#63272=CARTESIAN_POINT ( 'NONE',  ( 21.53943276465977519, 0.05219959533937863772, 71.25109039468568994 ) ) ;
#63273=CARTESIAN_POINT ( 'NONE',  ( -16.52544592524335698, -4.483927247898792601, 38.95942372801901854 ) ) ;
#63274=CARTESIAN_POINT ( 'NONE',  ( 16.53943276465976808, -0.05219959533910856209, 73.74890960531433848 ) ) ;
#63275=CARTESIAN_POINT ( 'NONE',  ( -15.80617190586768217, 15.72974639402176855, 88.12609039468570415 ) ) ;
#63276=CARTESIAN_POINT ( 'NONE',  ( 8.224510206698742110, 14.34966873604972548, 112.0844237280190185 ) ) ;
#63278=CARTESIAN_POINT ( 'NONE',  ( -4.379528057220086978, -16.55341960407618274, 39.79275706135235424 ) ) ;
#63279=CARTESIAN_POINT ( 'NONE',  ( 16.52544592524342804, -4.483927247898539470, 43.54057627198103830 ) ) ;
#63280=CARTESIAN_POINT ( 'NONE',  ( -4.379528057220086978, -16.55341960407618274, 89.79275706135236135 ) ) ;
#63281=CARTESIAN_POINT ( 'NONE',  ( -5.153800228976328057, -19.02544592524343514, 97.29057627198099567 ) ) ;
#63282=CARTESIAN_POINT ( 'NONE',  ( 19.03943276465977164, -0.05219959533909143690, 113.7489096053143669 ) ) ;
#63283=CARTESIAN_POINT ( 'NONE',  ( 21.55341960407619695, -5.719274019375665929, 101.0427570613523756 ) ) ;
#63284=CARTESIAN_POINT ( 'NONE',  ( 14.29746914071037800, 8.314922557961029526, 106.6677570613523756 ) ) ;
#63285=CARTESIAN_POINT ( 'NONE',  ( -12.06949235617756955, 12.14591786802309770, 75.62390960531439532 ) ) ;
#63286=CARTESIAN_POINT ( 'NONE',  ( -19.02544592524342804, 5.153800228976336051, 81.04057627198103830 ) ) ;
#63288=CARTESIAN_POINT ( 'NONE',  ( -14.34966873604972548, 8.224510206698743886, 23.33442372801901499 ) ) ;
#63289=CARTESIAN_POINT ( 'NONE',  ( 16.46253265017160672, -9.564922557960803928, 33.33224293864770260 ) ) ;
#63290=CARTESIAN_POINT ( 'NONE',  ( 9.474510206698971260, -16.51473224551069308, 87.91557627198102409 ) ) ;
#63291=CARTESIAN_POINT ( 'NONE',  ( 4.483927247898790824, -16.52544592524335698, 35.20942372801901854 ) ) ;
#63293=CARTESIAN_POINT ( 'NONE',  ( 5.049401038297881783, 19.05341960407617563, 37.29275706135232582 ) ) ;
#63294=CARTESIAN_POINT ( 'NONE',  ( -14.34966873604972548, 8.224510206698743886, 98.33442372801901854 ) ) ;
#63295=CARTESIAN_POINT ( 'NONE',  ( -19.02544592524334988, -5.153800228976617603, 108.9594237280189759 ) ) ;
#63296=CARTESIAN_POINT ( 'NONE',  ( -5.153800228976328057, -19.02544592524343514, 32.29057627198102409 ) ) ;
#63297=CARTESIAN_POINT ( 'NONE',  ( -8.224510206698735004, -14.34966873604973081, 79.58442372801903275 ) ) ;
#63298=CARTESIAN_POINT ( 'NONE',  ( 16.53943276465976808, 0.05219959533934440121, 66.25109039468567573 ) ) ;
#63299=CARTESIAN_POINT ( 'NONE',  ( -16.51473224551069308, -9.474510206698971260, 36.66557627198102409 ) ) ;
#63300=CARTESIAN_POINT ( 'NONE',  ( 5.049401038297881783, 19.05341960407617563, 72.29275706135234714 ) ) ;
#63301=CARTESIAN_POINT ( 'NONE',  ( -10.81492255796105439, 18.62759615963255655, 107.9177570613523471 ) ) ;
#63302=CARTESIAN_POINT ( 'NONE',  ( 16.46253265017160672, -9.564922557960803928, 53.33224293864768839 ) ) ;
#63304=CARTESIAN_POINT ( 'NONE',  ( -5.049401038298153566, 19.05341960407611168, 95.20724293864770971 ) ) ;
#63305=CARTESIAN_POINT ( 'NONE',  ( 4.379528057220339221, -16.55341960407611168, 87.70724293864769550 ) ) ;
#63307=CARTESIAN_POINT ( 'NONE',  ( -16.51473224551082808, 9.474510206698731452, 53.33442372801900433 ) ) ;
#63308=CARTESIAN_POINT ( 'NONE',  ( 21.55341960407610458, 5.719274019375980345, 53.95724293864770260 ) ) ;
#63309=CARTESIAN_POINT ( 'NONE',  ( -19.03943276465977164, -0.05219959533935918106, 28.75109039468566507 ) ) ;
#63310=CARTESIAN_POINT ( 'NONE',  ( -5.049401038298153566, 19.05341960407611168, 85.20724293864766707 ) ) ;
#63311=CARTESIAN_POINT ( 'NONE',  ( 5.153800228976615827, -19.02544592524334988, 20.20942372801899722 ) ) ;
#63312=CARTESIAN_POINT ( 'NONE',  ( 18.67979575497178502, 10.72451020669898547, 64.16557627198102409 ) ) ;
#63313=CARTESIAN_POINT ( 'NONE',  ( -5.153800228976328057, -19.02544592524343514, 107.2905762719810383 ) ) ;
#63314=CARTESIAN_POINT ( 'NONE',  ( -16.51473224551082808, 9.474510206698731452, 83.33442372801899012 ) ) ;
#63315=CARTESIAN_POINT ( 'NONE',  ( 0.05219959533909260263, 19.03943276465977164, 114.9989096053143669 ) ) ;
#63316=CARTESIAN_POINT ( 'NONE',  ( 9.474510206698729675, 16.51473224551082808, 112.0844237280190043 ) ) ;
#63317=CARTESIAN_POINT ( 'NONE',  ( 9.474510206698971260, -16.51473224551069308, 27.91557627198103120 ) ) ;
#63318=CARTESIAN_POINT ( 'NONE',  ( 16.51473224551069308, 9.474510206698969483, 99.16557627198102409 ) ) ;
#63319=CARTESIAN_POINT ( 'NONE',  ( 18.67979575497178502, 10.72451020669898547, 79.16557627198103830 ) ) ;
#63321=CARTESIAN_POINT ( 'NONE',  ( 16.53943276465976808, 0.05219959533934440121, 46.25109039468567573 ) ) ;
#63322=CARTESIAN_POINT ( 'NONE',  ( 18.67979575497194134, -10.72451020669871369, 40.83442372801901854 ) ) ;
#63323=CARTESIAN_POINT ( 'NONE',  ( 19.02544592524334988, 5.153800228976608722, 86.45942372801900433 ) ) ;
#63324=CARTESIAN_POINT ( 'NONE',  ( -0.05219959533937732626, 21.53943276465977519, 92.50109039468567573 ) ) ;
#63325=CARTESIAN_POINT ( 'NONE',  ( 16.52544592524335698, 4.483927247898782831, 91.45942372801901854 ) ) ;
#63326=CARTESIAN_POINT ( 'NONE',  ( 5.049401038298161559, -19.05341960407611168, 102.7072429386476955 ) ) ;
#63327=CARTESIAN_POINT ( 'NONE',  ( 8.314922557960818139, 14.29746914071049879, 84.58224293864769550 ) ) ;
#63328=CARTESIAN_POINT ( 'NONE',  ( -0.05219959533910754901, -16.53943276465976808, 37.49890960531436690 ) ) ;
#63329=CARTESIAN_POINT ( 'NONE',  ( 16.46253265017146816, 9.564922557961045513, 66.66775706135233293 ) ) ;
#63330=CARTESIAN_POINT ( 'NONE',  ( -21.52544592524334988, -5.823673210054445271, 53.95942372801900433 ) ) ;
#63331=CARTESIAN_POINT ( 'NONE',  ( 16.46253265017146816, 9.564922557961045513, 21.66775706135233648 ) ) ;
#63332=CARTESIAN_POINT ( 'NONE',  ( -12.14591786802309592, -12.06949235617757132, 91.87390960531436690 ) ) ;
#63333=CARTESIAN_POINT ( 'NONE',  ( 10.81492255796078972, 18.62759615963270932, 34.58224293864770260 ) ) ;
#63334=CARTESIAN_POINT ( 'NONE',  ( 16.52544592524335698, 4.483927247898782831, 111.4594237280190328 ) ) ;
#63336=CARTESIAN_POINT ( 'NONE',  ( -10.72451020669870658, -18.67979575497194134, 94.58442372801901854 ) ) ;
#63337=CARTESIAN_POINT ( 'NONE',  ( -8.314922557961024197, 14.29746914071037800, 62.91775706135236135 ) ) ;
#63338=CARTESIAN_POINT ( 'NONE',  ( 14.34966873604972726, -8.224510206698740333, 110.8344237280190043 ) ) ;
#63339=CARTESIAN_POINT ( 'NONE',  ( 5.719274019375673035, 21.55341960407619339, 52.29275706135236135 ) ) ;
#63340=CARTESIAN_POINT ( 'NONE',  ( -5.719274019375665041, -21.55341960407619695, 54.79275706135235424 ) ) ;
#63341=VERTEX_POINT ( 'NONE', #147524 ) ;
#63342=CARTESIAN_POINT ( 'NONE',  ( 15.80617190586769283, -15.72974639402175789, 30.62609039468567929 ) ) ;
#63343=CARTESIAN_POINT ( 'NONE',  ( 14.34966873604960469, 8.224510206698951720, 109.1655762719810383 ) ) ;
#63344=CARTESIAN_POINT ( 'NONE',  ( -16.46253265017160317, 9.564922557960807481, 30.83224293864769550 ) ) ;
#63345=CARTESIAN_POINT ( 'NONE',  ( 8.224510206698953496, -14.34966873604960469, 67.91557627198102409 ) ) ;
#63346=CARTESIAN_POINT ( 'NONE',  ( -16.46253265017160317, 9.564922557960807481, 65.83224293864769550 ) ) ;
#63347=CARTESIAN_POINT ( 'NONE',  ( 4.483927247898790824, -16.52544592524335698, 110.2094237280190185 ) ) ;
#63348=CARTESIAN_POINT ( 'NONE',  ( 21.53943276465977519, -0.05219959533907433946, 53.74890960531437401 ) ) ;
#63349=CARTESIAN_POINT ( 'NONE',  ( -4.379528057220328563, 16.55341960407611168, 95.20724293864769550 ) ) ;
#63350=CARTESIAN_POINT ( 'NONE',  ( 21.53943276465977519, -0.05219959533907433946, 98.74890960531438111 ) ) ;
#63351=CARTESIAN_POINT ( 'NONE',  ( -19.02544592524342804, 5.153800228976336051, 106.0405762719810241 ) ) ;
#63352=CARTESIAN_POINT ( 'NONE',  ( 5.049401038298161559, -19.05341960407611168, 47.70724293864770260 ) ) ;
#63353=CARTESIAN_POINT ( 'NONE',  ( -16.46253265017146816, -9.564922557961047289, 109.1677570613523471 ) ) ;
#63354=CARTESIAN_POINT ( 'NONE',  ( -15.72974639402197994, 15.80617190586746368, 50.62390960531435979 ) ) ;
#63355=CARTESIAN_POINT ( 'NONE',  ( -5.719274019375665041, -21.55341960407619695, 69.79275706135234714 ) ) ;
#63356=CARTESIAN_POINT ( 'NONE',  ( -5.049401038298153566, 19.05341960407611168, 70.20724293864769550 ) ) ;
#63357=CARTESIAN_POINT ( 'NONE',  ( 13.89961937509977652, -13.97604488694527269, 98.12390960531433848 ) ) ;
#63358=CARTESIAN_POINT ( 'NONE',  ( 14.34966873604972726, -8.224510206698740333, 65.83442372801900433 ) ) ;
#63359=CARTESIAN_POINT ( 'NONE',  ( 5.719274019375673035, 21.55341960407619339, 47.29275706135234003 ) ) ;
#63360=CARTESIAN_POINT ( 'NONE',  ( 21.53943276465977519, 0.05219959533937863772, 81.25109039468568994 ) ) ;
#63361=CARTESIAN_POINT ( 'NONE',  ( 10.72451020669898902, -18.67979575497178502, 92.91557627198103830 ) ) ;
#63362=CARTESIAN_POINT ( 'NONE',  ( -21.53943276465977519, -0.05219959533937600094, 38.75109039468567573 ) ) ;
#63363=CARTESIAN_POINT ( 'NONE',  ( -8.224510206698735004, -14.34966873604973081, 84.58442372801903275 ) ) ;
#63364=CARTESIAN_POINT ( 'NONE',  ( 0.05219959533907565091, 21.53943276465977519, 74.99890960531435269 ) ) ;
#63365=CARTESIAN_POINT ( 'NONE',  ( 19.02544592524334988, 5.153800228976608722, 31.45942372801900433 ) ) ;
#63366=CARTESIAN_POINT ( 'NONE',  ( -5.153800228976328057, -19.02544592524343514, 82.29057627198103830 ) ) ;
#63367=CARTESIAN_POINT ( 'NONE',  ( 16.55341960407611168, 4.379528057220329451, 23.95724293864769550 ) ) ;
#63368=CARTESIAN_POINT ( 'NONE',  ( -17.49999999999999645, -3.189878218039172264, 105.1294856257125758 ) ) ;
#63369=CARTESIAN_POINT ( 'NONE',  ( 9.474510206698971260, -16.51473224551069308, 97.91557627198102409 ) ) ;
#63371=CARTESIAN_POINT ( 'NONE',  ( 5.153800228976615827, -19.02544592524334988, 75.20942372801896170 ) ) ;
#63372=CARTESIAN_POINT ( 'NONE',  ( 15.72974639402199770, -15.80617190586745480, 58.12390960531435979 ) ) ;
#63373=CARTESIAN_POINT ( 'NONE',  ( -12.14591786802309592, -12.06949235617757132, 36.87390960531435979 ) ) ;
#63374=CARTESIAN_POINT ( 'NONE',  ( -9.474510206698720793, -16.51473224551083518, 109.5844237280190043 ) ) ;
#63375=CARTESIAN_POINT ( 'NONE',  ( 16.51473224551069308, 9.474510206698969483, 34.16557627198102409 ) ) ;
#63376=CARTESIAN_POINT ( 'NONE',  ( -16.53943276465976808, -0.05219959533934237506, 18.75109039468568639 ) ) ;
#63377=CARTESIAN_POINT ( 'NONE',  ( -18.67979575497178146, -10.72451020669898902, 96.66557627198102409 ) ) ;
#63378=CARTESIAN_POINT ( 'NONE',  ( -5.153800228976607833, 19.02544592524334988, 67.70942372801900433 ) ) ;
#63379=CARTESIAN_POINT ( 'NONE',  ( -8.314922557961024197, 14.29746914071037800, 82.91775706135234714 ) ) ;
#63380=CARTESIAN_POINT ( 'NONE',  ( 13.89961937509977652, -13.97604488694527269, 63.12390960531435979 ) ) ;
#63381=CARTESIAN_POINT ( 'NONE',  ( 0.05219959533910956823, 16.53943276465976808, 74.99890960531435269 ) ) ;
#63382=CARTESIAN_POINT ( 'NONE',  ( -9.564922557960796823, -16.46253265017161027, 62.08224293864769550 ) ) ;
#63383=CARTESIAN_POINT ( 'NONE',  ( 16.52544592524342804, -4.483927247898539470, 73.54057627198102409 ) ) ;
#63384=CARTESIAN_POINT ( 'NONE',  ( 9.564922557960805705, 16.46253265017160317, 24.58224293864769194 ) ) ;
#63386=CARTESIAN_POINT ( 'NONE',  ( -16.52544592524342804, 4.483927247898546575, 36.04057627198102409 ) ) ;
#63387=CARTESIAN_POINT ( 'NONE',  ( 19.05341960407611168, 5.049401038298154454, 78.95724293864769550 ) ) ;
#63388=DIRECTION ( 'NONE',  ( 0.000000000000000000, 0.000000000000000000, -1.000000000000000000 ) ) ;
#63389=CARTESIAN_POINT ( 'NONE',  ( 5.153800228976615827, -19.02544592524334988, 35.20942372801899722 ) ) ;
#63390=CARTESIAN_POINT ( 'NONE',  ( 12.14591786802327356, -12.06949235617739191, 55.62609039468568284 ) ) ;
#63391=CARTESIAN_POINT ( 'NONE',  ( -15.80617190586745835, -15.72974639402198527, 66.87390960531436690 ) ) ;
#63392=CARTESIAN_POINT ( 'NONE',  ( 10.72451020669871369, 18.67979575497193778, 112.0844237280190185 ) ) ;
#63393=CARTESIAN_POINT ( 'NONE',  ( -16.51473224551069308, -9.474510206698971260, 71.66557627198102409 ) ) ;
#63395=CARTESIAN_POINT ( 'NONE',  ( -21.55341960407610458, -5.719274019375992779, 21.45724293864769550 ) ) ;
#63396=CARTESIAN_POINT ( 'NONE',  ( 5.049401038298161559, -19.05341960407611168, 62.70724293864769550 ) ) ;
#63397=CARTESIAN_POINT ( 'NONE',  ( 18.67979575497194134, -10.72451020669871369, 35.83442372801901143 ) ) ;
#63398=CARTESIAN_POINT ( 'NONE',  ( 16.52544592524342804, -4.483927247898539470, 103.5405762719810383 ) ) ;
#63399=CARTESIAN_POINT ( 'NONE',  ( -21.52544592524343514, 5.823673210054127303, 106.0405762719810525 ) ) ;
#63400=CARTESIAN_POINT ( 'NONE',  ( -13.89961937509977652, 13.97604488694528158, 95.62390960531436690 ) ) ;
#63402=CARTESIAN_POINT ( 'NONE',  ( -18.67979575497193778, 10.72451020669871902, 28.33442372801902209 ) ) ;
#63404=CARTESIAN_POINT ( 'NONE',  ( 9.474510206698971260, -16.51473224551069308, 82.91557627198103830 ) ) ;
#63406=B_SPLINE_CURVE_WITH_KNOTS ( 'NONE', 3,
 ( #85740, #113077, #6891, #100897, #81725, #22079 ),
 .UNSPECIFIED., .F., .F.,
 ( 4, 2, 4 ),
 ( 3.469446951953613804E-18, 0.0003837532665554152424, 0.0007675065331108270154 ),
 .UNSPECIFIED. ) ;
#63408=CARTESIAN_POINT ( 'NONE',  ( -5.823673210054116645, -21.52544592524344225, 97.29057627198105251 ) ) ;
#63409=CARTESIAN_POINT ( 'NONE',  ( 5.153800228976335163, 19.02544592524342804, 44.79057627198103830 ) ) ;
#63410=CARTESIAN_POINT ( 'NONE',  ( 13.89961937509957401, 13.97604488694547697, 101.8760903946856331 ) ) ;
#63412=CARTESIAN_POINT ( 'NONE',  ( 16.46253265017160672, -9.564922557960803928, 23.33224293864769194 ) ) ;
#63413=CARTESIAN_POINT ( 'NONE',  ( -5.719274019375665041, -21.55341960407619695, 79.79275706135236135 ) ) ;
#63414=CARTESIAN_POINT ( 'NONE',  ( -19.02544592524342804, 5.153800228976336051, 81.04057627198103830 ) ) ;
#63415=CARTESIAN_POINT ( 'NONE',  ( 5.719274019375673035, 21.55341960407619339, 52.29275706135236135 ) ) ;
#63416=CARTESIAN_POINT ( 'NONE',  ( 21.55341960407619695, -5.719274019375665929, 31.04275706135234714 ) ) ;
#63418=CARTESIAN_POINT ( 'NONE',  ( 0.05219959533909260263, 19.03943276465977164, 89.99890960531436690 ) ) ;
#63419=CARTESIAN_POINT ( 'NONE',  ( 18.56399227203345248, 5.499999999999818812, 61.47830131249903474 ) ) ;
#63420=CARTESIAN_POINT ( 'NONE',  ( -12.14591786802326823, 12.06949235617739902, 38.12609039468567573 ) ) ;
#63421=CARTESIAN_POINT ( 'NONE',  ( 15.80617190586746368, 15.72974639402197994, 49.37390960531436690 ) ) ;
#63422=CARTESIAN_POINT ( 'NONE',  ( -15.72974639402176322, -15.80617190586768395, 39.37609039468567573 ) ) ;
#63423=CARTESIAN_POINT ( 'NONE',  ( -15.80617190586768217, 15.72974639402176855, 73.12609039468567573 ) ) ;
#63425=CARTESIAN_POINT ( 'NONE',  ( -19.05341960407617563, 5.049401038297882671, 108.5427570613523187 ) ) ;
#63426=CARTESIAN_POINT ( 'NONE',  ( -13.89961937509977652, 13.97604488694528158, 55.62390960531434558 ) ) ;
#63427=CARTESIAN_POINT ( 'NONE',  ( -16.46253265017160317, 9.564922557960807481, 80.83224293864769550 ) ) ;
#63428=CARTESIAN_POINT ( 'NONE',  ( 16.52544592524342804, -4.483927247898539470, 108.5405762719810241 ) ) ;
#63429=CARTESIAN_POINT ( 'NONE',  ( 4.379528057220339221, -16.55341960407611168, 107.7072429386476955 ) ) ;
#63430=CARTESIAN_POINT ( 'NONE',  ( -13.97604488694527625, -13.89961937509977652, 111.8739096053143243 ) ) ;
#63431=CARTESIAN_POINT ( 'NONE',  ( -12.06949235617739369, -12.14591786802326823, 84.37609039468570415 ) ) ;
#63432=CARTESIAN_POINT ( 'NONE',  ( -16.55341960407611168, -4.379528057220339221, 76.45724293864769550 ) ) ;
#63433=CARTESIAN_POINT ( 'NONE',  ( -5.049401038298153566, 19.05341960407611168, 60.20724293864768129 ) ) ;
#63434=CARTESIAN_POINT ( 'NONE',  ( -0.05219959533937732626, 21.53943276465977519, 82.50109039468568994 ) ) ;
#63435=CARTESIAN_POINT ( 'NONE',  ( 21.53943276465977519, 0.05219959533937863772, 66.25109039468567573 ) ) ;
#63436=CARTESIAN_POINT ( 'NONE',  ( 13.89961937509957401, 13.97604488694547697, 111.8760903946856757 ) ) ;
#63437=CARTESIAN_POINT ( 'NONE',  ( -14.34966873604960291, -8.224510206698953496, 61.66557627198103120 ) ) ;
#63438=CARTESIAN_POINT ( 'NONE',  ( 10.81492255796106328, -18.62759615963255655, 25.41775706135235779 ) ) ;
#63439=CARTESIAN_POINT ( 'NONE',  ( 0.05219959533907565091, 21.53943276465977519, 64.99890960531435269 ) ) ;
#63440=CARTESIAN_POINT ( 'NONE',  ( -17.49999999999999645, -5.500000000000000888, 104.2030961746582847 ) ) ;
#63442=CARTESIAN_POINT ( 'NONE',  ( 0.05219959533909260263, 19.03943276465977164, 69.99890960531435269 ) ) ;
#63443=CARTESIAN_POINT ( 'NONE',  ( 0.05219959533910956823, 16.53943276465976808, 39.99890960531436690 ) ) ;
#63445=CARTESIAN_POINT ( 'NONE',  ( -12.06949235617756955, 12.14591786802309770, 25.62390960531435624 ) ) ;
#63446=CARTESIAN_POINT ( 'NONE',  ( -8.314922557961024197, 14.29746914071037800, 92.91775706135236135 ) ) ;
#63447=CARTESIAN_POINT ( 'NONE',  ( 19.05341960407617918, -5.049401038297876454, 56.04275706135234714 ) ) ;
#63448=CARTESIAN_POINT ( 'NONE',  ( 17.12812012977023812, 6.668231424566063659, 48.85948759323144941 ) ) ;
#63449=CARTESIAN_POINT ( 'NONE',  ( -19.02544592524342804, 5.153800228976336051, 106.0405762719810241 ) ) ;
#63450=CARTESIAN_POINT ( 'NONE',  ( 0.05219959533910956823, 16.53943276465976808, 79.99890960531435269 ) ) ;
#63451=CARTESIAN_POINT ( 'NONE',  ( -16.46253265017146816, -9.564922557961047289, 44.16775706135232582 ) ) ;
#63452=CARTESIAN_POINT ( 'NONE',  ( 17.50000000000000000, -5.500000000000000888, 103.2969038253417153 ) ) ;
#63453=CARTESIAN_POINT ( 'NONE',  ( 19.05341960407611168, 5.049401038298154454, 113.9572429386477097 ) ) ;
#63454=CARTESIAN_POINT ( 'NONE',  ( 0.05219959533907565091, 21.53943276465977519, 59.99890960531436690 ) ) ;
#63455=VERTEX_POINT ( 'NONE', #133338 ) ;
#63456=CARTESIAN_POINT ( 'NONE',  ( -0.05219959533910754901, -16.53943276465976808, 102.4989096053143811 ) ) ;
#63457=CARTESIAN_POINT ( 'NONE',  ( 16.52544592524335698, 4.483927247898782831, 56.45942372801902565 ) ) ;
#63458=CARTESIAN_POINT ( 'NONE',  ( 14.29746914071049879, -8.314922557960816363, 93.33224293864769550 ) ) ;
#63460=CARTESIAN_POINT ( 'NONE',  ( -16.18388926212241685, 7.379444403734378710, 49.56046848633847191 ) ) ;
#63461=CARTESIAN_POINT ( 'NONE',  ( 19.03943276465977164, -0.05219959533909143690, 113.7489096053143669 ) ) ;
#63464=ORIENTED_EDGE ( 'NONE', *, *, #192158, .F. ) ;
#63465=CARTESIAN_POINT ( 'NONE',  ( 8.224510206698742110, 14.34966873604972548, 42.08442372801901854 ) ) ;
#63466=CARTESIAN_POINT ( 'NONE',  ( -12.06949235617756955, 12.14591786802309770, 35.62390960531437401 ) ) ;
#63467=CARTESIAN_POINT ( 'NONE',  ( -10.72451020669898014, 18.67979575497178502, 60.41557627198102409 ) ) ;
#63468=CARTESIAN_POINT ( 'NONE',  ( -9.474510206698720793, -16.51473224551083518, 89.58442372801900433 ) ) ;
#63469=CARTESIAN_POINT ( 'NONE',  ( 0.05219959533907565091, 21.53943276465977519, 49.99890960531437401 ) ) ;
#63470=CARTESIAN_POINT ( 'NONE',  ( -10.81492255796105439, 18.62759615963255655, 82.91775706135234714 ) ) ;
#63472=CARTESIAN_POINT ( 'NONE',  ( -0.05219959533934338120, 16.53943276465976808, 32.50109039468568284 ) ) ;
#63473=CARTESIAN_POINT ( 'NONE',  ( -0.05219959533909027116, -19.03943276465977164, 37.49890960531436690 ) ) ;
#63474=CARTESIAN_POINT ( 'NONE',  ( -13.89961937509977652, 13.97604488694528158, 105.6239096053143527 ) ) ;
#63475=CARTESIAN_POINT ( 'NONE',  ( 16.46253265017160672, -9.564922557960803928, 38.33224293864768839 ) ) ;
#63476=CARTESIAN_POINT ( 'NONE',  ( 12.14591786802309770, 12.06949235617756955, 104.3739096053143669 ) ) ;
#63477=CARTESIAN_POINT ( 'NONE',  ( -9.474510206698964154, 16.51473224551069663, 100.4155762719810241 ) ) ;
#63479=CARTESIAN_POINT ( 'NONE',  ( 16.55341960407618274, -4.379528057220086978, 51.04275706135234714 ) ) ;
#63480=CARTESIAN_POINT ( 'NONE',  ( 21.52544592524344225, -5.823673210054117533, 88.54057627198103830 ) ) ;
#63481=CARTESIAN_POINT ( 'NONE',  ( 0.05219959533909260263, 19.03943276465977164, 59.99890960531436690 ) ) ;
#63482=CARTESIAN_POINT ( 'NONE',  ( 18.62759615963255655, 10.81492255796105972, 21.66775706135235069 ) ) ;
#63483=CARTESIAN_POINT ( 'NONE',  ( -13.97604488694527625, -13.89961937509977652, 81.87390960531436690 ) ) ;
#63486=CARTESIAN_POINT ( 'NONE',  ( -12.06949235617739369, -12.14591786802326823, 44.37609039468567573 ) ) ;
#63487=CARTESIAN_POINT ( 'NONE',  ( -5.719274019375665041, -21.55341960407619695, 24.79275706135235779 ) ) ;
#63488=CARTESIAN_POINT ( 'NONE',  ( 9.474510206698971260, -16.51473224551069308, 22.91557627198102765 ) ) ;
#63489=CARTESIAN_POINT ( 'NONE',  ( -5.153800228976328057, -19.02544592524343514, 102.2905762719810383 ) ) ;
#63490=CARTESIAN_POINT ( 'NONE',  ( -9.564922557961040184, 16.46253265017147172, 77.91775706135234714 ) ) ;
#63492=CARTESIAN_POINT ( 'NONE',  ( -16.51473224551082808, 9.474510206698731452, 33.33442372801899722 ) ) ;
#63493=CARTESIAN_POINT ( 'NONE',  ( -15.72974639402197994, 15.80617190586746368, 85.62390960531436690 ) ) ;
#63494=CARTESIAN_POINT ( 'NONE',  ( 19.02544592524334988, 5.153800228976608722, 41.45942372801900433 ) ) ;
#63495=CARTESIAN_POINT ( 'NONE',  ( -4.483927247898782831, 16.52544592524335698, 72.70942372801901854 ) ) ;
#63496=CARTESIAN_POINT ( 'NONE',  ( -5.153800228976328057, -19.02544592524343514, 112.2905762719810099 ) ) ;
#63497=VERTEX_POINT ( 'NONE', #40334 ) ;
#63498=CARTESIAN_POINT ( 'NONE',  ( -13.89961937509977652, 13.97604488694528158, 60.62390960531436690 ) ) ;
#63500=CARTESIAN_POINT ( 'NONE',  ( -10.81492255796105439, 18.62759615963255655, 67.91775706135234714 ) ) ;
#63501=CARTESIAN_POINT ( 'NONE',  ( 15.80617190586769283, -15.72974639402175789, 85.62609039468568994 ) ) ;
#63502=CARTESIAN_POINT ( 'NONE',  ( -19.02544592524342804, 5.153800228976336051, 71.04057627198099567 ) ) ;
#63503=CARTESIAN_POINT ( 'NONE',  ( 18.62759615963255655, 10.81492255796105972, 46.66775706135234714 ) ) ;
#63504=CARTESIAN_POINT ( 'NONE',  ( 16.51473224551083163, -9.474510206698727899, 85.83442372801900433 ) ) ;
#63506=CARTESIAN_POINT ( 'NONE',  ( 5.153800228976335163, 19.02544592524342804, 54.79057627198103120 ) ) ;
#63507=CARTESIAN_POINT ( 'NONE',  ( 16.46253265017160672, -9.564922557960803928, 103.3322429386476955 ) ) ;
#63508=CARTESIAN_POINT ( 'NONE',  ( -19.03943276465977164, 0.05219959533909376836, 61.24890960531436690 ) ) ;
#63509=CARTESIAN_POINT ( 'NONE',  ( -5.153800228976328057, -19.02544592524343514, 112.2905762719810099 ) ) ;
#63510=CARTESIAN_POINT ( 'NONE',  ( -9.474510206698964154, 16.51473224551069663, 45.41557627198103120 ) ) ;
#63511=CARTESIAN_POINT ( 'NONE',  ( -15.80617190586745835, -15.72974639402198527, 101.8739096053143811 ) ) ;
#63512=CARTESIAN_POINT ( 'NONE',  ( -0.05219959533934338120, 16.53943276465976808, 77.50109039468567573 ) ) ;
#63514=CARTESIAN_POINT ( 'NONE',  ( 19.05341960407617918, -5.049401038297876454, 36.04275706135234003 ) ) ;
#63515=CARTESIAN_POINT ( 'NONE',  ( -9.474510206698964154, 16.51473224551069663, 70.41557627198102409 ) ) ;
#63516=CARTESIAN_POINT ( 'NONE',  ( -12.14591786802309592, -12.06949235617757132, 61.87390960531436690 ) ) ;
#63517=CARTESIAN_POINT ( 'NONE',  ( 14.34966873604960469, 8.224510206698951720, 99.16557627198100988 ) ) ;
#63518=CARTESIAN_POINT ( 'NONE',  ( 5.153800228976335163, 19.02544592524342804, 94.79057627198103830 ) ) ;
#63519=CARTESIAN_POINT ( 'NONE',  ( 16.46253265017160672, -9.564922557960803928, 88.33224293864769550 ) ) ;
#63520=CARTESIAN_POINT ( 'NONE',  ( -16.51473224551069308, -9.474510206698971260, 101.6655762719810241 ) ) ;
#63521=CARTESIAN_POINT ( 'NONE',  ( -5.049401038297874678, -19.05341960407617918, 19.79275706135233293 ) ) ;
#63522=CARTESIAN_POINT ( 'NONE',  ( 8.314922557961029526, -14.29746914071037800, 95.41775706135234714 ) ) ;
#63523=CARTESIAN_POINT ( 'NONE',  ( 5.719274019375673035, 21.55341960407619339, 37.29275706135235424 ) ) ;
#63524=CARTESIAN_POINT ( 'NONE',  ( -10.72451020669898014, 18.67979575497178502, 30.41557627198101699 ) ) ;
#63525=CARTESIAN_POINT ( 'NONE',  ( -18.67979575497178146, -10.72451020669898902, 106.6655762719810383 ) ) ;
#63526=CARTESIAN_POINT ( 'NONE',  ( -4.379528057220328563, 16.55341960407611168, 60.20724293864768839 ) ) ;
#63527=CARTESIAN_POINT ( 'NONE',  ( 5.153800228976335163, 19.02544592524342804, 49.79057627198100988 ) ) ;
#63528=CARTESIAN_POINT ( 'NONE',  ( 4.483927247898545687, 16.52544592524342804, 84.79057627198102409 ) ) ;
#63529=CARTESIAN_POINT ( 'NONE',  ( 15.80617190586746368, 15.72974639402197994, 39.37390960531436690 ) ) ;
#63530=CARTESIAN_POINT ( 'NONE',  ( -19.03943276465977164, -0.05219959533935918106, 38.75109039468566152 ) ) ;
#63531=CARTESIAN_POINT ( 'NONE',  ( -8.224510206698948167, 14.34966873604960824, 115.4155762719810241 ) ) ;
#63533=CARTESIAN_POINT ( 'NONE',  ( 4.483927247898790824, -16.52544592524335698, 65.20942372801901854 ) ) ;
#63534=CARTESIAN_POINT ( 'NONE',  ( 0.05219959533909260263, 19.03943276465977164, 64.99890960531436690 ) ) ;
#63536=CARTESIAN_POINT ( 'NONE',  ( -16.53943276465976808, 0.05219959533911058130, 86.24890960531436690 ) ) ;
#63537=CARTESIAN_POINT ( 'NONE',  ( -5.719274019375978568, 21.55341960407610458, 35.20724293864768839 ) ) ;
#63539=CARTESIAN_POINT ( 'NONE',  ( 8.314922557961029526, -14.29746914071037800, 105.4177570613523613 ) ) ;
#63540=CARTESIAN_POINT ( 'NONE',  ( -16.53943276465976808, -0.05219959533934237506, 23.75109039468567929 ) ) ;
#63541=CARTESIAN_POINT ( 'NONE',  ( -15.80617190586768217, 15.72974639402176855, 98.12609039468570415 ) ) ;
#63542=CARTESIAN_POINT ( 'NONE',  ( 19.05341960407611168, 5.049401038298154454, 83.95724293864766707 ) ) ;
#63543=CARTESIAN_POINT ( 'NONE',  ( 21.55341960407610458, 5.719274019375980345, 113.9572429386477239 ) ) ;
#63544=CARTESIAN_POINT ( 'NONE',  ( 5.153800228976335163, 19.02544592524342804, 29.79057627198102409 ) ) ;
#63545=CARTESIAN_POINT ( 'NONE',  ( 16.53943276465976808, 0.05219959533934440121, 36.25109039468567573 ) ) ;
#63546=CARTESIAN_POINT ( 'NONE',  ( -16.46253265017146816, -9.564922557961047289, 89.16775706135234714 ) ) ;
#63547=CARTESIAN_POINT ( 'NONE',  ( -15.80617190586745835, -15.72974639402198527, 91.87390960531436690 ) ) ;
#63548=CARTESIAN_POINT ( 'NONE',  ( 9.564922557961047289, -16.46253265017146816, 65.41775706135233293 ) ) ;
#63550=CARTESIAN_POINT ( 'NONE',  ( 18.67979575497178502, 10.72451020669898547, 114.1655762719810383 ) ) ;
#63551=CARTESIAN_POINT ( 'NONE',  ( 0.000000000000000000, 0.000000000000000000, 120.0000000000000142 ) ) ;
#63552=CARTESIAN_POINT ( 'NONE',  ( 5.049401038298161559, -19.05341960407611168, 77.70724293864765286 ) ) ;
#63553=CARTESIAN_POINT ( 'NONE',  ( 12.06949235617739724, 12.14591786802326823, 31.87609039468567929 ) ) ;
#63555=CARTESIAN_POINT ( 'NONE',  ( -9.564922557961040184, 16.46253265017147172, 57.91775706135233293 ) ) ;
#63556=CARTESIAN_POINT ( 'NONE',  ( -18.62759615963255300, -10.81492255796106328, 19.16775706135234714 ) ) ;
#63557=CARTESIAN_POINT ( 'NONE',  ( 16.55341960407611168, 4.379528057220329451, 78.95724293864769550 ) ) ;
#63558=CARTESIAN_POINT ( 'NONE',  ( 19.03943276465977164, -0.05219959533909143690, 78.74890960531436690 ) ) ;
#63559=CARTESIAN_POINT ( 'NONE',  ( 8.314922557961029526, -14.29746914071037800, 40.41775706135234714 ) ) ;
#63560=CARTESIAN_POINT ( 'NONE',  ( 0.05219959533936267826, -19.03943276465977164, 40.00109039468566152 ) ) ;
#63561=CARTESIAN_POINT ( 'NONE',  ( 15.72974639402176855, 15.80617190586768217, 66.87609039468568994 ) ) ;
#63562=CARTESIAN_POINT ( 'NONE',  ( -13.89961937509957401, -13.97604488694547875, 104.3760903946856757 ) ) ;
#63563=CARTESIAN_POINT ( 'NONE',  ( 0.05219959533909260263, 19.03943276465977164, 54.99890960531435979 ) ) ;
#63564=CARTESIAN_POINT ( 'NONE',  ( -16.51473224551082808, 9.474510206698731452, 83.33442372801899012 ) ) ;
#63565=CARTESIAN_POINT ( 'NONE',  ( 12.14591786802327356, -12.06949235617739191, 55.62609039468568284 ) ) ;
#63566=CARTESIAN_POINT ( 'NONE',  ( 5.823673210054444382, -21.52544592524334988, 100.2094237280190043 ) ) ;
#63567=CARTESIAN_POINT ( 'NONE',  ( -13.97604488694547697, 13.89961937509957934, 73.12609039468568994 ) ) ;
#63568=CARTESIAN_POINT ( 'NONE',  ( 19.05341960407611168, 5.049401038298154454, 53.95724293864770260 ) ) ;
#63569=CARTESIAN_POINT ( 'NONE',  ( -21.55341960407610458, -5.719274019375992779, 66.45724293864768129 ) ) ;
#63570=CARTESIAN_POINT ( 'NONE',  ( -4.379528057220328563, 16.55341960407611168, 60.20724293864768839 ) ) ;
#63571=CARTESIAN_POINT ( 'NONE',  ( -16.51473224551082808, 9.474510206698731452, 63.33442372801900433 ) ) ;
#63572=CARTESIAN_POINT ( 'NONE',  ( -17.26172910966780094, -6.454744622555795175, 24.19353091350776452 ) ) ;
#63573=CARTESIAN_POINT ( 'NONE',  ( -13.89961937509957401, -13.97604488694547875, 49.37609039468567573 ) ) ;
#63574=CARTESIAN_POINT ( 'NONE',  ( -14.34966873604972548, 8.224510206698743886, 98.33442372801901854 ) ) ;
#63575=CARTESIAN_POINT ( 'NONE',  ( 8.224510206698953496, -14.34966873604960469, 62.91557627198102409 ) ) ;
#63576=CARTESIAN_POINT ( 'NONE',  ( -5.719274019375665041, -21.55341960407619695, 94.79275706135234714 ) ) ;
#63578=CARTESIAN_POINT ( 'NONE',  ( 10.81492255796078972, 18.62759615963270932, 89.58224293864768129 ) ) ;
#63579=CARTESIAN_POINT ( 'NONE',  ( -19.05341960407611168, -5.049401038298163336, 56.45724293864768129 ) ) ;
#63580=CARTESIAN_POINT ( 'NONE',  ( -21.55341960407619339, 5.719274019375674811, 73.54275706135234714 ) ) ;
#63581=CARTESIAN_POINT ( 'NONE',  ( -9.564922557960796823, -16.46253265017161027, 52.08224293864768839 ) ) ;
#63583=CARTESIAN_POINT ( 'NONE',  ( 5.049401038298161559, -19.05341960407611168, 62.70724293864769550 ) ) ;
#63584=CARTESIAN_POINT ( 'NONE',  ( 19.03943276465977164, -0.05219959533909143690, 23.74890960531435269 ) ) ;
#63585=CARTESIAN_POINT ( 'NONE',  ( -19.03943276465977164, 0.05219959533909376836, 116.2489096053143669 ) ) ;
#63586=CARTESIAN_POINT ( 'NONE',  ( -4.483927247898539470, -16.52544592524342804, 57.29057627198103120 ) ) ;
#63587=CARTESIAN_POINT ( 'NONE',  ( -5.049401038298153566, 19.05341960407611168, 25.20724293864768484 ) ) ;
#63588=CARTESIAN_POINT ( 'NONE',  ( 4.483927247898545687, 16.52544592524342804, 89.79057627198103830 ) ) ;
#63589=CARTESIAN_POINT ( 'NONE',  ( -5.823673210054116645, -21.52544592524344225, 102.2905762719810383 ) ) ;
#63590=CARTESIAN_POINT ( 'NONE',  ( 21.55341960407619695, -5.719274019375665929, 31.04275706135234714 ) ) ;
#63592=CARTESIAN_POINT ( 'NONE',  ( -8.224510206698735004, -14.34966873604973081, 44.58442372801901854 ) ) ;
#63593=CARTESIAN_POINT ( 'NONE',  ( 21.52544592524344225, -5.823673210054117533, 78.54057627198103830 ) ) ;
#63594=CARTESIAN_POINT ( 'NONE',  ( -21.55341960407619339, 5.719274019375674811, 103.5427570613523613 ) ) ;
#63595=CARTESIAN_POINT ( 'NONE',  ( 9.564922557960805705, 16.46253265017160317, 109.5822429386476955 ) ) ;
#63596=CARTESIAN_POINT ( 'NONE',  ( -5.719274019375665041, -21.55341960407619695, 49.79275706135234714 ) ) ;
#63597=CARTESIAN_POINT ( 'NONE',  ( 10.81492255796078972, 18.62759615963270932, 39.58224293864769550 ) ) ;
#63598=CARTESIAN_POINT ( 'NONE',  ( -8.224510206698735004, -14.34966873604973081, 99.58442372801900433 ) ) ;
#63599=CARTESIAN_POINT ( 'NONE',  ( 21.52544592524334988, 5.823673210054432836, 61.45942372801901854 ) ) ;
#63600=CARTESIAN_POINT ( 'NONE',  ( -10.81492255796105439, 18.62759615963255655, 97.91775706135236135 ) ) ;
#63601=CARTESIAN_POINT ( 'NONE',  ( 9.474510206698729675, 16.51473224551082808, 37.08442372801899722 ) ) ;
#63602=CARTESIAN_POINT ( 'NONE',  ( -8.224510206698735004, -14.34966873604973081, 84.58442372801903275 ) ) ;
#63603=CARTESIAN_POINT ( 'NONE',  ( -0.05219959533937732626, 21.53943276465977519, 47.50109039468568994 ) ) ;
#63604=CARTESIAN_POINT ( 'NONE',  ( 19.05341960407611168, 5.049401038298154454, 48.95724293864768129 ) ) ;
#63605=CARTESIAN_POINT ( 'NONE',  ( -5.049401038297874678, -19.05341960407617918, 19.79275706135233293 ) ) ;
#63606=CARTESIAN_POINT ( 'NONE',  ( 18.62759615963271287, -10.81492255796078972, 23.33224293864769194 ) ) ;
#63607=CARTESIAN_POINT ( 'NONE',  ( -21.53943276465977519, 0.05219959533907696930, 111.2489096053143669 ) ) ;
#63608=CARTESIAN_POINT ( 'NONE',  ( 21.55341960407610458, 5.719274019375980345, 78.95724293864769550 ) ) ;
#63609=CARTESIAN_POINT ( 'NONE',  ( 14.34966873604972726, -8.224510206698740333, 35.83442372801901143 ) ) ;
#63610=CARTESIAN_POINT ( 'NONE',  ( -18.22780087662121673, -5.500000000000063061, 61.48459894673894155 ) ) ;
#63611=CARTESIAN_POINT ( 'NONE',  ( -5.823673210054116645, -21.52544592524344225, 82.29057627198103830 ) ) ;
#63612=CARTESIAN_POINT ( 'NONE',  ( 4.483927247898790824, -16.52544592524335698, 70.20942372801904696 ) ) ;
#63613=CARTESIAN_POINT ( 'NONE',  ( 4.379528057220339221, -16.55341960407611168, 62.70724293864769550 ) ) ;
#63615=CARTESIAN_POINT ( 'NONE',  ( 5.049401038297881783, 19.05341960407617563, 97.29275706135233293 ) ) ;
#63618=CARTESIAN_POINT ( 'NONE',  ( -12.06949235617739369, -12.14591786802326823, 39.37609039468567573 ) ) ;
#63619=CARTESIAN_POINT ( 'NONE',  ( 21.55341960407610458, 5.719274019375980345, 113.9572429386477239 ) ) ;
#63620=CARTESIAN_POINT ( 'NONE',  ( 10.81492255796078972, 18.62759615963270932, 74.58224293864768129 ) ) ;
#63621=CARTESIAN_POINT ( 'NONE',  ( 19.02544592524343514, -5.153800228976328945, 113.5405762719810241 ) ) ;
#63622=CARTESIAN_POINT ( 'NONE',  ( -0.05219959533934338120, 16.53943276465976808, 57.50109039468568994 ) ) ;
#63623=CARTESIAN_POINT ( 'NONE',  ( 13.89961937509977652, -13.97604488694527269, 68.12390960531436690 ) ) ;
#63624=CARTESIAN_POINT ( 'NONE',  ( 5.719274019375673035, 21.55341960407619339, 42.29275706135235424 ) ) ;
#63625=CARTESIAN_POINT ( 'NONE',  ( -13.97604488694547697, 13.89961937509957934, 108.1260903946856331 ) ) ;
#63626=CARTESIAN_POINT ( 'NONE',  ( 0.05219959533909260263, 19.03943276465977164, 114.9989096053143669 ) ) ;
#63627=CARTESIAN_POINT ( 'NONE',  ( 19.05341960407617918, -5.049401038297876454, 31.04275706135232227 ) ) ;
#63628=CARTESIAN_POINT ( 'NONE',  ( -14.29746914071037622, -8.314922557961029526, 44.16775706135234714 ) ) ;
#63629=CARTESIAN_POINT ( 'NONE',  ( 9.474510206698971260, -16.51473224551069308, 97.91557627198102409 ) ) ;
#63630=CARTESIAN_POINT ( 'NONE',  ( 5.823673210054125526, 21.52544592524343514, 109.7905762719810383 ) ) ;
#63631=CARTESIAN_POINT ( 'NONE',  ( -9.564922557960796823, -16.46253265017161027, 57.08224293864769550 ) ) ;
#63632=CARTESIAN_POINT ( 'NONE',  ( -16.62475595723696031, 7.163666690055234376, 25.52713351810466591 ) ) ;
#63633=CARTESIAN_POINT ( 'NONE',  ( 0.05219959533910956823, 16.53943276465976808, 84.99890960531436690 ) ) ;
#63634=CARTESIAN_POINT ( 'NONE',  ( -19.02544592524342804, 5.153800228976336051, 111.0405762719810099 ) ) ;
#63635=CARTESIAN_POINT ( 'NONE',  ( -17.44270441346513678, 5.991230190323086013, 33.63664920735774189 ) ) ;
#63636=CARTESIAN_POINT ( 'NONE',  ( 10.72451020669898902, -18.67979575497178502, 97.91557627198103830 ) ) ;
#63637=CARTESIAN_POINT ( 'NONE',  ( -0.05219959533936034679, 19.03943276465977164, 62.50109039468566863 ) ) ;
#63638=CARTESIAN_POINT ( 'NONE',  ( -5.719274019375978568, 21.55341960407610458, 30.20724293864769550 ) ) ;
#63639=CARTESIAN_POINT ( 'NONE',  ( -13.97604488694527625, -13.89961937509977652, 21.87390960531435979 ) ) ;
#63640=CARTESIAN_POINT ( 'NONE',  ( 21.53943276465977519, -0.05219959533907433946, 58.74890960531436690 ) ) ;
#63642=CARTESIAN_POINT ( 'NONE',  ( -16.46253265017160317, 9.564922557960807481, 100.8322429386477097 ) ) ;
#63643=CARTESIAN_POINT ( 'NONE',  ( -5.719274019375665041, -21.55341960407619695, 74.79275706135234714 ) ) ;
#63644=CARTESIAN_POINT ( 'NONE',  ( -9.474510206698964154, 16.51473224551069663, 50.41557627198102409 ) ) ;
#63645=CARTESIAN_POINT ( 'NONE',  ( 16.52544592524342804, -4.483927247898539470, 83.54057627198102409 ) ) ;
#63646=CARTESIAN_POINT ( 'NONE',  ( 0.05219959533934541429, -16.53943276465976808, 30.00109039468568284 ) ) ;
#63647=CARTESIAN_POINT ( 'NONE',  ( 19.03943276465977164, -0.05219959533909143690, 58.74890960531435979 ) ) ;
#63648=CARTESIAN_POINT ( 'NONE',  ( 5.823673210054444382, -21.52544592524334988, 65.20942372801901854 ) ) ;
#63649=EDGE_LOOP ( 'NONE', ( #119590, #37646, #82480, #150835 ) ) ;
#63650=CARTESIAN_POINT ( 'NONE',  ( -0.05219959533936034679, 19.03943276465977164, 22.50109039468566152 ) ) ;
#63652=CARTESIAN_POINT ( 'NONE',  ( 13.97604488694548053, -13.89961937509957401, 40.62609039468564731 ) ) ;
#63653=CARTESIAN_POINT ( 'NONE',  ( -17.50000000000002132, -5.499999999999948486, 91.28230962303565832 ) ) ;
#63654=CARTESIAN_POINT ( 'NONE',  ( 15.72974639402176855, 15.80617190586768217, 31.87609039468567929 ) ) ;
#63655=CARTESIAN_POINT ( 'NONE',  ( -18.22780087662121673, -5.500000000000063061, 46.48459894673893444 ) ) ;
#63656=CARTESIAN_POINT ( 'NONE',  ( -16.51473224551082808, 9.474510206698731452, 33.33442372801899722 ) ) ;
#63657=CARTESIAN_POINT ( 'NONE',  ( 19.02544592524343514, -5.153800228976328945, 83.54057627198100988 ) ) ;
#63658=CARTESIAN_POINT ( 'NONE',  ( 5.049401038298161559, -19.05341960407611168, 67.70724293864769550 ) ) ;
#63659=CARTESIAN_POINT ( 'NONE',  ( 16.52544592524342804, -4.483927247898539470, 23.54057627198102765 ) ) ;
#63660=CARTESIAN_POINT ( 'NONE',  ( -0.05219959533909027116, -19.03943276465977164, 112.4989096053143669 ) ) ;
#63661=CARTESIAN_POINT ( 'NONE',  ( -5.719274019375665041, -21.55341960407619695, 84.79275706135234714 ) ) ;
#63664=CARTESIAN_POINT ( 'NONE',  ( 5.823673210054444382, -21.52544592524334988, 90.20942372801903275 ) ) ;
#63666=CARTESIAN_POINT ( 'NONE',  ( 9.564922557960805705, 16.46253265017160317, 104.5822429386476955 ) ) ;
#63668=CARTESIAN_POINT ( 'NONE',  ( -5.823673210054116645, -21.52544592524344225, 67.29057627198103830 ) ) ;
#63669=CARTESIAN_POINT ( 'NONE',  ( -16.55341960407617563, 4.379528057220093196, 113.5427570613523756 ) ) ;
#63670=CARTESIAN_POINT ( 'NONE',  ( -8.224510206698948167, 14.34966873604960824, 110.4155762719810383 ) ) ;
#63671=CARTESIAN_POINT ( 'NONE',  ( 13.97604488694527802, 13.89961937509977652, 89.37390960531436690 ) ) ;
#63672=CARTESIAN_POINT ( 'NONE',  ( -19.02544592524334988, -5.153800228976617603, 18.95942372801899722 ) ) ;
#63673=CARTESIAN_POINT ( 'NONE',  ( -14.29746914071049879, 8.314922557960819915, 100.8322429386477097 ) ) ;
#63674=CARTESIAN_POINT ( 'NONE',  ( 5.719274019375673035, 21.55341960407619339, 62.29275706135236845 ) ) ;
#63676=CARTESIAN_POINT ( 'NONE',  ( -4.379528057220086978, -16.55341960407618274, 104.7927570613523898 ) ) ;
#63677=CARTESIAN_POINT ( 'NONE',  ( -9.564922557961040184, 16.46253265017147172, 62.91775706135233293 ) ) ;
#63679=CARTESIAN_POINT ( 'NONE',  ( 16.46253265017160672, -9.564922557960803928, 103.3322429386476955 ) ) ;
#63680=CARTESIAN_POINT ( 'NONE',  ( 8.314922557960818139, 14.29746914071049879, 79.58224293864769550 ) ) ;
#63681=CARTESIAN_POINT ( 'NONE',  ( -9.474510206698720793, -16.51473224551083518, 59.58442372801900433 ) ) ;
#63683=CARTESIAN_POINT ( 'NONE',  ( 19.03943276465977164, -0.05219959533909143690, 63.74890960531435979 ) ) ;
#63684=CARTESIAN_POINT ( 'NONE',  ( 16.55341960407611168, 4.379528057220329451, 63.95724293864770260 ) ) ;
#63685=CARTESIAN_POINT ( 'NONE',  ( 19.02544592524334988, 5.153800228976608722, 96.45942372801897591 ) ) ;
#63686=CARTESIAN_POINT ( 'NONE',  ( -10.81492255796078084, -18.62759615963271287, 47.08224293864770260 ) ) ;
#63688=CARTESIAN_POINT ( 'NONE',  ( 4.483927247898545687, 16.52544592524342804, 114.7905762719810383 ) ) ;
#63689=CARTESIAN_POINT ( 'NONE',  ( -17.31747979337949772, -6.344076630961024144, 31.37944868065185844 ) ) ;
#63690=CARTESIAN_POINT ( 'NONE',  ( 13.97604488694527802, 13.89961937509977652, 74.37390960531436690 ) ) ;
#63691=CARTESIAN_POINT ( 'NONE',  ( -5.719274019375978568, 21.55341960407610458, 65.20724293864768129 ) ) ;
#63692=CARTESIAN_POINT ( 'NONE',  ( 16.55341960407618274, -4.379528057220086978, 86.04275706135236135 ) ) ;
#63693=CARTESIAN_POINT ( 'NONE',  ( 5.153800228976335163, 19.02544592524342804, 74.79057627198103830 ) ) ;
#63694=CARTESIAN_POINT ( 'NONE',  ( 5.153800228976615827, -19.02544592524334988, 60.20942372801899012 ) ) ;
#63695=CARTESIAN_POINT ( 'NONE',  ( -10.72451020669870658, -18.67979575497194134, 79.58442372801903275 ) ) ;
#63696=CARTESIAN_POINT ( 'NONE',  ( 21.52544592524344225, -5.823673210054117533, 58.54057627198103120 ) ) ;
#63697=CARTESIAN_POINT ( 'NONE',  ( -5.153800228976328057, -19.02544592524343514, 107.2905762719810383 ) ) ;
#63698=CARTESIAN_POINT ( 'NONE',  ( 19.05341960407611168, 5.049401038298154454, 33.95724293864769550 ) ) ;
#63699=CARTESIAN_POINT ( 'NONE',  ( -14.29746914071037622, -8.314922557961029526, 104.1677570613523471 ) ) ;
#63700=CARTESIAN_POINT ( 'NONE',  ( 12.06949235617739724, 12.14591786802326823, 21.87609039468567573 ) ) ;
#63701=CARTESIAN_POINT ( 'NONE',  ( 17.50000000000000000, -5.500000000000000888, 43.29690382534172244 ) ) ;
#63702=CARTESIAN_POINT ( 'NONE',  ( -5.719274019375665041, -21.55341960407619695, 99.79275706135234714 ) ) ;
#63703=CARTESIAN_POINT ( 'NONE',  ( 14.29746914071049879, -8.314922557960816363, 63.33224293864770260 ) ) ;
#63704=CARTESIAN_POINT ( 'NONE',  ( 12.14591786802309770, 12.06949235617756955, 69.37390960531436690 ) ) ;
#63705=CARTESIAN_POINT ( 'NONE',  ( 18.67979575497178502, 10.72451020669898547, 94.16557627198103830 ) ) ;
#63706=CARTESIAN_POINT ( 'NONE',  ( -21.52544592524343514, 5.823673210054127303, 86.04057627198102409 ) ) ;
#63708=CARTESIAN_POINT ( 'NONE',  ( 18.62759615963271287, -10.81492255796078972, 48.33224293864770260 ) ) ;
#63709=CARTESIAN_POINT ( 'NONE',  ( 16.53943276465976808, 0.05219959533934440121, 61.25109039468567573 ) ) ;
#63710=CARTESIAN_POINT ( 'NONE',  ( -8.224510206698948167, 14.34966873604960824, 90.41557627198103830 ) ) ;
#63711=CARTESIAN_POINT ( 'NONE',  ( -19.02544592524342804, 5.153800228976336051, 51.04057627198103120 ) ) ;
#63713=CARTESIAN_POINT ( 'NONE',  ( -12.06949235617739369, -12.14591786802326823, 99.37609039468568994 ) ) ;
#63714=CARTESIAN_POINT ( 'NONE',  ( 21.52544592524334988, 5.823673210054432836, 31.45942372801901854 ) ) ;
#63715=CARTESIAN_POINT ( 'NONE',  ( -9.564922557960796823, -16.46253265017161027, 97.08224293864769550 ) ) ;
#63716=CARTESIAN_POINT ( 'NONE',  ( 10.72451020669871369, 18.67979575497193778, 67.08442372801901854 ) ) ;
#63717=CARTESIAN_POINT ( 'NONE',  ( -16.51473224551069308, -9.474510206698971260, 21.66557627198102765 ) ) ;
#63718=CARTESIAN_POINT ( 'NONE',  ( 19.05341960407611168, 5.049401038298154454, 23.95724293864769194 ) ) ;
#63720=CARTESIAN_POINT ( 'NONE',  ( -5.719274019375665041, -21.55341960407619695, 59.79275706135234714 ) ) ;
#63721=CARTESIAN_POINT ( 'NONE',  ( 9.564922557960805705, 16.46253265017160317, 49.58224293864770260 ) ) ;
#63722=CARTESIAN_POINT ( 'NONE',  ( 19.05341960407611168, 5.049401038298154454, 23.95724293864769194 ) ) ;
#63723=CARTESIAN_POINT ( 'NONE',  ( -16.51473224551069308, -9.474510206698971260, 96.66557627198102409 ) ) ;
#63724=CARTESIAN_POINT ( 'NONE',  ( 9.564922557961047289, -16.46253265017146816, 70.41775706135233293 ) ) ;
#63725=CARTESIAN_POINT ( 'NONE',  ( -21.53943276465977519, -0.05219959533937600094, 48.75109039468568284 ) ) ;
#63726=CARTESIAN_POINT ( 'NONE',  ( 16.51473224551083163, -9.474510206698727899, 60.83442372801900433 ) ) ;
#63727=CARTESIAN_POINT ( 'NONE',  ( -13.97604488694527625, -13.89961937509977652, 36.87390960531436690 ) ) ;
#63728=CARTESIAN_POINT ( 'NONE',  ( -16.55341960407617563, 4.379528057220093196, 108.5427570613523756 ) ) ;
#63729=CARTESIAN_POINT ( 'NONE',  ( -0.05219959533936034679, 19.03943276465977164, 77.50109039468566152 ) ) ;
#63730=CARTESIAN_POINT ( 'NONE',  ( -0.05219959533910754901, -16.53943276465976808, 32.49890960531435979 ) ) ;
#63731=CARTESIAN_POINT ( 'NONE',  ( -16.46253265017146816, -9.564922557961047289, 54.16775706135234003 ) ) ;
#63732=CARTESIAN_POINT ( 'NONE',  ( -13.97604488694527625, -13.89961937509977652, 96.87390960531433848 ) ) ;
#63733=CARTESIAN_POINT ( 'NONE',  ( 18.62759615963255655, 10.81492255796105972, 106.6677570613523756 ) ) ;
#63734=CARTESIAN_POINT ( 'NONE',  ( 19.05341960407617918, -5.049401038297876454, 26.04275706135233293 ) ) ;
#63735=CARTESIAN_POINT ( 'NONE',  ( 13.97604488694527802, 13.89961937509977652, 34.37390960531436690 ) ) ;
#63736=CARTESIAN_POINT ( 'NONE',  ( -0.05219959533937732626, 21.53943276465977519, 87.50109039468568994 ) ) ;
#63737=CARTESIAN_POINT ( 'NONE',  ( -4.483927247898782831, 16.52544592524335698, 37.70942372801900433 ) ) ;
#63739=CARTESIAN_POINT ( 'NONE',  ( -9.564922557960796823, -16.46253265017161027, 92.08224293864769550 ) ) ;
#63741=CARTESIAN_POINT ( 'NONE',  ( 16.46253265017160672, -9.564922557960803928, 73.33224293864769550 ) ) ;
#63743=CARTESIAN_POINT ( 'NONE',  ( 9.564922557961047289, -16.46253265017146816, 90.41775706135234714 ) ) ;
#63744=CARTESIAN_POINT ( 'NONE',  ( 9.474510206698971260, -16.51473224551069308, 102.9155762719810241 ) ) ;
#63745=CARTESIAN_POINT ( 'NONE',  ( 10.72451020669871369, 18.67979575497193778, 97.08442372801904696 ) ) ;
#63746=CARTESIAN_POINT ( 'NONE',  ( -0.05219959533910754901, -16.53943276465976808, 102.4989096053143811 ) ) ;
#63747=CARTESIAN_POINT ( 'NONE',  ( 16.51473224551069308, 9.474510206698969483, 24.16557627198102765 ) ) ;
#63748=CARTESIAN_POINT ( 'NONE',  ( -18.62759615963270932, 10.81492255796079327, 50.83224293864770971 ) ) ;
#63749=CARTESIAN_POINT ( 'NONE',  ( -15.72974639402197994, 15.80617190586746368, 30.62390960531436335 ) ) ;
#63750=CARTESIAN_POINT ( 'NONE',  ( 12.06949235617757843, -12.14591786802309237, 108.1239096053143811 ) ) ;
#63752=CARTESIAN_POINT ( 'NONE',  ( -16.51473224551082808, 9.474510206698731452, 58.33442372801900433 ) ) ;
#63753=CARTESIAN_POINT ( 'NONE',  ( -16.53943276465976808, 0.05219959533911058130, 41.24890960531435269 ) ) ;
#63754=CARTESIAN_POINT ( 'NONE',  ( -0.05219959533907301413, -21.53943276465977519, 22.49890960531436335 ) ) ;
#63755=CARTESIAN_POINT ( 'NONE',  ( 21.52544592524334988, 5.823673210054432836, 86.45942372801901854 ) ) ;
#63756=CARTESIAN_POINT ( 'NONE',  ( -0.05219959533907301413, -21.53943276465977519, 77.49890960531433848 ) ) ;
#63757=CARTESIAN_POINT ( 'NONE',  ( -10.72451020669870658, -18.67979575497194134, 44.58442372801901854 ) ) ;
#63758=CARTESIAN_POINT ( 'NONE',  ( 5.719274019375991003, -21.55341960407610458, 92.70724293864770971 ) ) ;
#63759=CARTESIAN_POINT ( 'NONE',  ( 18.67979575497194134, -10.72451020669871369, 55.83442372801901854 ) ) ;
#63760=CARTESIAN_POINT ( 'NONE',  ( 5.049401038298161559, -19.05341960407611168, 22.70724293864769194 ) ) ;
#63762=CARTESIAN_POINT ( 'NONE',  ( -19.02544592524342804, 5.153800228976336051, 86.04057627198103830 ) ) ;
#63763=CARTESIAN_POINT ( 'NONE',  ( 0.05219959533934541429, -16.53943276465976808, 80.00109039468568994 ) ) ;
#63764=CARTESIAN_POINT ( 'NONE',  ( 8.224510206698953496, -14.34966873604960469, 107.9155762719810241 ) ) ;
#63765=CARTESIAN_POINT ( 'NONE',  ( 13.89961937509977652, -13.97604488694527269, 108.1239096053143669 ) ) ;
#63766=CARTESIAN_POINT ( 'NONE',  ( -8.314922557960811034, -14.29746914071050412, 57.08224293864769550 ) ) ;
#63767=CARTESIAN_POINT ( 'NONE',  ( -8.224510206698948167, 14.34966873604960824, 25.41557627198103120 ) ) ;
#63768=CARTESIAN_POINT ( 'NONE',  ( 5.153800228976335163, 19.02544592524342804, 69.79057627198103830 ) ) ;
#63769=CARTESIAN_POINT ( 'NONE',  ( 16.51473224551069308, 9.474510206698969483, 29.16557627198103475 ) ) ;
#63770=CARTESIAN_POINT ( 'NONE',  ( -21.52544592524343514, 5.823673210054127303, 46.04057627198103830 ) ) ;
#63771=CARTESIAN_POINT ( 'NONE',  ( -13.89961937509957401, -13.97604488694547875, 34.37609039468566863 ) ) ;
#63773=CARTESIAN_POINT ( 'NONE',  ( -17.49999999999999645, -5.499999999999992895, 69.20309617465828467 ) ) ;
#63774=CARTESIAN_POINT ( 'NONE',  ( -12.14591786802309592, -12.06949235617757132, 31.87390960531435979 ) ) ;
#63775=CARTESIAN_POINT ( 'NONE',  ( 5.049401038298161559, -19.05341960407611168, 102.7072429386476955 ) ) ;
#63776=CARTESIAN_POINT ( 'NONE',  ( -5.719274019375665041, -21.55341960407619695, 64.79275706135234714 ) ) ;
#63778=CARTESIAN_POINT ( 'NONE',  ( -16.53943276465976808, -0.05219959533934237506, 58.75109039468568994 ) ) ;
#63779=CARTESIAN_POINT ( 'NONE',  ( -19.02544592524334988, -5.153800228976617603, 63.95942372801899012 ) ) ;
#63780=CARTESIAN_POINT ( 'NONE',  ( -16.53943276465976808, 0.05219959533911058130, 46.24890960531435979 ) ) ;
#63781=CARTESIAN_POINT ( 'NONE',  ( 17.50000000000000000, -5.499999999999992895, 51.21769037696435589 ) ) ;
#63782=CARTESIAN_POINT ( 'NONE',  ( -14.29746914071037622, -8.314922557961029526, 104.1677570613523471 ) ) ;
#63783=CARTESIAN_POINT ( 'NONE',  ( 5.049401038298161559, -19.05341960407611168, 37.70724293864768839 ) ) ;
#63784=CARTESIAN_POINT ( 'NONE',  ( -5.049401038298153566, 19.05341960407611168, 55.20724293864769550 ) ) ;
#63785=CARTESIAN_POINT ( 'NONE',  ( 16.51473224551069308, 9.474510206698969483, 29.16557627198103475 ) ) ;
#63786=CARTESIAN_POINT ( 'NONE',  ( -10.81492255796105439, 18.62759615963255655, 37.91775706135235424 ) ) ;
#63787=CARTESIAN_POINT ( 'NONE',  ( -0.05219959533909027116, -19.03943276465977164, 62.49890960531435979 ) ) ;
#63788=CARTESIAN_POINT ( 'NONE',  ( 5.049401038298161559, -19.05341960407611168, 112.7072429386476813 ) ) ;
#63789=CARTESIAN_POINT ( 'NONE',  ( -19.05341960407611168, -5.049401038298163336, 46.45724293864768129 ) ) ;
#63790=CARTESIAN_POINT ( 'NONE',  ( 18.62759615963271287, -10.81492255796078972, 23.33224293864769194 ) ) ;
#63791=CARTESIAN_POINT ( 'NONE',  ( 10.81492255796106328, -18.62759615963255655, 65.41775706135234714 ) ) ;
#63792=CARTESIAN_POINT ( 'NONE',  ( 19.02544592524343514, -5.153800228976328945, 23.54057627198102054 ) ) ;
#63793=CARTESIAN_POINT ( 'NONE',  ( 5.719274019375991003, -21.55341960407610458, 27.70724293864769905 ) ) ;
#63794=CARTESIAN_POINT ( 'NONE',  ( 12.14591786802327356, -12.06949235617739191, 75.62609039468567573 ) ) ;
#63795=CARTESIAN_POINT ( 'NONE',  ( -10.81492255796105439, 18.62759615963255655, 107.9177570613523471 ) ) ;
#63797=CARTESIAN_POINT ( 'NONE',  ( -4.483927247898782831, 16.52544592524335698, 72.70942372801901854 ) ) ;
#63798=CARTESIAN_POINT ( 'NONE',  ( 19.05341960407611168, 5.049401038298154454, 98.95724293864766707 ) ) ;
#63799=CARTESIAN_POINT ( 'NONE',  ( -12.14591786802326823, 12.06949235617739902, 48.12609039468568284 ) ) ;
#63800=CARTESIAN_POINT ( 'NONE',  ( 12.06949235617739724, 12.14591786802326823, 26.87609039468567218 ) ) ;
#63801=CARTESIAN_POINT ( 'NONE',  ( -4.483927247898782831, 16.52544592524335698, 97.70942372801904696 ) ) ;
#63802=CARTESIAN_POINT ( 'NONE',  ( 21.53943276465977519, 0.05219959533937863772, 56.25109039468568284 ) ) ;
#63803=CARTESIAN_POINT ( 'NONE',  ( -16.46253265017146816, -9.564922557961047289, 104.1677570613523329 ) ) ;
#63804=CARTESIAN_POINT ( 'NONE',  ( -0.05219959533907301413, -21.53943276465977519, 107.4989096053143669 ) ) ;
#63805=CARTESIAN_POINT ( 'NONE',  ( 4.483927247898545687, 16.52544592524342804, 99.79057627198103830 ) ) ;
#63806=CARTESIAN_POINT ( 'NONE',  ( -19.02544592524334988, -5.153800228976617603, 103.9594237280190043 ) ) ;
#63807=CARTESIAN_POINT ( 'NONE',  ( -14.29746914071037622, -8.314922557961029526, 89.16775706135236135 ) ) ;
#63809=CARTESIAN_POINT ( 'NONE',  ( 5.049401038297881783, 19.05341960407617563, 87.29275706135234714 ) ) ;
#63810=CARTESIAN_POINT ( 'NONE',  ( -14.29746914071049879, 8.314922557960819915, 40.83224293864769550 ) ) ;
#63811=CARTESIAN_POINT ( 'NONE',  ( -14.29746914071049879, 8.314922557960819915, 45.83224293864769550 ) ) ;
#63812=CARTESIAN_POINT ( 'NONE',  ( 14.34966873604960469, 8.224510206698951720, 109.1655762719810383 ) ) ;
#63813=CARTESIAN_POINT ( 'NONE',  ( 16.51473224551083163, -9.474510206698727899, 50.83442372801899722 ) ) ;
#63814=CARTESIAN_POINT ( 'NONE',  ( 5.719274019375673035, 21.55341960407619339, 32.29275706135235424 ) ) ;
#63815=CARTESIAN_POINT ( 'NONE',  ( -13.97604488694547697, 13.89961937509957934, 108.1260903946856331 ) ) ;
#63817=CARTESIAN_POINT ( 'NONE',  ( -16.46253265017160317, 9.564922557960807481, 110.8322429386476955 ) ) ;
#63818=CARTESIAN_POINT ( 'NONE',  ( 19.05341960407611168, 5.049401038298154454, 83.95724293864766707 ) ) ;
#63819=CARTESIAN_POINT ( 'NONE',  ( 18.62759615963271287, -10.81492255796078972, 58.33224293864768839 ) ) ;
#63820=CARTESIAN_POINT ( 'NONE',  ( -14.34966873604960291, -8.224510206698953496, 111.6655762719810525 ) ) ;
#63821=CARTESIAN_POINT ( 'NONE',  ( 19.05341960407611168, 5.049401038298154454, 68.95724293864769550 ) ) ;
#63822=CARTESIAN_POINT ( 'NONE',  ( -9.474510206698964154, 16.51473224551069663, 30.41557627198102054 ) ) ;
#63824=CARTESIAN_POINT ( 'NONE',  ( 10.72451020669871369, 18.67979575497193778, 32.08442372801901854 ) ) ;
#63825=CARTESIAN_POINT ( 'NONE',  ( 10.81492255796106328, -18.62759615963255655, 75.41775706135233293 ) ) ;
#63826=CARTESIAN_POINT ( 'NONE',  ( 14.29746914071037800, 8.314922557961029526, 96.66775706135234714 ) ) ;
#63827=CARTESIAN_POINT ( 'NONE',  ( 15.80617190586769283, -15.72974639402175789, 30.62609039468567929 ) ) ;
#63828=CARTESIAN_POINT ( 'NONE',  ( 15.80617190586769283, -15.72974639402175789, 30.62609039468567929 ) ) ;
#63829=CARTESIAN_POINT ( 'NONE',  ( -16.46253265017146816, -9.564922557961047289, 69.16775706135233293 ) ) ;
#63830=CARTESIAN_POINT ( 'NONE',  ( -5.153800228976328057, -19.02544592524343514, 77.29057627198099567 ) ) ;
#63831=CARTESIAN_POINT ( 'NONE',  ( 5.719274019375673035, 21.55341960407619339, 87.29275706135236135 ) ) ;
#63832=CARTESIAN_POINT ( 'NONE',  ( 15.80617190586746368, 15.72974639402197994, 84.37390960531438111 ) ) ;
#63833=CARTESIAN_POINT ( 'NONE',  ( -16.52544592524342804, 4.483927247898546575, 66.04057627198103830 ) ) ;
#63834=CARTESIAN_POINT ( 'NONE',  ( -21.55341960407619339, 5.719274019375674811, 98.54275706135234714 ) ) ;
#63835=CARTESIAN_POINT ( 'NONE',  ( 12.14591786802309770, 12.06949235617756955, 89.37390960531435269 ) ) ;
#63836=CARTESIAN_POINT ( 'NONE',  ( -9.474510206698964154, 16.51473224551069663, 25.41557627198103120 ) ) ;
#63837=CARTESIAN_POINT ( 'NONE',  ( 13.89961937509957401, 13.97604488694547697, 76.87609039468566152 ) ) ;
#63838=CARTESIAN_POINT ( 'NONE',  ( -16.52544592524342804, 4.483927247898546575, 31.04057627198102409 ) ) ;
#63839=CARTESIAN_POINT ( 'NONE',  ( 15.72974639402176855, 15.80617190586768217, 86.87609039468568994 ) ) ;
#63841=CARTESIAN_POINT ( 'NONE',  ( -5.153800228976328057, -19.02544592524343514, 87.29057627198103830 ) ) ;
#63842=CARTESIAN_POINT ( 'NONE',  ( -19.05341960407617563, 5.049401038297882671, 58.54275706135234003 ) ) ;
#63843=CARTESIAN_POINT ( 'NONE',  ( -5.719274019375978568, 21.55341960407610458, 70.20724293864769550 ) ) ;
#63844=CARTESIAN_POINT ( 'NONE',  ( -10.81492255796078084, -18.62759615963271287, 112.0822429386477097 ) ) ;
#63845=CARTESIAN_POINT ( 'NONE',  ( 8.224510206698742110, 14.34966873604972548, 22.08442372801901143 ) ) ;
#63846=CARTESIAN_POINT ( 'NONE',  ( -16.52544592524335698, -4.483927247898792601, 73.95942372801901854 ) ) ;
#63848=CARTESIAN_POINT ( 'NONE',  ( 15.72974639402176855, 15.80617190586768217, 21.87609039468567573 ) ) ;
#63849=( BOUNDED_CURVE ( )  B_SPLINE_CURVE ( 2, ( #144481, #5965, #114133, #175834, #37307, #98966, #160656, #22148, #191989, #53476, #115153, #176846, #38317 ),
 .UNSPECIFIED., .F., .T. ) 
 B_SPLINE_CURVE_WITH_KNOTS ( ( 3, 2, 2, 2, 2, 2, 3 ),
 ( 0.7129567522165188853, 0.7149122807017543879, 0.7192982456140351033, 0.7236842105263158187, 0.7280701754385965341, 0.7324561403508771384, 0.7343659890140226132 ),
 .UNSPECIFIED. ) 
 CURVE ( )  GEOMETRIC_REPRESENTATION_ITEM ( )  RATIONAL_B_SPLINE_CURVE ( ( 0.9831626618144007068, 0.9848076720550096308, 1.000000000000000000, 0.9659258262890683122, 1.000000000000000000, 0.9659258262890683122, 1.000000000000000000, 0.9659258262890683122, 1.000000000000000000, 0.9659258262890683122, 1.000000000000000000, 0.9851625545550091179, 0.9832469066685282089 ) ) 
 REPRESENTATION_ITEM ( '' )  );
#63850=CARTESIAN_POINT ( 'NONE',  ( 14.29746914071049879, -8.314922557960816363, 103.3322429386476955 ) ) ;
#63852=CARTESIAN_POINT ( 'NONE',  ( 4.379528057220092307, 16.55341960407617563, 32.29275706135235424 ) ) ;
#63853=CARTESIAN_POINT ( 'NONE',  ( 21.53943276465977519, -0.05219959533907433946, 63.74890960531435979 ) ) ;
#63854=CARTESIAN_POINT ( 'NONE',  ( -16.55341960407617563, 4.379528057220093196, 103.5427570613523613 ) ) ;
#63855=CARTESIAN_POINT ( 'NONE',  ( 4.379528057220092307, 16.55341960407617563, 42.29275706135235424 ) ) ;
#63856=CARTESIAN_POINT ( 'NONE',  ( 0.05219959533909260263, 19.03943276465977164, 34.99890960531435979 ) ) ;
#63857=CARTESIAN_POINT ( 'NONE',  ( -4.483927247898782831, 16.52544592524335698, 77.70942372801900433 ) ) ;
#63858=CARTESIAN_POINT ( 'NONE',  ( -19.02544592524334988, -5.153800228976617603, 68.95942372801896170 ) ) ;
#63859=CARTESIAN_POINT ( 'NONE',  ( -21.53943276465977519, 0.05219959533907696930, 76.24890960531435269 ) ) ;
#63860=CARTESIAN_POINT ( 'NONE',  ( -16.52544592524335698, -4.483927247898792601, 93.95942372801903275 ) ) ;
#63861=CARTESIAN_POINT ( 'NONE',  ( 15.80617190586769283, -15.72974639402175789, 80.62609039468567573 ) ) ;
#63862=CARTESIAN_POINT ( 'NONE',  ( 5.823673210054125526, 21.52544592524343514, 59.79057627198103120 ) ) ;
#63863=CARTESIAN_POINT ( 'NONE',  ( -15.80617190586745835, -15.72974639402198527, 46.87390960531435979 ) ) ;
#63864=ORIENTED_EDGE ( 'NONE', *, *, #14853, .T. ) ;
#63866=CARTESIAN_POINT ( 'NONE',  ( 14.34966873604972726, -8.224510206698740333, 75.83442372801900433 ) ) ;
#63867=CARTESIAN_POINT ( 'NONE',  ( -21.52544592524343514, 5.823673210054127303, 46.04057627198103830 ) ) ;
#63869=CARTESIAN_POINT ( 'NONE',  ( 19.05341960407611168, 5.049401038298154454, 108.9572429386477097 ) ) ;
#63871=CARTESIAN_POINT ( 'NONE',  ( -16.51473224551069308, -9.474510206698971260, 31.66557627198102054 ) ) ;
#63872=CARTESIAN_POINT ( 'NONE',  ( -5.719274019375978568, 21.55341960407610458, 65.20724293864768129 ) ) ;
#63873=CARTESIAN_POINT ( 'NONE',  ( -16.55341960407617563, 4.379528057220093196, 98.54275706135234714 ) ) ;
#63874=CARTESIAN_POINT ( 'NONE',  ( 15.72974639402176855, 15.80617190586768217, 46.87609039468568994 ) ) ;
#63875=CARTESIAN_POINT ( 'NONE',  ( -0.05219959533936034679, 19.03943276465977164, 97.50109039468567573 ) ) ;
#63876=CARTESIAN_POINT ( 'NONE',  ( 16.52544592524342804, -4.483927247898539470, 103.5405762719810383 ) ) ;
#63877=CARTESIAN_POINT ( 'NONE',  ( -5.049401038297874678, -19.05341960407617918, 104.7927570613523471 ) ) ;
#63878=CARTESIAN_POINT ( 'NONE',  ( -9.474510206698964154, 16.51473224551069663, 40.41557627198103120 ) ) ;
#63880=CARTESIAN_POINT ( 'NONE',  ( -5.153800228976328057, -19.02544592524343514, 97.29057627198099567 ) ) ;
#63881=CARTESIAN_POINT ( 'NONE',  ( 16.53943276465976808, 0.05219959533934440121, 71.25109039468568994 ) ) ;
#63882=CARTESIAN_POINT ( 'NONE',  ( 19.03943276465977164, 0.05219959533936151252, 76.25109039468566152 ) ) ;
#63883=CARTESIAN_POINT ( 'NONE',  ( 9.564922557961047289, -16.46253265017146816, 20.41775706135233293 ) ) ;
#63884=CARTESIAN_POINT ( 'NONE',  ( -21.52544592524343514, 5.823673210054127303, 56.04057627198102409 ) ) ;
#63885=CARTESIAN_POINT ( 'NONE',  ( -12.14591786802326823, 12.06949235617739902, 88.12609039468570415 ) ) ;
#63886=CARTESIAN_POINT ( 'NONE',  ( 5.049401038297881783, 19.05341960407617563, 77.29275706135231871 ) ) ;
#63887=CARTESIAN_POINT ( 'NONE',  ( -19.05341960407611168, -5.049401038298163336, 41.45724293864769550 ) ) ;
#63888=CARTESIAN_POINT ( 'NONE',  ( 13.89961937509977652, -13.97604488694527269, 73.12390960531436690 ) ) ;
#63889=CARTESIAN_POINT ( 'NONE',  ( -0.05219959533937732626, 21.53943276465977519, 52.50109039468567573 ) ) ;
#63890=CARTESIAN_POINT ( 'NONE',  ( -9.474510206698964154, 16.51473224551069663, 45.41557627198103120 ) ) ;
#63891=CARTESIAN_POINT ( 'NONE',  ( -16.46253265017146816, -9.564922557961047289, 79.16775706135234714 ) ) ;
#63892=LINE ( 'NONE', #191219, #173486 ) ;
#63893=CARTESIAN_POINT ( 'NONE',  ( 19.05341960407611168, 5.049401038298154454, 113.9572429386477097 ) ) ;
#63894=CARTESIAN_POINT ( 'NONE',  ( -4.379528057220328563, 16.55341960407611168, 60.20724293864768839 ) ) ;
#63895=CARTESIAN_POINT ( 'NONE',  ( 15.80617190586746368, 15.72974639402197994, 59.37390960531436690 ) ) ;
#63896=CARTESIAN_POINT ( 'NONE',  ( 20.28951144177217003, 1.856485852971841544, 102.5000000000000426 ) ) ;
#63897=CARTESIAN_POINT ( 'NONE',  ( 13.97604488694548053, -13.89961937509957401, 30.62609039468566863 ) ) ;
#63899=CARTESIAN_POINT ( 'NONE',  ( -0.05219959533909027116, -19.03943276465977164, 57.49890960531435979 ) ) ;
#63900=CARTESIAN_POINT ( 'NONE',  ( 16.51473224551069308, 9.474510206698969483, 79.16557627198103830 ) ) ;
#63901=CARTESIAN_POINT ( 'NONE',  ( 12.06949235617739724, 12.14591786802326823, 56.87609039468568994 ) ) ;
#63902=CARTESIAN_POINT ( 'NONE',  ( 16.51473224551083163, -9.474510206698727899, 80.83442372801899012 ) ) ;
#63903=CARTESIAN_POINT ( 'NONE',  ( -17.26172910966780805, 6.454744622555829814, 110.8064690864922568 ) ) ;
#63904=CARTESIAN_POINT ( 'NONE',  ( -4.483927247898782831, 16.52544592524335698, 87.70942372801901854 ) ) ;
#63906=CARTESIAN_POINT ( 'NONE',  ( -12.06949235617739369, -12.14591786802326823, 64.37609039468568994 ) ) ;
#63907=CARTESIAN_POINT ( 'NONE',  ( -8.314922557961024197, 14.29746914071037800, 37.91775706135235424 ) ) ;
#63908=CARTESIAN_POINT ( 'NONE',  ( 16.46253265017160672, -9.564922557960803928, 58.33224293864769550 ) ) ;
#63910=CARTESIAN_POINT ( 'NONE',  ( -0.05219959533937732626, 21.53943276465977519, 52.50109039468567573 ) ) ;
#63911=CARTESIAN_POINT ( 'NONE',  ( -16.51473224551082808, 9.474510206698731452, 68.33442372801900433 ) ) ;
#63912=CARTESIAN_POINT ( 'NONE',  ( -5.823673210054431948, 21.52544592524334988, 102.7094237280190185 ) ) ;
#63913=CARTESIAN_POINT ( 'NONE',  ( 5.153800228976335163, 19.02544592524342804, 24.79057627198102765 ) ) ;
#63915=CARTESIAN_POINT ( 'NONE',  ( -21.55341960407610458, -5.719274019375992779, 56.45724293864768839 ) ) ;
#63917=CARTESIAN_POINT ( 'NONE',  ( -19.02544592524342804, 5.153800228976336051, 111.0405762719810099 ) ) ;
#63918=CARTESIAN_POINT ( 'NONE',  ( 16.52544592524342804, -4.483927247898539470, 108.5405762719810241 ) ) ;
#63919=CARTESIAN_POINT ( 'NONE',  ( -16.53943276465976808, -0.05219959533934237506, 43.75109039468568284 ) ) ;
#63920=CARTESIAN_POINT ( 'NONE',  ( -12.14591786802309592, -12.06949235617757132, 26.87390960531435979 ) ) ;
#63922=CARTESIAN_POINT ( 'NONE',  ( -10.72451020669870658, -18.67979575497194134, 24.58442372801901499 ) ) ;
#63923=CARTESIAN_POINT ( 'NONE',  ( 14.34966873604960469, 8.224510206698951720, 39.16557627198102409 ) ) ;
#63924=CARTESIAN_POINT ( 'NONE',  ( -0.05219959533909027116, -19.03943276465977164, 107.4989096053143527 ) ) ;
#63925=CARTESIAN_POINT ( 'NONE',  ( 16.51473224551083163, -9.474510206698727899, 100.8344237280190043 ) ) ;
#63926=CARTESIAN_POINT ( 'NONE',  ( 13.89961937509957401, 13.97604488694547697, 26.87609039468566507 ) ) ;
#63927=CARTESIAN_POINT ( 'NONE',  ( -14.29746914071049879, 8.314922557960819915, 35.83224293864768839 ) ) ;
#63928=CARTESIAN_POINT ( 'NONE',  ( -0.05219959533907301413, -21.53943276465977519, 102.4989096053143811 ) ) ;
#63929=CARTESIAN_POINT ( 'NONE',  ( 0.05219959533907565091, 21.53943276465977519, 69.99890960531435269 ) ) ;
#63930=CARTESIAN_POINT ( 'NONE',  ( -5.049401038298153566, 19.05341960407611168, 80.20724293864769550 ) ) ;
#63931=CARTESIAN_POINT ( 'NONE',  ( 0.05219959533910956823, 16.53943276465976808, 44.99890960531435979 ) ) ;
#63932=CARTESIAN_POINT ( 'NONE',  ( 19.05341960407611168, 5.049401038298154454, 88.95724293864769550 ) ) ;
#63933=CARTESIAN_POINT ( 'NONE',  ( 13.97604488694527802, 13.89961937509977830, 79.37390960531436690 ) ) ;
#63934=CARTESIAN_POINT ( 'NONE',  ( 16.46253265017146816, 9.564922557961045513, 36.66775706135233293 ) ) ;
#63935=CARTESIAN_POINT ( 'NONE',  ( 15.80617190586746368, 15.72974639402197994, 89.37390960531435269 ) ) ;
#63936=CARTESIAN_POINT ( 'NONE',  ( 0.05219959533910956823, 16.53943276465976808, 99.99890960531436690 ) ) ;
#63937=CARTESIAN_POINT ( 'NONE',  ( 15.80617190586769283, -15.72974639402175789, 35.62609039468568994 ) ) ;
#63940=CARTESIAN_POINT ( 'NONE',  ( 16.53943276465976808, -0.05219959533910856209, 33.74890960531436690 ) ) ;
#63941=CARTESIAN_POINT ( 'NONE',  ( 5.153800228976335163, 19.02544592524342804, 29.79057627198102409 ) ) ;
#63942=CARTESIAN_POINT ( 'NONE',  ( 9.474510206698971260, -16.51473224551069308, 87.91557627198102409 ) ) ;
#63943=CARTESIAN_POINT ( 'NONE',  ( 18.62759615963271287, -10.81492255796078972, 58.33224293864768839 ) ) ;
#63945=CARTESIAN_POINT ( 'NONE',  ( -13.89961937509977652, 13.97604488694528158, 30.62390960531435269 ) ) ;
#63946=CARTESIAN_POINT ( 'NONE',  ( 4.483927247898545687, 16.52544592524342804, 44.79057627198103120 ) ) ;
#63947=CARTESIAN_POINT ( 'NONE',  ( -10.81492255796105439, 18.62759615963255655, 67.91775706135234714 ) ) ;
#63949=CARTESIAN_POINT ( 'NONE',  ( 16.55341960407618274, -4.379528057220086978, 66.04275706135236135 ) ) ;
#63950=CARTESIAN_POINT ( 'NONE',  ( 19.05341960407611168, 5.049401038298154454, 53.95724293864770260 ) ) ;
#63951=CARTESIAN_POINT ( 'NONE',  ( -16.46253265017160317, 9.564922557960807481, 70.83224293864770971 ) ) ;
#63953=CARTESIAN_POINT ( 'NONE',  ( -5.719274019375665041, -21.55341960407619695, 104.7927570613523898 ) ) ;
#63954=CARTESIAN_POINT ( 'NONE',  ( -16.52544592524335698, -4.483927247898792601, 78.95942372801901854 ) ) ;
#63955=CARTESIAN_POINT ( 'NONE',  ( 21.53943276465977519, 0.05219959533937863772, 101.2510903946856757 ) ) ;
#63956=CARTESIAN_POINT ( 'NONE',  ( 16.51473224551069308, 9.474510206698969483, 59.16557627198102409 ) ) ;
#63957=CARTESIAN_POINT ( 'NONE',  ( 21.55341960407610458, 5.719274019375980345, 28.95724293864769905 ) ) ;
#63958=CARTESIAN_POINT ( 'NONE',  ( -0.05219959533936034679, 19.03943276465977164, 102.5010903946856757 ) ) ;
#63959=CARTESIAN_POINT ( 'NONE',  ( 21.53943276465977519, 0.05219959533937863772, 86.25109039468568994 ) ) ;
#63960=CARTESIAN_POINT ( 'NONE',  ( -16.55341960407617563, 4.379528057220093196, 53.54275706135234714 ) ) ;
#63961=CARTESIAN_POINT ( 'NONE',  ( -10.72451020669898014, 18.67979575497178502, 100.4155762719810241 ) ) ;
#63962=CARTESIAN_POINT ( 'NONE',  ( -13.89961937509957401, -13.97604488694547875, 99.37609039468567573 ) ) ;
#63963=CARTESIAN_POINT ( 'NONE',  ( 5.153800228976335163, 19.02544592524342804, 84.79057627198099567 ) ) ;
#63964=CARTESIAN_POINT ( 'NONE',  ( -9.564922557961040184, 16.46253265017147172, 107.9177570613523471 ) ) ;
#63965=CARTESIAN_POINT ( 'NONE',  ( 0.05219959533909260263, 19.03943276465977164, 44.99890960531435979 ) ) ;
#63966=CARTESIAN_POINT ( 'NONE',  ( -4.379528057220086978, -16.55341960407618274, 24.79275706135235779 ) ) ;
#63967=CARTESIAN_POINT ( 'NONE',  ( 8.314922557960818139, 14.29746914071049879, 64.58224293864769550 ) ) ;
#63968=CARTESIAN_POINT ( 'NONE',  ( 16.52544592524335698, 4.483927247898782831, 71.45942372801901854 ) ) ;
#63969=CARTESIAN_POINT ( 'NONE',  ( -21.52544592524334988, -5.823673210054445271, 28.95942372801902209 ) ) ;
#63970=CARTESIAN_POINT ( 'NONE',  ( -16.51473224551069308, -9.474510206698971260, 56.66557627198103120 ) ) ;
#63971=CARTESIAN_POINT ( 'NONE',  ( -5.153800228976328057, -19.02544592524343514, 67.29057627198102409 ) ) ;
#63972=CARTESIAN_POINT ( 'NONE',  ( -12.14591786802326823, 12.06949235617739902, 73.12609039468567573 ) ) ;
#63975=CARTESIAN_POINT ( 'NONE',  ( -15.72974639402176322, -15.80617190586768395, 109.3760903946857042 ) ) ;
#63976=CARTESIAN_POINT ( 'NONE',  ( 5.049401038298161559, -19.05341960407611168, 37.70724293864768839 ) ) ;
#63979=CARTESIAN_POINT ( 'NONE',  ( -16.53943276465976808, -0.05219959533934237506, 28.75109039468567929 ) ) ;
#63980=CARTESIAN_POINT ( 'NONE',  ( -13.89961937509957401, -13.97604488694547875, 49.37609039468567573 ) ) ;
#63981=CARTESIAN_POINT ( 'NONE',  ( -4.379528057220086978, -16.55341960407618274, 44.79275706135234714 ) ) ;
#63982=CARTESIAN_POINT ( 'NONE',  ( 13.97604488694527802, 13.89961937509977652, 39.37390960531435269 ) ) ;
#63983=CARTESIAN_POINT ( 'NONE',  ( 5.153800228976335163, 19.02544592524342804, 69.79057627198103830 ) ) ;
#63984=CARTESIAN_POINT ( 'NONE',  ( -5.719274019375978568, 21.55341960407610458, 80.20724293864769550 ) ) ;
#63985=CARTESIAN_POINT ( 'NONE',  ( 16.46253265017160672, -9.564922557960803928, 83.33224293864768129 ) ) ;
#63986=CARTESIAN_POINT ( 'NONE',  ( 13.97604488694527802, 13.89961937509977652, 114.3739096053143669 ) ) ;
#63987=CARTESIAN_POINT ( 'NONE',  ( -19.05341960407611168, -5.049401038298163336, 61.45724293864769550 ) ) ;
#63988=DIRECTION ( 'NONE',  ( 0.000000000000000000, 0.000000000000000000, 1.000000000000000000 ) ) ;
#63989=CARTESIAN_POINT ( 'NONE',  ( 9.474510206698729675, 16.51473224551082808, 102.0844237280190043 ) ) ;
#63990=CARTESIAN_POINT ( 'NONE',  ( 13.89961937509957401, 13.97604488694547697, 26.87609039468566507 ) ) ;
#63991=CARTESIAN_POINT ( 'NONE',  ( -16.53943276465976808, 0.05219959533911058130, 56.24890960531436690 ) ) ;
#63992=CARTESIAN_POINT ( 'NONE',  ( 18.62759615963255655, 10.81492255796105972, 91.66775706135234714 ) ) ;
#63993=CARTESIAN_POINT ( 'NONE',  ( -16.52544592524342804, 4.483927247898546575, 116.0405762719810383 ) ) ;
#63994=EDGE_CURVE ( 'NONE', #197337, #169038, #135356, .T. ) ;
#63995=CARTESIAN_POINT ( 'NONE',  ( -12.14591786802309592, -12.06949235617757132, 31.87390960531435979 ) ) ;
#63996=CARTESIAN_POINT ( 'NONE',  ( -21.55341960407619339, 5.719274019375674811, 88.54275706135236135 ) ) ;
#63997=CARTESIAN_POINT ( 'NONE',  ( 16.51473224551069308, 9.474510206698969483, 74.16557627198103830 ) ) ;
#63998=CARTESIAN_POINT ( 'NONE',  ( -10.72451020669870658, -18.67979575497194134, 49.58442372801901143 ) ) ;
#63999=CARTESIAN_POINT ( 'NONE',  ( -0.05219959533909027116, -19.03943276465977164, 77.49890960531435269 ) ) ;
#64000=CARTESIAN_POINT ( 'NONE',  ( -14.29746914071049879, 8.314922557960819915, 100.8322429386477097 ) ) ;
#64001=CARTESIAN_POINT ( 'NONE',  ( 12.14591786802309770, 12.06949235617756955, 59.37390960531436690 ) ) ;
#64002=CARTESIAN_POINT ( 'NONE',  ( -0.05219959533907301413, -21.53943276465977519, 72.49890960531435269 ) ) ;
#64003=CARTESIAN_POINT ( 'NONE',  ( -0.05219959533909027116, -19.03943276465977164, 77.49890960531435269 ) ) ;
#64004=CARTESIAN_POINT ( 'NONE',  ( 5.823673210054125526, 21.52544592524343514, 89.79057627198103830 ) ) ;
#64005=CARTESIAN_POINT ( 'NONE',  ( -19.02544592524334988, -5.153800228976617603, 78.95942372801900433 ) ) ;
#64006=CARTESIAN_POINT ( 'NONE',  ( 16.46253265017146816, 9.564922557961045513, 36.66775706135233293 ) ) ;
#64007=CARTESIAN_POINT ( 'NONE',  ( -4.483927247898539470, -16.52544592524342804, 72.29057627198102409 ) ) ;
#64008=CARTESIAN_POINT ( 'NONE',  ( 9.564922557960805705, 16.46253265017160317, 64.58224293864769550 ) ) ;
#64009=CARTESIAN_POINT ( 'NONE',  ( 18.62759615963271287, -10.81492255796078972, 58.33224293864768839 ) ) ;
#64010=CARTESIAN_POINT ( 'NONE',  ( 16.38665767535054840, -7.295008042176022833, 27.76400864214547326 ) ) ;
#64011=CARTESIAN_POINT ( 'NONE',  ( 12.06949235617739724, 12.14591786802326823, 111.8760903946856615 ) ) ;
#64013=CARTESIAN_POINT ( 'NONE',  ( 16.46253265017146816, 9.564922557961045513, 101.6677570613523329 ) ) ;
#64014=CARTESIAN_POINT ( 'NONE',  ( -16.55341960407611168, -4.379528057220339221, 81.45724293864769550 ) ) ;
#64015=CARTESIAN_POINT ( 'NONE',  ( -17.49999999999998934, 4.013004640162638914, 35.44605720994410092 ) ) ;
#64016=CARTESIAN_POINT ( 'NONE',  ( 13.97604488694527802, 13.89961937509977652, 79.37390960531435269 ) ) ;
#64017=CARTESIAN_POINT ( 'NONE',  ( 5.153800228976335163, 19.02544592524342804, 29.79057627198102409 ) ) ;
#64018=CARTESIAN_POINT ( 'NONE',  ( -8.314922557960811034, -14.29746914071050412, 62.08224293864769550 ) ) ;
#64019=CARTESIAN_POINT ( 'NONE',  ( -19.02544592524342804, 5.153800228976336051, 96.04057627198103830 ) ) ;
#64020=CARTESIAN_POINT ( 'NONE',  ( -9.564922557961040184, 16.46253265017147172, 92.91775706135233293 ) ) ;
#64021=CARTESIAN_POINT ( 'NONE',  ( -19.02544592524342804, 5.153800228976336051, 61.04057627198103120 ) ) ;
#64022=CARTESIAN_POINT ( 'NONE',  ( 16.46253265017160672, -9.564922557960803928, 83.33224293864768129 ) ) ;
#64023=CARTESIAN_POINT ( 'NONE',  ( -18.67979575497178146, -10.72451020669898902, 81.66557627198103830 ) ) ;
#64024=CARTESIAN_POINT ( 'NONE',  ( -12.14591786802326823, 12.06949235617739902, 73.12609039468567573 ) ) ;
#64025=CARTESIAN_POINT ( 'NONE',  ( -19.03943276465977164, -0.05219959533935946555, 113.7510903946856757 ) ) ;
#64026=CARTESIAN_POINT ( 'NONE',  ( 19.03943276465977164, -0.05219959533909143690, 58.74890960531435979 ) ) ;
#64027=CARTESIAN_POINT ( 'NONE',  ( 15.72974639402199770, -15.80617190586745480, 68.12390960531436690 ) ) ;
#64028=CARTESIAN_POINT ( 'NONE',  ( -5.049401038297874678, -19.05341960407617918, 94.79275706135230450 ) ) ;
#64029=CARTESIAN_POINT ( 'NONE',  ( -16.53943276465976808, 0.05219959533911058130, 36.24890960531435979 ) ) ;
#64030=CARTESIAN_POINT ( 'NONE',  ( 10.81492255796106328, -18.62759615963255655, 45.41775706135234003 ) ) ;
#64032=CARTESIAN_POINT ( 'NONE',  ( -16.52544592524335698, -4.483927247898792601, 78.95942372801901854 ) ) ;
#64033=CARTESIAN_POINT ( 'NONE',  ( 5.049401038298161559, -19.05341960407611168, 107.7072429386476955 ) ) ;
#64034=CARTESIAN_POINT ( 'NONE',  ( 19.03943276465977164, -0.05219959533909143690, 108.7489096053143527 ) ) ;
#64035=CARTESIAN_POINT ( 'NONE',  ( -16.81555441253554051, -7.025013491695444756, 34.36314554665744225 ) ) ;
#64036=CARTESIAN_POINT ( 'NONE',  ( 12.14591786802327356, -12.06949235617739191, 95.62609039468568994 ) ) ;
#64037=CARTESIAN_POINT ( 'NONE',  ( 4.379528057220092307, 16.55341960407617563, 32.29275706135235424 ) ) ;
#64038=CARTESIAN_POINT ( 'NONE',  ( 13.89961937509977652, -13.97604488694527269, 48.12390960531435979 ) ) ;
#64039=CARTESIAN_POINT ( 'NONE',  ( -5.049401038298153566, 19.05341960407611168, 50.20724293864770260 ) ) ;
#64040=CARTESIAN_POINT ( 'NONE',  ( 0.05219959533909260263, 19.03943276465977164, 54.99890960531435979 ) ) ;
#64041=CARTESIAN_POINT ( 'NONE',  ( -21.53943276465977519, -0.05219959533937600094, 53.75109039468568994 ) ) ;
#64042=CARTESIAN_POINT ( 'NONE',  ( 16.52544592524335698, 4.483927247898782831, 66.45942372801903275 ) ) ;
#64043=CARTESIAN_POINT ( 'NONE',  ( 12.06949235617757843, -12.14591786802309237, 38.12390960531436690 ) ) ;
#64044=CARTESIAN_POINT ( 'NONE',  ( 16.51473224551069308, 9.474510206698969483, 39.16557627198103120 ) ) ;
#64045=CARTESIAN_POINT ( 'NONE',  ( -19.05341960407611168, -5.049401038298163336, 36.45724293864766707 ) ) ;
#64046=CARTESIAN_POINT ( 'NONE',  ( -4.379528057220086978, -16.55341960407618274, 34.79275706135235424 ) ) ;
#64047=CARTESIAN_POINT ( 'NONE',  ( -19.05341960407617563, 5.049401038297882671, 78.54275706135233293 ) ) ;
#64048=CARTESIAN_POINT ( 'NONE',  ( 16.52544592524342804, -4.483927247898539470, 83.54057627198102409 ) ) ;
#64049=CARTESIAN_POINT ( 'NONE',  ( 19.02544592524343514, -5.153800228976328945, 53.54057627198102409 ) ) ;
#64050=CARTESIAN_POINT ( 'NONE',  ( 13.89961937509957401, 13.97604488694547697, 81.87609039468564731 ) ) ;
#64052=CARTESIAN_POINT ( 'NONE',  ( 18.67979575497194134, -10.72451020669871369, 75.83442372801900433 ) ) ;
#64053=CARTESIAN_POINT ( 'NONE',  ( -8.314922557961024197, 14.29746914071037800, 52.91775706135235424 ) ) ;
#64054=CARTESIAN_POINT ( 'NONE',  ( -17.49999999999999645, 3.805241302050396346, 25.37352472782596280 ) ) ;
#64055=CARTESIAN_POINT ( 'NONE',  ( -18.67979575497178146, -10.72451020669898902, 51.66557627198102409 ) ) ;
#64056=CARTESIAN_POINT ( 'NONE',  ( -4.379528057220086978, -16.55341960407618274, 44.79275706135234714 ) ) ;
#64058=CARTESIAN_POINT ( 'NONE',  ( -5.153800228976607833, 19.02544592524334988, 22.70942372801899012 ) ) ;
#64060=CARTESIAN_POINT ( 'NONE',  ( -19.02544592524342804, 5.153800228976336051, 51.04057627198103120 ) ) ;
#64062=CARTESIAN_POINT ( 'NONE',  ( 9.564922557960805705, 16.46253265017160317, 69.58224293864770971 ) ) ;
#64063=CARTESIAN_POINT ( 'NONE',  ( 17.49999999999999645, -3.237210098469645470, 112.2123698737954243 ) ) ;
#64064=CARTESIAN_POINT ( 'NONE',  ( -13.97604488694547697, 13.89961937509957934, 23.12609039468565442 ) ) ;
#64065=CARTESIAN_POINT ( 'NONE',  ( 16.55341960407611168, 4.379528057220329451, 38.95724293864768839 ) ) ;
#64066=CARTESIAN_POINT ( 'NONE',  ( -13.89961937509977652, 13.97604488694528158, 45.62390960531433848 ) ) ;
#64067=CARTESIAN_POINT ( 'NONE',  ( -19.02544592524342804, 5.153800228976336051, 101.0405762719810241 ) ) ;
#64068=CARTESIAN_POINT ( 'NONE',  ( -15.72974639402176322, -15.80617190586768395, 74.37609039468568994 ) ) ;
#64069=CARTESIAN_POINT ( 'NONE',  ( -13.89961937509977652, 13.97604488694528158, 45.62390960531433848 ) ) ;
#64070=CARTESIAN_POINT ( 'NONE',  ( 15.72974639402176855, 15.80617190586768217, 66.87609039468568994 ) ) ;
#64071=CARTESIAN_POINT ( 'NONE',  ( 5.719274019375991003, -21.55341960407610458, 27.70724293864769905 ) ) ;
#64072=CARTESIAN_POINT ( 'NONE',  ( -5.153800228976328057, -19.02544592524343514, 32.29057627198102409 ) ) ;
#64073=CARTESIAN_POINT ( 'NONE',  ( -21.53943276465977519, -0.05219959533937600094, 28.75109039468567929 ) ) ;
#64074=CARTESIAN_POINT ( 'NONE',  ( 16.46253265017146816, 9.564922557961045513, 46.66775706135233293 ) ) ;
#64075=CARTESIAN_POINT ( 'NONE',  ( -16.51473224551069308, -9.474510206698971260, 26.66557627198103120 ) ) ;
#64076=CARTESIAN_POINT ( 'NONE',  ( -16.46253265017160317, 9.564922557960807481, 75.83224293864769550 ) ) ;
#64077=CARTESIAN_POINT ( 'NONE',  ( 5.153800228976615827, -19.02544592524334988, 105.2094237280190185 ) ) ;
#64078=CARTESIAN_POINT ( 'NONE',  ( -4.379528057220328563, 16.55341960407611168, 75.20724293864769550 ) ) ;
#64079=CARTESIAN_POINT ( 'NONE',  ( -0.05219959533907301413, -21.53943276465977519, 42.49890960531435979 ) ) ;
#64080=CARTESIAN_POINT ( 'NONE',  ( -5.049401038297874678, -19.05341960407617918, 99.79275706135234714 ) ) ;
#64081=CARTESIAN_POINT ( 'NONE',  ( 0.05219959533907565091, 21.53943276465977519, 109.9989096053143527 ) ) ;
#64082=CARTESIAN_POINT ( 'NONE',  ( 5.719274019375673035, 21.55341960407619339, 62.29275706135236845 ) ) ;
#64083=B_SPLINE_CURVE_WITH_KNOTS ( 'NONE', 3,
 ( #154783, #16280, #183149, #77932, #150831, #196355, #57823, #104316, #167971, #120464, #74967, #13302, #182156, #43640, #105303, #166991, #151811, #121457, #106286, #96089, #158750, #20239, #113243, #187141, #32441, #174934, #109270, #21246, #50598, #111260, #4071, #2092 ),
 .UNSPECIFIED., .F., .F.,
 ( 4, 2, 2, 2, 2, 2, 2, 2, 2, 2, 2, 2, 2, 2, 2, 4 ),
 ( 2.281672496420497865E-17, 0.0003712461730036943673, 0.0007424923460073658580, 0.001113738519011037457, 0.001484984692014708948, 0.002227477038022052363, 0.002598723211025727540, 0.002969969384029403584, 0.003341215557033078761, 0.003712461730036753938, 0.004083707903040429549, 0.004454954076044104726, 0.004826200249047780770, 0.005197446422051455947, 0.005568692595055131991, 0.005939938768058807168 ),
 .UNSPECIFIED. ) ;
#64084=CARTESIAN_POINT ( 'NONE',  ( -4.379528057220086978, -16.55341960407618274, 49.79275706135234714 ) ) ;
#64085=CARTESIAN_POINT ( 'NONE',  ( -12.06949235617739369, -12.14591786802326823, 49.37609039468569705 ) ) ;
#64086=CARTESIAN_POINT ( 'NONE',  ( 5.719274019375991003, -21.55341960407610458, 67.70724293864769550 ) ) ;
#64087=CARTESIAN_POINT ( 'NONE',  ( 5.049401038298161559, -19.05341960407611168, 42.70724293864767418 ) ) ;
#64088=CARTESIAN_POINT ( 'NONE',  ( -8.224510206698735004, -14.34966873604973081, 79.58442372801903275 ) ) ;
#64090=CARTESIAN_POINT ( 'NONE',  ( 10.72451020669898902, -18.67979575497178502, 102.9155762719810383 ) ) ;
#64091=CARTESIAN_POINT ( 'NONE',  ( -12.06949235617756955, 12.14591786802309770, 55.62390960531436690 ) ) ;
#64092=CARTESIAN_POINT ( 'NONE',  ( 16.46253265017160672, -9.564922557960803928, 68.33224293864770971 ) ) ;
#64093=CARTESIAN_POINT ( 'NONE',  ( 4.483927247898790824, -16.52544592524335698, 75.20942372801901854 ) ) ;
#64094=CARTESIAN_POINT ( 'NONE',  ( 14.34966873604972726, -8.224510206698740333, 20.83442372801901143 ) ) ;
#64095=CARTESIAN_POINT ( 'NONE',  ( -21.53943276465977519, 0.05219959533907696930, 116.2489096053143669 ) ) ;
#64096=CARTESIAN_POINT ( 'NONE',  ( 8.314922557960818139, 14.29746914071049879, 39.58224293864769550 ) ) ;
#64098=CARTESIAN_POINT ( 'NONE',  ( -17.40861289038999971, 6.110651285853370140, 73.62767529172565162 ) ) ;
#64099=( BOUNDED_CURVE ( )  B_SPLINE_CURVE ( 2, ( #1539, #139062, #185576, #199757, #197773, #170405, #91549, #30906, #60234, #137079, #119931, #123879, #181616 ),
 .UNSPECIFIED., .F., .T. ) 
 B_SPLINE_CURVE_WITH_KNOTS ( ( 3, 2, 2, 2, 2, 2, 3 ),
 ( 0.5551076951965037143, 0.5570175438596490780, 0.5614035087719297934, 0.5657894736842105088, 0.5701754385964912242, 0.5745614035087719396, 0.5765169319940076642 ),
 .UNSPECIFIED. ) 
 CURVE ( )  GEOMETRIC_REPRESENTATION_ITEM ( )  RATIONAL_B_SPLINE_CURVE ( ( 0.9832469066685283199, 0.9851625545550095620, 1.000000000000000000, 0.9659258262890683122, 1.000000000000000000, 0.9659258262890683122, 1.000000000000000000, 0.9659258262890683122, 1.000000000000000000, 0.9659258262890683122, 1.000000000000000000, 0.9848076720550078544, 0.9831626618144001517 ) ) 
 REPRESENTATION_ITEM ( '' )  );
#64100=CARTESIAN_POINT ( 'NONE',  ( -10.81492255796078084, -18.62759615963271287, 87.08224293864769550 ) ) ;
#64101=CARTESIAN_POINT ( 'NONE',  ( 14.34966873604960469, 8.224510206698951720, 24.16557627198103120 ) ) ;
#64102=ORIENTED_EDGE ( 'NONE', *, *, #166008, .T. ) ;
#64103=CARTESIAN_POINT ( 'NONE',  ( -17.44279575226823908, -5.990770900252486264, 54.16442432485681735 ) ) ;
#64104=CARTESIAN_POINT ( 'NONE',  ( 0.05219959533907565091, 21.53943276465977519, 99.99890960531436690 ) ) ;
#64105=CARTESIAN_POINT ( 'NONE',  ( 19.02544592524343514, -5.153800228976328945, 108.5405762719810383 ) ) ;
#64106=CARTESIAN_POINT ( 'NONE',  ( -15.72974639402197994, 15.80617190586746368, 115.6239096053143669 ) ) ;
#64107=CARTESIAN_POINT ( 'NONE',  ( 16.55341960407611168, 4.379528057220329451, 48.95724293864770971 ) ) ;
#64108=CARTESIAN_POINT ( 'NONE',  ( -16.53943276465976808, -0.05219959533934237506, 48.75109039468568284 ) ) ;
#64109=CARTESIAN_POINT ( 'NONE',  ( -5.049401038298153566, 19.05341960407611168, 55.20724293864769550 ) ) ;
#64111=CARTESIAN_POINT ( 'NONE',  ( -13.89961937509957401, -13.97604488694547875, 54.37609039468565442 ) ) ;
#64112=CARTESIAN_POINT ( 'NONE',  ( 16.46253265017160672, -9.564922557960803928, 83.33224293864768129 ) ) ;
#64114=CARTESIAN_POINT ( 'NONE',  ( -15.80617190586745835, -15.72974639402198527, 36.87390960531435979 ) ) ;
#64116=CARTESIAN_POINT ( 'NONE',  ( -19.03943276465977164, 0.05219959533909376836, 46.24890960531435979 ) ) ;
#64117=CARTESIAN_POINT ( 'NONE',  ( -19.05341960407617563, 5.049401038297882671, 113.5427570613523471 ) ) ;
#64118=CARTESIAN_POINT ( 'NONE',  ( 9.474510206698729675, 16.51473224551082808, 62.08442372801899722 ) ) ;
#64119=CARTESIAN_POINT ( 'NONE',  ( -15.80617190586745835, -15.72974639402198527, 101.8739096053143811 ) ) ;
#64120=CARTESIAN_POINT ( 'NONE',  ( -4.379528057220328563, 16.55341960407611168, 35.20724293864768839 ) ) ;
#64121=CARTESIAN_POINT ( 'NONE',  ( 0.05219959533909260263, 19.03943276465977164, 74.99890960531435269 ) ) ;
#64122=CARTESIAN_POINT ( 'NONE',  ( -0.05219959533907301413, -21.53943276465977519, 62.49890960531436690 ) ) ;
#64123=CARTESIAN_POINT ( 'NONE',  ( 0.05219959533907565091, 21.53943276465977519, 99.99890960531436690 ) ) ;
#64124=CARTESIAN_POINT ( 'NONE',  ( -16.52544592524335698, -4.483927247898792601, 23.95942372801901143 ) ) ;
#64125=CARTESIAN_POINT ( 'NONE',  ( -5.823673210054116645, -21.52544592524344225, 22.29057627198102765 ) ) ;
#64126=CARTESIAN_POINT ( 'NONE',  ( -10.72451020669870658, -18.67979575497194134, 94.58442372801901854 ) ) ;
#64127=CARTESIAN_POINT ( 'NONE',  ( -16.46253265017160317, 9.564922557960807481, 80.83224293864769550 ) ) ;
#64128=CARTESIAN_POINT ( 'NONE',  ( 19.02544592524343514, -5.153800228976328945, 23.54057627198102054 ) ) ;
#64129=CARTESIAN_POINT ( 'NONE',  ( -9.474510206698964154, 16.51473224551069663, 85.41557627198102409 ) ) ;
#64130=CARTESIAN_POINT ( 'NONE',  ( -16.53943276465976808, 0.05219959533911058130, 111.2489096053143669 ) ) ;
#64131=CARTESIAN_POINT ( 'NONE',  ( -0.05219959533909027116, -19.03943276465977164, 62.49890960531435979 ) ) ;
#64132=CARTESIAN_POINT ( 'NONE',  ( 16.53943276465976808, 0.05219959533934440121, 26.25109039468567573 ) ) ;
#64135=CARTESIAN_POINT ( 'NONE',  ( 0.05219959533937995610, -21.53943276465977519, 100.0010903946857042 ) ) ;
#64136=CARTESIAN_POINT ( 'NONE',  ( -13.97604488694527625, -13.89961937509977652, 111.8739096053143243 ) ) ;
#64137=CARTESIAN_POINT ( 'NONE',  ( 12.14591786802327356, -12.06949235617739191, 85.62609039468568994 ) ) ;
#64138=FACE_OUTER_BOUND ( 'NONE', #195502, .T. ) ;
#64139=CARTESIAN_POINT ( 'NONE',  ( 5.153800228976615827, -19.02544592524334988, 70.20942372801899012 ) ) ;
#64140=CARTESIAN_POINT ( 'NONE',  ( 5.049401038297881783, 19.05341960407617563, 37.29275706135232582 ) ) ;
#64142=CARTESIAN_POINT ( 'NONE',  ( 16.51473224551069308, 9.474510206698969483, 34.16557627198102409 ) ) ;
#64143=CARTESIAN_POINT ( 'NONE',  ( -12.14591786802309592, -12.06949235617757132, 36.87390960531435979 ) ) ;
#64145=CARTESIAN_POINT ( 'NONE',  ( 14.34966873604972726, -8.224510206698740333, 110.8344237280190043 ) ) ;
#64146=CARTESIAN_POINT ( 'NONE',  ( 16.38665767535055551, 7.295008042176072571, 67.23599135785453029 ) ) ;
#64147=CARTESIAN_POINT ( 'NONE',  ( -14.34966873604972548, 8.224510206698743886, 83.33442372801903275 ) ) ;
#64148=CARTESIAN_POINT ( 'NONE',  ( -16.51473224551069308, -9.474510206698971260, 36.66557627198102409 ) ) ;
#64149=CARTESIAN_POINT ( 'NONE',  ( 10.81492255796106328, -18.62759615963255655, 100.4177570613523471 ) ) ;
#64150=CARTESIAN_POINT ( 'NONE',  ( 9.474510206698729675, 16.51473224551082808, 97.08442372801900433 ) ) ;
#64151=CARTESIAN_POINT ( 'NONE',  ( -0.05219959533937732626, 21.53943276465977519, 77.50109039468567573 ) ) ;
#64152=CARTESIAN_POINT ( 'NONE',  ( -13.89961937509957401, -13.97604488694547875, 59.37609039468566863 ) ) ;
#64153=CARTESIAN_POINT ( 'NONE',  ( 19.05341960407611168, 5.049401038298154454, 98.95724293864766707 ) ) ;
#64154=CARTESIAN_POINT ( 'NONE',  ( -13.97604488694527625, -13.89961937509977652, 66.87390960531436690 ) ) ;
#64156=CARTESIAN_POINT ( 'NONE',  ( -12.06949235617756955, 12.14591786802309770, 65.62390960531436690 ) ) ;
#64157=CARTESIAN_POINT ( 'NONE',  ( 18.62759615963271287, -10.81492255796078972, 63.33224293864770260 ) ) ;
#64158=CARTESIAN_POINT ( 'NONE',  ( -9.474510206698964154, 16.51473224551069663, 50.41557627198102409 ) ) ;
#64159=CARTESIAN_POINT ( 'NONE',  ( 5.719274019375991003, -21.55341960407610458, 87.70724293864769550 ) ) ;
#64160=CARTESIAN_POINT ( 'NONE',  ( 16.53943276465976808, 0.05219959533934440121, 71.25109039468568994 ) ) ;
#64162=CARTESIAN_POINT ( 'NONE',  ( 19.02544592524343514, -5.153800228976328945, 43.54057627198103120 ) ) ;
#64163=CARTESIAN_POINT ( 'NONE',  ( 8.314922557960818139, 14.29746914071049879, 84.58224293864769550 ) ) ;
#64165=CARTESIAN_POINT ( 'NONE',  ( 16.51473224551069308, 9.474510206698969483, 54.16557627198103120 ) ) ;
#64166=CARTESIAN_POINT ( 'NONE',  ( -0.05219959533909027116, -19.03943276465977164, 22.49890960531436690 ) ) ;
#64167=CARTESIAN_POINT ( 'NONE',  ( -5.049401038297874678, -19.05341960407617918, 69.79275706135233293 ) ) ;
#64168=CARTESIAN_POINT ( 'NONE',  ( -14.29746914071049879, 8.314922557960819915, 70.83224293864770971 ) ) ;
#64169=CARTESIAN_POINT ( 'NONE',  ( -21.55341960407619339, 5.719274019375674811, 43.54275706135235424 ) ) ;
#64170=CARTESIAN_POINT ( 'NONE',  ( 16.51473224551069308, 9.474510206698969483, 39.16557627198103120 ) ) ;
#64171=CARTESIAN_POINT ( 'NONE',  ( -18.67979575497178146, -10.72451020669898902, 101.6655762719810383 ) ) ;
#64172=CARTESIAN_POINT ( 'NONE',  ( -17.50000000000000000, -5.499999999999992895, 37.50000000000000000 ) ) ;
#64173=CARTESIAN_POINT ( 'NONE',  ( 4.483927247898545687, 16.52544592524342804, 84.79057627198102409 ) ) ;
#64175=CARTESIAN_POINT ( 'NONE',  ( -16.46253265017160317, 9.564922557960807481, 40.83224293864769550 ) ) ;
#64176=CARTESIAN_POINT ( 'NONE',  ( 17.05116617787822975, 6.768360034955811955, 113.8432444674080557 ) ) ;
#64177=CARTESIAN_POINT ( 'NONE',  ( -19.03943276465977164, -0.05219959533935918106, 88.75109039468567573 ) ) ;
#64178=CARTESIAN_POINT ( 'NONE',  ( -5.823673210054431948, 21.52544592524334988, 42.70942372801901854 ) ) ;
#64179=CARTESIAN_POINT ( 'NONE',  ( -0.05219959533909027116, -19.03943276465977164, 77.49890960531435269 ) ) ;
#64180=CARTESIAN_POINT ( 'NONE',  ( 13.97604488694548053, -13.89961937509957401, 70.62609039468567573 ) ) ;
#64181=CARTESIAN_POINT ( 'NONE',  ( 5.153800228976335163, 19.02544592524342804, 39.79057627198100988 ) ) ;
#64182=CARTESIAN_POINT ( 'NONE',  ( -14.29746914071049879, 8.314922557960819915, 65.83224293864769550 ) ) ;
#64183=CARTESIAN_POINT ( 'NONE',  ( 0.05219959533910956823, 16.53943276465976808, 64.99890960531435269 ) ) ;
#64184=CARTESIAN_POINT ( 'NONE',  ( -13.89961937509977652, 13.97604488694528158, 70.62390960531432427 ) ) ;
#64185=CARTESIAN_POINT ( 'NONE',  ( -0.05219959533907301413, -21.53943276465977519, 97.49890960531436690 ) ) ;
#64186=CARTESIAN_POINT ( 'NONE',  ( 13.89961937509977652, -13.97604488694527269, 73.12390960531436690 ) ) ;
#64187=CARTESIAN_POINT ( 'NONE',  ( -15.80617190586768217, 15.72974639402176855, 108.1260903946856757 ) ) ;
#64188=CARTESIAN_POINT ( 'NONE',  ( 19.02544592524343514, -5.153800228976328945, 33.54057627198102409 ) ) ;
#64189=CARTESIAN_POINT ( 'NONE',  ( -12.14591786802309592, -12.06949235617757132, 21.87390960531436690 ) ) ;
#64190=CARTESIAN_POINT ( 'NONE',  ( 14.34966873604960469, 8.224510206698951720, 109.1655762719810383 ) ) ;
#64191=CARTESIAN_POINT ( 'NONE',  ( -13.89961937509957401, -13.97604488694547875, 99.37609039468567573 ) ) ;
#64193=CARTESIAN_POINT ( 'NONE',  ( 21.55341960407619695, -5.719274019375665929, 36.04275706135234714 ) ) ;
#64194=CARTESIAN_POINT ( 'NONE',  ( -19.02544592524334988, -5.153800228976617603, 53.95942372801898301 ) ) ;
#64195=CARTESIAN_POINT ( 'NONE',  ( -16.53943276465976808, -0.05219959533934237506, 113.7510903946856757 ) ) ;
#64196=CARTESIAN_POINT ( 'NONE',  ( 5.823673210054125526, 21.52544592524343514, 74.79057627198105251 ) ) ;
#64197=CARTESIAN_POINT ( 'NONE',  ( 10.72451020669898902, -18.67979575497178502, 22.91557627198102765 ) ) ;
#64198=CARTESIAN_POINT ( 'NONE',  ( 4.483927247898545687, 16.52544592524342804, 54.79057627198104541 ) ) ;
#64199=CARTESIAN_POINT ( 'NONE',  ( -19.02544592524342804, 5.153800228976336051, 36.04057627198100988 ) ) ;
#64200=CARTESIAN_POINT ( 'NONE',  ( -13.89961937509977652, 13.97604488694528158, 35.62390960531435269 ) ) ;
#64201=CARTESIAN_POINT ( 'NONE',  ( -19.03943276465977164, -0.05219959533935918106, 33.75109039468566863 ) ) ;
#64202=CARTESIAN_POINT ( 'NONE',  ( 4.483927247898790824, -16.52544592524335698, 90.20942372801903275 ) ) ;
#64203=CARTESIAN_POINT ( 'NONE',  ( -12.06949235617739369, -12.14591786802326823, 49.37609039468569705 ) ) ;
#64204=CARTESIAN_POINT ( 'NONE',  ( 21.55341960407610458, 5.719274019375980345, 23.95724293864769550 ) ) ;
#64205=CARTESIAN_POINT ( 'NONE',  ( 9.474510206698971260, -16.51473224551069308, 57.91557627198103120 ) ) ;
#64206=CARTESIAN_POINT ( 'NONE',  ( 21.53943276465977519, 0.05219959533937863772, 91.25109039468568994 ) ) ;
#64207=CARTESIAN_POINT ( 'NONE',  ( -5.049401038298153566, 19.05341960407611168, 85.20724293864766707 ) ) ;
#64208=CARTESIAN_POINT ( 'NONE',  ( -8.314922557961024197, 14.29746914071037800, 62.91775706135236135 ) ) ;
#64209=CARTESIAN_POINT ( 'NONE',  ( 16.55341960407611168, 4.379528057220329451, 108.9572429386476955 ) ) ;
#64211=CARTESIAN_POINT ( 'NONE',  ( -4.483927247898539470, -16.52544592524342804, 27.29057627198103120 ) ) ;
#64213=CARTESIAN_POINT ( 'NONE',  ( 15.80617190586769283, -15.72974639402175789, 70.62609039468567573 ) ) ;
#64214=CARTESIAN_POINT ( 'NONE',  ( 5.153800228976335163, 19.02544592524342804, 94.79057627198103830 ) ) ;
#64215=CARTESIAN_POINT ( 'NONE',  ( -19.03943276465977164, 0.05219959533909376836, 76.24890960531435269 ) ) ;
#64216=CARTESIAN_POINT ( 'NONE',  ( -13.97604488694527625, -13.89961937509977652, 111.8739096053143243 ) ) ;
#64217=CARTESIAN_POINT ( 'NONE',  ( -16.52544592524342804, 4.483927247898546575, 61.04057627198103120 ) ) ;
#64218=CARTESIAN_POINT ( 'NONE',  ( -14.29746914071037622, -8.314922557961029526, 109.1677570613523613 ) ) ;
#64220=CARTESIAN_POINT ( 'NONE',  ( -16.55341960407611168, -4.379528057220339221, 41.45724293864769550 ) ) ;
#64221=CARTESIAN_POINT ( 'NONE',  ( -8.224510206698735004, -14.34966873604973081, 39.58442372801901143 ) ) ;
#64223=CARTESIAN_POINT ( 'NONE',  ( -19.03943276465977164, -0.05219959533935918106, 33.75109039468566863 ) ) ;
#64224=CARTESIAN_POINT ( 'NONE',  ( 5.049401038298161559, -19.05341960407611168, 82.70724293864770971 ) ) ;
#64225=CARTESIAN_POINT ( 'NONE',  ( -19.02544592524334988, -5.153800228976617603, 53.95942372801898301 ) ) ;
#64228=CARTESIAN_POINT ( 'NONE',  ( 16.51473224551083163, -9.474510206698727899, 85.83442372801900433 ) ) ;
#64229=CARTESIAN_POINT ( 'NONE',  ( 8.224510206698742110, 14.34966873604972548, 82.08442372801901854 ) ) ;
#64230=CARTESIAN_POINT ( 'NONE',  ( -19.03943276465977164, 0.05219959533909376836, 26.24890960531435624 ) ) ;
#64231=CARTESIAN_POINT ( 'NONE',  ( 16.51473224551069308, 9.474510206698969483, 99.16557627198102409 ) ) ;
#64232=CARTESIAN_POINT ( 'NONE',  ( 10.81492255796106328, -18.62759615963255655, 45.41775706135234003 ) ) ;
#64233=CARTESIAN_POINT ( 'NONE',  ( 19.03943276465977164, 0.05219959533936151252, 96.25109039468567573 ) ) ;
#64235=CARTESIAN_POINT ( 'NONE',  ( 19.03943276465977164, -0.05219959533909143690, 53.74890960531436690 ) ) ;
#64236=CARTESIAN_POINT ( 'NONE',  ( -19.03943276465977164, 0.05219959533909376836, 106.2489096053143669 ) ) ;
#64237=CARTESIAN_POINT ( 'NONE',  ( 4.379528057220339221, -16.55341960407611168, 67.70724293864769550 ) ) ;
#64238=CARTESIAN_POINT ( 'NONE',  ( 9.474510206698971260, -16.51473224551069308, 52.91557627198102409 ) ) ;
#64239=CARTESIAN_POINT ( 'NONE',  ( -13.97604488694527625, -13.89961937509977652, 61.87390960531435979 ) ) ;
#64240=CARTESIAN_POINT ( 'NONE',  ( 0.05219959533936267826, -19.03943276465977164, 60.00109039468566863 ) ) ;
#64241=CARTESIAN_POINT ( 'NONE',  ( 19.03943276465977164, 0.05219959533936151252, 31.25109039468566863 ) ) ;
#64242=CARTESIAN_POINT ( 'NONE',  ( 9.474510206698971260, -16.51473224551069308, 62.91557627198102409 ) ) ;
#64243=CARTESIAN_POINT ( 'NONE',  ( 15.72974639402199770, -15.80617190586745480, 73.12390960531436690 ) ) ;
#64244=CARTESIAN_POINT ( 'NONE',  ( -4.483927247898539470, -16.52544592524342804, 62.29057627198102409 ) ) ;
#64245=CARTESIAN_POINT ( 'NONE',  ( 19.02544592524334988, 5.153800228976608722, 36.45942372801900433 ) ) ;
#64246=CARTESIAN_POINT ( 'NONE',  ( -18.67979575497178146, -10.72451020669898902, 51.66557627198102409 ) ) ;
#64247=CARTESIAN_POINT ( 'NONE',  ( -18.62759615963270932, 10.81492255796079327, 35.83224293864768839 ) ) ;
#64248=CARTESIAN_POINT ( 'NONE',  ( 5.153800228976335163, 19.02544592524342804, 59.79057627198100988 ) ) ;
#64249=CARTESIAN_POINT ( 'NONE',  ( 13.89961937509977652, -13.97604488694527269, 43.12390960531434558 ) ) ;
#64250=CARTESIAN_POINT ( 'NONE',  ( 0.05219959533910956823, 16.53943276465976808, 94.99890960531436690 ) ) ;
#64251=CARTESIAN_POINT ( 'NONE',  ( 0.05219959533907565091, 21.53943276465977519, 104.9989096053143669 ) ) ;
#64252=CARTESIAN_POINT ( 'NONE',  ( 9.564922557960805705, 16.46253265017160317, 109.5822429386476955 ) ) ;
#64253=CARTESIAN_POINT ( 'NONE',  ( 18.67979575497194134, -10.72451020669871369, 25.83442372801901499 ) ) ;
#64254=CARTESIAN_POINT ( 'NONE',  ( 9.564922557960805705, 16.46253265017160317, 39.58224293864768839 ) ) ;
#64255=CARTESIAN_POINT ( 'NONE',  ( 5.719274019375991003, -21.55341960407610458, 107.7072429386476955 ) ) ;
#64256=CARTESIAN_POINT ( 'NONE',  ( -16.46253265017146816, -9.564922557961047289, 49.16775706135233293 ) ) ;
#64257=CARTESIAN_POINT ( 'NONE',  ( -13.89961937509977652, 13.97604488694528158, 25.62390960531434558 ) ) ;
#64258=CARTESIAN_POINT ( 'NONE',  ( 18.87075004821566182, -5.500000000000074607, 76.17408112101045958 ) ) ;
#64260=CARTESIAN_POINT ( 'NONE',  ( -4.483927247898782831, 16.52544592524335698, 52.70942372801902565 ) ) ;
#64261=CARTESIAN_POINT ( 'NONE',  ( 19.05341960407611168, 5.049401038298154454, 23.95724293864769194 ) ) ;
#64263=CARTESIAN_POINT ( 'NONE',  ( 13.89961937509977652, -13.97604488694527269, 68.12390960531436690 ) ) ;
#64264=CARTESIAN_POINT ( 'NONE',  ( 4.379528057220339221, -16.55341960407611168, 107.7072429386476955 ) ) ;
#64265=CARTESIAN_POINT ( 'NONE',  ( -21.52544592524343514, 5.823673210054127303, 41.04057627198103120 ) ) ;
#64266=CARTESIAN_POINT ( 'NONE',  ( 8.314922557960818139, 14.29746914071049879, 79.58224293864769550 ) ) ;
#64267=CARTESIAN_POINT ( 'NONE',  ( -8.314922557961024197, 14.29746914071037800, 37.91775706135235424 ) ) ;
#64268=CARTESIAN_POINT ( 'NONE',  ( -5.823673210054431948, 21.52544592524334988, 87.70942372801901854 ) ) ;
#64269=CARTESIAN_POINT ( 'NONE',  ( -19.05341960407611168, -5.049401038298163336, 31.45724293864769550 ) ) ;
#64270=CARTESIAN_POINT ( 'NONE',  ( -14.34966873604972548, 8.224510206698743886, 113.3344237280190328 ) ) ;
#64271=CARTESIAN_POINT ( 'NONE',  ( -16.52544592524342804, 4.483927247898546575, 61.04057627198103120 ) ) ;
#64272=CARTESIAN_POINT ( 'NONE',  ( 9.564922557960805705, 16.46253265017160317, 54.58224293864769550 ) ) ;
#64273=CARTESIAN_POINT ( 'NONE',  ( -21.53943276465977519, -0.05219959533937600094, 93.75109039468567573 ) ) ;
#64274=CARTESIAN_POINT ( 'NONE',  ( 21.55341960407610458, 5.719274019375980345, 113.9572429386477239 ) ) ;
#64275=CARTESIAN_POINT ( 'NONE',  ( 18.67979575497194134, -10.72451020669871369, 70.83442372801901854 ) ) ;
#64276=CARTESIAN_POINT ( 'NONE',  ( -4.379528057220086978, -16.55341960407618274, 44.79275706135234714 ) ) ;
#64277=CARTESIAN_POINT ( 'NONE',  ( 0.05219959533910956823, 16.53943276465976808, 84.99890960531436690 ) ) ;
#64278=CARTESIAN_POINT ( 'NONE',  ( 18.62759615963255655, 10.81492255796105972, 86.66775706135234714 ) ) ;
#64279=CARTESIAN_POINT ( 'NONE',  ( -14.34966873604972548, 8.224510206698743886, 113.3344237280190328 ) ) ;
#64280=CARTESIAN_POINT ( 'NONE',  ( -17.50000000000000000, 5.624438216177581218, 115.8167034491465017 ) ) ;
#64281=CARTESIAN_POINT ( 'NONE',  ( 0.05219959533934541429, -16.53943276465976808, 40.00109039468567573 ) ) ;
#64282=CARTESIAN_POINT ( 'NONE',  ( -12.14591786802309592, -12.06949235617757132, 41.87390960531435979 ) ) ;
#64283=CARTESIAN_POINT ( 'NONE',  ( 12.14591786802327356, -12.06949235617739191, 85.62609039468568994 ) ) ;
#64284=CARTESIAN_POINT ( 'NONE',  ( 16.46253265017160672, -9.564922557960803928, 103.3322429386476955 ) ) ;
#64285=CARTESIAN_POINT ( 'NONE',  ( 16.51473224551069308, 9.474510206698969483, 94.16557627198103830 ) ) ;
#64286=CARTESIAN_POINT ( 'NONE',  ( -18.67979575497193778, 10.72451020669871902, 98.33442372801901854 ) ) ;
#64287=CARTESIAN_POINT ( 'NONE',  ( -0.05219959533934338120, 16.53943276465976808, 97.50109039468567573 ) ) ;
#64288=CARTESIAN_POINT ( 'NONE',  ( 8.314922557960818139, 14.29746914071049879, 69.58224293864769550 ) ) ;
#64289=CARTESIAN_POINT ( 'NONE',  ( 9.474510206698971260, -16.51473224551069308, 82.91557627198103830 ) ) ;
#64291=CARTESIAN_POINT ( 'NONE',  ( 8.224510206698742110, 14.34966873604972548, 27.08442372801901854 ) ) ;
#64292=CARTESIAN_POINT ( 'NONE',  ( 13.97604488694527802, 13.89961937509977652, 34.37390960531436690 ) ) ;
#64293=CARTESIAN_POINT ( 'NONE',  ( 13.97604488694527802, 13.89961937509977652, 89.37390960531436690 ) ) ;
#64294=CARTESIAN_POINT ( 'NONE',  ( -16.53943276465976808, -0.05219959533934237506, 28.75109039468567929 ) ) ;
#64295=CARTESIAN_POINT ( 'NONE',  ( 17.72662750342725602, 5.500000000000080824, 68.90179492283743912 ) ) ;
#64296=CARTESIAN_POINT ( 'NONE',  ( 13.89961937509957401, 13.97604488694547697, 41.87609039468566152 ) ) ;
#64297=CARTESIAN_POINT ( 'NONE',  ( 8.314922557961029526, -14.29746914071037800, 95.41775706135234714 ) ) ;
#64298=CARTESIAN_POINT ( 'NONE',  ( -5.153800228976607833, 19.02544592524334988, 107.7094237280189759 ) ) ;
#64299=CARTESIAN_POINT ( 'NONE',  ( 9.564922557960805705, 16.46253265017160317, 29.58224293864769550 ) ) ;
#64300=CARTESIAN_POINT ( 'NONE',  ( 16.55341960407618274, -4.379528057220086978, 86.04275706135236135 ) ) ;
#64301=CARTESIAN_POINT ( 'NONE',  ( 12.06949235617739724, 12.14591786802326823, 61.87609039468568284 ) ) ;
#64302=CARTESIAN_POINT ( 'NONE',  ( 0.05219959533909260263, 19.03943276465977164, 24.99890960531435269 ) ) ;
#64303=CARTESIAN_POINT ( 'NONE',  ( -19.03943276465977164, -0.05219959533935918106, 63.75109039468566863 ) ) ;
#64304=CARTESIAN_POINT ( 'NONE',  ( -10.72451020669870658, -18.67979575497194134, 109.5844237280190328 ) ) ;
#64305=CARTESIAN_POINT ( 'NONE',  ( 9.564922557960805705, 16.46253265017160317, 49.58224293864770260 ) ) ;
#64306=CARTESIAN_POINT ( 'NONE',  ( 19.05341960407611168, 5.049401038298154454, 88.95724293864769550 ) ) ;
#64307=CARTESIAN_POINT ( 'NONE',  ( 16.53943276465976808, -0.05219959533910856209, 83.74890960531435269 ) ) ;
#64308=CARTESIAN_POINT ( 'NONE',  ( 13.97604488694548053, -13.89961937509957401, 60.62609039468564731 ) ) ;
#64309=CARTESIAN_POINT ( 'NONE',  ( 5.823673210054125526, 21.52544592524343514, 49.79057627198102409 ) ) ;
#64310=CARTESIAN_POINT ( 'NONE',  ( -21.52544592524334988, -5.823673210054445271, 108.9594237280190185 ) ) ;
#64311=CARTESIAN_POINT ( 'NONE',  ( -13.89961937509977652, 13.97604488694528158, 90.62390960531432427 ) ) ;
#64312=CARTESIAN_POINT ( 'NONE',  ( 16.51473224551083163, -9.474510206698727899, 30.83442372801900433 ) ) ;
#64313=CARTESIAN_POINT ( 'NONE',  ( -15.72974639402197994, 15.80617190586746368, 60.62390960531437401 ) ) ;
#64314=CARTESIAN_POINT ( 'NONE',  ( -9.564922557960796823, -16.46253265017161027, 112.0822429386476955 ) ) ;
#64315=CARTESIAN_POINT ( 'NONE',  ( 5.153800228976615827, -19.02544592524334988, 85.20942372801900433 ) ) ;
#64317=CARTESIAN_POINT ( 'NONE',  ( 0.05219959533936267826, -19.03943276465977164, 110.0010903946856757 ) ) ;
#64318=CARTESIAN_POINT ( 'NONE',  ( 4.483927247898545687, 16.52544592524342804, 109.7905762719810383 ) ) ;
#64319=CARTESIAN_POINT ( 'NONE',  ( 5.153800228976335163, 19.02544592524342804, 99.79057627198102409 ) ) ;
#64320=CARTESIAN_POINT ( 'NONE',  ( -0.05219959533907301413, -21.53943276465977519, 72.49890960531435269 ) ) ;
#64321=AXIS2_PLACEMENT_3D ( 'NONE', #113127, #141492, #81773 ) ;
#64322=CARTESIAN_POINT ( 'NONE',  ( 14.29746914071037800, 8.314922557961029526, 41.66775706135235424 ) ) ;
#64323=CARTESIAN_POINT ( 'NONE',  ( 18.62759615963255655, 10.81492255796105972, 41.66775706135235424 ) ) ;
#64324=CARTESIAN_POINT ( 'NONE',  ( -5.823673210054431948, 21.52544592524334988, 97.70942372801904696 ) ) ;
#64325=CARTESIAN_POINT ( 'NONE',  ( 4.483927247898790824, -16.52544592524335698, 95.20942372801903275 ) ) ;
#64326=CARTESIAN_POINT ( 'NONE',  ( 0.05219959533909260263, 19.03943276465977164, 89.99890960531436690 ) ) ;
#64327=CARTESIAN_POINT ( 'NONE',  ( 16.53943276465976808, -0.05219959533910856209, 88.74890960531436690 ) ) ;
#64328=CARTESIAN_POINT ( 'NONE',  ( 0.05219959533910956823, 16.53943276465976808, 34.99890960531435979 ) ) ;
#64329=CARTESIAN_POINT ( 'NONE',  ( -5.049401038297874678, -19.05341960407617918, 69.79275706135233293 ) ) ;
#64330=CARTESIAN_POINT ( 'NONE',  ( 18.62759615963255655, 10.81492255796105972, 41.66775706135235424 ) ) ;
#64331=CARTESIAN_POINT ( 'NONE',  ( 13.97604488694548053, -13.89961937509957401, 25.62609039468566507 ) ) ;
#64332=CARTESIAN_POINT ( 'NONE',  ( -0.05219959533910754901, -16.53943276465976808, 92.49890960531436690 ) ) ;
#64333=CARTESIAN_POINT ( 'NONE',  ( 19.05341960407611168, 5.049401038298154454, 113.9572429386477097 ) ) ;
#64334=CARTESIAN_POINT ( 'NONE',  ( 8.224510206698742110, 14.34966873604972548, 112.0844237280190185 ) ) ;
#64335=CARTESIAN_POINT ( 'NONE',  ( 5.719274019375673035, 21.55341960407619339, 87.29275706135236135 ) ) ;
#64336=CARTESIAN_POINT ( 'NONE',  ( 16.53943276465976808, 0.05219959533934440121, 61.25109039468567573 ) ) ;
#64337=CARTESIAN_POINT ( 'NONE',  ( -4.483927247898782831, 16.52544592524335698, 102.7094237280190185 ) ) ;
#64338=CARTESIAN_POINT ( 'NONE',  ( -15.80617190586768217, 15.72974639402176855, 53.12609039468568284 ) ) ;
#64340=CARTESIAN_POINT ( 'NONE',  ( 18.62759615963255655, 10.81492255796105972, 31.66775706135234358 ) ) ;
#64341=CARTESIAN_POINT ( 'NONE',  ( -4.379528057220328563, 16.55341960407611168, 110.2072429386477239 ) ) ;
#64342=CARTESIAN_POINT ( 'NONE',  ( -9.564922557960796823, -16.46253265017161027, 22.08224293864768839 ) ) ;
#64343=CARTESIAN_POINT ( 'NONE',  ( 4.483927247898545687, 16.52544592524342804, 59.79057627198103120 ) ) ;
#64344=CARTESIAN_POINT ( 'NONE',  ( -9.474510206698964154, 16.51473224551069663, 75.41557627198103830 ) ) ;
#64345=CARTESIAN_POINT ( 'NONE',  ( -8.314922557961024197, 14.29746914071037800, 107.9177570613523471 ) ) ;
#64346=CARTESIAN_POINT ( 'NONE',  ( -0.05219959533909027116, -19.03943276465977164, 37.49890960531436690 ) ) ;
#64347=CARTESIAN_POINT ( 'NONE',  ( -21.53943276465977519, 0.05219959533907696930, 51.24890960531436690 ) ) ;
#64348=CARTESIAN_POINT ( 'NONE',  ( -8.314922557960811034, -14.29746914071050412, 97.08224293864770971 ) ) ;
#64349=CARTESIAN_POINT ( 'NONE',  ( -10.81492255796078084, -18.62759615963271287, 92.08224293864769550 ) ) ;
#64350=CARTESIAN_POINT ( 'NONE',  ( 5.153800228976335163, 19.02544592524342804, 94.79057627198103830 ) ) ;
#64351=CARTESIAN_POINT ( 'NONE',  ( -13.89961937509977652, 13.97604488694528158, 55.62390960531434558 ) ) ;
#64352=CARTESIAN_POINT ( 'NONE',  ( 16.51473224551083163, -9.474510206698727899, 95.83442372801900433 ) ) ;
#64353=CARTESIAN_POINT ( 'NONE',  ( 15.80617190586746368, 15.72974639402197994, 49.37390960531436690 ) ) ;
#64354=CARTESIAN_POINT ( 'NONE',  ( -21.52544592524334988, -5.823673210054445271, 68.95942372801901854 ) ) ;
#64355=CARTESIAN_POINT ( 'NONE',  ( -19.02544592524342804, 5.153800228976336051, 56.04057627198100988 ) ) ;
#64356=CARTESIAN_POINT ( 'NONE',  ( -0.05219959533909027116, -19.03943276465977164, 87.49890960531436690 ) ) ;
#64357=CARTESIAN_POINT ( 'NONE',  ( 0.05219959533934541429, -16.53943276465976808, 65.00109039468568994 ) ) ;
#64358=CARTESIAN_POINT ( 'NONE',  ( -15.72974639402176322, -15.80617190586768395, 49.37609039468569705 ) ) ;
#64359=CARTESIAN_POINT ( 'NONE',  ( -15.80617190586768217, 15.72974639402176855, 88.12609039468570415 ) ) ;
#64360=CARTESIAN_POINT ( 'NONE',  ( -21.55341960407610458, -5.719274019375992779, 101.4572429386476955 ) ) ;
#64361=CARTESIAN_POINT ( 'NONE',  ( 21.52544592524334988, 5.823673210054432836, 31.45942372801901854 ) ) ;
#64362=CARTESIAN_POINT ( 'NONE',  ( 12.14591786802327356, -12.06949235617739191, 65.62609039468568994 ) ) ;
#64363=CARTESIAN_POINT ( 'NONE',  ( 10.72451020669898902, -18.67979575497178502, 62.91557627198102409 ) ) ;
#64364=CARTESIAN_POINT ( 'NONE',  ( -16.51473224551082808, 9.474510206698731452, 33.33442372801899722 ) ) ;
#64365=CARTESIAN_POINT ( 'NONE',  ( -13.97604488694527625, -13.89961937509977652, 61.87390960531435979 ) ) ;
#64366=CARTESIAN_POINT ( 'NONE',  ( 14.34966873604960469, 8.224510206698951720, 29.16557627198103120 ) ) ;
#64368=CARTESIAN_POINT ( 'NONE',  ( -9.474510206698964154, 16.51473224551069663, 105.4155762719810383 ) ) ;
#64371=CARTESIAN_POINT ( 'NONE',  ( -19.02544592524334988, -5.153800228976617603, 83.95942372801901854 ) ) ;
#64372=CARTESIAN_POINT ( 'NONE',  ( 21.55341960407610458, 5.719274019375980345, 53.95724293864770260 ) ) ;
#64373=CARTESIAN_POINT ( 'NONE',  ( -14.34966873604960291, -8.224510206698953496, 36.66557627198103120 ) ) ;
#64374=CARTESIAN_POINT ( 'NONE',  ( 16.55341960407618274, -4.379528057220086978, 21.04275706135234714 ) ) ;
#64375=CARTESIAN_POINT ( 'NONE',  ( -16.51473224551069308, -9.474510206698971260, 31.66557627198102054 ) ) ;
#64376=CARTESIAN_POINT ( 'NONE',  ( 4.483927247898790824, -16.52544592524335698, 20.20942372801900788 ) ) ;
#64377=CARTESIAN_POINT ( 'NONE',  ( 5.823673210054125526, 21.52544592524343514, 94.79057627198105251 ) ) ;
#64378=CARTESIAN_POINT ( 'NONE',  ( 13.89961937509957401, 13.97604488694547697, 66.87609039468567573 ) ) ;
#64379=CARTESIAN_POINT ( 'NONE',  ( -4.483927247898782831, 16.52544592524335698, 82.70942372801900433 ) ) ;
#64380=CARTESIAN_POINT ( 'NONE',  ( 19.02544592524343514, -5.153800228976328945, 63.54057627198103830 ) ) ;
#64381=CARTESIAN_POINT ( 'NONE',  ( -4.379528057220328563, 16.55341960407611168, 70.20724293864769550 ) ) ;
#64382=CARTESIAN_POINT ( 'NONE',  ( -13.97604488694527625, -13.89961937509977652, 66.87390960531436690 ) ) ;
#64383=CARTESIAN_POINT ( 'NONE',  ( 4.483927247898545687, 16.52544592524342804, 59.79057627198103120 ) ) ;
#64384=CARTESIAN_POINT ( 'NONE',  ( -19.03943276465977164, 0.05219959533909376836, 21.24890960531436335 ) ) ;
#64386=CARTESIAN_POINT ( 'NONE',  ( 8.314922557960818139, 14.29746914071049879, 44.58224293864769550 ) ) ;
#64387=CARTESIAN_POINT ( 'NONE',  ( 16.51473224551069308, 9.474510206698969483, 74.16557627198103830 ) ) ;
#64389=CARTESIAN_POINT ( 'NONE',  ( 0.05219959533936267826, -19.03943276465977164, 40.00109039468566152 ) ) ;
#64390=CARTESIAN_POINT ( 'NONE',  ( 12.14591786802327356, -12.06949235617739191, 50.62609039468568994 ) ) ;
#64391=CARTESIAN_POINT ( 'NONE',  ( -18.67979575497178146, -10.72451020669898902, 66.66557627198102409 ) ) ;
#64392=CARTESIAN_POINT ( 'NONE',  ( 19.03943276465977164, 0.05219959533936151252, 21.25109039468565797 ) ) ;
#64393=CARTESIAN_POINT ( 'NONE',  ( 9.564922557960805705, 16.46253265017160317, 69.58224293864770971 ) ) ;
#64395=CARTESIAN_POINT ( 'NONE',  ( -13.97604488694527625, -13.89961937509977652, 111.8739096053143243 ) ) ;
#64396=CARTESIAN_POINT ( 'NONE',  ( -10.72451020669870658, -18.67979575497194134, 44.58442372801901854 ) ) ;
#64397=CARTESIAN_POINT ( 'NONE',  ( -16.53943276465976808, 0.05219959533911058130, 111.2489096053143669 ) ) ;
#64398=CARTESIAN_POINT ( 'NONE',  ( -15.72974639402197994, 15.80617190586746368, 95.62390960531436690 ) ) ;
#64399=CARTESIAN_POINT ( 'NONE',  ( 19.05341960407611168, 5.049401038298154454, 78.95724293864769550 ) ) ;
#64400=ORIENTED_EDGE ( 'NONE', *, *, #152637, .T. ) ;
#64401=CARTESIAN_POINT ( 'NONE',  ( 21.55341960407619695, -5.719274019375665929, 26.04275706135235779 ) ) ;
#64402=VERTEX_POINT ( 'NONE', #49046 ) ;
#64403=CARTESIAN_POINT ( 'NONE',  ( -5.049401038298153566, 19.05341960407611168, 90.20724293864766707 ) ) ;
#64405=CARTESIAN_POINT ( 'NONE',  ( 9.474510206698971260, -16.51473224551069308, 37.91557627198102409 ) ) ;
#64406=CARTESIAN_POINT ( 'NONE',  ( -9.564922557961040184, 16.46253265017147172, 102.9177570613523329 ) ) ;
#64408=CARTESIAN_POINT ( 'NONE',  ( -16.52544592524342804, 4.483927247898546575, 111.0405762719810525 ) ) ;
#64409=CARTESIAN_POINT ( 'NONE',  ( -15.72974639402176322, -15.80617190586768395, 84.37609039468570415 ) ) ;
#64410=CARTESIAN_POINT ( 'NONE',  ( 5.153800228976335163, 19.02544592524342804, 79.79057627198102409 ) ) ;
#64411=CARTESIAN_POINT ( 'NONE',  ( -18.62759615963255300, -10.81492255796106328, 44.16775706135234714 ) ) ;
#64412=CARTESIAN_POINT ( 'NONE',  ( -18.62759615963255300, -10.81492255796106328, 29.16775706135234003 ) ) ;
#64414=CARTESIAN_POINT ( 'NONE',  ( -13.97604488694527625, -13.89961937509977652, 86.87390960531436690 ) ) ;
#64416=CARTESIAN_POINT ( 'NONE',  ( -12.14591786802326823, 12.06949235617739902, 43.12609039468568284 ) ) ;
#64417=CARTESIAN_POINT ( 'NONE',  ( 15.72974639402199770, -15.80617190586745480, 38.12390960531436690 ) ) ;
#64418=CARTESIAN_POINT ( 'NONE',  ( 5.823673210054444382, -21.52544592524334988, 80.20942372801901854 ) ) ;
#64420=CARTESIAN_POINT ( 'NONE',  ( -14.29746914071037622, -8.314922557961029526, 19.16775706135234714 ) ) ;
#64421=CARTESIAN_POINT ( 'NONE',  ( -9.474510206698964154, 16.51473224551069663, 65.41557627198102409 ) ) ;
#64422=CARTESIAN_POINT ( 'NONE',  ( -19.02544592524342804, 5.153800228976336051, 91.04057627198100988 ) ) ;
#64423=CARTESIAN_POINT ( 'NONE',  ( -0.05219959533910754901, -16.53943276465976808, 107.4989096053143669 ) ) ;
#64424=CARTESIAN_POINT ( 'NONE',  ( 8.224510206698953496, -14.34966873604960469, 107.9155762719810241 ) ) ;
#64425=CARTESIAN_POINT ( 'NONE',  ( -5.049401038298153566, 19.05341960407611168, 105.2072429386476671 ) ) ;
#64426=CARTESIAN_POINT ( 'NONE',  ( 8.314922557961029526, -14.29746914071037800, 85.41775706135236135 ) ) ;
#64427=CARTESIAN_POINT ( 'NONE',  ( 16.52544592524342804, -4.483927247898539470, 53.54057627198103120 ) ) ;
#64428=CARTESIAN_POINT ( 'NONE',  ( 13.97604488694527802, 13.89961937509977652, 59.37390960531434558 ) ) ;
#64429=CARTESIAN_POINT ( 'NONE',  ( 15.72974639402176855, 15.80617190586768217, 76.87609039468567573 ) ) ;
#64430=CARTESIAN_POINT ( 'NONE',  ( 18.62759615963255655, 10.81492255796105972, 76.66775706135234714 ) ) ;
#64431=CARTESIAN_POINT ( 'NONE',  ( -0.05219959533936034679, 19.03943276465977164, 107.5010903946856615 ) ) ;
#64432=CARTESIAN_POINT ( 'NONE',  ( 16.53943276465976808, -0.05219959533910856209, 68.74890960531435269 ) ) ;
#64433=CARTESIAN_POINT ( 'NONE',  ( 15.80617190586769283, -15.72974639402175789, 20.62609039468568639 ) ) ;
#64434=CARTESIAN_POINT ( 'NONE',  ( 15.80617190586746368, 15.72974639402197994, 64.37390960531435269 ) ) ;
#64435=CARTESIAN_POINT ( 'NONE',  ( -16.88567814943161949, -6.947325034625708717, 106.2900112265259196 ) ) ;
#64437=CARTESIAN_POINT ( 'NONE',  ( 16.51473224551069308, 9.474510206698969483, 64.16557627198102409 ) ) ;
#64438=CARTESIAN_POINT ( 'NONE',  ( -4.483927247898539470, -16.52544592524342804, 37.29057627198102409 ) ) ;
#64439=CARTESIAN_POINT ( 'NONE',  ( -0.05219959533910754901, -16.53943276465976808, 22.49890960531436335 ) ) ;
#64440=CARTESIAN_POINT ( 'NONE',  ( -4.379528057220086978, -16.55341960407618274, 99.79275706135234714 ) ) ;
#64441=CARTESIAN_POINT ( 'NONE',  ( 5.049401038297881783, 19.05341960407617563, 57.29275706135231871 ) ) ;
#64443=CARTESIAN_POINT ( 'NONE',  ( -19.05341960407611168, -5.049401038298163336, 86.45724293864769550 ) ) ;
#64444=EDGE_CURVE ( 'NONE', #179366, #125647, #32586, .T. ) ;
#64445=CARTESIAN_POINT ( 'NONE',  ( -4.379528057220328563, 16.55341960407611168, 60.20724293864768839 ) ) ;
#64446=CARTESIAN_POINT ( 'NONE',  ( 16.62475595723698873, -7.163666690055304542, 103.0271335181047334 ) ) ;
#64447=CARTESIAN_POINT ( 'NONE',  ( -16.51473224551069308, -9.474510206698971260, 111.6655762719810383 ) ) ;
#64448=CARTESIAN_POINT ( 'NONE',  ( 21.53943276465977519, -0.05219959533907433946, 48.74890960531435979 ) ) ;
#64450=CARTESIAN_POINT ( 'NONE',  ( 16.55341960407611168, 4.379528057220329451, 103.9572429386476813 ) ) ;
#64451=CARTESIAN_POINT ( 'NONE',  ( 0.05219959533934541429, -16.53943276465976808, 55.00109039468568284 ) ) ;
#64452=CARTESIAN_POINT ( 'NONE',  ( 4.379528057220339221, -16.55341960407611168, 82.70724293864770971 ) ) ;
#64454=CARTESIAN_POINT ( 'NONE',  ( -16.51473224551082808, 9.474510206698731452, 78.33442372801900433 ) ) ;
#64455=CARTESIAN_POINT ( 'NONE',  ( 5.153800228976335163, 19.02544592524342804, 114.7905762719810241 ) ) ;
#64457=EDGE_CURVE ( 'NONE', #179909, #38745, #172381, .T. ) ;
#64460=CARTESIAN_POINT ( 'NONE',  ( -0.05219959533934338120, 16.53943276465976808, 42.50109039468567573 ) ) ;
#64461=CARTESIAN_POINT ( 'NONE',  ( -12.14591786802309592, -12.06949235617757132, 26.87390960531435979 ) ) ;
#64462=B_SPLINE_CURVE_WITH_KNOTS ( 'NONE', 3,
 ( #122734, #30742, #92390, #165295, #64054, #170241, #82170, #31735, #125724, #93383, #81185, #155069, #16564, #78211, #95374, #111544, #142867, #173229, #4346, #50875, #126697, #19540 ),
 .UNSPECIFIED., .F., .F.,
 ( 4, 2, 2, 2, 2, 2, 2, 2, 2, 2, 4 ),
 ( 1.179739509965479003E-17, 0.001309639967555226289, 0.001964459951332832386, 0.002291869943221635109, 0.002455574939166032568, 0.002619279935110430460, 0.002782984931054828352, 0.002946689926999226244, 0.003274099918888021595, 0.003928919902665609261, 0.005238559870220781123 ),
 .UNSPECIFIED. ) ;
#64463=CARTESIAN_POINT ( 'NONE',  ( 21.52544592524344225, -5.823673210054117533, 53.54057627198103120 ) ) ;
#64464=CARTESIAN_POINT ( 'NONE',  ( -13.89961937509957401, -13.97604488694547875, 79.37609039468567573 ) ) ;
#64465=CARTESIAN_POINT ( 'NONE',  ( 10.72451020669898902, -18.67979575497178502, 52.91557627198103830 ) ) ;
#64466=CARTESIAN_POINT ( 'NONE',  ( -18.67979575497193778, 10.72451020669871902, 78.33442372801901854 ) ) ;
#64468=CARTESIAN_POINT ( 'NONE',  ( -14.34966873604972548, 8.224510206698743886, 38.33442372801900433 ) ) ;
#64469=CARTESIAN_POINT ( 'NONE',  ( -16.46253265017160317, 9.564922557960807481, 35.83224293864768839 ) ) ;
#64470=CARTESIAN_POINT ( 'NONE',  ( 13.89961937509977652, -13.97604488694527269, 88.12390960531438111 ) ) ;
#64471=CARTESIAN_POINT ( 'NONE',  ( 9.474510206698971260, -16.51473224551069308, 37.91557627198102409 ) ) ;
#64472=CARTESIAN_POINT ( 'NONE',  ( -4.483927247898539470, -16.52544592524342804, 107.2905762719810525 ) ) ;
#64473=CARTESIAN_POINT ( 'NONE',  ( -5.153800228976328057, -19.02544592524343514, 107.2905762719810383 ) ) ;
#64475=CARTESIAN_POINT ( 'NONE',  ( 8.224510206698742110, 14.34966873604972548, 52.08442372801901854 ) ) ;
#64476=CARTESIAN_POINT ( 'NONE',  ( 0.05219959533907565091, 21.53943276465977519, 89.99890960531438111 ) ) ;
#64477=CARTESIAN_POINT ( 'NONE',  ( -13.89961937509977652, 13.97604488694528158, 40.62390960531435979 ) ) ;
#64478=CARTESIAN_POINT ( 'NONE',  ( -18.67979575497193778, 10.72451020669871902, 33.33442372801900433 ) ) ;
#64479=CARTESIAN_POINT ( 'NONE',  ( 5.049401038298161559, -19.05341960407611168, 77.70724293864765286 ) ) ;
#64482=CARTESIAN_POINT ( 'NONE',  ( -4.483927247898782831, 16.52544592524335698, 32.70942372801900433 ) ) ;
#64483=CARTESIAN_POINT ( 'NONE',  ( 21.52544592524344225, -5.823673210054117533, 113.5405762719810383 ) ) ;
#64484=CARTESIAN_POINT ( 'NONE',  ( 14.29746914071049879, -8.314922557960816363, 113.3322429386476955 ) ) ;
#64485=CARTESIAN_POINT ( 'NONE',  ( -19.03943276465977164, 0.05219959533909376836, 96.24890960531436690 ) ) ;
#64486=CARTESIAN_POINT ( 'NONE',  ( 19.03943276465977164, 0.05219959533936151252, 81.25109039468567573 ) ) ;
#64487=CARTESIAN_POINT ( 'NONE',  ( 16.46253265017146816, 9.564922557961045513, 31.66775706135232937 ) ) ;
#64488=CARTESIAN_POINT ( 'NONE',  ( -21.55341960407610458, -5.719274019375992779, 81.45724293864769550 ) ) ;
#64489=CARTESIAN_POINT ( 'NONE',  ( -19.02544592524334988, -5.153800228976617603, 28.95942372801900433 ) ) ;
#64490=CARTESIAN_POINT ( 'NONE',  ( 4.379528057220092307, 16.55341960407617563, 77.29275706135234714 ) ) ;
#64491=CARTESIAN_POINT ( 'NONE',  ( 0.05219959533909260263, 19.03943276465977164, 99.99890960531436690 ) ) ;
#64492=CARTESIAN_POINT ( 'NONE',  ( -5.153800228976328057, -19.02544592524343514, 57.29057627198103120 ) ) ;
#64494=CARTESIAN_POINT ( 'NONE',  ( 21.53943276465977519, 0.05219959533937863772, 46.25109039468567573 ) ) ;
#64495=CARTESIAN_POINT ( 'NONE',  ( 5.823673210054444382, -21.52544592524334988, 65.20942372801901854 ) ) ;
#64496=CARTESIAN_POINT ( 'NONE',  ( 5.153800228976335163, 19.02544592524342804, 79.79057627198102409 ) ) ;
#64497=CARTESIAN_POINT ( 'NONE',  ( -18.67979575497193778, 10.72451020669871902, 48.33442372801902565 ) ) ;
#64498=CARTESIAN_POINT ( 'NONE',  ( -19.03943276465977164, -0.05219959533935918106, 93.75109039468566152 ) ) ;
#64499=CARTESIAN_POINT ( 'NONE',  ( 19.03943276465977164, -0.05219959533909143690, 48.74890960531435979 ) ) ;
#64500=CARTESIAN_POINT ( 'NONE',  ( 16.46253265017160672, -9.564922557960803928, 98.33224293864769550 ) ) ;
#64501=CARTESIAN_POINT ( 'NONE',  ( -9.474510206698964154, 16.51473224551069663, 60.41557627198102409 ) ) ;
#64502=CARTESIAN_POINT ( 'NONE',  ( 13.97604488694527802, 13.89961937509977652, 114.3739096053143669 ) ) ;
#64503=CARTESIAN_POINT ( 'NONE',  ( -19.05341960407611168, -5.049401038298163336, 51.45724293864770260 ) ) ;
#64504=CARTESIAN_POINT ( 'NONE',  ( 21.52544592524344225, -5.823673210054117533, 83.54057627198102409 ) ) ;
#64505=CARTESIAN_POINT ( 'NONE',  ( -16.53943276465976808, -0.05219959533934237506, 73.75109039468567573 ) ) ;
#64507=CARTESIAN_POINT ( 'NONE',  ( 13.97604488694548053, -13.89961937509957401, 35.62609039468567573 ) ) ;
#64508=CARTESIAN_POINT ( 'NONE',  ( -5.153800228976328057, -19.02544592524343514, 62.29057627198100988 ) ) ;
#64509=CARTESIAN_POINT ( 'NONE',  ( -8.224510206698948167, 14.34966873604960824, 55.41557627198102409 ) ) ;
#64510=CARTESIAN_POINT ( 'NONE',  ( -14.29746914071049879, 8.314922557960819915, 95.83224293864770971 ) ) ;
#64511=CARTESIAN_POINT ( 'NONE',  ( 16.46253265017160672, -9.564922557960803928, 103.3322429386476955 ) ) ;
#64512=CARTESIAN_POINT ( 'NONE',  ( -9.474510206698964154, 16.51473224551069663, 90.41557627198103830 ) ) ;
#64513=CARTESIAN_POINT ( 'NONE',  ( -5.719274019375665041, -21.55341960407619695, 44.79275706135234714 ) ) ;
#64514=CARTESIAN_POINT ( 'NONE',  ( -13.97604488694527625, -13.89961937509977652, 101.8739096053143811 ) ) ;
#64515=CARTESIAN_POINT ( 'NONE',  ( 21.52544592524334988, 5.823673210054432836, 111.4594237280190328 ) ) ;
#64516=CARTESIAN_POINT ( 'NONE',  ( -12.06949235617739369, -12.14591786802326823, 74.37609039468568994 ) ) ;
#64517=CARTESIAN_POINT ( 'NONE',  ( 10.81492255796106328, -18.62759615963255655, 40.41775706135234714 ) ) ;
#64518=CARTESIAN_POINT ( 'NONE',  ( -21.53943276465977519, 0.05219959533907696930, 26.24890960531435624 ) ) ;
#64519=CARTESIAN_POINT ( 'NONE',  ( 5.719274019375991003, -21.55341960407610458, 102.7072429386476955 ) ) ;
#64520=CARTESIAN_POINT ( 'NONE',  ( 16.55341960407611168, 4.379528057220329451, 58.95724293864770971 ) ) ;
#64521=CARTESIAN_POINT ( 'NONE',  ( -5.049401038298153566, 19.05341960407611168, 55.20724293864769550 ) ) ;
#64522=CARTESIAN_POINT ( 'NONE',  ( -16.53943276465976808, 0.05219959533911058130, 76.24890960531435269 ) ) ;
#64523=CARTESIAN_POINT ( 'NONE',  ( 0.05219959533907565091, 21.53943276465977519, 44.99890960531435979 ) ) ;
#64524=CARTESIAN_POINT ( 'NONE',  ( -9.474510206698720793, -16.51473224551083518, 49.58442372801899722 ) ) ;
#64525=CARTESIAN_POINT ( 'NONE',  ( 12.14591786802309770, 12.06949235617756955, 114.3739096053143527 ) ) ;
#64527=CARTESIAN_POINT ( 'NONE',  ( -14.34966873604972548, 8.224510206698743886, 63.33442372801900433 ) ) ;
#64528=CARTESIAN_POINT ( 'NONE',  ( -0.05219959533909027116, -19.03943276465977164, 72.49890960531435269 ) ) ;
#64530=CARTESIAN_POINT ( 'NONE',  ( 16.55341960407611168, 4.379528057220329451, 88.95724293864769550 ) ) ;
#64531=CARTESIAN_POINT ( 'NONE',  ( -5.823673210054116645, -21.52544592524344225, 42.29057627198103120 ) ) ;
#64532=ORIENTED_EDGE ( 'NONE', *, *, #89272, .T. ) ;
#64533=CARTESIAN_POINT ( 'NONE',  ( 0.05219959533934541429, -16.53943276465976808, 110.0010903946856757 ) ) ;
#64534=CARTESIAN_POINT ( 'NONE',  ( -5.049401038297874678, -19.05341960407617918, 104.7927570613523471 ) ) ;
#64535=CARTESIAN_POINT ( 'NONE',  ( -21.52544592524334988, -5.823673210054445271, 83.95942372801900433 ) ) ;
#64536=CARTESIAN_POINT ( 'NONE',  ( 13.89961937509977652, -13.97604488694527269, 88.12390960531438111 ) ) ;
#64537=CARTESIAN_POINT ( 'NONE',  ( 0.05219959533907565091, 21.53943276465977519, 99.99890960531436690 ) ) ;
#64538=CARTESIAN_POINT ( 'NONE',  ( 4.483927247898790824, -16.52544592524335698, 60.20942372801902565 ) ) ;
#64539=CARTESIAN_POINT ( 'NONE',  ( 16.51473224551069308, 9.474510206698969483, 34.16557627198102409 ) ) ;
#64540=CARTESIAN_POINT ( 'NONE',  ( 16.52544592524335698, 4.483927247898782831, 26.45942372801901854 ) ) ;
#64541=CARTESIAN_POINT ( 'NONE',  ( 19.05341960407617918, -5.049401038297876454, 96.04275706135231871 ) ) ;
#64542=EDGE_CURVE ( 'NONE', #105512, #115616, #59090, .T. ) ;
#64543=CARTESIAN_POINT ( 'NONE',  ( 21.52544592524344225, -5.823673210054117533, 88.54057627198103830 ) ) ;
#64544=CARTESIAN_POINT ( 'NONE',  ( 19.05341960407617918, -5.049401038297876454, 61.04275706135232582 ) ) ;
#64546=CARTESIAN_POINT ( 'NONE',  ( -15.80617190586745835, -15.72974639402198527, 106.8739096053143811 ) ) ;
#64547=DIRECTION ( 'NONE',  ( -1.000000000000000000, 0.000000000000000000, -0.000000000000000000 ) ) ;
#64548=CARTESIAN_POINT ( 'NONE',  ( 16.46253265017160672, -9.564922557960803928, 78.33224293864769550 ) ) ;
#64549=CARTESIAN_POINT ( 'NONE',  ( -14.29746914071037622, -8.314922557961029526, 39.16775706135235424 ) ) ;
#64550=CARTESIAN_POINT ( 'NONE',  ( -17.97161686094259991, 5.499999999999981348, 100.9963720685924500 ) ) ;
#64551=B_SPLINE_CURVE_WITH_KNOTS ( 'NONE', 3,
 ( #89267, #104441, #195473, #197455, #180314, #118623, #149950, #55936, #117613, #102444, #150958, #25629, #151933, #13422, #24622, #56949, #164131, #41782, #12452, #103449 ),
 .UNSPECIFIED., .F., .F.,
 ( 4, 2, 2, 2, 2, 2, 2, 2, 2, 4 ),
 ( 3.469446951953614189E-18, 0.0004987090165372656553, 0.0009974180330745278412, 0.001246772541343162729, 0.001496127049611797400, 0.001994836066149071295, 0.002493545082686344973, 0.002742899590954982030, 0.002992254099223618218, 0.003989672132298151264 ),
 .UNSPECIFIED. ) ;
#64552=CARTESIAN_POINT ( 'NONE',  ( -19.03943276465977164, -0.05219959533935918106, 63.75109039468566863 ) ) ;
#64553=CARTESIAN_POINT ( 'NONE',  ( 18.67979575497178502, 10.72451020669898547, 114.1655762719810383 ) ) ;
#64554=CARTESIAN_POINT ( 'NONE',  ( -16.52544592524342804, 4.483927247898546575, 71.04057627198103830 ) ) ;
#64555=CARTESIAN_POINT ( 'NONE',  ( -13.89961937509977652, 13.97604488694528158, 70.62390960531432427 ) ) ;
#64556=CARTESIAN_POINT ( 'NONE',  ( -4.379528057220086978, -16.55341960407618274, 39.79275706135235424 ) ) ;
#64557=CARTESIAN_POINT ( 'NONE',  ( -19.03943276465977164, -0.05219959533935918106, 43.75109039468566863 ) ) ;
#64558=CARTESIAN_POINT ( 'NONE',  ( 15.80617190586769283, -15.72974639402175789, 55.62609039468568284 ) ) ;
#64559=CARTESIAN_POINT ( 'NONE',  ( -9.474510206698720793, -16.51473224551083518, 109.5844237280190043 ) ) ;
#64560=CARTESIAN_POINT ( 'NONE',  ( -16.46253265017160317, 9.564922557960807481, 50.83224293864770260 ) ) ;
#64561=CARTESIAN_POINT ( 'NONE',  ( 13.97604488694548053, -13.89961937509957401, 75.62609039468564731 ) ) ;
#64562=CARTESIAN_POINT ( 'NONE',  ( 10.72451020669871369, 18.67979575497193778, 97.08442372801904696 ) ) ;
#64563=CARTESIAN_POINT ( 'NONE',  ( -5.049401038297874678, -19.05341960407617918, 64.79275706135233293 ) ) ;
#64564=CARTESIAN_POINT ( 'NONE',  ( 5.153800228976335163, 19.02544592524342804, 34.79057627198102409 ) ) ;
#64565=CARTESIAN_POINT ( 'NONE',  ( -21.52544592524343514, 5.823673210054127303, 66.04057627198103830 ) ) ;
#64566=CARTESIAN_POINT ( 'NONE',  ( 0.05219959533910956823, 16.53943276465976808, 64.99890960531435269 ) ) ;
#64567=CARTESIAN_POINT ( 'NONE',  ( 16.46253265017146816, 9.564922557961045513, 66.66775706135233293 ) ) ;
#64569=CARTESIAN_POINT ( 'NONE',  ( -9.474510206698720793, -16.51473224551083518, 24.58442372801900078 ) ) ;
#64570=CARTESIAN_POINT ( 'NONE',  ( 8.314922557961029526, -14.29746914071037800, 95.41775706135234714 ) ) ;
#64571=CARTESIAN_POINT ( 'NONE',  ( -12.06949235617756955, 12.14591786802309770, 55.62390960531436690 ) ) ;
#64572=CARTESIAN_POINT ( 'NONE',  ( -21.55341960407619339, 5.719274019375674811, 83.54275706135234714 ) ) ;
#64574=CARTESIAN_POINT ( 'NONE',  ( -15.80617190586745835, -15.72974639402198527, 96.87390960531436690 ) ) ;
#64575=CARTESIAN_POINT ( 'NONE',  ( 16.46253265017160672, -9.564922557960803928, 53.33224293864768839 ) ) ;
#64576=CARTESIAN_POINT ( 'NONE',  ( -10.81492255796105439, 18.62759615963255655, 72.91775706135234714 ) ) ;
#64577=CARTESIAN_POINT ( 'NONE',  ( -19.05341960407611168, -5.049401038298163336, 51.45724293864770260 ) ) ;
#64578=CARTESIAN_POINT ( 'NONE',  ( -13.89961937509977652, 13.97604488694528158, 65.62390960531436690 ) ) ;
#64579=CARTESIAN_POINT ( 'NONE',  ( 4.379528057220339221, -16.55341960407611168, 112.7072429386476955 ) ) ;
#64580=CARTESIAN_POINT ( 'NONE',  ( -19.02544592524342804, 5.153800228976336051, 111.0405762719810099 ) ) ;
#64581=CARTESIAN_POINT ( 'NONE',  ( 16.53943276465976808, -0.05219959533910856209, 58.74890960531436690 ) ) ;
#64582=CARTESIAN_POINT ( 'NONE',  ( -0.05219959533909027116, -19.03943276465977164, 32.49890960531435979 ) ) ;
#64583=CARTESIAN_POINT ( 'NONE',  ( -16.52544592524342804, 4.483927247898546575, 86.04057627198102409 ) ) ;
#64584=CARTESIAN_POINT ( 'NONE',  ( -15.72974639402197994, 15.80617190586746368, 95.62390960531436690 ) ) ;
#64585=CARTESIAN_POINT ( 'NONE',  ( -15.80617190586768217, 15.72974639402176855, 38.12609039468567573 ) ) ;
#64587=CARTESIAN_POINT ( 'NONE',  ( -14.34966873604972548, 8.224510206698743886, 48.33442372801902565 ) ) ;
#64588=CARTESIAN_POINT ( 'NONE',  ( -15.80617190586745835, -15.72974639402198527, 86.87390960531438111 ) ) ;
#64590=CARTESIAN_POINT ( 'NONE',  ( -10.81492255796105439, 18.62759615963255655, 102.9177570613523756 ) ) ;
#64591=CARTESIAN_POINT ( 'NONE',  ( -13.89961937509977652, 13.97604488694528158, 95.62390960531436690 ) ) ;
#64592=CARTESIAN_POINT ( 'NONE',  ( -15.72974639402176322, -15.80617190586768395, 49.37609039468569705 ) ) ;
#64593=CARTESIAN_POINT ( 'NONE',  ( 0.05219959533907565091, 21.53943276465977519, 34.99890960531435979 ) ) ;
#64594=CARTESIAN_POINT ( 'NONE',  ( 12.06949235617739724, 12.14591786802326823, 101.8760903946857042 ) ) ;
#64595=CARTESIAN_POINT ( 'NONE',  ( 10.81492255796106328, -18.62759615963255655, 55.41775706135234714 ) ) ;
#64596=CARTESIAN_POINT ( 'NONE',  ( 18.67979575497194134, -10.72451020669871369, 80.83442372801901854 ) ) ;
#64597=CARTESIAN_POINT ( 'NONE',  ( -13.89961937509957401, -13.97604488694547875, 34.37609039468566863 ) ) ;
#64598=CARTESIAN_POINT ( 'NONE',  ( -16.55341960407617563, 4.379528057220093196, 93.54275706135234714 ) ) ;
#64599=CARTESIAN_POINT ( 'NONE',  ( 10.72451020669871369, 18.67979575497193778, 42.08442372801901854 ) ) ;
#64600=CARTESIAN_POINT ( 'NONE',  ( 9.474510206698971260, -16.51473224551069308, 42.91557627198103120 ) ) ;
#64601=CARTESIAN_POINT ( 'NONE',  ( 18.62759615963255655, 10.81492255796105972, 106.6677570613523756 ) ) ;
#64602=CARTESIAN_POINT ( 'NONE',  ( -5.823673210054116645, -21.52544592524344225, 27.29057627198103120 ) ) ;
#64603=CARTESIAN_POINT ( 'NONE',  ( -21.53943276465977519, -0.05219959533937600094, 18.75109039468568639 ) ) ;
#64605=CARTESIAN_POINT ( 'NONE',  ( -21.53943276465977519, 0.05219959533907696930, 76.24890960531435269 ) ) ;
#64606=CARTESIAN_POINT ( 'NONE',  ( -17.49999999999999645, -5.500000000000020428, 61.28230962303567964 ) ) ;
#64607=CARTESIAN_POINT ( 'NONE',  ( 10.81492255796078972, 18.62759615963270932, 69.58224293864769550 ) ) ;
#64608=CARTESIAN_POINT ( 'NONE',  ( 14.34966873604972726, -8.224510206698740333, 50.83442372801901143 ) ) ;
#64609=CARTESIAN_POINT ( 'NONE',  ( 8.224510206698953496, -14.34966873604960469, 57.91557627198103120 ) ) ;
#64611=CARTESIAN_POINT ( 'NONE',  ( 0.05219959533936267826, -19.03943276465977164, 85.00109039468567573 ) ) ;
#64614=CARTESIAN_POINT ( 'NONE',  ( -4.483927247898782831, 16.52544592524335698, 22.70942372801901499 ) ) ;
#64615=CARTESIAN_POINT ( 'NONE',  ( -10.72451020669898014, 18.67979575497178502, 95.41557627198102409 ) ) ;
#64616=CARTESIAN_POINT ( 'NONE',  ( -15.72974639402197994, 15.80617190586746368, 75.62390960531439532 ) ) ;
#64617=CARTESIAN_POINT ( 'NONE',  ( 16.51473224551069308, 9.474510206698969483, 109.1655762719810383 ) ) ;
#64618=CARTESIAN_POINT ( 'NONE',  ( -16.53943276465976808, -0.05219959533934237506, 63.75109039468568284 ) ) ;
#64619=CARTESIAN_POINT ( 'NONE',  ( -0.05219959533909027116, -19.03943276465977164, 77.49890960531435269 ) ) ;
#64620=CARTESIAN_POINT ( 'NONE',  ( -15.80617190586768217, 15.72974639402176855, 38.12609039468567573 ) ) ;
#64621=CARTESIAN_POINT ( 'NONE',  ( 16.51473224551083163, -9.474510206698727899, 110.8344237280190043 ) ) ;
#64622=CARTESIAN_POINT ( 'NONE',  ( 5.049401038298161559, -19.05341960407611168, 102.7072429386476955 ) ) ;
#64623=CARTESIAN_POINT ( 'NONE',  ( 9.564922557960805705, 16.46253265017160317, 104.5822429386476955 ) ) ;
#64624=CARTESIAN_POINT ( 'NONE',  ( -21.55341960407610458, -5.719274019375992779, 101.4572429386476955 ) ) ;
#64625=CARTESIAN_POINT ( 'NONE',  ( 13.89961937509977652, -13.97604488694527269, 63.12390960531435979 ) ) ;
#64626=CARTESIAN_POINT ( 'NONE',  ( -17.49999999999999645, 5.499999999999997335, 25.79690382534172244 ) ) ;
#64627=CARTESIAN_POINT ( 'NONE',  ( -4.483927247898539470, -16.52544592524342804, 87.29057627198103830 ) ) ;
#64628=CARTESIAN_POINT ( 'NONE',  ( 15.72974639402199770, -15.80617190586745480, 28.12390960531435979 ) ) ;
#64629=CARTESIAN_POINT ( 'NONE',  ( -5.153800228976328057, -19.02544592524343514, 22.29057627198102765 ) ) ;
#64630=CARTESIAN_POINT ( 'NONE',  ( 15.72974639402199770, -15.80617190586745480, 103.1239096053143811 ) ) ;
#64631=CARTESIAN_POINT ( 'NONE',  ( 0.05219959533936267826, -19.03943276465977164, 60.00109039468566863 ) ) ;
#64632=CARTESIAN_POINT ( 'NONE',  ( 19.03943276465977164, -0.05219959533909143690, 113.7489096053143669 ) ) ;
#64633=CARTESIAN_POINT ( 'NONE',  ( 5.153800228976335163, 19.02544592524342804, 24.79057627198102765 ) ) ;
#64634=CARTESIAN_POINT ( 'NONE',  ( -15.80617190586745835, -15.72974639402198527, 61.87390960531436690 ) ) ;
#64635=CARTESIAN_POINT ( 'NONE',  ( -19.02544592524342804, 5.153800228976336051, 96.04057627198103830 ) ) ;
#64636=CARTESIAN_POINT ( 'NONE',  ( -15.72974639402176322, -15.80617190586768395, 84.37609039468570415 ) ) ;
#64637=CARTESIAN_POINT ( 'NONE',  ( -19.05341960407611168, -5.049401038298163336, 46.45724293864768129 ) ) ;
#64639=CARTESIAN_POINT ( 'NONE',  ( 16.55341960407611168, 4.379528057220329451, 83.95724293864770971 ) ) ;
#64640=CARTESIAN_POINT ( 'NONE',  ( -14.29746914071037622, -8.314922557961029526, 39.16775706135235424 ) ) ;
#64641=CARTESIAN_POINT ( 'NONE',  ( 15.80617190586769283, -15.72974639402175789, 70.62609039468567573 ) ) ;
#64643=CARTESIAN_POINT ( 'NONE',  ( -13.97604488694547697, 13.89961937509957934, 23.12609039468565442 ) ) ;
#64644=CARTESIAN_POINT ( 'NONE',  ( 19.03943276465977164, 0.05219959533936151252, 86.25109039468567573 ) ) ;
#64645=CARTESIAN_POINT ( 'NONE',  ( 13.89961937509957401, 13.97604488694547697, 36.87609039468565442 ) ) ;
#64647=CARTESIAN_POINT ( 'NONE',  ( 5.719274019375673035, 21.55341960407619339, 42.29275706135235424 ) ) ;
#64648=CARTESIAN_POINT ( 'NONE',  ( -19.39720447994796970, -5.499999999999981348, 44.66317477297180005 ) ) ;
#64649=CARTESIAN_POINT ( 'NONE',  ( -16.46253265017146816, -9.564922557961047289, 34.16775706135233293 ) ) ;
#64650=CARTESIAN_POINT ( 'NONE',  ( 19.02544592524343514, -5.153800228976328945, 73.54057627198103830 ) ) ;
#64651=CARTESIAN_POINT ( 'NONE',  ( -0.05219959533910754901, -16.53943276465976808, 22.49890960531436335 ) ) ;
#64652=CARTESIAN_POINT ( 'NONE',  ( 13.89961937509977652, -13.97604488694527269, 113.1239096053143527 ) ) ;
#64653=CARTESIAN_POINT ( 'NONE',  ( -21.55341960407619339, 5.719274019375674811, 88.54275706135236135 ) ) ;
#64656=CARTESIAN_POINT ( 'NONE',  ( 21.55341960407619695, -5.719274019375665929, 91.04275706135236135 ) ) ;
#64657=CARTESIAN_POINT ( 'NONE',  ( 16.62475595723696742, -7.163666690055224606, 43.02713351810466946 ) ) ;
#64658=CARTESIAN_POINT ( 'NONE',  ( 0.05219959533909260263, 19.03943276465977164, 104.9989096053143669 ) ) ;
#64660=CARTESIAN_POINT ( 'NONE',  ( -19.05341960407611168, -5.049401038298163336, 56.45724293864768129 ) ) ;
#64661=CARTESIAN_POINT ( 'NONE',  ( -15.72974639402197994, 15.80617190586746368, 50.62390960531435979 ) ) ;
#64662=CARTESIAN_POINT ( 'NONE',  ( -16.53943276465976808, 0.05219959533911058130, 26.24890960531435624 ) ) ;
#64663=CARTESIAN_POINT ( 'NONE',  ( 14.34966873604960469, 8.224510206698951720, 109.1655762719810383 ) ) ;
#64664=CARTESIAN_POINT ( 'NONE',  ( 13.89961937509977652, -13.97604488694527269, 88.12390960531438111 ) ) ;
#64665=CARTESIAN_POINT ( 'NONE',  ( 5.153800228976615827, -19.02544592524334988, 25.20942372801900433 ) ) ;
#64666=CARTESIAN_POINT ( 'NONE',  ( -16.52544592524342804, 4.483927247898546575, 96.04057627198102409 ) ) ;
#64667=CARTESIAN_POINT ( 'NONE',  ( 15.72974639402176855, 15.80617190586768217, 56.87609039468568994 ) ) ;
#64668=CARTESIAN_POINT ( 'NONE',  ( 0.05219959533909260263, 19.03943276465977164, 114.9989096053143669 ) ) ;
#64669=CARTESIAN_POINT ( 'NONE',  ( 16.53943276465976808, 0.05219959533934440121, 101.2510903946856757 ) ) ;
#64670=CARTESIAN_POINT ( 'NONE',  ( -16.51473224551082808, 9.474510206698731452, 68.33442372801900433 ) ) ;
#64672=CARTESIAN_POINT ( 'NONE',  ( -19.03943276465977164, 0.05219959533909376836, 116.2489096053143669 ) ) ;
#64673=CARTESIAN_POINT ( 'NONE',  ( -12.06949235617756955, 12.14591786802309770, 75.62390960531439532 ) ) ;
#64674=CARTESIAN_POINT ( 'NONE',  ( 9.474510206698729675, 16.51473224551082808, 62.08442372801899722 ) ) ;
#64675=CARTESIAN_POINT ( 'NONE',  ( 5.049401038298161559, -19.05341960407611168, 57.70724293864769550 ) ) ;
#64676=CARTESIAN_POINT ( 'NONE',  ( -4.379528057220328563, 16.55341960407611168, 65.20724293864768129 ) ) ;
#64677=CARTESIAN_POINT ( 'NONE',  ( -5.153800228976607833, 19.02544592524334988, 92.70942372801901854 ) ) ;
#64678=CARTESIAN_POINT ( 'NONE',  ( 5.719274019375991003, -21.55341960407610458, 47.70724293864770260 ) ) ;
#64680=CARTESIAN_POINT ( 'NONE',  ( -14.29746914071049879, 8.314922557960819915, 100.8322429386477097 ) ) ;
#64681=CARTESIAN_POINT ( 'NONE',  ( -17.26058549869089376, -6.457015423128630971, 31.37745837476069255 ) ) ;
#64682=CARTESIAN_POINT ( 'NONE',  ( -9.474510206698964154, 16.51473224551069663, 55.41557627198103120 ) ) ;
#64683=CARTESIAN_POINT ( 'NONE',  ( -0.05219959533907301413, -21.53943276465977519, 57.49890960531435979 ) ) ;
#64684=CARTESIAN_POINT ( 'NONE',  ( 5.153800228976335163, 19.02544592524342804, 44.79057627198103830 ) ) ;
#64685=CARTESIAN_POINT ( 'NONE',  ( -16.55341960407617563, 4.379528057220093196, 93.54275706135234714 ) ) ;
#64686=CARTESIAN_POINT ( 'NONE',  ( 13.97604488694527802, 13.89961937509977652, 79.37390960531435269 ) ) ;
#64687=CARTESIAN_POINT ( 'NONE',  ( 19.02544592524334988, 5.153800228976608722, 56.45942372801898301 ) ) ;
#64688=CARTESIAN_POINT ( 'NONE',  ( 5.719274019375673035, 21.55341960407619339, 77.29275706135234714 ) ) ;
#64690=CARTESIAN_POINT ( 'NONE',  ( 10.72451020669898902, -18.67979575497178502, 57.91557627198103120 ) ) ;
#64691=CARTESIAN_POINT ( 'NONE',  ( 5.049401038298161559, -19.05341960407611168, 112.7072429386476813 ) ) ;
#64692=CARTESIAN_POINT ( 'NONE',  ( 9.474510206698971260, -16.51473224551069308, 37.91557627198102409 ) ) ;
#64693=CARTESIAN_POINT ( 'NONE',  ( 8.224510206698742110, 14.34966873604972548, 87.08442372801901854 ) ) ;
#64694=CARTESIAN_POINT ( 'NONE',  ( 16.46253265017146816, 9.564922557961045513, 106.6677570613523471 ) ) ;
#64695=CARTESIAN_POINT ( 'NONE',  ( -5.153800228976328057, -19.02544592524343514, 27.29057627198103120 ) ) ;
#64696=CARTESIAN_POINT ( 'NONE',  ( 17.26058549869089376, 6.457015423128627418, 53.87745837476069255 ) ) ;
#64697=CARTESIAN_POINT ( 'NONE',  ( -21.55341960407619339, 5.719274019375674811, 93.54275706135234714 ) ) ;
#64698=CARTESIAN_POINT ( 'NONE',  ( -14.29746914071049879, 8.314922557960819915, 60.83224293864769550 ) ) ;
#64699=CARTESIAN_POINT ( 'NONE',  ( -16.55341960407611168, -4.379528057220339221, 76.45724293864769550 ) ) ;
#64700=CARTESIAN_POINT ( 'NONE',  ( 15.72974639402199770, -15.80617190586745480, 93.12390960531436690 ) ) ;
#64701=CARTESIAN_POINT ( 'NONE',  ( 21.53943276465977519, -0.05219959533907433946, 88.74890960531436690 ) ) ;
#64703=CARTESIAN_POINT ( 'NONE',  ( -5.719274019375978568, 21.55341960407610458, 45.20724293864769550 ) ) ;
#64704=CARTESIAN_POINT ( 'NONE',  ( -0.05219959533934338120, 16.53943276465976808, 72.50109039468568994 ) ) ;
#64705=CARTESIAN_POINT ( 'NONE',  ( 14.34966873604960469, 8.224510206698951720, 89.16557627198102409 ) ) ;
#64706=CARTESIAN_POINT ( 'NONE',  ( -9.474510206698964154, 16.51473224551069663, 40.41557627198103120 ) ) ;
#64708=CARTESIAN_POINT ( 'NONE',  ( 16.53943276465976808, 0.05219959533934440121, 101.2510903946856757 ) ) ;
#64709=CARTESIAN_POINT ( 'NONE',  ( 0.05219959533937995610, -21.53943276465977519, 30.00109039468568284 ) ) ;
#64710=CARTESIAN_POINT ( 'NONE',  ( -19.02544592524342804, 5.153800228976336051, 86.04057627198103830 ) ) ;
#64711=CARTESIAN_POINT ( 'NONE',  ( 18.67979575497194134, -10.72451020669871369, 70.83442372801901854 ) ) ;
#64713=CARTESIAN_POINT ( 'NONE',  ( -0.05219959533909027116, -19.03943276465977164, 22.49890960531436690 ) ) ;
#64715=CARTESIAN_POINT ( 'NONE',  ( -5.719274019375665041, -21.55341960407619695, 54.79275706135235424 ) ) ;
#64716=CARTESIAN_POINT ( 'NONE',  ( -13.89961937509977652, 13.97604488694528158, 35.62390960531435269 ) ) ;
#64717=CARTESIAN_POINT ( 'NONE',  ( -0.05219959533909027116, -19.03943276465977164, 22.49890960531436690 ) ) ;
#64718=CARTESIAN_POINT ( 'NONE',  ( 0.05219959533909260263, 19.03943276465977164, 94.99890960531436690 ) ) ;
#64719=CARTESIAN_POINT ( 'NONE',  ( -16.51473224551082808, 9.474510206698731452, 73.33442372801900433 ) ) ;
#64720=CARTESIAN_POINT ( 'NONE',  ( -15.72974639402176322, -15.80617190586768395, 24.37609039468567573 ) ) ;
#64721=CARTESIAN_POINT ( 'NONE',  ( -19.02544592524334988, -5.153800228976617603, 53.95942372801898301 ) ) ;
#64722=CARTESIAN_POINT ( 'NONE',  ( 19.03943276465977164, -0.05219959533909143690, 33.74890960531435979 ) ) ;
#64723=CARTESIAN_POINT ( 'NONE',  ( -4.379528057220086978, -16.55341960407618274, 99.79275706135234714 ) ) ;
#64724=CARTESIAN_POINT ( 'NONE',  ( 9.474510206698729675, 16.51473224551082808, 82.08442372801899012 ) ) ;
#64725=CARTESIAN_POINT ( 'NONE',  ( -16.52544592524342804, 4.483927247898546575, 31.04057627198102409 ) ) ;
#64726=CARTESIAN_POINT ( 'NONE',  ( 19.05341960407617918, -5.049401038297876454, 56.04275706135234714 ) ) ;
#64727=CARTESIAN_POINT ( 'NONE',  ( 5.153800228976335163, 19.02544592524342804, 99.79057627198102409 ) ) ;
#64728=CARTESIAN_POINT ( 'NONE',  ( -5.719274019375665041, -21.55341960407619695, 104.7927570613523898 ) ) ;
#64730=CARTESIAN_POINT ( 'NONE',  ( -18.67979575497193778, 10.72451020669871902, 103.3344237280190043 ) ) ;
#64732=CARTESIAN_POINT ( 'NONE',  ( 18.67979575497194134, -10.72451020669871369, 85.83442372801901854 ) ) ;
#64733=CARTESIAN_POINT ( 'NONE',  ( -16.52544592524335698, -4.483927247898792601, 28.95942372801902209 ) ) ;
#64734=CARTESIAN_POINT ( 'NONE',  ( -0.05219959533909027116, -19.03943276465977164, 92.49890960531436690 ) ) ;
#64736=CARTESIAN_POINT ( 'NONE',  ( 5.049401038298161559, -19.05341960407611168, 72.70724293864768129 ) ) ;
#64737=CARTESIAN_POINT ( 'NONE',  ( 17.50000000000000000, 5.499999999999997335, 120.0000000000000142 ) ) ;
#64738=CARTESIAN_POINT ( 'NONE',  ( -5.049401038297874678, -19.05341960407617918, 64.79275706135233293 ) ) ;
#64739=CARTESIAN_POINT ( 'NONE',  ( -13.97604488694527625, -13.89961937509977652, 101.8739096053143811 ) ) ;
#64740=CARTESIAN_POINT ( 'NONE',  ( -18.62759615963255300, -10.81492255796106328, 99.16775706135234714 ) ) ;
#64741=CARTESIAN_POINT ( 'NONE',  ( -0.05219959533910754901, -16.53943276465976808, 97.49890960531436690 ) ) ;
#64742=CARTESIAN_POINT ( 'NONE',  ( 0.05219959533907565091, 21.53943276465977519, 44.99890960531435979 ) ) ;
#64743=CARTESIAN_POINT ( 'NONE',  ( -10.72451020669898014, 18.67979575497178502, 30.41557627198101699 ) ) ;
#64744=CARTESIAN_POINT ( 'NONE',  ( -16.53943276465976808, 0.05219959533911058130, 106.2489096053143811 ) ) ;
#64746=CARTESIAN_POINT ( 'NONE',  ( -19.03943276465977164, -0.05219959533935918106, 53.75109039468566863 ) ) ;
#64747=CARTESIAN_POINT ( 'NONE',  ( 8.224510206698953496, -14.34966873604960469, 32.91557627198102409 ) ) ;
#64748=CARTESIAN_POINT ( 'NONE',  ( -5.049401038298153566, 19.05341960407611168, 100.2072429386476955 ) ) ;
#64749=CARTESIAN_POINT ( 'NONE',  ( -10.72451020669870658, -18.67979575497194134, 79.58442372801903275 ) ) ;
#64750=CARTESIAN_POINT ( 'NONE',  ( 21.55341960407610458, 5.719274019375980345, 68.95724293864769550 ) ) ;
#64751=CARTESIAN_POINT ( 'NONE',  ( 0.05219959533937995610, -21.53943276465977519, 40.00109039468567573 ) ) ;
#64752=CARTESIAN_POINT ( 'NONE',  ( -21.55341960407610458, -5.719274019375992779, 101.4572429386476955 ) ) ;
#64753=CARTESIAN_POINT ( 'NONE',  ( -18.62759615963255300, -10.81492255796106328, 49.16775706135234003 ) ) ;
#64754=CARTESIAN_POINT ( 'NONE',  ( -13.97604488694527625, -13.89961937509977652, 31.87390960531435979 ) ) ;
#64755=CARTESIAN_POINT ( 'NONE',  ( -13.89961937509977652, 13.97604488694528158, 80.62390960531436690 ) ) ;
#64756=CARTESIAN_POINT ( 'NONE',  ( 16.53943276465976808, 0.05219959533934440121, 86.25109039468568994 ) ) ;
#64757=CARTESIAN_POINT ( 'NONE',  ( 12.14591786802309770, 12.06949235617756955, 104.3739096053143669 ) ) ;
#64758=CARTESIAN_POINT ( 'NONE',  ( 13.97604488694527802, 13.89961937509977652, 104.3739096053143385 ) ) ;
#64759=CARTESIAN_POINT ( 'NONE',  ( 14.29746914071049879, -8.314922557960816363, 58.33224293864768839 ) ) ;
#64760=CARTESIAN_POINT ( 'NONE',  ( -12.14591786802309592, -12.06949235617757132, 21.87390960531436690 ) ) ;
#64761=CARTESIAN_POINT ( 'NONE',  ( 19.03943276465977164, -0.05219959533909143690, 48.74890960531435979 ) ) ;
#64762=CARTESIAN_POINT ( 'NONE',  ( 16.46253265017160672, -9.564922557960803928, 28.33224293864769550 ) ) ;
#64763=CARTESIAN_POINT ( 'NONE',  ( -5.823673210054116645, -21.52544592524344225, 42.29057627198103120 ) ) ;
#64764=CARTESIAN_POINT ( 'NONE',  ( -19.03943276465977164, -0.05219959533935918106, 43.75109039468566863 ) ) ;
#64766=CARTESIAN_POINT ( 'NONE',  ( 8.314922557960818139, 14.29746914071049879, 39.58224293864769550 ) ) ;
#64767=VECTOR ( 'NONE', #16546, 1000.000000000000000 ) ;
#64768=CARTESIAN_POINT ( 'NONE',  ( 5.719274019375673035, 21.55341960407619339, 42.29275706135235424 ) ) ;
#64770=CARTESIAN_POINT ( 'NONE',  ( -14.34966873604972548, 8.224510206698743886, 53.33442372801901854 ) ) ;
#64771=CARTESIAN_POINT ( 'NONE',  ( 13.97604488694548053, -13.89961937509957401, 55.62609039468566863 ) ) ;
#64772=CARTESIAN_POINT ( 'NONE',  ( 0.05219959533910956823, 16.53943276465976808, 24.99890960531435624 ) ) ;
#64773=CARTESIAN_POINT ( 'NONE',  ( 16.20579543436676317, -7.371946100355162734, 51.93479165828130562 ) ) ;
#64774=CARTESIAN_POINT ( 'NONE',  ( 16.55341960407618274, -4.379528057220086978, 101.0427570613523756 ) ) ;
#64775=CARTESIAN_POINT ( 'NONE',  ( 19.02544592524343514, -5.153800228976328945, 33.54057627198102409 ) ) ;
#64777=CARTESIAN_POINT ( 'NONE',  ( -9.564922557960796823, -16.46253265017161027, 67.08224293864769550 ) ) ;
#64778=CARTESIAN_POINT ( 'NONE',  ( -9.564922557960796823, -16.46253265017161027, 27.08224293864769550 ) ) ;
#64779=CARTESIAN_POINT ( 'NONE',  ( -5.823673210054431948, 21.52544592524334988, 32.70942372801900433 ) ) ;
#64780=CARTESIAN_POINT ( 'NONE',  ( 9.564922557960805705, 16.46253265017160317, 49.58224293864770260 ) ) ;
#64781=CARTESIAN_POINT ( 'NONE',  ( -9.564922557960796823, -16.46253265017161027, 112.0822429386476955 ) ) ;
#64782=CARTESIAN_POINT ( 'NONE',  ( -9.564922557960796823, -16.46253265017161027, 52.08224293864768839 ) ) ;
#64783=CARTESIAN_POINT ( 'NONE',  ( 21.55341960407610458, 5.719274019375980345, 23.95724293864769550 ) ) ;
#64784=CARTESIAN_POINT ( 'NONE',  ( 10.72451020669871369, 18.67979575497193778, 57.08442372801901854 ) ) ;
#64785=CARTESIAN_POINT ( 'NONE',  ( 8.314922557960818139, 14.29746914071049879, 99.58224293864770971 ) ) ;
#64786=CARTESIAN_POINT ( 'NONE',  ( -21.52544592524343514, 5.823673210054127303, 26.04057627198103475 ) ) ;
#64787=CARTESIAN_POINT ( 'NONE',  ( -12.06949235617739369, -12.14591786802326823, 79.37609039468567573 ) ) ;
#64788=CARTESIAN_POINT ( 'NONE',  ( -18.62759615963255300, -10.81492255796106328, 94.16775706135237556 ) ) ;
#64789=CARTESIAN_POINT ( 'NONE',  ( 8.314922557961029526, -14.29746914071037800, 50.41775706135235424 ) ) ;
#64790=CARTESIAN_POINT ( 'NONE',  ( 0.05219959533909260263, 19.03943276465977164, 89.99890960531436690 ) ) ;
#64791=CARTESIAN_POINT ( 'NONE',  ( -16.55341960407617563, 4.379528057220093196, 43.54275706135235424 ) ) ;
#64792=CARTESIAN_POINT ( 'NONE',  ( -16.52544592524335698, -4.483927247898792601, 23.95942372801901143 ) ) ;
#64793=CARTESIAN_POINT ( 'NONE',  ( 14.34966873604972726, -8.224510206698740333, 100.8344237280190185 ) ) ;
#64794=CARTESIAN_POINT ( 'NONE',  ( 10.72451020669871369, 18.67979575497193778, 52.08442372801901854 ) ) ;
#64795=CARTESIAN_POINT ( 'NONE',  ( 19.05341960407617918, -5.049401038297876454, 101.0427570613523045 ) ) ;
#64796=CARTESIAN_POINT ( 'NONE',  ( -5.719274019375665041, -21.55341960407619695, 19.79275706135235069 ) ) ;
#64797=CARTESIAN_POINT ( 'NONE',  ( -16.52544592524342804, 4.483927247898546575, 101.0405762719810383 ) ) ;
#64798=CARTESIAN_POINT ( 'NONE',  ( -5.049401038297874678, -19.05341960407617918, 109.7927570613523187 ) ) ;
#64799=CARTESIAN_POINT ( 'NONE',  ( 14.29746914071037800, 8.314922557961029526, 71.66775706135234714 ) ) ;
#64801=CARTESIAN_POINT ( 'NONE',  ( 9.564922557961047289, -16.46253265017146816, 85.41775706135233293 ) ) ;
#64802=CARTESIAN_POINT ( 'NONE',  ( -16.55341960407611168, -4.379528057220339221, 46.45724293864769550 ) ) ;
#64803=CARTESIAN_POINT ( 'NONE',  ( 8.224510206698953496, -14.34966873604960469, 47.91557627198102409 ) ) ;
#64804=CARTESIAN_POINT ( 'NONE',  ( -16.53943276465976808, 0.05219959533911058130, 96.24890960531435269 ) ) ;
#64805=CARTESIAN_POINT ( 'NONE',  ( -9.474510206698720793, -16.51473224551083518, 29.58442372801900433 ) ) ;
#64806=CARTESIAN_POINT ( 'NONE',  ( -18.87075004821566537, 5.500000000000085265, 88.67408112101047379 ) ) ;
#64807=CARTESIAN_POINT ( 'NONE',  ( -21.55341960407619339, 5.719274019375674811, 38.54275706135234714 ) ) ;
#64808=CARTESIAN_POINT ( 'NONE',  ( 16.51473224551083163, -9.474510206698727899, 100.8344237280190043 ) ) ;
#64810=CARTESIAN_POINT ( 'NONE',  ( 19.03943276465977164, -0.05219959533909143690, 88.74890960531436690 ) ) ;
#64811=CARTESIAN_POINT ( 'NONE',  ( -5.153800228976328057, -19.02544592524343514, 87.29057627198103830 ) ) ;
#64812=CARTESIAN_POINT ( 'NONE',  ( -10.81492255796078084, -18.62759615963271287, 57.08224293864769550 ) ) ;
#64813=CARTESIAN_POINT ( 'NONE',  ( 14.29746914071049879, -8.314922557960816363, 98.33224293864769550 ) ) ;
#64814=CARTESIAN_POINT ( 'NONE',  ( 19.05341960407611168, 5.049401038298154454, 73.95724293864768129 ) ) ;
#64815=CARTESIAN_POINT ( 'NONE',  ( 16.46253265017160672, -9.564922557960803928, 23.33224293864769194 ) ) ;
#64816=CARTESIAN_POINT ( 'NONE',  ( -10.72451020669870658, -18.67979575497194134, 39.58442372801901143 ) ) ;
#64817=CARTESIAN_POINT ( 'NONE',  ( -15.72974639402176322, -15.80617190586768395, 69.37609039468567573 ) ) ;
#64818=CARTESIAN_POINT ( 'NONE',  ( 16.52544592524335698, 4.483927247898782831, 91.45942372801901854 ) ) ;
#64819=CARTESIAN_POINT ( 'NONE',  ( 0.05219959533937995610, -21.53943276465977519, 30.00109039468568284 ) ) ;
#64820=CARTESIAN_POINT ( 'NONE',  ( -21.55341960407619339, 5.719274019375674811, 23.54275706135235424 ) ) ;
#64821=CARTESIAN_POINT ( 'NONE',  ( 19.03943276465977164, 0.05219959533936151252, 51.25109039468567573 ) ) ;
#64822=CARTESIAN_POINT ( 'NONE',  ( 16.46253265017160672, -9.564922557960803928, 83.33224293864768129 ) ) ;
#64823=CARTESIAN_POINT ( 'NONE',  ( -15.80617190586768217, 15.72974639402176855, 83.12609039468568994 ) ) ;
#64824=CARTESIAN_POINT ( 'NONE',  ( 15.80617190586746368, 15.72974639402197994, 79.37390960531436690 ) ) ;
#64825=CARTESIAN_POINT ( 'NONE',  ( 16.55341960407611168, 4.379528057220329451, 53.95724293864770260 ) ) ;
#64826=CARTESIAN_POINT ( 'NONE',  ( 10.72451020669871369, 18.67979575497193778, 97.08442372801904696 ) ) ;
#64827=CARTESIAN_POINT ( 'NONE',  ( 13.89961937509957401, 13.97604488694547697, 31.87609039468566863 ) ) ;
#64828=CARTESIAN_POINT ( 'NONE',  ( 16.53943276465976808, -0.05219959533910856209, 73.74890960531433848 ) ) ;
#64829=CARTESIAN_POINT ( 'NONE',  ( 5.049401038298161559, -19.05341960407611168, 27.70724293864769550 ) ) ;
#64830=CARTESIAN_POINT ( 'NONE',  ( 5.049401038297881783, 19.05341960407617563, 77.29275706135231871 ) ) ;
#64831=CARTESIAN_POINT ( 'NONE',  ( -16.52544592524342804, 4.483927247898546575, 41.04057627198103120 ) ) ;
#64832=CARTESIAN_POINT ( 'NONE',  ( 21.53943276465977519, 0.05219959533937863772, 76.25109039468568994 ) ) ;
#64833=CARTESIAN_POINT ( 'NONE',  ( -5.049401038298153566, 19.05341960407611168, 80.20724293864769550 ) ) ;
#64834=CARTESIAN_POINT ( 'NONE',  ( -13.89961937509957401, -13.97604488694547875, 59.37609039468566863 ) ) ;
#64835=CARTESIAN_POINT ( 'NONE',  ( 5.823673210054125526, 21.52544592524343514, 69.79057627198102409 ) ) ;
#64836=CARTESIAN_POINT ( 'NONE',  ( -15.80617190586768217, 15.72974639402176855, 23.12609039468567573 ) ) ;
#64837=CARTESIAN_POINT ( 'NONE',  ( -19.05341960407617563, 5.049401038297882671, 108.5427570613523187 ) ) ;
#64838=CARTESIAN_POINT ( 'NONE',  ( 8.314922557961029526, -14.29746914071037800, 80.41775706135234714 ) ) ;
#64839=CARTESIAN_POINT ( 'NONE',  ( 17.48853670773241831, 5.747243402303172211, 63.83328700250011423 ) ) ;
#64840=CARTESIAN_POINT ( 'NONE',  ( -21.55341960407610458, -5.719274019375992779, 111.4572429386476813 ) ) ;
#64841=CARTESIAN_POINT ( 'NONE',  ( -16.52544592524342804, 4.483927247898546575, 101.0405762719810383 ) ) ;
#64842=CARTESIAN_POINT ( 'NONE',  ( -16.31925111598457434, -7.325300261831548809, 99.83575461032749843 ) ) ;
#64843=CARTESIAN_POINT ( 'NONE',  ( 14.29746914071037800, 8.314922557961029526, 31.66775706135234358 ) ) ;
#64844=CARTESIAN_POINT ( 'NONE',  ( -15.80617190586745835, -15.72974639402198527, 61.87390960531436690 ) ) ;
#64845=CARTESIAN_POINT ( 'NONE',  ( -14.29746914071037622, -8.314922557961029526, 99.16775706135234714 ) ) ;
#64846=CARTESIAN_POINT ( 'NONE',  ( -13.97604488694527625, -13.89961937509977652, 36.87390960531436690 ) ) ;
#64847=CARTESIAN_POINT ( 'NONE',  ( 16.55341960407618274, -4.379528057220086978, 61.04275706135234714 ) ) ;
#64848=CARTESIAN_POINT ( 'NONE',  ( 13.89961937509957401, 13.97604488694547697, 76.87609039468566152 ) ) ;
#64849=CARTESIAN_POINT ( 'NONE',  ( 15.72974639402176855, 15.80617190586768217, 46.87609039468568994 ) ) ;
#64850=CARTESIAN_POINT ( 'NONE',  ( 10.81492255796078972, 18.62759615963270932, 59.58224293864770260 ) ) ;
#64851=CARTESIAN_POINT ( 'NONE',  ( -16.55341960407617563, 4.379528057220093196, 98.54275706135234714 ) ) ;
#64852=CARTESIAN_POINT ( 'NONE',  ( -10.81492255796105439, 18.62759615963255655, 82.91775706135234714 ) ) ;
#64853=CARTESIAN_POINT ( 'NONE',  ( -18.67979575497178146, -10.72451020669898902, 51.66557627198102409 ) ) ;
#64854=CARTESIAN_POINT ( 'NONE',  ( -18.67979575497178146, -10.72451020669898902, 46.66557627198102409 ) ) ;
#64855=CARTESIAN_POINT ( 'NONE',  ( -12.14591786802326823, 12.06949235617739902, 78.12609039468570415 ) ) ;
#64856=CARTESIAN_POINT ( 'NONE',  ( -5.823673210054116645, -21.52544592524344225, 42.29057627198103120 ) ) ;
#64858=CARTESIAN_POINT ( 'NONE',  ( -5.153800228976328057, -19.02544592524343514, 102.2905762719810383 ) ) ;
#64860=CARTESIAN_POINT ( 'NONE',  ( 16.46253265017160672, -9.564922557960803928, 33.33224293864770260 ) ) ;
#64861=CARTESIAN_POINT ( 'NONE',  ( -21.53943276465977519, 0.05219959533907696930, 66.24890960531436690 ) ) ;
#64862=CARTESIAN_POINT ( 'NONE',  ( 0.05219959533934541429, -16.53943276465976808, 90.00109039468567573 ) ) ;
#64863=CARTESIAN_POINT ( 'NONE',  ( -5.719274019375665041, -21.55341960407619695, 44.79275706135234714 ) ) ;
#64864=CARTESIAN_POINT ( 'NONE',  ( 5.049401038297881783, 19.05341960407617563, 107.2927570613523187 ) ) ;
#64865=CARTESIAN_POINT ( 'NONE',  ( 0.05219959533910956823, 16.53943276465976808, 99.99890960531436690 ) ) ;
#64866=CARTESIAN_POINT ( 'NONE',  ( 19.02544592524334988, 5.153800228976608722, 111.4594237280190043 ) ) ;
#64867=CARTESIAN_POINT ( 'NONE',  ( 19.03943276465977164, -0.05219959533909143690, 38.74890960531436690 ) ) ;
#64869=CARTESIAN_POINT ( 'NONE',  ( 13.97604488694527802, 13.89961937509977652, 94.37390960531436690 ) ) ;
#64871=CARTESIAN_POINT ( 'NONE',  ( 16.55341960407618274, -4.379528057220086978, 76.04275706135237556 ) ) ;
#64872=CARTESIAN_POINT ( 'NONE',  ( -0.05219959533937732626, 21.53943276465977519, 112.5010903946857042 ) ) ;
#64873=CARTESIAN_POINT ( 'NONE',  ( 10.81492255796078972, 18.62759615963270932, 64.58224293864769550 ) ) ;
#64874=CARTESIAN_POINT ( 'NONE',  ( 16.53943276465976808, 0.05219959533934440121, 86.25109039468568994 ) ) ;
#64875=CARTESIAN_POINT ( 'NONE',  ( -9.564922557961040184, 16.46253265017147172, 82.91775706135233293 ) ) ;
#64876=CARTESIAN_POINT ( 'NONE',  ( 5.153800228976335163, 19.02544592524342804, 34.79057627198102409 ) ) ;
#64877=CARTESIAN_POINT ( 'NONE',  ( -19.03943276465977164, 0.05219959533909376836, 81.24890960531436690 ) ) ;
#64878=CARTESIAN_POINT ( 'NONE',  ( 13.97604488694527802, 13.89961937509977652, 29.37390960531435979 ) ) ;
#64879=CARTESIAN_POINT ( 'NONE',  ( -16.46253265017146816, -9.564922557961047289, 69.16775706135233293 ) ) ;
#64881=CARTESIAN_POINT ( 'NONE',  ( -19.05341960407611168, -5.049401038298163336, 111.4572429386476671 ) ) ;
#64882=CARTESIAN_POINT ( 'NONE',  ( -14.29746914071049879, 8.314922557960819915, 65.83224293864769550 ) ) ;
#64883=CARTESIAN_POINT ( 'NONE',  ( -18.62759615963270932, 10.81492255796079327, 60.83224293864769550 ) ) ;
#64885=CARTESIAN_POINT ( 'NONE',  ( 16.46253265017146816, 9.564922557961045513, 31.66775706135232937 ) ) ;
#64886=CARTESIAN_POINT ( 'NONE',  ( -18.22780087662122028, 5.500000000000031086, 88.51540105326107266 ) ) ;
#64887=CARTESIAN_POINT ( 'NONE',  ( -13.89961937509977652, 13.97604488694528158, 60.62390960531436690 ) ) ;
#64888=CARTESIAN_POINT ( 'NONE',  ( -19.03943276465977164, 0.05219959533909376836, 76.24890960531435269 ) ) ;
#64889=CARTESIAN_POINT ( 'NONE',  ( 16.53943276465976808, 0.05219959533934440121, 51.25109039468568994 ) ) ;
#64892=CARTESIAN_POINT ( 'NONE',  ( -14.34966873604972548, 8.224510206698743886, 73.33442372801901854 ) ) ;
#64893=CARTESIAN_POINT ( 'NONE',  ( -17.97182807773871005, 5.500000000000047073, 78.53038844047287625 ) ) ;
#64894=CARTESIAN_POINT ( 'NONE',  ( 16.55341960407618274, -4.379528057220086978, 61.04275706135234714 ) ) ;
#64895=CARTESIAN_POINT ( 'NONE',  ( 12.14591786802327356, -12.06949235617739191, 35.62609039468568994 ) ) ;
#64896=CARTESIAN_POINT ( 'NONE',  ( -9.564922557960796823, -16.46253265017161027, 52.08224293864768839 ) ) ;
#64898=CARTESIAN_POINT ( 'NONE',  ( 18.62759615963255655, 10.81492255796105972, 51.66775706135234714 ) ) ;
#64899=CARTESIAN_POINT ( 'NONE',  ( 9.474510206698729675, 16.51473224551082808, 62.08442372801899722 ) ) ;
#64900=CARTESIAN_POINT ( 'NONE',  ( -5.823673210054431948, 21.52544592524334988, 107.7094237280190328 ) ) ;
#64901=CARTESIAN_POINT ( 'NONE',  ( -9.564922557960796823, -16.46253265017161027, 27.08224293864769550 ) ) ;
#64903=CARTESIAN_POINT ( 'NONE',  ( 5.823673210054125526, 21.52544592524343514, 54.79057627198104541 ) ) ;
#64904=CARTESIAN_POINT ( 'NONE',  ( 5.049401038298161559, -19.05341960407611168, 107.7072429386476955 ) ) ;
#64905=CARTESIAN_POINT ( 'NONE',  ( 14.29746914071049879, -8.314922557960816363, 103.3322429386476955 ) ) ;
#64906=CARTESIAN_POINT ( 'NONE',  ( -16.53943276465976808, -0.05219959533934237506, 38.75109039468567573 ) ) ;
#64907=CARTESIAN_POINT ( 'NONE',  ( 4.483927247898545687, 16.52544592524342804, 34.79057627198103120 ) ) ;
#64909=CARTESIAN_POINT ( 'NONE',  ( -18.67979575497178146, -10.72451020669898902, 96.66557627198102409 ) ) ;
#64910=CARTESIAN_POINT ( 'NONE',  ( 4.379528057220339221, -16.55341960407611168, 42.70724293864770260 ) ) ;
#64911=CARTESIAN_POINT ( 'NONE',  ( -19.05341960407611168, -5.049401038298163336, 111.4572429386476671 ) ) ;
#64912=CARTESIAN_POINT ( 'NONE',  ( 0.05219959533936267826, -19.03943276465977164, 90.00109039468567573 ) ) ;
#64913=CARTESIAN_POINT ( 'NONE',  ( -19.05341960407617563, 5.049401038297882671, 28.54275706135232937 ) ) ;
#64914=CARTESIAN_POINT ( 'NONE',  ( 12.06949235617757843, -12.14591786802309237, 28.12390960531435979 ) ) ;
#64915=CARTESIAN_POINT ( 'NONE',  ( 5.823673210054125526, 21.52544592524343514, 109.7905762719810383 ) ) ;
#64916=CARTESIAN_POINT ( 'NONE',  ( -15.72974639402197994, 15.80617190586746368, 55.62390960531436690 ) ) ;
#64917=CARTESIAN_POINT ( 'NONE',  ( -9.564922557960796823, -16.46253265017161027, 82.08224293864768129 ) ) ;
#64918=CARTESIAN_POINT ( 'NONE',  ( 12.06949235617757843, -12.14591786802309237, 53.12390960531436690 ) ) ;
#64919=CARTESIAN_POINT ( 'NONE',  ( 19.02544592524343514, -5.153800228976328945, 88.54057627198102409 ) ) ;
#64922=CARTESIAN_POINT ( 'NONE',  ( -13.97604488694547697, 13.89961937509957934, 48.12609039468566863 ) ) ;
#64923=CARTESIAN_POINT ( 'NONE',  ( -5.719274019375978568, 21.55341960407610458, 85.20724293864770971 ) ) ;
#64924=CARTESIAN_POINT ( 'NONE',  ( 16.53943276465976808, -0.05219959533910856209, 103.7489096053143669 ) ) ;
#64925=CARTESIAN_POINT ( 'NONE',  ( 21.55341960407619695, -5.719274019375665929, 31.04275706135234714 ) ) ;
#64927=CARTESIAN_POINT ( 'NONE',  ( 14.29746914071037800, 8.314922557961029526, 106.6677570613523756 ) ) ;
#64928=CARTESIAN_POINT ( 'NONE',  ( 5.049401038298161559, -19.05341960407611168, 42.70724293864767418 ) ) ;
#64930=CARTESIAN_POINT ( 'NONE',  ( -19.02544592524342804, 5.153800228976336051, 81.04057627198103830 ) ) ;
#64932=CARTESIAN_POINT ( 'NONE',  ( 19.02544592524343514, -5.153800228976328945, 33.54057627198102409 ) ) ;
#64933=CARTESIAN_POINT ( 'NONE',  ( -12.14591786802309592, -12.06949235617757132, 36.87390960531435979 ) ) ;
#64934=CARTESIAN_POINT ( 'NONE',  ( 18.67979575497194134, -10.72451020669871369, 75.83442372801900433 ) ) ;
#64936=CARTESIAN_POINT ( 'NONE',  ( -16.55341960407617563, 4.379528057220093196, 68.54275706135234714 ) ) ;
#64937=CARTESIAN_POINT ( 'NONE',  ( -5.153800228976328057, -19.02544592524343514, 57.29057627198103120 ) ) ;
#64938=CARTESIAN_POINT ( 'NONE',  ( -9.474510206698964154, 16.51473224551069663, 65.41557627198102409 ) ) ;
#64939=ORIENTED_EDGE ( 'NONE', *, *, #19140, .T. ) ;
#64940=CARTESIAN_POINT ( 'NONE',  ( 0.05219959533937995610, -21.53943276465977519, 110.0010903946856757 ) ) ;
#64941=CARTESIAN_POINT ( 'NONE',  ( -14.29746914071037622, -8.314922557961029526, 69.16775706135234714 ) ) ;
#64942=CARTESIAN_POINT ( 'NONE',  ( 5.719274019375673035, 21.55341960407619339, 102.2927570613523613 ) ) ;
#64943=CARTESIAN_POINT ( 'NONE',  ( 19.02544592524343514, -5.153800228976328945, 68.54057627198103830 ) ) ;
#64944=CARTESIAN_POINT ( 'NONE',  ( -15.72974639402197994, 15.80617190586746368, 30.62390960531436335 ) ) ;
#64945=CARTESIAN_POINT ( 'NONE',  ( 19.05341960407617918, -5.049401038297876454, 111.0427570613523329 ) ) ;
#64946=CARTESIAN_POINT ( 'NONE',  ( -10.72451020669870658, -18.67979575497194134, 64.58442372801900433 ) ) ;
#64947=CARTESIAN_POINT ( 'NONE',  ( 4.379528057220092307, 16.55341960407617563, 52.29275706135236135 ) ) ;
#64948=CARTESIAN_POINT ( 'NONE',  ( -21.52544592524343514, 5.823673210054127303, 106.0405762719810525 ) ) ;
#64949=CARTESIAN_POINT ( 'NONE',  ( 16.51473224551083163, -9.474510206698727899, 100.8344237280190043 ) ) ;
#64950=CARTESIAN_POINT ( 'NONE',  ( -16.51473224551069308, -9.474510206698971260, 81.66557627198103830 ) ) ;
#64951=CARTESIAN_POINT ( 'NONE',  ( 5.049401038297881783, 19.05341960407617563, 112.2927570613523471 ) ) ;
#64952=CARTESIAN_POINT ( 'NONE',  ( -8.224510206698735004, -14.34966873604973081, 24.58442372801901499 ) ) ;
#64953=CARTESIAN_POINT ( 'NONE',  ( -14.29746914071049879, 8.314922557960819915, 60.83224293864769550 ) ) ;
#64954=CARTESIAN_POINT ( 'NONE',  ( 8.314922557961029526, -14.29746914071037800, 70.41775706135236135 ) ) ;
#64955=CARTESIAN_POINT ( 'NONE',  ( -15.72974639402197994, 15.80617190586746368, 115.6239096053143669 ) ) ;
#64956=CARTESIAN_POINT ( 'NONE',  ( -19.03943276465977164, 0.05219959533909376836, 56.24890960531435979 ) ) ;
#64957=CARTESIAN_POINT ( 'NONE',  ( -19.02544592524342804, 5.153800228976336051, 66.04057627198103830 ) ) ;
#64958=CARTESIAN_POINT ( 'NONE',  ( 8.224510206698742110, 14.34966873604972548, 67.08442372801901854 ) ) ;
#64961=CARTESIAN_POINT ( 'NONE',  ( 19.05341960407617918, -5.049401038297876454, 21.04275706135232582 ) ) ;
#64963=CARTESIAN_POINT ( 'NONE',  ( -16.46253265017160317, 9.564922557960807481, 35.83224293864768839 ) ) ;
#64965=CARTESIAN_POINT ( 'NONE',  ( -19.05341960407617563, 5.049401038297882671, 108.5427570613523187 ) ) ;
#64966=CARTESIAN_POINT ( 'NONE',  ( -9.564922557961040184, 16.46253265017147172, 42.91775706135234003 ) ) ;
#64967=CARTESIAN_POINT ( 'NONE',  ( -16.53943276465976808, -0.05219959533934237506, 23.75109039468567929 ) ) ;
#64968=CARTESIAN_POINT ( 'NONE',  ( 19.05341960407611168, 5.049401038298154454, 43.95724293864769550 ) ) ;
#64969=CARTESIAN_POINT ( 'NONE',  ( -5.153800228976328057, -19.02544592524343514, 62.29057627198100988 ) ) ;
#64970=CARTESIAN_POINT ( 'NONE',  ( 21.53943276465977519, -0.05219959533907433946, 88.74890960531436690 ) ) ;
#64971=CARTESIAN_POINT ( 'NONE',  ( 9.474510206698971260, -16.51473224551069308, 107.9155762719810383 ) ) ;
#64972=CARTESIAN_POINT ( 'NONE',  ( -13.97604488694527625, -13.89961937509977652, 56.87390960531434558 ) ) ;
#64974=CARTESIAN_POINT ( 'NONE',  ( -9.564922557961040184, 16.46253265017147172, 92.91775706135233293 ) ) ;
#64975=CARTESIAN_POINT ( 'NONE',  ( -15.72974639402197994, 15.80617190586746368, 75.62390960531439532 ) ) ;
#64976=CARTESIAN_POINT ( 'NONE',  ( 9.564922557961047289, -16.46253265017146816, 30.41775706135232937 ) ) ;
#64978=CARTESIAN_POINT ( 'NONE',  ( -4.379528057220328563, 16.55341960407611168, 65.20724293864768129 ) ) ;
#64979=CARTESIAN_POINT ( 'NONE',  ( 15.80617190586769283, -15.72974639402175789, 90.62609039468567573 ) ) ;
#64980=CARTESIAN_POINT ( 'NONE',  ( -13.89961937509977652, 13.97604488694528158, 25.62390960531434558 ) ) ;
#64981=CARTESIAN_POINT ( 'NONE',  ( -0.05219959533937732626, 21.53943276465977519, 87.50109039468568994 ) ) ;
#64982=CARTESIAN_POINT ( 'NONE',  ( 8.314922557960818139, 14.29746914071049879, 29.58224293864769905 ) ) ;
#64983=CARTESIAN_POINT ( 'NONE',  ( -5.823673210054431948, 21.52544592524334988, 87.70942372801901854 ) ) ;
#64984=CARTESIAN_POINT ( 'NONE',  ( 5.153800228976335163, 19.02544592524342804, 74.79057627198103830 ) ) ;
#64985=CARTESIAN_POINT ( 'NONE',  ( -21.55341960407619339, 5.719274019375674811, 38.54275706135234714 ) ) ;
#64986=CARTESIAN_POINT ( 'NONE',  ( -13.89961937509977652, 13.97604488694528158, 75.62390960531438111 ) ) ;
#64987=CARTESIAN_POINT ( 'NONE',  ( -16.53943276465976808, 0.05219959533911058130, 96.24890960531435269 ) ) ;
#64988=CARTESIAN_POINT ( 'NONE',  ( -8.314922557960811034, -14.29746914071050412, 67.08224293864770971 ) ) ;
#64989=CARTESIAN_POINT ( 'NONE',  ( -15.72974639402197994, 15.80617190586746368, 70.62390960531436690 ) ) ;
#64990=CARTESIAN_POINT ( 'NONE',  ( 16.46253265017160672, -9.564922557960803928, 73.33224293864769550 ) ) ;
#64991=CARTESIAN_POINT ( 'NONE',  ( -10.81492255796078084, -18.62759615963271287, 87.08224293864769550 ) ) ;
#64992=CARTESIAN_POINT ( 'NONE',  ( -9.564922557961040184, 16.46253265017147172, 77.91775706135234714 ) ) ;
#64993=CARTESIAN_POINT ( 'NONE',  ( -5.153800228976607833, 19.02544592524335343, 37.70942372801899722 ) ) ;
#64994=CARTESIAN_POINT ( 'NONE',  ( 4.483927247898545687, 16.52544592524342804, 79.79057627198102409 ) ) ;
#64995=CARTESIAN_POINT ( 'NONE',  ( -21.53943276465977519, 0.05219959533907696930, 51.24890960531436690 ) ) ;
#64997=CARTESIAN_POINT ( 'NONE',  ( -14.29746914071037622, -8.314922557961029526, 99.16775706135234714 ) ) ;
#64999=CARTESIAN_POINT ( 'NONE',  ( 16.51473224551083163, -9.474510206698727899, 105.8344237280190043 ) ) ;
#65000=CARTESIAN_POINT ( 'NONE',  ( 4.379528057220339221, -16.55341960407611168, 67.70724293864769550 ) ) ;
#65001=CARTESIAN_POINT ( 'NONE',  ( -17.50000000000001421, 3.209263204892553567, 34.76196825606270124 ) ) ;
#65002=CARTESIAN_POINT ( 'NONE',  ( 16.46253265017160672, -9.564922557960803928, 58.33224293864769550 ) ) ;
#65003=CARTESIAN_POINT ( 'NONE',  ( 8.314922557960818139, 14.29746914071049879, 54.58224293864769550 ) ) ;
#65005=CARTESIAN_POINT ( 'NONE',  ( -9.564922557960796823, -16.46253265017161027, 107.0822429386476955 ) ) ;
#65006=CARTESIAN_POINT ( 'NONE',  ( -5.049401038297874678, -19.05341960407617918, 89.79275706135230450 ) ) ;
#65007=CARTESIAN_POINT ( 'NONE',  ( 5.153800228976335163, 19.02544592524342804, 59.79057627198100988 ) ) ;
#65008=CARTESIAN_POINT ( 'NONE',  ( 0.05219959533909260263, 19.03943276465977164, 84.99890960531436690 ) ) ;
#65009=CARTESIAN_POINT ( 'NONE',  ( 5.049401038298161559, -19.05341960407611168, 92.70724293864769550 ) ) ;
#65010=CARTESIAN_POINT ( 'NONE',  ( 0.05219959533907565091, 21.53943276465977519, 64.99890960531435269 ) ) ;
#65011=CARTESIAN_POINT ( 'NONE',  ( -16.55341960407617563, 4.379528057220093196, 53.54275706135234714 ) ) ;
#65012=CARTESIAN_POINT ( 'NONE',  ( 9.474510206698729675, 16.51473224551082808, 102.0844237280190043 ) ) ;
#65013=CARTESIAN_POINT ( 'NONE',  ( 5.153800228976335163, 19.02544592524342804, 59.79057627198100988 ) ) ;
#65014=CARTESIAN_POINT ( 'NONE',  ( 18.62759615963271287, -10.81492255796078972, 63.33224293864770260 ) ) ;
#65015=SHAPE_REPRESENTATION ( 'Mica Insulated Heating Coil Unit', ( #82054 ), #78902 ) ;
#65016=CARTESIAN_POINT ( 'NONE',  ( 19.05341960407617918, -5.049401038297876454, 101.0427570613523045 ) ) ;
#65017=CARTESIAN_POINT ( 'NONE',  ( 16.53943276465976808, -0.05219959533910856209, 28.74890960531435624 ) ) ;
#65018=CARTESIAN_POINT ( 'NONE',  ( -10.72451020669870658, -18.67979575497194134, 44.58442372801901854 ) ) ;
#65020=CARTESIAN_POINT ( 'NONE',  ( -16.53943276465976808, -0.05219959533934237506, 78.75109039468568994 ) ) ;
#65021=CARTESIAN_POINT ( 'NONE',  ( 16.53943276465976808, 0.05219959533934440121, 96.25109039468568994 ) ) ;
#65023=CARTESIAN_POINT ( 'NONE',  ( -16.53943276465976808, -0.05219959533934237506, 78.75109039468568994 ) ) ;
#65024=CARTESIAN_POINT ( 'NONE',  ( -16.53943276465976808, -0.05219959533934237506, 33.75109039468568284 ) ) ;
#65025=CARTESIAN_POINT ( 'NONE',  ( -19.05341960407611168, -5.049401038298163336, 46.45724293864768129 ) ) ;
#65026=CARTESIAN_POINT ( 'NONE',  ( 9.564922557960805705, 16.46253265017160317, 54.58224293864769550 ) ) ;
#65027=CARTESIAN_POINT ( 'NONE',  ( -0.05219959533909027116, -19.03943276465977164, 62.49890960531435979 ) ) ;
#65028=CARTESIAN_POINT ( 'NONE',  ( -21.52544592524334988, -5.823673210054445271, 58.95942372801902565 ) ) ;
#65029=CARTESIAN_POINT ( 'NONE',  ( -12.06949235617739369, -12.14591786802326823, 49.37609039468569705 ) ) ;
#65030=CARTESIAN_POINT ( 'NONE',  ( -0.05219959533934338120, 16.53943276465976808, 112.5010903946857042 ) ) ;
#65031=CARTESIAN_POINT ( 'NONE',  ( 5.049401038298161559, -19.05341960407611168, 22.70724293864769194 ) ) ;
#65032=CARTESIAN_POINT ( 'NONE',  ( 19.05341960407611168, 5.049401038298154454, 38.95724293864767418 ) ) ;
#65033=CARTESIAN_POINT ( 'NONE',  ( -8.224510206698735004, -14.34966873604973081, 34.58442372801900433 ) ) ;
#65034=CARTESIAN_POINT ( 'NONE',  ( -13.97604488694547697, 13.89961937509957934, 88.12609039468563310 ) ) ;
#65035=CARTESIAN_POINT ( 'NONE',  ( 0.05219959533910956823, 16.53943276465976808, 84.99890960531436690 ) ) ;
#65036=CARTESIAN_POINT ( 'NONE',  ( 5.049401038298161559, -19.05341960407611168, 52.70724293864767418 ) ) ;
#65037=CARTESIAN_POINT ( 'NONE',  ( 13.89961937509957401, 13.97604488694547697, 71.87609039468567573 ) ) ;
#65038=CARTESIAN_POINT ( 'NONE',  ( 16.38665767535051998, -7.295008042176092999, 92.76400864214544129 ) ) ;
#65039=CARTESIAN_POINT ( 'NONE',  ( 5.719274019375673035, 21.55341960407619339, 77.29275706135234714 ) ) ;
#65040=CARTESIAN_POINT ( 'NONE',  ( -12.14591786802326823, 12.06949235617739902, 53.12609039468568284 ) ) ;
#65041=CARTESIAN_POINT ( 'NONE',  ( 17.50000000000000000, 5.499999999999997335, 36.70309617465829177 ) ) ;
#65042=CARTESIAN_POINT ( 'NONE',  ( -15.72974639402197994, 15.80617190586746368, 40.62390960531435269 ) ) ;
#65043=CARTESIAN_POINT ( 'NONE',  ( -14.29746914071037622, -8.314922557961029526, 29.16775706135234003 ) ) ;
#65044=CARTESIAN_POINT ( 'NONE',  ( -9.564922557960796823, -16.46253265017161027, 27.08224293864769550 ) ) ;
#65045=CARTESIAN_POINT ( 'NONE',  ( -9.474510206698720793, -16.51473224551083518, 29.58442372801900433 ) ) ;
#65047=CARTESIAN_POINT ( 'NONE',  ( 9.564922557960805705, 16.46253265017160317, 39.58224293864768839 ) ) ;
#65049=CARTESIAN_POINT ( 'NONE',  ( -9.474510206698964154, 16.51473224551069663, 75.41557627198103830 ) ) ;
#65050=CARTESIAN_POINT ( 'NONE',  ( -18.56101223717333326, -5.499999999999954703, 56.44978406935679516 ) ) ;
#65051=CARTESIAN_POINT ( 'NONE',  ( -5.049401038297874678, -19.05341960407617918, 19.79275706135233293 ) ) ;
#65052=CARTESIAN_POINT ( 'NONE',  ( -14.29746914071049879, 8.314922557960819915, 40.83224293864769550 ) ) ;
#65053=CARTESIAN_POINT ( 'NONE',  ( -13.89961937509977652, 13.97604488694528158, 40.62390960531435979 ) ) ;
#65054=CARTESIAN_POINT ( 'NONE',  ( -16.51473224551069308, -9.474510206698971260, 106.6655762719810383 ) ) ;
#65055=CARTESIAN_POINT ( 'NONE',  ( 21.55341960407619695, -5.719274019375665929, 66.04275706135236135 ) ) ;
#65056=CARTESIAN_POINT ( 'NONE',  ( -19.05341960407611168, -5.049401038298163336, 56.45724293864768129 ) ) ;
#65057=CARTESIAN_POINT ( 'NONE',  ( 15.80617190586769283, -15.72974639402175789, 70.62609039468567573 ) ) ;
#65058=CARTESIAN_POINT ( 'NONE',  ( 0.05219959533907565091, 21.53943276465977519, 24.99890960531435624 ) ) ;
#65059=CARTESIAN_POINT ( 'NONE',  ( 19.02544592524343514, -5.153800228976328945, 38.54057627198103120 ) ) ;
#65060=CARTESIAN_POINT ( 'NONE',  ( 0.05219959533937995610, -21.53943276465977519, 30.00109039468568284 ) ) ;
#65061=CARTESIAN_POINT ( 'NONE',  ( -19.02544592524334988, -5.153800228976617603, 53.95942372801898301 ) ) ;
#65062=CARTESIAN_POINT ( 'NONE',  ( -14.34966873604960291, -8.224510206698953496, 106.6655762719810383 ) ) ;
#65063=CARTESIAN_POINT ( 'NONE',  ( 13.89961937509977652, -13.97604488694527269, 58.12390960531436690 ) ) ;
#65064=CARTESIAN_POINT ( 'NONE',  ( -16.53943276465976808, -0.05219959533934237506, 18.75109039468568639 ) ) ;
#65065=CARTESIAN_POINT ( 'NONE',  ( -12.14591786802309592, -12.06949235617757132, 71.87390960531438111 ) ) ;
#65066=CARTESIAN_POINT ( 'NONE',  ( 16.51473224551069308, 9.474510206698969483, 114.1655762719810241 ) ) ;
#65067=CARTESIAN_POINT ( 'NONE',  ( -16.46253265017146816, -9.564922557961047289, 104.1677570613523329 ) ) ;
#65068=CARTESIAN_POINT ( 'NONE',  ( 5.823673210054125526, 21.52544592524343514, 109.7905762719810383 ) ) ;
#65069=CARTESIAN_POINT ( 'NONE',  ( -5.823673210054431948, 21.52544592524334988, 52.70942372801902565 ) ) ;
#65070=CARTESIAN_POINT ( 'NONE',  ( 12.14591786802327356, -12.06949235617739191, 60.62609039468567573 ) ) ;
#65071=CARTESIAN_POINT ( 'NONE',  ( 12.14591786802327356, -12.06949235617739191, 55.62609039468568284 ) ) ;
#65072=CARTESIAN_POINT ( 'NONE',  ( -21.52544592524343514, 5.823673210054127303, 51.04057627198103120 ) ) ;
#65073=CARTESIAN_POINT ( 'NONE',  ( 16.51473224551069308, 9.474510206698969483, 49.16557627198102409 ) ) ;
#65074=CARTESIAN_POINT ( 'NONE',  ( 12.06949235617739724, 12.14591786802326823, 76.87609039468567573 ) ) ;
#65075=CARTESIAN_POINT ( 'NONE',  ( -18.62759615963270932, 10.81492255796079327, 95.83224293864770971 ) ) ;
#65076=CARTESIAN_POINT ( 'NONE',  ( 8.314922557960818139, 14.29746914071049879, 54.58224293864769550 ) ) ;
#65077=CARTESIAN_POINT ( 'NONE',  ( -0.05219959533909027116, -19.03943276465977164, 67.49890960531436690 ) ) ;
#65078=CARTESIAN_POINT ( 'NONE',  ( -0.05219959533934338120, 16.53943276465976808, 72.50109039468568994 ) ) ;
#65079=CARTESIAN_POINT ( 'NONE',  ( -0.05219959533936034679, 19.03943276465977164, 107.5010903946856615 ) ) ;
#65080=CARTESIAN_POINT ( 'NONE',  ( 5.823673210054125526, 21.52544592524343514, 99.79057627198103830 ) ) ;
#65081=CARTESIAN_POINT ( 'NONE',  ( 14.34966873604960469, 8.224510206698951720, 44.16557627198103120 ) ) ;
#65083=CARTESIAN_POINT ( 'NONE',  ( -16.21995358207302473, 7.366697692864226710, 69.93551001512156517 ) ) ;
#65084=CARTESIAN_POINT ( 'NONE',  ( 18.67979575497178502, 10.72451020669898547, 84.16557627198103830 ) ) ;
#65085=CARTESIAN_POINT ( 'NONE',  ( 8.224510206698953496, -14.34966873604960469, 22.91557627198102765 ) ) ;
#65088=CARTESIAN_POINT ( 'NONE',  ( 18.67979575497178502, 10.72451020669898547, 99.16557627198100988 ) ) ;
#65089=CARTESIAN_POINT ( 'NONE',  ( 5.049401038298161559, -19.05341960407611168, 97.70724293864766707 ) ) ;
#65090=CARTESIAN_POINT ( 'NONE',  ( -5.719274019375665041, -21.55341960407619695, 19.79275706135235069 ) ) ;
#65091=CARTESIAN_POINT ( 'NONE',  ( 14.29746914071049879, -8.314922557960816363, 43.33224293864769550 ) ) ;
#65092=CARTESIAN_POINT ( 'NONE',  ( -16.52544592524335698, -4.483927247898792601, 53.95942372801900433 ) ) ;
#65093=CARTESIAN_POINT ( 'NONE',  ( 9.564922557960805705, 16.46253265017160317, 44.58224293864769550 ) ) ;
#65095=CARTESIAN_POINT ( 'NONE',  ( -19.03943276465977164, -0.05219959533935918106, 53.75109039468566863 ) ) ;
#65096=CARTESIAN_POINT ( 'NONE',  ( 16.46253265017160672, -9.564922557960803928, 78.33224293864769550 ) ) ;
#65097=CARTESIAN_POINT ( 'NONE',  ( -18.67979575497178146, -10.72451020669898902, 31.66557627198102054 ) ) ;
#65099=CARTESIAN_POINT ( 'NONE',  ( -0.05219959533936034679, 19.03943276465977164, 112.5010903946856757 ) ) ;
#65100=CARTESIAN_POINT ( 'NONE',  ( -5.153800228976607833, 19.02544592524334988, 47.70942372801900433 ) ) ;
#65101=CARTESIAN_POINT ( 'NONE',  ( 21.53943276465977519, -0.05219959533907433946, 98.74890960531438111 ) ) ;
#65102=CARTESIAN_POINT ( 'NONE',  ( 8.314922557960818139, 14.29746914071049879, 34.58224293864770260 ) ) ;
#65103=CARTESIAN_POINT ( 'NONE',  ( -0.05219959533909027116, -19.03943276465977164, 82.49890960531436690 ) ) ;
#65104=CARTESIAN_POINT ( 'NONE',  ( 5.719274019375991003, -21.55341960407610458, 62.70724293864769550 ) ) ;
#65105=CARTESIAN_POINT ( 'NONE',  ( -21.53943276465977519, 0.05219959533907696930, 101.2489096053143669 ) ) ;
#65106=CARTESIAN_POINT ( 'NONE',  ( 16.52544592524335698, 4.483927247898782831, 31.45942372801901854 ) ) ;
#65107=CARTESIAN_POINT ( 'NONE',  ( 18.67979575497178502, 10.72451020669898547, 24.16557627198103120 ) ) ;
#65108=CARTESIAN_POINT ( 'NONE',  ( 18.67979575497194134, -10.72451020669871369, 85.83442372801901854 ) ) ;
#65109=CARTESIAN_POINT ( 'NONE',  ( -19.02544592524342804, 5.153800228976336051, 86.04057627198103830 ) ) ;
#65110=CARTESIAN_POINT ( 'NONE',  ( -0.05219959533909027116, -19.03943276465977164, 22.49890960531436690 ) ) ;
#65111=CARTESIAN_POINT ( 'NONE',  ( 13.97604488694527802, 13.89961937509977652, 79.37390960531435269 ) ) ;
#65112=CARTESIAN_POINT ( 'NONE',  ( 12.06949235617757843, -12.14591786802309237, 108.1239096053143811 ) ) ;
#65113=CARTESIAN_POINT ( 'NONE',  ( -19.02544592524342804, 5.153800228976336051, 66.04057627198103830 ) ) ;
#65114=CARTESIAN_POINT ( 'NONE',  ( 9.474510206698729675, 16.51473224551082808, 112.0844237280190043 ) ) ;
#65115=CARTESIAN_POINT ( 'NONE',  ( 17.50000000000000355, 3.189878218039124302, 32.62948562571244793 ) ) ;
#65116=CARTESIAN_POINT ( 'NONE',  ( -5.153800228976328057, -19.02544592524343514, 72.29057627198102409 ) ) ;
#65117=CARTESIAN_POINT ( 'NONE',  ( -0.05219959533937732626, 21.53943276465977519, 102.5010903946856899 ) ) ;
#65118=CARTESIAN_POINT ( 'NONE',  ( 21.53943276465977519, -0.05219959533907433946, 23.74890960531435269 ) ) ;
#65119=CARTESIAN_POINT ( 'NONE',  ( 12.06949235617739724, 12.14591786802326823, 91.87609039468568994 ) ) ;
#65121=CARTESIAN_POINT ( 'NONE',  ( 19.02544592524334988, 5.153800228976608722, 76.45942372801897591 ) ) ;
#65122=CARTESIAN_POINT ( 'NONE',  ( -21.53943276465977519, -0.05219959533937600094, 113.7510903946856757 ) ) ;
#65123=CARTESIAN_POINT ( 'NONE',  ( -16.61371651742604172, -7.165104196376049117, 46.14584930007004715 ) ) ;
#65124=CARTESIAN_POINT ( 'NONE',  ( 13.97604488694527802, 13.89961937509977652, 34.37390960531436690 ) ) ;
#65125=CARTESIAN_POINT ( 'NONE',  ( 4.483927247898545687, 16.52544592524342804, 39.79057627198103830 ) ) ;
#65128=CARTESIAN_POINT ( 'NONE',  ( 16.55341960407618274, -4.379528057220086978, 101.0427570613523756 ) ) ;
#65129=CARTESIAN_POINT ( 'NONE',  ( -19.01529144963339846, -5.499999999999897859, 86.23431955728437970 ) ) ;
#65130=CARTESIAN_POINT ( 'NONE',  ( 16.55341960407618274, -4.379528057220086978, 76.04275706135237556 ) ) ;
#65131=CARTESIAN_POINT ( 'NONE',  ( 19.02544592524343514, -5.153800228976328945, 43.54057627198103120 ) ) ;
#65132=CARTESIAN_POINT ( 'NONE',  ( -10.81492255796105439, 18.62759615963255655, 92.91775706135236135 ) ) ;
#65133=CARTESIAN_POINT ( 'NONE',  ( -5.049401038297874678, -19.05341960407617918, 104.7927570613523471 ) ) ;
#65134=CARTESIAN_POINT ( 'NONE',  ( -18.62759615963255300, -10.81492255796106328, 79.16775706135234714 ) ) ;
#65135=CARTESIAN_POINT ( 'NONE',  ( -5.049401038297874678, -19.05341960407617918, 59.79275706135231871 ) ) ;
#65136=CARTESIAN_POINT ( 'NONE',  ( 9.474510206698971260, -16.51473224551069308, 82.91557627198103830 ) ) ;
#65137=CARTESIAN_POINT ( 'NONE',  ( 9.474510206698971260, -16.51473224551069308, 67.91557627198102409 ) ) ;
#65138=CARTESIAN_POINT ( 'NONE',  ( 16.31925111598459210, 7.325300261831483084, 72.33575461032744158 ) ) ;
#65139=CARTESIAN_POINT ( 'NONE',  ( -0.05219959533910754901, -16.53943276465976808, 72.49890960531435269 ) ) ;
#65140=CARTESIAN_POINT ( 'NONE',  ( 15.80617190586746368, 15.72974639402197994, 54.37390960531435979 ) ) ;
#65141=CARTESIAN_POINT ( 'NONE',  ( -9.564922557960796823, -16.46253265017161027, 47.08224293864769550 ) ) ;
#65142=CARTESIAN_POINT ( 'NONE',  ( -10.72451020669898014, 18.67979575497178502, 85.41557627198102409 ) ) ;
#65143=CARTESIAN_POINT ( 'NONE',  ( 16.53943276465976808, 0.05219959533934440121, 76.25109039468568994 ) ) ;
#65144=VERTEX_POINT ( 'NONE', #175368 ) ;
#65145=CARTESIAN_POINT ( 'NONE',  ( -8.314922557960811034, -14.29746914071050412, 77.08224293864769550 ) ) ;
#65147=CARTESIAN_POINT ( 'NONE',  ( -4.379528057220086978, -16.55341960407618274, 39.79275706135235424 ) ) ;
#65148=CARTESIAN_POINT ( 'NONE',  ( -12.06949235617756955, 12.14591786802309770, 110.6239096053143669 ) ) ;
#65149=CARTESIAN_POINT ( 'NONE',  ( -5.049401038297874678, -19.05341960407617918, 64.79275706135233293 ) ) ;
#65150=CARTESIAN_POINT ( 'NONE',  ( 16.53943276465976808, -0.05219959533910856209, 68.74890960531435269 ) ) ;
#65151=CARTESIAN_POINT ( 'NONE',  ( -10.72451020669870658, -18.67979575497194134, 44.58442372801901854 ) ) ;
#65152=DIRECTION ( 'NONE',  ( 0.000000000000000000, 0.000000000000000000, -1.000000000000000000 ) ) ;
#65153=CARTESIAN_POINT ( 'NONE',  ( 21.55341960407610458, 5.719274019375980345, 93.95724293864770971 ) ) ;
#65154=CARTESIAN_POINT ( 'NONE',  ( 16.46253265017160672, -9.564922557960803928, 113.3322429386476955 ) ) ;
#65155=CARTESIAN_POINT ( 'NONE',  ( -16.55341960407611168, -4.379528057220339221, 81.45724293864769550 ) ) ;
#65157=CARTESIAN_POINT ( 'NONE',  ( -16.46253265017160317, 9.564922557960807481, 45.83224293864769550 ) ) ;
#65159=CARTESIAN_POINT ( 'NONE',  ( 19.02544592524334988, 5.153800228976608722, 76.45942372801897591 ) ) ;
#65160=CARTESIAN_POINT ( 'NONE',  ( 15.72974639402176855, 15.80617190586768217, 36.87609039468568994 ) ) ;
#65161=CARTESIAN_POINT ( 'NONE',  ( 16.46253265017160672, -9.564922557960803928, 73.33224293864769550 ) ) ;
#65162=CARTESIAN_POINT ( 'NONE',  ( 9.564922557961047289, -16.46253265017146816, 60.41775706135233293 ) ) ;
#65163=CARTESIAN_POINT ( 'NONE',  ( -19.05341960407611168, -5.049401038298163336, 41.45724293864769550 ) ) ;
#65164=CARTESIAN_POINT ( 'NONE',  ( 4.379528057220339221, -16.55341960407611168, 57.70724293864770260 ) ) ;
#65165=CARTESIAN_POINT ( 'NONE',  ( -4.379528057220328563, 16.55341960407611168, 55.20724293864770260 ) ) ;
#65166=CARTESIAN_POINT ( 'NONE',  ( 13.89961937509977652, -13.97604488694527269, 78.12390960531433848 ) ) ;
#65167=CARTESIAN_POINT ( 'NONE',  ( -21.55341960407610458, -5.719274019375992779, 96.45724293864770971 ) ) ;
#65168=CARTESIAN_POINT ( 'NONE',  ( 13.97604488694527802, 13.89961937509977652, 74.37390960531436690 ) ) ;
#65169=CARTESIAN_POINT ( 'NONE',  ( 0.05219959533907565091, 21.53943276465977519, 79.99890960531435269 ) ) ;
#65170=CARTESIAN_POINT ( 'NONE',  ( -15.72974639402176322, -15.80617190586768395, 109.3760903946857042 ) ) ;
#65171=CARTESIAN_POINT ( 'NONE',  ( -16.51473224551069308, -9.474510206698971260, 31.66557627198102054 ) ) ;
#65172=CARTESIAN_POINT ( 'NONE',  ( -14.29746914071037622, -8.314922557961029526, 104.1677570613523471 ) ) ;
#65173=CARTESIAN_POINT ( 'NONE',  ( -8.314922557960811034, -14.29746914071050412, 97.08224293864770971 ) ) ;
#65174=CARTESIAN_POINT ( 'NONE',  ( -16.51473224551082808, 9.474510206698731452, 108.3344237280190043 ) ) ;
#65176=CARTESIAN_POINT ( 'NONE',  ( -15.80617190586768217, 15.72974639402176855, 33.12609039468569705 ) ) ;
#65177=CARTESIAN_POINT ( 'NONE',  ( -5.049401038297874678, -19.05341960407617918, 54.79275706135234003 ) ) ;
#65178=CARTESIAN_POINT ( 'NONE',  ( 16.52544592524342804, -4.483927247898539470, 23.54057627198102765 ) ) ;
#65179=CARTESIAN_POINT ( 'NONE',  ( -10.72451020669898014, 18.67979575497178502, 70.41557627198102409 ) ) ;
#65180=CARTESIAN_POINT ( 'NONE',  ( -19.03943276465977164, 0.05219959533909376836, 101.2489096053143669 ) ) ;
#65181=CARTESIAN_POINT ( 'NONE',  ( -14.34966873604960291, -8.224510206698953496, 61.66557627198103120 ) ) ;
#65182=CARTESIAN_POINT ( 'NONE',  ( -9.564922557960796823, -16.46253265017161027, 27.08224293864769550 ) ) ;
#65183=CARTESIAN_POINT ( 'NONE',  ( 19.03943276465977164, -0.05219959533909143690, 33.74890960531435979 ) ) ;
#65184=CARTESIAN_POINT ( 'NONE',  ( 13.97604488694548053, -13.89961937509957401, 25.62609039468566507 ) ) ;
#65185=CARTESIAN_POINT ( 'NONE',  ( -16.52544592524335698, -4.483927247898792601, 88.95942372801901854 ) ) ;
#65186=CARTESIAN_POINT ( 'NONE',  ( -5.823673210054431948, 21.52544592524334988, 37.70942372801900433 ) ) ;
#65187=CARTESIAN_POINT ( 'NONE',  ( -12.14591786802326823, 12.06949235617739902, 43.12609039468568284 ) ) ;
#65188=CARTESIAN_POINT ( 'NONE',  ( 0.05219959533909260263, 19.03943276465977164, 114.9989096053143669 ) ) ;
#65189=CARTESIAN_POINT ( 'NONE',  ( 5.049401038298161559, -19.05341960407611168, 57.70724293864769550 ) ) ;
#65190=CARTESIAN_POINT ( 'NONE',  ( 21.52544592524334988, 5.823673210054432836, 91.45942372801901854 ) ) ;
#65191=CARTESIAN_POINT ( 'NONE',  ( -9.474510206698964154, 16.51473224551069663, 75.41557627198103830 ) ) ;
#65192=CARTESIAN_POINT ( 'NONE',  ( 0.05219959533934541429, -16.53943276465976808, 65.00109039468568994 ) ) ;
#65193=CARTESIAN_POINT ( 'NONE',  ( 12.14591786802309770, 12.06949235617756955, 109.3739096053143811 ) ) ;
#65194=CARTESIAN_POINT ( 'NONE',  ( -12.06949235617739369, -12.14591786802326823, 109.3760903946857042 ) ) ;
#65196=CARTESIAN_POINT ( 'NONE',  ( 21.53943276465977519, 0.05219959533937863772, 56.25109039468568284 ) ) ;
#65197=CARTESIAN_POINT ( 'NONE',  ( -19.05341960407611168, -5.049401038298163336, 96.45724293864769550 ) ) ;
#65198=CARTESIAN_POINT ( 'NONE',  ( 9.474510206698971260, -16.51473224551069308, 82.91557627198103830 ) ) ;
#65199=CARTESIAN_POINT ( 'NONE',  ( 19.03943276465977164, -0.05219959533909143690, 103.7489096053143669 ) ) ;
#65200=CARTESIAN_POINT ( 'NONE',  ( -16.53943276465976808, 0.05219959533911058130, 46.24890960531435979 ) ) ;
#65201=CARTESIAN_POINT ( 'NONE',  ( 12.14591786802327356, -12.06949235617739191, 110.6260903946857042 ) ) ;
#65202=CARTESIAN_POINT ( 'NONE',  ( 12.06949235617757843, -12.14591786802309237, 43.12390960531435269 ) ) ;
#65204=CARTESIAN_POINT ( 'NONE',  ( 19.02544592524334988, 5.153800228976608722, 36.45942372801900433 ) ) ;
#65205=CARTESIAN_POINT ( 'NONE',  ( -19.02544592524342804, 5.153800228976336051, 81.04057627198103830 ) ) ;
#65206=CARTESIAN_POINT ( 'NONE',  ( 9.474510206698729675, 16.51473224551082808, 57.08442372801900433 ) ) ;
#65208=CARTESIAN_POINT ( 'NONE',  ( 18.22780087662119897, -5.500000000000096811, 68.51763182126893525 ) ) ;
#65209=CARTESIAN_POINT ( 'NONE',  ( 13.89961937509957401, 13.97604488694547697, 81.87609039468564731 ) ) ;
#65210=CARTESIAN_POINT ( 'NONE',  ( -8.224510206698735004, -14.34966873604973081, 74.58442372801901854 ) ) ;
#65211=DIRECTION ( 'NONE',  ( 6.718897857320949450E-15, -0.9991276842514722478, 0.04175967627138119087 ) ) ;
#65212=CARTESIAN_POINT ( 'NONE',  ( -0.05219959533909027116, -19.03943276465977164, 102.4989096053143669 ) ) ;
#65213=CARTESIAN_POINT ( 'NONE',  ( -18.67979575497193778, 10.72451020669871902, 23.33442372801901499 ) ) ;
#65214=CARTESIAN_POINT ( 'NONE',  ( -13.89961937509957401, -13.97604488694547875, 94.37609039468566152 ) ) ;
#65215=CARTESIAN_POINT ( 'NONE',  ( -13.89961937509977652, 13.97604488694528158, 115.6239096053143669 ) ) ;
#65216=CARTESIAN_POINT ( 'NONE',  ( -0.05219959533909027116, -19.03943276465977164, 47.49890960531435979 ) ) ;
#65217=CARTESIAN_POINT ( 'NONE',  ( 5.153800228976335163, 19.02544592524342804, 94.79057627198103830 ) ) ;
#65218=CARTESIAN_POINT ( 'NONE',  ( -16.53943276465976808, 0.05219959533911058130, 56.24890960531436690 ) ) ;
#65219=CARTESIAN_POINT ( 'NONE',  ( 13.97604488694527802, 13.89961937509977652, 54.37390960531435979 ) ) ;
#65220=CARTESIAN_POINT ( 'NONE',  ( 13.97604488694527802, 13.89961937509977652, 59.37390960531434558 ) ) ;
#65221=CARTESIAN_POINT ( 'NONE',  ( 19.02544592524334988, 5.153800228976608722, 61.45942372801900433 ) ) ;
#65222=CARTESIAN_POINT ( 'NONE',  ( 9.564922557961047289, -16.46253265017146816, 25.41775706135234003 ) ) ;
#65223=CARTESIAN_POINT ( 'NONE',  ( -5.049401038298153566, 19.05341960407611168, 60.20724293864768129 ) ) ;
#65224=CARTESIAN_POINT ( 'NONE',  ( 0.05219959533907565091, 21.53943276465977519, 69.99890960531435269 ) ) ;
#65225=CARTESIAN_POINT ( 'NONE',  ( 12.06949235617757843, -12.14591786802309237, 73.12390960531436690 ) ) ;
#65226=CARTESIAN_POINT ( 'NONE',  ( -5.049401038297874678, -19.05341960407617918, 29.79275706135232227 ) ) ;
#65228=CARTESIAN_POINT ( 'NONE',  ( -0.05219959533907301413, -21.53943276465977519, 52.49890960531435979 ) ) ;
#65229=CARTESIAN_POINT ( 'NONE',  ( -18.67979575497178146, -10.72451020669898902, 26.66557627198103475 ) ) ;
#65230=CARTESIAN_POINT ( 'NONE',  ( -13.97604488694527625, -13.89961937509977652, 46.87390960531435979 ) ) ;
#65231=CARTESIAN_POINT ( 'NONE',  ( 13.97604488694527802, 13.89961937509977652, 34.37390960531436690 ) ) ;
#65232=CARTESIAN_POINT ( 'NONE',  ( 12.14591786802309770, 12.06949235617756955, 104.3739096053143669 ) ) ;
#65233=CARTESIAN_POINT ( 'NONE',  ( 10.72451020669898902, -18.67979575497178502, 107.9155762719810241 ) ) ;
#65235=CARTESIAN_POINT ( 'NONE',  ( 18.62759615963255655, 10.81492255796105972, 31.66775706135234358 ) ) ;
#65236=CARTESIAN_POINT ( 'NONE',  ( -16.55341960407611168, -4.379528057220339221, 111.4572429386476813 ) ) ;
#65237=CARTESIAN_POINT ( 'NONE',  ( -18.67979575497193778, 10.72451020669871902, 83.33442372801903275 ) ) ;
#65238=CARTESIAN_POINT ( 'NONE',  ( 5.719274019375991003, -21.55341960407610458, 87.70724293864769550 ) ) ;
#65239=CARTESIAN_POINT ( 'NONE',  ( 9.564922557961047289, -16.46253265017146816, 40.41775706135234003 ) ) ;
#65240=CARTESIAN_POINT ( 'NONE',  ( 5.049401038298161559, -19.05341960407611168, 22.70724293864769194 ) ) ;
#65241=CARTESIAN_POINT ( 'NONE',  ( 18.22780087662123805, -5.499999999999976019, 78.51763182126894947 ) ) ;
#65243=CARTESIAN_POINT ( 'NONE',  ( -4.379528057220086978, -16.55341960407618274, 49.79275706135234714 ) ) ;
#65244=CARTESIAN_POINT ( 'NONE',  ( 5.153800228976335163, 19.02544592524342804, 29.79057627198102409 ) ) ;
#65246=CARTESIAN_POINT ( 'NONE',  ( -19.05341960407611168, -5.049401038298163336, 76.45724293864769550 ) ) ;
#65247=CARTESIAN_POINT ( 'NONE',  ( -8.314922557960811034, -14.29746914071050412, 97.08224293864770971 ) ) ;
#65248=CARTESIAN_POINT ( 'NONE',  ( -18.67979575497178146, -10.72451020669898902, 51.66557627198102409 ) ) ;
#65249=CARTESIAN_POINT ( 'NONE',  ( 12.14591786802309770, 12.06949235617756955, 79.37390960531436690 ) ) ;
#65250=CARTESIAN_POINT ( 'NONE',  ( -16.52544592524335698, -4.483927247898792601, 38.95942372801901854 ) ) ;
#65251=CARTESIAN_POINT ( 'NONE',  ( -15.72974639402176322, -15.80617190586768395, 89.37609039468568994 ) ) ;
#65252=CARTESIAN_POINT ( 'NONE',  ( -0.05219959533909027116, -19.03943276465977164, 27.49890960531435624 ) ) ;
#65253=CARTESIAN_POINT ( 'NONE',  ( 8.224510206698742110, 14.34966873604972548, 97.08442372801904696 ) ) ;
#65254=CARTESIAN_POINT ( 'NONE',  ( 16.53943276465976808, -0.05219959533910856209, 43.74890960531435979 ) ) ;
#65255=CARTESIAN_POINT ( 'NONE',  ( 13.97604488694527802, 13.89961937509977652, 49.37390960531434558 ) ) ;
#65256=CARTESIAN_POINT ( 'NONE',  ( 21.53943276465977519, 0.05219959533937863772, 91.25109039468568994 ) ) ;
#65257=CARTESIAN_POINT ( 'NONE',  ( -21.55341960407610458, -5.719274019375992779, 101.4572429386476955 ) ) ;
#65258=CARTESIAN_POINT ( 'NONE',  ( 5.823673210054444382, -21.52544592524334988, 65.20942372801901854 ) ) ;
#65259=CARTESIAN_POINT ( 'NONE',  ( 4.483927247898790824, -16.52544592524335698, 45.20942372801901854 ) ) ;
#65260=CARTESIAN_POINT ( 'NONE',  ( -14.29746914071049879, 8.314922557960819915, 70.83224293864770971 ) ) ;
#65261=CARTESIAN_POINT ( 'NONE',  ( 21.55341960407619695, -5.719274019375665929, 86.04275706135236135 ) ) ;
#65262=CARTESIAN_POINT ( 'NONE',  ( 8.224510206698953496, -14.34966873604960469, 22.91557627198102765 ) ) ;
#65263=CARTESIAN_POINT ( 'NONE',  ( 16.52216118717246118, -7.221426719304361974, 46.42400978952972679 ) ) ;
#65265=CARTESIAN_POINT ( 'NONE',  ( 4.379528057220339221, -16.55341960407611168, 47.70724293864770260 ) ) ;
#65266=CARTESIAN_POINT ( 'NONE',  ( -16.55341960407617563, 4.379528057220093196, 78.54275706135236135 ) ) ;
#65267=CARTESIAN_POINT ( 'NONE',  ( -13.89961937509977652, 13.97604488694528158, 90.62390960531432427 ) ) ;
#65268=CARTESIAN_POINT ( 'NONE',  ( -19.03943276465977164, 0.05219959533909376836, 101.2489096053143669 ) ) ;
#65269=CARTESIAN_POINT ( 'NONE',  ( -21.55341960407619339, 5.719274019375674811, 83.54275706135234714 ) ) ;
#65270=CARTESIAN_POINT ( 'NONE',  ( -16.53943276465976808, -0.05219959533934237506, 88.75109039468567573 ) ) ;
#65271=CARTESIAN_POINT ( 'NONE',  ( -8.314922557960811034, -14.29746914071050412, 67.08224293864770971 ) ) ;
#65272=CARTESIAN_POINT ( 'NONE',  ( 19.05341960407611168, 5.049401038298154454, 83.95724293864766707 ) ) ;
#65275=CARTESIAN_POINT ( 'NONE',  ( -14.34966873604972548, 8.224510206698743886, 28.33442372801902209 ) ) ;
#65276=CARTESIAN_POINT ( 'NONE',  ( 16.46253265017160672, -9.564922557960803928, 23.33224293864769194 ) ) ;
#65277=CARTESIAN_POINT ( 'NONE',  ( -5.049401038298153566, 19.05341960407611168, 95.20724293864770971 ) ) ;
#65278=CARTESIAN_POINT ( 'NONE',  ( 16.53943276465976808, 0.05219959533934440121, 26.25109039468567573 ) ) ;
#65280=CARTESIAN_POINT ( 'NONE',  ( 18.67979575497194134, -10.72451020669871369, 110.8344237280190043 ) ) ;
#65281=CARTESIAN_POINT ( 'NONE',  ( -14.29746914071037622, -8.314922557961029526, 89.16775706135236135 ) ) ;
#65282=CARTESIAN_POINT ( 'NONE',  ( 16.46253265017146816, 9.564922557961045513, 111.6677570613523329 ) ) ;
#65283=CARTESIAN_POINT ( 'NONE',  ( 19.05341960407611168, 5.049401038298154454, 38.95724293864767418 ) ) ;
#65284=CARTESIAN_POINT ( 'NONE',  ( 14.29746914071037800, 8.314922557961029526, 76.66775706135234714 ) ) ;
#65285=CARTESIAN_POINT ( 'NONE',  ( 8.224510206698742110, 14.34966873604972548, 67.08442372801901854 ) ) ;
#65287=CARTESIAN_POINT ( 'NONE',  ( 16.51473224551083163, -9.474510206698727899, 75.83442372801900433 ) ) ;
#65288=CARTESIAN_POINT ( 'NONE',  ( -10.72451020669870658, -18.67979575497194134, 104.5844237280190185 ) ) ;
#65289=CARTESIAN_POINT ( 'NONE',  ( -19.02544592524342804, 5.153800228976336051, 51.04057627198103120 ) ) ;
#65290=CARTESIAN_POINT ( 'NONE',  ( -0.05219959533909027116, -19.03943276465977164, 92.49890960531436690 ) ) ;
#65291=CARTESIAN_POINT ( 'NONE',  ( -8.314922557960811034, -14.29746914071050412, 82.08224293864768129 ) ) ;
#65292=CARTESIAN_POINT ( 'NONE',  ( 19.03943276465977164, 0.05219959533936151252, 51.25109039468567573 ) ) ;
#65293=CARTESIAN_POINT ( 'NONE',  ( -21.55341960407610458, -5.719274019375992779, 46.45724293864769550 ) ) ;
#65294=CARTESIAN_POINT ( 'NONE',  ( -21.53943276465977519, -0.05219959533937600094, 103.7510903946857042 ) ) ;
#65295=CARTESIAN_POINT ( 'NONE',  ( 19.05341960407611168, 5.049401038298154454, 93.95724293864769550 ) ) ;
#65296=CARTESIAN_POINT ( 'NONE',  ( 18.62759615963255655, 10.81492255796105972, 111.6677570613523613 ) ) ;
#65297=CARTESIAN_POINT ( 'NONE',  ( 21.55341960407610458, 5.719274019375980345, 58.95724293864770971 ) ) ;
#65298=CARTESIAN_POINT ( 'NONE',  ( -5.153800228976328057, -19.02544592524343514, 92.29057627198099567 ) ) ;
#65299=CARTESIAN_POINT ( 'NONE',  ( -13.89961937509957401, -13.97604488694547875, 84.37609039468567573 ) ) ;
#65300=CARTESIAN_POINT ( 'NONE',  ( 13.97604488694527802, 13.89961937509977652, 104.3739096053143385 ) ) ;
#65301=CARTESIAN_POINT ( 'NONE',  ( -4.379528057220086978, -16.55341960407618274, 19.79275706135235069 ) ) ;
#65302=CARTESIAN_POINT ( 'NONE',  ( 0.05219959533910956823, 16.53943276465976808, 109.9989096053143527 ) ) ;
#65303=CARTESIAN_POINT ( 'NONE',  ( 13.89961937509977652, -13.97604488694527269, 83.12390960531436690 ) ) ;
#65304=CARTESIAN_POINT ( 'NONE',  ( 10.72451020669898902, -18.67979575497178502, 77.91557627198102409 ) ) ;
#65305=CARTESIAN_POINT ( 'NONE',  ( 16.53943276465976808, 0.05219959533934440121, 41.25109039468568284 ) ) ;
#65306=CARTESIAN_POINT ( 'NONE',  ( -15.72974639402176322, -15.80617190586768395, 44.37609039468567573 ) ) ;
#65307=CARTESIAN_POINT ( 'NONE',  ( -15.80617190586768217, 15.72974639402176855, 98.12609039468570415 ) ) ;
#65308=CARTESIAN_POINT ( 'NONE',  ( 14.34966873604972726, -8.224510206698740333, 90.83442372801901854 ) ) ;
#65309=CARTESIAN_POINT ( 'NONE',  ( 13.97604488694527802, 13.89961937509977652, 94.37390960531436690 ) ) ;
#65310=CARTESIAN_POINT ( 'NONE',  ( -12.14591786802309592, -12.06949235617757132, 86.87390960531438111 ) ) ;
#65311=CARTESIAN_POINT ( 'NONE',  ( 14.34966873604960469, 8.224510206698951720, 29.16557627198103120 ) ) ;
#65312=CARTESIAN_POINT ( 'NONE',  ( -19.05341960407617563, 5.049401038297882671, 63.54275706135234003 ) ) ;
#65313=CARTESIAN_POINT ( 'NONE',  ( 18.67979575497194134, -10.72451020669871369, 45.83442372801901854 ) ) ;
#65314=CARTESIAN_POINT ( 'NONE',  ( -16.51473224551082808, 9.474510206698731452, 28.33442372801900433 ) ) ;
#65315=CARTESIAN_POINT ( 'NONE',  ( -4.483927247898539470, -16.52544592524342804, 97.29057627198105251 ) ) ;
#65316=CARTESIAN_POINT ( 'NONE',  ( 16.46253265017160672, -9.564922557960803928, 108.3322429386476955 ) ) ;
#65317=CARTESIAN_POINT ( 'NONE',  ( 4.379528057220092307, 16.55341960407617563, 112.2927570613523471 ) ) ;
#65318=CARTESIAN_POINT ( 'NONE',  ( -15.72974639402176322, -15.80617190586768395, 84.37609039468570415 ) ) ;
#65319=CARTESIAN_POINT ( 'NONE',  ( -0.05219959533934338120, 16.53943276465976808, 52.50109039468567573 ) ) ;
#65320=CARTESIAN_POINT ( 'NONE',  ( 8.314922557961029526, -14.29746914071037800, 100.4177570613523471 ) ) ;
#65321=CARTESIAN_POINT ( 'NONE',  ( -10.81492255796105439, 18.62759615963255655, 52.91775706135235424 ) ) ;
#65322=VERTEX_POINT ( 'NONE', #129829 ) ;
#65323=CARTESIAN_POINT ( 'NONE',  ( 0.05219959533937995610, -21.53943276465977519, 25.00109039468567218 ) ) ;
#65324=CARTESIAN_POINT ( 'NONE',  ( -12.14591786802309592, -12.06949235617757132, 106.8739096053143811 ) ) ;
#65325=CARTESIAN_POINT ( 'NONE',  ( 9.474510206698971260, -16.51473224551069308, 27.91557627198103120 ) ) ;
#65326=CARTESIAN_POINT ( 'NONE',  ( -16.53943276465976808, 0.05219959533911058130, 66.24890960531436690 ) ) ;
#65327=CARTESIAN_POINT ( 'NONE',  ( 9.474510206698971260, -16.51473224551069308, 77.91557627198103830 ) ) ;
#65328=CARTESIAN_POINT ( 'NONE',  ( 12.06949235617739724, 12.14591786802326823, 101.8760903946857042 ) ) ;
#65329=CARTESIAN_POINT ( 'NONE',  ( 5.153800228976335163, 19.02544592524342804, 39.79057627198100988 ) ) ;
#65330=CARTESIAN_POINT ( 'NONE',  ( -15.80617190586745835, -15.72974639402198527, 56.87390960531436690 ) ) ;
#65331=CARTESIAN_POINT ( 'NONE',  ( -0.05219959533910754901, -16.53943276465976808, 87.49890960531436690 ) ) ;
#65332=CARTESIAN_POINT ( 'NONE',  ( 21.52544592524344225, -5.823673210054117533, 88.54057627198103830 ) ) ;
#65333=CARTESIAN_POINT ( 'NONE',  ( 9.564922557960805705, 16.46253265017160317, 89.58224293864769550 ) ) ;
#65334=CARTESIAN_POINT ( 'NONE',  ( -0.05219959533909027116, -19.03943276465977164, 57.49890960531435979 ) ) ;
#65335=CARTESIAN_POINT ( 'NONE',  ( 19.03943276465977164, 0.05219959533936151252, 86.25109039468567573 ) ) ;
#65336=CARTESIAN_POINT ( 'NONE',  ( 10.81492255796078972, 18.62759615963270932, 44.58224293864769550 ) ) ;
#65337=CARTESIAN_POINT ( 'NONE',  ( -21.53943276465977519, -0.05219959533937600094, 73.75109039468567573 ) ) ;
#65338=CARTESIAN_POINT ( 'NONE',  ( 16.51473224551069308, 9.474510206698969483, 54.16557627198103120 ) ) ;
#65339=CARTESIAN_POINT ( 'NONE',  ( -16.46253265017160317, 9.564922557960807481, 80.83224293864769550 ) ) ;
#65340=CARTESIAN_POINT ( 'NONE',  ( 16.55341960407618274, -4.379528057220086978, 61.04275706135234714 ) ) ;
#65341=CARTESIAN_POINT ( 'NONE',  ( -18.62759615963255300, -10.81492255796106328, 44.16775706135234714 ) ) ;
#65342=CARTESIAN_POINT ( 'NONE',  ( 0.05219959533937995610, -21.53943276465977519, 70.00109039468568994 ) ) ;
#65343=CARTESIAN_POINT ( 'NONE',  ( 0.05219959533907565091, 21.53943276465977519, 24.99890960531435624 ) ) ;
#65344=CARTESIAN_POINT ( 'NONE',  ( 15.72974639402199770, -15.80617190586745480, 98.12390960531436690 ) ) ;
#65345=CARTESIAN_POINT ( 'NONE',  ( -15.80617190586768217, 15.72974639402176855, 33.12609039468569705 ) ) ;
#65346=CARTESIAN_POINT ( 'NONE',  ( -8.314922557961024197, 14.29746914071037800, 67.91775706135234714 ) ) ;
#65347=CARTESIAN_POINT ( 'NONE',  ( 5.823673210054125526, 21.52544592524343514, 59.79057627198103120 ) ) ;
#65348=CARTESIAN_POINT ( 'NONE',  ( -13.97604488694547697, 13.89961937509957934, 38.12609039468566152 ) ) ;
#65349=CARTESIAN_POINT ( 'NONE',  ( -16.46253265017160317, 9.564922557960807481, 70.83224293864770971 ) ) ;
#65350=CARTESIAN_POINT ( 'NONE',  ( 14.29746914071049879, -8.314922557960816363, 23.33224293864769194 ) ) ;
#65352=CARTESIAN_POINT ( 'NONE',  ( 19.05341960407611168, 5.049401038298154454, 103.9572429386476671 ) ) ;
#65354=CARTESIAN_POINT ( 'NONE',  ( -9.564922557961040184, 16.46253265017147172, 87.91775706135233293 ) ) ;
#65355=CARTESIAN_POINT ( 'NONE',  ( 15.80617190586746368, 15.72974639402197994, 54.37390960531435979 ) ) ;
#65356=CARTESIAN_POINT ( 'NONE',  ( -8.314922557960811034, -14.29746914071050412, 42.08224293864769550 ) ) ;
#65357=CARTESIAN_POINT ( 'NONE',  ( 19.02544592524334988, 5.153800228976608722, 96.45942372801897591 ) ) ;
#65358=CARTESIAN_POINT ( 'NONE',  ( -19.02544592524342804, 5.153800228976336051, 36.04057627198100988 ) ) ;
#65359=CARTESIAN_POINT ( 'NONE',  ( -19.05341960407617563, 5.049401038297882671, 108.5427570613523187 ) ) ;
#65360=CARTESIAN_POINT ( 'NONE',  ( 15.72974639402199770, -15.80617190586745480, 93.12390960531436690 ) ) ;
#65361=CARTESIAN_POINT ( 'NONE',  ( 9.564922557961047289, -16.46253265017146816, 60.41775706135233293 ) ) ;
#65362=CARTESIAN_POINT ( 'NONE',  ( -16.52544592524335698, -4.483927247898792601, 78.95942372801901854 ) ) ;
#65363=CARTESIAN_POINT ( 'NONE',  ( 0.05219959533909260263, 19.03943276465977164, 64.99890960531436690 ) ) ;
#65364=CARTESIAN_POINT ( 'NONE',  ( -8.314922557960811034, -14.29746914071050412, 77.08224293864769550 ) ) ;
#65366=CARTESIAN_POINT ( 'NONE',  ( 16.51473224551069308, 9.474510206698969483, 54.16557627198103120 ) ) ;
#65367=CARTESIAN_POINT ( 'NONE',  ( 0.05219959533910956823, 16.53943276465976808, 59.99890960531436690 ) ) ;
#65368=CARTESIAN_POINT ( 'NONE',  ( 16.51473224551069308, 9.474510206698969483, 24.16557627198102765 ) ) ;
#65370=CARTESIAN_POINT ( 'NONE',  ( 8.224510206698953496, -14.34966873604960469, 22.91557627198102765 ) ) ;
#65371=CARTESIAN_POINT ( 'NONE',  ( -0.05219959533909027116, -19.03943276465977164, 72.49890960531435269 ) ) ;
#65372=CARTESIAN_POINT ( 'NONE',  ( -18.09805431107246676, 5.500000000000103029, 51.01606229291886763 ) ) ;
#65373=CARTESIAN_POINT ( 'NONE',  ( -13.97604488694547697, 13.89961937509957934, 33.12609039468566863 ) ) ;
#65374=CARTESIAN_POINT ( 'NONE',  ( -8.314922557961024197, 14.29746914071037800, 47.91775706135234714 ) ) ;
#65375=CARTESIAN_POINT ( 'NONE',  ( 15.72974639402199770, -15.80617190586745480, 63.12390960531435979 ) ) ;
#65376=CARTESIAN_POINT ( 'NONE',  ( -16.46253265017146816, -9.564922557961047289, 19.16775706135233293 ) ) ;
#65377=CARTESIAN_POINT ( 'NONE',  ( -5.049401038298153566, 19.05341960407611168, 80.20724293864769550 ) ) ;
#65379=CARTESIAN_POINT ( 'NONE',  ( -16.46253265017160317, 9.564922557960807481, 115.8322429386477097 ) ) ;
#65380=CARTESIAN_POINT ( 'NONE',  ( 10.72451020669871369, 18.67979575497193778, 37.08442372801901143 ) ) ;
#65381=CARTESIAN_POINT ( 'NONE',  ( -16.55341960407611168, -4.379528057220339221, 101.4572429386476955 ) ) ;
#65382=CARTESIAN_POINT ( 'NONE',  ( -10.81492255796078084, -18.62759615963271287, 107.0822429386476955 ) ) ;
#65383=CARTESIAN_POINT ( 'NONE',  ( 19.02544592524343514, -5.153800228976328945, 78.54057627198099567 ) ) ;
#65385=CARTESIAN_POINT ( 'NONE',  ( -5.823673210054431948, 21.52544592524334988, 32.70942372801900433 ) ) ;
#65387=CARTESIAN_POINT ( 'NONE',  ( 19.05341960407611168, 5.049401038298154454, 88.95724293864769550 ) ) ;
#65388=CARTESIAN_POINT ( 'NONE',  ( -17.50000000000002842, -5.499999999999952927, 76.28230962303568674 ) ) ;
#65389=CARTESIAN_POINT ( 'NONE',  ( -9.474510206698964154, 16.51473224551069663, 25.41557627198103120 ) ) ;
#65390=CARTESIAN_POINT ( 'NONE',  ( 19.03943276465977164, -0.05219959533909143690, 38.74890960531436690 ) ) ;
#65391=CARTESIAN_POINT ( 'NONE',  ( 9.564922557961047289, -16.46253265017146816, 105.4177570613523471 ) ) ;
#65393=CARTESIAN_POINT ( 'NONE',  ( -16.53943276465976808, 0.05219959533911058130, 116.2489096053143669 ) ) ;
#65394=CARTESIAN_POINT ( 'NONE',  ( 21.55341960407619695, -5.719274019375665929, 86.04275706135236135 ) ) ;
#65395=CARTESIAN_POINT ( 'NONE',  ( -0.05219959533909027116, -19.03943276465977164, 57.49890960531435979 ) ) ;
#65396=CARTESIAN_POINT ( 'NONE',  ( 10.81492255796106328, -18.62759615963255655, 40.41775706135234714 ) ) ;
#65397=CARTESIAN_POINT ( 'NONE',  ( -18.67979575497193778, 10.72451020669871902, 28.33442372801902209 ) ) ;
#65399=CARTESIAN_POINT ( 'NONE',  ( 13.89961937509977652, -13.97604488694527269, 83.12390960531436690 ) ) ;
#65401=CARTESIAN_POINT ( 'NONE',  ( 0.05219959533934541429, -16.53943276465976808, 30.00109039468568284 ) ) ;
#65402=CARTESIAN_POINT ( 'NONE',  ( 5.823673210054125526, 21.52544592524343514, 44.79057627198103120 ) ) ;
#65403=CARTESIAN_POINT ( 'NONE',  ( 21.53943276465977519, 0.05219959533937863772, 76.25109039468568994 ) ) ;
#65404=CARTESIAN_POINT ( 'NONE',  ( 5.153800228976335163, 19.02544592524342804, 109.7905762719810099 ) ) ;
#65405=CARTESIAN_POINT ( 'NONE',  ( 9.564922557961047289, -16.46253265017146816, 100.4177570613523329 ) ) ;
#65406=CARTESIAN_POINT ( 'NONE',  ( 16.46253265017160672, -9.564922557960803928, 63.33224293864769550 ) ) ;
#65407=CARTESIAN_POINT ( 'NONE',  ( 5.153800228976335163, 19.02544592524342804, 89.79057627198102409 ) ) ;
#65408=CARTESIAN_POINT ( 'NONE',  ( -16.52544592524342804, 4.483927247898546575, 101.0405762719810383 ) ) ;
#65409=CARTESIAN_POINT ( 'NONE',  ( 8.314922557960818139, 14.29746914071049879, 104.5822429386477097 ) ) ;
#65410=CARTESIAN_POINT ( 'NONE',  ( 5.049401038298161559, -19.05341960407611168, 112.7072429386476813 ) ) ;
#65411=CARTESIAN_POINT ( 'NONE',  ( 16.53943276465976808, 0.05219959533934440121, 81.25109039468568994 ) ) ;
#65412=CARTESIAN_POINT ( 'NONE',  ( -0.05219959533910754901, -16.53943276465976808, 62.49890960531436690 ) ) ;
#65413=CARTESIAN_POINT ( 'NONE',  ( 13.97604488694527802, 13.89961937509977652, 44.37390960531435269 ) ) ;
#65414=CARTESIAN_POINT ( 'NONE',  ( -15.80617190586768217, 15.72974639402176855, 68.12609039468567573 ) ) ;
#65415=CARTESIAN_POINT ( 'NONE',  ( -9.564922557961040184, 16.46253265017147172, 92.91775706135233293 ) ) ;
#65416=CARTESIAN_POINT ( 'NONE',  ( -4.379528057220328563, 16.55341960407611168, 60.20724293864768839 ) ) ;
#65417=CARTESIAN_POINT ( 'NONE',  ( 21.53943276465977519, 0.05219959533937863772, 21.25109039468567218 ) ) ;
#65418=CARTESIAN_POINT ( 'NONE',  ( 10.81492255796078972, 18.62759615963270932, 49.58224293864769550 ) ) ;
#65419=CARTESIAN_POINT ( 'NONE',  ( -17.31747979337945509, -6.344076630961063223, 106.3794486806518194 ) ) ;
#65421=CARTESIAN_POINT ( 'NONE',  ( -19.03943276465977164, 0.05219959533909376836, 71.24890960531435269 ) ) ;
#65422=CARTESIAN_POINT ( 'NONE',  ( -16.52544592524342804, 4.483927247898546575, 41.04057627198103120 ) ) ;
#65423=CARTESIAN_POINT ( 'NONE',  ( -16.55341960407611168, -4.379528057220339221, 21.45724293864769550 ) ) ;
#65424=CARTESIAN_POINT ( 'NONE',  ( -12.14591786802326823, 12.06949235617739902, 83.12609039468568994 ) ) ;
#65425=CARTESIAN_POINT ( 'NONE',  ( 19.03943276465977164, 0.05219959533936151252, 36.25109039468567573 ) ) ;
#65427=CARTESIAN_POINT ( 'NONE',  ( -5.049401038298153566, 19.05341960407611168, 85.20724293864766707 ) ) ;
#65428=CARTESIAN_POINT ( 'NONE',  ( -12.14591786802309592, -12.06949235617757132, 66.87390960531436690 ) ) ;
#65429=CARTESIAN_POINT ( 'NONE',  ( 17.31728774477273802, -6.344390552232379576, 103.3190665168931730 ) ) ;
#65430=CARTESIAN_POINT ( 'NONE',  ( 13.97604488694527802, 13.89961937509977652, 114.3739096053143669 ) ) ;
#65431=CARTESIAN_POINT ( 'NONE',  ( 0.05219959533907565091, 21.53943276465977519, 49.99890960531437401 ) ) ;
#65433=CARTESIAN_POINT ( 'NONE',  ( 14.34966873604960469, 8.224510206698951720, 104.1655762719810241 ) ) ;
#65434=CARTESIAN_POINT ( 'NONE',  ( 12.06949235617739724, 12.14591786802326823, 41.87609039468568284 ) ) ;
#65435=CARTESIAN_POINT ( 'NONE',  ( 0.05219959533910956823, 16.53943276465976808, 84.99890960531436690 ) ) ;
#65437=CARTESIAN_POINT ( 'NONE',  ( 5.049401038297881783, 19.05341960407617563, 77.29275706135231871 ) ) ;
#65438=CARTESIAN_POINT ( 'NONE',  ( -15.80617190586745835, -15.72974639402198527, 26.87390960531435979 ) ) ;
#65440=CARTESIAN_POINT ( 'NONE',  ( -30.00000000000000000, -5.510910596163089556E-15, 47.50000000000000000 ) ) ;
#65441=CARTESIAN_POINT ( 'NONE',  ( 12.06949235617739724, 12.14591786802326823, 31.87609039468567929 ) ) ;
#65442=CARTESIAN_POINT ( 'NONE',  ( 4.379528057220339221, -16.55341960407611168, 32.70724293864770260 ) ) ;
#65443=CARTESIAN_POINT ( 'NONE',  ( 15.72974639402199770, -15.80617190586745480, 53.12390960531436690 ) ) ;
#65444=CARTESIAN_POINT ( 'NONE',  ( 5.049401038297881783, 19.05341960407617563, 67.29275706135234714 ) ) ;
#65445=CARTESIAN_POINT ( 'NONE',  ( -5.823673210054116645, -21.52544592524344225, 52.29057627198102409 ) ) ;
#65446=CARTESIAN_POINT ( 'NONE',  ( -18.62759615963255300, -10.81492255796106328, 69.16775706135234714 ) ) ;
#65448=CARTESIAN_POINT ( 'NONE',  ( -4.379528057220086978, -16.55341960407618274, 39.79275706135235424 ) ) ;
#65449=CARTESIAN_POINT ( 'NONE',  ( 13.97604488694527802, 13.89961937509977652, 29.37390960531435979 ) ) ;
#65450=CARTESIAN_POINT ( 'NONE',  ( -16.51473224551069308, -9.474510206698971260, 86.66557627198102409 ) ) ;
#65451=CARTESIAN_POINT ( 'NONE',  ( -19.05341960407611168, -5.049401038298163336, 31.45724293864769550 ) ) ;
#65452=CARTESIAN_POINT ( 'NONE',  ( -8.314922557960811034, -14.29746914071050412, 107.0822429386476955 ) ) ;
#65454=CARTESIAN_POINT ( 'NONE',  ( 9.474510206698971260, -16.51473224551069308, 97.91557627198102409 ) ) ;
#65456=CARTESIAN_POINT ( 'NONE',  ( -12.14591786802326823, 12.06949235617739902, 58.12609039468568994 ) ) ;
#65457=CARTESIAN_POINT ( 'NONE',  ( 10.72451020669898902, -18.67979575497178502, 92.91557627198103830 ) ) ;
#65458=CARTESIAN_POINT ( 'NONE',  ( 13.89961937509977652, -13.97604488694527269, 48.12390960531435979 ) ) ;
#65459=CARTESIAN_POINT ( 'NONE',  ( -19.03943276465977164, -0.05219959533935918106, 73.75109039468566152 ) ) ;
#65460=CARTESIAN_POINT ( 'NONE',  ( 18.62759615963271287, -10.81492255796078972, 108.3322429386477097 ) ) ;
#65461=CARTESIAN_POINT ( 'NONE',  ( -13.97604488694527625, -13.89961937509977652, 71.87390960531433848 ) ) ;
#65462=CARTESIAN_POINT ( 'NONE',  ( -5.049401038298153566, 19.05341960407611168, 110.2072429386476671 ) ) ;
#65463=VERTEX_POINT ( 'NONE', #189555 ) ;
#65464=CARTESIAN_POINT ( 'NONE',  ( 0.05219959533934541429, -16.53943276465976808, 40.00109039468567573 ) ) ;
#65465=CARTESIAN_POINT ( 'NONE',  ( 21.55341960407619695, -5.719274019375665929, 21.04275706135234714 ) ) ;
#65466=CARTESIAN_POINT ( 'NONE',  ( 0.05219959533910956823, 16.53943276465976808, 109.9989096053143527 ) ) ;
#65467=CARTESIAN_POINT ( 'NONE',  ( 16.51473224551069308, 9.474510206698969483, 94.16557627198103830 ) ) ;
#65468=CARTESIAN_POINT ( 'NONE',  ( 19.05341960407617918, -5.049401038297876454, 81.04275706135231871 ) ) ;
#65469=CARTESIAN_POINT ( 'NONE',  ( 10.72451020669898902, -18.67979575497178502, 87.91557627198103830 ) ) ;
#65470=CARTESIAN_POINT ( 'NONE',  ( 8.314922557960818139, 14.29746914071049879, 49.58224293864769550 ) ) ;
#65471=CARTESIAN_POINT ( 'NONE',  ( -19.03943276465977164, -0.05219959533935918106, 18.75109039468567218 ) ) ;
#65472=CARTESIAN_POINT ( 'NONE',  ( -16.52544592524335698, -4.483927247898792601, 73.95942372801901854 ) ) ;
#65473=CARTESIAN_POINT ( 'NONE',  ( 19.05341960407611168, 5.049401038298154454, 93.95724293864769550 ) ) ;
#65475=CARTESIAN_POINT ( 'NONE',  ( 9.564922557960805705, 16.46253265017160317, 44.58224293864769550 ) ) ;
#65476=CARTESIAN_POINT ( 'NONE',  ( -18.62759615963255300, -10.81492255796106328, 54.16775706135235424 ) ) ;
#65477=CARTESIAN_POINT ( 'NONE',  ( 21.53943276465977519, 0.05219959533937863772, 61.25109039468567573 ) ) ;
#65478=CARTESIAN_POINT ( 'NONE',  ( -5.049401038298153566, 19.05341960407611168, 55.20724293864769550 ) ) ;
#65479=CARTESIAN_POINT ( 'NONE',  ( -18.62759615963255300, -10.81492255796106328, 39.16775706135235424 ) ) ;
#65480=CARTESIAN_POINT ( 'NONE',  ( -16.51473224551082808, 9.474510206698731452, 83.33442372801899012 ) ) ;
#65481=CARTESIAN_POINT ( 'NONE',  ( -13.97604488694527625, -13.89961937509977652, 36.87390960531436690 ) ) ;
#65482=CARTESIAN_POINT ( 'NONE',  ( 16.55341960407618274, -4.379528057220086978, 86.04275706135236135 ) ) ;
#65483=CARTESIAN_POINT ( 'NONE',  ( -13.97604488694527625, -13.89961937509977652, 61.87390960531435979 ) ) ;
#65484=CARTESIAN_POINT ( 'NONE',  ( 16.46253265017160672, -9.564922557960803928, 108.3322429386476955 ) ) ;
#65485=CARTESIAN_POINT ( 'NONE',  ( 5.049401038298161559, -19.05341960407611168, 52.70724293864767418 ) ) ;
#65486=CARTESIAN_POINT ( 'NONE',  ( -21.55341960407610458, -5.719274019375992779, 91.45724293864769550 ) ) ;
#65487=CARTESIAN_POINT ( 'NONE',  ( -12.06949235617739369, -12.14591786802326823, 74.37609039468568994 ) ) ;
#65489=CARTESIAN_POINT ( 'NONE',  ( 19.03943276465977164, 0.05219959533936151252, 36.25109039468567573 ) ) ;
#65490=CARTESIAN_POINT ( 'NONE',  ( -19.03943276465977164, 0.05219959533909376836, 61.24890960531436690 ) ) ;
#65491=CARTESIAN_POINT ( 'NONE',  ( 12.14591786802309770, 12.06949235617756955, 54.37390960531435979 ) ) ;
#65492=CARTESIAN_POINT ( 'NONE',  ( -8.224510206698948167, 14.34966873604960824, 85.41557627198102409 ) ) ;
#65493=CARTESIAN_POINT ( 'NONE',  ( -5.049401038298153566, 19.05341960407611168, 100.2072429386476955 ) ) ;
#65494=CARTESIAN_POINT ( 'NONE',  ( 5.049401038298161559, -19.05341960407611168, 92.70724293864769550 ) ) ;
#65495=CARTESIAN_POINT ( 'NONE',  ( 15.80617190586769283, -15.72974639402175789, 50.62609039468568994 ) ) ;
#65496=CARTESIAN_POINT ( 'NONE',  ( -13.89961937509977652, 13.97604488694528158, 105.6239096053143527 ) ) ;
#65497=CARTESIAN_POINT ( 'NONE',  ( -5.719274019375665041, -21.55341960407619695, 109.7927570613523613 ) ) ;
#65498=CARTESIAN_POINT ( 'NONE',  ( -4.483927247898782831, 16.52544592524335698, 77.70942372801900433 ) ) ;
#65499=EDGE_CURVE ( 'NONE', #93191, #158898, #97714, .T. ) ;
#65500=CARTESIAN_POINT ( 'NONE',  ( 0.05219959533937995610, -21.53943276465977519, 35.00109039468568284 ) ) ;
#65501=CARTESIAN_POINT ( 'NONE',  ( 16.51473224551069308, 9.474510206698969483, 114.1655762719810241 ) ) ;
#65502=CARTESIAN_POINT ( 'NONE',  ( 5.823673210054125526, 21.52544592524343514, 104.7905762719810241 ) ) ;
#65503=CARTESIAN_POINT ( 'NONE',  ( 16.53943276465976808, -0.05219959533910856209, 58.74890960531436690 ) ) ;
#65504=CARTESIAN_POINT ( 'NONE',  ( -5.153800228976328057, -19.02544592524343514, 52.29057627198100988 ) ) ;
#65505=CARTESIAN_POINT ( 'NONE',  ( -0.05219959533910754901, -16.53943276465976808, 77.49890960531433848 ) ) ;
#65506=CARTESIAN_POINT ( 'NONE',  ( 18.67979575497178502, 10.72451020669898547, 34.16557627198102409 ) ) ;
#65507=CARTESIAN_POINT ( 'NONE',  ( -19.05341960407617563, 5.049401038297882671, 43.54275706135232582 ) ) ;
#65508=CARTESIAN_POINT ( 'NONE',  ( -9.564922557960796823, -16.46253265017161027, 22.08224293864768839 ) ) ;
#65510=CARTESIAN_POINT ( 'NONE',  ( 16.53943276465976808, 0.05219959533934440121, 61.25109039468567573 ) ) ;
#65511=CARTESIAN_POINT ( 'NONE',  ( 13.97604488694527802, 13.89961937509977652, 74.37390960531436690 ) ) ;
#65513=CARTESIAN_POINT ( 'NONE',  ( -14.29746914071049879, 8.314922557960819915, 90.83224293864769550 ) ) ;
#65514=CARTESIAN_POINT ( 'NONE',  ( -15.80617190586745835, -15.72974639402198527, 41.87390960531435979 ) ) ;
#65516=CARTESIAN_POINT ( 'NONE',  ( 14.29746914071037800, 8.314922557961029526, 106.6677570613523756 ) ) ;
#65517=CARTESIAN_POINT ( 'NONE',  ( 19.03943276465977164, 0.05219959533936151252, 111.2510903946856757 ) ) ;
#65518=CARTESIAN_POINT ( 'NONE',  ( 0.05219959533937995610, -21.53943276465977519, 75.00109039468568994 ) ) ;
#65519=CARTESIAN_POINT ( 'NONE',  ( -0.05219959533909027116, -19.03943276465977164, 87.49890960531436690 ) ) ;
#65520=CARTESIAN_POINT ( 'NONE',  ( -21.55341960407610458, -5.719274019375992779, 101.4572429386476955 ) ) ;
#65521=CARTESIAN_POINT ( 'NONE',  ( -16.52544592524335698, -4.483927247898792601, 48.95942372801902565 ) ) ;
#65522=CARTESIAN_POINT ( 'NONE',  ( -0.05219959533909027116, -19.03943276465977164, 32.49890960531435979 ) ) ;
#65523=CARTESIAN_POINT ( 'NONE',  ( -4.379528057220086978, -16.55341960407618274, 34.79275706135235424 ) ) ;
#65524=CARTESIAN_POINT ( 'NONE',  ( -5.049401038297874678, -19.05341960407617918, 94.79275706135230450 ) ) ;
#65525=CARTESIAN_POINT ( 'NONE',  ( 18.62759615963271287, -10.81492255796078972, 93.33224293864769550 ) ) ;
#65526=CARTESIAN_POINT ( 'NONE',  ( -9.564922557961040184, 16.46253265017147172, 52.91775706135233293 ) ) ;
#65528=CARTESIAN_POINT ( 'NONE',  ( -21.55341960407610458, -5.719274019375992779, 106.4572429386477097 ) ) ;
#65529=CARTESIAN_POINT ( 'NONE',  ( -17.50000000000000000, -5.499999999999992895, 102.5000000000000142 ) ) ;
#65530=CARTESIAN_POINT ( 'NONE',  ( -0.05219959533909027116, -19.03943276465977164, 72.49890960531435269 ) ) ;
#65532=CARTESIAN_POINT ( 'NONE',  ( -16.52544592524335698, -4.483927247898792601, 33.95942372801901143 ) ) ;
#65534=CARTESIAN_POINT ( 'NONE',  ( 10.72451020669871369, 18.67979575497193778, 22.08442372801901143 ) ) ;
#65535=CARTESIAN_POINT ( 'NONE',  ( 4.379528057220339221, -16.55341960407611168, 67.70724293864769550 ) ) ;
#65536=CARTESIAN_POINT ( 'NONE',  ( 13.89961937509977652, -13.97604488694527269, 73.12390960531436690 ) ) ;
#65537=CARTESIAN_POINT ( 'NONE',  ( -16.53943276465976808, -0.05219959533934237506, 43.75109039468568284 ) ) ;
#65538=CARTESIAN_POINT ( 'NONE',  ( 13.97604488694548053, -13.89961937509957401, 45.62609039468566863 ) ) ;
#65540=CARTESIAN_POINT ( 'NONE',  ( -21.52544592524334988, -5.823673210054445271, 53.95942372801900433 ) ) ;
#65541=CARTESIAN_POINT ( 'NONE',  ( -0.05219959533936034679, 19.03943276465977164, 102.5010903946856757 ) ) ;
#65542=CARTESIAN_POINT ( 'NONE',  ( 19.03943276465977164, -0.05219959533909143690, 58.74890960531435979 ) ) ;
#65543=CARTESIAN_POINT ( 'NONE',  ( -9.474510206698720793, -16.51473224551083518, 79.58442372801899012 ) ) ;
#65544=CARTESIAN_POINT ( 'NONE',  ( 0.05219959533937995610, -21.53943276465977519, 85.00109039468568994 ) ) ;
#65545=CARTESIAN_POINT ( 'NONE',  ( 9.564922557961047289, -16.46253265017146816, 65.41775706135233293 ) ) ;
#65546=CARTESIAN_POINT ( 'NONE',  ( -5.153800228976328057, -19.02544592524343514, 42.29057627198101699 ) ) ;
#65547=CARTESIAN_POINT ( 'NONE',  ( 21.52544592524344225, -5.823673210054117533, 53.54057627198103120 ) ) ;
#65548=CARTESIAN_POINT ( 'NONE',  ( 14.34966873604960469, 8.224510206698951720, 69.16557627198102409 ) ) ;
#65549=CARTESIAN_POINT ( 'NONE',  ( 19.05341960407617918, -5.049401038297876454, 66.04275706135233293 ) ) ;
#65550=CARTESIAN_POINT ( 'NONE',  ( -16.20579543436676673, -7.371946100355209808, 25.56520834171879386 ) ) ;
#65551=CARTESIAN_POINT ( 'NONE',  ( -16.46253265017146816, -9.564922557961047289, 24.16775706135233648 ) ) ;
#65552=CARTESIAN_POINT ( 'NONE',  ( 4.379528057220092307, 16.55341960407617563, 102.2927570613523613 ) ) ;
#65553=CARTESIAN_POINT ( 'NONE',  ( -0.05219959533910754901, -16.53943276465976808, 47.49890960531435979 ) ) ;
#65554=CARTESIAN_POINT ( 'NONE',  ( 18.67979575497194134, -10.72451020669871369, 85.83442372801901854 ) ) ;
#65556=CARTESIAN_POINT ( 'NONE',  ( -21.55341960407619339, 5.719274019375674811, 88.54275706135236135 ) ) ;
#65557=CARTESIAN_POINT ( 'NONE',  ( 15.80617190586746368, 15.72974639402197994, 94.37390960531436690 ) ) ;
#65558=CARTESIAN_POINT ( 'NONE',  ( 0.05219959533909260263, 19.03943276465977164, 49.99890960531435979 ) ) ;
#65559=CARTESIAN_POINT ( 'NONE',  ( -18.62759615963255300, -10.81492255796106328, 64.16775706135234714 ) ) ;
#65560=CARTESIAN_POINT ( 'NONE',  ( 16.51473224551069308, 9.474510206698969483, 49.16557627198102409 ) ) ;
#65561=CARTESIAN_POINT ( 'NONE',  ( 13.89961937509977652, -13.97604488694527269, 68.12390960531436690 ) ) ;
#65562=CARTESIAN_POINT ( 'NONE',  ( -8.224510206698948167, 14.34966873604960824, 105.4155762719810383 ) ) ;
#65563=CARTESIAN_POINT ( 'NONE',  ( -9.564922557960796823, -16.46253265017161027, 112.0822429386476955 ) ) ;
#65564=CARTESIAN_POINT ( 'NONE',  ( 4.483927247898545687, 16.52544592524342804, 49.79057627198102409 ) ) ;
#65565=CARTESIAN_POINT ( 'NONE',  ( 16.46253265017160672, -9.564922557960803928, 33.33224293864770260 ) ) ;
#65566=CARTESIAN_POINT ( 'NONE',  ( -0.05219959533910754901, -16.53943276465976808, 72.49890960531435269 ) ) ;
#65567=CARTESIAN_POINT ( 'NONE',  ( -21.53943276465977519, 0.05219959533907696930, 96.24890960531435269 ) ) ;
#65568=CARTESIAN_POINT ( 'NONE',  ( 10.72451020669871369, 18.67979575497193778, 37.08442372801901143 ) ) ;
#65571=CARTESIAN_POINT ( 'NONE',  ( -0.05219959533934338120, 16.53943276465976808, 42.50109039468567573 ) ) ;
#65572=CARTESIAN_POINT ( 'NONE',  ( -15.72974639402197994, 15.80617190586746368, 80.62390960531438111 ) ) ;
#65573=CARTESIAN_POINT ( 'NONE',  ( -9.474510206698720793, -16.51473224551083518, 19.58442372801899722 ) ) ;
#65574=CARTESIAN_POINT ( 'NONE',  ( 13.89961937509977652, -13.97604488694527269, 98.12390960531433848 ) ) ;
#65575=CARTESIAN_POINT ( 'NONE',  ( -15.80617190586768217, 15.72974639402176855, 38.12609039468567573 ) ) ;
#65577=CARTESIAN_POINT ( 'NONE',  ( -5.719274019375978568, 21.55341960407610458, 25.20724293864769550 ) ) ;
#65578=CARTESIAN_POINT ( 'NONE',  ( -8.314922557961024197, 14.29746914071037800, 97.91775706135236135 ) ) ;
#65579=CARTESIAN_POINT ( 'NONE',  ( -5.719274019375665041, -21.55341960407619695, 54.79275706135235424 ) ) ;
#65580=CARTESIAN_POINT ( 'NONE',  ( -15.72974639402176322, -15.80617190586768395, 89.37609039468568994 ) ) ;
#65581=CARTESIAN_POINT ( 'NONE',  ( 9.474510206698729675, 16.51473224551082808, 32.08442372801900433 ) ) ;
#65582=CARTESIAN_POINT ( 'NONE',  ( 14.29746914071037800, 8.314922557961029526, 86.66775706135234714 ) ) ;
#65583=CARTESIAN_POINT ( 'NONE',  ( -5.823673210054431948, 21.52544592524334988, 42.70942372801901854 ) ) ;
#65584=CARTESIAN_POINT ( 'NONE',  ( -0.05219959533909027116, -19.03943276465977164, 27.49890960531435624 ) ) ;
#65585=CARTESIAN_POINT ( 'NONE',  ( -18.67979575497193778, 10.72451020669871902, 98.33442372801901854 ) ) ;
#65586=CARTESIAN_POINT ( 'NONE',  ( 19.05341960407611168, 5.049401038298154454, 108.9572429386477097 ) ) ;
#65587=CARTESIAN_POINT ( 'NONE',  ( -18.67979575497178146, -10.72451020669898902, 106.6655762719810383 ) ) ;
#65588=CARTESIAN_POINT ( 'NONE',  ( 0.05219959533907565091, 21.53943276465977519, 59.99890960531436690 ) ) ;
#65589=DIRECTION ( 'NONE',  ( -0.000000000000000000, -0.000000000000000000, 1.000000000000000000 ) ) ;
#65590=CARTESIAN_POINT ( 'NONE',  ( -10.81492255796078084, -18.62759615963271287, 72.08224293864769550 ) ) ;
#65591=CARTESIAN_POINT ( 'NONE',  ( 14.29746914071037800, 8.314922557961029526, 46.66775706135234714 ) ) ;
#65592=CARTESIAN_POINT ( 'NONE',  ( 4.379528057220339221, -16.55341960407611168, 67.70724293864769550 ) ) ;
#65593=CARTESIAN_POINT ( 'NONE',  ( 18.22780087662122384, -5.500000000000022204, 101.0154010532610869 ) ) ;
#65594=CARTESIAN_POINT ( 'NONE',  ( -5.153800228976607833, 19.02544592524334988, 92.70942372801901854 ) ) ;
#65596=CARTESIAN_POINT ( 'NONE',  ( 0.05219959533934541429, -16.53943276465976808, 20.00109039468568639 ) ) ;
#65597=CARTESIAN_POINT ( 'NONE',  ( -5.823673210054116645, -21.52544592524344225, 92.29057627198103830 ) ) ;
#65598=CARTESIAN_POINT ( 'NONE',  ( 0.05219959533907565091, 21.53943276465977519, 79.99890960531435269 ) ) ;
#65599=CARTESIAN_POINT ( 'NONE',  ( 5.823673210054125526, 21.52544592524343514, 24.79057627198103120 ) ) ;
#65600=CARTESIAN_POINT ( 'NONE',  ( -4.483927247898782831, 16.52544592524335698, 52.70942372801902565 ) ) ;
#65601=CARTESIAN_POINT ( 'NONE',  ( 13.89961937509977652, -13.97604488694527269, 78.12390960531433848 ) ) ;
#65602=CARTESIAN_POINT ( 'NONE',  ( -21.53943276465977519, -0.05219959533937600094, 28.75109039468567929 ) ) ;
#65603=CARTESIAN_POINT ( 'NONE',  ( -12.06949235617739369, -12.14591786802326823, 19.37609039468568639 ) ) ;
#65604=CARTESIAN_POINT ( 'NONE',  ( -9.474510206698964154, 16.51473224551069663, 105.4155762719810383 ) ) ;
#65605=CARTESIAN_POINT ( 'NONE',  ( -5.153800228976328057, -19.02544592524343514, 82.29057627198103830 ) ) ;
#65606=CARTESIAN_POINT ( 'NONE',  ( 0.05219959533907565091, 21.53943276465977519, 84.99890960531436690 ) ) ;
#65607=CARTESIAN_POINT ( 'NONE',  ( -13.89961937509977652, 13.97604488694528158, 55.62390960531434558 ) ) ;
#65609=CARTESIAN_POINT ( 'NONE',  ( 16.55341960407611168, 4.379528057220329451, 63.95724293864770260 ) ) ;
#65610=CARTESIAN_POINT ( 'NONE',  ( -21.53943276465977519, 0.05219959533907696930, 26.24890960531435624 ) ) ;
#65611=CARTESIAN_POINT ( 'NONE',  ( -18.22780087662119541, 5.500000000000102141, 61.01763182126894947 ) ) ;
#65612=CARTESIAN_POINT ( 'NONE',  ( -21.53943276465977519, 0.05219959533907696930, 106.2489096053143811 ) ) ;
#65613=CARTESIAN_POINT ( 'NONE',  ( -19.03943276465977164, -0.05219959533935918106, 58.75109039468566863 ) ) ;
#65614=CARTESIAN_POINT ( 'NONE',  ( 5.049401038298161559, -19.05341960407611168, 112.7072429386476813 ) ) ;
#65615=CARTESIAN_POINT ( 'NONE',  ( 18.22780087662122739, 5.500000000000000888, 66.48236817873106475 ) ) ;
#65616=CARTESIAN_POINT ( 'NONE',  ( 15.72974639402199770, -15.80617190586745480, 58.12390960531435979 ) ) ;
#65617=CARTESIAN_POINT ( 'NONE',  ( -19.02544592524342804, 5.153800228976336051, 86.04057627198103830 ) ) ;
#65618=CARTESIAN_POINT ( 'NONE',  ( -15.80617190586768217, 15.72974639402176855, 83.12609039468568994 ) ) ;
#65619=CARTESIAN_POINT ( 'NONE',  ( 16.51473224551069308, 9.474510206698969483, 49.16557627198102409 ) ) ;
#65620=CARTESIAN_POINT ( 'NONE',  ( -16.53943276465976808, 0.05219959533911058130, 81.24890960531436690 ) ) ;
#65621=CARTESIAN_POINT ( 'NONE',  ( 16.53943276465976808, 0.05219959533934440121, 41.25109039468568284 ) ) ;
#65622=CARTESIAN_POINT ( 'NONE',  ( 21.52544592524334988, 5.823673210054432836, 66.45942372801903275 ) ) ;
#65623=ORIENTED_EDGE ( 'NONE', *, *, #118181, .T. ) ;
#65624=CARTESIAN_POINT ( 'NONE',  ( -19.05341960407617563, 5.049401038297882671, 23.54275706135233648 ) ) ;
#65625=CARTESIAN_POINT ( 'NONE',  ( 13.97604488694548053, -13.89961937509957401, 85.62609039468568994 ) ) ;
#65626=CARTESIAN_POINT ( 'NONE',  ( -5.153800228976607833, 19.02544592524334988, 37.70942372801899722 ) ) ;
#65628=CARTESIAN_POINT ( 'NONE',  ( -0.05219959533937732626, 21.53943276465977519, 37.50109039468568284 ) ) ;
#65629=CARTESIAN_POINT ( 'NONE',  ( -19.49190055781009079, -5.500000000000054179, 45.56116087098781264 ) ) ;
#65630=CARTESIAN_POINT ( 'NONE',  ( 5.153800228976615827, -19.02544592524334988, 30.20942372801900433 ) ) ;
#65631=CARTESIAN_POINT ( 'NONE',  ( -19.03943276465977164, 0.05219959533909376836, 61.24890960531436690 ) ) ;
#65632=CARTESIAN_POINT ( 'NONE',  ( 19.05341960407617918, -5.049401038297876454, 36.04275706135234003 ) ) ;
#65633=CARTESIAN_POINT ( 'NONE',  ( 12.14591786802327356, -12.06949235617739191, 100.6260903946857184 ) ) ;
#65634=CARTESIAN_POINT ( 'NONE',  ( -10.72451020669898014, 18.67979575497178502, 25.41557627198103120 ) ) ;
#65635=CARTESIAN_POINT ( 'NONE',  ( 10.72451020669871369, 18.67979575497193778, 87.08442372801901854 ) ) ;
#65637=CARTESIAN_POINT ( 'NONE',  ( -17.49999999999998934, -4.640572885337524767, 34.36211835451161534 ) ) ;
#65638=CARTESIAN_POINT ( 'NONE',  ( 21.53943276465977519, 0.05219959533937863772, 91.25109039468568994 ) ) ;
#65639=VECTOR ( 'NONE', #43937, 1000.000000000000000 ) ;
#65641=CARTESIAN_POINT ( 'NONE',  ( -9.564922557960796823, -16.46253265017161027, 97.08224293864769550 ) ) ;
#65643=CARTESIAN_POINT ( 'NONE',  ( 19.03943276465977164, -0.05219959533909143690, 53.74890960531436690 ) ) ;
#65644=CARTESIAN_POINT ( 'NONE',  ( -10.81492255796078084, -18.62759615963271287, 52.08224293864768839 ) ) ;
#65645=CARTESIAN_POINT ( 'NONE',  ( 4.379528057220339221, -16.55341960407611168, 22.70724293864769194 ) ) ;
#65646=CARTESIAN_POINT ( 'NONE',  ( -8.224510206698948167, 14.34966873604960824, 95.41557627198102409 ) ) ;
#65647=CARTESIAN_POINT ( 'NONE',  ( 19.02544592524343514, -5.153800228976328945, 98.54057627198100988 ) ) ;
#65648=CARTESIAN_POINT ( 'NONE',  ( 16.51473224551083163, -9.474510206698727899, 20.83442372801899722 ) ) ;
#65649=CARTESIAN_POINT ( 'NONE',  ( -5.153800228976328057, -19.02544592524343514, 42.29057627198101699 ) ) ;
#65650=CARTESIAN_POINT ( 'NONE',  ( 8.314922557960818139, 14.29746914071049879, 99.58224293864770971 ) ) ;
#65651=CARTESIAN_POINT ( 'NONE',  ( 15.72974639402176855, 15.80617190586768217, 51.87609039468568284 ) ) ;
#65652=CARTESIAN_POINT ( 'NONE',  ( 8.224510206698742110, 14.34966873604972548, 107.0844237280190043 ) ) ;
#65653=CARTESIAN_POINT ( 'NONE',  ( 0.05219959533936267826, -19.03943276465977164, 65.00109039468567573 ) ) ;
#65655=CARTESIAN_POINT ( 'NONE',  ( 9.474510206698971260, -16.51473224551069308, 107.9155762719810383 ) ) ;
#65656=CARTESIAN_POINT ( 'NONE',  ( 16.53943276465976808, -0.05219959533910856209, 78.74890960531436690 ) ) ;
#65657=CARTESIAN_POINT ( 'NONE',  ( 9.564922557961047289, -16.46253265017146816, 40.41775706135234003 ) ) ;
#65658=CARTESIAN_POINT ( 'NONE',  ( -19.03943276465977164, 0.05219959533909376836, 66.24890960531436690 ) ) ;
#65659=CARTESIAN_POINT ( 'NONE',  ( 14.34966873604960469, 8.224510206698951720, 64.16557627198102409 ) ) ;
#65660=CARTESIAN_POINT ( 'NONE',  ( -16.51473224551082808, 9.474510206698731452, 83.33442372801899012 ) ) ;
#65661=CARTESIAN_POINT ( 'NONE',  ( 10.72451020669898902, -18.67979575497178502, 42.91557627198103120 ) ) ;
#65663=CARTESIAN_POINT ( 'NONE',  ( -12.06949235617756955, 12.14591786802309770, 105.6239096053143669 ) ) ;
#65664=CARTESIAN_POINT ( 'NONE',  ( -17.50000000000003908, -4.658240926743031807, 26.05529582183195103 ) ) ;
#65665=CARTESIAN_POINT ( 'NONE',  ( -5.049401038298153566, 19.05341960407611168, 55.20724293864769550 ) ) ;
#65666=CARTESIAN_POINT ( 'NONE',  ( -15.80617190586745835, -15.72974639402198527, 56.87390960531436690 ) ) ;
#65667=CARTESIAN_POINT ( 'NONE',  ( 16.51473224551069308, 9.474510206698969483, 49.16557627198102409 ) ) ;
#65668=CARTESIAN_POINT ( 'NONE',  ( 16.53943276465976808, 0.05219959533934440121, 96.25109039468568994 ) ) ;
#65669=CARTESIAN_POINT ( 'NONE',  ( -19.03943276465977164, 0.05219959533909376836, 76.24890960531435269 ) ) ;
#65670=CARTESIAN_POINT ( 'NONE',  ( -16.46253265017146816, -9.564922557961047289, 59.16775706135233293 ) ) ;
#65671=CARTESIAN_POINT ( 'NONE',  ( 15.72974639402176855, 15.80617190586768217, 71.87609039468568994 ) ) ;
#65672=CARTESIAN_POINT ( 'NONE',  ( 0.05219959533907565091, 21.53943276465977519, 44.99890960531435979 ) ) ;
#65673=CARTESIAN_POINT ( 'NONE',  ( -5.049401038298153566, 19.05341960407611168, 100.2072429386476955 ) ) ;
#65674=CARTESIAN_POINT ( 'NONE',  ( 9.564922557960805705, 16.46253265017160317, 24.58224293864769194 ) ) ;
#65675=CARTESIAN_POINT ( 'NONE',  ( -14.34966873604972548, 8.224510206698743886, 93.33442372801901854 ) ) ;
#65676=CARTESIAN_POINT ( 'NONE',  ( 16.46253265017146816, 9.564922557961045513, 101.6677570613523329 ) ) ;
#65679=CARTESIAN_POINT ( 'NONE',  ( -18.67979575497193778, 10.72451020669871902, 93.33442372801901854 ) ) ;
#65680=CARTESIAN_POINT ( 'NONE',  ( 12.06949235617757843, -12.14591786802309237, 63.12390960531435979 ) ) ;
#65681=CARTESIAN_POINT ( 'NONE',  ( 16.55341960407611168, 4.379528057220329451, 68.95724293864769550 ) ) ;
#65682=CARTESIAN_POINT ( 'NONE',  ( 21.53943276465977519, -0.05219959533907433946, 98.74890960531438111 ) ) ;
#65683=CARTESIAN_POINT ( 'NONE',  ( 5.719274019375991003, -21.55341960407610458, 82.70724293864770971 ) ) ;
#65684=CARTESIAN_POINT ( 'NONE',  ( 17.50000000000001066, -5.622605283950869115, 96.18792689403893803 ) ) ;
#65685=CARTESIAN_POINT ( 'NONE',  ( 15.80617190586746368, 15.72974639402197994, 39.37390960531436690 ) ) ;
#65686=CARTESIAN_POINT ( 'NONE',  ( 16.55341960407618274, -4.379528057220086978, 61.04275706135234714 ) ) ;
#65687=CARTESIAN_POINT ( 'NONE',  ( 16.52544592524342804, -4.483927247898539470, 88.54057627198103830 ) ) ;
#65688=CARTESIAN_POINT ( 'NONE',  ( 0.05219959533909260263, 19.03943276465977164, 49.99890960531435979 ) ) ;
#65690=CARTESIAN_POINT ( 'NONE',  ( 4.379528057220092307, 16.55341960407617563, 102.2927570613523613 ) ) ;
#65691=CARTESIAN_POINT ( 'NONE',  ( 21.53943276465977519, 0.05219959533937863772, 31.25109039468568639 ) ) ;
#65692=CARTESIAN_POINT ( 'NONE',  ( -19.03943276465977164, 0.05219959533909376836, 86.24890960531436690 ) ) ;
#65693=CARTESIAN_POINT ( 'NONE',  ( 5.823673210054444382, -21.52544592524334988, 65.20942372801901854 ) ) ;
#65694=CARTESIAN_POINT ( 'NONE',  ( 16.51473224551069308, 9.474510206698969483, 109.1655762719810383 ) ) ;
#65697=CARTESIAN_POINT ( 'NONE',  ( 21.53943276465977519, 0.05219959533937863772, 61.25109039468567573 ) ) ;
#65698=CARTESIAN_POINT ( 'NONE',  ( -13.97604488694527625, -13.89961937509977652, 36.87390960531436690 ) ) ;
#65699=CARTESIAN_POINT ( 'NONE',  ( 16.51473224551069308, 9.474510206698969483, 114.1655762719810241 ) ) ;
#65700=CARTESIAN_POINT ( 'NONE',  ( -16.46253265017146816, -9.564922557961047289, 64.16775706135233293 ) ) ;
#65701=CARTESIAN_POINT ( 'NONE',  ( -18.67979575497193778, 10.72451020669871902, 28.33442372801902209 ) ) ;
#65702=CARTESIAN_POINT ( 'NONE',  ( -13.97604488694547697, 13.89961937509957934, 53.12609039468565442 ) ) ;
#65703=CARTESIAN_POINT ( 'NONE',  ( 19.02544592524343514, -5.153800228976328945, 28.54057627198102409 ) ) ;
#65704=CARTESIAN_POINT ( 'NONE',  ( -0.05219959533934338120, 16.53943276465976808, 97.50109039468567573 ) ) ;
#65705=CARTESIAN_POINT ( 'NONE',  ( 19.03943276465977164, 0.05219959533936151252, 61.25109039468566863 ) ) ;
#65706=CARTESIAN_POINT ( 'NONE',  ( -14.34966873604972548, 8.224510206698743886, 113.3344237280190328 ) ) ;
#65707=CARTESIAN_POINT ( 'NONE',  ( 13.97604488694548053, -13.89961937509957401, 50.62609039468566152 ) ) ;
#65709=CARTESIAN_POINT ( 'NONE',  ( -9.564922557960796823, -16.46253265017161027, 92.08224293864769550 ) ) ;
#65710=CARTESIAN_POINT ( 'NONE',  ( -18.62759615963255300, -10.81492255796106328, 99.16775706135234714 ) ) ;
#65711=CARTESIAN_POINT ( 'NONE',  ( 15.80617190586769283, -15.72974639402175789, 110.6260903946857042 ) ) ;
#65713=CARTESIAN_POINT ( 'NONE',  ( -21.53943276465977519, -0.05219959533937600094, 88.75109039468567573 ) ) ;
#65714=CARTESIAN_POINT ( 'NONE',  ( -14.29746914071037622, -8.314922557961029526, 34.16775706135234714 ) ) ;
#65715=CARTESIAN_POINT ( 'NONE',  ( 5.049401038298161559, -19.05341960407611168, 87.70724293864769550 ) ) ;
#65716=CARTESIAN_POINT ( 'NONE',  ( -5.719274019375978568, 21.55341960407610458, 30.20724293864769550 ) ) ;
#65718=CARTESIAN_POINT ( 'NONE',  ( 16.46253265017160672, -9.564922557960803928, 83.33224293864768129 ) ) ;
#65719=CARTESIAN_POINT ( 'NONE',  ( -19.34837522270367671, -5.499999999999745981, 40.86337684832578532 ) ) ;
#65720=CARTESIAN_POINT ( 'NONE',  ( 5.153800228976615827, -19.02544592524334988, 75.20942372801896170 ) ) ;
#65721=CARTESIAN_POINT ( 'NONE',  ( -9.474510206698964154, 16.51473224551069663, 100.4155762719810241 ) ) ;
#65722=CARTESIAN_POINT ( 'NONE',  ( -5.823673210054431948, 21.52544592524334988, 102.7094237280190185 ) ) ;
#65723=CARTESIAN_POINT ( 'NONE',  ( 16.52544592524342804, -4.483927247898539470, 103.5405762719810383 ) ) ;
#65724=CARTESIAN_POINT ( 'NONE',  ( 10.81492255796078972, 18.62759615963270932, 44.58224293864769550 ) ) ;
#65725=CARTESIAN_POINT ( 'NONE',  ( -10.81492255796078084, -18.62759615963271287, 42.08224293864769550 ) ) ;
#65726=CARTESIAN_POINT ( 'NONE',  ( -12.06949235617756955, 12.14591786802309770, 100.6239096053143811 ) ) ;
#65728=CARTESIAN_POINT ( 'NONE',  ( 9.474510206698729675, 16.51473224551082808, 57.08442372801900433 ) ) ;
#65729=CARTESIAN_POINT ( 'NONE',  ( -8.314922557961024197, 14.29746914071037800, 112.9177570613523329 ) ) ;
#65730=CARTESIAN_POINT ( 'NONE',  ( -19.02544592524342804, 5.153800228976336051, 96.04057627198103830 ) ) ;
#65732=CARTESIAN_POINT ( 'NONE',  ( 5.823673210054444382, -21.52544592524334988, 85.20942372801901854 ) ) ;
#65733=CARTESIAN_POINT ( 'NONE',  ( 15.80617190586746368, 15.72974639402197994, 59.37390960531436690 ) ) ;
#65734=CARTESIAN_POINT ( 'NONE',  ( 10.81492255796106328, -18.62759615963255655, 50.41775706135235424 ) ) ;
#65735=CARTESIAN_POINT ( 'NONE',  ( 21.55341960407610458, 5.719274019375980345, 93.95724293864770971 ) ) ;
#65736=CARTESIAN_POINT ( 'NONE',  ( 21.55341960407619695, -5.719274019375665929, 41.04275706135236135 ) ) ;
#65737=CARTESIAN_POINT ( 'NONE',  ( -19.05341960407611168, -5.049401038298163336, 21.45724293864768839 ) ) ;
#65738=CARTESIAN_POINT ( 'NONE',  ( -5.153800228976328057, -19.02544592524343514, 87.29057627198103830 ) ) ;
#65739=CARTESIAN_POINT ( 'NONE',  ( -8.224510206698735004, -14.34966873604973081, 84.58442372801903275 ) ) ;
#65740=CARTESIAN_POINT ( 'NONE',  ( -0.05219959533910754901, -16.53943276465976808, 107.4989096053143669 ) ) ;
#65741=CARTESIAN_POINT ( 'NONE',  ( 9.474510206698971260, -16.51473224551069308, 112.9155762719810383 ) ) ;
#65742=CARTESIAN_POINT ( 'NONE',  ( -4.379528057220328563, 16.55341960407611168, 55.20724293864770260 ) ) ;
#65743=CARTESIAN_POINT ( 'NONE',  ( 12.06949235617739724, 12.14591786802326823, 111.8760903946856615 ) ) ;
#65744=CARTESIAN_POINT ( 'NONE',  ( 0.05219959533909260263, 19.03943276465977164, 54.99890960531435979 ) ) ;
#65745=CARTESIAN_POINT ( 'NONE',  ( 9.474510206698971260, -16.51473224551069308, 32.91557627198102409 ) ) ;
#65746=CARTESIAN_POINT ( 'NONE',  ( 21.55341960407610458, 5.719274019375980345, 48.95724293864770971 ) ) ;
#65747=CARTESIAN_POINT ( 'NONE',  ( 19.03943276465977164, 0.05219959533936151252, 21.25109039468565797 ) ) ;
#65749=CARTESIAN_POINT ( 'NONE',  ( -16.53943276465976808, 0.05219959533911058130, 36.24890960531435979 ) ) ;
#65750=CARTESIAN_POINT ( 'NONE',  ( 0.05219959533937995610, -21.53943276465977519, 50.00109039468568994 ) ) ;
#65751=CARTESIAN_POINT ( 'NONE',  ( -19.03943276465977164, 0.05219959533909376836, 116.2489096053143669 ) ) ;
#65752=CARTESIAN_POINT ( 'NONE',  ( 4.379528057220092307, 16.55341960407617563, 57.29275706135234714 ) ) ;
#65753=CARTESIAN_POINT ( 'NONE',  ( 9.564922557961047289, -16.46253265017146816, 65.41775706135233293 ) ) ;
#65755=CARTESIAN_POINT ( 'NONE',  ( -12.14591786802309592, -12.06949235617757132, 31.87390960531435979 ) ) ;
#65756=CARTESIAN_POINT ( 'NONE',  ( 14.34966873604972726, -8.224510206698740333, 110.8344237280190043 ) ) ;
#65757=CARTESIAN_POINT ( 'NONE',  ( -5.153800228976328057, -19.02544592524343514, 42.29057627198101699 ) ) ;
#65758=CARTESIAN_POINT ( 'NONE',  ( 0.05219959533909260263, 19.03943276465977164, 59.99890960531436690 ) ) ;
#65759=CARTESIAN_POINT ( 'NONE',  ( 16.51473224551069308, 9.474510206698969483, 24.16557627198102765 ) ) ;
#65760=CARTESIAN_POINT ( 'NONE',  ( 21.53943276465977519, 0.05219959533937863772, 36.25109039468567573 ) ) ;
#65761=CARTESIAN_POINT ( 'NONE',  ( -5.153800228976328057, -19.02544592524343514, 47.29057627198102409 ) ) ;
#65763=CARTESIAN_POINT ( 'NONE',  ( -5.049401038298153566, 19.05341960407611168, 40.20724293864768839 ) ) ;
#65764=CARTESIAN_POINT ( 'NONE',  ( 10.81492255796078972, 18.62759615963270932, 29.58224293864769905 ) ) ;
#65765=CARTESIAN_POINT ( 'NONE',  ( 18.67979575497194134, -10.72451020669871369, 55.83442372801901854 ) ) ;
#65766=CARTESIAN_POINT ( 'NONE',  ( 16.55341960407611168, 4.379528057220329451, 103.9572429386476813 ) ) ;
#65767=CARTESIAN_POINT ( 'NONE',  ( 5.049401038298161559, -19.05341960407611168, 107.7072429386476955 ) ) ;
#65768=VECTOR ( 'NONE', #136928, 1000.000000000000000 ) ;
#65769=CARTESIAN_POINT ( 'NONE',  ( -8.314922557961024197, 14.29746914071037800, 82.91775706135234714 ) ) ;
#65770=CARTESIAN_POINT ( 'NONE',  ( 18.62759615963255655, 10.81492255796105972, 86.66775706135234714 ) ) ;
#65771=CARTESIAN_POINT ( 'NONE',  ( -8.314922557961024197, 14.29746914071037800, 57.91775706135234714 ) ) ;
#65772=CARTESIAN_POINT ( 'NONE',  ( 13.89961937509977652, -13.97604488694527269, 98.12390960531433848 ) ) ;
#65773=CARTESIAN_POINT ( 'NONE',  ( 12.06949235617739724, 12.14591786802326823, 46.87609039468568994 ) ) ;
#65774=CARTESIAN_POINT ( 'NONE',  ( -4.379528057220086978, -16.55341960407618274, 24.79275706135235779 ) ) ;
#65775=CARTESIAN_POINT ( 'NONE',  ( 4.379528057220092307, 16.55341960407617563, 87.29275706135236135 ) ) ;
#65776=CARTESIAN_POINT ( 'NONE',  ( -0.05219959533936034679, 19.03943276465977164, 112.5010903946856757 ) ) ;
#65777=CARTESIAN_POINT ( 'NONE',  ( 21.52544592524344225, -5.823673210054117533, 98.54057627198105251 ) ) ;
#65778=CARTESIAN_POINT ( 'NONE',  ( 14.29746914071049879, -8.314922557960816363, 103.3322429386476955 ) ) ;
#65779=CARTESIAN_POINT ( 'NONE',  ( -19.02544592524334988, -5.153800228976617603, 98.95942372801900433 ) ) ;
#65780=CARTESIAN_POINT ( 'NONE',  ( 8.314922557961029526, -14.29746914071037800, 75.41775706135233293 ) ) ;
#65781=CARTESIAN_POINT ( 'NONE',  ( -16.29526858892908336, 7.335722546920052878, 44.20329402199734403 ) ) ;
#65782=CARTESIAN_POINT ( 'NONE',  ( -13.89961937509957401, -13.97604488694547875, 74.37609039468566152 ) ) ;
#65783=CARTESIAN_POINT ( 'NONE',  ( 16.52544592524342804, -4.483927247898539470, 48.54057627198103120 ) ) ;
#65784=CARTESIAN_POINT ( 'NONE',  ( 16.55341960407611168, 4.379528057220329451, 28.95724293864769905 ) ) ;
#65785=CARTESIAN_POINT ( 'NONE',  ( -4.379528057220328563, 16.55341960407611168, 90.20724293864770971 ) ) ;
#65786=CARTESIAN_POINT ( 'NONE',  ( -9.474510206698720793, -16.51473224551083518, 39.58442372801899722 ) ) ;
#65787=CARTESIAN_POINT ( 'NONE',  ( -17.26058549869092218, 6.457015423128481757, 88.62254162523936429 ) ) ;
#65788=CARTESIAN_POINT ( 'NONE',  ( -10.72451020669870658, -18.67979575497194134, 39.58442372801901143 ) ) ;
#65789=CARTESIAN_POINT ( 'NONE',  ( -5.153800228976607833, 19.02544592524334988, 92.70942372801901854 ) ) ;
#65791=CARTESIAN_POINT ( 'NONE',  ( -16.46253265017160317, 9.564922557960807481, 85.83224293864769550 ) ) ;
#65792=CARTESIAN_POINT ( 'NONE',  ( -19.03943276465977164, 0.05219959533909376836, 96.24890960531436690 ) ) ;
#65793=CARTESIAN_POINT ( 'NONE',  ( -15.72974639402197994, 15.80617190586746368, 50.62390960531435979 ) ) ;
#65794=CARTESIAN_POINT ( 'NONE',  ( 12.06949235617757843, -12.14591786802309237, 88.12390960531436690 ) ) ;
#65795=CARTESIAN_POINT ( 'NONE',  ( -13.97604488694527625, -13.89961937509977652, 76.87390960531433848 ) ) ;
#65796=CARTESIAN_POINT ( 'NONE',  ( -16.51473224551069308, -9.474510206698971260, 26.66557627198103120 ) ) ;
#65797=CARTESIAN_POINT ( 'NONE',  ( 5.719274019375673035, 21.55341960407619339, 37.29275706135235424 ) ) ;
#65798=CARTESIAN_POINT ( 'NONE',  ( 5.823673210054444382, -21.52544592524334988, 80.20942372801901854 ) ) ;
#65799=CARTESIAN_POINT ( 'NONE',  ( 19.05341960407611168, 5.049401038298154454, 58.95724293864768129 ) ) ;
#65801=CARTESIAN_POINT ( 'NONE',  ( -0.05219959533934338120, 16.53943276465976808, 82.50109039468568994 ) ) ;
#65802=CARTESIAN_POINT ( 'NONE',  ( 10.81492255796106328, -18.62759615963255655, 30.41775706135234358 ) ) ;
#65803=CARTESIAN_POINT ( 'NONE',  ( 18.67979575497194134, -10.72451020669871369, 30.83442372801902209 ) ) ;
#65804=CARTESIAN_POINT ( 'NONE',  ( -5.153800228976607833, 19.02544592524334988, 47.70942372801900433 ) ) ;
#65805=CARTESIAN_POINT ( 'NONE',  ( 0.05219959533909260263, 19.03943276465977164, 84.99890960531436690 ) ) ;
#65806=CARTESIAN_POINT ( 'NONE',  ( -9.474510206698720793, -16.51473224551083518, 34.58442372801899722 ) ) ;
#65807=CARTESIAN_POINT ( 'NONE',  ( -5.823673210054431948, 21.52544592524334988, 82.70942372801900433 ) ) ;
#65808=CARTESIAN_POINT ( 'NONE',  ( -10.81492255796078084, -18.62759615963271287, 67.08224293864770971 ) ) ;
#65809=CARTESIAN_POINT ( 'NONE',  ( -0.05219959533910754901, -16.53943276465976808, 57.49890960531435979 ) ) ;
#65810=CARTESIAN_POINT ( 'NONE',  ( -10.72451020669870658, -18.67979575497194134, 84.58442372801903275 ) ) ;
#65811=CARTESIAN_POINT ( 'NONE',  ( 5.153800228976615827, -19.02544592524334988, 25.20942372801900433 ) ) ;
#65812=CARTESIAN_POINT ( 'NONE',  ( -14.34966873604960291, -8.224510206698953496, 76.66557627198103830 ) ) ;
#65813=CARTESIAN_POINT ( 'NONE',  ( -14.34966873604960291, -8.224510206698953496, 111.6655762719810525 ) ) ;
#65814=CARTESIAN_POINT ( 'NONE',  ( -16.46253265017146816, -9.564922557961047289, 74.16775706135234714 ) ) ;
#65815=CARTESIAN_POINT ( 'NONE',  ( 14.34966873604960469, 8.224510206698951720, 34.16557627198102409 ) ) ;
#65816=CARTESIAN_POINT ( 'NONE',  ( -21.55341960407619339, 5.719274019375674811, 78.54275706135236135 ) ) ;
#65817=CARTESIAN_POINT ( 'NONE',  ( 19.02544592524343514, -5.153800228976328945, 73.54057627198103830 ) ) ;
#65818=CARTESIAN_POINT ( 'NONE',  ( -19.03943276465977164, -0.05219959533935918106, 53.75109039468566863 ) ) ;
#65819=CARTESIAN_POINT ( 'NONE',  ( 5.719274019375991003, -21.55341960407610458, 47.70724293864770260 ) ) ;
#65820=CARTESIAN_POINT ( 'NONE',  ( -0.05219959533907301413, -21.53943276465977519, 97.49890960531436690 ) ) ;
#65821=CARTESIAN_POINT ( 'NONE',  ( 14.34966873604972726, -8.224510206698740333, 20.83442372801901143 ) ) ;
#65822=CARTESIAN_POINT ( 'NONE',  ( -8.314922557961024197, 14.29746914071037800, 67.91775706135234714 ) ) ;
#65823=CARTESIAN_POINT ( 'NONE',  ( 16.20579543436681647, 7.371946100354970000, 63.06520834171877254 ) ) ;
#65824=CARTESIAN_POINT ( 'NONE',  ( -5.823673210054116645, -21.52544592524344225, 102.2905762719810383 ) ) ;
#65825=CARTESIAN_POINT ( 'NONE',  ( -8.224510206698948167, 14.34966873604960824, 105.4155762719810383 ) ) ;
#65826=CARTESIAN_POINT ( 'NONE',  ( -17.49999999999998934, -3.305555262949607886, 30.37482847843398659 ) ) ;
#65827=CARTESIAN_POINT ( 'NONE',  ( -14.29746914071037622, -8.314922557961029526, 39.16775706135235424 ) ) ;
#65828=CARTESIAN_POINT ( 'NONE',  ( 10.72451020669898902, -18.67979575497178502, 57.91557627198103120 ) ) ;
#65829=CARTESIAN_POINT ( 'NONE',  ( 4.483927247898790824, -16.52544592524335698, 110.2094237280190185 ) ) ;
#65830=CARTESIAN_POINT ( 'NONE',  ( -19.03943276465977164, 0.05219959533909376836, 31.24890960531435979 ) ) ;
#65831=CARTESIAN_POINT ( 'NONE',  ( 16.55341960407618274, -4.379528057220086978, 71.04275706135234714 ) ) ;
#65832=CARTESIAN_POINT ( 'NONE',  ( -0.05219959533936034679, 19.03943276465977164, 57.50109039468566863 ) ) ;
#65833=CARTESIAN_POINT ( 'NONE',  ( -15.72974639402176322, -15.80617190586768395, 39.37609039468567573 ) ) ;
#65834=CARTESIAN_POINT ( 'NONE',  ( 5.823673210054125526, 21.52544592524343514, 59.79057627198103120 ) ) ;
#65835=CARTESIAN_POINT ( 'NONE',  ( -14.34966873604972548, 8.224510206698743886, 98.33442372801901854 ) ) ;
#65836=CARTESIAN_POINT ( 'NONE',  ( 10.81492255796106328, -18.62759615963255655, 80.41775706135234714 ) ) ;
#65837=CARTESIAN_POINT ( 'NONE',  ( -18.67979575497178146, -10.72451020669898902, 46.66557627198102409 ) ) ;
#65838=CARTESIAN_POINT ( 'NONE',  ( -10.81492255796078084, -18.62759615963271287, 32.08224293864769550 ) ) ;
#65839=CARTESIAN_POINT ( 'NONE',  ( -16.53943276465976808, -0.05219959533934237506, 78.75109039468568994 ) ) ;
#65840=CARTESIAN_POINT ( 'NONE',  ( 21.52544592524344225, -5.823673210054117533, 38.54057627198103120 ) ) ;
#65841=ORIENTED_EDGE ( 'NONE', *, *, #9309, .T. ) ;
#65842=CARTESIAN_POINT ( 'NONE',  ( 9.474510206698971260, -16.51473224551069308, 97.91557627198102409 ) ) ;
#65843=CARTESIAN_POINT ( 'NONE',  ( -4.483927247898539470, -16.52544592524342804, 27.29057627198103120 ) ) ;
#65845=CARTESIAN_POINT ( 'NONE',  ( 12.06949235617757843, -12.14591786802309237, 108.1239096053143811 ) ) ;
#65846=CARTESIAN_POINT ( 'NONE',  ( 10.81492255796078972, 18.62759615963270932, 64.58224293864769550 ) ) ;
#65847=CARTESIAN_POINT ( 'NONE',  ( 12.14591786802327356, -12.06949235617739191, 85.62609039468568994 ) ) ;
#65848=CARTESIAN_POINT ( 'NONE',  ( 15.80617190586769283, -15.72974639402175789, 45.62609039468567573 ) ) ;
#65849=CARTESIAN_POINT ( 'NONE',  ( -16.51473224551082808, 9.474510206698731452, 103.3344237280190043 ) ) ;
#65850=CARTESIAN_POINT ( 'NONE',  ( -14.34966873604960291, -8.224510206698953496, 106.6655762719810383 ) ) ;
#65851=CARTESIAN_POINT ( 'NONE',  ( -13.97604488694547697, 13.89961937509957934, 108.1260903946856331 ) ) ;
#65852=CARTESIAN_POINT ( 'NONE',  ( -13.97604488694527625, -13.89961937509977652, 36.87390960531436690 ) ) ;
#65854=CARTESIAN_POINT ( 'NONE',  ( -5.049401038298153566, 19.05341960407611168, 90.20724293864766707 ) ) ;
#65855=CARTESIAN_POINT ( 'NONE',  ( -16.55341960407617563, 4.379528057220093196, 78.54275706135236135 ) ) ;
#65856=CARTESIAN_POINT ( 'NONE',  ( 21.52544592524334988, 5.823673210054432836, 101.4594237280190185 ) ) ;
#65857=CARTESIAN_POINT ( 'NONE',  ( 18.67979575497178502, 10.72451020669898547, 64.16557627198102409 ) ) ;
#65858=CARTESIAN_POINT ( 'NONE',  ( 4.483927247898790824, -16.52544592524335698, 85.20942372801901854 ) ) ;
#65859=VECTOR ( 'NONE', #26409, 1000.000000000000000 ) ;
#65860=CARTESIAN_POINT ( 'NONE',  ( -5.153800228976607833, 19.02544592524334988, 82.70942372801897591 ) ) ;
#65861=CARTESIAN_POINT ( 'NONE',  ( 19.03943276465977164, -0.05219959533909143690, 38.74890960531436690 ) ) ;
#65862=CARTESIAN_POINT ( 'NONE',  ( 9.564922557960805705, 16.46253265017160317, 79.58224293864769550 ) ) ;
#65863=CARTESIAN_POINT ( 'NONE',  ( 9.474510206698971260, -16.51473224551069308, 27.91557627198103120 ) ) ;
#65864=CARTESIAN_POINT ( 'NONE',  ( 9.474510206698729675, 16.51473224551082808, 67.08442372801900433 ) ) ;
#65866=CARTESIAN_POINT ( 'NONE',  ( -9.474510206698964154, 16.51473224551069663, 100.4155762719810241 ) ) ;
#65867=CARTESIAN_POINT ( 'NONE',  ( -0.05219959533910754901, -16.53943276465976808, 57.49890960531435979 ) ) ;
#65868=CARTESIAN_POINT ( 'NONE',  ( -0.05219959533907301413, -21.53943276465977519, 62.49890960531436690 ) ) ;
#65869=CARTESIAN_POINT ( 'NONE',  ( 17.97182807773874202, -5.499999999999957367, 91.03038844047289047 ) ) ;
#65870=CARTESIAN_POINT ( 'NONE',  ( -16.46253265017146816, -9.564922557961047289, 34.16775706135233293 ) ) ;
#65872=CARTESIAN_POINT ( 'NONE',  ( -13.97604488694527625, -13.89961937509977652, 56.87390960531434558 ) ) ;
#65873=CARTESIAN_POINT ( 'NONE',  ( 13.89961937509977652, -13.97604488694527269, 68.12390960531436690 ) ) ;
#65874=CARTESIAN_POINT ( 'NONE',  ( -16.52544592524335698, -4.483927247898792601, 38.95942372801901854 ) ) ;
#65877=CARTESIAN_POINT ( 'NONE',  ( 16.55341960407618274, -4.379528057220086978, 71.04275706135234714 ) ) ;
#65878=CARTESIAN_POINT ( 'NONE',  ( -14.34966873604972548, 8.224510206698743886, 68.33442372801900433 ) ) ;
#65879=CARTESIAN_POINT ( 'NONE',  ( -0.05219959533907301413, -21.53943276465977519, 97.49890960531436690 ) ) ;
#65880=CARTESIAN_POINT ( 'NONE',  ( 12.06949235617739724, 12.14591786802326823, 46.87609039468568994 ) ) ;
#65881=CARTESIAN_POINT ( 'NONE',  ( -9.564922557960796823, -16.46253265017161027, 42.08224293864769550 ) ) ;
#65883=CARTESIAN_POINT ( 'NONE',  ( 10.81492255796106328, -18.62759615963255655, 60.41775706135235424 ) ) ;
#65884=CARTESIAN_POINT ( 'NONE',  ( -9.564922557961040184, 16.46253265017147172, 62.91775706135233293 ) ) ;
#65885=CARTESIAN_POINT ( 'NONE',  ( 15.80617190586769283, -15.72974639402175789, 95.62609039468568994 ) ) ;
#65886=CARTESIAN_POINT ( 'NONE',  ( 19.03943276465977164, -0.05219959533909143690, 33.74890960531435979 ) ) ;
#65888=CARTESIAN_POINT ( 'NONE',  ( -18.67979575497178146, -10.72451020669898902, 56.66557627198103830 ) ) ;
#65889=CARTESIAN_POINT ( 'NONE',  ( 13.97604488694527802, 13.89961937509977652, 99.37390960531436690 ) ) ;
#65890=CARTESIAN_POINT ( 'NONE',  ( -16.52544592524342804, 4.483927247898546575, 101.0405762719810383 ) ) ;
#65891=CARTESIAN_POINT ( 'NONE',  ( 0.05219959533934541429, -16.53943276465976808, 40.00109039468567573 ) ) ;
#65892=CARTESIAN_POINT ( 'NONE',  ( -12.06949235617739369, -12.14591786802326823, 109.3760903946857042 ) ) ;
#65895=CARTESIAN_POINT ( 'NONE',  ( 21.55341960407610458, 5.719274019375980345, 98.95724293864770971 ) ) ;
#65896=CARTESIAN_POINT ( 'NONE',  ( -12.14591786802309592, -12.06949235617757132, 41.87390960531435979 ) ) ;
#65897=CARTESIAN_POINT ( 'NONE',  ( -9.474510206698964154, 16.51473224551069663, 110.4155762719810383 ) ) ;
#65898=CARTESIAN_POINT ( 'NONE',  ( -19.05341960407617563, 5.049401038297882671, 88.54275706135230450 ) ) ;
#65899=CARTESIAN_POINT ( 'NONE',  ( 19.05341960407617918, -5.049401038297876454, 31.04275706135232227 ) ) ;
#65900=CARTESIAN_POINT ( 'NONE',  ( -0.05219959533910754901, -16.53943276465976808, 32.49890960531435979 ) ) ;
#65901=CARTESIAN_POINT ( 'NONE',  ( -21.53943276465977519, 0.05219959533907696930, 96.24890960531435269 ) ) ;
#65902=CARTESIAN_POINT ( 'NONE',  ( -15.80617190586745835, -15.72974639402198527, 56.87390960531436690 ) ) ;
#65904=CARTESIAN_POINT ( 'NONE',  ( 9.564922557960805705, 16.46253265017160317, 69.58224293864770971 ) ) ;
#65905=CARTESIAN_POINT ( 'NONE',  ( 8.314922557960818139, 14.29746914071049879, 34.58224293864770260 ) ) ;
#65906=CARTESIAN_POINT ( 'NONE',  ( 5.049401038298161559, -19.05341960407611168, 92.70724293864769550 ) ) ;
#65908=CARTESIAN_POINT ( 'NONE',  ( 18.39443945427642291, -5.499999999999864997, 61.01745347608654413 ) ) ;
#65909=CARTESIAN_POINT ( 'NONE',  ( -5.153800228976607833, 19.02544592524334988, 42.70942372801901143 ) ) ;
#65910=CARTESIAN_POINT ( 'NONE',  ( -5.719274019375978568, 21.55341960407610458, 75.20724293864769550 ) ) ;
#65911=CARTESIAN_POINT ( 'NONE',  ( -4.483927247898539470, -16.52544592524342804, 102.2905762719810383 ) ) ;
#65913=CARTESIAN_POINT ( 'NONE',  ( 15.72974639402176855, 15.80617190586768217, 36.87609039468568994 ) ) ;
#65915=CARTESIAN_POINT ( 'NONE',  ( -16.52544592524335698, -4.483927247898792601, 108.9594237280190185 ) ) ;
#65916=CARTESIAN_POINT ( 'NONE',  ( -9.474510206698964154, 16.51473224551069663, 40.41557627198103120 ) ) ;
#65917=CARTESIAN_POINT ( 'NONE',  ( 5.153800228976335163, 19.02544592524342804, 84.79057627198099567 ) ) ;
#65919=CARTESIAN_POINT ( 'NONE',  ( -5.153800228976328057, -19.02544592524343514, 27.29057627198103120 ) ) ;
#65920=CARTESIAN_POINT ( 'NONE',  ( -4.379528057220328563, 16.55341960407611168, 40.20724293864769550 ) ) ;
#65921=CARTESIAN_POINT ( 'NONE',  ( 10.81492255796106328, -18.62759615963255655, 75.41775706135233293 ) ) ;
#65923=CARTESIAN_POINT ( 'NONE',  ( -4.483927247898782831, 16.52544592524335698, 72.70942372801901854 ) ) ;
#65924=CARTESIAN_POINT ( 'NONE',  ( -13.89961937509977652, 13.97604488694528158, 55.62390960531434558 ) ) ;
#65925=CARTESIAN_POINT ( 'NONE',  ( 0.05219959533909260263, 19.03943276465977164, 64.99890960531436690 ) ) ;
#65927=CARTESIAN_POINT ( 'NONE',  ( 21.52544592524334988, 5.823673210054432836, 111.4594237280190328 ) ) ;
#65928=CARTESIAN_POINT ( 'NONE',  ( -16.55341960407617563, 4.379528057220093196, 68.54275706135234714 ) ) ;
#65929=CARTESIAN_POINT ( 'NONE',  ( -5.823673210054431948, 21.52544592524334988, 97.70942372801904696 ) ) ;
#65930=CARTESIAN_POINT ( 'NONE',  ( -19.05341960407611168, -5.049401038298163336, 56.45724293864768129 ) ) ;
#65931=CARTESIAN_POINT ( 'NONE',  ( 10.81492255796078972, 18.62759615963270932, 34.58224293864770260 ) ) ;
#65932=CARTESIAN_POINT ( 'NONE',  ( 9.564922557961047289, -16.46253265017146816, 105.4177570613523471 ) ) ;
#65933=CARTESIAN_POINT ( 'NONE',  ( -5.823673210054431948, 21.52544592524334988, 62.70942372801902565 ) ) ;
#65934=CARTESIAN_POINT ( 'NONE',  ( -8.224510206698735004, -14.34966873604973081, 54.58442372801901143 ) ) ;
#65935=CARTESIAN_POINT ( 'NONE',  ( -21.55341960407610458, -5.719274019375992779, 96.45724293864770971 ) ) ;
#65936=CARTESIAN_POINT ( 'NONE',  ( -13.89961937509957401, -13.97604488694547875, 104.3760903946856757 ) ) ;
#65937=CARTESIAN_POINT ( 'NONE',  ( 0.05219959533909260263, 19.03943276465977164, 74.99890960531435269 ) ) ;
#65938=CARTESIAN_POINT ( 'NONE',  ( -14.29746914071037622, -8.314922557961029526, 19.16775706135234714 ) ) ;
#65940=CARTESIAN_POINT ( 'NONE',  ( 19.05341960407617918, -5.049401038297876454, 106.0427570613523471 ) ) ;
#65941=CARTESIAN_POINT ( 'NONE',  ( -8.314922557960811034, -14.29746914071050412, 62.08224293864769550 ) ) ;
#65942=CARTESIAN_POINT ( 'NONE',  ( 8.224510206698742110, 14.34966873604972548, 77.08442372801901854 ) ) ;
#65943=CARTESIAN_POINT ( 'NONE',  ( 15.72974639402176855, 15.80617190586768217, 21.87609039468567573 ) ) ;
#65944=CARTESIAN_POINT ( 'NONE',  ( -5.049401038298153566, 19.05341960407611168, 55.20724293864769550 ) ) ;
#65945=CARTESIAN_POINT ( 'NONE',  ( -19.03943276465977164, 0.05219959533909376836, 61.24890960531436690 ) ) ;
#65946=CARTESIAN_POINT ( 'NONE',  ( 12.14591786802327356, -12.06949235617739191, 75.62609039468567573 ) ) ;
#65949=CARTESIAN_POINT ( 'NONE',  ( 0.05219959533937995610, -21.53943276465977519, 110.0010903946856757 ) ) ;
#65952=CARTESIAN_POINT ( 'NONE',  ( 0.05219959533936267826, -19.03943276465977164, 105.0010903946856615 ) ) ;
#65953=CARTESIAN_POINT ( 'NONE',  ( 18.62759615963271287, -10.81492255796078972, 48.33224293864770260 ) ) ;
#65954=CARTESIAN_POINT ( 'NONE',  ( -19.05341960407617563, 5.049401038297882671, 38.54275706135233293 ) ) ;
#65955=CARTESIAN_POINT ( 'NONE',  ( -4.483927247898782831, 16.52544592524335698, 22.70942372801901499 ) ) ;
#65956=CARTESIAN_POINT ( 'NONE',  ( 13.89961937509977652, -13.97604488694527269, 43.12390960531434558 ) ) ;
#65957=CARTESIAN_POINT ( 'NONE',  ( -19.03943276465977164, 0.05219959533909376836, 66.24890960531436690 ) ) ;
#65958=CARTESIAN_POINT ( 'NONE',  ( 15.80617190586746368, 15.72974639402197994, 84.37390960531438111 ) ) ;
#65959=CARTESIAN_POINT ( 'NONE',  ( -9.564922557960796823, -16.46253265017161027, 112.0822429386476955 ) ) ;
#65960=CARTESIAN_POINT ( 'NONE',  ( 5.153800228976335163, 19.02544592524342804, 49.79057627198100988 ) ) ;
#65962=CARTESIAN_POINT ( 'NONE',  ( 16.46253265017146816, 9.564922557961045513, 96.66775706135233293 ) ) ;
#65963=CARTESIAN_POINT ( 'NONE',  ( -16.52544592524342804, 4.483927247898546575, 66.04057627198103830 ) ) ;
#65964=CARTESIAN_POINT ( 'NONE',  ( 9.564922557961047289, -16.46253265017146816, 25.41775706135234003 ) ) ;
#65966=CARTESIAN_POINT ( 'NONE',  ( -0.05219959533910754901, -16.53943276465976808, 57.49890960531435979 ) ) ;
#65967=CARTESIAN_POINT ( 'NONE',  ( -18.67979575497193778, 10.72451020669871902, 83.33442372801903275 ) ) ;
#65968=CARTESIAN_POINT ( 'NONE',  ( 5.049401038298161559, -19.05341960407611168, 32.70724293864768129 ) ) ;
#65969=CARTESIAN_POINT ( 'NONE',  ( -10.81492255796105439, 18.62759615963255655, 92.91775706135236135 ) ) ;
#65970=CARTESIAN_POINT ( 'NONE',  ( -14.34966873604960291, -8.224510206698953496, 26.66557627198103475 ) ) ;
#65971=CARTESIAN_POINT ( 'NONE',  ( -10.81492255796105439, 18.62759615963255655, 77.91775706135231871 ) ) ;
#65972=CARTESIAN_POINT ( 'NONE',  ( -13.89961937509977652, 13.97604488694528158, 65.62390960531436690 ) ) ;
#65974=CARTESIAN_POINT ( 'NONE',  ( -5.719274019375665041, -21.55341960407619695, 44.79275706135234714 ) ) ;
#65975=CARTESIAN_POINT ( 'NONE',  ( -13.89961937509977652, 13.97604488694528158, 85.62390960531433848 ) ) ;
#65976=CARTESIAN_POINT ( 'NONE',  ( 4.379528057220339221, -16.55341960407611168, 97.70724293864772392 ) ) ;
#65977=CARTESIAN_POINT ( 'NONE',  ( -16.55341960407611168, -4.379528057220339221, 66.45724293864768129 ) ) ;
#65978=CARTESIAN_POINT ( 'NONE',  ( -21.52544592524343514, 5.823673210054127303, 66.04057627198103830 ) ) ;
#65979=CARTESIAN_POINT ( 'NONE',  ( 9.474510206698971260, -16.51473224551069308, 72.91557627198102409 ) ) ;
#65980=CARTESIAN_POINT ( 'NONE',  ( 21.53943276465977519, -0.05219959533907433946, 83.74890960531435269 ) ) ;
#65981=CARTESIAN_POINT ( 'NONE',  ( 5.049401038297881783, 19.05341960407617563, 67.29275706135234714 ) ) ;
#65982=CARTESIAN_POINT ( 'NONE',  ( -16.51473224551082808, 9.474510206698731452, 38.33442372801899722 ) ) ;
#65983=CARTESIAN_POINT ( 'NONE',  ( -4.379528057220328563, 16.55341960407611168, 80.20724293864769550 ) ) ;
#65984=CARTESIAN_POINT ( 'NONE',  ( 10.72451020669898902, -18.67979575497178502, 47.91557627198102409 ) ) ;
#65986=CARTESIAN_POINT ( 'NONE',  ( -4.483927247898782831, 16.52544592524335698, 92.70942372801901854 ) ) ;
#65988=CARTESIAN_POINT ( 'NONE',  ( 9.474510206698729675, 16.51473224551082808, 107.0844237280190043 ) ) ;
#65989=EDGE_CURVE ( 'NONE', #134824, #103535, #22203, .T. ) ;
#65990=CARTESIAN_POINT ( 'NONE',  ( -12.14591786802309592, -12.06949235617757132, 61.87390960531436690 ) ) ;
#65992=CARTESIAN_POINT ( 'NONE',  ( 5.153800228976335163, 19.02544592524342804, 54.79057627198103120 ) ) ;
#65993=CARTESIAN_POINT ( 'NONE',  ( -8.224510206698948167, 14.34966873604960824, 55.41557627198102409 ) ) ;
#65994=CARTESIAN_POINT ( 'NONE',  ( 13.97604488694527802, 13.89961937509977652, 99.37390960531436690 ) ) ;
#65995=CARTESIAN_POINT ( 'NONE',  ( -19.05341960407617563, 5.049401038297882671, 78.54275706135233293 ) ) ;
#65996=CARTESIAN_POINT ( 'NONE',  ( 0.05219959533909260263, 19.03943276465977164, 64.99890960531436690 ) ) ;
#65997=CARTESIAN_POINT ( 'NONE',  ( 13.89961937509977652, -13.97604488694527269, 83.12390960531436690 ) ) ;
#65998=CARTESIAN_POINT ( 'NONE',  ( -5.049401038298153566, 19.05341960407611168, 90.20724293864766707 ) ) ;
#65999=CARTESIAN_POINT ( 'NONE',  ( -10.81492255796078084, -18.62759615963271287, 62.08224293864769550 ) ) ;
#66000=CARTESIAN_POINT ( 'NONE',  ( 14.34966873604972726, -8.224510206698740333, 60.83442372801901854 ) ) ;
#66001=CARTESIAN_POINT ( 'NONE',  ( 5.049401038297881783, 19.05341960407617918, 102.2927570613523187 ) ) ;
#66002=CARTESIAN_POINT ( 'NONE',  ( -16.51473224551069308, -9.474510206698971260, 46.66557627198102409 ) ) ;
#66003=CARTESIAN_POINT ( 'NONE',  ( -10.81492255796078084, -18.62759615963271287, 52.08224293864768839 ) ) ;
#66004=CARTESIAN_POINT ( 'NONE',  ( -16.46253265017146816, -9.564922557961047289, 99.16775706135233293 ) ) ;
#66006=CARTESIAN_POINT ( 'NONE',  ( 4.379528057220339221, -16.55341960407611168, 27.70724293864769905 ) ) ;
#66007=CARTESIAN_POINT ( 'NONE',  ( 10.72451020669871369, 18.67979575497193778, 47.08442372801901854 ) ) ;
#66008=CARTESIAN_POINT ( 'NONE',  ( 19.02544592524334988, 5.153800228976608722, 36.45942372801900433 ) ) ;
#66009=CARTESIAN_POINT ( 'NONE',  ( 8.314922557961029526, -14.29746914071037800, 55.41775706135234714 ) ) ;
#66010=CARTESIAN_POINT ( 'NONE',  ( 16.55341960407618274, -4.379528057220086978, 91.04275706135236135 ) ) ;
#66011=CARTESIAN_POINT ( 'NONE',  ( -17.49999999999999645, 5.499999999999992895, 53.71769037696436300 ) ) ;
#66012=CARTESIAN_POINT ( 'NONE',  ( 4.379528057220092307, 16.55341960407617563, 87.29275706135236135 ) ) ;
#66013=CARTESIAN_POINT ( 'NONE',  ( 4.483927247898790824, -16.52544592524335698, 30.20942372801902565 ) ) ;
#66014=CARTESIAN_POINT ( 'NONE',  ( 9.474510206698971260, -16.51473224551069308, 42.91557627198103120 ) ) ;
#66015=CARTESIAN_POINT ( 'NONE',  ( 13.89961937509977652, -13.97604488694527269, 48.12390960531435979 ) ) ;
#66016=CARTESIAN_POINT ( 'NONE',  ( -19.02544592524342804, 5.153800228976336051, 61.04057627198103120 ) ) ;
#66017=CARTESIAN_POINT ( 'NONE',  ( -21.55341960407619339, 5.719274019375674811, 53.54275706135234714 ) ) ;
#66018=CARTESIAN_POINT ( 'NONE',  ( -16.55341960407617563, 4.379528057220093196, 43.54275706135235424 ) ) ;
#66019=CARTESIAN_POINT ( 'NONE',  ( 0.05219959533934541429, -16.53943276465976808, 110.0010903946856757 ) ) ;
#66020=CARTESIAN_POINT ( 'NONE',  ( 16.46253265017160672, -9.564922557960803928, 28.33224293864769550 ) ) ;
#66021=CARTESIAN_POINT ( 'NONE',  ( -5.153800228976607833, 19.02544592524334988, 22.70942372801899012 ) ) ;
#66022=CARTESIAN_POINT ( 'NONE',  ( 16.53943276465976808, 0.05219959533934440121, 21.25109039468567218 ) ) ;
#66024=CARTESIAN_POINT ( 'NONE',  ( 5.153800228976615827, -19.02544592524334988, 75.20942372801896170 ) ) ;
#66025=CARTESIAN_POINT ( 'NONE',  ( -4.379528057220328563, 16.55341960407611168, 85.20724293864770971 ) ) ;
#66026=CARTESIAN_POINT ( 'NONE',  ( 19.05341960407611168, 5.049401038298154454, 38.95724293864767418 ) ) ;
#66027=CARTESIAN_POINT ( 'NONE',  ( -16.46253265017146816, -9.564922557961047289, 79.16775706135234714 ) ) ;
#66028=CARTESIAN_POINT ( 'NONE',  ( 16.61371651742601685, -7.165104196376144152, 91.35415069992995996 ) ) ;
#66029=CARTESIAN_POINT ( 'NONE',  ( -5.823673210054431948, 21.52544592524334988, 82.70942372801900433 ) ) ;
#66030=CARTESIAN_POINT ( 'NONE',  ( -12.14591786802326823, 12.06949235617739902, 43.12609039468568284 ) ) ;
#66032=CARTESIAN_POINT ( 'NONE',  ( 21.53943276465977519, -0.05219959533907433946, 38.74890960531435979 ) ) ;
#66033=CARTESIAN_POINT ( 'NONE',  ( -12.14591786802326823, 12.06949235617739902, 28.12609039468568284 ) ) ;
#66034=CARTESIAN_POINT ( 'NONE',  ( 13.89961937509978007, -13.97604488694527269, 23.12390960531435979 ) ) ;
#66035=CARTESIAN_POINT ( 'NONE',  ( -9.564922557961040184, 16.46253265017147172, 32.91775706135233293 ) ) ;
#66037=CARTESIAN_POINT ( 'NONE',  ( 16.46253265017160672, -9.564922557960803928, 43.33224293864769550 ) ) ;
#66039=CARTESIAN_POINT ( 'NONE',  ( -9.564922557960796823, -16.46253265017161027, 72.08224293864770971 ) ) ;
#66040=CARTESIAN_POINT ( 'NONE',  ( -19.01533133064923575, 5.499999999999444000, 98.76586590595738357 ) ) ;
#66041=CARTESIAN_POINT ( 'NONE',  ( -16.51473224551082808, 9.474510206698731452, 23.33442372801900078 ) ) ;
#66042=CARTESIAN_POINT ( 'NONE',  ( 0.05219959533910956823, 16.53943276465976808, 34.99890960531435979 ) ) ;
#66043=CARTESIAN_POINT ( 'NONE',  ( -19.02544592524342804, 5.153800228976336051, 46.04057627198101699 ) ) ;
#66044=CARTESIAN_POINT ( 'NONE',  ( 5.049401038298161559, -19.05341960407611168, 97.70724293864766707 ) ) ;
#66045=CARTESIAN_POINT ( 'NONE',  ( -0.05219959533937732626, 21.53943276465977519, 72.50109039468568994 ) ) ;
#66046=CARTESIAN_POINT ( 'NONE',  ( 19.02544592524343514, -5.153800228976328945, 48.54057627198103120 ) ) ;
#66047=CARTESIAN_POINT ( 'NONE',  ( -10.72451020669870658, -18.67979575497194134, 64.58442372801900433 ) ) ;
#66048=CARTESIAN_POINT ( 'NONE',  ( 19.05341960407611168, 5.049401038298154454, 113.9572429386477097 ) ) ;
#66049=CARTESIAN_POINT ( 'NONE',  ( 13.97604488694527802, 13.89961937509977652, 29.37390960531435979 ) ) ;
#66050=CARTESIAN_POINT ( 'NONE',  ( 5.719274019375991003, -21.55341960407610458, 112.7072429386476955 ) ) ;
#66051=CARTESIAN_POINT ( 'NONE',  ( -16.46253265017146816, -9.564922557961047289, 29.16775706135232937 ) ) ;
#66052=CARTESIAN_POINT ( 'NONE',  ( -16.53943276465976808, 0.05219959533911058130, 106.2489096053143811 ) ) ;
#66053=CARTESIAN_POINT ( 'NONE',  ( -0.05219959533909027116, -19.03943276465977164, 67.49890960531436690 ) ) ;
#66054=CARTESIAN_POINT ( 'NONE',  ( -19.05341960407617563, 5.049401038297882671, 113.5427570613523471 ) ) ;
#66055=AXIS2_PLACEMENT_3D ( 'NONE', #196597, #27747, #103577 ) ;
#66056=CARTESIAN_POINT ( 'NONE',  ( 14.34966873604960469, 8.224510206698951720, 74.16557627198102409 ) ) ;
#66057=CARTESIAN_POINT ( 'NONE',  ( -16.46253265017160317, 9.564922557960807481, 115.8322429386477097 ) ) ;
#66058=CARTESIAN_POINT ( 'NONE',  ( 19.02544592524334988, 5.153800228976608722, 86.45942372801900433 ) ) ;
#66059=CARTESIAN_POINT ( 'NONE',  ( 15.72974639402199770, -15.80617190586745480, 88.12390960531436690 ) ) ;
#66060=CARTESIAN_POINT ( 'NONE',  ( 21.53943276465977519, 0.05219959533937863772, 61.25109039468567573 ) ) ;
#66061=CARTESIAN_POINT ( 'NONE',  ( -0.05219959533934338120, 16.53943276465976808, 62.50109039468568284 ) ) ;
#66062=CARTESIAN_POINT ( 'NONE',  ( 14.34966873604972726, -8.224510206698740333, 55.83442372801901854 ) ) ;
#66063=CARTESIAN_POINT ( 'NONE',  ( 0.05219959533907565091, 21.53943276465977519, 59.99890960531436690 ) ) ;
#66065=CARTESIAN_POINT ( 'NONE',  ( -19.02544592524342804, 5.153800228976336051, 46.04057627198101699 ) ) ;
#66067=CARTESIAN_POINT ( 'NONE',  ( 14.29746914071037800, 8.314922557961029526, 81.66775706135236135 ) ) ;
#66068=CARTESIAN_POINT ( 'NONE',  ( -21.53943276465977519, 0.05219959533907696930, 101.2489096053143669 ) ) ;
#66069=CARTESIAN_POINT ( 'NONE',  ( 0.05219959533910956823, 16.53943276465976808, 49.99890960531437401 ) ) ;
#66070=CARTESIAN_POINT ( 'NONE',  ( -16.53943276465976808, -0.05219959533934237506, 58.75109039468568994 ) ) ;
#66071=CARTESIAN_POINT ( 'NONE',  ( 16.46253265017146816, 9.564922557961045513, 106.6677570613523471 ) ) ;
#66072=CARTESIAN_POINT ( 'NONE',  ( 21.52544592524344225, -5.823673210054117533, 93.54057627198103830 ) ) ;
#66073=CARTESIAN_POINT ( 'NONE',  ( -12.06949235617756955, 12.14591786802309770, 50.62390960531435979 ) ) ;
#66075=CARTESIAN_POINT ( 'NONE',  ( -17.44270441346519362, 5.991230190322972327, 68.63664920735773478 ) ) ;
#66076=CARTESIAN_POINT ( 'NONE',  ( 21.55341960407610458, 5.719274019375980345, 78.95724293864769550 ) ) ;
#66077=CARTESIAN_POINT ( 'NONE',  ( 8.224510206698953496, -14.34966873604960469, 27.91557627198103830 ) ) ;
#66080=CARTESIAN_POINT ( 'NONE',  ( -0.05219959533907301413, -21.53943276465977519, 102.4989096053143811 ) ) ;
#66081=CARTESIAN_POINT ( 'NONE',  ( -18.67979575497193778, 10.72451020669871902, 23.33442372801901499 ) ) ;
#66082=CARTESIAN_POINT ( 'NONE',  ( 14.29746914071049879, -8.314922557960816363, 33.33224293864769550 ) ) ;
#66084=CARTESIAN_POINT ( 'NONE',  ( -14.34966873604972548, 8.224510206698743886, 48.33442372801902565 ) ) ;
#66085=CARTESIAN_POINT ( 'NONE',  ( 13.97604488694527802, 13.89961937509977652, 49.37390960531434558 ) ) ;
#66086=CARTESIAN_POINT ( 'NONE',  ( -19.05341960407611168, -5.049401038298163336, 81.45724293864769550 ) ) ;
#66088=CARTESIAN_POINT ( 'NONE',  ( -18.62759615963270932, 10.81492255796079327, 30.83224293864770260 ) ) ;
#66089=CARTESIAN_POINT ( 'NONE',  ( -13.89961937509977830, 13.97604488694528158, 65.62390960531436690 ) ) ;
#66090=CARTESIAN_POINT ( 'NONE',  ( 4.379528057220092307, 16.55341960407617563, 22.29275706135235069 ) ) ;
#66091=CARTESIAN_POINT ( 'NONE',  ( -13.89961937509957401, -13.97604488694547875, 49.37609039468567573 ) ) ;
#66092=CARTESIAN_POINT ( 'NONE',  ( -10.81492255796078084, -18.62759615963271287, 97.08224293864770971 ) ) ;
#66093=CARTESIAN_POINT ( 'NONE',  ( 14.34966873604960469, 8.224510206698951720, 39.16557627198102409 ) ) ;
#66094=CARTESIAN_POINT ( 'NONE',  ( 16.46253265017160672, -9.564922557960803928, 78.33224293864769550 ) ) ;
#66095=CARTESIAN_POINT ( 'NONE',  ( -5.823673210054116645, -21.52544592524344225, 57.29057627198103120 ) ) ;
#66096=CARTESIAN_POINT ( 'NONE',  ( -10.81492255796078084, -18.62759615963271287, 97.08224293864770971 ) ) ;
#66097=CARTESIAN_POINT ( 'NONE',  ( -19.05341960407617563, 5.049401038297882671, 113.5427570613523471 ) ) ;
#66099=CARTESIAN_POINT ( 'NONE',  ( 5.719274019375991003, -21.55341960407610458, 27.70724293864769905 ) ) ;
#66100=CARTESIAN_POINT ( 'NONE',  ( -18.67979575497193778, 10.72451020669871902, 83.33442372801903275 ) ) ;
#66101=CARTESIAN_POINT ( 'NONE',  ( -5.153800228976328057, -19.02544592524343514, 72.29057627198102409 ) ) ;
#66102=CARTESIAN_POINT ( 'NONE',  ( -13.89961937509977652, 13.97604488694528158, 30.62390960531435269 ) ) ;
#66103=CARTESIAN_POINT ( 'NONE',  ( -13.97604488694527625, -13.89961937509977652, 81.87390960531436690 ) ) ;
#66104=CARTESIAN_POINT ( 'NONE',  ( -8.224510206698948167, 14.34966873604960824, 100.4155762719810241 ) ) ;
#66105=ORIENTED_EDGE ( 'NONE', *, *, #89035, .T. ) ;
#66106=CARTESIAN_POINT ( 'NONE',  ( 5.153800228976615827, -19.02544592524334988, 105.2094237280190185 ) ) ;
#66108=CARTESIAN_POINT ( 'NONE',  ( -0.05219959533909027116, -19.03943276465977164, 72.49890960531435269 ) ) ;
#66109=CARTESIAN_POINT ( 'NONE',  ( -18.62759615963255300, -10.81492255796106328, 99.16775706135234714 ) ) ;
#66110=CARTESIAN_POINT ( 'NONE',  ( -19.05341960407611168, -5.049401038298163336, 111.4572429386476671 ) ) ;
#66111=CARTESIAN_POINT ( 'NONE',  ( 14.34966873604972726, -8.224510206698740333, 90.83442372801901854 ) ) ;
#66113=CARTESIAN_POINT ( 'NONE',  ( -16.31925111598454947, -7.325300261831594106, 74.83575461032751264 ) ) ;
#66114=CARTESIAN_POINT ( 'NONE',  ( -19.05341960407617563, 5.049401038297882671, 63.54275706135234003 ) ) ;
#66115=CARTESIAN_POINT ( 'NONE',  ( 5.823673210054444382, -21.52544592524334988, 110.2094237280190185 ) ) ;
#66117=CARTESIAN_POINT ( 'NONE',  ( -9.564922557960796823, -16.46253265017161027, 22.08224293864768839 ) ) ;
#66118=CARTESIAN_POINT ( 'NONE',  ( 12.14591786802309770, 12.06949235617756955, 29.37390960531435269 ) ) ;
#66120=CARTESIAN_POINT ( 'NONE',  ( 14.29746914071037800, 8.314922557961029526, 106.6677570613523756 ) ) ;
#66121=CARTESIAN_POINT ( 'NONE',  ( -18.22780087662123094, -5.499999999999984901, 86.48459894673892734 ) ) ;
#66122=CARTESIAN_POINT ( 'NONE',  ( -4.483927247898782831, 16.52544592524335698, 87.70942372801901854 ) ) ;
#66123=CARTESIAN_POINT ( 'NONE',  ( 19.05341960407611168, 5.049401038298154454, 28.95724293864769550 ) ) ;
#66124=CARTESIAN_POINT ( 'NONE',  ( 21.53943276465977519, 0.05219959533937863772, 91.25109039468568994 ) ) ;
#66125=CARTESIAN_POINT ( 'NONE',  ( -19.03943276465977164, -0.05219959533935918106, 103.7510903946856757 ) ) ;
#66126=CARTESIAN_POINT ( 'NONE',  ( -18.67979575497193778, 10.72451020669871902, 63.33442372801900433 ) ) ;
#66127=CARTESIAN_POINT ( 'NONE',  ( 5.049401038297881783, 19.05341960407617563, 37.29275706135232582 ) ) ;
#66128=CARTESIAN_POINT ( 'NONE',  ( 19.05341960407611168, 5.049401038298154454, 83.95724293864766707 ) ) ;
#66129=CARTESIAN_POINT ( 'NONE',  ( -19.03943276465977164, 0.05219959533909376836, 76.24890960531435269 ) ) ;
#66131=CARTESIAN_POINT ( 'NONE',  ( -15.80617190586745835, -15.72974639402198527, 41.87390960531435979 ) ) ;
#66132=CARTESIAN_POINT ( 'NONE',  ( -13.97604488694527625, -13.89961937509977652, 51.87390960531436690 ) ) ;
#66133=CARTESIAN_POINT ( 'NONE',  ( -14.34966873604972548, 8.224510206698743886, 78.33442372801901854 ) ) ;
#66134=ORIENTED_EDGE ( 'NONE', *, *, #135901, .F. ) ;
#66137=CARTESIAN_POINT ( 'NONE',  ( 8.224510206698953496, -14.34966873604960469, 72.91557627198103830 ) ) ;
#66139=CARTESIAN_POINT ( 'NONE',  ( 4.483927247898790824, -16.52544592524335698, 40.20942372801901854 ) ) ;
#66140=CARTESIAN_POINT ( 'NONE',  ( -5.153800228976328057, -19.02544592524343514, 22.29057627198102765 ) ) ;
#66141=CARTESIAN_POINT ( 'NONE',  ( 5.049401038297881783, 19.05341960407617563, 62.29275706135234003 ) ) ;
#66142=CARTESIAN_POINT ( 'NONE',  ( -8.314922557960811034, -14.29746914071050412, 67.08224293864770971 ) ) ;
#66143=CARTESIAN_POINT ( 'NONE',  ( -21.55341960407619339, 5.719274019375674811, 28.54275706135234358 ) ) ;
#66144=CARTESIAN_POINT ( 'NONE',  ( -16.46253265017160317, 9.564922557960807481, 25.83224293864769194 ) ) ;
#66145=CARTESIAN_POINT ( 'NONE',  ( -18.67979575497178146, -10.72451020669898902, 86.66557627198102409 ) ) ;
#66146=CARTESIAN_POINT ( 'NONE',  ( -13.89961937509977652, 13.97604488694528158, 115.6239096053143669 ) ) ;
#66147=CARTESIAN_POINT ( 'NONE',  ( -8.224510206698948167, 14.34966873604960824, 70.41557627198102409 ) ) ;
#66149=CARTESIAN_POINT ( 'NONE',  ( -13.89961937509977652, 13.97604488694528158, 50.62390960531435979 ) ) ;
#66151=CARTESIAN_POINT ( 'NONE',  ( 5.049401038297881783, 19.05341960407617563, 87.29275706135234714 ) ) ;
#66152=CARTESIAN_POINT ( 'NONE',  ( 21.53943276465977519, 0.05219959533937863772, 21.25109039468567218 ) ) ;
#66153=CARTESIAN_POINT ( 'NONE',  ( -9.564922557960796823, -16.46253265017161027, 67.08224293864769550 ) ) ;
#66154=CARTESIAN_POINT ( 'NONE',  ( -19.02544592524334988, -5.153800228976617603, 58.95942372801900433 ) ) ;
#66155=CARTESIAN_POINT ( 'NONE',  ( -5.049401038298153566, 19.05341960407611168, 40.20724293864768839 ) ) ;
#66156=CARTESIAN_POINT ( 'NONE',  ( -12.06949235617756955, 12.14591786802309770, 65.62390960531436690 ) ) ;
#66157=CARTESIAN_POINT ( 'NONE',  ( 16.52544592524342804, -4.483927247898539470, 48.54057627198103120 ) ) ;
#66158=CARTESIAN_POINT ( 'NONE',  ( -9.474510206698964154, 16.51473224551069663, 80.41557627198103830 ) ) ;
#66160=CARTESIAN_POINT ( 'NONE',  ( 21.53943276465977519, -0.05219959533907433946, 83.74890960531435269 ) ) ;
#66161=CARTESIAN_POINT ( 'NONE',  ( -5.153800228976328057, -19.02544592524343514, 77.29057627198099567 ) ) ;
#66162=CARTESIAN_POINT ( 'NONE',  ( 21.53943276465977519, -0.05219959533907433946, 73.74890960531433848 ) ) ;
#66163=CARTESIAN_POINT ( 'NONE',  ( 10.72451020669871369, 18.67979575497193778, 112.0844237280190185 ) ) ;
#66164=CARTESIAN_POINT ( 'NONE',  ( -5.153800228976328057, -19.02544592524343514, 22.29057627198102765 ) ) ;
#66165=CARTESIAN_POINT ( 'NONE',  ( -4.379528057220086978, -16.55341960407618274, 109.7927570613523613 ) ) ;
#66166=CARTESIAN_POINT ( 'NONE',  ( 16.55341960407611168, 4.379528057220329451, 93.95724293864770971 ) ) ;
#66167=CARTESIAN_POINT ( 'NONE',  ( -13.97604488694547697, 13.89961937509957934, 103.1260903946856473 ) ) ;
#66169=CARTESIAN_POINT ( 'NONE',  ( -18.62759615963270932, 10.81492255796079327, 115.8322429386477097 ) ) ;
#66170=CARTESIAN_POINT ( 'NONE',  ( 0.05219959533936267826, -19.03943276465977164, 55.00109039468566863 ) ) ;
#66171=CARTESIAN_POINT ( 'NONE',  ( -16.53943276465976808, 0.05219959533911058130, 21.24890960531436690 ) ) ;
#66172=CARTESIAN_POINT ( 'NONE',  ( -5.719274019375978568, 21.55341960407610458, 70.20724293864769550 ) ) ;
#66173=CARTESIAN_POINT ( 'NONE',  ( -5.153800228976328057, -19.02544592524343514, 102.2905762719810383 ) ) ;
#66174=CARTESIAN_POINT ( 'NONE',  ( 16.52544592524342804, -4.483927247898539470, 58.54057627198103120 ) ) ;
#66176=CARTESIAN_POINT ( 'NONE',  ( 5.153800228976335163, 19.02544592524342804, 39.79057627198100988 ) ) ;
#66177=CARTESIAN_POINT ( 'NONE',  ( 15.80617190586769283, -15.72974639402175789, 110.6260903946857042 ) ) ;
#66178=CARTESIAN_POINT ( 'NONE',  ( 12.14591786802327356, -12.06949235617739191, 85.62609039468568994 ) ) ;
#66179=CARTESIAN_POINT ( 'NONE',  ( -21.52544592524334988, -5.823673210054445271, 43.95942372801902565 ) ) ;
#66180=CARTESIAN_POINT ( 'NONE',  ( -16.55341960407617563, 4.379528057220093196, 38.54275706135234714 ) ) ;
#66181=CARTESIAN_POINT ( 'NONE',  ( 21.53943276465977519, -0.05219959533907433946, 28.74890960531435624 ) ) ;
#66182=CARTESIAN_POINT ( 'NONE',  ( 19.03943276465977164, -0.05219959533909143690, 53.74890960531436690 ) ) ;
#66183=CARTESIAN_POINT ( 'NONE',  ( 16.51473224551069308, 9.474510206698969483, 64.16557627198102409 ) ) ;
#66185=CARTESIAN_POINT ( 'NONE',  ( 16.53943276465976808, 0.05219959533934440121, 56.25109039468568284 ) ) ;
#66186=CARTESIAN_POINT ( 'NONE',  ( 8.224510206698953496, -14.34966873604960469, 102.9155762719810383 ) ) ;
#66187=CARTESIAN_POINT ( 'NONE',  ( -0.05219959533910754901, -16.53943276465976808, 27.49890960531435269 ) ) ;
#66189=CARTESIAN_POINT ( 'NONE',  ( 15.72974639402176855, 15.80617190586768217, 51.87609039468568284 ) ) ;
#66190=CARTESIAN_POINT ( 'NONE',  ( -19.02544592524342804, 5.153800228976336051, 91.04057627198100988 ) ) ;
#66191=CARTESIAN_POINT ( 'NONE',  ( 19.05341960407611168, 5.049401038298154454, 83.95724293864766707 ) ) ;
#66192=CARTESIAN_POINT ( 'NONE',  ( 9.564922557960805705, 16.46253265017160317, 99.58224293864770971 ) ) ;
#66193=CARTESIAN_POINT ( 'NONE',  ( -12.14591786802309592, -12.06949235617757132, 41.87390960531435979 ) ) ;
#66194=CARTESIAN_POINT ( 'NONE',  ( 4.483927247898790824, -16.52544592524335698, 110.2094237280190185 ) ) ;
#66195=CARTESIAN_POINT ( 'NONE',  ( 14.29746914071049879, -8.314922557960816363, 43.33224293864769550 ) ) ;
#66197=CARTESIAN_POINT ( 'NONE',  ( 19.03943276465977164, 0.05219959533936151252, 41.25109039468566152 ) ) ;
#66198=CARTESIAN_POINT ( 'NONE',  ( -16.46253265017160317, 9.564922557960807481, 80.83224293864769550 ) ) ;
#66199=CARTESIAN_POINT ( 'NONE',  ( 16.46253265017146816, 9.564922557961045513, 56.66775706135233293 ) ) ;
#66203=CARTESIAN_POINT ( 'NONE',  ( -9.474510206698720793, -16.51473224551083518, 89.58442372801900433 ) ) ;
#66204=CARTESIAN_POINT ( 'NONE',  ( 4.483927247898790824, -16.52544592524335698, 75.20942372801901854 ) ) ;
#66205=CARTESIAN_POINT ( 'NONE',  ( 0.05219959533936267826, -19.03943276465977164, 20.00109039468567218 ) ) ;
#66206=CARTESIAN_POINT ( 'NONE',  ( -17.50000000000000355, -5.500000000000022204, 66.28230962303567253 ) ) ;
#66208=CARTESIAN_POINT ( 'NONE',  ( -16.51473224551069308, -9.474510206698971260, 101.6655762719810241 ) ) ;
#66209=CARTESIAN_POINT ( 'NONE',  ( -15.80617190586768217, 15.72974639402176855, 28.12609039468568284 ) ) ;
#66210=CARTESIAN_POINT ( 'NONE',  ( -19.05341960407617563, 5.049401038297882671, 88.54275706135230450 ) ) ;
#66211=CARTESIAN_POINT ( 'NONE',  ( 16.62475595723699939, 7.163666690055252140, 86.97286648189536606 ) ) ;
#66212=CARTESIAN_POINT ( 'NONE',  ( -5.049401038298153566, 19.05341960407611168, 45.20724293864769550 ) ) ;
#66213=CARTESIAN_POINT ( 'NONE',  ( -19.05341960407611168, -5.049401038298163336, 86.45724293864769550 ) ) ;
#66214=CARTESIAN_POINT ( 'NONE',  ( 16.53943276465976808, -0.05219959533910856209, 43.74890960531435979 ) ) ;
#66215=CARTESIAN_POINT ( 'NONE',  ( 19.03943276465977164, -0.05219959533909143690, 53.74890960531436690 ) ) ;
#66216=CARTESIAN_POINT ( 'NONE',  ( 5.049401038297881783, 19.05341960407617563, 62.29275706135234003 ) ) ;
#66217=CARTESIAN_POINT ( 'NONE',  ( -16.46253265017146816, -9.564922557961047289, 24.16775706135233648 ) ) ;
#66218=CARTESIAN_POINT ( 'NONE',  ( -9.474510206698964154, 16.51473224551069663, 60.41557627198102409 ) ) ;
#66219=CARTESIAN_POINT ( 'NONE',  ( -10.81492255796078084, -18.62759615963271287, 67.08224293864770971 ) ) ;
#66220=CARTESIAN_POINT ( 'NONE',  ( -16.55341960407611168, -4.379528057220339221, 66.45724293864768129 ) ) ;
#66221=CARTESIAN_POINT ( 'NONE',  ( -16.51473224551082808, 9.474510206698731452, 23.33442372801900078 ) ) ;
#66222=CARTESIAN_POINT ( 'NONE',  ( -17.60691670004650788, -5.500000000000066613, 54.13333313366441502 ) ) ;
#66223=CARTESIAN_POINT ( 'NONE',  ( -13.89961937509977652, 13.97604488694528158, 115.6239096053143669 ) ) ;
#66224=CARTESIAN_POINT ( 'NONE',  ( -19.05341960407611168, -5.049401038298163336, 51.45724293864770260 ) ) ;
#66225=CARTESIAN_POINT ( 'NONE',  ( -13.97604488694527625, -13.89961937509977652, 36.87390960531436690 ) ) ;
#66226=CARTESIAN_POINT ( 'NONE',  ( -12.06949235617756955, 12.14591786802309770, 100.6239096053143811 ) ) ;
#66227=AXIS2_PLACEMENT_3D ( 'NONE', #105942, #43287, #89784 ) ;
#66228=CARTESIAN_POINT ( 'NONE',  ( -5.719274019375978568, 21.55341960407610458, 110.2072429386477239 ) ) ;
#66230=CARTESIAN_POINT ( 'NONE',  ( -18.67979575497193778, 10.72451020669871902, 28.33442372801902209 ) ) ;
#66231=CARTESIAN_POINT ( 'NONE',  ( -5.049401038298153566, 19.05341960407611168, 100.2072429386476955 ) ) ;
#66232=CARTESIAN_POINT ( 'NONE',  ( 16.46253265017160672, -9.564922557960803928, 23.33224293864769194 ) ) ;
#66233=CARTESIAN_POINT ( 'NONE',  ( -21.55341960407619339, 5.719274019375674811, 73.54275706135234714 ) ) ;
#66234=CARTESIAN_POINT ( 'NONE',  ( 15.72974639402199770, -15.80617190586745480, 88.12390960531436690 ) ) ;
#66235=CARTESIAN_POINT ( 'NONE',  ( 5.153800228976615827, -19.02544592524334988, 40.20942372801898301 ) ) ;
#66236=CARTESIAN_POINT ( 'NONE',  ( -16.46253265017160317, 9.564922557960807481, 25.83224293864769194 ) ) ;
#66239=CARTESIAN_POINT ( 'NONE',  ( -8.314922557961024197, 14.29746914071037800, 47.91775706135234714 ) ) ;
#66240=CARTESIAN_POINT ( 'NONE',  ( -0.05219959533910754901, -16.53943276465976808, 102.4989096053143811 ) ) ;
#66242=CARTESIAN_POINT ( 'NONE',  ( -13.89961937509977652, 13.97604488694528158, 70.62390960531432427 ) ) ;
#66243=CARTESIAN_POINT ( 'NONE',  ( 4.379528057220339221, -16.55341960407611168, 97.70724293864772392 ) ) ;
#66244=CARTESIAN_POINT ( 'NONE',  ( -21.53943276465977519, 0.05219959533907696930, 51.24890960531436690 ) ) ;
#66245=CARTESIAN_POINT ( 'NONE',  ( 0.05219959533910956823, 16.53943276465976808, 64.99890960531435269 ) ) ;
#66246=CARTESIAN_POINT ( 'NONE',  ( -16.53943276465976808, -0.05219959533934237506, 28.75109039468567929 ) ) ;
#66247=CARTESIAN_POINT ( 'NONE',  ( -10.81492255796105439, 18.62759615963255655, 82.91775706135234714 ) ) ;
#66249=CARTESIAN_POINT ( 'NONE',  ( 8.224510206698742110, 14.34966873604972548, 102.0844237280190185 ) ) ;
#66250=CARTESIAN_POINT ( 'NONE',  ( -4.379528057220328563, 16.55341960407611168, 40.20724293864769550 ) ) ;
#66251=CARTESIAN_POINT ( 'NONE',  ( 13.89961937509977652, -13.97604488694527269, 38.12390960531436690 ) ) ;
#66252=CARTESIAN_POINT ( 'NONE',  ( 5.049401038298161559, -19.05341960407611168, 82.70724293864770971 ) ) ;
#66253=CARTESIAN_POINT ( 'NONE',  ( 15.72974639402199770, -15.80617190586745480, 113.1239096053143953 ) ) ;
#66254=CARTESIAN_POINT ( 'NONE',  ( 18.67979575497194134, -10.72451020669871369, 55.83442372801901854 ) ) ;
#66255=CARTESIAN_POINT ( 'NONE',  ( 16.52544592524335698, 4.483927247898782831, 36.45942372801901143 ) ) ;
#66256=CARTESIAN_POINT ( 'NONE',  ( 16.53943276465976808, -0.05219959533910856209, 58.74890960531436690 ) ) ;
#66257=CARTESIAN_POINT ( 'NONE',  ( 21.55341960407619695, -5.719274019375665929, 91.04275706135236135 ) ) ;
#66258=CARTESIAN_POINT ( 'NONE',  ( 16.53943276465976808, 0.05219959533934440121, 96.25109039468568994 ) ) ;
#66259=CARTESIAN_POINT ( 'NONE',  ( 17.48847506799968698, 5.747544572773807481, 26.67302562156720924 ) ) ;
#66260=CARTESIAN_POINT ( 'NONE',  ( -19.49190055781010145, -5.500000000000057732, 65.56116087098779133 ) ) ;
#66261=CARTESIAN_POINT ( 'NONE',  ( 12.06949235617757843, -12.14591786802309237, 33.12390960531435979 ) ) ;
#66262=CARTESIAN_POINT ( 'NONE',  ( 8.314922557961029526, -14.29746914071037800, 70.41775706135236135 ) ) ;
#66263=CARTESIAN_POINT ( 'NONE',  ( 19.02544592524343514, -5.153800228976328945, 83.54057627198100988 ) ) ;
#66264=CARTESIAN_POINT ( 'NONE',  ( 0.05219959533909260263, 19.03943276465977164, 94.99890960531436690 ) ) ;
#66265=CARTESIAN_POINT ( 'NONE',  ( -10.72451020669870658, -18.67979575497194134, 79.58442372801903275 ) ) ;
#66266=EDGE_CURVE ( 'NONE', #81647, #194062, #8617, .T. ) ;
#66267=CARTESIAN_POINT ( 'NONE',  ( -12.06949235617739369, -12.14591786802326823, 89.37609039468568994 ) ) ;
#66268=CARTESIAN_POINT ( 'NONE',  ( -16.55341960407611168, -4.379528057220339221, 66.45724293864768129 ) ) ;
#66269=CARTESIAN_POINT ( 'NONE',  ( 5.049401038298161559, -19.05341960407611168, 67.70724293864769550 ) ) ;
#66270=ORIENTED_EDGE ( 'NONE', *, *, #90349, .T. ) ;
#66271=CARTESIAN_POINT ( 'NONE',  ( -0.05219959533934338120, 16.53943276465976808, 22.50109039468567573 ) ) ;
#66272=CARTESIAN_POINT ( 'NONE',  ( -19.02544592524342804, 5.153800228976336051, 31.04057627198102409 ) ) ;
#66273=CARTESIAN_POINT ( 'NONE',  ( -5.049401038298153566, 19.05341960407611168, 75.20724293864769550 ) ) ;
#66274=CARTESIAN_POINT ( 'NONE',  ( 12.14591786802327356, -12.06949235617739191, 20.62609039468568639 ) ) ;
#66276=CARTESIAN_POINT ( 'NONE',  ( -5.153800228976607833, 19.02544592524334988, 27.70942372801899722 ) ) ;
#66277=CARTESIAN_POINT ( 'NONE',  ( -14.29746914071037622, -8.314922557961029526, 79.16775706135234714 ) ) ;
#66278=CARTESIAN_POINT ( 'NONE',  ( 13.89961937509957401, 13.97604488694547697, 101.8760903946856331 ) ) ;
#66279=CARTESIAN_POINT ( 'NONE',  ( 0.05219959533909260263, 19.03943276465977164, 24.99890960531435269 ) ) ;
#66280=CARTESIAN_POINT ( 'NONE',  ( 8.314922557961029526, -14.29746914071037800, 70.41775706135236135 ) ) ;
#66281=CARTESIAN_POINT ( 'NONE',  ( 16.53943276465976808, 0.05219959533934440121, 56.25109039468568284 ) ) ;
#66282=CARTESIAN_POINT ( 'NONE',  ( 19.02544592524343514, -5.153800228976328945, 23.54057627198102054 ) ) ;
#66283=CARTESIAN_POINT ( 'NONE',  ( -5.049401038297874678, -19.05341960407617918, 74.79275706135231871 ) ) ;
#66284=CARTESIAN_POINT ( 'NONE',  ( 0.05219959533936267826, -19.03943276465977164, 20.00109039468567218 ) ) ;
#66285=CARTESIAN_POINT ( 'NONE',  ( -9.474510206698964154, 16.51473224551069663, 30.41557627198102054 ) ) ;
#66286=CARTESIAN_POINT ( 'NONE',  ( 9.474510206698971260, -16.51473224551069308, 82.91557627198103830 ) ) ;
#66287=CARTESIAN_POINT ( 'NONE',  ( -12.06949235617756955, 12.14591786802309770, 75.62390960531439532 ) ) ;
#66288=CARTESIAN_POINT ( 'NONE',  ( 9.564922557961047289, -16.46253265017146816, 45.41775706135232582 ) ) ;
#66289=CARTESIAN_POINT ( 'NONE',  ( -0.05219959533907301413, -21.53943276465977519, 42.49890960531435979 ) ) ;
#66290=CARTESIAN_POINT ( 'NONE',  ( -18.67979575497193778, 10.72451020669871902, 113.3344237280190328 ) ) ;
#66291=CARTESIAN_POINT ( 'NONE',  ( -19.05341960407611168, -5.049401038298163336, 96.45724293864769550 ) ) ;
#66292=CARTESIAN_POINT ( 'NONE',  ( -15.80617190586768217, 15.72974639402176855, 103.1260903946856757 ) ) ;
#66293=CARTESIAN_POINT ( 'NONE',  ( 10.72451020669898902, -18.67979575497178502, 57.91557627198103120 ) ) ;
#66294=CARTESIAN_POINT ( 'NONE',  ( 16.46253265017160672, -9.564922557960803928, 98.33224293864769550 ) ) ;
#66295=CARTESIAN_POINT ( 'NONE',  ( 5.049401038297881783, 19.05341960407617563, 92.29275706135234714 ) ) ;
#66296=CARTESIAN_POINT ( 'NONE',  ( 9.474510206698971260, -16.51473224551069308, 107.9155762719810383 ) ) ;
#66297=CARTESIAN_POINT ( 'NONE',  ( 9.474510206698729675, 16.51473224551082808, 97.08442372801900433 ) ) ;
#66298=CARTESIAN_POINT ( 'NONE',  ( 0.05219959533910956823, 16.53943276465976808, 114.9989096053143669 ) ) ;
#66299=CARTESIAN_POINT ( 'NONE',  ( 0.05219959533909260263, 19.03943276465977164, 84.99890960531436690 ) ) ;
#66300=CARTESIAN_POINT ( 'NONE',  ( 5.823673210054125526, 21.52544592524343514, 64.79057627198103830 ) ) ;
#66301=CARTESIAN_POINT ( 'NONE',  ( -8.224510206698735004, -14.34966873604973081, 39.58442372801901143 ) ) ;
#66302=CARTESIAN_POINT ( 'NONE',  ( 0.05219959533937995610, -21.53943276465977519, 45.00109039468568284 ) ) ;
#66303=CARTESIAN_POINT ( 'NONE',  ( -18.62759615963255300, -10.81492255796106328, 99.16775706135234714 ) ) ;
#66304=CARTESIAN_POINT ( 'NONE',  ( -8.314922557961024197, 14.29746914071037800, 97.91775706135236135 ) ) ;
#66305=CARTESIAN_POINT ( 'NONE',  ( 19.05341960407611168, 5.049401038298154454, 88.95724293864769550 ) ) ;
#66306=CARTESIAN_POINT ( 'NONE',  ( -12.06949235617756955, 12.14591786802309770, 95.62390960531436690 ) ) ;
#66307=CARTESIAN_POINT ( 'NONE',  ( 12.14591786802309770, 12.06949235617756955, 24.37390960531435979 ) ) ;
#66308=CARTESIAN_POINT ( 'NONE',  ( 5.153800228976615827, -19.02544592524334988, 75.20942372801896170 ) ) ;
#66309=CARTESIAN_POINT ( 'NONE',  ( -15.80617190586768217, 15.72974639402176855, 48.12609039468568284 ) ) ;
#66310=CARTESIAN_POINT ( 'NONE',  ( 4.379528057220339221, -16.55341960407611168, 92.70724293864770971 ) ) ;
#66311=CARTESIAN_POINT ( 'NONE',  ( 16.46253265017160672, -9.564922557960803928, 113.3322429386476955 ) ) ;
#66312=CARTESIAN_POINT ( 'NONE',  ( -4.379528057220328563, 16.55341960407611168, 25.20724293864769550 ) ) ;
#66313=CARTESIAN_POINT ( 'NONE',  ( -21.52544592524334988, -5.823673210054445271, 83.95942372801900433 ) ) ;
#66314=CARTESIAN_POINT ( 'NONE',  ( 16.52544592524335698, 4.483927247898782831, 46.45942372801901854 ) ) ;
#66315=CARTESIAN_POINT ( 'NONE',  ( 21.53943276465977519, 0.05219959533937863772, 41.25109039468568284 ) ) ;
#66316=ORIENTED_EDGE ( 'NONE', *, *, #195850, .T. ) ;
#66317=CARTESIAN_POINT ( 'NONE',  ( -15.80617190586768217, 15.72974639402176855, 28.12609039468568284 ) ) ;
#66318=CARTESIAN_POINT ( 'NONE',  ( -16.55341960407611168, -4.379528057220339221, 96.45724293864770971 ) ) ;
#66319=CARTESIAN_POINT ( 'NONE',  ( 20.22402473803820300, 1.857821124618833641, 37.49999999999998579 ) ) ;
#66320=CARTESIAN_POINT ( 'NONE',  ( -12.14591786802309592, -12.06949235617757132, 66.87390960531436690 ) ) ;
#66321=CARTESIAN_POINT ( 'NONE',  ( 9.474510206698971260, -16.51473224551069308, 52.91557627198102409 ) ) ;
#66322=CARTESIAN_POINT ( 'NONE',  ( 4.483927247898790824, -16.52544592524335698, 105.2094237280190328 ) ) ;
#66323=CARTESIAN_POINT ( 'NONE',  ( -19.03943276465977164, 0.05219959533909376836, 41.24890960531435269 ) ) ;
#66324=CARTESIAN_POINT ( 'NONE',  ( 21.55341960407610458, 5.719274019375980345, 48.95724293864770971 ) ) ;
#66325=CARTESIAN_POINT ( 'NONE',  ( -8.224510206698948167, 14.34966873604960824, 75.41557627198102409 ) ) ;
#66326=VECTOR ( 'NONE', #181084, 1000.000000000000000 ) ;
#66327=CARTESIAN_POINT ( 'NONE',  ( 21.55341960407610458, 5.719274019375980345, 98.95724293864770971 ) ) ;
#66328=CARTESIAN_POINT ( 'NONE',  ( 13.97604488694527802, 13.89961937509977652, 94.37390960531436690 ) ) ;
#66329=CARTESIAN_POINT ( 'NONE',  ( 19.03943276465977164, -0.05219959533909143690, 43.74890960531435979 ) ) ;
#66330=CARTESIAN_POINT ( 'NONE',  ( -9.564922557961040184, 16.46253265017147172, 87.91775706135233293 ) ) ;
#66331=CARTESIAN_POINT ( 'NONE',  ( 18.67979575497178502, 10.72451020669898547, 49.16557627198102409 ) ) ;
#66332=CARTESIAN_POINT ( 'NONE',  ( -18.67979575497193778, 10.72451020669871902, 68.33442372801900433 ) ) ;
#66333=CARTESIAN_POINT ( 'NONE',  ( 13.97604488694527802, 13.89961937509977652, 54.37390960531435979 ) ) ;
#66334=CARTESIAN_POINT ( 'NONE',  ( -16.51473224551069308, -9.474510206698971260, 86.66557627198102409 ) ) ;
#66336=CARTESIAN_POINT ( 'NONE',  ( -4.379528057220086978, -16.55341960407618274, 59.79275706135234714 ) ) ;
#66337=CARTESIAN_POINT ( 'NONE',  ( 15.80617190586769283, -15.72974639402175789, 50.62609039468568994 ) ) ;
#66338=CARTESIAN_POINT ( 'NONE',  ( 10.72451020669871369, 18.67979575497193778, 72.08442372801899012 ) ) ;
#66339=CARTESIAN_POINT ( 'NONE',  ( -10.81492255796078084, -18.62759615963271287, 22.08224293864769194 ) ) ;
#66340=CARTESIAN_POINT ( 'NONE',  ( -18.62759615963270932, 10.81492255796079327, 105.8322429386476955 ) ) ;
#66341=CARTESIAN_POINT ( 'NONE',  ( -5.823673210054431948, 21.52544592524334988, 32.70942372801900433 ) ) ;
#66342=CARTESIAN_POINT ( 'NONE',  ( 12.06949235617739724, 12.14591786802326823, 66.87609039468568994 ) ) ;
#66343=CARTESIAN_POINT ( 'NONE',  ( 21.53943276465977519, -0.05219959533907433946, 63.74890960531435979 ) ) ;
#66344=CARTESIAN_POINT ( 'NONE',  ( -9.564922557961040184, 16.46253265017147172, 37.91775706135233293 ) ) ;
#66345=CARTESIAN_POINT ( 'NONE',  ( -19.05341960407611168, -5.049401038298163336, 66.45724293864769550 ) ) ;
#66346=CARTESIAN_POINT ( 'NONE',  ( 14.29746914071037800, 8.314922557961029526, 101.6677570613523613 ) ) ;
#66347=CARTESIAN_POINT ( 'NONE',  ( -22.00000000000000000, -1.163414459189985801E-14, 97.50000000000000000 ) ) ;
#66348=CARTESIAN_POINT ( 'NONE',  ( -5.049401038298153566, 19.05341960407611168, 100.2072429386476955 ) ) ;
#66350=CARTESIAN_POINT ( 'NONE',  ( 9.474510206698729675, 16.51473224551082808, 87.08442372801900433 ) ) ;
#66352=CARTESIAN_POINT ( 'NONE',  ( 0.05219959533907565091, 21.53943276465977519, 64.99890960531435269 ) ) ;
#66353=CARTESIAN_POINT ( 'NONE',  ( -0.05219959533910754901, -16.53943276465976808, 32.49890960531435979 ) ) ;
#66354=CARTESIAN_POINT ( 'NONE',  ( 13.97604488694548053, -13.89961937509957401, 95.62609039468563310 ) ) ;
#66356=CARTESIAN_POINT ( 'NONE',  ( -13.97604488694547697, 13.89961937509957934, 93.12609039468566152 ) ) ;
#66357=CARTESIAN_POINT ( 'NONE',  ( -15.80617190586745835, -15.72974639402198527, 81.87390960531435269 ) ) ;
#66358=CARTESIAN_POINT ( 'NONE',  ( -19.03943276465977164, -0.05219959533935918106, 63.75109039468566863 ) ) ;
#66360=CARTESIAN_POINT ( 'NONE',  ( -9.474510206698964154, 16.51473224551069663, 70.41557627198102409 ) ) ;
#66361=CARTESIAN_POINT ( 'NONE',  ( -16.55341960407611168, -4.379528057220339221, 61.45724293864770260 ) ) ;
#66363=CARTESIAN_POINT ( 'NONE',  ( -13.89961937509977652, 13.97604488694528158, 50.62390960531435979 ) ) ;
#66364=CARTESIAN_POINT ( 'NONE',  ( 12.06949235617757843, -12.14591786802309237, 48.12390960531436690 ) ) ;
#66365=CARTESIAN_POINT ( 'NONE',  ( 19.05341960407611168, 5.049401038298154454, 23.95724293864769194 ) ) ;
#66367=CARTESIAN_POINT ( 'NONE',  ( 12.14591786802309770, 12.06949235617756955, 34.37390960531435979 ) ) ;
#66368=CARTESIAN_POINT ( 'NONE',  ( -19.05341960407611168, -5.049401038298163336, 76.45724293864769550 ) ) ;
#66370=CARTESIAN_POINT ( 'NONE',  ( 0.05219959533936267826, -19.03943276465977164, 35.00109039468566863 ) ) ;
#66371=CARTESIAN_POINT ( 'NONE',  ( -0.05219959533934338120, 16.53943276465976808, 47.50109039468568994 ) ) ;
#66372=CARTESIAN_POINT ( 'NONE',  ( 0.05219959533907565091, 21.53943276465977519, 49.99890960531437401 ) ) ;
#66373=CARTESIAN_POINT ( 'NONE',  ( 0.05219959533937995610, -21.53943276465977519, 110.0010903946856757 ) ) ;
#66374=CARTESIAN_POINT ( 'NONE',  ( -13.97604488694527625, -13.89961937509977652, 76.87390960531433848 ) ) ;
#66375=CARTESIAN_POINT ( 'NONE',  ( 16.46253265017160672, -9.564922557960803928, 113.3322429386476955 ) ) ;
#66376=CARTESIAN_POINT ( 'NONE',  ( -16.51473224551069308, -9.474510206698971260, 106.6655762719810383 ) ) ;
#66377=CARTESIAN_POINT ( 'NONE',  ( -10.72451020669870658, -18.67979575497194134, 39.58442372801901143 ) ) ;
#66378=CARTESIAN_POINT ( 'NONE',  ( -4.483927247898539470, -16.52544592524342804, 92.29057627198103830 ) ) ;
#66379=CARTESIAN_POINT ( 'NONE',  ( -5.823673210054116645, -21.52544592524344225, 92.29057627198103830 ) ) ;
#66380=CARTESIAN_POINT ( 'NONE',  ( 13.89961937509977652, -13.97604488694527269, 88.12390960531438111 ) ) ;
#66382=CARTESIAN_POINT ( 'NONE',  ( 21.55341960407619695, -5.719274019375665929, 21.04275706135234714 ) ) ;
#66384=CARTESIAN_POINT ( 'NONE',  ( -16.46253265017160317, 9.564922557960807481, 80.83224293864769550 ) ) ;
#66385=CARTESIAN_POINT ( 'NONE',  ( 17.50000000001358558, -5.500000000000039968, 48.29690382535059001 ) ) ;
#66386=CARTESIAN_POINT ( 'NONE',  ( -12.06949235617756955, 12.14591786802309770, 115.6239096053143669 ) ) ;
#66387=CARTESIAN_POINT ( 'NONE',  ( 19.05341960407611168, 5.049401038298154454, 38.95724293864767418 ) ) ;
#66388=CARTESIAN_POINT ( 'NONE',  ( 19.02544592524334988, 5.153800228976608722, 106.4594237280190185 ) ) ;
#66390=CARTESIAN_POINT ( 'NONE',  ( 12.06949235617757843, -12.14591786802309237, 113.1239096053143953 ) ) ;
#66391=CARTESIAN_POINT ( 'NONE',  ( 21.52544592524334988, 5.823673210054432836, 81.45942372801900433 ) ) ;
#66392=CARTESIAN_POINT ( 'NONE',  ( -13.97604488694527625, -13.89961937509977652, 61.87390960531435979 ) ) ;
#66393=CARTESIAN_POINT ( 'NONE',  ( -10.81492255796105439, 18.62759615963255655, 32.91775706135234714 ) ) ;
#66394=CARTESIAN_POINT ( 'NONE',  ( -15.80617190586745835, -15.72974639402198527, 111.8739096053143669 ) ) ;
#66396=CARTESIAN_POINT ( 'NONE',  ( -13.89961937509977652, 13.97604488694528158, 90.62390960531432427 ) ) ;
#66398=CARTESIAN_POINT ( 'NONE',  ( -16.53943276465976808, -0.05219959533934237506, 28.75109039468567929 ) ) ;
#66399=CARTESIAN_POINT ( 'NONE',  ( 18.62759615963271287, -10.81492255796078972, 43.33224293864769550 ) ) ;
#66400=CARTESIAN_POINT ( 'NONE',  ( -10.72451020669870658, -18.67979575497194134, 59.58442372801901854 ) ) ;
#66401=CARTESIAN_POINT ( 'NONE',  ( 19.03943276465977164, -0.05219959533909143690, 108.7489096053143527 ) ) ;
#66402=CARTESIAN_POINT ( 'NONE',  ( -16.51473224551082808, 9.474510206698731452, 98.33442372801900433 ) ) ;
#66403=CARTESIAN_POINT ( 'NONE',  ( -0.05219959533909027116, -19.03943276465977164, 62.49890960531435979 ) ) ;
#66404=CARTESIAN_POINT ( 'NONE',  ( 5.049401038298161559, -19.05341960407611168, 82.70724293864770971 ) ) ;
#66405=CARTESIAN_POINT ( 'NONE',  ( 16.52544592524342804, -4.483927247898539470, 93.54057627198103830 ) ) ;
#66406=CARTESIAN_POINT ( 'NONE',  ( 12.06949235617757843, -12.14591786802309237, 103.1239096053143811 ) ) ;
#66407=CARTESIAN_POINT ( 'NONE',  ( -21.55341960407610458, -5.719274019375992779, 21.45724293864769550 ) ) ;
#66408=CARTESIAN_POINT ( 'NONE',  ( 4.483927247898545687, 16.52544592524342804, 59.79057627198103120 ) ) ;
#66409=CARTESIAN_POINT ( 'NONE',  ( -5.049401038298153566, 19.05341960407611168, 35.20724293864768839 ) ) ;
#66410=CARTESIAN_POINT ( 'NONE',  ( -10.81492255796105439, 18.62759615963255655, 67.91775706135234714 ) ) ;
#66411=CARTESIAN_POINT ( 'NONE',  ( -5.049401038297874678, -19.05341960407617918, 89.79275706135230450 ) ) ;
#66412=CARTESIAN_POINT ( 'NONE',  ( -0.05219959533910754901, -16.53943276465976808, 67.49890960531436690 ) ) ;
#66413=CARTESIAN_POINT ( 'NONE',  ( -21.55341960407610458, -5.719274019375992779, 106.4572429386477097 ) ) ;
#66414=CARTESIAN_POINT ( 'NONE',  ( -21.53943276465977519, 0.05219959533907696930, 46.24890960531435979 ) ) ;
#66416=CARTESIAN_POINT ( 'NONE',  ( -19.05341960407611168, -5.049401038298163336, 111.4572429386476671 ) ) ;
#66418=CARTESIAN_POINT ( 'NONE',  ( -0.05219959533909027116, -19.03943276465977164, 72.49890960531435269 ) ) ;
#66419=CARTESIAN_POINT ( 'NONE',  ( 16.55341960407611168, 4.379528057220329451, 33.95724293864769550 ) ) ;
#66420=CARTESIAN_POINT ( 'NONE',  ( -4.483927247898782831, 16.52544592524335698, 107.7094237280190328 ) ) ;
#66421=CARTESIAN_POINT ( 'NONE',  ( -16.55341960407617563, 4.379528057220093196, 88.54275706135236135 ) ) ;
#66422=CARTESIAN_POINT ( 'NONE',  ( -0.05219959533936034679, 19.03943276465977164, 42.50109039468566152 ) ) ;
#66423=CARTESIAN_POINT ( 'NONE',  ( -18.22780087662122028, -5.500000000000014211, 101.4845989467389273 ) ) ;
#66424=CARTESIAN_POINT ( 'NONE',  ( -5.049401038298153566, 19.05341960407611168, 95.20724293864770971 ) ) ;
#66425=CARTESIAN_POINT ( 'NONE',  ( 16.51473224551069308, 9.474510206698969483, 44.16557627198103120 ) ) ;
#66426=CARTESIAN_POINT ( 'NONE',  ( 4.483927247898545687, 16.52544592524342804, 54.79057627198104541 ) ) ;
#66427=CARTESIAN_POINT ( 'NONE',  ( -13.89961937509977652, 13.97604488694528158, 25.62390960531434558 ) ) ;
#66428=CARTESIAN_POINT ( 'NONE',  ( -16.46253265017160317, 9.564922557960807481, 115.8322429386477097 ) ) ;
#66429=CARTESIAN_POINT ( 'NONE',  ( -15.72974639402197994, 15.80617190586746368, 55.62390960531436690 ) ) ;
#66430=CARTESIAN_POINT ( 'NONE',  ( -4.379528057220328563, 16.55341960407611168, 90.20724293864770971 ) ) ;
#66431=CARTESIAN_POINT ( 'NONE',  ( -12.14591786802326823, 12.06949235617739902, 33.12609039468569705 ) ) ;
#66432=CARTESIAN_POINT ( 'NONE',  ( 4.483927247898545687, 16.52544592524342804, 79.79057627198102409 ) ) ;
#66433=CARTESIAN_POINT ( 'NONE',  ( -19.48894818550241581, 5.500000000000113687, 65.10307310435243267 ) ) ;
#66434=CARTESIAN_POINT ( 'NONE',  ( -19.02544592524334988, -5.153800228976617603, 73.95942372801900433 ) ) ;
#66435=CARTESIAN_POINT ( 'NONE',  ( -19.05341960407611168, -5.049401038298163336, 111.4572429386476671 ) ) ;
#66438=CARTESIAN_POINT ( 'NONE',  ( -4.379528057220086978, -16.55341960407618274, 24.79275706135235779 ) ) ;
#66439=CARTESIAN_POINT ( 'NONE',  ( -16.53943276465976808, -0.05219959533934237506, 113.7510903946856757 ) ) ;
#66440=CARTESIAN_POINT ( 'NONE',  ( 19.02544592524334988, 5.153800228976608722, 71.45942372801900433 ) ) ;
#66441=CARTESIAN_POINT ( 'NONE',  ( 15.80617190586746368, 15.72974639402197994, 49.37390960531436690 ) ) ;
#66442=CARTESIAN_POINT ( 'NONE',  ( 18.67979575497194134, -10.72451020669871369, 70.83442372801901854 ) ) ;
#66444=CARTESIAN_POINT ( 'NONE',  ( 16.52544592524335698, 4.483927247898782831, 36.45942372801901143 ) ) ;
#66445=CARTESIAN_POINT ( 'NONE',  ( -9.474510206698964154, 16.51473224551069663, 30.41557627198102054 ) ) ;
#66446=CARTESIAN_POINT ( 'NONE',  ( 5.153800228976335163, 19.02544592524342804, 84.79057627198099567 ) ) ;
#66447=CARTESIAN_POINT ( 'NONE',  ( -13.97604488694527625, -13.89961937509977652, 21.87390960531435979 ) ) ;
#66448=CARTESIAN_POINT ( 'NONE',  ( -14.34966873604960291, -8.224510206698953496, 96.66557627198102409 ) ) ;
#66450=CARTESIAN_POINT ( 'NONE',  ( 5.049401038298161559, -19.05341960407611168, 97.70724293864766707 ) ) ;
#66451=ORIENTED_EDGE ( 'NONE', *, *, #11076, .F. ) ;
#66452=CARTESIAN_POINT ( 'NONE',  ( 9.564922557961047289, -16.46253265017146816, 110.4177570613523471 ) ) ;
#66453=CARTESIAN_POINT ( 'NONE',  ( 0.05219959533907565091, 21.53943276465977519, 74.99890960531435269 ) ) ;
#66454=CARTESIAN_POINT ( 'NONE',  ( 16.46253265017160672, -9.564922557960803928, 48.33224293864769550 ) ) ;
#66455=CARTESIAN_POINT ( 'NONE',  ( 19.05341960407617918, -5.049401038297876454, 71.04275706135234714 ) ) ;
#66456=CARTESIAN_POINT ( 'NONE',  ( -10.81492255796078084, -18.62759615963271287, 112.0822429386477097 ) ) ;
#66457=CARTESIAN_POINT ( 'NONE',  ( 13.89961937509977652, -13.97604488694527269, 73.12390960531436690 ) ) ;
#66458=CARTESIAN_POINT ( 'NONE',  ( -19.05341960407611168, -5.049401038298163336, 106.4572429386476955 ) ) ;
#66460=CARTESIAN_POINT ( 'NONE',  ( 16.53943276465976808, 0.05219959533934440121, 36.25109039468567573 ) ) ;
#66461=( BOUNDED_CURVE ( )  B_SPLINE_CURVE ( 2, ( #11561, #61000, #122672, #134898, #28712, #73227, #184361, #169171, #44856, #61984, #185348, #30675, #90348 ),
 .UNSPECIFIED., .F., .F. ) 
 B_SPLINE_CURVE_WITH_KNOTS ( ( 3, 2, 2, 2, 2, 2, 3 ),
 ( 0.4761146469533609205, 0.4780701754385964786, 0.4824561403508771940, 0.4868421052631579093, 0.4912280701754385692, 0.4956140350877192846, 0.4975238837508647594 ),
 .UNSPECIFIED. ) 
 CURVE ( )  GEOMETRIC_REPRESENTATION_ITEM ( )  RATIONAL_B_SPLINE_CURVE ( ( 0.9831626618144004848, 0.9848076720550091867, 1.000000000000000000, 0.9659258262890683122, 1.000000000000000000, 0.9659258262890683122, 1.000000000000000000, 0.9659258262890683122, 1.000000000000000000, 0.9659258262890683122, 1.000000000000000000, 0.9851625545550091179, 0.9832469066685282089 ) ) 
 REPRESENTATION_ITEM ( '' )  );
#66462=CARTESIAN_POINT ( 'NONE',  ( 21.55341960407610458, 5.719274019375980345, 98.95724293864770971 ) ) ;
#66463=CARTESIAN_POINT ( 'NONE',  ( 8.224510206698953496, -14.34966873604960469, 102.9155762719810383 ) ) ;
#66464=CARTESIAN_POINT ( 'NONE',  ( -5.153800228976328057, -19.02544592524343514, 92.29057627198099567 ) ) ;
#66465=CARTESIAN_POINT ( 'NONE',  ( 5.049401038297881783, 19.05341960407617563, 62.29275706135234003 ) ) ;
#66466=CARTESIAN_POINT ( 'NONE',  ( -10.81492255796078084, -18.62759615963271287, 92.08224293864769550 ) ) ;
#66467=CARTESIAN_POINT ( 'NONE',  ( -16.55341960407611168, -4.379528057220339221, 51.45724293864770260 ) ) ;
#66468=CARTESIAN_POINT ( 'NONE',  ( 13.89961937509957401, 13.97604488694547697, 26.87609039468566507 ) ) ;
#66469=CARTESIAN_POINT ( 'NONE',  ( 8.314922557961029526, -14.29746914071037800, 65.41775706135234714 ) ) ;
#66470=CARTESIAN_POINT ( 'NONE',  ( 5.049401038298161559, -19.05341960407611168, 87.70724293864769550 ) ) ;
#66472=CARTESIAN_POINT ( 'NONE',  ( 19.02544592524343514, -5.153800228976328945, 43.54057627198103120 ) ) ;
#66473=CARTESIAN_POINT ( 'NONE',  ( -5.719274019375665041, -21.55341960407619695, 54.79275706135235424 ) ) ;
#66475=CARTESIAN_POINT ( 'NONE',  ( 18.67979575497194134, -10.72451020669871369, 65.83442372801900433 ) ) ;
#66476=CARTESIAN_POINT ( 'NONE',  ( 5.049401038298161559, -19.05341960407611168, 67.70724293864769550 ) ) ;
#66477=CARTESIAN_POINT ( 'NONE',  ( 0.05219959533937995610, -21.53943276465977519, 30.00109039468568284 ) ) ;
#66478=CARTESIAN_POINT ( 'NONE',  ( -9.564922557961040184, 16.46253265017147172, 72.91775706135233293 ) ) ;
#66479=CARTESIAN_POINT ( 'NONE',  ( 13.97604488694527802, 13.89961937509977652, 39.37390960531435269 ) ) ;
#66480=CARTESIAN_POINT ( 'NONE',  ( 12.06949235617739724, 12.14591786802326823, 86.87609039468568994 ) ) ;
#66481=CARTESIAN_POINT ( 'NONE',  ( 5.049401038298161559, -19.05341960407611168, 52.70724293864767418 ) ) ;
#66482=CARTESIAN_POINT ( 'NONE',  ( -19.03943276465977164, 0.05219959533909376836, 106.2489096053143669 ) ) ;
#66483=CARTESIAN_POINT ( 'NONE',  ( 16.51473224551069308, 9.474510206698969483, 34.16557627198102409 ) ) ;
#66484=CARTESIAN_POINT ( 'NONE',  ( -10.81492255796078084, -18.62759615963271287, 87.08224293864769550 ) ) ;
#66485=CARTESIAN_POINT ( 'NONE',  ( -16.53943276465976808, -0.05219959533934237506, 68.75109039468568994 ) ) ;
#66487=CARTESIAN_POINT ( 'NONE',  ( 9.564922557961047289, -16.46253265017146816, 30.41775706135232937 ) ) ;
#66488=CARTESIAN_POINT ( 'NONE',  ( 19.03943276465977164, -0.05219959533909143690, 53.74890960531436690 ) ) ;
#66489=CARTESIAN_POINT ( 'NONE',  ( -12.14591786802309592, -12.06949235617757132, 46.87390960531435979 ) ) ;
#66490=CARTESIAN_POINT ( 'NONE',  ( -4.483927247898539470, -16.52544592524342804, 77.29057627198102409 ) ) ;
#66491=CARTESIAN_POINT ( 'NONE',  ( 13.97604488694527802, 13.89961937509977652, 104.3739096053143385 ) ) ;
#66492=CARTESIAN_POINT ( 'NONE',  ( 19.03943276465977164, -0.05219959533909143690, 78.74890960531436690 ) ) ;
#66493=CARTESIAN_POINT ( 'NONE',  ( -21.52544592524334988, -5.823673210054445271, 53.95942372801900433 ) ) ;
#66494=CARTESIAN_POINT ( 'NONE',  ( 9.564922557960805705, 16.46253265017160317, 94.58224293864769550 ) ) ;
#66495=CARTESIAN_POINT ( 'NONE',  ( 5.823673210054444382, -21.52544592524334988, 95.20942372801903275 ) ) ;
#66496=CARTESIAN_POINT ( 'NONE',  ( 4.483927247898790824, -16.52544592524335698, 80.20942372801901854 ) ) ;
#66497=CARTESIAN_POINT ( 'NONE',  ( -10.72451020669870658, -18.67979575497194134, 24.58442372801901499 ) ) ;
#66498=CARTESIAN_POINT ( 'NONE',  ( -15.72974639402197994, 15.80617190586746368, 105.6239096053143669 ) ) ;
#66499=CARTESIAN_POINT ( 'NONE',  ( 0.05219959533910956823, 16.53943276465976808, 64.99890960531435269 ) ) ;
#66500=CARTESIAN_POINT ( 'NONE',  ( 19.03943276465977164, -0.05219959533909143690, 38.74890960531436690 ) ) ;
#66501=CARTESIAN_POINT ( 'NONE',  ( -12.14591786802309592, -12.06949235617757132, 66.87390960531436690 ) ) ;
#66502=CARTESIAN_POINT ( 'NONE',  ( 21.55341960407610458, 5.719274019375980345, 23.95724293864769550 ) ) ;
#66503=CARTESIAN_POINT ( 'NONE',  ( -19.02544592524334988, -5.153800228976617603, 28.95942372801900433 ) ) ;
#66505=CARTESIAN_POINT ( 'NONE',  ( 4.379528057220339221, -16.55341960407611168, 102.7072429386476955 ) ) ;
#66506=ORIENTED_EDGE ( 'NONE', *, *, #92660, .T. ) ;
#66507=CARTESIAN_POINT ( 'NONE',  ( -16.55341960407617563, 4.379528057220093196, 63.54275706135234003 ) ) ;
#66508=CARTESIAN_POINT ( 'NONE',  ( -19.03943276465977164, 0.05219959533909376836, 66.24890960531436690 ) ) ;
#66509=CARTESIAN_POINT ( 'NONE',  ( -16.61815367056139436, -6.523988306745442500, 20.69395534479570387 ) ) ;
#66510=CARTESIAN_POINT ( 'NONE',  ( 14.34966873604960469, 8.224510206698951720, 84.16557627198103830 ) ) ;
#66511=CARTESIAN_POINT ( 'NONE',  ( -21.53943276465977519, 0.05219959533907696930, 31.24890960531435979 ) ) ;
#66512=CARTESIAN_POINT ( 'NONE',  ( 4.379528057220092307, 16.55341960407617563, 97.29275706135234714 ) ) ;
#66513=CARTESIAN_POINT ( 'NONE',  ( -19.03943276465977164, -0.05219959533935918106, 113.7510903946856757 ) ) ;
#66514=CARTESIAN_POINT ( 'NONE',  ( 10.72451020669871369, 18.67979575497193778, 82.08442372801901854 ) ) ;
#66515=CARTESIAN_POINT ( 'NONE',  ( 9.564922557960805705, 16.46253265017160317, 89.58224293864769550 ) ) ;
#66516=CARTESIAN_POINT ( 'NONE',  ( 15.72974639402199770, -15.80617190586745480, 108.1239096053143811 ) ) ;
#66517=CARTESIAN_POINT ( 'NONE',  ( 12.14591786802327356, -12.06949235617739191, 60.62609039468567573 ) ) ;
#66518=CARTESIAN_POINT ( 'NONE',  ( 4.483927247898545687, 16.52544592524342804, 114.7905762719810383 ) ) ;
#66519=CARTESIAN_POINT ( 'NONE',  ( 4.379528057220092307, 16.55341960407617563, 22.29275706135235069 ) ) ;
#66520=CARTESIAN_POINT ( 'NONE',  ( -16.46253265017146816, -9.564922557961047289, 84.16775706135233293 ) ) ;
#66521=CARTESIAN_POINT ( 'NONE',  ( -10.81492255796078084, -18.62759615963271287, 72.08224293864769550 ) ) ;
#66522=CARTESIAN_POINT ( 'NONE',  ( -13.97604488694547697, 13.89961937509957934, 53.12609039468565442 ) ) ;
#66524=CARTESIAN_POINT ( 'NONE',  ( 21.53943276465977519, -0.05219959533907433946, 108.7489096053143669 ) ) ;
#66526=CARTESIAN_POINT ( 'NONE',  ( 0.05219959533909260263, 19.03943276465977164, 74.99890960531435269 ) ) ;
#66528=CARTESIAN_POINT ( 'NONE',  ( -14.29746914071037622, -8.314922557961029526, 29.16775706135234003 ) ) ;
#66530=CARTESIAN_POINT ( 'NONE',  ( 15.80617190586746368, 15.72974639402197994, 99.37390960531436690 ) ) ;
#66531=CARTESIAN_POINT ( 'NONE',  ( -12.06949235617756955, 12.14591786802309770, 60.62390960531437401 ) ) ;
#66532=CARTESIAN_POINT ( 'NONE',  ( 13.97604488694527802, 13.89961937509977652, 64.37390960531436690 ) ) ;
#66533=CARTESIAN_POINT ( 'NONE',  ( 15.80617190586769283, -15.72974639402175789, 90.62609039468567573 ) ) ;
#66534=CARTESIAN_POINT ( 'NONE',  ( -4.483927247898782831, 16.52544592524335698, 37.70942372801900433 ) ) ;
#66535=CARTESIAN_POINT ( 'NONE',  ( -13.97604488694547697, 13.89961937509957934, 48.12609039468566863 ) ) ;
#66536=CARTESIAN_POINT ( 'NONE',  ( -18.67979575497193778, 10.72451020669871902, 53.33442372801901854 ) ) ;
#66537=CARTESIAN_POINT ( 'NONE',  ( 21.53943276465977519, -0.05219959533907433946, 58.74890960531436690 ) ) ;
#66538=CARTESIAN_POINT ( 'NONE',  ( -13.89961937509957401, -13.97604488694547875, 109.3760903946856331 ) ) ;
#66539=CARTESIAN_POINT ( 'NONE',  ( 5.153800228976335163, 19.02544592524342804, 59.79057627198100988 ) ) ;
#66540=CARTESIAN_POINT ( 'NONE',  ( 19.05341960407617918, -5.049401038297876454, 86.04275706135233293 ) ) ;
#66541=CARTESIAN_POINT ( 'NONE',  ( -5.719274019375665041, -21.55341960407619695, 79.79275706135236135 ) ) ;
#66542=CARTESIAN_POINT ( 'NONE',  ( 13.89961937509957401, 13.97604488694547697, 71.87609039468567573 ) ) ;
#66543=CARTESIAN_POINT ( 'NONE',  ( -19.02544592524342804, 5.153800228976336051, 41.04057627198103120 ) ) ;
#66544=CARTESIAN_POINT ( 'NONE',  ( -10.72451020669898014, 18.67979575497178502, 55.41557627198102409 ) ) ;
#66545=CARTESIAN_POINT ( 'NONE',  ( -8.224510206698948167, 14.34966873604960824, 65.41557627198102409 ) ) ;
#66546=CARTESIAN_POINT ( 'NONE',  ( 15.50000000000000178, -5.500000000000000888, 20.00000000000000000 ) ) ;
#66547=CARTESIAN_POINT ( 'NONE',  ( -5.153800228976607833, 19.02544592524334988, 27.70942372801899722 ) ) ;
#66548=CARTESIAN_POINT ( 'NONE',  ( 16.52544592524335698, 4.483927247898782831, 96.45942372801901854 ) ) ;
#66549=CARTESIAN_POINT ( 'NONE',  ( -8.314922557960811034, -14.29746914071050412, 52.08224293864768839 ) ) ;
#66550=CARTESIAN_POINT ( 'NONE',  ( 15.72974639402176855, 15.80617190586768217, 91.87609039468568994 ) ) ;
#66551=CARTESIAN_POINT ( 'NONE',  ( 10.81492255796106328, -18.62759615963255655, 85.41775706135236135 ) ) ;
#66552=CARTESIAN_POINT ( 'NONE',  ( 0.05219959533907565091, 21.53943276465977519, 89.99890960531438111 ) ) ;
#66553=CARTESIAN_POINT ( 'NONE',  ( 5.049401038298161559, -19.05341960407611168, 52.70724293864767418 ) ) ;
#66554=CARTESIAN_POINT ( 'NONE',  ( -15.72974639402176322, -15.80617190586768395, 64.37609039468568994 ) ) ;
#66555=CARTESIAN_POINT ( 'NONE',  ( -9.474510206698964154, 16.51473224551069663, 45.41557627198103120 ) ) ;
#66556=CARTESIAN_POINT ( 'NONE',  ( -19.03943276465977164, 0.05219959533909376836, 61.24890960531436690 ) ) ;
#66557=CARTESIAN_POINT ( 'NONE',  ( -4.483927247898539470, -16.52544592524342804, 102.2905762719810383 ) ) ;
#66558=CARTESIAN_POINT ( 'NONE',  ( -19.05341960407611168, -5.049401038298163336, 96.45724293864769550 ) ) ;
#66559=CARTESIAN_POINT ( 'NONE',  ( 12.14591786802309770, 12.06949235617756955, 54.37390960531435979 ) ) ;
#66560=CARTESIAN_POINT ( 'NONE',  ( -8.224510206698948167, 14.34966873604960824, 110.4155762719810383 ) ) ;
#66561=CARTESIAN_POINT ( 'NONE',  ( -21.55341960407610458, -5.719274019375992779, 81.45724293864769550 ) ) ;
#66562=CARTESIAN_POINT ( 'NONE',  ( -15.80617190586768217, 15.72974639402176855, 33.12609039468569705 ) ) ;
#66564=CARTESIAN_POINT ( 'NONE',  ( 4.379528057220092307, 16.55341960407617563, 42.29275706135235424 ) ) ;
#66565=CARTESIAN_POINT ( 'NONE',  ( -5.823673210054116645, -21.52544592524344225, 87.29057627198103830 ) ) ;
#66566=CARTESIAN_POINT ( 'NONE',  ( 15.80617190586769283, -15.72974639402175789, 105.6260903946856899 ) ) ;
#66567=CARTESIAN_POINT ( 'NONE',  ( 19.03943276465977164, -0.05219959533909143690, 93.74890960531435269 ) ) ;
#66568=CARTESIAN_POINT ( 'NONE',  ( 5.719274019375673035, 21.55341960407619339, 37.29275706135235424 ) ) ;
#66569=CARTESIAN_POINT ( 'NONE',  ( -21.55341960407610458, -5.719274019375992779, 31.45724293864769550 ) ) ;
#66570=CARTESIAN_POINT ( 'NONE',  ( -14.29746914071037622, -8.314922557961029526, 99.16775706135234714 ) ) ;
#66571=CARTESIAN_POINT ( 'NONE',  ( -21.53943276465977519, -0.05219959533937600094, 48.75109039468568284 ) ) ;
#66572=CARTESIAN_POINT ( 'NONE',  ( 15.80617190586769283, -15.72974639402175789, 80.62609039468567573 ) ) ;
#66573=CARTESIAN_POINT ( 'NONE',  ( -18.67979575497193778, 10.72451020669871902, 108.3344237280190185 ) ) ;
#66574=CARTESIAN_POINT ( 'NONE',  ( -4.483927247898782831, 16.52544592524335698, 77.70942372801900433 ) ) ;
#66575=CARTESIAN_POINT ( 'NONE',  ( 18.67979575497194134, -10.72451020669871369, 40.83442372801901854 ) ) ;
#66576=CARTESIAN_POINT ( 'NONE',  ( -16.46253265017160317, 9.564922557960807481, 35.83224293864768839 ) ) ;
#66577=CARTESIAN_POINT ( 'NONE',  ( -10.81492255796105439, 18.62759615963255655, 107.9177570613523471 ) ) ;
#66578=CARTESIAN_POINT ( 'NONE',  ( 9.564922557960805705, 16.46253265017160317, 109.5822429386476955 ) ) ;
#66579=CARTESIAN_POINT ( 'NONE',  ( -21.53943276465977519, 0.05219959533907696930, 101.2489096053143669 ) ) ;
#66580=CARTESIAN_POINT ( 'NONE',  ( 18.87255363501903815, 5.499999999999947597, 83.82513748171827217 ) ) ;
#66581=CARTESIAN_POINT ( 'NONE',  ( -0.05219959533907301413, -21.53943276465977519, 72.49890960531435269 ) ) ;
#66582=CARTESIAN_POINT ( 'NONE',  ( 16.55341960407618274, -4.379528057220086978, 46.04275706135234714 ) ) ;
#66584=CARTESIAN_POINT ( 'NONE',  ( 14.34966873604960469, 8.224510206698951720, 54.16557627198103120 ) ) ;
#66585=DIRECTION ( 'NONE',  ( -0.000000000000000000, -0.000000000000000000, 1.000000000000000000 ) ) ;
#66586=CARTESIAN_POINT ( 'NONE',  ( -13.89961937509957401, -13.97604488694547875, 89.37609039468563310 ) ) ;
#66588=CARTESIAN_POINT ( 'NONE',  ( 14.34966873604972726, -8.224510206698740333, 30.83442372801902209 ) ) ;
#66589=CARTESIAN_POINT ( 'NONE',  ( 10.72451020669898902, -18.67979575497178502, 102.9155762719810383 ) ) ;
#66590=CARTESIAN_POINT ( 'NONE',  ( -21.52544592524343514, 5.823673210054127303, 71.04057627198103830 ) ) ;
#66591=CARTESIAN_POINT ( 'NONE',  ( 0.05219959533909260263, 19.03943276465977164, 109.9989096053143669 ) ) ;
#66592=CARTESIAN_POINT ( 'NONE',  ( -14.29746914071037622, -8.314922557961029526, 44.16775706135234714 ) ) ;
#66593=CARTESIAN_POINT ( 'NONE',  ( -9.564922557960796823, -16.46253265017161027, 72.08224293864770971 ) ) ;
#66594=CARTESIAN_POINT ( 'NONE',  ( 18.62759615963255655, 10.81492255796105972, 26.66775706135235424 ) ) ;
#66595=CARTESIAN_POINT ( 'NONE',  ( -9.474510206698720793, -16.51473224551083518, 94.58442372801900433 ) ) ;
#66596=CARTESIAN_POINT ( 'NONE',  ( -5.153800228976328057, -19.02544592524343514, 107.2905762719810383 ) ) ;
#66597=CARTESIAN_POINT ( 'NONE',  ( 19.05341960407611168, 5.049401038298154454, 93.95724293864769550 ) ) ;
#66598=CARTESIAN_POINT ( 'NONE',  ( -0.05219959533907301413, -21.53943276465977519, 87.49890960531436690 ) ) ;
#66599=CARTESIAN_POINT ( 'NONE',  ( 13.97604488694527802, 13.89961937509977652, 54.37390960531435979 ) ) ;
#66600=CARTESIAN_POINT ( 'NONE',  ( -17.26172910966778318, -6.454744622555873335, 59.19353091350777873 ) ) ;
#66601=CARTESIAN_POINT ( 'NONE',  ( 12.14591786802309770, 12.06949235617756955, 69.37390960531436690 ) ) ;
#66602=CARTESIAN_POINT ( 'NONE',  ( -5.823673210054116645, -21.52544592524344225, 27.29057627198103120 ) ) ;
#66604=CARTESIAN_POINT ( 'NONE',  ( 15.80617190586746368, 15.72974639402197994, 89.37390960531435269 ) ) ;
#66605=CARTESIAN_POINT ( 'NONE',  ( 19.05341960407617918, -5.049401038297876454, 66.04275706135233293 ) ) ;
#66606=CARTESIAN_POINT ( 'NONE',  ( -18.67979575497178146, -10.72451020669898902, 21.66557627198102409 ) ) ;
#66607=CARTESIAN_POINT ( 'NONE',  ( 19.39720447994795549, 5.499999999999969802, 67.16317477297174321 ) ) ;
#66608=CARTESIAN_POINT ( 'NONE',  ( -21.53943276465977519, 0.05219959533907696930, 61.24890960531435979 ) ) ;
#66609=CARTESIAN_POINT ( 'NONE',  ( -19.03943276465977164, 0.05219959533909376836, 81.24890960531436690 ) ) ;
#66610=B_SPLINE_CURVE_WITH_KNOTS ( 'NONE', 3,
 ( #55223, #43056, #57238, #116892, #178584, #42070, #163413, #10734, #179595, #24909, #151237, #101724, #9734, #71398, #180596, #166414, #133062, #27908, #12726, #194752, #164419, #141007, #1493, #64176, #90533, #15690, #154200, #137036, #171360, #46022, #31853, #109679 ),
 .UNSPECIFIED., .F., .F.,
 ( 4, 2, 2, 2, 2, 2, 2, 2, 2, 2, 2, 2, 2, 2, 2, 4 ),
 ( 8.673617379884035472E-19, 0.0003712461730036666118, 0.0007424923460073323562, 0.001113738519010998209, 0.001484984692014663845, 0.002227477038021997285, 0.002598723211025675064, 0.002969969384029352410, 0.003341215557033029755, 0.003712461730036707968, 0.004083707903040385313, 0.004454954076044063092, 0.004826200249047740004, 0.005197446422051418650, 0.005568692595055095562, 0.005939938768058774209 ),
 .UNSPECIFIED. ) ;
#66611=CARTESIAN_POINT ( 'NONE',  ( 21.55341960407619695, -5.719274019375665929, 76.04275706135237556 ) ) ;
#66612=CARTESIAN_POINT ( 'NONE',  ( 9.474510206698971260, -16.51473224551069308, 57.91557627198103120 ) ) ;
#66613=CARTESIAN_POINT ( 'NONE',  ( -12.06949235617756955, 12.14591786802309770, 75.62390960531439532 ) ) ;
#66614=CARTESIAN_POINT ( 'NONE',  ( 4.483927247898790824, -16.52544592524335698, 40.20942372801901854 ) ) ;
#66615=CARTESIAN_POINT ( 'NONE',  ( 21.52544592524334988, 5.823673210054432836, 71.45942372801901854 ) ) ;
#66617=CARTESIAN_POINT ( 'NONE',  ( -16.46253265017146816, -9.564922557961047289, 19.16775706135233293 ) ) ;
#66618=CARTESIAN_POINT ( 'NONE',  ( 19.03943276465977164, 0.05219959533936151252, 76.25109039468566152 ) ) ;
#66620=CARTESIAN_POINT ( 'NONE',  ( -21.55341960407619339, 5.719274019375674811, 38.54275706135234714 ) ) ;
#66622=CARTESIAN_POINT ( 'NONE',  ( -9.564922557961040184, 16.46253265017147172, 32.91775706135233293 ) ) ;
#66623=CARTESIAN_POINT ( 'NONE',  ( -13.97604488694527625, -13.89961937509977652, 56.87390960531434558 ) ) ;
#66624=CARTESIAN_POINT ( 'NONE',  ( 5.049401038297881783, 19.05341960407617563, 32.29275706135233293 ) ) ;
#66625=CARTESIAN_POINT ( 'NONE',  ( 0.05219959533934541429, -16.53943276465976808, 105.0010903946856757 ) ) ;
#66626=CARTESIAN_POINT ( 'NONE',  ( -5.153800228976328057, -19.02544592524343514, 107.2905762719810383 ) ) ;
#66627=CARTESIAN_POINT ( 'NONE',  ( -15.72974639402176322, -15.80617190586768395, 69.37609039468567573 ) ) ;
#66630=CARTESIAN_POINT ( 'NONE',  ( -21.52544592524334988, -5.823673210054445271, 88.95942372801901854 ) ) ;
#66631=CARTESIAN_POINT ( 'NONE',  ( 17.48853670773242897, -5.747243402303147342, 41.16671299749989998 ) ) ;
#66632=CARTESIAN_POINT ( 'NONE',  ( 19.05341960407611168, 5.049401038298154454, 98.95724293864766707 ) ) ;
#66633=ADVANCED_FACE ( 'NONE', ( #75672 ), #165717, .F. ) ;
#66634=CARTESIAN_POINT ( 'NONE',  ( 5.049401038297881783, 19.05341960407617563, 27.29275706135232937 ) ) ;
#66636=CARTESIAN_POINT ( 'NONE',  ( 0.05219959533909260263, 19.03943276465977164, 44.99890960531435979 ) ) ;
#66637=CARTESIAN_POINT ( 'NONE',  ( 18.62759615963271287, -10.81492255796078972, 53.33224293864769550 ) ) ;
#66638=CARTESIAN_POINT ( 'NONE',  ( -12.06949235617756955, 12.14591786802309770, 25.62390960531435624 ) ) ;
#66639=CARTESIAN_POINT ( 'NONE',  ( -8.314922557960811034, -14.29746914071050412, 92.08224293864769550 ) ) ;
#66640=CARTESIAN_POINT ( 'NONE',  ( 0.05219959533909260263, 19.03943276465977164, 74.99890960531435269 ) ) ;
#66641=CARTESIAN_POINT ( 'NONE',  ( 0.05219959533937995610, -21.53943276465977519, 100.0010903946857042 ) ) ;
#66642=CARTESIAN_POINT ( 'NONE',  ( -19.05341960407611168, -5.049401038298163336, 31.45724293864769550 ) ) ;
#66643=CARTESIAN_POINT ( 'NONE',  ( -4.379528057220328563, 16.55341960407611168, 105.2072429386477097 ) ) ;
#66644=CARTESIAN_POINT ( 'NONE',  ( 21.53943276465977519, 0.05219959533937863772, 56.25109039468568284 ) ) ;
#66646=CARTESIAN_POINT ( 'NONE',  ( -10.81492255796078084, -18.62759615963271287, 82.08224293864768129 ) ) ;
#66647=CARTESIAN_POINT ( 'NONE',  ( -19.02544592524334988, -5.153800228976617603, 48.95942372801900433 ) ) ;
#66649=CARTESIAN_POINT ( 'NONE',  ( 5.153800228976335163, 19.02544592524342804, 104.7905762719809957 ) ) ;
#66650=CARTESIAN_POINT ( 'NONE',  ( -16.55341960407611168, -4.379528057220339221, 76.45724293864769550 ) ) ;
#66652=CARTESIAN_POINT ( 'NONE',  ( -19.02544592524334988, -5.153800228976617603, 38.95942372801900433 ) ) ;
#66653=CARTESIAN_POINT ( 'NONE',  ( -16.46253265017160317, 9.564922557960807481, 60.83224293864769550 ) ) ;
#66654=CARTESIAN_POINT ( 'NONE',  ( -16.53943276465976808, 0.05219959533911058130, 61.24890960531435979 ) ) ;
#66655=CARTESIAN_POINT ( 'NONE',  ( -16.51473224551082808, 9.474510206698731452, 73.33442372801900433 ) ) ;
#66656=CARTESIAN_POINT ( 'NONE',  ( -5.049401038297874678, -19.05341960407618274, 89.79275706135233293 ) ) ;
#66657=CARTESIAN_POINT ( 'NONE',  ( -0.05219959533907301413, -21.53943276465977519, 32.49890960531435979 ) ) ;
#66658=VERTEX_POINT ( 'NONE', #166716 ) ;
#66659=CARTESIAN_POINT ( 'NONE',  ( -4.379528057220328563, 16.55341960407611168, 95.20724293864769550 ) ) ;
#66661=CARTESIAN_POINT ( 'NONE',  ( 19.02544592524343514, -5.153800228976328945, 58.54057627198102409 ) ) ;
#66662=CARTESIAN_POINT ( 'NONE',  ( -15.80617190586745835, -15.72974639402198527, 66.87390960531436690 ) ) ;
#66663=CARTESIAN_POINT ( 'NONE',  ( 9.474510206698971260, -16.51473224551069308, 32.91557627198102409 ) ) ;
#66664=CARTESIAN_POINT ( 'NONE',  ( 12.06949235617739724, 12.14591786802326823, 76.87609039468567573 ) ) ;
#66665=CARTESIAN_POINT ( 'NONE',  ( -9.564922557960796823, -16.46253265017161027, 57.08224293864769550 ) ) ;
#66666=CARTESIAN_POINT ( 'NONE',  ( 19.05341960407617918, -5.049401038297876454, 51.04275706135231871 ) ) ;
#66667=CARTESIAN_POINT ( 'NONE',  ( -5.823673210054431948, 21.52544592524334988, 62.70942372801902565 ) ) ;
#66668=CARTESIAN_POINT ( 'NONE',  ( -18.62759615963270932, 10.81492255796079327, 50.83224293864770971 ) ) ;
#66669=CARTESIAN_POINT ( 'NONE',  ( 14.29746914071049879, -8.314922557960816363, 113.3322429386476955 ) ) ;
#66670=CARTESIAN_POINT ( 'NONE',  ( -14.34966873604972548, 8.224510206698743886, 83.33442372801903275 ) ) ;
#66671=CARTESIAN_POINT ( 'NONE',  ( -9.564922557961040184, 16.46253265017147172, 102.9177570613523329 ) ) ;
#66673=CARTESIAN_POINT ( 'NONE',  ( 17.50000000000001421, 5.622605283950889543, 53.81207310596115434 ) ) ;
#66674=CARTESIAN_POINT ( 'NONE',  ( 15.80617190586769283, -15.72974639402175789, 100.6260903946857184 ) ) ;
#66676=CARTESIAN_POINT ( 'NONE',  ( -12.14591786802309592, -12.06949235617757132, 51.87390960531437401 ) ) ;
#66677=CARTESIAN_POINT ( 'NONE',  ( -14.29746914071049879, 8.314922557960819915, 55.83224293864770260 ) ) ;
#66678=CARTESIAN_POINT ( 'NONE',  ( 5.719274019375991003, -21.55341960407610458, 92.70724293864770971 ) ) ;
#66679=CARTESIAN_POINT ( 'NONE',  ( -10.81492255796078084, -18.62759615963271287, 92.08224293864769550 ) ) ;
#66681=CARTESIAN_POINT ( 'NONE',  ( -0.05219959533907301413, -21.53943276465977519, 32.49890960531435979 ) ) ;
#66682=CARTESIAN_POINT ( 'NONE',  ( 12.06949235617739724, 12.14591786802326823, 71.87609039468568994 ) ) ;
#66683=CARTESIAN_POINT ( 'NONE',  ( -12.14591786802309592, -12.06949235617757132, 76.87390960531439532 ) ) ;
#66684=CARTESIAN_POINT ( 'NONE',  ( -13.89961937509977652, 13.97604488694528158, 50.62390960531435979 ) ) ;
#66687=CARTESIAN_POINT ( 'NONE',  ( 14.34966873604972726, -8.224510206698740333, 95.83442372801903275 ) ) ;
#66688=CARTESIAN_POINT ( 'NONE',  ( -15.72974639402197994, 15.80617190586746368, 115.6239096053143669 ) ) ;
#66689=CARTESIAN_POINT ( 'NONE',  ( 19.05341960407611168, 5.049401038298154454, 88.95724293864769550 ) ) ;
#66690=CARTESIAN_POINT ( 'NONE',  ( 18.67979575497194134, -10.72451020669871369, 50.83442372801901143 ) ) ;
#66693=CARTESIAN_POINT ( 'NONE',  ( 5.719274019375673035, 21.55341960407619339, 52.29275706135236135 ) ) ;
#66694=CARTESIAN_POINT ( 'NONE',  ( 13.97604488694527802, 13.89961937509977652, 39.37390960531435269 ) ) ;
#66695=CARTESIAN_POINT ( 'NONE',  ( 0.05219959533909260263, 19.03943276465977164, 114.9989096053143669 ) ) ;
#66696=CARTESIAN_POINT ( 'NONE',  ( 9.564922557961047289, -16.46253265017146816, 50.41775706135233293 ) ) ;
#66697=CARTESIAN_POINT ( 'NONE',  ( 21.53943276465977519, 0.05219959533937863772, 26.25109039468567573 ) ) ;
#66698=CARTESIAN_POINT ( 'NONE',  ( 5.153800228976615827, -19.02544592524334988, 65.20942372801900433 ) ) ;
#66699=CARTESIAN_POINT ( 'NONE',  ( -9.474510206698964154, 16.51473224551069663, 25.41557627198103120 ) ) ;
#66700=CARTESIAN_POINT ( 'NONE',  ( 4.379528057220092307, 16.55341960407617563, 87.29275706135236135 ) ) ;
#66701=CARTESIAN_POINT ( 'NONE',  ( 5.153800228976615827, -19.02544592524334988, 65.20942372801900433 ) ) ;
#66702=CARTESIAN_POINT ( 'NONE',  ( 4.379528057220092307, 16.55341960407617563, 107.2927570613523471 ) ) ;
#66705=CARTESIAN_POINT ( 'NONE',  ( -13.97604488694527625, -13.89961937509977652, 91.87390960531432427 ) ) ;
#66707=CARTESIAN_POINT ( 'NONE',  ( -15.72974639402176322, -15.80617190586768395, 99.37609039468568994 ) ) ;
#66708=CARTESIAN_POINT ( 'NONE',  ( -21.52544592524334988, -5.823673210054445271, 108.9594237280190185 ) ) ;
#66711=CARTESIAN_POINT ( 'NONE',  ( 13.89961937509977652, -13.97604488694527269, 98.12390960531433848 ) ) ;
#66712=CARTESIAN_POINT ( 'NONE',  ( -10.72451020669870658, -18.67979575497194134, 74.58442372801901854 ) ) ;
#66713=CARTESIAN_POINT ( 'NONE',  ( -12.06949235617739369, -12.14591786802326823, 19.37609039468568639 ) ) ;
#66714=CARTESIAN_POINT ( 'NONE',  ( 13.89961937509977652, -13.97604488694527269, 78.12390960531433848 ) ) ;
#66715=CARTESIAN_POINT ( 'NONE',  ( 15.72974639402199770, -15.80617190586745480, 33.12390960531435979 ) ) ;
#66716=CARTESIAN_POINT ( 'NONE',  ( 0.05219959533909260263, 19.03943276465977164, 94.99890960531436690 ) ) ;
#66718=CARTESIAN_POINT ( 'NONE',  ( 16.51473224551069308, 9.474510206698969483, 59.16557627198102409 ) ) ;
#66719=CARTESIAN_POINT ( 'NONE',  ( -16.52544592524342804, 4.483927247898546575, 26.04057627198103475 ) ) ;
#66721=CARTESIAN_POINT ( 'NONE',  ( -9.474510206698720793, -16.51473224551083518, 69.58442372801901854 ) ) ;
#66722=CARTESIAN_POINT ( 'NONE',  ( -16.46253265017160317, 9.564922557960807481, 100.8322429386477097 ) ) ;
#66723=CARTESIAN_POINT ( 'NONE',  ( -21.55341960407619339, 5.719274019375674811, 98.54275706135234714 ) ) ;
#66724=CARTESIAN_POINT ( 'NONE',  ( 8.314922557960818139, 14.29746914071049879, 79.58224293864769550 ) ) ;
#66725=CARTESIAN_POINT ( 'NONE',  ( 0.05219959533907565091, 21.53943276465977519, 49.99890960531437401 ) ) ;
#66726=CARTESIAN_POINT ( 'NONE',  ( -18.67979575497178146, -10.72451020669898902, 41.66557627198103120 ) ) ;
#66727=CARTESIAN_POINT ( 'NONE',  ( 14.29746914071049879, -8.314922557960816363, 108.3322429386477097 ) ) ;
#66729=CARTESIAN_POINT ( 'NONE',  ( 13.97604488694548053, -13.89961937509957401, 45.62609039468566863 ) ) ;
#66730=CARTESIAN_POINT ( 'NONE',  ( -14.29746914071049879, 8.314922557960819915, 25.83224293864769194 ) ) ;
#66731=CARTESIAN_POINT ( 'NONE',  ( -5.153800228976328057, -19.02544592524343514, 97.29057627198099567 ) ) ;
#66732=CARTESIAN_POINT ( 'NONE',  ( 21.52544592524334988, 5.823673210054432836, 71.45942372801901854 ) ) ;
#66733=CARTESIAN_POINT ( 'NONE',  ( 21.52544592524344225, -5.823673210054117533, 53.54057627198103120 ) ) ;
#66734=CARTESIAN_POINT ( 'NONE',  ( -21.53943276465977519, -0.05219959533937600094, 48.75109039468568284 ) ) ;
#66735=CARTESIAN_POINT ( 'NONE',  ( -18.62759615963270932, 10.81492255796079327, 95.83224293864770971 ) ) ;
#66736=CARTESIAN_POINT ( 'NONE',  ( 18.67979575497194134, -10.72451020669871369, 35.83442372801901143 ) ) ;
#66737=CARTESIAN_POINT ( 'NONE',  ( -14.34966873604960291, -8.224510206698953496, 101.6655762719810383 ) ) ;
#66738=CARTESIAN_POINT ( 'NONE',  ( -5.049401038297874678, -19.05341960407617918, 69.79275706135233293 ) ) ;
#66739=CARTESIAN_POINT ( 'NONE',  ( 4.483927247898545687, 16.52544592524342804, 109.7905762719810383 ) ) ;
#66740=CARTESIAN_POINT ( 'NONE',  ( -9.564922557960796823, -16.46253265017161027, 107.0822429386476955 ) ) ;
#66741=CARTESIAN_POINT ( 'NONE',  ( 16.55341960407611168, 4.379528057220329451, 48.95724293864770971 ) ) ;
#66742=CARTESIAN_POINT ( 'NONE',  ( 0.05219959533910956823, 16.53943276465976808, 24.99890960531435624 ) ) ;
#66743=CARTESIAN_POINT ( 'NONE',  ( 16.51473224551069308, 9.474510206698969483, 49.16557627198102409 ) ) ;
#66744=CARTESIAN_POINT ( 'NONE',  ( -13.97604488694527625, -13.89961937509977652, 26.87390960531434558 ) ) ;
#66745=CARTESIAN_POINT ( 'NONE',  ( 21.52544592524344225, -5.823673210054117533, 28.54057627198103120 ) ) ;
#66746=CARTESIAN_POINT ( 'NONE',  ( -19.02544592524334988, -5.153800228976617603, 18.95942372801899722 ) ) ;
#66748=CARTESIAN_POINT ( 'NONE',  ( 16.52544592524342804, -4.483927247898539470, 33.54057627198102409 ) ) ;
#66749=CARTESIAN_POINT ( 'NONE',  ( 21.55341960407619695, -5.719274019375665929, 51.04275706135234714 ) ) ;
#66751=CARTESIAN_POINT ( 'NONE',  ( 4.483927247898790824, -16.52544592524335698, 55.20942372801902565 ) ) ;
#66752=CARTESIAN_POINT ( 'NONE',  ( 14.34966873604960469, 8.224510206698951720, 29.16557627198103120 ) ) ;
#66753=CARTESIAN_POINT ( 'NONE',  ( -16.53943276465976808, -0.05219959533934237506, 108.7510903946857042 ) ) ;
#66754=CARTESIAN_POINT ( 'NONE',  ( 5.049401038298161559, -19.05341960407611168, 32.70724293864768129 ) ) ;
#66755=CARTESIAN_POINT ( 'NONE',  ( 9.564922557960805705, 16.46253265017160317, 59.58224293864769550 ) ) ;
#66756=CARTESIAN_POINT ( 'NONE',  ( 16.46253265017160672, -9.564922557960803928, 23.33224293864769194 ) ) ;
#66757=CARTESIAN_POINT ( 'NONE',  ( 10.81492255796106328, -18.62759615963255655, 30.41775706135234358 ) ) ;
#66758=CARTESIAN_POINT ( 'NONE',  ( -13.97604488694527625, -13.89961937509977652, 46.87390960531435979 ) ) ;
#66760=CARTESIAN_POINT ( 'NONE',  ( 16.46253265017160672, -9.564922557960803928, 33.33224293864770260 ) ) ;
#66761=CARTESIAN_POINT ( 'NONE',  ( -16.51473224551069308, -9.474510206698971260, 111.6655762719810383 ) ) ;
#66762=CARTESIAN_POINT ( 'NONE',  ( -10.81492255796105439, 18.62759615963255655, 62.91775706135236135 ) ) ;
#66763=CARTESIAN_POINT ( 'NONE',  ( -4.379528057220328563, 16.55341960407611168, 110.2072429386477239 ) ) ;
#66764=CARTESIAN_POINT ( 'NONE',  ( -9.564922557960796823, -16.46253265017161027, 112.0822429386476955 ) ) ;
#66765=CARTESIAN_POINT ( 'NONE',  ( -14.34966873604972548, 8.224510206698743886, 78.33442372801901854 ) ) ;
#66766=CARTESIAN_POINT ( 'NONE',  ( -18.62759615963255300, -10.81492255796106328, 89.16775706135236135 ) ) ;
#66767=CARTESIAN_POINT ( 'NONE',  ( -4.483927247898782831, 16.52544592524335698, 47.70942372801902565 ) ) ;
#66768=CARTESIAN_POINT ( 'NONE',  ( -0.05219959533909027116, -19.03943276465977164, 97.49890960531436690 ) ) ;
#66769=CARTESIAN_POINT ( 'NONE',  ( 14.34966873604972726, -8.224510206698740333, 45.83442372801901854 ) ) ;
#66770=CARTESIAN_POINT ( 'NONE',  ( 8.314922557961029526, -14.29746914071037800, 25.41775706135235779 ) ) ;
#66771=CARTESIAN_POINT ( 'NONE',  ( 14.34966873604972726, -8.224510206698740333, 80.83442372801901854 ) ) ;
#66772=CARTESIAN_POINT ( 'NONE',  ( 5.153800228976615827, -19.02544592524334988, 110.2094237280189901 ) ) ;
#66773=CARTESIAN_POINT ( 'NONE',  ( 5.153800228976335163, 19.02544592524342804, 79.79057627198102409 ) ) ;
#66774=CARTESIAN_POINT ( 'NONE',  ( -0.05219959533907301413, -21.53943276465977519, 102.4989096053143811 ) ) ;
#66775=CARTESIAN_POINT ( 'NONE',  ( 4.379528057220339221, -16.55341960407611168, 107.7072429386476955 ) ) ;
#66776=CARTESIAN_POINT ( 'NONE',  ( -19.05341960407617563, 5.049401038297882671, 108.5427570613523187 ) ) ;
#66777=CARTESIAN_POINT ( 'NONE',  ( -4.483927247898782831, 16.52544592524335698, 72.70942372801901854 ) ) ;
#66779=CARTESIAN_POINT ( 'NONE',  ( 19.05341960407617918, -5.049401038297876454, 76.04275706135230450 ) ) ;
#66780=CARTESIAN_POINT ( 'NONE',  ( -16.52544592524342804, 4.483927247898546575, 46.04057627198103830 ) ) ;
#66781=CARTESIAN_POINT ( 'NONE',  ( -14.34966873604960291, -8.224510206698953496, 96.66557627198102409 ) ) ;
#66782=CARTESIAN_POINT ( 'NONE',  ( 19.03943276465977164, 0.05219959533936151252, 31.25109039468566863 ) ) ;
#66783=CARTESIAN_POINT ( 'NONE',  ( -5.719274019375665041, -21.55341960407619695, 39.79275706135235424 ) ) ;
#66784=CARTESIAN_POINT ( 'NONE',  ( -19.02544592524334988, -5.153800228976617603, 93.95942372801900433 ) ) ;
#66785=CARTESIAN_POINT ( 'NONE',  ( -16.46253265017160317, 9.564922557960807481, 90.83224293864769550 ) ) ;
#66786=CARTESIAN_POINT ( 'NONE',  ( 5.719274019375673035, 21.55341960407619339, 112.2927570613523471 ) ) ;
#66787=CARTESIAN_POINT ( 'NONE',  ( 16.51473224551069308, 9.474510206698969483, 94.16557627198103830 ) ) ;
#66788=CARTESIAN_POINT ( 'NONE',  ( 18.62759615963271287, -10.81492255796078972, 53.33224293864769550 ) ) ;
#66789=CARTESIAN_POINT ( 'NONE',  ( -0.05219959533910754901, -16.53943276465976808, 87.49890960531436690 ) ) ;
#66790=CARTESIAN_POINT ( 'NONE',  ( -9.474510206698964154, 16.51473224551069663, 75.41557627198103830 ) ) ;
#66791=CARTESIAN_POINT ( 'NONE',  ( -4.379528057220328563, 16.55341960407611168, 115.2072429386476955 ) ) ;
#66793=CARTESIAN_POINT ( 'NONE',  ( 21.53943276465977519, 0.05219959533937863772, 31.25109039468568639 ) ) ;
#66794=CARTESIAN_POINT ( 'NONE',  ( 15.80617190586769283, -15.72974639402175789, 75.62609039468567573 ) ) ;
#66795=CARTESIAN_POINT ( 'NONE',  ( -13.89961937509977652, 13.97604488694528158, 45.62390960531433848 ) ) ;
#66796=CARTESIAN_POINT ( 'NONE',  ( 8.224510206698742110, 14.34966873604972548, 72.08442372801899012 ) ) ;
#66797=CARTESIAN_POINT ( 'NONE',  ( 15.72974639402176855, 15.80617190586768217, 26.87609039468567218 ) ) ;
#66798=CARTESIAN_POINT ( 'NONE',  ( 15.80617190586769283, -15.72974639402175789, 25.62609039468567929 ) ) ;
#66799=CARTESIAN_POINT ( 'NONE',  ( -19.03943276465977164, -0.05219959533935918106, 58.75109039468566863 ) ) ;
#66800=CARTESIAN_POINT ( 'NONE',  ( -19.02544592524342804, 5.153800228976336051, 66.04057627198103830 ) ) ;
#66801=CARTESIAN_POINT ( 'NONE',  ( 19.02544592524334988, 5.153800228976608722, 26.45942372801899722 ) ) ;
#66802=CARTESIAN_POINT ( 'NONE',  ( 10.72451020669871369, 18.67979575497193778, 87.08442372801901854 ) ) ;
#66803=CARTESIAN_POINT ( 'NONE',  ( 5.823673210054125526, 21.52544592524343514, 64.79057627198103830 ) ) ;
#66804=CARTESIAN_POINT ( 'NONE',  ( 0.05219959533910956823, 16.53943276465976808, 54.99890960531435269 ) ) ;
#66805=CARTESIAN_POINT ( 'NONE',  ( -5.719274019375665041, -21.55341960407619695, 84.79275706135234714 ) ) ;
#66806=CARTESIAN_POINT ( 'NONE',  ( -19.03943276465977164, -0.05219959533935918106, 23.75109039468566152 ) ) ;
#66807=CARTESIAN_POINT ( 'NONE',  ( 14.34966873604960469, 8.224510206698951720, 74.16557627198102409 ) ) ;
#66808=CARTESIAN_POINT ( 'NONE',  ( 9.564922557960805705, 16.46253265017160317, 29.58224293864769550 ) ) ;
#66809=CARTESIAN_POINT ( 'NONE',  ( -19.02544592524334988, -5.153800228976617603, 53.95942372801898301 ) ) ;
#66810=CARTESIAN_POINT ( 'NONE',  ( -16.55341960407611168, -4.379528057220339221, 31.45724293864769550 ) ) ;
#66812=CARTESIAN_POINT ( 'NONE',  ( 15.80617190586769283, -15.72974639402175789, 80.62609039468567573 ) ) ;
#66813=CARTESIAN_POINT ( 'NONE',  ( -9.474510206698964154, 16.51473224551069663, 75.41557627198103830 ) ) ;
#66814=CARTESIAN_POINT ( 'NONE',  ( 16.51473224551083163, -9.474510206698727899, 50.83442372801899722 ) ) ;
#66815=CARTESIAN_POINT ( 'NONE',  ( -21.55341960407610458, -5.719274019375992779, 46.45724293864769550 ) ) ;
#66816=CARTESIAN_POINT ( 'NONE',  ( -21.52544592524334988, -5.823673210054445271, 38.95942372801901854 ) ) ;
#66817=CARTESIAN_POINT ( 'NONE',  ( -21.53943276465977519, 0.05219959533907696930, 96.24890960531435269 ) ) ;
#66818=CARTESIAN_POINT ( 'NONE',  ( 16.46253265017146816, 9.564922557961045513, 96.66775706135233293 ) ) ;
#66819=CARTESIAN_POINT ( 'NONE',  ( 12.06949235617739724, 12.14591786802326823, 61.87609039468568284 ) ) ;
#66821=CARTESIAN_POINT ( 'NONE',  ( -18.62759615963270932, 10.81492255796079327, 100.8322429386477097 ) ) ;
#66822=CARTESIAN_POINT ( 'NONE',  ( 4.483927247898545687, 16.52544592524342804, 109.7905762719810383 ) ) ;
#66823=CARTESIAN_POINT ( 'NONE',  ( -17.49999999999999645, -5.499999999999992895, 99.20309617465831309 ) ) ;
#66824=CARTESIAN_POINT ( 'NONE',  ( 14.34966873604972726, -8.224510206698740333, 30.83442372801902209 ) ) ;
#66825=CARTESIAN_POINT ( 'NONE',  ( -21.55341960407610458, -5.719274019375992779, 66.45724293864768129 ) ) ;
#66826=CARTESIAN_POINT ( 'NONE',  ( -4.483927247898782831, 16.52544592524335698, 97.70942372801904696 ) ) ;
#66827=CARTESIAN_POINT ( 'NONE',  ( 5.049401038298161559, -19.05341960407611168, 32.70724293864768129 ) ) ;
#66828=CARTESIAN_POINT ( 'NONE',  ( -14.34966873604972548, 8.224510206698743886, 63.33442372801900433 ) ) ;
#66829=CARTESIAN_POINT ( 'NONE',  ( -5.049401038297874678, -19.05341960407617918, 54.79275706135234003 ) ) ;
#66830=CARTESIAN_POINT ( 'NONE',  ( 21.52544592524334988, 5.823673210054432836, 41.45942372801901143 ) ) ;
#66831=CARTESIAN_POINT ( 'NONE',  ( -5.823673210054116645, -21.52544592524344225, 62.29057627198102409 ) ) ;
#66832=CARTESIAN_POINT ( 'NONE',  ( -12.06949235617739369, -12.14591786802326823, 89.37609039468568994 ) ) ;
#66833=CARTESIAN_POINT ( 'NONE',  ( -21.55341960407619339, 5.719274019375674811, 73.54275706135234714 ) ) ;
#66834=CARTESIAN_POINT ( 'NONE',  ( -10.81492255796078084, -18.62759615963271287, 57.08224293864769550 ) ) ;
#66835=CARTESIAN_POINT ( 'NONE',  ( -5.719274019375978568, 21.55341960407610458, 40.20724293864769550 ) ) ;
#66837=CARTESIAN_POINT ( 'NONE',  ( 16.55341960407618274, -4.379528057220086978, 71.04275706135234714 ) ) ;
#66838=CARTESIAN_POINT ( 'NONE',  ( 18.67979575497178502, 10.72451020669898547, 34.16557627198102409 ) ) ;
#66839=VERTEX_POINT ( 'NONE', #26217 ) ;
#66840=CARTESIAN_POINT ( 'NONE',  ( -13.89961937509977652, 13.97604488694528158, 100.6239096053143669 ) ) ;
#66841=CARTESIAN_POINT ( 'NONE',  ( -0.05219959533934338120, 16.53943276465976808, 112.5010903946857042 ) ) ;
#66843=CARTESIAN_POINT ( 'NONE',  ( 4.379528057220339221, -16.55341960407611168, 102.7072429386476955 ) ) ;
#66844=CARTESIAN_POINT ( 'NONE',  ( -0.05219959533907301413, -21.53943276465977519, 67.49890960531436690 ) ) ;
#66845=CARTESIAN_POINT ( 'NONE',  ( -4.379528057220086978, -16.55341960407618274, 84.79275706135234714 ) ) ;
#66846=CARTESIAN_POINT ( 'NONE',  ( -21.53943276465977519, -0.05219959533937600094, 48.75109039468568284 ) ) ;
#66847=CARTESIAN_POINT ( 'NONE',  ( 9.564922557961047289, -16.46253265017146816, 105.4177570613523471 ) ) ;
#66848=CARTESIAN_POINT ( 'NONE',  ( -12.06949235617756955, 12.14591786802309770, 105.6239096053143669 ) ) ;
#66849=CARTESIAN_POINT ( 'NONE',  ( -16.51473224551069308, -9.474510206698971260, 51.66557627198102409 ) ) ;
#66851=CARTESIAN_POINT ( 'NONE',  ( -19.03943276465977164, 0.05219959533909376836, 26.24890960531435624 ) ) ;
#66853=CARTESIAN_POINT ( 'NONE',  ( -19.03943276465977164, 0.05219959533909376836, 96.24890960531436690 ) ) ;
#66854=CARTESIAN_POINT ( 'NONE',  ( -16.53943276465976808, -0.05219959533934237506, 73.75109039468567573 ) ) ;
#66855=CARTESIAN_POINT ( 'NONE',  ( 21.53943276465977519, 0.05219959533937863772, 111.2510903946856899 ) ) ;
#66856=CARTESIAN_POINT ( 'NONE',  ( -5.823673210054116645, -21.52544592524344225, 47.29057627198103120 ) ) ;
#66857=CARTESIAN_POINT ( 'NONE',  ( 4.483927247898790824, -16.52544592524335698, 75.20942372801901854 ) ) ;
#66858=CARTESIAN_POINT ( 'NONE',  ( -13.97604488694547697, 13.89961937509957934, 78.12609039468567573 ) ) ;
#66859=CARTESIAN_POINT ( 'NONE',  ( 5.153800228976335163, 19.02544592524342804, 39.79057627198100988 ) ) ;
#66860=CARTESIAN_POINT ( 'NONE',  ( -9.474510206698964154, 16.51473224551069663, 80.41557627198103830 ) ) ;
#66861=CARTESIAN_POINT ( 'NONE',  ( 5.049401038298161559, -19.05341960407611168, 37.70724293864768839 ) ) ;
#66862=CARTESIAN_POINT ( 'NONE',  ( -16.46253265017146816, -9.564922557961047289, 74.16775706135234714 ) ) ;
#66864=CARTESIAN_POINT ( 'NONE',  ( -5.049401038298153566, 19.05341960407611168, 100.2072429386476955 ) ) ;
#66865=CARTESIAN_POINT ( 'NONE',  ( 0.05219959533910956823, 16.53943276465976808, 54.99890960531435269 ) ) ;
#66866=CARTESIAN_POINT ( 'NONE',  ( 5.719274019375991003, -21.55341960407610458, 47.70724293864770260 ) ) ;
#66867=CARTESIAN_POINT ( 'NONE',  ( -17.50000000000000000, 3.471454075611697832, 104.4833258114436347 ) ) ;
#66868=CARTESIAN_POINT ( 'NONE',  ( 5.153800228976615827, -19.02544592524334988, 35.20942372801899722 ) ) ;
#66870=CARTESIAN_POINT ( 'NONE',  ( -19.02544592524342804, 5.153800228976336051, 56.04057627198100988 ) ) ;
#66872=CARTESIAN_POINT ( 'NONE',  ( -14.29746914071037622, -8.314922557961029526, 34.16775706135234714 ) ) ;
#66875=CARTESIAN_POINT ( 'NONE',  ( 8.224510206698742110, 14.34966873604972548, 82.08442372801901854 ) ) ;
#66876=CARTESIAN_POINT ( 'NONE',  ( -15.72974639402197994, 15.80617190586746368, 100.6239096053143811 ) ) ;
#66877=CARTESIAN_POINT ( 'NONE',  ( 4.483927247898790824, -16.52544592524335698, 40.20942372801901854 ) ) ;
#66878=CARTESIAN_POINT ( 'NONE',  ( 16.46253265017160672, -9.564922557960803928, 48.33224293864769550 ) ) ;
#66879=CARTESIAN_POINT ( 'NONE',  ( 5.153800228976335163, 19.02544592524342804, 114.7905762719810241 ) ) ;
#66880=CARTESIAN_POINT ( 'NONE',  ( -21.52544592524334988, -5.823673210054445271, 43.95942372801902565 ) ) ;
#66881=CARTESIAN_POINT ( 'NONE',  ( 16.51473224551083163, -9.474510206698727899, 55.83442372801899722 ) ) ;
#66882=CARTESIAN_POINT ( 'NONE',  ( 0.05219959533937995610, -21.53943276465977519, 100.0010903946857042 ) ) ;
#66883=CARTESIAN_POINT ( 'NONE',  ( 9.474510206698971260, -16.51473224551069308, 22.91557627198102765 ) ) ;
#66884=CARTESIAN_POINT ( 'NONE',  ( 16.53943276465976808, -0.05219959533910856209, 43.74890960531435979 ) ) ;
#66885=CARTESIAN_POINT ( 'NONE',  ( 19.01529144963332030, 5.500000000000156319, 43.73431955728440101 ) ) ;
#66886=CARTESIAN_POINT ( 'NONE',  ( -5.823673210054116645, -21.52544592524344225, 57.29057627198103120 ) ) ;
#66888=CARTESIAN_POINT ( 'NONE',  ( 9.474510206698971260, -16.51473224551069308, 102.9155762719810241 ) ) ;
#66889=CARTESIAN_POINT ( 'NONE',  ( 4.379528057220339221, -16.55341960407611168, 97.70724293864772392 ) ) ;
#66890=CARTESIAN_POINT ( 'NONE',  ( -14.29746914071037622, -8.314922557961029526, 19.16775706135234714 ) ) ;
#66891=CARTESIAN_POINT ( 'NONE',  ( 0.05219959533934541429, -16.53943276465976808, 105.0010903946856757 ) ) ;
#66893=CARTESIAN_POINT ( 'NONE',  ( -13.97604488694527625, -13.89961937509977652, 101.8739096053143811 ) ) ;
#66894=CARTESIAN_POINT ( 'NONE',  ( 18.67979575497178502, 10.72451020669898547, 104.1655762719810241 ) ) ;
#66895=CARTESIAN_POINT ( 'NONE',  ( -4.379528057220328563, 16.55341960407611168, 30.20724293864769550 ) ) ;
#66897=CARTESIAN_POINT ( 'NONE',  ( 5.153800228976615827, -19.02544592524334988, 95.20942372801897591 ) ) ;
#66898=CARTESIAN_POINT ( 'NONE',  ( -10.81492255796105439, 18.62759615963255655, 107.9177570613523471 ) ) ;
#66899=CARTESIAN_POINT ( 'NONE',  ( 16.55341960407611168, 4.379528057220329451, 33.95724293864769550 ) ) ;
#66900=CARTESIAN_POINT ( 'NONE',  ( 18.67979575497178502, 10.72451020669898547, 94.16557627198103830 ) ) ;
#66901=CARTESIAN_POINT ( 'NONE',  ( 18.62759615963271287, -10.81492255796078972, 53.33224293864769550 ) ) ;
#66902=CARTESIAN_POINT ( 'NONE',  ( 5.049401038298161559, -19.05341960407611168, 62.70724293864769550 ) ) ;
#66903=CARTESIAN_POINT ( 'NONE',  ( 16.52544592524342804, -4.483927247898539470, 28.54057627198103120 ) ) ;
#66904=CARTESIAN_POINT ( 'NONE',  ( -0.05219959533909027116, -19.03943276465977164, 82.49890960531436690 ) ) ;
#66905=ORIENTED_EDGE ( 'NONE', *, *, #74286, .T. ) ;
#66906=CARTESIAN_POINT ( 'NONE',  ( -9.474510206698964154, 16.51473224551069663, 80.41557627198103830 ) ) ;
#66907=CARTESIAN_POINT ( 'NONE',  ( -19.05341960407617563, 5.049401038297882671, 38.54275706135233293 ) ) ;
#66908=CARTESIAN_POINT ( 'NONE',  ( -10.72451020669898014, 18.67979575497178502, 80.41557627198103830 ) ) ;
#66909=CARTESIAN_POINT ( 'NONE',  ( 12.14591786802309770, 12.06949235617756955, 84.37390960531438111 ) ) ;
#66910=CARTESIAN_POINT ( 'NONE',  ( -21.55341960407619339, 5.719274019375674811, 38.54275706135234714 ) ) ;
#66912=CARTESIAN_POINT ( 'NONE',  ( -8.224510206698735004, -14.34966873604973081, 109.5844237280190328 ) ) ;
#66913=CARTESIAN_POINT ( 'NONE',  ( 12.14591786802309770, 12.06949235617756955, 114.3739096053143527 ) ) ;
#66914=CARTESIAN_POINT ( 'NONE',  ( -9.564922557960796823, -16.46253265017161027, 82.08224293864768129 ) ) ;
#66916=CARTESIAN_POINT ( 'NONE',  ( -9.564922557960796823, -16.46253265017161027, 22.08224293864768839 ) ) ;
#66917=CARTESIAN_POINT ( 'NONE',  ( 14.29746914071049879, -8.314922557960816363, 48.33224293864770260 ) ) ;
#66918=CARTESIAN_POINT ( 'NONE',  ( 15.72974639402176855, 15.80617190586768217, 56.87609039468568994 ) ) ;
#66920=CARTESIAN_POINT ( 'NONE',  ( -5.049401038298153566, 19.05341960407611168, 40.20724293864768839 ) ) ;
#66921=CARTESIAN_POINT ( 'NONE',  ( 19.03943276465977164, -0.05219959533909143690, 53.74890960531436690 ) ) ;
#66923=CARTESIAN_POINT ( 'NONE',  ( 10.72451020669871369, 18.67979575497193778, 107.0844237280190043 ) ) ;
#66924=CARTESIAN_POINT ( 'NONE',  ( -4.379528057220086978, -16.55341960407618274, 64.79275706135234714 ) ) ;
#66925=B_SPLINE_CURVE_WITH_KNOTS ( 'NONE', 3,
 ( #20345, #81994, #113350, #175042, #77630, #167668, #59475, #124122, #154477, #32132, #14974, #76634, #125135, #31141, #151509, #15970, #186833, #13001, #121149, #60465, #153478, #109958, #185821, #74664, #182842, #48301, #183828, #138312, #46302, #107958, #92789, #89828 ),
 .UNSPECIFIED., .F., .F.,
 ( 4, 2, 2, 2, 2, 2, 2, 2, 2, 2, 2, 2, 2, 2, 2, 4 ),
 ( 1.599336020787782259E-17, 0.0003712461730036926326, 0.0007424923460073693275, 0.001113738519011045914, 0.001484984692014722609, 0.002227477038022073613, 0.002598723211025752260, 0.002969969384029431340, 0.003341215557033109986, 0.003712461730036789500, 0.004083707903040468580, 0.004454954076044147226, 0.004826200249047826740, 0.005197446422051505387, 0.005568692595055184900, 0.005939938768058864414 ),
 .UNSPECIFIED. ) ;
#66926=CARTESIAN_POINT ( 'NONE',  ( 21.53943276465977519, 0.05219959533937863772, 96.25109039468568994 ) ) ;
#66927=CARTESIAN_POINT ( 'NONE',  ( 19.03943276465977164, -0.05219959533909143690, 113.7489096053143669 ) ) ;
#66928=CARTESIAN_POINT ( 'NONE',  ( -0.05219959533936034679, 19.03943276465977164, 107.5010903946856615 ) ) ;
#66929=CARTESIAN_POINT ( 'NONE',  ( -15.80617190586768217, 15.72974639402176855, 68.12609039468567573 ) ) ;
#66930=CARTESIAN_POINT ( 'NONE',  ( -16.52544592524335698, -4.483927247898792601, 33.95942372801901143 ) ) ;
#66931=CARTESIAN_POINT ( 'NONE',  ( -10.72451020669898014, 18.67979575497178502, 90.41557627198103830 ) ) ;
#66932=CARTESIAN_POINT ( 'NONE',  ( -19.05341960407617563, 5.049401038297882671, 98.54275706135233293 ) ) ;
#66933=CARTESIAN_POINT ( 'NONE',  ( -13.89961937509977652, 13.97604488694528158, 65.62390960531436690 ) ) ;
#66934=CARTESIAN_POINT ( 'NONE',  ( -19.05341960407617563, 5.049401038297882671, 108.5427570613523187 ) ) ;
#66936=CARTESIAN_POINT ( 'NONE',  ( 5.153800228976615827, -19.02544592524334988, 100.2094237280190043 ) ) ;
#66937=CARTESIAN_POINT ( 'NONE',  ( 4.483927247898545687, 16.52544592524342804, 59.79057627198103120 ) ) ;
#66938=CARTESIAN_POINT ( 'NONE',  ( 0.05219959533936267826, -19.03943276465977164, 75.00109039468566152 ) ) ;
#66939=CARTESIAN_POINT ( 'NONE',  ( -4.379528057220086978, -16.55341960407618274, 79.79275706135236135 ) ) ;
#66940=ADVANCED_FACE ( 'NONE', ( #136363 ), #7389, .T. ) ;
#66941=CARTESIAN_POINT ( 'NONE',  ( 21.53943276465977519, -0.05219959533907433946, 113.7489096053143527 ) ) ;
#66942=CARTESIAN_POINT ( 'NONE',  ( 0.05219959533909260263, 19.03943276465977164, 44.99890960531435979 ) ) ;
#66943=CARTESIAN_POINT ( 'NONE',  ( -0.05219959533909027116, -19.03943276465977164, 62.49890960531435979 ) ) ;
#66944=CARTESIAN_POINT ( 'NONE',  ( -8.314922557961024197, 14.29746914071037800, 77.91775706135231871 ) ) ;
#66947=ORIENTED_EDGE ( 'NONE', *, *, #8998, .T. ) ;
#66948=CARTESIAN_POINT ( 'NONE',  ( 15.80617190586769283, -15.72974639402175789, 110.6260903946857042 ) ) ;
#66949=CARTESIAN_POINT ( 'NONE',  ( -16.51473224551069308, -9.474510206698971260, 26.66557627198103120 ) ) ;
#66951=CARTESIAN_POINT ( 'NONE',  ( 16.55341960407618274, -4.379528057220086978, 21.04275706135234714 ) ) ;
#66952=CARTESIAN_POINT ( 'NONE',  ( 15.72974639402199770, -15.80617190586745480, 48.12390960531436690 ) ) ;
#66953=CARTESIAN_POINT ( 'NONE',  ( 9.474510206698729675, 16.51473224551082808, 47.08442372801900433 ) ) ;
#66954=CARTESIAN_POINT ( 'NONE',  ( -8.314922557961024197, 14.29746914071037800, 32.91775706135234714 ) ) ;
#66955=CARTESIAN_POINT ( 'NONE',  ( -9.564922557960796823, -16.46253265017161027, 27.08224293864769550 ) ) ;
#66956=B_SPLINE_CURVE_WITH_KNOTS ( 'NONE', 3,
 ( #53867, #191372, #161037, #69025, #177229, #178223 ),
 .UNSPECIFIED., .F., .F.,
 ( 4, 2, 4 ),
 ( 0.000000000000000000, 0.0003837532665554159472, 0.0007675065331108318943 ),
 .UNSPECIFIED. ) ;
#66957=CARTESIAN_POINT ( 'NONE',  ( 19.05341960407611168, 5.049401038298154454, 53.95724293864770260 ) ) ;
#66958=CARTESIAN_POINT ( 'NONE',  ( 21.52544592524344225, -5.823673210054117533, 88.54057627198103830 ) ) ;
#66960=CARTESIAN_POINT ( 'NONE',  ( 19.03943276465977164, -0.05219959533909143690, 48.74890960531435979 ) ) ;
#66962=CARTESIAN_POINT ( 'NONE',  ( 19.03943276465977164, 0.05219959533936151252, 91.25109039468566152 ) ) ;
#66963=CARTESIAN_POINT ( 'NONE',  ( -12.06949235617756955, 12.14591786802309770, 60.62390960531437401 ) ) ;
#66965=CARTESIAN_POINT ( 'NONE',  ( 5.719274019375673035, 21.55341960407619339, 102.2927570613523613 ) ) ;
#66966=CARTESIAN_POINT ( 'NONE',  ( -18.67979575497178146, -10.72451020669898902, 101.6655762719810383 ) ) ;
#66967=CARTESIAN_POINT ( 'NONE',  ( 21.53943276465977519, 0.05219959533937863772, 86.25109039468568994 ) ) ;
#66968=CARTESIAN_POINT ( 'NONE',  ( 9.474510206698971260, -16.51473224551069308, 27.91557627198103120 ) ) ;
#66969=CARTESIAN_POINT ( 'NONE',  ( 5.823673210054444382, -21.52544592524334988, 80.20942372801901854 ) ) ;
#66970=CARTESIAN_POINT ( 'NONE',  ( -12.14591786802326823, 12.06949235617739902, 113.1260903946856899 ) ) ;
#66971=CARTESIAN_POINT ( 'NONE',  ( -21.52544592524334988, -5.823673210054445271, 73.95942372801901854 ) ) ;
#66972=CARTESIAN_POINT ( 'NONE',  ( -5.049401038298153566, 19.05341960407611168, 70.20724293864769550 ) ) ;
#66973=CARTESIAN_POINT ( 'NONE',  ( 5.719274019375673035, 21.55341960407619339, 37.29275706135235424 ) ) ;
#66974=CARTESIAN_POINT ( 'NONE',  ( -19.03943276465977164, 0.05219959533909376836, 86.24890960531436690 ) ) ;
#66975=CARTESIAN_POINT ( 'NONE',  ( 14.29746914071049879, -8.314922557960816363, 98.33224293864769550 ) ) ;
#66976=CARTESIAN_POINT ( 'NONE',  ( -4.483927247898539470, -16.52544592524342804, 67.29057627198103830 ) ) ;
#66977=CARTESIAN_POINT ( 'NONE',  ( -10.81492255796078084, -18.62759615963271287, 67.08224293864770971 ) ) ;
#66978=CARTESIAN_POINT ( 'NONE',  ( -0.05219959533909027116, -19.03943276465977164, 67.49890960531436690 ) ) ;
#66979=CARTESIAN_POINT ( 'NONE',  ( 21.55341960407610458, 5.719274019375980345, 88.95724293864769550 ) ) ;
#66980=CARTESIAN_POINT ( 'NONE',  ( 13.97604488694548053, -13.89961937509957401, 60.62609039468564731 ) ) ;
#66981=CARTESIAN_POINT ( 'NONE',  ( -9.564922557961040184, 16.46253265017147172, 37.91775706135233293 ) ) ;
#66982=CARTESIAN_POINT ( 'NONE',  ( -16.55341960407611168, -4.379528057220339221, 76.45724293864769550 ) ) ;
#66984=CARTESIAN_POINT ( 'NONE',  ( 10.81492255796078972, 18.62759615963270932, 59.58224293864770260 ) ) ;
#66986=CARTESIAN_POINT ( 'NONE',  ( -12.06949235617739369, -12.14591786802326823, 94.37609039468568994 ) ) ;
#66988=CARTESIAN_POINT ( 'NONE',  ( 16.51473224551083163, -9.474510206698727899, 95.83442372801900433 ) ) ;
#66989=CARTESIAN_POINT ( 'NONE',  ( 16.52544592524342804, -4.483927247898539470, 63.54057627198103830 ) ) ;
#66991=CARTESIAN_POINT ( 'NONE',  ( 19.05341960407611168, 5.049401038298154454, 58.95724293864768129 ) ) ;
#66992=CARTESIAN_POINT ( 'NONE',  ( 4.379528057220339221, -16.55341960407611168, 57.70724293864770260 ) ) ;
#66993=CARTESIAN_POINT ( 'NONE',  ( -5.049401038298153566, 19.05341960407611168, 105.2072429386476671 ) ) ;
#66994=CARTESIAN_POINT ( 'NONE',  ( -5.153800228976607833, 19.02544592524334988, 72.70942372801900433 ) ) ;
#66995=CARTESIAN_POINT ( 'NONE',  ( -5.049401038298153566, 19.05341960407611168, 70.20724293864769550 ) ) ;
#66996=CARTESIAN_POINT ( 'NONE',  ( -0.05219959533909027116, -19.03943276465977164, 82.49890960531436690 ) ) ;
#66997=CARTESIAN_POINT ( 'NONE',  ( 5.153800228976335163, 19.02544592524342804, 69.79057627198103830 ) ) ;
#66998=CARTESIAN_POINT ( 'NONE',  ( -15.72974639402197994, 15.80617190586746368, 65.62390960531436690 ) ) ;
#66999=CARTESIAN_POINT ( 'NONE',  ( 8.314922557961029526, -14.29746914071037800, 60.41775706135235424 ) ) ;
#67000=CARTESIAN_POINT ( 'NONE',  ( -16.46253265017146816, -9.564922557961047289, 104.1677570613523329 ) ) ;
#67001=CARTESIAN_POINT ( 'NONE',  ( 19.02544592524343514, -5.153800228976328945, 43.54057627198103120 ) ) ;
#67002=CARTESIAN_POINT ( 'NONE',  ( 15.80617190586746368, 15.72974639402197994, 49.37390960531436690 ) ) ;
#67003=CARTESIAN_POINT ( 'NONE',  ( 16.46253265017146816, 9.564922557961045513, 91.66775706135234714 ) ) ;
#67004=CARTESIAN_POINT ( 'NONE',  ( -16.55341960407611168, -4.379528057220339221, 26.45724293864768839 ) ) ;
#67005=CARTESIAN_POINT ( 'NONE',  ( 10.72451020669871369, 18.67979575497193778, 32.08442372801901854 ) ) ;
#67006=CARTESIAN_POINT ( 'NONE',  ( 19.03943276465977164, 0.05219959533936151252, 31.25109039468566863 ) ) ;
#67007=CARTESIAN_POINT ( 'NONE',  ( 16.52544592524335698, 4.483927247898782831, 66.45942372801903275 ) ) ;
#67008=CARTESIAN_POINT ( 'NONE',  ( -8.224510206698735004, -14.34966873604973081, 99.58442372801900433 ) ) ;
#67010=CARTESIAN_POINT ( 'NONE',  ( -8.224510206698735004, -14.34966873604973081, 84.58442372801903275 ) ) ;
#67011=CARTESIAN_POINT ( 'NONE',  ( -15.80617190586745835, -15.72974639402198527, 31.87390960531435979 ) ) ;
#67012=CARTESIAN_POINT ( 'NONE',  ( -14.34966873604972548, 8.224510206698743886, 33.33442372801900433 ) ) ;
#67013=CARTESIAN_POINT ( 'NONE',  ( -13.89961937509977652, 13.97604488694528158, 40.62390960531435979 ) ) ;
#67014=CARTESIAN_POINT ( 'NONE',  ( 19.03943276465977164, -0.05219959533909143690, 43.74890960531435979 ) ) ;
#67015=CARTESIAN_POINT ( 'NONE',  ( -9.564922557960796823, -16.46253265017161027, 67.08224293864769550 ) ) ;
#67016=CARTESIAN_POINT ( 'NONE',  ( -10.72451020669870658, -18.67979575497194134, 44.58442372801901854 ) ) ;
#67017=CARTESIAN_POINT ( 'NONE',  ( 16.53943276465976808, 0.05219959533934440121, 46.25109039468567573 ) ) ;
#67018=CARTESIAN_POINT ( 'NONE',  ( -12.14591786802309592, -12.06949235617757132, 21.87390960531436690 ) ) ;
#67019=CARTESIAN_POINT ( 'NONE',  ( 19.05341960407611168, 5.049401038298154454, 33.95724293864769550 ) ) ;
#67020=CARTESIAN_POINT ( 'NONE',  ( -18.67979575497193778, 10.72451020669871902, 113.3344237280190328 ) ) ;
#67021=CARTESIAN_POINT ( 'NONE',  ( -13.89961937509957401, -13.97604488694547875, 104.3760903946856757 ) ) ;
#67022=CARTESIAN_POINT ( 'NONE',  ( 9.564922557961047289, -16.46253265017146816, 75.41775706135234714 ) ) ;
#67023=CARTESIAN_POINT ( 'NONE',  ( -8.314922557960811034, -14.29746914071050412, 67.08224293864770971 ) ) ;
#67024=CARTESIAN_POINT ( 'NONE',  ( 5.049401038298161559, -19.05341960407611168, 32.70724293864768129 ) ) ;
#67025=CARTESIAN_POINT ( 'NONE',  ( 5.049401038297881783, 19.05341960407617563, 77.29275706135231871 ) ) ;
#67027=CARTESIAN_POINT ( 'NONE',  ( -18.67979575497193778, 10.72451020669871902, 78.33442372801901854 ) ) ;
#67028=CARTESIAN_POINT ( 'NONE',  ( -12.06949235617739369, -12.14591786802326823, 34.37609039468568284 ) ) ;
#67030=CARTESIAN_POINT ( 'NONE',  ( -5.719274019375978568, 21.55341960407610458, 30.20724293864769550 ) ) ;
#67031=CARTESIAN_POINT ( 'NONE',  ( -16.55341960407617563, 4.379528057220093196, 28.54275706135234358 ) ) ;
#67032=CARTESIAN_POINT ( 'NONE',  ( 13.97604488694527802, 13.89961937509977830, 29.37390960531435624 ) ) ;
#67033=CARTESIAN_POINT ( 'NONE',  ( 19.05341960407617918, -5.049401038297876454, 31.04275706135232227 ) ) ;
#67035=CARTESIAN_POINT ( 'NONE',  ( 5.153800228976335163, 19.02544592524342804, 39.79057627198100988 ) ) ;
#67036=CARTESIAN_POINT ( 'NONE',  ( 18.22780087662126647, 5.499999999999818812, 56.48236817873107185 ) ) ;
#67037=CARTESIAN_POINT ( 'NONE',  ( -5.049401038298153566, 19.05341960407611168, 55.20724293864769550 ) ) ;
#67038=CARTESIAN_POINT ( 'NONE',  ( 17.50000000000001776, -4.049696124445898882, 111.6803967066594794 ) ) ;
#67039=CARTESIAN_POINT ( 'NONE',  ( 19.05341960407617918, -5.049401038297876454, 26.04275706135233293 ) ) ;
#67040=CARTESIAN_POINT ( 'NONE',  ( -14.29746914071049879, 8.314922557960819915, 30.83224293864770260 ) ) ;
#67041=CARTESIAN_POINT ( 'NONE',  ( 16.51473224551069308, 9.474510206698969483, 34.16557627198102409 ) ) ;
#67042=CARTESIAN_POINT ( 'NONE',  ( 9.474510206698971260, -16.51473224551069308, 92.91557627198103830 ) ) ;
#67043=CARTESIAN_POINT ( 'NONE',  ( -15.80617190586768217, 15.72974639402176855, 68.12609039468567573 ) ) ;
#67044=CARTESIAN_POINT ( 'NONE',  ( 16.46253265017160672, -9.564922557960803928, 33.33224293864770260 ) ) ;
#67046=CARTESIAN_POINT ( 'NONE',  ( 18.62759615963255655, 10.81492255796105972, 71.66775706135234714 ) ) ;
#67047=CARTESIAN_POINT ( 'NONE',  ( -16.51473224551082808, 9.474510206698731452, 93.33442372801900433 ) ) ;
#67048=CARTESIAN_POINT ( 'NONE',  ( -5.719274019375978568, 21.55341960407610458, 30.20724293864769550 ) ) ;
#67049=CARTESIAN_POINT ( 'NONE',  ( 9.564922557960805705, 16.46253265017160317, 39.58224293864768839 ) ) ;
#67050=CARTESIAN_POINT ( 'NONE',  ( 10.81492255796078972, 18.62759615963270932, 114.5822429386477097 ) ) ;
#67051=CARTESIAN_POINT ( 'NONE',  ( -9.474510206698720793, -16.51473224551083518, 29.58442372801900433 ) ) ;
#67052=CARTESIAN_POINT ( 'NONE',  ( 14.34966873604960469, 8.224510206698951720, 114.1655762719810383 ) ) ;
#67053=CARTESIAN_POINT ( 'NONE',  ( -19.05341960407611168, -5.049401038298163336, 66.45724293864769550 ) ) ;
#67054=CARTESIAN_POINT ( 'NONE',  ( 19.05341960407617918, -5.049401038297876454, 101.0427570613523045 ) ) ;
#67055=CARTESIAN_POINT ( 'NONE',  ( -14.29746914071049879, 8.314922557960819915, 75.83224293864769550 ) ) ;
#67056=CARTESIAN_POINT ( 'NONE',  ( 21.55341960407610458, 5.719274019375980345, 23.95724293864769550 ) ) ;
#67057=CARTESIAN_POINT ( 'NONE',  ( -9.564922557961040184, 16.46253265017147172, 82.91775706135233293 ) ) ;
#67058=CARTESIAN_POINT ( 'NONE',  ( -10.81492255796078084, -18.62759615963271287, 87.08224293864769550 ) ) ;
#67059=CARTESIAN_POINT ( 'NONE',  ( 0.05219959533937995610, -21.53943276465977519, 45.00109039468568284 ) ) ;
#67060=CARTESIAN_POINT ( 'NONE',  ( -12.06949235617739369, -12.14591786802326823, 49.37609039468569705 ) ) ;
#67061=CARTESIAN_POINT ( 'NONE',  ( -8.224510206698735004, -14.34966873604973081, 49.58442372801901143 ) ) ;
#67062=CARTESIAN_POINT ( 'NONE',  ( 0.05219959533937995610, -21.53943276465977519, 55.00109039468568284 ) ) ;
#67063=CARTESIAN_POINT ( 'NONE',  ( 15.80617190586746368, 15.72974639402197994, 59.37390960531436690 ) ) ;
#67064=CARTESIAN_POINT ( 'NONE',  ( -5.153800228976328057, -19.02544592524343514, 47.29057627198102409 ) ) ;
#67066=CARTESIAN_POINT ( 'NONE',  ( 14.34966873604972726, -8.224510206698740333, 80.83442372801901854 ) ) ;
#67067=CARTESIAN_POINT ( 'NONE',  ( -21.52544592524343514, 5.823673210054127303, 101.0405762719810383 ) ) ;
#67068=CARTESIAN_POINT ( 'NONE',  ( 0.05219959533910956823, 16.53943276465976808, 54.99890960531435269 ) ) ;
#67069=CARTESIAN_POINT ( 'NONE',  ( 4.379528057220092307, 16.55341960407617563, 62.29275706135236845 ) ) ;
#67070=CARTESIAN_POINT ( 'NONE',  ( -19.02544592524334988, -5.153800228976617603, 103.9594237280190043 ) ) ;
#67071=CARTESIAN_POINT ( 'NONE',  ( 15.80617190586746368, 15.72974639402197994, 99.37390960531436690 ) ) ;
#67072=CARTESIAN_POINT ( 'NONE',  ( 8.224510206698953496, -14.34966873604960469, 42.91557627198103120 ) ) ;
#67073=ORIENTED_EDGE ( 'NONE', *, *, #19257, .F. ) ;
#67075=CARTESIAN_POINT ( 'NONE',  ( -5.719274019375978568, 21.55341960407610458, 75.20724293864769550 ) ) ;
#67076=CARTESIAN_POINT ( 'NONE',  ( -8.314922557960811034, -14.29746914071050412, 22.08224293864769194 ) ) ;
#67077=ORIENTED_EDGE ( 'NONE', *, *, #69228, .T. ) ;
#67079=CARTESIAN_POINT ( 'NONE',  ( 21.52544592524344225, -5.823673210054117533, 103.5405762719810383 ) ) ;
#67080=CARTESIAN_POINT ( 'NONE',  ( -5.719274019375978568, 21.55341960407610458, 110.2072429386477239 ) ) ;
#67081=CARTESIAN_POINT ( 'NONE',  ( -12.14591786802309592, -12.06949235617757132, 36.87390960531435979 ) ) ;
#67082=CARTESIAN_POINT ( 'NONE',  ( 16.53943276465976808, 0.05219959533934440121, 46.25109039468567573 ) ) ;
#67084=CARTESIAN_POINT ( 'NONE',  ( -13.97604488694527625, -13.89961937509977652, 51.87390960531436690 ) ) ;
#67085=CARTESIAN_POINT ( 'NONE',  ( -16.46253265017160317, 9.564922557960807481, 70.83224293864770971 ) ) ;
#67087=CARTESIAN_POINT ( 'NONE',  ( -18.67979575497178146, -10.72451020669898902, 36.66557627198103120 ) ) ;
#67089=CARTESIAN_POINT ( 'NONE',  ( 9.474510206698729675, 16.51473224551082808, 102.0844237280190043 ) ) ;
#67090=CARTESIAN_POINT ( 'NONE',  ( -9.564922557961040184, 16.46253265017147172, 52.91775706135233293 ) ) ;
#67091=CARTESIAN_POINT ( 'NONE',  ( 18.62759615963271287, -10.81492255796078972, 108.3322429386477097 ) ) ;
#67092=CARTESIAN_POINT ( 'NONE',  ( 12.14591786802309770, 12.06949235617756955, 29.37390960531435269 ) ) ;
#67093=CARTESIAN_POINT ( 'NONE',  ( 13.89961937509977652, -13.97604488694527269, 78.12390960531433848 ) ) ;
#67094=CARTESIAN_POINT ( 'NONE',  ( 5.719274019375991003, -21.55341960407610458, 42.70724293864770260 ) ) ;
#67095=CARTESIAN_POINT ( 'NONE',  ( 21.53943276465977519, -0.05219959533907433946, 83.74890960531435269 ) ) ;
#67096=CARTESIAN_POINT ( 'NONE',  ( -8.314922557961024197, 14.29746914071037800, 27.91775706135234358 ) ) ;
#67097=CARTESIAN_POINT ( 'NONE',  ( 15.80617190586746368, 15.72974639402197994, 29.37390960531435269 ) ) ;
#67098=CARTESIAN_POINT ( 'NONE',  ( -5.823673210054431948, 21.52544592524334988, 77.70942372801900433 ) ) ;
#67099=CARTESIAN_POINT ( 'NONE',  ( 13.89961937509977652, -13.97604488694527269, 73.12390960531436690 ) ) ;
#67100=CARTESIAN_POINT ( 'NONE',  ( 13.97604488694527802, 13.89961937509977652, 34.37390960531436690 ) ) ;
#67101=CARTESIAN_POINT ( 'NONE',  ( 19.05341960407611168, 5.049401038298154454, 83.95724293864766707 ) ) ;
#67102=CARTESIAN_POINT ( 'NONE',  ( -14.34966873604960291, -8.224510206698953496, 91.66557627198103830 ) ) ;
#67103=ORIENTED_EDGE ( 'NONE', *, *, #92660, .F. ) ;
#67104=CARTESIAN_POINT ( 'NONE',  ( -13.97604488694547697, 13.89961937509957934, 108.1260903946856331 ) ) ;
#67106=CARTESIAN_POINT ( 'NONE',  ( 5.049401038298161559, -19.05341960407611168, 67.70724293864769550 ) ) ;
#67108=CARTESIAN_POINT ( 'NONE',  ( 18.67979575497194134, -10.72451020669871369, 90.83442372801901854 ) ) ;
#67109=CARTESIAN_POINT ( 'NONE',  ( 16.51473224551069308, 9.474510206698969483, 114.1655762719810241 ) ) ;
#67110=CARTESIAN_POINT ( 'NONE',  ( -4.483927247898782831, 16.52544592524335698, 82.70942372801900433 ) ) ;
#67112=CARTESIAN_POINT ( 'NONE',  ( -0.05219959533936034679, 19.03943276465977164, 52.50109039468566863 ) ) ;
#67113=CARTESIAN_POINT ( 'NONE',  ( 0.05219959533936267826, -19.03943276465977164, 20.00109039468567218 ) ) ;
#67117=CARTESIAN_POINT ( 'NONE',  ( -12.14591786802309592, -12.06949235617757132, 26.87390960531435979 ) ) ;
#67119=CARTESIAN_POINT ( 'NONE',  ( -16.52544592524335698, -4.483927247898792601, 103.9594237280190185 ) ) ;
#67121=CARTESIAN_POINT ( 'NONE',  ( 16.53943276465976808, 0.05219959533934440121, 86.25109039468568994 ) ) ;
#67122=CARTESIAN_POINT ( 'NONE',  ( 5.823673210054444382, -21.52544592524334988, 100.2094237280190043 ) ) ;
#67123=CARTESIAN_POINT ( 'NONE',  ( -13.97604488694547697, 13.89961937509957934, 108.1260903946856331 ) ) ;
#67124=CARTESIAN_POINT ( 'NONE',  ( 18.67979575497194134, -10.72451020669871369, 60.83442372801901854 ) ) ;
#67125=CARTESIAN_POINT ( 'NONE',  ( -19.02544592524334988, -5.153800228976617603, 38.95942372801900433 ) ) ;
#67126=CARTESIAN_POINT ( 'NONE',  ( -16.51473224551069308, -9.474510206698971260, 81.66557627198103830 ) ) ;
#67127=CARTESIAN_POINT ( 'NONE',  ( -19.03943276465977164, 0.05219959533909376836, 56.24890960531435979 ) ) ;
#67129=CARTESIAN_POINT ( 'NONE',  ( -18.67979575497178146, -10.72451020669898902, 96.66557627198102409 ) ) ;
#67130=CARTESIAN_POINT ( 'NONE',  ( 21.55341960407610458, 5.719274019375980345, 48.95724293864770971 ) ) ;
#67131=CARTESIAN_POINT ( 'NONE',  ( -0.05219959533909027116, -19.03943276465977164, 42.49890960531435269 ) ) ;
#67132=CARTESIAN_POINT ( 'NONE',  ( -12.14591786802326823, 12.06949235617739902, 63.12609039468568994 ) ) ;
#67133=EDGE_CURVE ( 'NONE', #174275, #44164, #61583, .T. ) ;
#67134=ORIENTED_EDGE ( 'NONE', *, *, #34865, .T. ) ;
#67135=CARTESIAN_POINT ( 'NONE',  ( -15.72974639402176322, -15.80617190586768395, 49.37609039468569705 ) ) ;
#67136=CARTESIAN_POINT ( 'NONE',  ( -16.52544592524342804, 4.483927247898546575, 66.04057627198103830 ) ) ;
#67138=CARTESIAN_POINT ( 'NONE',  ( 4.483927247898790824, -16.52544592524335698, 45.20942372801901854 ) ) ;
#67139=CARTESIAN_POINT ( 'NONE',  ( -8.314922557960811034, -14.29746914071050412, 107.0822429386476955 ) ) ;
#67140=CARTESIAN_POINT ( 'NONE',  ( -16.51473224551082808, 9.474510206698731452, 58.33442372801900433 ) ) ;
#67141=CARTESIAN_POINT ( 'NONE',  ( 0.05219959533910956823, 16.53943276465976808, 74.99890960531435269 ) ) ;
#67142=CARTESIAN_POINT ( 'NONE',  ( 18.62759615963255655, 10.81492255796105972, 26.66775706135235424 ) ) ;
#67144=CARTESIAN_POINT ( 'NONE',  ( -15.72974639402197994, 15.80617190586746368, 90.62390960531436690 ) ) ;
#67145=CARTESIAN_POINT ( 'NONE',  ( -0.05219959533909027116, -19.03943276465977164, 97.49890960531436690 ) ) ;
#67146=CARTESIAN_POINT ( 'NONE',  ( 14.29746914071049879, -8.314922557960816363, 78.33224293864770971 ) ) ;
#67149=CARTESIAN_POINT ( 'NONE',  ( 19.02544592524334988, 5.153800228976608722, 86.45942372801900433 ) ) ;
#67150=CARTESIAN_POINT ( 'NONE',  ( 15.72974639402176855, 15.80617190586768217, 26.87609039468567218 ) ) ;
#67151=CARTESIAN_POINT ( 'NONE',  ( -19.05341960407611168, -5.049401038298163336, 76.45724293864769550 ) ) ;
#67152=CARTESIAN_POINT ( 'NONE',  ( -9.474510206698720793, -16.51473224551083518, 59.58442372801900433 ) ) ;
#67153=CARTESIAN_POINT ( 'NONE',  ( 19.02544592524343514, -5.153800228976328945, 43.54057627198103120 ) ) ;
#67155=CARTESIAN_POINT ( 'NONE',  ( -12.06949235617756955, 12.14591786802309770, 60.62390960531437401 ) ) ;
#67156=CARTESIAN_POINT ( 'NONE',  ( 4.379528057220339221, -16.55341960407611168, 57.70724293864770260 ) ) ;
#67157=CARTESIAN_POINT ( 'NONE',  ( -9.564922557960796823, -16.46253265017161027, 77.08224293864769550 ) ) ;
#67158=CARTESIAN_POINT ( 'NONE',  ( -21.53943276465977519, 0.05219959533907696930, 81.24890960531436690 ) ) ;
#67159=CARTESIAN_POINT ( 'NONE',  ( -9.564922557960796823, -16.46253265017161027, 67.08224293864769550 ) ) ;
#67160=CARTESIAN_POINT ( 'NONE',  ( -5.719274019375978568, 21.55341960407610458, 85.20724293864770971 ) ) ;
#67161=CARTESIAN_POINT ( 'NONE',  ( 0.05219959533936267826, -19.03943276465977164, 20.00109039468567218 ) ) ;
#67162=DIRECTION ( 'NONE',  ( 1.000000000000000000, 0.000000000000000000, 0.000000000000000000 ) ) ;
#67163=CARTESIAN_POINT ( 'NONE',  ( 8.314922557961029526, -14.29746914071037800, 110.4177570613523756 ) ) ;
#67164=CARTESIAN_POINT ( 'NONE',  ( -14.29746914071049879, 8.314922557960819915, 90.83224293864769550 ) ) ;
#67165=CARTESIAN_POINT ( 'NONE',  ( -19.05341960407617563, 5.049401038297882671, 88.54275706135230450 ) ) ;
#67167=CARTESIAN_POINT ( 'NONE',  ( -18.62759615963255300, -10.81492255796106328, 24.16775706135235424 ) ) ;
#67168=CARTESIAN_POINT ( 'NONE',  ( -16.46253265017146816, -9.564922557961047289, 59.16775706135233293 ) ) ;
#67169=CARTESIAN_POINT ( 'NONE',  ( -8.224510206698735004, -14.34966873604973081, 99.58442372801900433 ) ) ;
#67170=CARTESIAN_POINT ( 'NONE',  ( 9.564922557961047289, -16.46253265017146816, 45.41775706135232582 ) ) ;
#67171=CARTESIAN_POINT ( 'NONE',  ( -19.02544592524342804, 5.153800228976336051, 101.0405762719810241 ) ) ;
#67172=CARTESIAN_POINT ( 'NONE',  ( 4.483927247898545687, 16.52544592524342804, 59.79057627198103120 ) ) ;
#67173=DIRECTION ( 'NONE',  ( 0.000000000000000000, 0.000000000000000000, -1.000000000000000000 ) ) ;
#67174=CARTESIAN_POINT ( 'NONE',  ( 13.89961937509977652, -13.97604488694527269, 38.12390960531436690 ) ) ;
#67175=CARTESIAN_POINT ( 'NONE',  ( -5.823673210054431948, 21.52544592524334988, 102.7094237280190185 ) ) ;
#67176=CARTESIAN_POINT ( 'NONE',  ( -16.52544592524335698, -4.483927247898792601, 78.95942372801901854 ) ) ;
#67177=CARTESIAN_POINT ( 'NONE',  ( -21.55341960407619339, 5.719274019375674811, 38.54275706135234714 ) ) ;
#67178=CARTESIAN_POINT ( 'NONE',  ( 16.55341960407618274, -4.379528057220086978, 41.04275706135236135 ) ) ;
#67179=CARTESIAN_POINT ( 'NONE',  ( -19.02544592524342804, 5.153800228976336051, 101.0405762719810241 ) ) ;
#67180=CARTESIAN_POINT ( 'NONE',  ( 19.05341960407611168, 5.049401038298154454, 53.95724293864770260 ) ) ;
#67181=CARTESIAN_POINT ( 'NONE',  ( 16.46253265017160672, -9.564922557960803928, 68.33224293864770971 ) ) ;
#67182=CARTESIAN_POINT ( 'NONE',  ( 16.53943276465976808, 0.05219959533934440121, 51.25109039468568994 ) ) ;
#67183=CARTESIAN_POINT ( 'NONE',  ( -8.314922557960811034, -14.29746914071050412, 112.0822429386477097 ) ) ;
#67184=CARTESIAN_POINT ( 'NONE',  ( -0.05219959533910754901, -16.53943276465976808, 22.49890960531436335 ) ) ;
#67186=CARTESIAN_POINT ( 'NONE',  ( -18.62759615963255300, -10.81492255796106328, 54.16775706135235424 ) ) ;
#67187=CARTESIAN_POINT ( 'NONE',  ( 16.46253265017160672, -9.564922557960803928, 93.33224293864769550 ) ) ;
#67188=CARTESIAN_POINT ( 'NONE',  ( 16.46253265017160672, -9.564922557960803928, 58.33224293864769550 ) ) ;
#67189=CARTESIAN_POINT ( 'NONE',  ( 16.51473224551069308, 9.474510206698969483, 94.16557627198103830 ) ) ;
#67190=CARTESIAN_POINT ( 'NONE',  ( 16.53943276465976808, -0.05219959533910856209, 38.74890960531435979 ) ) ;
#67191=CARTESIAN_POINT ( 'NONE',  ( 16.53943276465976808, 0.05219959533934440121, 111.2510903946856899 ) ) ;
#67192=CARTESIAN_POINT ( 'NONE',  ( -12.06949235617756955, 12.14591786802309770, 35.62390960531437401 ) ) ;
#67193=CARTESIAN_POINT ( 'NONE',  ( 18.09867054820433907, 5.499999999999817923, 56.48393025253586330 ) ) ;
#67194=CARTESIAN_POINT ( 'NONE',  ( -9.564922557960796823, -16.46253265017161027, 67.08224293864769550 ) ) ;
#67195=CARTESIAN_POINT ( 'NONE',  ( -0.05219959533936034679, 19.03943276465977164, 42.50109039468566152 ) ) ;
#67197=CARTESIAN_POINT ( 'NONE',  ( 9.474510206698971260, -16.51473224551069308, 67.91557627198102409 ) ) ;
#67198=CARTESIAN_POINT ( 'NONE',  ( -9.564922557961040184, 16.46253265017147172, 82.91775706135233293 ) ) ;
#67199=CARTESIAN_POINT ( 'NONE',  ( -4.483927247898782831, 16.52544592524335698, 62.70942372801902565 ) ) ;
#67201=CARTESIAN_POINT ( 'NONE',  ( 16.51473224551069308, 9.474510206698969483, 94.16557627198103830 ) ) ;
#67202=CARTESIAN_POINT ( 'NONE',  ( -5.719274019375665041, -21.55341960407619695, 24.79275706135235779 ) ) ;
#67203=CARTESIAN_POINT ( 'NONE',  ( 16.51473224551083163, -9.474510206698727899, 85.83442372801900433 ) ) ;
#67204=CARTESIAN_POINT ( 'NONE',  ( 17.26172910966779028, 6.454744622555872446, 86.69353091350778584 ) ) ;
#67205=CARTESIAN_POINT ( 'NONE',  ( 16.46253265017160672, -9.564922557960803928, 53.33224293864768839 ) ) ;
#67206=CARTESIAN_POINT ( 'NONE',  ( -13.89961937509977652, 13.97604488694528158, 85.62390960531433848 ) ) ;
#67207=CARTESIAN_POINT ( 'NONE',  ( -16.55341960407611168, -4.379528057220339221, 51.45724293864770260 ) ) ;
#67208=CARTESIAN_POINT ( 'NONE',  ( -16.46253265017160317, 9.564922557960807481, 45.83224293864769550 ) ) ;
#67209=CARTESIAN_POINT ( 'NONE',  ( -5.049401038297874678, -19.05341960407617918, 64.79275706135233293 ) ) ;
#67210=CARTESIAN_POINT ( 'NONE',  ( -14.29746914071049879, 8.314922557960819915, 90.83224293864769550 ) ) ;
#67211=CARTESIAN_POINT ( 'NONE',  ( 19.05341960407617918, -5.049401038297876454, 31.04275706135232227 ) ) ;
#67212=CARTESIAN_POINT ( 'NONE',  ( 13.89961937509977652, -13.97604488694527269, 68.12390960531436690 ) ) ;
#67213=CARTESIAN_POINT ( 'NONE',  ( 5.823673210054125526, 21.52544592524343514, 64.79057627198103830 ) ) ;
#67214=CARTESIAN_POINT ( 'NONE',  ( -16.53943276465976808, 0.05219959533911058130, 66.24890960531436690 ) ) ;
#67215=CARTESIAN_POINT ( 'NONE',  ( 21.53943276465977519, 0.05219959533937863772, 111.2510903946856899 ) ) ;
#67216=CARTESIAN_POINT ( 'NONE',  ( 9.564922557960805705, 16.46253265017160317, 109.5822429386476955 ) ) ;
#67217=CARTESIAN_POINT ( 'NONE',  ( -21.52544592524343514, 5.823673210054127303, 31.04057627198102409 ) ) ;
#67218=CARTESIAN_POINT ( 'NONE',  ( 9.474510206698971260, -16.51473224551069308, 47.91557627198102409 ) ) ;
#67219=CARTESIAN_POINT ( 'NONE',  ( 13.97604488694527802, 13.89961937509977652, 44.37390960531435269 ) ) ;
#67220=CARTESIAN_POINT ( 'NONE',  ( -8.224510206698948167, 14.34966873604960824, 95.41557627198102409 ) ) ;
#67221=CARTESIAN_POINT ( 'NONE',  ( 0.05219959533907565091, 21.53943276465977519, 114.9989096053143669 ) ) ;
#67222=CARTESIAN_POINT ( 'NONE',  ( 9.474510206698971260, -16.51473224551069308, 97.91557627198102409 ) ) ;
#67223=CARTESIAN_POINT ( 'NONE',  ( -18.62759615963255300, -10.81492255796106328, 34.16775706135234714 ) ) ;
#67224=CARTESIAN_POINT ( 'NONE',  ( -19.02544592524342804, 5.153800228976336051, 101.0405762719810241 ) ) ;
#67225=CARTESIAN_POINT ( 'NONE',  ( 5.049401038298161559, -19.05341960407611168, 22.70724293864769194 ) ) ;
#67226=CARTESIAN_POINT ( 'NONE',  ( -21.52544592524334988, -5.823673210054445271, 83.95942372801900433 ) ) ;
#67227=CARTESIAN_POINT ( 'NONE',  ( -5.823673210054116645, -21.52544592524344225, 97.29057627198105251 ) ) ;
#67229=CARTESIAN_POINT ( 'NONE',  ( -18.22780087662121673, -5.500000000000062172, 51.48459894673893444 ) ) ;
#67231=CARTESIAN_POINT ( 'NONE',  ( -16.52544592524335698, -4.483927247898792601, 48.95942372801902565 ) ) ;
#67232=CARTESIAN_POINT ( 'NONE',  ( -14.34966873604960291, -8.224510206698953496, 101.6655762719810383 ) ) ;
#67234=CARTESIAN_POINT ( 'NONE',  ( 9.564922557960805705, 16.46253265017160317, 54.58224293864769550 ) ) ;
#67235=CARTESIAN_POINT ( 'NONE',  ( -16.52544592524342804, 4.483927247898546575, 91.04057627198103830 ) ) ;
#67236=CARTESIAN_POINT ( 'NONE',  ( 10.72451020669898902, -18.67979575497178502, 42.91557627198103120 ) ) ;
#67237=CARTESIAN_POINT ( 'NONE',  ( -4.483927247898539470, -16.52544592524342804, 62.29057627198102409 ) ) ;
#67238=CARTESIAN_POINT ( 'NONE',  ( 8.224510206698742110, 14.34966873604972548, 27.08442372801901854 ) ) ;
#67239=CARTESIAN_POINT ( 'NONE',  ( 21.55341960407619695, -5.719274019375665929, 86.04275706135236135 ) ) ;
#67240=CARTESIAN_POINT ( 'NONE',  ( 17.44270441346514389, -5.991230190323080684, 76.13664920735770636 ) ) ;
#67241=CARTESIAN_POINT ( 'NONE',  ( -16.55341960407617563, 4.379528057220093196, 93.54275706135234714 ) ) ;
#67242=CARTESIAN_POINT ( 'NONE',  ( 16.55341960407611168, 4.379528057220329451, 38.95724293864768839 ) ) ;
#67243=CARTESIAN_POINT ( 'NONE',  ( 19.02544592524343514, -5.153800228976328945, 38.54057627198103120 ) ) ;
#67244=CARTESIAN_POINT ( 'NONE',  ( -16.46253265017160317, 9.564922557960807481, 85.83224293864769550 ) ) ;
#67245=CARTESIAN_POINT ( 'NONE',  ( 5.823673210054125526, 21.52544592524343514, 99.79057627198103830 ) ) ;
#67246=CARTESIAN_POINT ( 'NONE',  ( -12.06949235617739369, -12.14591786802326823, 44.37609039468567573 ) ) ;
#67247=CARTESIAN_POINT ( 'NONE',  ( -4.483927247898539470, -16.52544592524342804, 62.29057627198102409 ) ) ;
#67248=CARTESIAN_POINT ( 'NONE',  ( 15.72974639402176855, 15.80617190586768217, 86.87609039468568994 ) ) ;
#67250=CARTESIAN_POINT ( 'NONE',  ( 8.314922557961029526, -14.29746914071037800, 100.4177570613523471 ) ) ;
#67251=CARTESIAN_POINT ( 'NONE',  ( 16.21995358207305671, 7.366697692864113911, 27.56448998487843127 ) ) ;
#67253=CARTESIAN_POINT ( 'NONE',  ( 16.55341960407611168, 4.379528057220329451, 23.95724293864769550 ) ) ;
#67254=CARTESIAN_POINT ( 'NONE',  ( 14.34966873604972726, -8.224510206698740333, 75.83442372801900433 ) ) ;
#67255=CARTESIAN_POINT ( 'NONE',  ( -16.46253265017160317, 9.564922557960807481, 80.83224293864769550 ) ) ;
#67256=CARTESIAN_POINT ( 'NONE',  ( 5.153800228976335163, 19.02544592524342804, 94.79057627198103830 ) ) ;
#67257=CARTESIAN_POINT ( 'NONE',  ( -5.719274019375665041, -21.55341960407619695, 89.79275706135236135 ) ) ;
#67258=CARTESIAN_POINT ( 'NONE',  ( 16.52544592524335698, 4.483927247898782831, 86.45942372801901854 ) ) ;
#67259=CARTESIAN_POINT ( 'NONE',  ( -14.34966873604960291, -8.224510206698953496, 66.66557627198102409 ) ) ;
#67260=CARTESIAN_POINT ( 'NONE',  ( 5.049401038298161559, -19.05341960407611168, 72.70724293864768129 ) ) ;
#67262=CARTESIAN_POINT ( 'NONE',  ( -19.03943276465977164, -0.05219959533935918106, 103.7510903946856757 ) ) ;
#67263=CARTESIAN_POINT ( 'NONE',  ( 16.52544592524342804, -4.483927247898539470, 108.5405762719810241 ) ) ;
#67264=CARTESIAN_POINT ( 'NONE',  ( -9.564922557960796823, -16.46253265017161027, 72.08224293864770971 ) ) ;
#67265=CARTESIAN_POINT ( 'NONE',  ( -0.05219959533936034679, 19.03943276465977164, 112.5010903946856757 ) ) ;
#67267=CARTESIAN_POINT ( 'NONE',  ( -19.03943276465977164, -0.05219959533935918106, 18.75109039468567218 ) ) ;
#67268=CARTESIAN_POINT ( 'NONE',  ( 4.379528057220092307, 16.55341960407617563, 87.29275706135236135 ) ) ;
#67269=CARTESIAN_POINT ( 'NONE',  ( 13.89961937509957401, 13.97604488694547697, 106.8760903946856757 ) ) ;
#67270=CARTESIAN_POINT ( 'NONE',  ( -16.52544592524342804, 4.483927247898546575, 116.0405762719810383 ) ) ;
#67271=CARTESIAN_POINT ( 'NONE',  ( 4.379528057220092307, 16.55341960407617563, 72.29275706135236135 ) ) ;
#67272=CARTESIAN_POINT ( 'NONE',  ( -8.314922557961024197, 14.29746914071037800, 47.91775706135234714 ) ) ;
#67274=CARTESIAN_POINT ( 'NONE',  ( -19.02544592524334988, -5.153800228976617603, 73.95942372801900433 ) ) ;
#67275=CARTESIAN_POINT ( 'NONE',  ( 5.719274019375673035, 21.55341960407619339, 112.2927570613523471 ) ) ;
#67276=CARTESIAN_POINT ( 'NONE',  ( -9.564922557960796823, -16.46253265017161027, 32.08224293864769550 ) ) ;
#67277=CARTESIAN_POINT ( 'NONE',  ( 13.89961937509977652, -13.97604488694527269, 73.12390960531436690 ) ) ;
#67278=CARTESIAN_POINT ( 'NONE',  ( 12.06949235617757843, -12.14591786802309237, 68.12390960531436690 ) ) ;
#67279=CARTESIAN_POINT ( 'NONE',  ( 9.474510206698729675, 16.51473224551082808, 47.08442372801900433 ) ) ;
#67280=CARTESIAN_POINT ( 'NONE',  ( 21.53943276465977519, -0.05219959533907433946, 43.74890960531435979 ) ) ;
#67281=CARTESIAN_POINT ( 'NONE',  ( -0.05219959533937732626, 21.53943276465977519, 112.5010903946857042 ) ) ;
#67282=CARTESIAN_POINT ( 'NONE',  ( -19.02544592524342804, 5.153800228976336051, 86.04057627198103830 ) ) ;
#67284=CARTESIAN_POINT ( 'NONE',  ( -21.53943276465977519, -0.05219959533937600094, 103.7510903946857042 ) ) ;
#67285=CARTESIAN_POINT ( 'NONE',  ( -21.52544592524343514, 5.823673210054127303, 61.04057627198103120 ) ) ;
#67286=CARTESIAN_POINT ( 'NONE',  ( -13.89961937509977652, 13.97604488694528158, 90.62390960531432427 ) ) ;
#67287=CARTESIAN_POINT ( 'NONE',  ( -9.564922557961040184, 16.46253265017147172, 72.91775706135233293 ) ) ;
#67288=CARTESIAN_POINT ( 'NONE',  ( -5.153800228976328057, -19.02544592524343514, 97.29057627198099567 ) ) ;
#67289=CARTESIAN_POINT ( 'NONE',  ( -0.05219959533936034679, 19.03943276465977164, 102.5010903946856757 ) ) ;
#67290=CARTESIAN_POINT ( 'NONE',  ( 8.314922557961029526, -14.29746914071037800, 60.41775706135235424 ) ) ;
#67291=CARTESIAN_POINT ( 'NONE',  ( -16.51473224551069308, -9.474510206698971260, 21.66557627198102765 ) ) ;
#67292=CARTESIAN_POINT ( 'NONE',  ( 16.51473224551069308, 9.474510206698969483, 79.16557627198103830 ) ) ;
#67293=CARTESIAN_POINT ( 'NONE',  ( -10.81492255796078084, -18.62759615963271287, 62.08224293864769550 ) ) ;
#67294=CARTESIAN_POINT ( 'NONE',  ( -16.52544592524335698, -4.483927247898792601, 38.95942372801901854 ) ) ;
#67295=CARTESIAN_POINT ( 'NONE',  ( -21.53943276465977519, -0.05219959533937600094, 28.75109039468567929 ) ) ;
#67296=CARTESIAN_POINT ( 'NONE',  ( -21.52544592524334988, -5.823673210054445271, 83.95942372801900433 ) ) ;
#67297=CARTESIAN_POINT ( 'NONE',  ( 14.34966873604972726, -8.224510206698740333, 100.8344237280190185 ) ) ;
#67298=CARTESIAN_POINT ( 'NONE',  ( 16.46253265017160672, -9.564922557960803928, 83.33224293864768129 ) ) ;
#67299=CARTESIAN_POINT ( 'NONE',  ( -14.29746914071049879, 8.314922557960819915, 75.83224293864769550 ) ) ;
#67300=CARTESIAN_POINT ( 'NONE',  ( 8.314922557960818139, 14.29746914071049879, 24.58224293864768839 ) ) ;
#67301=CARTESIAN_POINT ( 'NONE',  ( -13.89961937509957401, -13.97604488694547875, 74.37609039468566152 ) ) ;
#67302=CARTESIAN_POINT ( 'NONE',  ( 5.823673210054444382, -21.52544592524334988, 50.20942372801901854 ) ) ;
#67303=CARTESIAN_POINT ( 'NONE',  ( -0.05219959533910754901, -16.53943276465976808, 97.49890960531436690 ) ) ;
#67304=CARTESIAN_POINT ( 'NONE',  ( -19.03943276465977164, 0.05219959533909376836, 116.2489096053143669 ) ) ;
#67305=CARTESIAN_POINT ( 'NONE',  ( -8.224510206698735004, -14.34966873604973081, 99.58442372801900433 ) ) ;
#67306=CARTESIAN_POINT ( 'NONE',  ( 10.72451020669871369, 18.67979575497193778, 92.08442372801901854 ) ) ;
#67307=CARTESIAN_POINT ( 'NONE',  ( 0.05219959533934541429, -16.53943276465976808, 40.00109039468567573 ) ) ;
#67308=CARTESIAN_POINT ( 'NONE',  ( 21.52544592524334988, 5.823673210054432836, 36.45942372801901143 ) ) ;
#67310=CARTESIAN_POINT ( 'NONE',  ( -21.52544592524343514, 5.823673210054127303, 116.0405762719810383 ) ) ;
#67311=CARTESIAN_POINT ( 'NONE',  ( 4.379528057220339221, -16.55341960407611168, 87.70724293864769550 ) ) ;
#67313=CARTESIAN_POINT ( 'NONE',  ( -4.483927247898539470, -16.52544592524342804, 62.29057627198102409 ) ) ;
#67314=CARTESIAN_POINT ( 'NONE',  ( -12.06949235617739369, -12.14591786802326823, 104.3760903946856899 ) ) ;
#67315=CARTESIAN_POINT ( 'NONE',  ( -16.51473224551069308, -9.474510206698971260, 36.66557627198102409 ) ) ;
#67316=CARTESIAN_POINT ( 'NONE',  ( 5.823673210054125526, 21.52544592524343514, 39.79057627198103830 ) ) ;
#67317=CARTESIAN_POINT ( 'NONE',  ( -4.483927247898539470, -16.52544592524342804, 72.29057627198102409 ) ) ;
#67318=CARTESIAN_POINT ( 'NONE',  ( -21.52544592524343514, 5.823673210054127303, 81.04057627198102409 ) ) ;
#67319=CARTESIAN_POINT ( 'NONE',  ( 13.89961937509977652, -13.97604488694527269, 83.12390960531436690 ) ) ;
#67320=CARTESIAN_POINT ( 'NONE',  ( -16.46253265017160317, 9.564922557960807481, 35.83224293864768839 ) ) ;
#67321=CARTESIAN_POINT ( 'NONE',  ( 5.153800228976615827, -19.02544592524334988, 95.20942372801897591 ) ) ;
#67322=CARTESIAN_POINT ( 'NONE',  ( -21.53943276465977519, 0.05219959533907696930, 36.24890960531435979 ) ) ;
#67323=CARTESIAN_POINT ( 'NONE',  ( 0.05219959533937995610, -21.53943276465977519, 70.00109039468568994 ) ) ;
#67324=CARTESIAN_POINT ( 'NONE',  ( 5.049401038298161559, -19.05341960407611168, 47.70724293864770260 ) ) ;
#67325=CARTESIAN_POINT ( 'NONE',  ( 5.153800228976335163, 19.02544592524342804, 89.79057627198102409 ) ) ;
#67326=VERTEX_POINT ( 'NONE', #124300 ) ;
#67327=CARTESIAN_POINT ( 'NONE',  ( 4.483927247898790824, -16.52544592524335698, 65.20942372801901854 ) ) ;
#67328=CARTESIAN_POINT ( 'NONE',  ( -5.823673210054431948, 21.52544592524334988, 42.70942372801901854 ) ) ;
#67329=CARTESIAN_POINT ( 'NONE',  ( -21.53943276465977519, -0.05219959533937600094, 78.75109039468568994 ) ) ;
#67330=CARTESIAN_POINT ( 'NONE',  ( -15.72974639402197994, 15.80617190586746368, 25.62390960531435624 ) ) ;
#67331=CARTESIAN_POINT ( 'NONE',  ( -18.67979575497178146, -10.72451020669898902, 91.66557627198103830 ) ) ;
#67332=CARTESIAN_POINT ( 'NONE',  ( -15.72974639402176322, -15.80617190586768395, 19.37609039468568639 ) ) ;
#67333=CARTESIAN_POINT ( 'NONE',  ( 16.52544592524335698, 4.483927247898782831, 66.45942372801903275 ) ) ;
#67334=CARTESIAN_POINT ( 'NONE',  ( 5.719274019375991003, -21.55341960407610458, 57.70724293864770260 ) ) ;
#67335=CARTESIAN_POINT ( 'NONE',  ( -19.05341960407617563, 5.049401038297882671, 23.54275706135233648 ) ) ;
#67336=CARTESIAN_POINT ( 'NONE',  ( 19.03943276465977164, -0.05219959533909143690, 63.74890960531435979 ) ) ;
#67337=CARTESIAN_POINT ( 'NONE',  ( 8.224510206698742110, 14.34966873604972548, 107.0844237280190043 ) ) ;
#67340=CARTESIAN_POINT ( 'NONE',  ( 5.049401038298161559, -19.05341960407611168, 92.70724293864769550 ) ) ;
#67342=CARTESIAN_POINT ( 'NONE',  ( 19.02544592524334988, 5.153800228976608722, 76.45942372801897591 ) ) ;
#67343=CARTESIAN_POINT ( 'NONE',  ( 21.53943276465977519, -0.05219959533907433946, 58.74890960531436690 ) ) ;
#67344=CARTESIAN_POINT ( 'NONE',  ( 0.05219959533910956823, 16.53943276465976808, 24.99890960531435624 ) ) ;
#67345=CARTESIAN_POINT ( 'NONE',  ( -13.97604488694547697, 13.89961937509957934, 93.12609039468566152 ) ) ;
#67346=CARTESIAN_POINT ( 'NONE',  ( -16.46253265017160317, 9.564922557960807481, 40.83224293864769550 ) ) ;
#67347=CARTESIAN_POINT ( 'NONE',  ( 19.03943276465977164, 0.05219959533936151252, 91.25109039468566152 ) ) ;
#67348=CARTESIAN_POINT ( 'NONE',  ( 21.52544592524344225, -5.823673210054117533, 93.54057627198103830 ) ) ;
#67349=CARTESIAN_POINT ( 'NONE',  ( -16.46253265017146816, -9.564922557961047289, 64.16775706135233293 ) ) ;
#67350=CARTESIAN_POINT ( 'NONE',  ( 17.31728774477274513, 6.344390552232368918, 106.6809334831068128 ) ) ;
#67351=CARTESIAN_POINT ( 'NONE',  ( -19.03943276465977164, 0.05219959533909376836, 51.24890960531436690 ) ) ;
#67352=CARTESIAN_POINT ( 'NONE',  ( -0.05219959533910754901, -16.53943276465976808, 62.49890960531436690 ) ) ;
#67353=CARTESIAN_POINT ( 'NONE',  ( 19.05341960407611168, 5.049401038298154454, 48.95724293864768129 ) ) ;
#67354=CARTESIAN_POINT ( 'NONE',  ( 14.34966873604960469, 8.224510206698951720, 49.16557627198102409 ) ) ;
#67357=CARTESIAN_POINT ( 'NONE',  ( 12.06949235617757843, -12.14591786802309237, 33.12390960531435979 ) ) ;
#67358=CARTESIAN_POINT ( 'NONE',  ( 19.02544592524343514, -5.153800228976328945, 58.54057627198102409 ) ) ;
#67359=CARTESIAN_POINT ( 'NONE',  ( -9.564922557961040184, 16.46253265017147172, 72.91775706135233293 ) ) ;
#67360=CARTESIAN_POINT ( 'NONE',  ( -19.05341960407617563, 5.049401038297882671, 43.54275706135232582 ) ) ;
#67361=CARTESIAN_POINT ( 'NONE',  ( 8.224510206698742110, 14.34966873604972548, 47.08442372801901854 ) ) ;
#67362=CARTESIAN_POINT ( 'NONE',  ( -5.823673210054116645, -21.52544592524344225, 47.29057627198103120 ) ) ;
#67363=CARTESIAN_POINT ( 'NONE',  ( -10.72451020669870658, -18.67979575497194134, 109.5844237280190328 ) ) ;
#67364=CARTESIAN_POINT ( 'NONE',  ( -5.049401038298153566, 19.05341960407611168, 70.20724293864769550 ) ) ;
#67366=CARTESIAN_POINT ( 'NONE',  ( 19.03943276465977164, -0.05219959533909143690, 113.7489096053143669 ) ) ;
#67368=CARTESIAN_POINT ( 'NONE',  ( 0.05219959533937995610, -21.53943276465977519, 45.00109039468568284 ) ) ;
#67369=CARTESIAN_POINT ( 'NONE',  ( -4.483927247898539470, -16.52544592524342804, 87.29057627198103830 ) ) ;
#67370=CARTESIAN_POINT ( 'NONE',  ( -15.72974639402197994, 15.80617190586746368, 90.62390960531436690 ) ) ;
#67371=CARTESIAN_POINT ( 'NONE',  ( -0.05219959533909027116, -19.03943276465977164, 87.49890960531436690 ) ) ;
#67372=CARTESIAN_POINT ( 'NONE',  ( 13.89961937509977652, -13.97604488694527269, 83.12390960531436690 ) ) ;
#67373=CARTESIAN_POINT ( 'NONE',  ( -21.55341960407619339, 5.719274019375674811, 23.54275706135235424 ) ) ;
#67376=CARTESIAN_POINT ( 'NONE',  ( -5.153800228976328057, -19.02544592524343514, 77.29057627198099567 ) ) ;
#67378=CARTESIAN_POINT ( 'NONE',  ( -9.564922557960796823, -16.46253265017161027, 22.08224293864768839 ) ) ;
#67379=CARTESIAN_POINT ( 'NONE',  ( -16.51473224551069308, -9.474510206698971260, 36.66557627198102409 ) ) ;
#67380=CARTESIAN_POINT ( 'NONE',  ( 19.03943276465977164, 0.05219959533936151252, 106.2510903946856615 ) ) ;
#67382=CARTESIAN_POINT ( 'NONE',  ( -14.34966873604960291, -8.224510206698953496, 111.6655762719810525 ) ) ;
#67383=CARTESIAN_POINT ( 'NONE',  ( 21.52544592524334988, 5.823673210054432836, 76.45942372801901854 ) ) ;
#67384=CARTESIAN_POINT ( 'NONE',  ( 16.46253265017160672, -9.564922557960803928, 68.33224293864770971 ) ) ;
#67385=CARTESIAN_POINT ( 'NONE',  ( -5.719274019375665041, -21.55341960407619695, 29.79275706135234358 ) ) ;
#67386=CARTESIAN_POINT ( 'NONE',  ( 18.67979575497178502, 10.72451020669898547, 114.1655762719810383 ) ) ;
#67388=CARTESIAN_POINT ( 'NONE',  ( 0.05219959533909260263, 19.03943276465977164, 79.99890960531436690 ) ) ;
#67390=CARTESIAN_POINT ( 'NONE',  ( -14.34966873604972548, 8.224510206698743886, 28.33442372801902209 ) ) ;
#67391=CARTESIAN_POINT ( 'NONE',  ( 10.81492255796078972, 18.62759615963270932, 39.58224293864769550 ) ) ;
#67392=CARTESIAN_POINT ( 'NONE',  ( -0.05219959533937732626, 21.53943276465977519, 62.50109039468568284 ) ) ;
#67393=CARTESIAN_POINT ( 'NONE',  ( 19.02544592524343514, -5.153800228976328945, 108.5405762719810383 ) ) ;
#67394=( BOUNDED_CURVE ( )  B_SPLINE_CURVE ( 2, ( #132814, #194500, #27662, #197489, #135819, #102480, #40810, #116646, #58956, #117650, #178336, #100471, #179347 ),
 .UNSPECIFIED., .F., .T. ) 
 B_SPLINE_CURVE_WITH_KNOTS ( ( 3, 2, 2, 2, 2, 2, 3 ),
 ( 0.1603251732691504117, 0.1622807017543859698, 0.1666666666666666574, 0.1710526315789473728, 0.1754385964912280604, 0.1798245614035087758, 0.1817344100666542506 ),
 .UNSPECIFIED. ) 
 CURVE ( )  GEOMETRIC_REPRESENTATION_ITEM ( )  RATIONAL_B_SPLINE_CURVE ( ( 0.9831626618144004848, 0.9848076720550091867, 1.000000000000000000, 0.9659258262890683122, 1.000000000000000000, 0.9659258262890683122, 1.000000000000000000, 0.9659258262890683122, 1.000000000000000000, 0.9659258262890683122, 1.000000000000000000, 0.9851625545550090068, 0.9832469066685280978 ) ) 
 REPRESENTATION_ITEM ( '' )  );
#67395=CARTESIAN_POINT ( 'NONE',  ( -9.564922557961040184, 16.46253265017147172, 97.91775706135233293 ) ) ;
#67396=CARTESIAN_POINT ( 'NONE',  ( 19.05341960407611168, 5.049401038298154454, 43.95724293864769550 ) ) ;
#67397=CARTESIAN_POINT ( 'NONE',  ( 5.049401038298161559, -19.05341960407611168, 87.70724293864769550 ) ) ;
#67398=CARTESIAN_POINT ( 'NONE',  ( -12.14591786802309592, -12.06949235617757132, 91.87390960531436690 ) ) ;
#67399=CARTESIAN_POINT ( 'NONE',  ( 0.05219959533910956823, 16.53943276465976808, 94.99890960531436690 ) ) ;
#67400=CARTESIAN_POINT ( 'NONE',  ( 13.89961937509977652, -13.97604488694527269, 108.1239096053143669 ) ) ;
#67402=CARTESIAN_POINT ( 'NONE',  ( -16.52544592524342804, 4.483927247898546575, 51.04057627198103120 ) ) ;
#67403=CARTESIAN_POINT ( 'NONE',  ( 19.02544592524343514, -5.153800228976328945, 38.54057627198103120 ) ) ;
#67404=CARTESIAN_POINT ( 'NONE',  ( 0.05219959533937995610, -21.53943276465977519, 60.00109039468568284 ) ) ;
#67405=CARTESIAN_POINT ( 'NONE',  ( 19.05341960407617918, -5.049401038297876454, 96.04275706135231871 ) ) ;
#67406=CARTESIAN_POINT ( 'NONE',  ( -4.483927247898539470, -16.52544592524342804, 57.29057627198103120 ) ) ;
#67407=CARTESIAN_POINT ( 'NONE',  ( -10.72451020669898014, 18.67979575497178502, 115.4155762719810241 ) ) ;
#67408=CARTESIAN_POINT ( 'NONE',  ( 21.55341960407610458, 5.719274019375980345, 48.95724293864770971 ) ) ;
#67409=CARTESIAN_POINT ( 'NONE',  ( -19.05341960407611168, -5.049401038298163336, 106.4572429386476955 ) ) ;
#67411=CARTESIAN_POINT ( 'NONE',  ( -13.97604488694527625, -13.89961937509977652, 61.87390960531435979 ) ) ;
#67412=CARTESIAN_POINT ( 'NONE',  ( 16.53943276465976808, -0.05219959533910856209, 38.74890960531435979 ) ) ;
#67413=CARTESIAN_POINT ( 'NONE',  ( 4.379528057220092307, 16.55341960407617563, 97.29275706135234714 ) ) ;
#67414=CARTESIAN_POINT ( 'NONE',  ( -12.06949235617739369, -12.14591786802326823, 79.37609039468567573 ) ) ;
#67415=CARTESIAN_POINT ( 'NONE',  ( -16.51473224551082808, 9.474510206698731452, 33.33442372801899722 ) ) ;
#67417=CARTESIAN_POINT ( 'NONE',  ( -13.89961937509977652, 13.97604488694528158, 95.62390960531436690 ) ) ;
#67418=CARTESIAN_POINT ( 'NONE',  ( 16.46253265017160672, -9.564922557960803928, 48.33224293864769550 ) ) ;
#67419=CARTESIAN_POINT ( 'NONE',  ( -16.53943276465976808, 0.05219959533911058130, 56.24890960531436690 ) ) ;
#67420=CARTESIAN_POINT ( 'NONE',  ( -13.97604488694527625, -13.89961937509977652, 21.87390960531435979 ) ) ;
#67421=CARTESIAN_POINT ( 'NONE',  ( 21.55341960407610458, 5.719274019375980345, 23.95724293864769550 ) ) ;
#67422=CARTESIAN_POINT ( 'NONE',  ( -18.62759615963270932, 10.81492255796079327, 40.83224293864769550 ) ) ;
#67423=CARTESIAN_POINT ( 'NONE',  ( 16.55341960407611168, 4.379528057220329451, 83.95724293864770971 ) ) ;
#67424=CARTESIAN_POINT ( 'NONE',  ( 4.379528057220092307, 16.55341960407617563, 32.29275706135235424 ) ) ;
#67425=CARTESIAN_POINT ( 'NONE',  ( 8.224510206698953496, -14.34966873604960469, 72.91557627198103830 ) ) ;
#67427=CARTESIAN_POINT ( 'NONE',  ( -16.51473224551082808, 9.474510206698731452, 73.33442372801900433 ) ) ;
#67428=CARTESIAN_POINT ( 'NONE',  ( 13.97604488694527802, 13.89961937509977652, 104.3739096053143385 ) ) ;
#67430=CARTESIAN_POINT ( 'NONE',  ( 18.82182630884605601, 5.499999999999964473, 101.5751632728302383 ) ) ;
#67431=CARTESIAN_POINT ( 'NONE',  ( -14.34966873604972548, 8.224510206698743886, 33.33442372801900433 ) ) ;
#67432=CARTESIAN_POINT ( 'NONE',  ( -16.53943276465976808, 0.05219959533911058130, 21.24890960531436690 ) ) ;
#67433=CARTESIAN_POINT ( 'NONE',  ( 9.474510206698729675, 16.51473224551082808, 77.08442372801900433 ) ) ;
#67434=CARTESIAN_POINT ( 'NONE',  ( -10.72451020669898014, 18.67979575497178502, 55.41557627198102409 ) ) ;
#67435=CARTESIAN_POINT ( 'NONE',  ( -21.55341960407619339, 5.719274019375674811, 68.54275706135234714 ) ) ;
#67437=CARTESIAN_POINT ( 'NONE',  ( 12.14591786802327356, -12.06949235617739191, 40.62609039468567573 ) ) ;
#67438=CARTESIAN_POINT ( 'NONE',  ( 19.03943276465977164, -0.05219959533909143690, 28.74890960531435624 ) ) ;
#67439=CARTESIAN_POINT ( 'NONE',  ( -19.05341960407611168, -5.049401038298163336, 81.45724293864769550 ) ) ;
#67440=CARTESIAN_POINT ( 'NONE',  ( 19.03943276465977164, -0.05219959533909143690, 23.74890960531435269 ) ) ;
#67441=CARTESIAN_POINT ( 'NONE',  ( 8.314922557960818139, 14.29746914071049879, 84.58224293864769550 ) ) ;
#67443=CARTESIAN_POINT ( 'NONE',  ( 16.51473224551069308, 9.474510206698969483, 89.16557627198103830 ) ) ;
#67445=CARTESIAN_POINT ( 'NONE',  ( 5.153800228976615827, -19.02544592524334988, 100.2094237280190043 ) ) ;
#67446=CARTESIAN_POINT ( 'NONE',  ( -21.55341960407610458, -5.719274019375992779, 76.45724293864769550 ) ) ;
#67447=CARTESIAN_POINT ( 'NONE',  ( -5.153800228976328057, -19.02544592524343514, 47.29057627198102409 ) ) ;
#67448=CARTESIAN_POINT ( 'NONE',  ( -13.97604488694547697, 13.89961937509957934, 68.12609039468563310 ) ) ;
#67449=CARTESIAN_POINT ( 'NONE',  ( 10.81492255796106328, -18.62759615963255655, 20.41775706135234714 ) ) ;
#67450=CARTESIAN_POINT ( 'NONE',  ( 19.03943276465977164, -0.05219959533909143690, 63.74890960531435979 ) ) ;
#67451=CARTESIAN_POINT ( 'NONE',  ( 13.97604488694527802, 13.89961937509977652, 109.3739096053143669 ) ) ;
#67452=ORIENTED_EDGE ( 'NONE', *, *, #128971, .T. ) ;
#67453=CARTESIAN_POINT ( 'NONE',  ( 16.52544592524335698, 4.483927247898782831, 31.45942372801901854 ) ) ;
#67454=CARTESIAN_POINT ( 'NONE',  ( 15.72974639402199770, -15.80617190586745480, 103.1239096053143811 ) ) ;
#67455=CARTESIAN_POINT ( 'NONE',  ( 16.52544592524342804, -4.483927247898539470, 103.5405762719810383 ) ) ;
#67456=CARTESIAN_POINT ( 'NONE',  ( -16.51473224551069308, -9.474510206698971260, 91.66557627198103830 ) ) ;
#67457=CARTESIAN_POINT ( 'NONE',  ( 19.03943276465977164, 0.05219959533936151252, 66.25109039468567573 ) ) ;
#67458=CARTESIAN_POINT ( 'NONE',  ( -21.55341960407610458, -5.719274019375992779, 86.45724293864770971 ) ) ;
#67459=CARTESIAN_POINT ( 'NONE',  ( -0.05219959533910754901, -16.53943276465976808, 52.49890960531435979 ) ) ;
#67460=CARTESIAN_POINT ( 'NONE',  ( 9.474510206698729675, 16.51473224551082808, 22.08442372801899722 ) ) ;
#67461=CARTESIAN_POINT ( 'NONE',  ( -16.53943276465976808, -0.05219959533934237506, 58.75109039468568994 ) ) ;
#67462=CARTESIAN_POINT ( 'NONE',  ( 9.564922557960805705, 16.46253265017160317, 94.58224293864769550 ) ) ;
#67463=CARTESIAN_POINT ( 'NONE',  ( -19.03943276465977164, 0.05219959533909376836, 41.24890960531435269 ) ) ;
#67464=CARTESIAN_POINT ( 'NONE',  ( -0.05219959533937732626, 21.53943276465977519, 52.50109039468567573 ) ) ;
#67465=CARTESIAN_POINT ( 'NONE',  ( 5.719274019375673035, 21.55341960407619339, 67.29275706135234714 ) ) ;
#67466=CARTESIAN_POINT ( 'NONE',  ( 5.153800228976335163, 19.02544592524342804, 54.79057627198103120 ) ) ;
#67467=CARTESIAN_POINT ( 'NONE',  ( -15.80617190586768217, 15.72974639402176855, 33.12609039468569705 ) ) ;
#67468=CARTESIAN_POINT ( 'NONE',  ( -13.89961937509957401, -13.97604488694547875, 69.37609039468564731 ) ) ;
#67469=CARTESIAN_POINT ( 'NONE',  ( -5.153800228976607833, 19.02544592524334988, 72.70942372801900433 ) ) ;
#67470=CARTESIAN_POINT ( 'NONE',  ( 19.03943276465977164, -0.05219959533909143690, 33.74890960531435979 ) ) ;
#67471=CARTESIAN_POINT ( 'NONE',  ( 12.14591786802327356, -12.06949235617739191, 85.62609039468568994 ) ) ;
#67472=CARTESIAN_POINT ( 'NONE',  ( -5.049401038298153566, 19.05341960407611168, 50.20724293864770260 ) ) ;
#67473=CARTESIAN_POINT ( 'NONE',  ( 19.05341960407611168, 5.049401038298154454, 23.95724293864769194 ) ) ;
#67474=CARTESIAN_POINT ( 'NONE',  ( 19.02544592524343514, -5.153800228976328945, 98.54057627198100988 ) ) ;
#67475=CARTESIAN_POINT ( 'NONE',  ( 19.03943276465977164, -0.05219959533909143690, 38.74890960531436690 ) ) ;
#67476=CARTESIAN_POINT ( 'NONE',  ( -0.05219959533907301413, -21.53943276465977519, 87.49890960531436690 ) ) ;
#67477=CARTESIAN_POINT ( 'NONE',  ( -0.05219959533934338120, 16.53943276465976808, 57.50109039468568994 ) ) ;
#67478=CARTESIAN_POINT ( 'NONE',  ( -0.05219959533936034679, 19.03943276465977164, 32.50109039468566863 ) ) ;
#67480=CARTESIAN_POINT ( 'NONE',  ( 19.05341960407611168, 5.049401038298154454, 53.95724293864770260 ) ) ;
#67481=CARTESIAN_POINT ( 'NONE',  ( -8.224510206698948167, 14.34966873604960824, 50.41557627198103120 ) ) ;
#67482=CARTESIAN_POINT ( 'NONE',  ( -0.05219959533910754901, -16.53943276465976808, 82.49890960531436690 ) ) ;
#67484=CARTESIAN_POINT ( 'NONE',  ( -19.02544592524342804, 5.153800228976336051, 91.04057627198100988 ) ) ;
#67485=CARTESIAN_POINT ( 'NONE',  ( -19.02544592524342804, 5.153800228976336051, 76.04057627198102409 ) ) ;
#67486=CARTESIAN_POINT ( 'NONE',  ( 18.62759615963255655, 10.81492255796105972, 31.66775706135234358 ) ) ;
#67487=CARTESIAN_POINT ( 'NONE',  ( -13.97604488694527625, -13.89961937509977652, 96.87390960531433848 ) ) ;
#67488=CARTESIAN_POINT ( 'NONE',  ( -15.72974639402176322, -15.80617190586768395, 94.37609039468568994 ) ) ;
#67489=CARTESIAN_POINT ( 'NONE',  ( -16.53943276465976808, -0.05219959533934237506, 73.75109039468567573 ) ) ;
#67490=CARTESIAN_POINT ( 'NONE',  ( -15.72974639402176322, -15.80617190586768395, 29.37609039468568284 ) ) ;
#67492=CARTESIAN_POINT ( 'NONE',  ( -21.53943276465977519, 0.05219959533907696930, 96.24890960531435269 ) ) ;
#67493=CARTESIAN_POINT ( 'NONE',  ( -4.379528057220328563, 16.55341960407611168, 45.20724293864769550 ) ) ;
#67494=CARTESIAN_POINT ( 'NONE',  ( -19.05341960407611168, -5.049401038298163336, 36.45724293864766707 ) ) ;
#67495=CARTESIAN_POINT ( 'NONE',  ( -4.483927247898539470, -16.52544592524342804, 72.29057627198102409 ) ) ;
#67496=CARTESIAN_POINT ( 'NONE',  ( -0.05219959533907301413, -21.53943276465977519, 32.49890960531435979 ) ) ;
#67497=CARTESIAN_POINT ( 'NONE',  ( -19.05341960407617563, 5.049401038297882671, 28.54275706135232937 ) ) ;
#67498=CARTESIAN_POINT ( 'NONE',  ( -14.34966873604960291, -8.224510206698953496, 101.6655762719810383 ) ) ;
#67499=CARTESIAN_POINT ( 'NONE',  ( 0.05219959533909260263, 19.03943276465977164, 104.9989096053143669 ) ) ;
#67500=ORIENTED_EDGE ( 'NONE', *, *, #198323, .F. ) ;
#67501=CARTESIAN_POINT ( 'NONE',  ( 12.14591786802327356, -12.06949235617739191, 55.62609039468568284 ) ) ;
#67502=CARTESIAN_POINT ( 'NONE',  ( 13.97604488694527802, 13.89961937509977652, 69.37390960531436690 ) ) ;
#67504=CARTESIAN_POINT ( 'NONE',  ( 5.823673210054125526, 21.52544592524343514, 29.79057627198102409 ) ) ;
#67505=CARTESIAN_POINT ( 'NONE',  ( 14.29746914071037800, 8.314922557961029526, 91.66775706135234714 ) ) ;
#67506=CARTESIAN_POINT ( 'NONE',  ( -0.05219959533936034679, 19.03943276465977164, 112.5010903946856757 ) ) ;
#67507=CARTESIAN_POINT ( 'NONE',  ( -10.72451020669870658, -18.67979575497194134, 79.58442372801903275 ) ) ;
#67508=CARTESIAN_POINT ( 'NONE',  ( 0.05219959533909260263, 19.03943276465977164, 69.99890960531435269 ) ) ;
#67509=CARTESIAN_POINT ( 'NONE',  ( -5.719274019375978568, 21.55341960407610458, 110.2072429386477239 ) ) ;
#67510=CARTESIAN_POINT ( 'NONE',  ( 14.29746914071037800, 8.314922557961029526, 56.66775706135235424 ) ) ;
#67511=CARTESIAN_POINT ( 'NONE',  ( 16.55341960407611168, 4.379528057220329451, 113.9572429386477239 ) ) ;
#67512=CARTESIAN_POINT ( 'NONE',  ( -12.06949235617739369, -12.14591786802326823, 24.37609039468567573 ) ) ;
#67513=CARTESIAN_POINT ( 'NONE',  ( -13.97604488694547697, 13.89961937509957934, 88.12609039468563310 ) ) ;
#67514=CARTESIAN_POINT ( 'NONE',  ( 18.67979575497178502, 10.72451020669898547, 74.16557627198102409 ) ) ;
#67515=CARTESIAN_POINT ( 'NONE',  ( 5.049401038297881783, 19.05341960407617563, 57.29275706135231871 ) ) ;
#67517=CARTESIAN_POINT ( 'NONE',  ( -5.823673210054116645, -21.52544592524344225, 97.29057627198105251 ) ) ;
#67519=CARTESIAN_POINT ( 'NONE',  ( -9.564922557960796823, -16.46253265017161027, 72.08224293864770971 ) ) ;
#67521=CARTESIAN_POINT ( 'NONE',  ( 16.53943276465976808, 0.05219959533934440121, 26.25109039468567573 ) ) ;
#67523=CARTESIAN_POINT ( 'NONE',  ( -15.80617190586745835, -15.72974639402198527, 96.87390960531436690 ) ) ;
#67524=CARTESIAN_POINT ( 'NONE',  ( -8.314922557960811034, -14.29746914071050412, 62.08224293864769550 ) ) ;
#67525=CARTESIAN_POINT ( 'NONE',  ( 19.03943276465977164, -0.05219959533909143690, 73.74890960531435269 ) ) ;
#67526=CARTESIAN_POINT ( 'NONE',  ( -15.72974639402176322, -15.80617190586768395, 74.37609039468568994 ) ) ;
#67527=CARTESIAN_POINT ( 'NONE',  ( 12.14591786802327356, -12.06949235617739191, 35.62609039468568994 ) ) ;
#67528=CARTESIAN_POINT ( 'NONE',  ( -13.89961937509957401, -13.97604488694547875, 44.37609039468566863 ) ) ;
#67529=CARTESIAN_POINT ( 'NONE',  ( 21.55341960407619695, -5.719274019375665929, 46.04275706135234714 ) ) ;
#67530=CARTESIAN_POINT ( 'NONE',  ( 0.05219959533907565091, 21.53943276465977519, 64.99890960531435269 ) ) ;
#67531=CARTESIAN_POINT ( 'NONE',  ( -16.53943276465976808, -0.05219959533934237506, 18.75109039468568639 ) ) ;
#67532=CARTESIAN_POINT ( 'NONE',  ( 16.51473224551069308, 9.474510206698969483, 54.16557627198103120 ) ) ;
#67533=CARTESIAN_POINT ( 'NONE',  ( -9.564922557961040184, 16.46253265017147172, 72.91775706135233293 ) ) ;
#67534=CARTESIAN_POINT ( 'NONE',  ( 18.62759615963255655, 10.81492255796105972, 86.66775706135234714 ) ) ;
#67535=CARTESIAN_POINT ( 'NONE',  ( -9.474510206698720793, -16.51473224551083518, 54.58442372801899722 ) ) ;
#67536=CARTESIAN_POINT ( 'NONE',  ( -13.89961937509977652, 13.97604488694528158, 35.62390960531435269 ) ) ;
#67537=CARTESIAN_POINT ( 'NONE',  ( -5.823673210054116645, -21.52544592524344225, 62.29057627198102409 ) ) ;
#67538=CARTESIAN_POINT ( 'NONE',  ( -8.314922557960811034, -14.29746914071050412, 47.08224293864770260 ) ) ;
#67540=CARTESIAN_POINT ( 'NONE',  ( -19.02544592524334988, -5.153800228976617603, 33.95942372801897591 ) ) ;
#67541=CARTESIAN_POINT ( 'NONE',  ( -14.34966873604972548, 8.224510206698743886, 83.33442372801903275 ) ) ;
#67542=CARTESIAN_POINT ( 'NONE',  ( 16.52544592524342804, -4.483927247898539470, 58.54057627198103120 ) ) ;
#67543=CARTESIAN_POINT ( 'NONE',  ( -21.53943276465977519, -0.05219959533937600094, 93.75109039468567573 ) ) ;
#67544=CARTESIAN_POINT ( 'NONE',  ( 15.80617190586769283, -15.72974639402175789, 85.62609039468568994 ) ) ;
#67545=CARTESIAN_POINT ( 'NONE',  ( -0.05219959533907301413, -21.53943276465977519, 87.49890960531436690 ) ) ;
#67546=CARTESIAN_POINT ( 'NONE',  ( -19.02544592524342804, 5.153800228976336051, 51.04057627198103120 ) ) ;
#67547=CARTESIAN_POINT ( 'NONE',  ( 0.05219959533937995610, -21.53943276465977519, 60.00109039468568284 ) ) ;
#67548=CARTESIAN_POINT ( 'NONE',  ( -19.03943276465977164, 0.05219959533909376836, 36.24890960531436690 ) ) ;
#67550=CARTESIAN_POINT ( 'NONE',  ( -19.03943276465977164, 0.05219959533909376836, 56.24890960531435979 ) ) ;
#67551=CARTESIAN_POINT ( 'NONE',  ( 12.14591786802309770, 12.06949235617756955, 109.3739096053143811 ) ) ;
#67552=CARTESIAN_POINT ( 'NONE',  ( -13.89961937509977652, 13.97604488694528158, 95.62390960531436690 ) ) ;
#67553=CARTESIAN_POINT ( 'NONE',  ( -0.05219959533910754901, -16.53943276465976808, 57.49890960531435979 ) ) ;
#67554=CARTESIAN_POINT ( 'NONE',  ( -14.34966873604960291, -8.224510206698953496, 106.6655762719810383 ) ) ;
#67555=CARTESIAN_POINT ( 'NONE',  ( 15.80617190586746368, 15.72974639402197994, 79.37390960531436690 ) ) ;
#67556=CARTESIAN_POINT ( 'NONE',  ( -21.52544592524334988, -5.823673210054445271, 23.95942372801901143 ) ) ;
#67558=CARTESIAN_POINT ( 'NONE',  ( -8.314922557961024197, 14.29746914071037800, 42.91775706135235424 ) ) ;
#67559=ORIENTED_EDGE ( 'NONE', *, *, #193913, .F. ) ;
#67560=CARTESIAN_POINT ( 'NONE',  ( -5.823673210054116645, -21.52544592524344225, 67.29057627198103830 ) ) ;
#67561=CARTESIAN_POINT ( 'NONE',  ( 10.72451020669871369, 18.67979575497193778, 112.0844237280190185 ) ) ;
#67562=CARTESIAN_POINT ( 'NONE',  ( -0.05219959533909027116, -19.03943276465977164, 92.49890960531436690 ) ) ;
#67563=CARTESIAN_POINT ( 'NONE',  ( 10.72451020669871369, 18.67979575497193778, 27.08442372801901854 ) ) ;
#67564=CARTESIAN_POINT ( 'NONE',  ( -10.72451020669898014, 18.67979575497178502, 30.41557627198101699 ) ) ;
#67565=CARTESIAN_POINT ( 'NONE',  ( 14.34966873604972726, -8.224510206698740333, 105.8344237280190328 ) ) ;
#67566=CARTESIAN_POINT ( 'NONE',  ( 18.62759615963255655, 10.81492255796105972, 46.66775706135234714 ) ) ;
#67567=CARTESIAN_POINT ( 'NONE',  ( 18.67979575497194134, -10.72451020669871369, 85.83442372801901854 ) ) ;
#67568=CARTESIAN_POINT ( 'NONE',  ( -16.46253265017146816, -9.564922557961047289, 19.16775706135233293 ) ) ;
#67569=CARTESIAN_POINT ( 'NONE',  ( 8.314922557961029526, -14.29746914071037800, 70.41775706135236135 ) ) ;
#67570=CARTESIAN_POINT ( 'NONE',  ( -15.72974639402176322, -15.80617190586768395, 44.37609039468567573 ) ) ;
#67571=CARTESIAN_POINT ( 'NONE',  ( -19.05341960407611168, -5.049401038298163336, 36.45724293864766707 ) ) ;
#67572=CARTESIAN_POINT ( 'NONE',  ( -21.53943276465977519, -0.05219959533937600094, 103.7510903946857042 ) ) ;
#67573=CARTESIAN_POINT ( 'NONE',  ( 13.89961937509977652, -13.97604488694527269, 113.1239096053143527 ) ) ;
#67574=B_SPLINE_CURVE_WITH_KNOTS ( 'NONE', 3,
 ( #115457, #116454, #98253, #190300, #117451, #144780 ),
 .UNSPECIFIED., .F., .F.,
 ( 4, 2, 4 ),
 ( 0.000000000000000000, 0.0003837532665554014731, 0.0007675065331108029461 ),
 .UNSPECIFIED. ) ;
#67575=CARTESIAN_POINT ( 'NONE',  ( -0.05219959533907301413, -21.53943276465977519, 107.4989096053143669 ) ) ;
#67576=CARTESIAN_POINT ( 'NONE',  ( 19.01529144963338069, 5.499999999999978684, 83.73431955728436549 ) ) ;
#67577=CARTESIAN_POINT ( 'NONE',  ( 5.823673210054125526, 21.52544592524343514, 64.79057627198103830 ) ) ;
#67578=CARTESIAN_POINT ( 'NONE',  ( -14.34966873604972548, 8.224510206698743886, 48.33442372801902565 ) ) ;
#67579=CARTESIAN_POINT ( 'NONE',  ( 14.29746914071049879, -8.314922557960816363, 43.33224293864769550 ) ) ;
#67581=CARTESIAN_POINT ( 'NONE',  ( -16.46253265017146816, -9.564922557961047289, 79.16775706135234714 ) ) ;
#67582=CARTESIAN_POINT ( 'NONE',  ( -16.88567814943161949, 6.947325034625681184, 103.7099887734741372 ) ) ;
#67583=CARTESIAN_POINT ( 'NONE',  ( 8.314922557961029526, -14.29746914071037800, 30.41775706135234358 ) ) ;
#67584=CARTESIAN_POINT ( 'NONE',  ( 21.55341960407610458, 5.719274019375980345, 98.95724293864770971 ) ) ;
#67585=CARTESIAN_POINT ( 'NONE',  ( 0.05219959533910956823, 16.53943276465976808, 64.99890960531435269 ) ) ;
#67586=CARTESIAN_POINT ( 'NONE',  ( 16.46253265017160672, -9.564922557960803928, 108.3322429386476955 ) ) ;
#67587=CARTESIAN_POINT ( 'NONE',  ( -0.05219959533934338120, 16.53943276465976808, 42.50109039468567573 ) ) ;
#67588=CARTESIAN_POINT ( 'NONE',  ( 5.049401038298161559, -19.05341960407611168, 62.70724293864769550 ) ) ;
#67589=CARTESIAN_POINT ( 'NONE',  ( -15.72974639402176322, -15.80617190586768395, 34.37609039468568284 ) ) ;
#67590=CARTESIAN_POINT ( 'NONE',  ( 5.049401038297881783, 19.05341960407617563, 92.29275706135234714 ) ) ;
#67591=CARTESIAN_POINT ( 'NONE',  ( -0.05219959533909027116, -19.03943276465977164, 112.4989096053143669 ) ) ;
#67592=CARTESIAN_POINT ( 'NONE',  ( -16.46253265017160317, 9.564922557960807481, 90.83224293864769550 ) ) ;
#67593=CARTESIAN_POINT ( 'NONE',  ( -18.62759615963270932, 10.81492255796079327, 95.83224293864770971 ) ) ;
#67594=CARTESIAN_POINT ( 'NONE',  ( 16.51473224551069308, 9.474510206698969483, 59.16557627198102409 ) ) ;
#67596=CARTESIAN_POINT ( 'NONE',  ( 16.55341960407611168, 4.379528057220329451, 68.95724293864769550 ) ) ;
#67597=CARTESIAN_POINT ( 'NONE',  ( -13.89961937509977652, 13.97604488694528158, 105.6239096053143527 ) ) ;
#67599=CARTESIAN_POINT ( 'NONE',  ( -13.89961937509957401, -13.97604488694547875, 84.37609039468567573 ) ) ;
#67600=CARTESIAN_POINT ( 'NONE',  ( -21.53943276465977519, 0.05219959533907696930, 86.24890960531436690 ) ) ;
#67601=CARTESIAN_POINT ( 'NONE',  ( 19.05341960407617918, -5.049401038297876454, 46.04275706135233293 ) ) ;
#67602=CARTESIAN_POINT ( 'NONE',  ( -19.02544592524342804, 5.153800228976336051, 111.0405762719810099 ) ) ;
#67603=CARTESIAN_POINT ( 'NONE',  ( 10.81492255796078972, 18.62759615963270932, 59.58224293864770260 ) ) ;
#67604=CARTESIAN_POINT ( 'NONE',  ( 13.89961937509977652, -13.97604488694527269, 83.12390960531436690 ) ) ;
#67605=CARTESIAN_POINT ( 'NONE',  ( 21.55341960407619695, -5.719274019375665929, 81.04275706135236135 ) ) ;
#67606=CARTESIAN_POINT ( 'NONE',  ( 19.02544592524343514, -5.153800228976328945, 43.54057627198103120 ) ) ;
#67607=CARTESIAN_POINT ( 'NONE',  ( 0.05219959533910956823, 16.53943276465976808, 69.99890960531435269 ) ) ;
#67608=CARTESIAN_POINT ( 'NONE',  ( 14.34966873604972726, -8.224510206698740333, 25.83442372801901499 ) ) ;
#67609=CARTESIAN_POINT ( 'NONE',  ( 10.72451020669871369, 18.67979575497193778, 72.08442372801899012 ) ) ;
#67611=CARTESIAN_POINT ( 'NONE',  ( 5.049401038297881783, 19.05341960407617563, 32.29275706135233293 ) ) ;
#67612=CARTESIAN_POINT ( 'NONE',  ( 19.03943276465977164, 0.05219959533936151252, 81.25109039468567573 ) ) ;
#67614=CARTESIAN_POINT ( 'NONE',  ( -21.52544592524343514, 5.823673210054127303, 116.0405762719810383 ) ) ;
#67616=CARTESIAN_POINT ( 'NONE',  ( -9.474510206698720793, -16.51473224551083518, 24.58442372801900078 ) ) ;
#67617=CARTESIAN_POINT ( 'NONE',  ( -0.05219959533909027116, -19.03943276465977164, 57.49890960531435979 ) ) ;
#67618=CARTESIAN_POINT ( 'NONE',  ( -0.05219959533936034679, 19.03943276465977164, 22.50109039468566152 ) ) ;
#67619=CARTESIAN_POINT ( 'NONE',  ( -12.06949235617739369, -12.14591786802326823, 104.3760903946856899 ) ) ;
#67620=CARTESIAN_POINT ( 'NONE',  ( 19.02544592524343514, -5.153800228976328945, 98.54057627198100988 ) ) ;
#67621=CARTESIAN_POINT ( 'NONE',  ( 18.62759615963255655, 10.81492255796105972, 66.66775706135234714 ) ) ;
#67625=CARTESIAN_POINT ( 'NONE',  ( -0.05219959533937732626, 21.53943276465977519, 87.50109039468568994 ) ) ;
#67626=CARTESIAN_POINT ( 'NONE',  ( 18.67979575497194134, -10.72451020669871369, 100.8344237280190185 ) ) ;
#67628=CARTESIAN_POINT ( 'NONE',  ( 13.97604488694527802, 13.89961937509977652, 104.3739096053143385 ) ) ;
#67629=CARTESIAN_POINT ( 'NONE',  ( 13.97604488694548053, -13.89961937509957401, 25.62609039468566507 ) ) ;
#67631=CARTESIAN_POINT ( 'NONE',  ( -5.049401038298153566, 19.05341960407611168, 35.20724293864768839 ) ) ;
#67632=CARTESIAN_POINT ( 'NONE',  ( -21.55341960407610458, -5.719274019375992779, 61.45724293864770260 ) ) ;
#67634=CARTESIAN_POINT ( 'NONE',  ( -4.483927247898782831, 16.52544592524335698, 102.7094237280190185 ) ) ;
#67635=CARTESIAN_POINT ( 'NONE',  ( -4.483927247898539470, -16.52544592524342804, 102.2905762719810383 ) ) ;
#67636=CARTESIAN_POINT ( 'NONE',  ( -19.05341960407611168, -5.049401038298163336, 81.45724293864769550 ) ) ;
#67637=CARTESIAN_POINT ( 'NONE',  ( 18.67979575497194134, -10.72451020669871369, 100.8344237280190185 ) ) ;
#67638=CARTESIAN_POINT ( 'NONE',  ( 9.564922557960805705, 16.46253265017160317, 34.58224293864770260 ) ) ;
#67639=CARTESIAN_POINT ( 'NONE',  ( -0.05219959533910754901, -16.53943276465976808, 97.49890960531436690 ) ) ;
#67640=CARTESIAN_POINT ( 'NONE',  ( -5.823673210054431948, 21.52544592524334988, 52.70942372801902565 ) ) ;
#67641=CARTESIAN_POINT ( 'NONE',  ( -10.81492255796078084, -18.62759615963271287, 92.08224293864769550 ) ) ;
#67642=CARTESIAN_POINT ( 'NONE',  ( -16.46253265017146816, -9.564922557961047289, 49.16775706135233293 ) ) ;
#67644=CARTESIAN_POINT ( 'NONE',  ( 16.46253265017160672, -9.564922557960803928, 93.33224293864769550 ) ) ;
#67645=CARTESIAN_POINT ( 'NONE',  ( -8.224510206698948167, 14.34966873604960824, 75.41557627198102409 ) ) ;
#67647=CARTESIAN_POINT ( 'NONE',  ( 5.153800228976615827, -19.02544592524334988, 50.20942372801897591 ) ) ;
#67648=CARTESIAN_POINT ( 'NONE',  ( 16.51473224551069308, 9.474510206698969483, 69.16557627198102409 ) ) ;
#67649=VECTOR ( 'NONE', #170791, 1000.000000000000000 ) ;
#67650=CARTESIAN_POINT ( 'NONE',  ( -4.379528057220328563, 16.55341960407611168, 50.20724293864769550 ) ) ;
#67651=CARTESIAN_POINT ( 'NONE',  ( -13.89961937509957401, -13.97604488694547875, 84.37609039468567573 ) ) ;
#67653=CARTESIAN_POINT ( 'NONE',  ( 5.823673210054125526, 21.52544592524343514, 34.79057627198103120 ) ) ;
#67654=CARTESIAN_POINT ( 'NONE',  ( 16.52544592524342804, -4.483927247898539470, 103.5405762719810383 ) ) ;
#67655=CARTESIAN_POINT ( 'NONE',  ( -17.50000000000001776, -3.850315288878612741, 25.73370869396545046 ) ) ;
#67656=CARTESIAN_POINT ( 'NONE',  ( -19.05341960407611168, -5.049401038298163336, 61.45724293864769550 ) ) ;
#67657=CARTESIAN_POINT ( 'NONE',  ( 18.62759615963271287, -10.81492255796078972, 58.33224293864768839 ) ) ;
#67658=CARTESIAN_POINT ( 'NONE',  ( 9.474510206698971260, -16.51473224551069308, 27.91557627198103120 ) ) ;
#67659=CARTESIAN_POINT ( 'NONE',  ( -14.34966873604972548, 8.224510206698743886, 83.33442372801903275 ) ) ;
#67660=CARTESIAN_POINT ( 'NONE',  ( 5.153800228976335163, 19.02544592524342804, 59.79057627198100988 ) ) ;
#67661=CARTESIAN_POINT ( 'NONE',  ( -16.46253265017146816, -9.564922557961047289, 54.16775706135234003 ) ) ;
#67662=CARTESIAN_POINT ( 'NONE',  ( -21.53943276465977519, -0.05219959533937600094, 68.75109039468568994 ) ) ;
#67664=CARTESIAN_POINT ( 'NONE',  ( -15.80617190586745835, -15.72974639402198527, 46.87390960531435979 ) ) ;
#67665=CARTESIAN_POINT ( 'NONE',  ( -16.51473224551069308, -9.474510206698971260, 26.66557627198103120 ) ) ;
#67666=CARTESIAN_POINT ( 'NONE',  ( 0.05219959533934541429, -16.53943276465976808, 90.00109039468567573 ) ) ;
#67667=CARTESIAN_POINT ( 'NONE',  ( -5.153800228976607833, 19.02544592524334988, 107.7094237280189759 ) ) ;
#67668=CARTESIAN_POINT ( 'NONE',  ( -9.474510206698964154, 16.51473224551069663, 25.41557627198103120 ) ) ;
#67669=CARTESIAN_POINT ( 'NONE',  ( 17.48853670773243962, 5.747243402303178428, 53.83328700250012133 ) ) ;
#67670=CARTESIAN_POINT ( 'NONE',  ( -21.53943276465977519, 0.05219959533907696930, 56.24890960531436690 ) ) ;
#67671=CARTESIAN_POINT ( 'NONE',  ( -21.52544592524334988, -5.823673210054445271, 93.95942372801903275 ) ) ;
#67672=CARTESIAN_POINT ( 'NONE',  ( -14.29746914071049879, 8.314922557960819915, 50.83224293864770971 ) ) ;
#67673=CARTESIAN_POINT ( 'NONE',  ( -16.53943276465976808, 0.05219959533911058130, 51.24890960531436690 ) ) ;
#67674=CARTESIAN_POINT ( 'NONE',  ( -0.05219959533907301413, -21.53943276465977519, 82.49890960531436690 ) ) ;
#67675=CARTESIAN_POINT ( 'NONE',  ( -18.67979575497178146, -10.72451020669898902, 91.66557627198103830 ) ) ;
#67677=CARTESIAN_POINT ( 'NONE',  ( 21.53943276465977519, -0.05219959533907433946, 38.74890960531435979 ) ) ;
#67678=CARTESIAN_POINT ( 'NONE',  ( 4.483927247898790824, -16.52544592524335698, 70.20942372801904696 ) ) ;
#67679=CARTESIAN_POINT ( 'NONE',  ( -14.29746914071049879, 8.314922557960819915, 75.83224293864769550 ) ) ;
#67680=CARTESIAN_POINT ( 'NONE',  ( 19.03943276465977164, -0.05219959533909143690, 38.74890960531436690 ) ) ;
#67684=CARTESIAN_POINT ( 'NONE',  ( 4.483927247898790824, -16.52544592524335698, 90.20942372801903275 ) ) ;
#67685=CARTESIAN_POINT ( 'NONE',  ( 15.72974639402199770, -15.80617190586745480, 113.1239096053143953 ) ) ;
#67686=CARTESIAN_POINT ( 'NONE',  ( -5.049401038298153566, 19.05341960407611168, 80.20724293864769550 ) ) ;
#67687=CARTESIAN_POINT ( 'NONE',  ( -0.05219959533937732626, 21.53943276465977519, 52.50109039468567573 ) ) ;
#67688=CARTESIAN_POINT ( 'NONE',  ( -19.03943276465977164, 0.05219959533909376836, 106.2489096053143669 ) ) ;
#67691=CARTESIAN_POINT ( 'NONE',  ( -15.80617190586768217, 15.72974639402176855, 43.12609039468568284 ) ) ;
#67692=CARTESIAN_POINT ( 'NONE',  ( 5.049401038298161559, -19.05341960407611168, 37.70724293864768839 ) ) ;
#67693=CARTESIAN_POINT ( 'NONE',  ( 5.049401038298161559, -19.05341960407611168, 97.70724293864766707 ) ) ;
#67694=CARTESIAN_POINT ( 'NONE',  ( -9.474510206698720793, -16.51473224551083518, 54.58442372801899722 ) ) ;
#67695=CARTESIAN_POINT ( 'NONE',  ( -5.823673210054431948, 21.52544592524334988, 32.70942372801900433 ) ) ;
#67696=CARTESIAN_POINT ( 'NONE',  ( 19.03943276465977164, 0.05219959533936151252, 51.25109039468567573 ) ) ;
#67697=CARTESIAN_POINT ( 'NONE',  ( -16.46253265017160317, 9.564922557960807481, 25.83224293864769194 ) ) ;
#67698=CARTESIAN_POINT ( 'NONE',  ( -12.14591786802326823, 12.06949235617739902, 93.12609039468568994 ) ) ;
#67699=CARTESIAN_POINT ( 'NONE',  ( 16.46253265017146816, 9.564922557961045513, 61.66775706135234003 ) ) ;
#67700=CARTESIAN_POINT ( 'NONE',  ( -12.14591786802326823, 12.06949235617739902, 108.1260903946856757 ) ) ;
#67702=CARTESIAN_POINT ( 'NONE',  ( -5.049401038298153566, 19.05341960407611168, 80.20724293864769550 ) ) ;
#67703=CARTESIAN_POINT ( 'NONE',  ( -10.81492255796105439, 18.62759615963255655, 97.91775706135236135 ) ) ;
#67704=CARTESIAN_POINT ( 'NONE',  ( 10.81492255796106328, -18.62759615963255655, 105.4177570613523613 ) ) ;
#67706=CARTESIAN_POINT ( 'NONE',  ( -13.89961937509977652, 13.97604488694528158, 100.6239096053143669 ) ) ;
#67707=CARTESIAN_POINT ( 'NONE',  ( -15.72974639402176322, -15.80617190586768395, 69.37609039468567573 ) ) ;
#67708=CARTESIAN_POINT ( 'NONE',  ( 4.483927247898790824, -16.52544592524335698, 20.20942372801900788 ) ) ;
#67709=CARTESIAN_POINT ( 'NONE',  ( 0.05219959533909260263, 19.03943276465977164, 79.99890960531436690 ) ) ;
#67710=CARTESIAN_POINT ( 'NONE',  ( 18.62759615963271287, -10.81492255796078972, 28.33224293864769550 ) ) ;
#67711=CARTESIAN_POINT ( 'NONE',  ( -19.03943276465977164, 0.05219959533909376836, 91.24890960531436690 ) ) ;
#67713=CARTESIAN_POINT ( 'NONE',  ( 13.97604488694527802, 13.89961937509977652, 74.37390960531436690 ) ) ;
#67714=CARTESIAN_POINT ( 'NONE',  ( -9.564922557960796823, -16.46253265017161027, 67.08224293864769550 ) ) ;
#67715=CARTESIAN_POINT ( 'NONE',  ( -14.29746914071037622, -8.314922557961029526, 109.1677570613523613 ) ) ;
#67716=CARTESIAN_POINT ( 'NONE',  ( -19.01529144963332030, -5.500000000000166978, 41.23431955728439391 ) ) ;
#67717=CARTESIAN_POINT ( 'NONE',  ( 9.564922557961047289, -16.46253265017146816, 70.41775706135233293 ) ) ;
#67718=CARTESIAN_POINT ( 'NONE',  ( 16.46253265017160672, -9.564922557960803928, 88.33224293864769550 ) ) ;
#67719=CARTESIAN_POINT ( 'NONE',  ( -12.14591786802309592, -12.06949235617757132, 86.87390960531438111 ) ) ;
#67720=CARTESIAN_POINT ( 'NONE',  ( -18.62759615963270932, 10.81492255796079327, 40.83224293864769550 ) ) ;
#67721=CARTESIAN_POINT ( 'NONE',  ( 21.53943276465977519, -0.05219959533907433946, 23.74890960531435269 ) ) ;
#67722=CARTESIAN_POINT ( 'NONE',  ( -14.34966873604960291, -8.224510206698953496, 106.6655762719810383 ) ) ;
#67723=CARTESIAN_POINT ( 'NONE',  ( -17.48853670773242541, 5.747243402303156223, 53.66671299749993551 ) ) ;
#67724=CARTESIAN_POINT ( 'NONE',  ( -16.46253265017146816, -9.564922557961047289, 39.16775706135234003 ) ) ;
#67725=CARTESIAN_POINT ( 'NONE',  ( 12.06949235617757843, -12.14591786802309237, 28.12390960531435979 ) ) ;
#67726=CARTESIAN_POINT ( 'NONE',  ( -5.049401038298153566, 19.05341960407611168, 105.2072429386476671 ) ) ;
#67727=CARTESIAN_POINT ( 'NONE',  ( -10.72451020669870658, -18.67979575497194134, 64.58442372801900433 ) ) ;
#67728=CARTESIAN_POINT ( 'NONE',  ( 0.05219959533907565091, 21.53943276465977519, 59.99890960531436690 ) ) ;
#67729=CARTESIAN_POINT ( 'NONE',  ( 10.81492255796106328, -18.62759615963255655, 25.41775706135235779 ) ) ;
#67730=CARTESIAN_POINT ( 'NONE',  ( -15.72974639402197994, 15.80617190586746368, 80.62390960531438111 ) ) ;
#67731=CARTESIAN_POINT ( 'NONE',  ( -21.53943276465977519, -0.05219959533937600094, 43.75109039468568284 ) ) ;
#67732=CARTESIAN_POINT ( 'NONE',  ( 14.29746914071049879, -8.314922557960816363, 108.3322429386477097 ) ) ;
#67733=CARTESIAN_POINT ( 'NONE',  ( -16.46253265017146816, -9.564922557961047289, 64.16775706135233293 ) ) ;
#67734=CARTESIAN_POINT ( 'NONE',  ( 13.97604488694527802, 13.89961937509977652, 49.37390960531434558 ) ) ;
#67735=CARTESIAN_POINT ( 'NONE',  ( -16.52544592524342804, 4.483927247898546575, 86.04057627198102409 ) ) ;
#67736=CARTESIAN_POINT ( 'NONE',  ( 19.05341960407611168, 5.049401038298154454, 103.9572429386476671 ) ) ;
#67737=CARTESIAN_POINT ( 'NONE',  ( -19.03943276465977164, 0.05219959533909376836, 26.24890960531435624 ) ) ;
#67738=CARTESIAN_POINT ( 'NONE',  ( -8.314922557960811034, -14.29746914071050412, 42.08224293864769550 ) ) ;
#67739=CARTESIAN_POINT ( 'NONE',  ( -8.224510206698735004, -14.34966873604973081, 94.58442372801901854 ) ) ;
#67740=CARTESIAN_POINT ( 'NONE',  ( -19.03943276465977164, 0.05219959533909376836, 56.24890960531435979 ) ) ;
#67741=CARTESIAN_POINT ( 'NONE',  ( 19.02544592524343514, -5.153800228976328945, 23.54057627198102054 ) ) ;
#67742=CARTESIAN_POINT ( 'NONE',  ( 16.46253265017146816, 9.564922557961045513, 26.66775706135234003 ) ) ;
#67743=CARTESIAN_POINT ( 'NONE',  ( 5.153800228976335163, 19.02544592524342804, 109.7905762719810099 ) ) ;
#67744=CARTESIAN_POINT ( 'NONE',  ( -8.224510206698948167, 14.34966873604960824, 35.41557627198102409 ) ) ;
#67745=CARTESIAN_POINT ( 'NONE',  ( 18.67979575497194134, -10.72451020669871369, 45.83442372801901854 ) ) ;
#67746=CARTESIAN_POINT ( 'NONE',  ( 19.05341960407611168, 5.049401038298154454, 113.9572429386477097 ) ) ;
#67747=CARTESIAN_POINT ( 'NONE',  ( 4.379528057220092307, 16.55341960407617563, 62.29275706135236845 ) ) ;
#67748=CARTESIAN_POINT ( 'NONE',  ( 16.53943276465976808, -0.05219959533910856209, 23.74890960531435269 ) ) ;
#67749=CARTESIAN_POINT ( 'NONE',  ( 16.55341960407618274, -4.379528057220086978, 106.0427570613523471 ) ) ;
#67750=CARTESIAN_POINT ( 'NONE',  ( -8.314922557961024197, 14.29746914071037800, 22.91775706135235069 ) ) ;
#67751=CARTESIAN_POINT ( 'NONE',  ( 9.474510206698971260, -16.51473224551069308, 47.91557627198102409 ) ) ;
#67752=CARTESIAN_POINT ( 'NONE',  ( 12.06949235617757843, -12.14591786802309237, 108.1239096053143811 ) ) ;
#67753=CARTESIAN_POINT ( 'NONE',  ( -18.62759615963255300, -10.81492255796106328, 24.16775706135235424 ) ) ;
#67754=CARTESIAN_POINT ( 'NONE',  ( 13.89961937509977652, -13.97604488694527269, 43.12390960531434558 ) ) ;
#67756=CARTESIAN_POINT ( 'NONE',  ( -16.46253265017160317, 9.564922557960807481, 35.83224293864768839 ) ) ;
#67757=CARTESIAN_POINT ( 'NONE',  ( 10.72451020669898902, -18.67979575497178502, 22.91557627198102765 ) ) ;
#67758=CARTESIAN_POINT ( 'NONE',  ( -17.26172910966780805, -6.454744622555800504, 34.19353091350776452 ) ) ;
#67760=CARTESIAN_POINT ( 'NONE',  ( -19.05341960407611168, -5.049401038298163336, 96.45724293864769550 ) ) ;
#67761=CARTESIAN_POINT ( 'NONE',  ( 15.72974639402176855, 15.80617190586768217, 46.87609039468568994 ) ) ;
#67762=CARTESIAN_POINT ( 'NONE',  ( -12.06949235617756955, 12.14591786802309770, 100.6239096053143811 ) ) ;
#67763=CARTESIAN_POINT ( 'NONE',  ( 19.02544592524343514, -5.153800228976328945, 108.5405762719810383 ) ) ;
#67765=CARTESIAN_POINT ( 'NONE',  ( -14.29746914071037622, -8.314922557961029526, 74.16775706135231871 ) ) ;
#67766=CARTESIAN_POINT ( 'NONE',  ( -5.823673210054431948, 21.52544592524334988, 97.70942372801904696 ) ) ;
#67767=CARTESIAN_POINT ( 'NONE',  ( -4.483927247898782831, 16.52544592524335698, 52.70942372801902565 ) ) ;
#67768=CARTESIAN_POINT ( 'NONE',  ( 9.474510206698971260, -16.51473224551069308, 97.91557627198102409 ) ) ;
#67769=CARTESIAN_POINT ( 'NONE',  ( -4.379528057220086978, -16.55341960407618274, 44.79275706135234714 ) ) ;
#67770=CARTESIAN_POINT ( 'NONE',  ( 13.89961937509957401, 13.97604488694547697, 111.8760903946856757 ) ) ;
#67771=CARTESIAN_POINT ( 'NONE',  ( -16.55341960407617563, 4.379528057220093196, 88.54275706135236135 ) ) ;
#67772=CARTESIAN_POINT ( 'NONE',  ( 5.049401038297881783, 19.05341960407617563, 112.2927570613523471 ) ) ;
#67773=CARTESIAN_POINT ( 'NONE',  ( -19.05341960407611168, -5.049401038298163336, 76.45724293864769550 ) ) ;
#67774=CARTESIAN_POINT ( 'NONE',  ( -21.55341960407610458, -5.719274019375992779, 91.45724293864769550 ) ) ;
#67775=CARTESIAN_POINT ( 'NONE',  ( 4.483927247898545687, 16.52544592524342804, 104.7905762719810241 ) ) ;
#67776=CARTESIAN_POINT ( 'NONE',  ( 9.564922557961047289, -16.46253265017146816, 105.4177570613523471 ) ) ;
#67777=CARTESIAN_POINT ( 'NONE',  ( 16.55341960407618274, -4.379528057220086978, 71.04275706135234714 ) ) ;
#67779=CARTESIAN_POINT ( 'NONE',  ( 19.05341960407617918, -5.049401038297876454, 71.04275706135234714 ) ) ;
#67780=CARTESIAN_POINT ( 'NONE',  ( -16.53943276465976808, 0.05219959533911058130, 26.24890960531435624 ) ) ;
#67781=CARTESIAN_POINT ( 'NONE',  ( 16.53943276465976808, -0.05219959533910856209, 93.74890960531436690 ) ) ;
#67782=CARTESIAN_POINT ( 'NONE',  ( 9.474510206698729675, 16.51473224551082808, 37.08442372801899722 ) ) ;
#67783=CARTESIAN_POINT ( 'NONE',  ( -17.12812012977028431, 6.668231424565927767, 88.64051240676862164 ) ) ;
#67784=CARTESIAN_POINT ( 'NONE',  ( -15.80617190586768217, 15.72974639402176855, 33.12609039468569705 ) ) ;
#67785=CARTESIAN_POINT ( 'NONE',  ( 5.049401038297881783, 19.05341960407617563, 92.29275706135234714 ) ) ;
#67786=CARTESIAN_POINT ( 'NONE',  ( -16.46253265017160317, 9.564922557960807481, 115.8322429386477097 ) ) ;
#67787=CARTESIAN_POINT ( 'NONE',  ( 0.05219959533909260263, 19.03943276465977164, 94.99890960531436690 ) ) ;
#67788=CARTESIAN_POINT ( 'NONE',  ( 5.823673210054444382, -21.52544592524334988, 90.20942372801903275 ) ) ;
#67789=CARTESIAN_POINT ( 'NONE',  ( 19.02544592524343514, -5.153800228976328945, 73.54057627198103830 ) ) ;
#67791=CARTESIAN_POINT ( 'NONE',  ( -21.53943276465977519, 0.05219959533907696930, 41.24890960531435269 ) ) ;
#67792=CARTESIAN_POINT ( 'NONE',  ( 12.14591786802309770, 12.06949235617756955, 99.37390960531436690 ) ) ;
#67793=CARTESIAN_POINT ( 'NONE',  ( 13.89961937509977652, -13.97604488694527269, 53.12390960531434558 ) ) ;
#67794=CARTESIAN_POINT ( 'NONE',  ( 14.29746914071049879, -8.314922557960816363, 108.3322429386477097 ) ) ;
#67795=CARTESIAN_POINT ( 'NONE',  ( 15.72974639402176855, 15.80617190586768217, 26.87609039468567218 ) ) ;
#67797=CARTESIAN_POINT ( 'NONE',  ( 10.72451020669871369, 18.67979575497193778, 77.08442372801901854 ) ) ;
#67798=CARTESIAN_POINT ( 'NONE',  ( 0.05219959533909260263, 19.03943276465977164, 44.99890960531435979 ) ) ;
#67799=CARTESIAN_POINT ( 'NONE',  ( -16.53943276465976808, -0.05219959533934237506, 78.75109039468568994 ) ) ;
#67800=CARTESIAN_POINT ( 'NONE',  ( 21.53943276465977519, 0.05219959533937863772, 21.25109039468567218 ) ) ;
#67802=CARTESIAN_POINT ( 'NONE',  ( 15.72974639402176855, 15.80617190586768217, 31.87609039468567929 ) ) ;
#67803=CARTESIAN_POINT ( 'NONE',  ( 0.05219959533936267826, -19.03943276465977164, 55.00109039468566863 ) ) ;
#67804=CARTESIAN_POINT ( 'NONE',  ( -16.51473224551069308, -9.474510206698971260, 61.66557627198103120 ) ) ;
#67805=CARTESIAN_POINT ( 'NONE',  ( -19.05341960407617563, 5.049401038297882671, 38.54275706135233293 ) ) ;
#67806=CARTESIAN_POINT ( 'NONE',  ( 5.719274019375673035, 21.55341960407619339, 72.29275706135236135 ) ) ;
#67807=CARTESIAN_POINT ( 'NONE',  ( 18.67979575497178502, 10.72451020669898547, 74.16557627198102409 ) ) ;
#67808=CARTESIAN_POINT ( 'NONE',  ( -14.29746914071049879, 8.314922557960819915, 45.83224293864769550 ) ) ;
#67809=CARTESIAN_POINT ( 'NONE',  ( -18.67979575497193778, 10.72451020669871902, 93.33442372801901854 ) ) ;
#67810=CARTESIAN_POINT ( 'NONE',  ( -9.474510206698720793, -16.51473224551083518, 34.58442372801899722 ) ) ;
#67811=CARTESIAN_POINT ( 'NONE',  ( 4.379528057220339221, -16.55341960407611168, 67.70724293864769550 ) ) ;
#67812=CARTESIAN_POINT ( 'NONE',  ( -4.379528057220328563, 16.55341960407611168, 115.2072429386476955 ) ) ;
#67813=CARTESIAN_POINT ( 'NONE',  ( -0.05219959533936034679, 19.03943276465977164, 52.50109039468566863 ) ) ;
#67814=CARTESIAN_POINT ( 'NONE',  ( -12.14591786802326823, 12.06949235617739902, 113.1260903946856899 ) ) ;
#67815=CARTESIAN_POINT ( 'NONE',  ( 15.80617190586769283, -15.72974639402175789, 85.62609039468568994 ) ) ;
#67816=CARTESIAN_POINT ( 'NONE',  ( -16.46253265017146816, -9.564922557961047289, 44.16775706135232582 ) ) ;
#67817=CARTESIAN_POINT ( 'NONE',  ( -21.55341960407610458, -5.719274019375992779, 56.45724293864768839 ) ) ;
#67818=CARTESIAN_POINT ( 'NONE',  ( -18.62759615963255300, -10.81492255796106328, 49.16775706135234003 ) ) ;
#67819=CARTESIAN_POINT ( 'NONE',  ( 15.72974639402199770, -15.80617190586745480, 98.12390960531436690 ) ) ;
#67820=CARTESIAN_POINT ( 'NONE',  ( -16.46253265017146816, -9.564922557961047289, 99.16775706135233293 ) ) ;
#67821=CARTESIAN_POINT ( 'NONE',  ( 14.34966873604972726, -8.224510206698740333, 70.83442372801901854 ) ) ;
#67823=CARTESIAN_POINT ( 'NONE',  ( 21.55341960407610458, 5.719274019375980345, 103.9572429386476813 ) ) ;
#67824=CARTESIAN_POINT ( 'NONE',  ( -14.34966873604960291, -8.224510206698953496, 91.66557627198103830 ) ) ;
#67825=CARTESIAN_POINT ( 'NONE',  ( -17.50000000000011369, -3.417042746627175109, 29.82619603767520644 ) ) ;
#67826=CARTESIAN_POINT ( 'NONE',  ( 14.34966873604972726, -8.224510206698740333, 35.83442372801901143 ) ) ;
#67827=CARTESIAN_POINT ( 'NONE',  ( 15.80617190586746368, 15.72974639402197994, 54.37390960531435979 ) ) ;
#67828=CARTESIAN_POINT ( 'NONE',  ( 14.34966873604972726, -8.224510206698740333, 95.83442372801903275 ) ) ;
#67829=DIRECTION ( 'NONE',  ( 0.000000000000000000, 0.000000000000000000, -1.000000000000000000 ) ) ;
#67830=CARTESIAN_POINT ( 'NONE',  ( -8.314922557961024197, 14.29746914071037800, 72.91775706135234714 ) ) ;
#67831=CARTESIAN_POINT ( 'NONE',  ( 0.05219959533937995610, -21.53943276465977519, 45.00109039468568284 ) ) ;
#67832=CARTESIAN_POINT ( 'NONE',  ( 21.52544592524344225, -5.823673210054117533, 63.54057627198103830 ) ) ;
#67833=CARTESIAN_POINT ( 'NONE',  ( -16.53943276465976808, -0.05219959533934237506, 83.75109039468568994 ) ) ;
#67834=CARTESIAN_POINT ( 'NONE',  ( 21.53943276465977519, 0.05219959533937863772, 76.25109039468568994 ) ) ;
#67835=CARTESIAN_POINT ( 'NONE',  ( 21.55341960407610458, 5.719274019375980345, 58.95724293864770971 ) ) ;
#67836=CARTESIAN_POINT ( 'NONE',  ( -18.67979575497178146, -10.72451020669898902, 36.66557627198103120 ) ) ;
#67837=CARTESIAN_POINT ( 'NONE',  ( -12.06949235617739369, -12.14591786802326823, 59.37609039468568284 ) ) ;
#67838=CARTESIAN_POINT ( 'NONE',  ( -10.81492255796078084, -18.62759615963271287, 32.08224293864769550 ) ) ;
#67840=CARTESIAN_POINT ( 'NONE',  ( 9.474510206698971260, -16.51473224551069308, 92.91557627198103830 ) ) ;
#67841=CARTESIAN_POINT ( 'NONE',  ( 12.06949235617739724, 12.14591786802326823, 106.8760903946856899 ) ) ;
#67843=CARTESIAN_POINT ( 'NONE',  ( 16.55341960407611168, 4.379528057220329451, 113.9572429386477239 ) ) ;
#67844=CARTESIAN_POINT ( 'NONE',  ( -0.05219959533907301413, -21.53943276465977519, 52.49890960531435979 ) ) ;
#67845=CARTESIAN_POINT ( 'NONE',  ( 16.51473224551069308, 9.474510206698969483, 49.16557627198102409 ) ) ;
#67846=CARTESIAN_POINT ( 'NONE',  ( 4.483927247898790824, -16.52544592524335698, 95.20942372801903275 ) ) ;
#67847=CARTESIAN_POINT ( 'NONE',  ( -5.719274019375665041, -21.55341960407619695, 39.79275706135235424 ) ) ;
#67848=CARTESIAN_POINT ( 'NONE',  ( 5.153800228976615827, -19.02544592524334988, 85.20942372801900433 ) ) ;
#67849=CARTESIAN_POINT ( 'NONE',  ( -16.52544592524342804, 4.483927247898546575, 106.0405762719810525 ) ) ;
#67850=CARTESIAN_POINT ( 'NONE',  ( 9.564922557960805705, 16.46253265017160317, 54.58224293864769550 ) ) ;
#67852=CARTESIAN_POINT ( 'NONE',  ( 17.97161686093727795, -5.499999999999996447, 63.49637206859166838 ) ) ;
#67853=CARTESIAN_POINT ( 'NONE',  ( 13.97604488694527802, 13.89961937509977652, 79.37390960531435269 ) ) ;
#67854=CARTESIAN_POINT ( 'NONE',  ( -16.52544592524335698, -4.483927247898792601, 68.95942372801901854 ) ) ;
#67855=CARTESIAN_POINT ( 'NONE',  ( 21.53943276465977519, 0.05219959533937863772, 106.2510903946856757 ) ) ;
#67856=CARTESIAN_POINT ( 'NONE',  ( -10.81492255796078084, -18.62759615963271287, 47.08224293864770260 ) ) ;
#67857=CARTESIAN_POINT ( 'NONE',  ( 4.483927247898790824, -16.52544592524335698, 70.20942372801904696 ) ) ;
#67858=CARTESIAN_POINT ( 'NONE',  ( -9.564922557961040184, 16.46253265017147172, 67.91775706135233293 ) ) ;
#67860=CARTESIAN_POINT ( 'NONE',  ( -21.55341960407619339, 5.719274019375674811, 68.54275706135234714 ) ) ;
#67861=CARTESIAN_POINT ( 'NONE',  ( 0.05219959533909260263, 19.03943276465977164, 64.99890960531436690 ) ) ;
#67862=CARTESIAN_POINT ( 'NONE',  ( 13.97604488694527802, 13.89961937509977652, 34.37390960531436690 ) ) ;
#67863=CARTESIAN_POINT ( 'NONE',  ( -13.97604488694547697, 13.89961937509957934, 53.12609039468565442 ) ) ;
#67864=CARTESIAN_POINT ( 'NONE',  ( -16.46253265017160317, 9.564922557960807481, 115.8322429386477097 ) ) ;
#67865=CARTESIAN_POINT ( 'NONE',  ( -16.51473224551069308, -9.474510206698971260, 91.66557627198103830 ) ) ;
#67866=CARTESIAN_POINT ( 'NONE',  ( 4.379528057220339221, -16.55341960407611168, 57.70724293864770260 ) ) ;
#67867=CARTESIAN_POINT ( 'NONE',  ( 10.81492255796078972, 18.62759615963270932, 44.58224293864769550 ) ) ;
#67869=CARTESIAN_POINT ( 'NONE',  ( 13.89961937509957401, 13.97604488694547697, 26.87609039468566507 ) ) ;
#67871=CARTESIAN_POINT ( 'NONE',  ( 19.02544592524343514, -5.153800228976328945, 48.54057627198103120 ) ) ;
#67872=CARTESIAN_POINT ( 'NONE',  ( 16.52544592524335698, 4.483927247898782831, 31.45942372801901854 ) ) ;
#67873=CARTESIAN_POINT ( 'NONE',  ( -18.39639308325437739, -5.500000000000015099, 101.4825224618219863 ) ) ;
#67875=CARTESIAN_POINT ( 'NONE',  ( -16.53943276465976808, -0.05219959533934237506, 78.75109039468568994 ) ) ;
#67876=CARTESIAN_POINT ( 'NONE',  ( -0.05219959533907301413, -21.53943276465977519, 102.4989096053143811 ) ) ;
#67877=EDGE_CURVE ( 'NONE', #48812, #96464, #102423, .T. ) ;
#67878=CARTESIAN_POINT ( 'NONE',  ( 13.97604488694527802, 13.89961937509977652, 39.37390960531435269 ) ) ;
#67880=CARTESIAN_POINT ( 'NONE',  ( 10.72451020669871369, 18.67979575497193778, 37.08442372801901143 ) ) ;
#67881=CARTESIAN_POINT ( 'NONE',  ( 9.564922557961047289, -16.46253265017146816, 50.41775706135233293 ) ) ;
#67882=CARTESIAN_POINT ( 'NONE',  ( 5.153800228976335163, 19.02544592524342804, 44.79057627198103830 ) ) ;
#67883=CARTESIAN_POINT ( 'NONE',  ( 21.55341960407619695, -5.719274019375665929, 101.0427570613523756 ) ) ;
#67884=CARTESIAN_POINT ( 'NONE',  ( -13.97604488694527625, -13.89961937509977652, 21.87390960531435979 ) ) ;
#67885=CARTESIAN_POINT ( 'NONE',  ( -4.483927247898539470, -16.52544592524342804, 42.29057627198103120 ) ) ;
#67886=CARTESIAN_POINT ( 'NONE',  ( 19.35543954521082100, 5.499999999999578115, 42.08901960356453031 ) ) ;
#67887=CARTESIAN_POINT ( 'NONE',  ( -10.72451020669898014, 18.67979575497178502, 60.41557627198102409 ) ) ;
#67889=CARTESIAN_POINT ( 'NONE',  ( 13.97604488694527802, 13.89961937509977652, 109.3739096053143669 ) ) ;
#67890=CARTESIAN_POINT ( 'NONE',  ( 16.55341960407611168, 4.379528057220329451, 88.95724293864769550 ) ) ;
#67891=CARTESIAN_POINT ( 'NONE',  ( -14.34966873604972548, 8.224510206698743886, 28.33442372801902209 ) ) ;
#67892=CARTESIAN_POINT ( 'NONE',  ( -16.55341960407617563, 4.379528057220093196, 103.5427570613523613 ) ) ;
#67894=CARTESIAN_POINT ( 'NONE',  ( -5.049401038298153566, 19.05341960407611168, 100.2072429386476955 ) ) ;
#67895=CARTESIAN_POINT ( 'NONE',  ( 18.67979575497178502, 10.72451020669898547, 99.16557627198100988 ) ) ;
#67896=CARTESIAN_POINT ( 'NONE',  ( 12.06949235617757843, -12.14591786802309237, 28.12390960531435979 ) ) ;
#67897=CARTESIAN_POINT ( 'NONE',  ( -5.153800228976328057, -19.02544592524343514, 97.29057627198099567 ) ) ;
#67898=CARTESIAN_POINT ( 'NONE',  ( -16.51473224551082808, 9.474510206698731452, 93.33442372801900433 ) ) ;
#67899=CARTESIAN_POINT ( 'NONE',  ( 21.52544592524334988, 5.823673210054432836, 106.4594237280190328 ) ) ;
#67900=CARTESIAN_POINT ( 'NONE',  ( -10.72451020669898014, 18.67979575497178502, 85.41557627198102409 ) ) ;
#67901=CARTESIAN_POINT ( 'NONE',  ( 15.80617190586746368, 15.72974639402197994, 54.37390960531435979 ) ) ;
#67902=CARTESIAN_POINT ( 'NONE',  ( 5.049401038298161559, -19.05341960407611168, 57.70724293864769550 ) ) ;
#67903=CARTESIAN_POINT ( 'NONE',  ( -16.55341960407611168, -4.379528057220339221, 36.45724293864768839 ) ) ;
#67904=CARTESIAN_POINT ( 'NONE',  ( 0.05219959533909260263, 19.03943276465977164, 79.99890960531436690 ) ) ;
#67907=CARTESIAN_POINT ( 'NONE',  ( -16.51473224551082808, 9.474510206698731452, 43.33442372801900433 ) ) ;
#67908=CARTESIAN_POINT ( 'NONE',  ( -0.05219959533907301413, -21.53943276465977519, 77.49890960531433848 ) ) ;
#67909=CARTESIAN_POINT ( 'NONE',  ( 14.29746914071049879, -8.314922557960816363, 83.33224293864769550 ) ) ;
#67910=CARTESIAN_POINT ( 'NONE',  ( -18.67979575497193778, 10.72451020669871902, 23.33442372801901499 ) ) ;
#67912=CARTESIAN_POINT ( 'NONE',  ( 4.483927247898790824, -16.52544592524335698, 110.2094237280190185 ) ) ;
#67913=CARTESIAN_POINT ( 'NONE',  ( -5.049401038298153566, 19.05341960407611168, 25.20724293864768484 ) ) ;
#67914=CARTESIAN_POINT ( 'NONE',  ( -19.03943276465977164, 0.05219959533909376836, 71.24890960531435269 ) ) ;
#67917=CARTESIAN_POINT ( 'NONE',  ( 16.53943276465976808, -0.05219959533910856209, 48.74890960531435979 ) ) ;
#67918=CARTESIAN_POINT ( 'NONE',  ( 10.81492255796106328, -18.62759615963255655, 55.41775706135234714 ) ) ;
#67920=CARTESIAN_POINT ( 'NONE',  ( -5.153800228976328057, -19.02544592524343514, 37.29057627198102409 ) ) ;
#67921=CARTESIAN_POINT ( 'NONE',  ( 0.05219959533909260263, 19.03943276465977164, 54.99890960531435979 ) ) ;
#67923=CARTESIAN_POINT ( 'NONE',  ( -15.72974639402176322, -15.80617190586768395, 109.3760903946857042 ) ) ;
#67924=CARTESIAN_POINT ( 'NONE',  ( -16.53943276465976808, -0.05219959533934237506, 63.75109039468568284 ) ) ;
#67925=CARTESIAN_POINT ( 'NONE',  ( 21.52544592524334988, 5.823673210054432836, 86.45942372801901854 ) ) ;
#67926=CARTESIAN_POINT ( 'NONE',  ( -19.02544592524342804, 5.153800228976336051, 116.0405762719810383 ) ) ;
#67927=CARTESIAN_POINT ( 'NONE',  ( 0.05219959533936267826, -19.03943276465977164, 95.00109039468567573 ) ) ;
#67928=CARTESIAN_POINT ( 'NONE',  ( -21.53943276465977519, -0.05219959533937600094, 68.75109039468568994 ) ) ;
#67929=CARTESIAN_POINT ( 'NONE',  ( 16.52544592524335698, 4.483927247898782831, 41.45942372801901143 ) ) ;
#67930=CARTESIAN_POINT ( 'NONE',  ( 21.53943276465977519, -0.05219959533907433946, 88.74890960531436690 ) ) ;
#67931=CARTESIAN_POINT ( 'NONE',  ( 9.564922557961047289, -16.46253265017146816, 105.4177570613523471 ) ) ;
#67932=CARTESIAN_POINT ( 'NONE',  ( 16.51473224551069308, 9.474510206698969483, 59.16557627198102409 ) ) ;
#67933=CARTESIAN_POINT ( 'NONE',  ( 13.97604488694548053, -13.89961937509957401, 95.62609039468563310 ) ) ;
#67935=CARTESIAN_POINT ( 'NONE',  ( -9.564922557961040184, 16.46253265017147172, 97.91775706135233293 ) ) ;
#67936=CARTESIAN_POINT ( 'NONE',  ( -0.05219959533910754901, -16.53943276465976808, 52.49890960531435979 ) ) ;
#67937=CARTESIAN_POINT ( 'NONE',  ( -5.153800228976607833, 19.02544592524334988, 82.70942372801897591 ) ) ;
#67938=CARTESIAN_POINT ( 'NONE',  ( 16.53943276465976808, 0.05219959533934440121, 61.25109039468567573 ) ) ;
#67939=CARTESIAN_POINT ( 'NONE',  ( -21.52544592524334988, -5.823673210054445271, 18.95942372801901143 ) ) ;
#67940=CARTESIAN_POINT ( 'NONE',  ( 13.89961937509977652, -13.97604488694527269, 38.12390960531436690 ) ) ;
#67941=CARTESIAN_POINT ( 'NONE',  ( 9.564922557960805705, 16.46253265017160317, 49.58224293864770260 ) ) ;
#67942=CARTESIAN_POINT ( 'NONE',  ( -14.29746914071037622, -8.314922557961029526, 54.16775706135235424 ) ) ;
#67945=CARTESIAN_POINT ( 'NONE',  ( -5.049401038298153566, 19.05341960407611168, 100.2072429386476955 ) ) ;
#67947=CARTESIAN_POINT ( 'NONE',  ( -5.153800228976607833, 19.02544592524334988, 112.7094237280190043 ) ) ;
#67948=CARTESIAN_POINT ( 'NONE',  ( 5.823673210054125526, 21.52544592524343514, 34.79057627198103120 ) ) ;
#67949=CARTESIAN_POINT ( 'NONE',  ( 9.474510206698729675, 16.51473224551082808, 42.08442372801900433 ) ) ;
#67950=CARTESIAN_POINT ( 'NONE',  ( -8.224510206698735004, -14.34966873604973081, 34.58442372801900433 ) ) ;
#67951=CARTESIAN_POINT ( 'NONE',  ( 19.05341960407611168, 5.049401038298154454, 33.95724293864769550 ) ) ;
#67952=CARTESIAN_POINT ( 'NONE',  ( -13.97604488694527625, -13.89961937509977652, 51.87390960531436690 ) ) ;
#67953=CARTESIAN_POINT ( 'NONE',  ( 15.72974639402199770, -15.80617190586745480, 88.12390960531436690 ) ) ;
#67954=CARTESIAN_POINT ( 'NONE',  ( -5.153800228976328057, -19.02544592524343514, 97.29057627198099567 ) ) ;
#67955=CARTESIAN_POINT ( 'NONE',  ( -5.153800228976328057, -19.02544592524343514, 47.29057627198102409 ) ) ;
#67957=CARTESIAN_POINT ( 'NONE',  ( -16.46253265017146816, -9.564922557961047289, 84.16775706135233293 ) ) ;
#67958=CARTESIAN_POINT ( 'NONE',  ( -4.483927247898539470, -16.52544592524342804, 72.29057627198102409 ) ) ;
#67959=CARTESIAN_POINT ( 'NONE',  ( 18.67979575497194134, -10.72451020669871369, 100.8344237280190185 ) ) ;
#67960=CARTESIAN_POINT ( 'NONE',  ( 21.55341960407610458, 5.719274019375980345, 93.95724293864770971 ) ) ;
#67961=CARTESIAN_POINT ( 'NONE',  ( -5.823673210054431948, 21.52544592524334988, 82.70942372801900433 ) ) ;
#67963=CARTESIAN_POINT ( 'NONE',  ( 15.80617190586769283, -15.72974639402175789, 80.62609039468567573 ) ) ;
#67964=CARTESIAN_POINT ( 'NONE',  ( 13.89961937509977652, -13.97604488694527269, 103.1239096053143527 ) ) ;
#67965=CARTESIAN_POINT ( 'NONE',  ( 0.05219959533934541429, -16.53943276465976808, 110.0010903946856757 ) ) ;
#67966=CARTESIAN_POINT ( 'NONE',  ( 18.67979575497194134, -10.72451020669871369, 80.83442372801901854 ) ) ;
#67967=CARTESIAN_POINT ( 'NONE',  ( -19.03943276465977164, 0.05219959533909376836, 61.24890960531436690 ) ) ;
#67968=CARTESIAN_POINT ( 'NONE',  ( -21.55341960407619339, 5.719274019375674811, 43.54275706135235424 ) ) ;
#67969=CARTESIAN_POINT ( 'NONE',  ( -13.97604488694527625, -13.89961937509977652, 81.87390960531436690 ) ) ;
#67970=CARTESIAN_POINT ( 'NONE',  ( 4.379528057220339221, -16.55341960407611168, 82.70724293864770971 ) ) ;
#67971=CARTESIAN_POINT ( 'NONE',  ( 8.314922557960818139, 14.29746914071049879, 54.58224293864769550 ) ) ;
#67972=CARTESIAN_POINT ( 'NONE',  ( 10.81492255796078972, 18.62759615963270932, 54.58224293864769550 ) ) ;
#67973=CARTESIAN_POINT ( 'NONE',  ( 5.049401038298161559, -19.05341960407611168, 62.70724293864769550 ) ) ;
#67974=CARTESIAN_POINT ( 'NONE',  ( -0.05219959533907301413, -21.53943276465977519, 77.49890960531433848 ) ) ;
#67975=CARTESIAN_POINT ( 'NONE',  ( 19.05341960407617918, -5.049401038297876454, 71.04275706135234714 ) ) ;
#67976=CARTESIAN_POINT ( 'NONE',  ( 13.97604488694548053, -13.89961937509957401, 35.62609039468567573 ) ) ;
#67977=CARTESIAN_POINT ( 'NONE',  ( -0.05219959533910754901, -16.53943276465976808, 72.49890960531435269 ) ) ;
#67978=CARTESIAN_POINT ( 'NONE',  ( 21.53943276465977519, -0.05219959533907433946, 58.74890960531436690 ) ) ;
#67979=CARTESIAN_POINT ( 'NONE',  ( -17.49999999999999289, 5.500000000000032863, 70.79690382534172954 ) ) ;
#67980=CARTESIAN_POINT ( 'NONE',  ( 14.34966873604972726, -8.224510206698740333, 95.83442372801903275 ) ) ;
#67982=CARTESIAN_POINT ( 'NONE',  ( 0.05219959533936267826, -19.03943276465977164, 105.0010903946856615 ) ) ;
#67983=CARTESIAN_POINT ( 'NONE',  ( -16.55341960407611168, -4.379528057220339221, 71.45724293864769550 ) ) ;
#67984=CARTESIAN_POINT ( 'NONE',  ( -17.50000000000002132, 3.850315288878720654, 34.26629130603451046 ) ) ;
#67985=CARTESIAN_POINT ( 'NONE',  ( -0.05219959533909027116, -19.03943276465977164, 62.49890960531435979 ) ) ;
#67986=CARTESIAN_POINT ( 'NONE',  ( 8.224510206698953496, -14.34966873604960469, 47.91557627198102409 ) ) ;
#67987=CARTESIAN_POINT ( 'NONE',  ( -13.97604488694527625, -13.89961937509977652, 91.87390960531432427 ) ) ;
#67988=CARTESIAN_POINT ( 'NONE',  ( 13.89961937509957401, 13.97604488694547697, 76.87609039468566152 ) ) ;
#67989=CARTESIAN_POINT ( 'NONE',  ( -19.03943276465977164, 0.05219959533909376836, 61.24890960531436690 ) ) ;
#67990=CARTESIAN_POINT ( 'NONE',  ( 19.02544592524343514, -5.153800228976328945, 83.54057627198100988 ) ) ;
#67992=CARTESIAN_POINT ( 'NONE',  ( -0.05219959533909027116, -19.03943276465977164, 67.49890960531436690 ) ) ;
#67993=CARTESIAN_POINT ( 'NONE',  ( -21.53943276465977519, 0.05219959533907696930, 66.24890960531436690 ) ) ;
#67994=CARTESIAN_POINT ( 'NONE',  ( -14.29746914071037622, -8.314922557961029526, 54.16775706135235424 ) ) ;
#67995=CARTESIAN_POINT ( 'NONE',  ( -16.51473224551082808, 9.474510206698731452, 103.3344237280190043 ) ) ;
#67996=CARTESIAN_POINT ( 'NONE',  ( 5.153800228976335163, 19.02544592524342804, 44.79057627198103830 ) ) ;
#67997=CARTESIAN_POINT ( 'NONE',  ( -18.67979575497178146, -10.72451020669898902, 56.66557627198103830 ) ) ;
#67998=CARTESIAN_POINT ( 'NONE',  ( 19.03943276465977164, 0.05219959533936151252, 81.25109039468567573 ) ) ;
#67999=CARTESIAN_POINT ( 'NONE',  ( 8.224510206698953496, -14.34966873604960469, 22.91557627198102765 ) ) ;
#68001=CARTESIAN_POINT ( 'NONE',  ( 19.03943276465977164, 0.05219959533936151252, 41.25109039468566152 ) ) ;
#68002=CARTESIAN_POINT ( 'NONE',  ( 14.34966873604972726, -8.224510206698740333, 60.83442372801901854 ) ) ;
#68003=CARTESIAN_POINT ( 'NONE',  ( -12.06949235617739369, -12.14591786802326823, 99.37609039468568994 ) ) ;
#68004=CARTESIAN_POINT ( 'NONE',  ( -17.97182807773874558, 5.499999999999870326, 53.53038844047288336 ) ) ;
#68005=CARTESIAN_POINT ( 'NONE',  ( -12.06949235617739369, -12.14591786802326823, 79.37609039468567573 ) ) ;
#68006=CARTESIAN_POINT ( 'NONE',  ( 21.53943276465977519, -0.05219959533907433946, 23.74890960531435269 ) ) ;
#68007=CARTESIAN_POINT ( 'NONE',  ( -19.02544592524342804, 5.153800228976336051, 46.04057627198101699 ) ) ;
#68008=CARTESIAN_POINT ( 'NONE',  ( -16.51473224551069308, -9.474510206698971260, 46.66557627198102409 ) ) ;
#68009=CARTESIAN_POINT ( 'NONE',  ( -16.51473224551069308, -9.474510206698971260, 46.66557627198102409 ) ) ;
#68010=CARTESIAN_POINT ( 'NONE',  ( 10.81492255796106328, -18.62759615963255655, 40.41775706135234714 ) ) ;
#68011=CARTESIAN_POINT ( 'NONE',  ( -8.314922557961024197, 14.29746914071037800, 47.91775706135234714 ) ) ;
#68012=CARTESIAN_POINT ( 'NONE',  ( 14.29746914071037800, 8.314922557961029526, 111.6677570613523613 ) ) ;
#68013=CARTESIAN_POINT ( 'NONE',  ( -19.02544592524342804, 5.153800228976336051, 26.04057627198103120 ) ) ;
#68014=CARTESIAN_POINT ( 'NONE',  ( -13.89961937509957401, -13.97604488694547875, 19.37609039468566507 ) ) ;
#68015=CARTESIAN_POINT ( 'NONE',  ( 0.05219959533936267826, -19.03943276465977164, 110.0010903946856757 ) ) ;
#68016=CARTESIAN_POINT ( 'NONE',  ( 5.049401038297881783, 19.05341960407617563, 62.29275706135234003 ) ) ;
#68017=CARTESIAN_POINT ( 'NONE',  ( 16.53943276465976808, -0.05219959533910856209, 63.74890960531435979 ) ) ;
#68018=CARTESIAN_POINT ( 'NONE',  ( 16.46253265017160672, -9.564922557960803928, 38.33224293864768839 ) ) ;
#68019=CARTESIAN_POINT ( 'NONE',  ( -19.02544592524334988, -5.153800228976617603, 73.95942372801900433 ) ) ;
#68020=CARTESIAN_POINT ( 'NONE',  ( 17.31728774477273092, -6.344390552232384017, 93.31906651689317300 ) ) ;
#68021=CARTESIAN_POINT ( 'NONE',  ( -15.72974639402176322, -15.80617190586768395, 74.37609039468568994 ) ) ;
#68022=CARTESIAN_POINT ( 'NONE',  ( 8.224510206698742110, 14.34966873604972548, 37.08442372801901143 ) ) ;
#68024=CARTESIAN_POINT ( 'NONE',  ( 15.72974639402199770, -15.80617190586745480, 33.12390960531435979 ) ) ;
#68025=CARTESIAN_POINT ( 'NONE',  ( 14.34966873604972726, -8.224510206698740333, 25.83442372801901499 ) ) ;
#68026=CARTESIAN_POINT ( 'NONE',  ( -16.46253265017160317, 9.564922557960807481, 30.83224293864769550 ) ) ;
#68027=CARTESIAN_POINT ( 'NONE',  ( -19.02544592524334988, -5.153800228976617603, 18.95942372801899722 ) ) ;
#68028=DIRECTION ( 'NONE',  ( 1.000000000000000000, 0.000000000000000000, 0.000000000000000000 ) ) ;
#68029=CARTESIAN_POINT ( 'NONE',  ( 9.474510206698971260, -16.51473224551069308, 37.91557627198102409 ) ) ;
#68030=CARTESIAN_POINT ( 'NONE',  ( -13.97604488694547520, 13.89961937509957934, 58.12609039468566863 ) ) ;
#68031=CARTESIAN_POINT ( 'NONE',  ( -9.564922557960796823, -16.46253265017161027, 62.08224293864769550 ) ) ;
#68032=CARTESIAN_POINT ( 'NONE',  ( -15.72974639402176322, -15.80617190586768395, 64.37609039468568994 ) ) ;
#68033=CARTESIAN_POINT ( 'NONE',  ( 21.55341960407619695, -5.719274019375665929, 111.0427570613523613 ) ) ;
#68034=CARTESIAN_POINT ( 'NONE',  ( 8.224510206698953496, -14.34966873604960469, 27.91557627198103830 ) ) ;
#68035=CARTESIAN_POINT ( 'NONE',  ( 19.05341960407611168, 5.049401038298154454, 28.95724293864769550 ) ) ;
#68036=CARTESIAN_POINT ( 'NONE',  ( -16.51473224551069308, -9.474510206698971260, 96.66557627198102409 ) ) ;
#68037=CARTESIAN_POINT ( 'NONE',  ( -5.719274019375665041, -21.55341960407619695, 59.79275706135234714 ) ) ;
#68038=CARTESIAN_POINT ( 'NONE',  ( -19.02544592524342804, 5.153800228976336051, 36.04057627198100988 ) ) ;
#68039=CARTESIAN_POINT ( 'NONE',  ( 5.719274019375673035, 21.55341960407619339, 62.29275706135236845 ) ) ;
#68040=CARTESIAN_POINT ( 'NONE',  ( 0.05219959533936267826, -19.03943276465977164, 90.00109039468567573 ) ) ;
#68041=CARTESIAN_POINT ( 'NONE',  ( -9.564922557960796823, -16.46253265017161027, 107.0822429386476955 ) ) ;
#68042=CARTESIAN_POINT ( 'NONE',  ( -16.51473224551069308, -9.474510206698971260, 26.66557627198103120 ) ) ;
#68043=CARTESIAN_POINT ( 'NONE',  ( 10.72451020669898902, -18.67979575497178502, 112.9155762719810383 ) ) ;
#68044=CARTESIAN_POINT ( 'NONE',  ( 13.97604488694548053, -13.89961937509957401, 30.62609039468566863 ) ) ;
#68045=CARTESIAN_POINT ( 'NONE',  ( 14.29746914071049879, -8.314922557960816363, 113.3322429386476955 ) ) ;
#68046=CARTESIAN_POINT ( 'NONE',  ( 9.564922557960805705, 16.46253265017160317, 59.58224293864769550 ) ) ;
#68047=CARTESIAN_POINT ( 'NONE',  ( -19.05341960407617563, 5.049401038297882671, 98.54275706135233293 ) ) ;
#68048=CARTESIAN_POINT ( 'NONE',  ( 8.224510206698953496, -14.34966873604960469, 62.91557627198102409 ) ) ;
#68049=CARTESIAN_POINT ( 'NONE',  ( 5.823673210054125526, 21.52544592524343514, 24.79057627198103120 ) ) ;
#68050=CARTESIAN_POINT ( 'NONE',  ( -19.05341960407617563, 5.049401038297882671, 88.54275706135230450 ) ) ;
#68051=CARTESIAN_POINT ( 'NONE',  ( -15.72974639402197994, 15.80617190586746368, 85.62390960531436690 ) ) ;
#68052=CARTESIAN_POINT ( 'NONE',  ( -0.05219959533937732626, 21.53943276465977519, 47.50109039468568994 ) ) ;
#68053=CARTESIAN_POINT ( 'NONE',  ( -14.34966873604972548, 8.224510206698743886, 38.33442372801900433 ) ) ;
#68054=CARTESIAN_POINT ( 'NONE',  ( -16.55341960407617563, 4.379528057220093196, 38.54275706135234714 ) ) ;
#68055=CARTESIAN_POINT ( 'NONE',  ( -21.52544592524334988, -5.823673210054445271, 53.95942372801900433 ) ) ;
#68056=CARTESIAN_POINT ( 'NONE',  ( -21.52544592524343514, 5.823673210054127303, 61.04057627198103120 ) ) ;
#68057=CARTESIAN_POINT ( 'NONE',  ( 19.05341960407611168, 5.049401038298154454, 33.95724293864769550 ) ) ;
#68059=CARTESIAN_POINT ( 'NONE',  ( -4.379528057220086978, -16.55341960407618274, 69.79275706135234714 ) ) ;
#68060=CARTESIAN_POINT ( 'NONE',  ( 21.53943276465977519, -0.05219959533907433946, 103.7489096053143669 ) ) ;
#68061=CARTESIAN_POINT ( 'NONE',  ( -12.14591786802309592, -12.06949235617757132, 41.87390960531435979 ) ) ;
#68062=CARTESIAN_POINT ( 'NONE',  ( -4.483927247898782831, 16.52544592524335698, 62.70942372801902565 ) ) ;
#68063=CARTESIAN_POINT ( 'NONE',  ( 9.564922557961047289, -16.46253265017146816, 100.4177570613523329 ) ) ;
#68064=CARTESIAN_POINT ( 'NONE',  ( 15.72974639402199770, -15.80617190586745480, 98.12390960531436690 ) ) ;
#68065=CARTESIAN_POINT ( 'NONE',  ( -8.314922557960811034, -14.29746914071050412, 27.08224293864769550 ) ) ;
#68067=CARTESIAN_POINT ( 'NONE',  ( -16.52544592524335698, -4.483927247898792601, 78.95942372801901854 ) ) ;
#68069=CARTESIAN_POINT ( 'NONE',  ( 10.81492255796078972, 18.62759615963270932, 74.58224293864768129 ) ) ;
#68070=CARTESIAN_POINT ( 'NONE',  ( 4.483927247898790824, -16.52544592524335698, 110.2094237280190185 ) ) ;
#68073=CARTESIAN_POINT ( 'NONE',  ( -5.823673210054116645, -21.52544592524344225, 102.2905762719810383 ) ) ;
#68074=CARTESIAN_POINT ( 'NONE',  ( -21.53943276465977519, 0.05219959533907696930, 106.2489096053143811 ) ) ;
#68075=CARTESIAN_POINT ( 'NONE',  ( -16.55341960407611168, -4.379528057220339221, 36.45724293864768839 ) ) ;
#68076=CARTESIAN_POINT ( 'NONE',  ( 12.06949235617739724, 12.14591786802326823, 41.87609039468568284 ) ) ;
#68077=CARTESIAN_POINT ( 'NONE',  ( 19.02544592524343514, -5.153800228976328945, 43.54057627198103120 ) ) ;
#68078=CARTESIAN_POINT ( 'NONE',  ( -9.564922557960796823, -16.46253265017161027, 62.08224293864769550 ) ) ;
#68081=CARTESIAN_POINT ( 'NONE',  ( -13.89961937509977652, 13.97604488694528158, 110.6239096053143243 ) ) ;
#68083=CARTESIAN_POINT ( 'NONE',  ( 0.05219959533936267826, -19.03943276465977164, 105.0010903946856615 ) ) ;
#68084=CARTESIAN_POINT ( 'NONE',  ( 13.89961937509957401, 13.97604488694547697, 46.87609039468565442 ) ) ;
#68085=CARTESIAN_POINT ( 'NONE',  ( 15.72974639402199770, -15.80617190586745480, 83.12390960531436690 ) ) ;
#68086=CARTESIAN_POINT ( 'NONE',  ( -0.05219959533934338120, 16.53943276465976808, 112.5010903946857042 ) ) ;
#68087=CARTESIAN_POINT ( 'NONE',  ( -10.81492255796078084, -18.62759615963271287, 47.08224293864770260 ) ) ;
#68088=CARTESIAN_POINT ( 'NONE',  ( 5.719274019375991003, -21.55341960407610458, 82.70724293864770971 ) ) ;
#68089=CARTESIAN_POINT ( 'NONE',  ( 9.564922557961047289, -16.46253265017146816, 110.4177570613523471 ) ) ;
#68090=CARTESIAN_POINT ( 'NONE',  ( 15.80617190586746368, 15.72974639402197994, 24.37390960531435979 ) ) ;
#68091=CARTESIAN_POINT ( 'NONE',  ( 18.62759615963255655, 10.81492255796105972, 76.66775706135234714 ) ) ;
#68092=CARTESIAN_POINT ( 'NONE',  ( 19.03943276465977164, -0.05219959533909143690, 73.74890960531435269 ) ) ;
#68095=CARTESIAN_POINT ( 'NONE',  ( -13.97604488694527625, -13.89961937509977652, 76.87390960531433848 ) ) ;
#68096=CARTESIAN_POINT ( 'NONE',  ( -8.314922557960811034, -14.29746914071050412, 87.08224293864769550 ) ) ;
#68098=CARTESIAN_POINT ( 'NONE',  ( 19.05341960407617918, -5.049401038297876454, 111.0427570613523329 ) ) ;
#68099=CARTESIAN_POINT ( 'NONE',  ( 17.50000000000000355, -5.624438216177593652, 83.31670344914645909 ) ) ;
#68100=CARTESIAN_POINT ( 'NONE',  ( -13.97604488694527625, -13.89961937509977652, 76.87390960531433848 ) ) ;
#68101=CARTESIAN_POINT ( 'NONE',  ( -15.72974639402176322, -15.80617190586768395, 79.37609039468567573 ) ) ;
#68102=CARTESIAN_POINT ( 'NONE',  ( -19.02544592524342804, 5.153800228976336051, 96.04057627198103830 ) ) ;
#68103=CARTESIAN_POINT ( 'NONE',  ( -8.224510206698735004, -14.34966873604973081, 74.58442372801901854 ) ) ;
#68104=CARTESIAN_POINT ( 'NONE',  ( -17.26058549869093284, -6.457015423128470211, 76.37745837476069255 ) ) ;
#68105=CARTESIAN_POINT ( 'NONE',  ( 19.02544592524334988, 5.153800228976608722, 61.45942372801900433 ) ) ;
#68106=CARTESIAN_POINT ( 'NONE',  ( 13.89961937509957401, 13.97604488694547697, 21.87609039468566152 ) ) ;
#68110=CARTESIAN_POINT ( 'NONE',  ( -14.34966873604960291, -8.224510206698953496, 26.66557627198103475 ) ) ;
#68112=CARTESIAN_POINT ( 'NONE',  ( 14.29746914071037800, 8.314922557961029526, 101.6677570613523613 ) ) ;
#68113=CARTESIAN_POINT ( 'NONE',  ( 16.19135201231365784, 7.376712067591955524, 67.68680854052030327 ) ) ;
#68114=CARTESIAN_POINT ( 'NONE',  ( 4.483927247898790824, -16.52544592524335698, 80.20942372801901854 ) ) ;
#68115=CARTESIAN_POINT ( 'NONE',  ( 10.81492255796106328, -18.62759615963255655, 85.41775706135236135 ) ) ;
#68116=CARTESIAN_POINT ( 'NONE',  ( -5.049401038297874678, -19.05341960407617918, 94.79275706135230450 ) ) ;
#68117=CARTESIAN_POINT ( 'NONE',  ( -5.153800228976607833, 19.02544592524334988, 42.70942372801901143 ) ) ;
#68118=CARTESIAN_POINT ( 'NONE',  ( 16.51473224551069308, 9.474510206698969483, 74.16557627198103830 ) ) ;
#68119=CARTESIAN_POINT ( 'NONE',  ( -19.05341960407611168, -5.049401038298163336, 51.45724293864770260 ) ) ;
#68120=CARTESIAN_POINT ( 'NONE',  ( 18.22780087662123805, -5.499999999999976019, 88.51763182126893525 ) ) ;
#68121=CARTESIAN_POINT ( 'NONE',  ( -15.72974639402197994, 15.80617190586746368, 95.62390960531436690 ) ) ;
#68122=CARTESIAN_POINT ( 'NONE',  ( 10.81492255796078972, 18.62759615963270932, 44.58224293864769550 ) ) ;
#68123=CARTESIAN_POINT ( 'NONE',  ( 5.049401038298161559, -19.05341960407611168, 42.70724293864767418 ) ) ;
#68124=CARTESIAN_POINT ( 'NONE',  ( -8.314922557961024197, 14.29746914071037800, 57.91775706135234714 ) ) ;
#68126=VERTEX_POINT ( 'NONE', #8937 ) ;
#68127=CARTESIAN_POINT ( 'NONE',  ( -21.53943276465977519, -0.05219959533937600094, 48.75109039468568284 ) ) ;
#68128=CARTESIAN_POINT ( 'NONE',  ( 0.05219959533910956823, 16.53943276465976808, 64.99890960531435269 ) ) ;
#68130=CARTESIAN_POINT ( 'NONE',  ( -14.34966873604972548, 8.224510206698743886, 43.33442372801901143 ) ) ;
#68131=CARTESIAN_POINT ( 'NONE',  ( -12.06949235617756955, 12.14591786802309770, 105.6239096053143669 ) ) ;
#68132=CARTESIAN_POINT ( 'NONE',  ( -9.564922557961040184, 16.46253265017147172, 57.91775706135233293 ) ) ;
#68133=CARTESIAN_POINT ( 'NONE',  ( 14.34966873604960469, 8.224510206698951720, 69.16557627198102409 ) ) ;
#68134=CARTESIAN_POINT ( 'NONE',  ( -0.05219959533937732626, 21.53943276465977519, 32.50109039468568284 ) ) ;
#68136=CARTESIAN_POINT ( 'NONE',  ( 15.80617190586746368, 15.72974639402197994, 94.37390960531436690 ) ) ;
#68137=CARTESIAN_POINT ( 'NONE',  ( -5.153800228976328057, -19.02544592524343514, 107.2905762719810383 ) ) ;
#68138=CARTESIAN_POINT ( 'NONE',  ( 12.06949235617757843, -12.14591786802309237, 68.12390960531436690 ) ) ;
#68139=CARTESIAN_POINT ( 'NONE',  ( 13.97604488694527802, 13.89961937509977652, 114.3739096053143669 ) ) ;
#68141=CARTESIAN_POINT ( 'NONE',  ( 9.474510206698729675, 16.51473224551082808, 77.08442372801900433 ) ) ;
#68142=CARTESIAN_POINT ( 'NONE',  ( -15.72974639402176322, -15.80617190586768395, 29.37609039468568284 ) ) ;
#68143=CARTESIAN_POINT ( 'NONE',  ( 9.474510206698971260, -16.51473224551069308, 72.91557627198102409 ) ) ;
#68144=CARTESIAN_POINT ( 'NONE',  ( -5.153800228976607833, 19.02544592524334988, 57.70942372801899012 ) ) ;
#68145=CARTESIAN_POINT ( 'NONE',  ( 16.51473224551069308, 9.474510206698969483, 29.16557627198103475 ) ) ;
#68146=CARTESIAN_POINT ( 'NONE',  ( 21.55341960407619695, -5.719274019375665929, 76.04275706135237556 ) ) ;
#68147=CARTESIAN_POINT ( 'NONE',  ( 16.53943276465976808, -0.05219959533910856209, 63.74890960531435979 ) ) ;
#68148=CARTESIAN_POINT ( 'NONE',  ( -4.379528057220328563, 16.55341960407611168, 60.20724293864768839 ) ) ;
#68149=CARTESIAN_POINT ( 'NONE',  ( -16.46253265017160317, 9.564922557960807481, 65.83224293864769550 ) ) ;
#68150=CARTESIAN_POINT ( 'NONE',  ( -21.55341960407610458, -5.719274019375992779, 91.45724293864769550 ) ) ;
#68151=CARTESIAN_POINT ( 'NONE',  ( 9.474510206698971260, -16.51473224551069308, 62.91557627198102409 ) ) ;
#68152=CARTESIAN_POINT ( 'NONE',  ( -18.67979575497178146, -10.72451020669898902, 76.66557627198103830 ) ) ;
#68153=CARTESIAN_POINT ( 'NONE',  ( 0.05219959533937995610, -21.53943276465977519, 100.0010903946857042 ) ) ;
#68154=DIRECTION ( 'NONE',  ( 0.000000000000000000, 0.000000000000000000, -1.000000000000000000 ) ) ;
#68155=CARTESIAN_POINT ( 'NONE',  ( -16.52544592524335698, -4.483927247898792601, 108.9594237280190185 ) ) ;
#68156=CARTESIAN_POINT ( 'NONE',  ( -16.53943276465976808, 0.05219959533911058130, 101.2489096053143669 ) ) ;
#68157=CARTESIAN_POINT ( 'NONE',  ( -19.05341960407617563, 5.049401038297882671, 98.54275706135233293 ) ) ;
#68158=VERTEX_POINT ( 'NONE', #163617 ) ;
#68159=CARTESIAN_POINT ( 'NONE',  ( 0.05219959533907565091, 21.53943276465977519, 114.9989096053143669 ) ) ;
#68160=CARTESIAN_POINT ( 'NONE',  ( -9.564922557961040184, 16.46253265017147172, 57.91775706135233293 ) ) ;
#68161=CARTESIAN_POINT ( 'NONE',  ( -8.314922557961024197, 14.29746914071037800, 97.91775706135236135 ) ) ;
#68162=CARTESIAN_POINT ( 'NONE',  ( 19.03943276465977164, 0.05219959533936151252, 36.25109039468567573 ) ) ;
#68163=CARTESIAN_POINT ( 'NONE',  ( -5.049401038298153566, 19.05341960407611168, 105.2072429386476671 ) ) ;
#68164=CARTESIAN_POINT ( 'NONE',  ( -18.62759615963270932, 10.81492255796079327, 65.83224293864769550 ) ) ;
#68166=CARTESIAN_POINT ( 'NONE',  ( -5.049401038298153566, 19.05341960407611168, 30.20724293864768839 ) ) ;
#68167=CARTESIAN_POINT ( 'NONE',  ( -19.03943276465977164, -0.05219959533935918106, 18.75109039468567218 ) ) ;
#68168=CARTESIAN_POINT ( 'NONE',  ( 8.314922557961029526, -14.29746914071037800, 70.41775706135236135 ) ) ;
#68169=CARTESIAN_POINT ( 'NONE',  ( 0.05219959533937995610, -21.53943276465977519, 25.00109039468567218 ) ) ;
#68170=CARTESIAN_POINT ( 'NONE',  ( -0.05219959533934338120, 16.53943276465976808, 42.50109039468567573 ) ) ;
#68171=CARTESIAN_POINT ( 'NONE',  ( -19.05341960407611168, -5.049401038298163336, 106.4572429386476955 ) ) ;
#68172=CARTESIAN_POINT ( 'NONE',  ( -19.02544592524342804, 5.153800228976336051, 51.04057627198103120 ) ) ;
#68173=CARTESIAN_POINT ( 'NONE',  ( 9.474510206698971260, -16.51473224551069308, 62.91557627198102409 ) ) ;
#68174=CARTESIAN_POINT ( 'NONE',  ( 4.379528057220092307, 16.55341960407617563, 52.29275706135236135 ) ) ;
#68175=CARTESIAN_POINT ( 'NONE',  ( 16.52544592524342804, -4.483927247898539470, 93.54057627198103830 ) ) ;
#68176=CARTESIAN_POINT ( 'NONE',  ( 16.55341960407618274, -4.379528057220086978, 106.0427570613523471 ) ) ;
#68178=CARTESIAN_POINT ( 'NONE',  ( -21.53943276465977519, -0.05219959533937600094, 53.75109039468568994 ) ) ;
#68179=CARTESIAN_POINT ( 'NONE',  ( -9.564922557960796823, -16.46253265017161027, 77.08224293864769550 ) ) ;
#68180=CARTESIAN_POINT ( 'NONE',  ( -0.05219959533909027116, -19.03943276465977164, 62.49890960531435979 ) ) ;
#68181=CARTESIAN_POINT ( 'NONE',  ( -16.46253265017160317, 9.564922557960807481, 90.83224293864769550 ) ) ;
#68182=CARTESIAN_POINT ( 'NONE',  ( 12.06949235617757843, -12.14591786802309237, 48.12390960531436690 ) ) ;
#68183=CARTESIAN_POINT ( 'NONE',  ( 16.52544592524335698, 4.483927247898782831, 96.45942372801901854 ) ) ;
#68184=CARTESIAN_POINT ( 'NONE',  ( 8.314922557960818139, 14.29746914071049879, 39.58224293864769550 ) ) ;
#68185=ORIENTED_EDGE ( 'NONE', *, *, #141668, .F. ) ;
#68186=CARTESIAN_POINT ( 'NONE',  ( -5.153800228976607833, 19.02544592524334988, 37.70942372801899722 ) ) ;
#68187=CARTESIAN_POINT ( 'NONE',  ( 16.51473224551069308, 9.474510206698969483, 114.1655762719810241 ) ) ;
#68188=CARTESIAN_POINT ( 'NONE',  ( -0.05219959533909027116, -19.03943276465977164, 62.49890960531435979 ) ) ;
#68189=CARTESIAN_POINT ( 'NONE',  ( -9.564922557961040184, 16.46253265017147172, 37.91775706135233293 ) ) ;
#68191=CARTESIAN_POINT ( 'NONE',  ( 17.97214573761830536, 5.500000000000079048, 58.96970049038655759 ) ) ;
#68192=CARTESIAN_POINT ( 'NONE',  ( 19.05341960407617918, -5.049401038297876454, 81.04275706135231871 ) ) ;
#68193=CARTESIAN_POINT ( 'NONE',  ( -8.314922557961024197, 14.29746914071037800, 67.91775706135234714 ) ) ;
#68194=DIRECTION ( 'NONE',  ( 0.000000000000000000, -0.04175967627138118393, -0.9991276842514721368 ) ) ;
#68195=CARTESIAN_POINT ( 'NONE',  ( -19.03943276465977164, 0.05219959533909376836, 86.24890960531436690 ) ) ;
#68196=CARTESIAN_POINT ( 'NONE',  ( 5.719274019375673035, 21.55341960407619339, 32.29275706135235424 ) ) ;
#68197=CARTESIAN_POINT ( 'NONE',  ( -19.02544592524334988, -5.153800228976617603, 73.95942372801900433 ) ) ;
#68199=CARTESIAN_POINT ( 'NONE',  ( -19.03943276465977164, 0.05219959533909376836, 46.24890960531435979 ) ) ;
#68200=CARTESIAN_POINT ( 'NONE',  ( -5.153800228976328057, -19.02544592524343514, 92.29057627198099567 ) ) ;
#68201=CARTESIAN_POINT ( 'NONE',  ( 16.53943276465976808, -0.05219959533910856209, 48.74890960531435979 ) ) ;
#68202=CARTESIAN_POINT ( 'NONE',  ( 19.05341960407611168, 5.049401038298154454, 33.95724293864769550 ) ) ;
#68203=CARTESIAN_POINT ( 'NONE',  ( 16.46253265017146816, 9.564922557961045513, 46.66775706135233293 ) ) ;
#68204=CARTESIAN_POINT ( 'NONE',  ( 14.34966873604960469, 8.224510206698951720, 89.16557627198102409 ) ) ;
#68205=CARTESIAN_POINT ( 'NONE',  ( -16.46253265017146816, -9.564922557961047289, 29.16775706135232937 ) ) ;
#68206=CARTESIAN_POINT ( 'NONE',  ( -19.03943276465977164, 0.05219959533909376836, 71.24890960531435269 ) ) ;
#68208=CARTESIAN_POINT ( 'NONE',  ( 21.55341960407610458, 5.719274019375980345, 63.95724293864770260 ) ) ;
#68209=CARTESIAN_POINT ( 'NONE',  ( -0.05219959533910754901, -16.53943276465976808, 57.49890960531435979 ) ) ;
#68210=CARTESIAN_POINT ( 'NONE',  ( -5.153800228976607833, 19.02544592524334988, 27.70942372801899722 ) ) ;
#68211=CARTESIAN_POINT ( 'NONE',  ( 9.474510206698971260, -16.51473224551069308, 112.9155762719810383 ) ) ;
#68212=CARTESIAN_POINT ( 'NONE',  ( 5.823673210054125526, 21.52544592524343514, 24.79057627198103120 ) ) ;
#68213=CARTESIAN_POINT ( 'NONE',  ( -16.51473224551069308, -9.474510206698971260, 46.66557627198102409 ) ) ;
#68214=CARTESIAN_POINT ( 'NONE',  ( 19.03943276465977164, -0.05219959533909143690, 43.74890960531435979 ) ) ;
#68215=CARTESIAN_POINT ( 'NONE',  ( 16.55341960407611168, 4.379528057220329451, 103.9572429386476813 ) ) ;
#68216=CARTESIAN_POINT ( 'NONE',  ( 18.67979575497178502, 10.72451020669898547, 109.1655762719810383 ) ) ;
#68217=CARTESIAN_POINT ( 'NONE',  ( 0.05219959533909260263, 19.03943276465977164, 94.99890960531436690 ) ) ;
#68218=CARTESIAN_POINT ( 'NONE',  ( 5.823673210054444382, -21.52544592524334988, 20.20942372801900788 ) ) ;
#68219=CARTESIAN_POINT ( 'NONE',  ( -13.97604488694527625, -13.89961937509977652, 101.8739096053143811 ) ) ;
#68220=CARTESIAN_POINT ( 'NONE',  ( 8.224510206698953496, -14.34966873604960469, 112.9155762719810383 ) ) ;
#68221=CARTESIAN_POINT ( 'NONE',  ( -5.823673210054431948, 21.52544592524334988, 82.70942372801900433 ) ) ;
#68222=CARTESIAN_POINT ( 'NONE',  ( 21.53943276465977519, -0.05219959533907433946, 93.74890960531436690 ) ) ;
#68223=CARTESIAN_POINT ( 'NONE',  ( 16.52216118717207749, -7.221426719304518294, 106.4240097895300892 ) ) ;
#68224=CARTESIAN_POINT ( 'NONE',  ( 9.564922557960805705, 16.46253265017160317, 59.58224293864769550 ) ) ;
#68225=CARTESIAN_POINT ( 'NONE',  ( -12.06949235617739369, -12.14591786802326823, 44.37609039468567573 ) ) ;
#68226=CARTESIAN_POINT ( 'NONE',  ( 8.224510206698953496, -14.34966873604960469, 107.9155762719810241 ) ) ;
#68227=CARTESIAN_POINT ( 'NONE',  ( -17.50000000000001066, -3.237210098469584185, 110.2876301262045615 ) ) ;
#68228=CARTESIAN_POINT ( 'NONE',  ( 9.474510206698971260, -16.51473224551069308, 52.91557627198102409 ) ) ;
#68229=CARTESIAN_POINT ( 'NONE',  ( 4.483927247898545687, 16.52544592524342804, 99.79057627198103830 ) ) ;
#68230=CARTESIAN_POINT ( 'NONE',  ( -0.05219959533907301413, -21.53943276465977519, 47.49890960531435979 ) ) ;
#68231=CARTESIAN_POINT ( 'NONE',  ( 12.14591786802309770, 12.06949235617756955, 64.37390960531435269 ) ) ;
#68232=CARTESIAN_POINT ( 'NONE',  ( -12.06949235617739369, -12.14591786802326823, 24.37609039468567573 ) ) ;
#68233=CARTESIAN_POINT ( 'NONE',  ( -15.80617190586768217, 15.72974639402176855, 68.12609039468567573 ) ) ;
#68234=CARTESIAN_POINT ( 'NONE',  ( 16.46253265017146816, 9.564922557961045513, 61.66775706135234003 ) ) ;
#68235=CARTESIAN_POINT ( 'NONE',  ( 16.55341960407618274, -4.379528057220086978, 101.0427570613523756 ) ) ;
#68236=CARTESIAN_POINT ( 'NONE',  ( 0.05219959533910956823, 16.53943276465976808, 44.99890960531435979 ) ) ;
#68237=CARTESIAN_POINT ( 'NONE',  ( 5.049401038298161559, -19.05341960407611168, 37.70724293864768839 ) ) ;
#68238=CARTESIAN_POINT ( 'NONE',  ( -19.05341960407611168, -5.049401038298163336, 91.45724293864766707 ) ) ;
#68239=CARTESIAN_POINT ( 'NONE',  ( 21.52544592524344225, -5.823673210054117533, 98.54057627198105251 ) ) ;
#68240=CARTESIAN_POINT ( 'NONE',  ( 4.483927247898790824, -16.52544592524335698, 30.20942372801902565 ) ) ;
#68241=CARTESIAN_POINT ( 'NONE',  ( -12.14591786802309592, -12.06949235617757132, 61.87390960531436690 ) ) ;
#68242=CARTESIAN_POINT ( 'NONE',  ( 18.67979575497194134, -10.72451020669871369, 75.83442372801900433 ) ) ;
#68245=CARTESIAN_POINT ( 'NONE',  ( -16.55341960407617563, 4.379528057220093196, 93.54275706135234714 ) ) ;
#68248=CARTESIAN_POINT ( 'NONE',  ( -4.483927247898539470, -16.52544592524342804, 22.29057627198102765 ) ) ;
#68249=CARTESIAN_POINT ( 'NONE',  ( 14.29746914071037800, 8.314922557961029526, 71.66775706135234714 ) ) ;
#68250=CARTESIAN_POINT ( 'NONE',  ( -16.46253265017160317, 9.564922557960807481, 85.83224293864769550 ) ) ;
#68251=CARTESIAN_POINT ( 'NONE',  ( -5.049401038298153566, 19.05341960407611168, 105.2072429386476671 ) ) ;
#68252=CARTESIAN_POINT ( 'NONE',  ( -18.67979575497193778, 10.72451020669871902, 83.33442372801903275 ) ) ;
#68253=CARTESIAN_POINT ( 'NONE',  ( -16.55341960407617563, 4.379528057220093196, 93.54275706135234714 ) ) ;
#68254=CARTESIAN_POINT ( 'NONE',  ( -14.34966873604960291, -8.224510206698953496, 56.66557627198103830 ) ) ;
#68255=CARTESIAN_POINT ( 'NONE',  ( -13.97604488694527625, -13.89961937509977652, 71.87390960531433848 ) ) ;
#68256=ORIENTED_EDGE ( 'NONE', *, *, #42127, .F. ) ;
#68257=CARTESIAN_POINT ( 'NONE',  ( -16.51473224551082808, 9.474510206698731452, 113.3344237280190043 ) ) ;
#68258=CARTESIAN_POINT ( 'NONE',  ( -12.14591786802309592, -12.06949235617757132, 106.8739096053143811 ) ) ;
#68259=CARTESIAN_POINT ( 'NONE',  ( 13.89961937509977652, -13.97604488694527269, 73.12390960531436690 ) ) ;
#68260=CARTESIAN_POINT ( 'NONE',  ( 8.314922557961029526, -14.29746914071037800, 25.41775706135235779 ) ) ;
#68262=CARTESIAN_POINT ( 'NONE',  ( -13.89961937509957401, -13.97604488694547875, 19.37609039468566507 ) ) ;
#68263=CARTESIAN_POINT ( 'NONE',  ( 12.06949235617739724, 12.14591786802326823, 76.87609039468567573 ) ) ;
#68264=CARTESIAN_POINT ( 'NONE',  ( 0.05219959533936267826, -19.03943276465977164, 95.00109039468567573 ) ) ;
#68265=CARTESIAN_POINT ( 'NONE',  ( 9.564922557960805705, 16.46253265017160317, 24.58224293864769194 ) ) ;
#68266=CARTESIAN_POINT ( 'NONE',  ( 8.224510206698742110, 14.34966873604972548, 67.08442372801901854 ) ) ;
#68267=CARTESIAN_POINT ( 'NONE',  ( -16.55341960407617563, 4.379528057220093196, 58.54275706135235424 ) ) ;
#68268=CARTESIAN_POINT ( 'NONE',  ( -13.97604488694527625, -13.89961937509977652, 26.87390960531434558 ) ) ;
#68269=CARTESIAN_POINT ( 'NONE',  ( 19.03943276465977164, 0.05219959533936151252, 51.25109039468567573 ) ) ;
#68270=CARTESIAN_POINT ( 'NONE',  ( 5.719274019375673035, 21.55341960407619339, 92.29275706135236135 ) ) ;
#68271=CARTESIAN_POINT ( 'NONE',  ( 9.564922557960805705, 16.46253265017160317, 29.58224293864769550 ) ) ;
#68272=CARTESIAN_POINT ( 'NONE',  ( 19.02544592524343514, -5.153800228976328945, 73.54057627198103830 ) ) ;
#68273=CARTESIAN_POINT ( 'NONE',  ( 12.06949235617757843, -12.14591786802309237, 73.12390960531436690 ) ) ;
#68274=CARTESIAN_POINT ( 'NONE',  ( -18.62759615963255300, -10.81492255796106328, 89.16775706135236135 ) ) ;
#68276=CARTESIAN_POINT ( 'NONE',  ( -13.89961937509957401, -13.97604488694547875, 64.37609039468567573 ) ) ;
#68277=CARTESIAN_POINT ( 'NONE',  ( -5.153800228976607833, 19.02544592524334988, 42.70942372801901143 ) ) ;
#68278=CARTESIAN_POINT ( 'NONE',  ( 21.52544592524344225, -5.823673210054117533, 38.54057627198103120 ) ) ;
#68279=CARTESIAN_POINT ( 'NONE',  ( 18.67979575497194134, -10.72451020669871369, 105.8344237280190328 ) ) ;
#68280=CARTESIAN_POINT ( 'NONE',  ( -0.05219959533909027116, -19.03943276465977164, 77.49890960531435269 ) ) ;
#68281=CARTESIAN_POINT ( 'NONE',  ( -18.67979575497193778, 10.72451020669871902, 103.3344237280190043 ) ) ;
#68282=CARTESIAN_POINT ( 'NONE',  ( 0.05219959533907565091, 21.53943276465977519, 44.99890960531435979 ) ) ;
#68283=CARTESIAN_POINT ( 'NONE',  ( 5.153800228976335163, 19.02544592524342804, 99.79057627198102409 ) ) ;
#68284=CARTESIAN_POINT ( 'NONE',  ( 5.049401038297881783, 19.05341960407617563, 77.29275706135231871 ) ) ;
#68285=CARTESIAN_POINT ( 'NONE',  ( -9.564922557960796823, -16.46253265017161027, 107.0822429386476955 ) ) ;
#68286=CARTESIAN_POINT ( 'NONE',  ( -5.153800228976607833, 19.02544592524334988, 92.70942372801901854 ) ) ;
#68287=CARTESIAN_POINT ( 'NONE',  ( 16.52544592524335698, 4.483927247898782831, 41.45942372801901143 ) ) ;
#68288=CARTESIAN_POINT ( 'NONE',  ( -12.14591786802309592, -12.06949235617757132, 96.87390960531436690 ) ) ;
#68289=CARTESIAN_POINT ( 'NONE',  ( 16.51473224551069308, 9.474510206698969483, 89.16557627198103830 ) ) ;
#68290=CARTESIAN_POINT ( 'NONE',  ( -21.53943276465977519, 0.05219959533907696930, 66.24890960531436690 ) ) ;
#68291=CARTESIAN_POINT ( 'NONE',  ( -0.05219959533934338120, 16.53943276465976808, 32.50109039468568284 ) ) ;
#68292=CARTESIAN_POINT ( 'NONE',  ( -5.823673210054431948, 21.52544592524334988, 27.70942372801901854 ) ) ;
#68293=CARTESIAN_POINT ( 'NONE',  ( -15.80617190586768217, 15.72974639402176855, 83.12609039468568994 ) ) ;
#68294=CARTESIAN_POINT ( 'NONE',  ( -4.483927247898782831, 16.52544592524335698, 87.70942372801901854 ) ) ;
#68295=CARTESIAN_POINT ( 'NONE',  ( 19.03943276465977164, -0.05219959533909143690, 78.74890960531436690 ) ) ;
#68296=CARTESIAN_POINT ( 'NONE',  ( -14.29746914071049879, 8.314922557960819915, 80.83224293864769550 ) ) ;
#68297=CARTESIAN_POINT ( 'NONE',  ( -16.53943276465976808, -0.05219959533934237506, 113.7510903946856757 ) ) ;
#68298=CARTESIAN_POINT ( 'NONE',  ( -19.05341960407617563, 5.049401038297882671, 58.54275706135234003 ) ) ;
#68299=CARTESIAN_POINT ( 'NONE',  ( -18.62759615963255300, -10.81492255796106328, 39.16775706135235424 ) ) ;
#68300=CARTESIAN_POINT ( 'NONE',  ( 12.06949235617757843, -12.14591786802309237, 78.12390960531436690 ) ) ;
#68301=CARTESIAN_POINT ( 'NONE',  ( 19.05341960407611168, 5.049401038298154454, 108.9572429386477097 ) ) ;
#68302=CARTESIAN_POINT ( 'NONE',  ( 16.53943276465976808, 0.05219959533934440121, 96.25109039468568994 ) ) ;
#68303=CARTESIAN_POINT ( 'NONE',  ( 15.80617190586769283, -15.72974639402175789, 80.62609039468567573 ) ) ;
#68304=CARTESIAN_POINT ( 'NONE',  ( 16.53943276465976808, 0.05219959533934440121, 41.25109039468568284 ) ) ;
#68305=CARTESIAN_POINT ( 'NONE',  ( -15.80617190586768217, 15.72974639402176855, 43.12609039468568284 ) ) ;
#68307=CARTESIAN_POINT ( 'NONE',  ( -10.72451020669870658, -18.67979575497194134, 19.58442372801901143 ) ) ;
#68308=CARTESIAN_POINT ( 'NONE',  ( -8.224510206698948167, 14.34966873604960824, 95.41557627198102409 ) ) ;
#68309=CARTESIAN_POINT ( 'NONE',  ( -18.22780087662121673, -5.500000000000063061, 51.48459894673893444 ) ) ;
#68310=CARTESIAN_POINT ( 'NONE',  ( 14.29746914071049879, -8.314922557960816363, 53.33224293864769550 ) ) ;
#68311=CARTESIAN_POINT ( 'NONE',  ( -8.314922557961024197, 14.29746914071037800, 97.91775706135236135 ) ) ;
#68312=CARTESIAN_POINT ( 'NONE',  ( -13.89961937509977652, 13.97604488694528158, 35.62390960531435269 ) ) ;
#68313=CARTESIAN_POINT ( 'NONE',  ( -15.72974639402197994, 15.80617190586746368, 40.62390960531435269 ) ) ;
#68314=CARTESIAN_POINT ( 'NONE',  ( 4.379528057220339221, -16.55341960407611168, 82.70724293864770971 ) ) ;
#68315=CARTESIAN_POINT ( 'NONE',  ( -10.81492255796078084, -18.62759615963271287, 77.08224293864769550 ) ) ;
#68316=CARTESIAN_POINT ( 'NONE',  ( -16.51473224551069308, -9.474510206698971260, 91.66557627198103830 ) ) ;
#68317=CARTESIAN_POINT ( 'NONE',  ( 16.51473224551069308, 9.474510206698969483, 44.16557627198103120 ) ) ;
#68318=CARTESIAN_POINT ( 'NONE',  ( 9.474510206698729675, 16.51473224551082808, 92.08442372801900433 ) ) ;
#68320=CARTESIAN_POINT ( 'NONE',  ( -18.67979575497178146, -10.72451020669898902, 26.66557627198103475 ) ) ;
#68321=CARTESIAN_POINT ( 'NONE',  ( -0.05219959533937732626, 21.53943276465977519, 52.50109039468567573 ) ) ;
#68322=CARTESIAN_POINT ( 'NONE',  ( 16.51473224551069308, 9.474510206698969483, 49.16557627198102409 ) ) ;
#68323=CARTESIAN_POINT ( 'NONE',  ( -19.03943276465977164, 0.05219959533909376836, 86.24890960531436690 ) ) ;
#68325=CARTESIAN_POINT ( 'NONE',  ( -12.06949235617739369, -12.14591786802326823, 54.37609039468568994 ) ) ;
#68326=CARTESIAN_POINT ( 'NONE',  ( 15.80617190586769283, -15.72974639402175789, 25.62609039468567929 ) ) ;
#68327=CARTESIAN_POINT ( 'NONE',  ( -18.62759615963255300, -10.81492255796106328, 79.16775706135234714 ) ) ;
#68328=CARTESIAN_POINT ( 'NONE',  ( 18.62759615963271287, -10.81492255796078972, 23.33224293864769194 ) ) ;
#68329=CARTESIAN_POINT ( 'NONE',  ( -0.05219959533907301413, -21.53943276465977519, 87.49890960531436690 ) ) ;
#68330=CARTESIAN_POINT ( 'NONE',  ( -21.53943276465977519, 0.05219959533907696930, 116.2489096053143669 ) ) ;
#68331=CARTESIAN_POINT ( 'NONE',  ( 4.483927247898790824, -16.52544592524335698, 60.20942372801902565 ) ) ;
#68332=CARTESIAN_POINT ( 'NONE',  ( -18.62759615963270932, 10.81492255796079327, 60.83224293864769550 ) ) ;
#68333=CARTESIAN_POINT ( 'NONE',  ( 16.46253265017146816, 9.564922557961045513, 21.66775706135233648 ) ) ;
#68334=CARTESIAN_POINT ( 'NONE',  ( 0.05219959533909260263, 19.03943276465977164, 64.99890960531436690 ) ) ;
#68335=CARTESIAN_POINT ( 'NONE',  ( -19.05341960407611168, -5.049401038298163336, 106.4572429386476955 ) ) ;
#68336=CARTESIAN_POINT ( 'NONE',  ( -19.03943276465977164, 0.05219959533909376836, 86.24890960531436690 ) ) ;
#68338=CARTESIAN_POINT ( 'NONE',  ( -16.51473224551082808, 9.474510206698731452, 63.33442372801900433 ) ) ;
#68339=CARTESIAN_POINT ( 'NONE',  ( -18.67979575497178146, -10.72451020669898902, 51.66557627198102409 ) ) ;
#68340=CARTESIAN_POINT ( 'NONE',  ( -14.34966873604960291, -8.224510206698953496, 26.66557627198103475 ) ) ;
#68341=CARTESIAN_POINT ( 'NONE',  ( -16.51473224551082808, 9.474510206698731452, 103.3344237280190043 ) ) ;
#68343=CARTESIAN_POINT ( 'NONE',  ( 5.049401038297881783, 19.05341960407617563, 97.29275706135233293 ) ) ;
#68344=CARTESIAN_POINT ( 'NONE',  ( -18.62759615963270932, 10.81492255796079327, 90.83224293864769550 ) ) ;
#68345=CARTESIAN_POINT ( 'NONE',  ( 9.474510206698729675, 16.51473224551082808, 52.08442372801900433 ) ) ;
#68346=CARTESIAN_POINT ( 'NONE',  ( 17.05587630539787369, 6.762274262135677283, 106.7581969096268750 ) ) ;
#68347=CARTESIAN_POINT ( 'NONE',  ( -19.02544592524342804, 5.153800228976336051, 61.04057627198103120 ) ) ;
#68348=CARTESIAN_POINT ( 'NONE',  ( -12.14591786802309592, -12.06949235617757132, 61.87390960531436690 ) ) ;
#68349=CARTESIAN_POINT ( 'NONE',  ( 5.049401038298161559, -19.05341960407611168, 42.70724293864767418 ) ) ;
#68350=CARTESIAN_POINT ( 'NONE',  ( 14.34966873604960469, 8.224510206698951720, 59.16557627198103120 ) ) ;
#68352=CARTESIAN_POINT ( 'NONE',  ( -16.52544592524342804, 4.483927247898546575, 26.04057627198103475 ) ) ;
#68353=CARTESIAN_POINT ( 'NONE',  ( -19.03943276465977164, 0.05219959533909376836, 61.24890960531436690 ) ) ;
#68354=CARTESIAN_POINT ( 'NONE',  ( -17.60728821186567217, 5.500000000000037303, 50.86690927743004664 ) ) ;
#68355=CARTESIAN_POINT ( 'NONE',  ( -16.51473224551082808, 9.474510206698731452, 23.33442372801900078 ) ) ;
#68356=CARTESIAN_POINT ( 'NONE',  ( -14.29746914071037622, -8.314922557961029526, 44.16775706135234714 ) ) ;
#68357=CARTESIAN_POINT ( 'NONE',  ( -21.55341960407610458, -5.719274019375992779, 51.45724293864770260 ) ) ;
#68358=CARTESIAN_POINT ( 'NONE',  ( -15.80617190586768217, 15.72974639402176855, 103.1260903946856757 ) ) ;
#68359=ORIENTED_EDGE ( 'NONE', *, *, #190638, .F. ) ;
#68360=CARTESIAN_POINT ( 'NONE',  ( -5.153800228976328057, -19.02544592524343514, 57.29057627198103120 ) ) ;
#68362=CARTESIAN_POINT ( 'NONE',  ( -16.46253265017160317, 9.564922557960807481, 95.83224293864769550 ) ) ;
#68364=CARTESIAN_POINT ( 'NONE',  ( -18.62759615963255300, -10.81492255796106328, 24.16775706135235424 ) ) ;
#68365=CARTESIAN_POINT ( 'NONE',  ( 8.314922557960818139, 14.29746914071049879, 99.58224293864770971 ) ) ;
#68366=CARTESIAN_POINT ( 'NONE',  ( -21.55341960407610458, -5.719274019375992779, 86.45724293864770971 ) ) ;
#68367=CARTESIAN_POINT ( 'NONE',  ( 9.474510206698971260, -16.51473224551069308, 67.91557627198102409 ) ) ;
#68368=CARTESIAN_POINT ( 'NONE',  ( 9.474510206698971260, -16.51473224551069308, 82.91557627198103830 ) ) ;
#68369=CARTESIAN_POINT ( 'NONE',  ( -18.62759615963270932, 10.81492255796079327, 110.8322429386476955 ) ) ;
#68370=ORIENTED_EDGE ( 'NONE', *, *, #142150, .F. ) ;
#68371=CARTESIAN_POINT ( 'NONE',  ( 19.05341960407611168, 5.049401038298154454, 68.95724293864769550 ) ) ;
#68372=CARTESIAN_POINT ( 'NONE',  ( 19.46398650005388120, -5.500000000000036415, 97.68269651486373562 ) ) ;
#68373=CARTESIAN_POINT ( 'NONE',  ( 0.05219959533910956823, 16.53943276465976808, 109.9989096053143527 ) ) ;
#68374=CARTESIAN_POINT ( 'NONE',  ( -13.89961937509977652, 13.97604488694528158, 35.62390960531435269 ) ) ;
#68375=CARTESIAN_POINT ( 'NONE',  ( 5.049401038297881783, 19.05341960407617563, 97.29275706135233293 ) ) ;
#68376=CARTESIAN_POINT ( 'NONE',  ( 4.483927247898545687, 16.52544592524342804, 104.7905762719810241 ) ) ;
#68377=CARTESIAN_POINT ( 'NONE',  ( 5.719274019375673035, 21.55341960407619339, 72.29275706135236135 ) ) ;
#68378=CARTESIAN_POINT ( 'NONE',  ( -5.153800228976328057, -19.02544592524343514, 57.29057627198103120 ) ) ;
#68379=CARTESIAN_POINT ( 'NONE',  ( 15.72974639402176855, 15.80617190586768217, 36.87609039468568994 ) ) ;
#68380=CARTESIAN_POINT ( 'NONE',  ( -10.72451020669870658, -18.67979575497194134, 19.58442372801901143 ) ) ;
#68382=CARTESIAN_POINT ( 'NONE',  ( 9.564922557960805705, 16.46253265017160317, 69.58224293864770971 ) ) ;
#68384=CARTESIAN_POINT ( 'NONE',  ( -16.55341960407617563, 4.379528057220093196, 23.54275706135235424 ) ) ;
#68385=CARTESIAN_POINT ( 'NONE',  ( -15.80617190586745835, -15.72974639402198527, 26.87390960531435979 ) ) ;
#68386=CARTESIAN_POINT ( 'NONE',  ( -21.52544592524334988, -5.823673210054445271, 63.95942372801901854 ) ) ;
#68387=CARTESIAN_POINT ( 'NONE',  ( -19.05341960407611168, -5.049401038298163336, 106.4572429386476955 ) ) ;
#68388=CARTESIAN_POINT ( 'NONE',  ( 19.02544592524334988, 5.153800228976608722, 101.4594237280189759 ) ) ;
#68389=CARTESIAN_POINT ( 'NONE',  ( 0.05219959533909260263, 19.03943276465977164, 49.99890960531435979 ) ) ;
#68390=CARTESIAN_POINT ( 'NONE',  ( 9.564922557960805705, 16.46253265017160317, 74.58224293864769550 ) ) ;
#68391=CARTESIAN_POINT ( 'NONE',  ( 4.379528057220339221, -16.55341960407611168, 92.70724293864770971 ) ) ;
#68392=CARTESIAN_POINT ( 'NONE',  ( 19.02544592524343514, -5.153800228976328945, 108.5405762719810383 ) ) ;
#68393=CARTESIAN_POINT ( 'NONE',  ( -16.53943276465976808, 0.05219959533911058130, 86.24890960531436690 ) ) ;
#68394=CARTESIAN_POINT ( 'NONE',  ( -19.05341960407611168, -5.049401038298163336, 101.4572429386476955 ) ) ;
#68395=CARTESIAN_POINT ( 'NONE',  ( 12.06949235617757843, -12.14591786802309237, 63.12390960531435979 ) ) ;
#68396=CARTESIAN_POINT ( 'NONE',  ( -13.89961937509977652, 13.97604488694528158, 35.62390960531435269 ) ) ;
#68397=CARTESIAN_POINT ( 'NONE',  ( 5.823673210054444382, -21.52544592524334988, 55.20942372801902565 ) ) ;
#68398=CARTESIAN_POINT ( 'NONE',  ( 5.153800228976615827, -19.02544592524334988, 95.20942372801897591 ) ) ;
#68399=CARTESIAN_POINT ( 'NONE',  ( 8.314922557960818139, 14.29746914071049879, 49.58224293864769550 ) ) ;
#68400=CARTESIAN_POINT ( 'NONE',  ( 18.67979575497194134, -10.72451020669871369, 20.83442372801901143 ) ) ;
#68401=CARTESIAN_POINT ( 'NONE',  ( -5.823673210054116645, -21.52544592524344225, 42.29057627198103120 ) ) ;
#68402=CARTESIAN_POINT ( 'NONE',  ( 0.05219959533909260263, 19.03943276465977164, 114.9989096053143669 ) ) ;
#68403=CARTESIAN_POINT ( 'NONE',  ( 4.483927247898545687, 16.52544592524342804, 89.79057627198103830 ) ) ;
#68405=CARTESIAN_POINT ( 'NONE',  ( 9.474510206698971260, -16.51473224551069308, 62.91557627198102409 ) ) ;
#68406=CARTESIAN_POINT ( 'NONE',  ( -8.314922557961024197, 14.29746914071037800, 112.9177570613523329 ) ) ;
#68407=CARTESIAN_POINT ( 'NONE',  ( 14.29746914071037800, 8.314922557961029526, 101.6677570613523613 ) ) ;
#68408=CARTESIAN_POINT ( 'NONE',  ( 0.05219959533934541429, -16.53943276465976808, 80.00109039468568994 ) ) ;
#68409=CARTESIAN_POINT ( 'NONE',  ( -19.02544592524334988, -5.153800228976617603, 38.95942372801900433 ) ) ;
#68411=CARTESIAN_POINT ( 'NONE',  ( 9.474510206698971260, -16.51473224551069308, 97.91557627198102409 ) ) ;
#68412=CARTESIAN_POINT ( 'NONE',  ( 5.049401038298161559, -19.05341960407611168, 47.70724293864770260 ) ) ;
#68413=CARTESIAN_POINT ( 'NONE',  ( 14.29746914071049879, -8.314922557960816363, 58.33224293864768839 ) ) ;
#68414=CARTESIAN_POINT ( 'NONE',  ( 9.474510206698971260, -16.51473224551069308, 112.9155762719810383 ) ) ;
#68415=CARTESIAN_POINT ( 'NONE',  ( -13.97604488694527625, -13.89961937509977652, 106.8739096053143669 ) ) ;
#68416=CARTESIAN_POINT ( 'NONE',  ( -10.72451020669898014, 18.67979575497178502, 45.41557627198103830 ) ) ;
#68417=CARTESIAN_POINT ( 'NONE',  ( 0.05219959533910956823, 16.53943276465976808, 84.99890960531436690 ) ) ;
#68418=CARTESIAN_POINT ( 'NONE',  ( -14.29746914071037622, -8.314922557961029526, 39.16775706135235424 ) ) ;
#68421=CARTESIAN_POINT ( 'NONE',  ( 14.29746914071049879, -8.314922557960816363, 78.33224293864770971 ) ) ;
#68423=CARTESIAN_POINT ( 'NONE',  ( 16.46253265017146816, 9.564922557961045513, 71.66775706135233293 ) ) ;
#68424=CARTESIAN_POINT ( 'NONE',  ( 19.05341960407611168, 5.049401038298154454, 108.9572429386477097 ) ) ;
#68425=CARTESIAN_POINT ( 'NONE',  ( -19.03943276465977164, -0.05219959533935918106, 73.75109039468566152 ) ) ;
#68426=DIRECTION ( 'NONE',  ( -0.000000000000000000, -0.000000000000000000, 1.000000000000000000 ) ) ;
#68427=CARTESIAN_POINT ( 'NONE',  ( -14.29746914071037622, -8.314922557961029526, 24.16775706135235424 ) ) ;
#68428=CARTESIAN_POINT ( 'NONE',  ( -4.379528057220086978, -16.55341960407618274, 109.7927570613523613 ) ) ;
#68429=CARTESIAN_POINT ( 'NONE',  ( 19.03943276465977164, 0.05219959533936151252, 71.25109039468566152 ) ) ;
#68430=CARTESIAN_POINT ( 'NONE',  ( 15.72974639402199770, -15.80617190586745480, 33.12390960531435979 ) ) ;
#68431=CARTESIAN_POINT ( 'NONE',  ( 21.53943276465977519, 0.05219959533937863772, 71.25109039468568994 ) ) ;
#68433=CARTESIAN_POINT ( 'NONE',  ( -4.379528057220086978, -16.55341960407618274, 24.79275706135235779 ) ) ;
#68435=CARTESIAN_POINT ( 'NONE',  ( 13.89961937509977652, -13.97604488694527269, 93.12390960531436690 ) ) ;
#68436=CARTESIAN_POINT ( 'NONE',  ( 5.049401038298161559, -19.05341960407611168, 27.70724293864769550 ) ) ;
#68437=CARTESIAN_POINT ( 'NONE',  ( 14.34966873604960469, 8.224510206698951720, 94.16557627198103830 ) ) ;
#68438=CARTESIAN_POINT ( 'NONE',  ( -19.02544592524342804, 5.153800228976336051, 86.04057627198103830 ) ) ;
#68440=CARTESIAN_POINT ( 'NONE',  ( -16.51473224551069308, -9.474510206698971260, 81.66557627198103830 ) ) ;
#68442=CARTESIAN_POINT ( 'NONE',  ( 5.153800228976615827, -19.02544592524334988, 85.20942372801900433 ) ) ;
#68443=CARTESIAN_POINT ( 'NONE',  ( -0.05219959533907301413, -21.53943276465977519, 77.49890960531433848 ) ) ;
#68444=CARTESIAN_POINT ( 'NONE',  ( -9.564922557960796823, -16.46253265017161027, 42.08224293864769550 ) ) ;
#68445=CARTESIAN_POINT ( 'NONE',  ( -5.049401038297874678, -19.05341960407617918, 74.79275706135231871 ) ) ;
#68446=CARTESIAN_POINT ( 'NONE',  ( -0.05219959533907301413, -21.53943276465977519, 112.4989096053143669 ) ) ;
#68447=CARTESIAN_POINT ( 'NONE',  ( -19.02544592524342804, 5.153800228976336051, 71.04057627198099567 ) ) ;
#68448=CARTESIAN_POINT ( 'NONE',  ( 0.05219959533909260263, 19.03943276465977164, 104.9989096053143669 ) ) ;
#68450=CARTESIAN_POINT ( 'NONE',  ( -8.314922557961024197, 14.29746914071037800, 32.91775706135234714 ) ) ;
#68451=CARTESIAN_POINT ( 'NONE',  ( 18.67979575497178502, 10.72451020669898547, 104.1655762719810241 ) ) ;
#68452=CARTESIAN_POINT ( 'NONE',  ( -14.34966873604960291, -8.224510206698953496, 101.6655762719810383 ) ) ;
#68453=CARTESIAN_POINT ( 'NONE',  ( 9.474510206698971260, -16.51473224551069308, 82.91557627198103830 ) ) ;
#68454=CARTESIAN_POINT ( 'NONE',  ( -13.89961937509957401, -13.97604488694547875, 59.37609039468566863 ) ) ;
#68455=CARTESIAN_POINT ( 'NONE',  ( 10.72451020669898902, -18.67979575497178502, 92.91557627198103830 ) ) ;
#68456=CARTESIAN_POINT ( 'NONE',  ( 10.81492255796078972, 18.62759615963270932, 69.58224293864769550 ) ) ;
#68457=CARTESIAN_POINT ( 'NONE',  ( 4.379528057220339221, -16.55341960407611168, 42.70724293864770260 ) ) ;
#68458=CARTESIAN_POINT ( 'NONE',  ( 13.89961937509957401, 13.97604488694547697, 21.87609039468566152 ) ) ;
#68459=CARTESIAN_POINT ( 'NONE',  ( -4.483927247898782831, 16.52544592524335698, 67.70942372801901854 ) ) ;
#68460=CARTESIAN_POINT ( 'NONE',  ( -19.05341960407611168, -5.049401038298163336, 96.45724293864769550 ) ) ;
#68461=CARTESIAN_POINT ( 'NONE',  ( 16.51473224551069308, 9.474510206698969483, 49.16557627198102409 ) ) ;
#68462=CARTESIAN_POINT ( 'NONE',  ( 10.72451020669871369, 18.67979575497193778, 47.08442372801901854 ) ) ;
#68463=CARTESIAN_POINT ( 'NONE',  ( -21.53943276465977519, -0.05219959533937600094, 48.75109039468568284 ) ) ;
#68464=CARTESIAN_POINT ( 'NONE',  ( 19.05341960407611168, 5.049401038298154454, 63.95724293864769550 ) ) ;
#68465=CARTESIAN_POINT ( 'NONE',  ( 21.52544592524334988, 5.823673210054432836, 36.45942372801901143 ) ) ;
#68466=CARTESIAN_POINT ( 'NONE',  ( -5.153800228976607833, 19.02544592524334988, 72.70942372801900433 ) ) ;
#68467=CARTESIAN_POINT ( 'NONE',  ( 5.153800228976615827, -19.02544592524334988, 75.20942372801896170 ) ) ;
#68468=CARTESIAN_POINT ( 'NONE',  ( 0.05219959533909260263, 19.03943276465977164, 39.99890960531436690 ) ) ;
#68469=CARTESIAN_POINT ( 'NONE',  ( 16.55341960407618274, -4.379528057220086978, 91.04275706135236135 ) ) ;
#68470=CARTESIAN_POINT ( 'NONE',  ( 16.51473224551069308, 9.474510206698969483, 59.16557627198102409 ) ) ;
#68472=CARTESIAN_POINT ( 'NONE',  ( 13.89961937509977652, -13.97604488694527269, 98.12390960531433848 ) ) ;
#68473=CARTESIAN_POINT ( 'NONE',  ( -13.89961937509977652, 13.97604488694528158, 35.62390960531435269 ) ) ;
#68474=CARTESIAN_POINT ( 'NONE',  ( 5.823673210054125526, 21.52544592524343514, 89.79057627198103830 ) ) ;
#68475=CARTESIAN_POINT ( 'NONE',  ( 0.05219959533934541429, -16.53943276465976808, 65.00109039468568994 ) ) ;
#68476=CARTESIAN_POINT ( 'NONE',  ( -15.80617190586768217, 15.72974639402176855, 108.1260903946856757 ) ) ;
#68477=CARTESIAN_POINT ( 'NONE',  ( -16.51473224551069308, -9.474510206698971260, 46.66557627198102409 ) ) ;
#68478=CARTESIAN_POINT ( 'NONE',  ( 12.06949235617757843, -12.14591786802309237, 48.12390960531436690 ) ) ;
#68479=CARTESIAN_POINT ( 'NONE',  ( -8.314922557960811034, -14.29746914071050412, 82.08224293864768129 ) ) ;
#68480=CARTESIAN_POINT ( 'NONE',  ( -0.05219959533909027116, -19.03943276465977164, 72.49890960531435269 ) ) ;
#68481=CARTESIAN_POINT ( 'NONE',  ( 10.72451020669871369, 18.67979575497193778, 37.08442372801901143 ) ) ;
#68482=CARTESIAN_POINT ( 'NONE',  ( 13.89961937509977652, -13.97604488694527269, 98.12390960531433848 ) ) ;
#68483=CARTESIAN_POINT ( 'NONE',  ( 15.80617190586769283, -15.72974639402175789, 95.62609039468568994 ) ) ;
#68484=CARTESIAN_POINT ( 'NONE',  ( 8.224510206698742110, 14.34966873604972548, 82.08442372801901854 ) ) ;
#68485=CARTESIAN_POINT ( 'NONE',  ( -15.72974639402176322, -15.80617190586768395, 24.37609039468567573 ) ) ;
#68486=CARTESIAN_POINT ( 'NONE',  ( 16.51473224551069308, 9.474510206698969483, 114.1655762719810241 ) ) ;
#68487=CARTESIAN_POINT ( 'NONE',  ( 5.823673210054125526, 21.52544592524343514, 84.79057627198102409 ) ) ;
#68488=CARTESIAN_POINT ( 'NONE',  ( 14.29746914071049879, -8.314922557960816363, 53.33224293864769550 ) ) ;
#68489=CARTESIAN_POINT ( 'NONE',  ( 9.474510206698971260, -16.51473224551069308, 42.91557627198103120 ) ) ;
#68490=CARTESIAN_POINT ( 'NONE',  ( 16.52544592524342804, -4.483927247898539470, 63.54057627198103830 ) ) ;
#68491=CARTESIAN_POINT ( 'NONE',  ( 10.81492255796078972, 18.62759615963270932, 34.58224293864770260 ) ) ;
#68492=CARTESIAN_POINT ( 'NONE',  ( -16.51473224551082808, 9.474510206698731452, 28.33442372801900433 ) ) ;
#68493=CARTESIAN_POINT ( 'NONE',  ( 16.53943276465976808, -0.05219959533910856209, 93.74890960531436690 ) ) ;
#68494=CARTESIAN_POINT ( 'NONE',  ( -5.049401038298153566, 19.05341960407611168, 105.2072429386476671 ) ) ;
#68496=CARTESIAN_POINT ( 'NONE',  ( 8.224510206698742110, 14.34966873604972548, 47.08442372801901854 ) ) ;
#68497=CARTESIAN_POINT ( 'NONE',  ( -5.153800228976328057, -19.02544592524343514, 52.29057627198100988 ) ) ;
#68499=CARTESIAN_POINT ( 'NONE',  ( 8.314922557961029526, -14.29746914071037800, 95.41775706135234714 ) ) ;
#68500=CARTESIAN_POINT ( 'NONE',  ( -16.51473224551082808, 9.474510206698731452, 103.3344237280190043 ) ) ;
#68501=CARTESIAN_POINT ( 'NONE',  ( 21.53943276465977519, 0.05219959533937863772, 76.25109039468568994 ) ) ;
#68502=CARTESIAN_POINT ( 'NONE',  ( 9.564922557960805705, 16.46253265017160317, 69.58224293864770971 ) ) ;
#68503=CARTESIAN_POINT ( 'NONE',  ( -15.72974639402197994, 15.80617190586746368, 110.6239096053143669 ) ) ;
#68504=CARTESIAN_POINT ( 'NONE',  ( 16.52544592524335698, 4.483927247898782831, 51.45942372801901854 ) ) ;
#68505=CARTESIAN_POINT ( 'NONE',  ( -8.224510206698948167, 14.34966873604960824, 115.4155762719810241 ) ) ;
#68506=CARTESIAN_POINT ( 'NONE',  ( -14.34966873604972548, 8.224510206698743886, 23.33442372801901499 ) ) ;
#68508=CARTESIAN_POINT ( 'NONE',  ( 9.564922557961047289, -16.46253265017146816, 80.41775706135234714 ) ) ;
#68509=CARTESIAN_POINT ( 'NONE',  ( -5.823673210054116645, -21.52544592524344225, 82.29057627198103830 ) ) ;
#68510=CARTESIAN_POINT ( 'NONE',  ( 0.05219959533936267826, -19.03943276465977164, 60.00109039468566863 ) ) ;
#68511=CARTESIAN_POINT ( 'NONE',  ( 5.153800228976335163, 19.02544592524342804, 114.7905762719810241 ) ) ;
#68512=CARTESIAN_POINT ( 'NONE',  ( -5.823673210054116645, -21.52544592524344225, 102.2905762719810383 ) ) ;
#68514=CARTESIAN_POINT ( 'NONE',  ( -16.46253265017160317, 9.564922557960807481, 65.83224293864769550 ) ) ;
#68515=CARTESIAN_POINT ( 'NONE',  ( -17.49999999999999645, 7.499999999999998224, 22.00000000000000711 ) ) ;
#68516=CARTESIAN_POINT ( 'NONE',  ( 19.02544592524334988, 5.153800228976608722, 111.4594237280190043 ) ) ;
#68518=CARTESIAN_POINT ( 'NONE',  ( -21.52544592524334988, -5.823673210054445271, 53.95942372801900433 ) ) ;
#68519=CARTESIAN_POINT ( 'NONE',  ( -15.80617190586745835, -15.72974639402198527, 106.8739096053143811 ) ) ;
#68520=CARTESIAN_POINT ( 'NONE',  ( -12.14591786802309592, -12.06949235617757132, 66.87390960531436690 ) ) ;
#68521=CARTESIAN_POINT ( 'NONE',  ( -13.97604488694527625, -13.89961937509977652, 71.87390960531433848 ) ) ;
#68522=CARTESIAN_POINT ( 'NONE',  ( 15.72974639402176855, 15.80617190586768217, 76.87609039468567573 ) ) ;
#68523=CARTESIAN_POINT ( 'NONE',  ( 4.379528057220092307, 16.55341960407617563, 27.29275706135234358 ) ) ;
#68524=CARTESIAN_POINT ( 'NONE',  ( 19.05341960407617918, -5.049401038297876454, 31.04275706135232227 ) ) ;
#68525=CARTESIAN_POINT ( 'NONE',  ( 18.67979575497194134, -10.72451020669871369, 45.83442372801901854 ) ) ;
#68526=CARTESIAN_POINT ( 'NONE',  ( 0.05219959533907565091, 21.53943276465977519, 109.9989096053143527 ) ) ;
#68527=CARTESIAN_POINT ( 'NONE',  ( -10.81492255796078084, -18.62759615963271287, 62.08224293864769550 ) ) ;
#68528=CARTESIAN_POINT ( 'NONE',  ( -19.05341960407617563, 5.049401038297882671, 93.54275706135234714 ) ) ;
#68529=CARTESIAN_POINT ( 'NONE',  ( 19.02544592524334988, 5.153800228976608722, 66.45942372801899012 ) ) ;
#68530=CARTESIAN_POINT ( 'NONE',  ( 18.67979575497194134, -10.72451020669871369, 85.83442372801901854 ) ) ;
#68531=CARTESIAN_POINT ( 'NONE',  ( 13.89961937509957401, 13.97604488694547697, 51.87609039468566863 ) ) ;
#68532=CARTESIAN_POINT ( 'NONE',  ( -16.46253265017160317, 9.564922557960807481, 35.83224293864768839 ) ) ;
#68533=CARTESIAN_POINT ( 'NONE',  ( 21.52544592524344225, -5.823673210054117533, 58.54057627198103120 ) ) ;
#68534=CARTESIAN_POINT ( 'NONE',  ( -12.06949235617756955, 12.14591786802309770, 55.62390960531436690 ) ) ;
#68535=CARTESIAN_POINT ( 'NONE',  ( -18.56453257813365809, 5.499999999999960920, 95.99000423690688422 ) ) ;
#68536=CARTESIAN_POINT ( 'NONE',  ( -16.46253265017146816, -9.564922557961047289, 29.16775706135232937 ) ) ;
#68537=CARTESIAN_POINT ( 'NONE',  ( 14.29746914071037800, 8.314922557961029526, 86.66775706135234714 ) ) ;
#68538=CARTESIAN_POINT ( 'NONE',  ( 4.483927247898545687, 16.52544592524342804, 54.79057627198104541 ) ) ;
#68539=CARTESIAN_POINT ( 'NONE',  ( 10.81492255796106328, -18.62759615963255655, 80.41775706135234714 ) ) ;
#68540=CARTESIAN_POINT ( 'NONE',  ( 10.72451020669871369, 18.67979575497193778, 77.08442372801901854 ) ) ;
#68541=CARTESIAN_POINT ( 'NONE',  ( -10.72451020669898014, 18.67979575497178502, 75.41557627198102409 ) ) ;
#68542=CARTESIAN_POINT ( 'NONE',  ( 13.97604488694527802, 13.89961937509977652, 39.37390960531435269 ) ) ;
#68543=CARTESIAN_POINT ( 'NONE',  ( -10.72451020669870658, -18.67979575497194134, 54.58442372801901143 ) ) ;
#68544=CARTESIAN_POINT ( 'NONE',  ( 19.05341960407611168, 5.049401038298154454, 33.95724293864769550 ) ) ;
#68545=CARTESIAN_POINT ( 'NONE',  ( -19.05341960407611168, -5.049401038298163336, 46.45724293864768129 ) ) ;
#68546=CARTESIAN_POINT ( 'NONE',  ( -16.53943276465976808, 0.05219959533911058130, 106.2489096053143811 ) ) ;
#68547=CARTESIAN_POINT ( 'NONE',  ( 16.51473224551069308, 9.474510206698969483, 104.1655762719810241 ) ) ;
#68548=CARTESIAN_POINT ( 'NONE',  ( 16.52544592524342804, -4.483927247898539470, 38.54057627198103120 ) ) ;
#68549=CARTESIAN_POINT ( 'NONE',  ( 16.55341960407611168, 4.379528057220329451, 113.9572429386477239 ) ) ;
#68550=CARTESIAN_POINT ( 'NONE',  ( 15.72974639402199770, -15.80617190586745480, 88.12390960531436690 ) ) ;
#68551=CARTESIAN_POINT ( 'NONE',  ( 0.05219959533937995610, -21.53943276465977519, 20.00109039468568639 ) ) ;
#68553=CARTESIAN_POINT ( 'NONE',  ( -0.05219959533934338120, 16.53943276465976808, 32.50109039468568284 ) ) ;
#68555=CARTESIAN_POINT ( 'NONE',  ( -15.80617190586745835, -15.72974639402198527, 66.87390960531436690 ) ) ;
#68556=CARTESIAN_POINT ( 'NONE',  ( -18.67979575497193778, 10.72451020669871902, 88.33442372801901854 ) ) ;
#68557=CARTESIAN_POINT ( 'NONE',  ( 13.97604488694527802, 13.89961937509977652, 89.37390960531436690 ) ) ;
#68558=CARTESIAN_POINT ( 'NONE',  ( 21.53943276465977519, 0.05219959533937863772, 36.25109039468567573 ) ) ;
#68559=CARTESIAN_POINT ( 'NONE',  ( -18.67979575497178146, -10.72451020669898902, 26.66557627198103475 ) ) ;
#68560=CARTESIAN_POINT ( 'NONE',  ( 16.55341960407618274, -4.379528057220086978, 86.04275706135236135 ) ) ;
#68561=CARTESIAN_POINT ( 'NONE',  ( -21.52544592524334988, -5.823673210054445271, 88.95942372801901854 ) ) ;
#68562=CARTESIAN_POINT ( 'NONE',  ( -5.153800228976607833, 19.02544592524334988, 22.70942372801899012 ) ) ;
#68563=CARTESIAN_POINT ( 'NONE',  ( 16.52544592524335698, 4.483927247898782831, 71.45942372801901854 ) ) ;
#68564=CARTESIAN_POINT ( 'NONE',  ( -18.67979575497193778, 10.72451020669871902, 23.33442372801901499 ) ) ;
#68565=CARTESIAN_POINT ( 'NONE',  ( 9.564922557960805705, 16.46253265017160317, 34.58224293864770260 ) ) ;
#68566=CARTESIAN_POINT ( 'NONE',  ( -18.62759615963255300, -10.81492255796106328, 109.1677570613523613 ) ) ;
#68567=CARTESIAN_POINT ( 'NONE',  ( 13.89961937509977652, -13.97604488694527269, 108.1239096053143669 ) ) ;
#68568=CARTESIAN_POINT ( 'NONE',  ( 10.72451020669898902, -18.67979575497178502, 107.9155762719810241 ) ) ;
#68570=CARTESIAN_POINT ( 'NONE',  ( -18.62759615963270932, 10.81492255796079327, 60.83224293864769550 ) ) ;
#68571=CARTESIAN_POINT ( 'NONE',  ( 14.29746914071037800, 8.314922557961029526, 51.66775706135234714 ) ) ;
#68572=CARTESIAN_POINT ( 'NONE',  ( 4.483927247898545687, 16.52544592524342804, 54.79057627198104541 ) ) ;
#68573=CARTESIAN_POINT ( 'NONE',  ( 19.33860699428957020, -5.500000000000004441, 101.6010922787093733 ) ) ;
#68574=CARTESIAN_POINT ( 'NONE',  ( 5.049401038297881783, 19.05341960407617563, 72.29275706135234714 ) ) ;
#68576=CARTESIAN_POINT ( 'NONE',  ( -17.49999999999999645, 5.624438216177585659, 105.8167034491464449 ) ) ;
#68577=CARTESIAN_POINT ( 'NONE',  ( 4.379528057220092307, 16.55341960407617563, 22.29275706135235069 ) ) ;
#68578=CARTESIAN_POINT ( 'NONE',  ( -5.719274019375978568, 21.55341960407610458, 100.2072429386476955 ) ) ;
#68579=CARTESIAN_POINT ( 'NONE',  ( 16.53943276465976808, -0.05219959533910856209, 58.74890960531436690 ) ) ;
#68580=CARTESIAN_POINT ( 'NONE',  ( -9.564922557960796823, -16.46253265017161027, 107.0822429386476955 ) ) ;
#68581=CARTESIAN_POINT ( 'NONE',  ( 16.53943276465976808, 0.05219959533934440121, 46.25109039468567573 ) ) ;
#68582=CARTESIAN_POINT ( 'NONE',  ( -0.05219959533909027116, -19.03943276465977164, 52.49890960531436690 ) ) ;
#68583=CARTESIAN_POINT ( 'NONE',  ( -21.55341960407619339, 5.719274019375674811, 28.54275706135234358 ) ) ;
#68584=CARTESIAN_POINT ( 'NONE',  ( -13.97604488694547697, 13.89961937509957934, 103.1260903946856473 ) ) ;
#68585=CARTESIAN_POINT ( 'NONE',  ( -16.51473224551069308, -9.474510206698971260, 101.6655762719810241 ) ) ;
#68586=CARTESIAN_POINT ( 'NONE',  ( -16.46253265017160317, 9.564922557960807481, 85.83224293864769550 ) ) ;
#68587=CARTESIAN_POINT ( 'NONE',  ( -5.823673210054116645, -21.52544592524344225, 92.29057627198103830 ) ) ;
#68588=CARTESIAN_POINT ( 'NONE',  ( -9.564922557960796823, -16.46253265017161027, 52.08224293864768839 ) ) ;
#68590=CARTESIAN_POINT ( 'NONE',  ( -16.53943276465976808, 0.05219959533911058130, 66.24890960531436690 ) ) ;
#68591=CARTESIAN_POINT ( 'NONE',  ( 5.153800228976335163, 19.02544592524342804, 109.7905762719810099 ) ) ;
#68593=CARTESIAN_POINT ( 'NONE',  ( 16.51473224551083163, -9.474510206698727899, 80.83442372801899012 ) ) ;
#68594=CARTESIAN_POINT ( 'NONE',  ( -10.72451020669898014, 18.67979575497178502, 85.41557627198102409 ) ) ;
#68595=CARTESIAN_POINT ( 'NONE',  ( 5.153800228976615827, -19.02544592524334988, 45.20942372801901143 ) ) ;
#68596=CARTESIAN_POINT ( 'NONE',  ( 16.51473224551069308, 9.474510206698969483, 104.1655762719810241 ) ) ;
#68597=CARTESIAN_POINT ( 'NONE',  ( 17.72560187377284890, 5.500000000000043521, 76.57814504131320632 ) ) ;
#68598=CARTESIAN_POINT ( 'NONE',  ( 15.80617190586746368, 15.72974639402197994, 39.37390960531436690 ) ) ;
#68599=CARTESIAN_POINT ( 'NONE',  ( -9.564922557960796823, -16.46253265017161027, 82.08224293864768129 ) ) ;
#68600=CARTESIAN_POINT ( 'NONE',  ( -10.81492255796105439, 18.62759615963255655, 67.91775706135234714 ) ) ;
#68601=CARTESIAN_POINT ( 'NONE',  ( 19.05341960407611168, 5.049401038298154454, 33.95724293864769550 ) ) ;
#68602=CARTESIAN_POINT ( 'NONE',  ( -16.53943276465976808, 0.05219959533911058130, 71.24890960531435269 ) ) ;
#68603=CARTESIAN_POINT ( 'NONE',  ( 16.55341960407618274, -4.379528057220086978, 21.04275706135234714 ) ) ;
#68604=CARTESIAN_POINT ( 'NONE',  ( 5.719274019375673035, 21.55341960407619339, 52.29275706135236135 ) ) ;
#68605=ORIENTED_EDGE ( 'NONE', *, *, #42638, .T. ) ;
#68607=CARTESIAN_POINT ( 'NONE',  ( 5.153800228976615827, -19.02544592524334988, 75.20942372801896170 ) ) ;
#68609=CARTESIAN_POINT ( 'NONE',  ( 15.72974639402176855, 15.80617190586768217, 26.87609039468567218 ) ) ;
#68611=CARTESIAN_POINT ( 'NONE',  ( -19.25176906914649422, -5.499999999999741540, 45.99927264242278113 ) ) ;
#68612=CARTESIAN_POINT ( 'NONE',  ( -21.53943276465977519, -0.05219959533937600094, 108.7510903946857042 ) ) ;
#68613=CARTESIAN_POINT ( 'NONE',  ( 9.564922557960805705, 16.46253265017160317, 49.58224293864770260 ) ) ;
#68614=CARTESIAN_POINT ( 'NONE',  ( 18.67979575497194134, -10.72451020669871369, 110.8344237280190043 ) ) ;
#68615=CARTESIAN_POINT ( 'NONE',  ( 16.55341960407618274, -4.379528057220086978, 101.0427570613523756 ) ) ;
#68616=CARTESIAN_POINT ( 'NONE',  ( -13.97604488694527625, -13.89961937509977652, 96.87390960531433848 ) ) ;
#68617=CARTESIAN_POINT ( 'NONE',  ( -10.72451020669870658, -18.67979575497194134, 79.58442372801903275 ) ) ;
#68619=CARTESIAN_POINT ( 'NONE',  ( -18.10062525802553424, 5.500000000000031974, 98.51383468041922242 ) ) ;
#68621=CARTESIAN_POINT ( 'NONE',  ( 18.62759615963255655, 10.81492255796105972, 71.66775706135234714 ) ) ;
#68622=CARTESIAN_POINT ( 'NONE',  ( 5.719274019375673035, 21.55341960407619339, 107.2927570613523471 ) ) ;
#68624=CARTESIAN_POINT ( 'NONE',  ( -9.564922557960796823, -16.46253265017161027, 87.08224293864769550 ) ) ;
#68625=CARTESIAN_POINT ( 'NONE',  ( -0.05219959533936034679, 19.03943276465977164, 27.50109039468566507 ) ) ;
#68626=EDGE_CURVE ( 'NONE', #91848, #141307, #100919, .T. ) ;
#68628=CARTESIAN_POINT ( 'NONE',  ( 13.97604488694527802, 13.89961937509977652, 34.37390960531436690 ) ) ;
#68629=CARTESIAN_POINT ( 'NONE',  ( -18.62759615963270932, 10.81492255796079327, 55.83224293864770260 ) ) ;
#68630=CARTESIAN_POINT ( 'NONE',  ( -14.34966873604972548, 8.224510206698743886, 103.3344237280190043 ) ) ;
#68631=CARTESIAN_POINT ( 'NONE',  ( 14.29746914071049879, -8.314922557960816363, 98.33224293864769550 ) ) ;
#68632=CARTESIAN_POINT ( 'NONE',  ( -5.153800228976328057, -19.02544592524343514, 87.29057627198103830 ) ) ;
#68633=CARTESIAN_POINT ( 'NONE',  ( -10.72451020669870658, -18.67979575497194134, 104.5844237280190185 ) ) ;
#68634=CARTESIAN_POINT ( 'NONE',  ( -13.97604488694527625, -13.89961937509977652, 41.87390960531435979 ) ) ;
#68635=CARTESIAN_POINT ( 'NONE',  ( 14.34966873604960469, 8.224510206698951720, 89.16557627198102409 ) ) ;
#68636=CARTESIAN_POINT ( 'NONE',  ( -18.62759615963255300, -10.81492255796106328, 49.16775706135234003 ) ) ;
#68637=CARTESIAN_POINT ( 'NONE',  ( -0.05219959533907301413, -21.53943276465977519, 87.49890960531436690 ) ) ;
#68638=CARTESIAN_POINT ( 'NONE',  ( 5.049401038297881783, 19.05341960407617563, 52.29275706135234003 ) ) ;
#68640=CARTESIAN_POINT ( 'NONE',  ( -13.97604488694527625, -13.89961937509977652, 91.87390960531432427 ) ) ;
#68641=CARTESIAN_POINT ( 'NONE',  ( 8.224510206698953496, -14.34966873604960469, 57.91557627198103120 ) ) ;
#68642=CARTESIAN_POINT ( 'NONE',  ( 19.02544592524334988, 5.153800228976608722, 46.45942372801899012 ) ) ;
#68643=CARTESIAN_POINT ( 'NONE',  ( 0.05219959533909260263, 19.03943276465977164, 49.99890960531435979 ) ) ;
#68644=CARTESIAN_POINT ( 'NONE',  ( -8.224510206698948167, 14.34966873604960824, 45.41557627198103830 ) ) ;
#68645=CARTESIAN_POINT ( 'NONE',  ( 9.564922557961047289, -16.46253265017146816, 80.41775706135234714 ) ) ;
#68646=CARTESIAN_POINT ( 'NONE',  ( -19.01533133064924996, 5.499999999999451106, 83.76586590595742621 ) ) ;
#68647=CARTESIAN_POINT ( 'NONE',  ( -10.81492255796078084, -18.62759615963271287, 42.08224293864769550 ) ) ;
#68648=CARTESIAN_POINT ( 'NONE',  ( 0.05219959533910956823, 16.53943276465976808, 104.9989096053143669 ) ) ;
#68650=CARTESIAN_POINT ( 'NONE',  ( 13.97604488694527802, 13.89961937509977652, 54.37390960531435979 ) ) ;
#68651=CARTESIAN_POINT ( 'NONE',  ( -21.52544592524343514, 5.823673210054127303, 51.04057627198103120 ) ) ;
#68652=CARTESIAN_POINT ( 'NONE',  ( -9.474510206698964154, 16.51473224551069663, 30.41557627198102054 ) ) ;
#68653=CARTESIAN_POINT ( 'NONE',  ( -8.314922557961024197, 14.29746914071037800, 77.91775706135231871 ) ) ;
#68654=CARTESIAN_POINT ( 'NONE',  ( -13.97604488694527625, -13.89961937509977652, 61.87390960531435979 ) ) ;
#68655=CARTESIAN_POINT ( 'NONE',  ( 13.89961937509957401, 13.97604488694547697, 46.87609039468565442 ) ) ;
#68657=CARTESIAN_POINT ( 'NONE',  ( -10.81492255796105439, 18.62759615963255655, 67.91775706135234714 ) ) ;
#68658=CARTESIAN_POINT ( 'NONE',  ( 15.72974639402199770, -15.80617190586745480, 48.12390960531436690 ) ) ;
#68659=CARTESIAN_POINT ( 'NONE',  ( 19.03943276465977164, -0.05219959533909143690, 28.74890960531435624 ) ) ;
#68660=CARTESIAN_POINT ( 'NONE',  ( 19.03943276465977164, 0.05219959533936151252, 106.2510903946856615 ) ) ;
#68661=CARTESIAN_POINT ( 'NONE',  ( -0.05219959533909027116, -19.03943276465977164, 22.49890960531436690 ) ) ;
#68663=CARTESIAN_POINT ( 'NONE',  ( 21.53943276465977519, -0.05219959533907433946, 53.74890960531437401 ) ) ;
#68664=CARTESIAN_POINT ( 'NONE',  ( 5.049401038298161559, -19.05341960407611168, 22.70724293864769194 ) ) ;
#68665=CARTESIAN_POINT ( 'NONE',  ( -21.55341960407619339, 5.719274019375674811, 78.54275706135236135 ) ) ;
#68666=CARTESIAN_POINT ( 'NONE',  ( 16.55341960407611168, 4.379528057220329451, 48.95724293864770971 ) ) ;
#68667=CARTESIAN_POINT ( 'NONE',  ( 12.06949235617757843, -12.14591786802309237, 58.12390960531435979 ) ) ;
#68668=CARTESIAN_POINT ( 'NONE',  ( -5.823673210054116645, -21.52544592524344225, 77.29057627198102409 ) ) ;
#68670=CARTESIAN_POINT ( 'NONE',  ( 5.719274019375991003, -21.55341960407610458, 72.70724293864769550 ) ) ;
#68672=CARTESIAN_POINT ( 'NONE',  ( 18.67979575497178502, 10.72451020669898547, 29.16557627198103120 ) ) ;
#68673=CARTESIAN_POINT ( 'NONE',  ( -12.14591786802326823, 12.06949235617739902, 48.12609039468568284 ) ) ;
#68674=CARTESIAN_POINT ( 'NONE',  ( 16.55341960407611168, 4.379528057220329451, 83.95724293864770971 ) ) ;
#68675=CARTESIAN_POINT ( 'NONE',  ( -13.97604488694527625, -13.89961937509977652, 26.87390960531434558 ) ) ;
#68676=CARTESIAN_POINT ( 'NONE',  ( 18.09918380851992481, 5.500000000000035527, 48.98618307335610922 ) ) ;
#68678=CARTESIAN_POINT ( 'NONE',  ( -8.224510206698735004, -14.34966873604973081, 84.58442372801903275 ) ) ;
#68679=CARTESIAN_POINT ( 'NONE',  ( 5.823673210054444382, -21.52544592524334988, 25.20942372801901854 ) ) ;
#68680=CARTESIAN_POINT ( 'NONE',  ( -5.049401038298153566, 19.05341960407611168, 85.20724293864766707 ) ) ;
#68681=CARTESIAN_POINT ( 'NONE',  ( 18.62759615963255655, 10.81492255796105972, 51.66775706135234714 ) ) ;
#68682=CARTESIAN_POINT ( 'NONE',  ( -16.51473224551069308, -9.474510206698971260, 111.6655762719810383 ) ) ;
#68685=CARTESIAN_POINT ( 'NONE',  ( -5.719274019375665041, -21.55341960407619695, 39.79275706135235424 ) ) ;
#68686=CARTESIAN_POINT ( 'NONE',  ( 13.97604488694527802, 13.89961937509977652, 34.37390960531436690 ) ) ;
#68687=CARTESIAN_POINT ( 'NONE',  ( 0.05219959533909260263, 19.03943276465977164, 104.9989096053143669 ) ) ;
#68688=CARTESIAN_POINT ( 'NONE',  ( -0.05219959533936034679, 19.03943276465977164, 52.50109039468566863 ) ) ;
#68689=CARTESIAN_POINT ( 'NONE',  ( -10.72451020669870658, -18.67979575497194134, 29.58442372801901854 ) ) ;
#68690=CARTESIAN_POINT ( 'NONE',  ( -16.46253265017146816, -9.564922557961047289, 44.16775706135232582 ) ) ;
#68691=CARTESIAN_POINT ( 'NONE',  ( -5.049401038298153566, 19.05341960407611168, 25.20724293864768484 ) ) ;
#68692=CARTESIAN_POINT ( 'NONE',  ( -8.224510206698735004, -14.34966873604973081, 89.58442372801901854 ) ) ;
#68693=CARTESIAN_POINT ( 'NONE',  ( -0.05219959533936034679, 19.03943276465977164, 67.50109039468566152 ) ) ;
#68694=CARTESIAN_POINT ( 'NONE',  ( -16.55341960407617563, 4.379528057220093196, 108.5427570613523756 ) ) ;
#68696=CARTESIAN_POINT ( 'NONE',  ( -0.05219959533909027116, -19.03943276465977164, 87.49890960531436690 ) ) ;
#68697=CARTESIAN_POINT ( 'NONE',  ( -0.05219959533937732626, 21.53943276465977519, 97.50109039468567573 ) ) ;
#68698=CARTESIAN_POINT ( 'NONE',  ( -10.81492255796105439, 18.62759615963255655, 107.9177570613523471 ) ) ;
#68700=CARTESIAN_POINT ( 'NONE',  ( -19.05341960407611168, -5.049401038298163336, 106.4572429386476955 ) ) ;
#68701=CARTESIAN_POINT ( 'NONE',  ( -21.52544592524334988, -5.823673210054445271, 68.95942372801901854 ) ) ;
#68702=CARTESIAN_POINT ( 'NONE',  ( 16.53943276465976808, 0.05219959533934440121, 21.25109039468567218 ) ) ;
#68703=CARTESIAN_POINT ( 'NONE',  ( 19.05341960407611168, 5.049401038298154454, 83.95724293864766707 ) ) ;
#68704=CARTESIAN_POINT ( 'NONE',  ( 10.81492255796078972, 18.62759615963270932, 29.58224293864769905 ) ) ;
#68705=CARTESIAN_POINT ( 'NONE',  ( 13.97604488694527802, 13.89961937509977652, 94.37390960531436690 ) ) ;
#68706=CARTESIAN_POINT ( 'NONE',  ( -16.52216118717209170, -7.221426719304498754, 91.07599021046998189 ) ) ;
#68707=CARTESIAN_POINT ( 'NONE',  ( -9.564922557960796823, -16.46253265017161027, 72.08224293864770971 ) ) ;
#68708=CARTESIAN_POINT ( 'NONE',  ( -13.89961937509977652, 13.97604488694528158, 70.62390960531432427 ) ) ;
#68709=CARTESIAN_POINT ( 'NONE',  ( 16.55341960407618274, -4.379528057220086978, 106.0427570613523471 ) ) ;
#68711=CARTESIAN_POINT ( 'NONE',  ( -5.049401038297874678, -19.05341960407617918, 69.79275706135233293 ) ) ;
#68712=CARTESIAN_POINT ( 'NONE',  ( 19.05341960407611168, 5.049401038298154454, 98.95724293864766707 ) ) ;
#68713=CARTESIAN_POINT ( 'NONE',  ( -4.379528057220328563, 16.55341960407611168, 85.20724293864770971 ) ) ;
#68714=CARTESIAN_POINT ( 'NONE',  ( -10.72451020669898014, 18.67979575497178502, 30.41557627198101699 ) ) ;
#68715=CARTESIAN_POINT ( 'NONE',  ( 9.564922557960805705, 16.46253265017160317, 114.5822429386476955 ) ) ;
#68716=CARTESIAN_POINT ( 'NONE',  ( -4.379528057220328563, 16.55341960407611168, 90.20724293864770971 ) ) ;
#68718=CARTESIAN_POINT ( 'NONE',  ( 16.46253265017146816, 9.564922557961045513, 41.66775706135234003 ) ) ;
#68719=CARTESIAN_POINT ( 'NONE',  ( -4.483927247898539470, -16.52544592524342804, 27.29057627198103120 ) ) ;
#68720=CARTESIAN_POINT ( 'NONE',  ( -0.05219959533909027116, -19.03943276465977164, 102.4989096053143669 ) ) ;
#68721=CARTESIAN_POINT ( 'NONE',  ( 0.05219959533937995610, -21.53943276465977519, 60.00109039468568284 ) ) ;
#68722=CARTESIAN_POINT ( 'NONE',  ( 21.53943276465977519, -0.05219959533907433946, 53.74890960531437401 ) ) ;
#68723=CARTESIAN_POINT ( 'NONE',  ( 5.719274019375673035, 21.55341960407619339, 32.29275706135235424 ) ) ;
#68724=CARTESIAN_POINT ( 'NONE',  ( -15.80617190586745835, -15.72974639402198527, 76.87390960531439532 ) ) ;
#68725=CARTESIAN_POINT ( 'NONE',  ( 10.81492255796106328, -18.62759615963255655, 35.41775706135234003 ) ) ;
#68726=CARTESIAN_POINT ( 'NONE',  ( 12.14591786802309770, 12.06949235617756955, 104.3739096053143669 ) ) ;
#68727=CARTESIAN_POINT ( 'NONE',  ( -16.46253265017146816, -9.564922557961047289, 69.16775706135233293 ) ) ;
#68728=CARTESIAN_POINT ( 'NONE',  ( 9.474510206698971260, -16.51473224551069308, 47.91557627198102409 ) ) ;
#68729=CARTESIAN_POINT ( 'NONE',  ( 16.52544592524342804, -4.483927247898539470, 93.54057627198103830 ) ) ;
#68730=CARTESIAN_POINT ( 'NONE',  ( -9.564922557960796823, -16.46253265017161027, 92.08224293864769550 ) ) ;
#68731=CARTESIAN_POINT ( 'NONE',  ( -13.89961937509977652, 13.97604488694528158, 95.62390960531436690 ) ) ;
#68732=CARTESIAN_POINT ( 'NONE',  ( 12.06949235617757843, -12.14591786802309237, 113.1239096053143953 ) ) ;
#68733=CARTESIAN_POINT ( 'NONE',  ( 16.55341960407611168, 4.379528057220329451, 43.95724293864769550 ) ) ;
#68734=CARTESIAN_POINT ( 'NONE',  ( -0.05219959533934338120, 16.53943276465976808, 97.50109039468567573 ) ) ;
#68735=CARTESIAN_POINT ( 'NONE',  ( 16.51473224551069308, 9.474510206698969483, 54.16557627198103120 ) ) ;
#68736=CARTESIAN_POINT ( 'NONE',  ( -16.51473224551069308, -9.474510206698971260, 21.66557627198102765 ) ) ;
#68737=CARTESIAN_POINT ( 'NONE',  ( 16.46253265017146816, 9.564922557961045513, 21.66775706135233648 ) ) ;
#68739=CARTESIAN_POINT ( 'NONE',  ( 14.34966873604960469, 8.224510206698951720, 24.16557627198103120 ) ) ;
#68740=CARTESIAN_POINT ( 'NONE',  ( -5.823673210054431948, 21.52544592524334988, 47.70942372801902565 ) ) ;
#68741=CARTESIAN_POINT ( 'NONE',  ( 19.02544592524343514, -5.153800228976328945, 108.5405762719810383 ) ) ;
#68742=CARTESIAN_POINT ( 'NONE',  ( 8.314922557961029526, -14.29746914071037800, 45.41775706135234003 ) ) ;
#68743=CARTESIAN_POINT ( 'NONE',  ( -0.05219959533910754901, -16.53943276465976808, 32.49890960531435979 ) ) ;
#68744=CARTESIAN_POINT ( 'NONE',  ( 0.05219959533909260263, 19.03943276465977164, 49.99890960531435979 ) ) ;
#68745=CARTESIAN_POINT ( 'NONE',  ( 8.314922557961029526, -14.29746914071037800, 90.41775706135236135 ) ) ;
#68746=CARTESIAN_POINT ( 'NONE',  ( 16.52544592524335698, 4.483927247898782831, 26.45942372801901854 ) ) ;
#68747=CARTESIAN_POINT ( 'NONE',  ( -16.51473224551069308, -9.474510206698971260, 41.66557627198103120 ) ) ;
#68749=CARTESIAN_POINT ( 'NONE',  ( -4.483927247898539470, -16.52544592524342804, 102.2905762719810383 ) ) ;
#68750=CARTESIAN_POINT ( 'NONE',  ( -18.62759615963255300, -10.81492255796106328, 19.16775706135234714 ) ) ;
#68751=CARTESIAN_POINT ( 'NONE',  ( 5.153800228976335163, 19.02544592524342804, 44.79057627198103830 ) ) ;
#68752=CARTESIAN_POINT ( 'NONE',  ( 13.89961937509977652, -13.97604488694527269, 103.1239096053143527 ) ) ;
#68753=CARTESIAN_POINT ( 'NONE',  ( 5.153800228976335163, 19.02544592524342804, 29.79057627198102409 ) ) ;
#68754=CARTESIAN_POINT ( 'NONE',  ( -9.564922557960796823, -16.46253265017161027, 107.0822429386476955 ) ) ;
#68755=CARTESIAN_POINT ( 'NONE',  ( -17.49999999999999645, -5.500000000000000888, 104.2030961746582847 ) ) ;
#68756=CARTESIAN_POINT ( 'NONE',  ( -13.97604488694527625, -13.89961937509977652, 101.8739096053143811 ) ) ;
#68757=CARTESIAN_POINT ( 'NONE',  ( -15.72974639402176322, -15.80617190586768395, 39.37609039468567573 ) ) ;
#68758=CARTESIAN_POINT ( 'NONE',  ( 12.06949235617757843, -12.14591786802309237, 103.1239096053143811 ) ) ;
#68759=CARTESIAN_POINT ( 'NONE',  ( 5.153800228976335163, 19.02544592524342804, 104.7905762719809957 ) ) ;
#68761=CARTESIAN_POINT ( 'NONE',  ( 8.224510206698742110, 14.34966873604972548, 67.08442372801901854 ) ) ;
#68762=CARTESIAN_POINT ( 'NONE',  ( -10.81492255796105439, 18.62759615963255655, 87.91775706135234714 ) ) ;
#68763=CARTESIAN_POINT ( 'NONE',  ( -12.14591786802326823, 12.06949235617739902, 38.12609039468567573 ) ) ;
#68764=CARTESIAN_POINT ( 'NONE',  ( -19.05341960407611168, -5.049401038298163336, 76.45724293864769550 ) ) ;
#68765=CARTESIAN_POINT ( 'NONE',  ( -0.05219959533934338120, 16.53943276465976808, 37.50109039468568284 ) ) ;
#68766=CARTESIAN_POINT ( 'NONE',  ( 5.049401038297881783, 19.05341960407617563, 102.2927570613523045 ) ) ;
#68767=CARTESIAN_POINT ( 'NONE',  ( -0.05219959533934338120, 16.53943276465976808, 82.50109039468568994 ) ) ;
#68768=CARTESIAN_POINT ( 'NONE',  ( -19.02544592524334988, -5.153800228976617603, 93.95942372801900433 ) ) ;
#68769=CARTESIAN_POINT ( 'NONE',  ( -13.89961937509977652, 13.97604488694528158, 75.62390960531438111 ) ) ;
#68770=CARTESIAN_POINT ( 'NONE',  ( -10.72451020669898014, 18.67979575497178502, 100.4155762719810241 ) ) ;
#68771=CARTESIAN_POINT ( 'NONE',  ( -4.379528057220328563, 16.55341960407611168, 95.20724293864769550 ) ) ;
#68772=CARTESIAN_POINT ( 'NONE',  ( 19.03943276465977164, 0.05219959533936151252, 91.25109039468566152 ) ) ;
#68773=CARTESIAN_POINT ( 'NONE',  ( -14.29746914071037622, -8.314922557961029526, 74.16775706135231871 ) ) ;
#68774=CARTESIAN_POINT ( 'NONE',  ( -16.20579543436696568, 7.371946100355094345, 44.43479165828048849 ) ) ;
#68775=CARTESIAN_POINT ( 'NONE',  ( -16.46253265017146816, -9.564922557961047289, 74.16775706135234714 ) ) ;
#68777=CARTESIAN_POINT ( 'NONE',  ( 14.29746914071049879, -8.314922557960816363, 33.33224293864769550 ) ) ;
#68778=CARTESIAN_POINT ( 'NONE',  ( 4.483927247898545687, 16.52544592524342804, 99.79057627198103830 ) ) ;
#68779=CARTESIAN_POINT ( 'NONE',  ( -16.51473224551082808, 9.474510206698731452, 33.33442372801899722 ) ) ;
#68780=CARTESIAN_POINT ( 'NONE',  ( 5.153800228976617603, -19.02544592524335343, 45.20942372801900433 ) ) ;
#68781=CARTESIAN_POINT ( 'NONE',  ( -15.72974639402197994, 15.80617190586746368, 115.6239096053143669 ) ) ;
#68782=CARTESIAN_POINT ( 'NONE',  ( 15.50000000000000178, -5.500000000000000888, 22.00000000000000000 ) ) ;
#68783=CARTESIAN_POINT ( 'NONE',  ( 13.89961937509977652, -13.97604488694527269, 93.12390960531436690 ) ) ;
#68784=CARTESIAN_POINT ( 'NONE',  ( -10.81492255796105439, 18.62759615963255655, 102.9177570613523756 ) ) ;
#68785=CARTESIAN_POINT ( 'NONE',  ( -19.03943276465977164, 0.05219959533909376836, 71.24890960531435269 ) ) ;
#68786=CARTESIAN_POINT ( 'NONE',  ( -5.823673210054116645, -21.52544592524344225, 47.29057627198103120 ) ) ;
#68787=CARTESIAN_POINT ( 'NONE',  ( 4.483927247898545687, 16.52544592524342804, 94.79057627198105251 ) ) ;
#68788=CARTESIAN_POINT ( 'NONE',  ( -9.474510206698964154, 16.51473224551069663, 60.41557627198102409 ) ) ;
#68790=CARTESIAN_POINT ( 'NONE',  ( 16.55341960407611168, 4.379528057220329451, 108.9572429386476955 ) ) ;
#68791=CARTESIAN_POINT ( 'NONE',  ( -18.62759615963255300, -10.81492255796106328, 29.16775706135234003 ) ) ;
#68792=CARTESIAN_POINT ( 'NONE',  ( -15.80617190586768217, 15.72974639402176855, 68.12609039468567573 ) ) ;
#68793=CARTESIAN_POINT ( 'NONE',  ( 19.03943276465977164, -0.05219959533909143690, 48.74890960531435979 ) ) ;
#68794=CARTESIAN_POINT ( 'NONE',  ( -14.34966873604972548, 8.224510206698743886, 83.33442372801903275 ) ) ;
#68795=CARTESIAN_POINT ( 'NONE',  ( 21.55341960407610458, 5.719274019375980345, 113.9572429386477239 ) ) ;
#68796=VERTEX_POINT ( 'NONE', #149440 ) ;
#68797=CARTESIAN_POINT ( 'NONE',  ( -5.823673210054116645, -21.52544592524344225, 107.2905762719810525 ) ) ;
#68798=CARTESIAN_POINT ( 'NONE',  ( -19.05341960407617563, 5.049401038297882671, 53.54275706135231871 ) ) ;
#68799=CARTESIAN_POINT ( 'NONE',  ( -9.474510206698964154, 16.51473224551069663, 60.41557627198102409 ) ) ;
#68800=CARTESIAN_POINT ( 'NONE',  ( 5.153800228976615827, -19.02544592524334988, 35.20942372801899722 ) ) ;
#68801=CARTESIAN_POINT ( 'NONE',  ( 10.81492255796106328, -18.62759615963255655, 70.41775706135236135 ) ) ;
#68802=CARTESIAN_POINT ( 'NONE',  ( 21.52544592524344225, -5.823673210054117533, 68.54057627198103830 ) ) ;
#68803=CARTESIAN_POINT ( 'NONE',  ( 14.34966873604960469, 8.224510206698951720, 54.16557627198103120 ) ) ;
#68804=CARTESIAN_POINT ( 'NONE',  ( -5.719274019375665041, -21.55341960407619695, 89.79275706135236135 ) ) ;
#68805=CARTESIAN_POINT ( 'NONE',  ( 13.97604488694548053, -13.89961937509957401, 30.62609039468566863 ) ) ;
#68806=CARTESIAN_POINT ( 'NONE',  ( -4.379528057220328563, 16.55341960407611168, 65.20724293864768129 ) ) ;
#68807=CARTESIAN_POINT ( 'NONE',  ( 12.06949235617757843, -12.14591786802309237, 108.1239096053143811 ) ) ;
#68808=CARTESIAN_POINT ( 'NONE',  ( 19.02544592524334988, 5.153800228976608722, 51.45942372801900433 ) ) ;
#68809=CARTESIAN_POINT ( 'NONE',  ( 8.314922557960818139, 14.29746914071049879, 24.58224293864768839 ) ) ;
#68810=CARTESIAN_POINT ( 'NONE',  ( -21.53943276465977519, -0.05219959533937600094, 73.75109039468567573 ) ) ;
#68811=B_SPLINE_CURVE_WITH_KNOTS ( 'NONE', 3,
 ( #125612, #139770, #17443, #170126, #109442, #184314, #93271, #92279, #107447, #49769, #3257, #157941, #95266, #153963, #4238, #45795, #62935, #124615, #173121, #77117 ),
 .UNSPECIFIED., .F., .F.,
 ( 4, 2, 2, 2, 2, 2, 2, 2, 2, 4 ),
 ( 0.004000878361811927020, 0.004499404418915936912, 0.004997930476019946805, 0.005496456533123957565, 0.005994982590227967457, 0.006244245618779961995, 0.006493508647331957401, 0.006992034704435969895, 0.007490560761539982390, 0.007989086818643994017 ),
 .UNSPECIFIED. ) ;
#68812=CARTESIAN_POINT ( 'NONE',  ( -16.51473224551069308, -9.474510206698971260, 71.66557627198102409 ) ) ;
#68813=CARTESIAN_POINT ( 'NONE',  ( 13.97604488694548053, -13.89961937509957401, 45.62609039468566863 ) ) ;
#68814=CARTESIAN_POINT ( 'NONE',  ( -0.05219959533907301413, -21.53943276465977519, 52.49890960531435979 ) ) ;
#68815=CARTESIAN_POINT ( 'NONE',  ( -15.72974639402176322, -15.80617190586768395, 44.37609039468567573 ) ) ;
#68816=CARTESIAN_POINT ( 'NONE',  ( -0.05219959533907301413, -21.53943276465977519, 107.4989096053143669 ) ) ;
#68817=CARTESIAN_POINT ( 'NONE',  ( -9.474510206698720793, -16.51473224551083518, 104.5844237280190043 ) ) ;
#68818=CARTESIAN_POINT ( 'NONE',  ( 12.06949235617739724, 12.14591786802326823, 71.87609039468568994 ) ) ;
#68820=CARTESIAN_POINT ( 'NONE',  ( -5.719274019375978568, 21.55341960407610458, 105.2072429386477097 ) ) ;
#68821=CARTESIAN_POINT ( 'NONE',  ( -16.52544592524342804, 4.483927247898546575, 96.04057627198102409 ) ) ;
#68822=CARTESIAN_POINT ( 'NONE',  ( -17.49999999999998579, -3.805241302050414998, 29.62647527217406562 ) ) ;
#68823=CARTESIAN_POINT ( 'NONE',  ( 16.53943276465976808, 0.05219959533934440121, 26.25109039468567573 ) ) ;
#68824=CARTESIAN_POINT ( 'NONE',  ( -21.53943276465977519, 0.05219959533907696930, 46.24890960531435979 ) ) ;
#68825=CARTESIAN_POINT ( 'NONE',  ( 0.05219959533934541429, -16.53943276465976808, 85.00109039468568994 ) ) ;
#68828=CARTESIAN_POINT ( 'NONE',  ( 4.379528057220092307, 16.55341960407617563, 62.29275706135236845 ) ) ;
#68829=CARTESIAN_POINT ( 'NONE',  ( 0.05219959533937995610, -21.53943276465977519, 35.00109039468568284 ) ) ;
#68830=CARTESIAN_POINT ( 'NONE',  ( -21.52544592524343514, 5.823673210054127303, 61.04057627198103120 ) ) ;
#68831=CARTESIAN_POINT ( 'NONE',  ( -14.29746914071037622, -8.314922557961029526, 84.16775706135234714 ) ) ;
#68832=CARTESIAN_POINT ( 'NONE',  ( -0.05219959533909027116, -19.03943276465977164, 102.4989096053143669 ) ) ;
#68833=CARTESIAN_POINT ( 'NONE',  ( 10.81492255796106328, -18.62759615963255655, 70.41775706135236135 ) ) ;
#68834=CARTESIAN_POINT ( 'NONE',  ( -15.72974639402197994, 15.80617190586746368, 45.62390960531436690 ) ) ;
#68835=CARTESIAN_POINT ( 'NONE',  ( -21.52544592524343514, 5.823673210054127303, 31.04057627198102409 ) ) ;
#68837=CARTESIAN_POINT ( 'NONE',  ( -16.51473224551082808, 9.474510206698731452, 58.33442372801900433 ) ) ;
#68838=CARTESIAN_POINT ( 'NONE',  ( -14.34966873604972548, 8.224510206698743886, 68.33442372801900433 ) ) ;
#68839=CARTESIAN_POINT ( 'NONE',  ( -0.05219959533907301413, -21.53943276465977519, 37.49890960531436690 ) ) ;
#68841=CARTESIAN_POINT ( 'NONE',  ( -16.46253265017160317, 9.564922557960807481, 85.83224293864769550 ) ) ;
#68842=CARTESIAN_POINT ( 'NONE',  ( -16.52544592524342804, 4.483927247898546575, 26.04057627198103475 ) ) ;
#68844=CARTESIAN_POINT ( 'NONE',  ( -12.06949235617756955, 12.14591786802309770, 110.6239096053143669 ) ) ;
#68845=CARTESIAN_POINT ( 'NONE',  ( -5.719274019375978568, 21.55341960407610458, 50.20724293864769550 ) ) ;
#68846=CARTESIAN_POINT ( 'NONE',  ( -9.474510206698964154, 16.51473224551069663, 50.41557627198102409 ) ) ;
#68847=CARTESIAN_POINT ( 'NONE',  ( -14.29746914071037622, -8.314922557961029526, 89.16775706135236135 ) ) ;
#68848=CARTESIAN_POINT ( 'NONE',  ( 21.52544592524334988, 5.823673210054432836, 36.45942372801901143 ) ) ;
#68849=CARTESIAN_POINT ( 'NONE',  ( 16.51473224551083163, -9.474510206698727899, 85.83442372801900433 ) ) ;
#68850=CARTESIAN_POINT ( 'NONE',  ( 4.379528057220339221, -16.55341960407611168, 92.70724293864770971 ) ) ;
#68851=CARTESIAN_POINT ( 'NONE',  ( 13.89961937509977652, -13.97604488694527269, 58.12390960531436690 ) ) ;
#68852=CARTESIAN_POINT ( 'NONE',  ( -19.05341960407611168, -5.049401038298163336, 31.45724293864769550 ) ) ;
#68853=DIRECTION ( 'NONE',  ( 0.000000000000000000, 0.000000000000000000, -1.000000000000000000 ) ) ;
#68854=CARTESIAN_POINT ( 'NONE',  ( -0.05219959533909027116, -19.03943276465977164, 72.49890960531435269 ) ) ;
#68855=CARTESIAN_POINT ( 'NONE',  ( -8.314922557961024197, 14.29746914071037800, 57.91775706135234714 ) ) ;
#68856=CARTESIAN_POINT ( 'NONE',  ( -18.67979575497193778, 10.72451020669871902, 108.3344237280190185 ) ) ;
#68857=CARTESIAN_POINT ( 'NONE',  ( -5.719274019375978568, 21.55341960407610458, 55.20724293864770260 ) ) ;
#68858=CARTESIAN_POINT ( 'NONE',  ( -8.224510206698735004, -14.34966873604973081, 69.58442372801900433 ) ) ;
#68859=CARTESIAN_POINT ( 'NONE',  ( -5.049401038297874678, -19.05341960407617918, 54.79275706135234003 ) ) ;
#68860=CARTESIAN_POINT ( 'NONE',  ( 16.46253265017146816, 9.564922557961045513, 61.66775706135234003 ) ) ;
#68861=ORIENTED_EDGE ( 'NONE', *, *, #163318, .F. ) ;
#68862=CARTESIAN_POINT ( 'NONE',  ( 5.719274019375673035, 21.55341960407619339, 62.29275706135236845 ) ) ;
#68863=CARTESIAN_POINT ( 'NONE',  ( 9.564922557960805705, 16.46253265017160317, 64.58224293864769550 ) ) ;
#68864=CARTESIAN_POINT ( 'NONE',  ( -19.02544592524342804, 5.153800228976336051, 31.04057627198102409 ) ) ;
#68865=CARTESIAN_POINT ( 'NONE',  ( -19.02544592524334988, -5.153800228976617603, 58.95942372801900433 ) ) ;
#68866=CARTESIAN_POINT ( 'NONE',  ( 19.05341960407611168, 5.049401038298154454, 113.9572429386477097 ) ) ;
#68867=CARTESIAN_POINT ( 'NONE',  ( 16.46253265017160672, -9.564922557960803928, 93.33224293864769550 ) ) ;
#68868=CARTESIAN_POINT ( 'NONE',  ( -16.53943276465976808, 0.05219959533911058130, 56.24890960531436690 ) ) ;
#68869=CARTESIAN_POINT ( 'NONE',  ( 5.719274019375991003, -21.55341960407610458, 52.70724293864769550 ) ) ;
#68870=CARTESIAN_POINT ( 'NONE',  ( -17.50000000000000355, 5.076555817581253294, 103.8204850795022907 ) ) ;
#68871=CARTESIAN_POINT ( 'NONE',  ( 15.72974639402176855, 15.80617190586768217, 111.8760903946856615 ) ) ;
#68872=CARTESIAN_POINT ( 'NONE',  ( -17.05587630539788435, -6.762274262135696823, 79.25819690962690345 ) ) ;
#68873=CARTESIAN_POINT ( 'NONE',  ( 0.05219959533909260263, 19.03943276465977164, 49.99890960531435979 ) ) ;
#68876=CARTESIAN_POINT ( 'NONE',  ( 4.483927247898790824, -16.52544592524335698, 70.20942372801904696 ) ) ;
#68877=CARTESIAN_POINT ( 'NONE',  ( 18.67979575497178502, 10.72451020669898547, 94.16557627198103830 ) ) ;
#68878=CARTESIAN_POINT ( 'NONE',  ( 4.379528057220339221, -16.55341960407611168, 47.70724293864770260 ) ) ;
#68879=CARTESIAN_POINT ( 'NONE',  ( 13.89961937509977652, -13.97604488694527269, 48.12390960531435979 ) ) ;
#68881=CARTESIAN_POINT ( 'NONE',  ( 0.05219959533937995610, -21.53943276465977519, 35.00109039468568284 ) ) ;
#68882=CARTESIAN_POINT ( 'NONE',  ( 5.153800228976615827, -19.02544592524334988, 45.20942372801901143 ) ) ;
#68883=CARTESIAN_POINT ( 'NONE',  ( -16.46253265017160317, 9.564922557960807481, 45.83224293864769550 ) ) ;
#68884=CARTESIAN_POINT ( 'NONE',  ( -15.80617190586768217, 15.72974639402176855, 98.12609039468570415 ) ) ;
#68885=CARTESIAN_POINT ( 'NONE',  ( 17.44270441346517941, 5.991230190323027394, 98.86335079264229364 ) ) ;
#68887=CARTESIAN_POINT ( 'NONE',  ( 4.483927247898545687, 16.52544592524342804, 44.79057627198103120 ) ) ;
#68888=CARTESIAN_POINT ( 'NONE',  ( 19.49190055781009079, 5.500000000000045297, 43.06116087098784817 ) ) ;
#68889=CARTESIAN_POINT ( 'NONE',  ( -5.823673210054116645, -21.52544592524344225, 47.29057627198103120 ) ) ;
#68891=CARTESIAN_POINT ( 'NONE',  ( -16.51473224551069308, -9.474510206698971260, 101.6655762719810241 ) ) ;
#68892=CARTESIAN_POINT ( 'NONE',  ( 0.05219959533910956823, 16.53943276465976808, 84.99890960531436690 ) ) ;
#68893=CARTESIAN_POINT ( 'NONE',  ( 0.05219959533934541429, -16.53943276465976808, 20.00109039468568639 ) ) ;
#68894=CARTESIAN_POINT ( 'NONE',  ( 0.05219959533934541429, -16.53943276465976808, 110.0010903946856757 ) ) ;
#68896=CARTESIAN_POINT ( 'NONE',  ( 19.03943276465977164, -0.05219959533909143690, 93.74890960531435269 ) ) ;
#68897=CARTESIAN_POINT ( 'NONE',  ( -15.72974639402197994, 15.80617190586746368, 105.6239096053143669 ) ) ;
#68899=CARTESIAN_POINT ( 'NONE',  ( -12.06949235617756955, 12.14591786802309770, 30.62390960531436335 ) ) ;
#68900=CARTESIAN_POINT ( 'NONE',  ( 0.05219959533909260263, 19.03943276465977164, 104.9989096053143669 ) ) ;
#68901=CARTESIAN_POINT ( 'NONE',  ( -5.153800228976607833, 19.02544592524334988, 77.70942372801900433 ) ) ;
#68902=CARTESIAN_POINT ( 'NONE',  ( -19.03943276465977164, -0.05219959533935918106, 18.75109039468567218 ) ) ;
#68903=CARTESIAN_POINT ( 'NONE',  ( 21.55341960407610458, 5.719274019375980345, 88.95724293864769550 ) ) ;
#68904=CARTESIAN_POINT ( 'NONE',  ( -18.67979575497178146, -10.72451020669898902, 56.66557627198103830 ) ) ;
#68905=CARTESIAN_POINT ( 'NONE',  ( -13.97604488694527625, -13.89961937509977652, 66.87390960531436690 ) ) ;
#68906=CARTESIAN_POINT ( 'NONE',  ( -12.14591786802309592, -12.06949235617757132, 31.87390960531435979 ) ) ;
#68907=CARTESIAN_POINT ( 'NONE',  ( 5.049401038298161559, -19.05341960407611168, 72.70724293864768129 ) ) ;
#68910=CARTESIAN_POINT ( 'NONE',  ( -13.89961937509957401, -13.97604488694547875, 29.37609039468565797 ) ) ;
#68911=CARTESIAN_POINT ( 'NONE',  ( 8.314922557960818139, 14.29746914071049879, 84.58224293864769550 ) ) ;
#68912=CARTESIAN_POINT ( 'NONE',  ( 5.719274019375673035, 21.55341960407619339, 27.29275706135234358 ) ) ;
#68914=CARTESIAN_POINT ( 'NONE',  ( 8.314922557961029526, -14.29746914071037800, 100.4177570613523471 ) ) ;
#68915=CARTESIAN_POINT ( 'NONE',  ( -19.05341960407611168, -5.049401038298163336, 21.45724293864768839 ) ) ;
#68916=CARTESIAN_POINT ( 'NONE',  ( -5.153800228976328057, -19.02544592524343514, 72.29057627198102409 ) ) ;
#68919=CARTESIAN_POINT ( 'NONE',  ( 12.14591786802309770, 12.06949235617756955, 29.37390960531435269 ) ) ;
#68920=CARTESIAN_POINT ( 'NONE',  ( -18.62759615963255300, -10.81492255796106328, 59.16775706135234714 ) ) ;
#68922=CARTESIAN_POINT ( 'NONE',  ( -15.80617190586768217, 15.72974639402176855, 88.12609039468570415 ) ) ;
#68923=CARTESIAN_POINT ( 'NONE',  ( 16.46253265017160672, -9.564922557960803928, 43.33224293864769550 ) ) ;
#68924=CARTESIAN_POINT ( 'NONE',  ( 9.564922557960805705, 16.46253265017160317, 54.58224293864769550 ) ) ;
#68926=CARTESIAN_POINT ( 'NONE',  ( 18.67979575497194134, -10.72451020669871369, 100.8344237280190185 ) ) ;
#68927=CARTESIAN_POINT ( 'NONE',  ( -4.483927247898782831, 16.52544592524335698, 62.70942372801902565 ) ) ;
#68928=CARTESIAN_POINT ( 'NONE',  ( -5.823673210054431948, 21.52544592524334988, 82.70942372801900433 ) ) ;
#68929=CARTESIAN_POINT ( 'NONE',  ( 15.72974639402199770, -15.80617190586745480, 28.12390960531435979 ) ) ;
#68930=CARTESIAN_POINT ( 'NONE',  ( 16.51473224551083163, -9.474510206698727899, 90.83442372801900433 ) ) ;
#68931=CARTESIAN_POINT ( 'NONE',  ( -15.72974639402176322, -15.80617190586768395, 64.37609039468568994 ) ) ;
#68932=CARTESIAN_POINT ( 'NONE',  ( 4.483927247898790824, -16.52544592524335698, 40.20942372801901854 ) ) ;
#68933=CARTESIAN_POINT ( 'NONE',  ( 15.72974639402199770, -15.80617190586745480, 83.12390960531436690 ) ) ;
#68934=CARTESIAN_POINT ( 'NONE',  ( 9.474510206698729675, 16.51473224551082808, 82.08442372801899012 ) ) ;
#68935=CARTESIAN_POINT ( 'NONE',  ( -16.46253265017160317, 9.564922557960807481, 65.83224293864769550 ) ) ;
#68936=CARTESIAN_POINT ( 'NONE',  ( -9.474510206698720793, -16.51473224551083518, 94.58442372801900433 ) ) ;
#68937=CARTESIAN_POINT ( 'NONE',  ( 16.51473224551083163, -9.474510206698727899, 105.8344237280190043 ) ) ;
#68938=CARTESIAN_POINT ( 'NONE',  ( -16.52544592524342804, 4.483927247898546575, 51.04057627198103120 ) ) ;
#68939=CARTESIAN_POINT ( 'NONE',  ( 13.97604488694548053, -13.89961937509957401, 80.62609039468567573 ) ) ;
#68940=CARTESIAN_POINT ( 'NONE',  ( 0.05219959533934541429, -16.53943276465976808, 65.00109039468568994 ) ) ;
#68941=CARTESIAN_POINT ( 'NONE',  ( 19.03943276465977164, -0.05219959533909143690, 38.74890960531436690 ) ) ;
#68942=CARTESIAN_POINT ( 'NONE',  ( -19.05341960407611168, -5.049401038298163336, 56.45724293864768129 ) ) ;
#68943=CARTESIAN_POINT ( 'NONE',  ( 16.53943276465976808, 0.05219959533934440121, 56.25109039468568284 ) ) ;
#68946=CARTESIAN_POINT ( 'NONE',  ( -9.564922557960796823, -16.46253265017161027, 112.0822429386476955 ) ) ;
#68947=CARTESIAN_POINT ( 'NONE',  ( -9.564922557960796823, -16.46253265017161027, 27.08224293864769550 ) ) ;
#68949=CARTESIAN_POINT ( 'NONE',  ( -16.51473224551082808, 9.474510206698731452, 108.3344237280190043 ) ) ;
#68950=CARTESIAN_POINT ( 'NONE',  ( -0.05219959533907301413, -21.53943276465977519, 42.49890960531435979 ) ) ;
#68951=CARTESIAN_POINT ( 'NONE',  ( -9.564922557961040184, 16.46253265017147172, 32.91775706135233293 ) ) ;
#68952=CARTESIAN_POINT ( 'NONE',  ( 4.483927247898790824, -16.52544592524335698, 30.20942372801902565 ) ) ;
#68953=CARTESIAN_POINT ( 'NONE',  ( -5.049401038298153566, 19.05341960407611168, 25.20724293864768484 ) ) ;
#68954=CARTESIAN_POINT ( 'NONE',  ( 19.03943276465977164, -0.05219959533909143690, 48.74890960531435979 ) ) ;
#68955=CARTESIAN_POINT ( 'NONE',  ( -0.05219959533907301413, -21.53943276465977519, 77.49890960531433848 ) ) ;
#68956=CARTESIAN_POINT ( 'NONE',  ( -16.51473224551069308, -9.474510206698971260, 96.66557627198102409 ) ) ;
#68957=VECTOR ( 'NONE', #99707, 1000.000000000000000 ) ;
#68958=CARTESIAN_POINT ( 'NONE',  ( 13.97604488694527802, 13.89961937509977652, 44.37390960531435269 ) ) ;
#68960=CARTESIAN_POINT ( 'NONE',  ( -9.474510206698720793, -16.51473224551083518, 79.58442372801899012 ) ) ;
#68961=CARTESIAN_POINT ( 'NONE',  ( 14.29746914071049879, -8.314922557960816363, 68.33224293864769550 ) ) ;
#68962=CARTESIAN_POINT ( 'NONE',  ( 10.72451020669898902, -18.67979575497178502, 52.91557627198103830 ) ) ;
#68963=CARTESIAN_POINT ( 'NONE',  ( 21.52544592524334988, 5.823673210054432836, 111.4594237280190328 ) ) ;
#68964=CARTESIAN_POINT ( 'NONE',  ( 21.55341960407610458, 5.719274019375980345, 98.95724293864770971 ) ) ;
#68965=CARTESIAN_POINT ( 'NONE',  ( 10.81492255796106328, -18.62759615963255655, 70.41775706135236135 ) ) ;
#68966=CARTESIAN_POINT ( 'NONE',  ( 0.05219959533937995610, -21.53943276465977519, 80.00109039468568994 ) ) ;
#68967=CARTESIAN_POINT ( 'NONE',  ( 19.05341960407611168, 5.049401038298154454, 113.9572429386477097 ) ) ;
#68968=CARTESIAN_POINT ( 'NONE',  ( 16.53943276465976808, 0.05219959533934440121, 106.2510903946856757 ) ) ;
#68969=CARTESIAN_POINT ( 'NONE',  ( 10.72451020669871369, 18.67979575497193778, 72.08442372801899012 ) ) ;
#68970=CARTESIAN_POINT ( 'NONE',  ( -13.97604488694527625, -13.89961937509977652, 66.87390960531436690 ) ) ;
#68971=CARTESIAN_POINT ( 'NONE',  ( 0.05219959533937995610, -21.53943276465977519, 30.00109039468568284 ) ) ;
#68972=CARTESIAN_POINT ( 'NONE',  ( -16.46253265017160317, 9.564922557960807481, 65.83224293864769550 ) ) ;
#68973=CARTESIAN_POINT ( 'NONE',  ( 8.314922557960818139, 14.29746914071049879, 74.58224293864768129 ) ) ;
#68974=CARTESIAN_POINT ( 'NONE',  ( 14.34966873604960469, 8.224510206698951720, 54.16557627198103120 ) ) ;
#68975=CARTESIAN_POINT ( 'NONE',  ( 21.53943276465977519, -0.05219959533907433946, 53.74890960531437401 ) ) ;
#68976=CARTESIAN_POINT ( 'NONE',  ( 5.049401038298161559, -19.05341960407611168, 67.70724293864769550 ) ) ;
#68977=CARTESIAN_POINT ( 'NONE',  ( -10.72451020669898014, 18.67979575497178502, 75.41557627198102409 ) ) ;
#68978=CARTESIAN_POINT ( 'NONE',  ( 19.03943276465977164, 0.05219959533936151252, 61.25109039468566863 ) ) ;
#68979=CARTESIAN_POINT ( 'NONE',  ( -5.153800228976607833, 19.02544592524335343, 22.70942372801899367 ) ) ;
#68980=CARTESIAN_POINT ( 'NONE',  ( -12.14591786802309592, -12.06949235617757132, 66.87390960531436690 ) ) ;
#68981=CARTESIAN_POINT ( 'NONE',  ( -0.05219959533907301413, -21.53943276465977519, 37.49890960531436690 ) ) ;
#68982=ORIENTED_EDGE ( 'NONE', *, *, #9460, .F. ) ;
#68984=CARTESIAN_POINT ( 'NONE',  ( -17.72662750342724891, -5.500000000000089706, 41.40179492283743912 ) ) ;
#68985=CARTESIAN_POINT ( 'NONE',  ( 8.224510206698742110, 14.34966873604972548, 97.08442372801904696 ) ) ;
#68987=CARTESIAN_POINT ( 'NONE',  ( -16.46253265017146816, -9.564922557961047289, 94.16775706135233293 ) ) ;
#68988=CARTESIAN_POINT ( 'NONE',  ( 4.379528057220339221, -16.55341960407611168, 72.70724293864769550 ) ) ;
#68990=CARTESIAN_POINT ( 'NONE',  ( -9.564922557960796823, -16.46253265017161027, 57.08224293864769550 ) ) ;
#68991=CARTESIAN_POINT ( 'NONE',  ( 12.06949235617757843, -12.14591786802309237, 58.12390960531435979 ) ) ;
#68992=CARTESIAN_POINT ( 'NONE',  ( 19.02544592524343514, -5.153800228976328945, 83.54057627198100988 ) ) ;
#68993=CARTESIAN_POINT ( 'NONE',  ( -19.03943276465977164, -0.05219959533935918106, 78.75109039468567573 ) ) ;
#68994=CARTESIAN_POINT ( 'NONE',  ( -19.02544592524342804, 5.153800228976336051, 51.04057627198103120 ) ) ;
#68995=CARTESIAN_POINT ( 'NONE',  ( -13.89961937509977652, 13.97604488694528158, 80.62390960531436690 ) ) ;
#68996=CARTESIAN_POINT ( 'NONE',  ( 9.564922557960805705, 16.46253265017160317, 69.58224293864770971 ) ) ;
#68997=CARTESIAN_POINT ( 'NONE',  ( -21.55341960407610458, -5.719274019375992779, 61.45724293864770260 ) ) ;
#68998=CARTESIAN_POINT ( 'NONE',  ( 13.97604488694527802, 13.89961937509977652, 49.37390960531434558 ) ) ;
#68999=CARTESIAN_POINT ( 'NONE',  ( -18.67979575497178146, -10.72451020669898902, 51.66557627198102409 ) ) ;
#69000=CARTESIAN_POINT ( 'NONE',  ( 5.049401038297881783, 19.05341960407617563, 77.29275706135231871 ) ) ;
#69001=CARTESIAN_POINT ( 'NONE',  ( -8.314922557961024197, 14.29746914071037800, 97.91775706135236135 ) ) ;
#69002=CARTESIAN_POINT ( 'NONE',  ( 5.049401038297881783, 19.05341960407617563, 32.29275706135233293 ) ) ;
#69003=CARTESIAN_POINT ( 'NONE',  ( 14.34966873604972726, -8.224510206698740333, 65.83442372801900433 ) ) ;
#69004=CARTESIAN_POINT ( 'NONE',  ( -14.29746914071037622, -8.314922557961029526, 94.16775706135237556 ) ) ;
#69006=CARTESIAN_POINT ( 'NONE',  ( 4.379528057220092307, 16.55341960407617563, 77.29275706135234714 ) ) ;
#69007=CARTESIAN_POINT ( 'NONE',  ( 15.80617190586746368, 15.72974639402197994, 29.37390960531435269 ) ) ;
#69008=CARTESIAN_POINT ( 'NONE',  ( -19.03943276465977164, 0.05219959533909376836, 36.24890960531436690 ) ) ;
#69009=CARTESIAN_POINT ( 'NONE',  ( 14.34966873604972726, -8.224510206698740333, 35.83442372801901143 ) ) ;
#69010=CARTESIAN_POINT ( 'NONE',  ( 5.153800228976335163, 19.02544592524342804, 44.79057627198103830 ) ) ;
#69011=CARTESIAN_POINT ( 'NONE',  ( 21.55341960407619695, -5.719274019375665929, 46.04275706135234714 ) ) ;
#69012=CARTESIAN_POINT ( 'NONE',  ( -4.379528057220086978, -16.55341960407618274, 44.79275706135234714 ) ) ;
#69013=CARTESIAN_POINT ( 'NONE',  ( -16.53943276465976808, 0.05219959533911058130, 21.24890960531436690 ) ) ;
#69014=CARTESIAN_POINT ( 'NONE',  ( -13.89961937509977652, 13.97604488694528158, 30.62390960531435269 ) ) ;
#69015=CARTESIAN_POINT ( 'NONE',  ( 0.05219959533936267826, -19.03943276465977164, 25.00109039468566152 ) ) ;
#69016=CARTESIAN_POINT ( 'NONE',  ( -5.153800228976607833, 19.02544592524334988, 107.7094237280189759 ) ) ;
#69018=CARTESIAN_POINT ( 'NONE',  ( -13.97604488694547697, 13.89961937509957934, 68.12609039468563310 ) ) ;
#69019=CARTESIAN_POINT ( 'NONE',  ( 8.224510206698953496, -14.34966873604960469, 72.91557627198103830 ) ) ;
#69020=CARTESIAN_POINT ( 'NONE',  ( 9.564922557960805705, 16.46253265017160317, 34.58224293864770260 ) ) ;
#69021=CARTESIAN_POINT ( 'NONE',  ( -13.97604488694547697, 13.89961937509957934, 68.12609039468563310 ) ) ;
#69023=CARTESIAN_POINT ( 'NONE',  ( -21.55341960407619339, 5.719274019375674811, 68.54275706135234714 ) ) ;
#69024=CARTESIAN_POINT ( 'NONE',  ( 8.314922557961029526, -14.29746914071037800, 45.41775706135234003 ) ) ;
#69025=CARTESIAN_POINT ( 'NONE',  ( 17.72517630441461023, -5.499999999999981348, 73.42175719257603816 ) ) ;
#69026=CARTESIAN_POINT ( 'NONE',  ( 5.719274019375991003, -21.55341960407610458, 32.70724293864770260 ) ) ;
#69027=CARTESIAN_POINT ( 'NONE',  ( -4.483927247898782831, 16.52544592524335698, 22.70942372801901499 ) ) ;
#69028=CARTESIAN_POINT ( 'NONE',  ( 17.97161686093727795, -5.499999999999970690, 98.49637206859168259 ) ) ;
#69030=CARTESIAN_POINT ( 'NONE',  ( -9.564922557960796823, -16.46253265017161027, 42.08224293864769550 ) ) ;
#69031=CARTESIAN_POINT ( 'NONE',  ( -15.72974639402176322, -15.80617190586768395, 109.3760903946857042 ) ) ;
#69032=CARTESIAN_POINT ( 'NONE',  ( -16.51473224551069308, -9.474510206698971260, 51.66557627198102409 ) ) ;
#69033=CARTESIAN_POINT ( 'NONE',  ( 18.62759615963255655, 10.81492255796105972, 66.66775706135234714 ) ) ;
#69034=CARTESIAN_POINT ( 'NONE',  ( -10.81492255796105439, 18.62759615963255655, 107.9177570613523471 ) ) ;
#69035=CARTESIAN_POINT ( 'NONE',  ( -16.53943276465976808, -0.05219959533934237506, 113.7510903946856757 ) ) ;
#69036=CARTESIAN_POINT ( 'NONE',  ( -16.46253265017160317, 9.564922557960807481, 35.83224293864768839 ) ) ;
#69037=CARTESIAN_POINT ( 'NONE',  ( -13.89961937509977652, 13.97604488694528158, 90.62390960531432427 ) ) ;
#69038=CARTESIAN_POINT ( 'NONE',  ( -10.81492255796105439, 18.62759615963255655, 52.91775706135235424 ) ) ;
#69039=CARTESIAN_POINT ( 'NONE',  ( -19.05341960407611168, -5.049401038298163336, 36.45724293864766707 ) ) ;
#69041=CARTESIAN_POINT ( 'NONE',  ( -21.53943276465977519, -0.05219959533937600094, 48.75109039468568284 ) ) ;
#69042=CARTESIAN_POINT ( 'NONE',  ( 13.89961937509957401, 13.97604488694547697, 96.87609039468566152 ) ) ;
#69043=CARTESIAN_POINT ( 'NONE',  ( 19.02544592524343514, -5.153800228976328945, 103.5405762719809957 ) ) ;
#69044=CARTESIAN_POINT ( 'NONE',  ( -8.314922557960811034, -14.29746914071050412, 112.0822429386477097 ) ) ;
#69045=CARTESIAN_POINT ( 'NONE',  ( -18.62759615963270932, 10.81492255796079327, 110.8322429386476955 ) ) ;
#69046=CARTESIAN_POINT ( 'NONE',  ( -9.474510206698720793, -16.51473224551083518, 34.58442372801899722 ) ) ;
#69047=CARTESIAN_POINT ( 'NONE',  ( 16.55341960407611168, 4.379528057220329451, 113.9572429386477239 ) ) ;
#69048=CARTESIAN_POINT ( 'NONE',  ( 13.89961937509977652, -13.97604488694527269, 63.12390960531435979 ) ) ;
#69049=CARTESIAN_POINT ( 'NONE',  ( 16.46253265017146816, 9.564922557961045513, 96.66775706135233293 ) ) ;
#69050=CARTESIAN_POINT ( 'NONE',  ( 14.29746914071049879, -8.314922557960816363, 68.33224293864769550 ) ) ;
#69051=CARTESIAN_POINT ( 'NONE',  ( -16.46253265017146816, -9.564922557961047289, 24.16775706135233648 ) ) ;
#69052=CARTESIAN_POINT ( 'NONE',  ( 19.02544592524343514, -5.153800228976328945, 113.5405762719810241 ) ) ;
#69053=CARTESIAN_POINT ( 'NONE',  ( -5.153800228976607833, 19.02544592524334988, 92.70942372801901854 ) ) ;
#69054=CARTESIAN_POINT ( 'NONE',  ( 0.05219959533907565091, 21.53943276465977519, 89.99890960531438111 ) ) ;
#69055=CARTESIAN_POINT ( 'NONE',  ( -21.52544592524334988, -5.823673210054445271, 38.95942372801901854 ) ) ;
#69056=CARTESIAN_POINT ( 'NONE',  ( 12.06949235617739724, 12.14591786802326823, 46.87609039468568994 ) ) ;
#69057=CARTESIAN_POINT ( 'NONE',  ( -14.34966873604972548, 8.224510206698743886, 103.3344237280190043 ) ) ;
#69058=CARTESIAN_POINT ( 'NONE',  ( -16.53943276465976808, -0.05219959533934237506, 43.75109039468568284 ) ) ;
#69059=CARTESIAN_POINT ( 'NONE',  ( -15.72974639402176322, -15.80617190586768395, 44.37609039468567573 ) ) ;
#69060=CARTESIAN_POINT ( 'NONE',  ( 0.05219959533907565091, 21.53943276465977519, 49.99890960531437401 ) ) ;
#69061=CARTESIAN_POINT ( 'NONE',  ( 13.97604488694527802, 13.89961937509977652, 29.37390960531435979 ) ) ;
#69063=CARTESIAN_POINT ( 'NONE',  ( 16.55341960407618274, -4.379528057220086978, 61.04275706135234714 ) ) ;
#69064=CARTESIAN_POINT ( 'NONE',  ( 18.67979575497178502, 10.72451020669898547, 89.16557627198102409 ) ) ;
#69065=CARTESIAN_POINT ( 'NONE',  ( 4.483927247898545687, 16.52544592524342804, 44.79057627198103120 ) ) ;
#69066=CARTESIAN_POINT ( 'NONE',  ( 12.06949235617739724, 12.14591786802326823, 66.87609039468568994 ) ) ;
#69067=CARTESIAN_POINT ( 'NONE',  ( 9.564922557961047289, -16.46253265017146816, 105.4177570613523471 ) ) ;
#69068=CARTESIAN_POINT ( 'NONE',  ( 10.72451020669898902, -18.67979575497178502, 97.91557627198103830 ) ) ;
#69069=CARTESIAN_POINT ( 'NONE',  ( -12.14591786802309592, -12.06949235617757132, 36.87390960531435979 ) ) ;
#69070=ORIENTED_EDGE ( 'NONE', *, *, #120968, .T. ) ;
#69071=CARTESIAN_POINT ( 'NONE',  ( -8.224510206698735004, -14.34966873604973081, 79.58442372801903275 ) ) ;
#69073=CARTESIAN_POINT ( 'NONE',  ( -18.62759615963270932, 10.81492255796079327, 80.83224293864769550 ) ) ;
#69074=ORIENTED_EDGE ( 'NONE', *, *, #53677, .T. ) ;
#69075=CARTESIAN_POINT ( 'NONE',  ( -16.55341960407617563, 4.379528057220093196, 103.5427570613523613 ) ) ;
#69076=ORIENTED_EDGE ( 'NONE', *, *, #107363, .F. ) ;
#69077=CARTESIAN_POINT ( 'NONE',  ( 19.52851543214743657, 5.500000000000030198, 87.89357721762581832 ) ) ;
#69078=CARTESIAN_POINT ( 'NONE',  ( -5.719274019375978568, 21.55341960407610458, 90.20724293864770971 ) ) ;
#69079=CARTESIAN_POINT ( 'NONE',  ( 0.05219959533907565091, 21.53943276465977519, 104.9989096053143669 ) ) ;
#69080=CARTESIAN_POINT ( 'NONE',  ( 12.06949235617757843, -12.14591786802309237, 38.12390960531436690 ) ) ;
#69081=CARTESIAN_POINT ( 'NONE',  ( -12.06949235617739369, -12.14591786802326823, 29.37609039468568284 ) ) ;
#69082=CARTESIAN_POINT ( 'NONE',  ( -19.05341960407611168, -5.049401038298163336, 41.45724293864769550 ) ) ;
#69083=CARTESIAN_POINT ( 'NONE',  ( -13.89961937509977652, 13.97604488694528158, 65.62390960531436690 ) ) ;
#69084=CARTESIAN_POINT ( 'NONE',  ( 5.719274019375991003, -21.55341960407610458, 27.70724293864769905 ) ) ;
#69085=CARTESIAN_POINT ( 'NONE',  ( -13.89961937509977652, 13.97604488694528158, 115.6239096053143669 ) ) ;
#69086=CARTESIAN_POINT ( 'NONE',  ( 9.474510206698729675, 16.51473224551082808, 107.0844237280190043 ) ) ;
#69087=CARTESIAN_POINT ( 'NONE',  ( 13.97604488694548053, -13.89961937509957401, 50.62609039468566152 ) ) ;
#69088=CARTESIAN_POINT ( 'NONE',  ( -10.72451020669898014, 18.67979575497178502, 90.41557627198103830 ) ) ;
#69089=CARTESIAN_POINT ( 'NONE',  ( 8.224510206698742110, 14.34966873604972548, 107.0844237280190043 ) ) ;
#69090=CARTESIAN_POINT ( 'NONE',  ( -15.80617190586745835, -15.72974639402198527, 46.87390960531435979 ) ) ;
#69091=CARTESIAN_POINT ( 'NONE',  ( -21.55341960407610458, -5.719274019375992779, 86.45724293864770971 ) ) ;
#69092=CARTESIAN_POINT ( 'NONE',  ( 19.05341960407617918, -5.049401038297876454, 111.0427570613523329 ) ) ;
#69093=CARTESIAN_POINT ( 'NONE',  ( -13.89961937509977652, 13.97604488694528158, 100.6239096053143669 ) ) ;
#69094=CARTESIAN_POINT ( 'NONE',  ( -15.80617190586768217, 15.72974639402176855, 78.12609039468570415 ) ) ;
#69095=CARTESIAN_POINT ( 'NONE',  ( -16.51473224551069308, -9.474510206698971260, 71.66557627198102409 ) ) ;
#69097=CARTESIAN_POINT ( 'NONE',  ( -13.89961937509977652, 13.97604488694528158, 70.62390960531432427 ) ) ;
#69098=CARTESIAN_POINT ( 'NONE',  ( 16.55341960407611168, 4.379528057220329451, 88.95724293864769550 ) ) ;
#69100=CARTESIAN_POINT ( 'NONE',  ( 16.51473224551083163, -9.474510206698727899, 110.8344237280190043 ) ) ;
#69102=CARTESIAN_POINT ( 'NONE',  ( 16.19135201231366494, -7.376712067591922661, 82.31319145947968252 ) ) ;
#69103=CARTESIAN_POINT ( 'NONE',  ( 16.51473224551069308, 9.474510206698969483, 69.16557627198102409 ) ) ;
#69104=CARTESIAN_POINT ( 'NONE',  ( -18.67979575497193778, 10.72451020669871902, 88.33442372801901854 ) ) ;
#69105=CARTESIAN_POINT ( 'NONE',  ( -16.51473224551069308, -9.474510206698971260, 106.6655762719810383 ) ) ;
#69106=CARTESIAN_POINT ( 'NONE',  ( 16.55341960407618274, -4.379528057220086978, 76.04275706135237556 ) ) ;
#69108=CARTESIAN_POINT ( 'NONE',  ( 9.564922557961047289, -16.46253265017146816, 50.41775706135233293 ) ) ;
#69109=CARTESIAN_POINT ( 'NONE',  ( -10.81492255796105439, 18.62759615963255655, 107.9177570613523471 ) ) ;
#69113=CARTESIAN_POINT ( 'NONE',  ( 0.05219959533934541429, -16.53943276465976808, 110.0010903946856757 ) ) ;
#69115=CARTESIAN_POINT ( 'NONE',  ( 14.29746914071037800, 8.314922557961029526, 91.66775706135234714 ) ) ;
#69117=CARTESIAN_POINT ( 'NONE',  ( 14.29746914071037800, 8.314922557961029526, 66.66775706135234714 ) ) ;
#69118=CARTESIAN_POINT ( 'NONE',  ( -5.823673210054431948, 21.52544592524334988, 77.70942372801900433 ) ) ;
#69119=CARTESIAN_POINT ( 'NONE',  ( 19.02544592524334988, 5.153800228976608722, 86.45942372801900433 ) ) ;
#69120=CARTESIAN_POINT ( 'NONE',  ( 16.51473224551083163, -9.474510206698727899, 35.83442372801899722 ) ) ;
#69121=CARTESIAN_POINT ( 'NONE',  ( -5.049401038298153566, 19.05341960407611168, 65.20724293864765286 ) ) ;
#69122=CARTESIAN_POINT ( 'NONE',  ( -19.02544592524342804, 5.153800228976336051, 56.04057627198100988 ) ) ;
#69123=CARTESIAN_POINT ( 'NONE',  ( -9.564922557960796823, -16.46253265017161027, 87.08224293864769550 ) ) ;
#69124=CARTESIAN_POINT ( 'NONE',  ( -10.72451020669898014, 18.67979575497178502, 85.41557627198102409 ) ) ;
#69126=CARTESIAN_POINT ( 'NONE',  ( -10.81492255796078084, -18.62759615963271287, 52.08224293864768839 ) ) ;
#69127=CARTESIAN_POINT ( 'NONE',  ( -19.05341960407611168, -5.049401038298163336, 31.45724293864769550 ) ) ;
#69128=CARTESIAN_POINT ( 'NONE',  ( 16.53943276465976808, 0.05219959533934440121, 66.25109039468567573 ) ) ;
#69130=CARTESIAN_POINT ( 'NONE',  ( -10.81492255796105439, 18.62759615963255655, 47.91775706135234714 ) ) ;
#69131=CARTESIAN_POINT ( 'NONE',  ( -4.483927247898539470, -16.52544592524342804, 62.29057627198102409 ) ) ;
#69133=CARTESIAN_POINT ( 'NONE',  ( -0.05219959533934338120, 16.53943276465976808, 37.50109039468568284 ) ) ;
#69134=CARTESIAN_POINT ( 'NONE',  ( 0.05219959533910956823, 16.53943276465976808, 104.9989096053143669 ) ) ;
#69135=CARTESIAN_POINT ( 'NONE',  ( -19.05341960407617563, 5.049401038297882671, 58.54275706135234003 ) ) ;
#69136=CARTESIAN_POINT ( 'NONE',  ( 12.14591786802309770, 12.06949235617756955, 54.37390960531435979 ) ) ;
#69137=CARTESIAN_POINT ( 'NONE',  ( -15.80617190586768217, 15.72974639402176855, 38.12609039468567573 ) ) ;
#69138=CARTESIAN_POINT ( 'NONE',  ( 13.97604488694527802, 13.89961937509977652, 24.37390960531435624 ) ) ;
#69139=CARTESIAN_POINT ( 'NONE',  ( 10.72451020669898902, -18.67979575497178502, 92.91557627198103830 ) ) ;
#69140=CARTESIAN_POINT ( 'NONE',  ( 9.474510206698971260, -16.51473224551069308, 97.91557627198102409 ) ) ;
#69141=CARTESIAN_POINT ( 'NONE',  ( 4.483927247898545687, 16.52544592524342804, 79.79057627198102409 ) ) ;
#69142=CARTESIAN_POINT ( 'NONE',  ( -5.153800228976328057, -19.02544592524343514, 112.2905762719810099 ) ) ;
#69144=CARTESIAN_POINT ( 'NONE',  ( -13.89961937509957401, -13.97604488694547875, 79.37609039468567573 ) ) ;
#69145=CARTESIAN_POINT ( 'NONE',  ( -15.72974639402176322, -15.80617190586768395, 24.37609039468567573 ) ) ;
#69146=CARTESIAN_POINT ( 'NONE',  ( 5.153800228976335163, 19.02544592524342804, 64.79057627198100988 ) ) ;
#69147=CARTESIAN_POINT ( 'NONE',  ( -13.97604488694547697, 13.89961937509957934, 63.12609039468566152 ) ) ;
#69148=CARTESIAN_POINT ( 'NONE',  ( 19.05341960407611168, 5.049401038298154454, 28.95724293864769550 ) ) ;
#69150=CARTESIAN_POINT ( 'NONE',  ( 21.55341960407619695, -5.719274019375665929, 66.04275706135236135 ) ) ;
#69151=CARTESIAN_POINT ( 'NONE',  ( -16.31925111598454947, -7.325300261831595883, 69.83575461032751264 ) ) ;
#69152=CARTESIAN_POINT ( 'NONE',  ( -4.483927247898539470, -16.52544592524342804, 52.29057627198102409 ) ) ;
#69153=CARTESIAN_POINT ( 'NONE',  ( 0.05219959533909260263, 19.03943276465977164, 59.99890960531436690 ) ) ;
#69154=CARTESIAN_POINT ( 'NONE',  ( -21.55341960407610458, -5.719274019375992779, 86.45724293864770971 ) ) ;
#69155=CARTESIAN_POINT ( 'NONE',  ( 16.46253265017160672, -9.564922557960803928, 63.33224293864769550 ) ) ;
#69156=ORIENTED_EDGE ( 'NONE', *, *, #22880, .F. ) ;
#69157=CARTESIAN_POINT ( 'NONE',  ( 21.53943276465977519, -0.05219959533907433946, 78.74890960531436690 ) ) ;
#69158=CARTESIAN_POINT ( 'NONE',  ( 18.67979575497194134, -10.72451020669871369, 95.83442372801903275 ) ) ;
#69159=CARTESIAN_POINT ( 'NONE',  ( -16.51473224551069308, -9.474510206698971260, 21.66557627198102765 ) ) ;
#69160=CARTESIAN_POINT ( 'NONE',  ( 4.379528057220092307, 16.55341960407617563, 97.29275706135234714 ) ) ;
#69161=CARTESIAN_POINT ( 'NONE',  ( 4.379528057220339221, -16.55341960407611168, 97.70724293864772392 ) ) ;
#69162=CARTESIAN_POINT ( 'NONE',  ( 9.474510206698729675, 16.51473224551082808, 87.08442372801900433 ) ) ;
#69164=CARTESIAN_POINT ( 'NONE',  ( -15.72974639402176322, -15.80617190586768395, 24.37609039468567573 ) ) ;
#69165=CARTESIAN_POINT ( 'NONE',  ( 19.03943276465977164, 0.05219959533936151252, 46.25109039468566863 ) ) ;
#69166=CARTESIAN_POINT ( 'NONE',  ( -12.14591786802326823, 12.06949235617739902, 103.1260903946856757 ) ) ;
#69167=CARTESIAN_POINT ( 'NONE',  ( 16.51473224551083163, -9.474510206698727899, 35.83442372801899722 ) ) ;
#69168=CARTESIAN_POINT ( 'NONE',  ( 19.03943276465977164, -0.05219959533909143690, 98.74890960531436690 ) ) ;
#69169=CARTESIAN_POINT ( 'NONE',  ( 10.72451020669898902, -18.67979575497178502, 62.91557627198102409 ) ) ;
#69171=CARTESIAN_POINT ( 'NONE',  ( 13.97604488694527802, 13.89961937509977652, 24.37390960531435624 ) ) ;
#69172=EDGE_CURVE ( 'NONE', #63497, #71844, #108895, .T. ) ;
#69173=CARTESIAN_POINT ( 'NONE',  ( -19.02544592524334988, -5.153800228976617603, 18.95942372801899722 ) ) ;
#69174=CARTESIAN_POINT ( 'NONE',  ( 16.55341960407618274, -4.379528057220086978, 71.04275706135234714 ) ) ;
#69175=CARTESIAN_POINT ( 'NONE',  ( 15.72974639402176855, 15.80617190586768217, 31.87609039468567929 ) ) ;
#69176=CARTESIAN_POINT ( 'NONE',  ( 4.483927247898790824, -16.52544592524335698, 35.20942372801901854 ) ) ;
#69177=CARTESIAN_POINT ( 'NONE',  ( 19.03943276465977164, -0.05219959533909143690, 103.7489096053143669 ) ) ;
#69178=CARTESIAN_POINT ( 'NONE',  ( -5.153800228976328057, -19.02544592524343514, 42.29057627198101699 ) ) ;
#69179=CARTESIAN_POINT ( 'NONE',  ( -5.153800228976328057, -19.02544592524343514, 72.29057627198102409 ) ) ;
#69180=CARTESIAN_POINT ( 'NONE',  ( -12.14591786802326823, 12.06949235617739902, 48.12609039468568284 ) ) ;
#69181=CARTESIAN_POINT ( 'NONE',  ( -4.483927247898539470, -16.52544592524342804, 87.29057627198103830 ) ) ;
#69182=CARTESIAN_POINT ( 'NONE',  ( 16.53943276465976808, 0.05219959533934440121, 96.25109039468568994 ) ) ;
#69183=CARTESIAN_POINT ( 'NONE',  ( 21.55341960407619695, -5.719274019375665929, 56.04275706135235424 ) ) ;
#69184=CARTESIAN_POINT ( 'NONE',  ( -19.02544592524342804, 5.153800228976336051, 76.04057627198102409 ) ) ;
#69185=CARTESIAN_POINT ( 'NONE',  ( 19.03943276465977164, -0.05219959533909143690, 58.74890960531435979 ) ) ;
#69186=CARTESIAN_POINT ( 'NONE',  ( -19.02544592524342804, 5.153800228976336051, 91.04057627198100988 ) ) ;
#69187=CARTESIAN_POINT ( 'NONE',  ( 16.52544592524342804, -4.483927247898539470, 43.54057627198103830 ) ) ;
#69188=CARTESIAN_POINT ( 'NONE',  ( -16.55341960407617563, 4.379528057220093196, 93.54275706135234714 ) ) ;
#69190=CARTESIAN_POINT ( 'NONE',  ( 13.97604488694548053, -13.89961937509957401, 50.62609039468566152 ) ) ;
#69191=CARTESIAN_POINT ( 'NONE',  ( 5.153800228976335163, 19.02544592524342804, 114.7905762719810241 ) ) ;
#69192=CARTESIAN_POINT ( 'NONE',  ( 13.89961937509977652, -13.97604488694527269, 63.12390960531435979 ) ) ;
#69193=CARTESIAN_POINT ( 'NONE',  ( -19.05341960407617563, 5.049401038297882671, 33.54275706135231871 ) ) ;
#69195=CARTESIAN_POINT ( 'NONE',  ( 19.25663599770061651, -5.499999999999440448, 71.49419308057203182 ) ) ;
#69196=CARTESIAN_POINT ( 'NONE',  ( 14.29746914071037800, 8.314922557961029526, 51.66775706135234714 ) ) ;
#69197=CARTESIAN_POINT ( 'NONE',  ( -0.05219959533936034679, 19.03943276465977164, 77.50109039468566152 ) ) ;
#69198=CARTESIAN_POINT ( 'NONE',  ( -16.52544592524335698, -4.483927247898792601, 73.95942372801901854 ) ) ;
#69199=CARTESIAN_POINT ( 'NONE',  ( 17.44270441346517231, 5.991230190323027394, 93.86335079264232206 ) ) ;
#69200=CARTESIAN_POINT ( 'NONE',  ( 13.97604488694527802, 13.89961937509977652, 84.37390960531433848 ) ) ;
#69201=CARTESIAN_POINT ( 'NONE',  ( 21.55341960407619695, -5.719274019375665929, 31.04275706135234714 ) ) ;
#69202=CARTESIAN_POINT ( 'NONE',  ( 9.474510206698729675, 16.51473224551082808, 82.08442372801899012 ) ) ;
#69203=CARTESIAN_POINT ( 'NONE',  ( 16.31925111598457434, 7.325300261831476867, 87.33575461032751264 ) ) ;
#69204=CARTESIAN_POINT ( 'NONE',  ( 9.564922557960805705, 16.46253265017160317, 39.58224293864768839 ) ) ;
#69205=CARTESIAN_POINT ( 'NONE',  ( -19.05341960407611168, -5.049401038298163336, 96.45724293864769550 ) ) ;
#69206=CARTESIAN_POINT ( 'NONE',  ( 8.224510206698953496, -14.34966873604960469, 42.91557627198103120 ) ) ;
#69207=CARTESIAN_POINT ( 'NONE',  ( -9.564922557960796823, -16.46253265017161027, 42.08224293864769550 ) ) ;
#69208=CARTESIAN_POINT ( 'NONE',  ( -16.46253265017146816, -9.564922557961047289, 49.16775706135233293 ) ) ;
#69209=CARTESIAN_POINT ( 'NONE',  ( 8.224510206698953496, -14.34966873604960469, 82.91557627198103830 ) ) ;
#69210=CARTESIAN_POINT ( 'NONE',  ( 16.51473224551083163, -9.474510206698727899, 20.83442372801899722 ) ) ;
#69211=CARTESIAN_POINT ( 'NONE',  ( 5.049401038298161559, -19.05341960407611168, 52.70724293864767418 ) ) ;
#69213=CARTESIAN_POINT ( 'NONE',  ( 18.67979575497178502, 10.72451020669898547, 59.16557627198103120 ) ) ;
#69214=CARTESIAN_POINT ( 'NONE',  ( 0.05219959533910956823, 16.53943276465976808, 54.99890960531435269 ) ) ;
#69215=CARTESIAN_POINT ( 'NONE',  ( 19.05341960407617918, -5.049401038297876454, 21.04275706135232582 ) ) ;
#69216=CARTESIAN_POINT ( 'NONE',  ( 16.51473224551069308, 9.474510206698969483, 104.1655762719810241 ) ) ;
#69217=CARTESIAN_POINT ( 'NONE',  ( 13.89961937509977652, -13.97604488694527269, 113.1239096053143527 ) ) ;
#69218=CARTESIAN_POINT ( 'NONE',  ( 13.97604488694527802, 13.89961937509977652, 49.37390960531434558 ) ) ;
#69219=CARTESIAN_POINT ( 'NONE',  ( 19.05341960407611168, 5.049401038298154454, 23.95724293864769194 ) ) ;
#69220=CARTESIAN_POINT ( 'NONE',  ( 14.34966873604960469, 8.224510206698951720, 94.16557627198103830 ) ) ;
#69221=CARTESIAN_POINT ( 'NONE',  ( -0.05219959533907301413, -21.53943276465977519, 102.4989096053143811 ) ) ;
#69222=CARTESIAN_POINT ( 'NONE',  ( -19.05341960407611168, -5.049401038298163336, 106.4572429386476955 ) ) ;
#69223=CARTESIAN_POINT ( 'NONE',  ( 10.81492255796078972, 18.62759615963270932, 114.5822429386477097 ) ) ;
#69224=CARTESIAN_POINT ( 'NONE',  ( -0.05219959533909027116, -19.03943276465977164, 102.4989096053143669 ) ) ;
#69225=CARTESIAN_POINT ( 'NONE',  ( -5.153800228976328057, -19.02544592524343514, 22.29057627198102765 ) ) ;
#69226=CARTESIAN_POINT ( 'NONE',  ( -18.62759615963255300, -10.81492255796106328, 79.16775706135234714 ) ) ;
#69227=CARTESIAN_POINT ( 'NONE',  ( -18.67979575497178146, -10.72451020669898902, 91.66557627198103830 ) ) ;
#69228=EDGE_CURVE ( 'NONE', #33312, #61533, #2711, .T. ) ;
#69230=CARTESIAN_POINT ( 'NONE',  ( -16.51473224551069308, -9.474510206698971260, 51.66557627198102409 ) ) ;
#69232=CARTESIAN_POINT ( 'NONE',  ( 8.314922557961029526, -14.29746914071037800, 35.41775706135234003 ) ) ;
#69233=CARTESIAN_POINT ( 'NONE',  ( 8.314922557960818139, 14.29746914071049879, 104.5822429386477097 ) ) ;
#69234=VECTOR ( 'NONE', #90097, 1000.000000000000000 ) ;
#69235=CARTESIAN_POINT ( 'NONE',  ( -17.50000000000013500, -3.292511757969763586, 109.9347972978946331 ) ) ;
#69236=CARTESIAN_POINT ( 'NONE',  ( 13.97604488694527802, 13.89961937509977652, 59.37390960531434558 ) ) ;
#69237=CARTESIAN_POINT ( 'NONE',  ( 12.06949235617757843, -12.14591786802309237, 93.12390960531436690 ) ) ;
#69238=CARTESIAN_POINT ( 'NONE',  ( 18.67979575497178502, 10.72451020669898547, 39.16557627198102409 ) ) ;
#69239=CARTESIAN_POINT ( 'NONE',  ( -14.29746914071049879, 8.314922557960819915, 65.83224293864769550 ) ) ;
#69240=CARTESIAN_POINT ( 'NONE',  ( 0.05219959533934541429, -16.53943276465976808, 20.00109039468568639 ) ) ;
#69241=CARTESIAN_POINT ( 'NONE',  ( 10.72451020669871369, 18.67979575497193778, 67.08442372801901854 ) ) ;
#69243=CARTESIAN_POINT ( 'NONE',  ( 9.474510206698971260, -16.51473224551069308, 107.9155762719810383 ) ) ;
#69244=CARTESIAN_POINT ( 'NONE',  ( 4.483927247898790824, -16.52544592524335698, 100.2094237280190043 ) ) ;
#69245=CARTESIAN_POINT ( 'NONE',  ( -0.05219959533909027116, -19.03943276465977164, 42.49890960531435269 ) ) ;
#69246=CARTESIAN_POINT ( 'NONE',  ( -13.89961937509977652, 13.97604488694528158, 85.62390960531433848 ) ) ;
#69247=CARTESIAN_POINT ( 'NONE',  ( -5.823673210054116645, -21.52544592524344225, 92.29057627198103830 ) ) ;
#69248=CARTESIAN_POINT ( 'NONE',  ( -4.379528057220086978, -16.55341960407618274, 19.79275706135235069 ) ) ;
#69249=CARTESIAN_POINT ( 'NONE',  ( -8.224510206698948167, 14.34966873604960824, 60.41557627198102409 ) ) ;
#69250=CARTESIAN_POINT ( 'NONE',  ( -5.823673210054431948, 21.52544592524334988, 67.70942372801901854 ) ) ;
#69251=CARTESIAN_POINT ( 'NONE',  ( 12.06949235617739724, 12.14591786802326823, 101.8760903946857042 ) ) ;
#69252=CARTESIAN_POINT ( 'NONE',  ( 16.38665767535053774, 7.295008042176051255, 27.23599135785455871 ) ) ;
#69254=CARTESIAN_POINT ( 'NONE',  ( -4.379528057220328563, 16.55341960407611168, 25.20724293864769550 ) ) ;
#69255=CARTESIAN_POINT ( 'NONE',  ( -16.53943276465976808, -0.05219959533934237506, 68.75109039468568994 ) ) ;
#69256=CARTESIAN_POINT ( 'NONE',  ( -9.564922557960796823, -16.46253265017161027, 92.08224293864769550 ) ) ;
#69257=CARTESIAN_POINT ( 'NONE',  ( -19.02544592524342804, 5.153800228976336051, 81.04057627198103830 ) ) ;
#69258=CARTESIAN_POINT ( 'NONE',  ( -15.72974639402176322, -15.80617190586768395, 84.37609039468570415 ) ) ;
#69259=CARTESIAN_POINT ( 'NONE',  ( -4.483927247898782831, 16.52544592524335698, 87.70942372801901854 ) ) ;
#69260=CARTESIAN_POINT ( 'NONE',  ( -8.314922557960811034, -14.29746914071050412, 57.08224293864769550 ) ) ;
#69261=CARTESIAN_POINT ( 'NONE',  ( -0.05219959533909027116, -19.03943276465977164, 67.49890960531436690 ) ) ;
#69263=CARTESIAN_POINT ( 'NONE',  ( -9.564922557961040184, 16.46253265017147172, 112.9177570613523329 ) ) ;
#69264=CARTESIAN_POINT ( 'NONE',  ( 0.05219959533910956823, 16.53943276465976808, 114.9989096053143669 ) ) ;
#69265=CARTESIAN_POINT ( 'NONE',  ( 13.89961937509977652, -13.97604488694527269, 78.12390960531433848 ) ) ;
#69266=CARTESIAN_POINT ( 'NONE',  ( -13.97604488694547697, 13.89961937509957934, 108.1260903946856331 ) ) ;
#69268=CARTESIAN_POINT ( 'NONE',  ( -19.05341960407617563, 5.049401038297882671, 28.54275706135232937 ) ) ;
#69269=CARTESIAN_POINT ( 'NONE',  ( 8.314922557961029526, -14.29746914071037800, 80.41775706135234714 ) ) ;
#69270=CARTESIAN_POINT ( 'NONE',  ( -19.03943276465977164, -0.05219959533935918106, 88.75109039468567573 ) ) ;
#69271=CARTESIAN_POINT ( 'NONE',  ( 0.05219959533910956823, 16.53943276465976808, 109.9989096053143527 ) ) ;
#69272=CARTESIAN_POINT ( 'NONE',  ( 16.52544592524335698, 4.483927247898782831, 71.45942372801901854 ) ) ;
#69273=CARTESIAN_POINT ( 'NONE',  ( -17.49999999999999645, -5.500000000000000888, 34.20309617465829177 ) ) ;
#69274=CARTESIAN_POINT ( 'NONE',  ( -9.474510206698720793, -16.51473224551083518, 54.58442372801899722 ) ) ;
#69275=CARTESIAN_POINT ( 'NONE',  ( 21.55341960407619695, -5.719274019375665929, 96.04275706135236135 ) ) ;
#69276=CARTESIAN_POINT ( 'NONE',  ( -5.049401038298153566, 19.05341960407611168, 40.20724293864768839 ) ) ;
#69277=CARTESIAN_POINT ( 'NONE',  ( -5.153800228976328057, -19.02544592524343514, 77.29057627198099567 ) ) ;
#69278=CARTESIAN_POINT ( 'NONE',  ( -0.05219959533910754901, -16.53943276465976808, 72.49890960531435269 ) ) ;
#69280=CARTESIAN_POINT ( 'NONE',  ( 5.823673210054444382, -21.52544592524334988, 85.20942372801901854 ) ) ;
#69281=CARTESIAN_POINT ( 'NONE',  ( 5.049401038297881783, 19.05341960407617563, 57.29275706135231871 ) ) ;
#69282=CARTESIAN_POINT ( 'NONE',  ( 13.89961937509957401, 13.97604488694547697, 46.87609039468565442 ) ) ;
#69283=CARTESIAN_POINT ( 'NONE',  ( -10.81492255796078084, -18.62759615963271287, 42.08224293864769550 ) ) ;
#69284=CARTESIAN_POINT ( 'NONE',  ( 21.55341960407619695, -5.719274019375665929, 96.04275706135236135 ) ) ;
#69285=CARTESIAN_POINT ( 'NONE',  ( 9.474510206698971260, -16.51473224551069308, 72.91557627198102409 ) ) ;
#69286=CARTESIAN_POINT ( 'NONE',  ( 10.72451020669871369, 18.67979575497193778, 107.0844237280190043 ) ) ;
#69287=CARTESIAN_POINT ( 'NONE',  ( -21.53943276465977519, 0.05219959533907696930, 56.24890960531436690 ) ) ;
#69288=CARTESIAN_POINT ( 'NONE',  ( 16.46253265017160672, -9.564922557960803928, 103.3322429386476955 ) ) ;
#69289=CARTESIAN_POINT ( 'NONE',  ( -13.89961937509957401, -13.97604488694547875, 69.37609039468564731 ) ) ;
#69290=CARTESIAN_POINT ( 'NONE',  ( 16.46253265017160672, -9.564922557960803928, 103.3322429386476955 ) ) ;
#69291=CARTESIAN_POINT ( 'NONE',  ( 19.03943276465977164, 0.05219959533936151252, 101.2510903946856757 ) ) ;
#69292=CARTESIAN_POINT ( 'NONE',  ( 8.224510206698742110, 14.34966873604972548, 42.08442372801901854 ) ) ;
#69293=CARTESIAN_POINT ( 'NONE',  ( 12.14591786802309770, 12.06949235617756955, 99.37390960531436690 ) ) ;
#69294=CARTESIAN_POINT ( 'NONE',  ( 13.97604488694527802, 13.89961937509977652, 89.37390960531436690 ) ) ;
#69295=CARTESIAN_POINT ( 'NONE',  ( 21.55341960407610458, 5.719274019375980345, 58.95724293864770971 ) ) ;
#69296=CARTESIAN_POINT ( 'NONE',  ( -12.14591786802326823, 12.06949235617739902, 33.12609039468569705 ) ) ;
#69297=CARTESIAN_POINT ( 'NONE',  ( -18.62759615963255300, -10.81492255796106328, 34.16775706135234714 ) ) ;
#69298=CARTESIAN_POINT ( 'NONE',  ( -10.81492255796105439, 18.62759615963255655, 77.91775706135231871 ) ) ;
#69299=CARTESIAN_POINT ( 'NONE',  ( 14.29746914071037800, 8.314922557961029526, 81.66775706135236135 ) ) ;
#69300=CARTESIAN_POINT ( 'NONE',  ( -19.03943276465977164, 0.05219959533909376836, 76.24890960531435269 ) ) ;
#69301=CARTESIAN_POINT ( 'NONE',  ( 12.06949235617757843, -12.14591786802309237, 73.12390960531436690 ) ) ;
#69302=CARTESIAN_POINT ( 'NONE',  ( -8.224510206698735004, -14.34966873604973081, 109.5844237280190328 ) ) ;
#69303=CARTESIAN_POINT ( 'NONE',  ( 16.46253265017146816, 9.564922557961045513, 56.66775706135233293 ) ) ;
#69304=CARTESIAN_POINT ( 'NONE',  ( 0.05219959533937995610, -21.53943276465977519, 30.00109039468568284 ) ) ;
#69305=CARTESIAN_POINT ( 'NONE',  ( -16.52544592524342804, 4.483927247898546575, 81.04057627198102409 ) ) ;
#69306=CARTESIAN_POINT ( 'NONE',  ( -19.02544592524342804, 5.153800228976336051, 106.0405762719810241 ) ) ;
#69307=CARTESIAN_POINT ( 'NONE',  ( 16.55341960407618274, -4.379528057220086978, 106.0427570613523471 ) ) ;
#69308=CARTESIAN_POINT ( 'NONE',  ( -10.72451020669870658, -18.67979575497194134, 69.58442372801900433 ) ) ;
#69309=CARTESIAN_POINT ( 'NONE',  ( -8.224510206698735004, -14.34966873604973081, 49.58442372801901143 ) ) ;
#69310=CARTESIAN_POINT ( 'NONE',  ( -18.62759615963255300, -10.81492255796106328, 44.16775706135234714 ) ) ;
#69311=CARTESIAN_POINT ( 'NONE',  ( -12.14591786802309592, -12.06949235617757132, 66.87390960531436690 ) ) ;
#69313=CARTESIAN_POINT ( 'NONE',  ( -15.72974639402176322, -15.80617190586768395, 19.37609039468568639 ) ) ;
#69314=CARTESIAN_POINT ( 'NONE',  ( -16.55341960407611168, -4.379528057220339221, 91.45724293864769550 ) ) ;
#69315=CARTESIAN_POINT ( 'NONE',  ( -19.49671883438229258, -5.499999999999982236, 49.89279849105685116 ) ) ;
#69316=CARTESIAN_POINT ( 'NONE',  ( -16.55341960407611168, -4.379528057220339221, 46.45724293864769550 ) ) ;
#69317=CARTESIAN_POINT ( 'NONE',  ( -19.05341960407611168, -5.049401038298163336, 26.45724293864769550 ) ) ;
#69318=CARTESIAN_POINT ( 'NONE',  ( -21.55341960407610458, -5.719274019375992779, 41.45724293864769550 ) ) ;
#69319=CARTESIAN_POINT ( 'NONE',  ( 8.224510206698953496, -14.34966873604960469, 82.91557627198103830 ) ) ;
#69320=CARTESIAN_POINT ( 'NONE',  ( 15.72974639402199770, -15.80617190586745480, 83.12390960531436690 ) ) ;
#69321=CARTESIAN_POINT ( 'NONE',  ( 9.564922557960805705, 16.46253265017160317, 84.58224293864769550 ) ) ;
#69322=CARTESIAN_POINT ( 'NONE',  ( 16.46253265017160672, -9.564922557960803928, 43.33224293864769550 ) ) ;
#69323=CARTESIAN_POINT ( 'NONE',  ( -9.474510206698720793, -16.51473224551083518, 74.58442372801900433 ) ) ;
#69324=CARTESIAN_POINT ( 'NONE',  ( -18.67979575497193778, 10.72451020669871902, 58.33442372801901143 ) ) ;
#69325=CARTESIAN_POINT ( 'NONE',  ( -5.823673210054116645, -21.52544592524344225, 62.29057627198102409 ) ) ;
#69326=CARTESIAN_POINT ( 'NONE',  ( -16.46253265017160317, 9.564922557960807481, 40.83224293864769550 ) ) ;
#69327=CARTESIAN_POINT ( 'NONE',  ( -5.049401038298153566, 19.05341960407611168, 70.20724293864769550 ) ) ;
#69329=CARTESIAN_POINT ( 'NONE',  ( 14.29746914071037800, 8.314922557961029526, 51.66775706135234714 ) ) ;
#69330=CARTESIAN_POINT ( 'NONE',  ( -0.05219959533937732626, 21.53943276465977519, 32.50109039468568284 ) ) ;
#69331=CARTESIAN_POINT ( 'NONE',  ( -15.72974639402176322, -15.80617190586768395, 74.37609039468568994 ) ) ;
#69332=CARTESIAN_POINT ( 'NONE',  ( 21.52544592524344225, -5.823673210054117533, 28.54057627198103120 ) ) ;
#69333=CARTESIAN_POINT ( 'NONE',  ( -10.72451020669898014, 18.67979575497178502, 80.41557627198103830 ) ) ;
#69334=CARTESIAN_POINT ( 'NONE',  ( -10.72451020669870658, -18.67979575497194134, 19.58442372801901143 ) ) ;
#69335=CARTESIAN_POINT ( 'NONE',  ( 12.14591786802327356, -12.06949235617739191, 50.62609039468568994 ) ) ;
#69336=CARTESIAN_POINT ( 'NONE',  ( -18.62759615963270932, 10.81492255796079327, 45.83224293864769550 ) ) ;
#69337=CARTESIAN_POINT ( 'NONE',  ( 0.05219959533937995610, -21.53943276465977519, 110.0010903946856757 ) ) ;
#69338=CARTESIAN_POINT ( 'NONE',  ( -5.153800228976328057, -19.02544592524343514, 52.29057627198100988 ) ) ;
#69339=CARTESIAN_POINT ( 'NONE',  ( -13.89961937509977652, 13.97604488694528158, 115.6239096053143669 ) ) ;
#69340=CARTESIAN_POINT ( 'NONE',  ( 9.564922557960805705, 16.46253265017160317, 94.58224293864769550 ) ) ;
#69342=CARTESIAN_POINT ( 'NONE',  ( -13.89961937509957401, -13.97604488694547875, 74.37609039468566152 ) ) ;
#69343=CARTESIAN_POINT ( 'NONE',  ( -18.67979575497178146, -10.72451020669898902, 46.66557627198102409 ) ) ;
#69344=CARTESIAN_POINT ( 'NONE',  ( -4.483927247898539470, -16.52544592524342804, 27.29057627198103120 ) ) ;
#69345=CARTESIAN_POINT ( 'NONE',  ( -9.564922557961040184, 16.46253265017147172, 102.9177570613523329 ) ) ;
#69346=CARTESIAN_POINT ( 'NONE',  ( 17.60769864724392875, -5.499999999999830358, 51.15024842019163742 ) ) ;
#69347=CARTESIAN_POINT ( 'NONE',  ( -19.03943276465977164, -0.05219959533935918106, 18.75109039468567218 ) ) ;
#69348=CARTESIAN_POINT ( 'NONE',  ( -9.564922557961040184, 16.46253265017147172, 92.91775706135233293 ) ) ;
#69349=CARTESIAN_POINT ( 'NONE',  ( -21.55341960407610458, -5.719274019375992779, 81.45724293864769550 ) ) ;
#69350=CARTESIAN_POINT ( 'NONE',  ( 13.89961937509957401, 13.97604488694547697, 56.87609039468564731 ) ) ;
#69351=CARTESIAN_POINT ( 'NONE',  ( 18.22780087662126647, 5.499999999999818812, 51.48236817873107896 ) ) ;
#69352=CARTESIAN_POINT ( 'NONE',  ( -13.97604488694527625, -13.89961937509977652, 56.87390960531434558 ) ) ;
#69353=CARTESIAN_POINT ( 'NONE',  ( 16.55341960407611168, 4.379528057220329451, 68.95724293864769550 ) ) ;
#69354=CARTESIAN_POINT ( 'NONE',  ( -0.05219959533909027116, -19.03943276465977164, 37.49890960531436690 ) ) ;
#69355=CARTESIAN_POINT ( 'NONE',  ( -8.314922557960811034, -14.29746914071050412, 37.08224293864768129 ) ) ;
#69357=CARTESIAN_POINT ( 'NONE',  ( -16.52544592524335698, -4.483927247898792601, 108.9594237280190185 ) ) ;
#69358=CARTESIAN_POINT ( 'NONE',  ( 13.89961937509977652, -13.97604488694527269, 58.12390960531436690 ) ) ;
#69359=CARTESIAN_POINT ( 'NONE',  ( -5.049401038297874678, -19.05341960407617918, 24.79275706135233648 ) ) ;
#69360=CARTESIAN_POINT ( 'NONE',  ( -12.14591786802326823, 12.06949235617739902, 38.12609039468567573 ) ) ;
#69361=CARTESIAN_POINT ( 'NONE',  ( -10.72451020669898014, 18.67979575497178502, 55.41557627198102409 ) ) ;
#69362=CARTESIAN_POINT ( 'NONE',  ( -5.823673210054431948, 21.52544592524334988, 102.7094237280190185 ) ) ;
#69363=ORIENTED_EDGE ( 'NONE', *, *, #25526, .T. ) ;
#69364=CARTESIAN_POINT ( 'NONE',  ( -13.97604488694527625, -13.89961937509977652, 56.87390960531434558 ) ) ;
#69365=CARTESIAN_POINT ( 'NONE',  ( 13.97604488694527802, 13.89961937509977652, 114.3739096053143669 ) ) ;
#69366=CARTESIAN_POINT ( 'NONE',  ( -19.03943276465977164, 0.05219959533909376836, 96.24890960531436690 ) ) ;
#69368=CARTESIAN_POINT ( 'NONE',  ( 21.53943276465977519, 0.05219959533937863772, 21.25109039468567218 ) ) ;
#69369=CARTESIAN_POINT ( 'NONE',  ( -4.379528057220328563, 16.55341960407611168, 95.20724293864769550 ) ) ;
#69370=CARTESIAN_POINT ( 'NONE',  ( -10.81492255796078084, -18.62759615963271287, 87.08224293864769550 ) ) ;
#69371=CARTESIAN_POINT ( 'NONE',  ( 5.153800228976335163, 19.02544592524342804, 64.79057627198100988 ) ) ;
#69372=CARTESIAN_POINT ( 'NONE',  ( 19.02544592524343514, -5.153800228976328945, 68.54057627198103830 ) ) ;
#69373=CARTESIAN_POINT ( 'NONE',  ( 18.67979575497178502, 10.72451020669898547, 114.1655762719810383 ) ) ;
#69374=ORIENTED_EDGE ( 'NONE', *, *, #148621, .T. ) ;
#69375=CARTESIAN_POINT ( 'NONE',  ( 13.89961937509977652, -13.97604488694527269, 73.12390960531436690 ) ) ;
#69377=CARTESIAN_POINT ( 'NONE',  ( 0.05219959533910956823, 16.53943276465976808, 104.9989096053143669 ) ) ;
#69378=CARTESIAN_POINT ( 'NONE',  ( 9.474510206698971260, -16.51473224551069308, 22.91557627198102765 ) ) ;
#69379=CARTESIAN_POINT ( 'NONE',  ( -13.89961937509957401, -13.97604488694547875, 99.37609039468567573 ) ) ;
#69381=CARTESIAN_POINT ( 'NONE',  ( 12.14591786802309770, 12.06949235617756955, 94.37390960531436690 ) ) ;
#69382=CARTESIAN_POINT ( 'NONE',  ( 21.55341960407619695, -5.719274019375665929, 76.04275706135237556 ) ) ;
#69383=CARTESIAN_POINT ( 'NONE',  ( 16.51473224551069308, 9.474510206698969483, 59.16557627198102409 ) ) ;
#69384=CARTESIAN_POINT ( 'NONE',  ( 5.719274019375673035, 21.55341960407619339, 32.29275706135235424 ) ) ;
#69385=CARTESIAN_POINT ( 'NONE',  ( -10.81492255796078084, -18.62759615963271287, 112.0822429386477097 ) ) ;
#69387=CARTESIAN_POINT ( 'NONE',  ( 13.97604488694527802, 13.89961937509977652, 74.37390960531436690 ) ) ;
#69389=CARTESIAN_POINT ( 'NONE',  ( -14.29746914071037622, -8.314922557961029526, 24.16775706135235424 ) ) ;
#69390=CARTESIAN_POINT ( 'NONE',  ( 18.67979575497178502, 10.72451020669898547, 24.16557627198103120 ) ) ;
#69391=CARTESIAN_POINT ( 'NONE',  ( 15.72974639402176855, 15.80617190586768217, 66.87609039468568994 ) ) ;
#69393=CARTESIAN_POINT ( 'NONE',  ( -5.049401038298153566, 19.05341960407611168, 105.2072429386476671 ) ) ;
#69394=CARTESIAN_POINT ( 'NONE',  ( -19.02544592524334988, -5.153800228976617603, 98.95942372801900433 ) ) ;
#69395=CARTESIAN_POINT ( 'NONE',  ( -9.474510206698964154, 16.51473224551069663, 45.41557627198103120 ) ) ;
#69396=CARTESIAN_POINT ( 'NONE',  ( 5.049401038298161559, -19.05341960407611168, 72.70724293864768129 ) ) ;
#69398=CARTESIAN_POINT ( 'NONE',  ( -14.29746914071049879, 8.314922557960819915, 95.83224293864770971 ) ) ;
#69399=CARTESIAN_POINT ( 'NONE',  ( 16.51473224551069308, 9.474510206698969483, 99.16557627198102409 ) ) ;
#69400=CARTESIAN_POINT ( 'NONE',  ( -14.29746914071049879, 8.314922557960819915, 90.83224293864769550 ) ) ;
#69401=CARTESIAN_POINT ( 'NONE',  ( 13.89961937509977652, -13.97604488694527269, 103.1239096053143527 ) ) ;
#69402=CARTESIAN_POINT ( 'NONE',  ( 14.29746914071049879, -8.314922557960816363, 48.33224293864770260 ) ) ;
#69404=CARTESIAN_POINT ( 'NONE',  ( -13.89961937509977652, 13.97604488694528158, 45.62390960531433848 ) ) ;
#69405=CARTESIAN_POINT ( 'NONE',  ( -5.823673210054431948, 21.52544592524334988, 62.70942372801902565 ) ) ;
#69406=CARTESIAN_POINT ( 'NONE',  ( 19.02544592524334988, 5.153800228976608722, 96.45942372801897591 ) ) ;
#69407=CARTESIAN_POINT ( 'NONE',  ( 0.05219959533910956823, 16.53943276465976808, 44.99890960531435979 ) ) ;
#69408=CARTESIAN_POINT ( 'NONE',  ( -5.823673210054116645, -21.52544592524344225, 102.2905762719810383 ) ) ;
#69409=CARTESIAN_POINT ( 'NONE',  ( 15.72974639402199770, -15.80617190586745480, 48.12390960531436690 ) ) ;
#69410=CARTESIAN_POINT ( 'NONE',  ( -13.89961937509977652, 13.97604488694528158, 110.6239096053143243 ) ) ;
#69411=CARTESIAN_POINT ( 'NONE',  ( 16.52544592524342804, -4.483927247898539470, 83.54057627198102409 ) ) ;
#69412=CARTESIAN_POINT ( 'NONE',  ( -16.51473224551069308, -9.474510206698971260, 56.66557627198103120 ) ) ;
#69413=CARTESIAN_POINT ( 'NONE',  ( 4.379528057220339221, -16.55341960407611168, 27.70724293864769905 ) ) ;
#69414=CARTESIAN_POINT ( 'NONE',  ( 0.05219959533934541429, -16.53943276465976808, 105.0010903946856757 ) ) ;
#69415=CARTESIAN_POINT ( 'NONE',  ( -14.29746914071037622, -8.314922557961029526, 84.16775706135234714 ) ) ;
#69416=CARTESIAN_POINT ( 'NONE',  ( -13.97604488694547697, 13.89961937509957934, 38.12609039468566152 ) ) ;
#69418=CARTESIAN_POINT ( 'NONE',  ( 9.564922557960805705, 16.46253265017160317, 104.5822429386476955 ) ) ;
#69419=CARTESIAN_POINT ( 'NONE',  ( 19.02544592524343514, -5.153800228976328945, 73.54057627198103830 ) ) ;
#69420=CARTESIAN_POINT ( 'NONE',  ( 13.97604488694527802, 13.89961937509977652, 34.37390960531436690 ) ) ;
#69421=CARTESIAN_POINT ( 'NONE',  ( -8.314922557960811034, -14.29746914071050412, 42.08224293864769550 ) ) ;
#69422=CARTESIAN_POINT ( 'NONE',  ( 19.05341960407611168, 5.049401038298154454, 113.9572429386477097 ) ) ;
#69423=CARTESIAN_POINT ( 'NONE',  ( -9.564922557960796823, -16.46253265017161027, 102.0822429386477097 ) ) ;
#69424=CARTESIAN_POINT ( 'NONE',  ( -21.52544592524343514, 5.823673210054127303, 46.04057627198103830 ) ) ;
#69425=CARTESIAN_POINT ( 'NONE',  ( -12.14591786802309592, -12.06949235617757132, 86.87390960531438111 ) ) ;
#69426=CARTESIAN_POINT ( 'NONE',  ( -12.14591786802326823, 12.06949235617739902, 38.12609039468567573 ) ) ;
#69427=CARTESIAN_POINT ( 'NONE',  ( 4.483927247898545687, 16.52544592524342804, 59.79057627198103120 ) ) ;
#69429=CARTESIAN_POINT ( 'NONE',  ( 13.97604488694548053, -13.89961937509957401, 60.62609039468564731 ) ) ;
#69430=CARTESIAN_POINT ( 'NONE',  ( 19.02544592524343514, -5.153800228976328945, 98.54057627198100988 ) ) ;
#69431=CARTESIAN_POINT ( 'NONE',  ( -0.05219959533936034679, 19.03943276465977164, 72.50109039468566152 ) ) ;
#69432=CARTESIAN_POINT ( 'NONE',  ( 16.51473224551083163, -9.474510206698727899, 95.83442372801900433 ) ) ;
#69433=CARTESIAN_POINT ( 'NONE',  ( 16.55341960407618274, -4.379528057220086978, 31.04275706135234714 ) ) ;
#69434=CARTESIAN_POINT ( 'NONE',  ( -8.314922557961024197, 14.29746914071037800, 102.9177570613523756 ) ) ;
#69435=CARTESIAN_POINT ( 'NONE',  ( 16.51473224551083163, -9.474510206698727899, 70.83442372801900433 ) ) ;
#69436=CARTESIAN_POINT ( 'NONE',  ( 18.67979575497178502, 10.72451020669898547, 39.16557627198102409 ) ) ;
#69437=CARTESIAN_POINT ( 'NONE',  ( -5.719274019375665041, -21.55341960407619695, 69.79275706135234714 ) ) ;
#69439=CARTESIAN_POINT ( 'NONE',  ( 19.05341960407617918, -5.049401038297876454, 111.0427570613523329 ) ) ;
#69441=CARTESIAN_POINT ( 'NONE',  ( -13.89961937509977652, 13.97604488694528158, 75.62390960531438111 ) ) ;
#69443=CARTESIAN_POINT ( 'NONE',  ( 16.53943276465976808, -0.05219959533910856209, 83.74890960531435269 ) ) ;
#69444=CARTESIAN_POINT ( 'NONE',  ( -0.05219959533909027116, -19.03943276465977164, 72.49890960531435269 ) ) ;
#69446=CARTESIAN_POINT ( 'NONE',  ( 19.03943276465977164, -0.05219959533909143690, 93.74890960531435269 ) ) ;
#69448=CARTESIAN_POINT ( 'NONE',  ( 9.474510206698729675, 16.51473224551082808, 87.08442372801900433 ) ) ;
#69449=CARTESIAN_POINT ( 'NONE',  ( -21.52544592524343514, 5.823673210054127303, 76.04057627198102409 ) ) ;
#69450=CARTESIAN_POINT ( 'NONE',  ( -13.97604488694527625, -13.89961937509977652, 26.87390960531434558 ) ) ;
#69451=CARTESIAN_POINT ( 'NONE',  ( -9.564922557961040184, 16.46253265017147172, 72.91775706135233293 ) ) ;
#69452=CARTESIAN_POINT ( 'NONE',  ( -21.53943276465977519, 0.05219959533907696930, 111.2489096053143669 ) ) ;
#69453=CARTESIAN_POINT ( 'NONE',  ( -5.153800228976328057, -19.02544592524343514, 72.29057627198102409 ) ) ;
#69454=CARTESIAN_POINT ( 'NONE',  ( -9.564922557960796823, -16.46253265017161027, 102.0822429386477097 ) ) ;
#69456=CARTESIAN_POINT ( 'NONE',  ( 15.80617190586746368, 15.72974639402197994, 99.37390960531436690 ) ) ;
#69457=CARTESIAN_POINT ( 'NONE',  ( -4.483927247898539470, -16.52544592524342804, 97.29057627198105251 ) ) ;
#69458=CARTESIAN_POINT ( 'NONE',  ( 0.05219959533909260263, 19.03943276465977164, 84.99890960531436690 ) ) ;
#69459=CARTESIAN_POINT ( 'NONE',  ( -0.05219959533936034679, 19.03943276465977164, 57.50109039468566863 ) ) ;
#69460=CARTESIAN_POINT ( 'NONE',  ( 21.52544592524344225, -5.823673210054117533, 83.54057627198102409 ) ) ;
#69461=CARTESIAN_POINT ( 'NONE',  ( -5.823673210054116645, -21.52544592524344225, 67.29057627198103830 ) ) ;
#69463=CARTESIAN_POINT ( 'NONE',  ( -4.379528057220328563, 16.55341960407611168, 40.20724293864769550 ) ) ;
#69464=CARTESIAN_POINT ( 'NONE',  ( 15.80617190586769283, -15.72974639402175789, 110.6260903946857042 ) ) ;
#69465=CARTESIAN_POINT ( 'NONE',  ( 8.224510206698742110, 14.34966873604972548, 62.08442372801901143 ) ) ;
#69466=CARTESIAN_POINT ( 'NONE',  ( -16.46253265017160317, 9.564922557960807481, 90.83224293864769550 ) ) ;
#69467=CARTESIAN_POINT ( 'NONE',  ( -19.05341960407611168, -5.049401038298163336, 31.45724293864769550 ) ) ;
#69468=CARTESIAN_POINT ( 'NONE',  ( 18.67979575497194134, -10.72451020669871369, 40.83442372801901854 ) ) ;
#69469=CARTESIAN_POINT ( 'NONE',  ( 5.719274019375673035, 21.55341960407619339, 57.29275706135234714 ) ) ;
#69470=CARTESIAN_POINT ( 'NONE',  ( 13.97604488694527802, 13.89961937509977652, 64.37390960531436690 ) ) ;
#69471=CARTESIAN_POINT ( 'NONE',  ( -21.53943276465977519, -0.05219959533937600094, 33.75109039468568284 ) ) ;
#69473=CARTESIAN_POINT ( 'NONE',  ( 19.05341960407617918, -5.049401038297876454, 76.04275706135230450 ) ) ;
#69474=CARTESIAN_POINT ( 'NONE',  ( 13.97604488694548053, -13.89961937509957401, 75.62609039468564731 ) ) ;
#69475=CARTESIAN_POINT ( 'NONE',  ( 19.05341960407611168, 5.049401038298154454, 43.95724293864769550 ) ) ;
#69476=CARTESIAN_POINT ( 'NONE',  ( -16.53943276465976808, -0.05219959533934237506, 83.75109039468568994 ) ) ;
#69477=CARTESIAN_POINT ( 'NONE',  ( 9.474510206698971260, -16.51473224551069308, 57.91557627198103120 ) ) ;
#69479=CARTESIAN_POINT ( 'NONE',  ( 13.97604488694527802, 13.89961937509977652, 99.37390960531436690 ) ) ;
#69480=CARTESIAN_POINT ( 'NONE',  ( 13.89961937509977652, -13.97604488694527269, 43.12390960531434558 ) ) ;
#69482=CARTESIAN_POINT ( 'NONE',  ( 0.05219959533907565091, 21.53943276465977519, 74.99890960531435269 ) ) ;
#69483=CARTESIAN_POINT ( 'NONE',  ( -8.314922557961024197, 14.29746914071037800, 62.91775706135236135 ) ) ;
#69484=CARTESIAN_POINT ( 'NONE',  ( -19.02544592524334988, -5.153800228976617603, 18.95942372801899722 ) ) ;
#69485=CARTESIAN_POINT ( 'NONE',  ( 16.46253265017160672, -9.564922557960803928, 48.33224293864769550 ) ) ;
#69486=CARTESIAN_POINT ( 'NONE',  ( 8.224510206698953496, -14.34966873604960469, 47.91557627198102409 ) ) ;
#69487=CARTESIAN_POINT ( 'NONE',  ( -12.14591786802309592, -12.06949235617757132, 76.87390960531439532 ) ) ;
#69488=CARTESIAN_POINT ( 'NONE',  ( -5.153800228976328057, -19.02544592524343514, 82.29057627198103830 ) ) ;
#69489=CARTESIAN_POINT ( 'NONE',  ( 21.55341960407619695, -5.719274019375665929, 41.04275706135236135 ) ) ;
#69490=CARTESIAN_POINT ( 'NONE',  ( 19.05341960407611168, 5.049401038298154454, 93.95724293864769550 ) ) ;
#69491=CARTESIAN_POINT ( 'NONE',  ( 18.67979575497194134, -10.72451020669871369, 105.8344237280190328 ) ) ;
#69492=CARTESIAN_POINT ( 'NONE',  ( -12.14591786802326823, 12.06949235617739902, 63.12609039468568994 ) ) ;
#69493=CARTESIAN_POINT ( 'NONE',  ( -15.80617190586768217, 15.72974639402176855, 28.12609039468568284 ) ) ;
#69494=CARTESIAN_POINT ( 'NONE',  ( -16.46253265017160317, 9.564922557960807481, 105.8322429386476955 ) ) ;
#69495=CARTESIAN_POINT ( 'NONE',  ( 21.55341960407610458, 5.719274019375980345, 88.95724293864769550 ) ) ;
#69496=CARTESIAN_POINT ( 'NONE',  ( 16.53943276465976808, -0.05219959533910856209, 48.74890960531435979 ) ) ;
#69497=CARTESIAN_POINT ( 'NONE',  ( -9.474510206698964154, 16.51473224551069663, 35.41557627198102409 ) ) ;
#69498=CARTESIAN_POINT ( 'NONE',  ( -12.06949235617756955, 12.14591786802309770, 65.62390960531436690 ) ) ;
#69499=CARTESIAN_POINT ( 'NONE',  ( -5.823673210054116645, -21.52544592524344225, 32.29057627198102409 ) ) ;
#69500=CARTESIAN_POINT ( 'NONE',  ( 16.46253265017146816, 9.564922557961045513, 26.66775706135234003 ) ) ;
#69501=CARTESIAN_POINT ( 'NONE',  ( -14.29746914071049879, 8.314922557960819915, 95.83224293864770971 ) ) ;
#69502=CARTESIAN_POINT ( 'NONE',  ( -16.46253265017160317, 9.564922557960807481, 105.8322429386476955 ) ) ;
#69504=CARTESIAN_POINT ( 'NONE',  ( -16.52544592524335698, -4.483927247898792601, 53.95942372801900433 ) ) ;
#69505=CARTESIAN_POINT ( 'NONE',  ( 13.89961937509977652, -13.97604488694527269, 53.12390960531434558 ) ) ;
#69506=CARTESIAN_POINT ( 'NONE',  ( -16.60608727067442558, -6.680868421854470718, 20.82238414752631073 ) ) ;
#69507=CARTESIAN_POINT ( 'NONE',  ( 13.97604488694548053, -13.89961937509957401, 65.62609039468567573 ) ) ;
#69508=CARTESIAN_POINT ( 'NONE',  ( -8.314922557961024197, 14.29746914071037800, 92.91775706135236135 ) ) ;
#69509=CARTESIAN_POINT ( 'NONE',  ( 9.564922557961047289, -16.46253265017146816, 100.4177570613523329 ) ) ;
#69510=CARTESIAN_POINT ( 'NONE',  ( 21.53943276465977519, 0.05219959533937863772, 71.25109039468568994 ) ) ;
#69511=CARTESIAN_POINT ( 'NONE',  ( -9.564922557960796823, -16.46253265017161027, 72.08224293864770971 ) ) ;
#69512=CARTESIAN_POINT ( 'NONE',  ( -21.55341960407610458, -5.719274019375992779, 86.45724293864770971 ) ) ;
#69513=CARTESIAN_POINT ( 'NONE',  ( -4.379528057220086978, -16.55341960407618274, 44.79275706135234714 ) ) ;
#69514=VECTOR ( 'NONE', #113856, 1000.000000000000000 ) ;
#69515=CARTESIAN_POINT ( 'NONE',  ( 16.55341960407611168, 4.379528057220329451, 108.9572429386476955 ) ) ;
#69516=CARTESIAN_POINT ( 'NONE',  ( -5.153800228976607833, 19.02544592524334988, 82.70942372801897591 ) ) ;
#69517=CARTESIAN_POINT ( 'NONE',  ( -15.80617190586745835, -15.72974639402198527, 71.87390960531438111 ) ) ;
#69518=CARTESIAN_POINT ( 'NONE',  ( -5.049401038297874678, -19.05341960407617918, 44.79275706135232582 ) ) ;
#69520=CARTESIAN_POINT ( 'NONE',  ( 0.05219959533907565091, 21.53943276465977519, 89.99890960531438111 ) ) ;
#69521=CARTESIAN_POINT ( 'NONE',  ( 17.50000000000147082, 3.202012800152233662, 27.57177583972747215 ) ) ;
#69522=CARTESIAN_POINT ( 'NONE',  ( -5.049401038298153566, 19.05341960407611168, 65.20724293864765286 ) ) ;
#69524=CARTESIAN_POINT ( 'NONE',  ( -14.29746914071037622, -8.314922557961029526, 24.16775706135235424 ) ) ;
#69526=CARTESIAN_POINT ( 'NONE',  ( -9.564922557960796823, -16.46253265017161027, 52.08224293864768839 ) ) ;
#69527=CARTESIAN_POINT ( 'NONE',  ( 5.719274019375991003, -21.55341960407610458, 107.7072429386476955 ) ) ;
#69528=CARTESIAN_POINT ( 'NONE',  ( -0.05219959533910754901, -16.53943276465976808, 57.49890960531435979 ) ) ;
#69529=CARTESIAN_POINT ( 'NONE',  ( 19.02544592524343514, -5.153800228976328945, 53.54057627198102409 ) ) ;
#69531=CARTESIAN_POINT ( 'NONE',  ( -21.52544592524334988, -5.823673210054445271, 73.95942372801901854 ) ) ;
#69532=CARTESIAN_POINT ( 'NONE',  ( 4.483927247898790824, -16.52544592524335698, 20.20942372801900788 ) ) ;
#69533=CARTESIAN_POINT ( 'NONE',  ( 19.05341960407617918, -5.049401038297876454, 26.04275706135233293 ) ) ;
#69534=CARTESIAN_POINT ( 'NONE',  ( 16.52544592524342804, -4.483927247898539470, 33.54057627198102409 ) ) ;
#69535=CARTESIAN_POINT ( 'NONE',  ( -5.719274019375665041, -21.55341960407619695, 44.79275706135234714 ) ) ;
#69536=CARTESIAN_POINT ( 'NONE',  ( 10.81492255796106328, -18.62759615963255655, 20.41775706135234714 ) ) ;
#69537=CARTESIAN_POINT ( 'NONE',  ( -15.72974639402197994, 15.80617190586746368, 65.62390960531436690 ) ) ;
#69538=CARTESIAN_POINT ( 'NONE',  ( 5.153800228976615827, -19.02544592524334988, 95.20942372801897591 ) ) ;
#69539=CARTESIAN_POINT ( 'NONE',  ( -0.05219959533936034679, 19.03943276465977164, 62.50109039468566863 ) ) ;
#69540=CARTESIAN_POINT ( 'NONE',  ( 18.67979575497194134, -10.72451020669871369, 65.83442372801900433 ) ) ;
#69541=CARTESIAN_POINT ( 'NONE',  ( -13.89961937509957401, -13.97604488694547875, 54.37609039468565442 ) ) ;
#69542=CARTESIAN_POINT ( 'NONE',  ( -19.03943276465977164, 0.05219959533909376836, 21.24890960531436335 ) ) ;
#69543=CARTESIAN_POINT ( 'NONE',  ( 15.80617190586746368, 15.72974639402197994, 59.37390960531436690 ) ) ;
#69544=CARTESIAN_POINT ( 'NONE',  ( -0.05219959533910754901, -16.53943276465976808, 47.49890960531435979 ) ) ;
#69545=CARTESIAN_POINT ( 'NONE',  ( -19.35633801406907750, 5.499999999999677591, 94.13373818172762242 ) ) ;
#69546=CARTESIAN_POINT ( 'NONE',  ( 21.52544592524334988, 5.823673210054432836, 111.4594237280190328 ) ) ;
#69547=CARTESIAN_POINT ( 'NONE',  ( 8.224510206698742110, 14.34966873604972548, 87.08442372801901854 ) ) ;
#69548=CARTESIAN_POINT ( 'NONE',  ( 16.55341960407611168, 4.379528057220329451, 38.95724293864768839 ) ) ;
#69549=CARTESIAN_POINT ( 'NONE',  ( -5.719274019375665041, -21.55341960407619695, 79.79275706135236135 ) ) ;
#69550=CARTESIAN_POINT ( 'NONE',  ( 10.81492255796106328, -18.62759615963255655, 75.41775706135233293 ) ) ;
#69551=CARTESIAN_POINT ( 'NONE',  ( -21.55341960407610458, -5.719274019375992779, 81.45724293864769550 ) ) ;
#69552=CARTESIAN_POINT ( 'NONE',  ( 19.02544592524343514, -5.153800228976328945, 43.54057627198103120 ) ) ;
#69553=CARTESIAN_POINT ( 'NONE',  ( 21.55341960407619695, -5.719274019375665929, 61.04275706135234714 ) ) ;
#69554=CARTESIAN_POINT ( 'NONE',  ( -9.474510206698964154, 16.51473224551069663, 35.41557627198102409 ) ) ;
#69555=CARTESIAN_POINT ( 'NONE',  ( 19.02544592524343514, -5.153800228976328945, 53.54057627198102409 ) ) ;
#69556=CARTESIAN_POINT ( 'NONE',  ( 12.06949235617757843, -12.14591786802309237, 88.12390960531436690 ) ) ;
#69557=CARTESIAN_POINT ( 'NONE',  ( -16.46253265017160317, 9.564922557960807481, 100.8322429386477097 ) ) ;
#69558=CARTESIAN_POINT ( 'NONE',  ( -14.29746914071049879, 8.314922557960819915, 40.83224293864769550 ) ) ;
#69559=CARTESIAN_POINT ( 'NONE',  ( -4.379528057220328563, 16.55341960407611168, 110.2072429386477239 ) ) ;
#69560=CARTESIAN_POINT ( 'NONE',  ( -15.72974639402197994, 15.80617190586746368, 80.62390960531438111 ) ) ;
#69561=CARTESIAN_POINT ( 'NONE',  ( -0.05219959533937732626, 21.53943276465977519, 22.50109039468567573 ) ) ;
#69563=CARTESIAN_POINT ( 'NONE',  ( -16.52544592524335698, -4.483927247898792601, 38.95942372801901854 ) ) ;
#69564=CARTESIAN_POINT ( 'NONE',  ( 0.05219959533907565091, 21.53943276465977519, 74.99890960531435269 ) ) ;
#69565=CARTESIAN_POINT ( 'NONE',  ( -5.719274019375665041, -21.55341960407619695, 94.79275706135234714 ) ) ;
#69566=CARTESIAN_POINT ( 'NONE',  ( -19.02544592524342804, 5.153800228976336051, 76.04057627198102409 ) ) ;
#69567=CARTESIAN_POINT ( 'NONE',  ( -15.72974639402176322, -15.80617190586768395, 24.37609039468567573 ) ) ;
#69569=CARTESIAN_POINT ( 'NONE',  ( 0.05219959533909260263, 19.03943276465977164, 114.9989096053143669 ) ) ;
#69570=CARTESIAN_POINT ( 'NONE',  ( 14.34966873604972726, -8.224510206698740333, 95.83442372801903275 ) ) ;
#69571=CARTESIAN_POINT ( 'NONE',  ( -15.80617190586768217, 15.72974639402176855, 73.12609039468567573 ) ) ;
#69572=CARTESIAN_POINT ( 'NONE',  ( 13.97604488694548053, -13.89961937509957401, 20.62609039468567573 ) ) ;
#69573=CARTESIAN_POINT ( 'NONE',  ( 16.53943276465976808, 0.05219959533934440121, 71.25109039468568994 ) ) ;
#69574=CARTESIAN_POINT ( 'NONE',  ( 0.05219959533937995610, -21.53943276465977519, 30.00109039468568284 ) ) ;
#69575=CARTESIAN_POINT ( 'NONE',  ( -16.46253265017160317, 9.564922557960807481, 30.83224293864769550 ) ) ;
#69576=CARTESIAN_POINT ( 'NONE',  ( -15.72974639402176322, -15.80617190586768395, 89.37609039468568994 ) ) ;
#69577=CARTESIAN_POINT ( 'NONE',  ( 5.153800228976335163, 19.02544592524342804, 94.79057627198103830 ) ) ;
#69578=CARTESIAN_POINT ( 'NONE',  ( -18.67979575497178146, -10.72451020669898902, 96.66557627198102409 ) ) ;
#69580=CARTESIAN_POINT ( 'NONE',  ( 5.823673210054125526, 21.52544592524343514, 54.79057627198104541 ) ) ;
#69581=CARTESIAN_POINT ( 'NONE',  ( -16.51473224551069308, -9.474510206698971260, 96.66557627198102409 ) ) ;
#69582=CARTESIAN_POINT ( 'NONE',  ( 12.06949235617757843, -12.14591786802309237, 48.12390960531436690 ) ) ;
#69584=CARTESIAN_POINT ( 'NONE',  ( 16.51473224551083163, -9.474510206698727899, 75.83442372801900433 ) ) ;
#69586=CARTESIAN_POINT ( 'NONE',  ( 5.049401038297881783, 19.05341960407617563, 107.2927570613523187 ) ) ;
#69587=CARTESIAN_POINT ( 'NONE',  ( 15.80617190586746368, 15.72974639402197994, 89.37390960531435269 ) ) ;
#69588=CARTESIAN_POINT ( 'NONE',  ( -16.55341960407611168, -4.379528057220339221, 66.45724293864768129 ) ) ;
#69589=CARTESIAN_POINT ( 'NONE',  ( -16.51473224551069308, -9.474510206698971260, 96.66557627198102409 ) ) ;
#69590=CARTESIAN_POINT ( 'NONE',  ( -16.52544592524335698, -4.483927247898792601, 38.95942372801901854 ) ) ;
#69591=CARTESIAN_POINT ( 'NONE',  ( -13.89961937509977652, 13.97604488694528158, 55.62390960531434558 ) ) ;
#69592=CARTESIAN_POINT ( 'NONE',  ( 15.72974639402176855, 15.80617190586768217, 26.87609039468567218 ) ) ;
#69593=CARTESIAN_POINT ( 'NONE',  ( -16.51473224551082808, 9.474510206698731452, 98.33442372801900433 ) ) ;
#69594=CARTESIAN_POINT ( 'NONE',  ( -5.049401038298153566, 19.05341960407611168, 100.2072429386476955 ) ) ;
#69595=CARTESIAN_POINT ( 'NONE',  ( 5.049401038298161559, -19.05341960407611168, 87.70724293864769550 ) ) ;
#69596=CARTESIAN_POINT ( 'NONE',  ( -10.72451020669898014, 18.67979575497178502, 90.41557627198103830 ) ) ;
#69597=CARTESIAN_POINT ( 'NONE',  ( 16.46253265017160672, -9.564922557960803928, 48.33224293864769550 ) ) ;
#69598=CARTESIAN_POINT ( 'NONE',  ( -17.05116617787826883, -6.768360034955705373, 61.34324446740804859 ) ) ;
#69599=CARTESIAN_POINT ( 'NONE',  ( 14.34966873604960469, 8.224510206698951720, 74.16557627198102409 ) ) ;
#69600=CARTESIAN_POINT ( 'NONE',  ( -16.51473224551069308, -9.474510206698971260, 106.6655762719810383 ) ) ;
#69602=CARTESIAN_POINT ( 'NONE',  ( -5.049401038297874678, -19.05341960407617918, 59.79275706135231871 ) ) ;
#69604=CARTESIAN_POINT ( 'NONE',  ( -21.55341960407610458, -5.719274019375992779, 86.45724293864770971 ) ) ;
#69605=CARTESIAN_POINT ( 'NONE',  ( 13.97604488694548053, -13.89961937509957401, 55.62609039468566863 ) ) ;
#69606=CARTESIAN_POINT ( 'NONE',  ( -19.03943276465977164, 0.05219959533909376836, 106.2489096053143669 ) ) ;
#69608=CARTESIAN_POINT ( 'NONE',  ( -18.62759615963270932, 10.81492255796079327, 40.83224293864769550 ) ) ;
#69609=CARTESIAN_POINT ( 'NONE',  ( 16.46253265017160672, -9.564922557960803928, 88.33224293864769550 ) ) ;
#69610=CARTESIAN_POINT ( 'NONE',  ( 21.55341960407619695, -5.719274019375665929, 66.04275706135236135 ) ) ;
#69611=CARTESIAN_POINT ( 'NONE',  ( -9.564922557960796823, -16.46253265017161027, 32.08224293864769550 ) ) ;
#69612=CARTESIAN_POINT ( 'NONE',  ( -16.52544592524342804, 4.483927247898546575, 76.04057627198102409 ) ) ;
#69613=CARTESIAN_POINT ( 'NONE',  ( -8.314922557961024197, 14.29746914071037800, 22.91775706135235069 ) ) ;
#69614=CARTESIAN_POINT ( 'NONE',  ( 18.62759615963255655, 10.81492255796105972, 56.66775706135235424 ) ) ;
#69615=ORIENTED_EDGE ( 'NONE', *, *, #157116, .T. ) ;
#69616=CARTESIAN_POINT ( 'NONE',  ( -9.474510206698964154, 16.51473224551069663, 115.4155762719810241 ) ) ;
#69617=CARTESIAN_POINT ( 'NONE',  ( 5.049401038297881783, 19.05341960407617563, 62.29275706135234003 ) ) ;
#69619=CARTESIAN_POINT ( 'NONE',  ( 15.80617190586769283, -15.72974639402175789, 20.62609039468568639 ) ) ;
#69620=CARTESIAN_POINT ( 'NONE',  ( 19.03943276465977164, -0.05219959533909143690, 63.74890960531435979 ) ) ;
#69622=CARTESIAN_POINT ( 'NONE',  ( -16.46253265017146816, -9.564922557961047289, 24.16775706135233648 ) ) ;
#69623=CARTESIAN_POINT ( 'NONE',  ( -19.05341960407611168, -5.049401038298163336, 56.45724293864768129 ) ) ;
#69624=CARTESIAN_POINT ( 'NONE',  ( -21.55341960407619339, 5.719274019375674811, 108.5427570613523756 ) ) ;
#69625=CARTESIAN_POINT ( 'NONE',  ( 14.34966873604972726, -8.224510206698740333, 105.8344237280190328 ) ) ;
#69626=CARTESIAN_POINT ( 'NONE',  ( 9.474510206698971260, -16.51473224551069308, 107.9155762719810383 ) ) ;
#69627=CARTESIAN_POINT ( 'NONE',  ( -15.80617190586768217, 15.72974639402176855, 73.12609039468567573 ) ) ;
#69629=CARTESIAN_POINT ( 'NONE',  ( 5.153800228976335163, 19.02544592524342804, 109.7905762719810099 ) ) ;
#69630=CARTESIAN_POINT ( 'NONE',  ( 17.50000000000000000, 5.499999999999992895, 96.70309617465829888 ) ) ;
#69631=CARTESIAN_POINT ( 'NONE',  ( 8.314922557961029526, -14.29746914071037800, 60.41775706135235424 ) ) ;
#69632=CARTESIAN_POINT ( 'NONE',  ( -21.52544592524334988, -5.823673210054445271, 73.95942372801901854 ) ) ;
#69633=CARTESIAN_POINT ( 'NONE',  ( -21.53943276465977519, -0.05219959533937600094, 108.7510903946857042 ) ) ;
#69635=CARTESIAN_POINT ( 'NONE',  ( 16.46253265017160672, -9.564922557960803928, 88.33224293864769550 ) ) ;
#69636=CARTESIAN_POINT ( 'NONE',  ( -19.03943276465977164, 0.05219959533909376836, 106.2489096053143669 ) ) ;
#69638=CARTESIAN_POINT ( 'NONE',  ( 17.48847506799967277, 5.747544572773803928, 41.67302562156719858 ) ) ;
#69639=CARTESIAN_POINT ( 'NONE',  ( 9.564922557960805705, 16.46253265017160317, 39.58224293864768839 ) ) ;
#69640=CARTESIAN_POINT ( 'NONE',  ( 10.81492255796078972, 18.62759615963270932, 39.58224293864769550 ) ) ;
#69641=CARTESIAN_POINT ( 'NONE',  ( 8.314922557961029526, -14.29746914071037800, 110.4177570613523756 ) ) ;
#69642=CARTESIAN_POINT ( 'NONE',  ( 16.55341960407611168, 4.379528057220329451, 98.95724293864770971 ) ) ;
#69643=CARTESIAN_POINT ( 'NONE',  ( 9.474510206698971260, -16.51473224551069308, 82.91557627198103830 ) ) ;
#69644=CARTESIAN_POINT ( 'NONE',  ( -21.55341960407619339, 5.719274019375674811, 103.5427570613523613 ) ) ;
#69645=CARTESIAN_POINT ( 'NONE',  ( 16.51473224551069308, 9.474510206698969483, 34.16557627198102409 ) ) ;
#69646=CARTESIAN_POINT ( 'NONE',  ( 16.52544592524342804, -4.483927247898539470, 93.54057627198103830 ) ) ;
#69647=CARTESIAN_POINT ( 'NONE',  ( 10.81492255796106328, -18.62759615963255655, 40.41775706135234714 ) ) ;
#69648=CARTESIAN_POINT ( 'NONE',  ( 15.80617190586746368, 15.72974639402197994, 84.37390960531438111 ) ) ;
#69649=CARTESIAN_POINT ( 'NONE',  ( -9.474510206698720793, -16.51473224551083518, 49.58442372801899722 ) ) ;
#69650=CARTESIAN_POINT ( 'NONE',  ( 18.22780087662121673, 5.500000000000056843, 63.98459894673894155 ) ) ;
#69651=CARTESIAN_POINT ( 'NONE',  ( 9.564922557960805705, 16.46253265017160317, 99.58224293864770971 ) ) ;
#69652=CARTESIAN_POINT ( 'NONE',  ( 12.14591786802309770, 12.06949235617756955, 69.37390960531436690 ) ) ;
#69653=CARTESIAN_POINT ( 'NONE',  ( 16.53943276465976808, -0.05219959533910856209, 53.74890960531437401 ) ) ;
#69654=CARTESIAN_POINT ( 'NONE',  ( -9.474510206698720793, -16.51473224551083518, 84.58442372801900433 ) ) ;
#69656=CARTESIAN_POINT ( 'NONE',  ( 21.53943276465977519, -0.05219959533907433946, 23.74890960531435269 ) ) ;
#69658=CARTESIAN_POINT ( 'NONE',  ( -14.29746914071049879, 8.314922557960819915, 90.83224293864769550 ) ) ;
#69660=CARTESIAN_POINT ( 'NONE',  ( -19.02544592524342804, 5.153800228976336051, 51.04057627198103120 ) ) ;
#69661=CARTESIAN_POINT ( 'NONE',  ( 21.53943276465977519, -0.05219959533907433946, 53.74890960531437401 ) ) ;
#69662=CARTESIAN_POINT ( 'NONE',  ( -19.05341960407611168, -5.049401038298163336, 31.45724293864769550 ) ) ;
#69663=CARTESIAN_POINT ( 'NONE',  ( -16.55341960407617563, 4.379528057220093196, 73.54275706135234714 ) ) ;
#69664=CARTESIAN_POINT ( 'NONE',  ( 19.05341960407611168, 5.049401038298154454, 63.95724293864769550 ) ) ;
#69665=CARTESIAN_POINT ( 'NONE',  ( -5.049401038297874678, -19.05341960407617918, 34.79275706135233293 ) ) ;
#69666=CARTESIAN_POINT ( 'NONE',  ( -21.52544592524334988, -5.823673210054445271, 73.95942372801901854 ) ) ;
#69667=CARTESIAN_POINT ( 'NONE',  ( -21.53943276465977519, 0.05219959533907696930, 31.24890960531435979 ) ) ;
#69668=CARTESIAN_POINT ( 'NONE',  ( -0.05219959533910754901, -16.53943276465976808, 112.4989096053143669 ) ) ;
#69669=CARTESIAN_POINT ( 'NONE',  ( -19.02544592524334988, -5.153800228976617603, 88.95942372801897591 ) ) ;
#69671=CARTESIAN_POINT ( 'NONE',  ( 17.50000000000000711, 3.556738311678228737, 37.24728836128200982 ) ) ;
#69672=CARTESIAN_POINT ( 'NONE',  ( 5.719274019375991003, -21.55341960407610458, 42.70724293864770260 ) ) ;
#69673=CARTESIAN_POINT ( 'NONE',  ( 16.52216118717209525, -7.221426719304495201, 66.42400978953006074 ) ) ;
#69674=CARTESIAN_POINT ( 'NONE',  ( 10.72451020669871369, 18.67979575497193778, 77.08442372801901854 ) ) ;
#69675=CARTESIAN_POINT ( 'NONE',  ( -12.14591786802309592, -12.06949235617757132, 46.87390960531435979 ) ) ;
#69676=CARTESIAN_POINT ( 'NONE',  ( 0.05219959533934541429, -16.53943276465976808, 75.00109039468568994 ) ) ;
#69677=CARTESIAN_POINT ( 'NONE',  ( 4.483927247898545687, 16.52544592524342804, 54.79057627198104541 ) ) ;
#69678=CARTESIAN_POINT ( 'NONE',  ( -15.72974639402197994, 15.80617190586746368, 80.62390960531438111 ) ) ;
#69679=CARTESIAN_POINT ( 'NONE',  ( -21.53943276465977519, 0.05219959533907696930, 81.24890960531436690 ) ) ;
#69681=CARTESIAN_POINT ( 'NONE',  ( -15.80617190586745835, -15.72974639402198527, 26.87390960531435979 ) ) ;
#69682=CARTESIAN_POINT ( 'NONE',  ( -4.483927247898782831, 16.52544592524335698, 47.70942372801902565 ) ) ;
#69683=CARTESIAN_POINT ( 'NONE',  ( -16.55341960407611168, -4.379528057220339221, 76.45724293864769550 ) ) ;
#69684=CARTESIAN_POINT ( 'NONE',  ( 5.153800228976335163, 19.02544592524342804, 64.79057627198100988 ) ) ;
#69685=CARTESIAN_POINT ( 'NONE',  ( 9.474510206698971260, -16.51473224551069308, 37.91557627198102409 ) ) ;
#69687=CARTESIAN_POINT ( 'NONE',  ( -16.53943276465976808, -0.05219959533934237506, 83.75109039468568994 ) ) ;
#69688=CARTESIAN_POINT ( 'NONE',  ( 10.81492255796106328, -18.62759615963255655, 20.41775706135234714 ) ) ;
#69689=CARTESIAN_POINT ( 'NONE',  ( -19.05341960407611168, -5.049401038298163336, 66.45724293864769550 ) ) ;
#69690=CARTESIAN_POINT ( 'NONE',  ( -10.72451020669870658, -18.67979575497194134, 54.58442372801901143 ) ) ;
#69691=CARTESIAN_POINT ( 'NONE',  ( -16.46253265017160317, 9.564922557960807481, 115.8322429386477097 ) ) ;
#69693=ORIENTED_EDGE ( 'NONE', *, *, #12667, .T. ) ;
#69694=CARTESIAN_POINT ( 'NONE',  ( 18.67979575497194134, -10.72451020669871369, 45.83442372801901854 ) ) ;
#69695=CARTESIAN_POINT ( 'NONE',  ( -16.46253265017160317, 9.564922557960807481, 115.8322429386477097 ) ) ;
#69696=CARTESIAN_POINT ( 'NONE',  ( 19.05341960407611168, 5.049401038298154454, 103.9572429386476671 ) ) ;
#69697=CARTESIAN_POINT ( 'NONE',  ( -16.51473224551082808, 9.474510206698731452, 58.33442372801900433 ) ) ;
#69698=CARTESIAN_POINT ( 'NONE',  ( 21.53943276465977519, 0.05219959533937863772, 21.25109039468567218 ) ) ;
#69699=CARTESIAN_POINT ( 'NONE',  ( 5.153800228976615827, -19.02544592524334988, 45.20942372801901143 ) ) ;
#69700=CARTESIAN_POINT ( 'NONE',  ( -19.05341960407617563, 5.049401038297882671, 63.54275706135234003 ) ) ;
#69701=CARTESIAN_POINT ( 'NONE',  ( -14.34966873604972548, 8.224510206698743886, 103.3344237280190043 ) ) ;
#69704=CARTESIAN_POINT ( 'NONE',  ( -9.474510206698964154, 16.51473224551069663, 80.41557627198103830 ) ) ;
#69706=CARTESIAN_POINT ( 'NONE',  ( -0.05219959533937732626, 21.53943276465977519, 87.50109039468568994 ) ) ;
#69707=CARTESIAN_POINT ( 'NONE',  ( 18.62759615963255655, 10.81492255796105972, 91.66775706135234714 ) ) ;
#69709=CARTESIAN_POINT ( 'NONE',  ( -9.564922557960796823, -16.46253265017161027, 102.0822429386477097 ) ) ;
#69710=CARTESIAN_POINT ( 'NONE',  ( -18.62759615963255300, -10.81492255796106328, 79.16775706135234714 ) ) ;
#69711=CARTESIAN_POINT ( 'NONE',  ( -16.52544592524335698, -4.483927247898792601, 18.95942372801901143 ) ) ;
#69712=CARTESIAN_POINT ( 'NONE',  ( -13.89961937509977652, 13.97604488694528158, 75.62390960531438111 ) ) ;
#69713=CARTESIAN_POINT ( 'NONE',  ( 5.719274019375991003, -21.55341960407610458, 27.70724293864769905 ) ) ;
#69714=CARTESIAN_POINT ( 'NONE',  ( -16.46253265017160317, 9.564922557960807481, 90.83224293864769550 ) ) ;
#69715=CARTESIAN_POINT ( 'NONE',  ( -16.88567814943164436, -6.947325034625694506, 91.29001122652587696 ) ) ;
#69716=CARTESIAN_POINT ( 'NONE',  ( 9.564922557960805705, 16.46253265017160317, 79.58224293864769550 ) ) ;
#69717=CARTESIAN_POINT ( 'NONE',  ( 19.05341960407611168, 5.049401038298154454, 63.95724293864769550 ) ) ;
#69718=CARTESIAN_POINT ( 'NONE',  ( -15.72974639402197994, 15.80617190586746368, 110.6239096053143669 ) ) ;
#69719=CARTESIAN_POINT ( 'NONE',  ( -4.483927247898782831, 16.52544592524335698, 102.7094237280190185 ) ) ;
#69721=CARTESIAN_POINT ( 'NONE',  ( 0.05219959533936267826, -19.03943276465977164, 60.00109039468566863 ) ) ;
#69722=CARTESIAN_POINT ( 'NONE',  ( 9.474510206698971260, -16.51473224551069308, 97.91557627198102409 ) ) ;
#69723=CARTESIAN_POINT ( 'NONE',  ( -0.05219959533910754901, -16.53943276465976808, 87.49890960531436690 ) ) ;
#69724=CARTESIAN_POINT ( 'NONE',  ( 21.55341960407610458, 5.719274019375980345, 33.95724293864769550 ) ) ;
#69725=CARTESIAN_POINT ( 'NONE',  ( -5.153800228976328057, -19.02544592524343514, 112.2905762719810099 ) ) ;
#69726=CARTESIAN_POINT ( 'NONE',  ( 12.06949235617757843, -12.14591786802309237, 93.12390960531436690 ) ) ;
#69727=CARTESIAN_POINT ( 'NONE',  ( -17.31728774477274158, 6.344390552232391123, 55.81906651689321563 ) ) ;
#69728=CARTESIAN_POINT ( 'NONE',  ( 19.02544592524334988, 5.153800228976608722, 41.45942372801900433 ) ) ;
#69729=CARTESIAN_POINT ( 'NONE',  ( -14.29746914071037622, -8.314922557961029526, 104.1677570613523471 ) ) ;
#69730=CARTESIAN_POINT ( 'NONE',  ( 5.049401038298161559, -19.05341960407611168, 87.70724293864769550 ) ) ;
#69731=CARTESIAN_POINT ( 'NONE',  ( 15.72974639402176855, 15.80617190586768217, 66.87609039468568994 ) ) ;
#69732=CARTESIAN_POINT ( 'NONE',  ( -21.55341960407610458, -5.719274019375992779, 51.45724293864770260 ) ) ;
#69733=CARTESIAN_POINT ( 'NONE',  ( 15.80617190586769283, -15.72974639402175789, 35.62609039468568994 ) ) ;
#69734=CARTESIAN_POINT ( 'NONE',  ( 18.62759615963271287, -10.81492255796078972, 88.33224293864769550 ) ) ;
#69735=CARTESIAN_POINT ( 'NONE',  ( 16.52544592524342804, -4.483927247898539470, 103.5405762719810383 ) ) ;
#69736=CARTESIAN_POINT ( 'NONE',  ( -13.89961937509957401, -13.97604488694547875, 74.37609039468566152 ) ) ;
#69737=CARTESIAN_POINT ( 'NONE',  ( 9.564922557960805705, 16.46253265017160317, 44.58224293864769550 ) ) ;
#69738=CARTESIAN_POINT ( 'NONE',  ( 16.51473224551069308, 9.474510206698969483, 99.16557627198102409 ) ) ;
#69739=CARTESIAN_POINT ( 'NONE',  ( 19.05341960407611168, 5.049401038298154454, 88.95724293864769550 ) ) ;
#69740=CARTESIAN_POINT ( 'NONE',  ( 12.14591786802309770, 12.06949235617756955, 114.3739096053143527 ) ) ;
#69741=CARTESIAN_POINT ( 'NONE',  ( -4.379528057220328563, 16.55341960407611168, 45.20724293864769550 ) ) ;
#69742=CARTESIAN_POINT ( 'NONE',  ( -16.55341960407617563, 4.379528057220093196, 38.54275706135234714 ) ) ;
#69743=CARTESIAN_POINT ( 'NONE',  ( 5.153800228976335163, 19.02544592524342804, 24.79057627198102765 ) ) ;
#69744=CARTESIAN_POINT ( 'NONE',  ( 10.81492255796106328, -18.62759615963255655, 100.4177570613523471 ) ) ;
#69745=CARTESIAN_POINT ( 'NONE',  ( 19.03943276465977164, -0.05219959533909143690, 108.7489096053143527 ) ) ;
#69746=CARTESIAN_POINT ( 'NONE',  ( 4.379528057220339221, -16.55341960407611168, 22.70724293864769194 ) ) ;
#69747=CARTESIAN_POINT ( 'NONE',  ( -10.72451020669870658, -18.67979575497194134, 29.58442372801901854 ) ) ;
#69748=CARTESIAN_POINT ( 'NONE',  ( 0.05219959533909260263, 19.03943276465977164, 104.9989096053143669 ) ) ;
#69749=CARTESIAN_POINT ( 'NONE',  ( 12.06949235617739724, 12.14591786802326823, 51.87609039468568284 ) ) ;
#69750=CARTESIAN_POINT ( 'NONE',  ( 12.14591786802327356, -12.06949235617739191, 110.6260903946857042 ) ) ;
#69751=CARTESIAN_POINT ( 'NONE',  ( 8.224510206698742110, 14.34966873604972548, 87.08442372801901854 ) ) ;
#69752=CARTESIAN_POINT ( 'NONE',  ( 14.29746914071037800, 8.314922557961029526, 31.66775706135234358 ) ) ;
#69753=CARTESIAN_POINT ( 'NONE',  ( -13.97604488694527625, -13.89961937509977652, 51.87390960531436690 ) ) ;
#69754=CARTESIAN_POINT ( 'NONE',  ( 14.29746914071049879, -8.314922557960816363, 103.3322429386476955 ) ) ;
#69755=CARTESIAN_POINT ( 'NONE',  ( 18.67979575497194134, -10.72451020669871369, 20.83442372801901143 ) ) ;
#69756=CARTESIAN_POINT ( 'NONE',  ( -5.049401038298153566, 19.05341960407611168, 30.20724293864768839 ) ) ;
#69757=CARTESIAN_POINT ( 'NONE',  ( 16.51473224551069308, 9.474510206698969483, 99.16557627198102409 ) ) ;
#69758=CARTESIAN_POINT ( 'NONE',  ( -9.564922557960796823, -16.46253265017161027, 32.08224293864769550 ) ) ;
#69760=CARTESIAN_POINT ( 'NONE',  ( 16.46253265017160672, -9.564922557960803928, 98.33224293864769550 ) ) ;
#69762=CARTESIAN_POINT ( 'NONE',  ( -5.153800228976328057, -19.02544592524343514, 102.2905762719810383 ) ) ;
#69763=CARTESIAN_POINT ( 'NONE',  ( -21.52544592524334988, -5.823673210054445271, 43.95942372801902565 ) ) ;
#69764=CARTESIAN_POINT ( 'NONE',  ( 0.05219959533910956823, 16.53943276465976808, 94.99890960531436690 ) ) ;
#69765=CARTESIAN_POINT ( 'NONE',  ( 5.153800228976335163, 19.02544592524342804, 114.7905762719810241 ) ) ;
#69767=CARTESIAN_POINT ( 'NONE',  ( -8.314922557961024197, 14.29746914071037800, 62.91775706135236135 ) ) ;
#69768=( BOUNDED_SURFACE ( )  B_SPLINE_SURFACE ( 3, 2, ( 
 ( #65751, #82903, #110269, #34432, #7060, #112260, #96092, #125449, #173952, #187145, #4074, #67746, #35419, #158753, #127420, #171950, #156787, #114235, #48618, #20242, #79935, #141605, #152330, #86914, #45159, #121984, #84898, #162755, #29987, #195107, #198844, #29009, #102087, #163771, #105826, #147601, #24264, #68741, #161760, #71747, #115256, #85913, #120984, #59315, #131417, #133418, #9088, #137155, #25272, #146577, #106815, #101070, #13816, #8072, #69748, #75482, #148597, #182682, #70756, #193105, #44167, #10089, #168489, #167513, #60308, #132424, #194115, #192097, #90648, #53579, #55579, #176949, #183674, #54579, #117253, #91626, #153314, #178945, #130399, #38418, #40416, #100075, #23255, #116251, #177943, #39410, #199834, #50123, #109794, #3598, #138153, #110787, #107794, #48137, #80440, #96596, #142113, #169478, #184658, #32966, #126936, #65277, #188644, #171477, #111783, #78449, #49129, #94620, #33955, #172468, #170479, #61301, #46140, #95613, #156299, #173471, #140123, #34944, #122971, #2616, #14815, #17800, #30979, #79457, #125960, #76476, #92626, #141126, #155310, #64293, #154317, #15806, #77467, #1614, #139137, #614, #63290, #62284, #47142, #187658, #124970, #186667, #16799, #123952, #185650, #157298, #108800, #31969, #18795, #93625, #38936, #176461, #131944, #8603, #174461, #52098, #116770, #84418, #85425, #115778, #191610, #53089, #192622, #36922, #51109, #161275, #4580, #113755, #7579, #146095, #20760, #22770, #175451, #23775, #114767, #35930, #193628, #190623, #100593, #97576, #159264, #162275, #37934, #69265, #98584, #82415, #130931, #99595, #55100, #54104, #147116, #160278, #21769, #81415, #177467, #143101, #83420, #66273, #70276, #144104, #145097, #178461, #39928, #6580, #158285, #19774, #129910, #68259, #127932, #189634, #5584, #112768, #67264, #128922, #196636, #90408, #24786, #197612, #194629, #134958, #167271, #183430, #28770, #56099, #71276, #119775, #13577, #152093, #75244, #58105, #198602, #165290, #135942, #181459, #120744, #59077, #57114, #148120, #132941, #182443, #42937, #136915, #26783, #60070, #9611, #89427, #121738, #104601, #117780, #166289, #12608, #101597, #163285, #27785, #41948, #151116, #86434, #102611, #179474, #88425, #164297, #40939, #150119, #25790, #133950, #74272, #11620, #73288, #103614, #87436, #149121, #43923, #10612, #72273, #105585, #195641, #118788, #180477, #18551, #95369, #61057, #138893, #3361, #171232, #172222, #2369, #78206, #139876, #79210, #123710, #373, #44915, #33707, #157054, #124723, #80199, #32721, #137908, #108558, #186421, #106571, #64049, #168248, #29744, #141870, #65036, #1365, #63044, #170236, #47897, #93378, #91379, #153068, #45900, #126692, #187418, #14570, #125719, #48886, #76228, #199590, #122729, #184420, #109551, #94373, #107553, #156053, #169231, #31730, #30738, #92385, #17550, #154072, #15566, #140879, #110541, #77224, #155064, #62045, #185407, #46898, #16559, #35691, #85174, #100353, #162032, #70030, #99349, #160033, #52844, #50870, #161032, #173224, #130685, #144855, #112528, #81180, #98334, #159024, #21520, #19535, #114514, #142862, #83181, #192379, #6338, #4341, #49874, #97338, #190380, #20517, #66026, #145853, #188396, #68018, #22526, #115536, #174222, #129670, #177224, #176215, #38697, #84173, #191367, #158045, #37684, #23528, #146863, #8355, #7335, #82165, #127693, #69020, #189393, #143861, #53862, #111539, #34700, #5340, #96357, #175209, #67024, #128683, #36674, #51855, #113515, #167028, #10366, #25550, #101344, #135700, #89180, #133696, #103365, #147880, #118541, #116530, #72023, #41700, #104355, #180231, #194387, #90166, #195388, #151849, #164051, #88180, #56866, #165043, #26536, #178218, #39682, #42694, #120503, #9366, #166039, #11369, #12366, #149864, #105341, #182194, #71031, #87194, #13340, #57863, #58836, #150872, #73039, #134711, #27539, #196394, #148875, #131699, #24540, #119535, #163033, #181218 ),
 ( #197371, #74029, #43679, #28530, #132698, #193380, #54856, #86190, #55854, #117528, #179226, #40692, #102362, #139636, #59825, #138651, #183189, #47658, #14323, #15321, #140641, #1124, #123471, #93136, #78966, #46654, #107311, #77969, #121495, #91140, #44671, #106324, #110304, #169993, #63812, #198351, #170988, #168010, #108313, #2131, #156822, #125485, #29506, #152829, #154821, #187181, #48652, #171986, #31484, #33474, #132, #109309, #16319, #94134, #32481, #30488, #75988, #137661, #155813, #62798, #95132, #61801, #75004, #199348, #124480, #136669, #186176, #60813, #17311, #122487, #184178, #45660, #168984, #76980, #92139, #153826, #185163, #53615, #98089, #68778, #6101, #111299, #81922, #159787, #79971, #175976, #141639, #18314, #130435, #7096, #174970, #113279, #143614, #36434, #66781, #3129, #64804, #19304, #38454, #160797, #188163, #37445, #99105, #126465, #172988, #34466, #115291, #21282, #67781, #49636, #82939, #96125, #5098, #100109, #145617, #191137, #176984, #157814, #144617, #80952, #142627, #4106, #22285, #114272, #173984, #65785, #127454, #83936, #129438, #189160, #128442, #192134, #50633, #52610, #112294, #35453, #97104, #158788, #20276, #190139, #51614, #195144, #102122, #26299, #146613, #162789, #197136, #148634, #24298, #120269, #25308, #181961, #194149, #118299, #86950, #10124, #163806, #8105, #69783, #72800, #150635, #39443, #134470, #41458, #42454, #179991, #135468, #12131, #177975, #55613, #43443, #87940, #88944, #119295, #56625, #103123, #196155, #40448, #117287, #161793, #54611, #164804, #131451, #178981, #11125, #149627, #85946, #57628, #71784, #27297, #180978, #101103, #58603, #133454, #104118, #147635, #9124, #165800, #73795, #23288, #84932, #70790, #193138, #116285, #132458, #92901, #105112, #198120, #108072, #151620, #199107, #154587, #16083, #167778, #169756, #122250, #170756, #61569, #182955, #140406, #137427, #185936, #44438, #106092, #109077, #123238, #31251, #60574, #29276, #77741, #46414, #1895, #139407, #32245, #107078, #168750, #28299, #889, #89939, #30253, #13113, #62564, #90908, #45425, #93903, #124241, #153587, #184929, #155581, #76746, #183940, #47421, #74777, #121261, #136439, #59587, #63575, #200101, #17076, #152593, #78730, #14084, #138421, #125249, #186947, #166798, #75750, #91896, #15085, #160558, #175728, #114031, #4864, #82695, #49400, #83699, #156585, #67542, #144379, #3874, #94901, #18080, #5866, #143372, #145377, #112064, #98863, #79735, #36201, #6859, #189910, #64571, #51385, #159544, #22048, #68538, #81690, #188926, #113046, #33243, #111063, #130193, #35220, #172751, #48418, #173752, #110074, #80717, #66549, #96873, #158557, #50404, #141404, #2892, #21042, #37207, #126236, #129200, #128213, #190898, #174738, #171754, #187931, #34232, #142395, #95894, #97855, #157577, #52374, #19070, #65553, #127212, #20047, #85708, #99872, #56376, #161556, #117043, #11898, #119064, #164565, #150402, #23049, #133211, #53373, #192903, #57391, #7861, #177741, #10883, #165563, #39210, #88706, #103883, #27060, #73561, #102880, #163563, #118059, #54380, #26059, #176743, #134231, #148391, #116052, #84694, #101881, #162548, #25063, #146374, #179749, #69548, #86706, #195916, #9885, #131212, #115051, #100866, #193909, #24052, #147394, #149387, #191889, #71545, #87702, #180746, #8882, #194902, #42222, #41219, #38216, #72553, #70550, #132217, #55373, #178738, #40201, #32012, #92668, #105864, #151390, #138193, #74545, #182720, #14856, #106853, #108842, #197885, #58373, #122022, #59354, #44205, #183713, #123995, #120040, #170523, #13853, #29046, #104875, #139179, #154356, #137195, #168528, #12880, #45199, #181727, #75520, #30026, #107834, #62325, #185693, #76517, #47183, #123011, #28063, #198881, #199876, #196906, #15849, #43208, #135234, #93669, #155354, #91664, #153354, #60348, #61340, #184697, #166564, #89704, #136210, #16844, #77508, #121023, #655, #167551, #90686 ),
 ( #152368, #46181, #169518, #31018, #17844, #18839, #146902, #145889, #126979, #99385, #85212, #50168, #110831, #84209, #63338, #94665, #48182, #125015, #116566, #176252, #70067, #1660, #177260, #171521, #114554, #8392, #163070, #131735, #33010, #109838, #161068, #193417, #54892, #178255, #37723, #115573, #79502, #39716, #186711, #100390, #38732, #34000, #156344, #141171, #162068, #22563, #101379, #142158, #78494, #2660, #69057, #140167, #7372, #64337, #130724, #192416, #126006, #187702, #53898, #80484, #23564, #49172, #172515, #95656, #65320, #157344, #3642, #188688, #44707, #56901, #181253, #149898, #88214, #26571, #9400, #71066, #135736, #13376, #102398, #197407, #104392, #105378, #42730, #198387, #75040, #40728, #118575, #183226, #150909, #151886, #182232, #57898, #119570, #58873, #103399, #180265, #24575, #117563, #27578, #132732, #41735, #74065, #12403, #87228, #89216, #165077, #90203, #166075, #164085, #59864, #11405, #167065, #25584, #148910, #28566, #120539, #43717, #73074, #10400, #136706, #196428, #121531, #72057, #106361, #194420, #86224, #147914, #133731, #179263, #134746, #195424, #55890, #199384, #32517, #60848, #1159, #172019, #62834, #184213, #29542, #77015, #170030, #138687, #45695, #125518, #168045, #124518, #79001, #95167, #92176, #186213, #156855, #155848, #18350, #2167, #109344, #137699, #171026, #80005, #141674, #64838, #187215, #168, #107346, #94169, #169019, #15359, #47694, #139671, #3165, #30524, #91175, #154858, #153861, #61836, #16356, #126500, #152864, #188198, #46690, #123506, #122523, #33508, #48686, #31520, #17345, #185199, #78004, #14359, #108351, #140675, #63846, #49670, #76024, #110338, #93173, #99146, #4143, #175009, #52649, #173024, #68818, #34503, #111334, #161830, #100149, #67821, #6139, #36473, #129476, #159827, #96161, #157850, #112331, #131489, #53655, #80989, #130477, #192174, #19342, #65822, #127491, #146651, #191175, #160835, #142664, #176015, #189196, #98130, #193176, #38493, #83974, #69822, #50671, #114313, #174021, #35492, #177023, #97142, #158825, #115332, #84969, #20313, #8145, #23325, #81961, #143653, #22324, #5137, #66819, #128482, #37484, #190178, #51653, #113317, #145654, #7135, #21322, #82980, #144656, #73834, #150671, #10162, #101140, #24335, #12169, #149666, #89975, #118336, #105149, #162826, #42493, #151656, #196194, #70829, #57666, #165838, #28336, #13150, #87978, #195182, #119333, #39479, #55651, #74813, #41498, #117323, #136475, #180029, #54649, #86987, #11164, #103162, #164842, #56663, #85985, #147674, #27335, #43482, #132497, #88981, #134508, #135505, #72838, #116323, #166835, #194186, #148674, #178012, #181019, #181999, #197175, #104157, #58640, #120306, #133490, #71822, #9162, #179019, #40487, #102159, #26338, #163845, #25346, #137464, #31284, #168785, #170790, #184963, #152629, #78763, #45460, #185971, #14119, #75786, #109111, #46447, #92935, #107114, #199144, #169791, #154623, #140440, #16117, #32282, #153624, #15120, #121299, #77774, #182991, #76782, #44474, #139441, #60610, #91932, #93937, #923, #138453, #108107, #155616, #61603, #183974, #62597, #106129, #122285, #167813, #29312, #17112, #123272, #1930, #59625, #124275, #90942, #47455, #63609, #198155, #30287, #200134, #163494, #57316, #88632, #151317, #105791, #28972, #58302, #90614, #166492, #71475, #42151, #119969, #40128, #136138, #101806, #178665, #152296, #167477, #135161, #73488, #103811, #196834, #26987, #24992, #86636, #179676, #198808, #120949, #148319, #197814, #59279, #9814, #133140, #194831, #13780, #181655, #27990, #56304, #43134, #117986, #165491, #60273, #75447, #12806, #137122, #41148, #104803, #102811, #164496, #44132, #25989, #87632, #182648, #149318, #10812, #72482, #134155, #195843, #118992, #89629, #150328, #74473, #180675, #11823, #170562, #18878, #110869, #173556, #35025, #33048, #140206, #64376, #184736, #695, #96680, #186750, #62367, #158368, #63376 ),
 ( #80524, #17885, #19857, #50212, #15890, #93709, #81497, #126044, #127020, #157385, #94703, #156380, #34040, #78532, #155391, #199915, #92707, #2699, #46221, #16881, #49211, #187740, #124036, #172554, #1700, #65359, #79539, #77548, #61379, #32052, #142198, #139220, #185735, #3681, #95697, #154395, #141209, #188727, #123050, #111866, #47224, #169562, #107874, #31059, #108883, #125053, #48220, #109874, #171558, #178544, #51192, #162358, #39021, #98669, #189719, #112853, #100676, #38023, #40010, #6665, #193715, #174544, #131016, #176547, #36011, #113838, #23859, #54189, #116853, #101683, #99679, #83504, #7664, #128017, #144185, #163372, #129994, #5671, #24869, #68343, #143184, #175534, #161363, #191694, #53177, #145181, #97660, #159349, #115862, #132026, #20845, #177552, #22854, #85510, #84501, #4664, #55184, #82503, #37008, #66356, #69348, #70359, #147198, #146179, #192706, #8689, #21853, #160363, #67347, #129007, #190707, #52180, #114853, #136022, #74356, #149206, #151202, #103697, #152179, #43020, #164381, #121825, #118875, #167359, #25874, #87518, #90497, #104687, #12690, #180559, #10697, #89512, #27871, #183519, #197696, #13663, #88513, #150209, #9695, #59162, #71360, #11706, #194714, #120830, #72360, #26870, #75330, #182530, #135045, #166375, #137001, #58189, #42033, #44012, #133024, #102693, #56183, #117867, #45002, #181541, #198689, #179557, #106662, #73373, #60156, #41027, #105673, #119857, #134034, #57200, #28857, #168335, #86518, #148202, #195727, #196721, #165376, #14657, #30825, #65121, #16645, #92473, #188485, #93466, #49964, #62133, #186512, #155153, #78292, #31815, #76317, #137995, #140969, #18638, #107641, #2457, #109639, #110627, #47986, #3445, #80284, #45986, #123797, #111628, #156142, #157142, #187505, #63133, #124812, #64139, #108645, #185495, #29831, #122816, #32810, #199679, #46986, #79300, #17640, #154161, #94461, #170323, #141956, #139966, #1455, #61144, #33797, #48972, #171322, #125803, #169318, #172308, #184506, #95457, #126779, #91468, #153156, #15653, #77312, #138980, #458, #66114, #36762, #114606, #34788, #130774, #96443, #173313, #23619, #162122, #129757, #68105, #98425, #191454, #21610, #158130, #19622, #174308, #193469, #115625, #142945, #192466, #53949, #81264, #127779, #189479, #8445, #52931, #22616, #4427, #37775, #50957, #160122, #54946, #100442, #145943, #131789, #112616, #176303, #35777, #97424, #38785, #159110, #20604, #177314, #146957, #82256, #70118, #85266, #83268, #99439, #144942, #143948, #5428, #67112, #128770, #190469, #51942, #113602, #175296, #6424, #161119, #84262, #7424, #69108, #166132, #24628, #181308, #86276, #41789, #136760, #43771, #89275, #75093, #147967, #57954, #178307, #117620, #182291, #132785, #102451, #135791, #90257, #164139, #13429, #28620, #151940, #198445, #27634, #88269, #42786, #179318, #133788, #103456, #9455, #197462, #40782, #71119, #26626, #87280, #149957, #194472, #104449, #55944, #11463, #120596, #73134, #25636, #39770, #148965, #118630, #10454, #72115, #74120, #116618, #134804, #150965, #105435, #195480, #196484, #167120, #12460, #101434, #58928, #119625, #56956, #163125, #180321, #165134, #159625, #20124, #30582, #76077, #65632, #199437, #107403, #142475, #34311, #36277, #122581, #183280, #49479, #184269, #169076, #21120, #111142, #81768, #113122, #138742, #153919, #29595, #66624, #143455, #61892, #95974, #137753, #172832, #44762, #224, #157658, #35297, #189986, #174812, #3953, #97932, #50480, #152917, #123562, #127292, #121585, #4940, #106416, #59917, #82776, #51460, #19147, #80797, #144457, #173832, #189005, #112140, #45751, #77072, #188009, #91226, #128288, #92234, #14413, #96953, #15414, #158633, #60905, #168097, #37284, #39286, #9963, #100943, #22123, #67618, #115126, #7941, #176819, #83773, #163641, #5942, #162627, #117122, #133289, #130270, #24134, #194979, #193989, #56458, #40286, #147472, #175811, #8962 ),
 ( #52451, #99945, #55451, #178816, #25143, #38291, #161631, #118137, #85786, #145453, #41296, #23125, #86785, #6935, #68614, #71623, #70630, #132297, #84770, #191965, #101960, #148470, #102957, #179826, #164641, #69624, #131290, #129279, #26136, #190974, #192978, #114108, #87779, #53451, #146448, #98941, #160632, #54457, #116127, #177816, #121102, #181803, #152440, #134308, #165637, #119139, #195994, #184771, #44279, #138267, #72633, #45271, #42298, #182796, #14931, #31095, #76591, #103958, #180819, #167622, #61414, #199950, #123085, #105937, #183785, #150475, #46257, #57467, #168598, #106925, #104951, #27135, #88782, #30098, #29118, #107912, #11970, #73635, #60421, #169597, #135306, #122094, #90757, #91738, #13926, #149464, #10959, #196978, #43282, #58445, #75593, #120113, #153433, #137272, #198954, #166637, #28139, #89779, #151464, #12952, #74617, #136283, #197959, #59428, #80557, #111902, #125088, #1735, #4701, #49244, #170598, #128053, #186786, #173590, #32088, #93745, #96714, #110902, #18912, #48256, #155426, #95732, #34074, #189755, #142232, #158402, #94738, #156418, #15925, #157418, #77583, #17919, #731, #65394, #16916, #33082, #19891, #3717, #141243, #172588, #81532, #64409, #109910, #127055, #139255, #108918, #62403, #124073, #51227, #187774, #143219, #185774, #188762, #47261, #126078, #66391, #174582, #112888, #78569, #140243, #50246, #92743, #154431, #63413, #35059, #171594, #79574, #2732, #144222, #55217, #132060, #191728, #82540, #5706, #193749, #131051, #71392, #99712, #86550, #67383, #23892, #69382, #129040, #6699, #116886, #147231, #9728, #133056, #192741, #176582, #100709, #20882, #37046, #194746, #22888, #98705, #56218, #161396, #117900, #68377, #54223, #84534, #146211, #38056, #115894, #36047, #7699, #148234, #190741, #85545, #177584, #52215, #130029, #178578, #8723, #97696, #159387, #39051, #162389, #70392, #113872, #160399, #175569, #40043, #21888, #83538, #101717, #145217, #53210, #163407, #24903, #114888, #181572, #164413, #25905, #90527, #168366, #57232, #152209, #59192, #60187, #197726, #153186, #29862, #195758, #73404, #138028, #105704, #106693, #137030, #12720, #74386, #13693, #58218, #135075, #179589, #72392, #182561, #87550, #196751, #28887, #167391, #198720, #11737, #88544, #91499, #136051, #118906, #14689, #119887, #121857, #180590, #42064, #183549, #120861, #75360, #43050, #103728, #44044, #45035, #76351, #199711, #61176, #104716, #166407, #102724, #41061, #149237, #27902, #10728, #134068, #165408, #89545, #26901, #150242, #151231, #141000, #126808, #94491, #155185, #125834, #107672, #139011, #92505, #169349, #158159, #17672, #111658, #46016, #18667, #15684, #156173, #188516, #4453, #49993, #77345, #154194, #2488, #34816, #173345, #96471, #79330, #157173, #123828, #19651, #30858, #141986, #80313, #78324, #491, #62164, #3474, #65151, #47018, #185526, #32841, #93498, #64169, #108677, #187537, #170355, #49002, #81292, #110658, #31847, #184536, #16675, #124843, #139997, #1486, #142976, #122848, #172338, #33827, #63164, #186543, #95487, #48016, #109672, #171352, #100470, #7453, #35806, #69137, #54975, #193496, #163153, #23645, #36792, #82287, #130804, #5460, #113631, #145971, #37806, #39798, #128800, #189510, #52960, #190499, #175326, #24656, #114636, #85293, #116645, #144972, #160151, #97452, #70147, #146985, #68134, #99468, #143979, #176335, #50984, #6453, #161148, #38812, #178335, #101462, #192495, #86305, #53979, #159138, #129785, #115651, #127806, #8472, #112644, #66143, #147994, #174336, #22645, #84292, #191482, #177341, #162149, #20635, #67142, #51972, #98458, #131817, #21643, #83296, #167148, #194499, #164166, #102479, #44789, #27661, #58955, #117649, #74146, #179346, #134831, #29619, #136787, #182319, #168123, #40809, #150993, #71147, #10482, #75119, #25664, #195509, #28647, #183307, #56982, #106442, #121612, #91251, #9483, #120623, #181334, #135818, #72142 ),
 ( #55972, #43799, #198473, #87309, #105462, #89301, #90283, #12485, #132813, #59944, #148992, #103483, #133818, #197488, #118656, #151967, #42813, #104475, #13455, #88296, #165161, #180347, #41815, #26653, #149984, #11490, #73161, #196510, #57980, #119652, #166160, #64915, #109427, #30609, #188277, #185283, #33587, #92262, #153946, #156935, #171106, #79084, #46775, #15441, #155932, #94252, #49750, #140757, #18432, #154939, #16436, #76104, #17427, #137779, #78085, #60932, #125597, #77100, #93253, #80082, #2245, #1240, #32599, #141751, #124599, #108434, #63928, #199465, #169102, #122606, #184296, #111419, #47774, #3241, #45778, #48765, #107430, #186294, #126576, #34582, #173105, #138769, #250, #187294, #152942, #14441, #61919, #110420, #172101, #123589, #170110, #31604, #95250, #139753, #62919, #142743, #65901, #53742, #191253, #131577, #159913, #146737, #4223, #84059, #129553, #127575, #66900, #115416, #7218, #69911, #193261, #52728, #36555, #160915, #81065, #97219, #54735, #83060, #177105, #189276, #50752, #112410, #116407, #114393, #145737, #174102, #22408, #35571, #21402, #178096, #23408, #68903, #96239, #158905, #37565, #157927, #20396, #161914, #82043, #143740, #38576, #19417, #5219, #128563, #8233, #190258, #51735, #130562, #67900, #192260, #113397, #175087, #144734, #98209, #100232, #6221, #176095, #99228, #85056, #72925, #70913, #104240, #132581, #134594, #43566, #196280, #55736, #101224, #148757, #41583, #10246, #117410, #197258, #39566, #57749, #150756, #166919, #163934, #119419, #28420, #27419, #90057, #73916, #181103, #9246, #42577, #151739, #13232, #136558, #58720, #71905, #179107, #165923, #40576, #87072, #89065, #11251, #74895, #102246, #162913, #26422, #25431, #133577, #198239, #88062, #120389, #59710, #118422, #195267, #194269, #105231, #182083, #103247, #12254, #56751, #149749, #24421, #180115, #135586, #121383, #86070, #147760, #164929, #33358, #170875, #75872, #46538, #124363, #44558, #140527, #106213, #183075, #95017, #171869, #139525, #77858, #108197, #1008, #31372, #167897, #29397, #184061, #3013, #125371, #152713, #2017, #186059, #47542, #79857, #32366, #187067, #185050, #169879, #91027, #109196, #14204, #93022, #137548, #155700, #122372, #123357, #48537, #94019, #154710, #62682, #110191, #16203, #15207, #17195, #199231, #60696, #45544, #107199, #18199, #78849, #156705, #168869, #63696, #30374, #141525, #64690, #92018, #153711, #76866, #138536, #14, #61688, #53494, #192009, #82819, #160674, #127334, #161674, #34352, #145497, #22166, #81810, #172871, #96013, #83817, #21163, #23170, #190030, #176864, #157698, #114152, #159667, #19188, #96993, #6977, #37326, #99989, #84813, #144500, #66668, #191017, #111181, #189046, #146493, #113165, #50521, #7984, #51504, #126351, #158676, #112184, #142514, #68658, #188048, #5984, #98985, #115171, #173872, #67664, #38333, #175854, #49518, #130313, #129320, #80837, #52492, #3992, #65672, #35342, #20165, #143498, #4982, #128331, #174854, #36320, #97974, #44078, #46050, #132342, #193022, #59225, #194034, #178863, #30892, #120894, #91533, #122881, #151263, #166439, #39330, #76385, #29895, #74418, #105737, #85830, #182594, #54499, #12753, #13727, #131334, #70676, #138062, #147519, #55498, #153220, #107705, #117167, #169384, #184569, #92539, #154228, #183583, #167424, #137065, #43081, #89577, #197758, #100989, #14725, #104748, #162673, #28920, #27934, #90560, #24180, #198755, #9008, #152242, #199743, #75393, #136084, #60220, #121890, #69667, #45068, #106726, #61209, #116171, #168400, #177861, #143013, #140033, #33864, #4491, #3512, #66181, #50031, #157210, #185560, #18704, #127843, #189549, #112682, #173383, #186579, #31881, #80351, #155220, #63200, #95524, #187571, #51021, #78359, #139046, #2524, #1522, #124880, #174374, #64204, #34853, #35844, #94527, #109708, #47054, #19688, #96508, #17709, #49039, #93535, #125871, #526, #156209 ),
 ( #188553, #16709, #79366, #81330, #142023, #110694, #65188, #97490, #172374, #48052, #126847, #62198, #171390, #108711, #123862, #15718, #111696, #77378, #170390, #158198, #32877, #141037, #24695, #40846, #86344, #113668, #128836, #177379, #71186, #148031, #9520, #115691, #132850, #56009, #116682, #129823, #175362, #162187, #98496, #6491, #38851, #130843, #194538, #21679, #82325, #146009, #83333, #68171, #117687, #7492, #178372, #179384, #37846, #52999, #190535, #163191, #39836, #161187, #192534, #36830, #69177, #144015, #99506, #54017, #131855, #159176, #20671, #100508, #5496, #147025, #52009, #22683, #23685, #67179, #101502, #160189, #145010, #191522, #114677, #85333, #8509, #84330, #70187, #193538, #176373, #55012, #103522, #122643, #44826, #72183, #121649, #59982, #87346, #57021, #195547, #137819, #120659, #152005, #10520, #167185, #133857, #27696, #184333, #29657, #75156, #60969, #118694, #43835, #164203, #165198, #168160, #180386, #88333, #183344, #76141, #150024, #199503, #14479, #102520, #25701, #13491, #74184, #28684, #26693, #119687, #89337, #41856, #106481, #11529, #73199, #12520, #134869, #135854, #196547, #90319, #58017, #197524, #91289, #58992, #181370, #104514, #42849, #149032, #166195, #151029, #152980, #182357, #105499, #136827, #198511, #170146, #63963, #173140, #33622, #96274, #80116, #187330, #15481, #48801, #34615, #138807, #110455, #92300, #139789, #95285, #156969, #64950, #78120, #154975, #157960, #2280, #123624, #81099, #1277, #126609, #185319, #46810, #49788, #125632, #172136, #62954, #108469, #18465, #141784, #142777, #3278, #111454, #47811, #109461, #169142, #188311, #30647, #171144, #153984, #19451, #31641, #186329, #4258, #65937, #94287, #127609, #45815, #17462, #124635, #107466, #77138, #61957, #288, #93290, #16471, #140792, #32633, #155965, #79119, #82078, #22440, #54768, #70944, #116442, #143771, #158939, #7250, #101257, #178131, #39598, #145768, #23441, #190290, #24453, #97251, #8266, #85088, #144768, #35605, #20428, #146772, #84089, #86102, #52757, #162946, #5252, #177138, #68935, #66933, #159945, #69945, #100265, #147793, #9279, #130597, #129586, #53773, #174134, #51766, #189308, #176128, #113427, #50785, #112445, #6253, #128596, #175119, #114426, #37598, #191282, #36587, #98242, #161946, #21432, #83092, #131609, #192294, #193294, #115447, #67932, #99260, #160947, #38609, #91057, #58750, #59743, #90086, #165954, #27454, #166947, #11282, #26452, #132612, #104272, #106244, #195300, #55767, #119449, #56782, #41614, #152744, #181134, #151768, #183106, #72956, #88094, #102278, #136587, #13261, #134625, #89096, #148789, #42608, #117441, #196309, #150787, #105261, #121413, #44587, #12282, #167926, #120419, #25464, #57779, #73947, #194301, #74924, #179139, #40608, #29426, #14234, #135616, #197287, #182110, #43595, #28450, #163966, #87104, #133607, #10278, #198267, #71937, #118454, #180145, #103279, #164959, #149780, #111215, #94052, #125402, #184094, #140559, #45577, #1042, #96045, #3046, #48569, #34385, #107230, #17228, #137580, #76897, #141557, #92053, #61721, #95050, #49552, #123389, #172907, #188081, #157732, #75905, #187099, #47574, #2048, #138568, #93055, #62715, #168901, #156739, #46, #30407, #186092, #46570, #109226, #153743, #63727, #15238, #170905, #79887, #32397, #185081, #77890, #108231, #199263, #169912, #31404, #33391, #60730, #155730, #110222, #64722, #154742, #78880, #126384, #171903, #122404, #18233, #16238, #139558, #124397, #53526, #192045, #161709, #83848, #5017, #112214, #191050, #35373, #81841, #129355, #130346, #6018, #160708, #97025, #100022, #65703, #145530, #22199, #190059, #4025, #127369, #7009, #144532, #23205, #174887, #115204, #189081, #175888, #67697, #50554, #66699, #68691, #99017, #38367, #84848, #52523, #113198, #114184, #173904, #158706, #19221, #21197, #20195, #80871, #142547, #37359, #143529, #128363, #176896, #51535, #36353 ) ),
 .UNSPECIFIED., .T., .F., .F. ) 
 B_SPLINE_SURFACE_WITH_KNOTS ( ( 4, 3, 4 ),
 ( 3, 2, 2, 2, 2, 2, 2, 2, 2, 2, 2, 2, 2, 2, 2, 2, 2, 2, 2, 2, 2, 2, 2, 2, 2, 2, 2, 2, 2, 2, 2, 2, 2, 2, 2, 2, 2, 2, 2, 2, 2, 2, 2, 2, 2, 2, 2, 2, 2, 2, 2, 2, 2, 2, 2, 2, 2, 2, 2, 2, 2, 2, 2, 2, 2, 2, 2, 2, 2, 2, 2, 2, 2, 2, 2, 2, 2, 2, 2, 2, 2, 2, 2, 2, 2, 2, 2, 2, 2, 2, 2, 2, 2, 2, 2, 2, 2, 2, 2, 2, 2, 2, 2, 2, 2, 2, 2, 2, 2, 2, 2, 2, 2, 2, 2, 2, 2, 2, 2, 2, 2, 2, 2, 2, 2, 2, 2, 2, 2, 2, 2, 2, 2, 2, 2, 2, 2, 2, 2, 2, 2, 2, 2, 2, 2, 2, 2, 2, 2, 2, 2, 2, 2, 2, 2, 2, 2, 2, 2, 2, 2, 2, 2, 2, 2, 2, 2, 2, 2, 2, 2, 2, 2, 2, 2, 2, 2, 2, 2, 2, 2, 2, 2, 2, 2, 2, 2, 2, 2, 2, 2, 2, 2, 2, 2, 2, 2, 2, 2, 2, 2, 2, 2, 2, 2, 2, 2, 2, 2, 2, 2, 2, 2, 2, 2, 2, 2, 2, 2, 2, 2, 2, 2, 2, 2, 2, 2, 2, 3 ),
 ( 0.000000000000000000, 0.5000000000000000000, 1.000000000000000000 ),
 ( 0.000000000000000000, 0.004385964912280701511, 0.008771929824561403022, 0.01315789473684210453, 0.01754385964912280604, 0.02192982456140350755, 0.02631578947368420907, 0.03070175438596491058, 0.03508771929824561209, 0.03947368421052631360, 0.04385964912280701511, 0.04824561403508771662, 0.05263157894736841813, 0.05701754385964911964, 0.06140350877192982115, 0.06578947368421052266, 0.07017543859649122417, 0.07456140350877192569, 0.07894736842105262720, 0.08333333333333332871, 0.08771929824561403022, 0.09210526315789473173, 0.09649122807017543324, 0.1008771929824561348, 0.1052631578947368363, 0.1096491228070175378, 0.1140350877192982393, 0.1184210526315789408, 0.1228070175438596423, 0.1271929824561403577, 0.1315789473684210453, 0.1359649122807017607, 0.1403508771929824483, 0.1447368421052631637, 0.1491228070175438514, 0.1535087719298245668, 0.1578947368421052544, 0.1622807017543859698, 0.1666666666666666574, 0.1710526315789473728, 0.1754385964912280604, 0.1798245614035087758, 0.1842105263157894635, 0.1885964912280701788, 0.1929824561403508665, 0.1973684210526315819, 0.2017543859649122695, 0.2061403508771929849, 0.2105263157894736725, 0.2149122807017543879, 0.2192982456140350755, 0.2236842105263157909, 0.2280701754385964786, 0.2324561403508771940, 0.2368421052631578816, 0.2412280701754385970, 0.2456140350877192846, 0.2500000000000000000, 0.2543859649122807154, 0.2587719298245614308, 0.2631578947368420907, 0.2675438596491228060, 0.2719298245614035214, 0.2763157894736842368, 0.2807017543859648967, 0.2850877192982456121, 0.2894736842105263275, 0.2938596491228070429, 0.2982456140350877027, 0.3026315789473684181, 0.3070175438596491335, 0.3114035087719298489, 0.3157894736842105088, 0.3201754385964912242, 0.3245614035087719396, 0.3289473684210526550, 0.3333333333333333148, 0.3377192982456140302, 0.3421052631578947456, 0.3464912280701754610, 0.3508771929824561209, 0.3552631578947368363, 0.3596491228070175517, 0.3640350877192982670, 0.3684210526315789269, 0.3728070175438596423, 0.3771929824561403577, 0.3815789473684210731, 0.3859649122807017330, 0.3903508771929824483, 0.3947368421052631637, 0.3991228070175438791, 0.4035087719298245390, 0.4078947368421052544, 0.4122807017543859698, 0.4166666666666666852, 0.4210526315789473450, 0.4254385964912280604, 0.4298245614035087758, 0.4342105263157894912, 0.4385964912280701511, 0.4429824561403508665, 0.4473684210526315819, 0.4517543859649122973, 0.4561403508771929571, 0.4605263157894736725, 0.4649122807017543879, 0.4692982456140351033, 0.4736842105263157632, 0.4780701754385964786, 0.4824561403508771940, 0.4868421052631579093, 0.4912280701754385692, 0.4956140350877192846, 0.5000000000000000000, 0.5043859649122807154, 0.5087719298245614308, 0.5131578947368421462, 0.5175438596491228616, 0.5219298245614034659, 0.5263157894736841813, 0.5307017543859648967, 0.5350877192982456121, 0.5394736842105263275, 0.5438596491228070429, 0.5482456140350877583, 0.5526315789473684736, 0.5570175438596490780, 0.5614035087719297934, 0.5657894736842105088, 0.5701754385964912242, 0.5745614035087719396, 0.5789473684210526550, 0.5833333333333333703, 0.5877192982456140857, 0.5921052631578946901, 0.5964912280701754055, 0.6008771929824561209, 0.6052631578947368363, 0.6096491228070175517, 0.6140350877192982670, 0.6184210526315789824, 0.6228070175438596978, 0.6271929824561403022, 0.6315789473684210176, 0.6359649122807017330, 0.6403508771929824483, 0.6447368421052631637, 0.6491228070175438791, 0.6535087719298245945, 0.6578947368421053099, 0.6622807017543859143, 0.6666666666666666297, 0.6710526315789473450, 0.6754385964912280604, 0.6798245614035087758, 0.6842105263157894912, 0.6885964912280702066, 0.6929824561403509220, 0.6973684210526315264, 0.7017543859649122417, 0.7061403508771929571, 0.7105263157894736725, 0.7149122807017543879, 0.7192982456140351033, 0.7236842105263158187, 0.7280701754385965341, 0.7324561403508771384, 0.7368421052631578538, 0.7412280701754385692, 0.7456140350877192846, 0.7500000000000000000, 0.7543859649122807154, 0.7587719298245614308, 0.7631578947368421462, 0.7675438596491228616, 0.7719298245614034659, 0.7763157894736841813, 0.7807017543859648967, 0.7850877192982456121, 0.7894736842105263275, 0.7938596491228070429, 0.7982456140350877583, 0.8026315789473684736, 0.8070175438596490780, 0.8114035087719297934, 0.8157894736842105088, 0.8201754385964912242, 0.8245614035087719396, 0.8289473684210526550, 0.8333333333333333703, 0.8377192982456140857, 0.8421052631578946901, 0.8464912280701754055, 0.8508771929824561209, 0.8552631578947368363, 0.8596491228070175517, 0.8640350877192982670, 0.8684210526315789824, 0.8728070175438596978, 0.8771929824561403022, 0.8815789473684210176, 0.8859649122807017330, 0.8903508771929824483, 0.8947368421052631637, 0.8991228070175438791, 0.9035087719298245945, 0.9078947368421053099, 0.9122807017543859143, 0.9166666666666666297, 0.9210526315789473450, 0.9254385964912280604, 0.9298245614035087758, 0.9342105263157894912, 0.9385964912280702066, 0.9429824561403509220, 0.9473684210526315264, 0.9517543859649122417, 0.9561403508771929571, 0.9605263157894736725, 0.9649122807017543879, 0.9692982456140351033, 0.9736842105263158187, 0.9780701754385965341, 0.9824561403508771384, 0.9868421052631578538, 0.9912280701754385692, 0.9956140350877192846, 1.000000000000000000 ),
 .UNSPECIFIED. ) 
 GEOMETRIC_REPRESENTATION_ITEM ( )  RATIONAL_B_SPLINE_SURFACE ( (
 ( 1.000000000000000000, 0.9659258262890683122, 1.000000000000000000, 0.9659258262890683122, 1.000000000000000000, 0.9659258262890683122, 1.000000000000000000, 0.9659258262890683122, 1.000000000000000000, 0.9659258262890683122, 1.000000000000000000, 0.9659258262890683122, 1.000000000000000000, 0.9659258262890683122, 1.000000000000000000, 0.9659258262890683122, 1.000000000000000000, 0.9659258262890683122, 1.000000000000000000, 0.9659258262890683122, 1.000000000000000000, 0.9659258262890683122, 1.000000000000000000, 0.9659258262890683122, 1.000000000000000000, 0.9659258262890683122, 1.000000000000000000, 0.9659258262890683122, 1.000000000000000000, 0.9659258262890683122, 1.000000000000000000, 0.9659258262890683122, 1.000000000000000000, 0.9659258262890683122, 1.000000000000000000, 0.9659258262890683122, 1.000000000000000000, 0.9659258262890683122, 1.000000000000000000, 0.9659258262890683122, 1.000000000000000000, 0.9659258262890683122, 1.000000000000000000, 0.9659258262890683122, 1.000000000000000000, 0.9659258262890683122, 1.000000000000000000, 0.9659258262890683122, 1.000000000000000000, 0.9659258262890683122, 1.000000000000000000, 0.9659258262890683122, 1.000000000000000000, 0.9659258262890683122, 1.000000000000000000, 0.9659258262890683122, 1.000000000000000000, 0.9659258262890683122, 1.000000000000000000, 0.9659258262890683122, 1.000000000000000000, 0.9659258262890683122, 1.000000000000000000, 0.9659258262890683122, 1.000000000000000000, 0.9659258262890683122, 1.000000000000000000, 0.9659258262890683122, 1.000000000000000000, 0.9659258262890683122, 1.000000000000000000, 0.9659258262890683122, 1.000000000000000000, 0.9659258262890683122, 1.000000000000000000, 0.9659258262890683122, 1.000000000000000000, 0.9659258262890683122, 1.000000000000000000, 0.9659258262890683122, 1.000000000000000000, 0.9659258262890683122, 1.000000000000000000, 0.9659258262890683122, 1.000000000000000000, 0.9659258262890683122, 1.000000000000000000, 0.9659258262890683122, 1.000000000000000000, 0.9659258262890683122, 1.000000000000000000, 0.9659258262890683122, 1.000000000000000000, 0.9659258262890683122, 1.000000000000000000, 0.9659258262890683122, 1.000000000000000000, 0.9659258262890683122, 1.000000000000000000, 0.9659258262890683122, 1.000000000000000000, 0.9659258262890683122, 1.000000000000000000, 0.9659258262890683122, 1.000000000000000000, 0.9659258262890683122, 1.000000000000000000, 0.9659258262890683122, 1.000000000000000000, 0.9659258262890683122, 1.000000000000000000, 0.9659258262890683122, 1.000000000000000000, 0.9659258262890683122, 1.000000000000000000, 0.9659258262890683122, 1.000000000000000000, 0.9659258262890683122, 1.000000000000000000, 0.9659258262890683122, 1.000000000000000000, 0.9659258262890683122, 1.000000000000000000, 0.9659258262890683122, 1.000000000000000000, 0.9659258262890683122, 1.000000000000000000, 0.9659258262890683122, 1.000000000000000000, 0.9659258262890683122, 1.000000000000000000, 0.9659258262890683122, 1.000000000000000000, 0.9659258262890683122, 1.000000000000000000, 0.9659258262890683122, 1.000000000000000000, 0.9659258262890683122, 1.000000000000000000, 0.9659258262890683122, 1.000000000000000000, 0.9659258262890683122, 1.000000000000000000, 0.9659258262890683122, 1.000000000000000000, 0.9659258262890683122, 1.000000000000000000, 0.9659258262890683122, 1.000000000000000000, 0.9659258262890683122, 1.000000000000000000, 0.9659258262890683122, 1.000000000000000000, 0.9659258262890683122, 1.000000000000000000, 0.9659258262890683122, 1.000000000000000000, 0.9659258262890683122, 1.000000000000000000, 0.9659258262890683122, 1.000000000000000000, 0.9659258262890683122, 1.000000000000000000, 0.9659258262890683122, 1.000000000000000000, 0.9659258262890683122, 1.000000000000000000, 0.9659258262890683122, 1.000000000000000000, 0.9659258262890683122, 1.000000000000000000, 0.9659258262890683122, 1.000000000000000000, 0.9659258262890683122, 1.000000000000000000, 0.9659258262890683122, 1.000000000000000000, 0.9659258262890683122, 1.000000000000000000, 0.9659258262890683122, 1.000000000000000000, 0.9659258262890683122, 1.000000000000000000, 0.9659258262890683122, 1.000000000000000000, 0.9659258262890683122, 1.000000000000000000, 0.9659258262890683122, 1.000000000000000000, 0.9659258262890683122, 1.000000000000000000, 0.9659258262890683122, 1.000000000000000000, 0.9659258262890683122, 1.000000000000000000, 0.9659258262890683122, 1.000000000000000000, 0.9659258262890683122, 1.000000000000000000, 0.9659258262890683122, 1.000000000000000000, 0.9659258262890683122, 1.000000000000000000, 0.9659258262890683122, 1.000000000000000000, 0.9659258262890683122, 1.000000000000000000, 0.9659258262890683122, 1.000000000000000000, 0.9659258262890683122, 1.000000000000000000, 0.9659258262890683122, 1.000000000000000000, 0.9659258262890683122, 1.000000000000000000, 0.9659258262890683122, 1.000000000000000000, 0.9659258262890683122, 1.000000000000000000, 0.9659258262890683122, 1.000000000000000000, 0.9659258262890683122, 1.000000000000000000, 0.9659258262890683122, 1.000000000000000000, 0.9659258262890683122, 1.000000000000000000, 0.9659258262890683122, 1.000000000000000000, 0.9659258262890683122, 1.000000000000000000, 0.9659258262890683122, 1.000000000000000000, 0.9659258262890683122, 1.000000000000000000, 0.9659258262890683122, 1.000000000000000000, 0.9659258262890683122, 1.000000000000000000, 0.9659258262890683122, 1.000000000000000000, 0.9659258262890683122, 1.000000000000000000, 0.9659258262890683122, 1.000000000000000000, 0.9659258262890683122, 1.000000000000000000, 0.9659258262890683122, 1.000000000000000000, 0.9659258262890683122, 1.000000000000000000, 0.9659258262890683122, 1.000000000000000000, 0.9659258262890683122, 1.000000000000000000, 0.9659258262890683122, 1.000000000000000000, 0.9659258262890683122, 1.000000000000000000, 0.9659258262890683122, 1.000000000000000000, 0.9659258262890683122, 1.000000000000000000, 0.9659258262890683122, 1.000000000000000000, 0.9659258262890683122, 1.000000000000000000, 0.9659258262890683122, 1.000000000000000000, 0.9659258262890683122, 1.000000000000000000, 0.9659258262890683122, 1.000000000000000000, 0.9659258262890683122, 1.000000000000000000, 0.9659258262890683122, 1.000000000000000000, 0.9659258262890683122, 1.000000000000000000, 0.9659258262890683122, 1.000000000000000000, 0.9659258262890683122, 1.000000000000000000, 0.9659258262890683122, 1.000000000000000000, 0.9659258262890683122, 1.000000000000000000, 0.9659258262890683122, 1.000000000000000000, 0.9659258262890683122, 1.000000000000000000, 0.9659258262890683122, 1.000000000000000000, 0.9659258262890683122, 1.000000000000000000, 0.9659258262890683122, 1.000000000000000000, 0.9659258262890683122, 1.000000000000000000, 0.9659258262890683122, 1.000000000000000000, 0.9659258262890683122, 1.000000000000000000, 0.9659258262890683122, 1.000000000000000000, 0.9659258262890683122, 1.000000000000000000, 0.9659258262890683122, 1.000000000000000000, 0.9659258262890683122, 1.000000000000000000, 0.9659258262890683122, 1.000000000000000000, 0.9659258262890683122, 1.000000000000000000, 0.9659258262890683122, 1.000000000000000000, 0.9659258262890683122, 1.000000000000000000, 0.9659258262890683122, 1.000000000000000000, 0.9659258262890683122, 1.000000000000000000, 0.9659258262890683122, 1.000000000000000000, 0.9659258262890683122, 1.000000000000000000, 0.9659258262890683122, 1.000000000000000000, 0.9659258262890683122, 1.000000000000000000, 0.9659258262890683122, 1.000000000000000000, 0.9659258262890683122, 1.000000000000000000, 0.9659258262890683122, 1.000000000000000000, 0.9659258262890683122, 1.000000000000000000, 0.9659258262890683122, 1.000000000000000000, 0.9659258262890683122, 1.000000000000000000, 0.9659258262890683122, 1.000000000000000000, 0.9659258262890683122, 1.000000000000000000, 0.9659258262890683122, 1.000000000000000000, 0.9659258262890683122, 1.000000000000000000, 0.9659258262890683122, 1.000000000000000000, 0.9659258262890683122, 1.000000000000000000, 0.9659258262890683122, 1.000000000000000000, 0.9659258262890683122, 1.000000000000000000, 0.9659258262890683122, 1.000000000000000000, 0.9659258262890683122, 1.000000000000000000, 0.9659258262890683122, 1.000000000000000000, 0.9659258262890683122, 1.000000000000000000, 0.9659258262890683122, 1.000000000000000000, 0.9659258262890683122, 1.000000000000000000, 0.9659258262890683122, 1.000000000000000000, 0.9659258262890683122, 1.000000000000000000, 0.9659258262890683122, 1.000000000000000000, 0.9659258262890683122, 1.000000000000000000, 0.9659258262890683122, 1.000000000000000000, 0.9659258262890683122, 1.000000000000000000, 0.9659258262890683122, 1.000000000000000000, 0.9659258262890683122, 1.000000000000000000, 0.9659258262890683122, 1.000000000000000000, 0.9659258262890683122, 1.000000000000000000, 0.9659258262890683122, 1.000000000000000000, 0.9659258262890683122, 1.000000000000000000, 0.9659258262890683122, 1.000000000000000000, 0.9659258262890683122, 1.000000000000000000, 0.9659258262890683122, 1.000000000000000000, 0.9659258262890683122, 1.000000000000000000, 0.9659258262890683122, 1.000000000000000000, 0.9659258262890683122, 1.000000000000000000, 0.9659258262890683122, 1.000000000000000000, 0.9659258262890683122, 1.000000000000000000, 0.9659258262890683122, 1.000000000000000000, 0.9659258262890683122, 1.000000000000000000, 0.9659258262890683122, 1.000000000000000000, 0.9659258262890683122, 1.000000000000000000, 0.9659258262890683122, 1.000000000000000000, 0.9659258262890683122, 1.000000000000000000, 0.9659258262890683122, 1.000000000000000000, 0.9659258262890683122, 1.000000000000000000, 0.9659258262890683122, 1.000000000000000000, 0.9659258262890683122, 1.000000000000000000, 0.9659258262890683122, 1.000000000000000000, 0.9659258262890683122, 1.000000000000000000, 0.9659258262890683122, 1.000000000000000000, 0.9659258262890683122, 1.000000000000000000, 0.9659258262890683122, 1.000000000000000000, 0.9659258262890683122, 1.000000000000000000, 0.9659258262890683122, 1.000000000000000000, 0.9659258262890683122, 1.000000000000000000, 0.9659258262890683122, 1.000000000000000000, 0.9659258262890683122, 1.000000000000000000, 0.9659258262890683122, 1.000000000000000000, 0.9659258262890683122, 1.000000000000000000, 0.9659258262890683122, 1.000000000000000000),
 ( 0.3333333333333333703, 0.3219752754296894559, 0.3333333333333333703, 0.3219752754296894559, 0.3333333333333333703, 0.3219752754296894559, 0.3333333333333333703, 0.3219752754296894559, 0.3333333333333333703, 0.3219752754296894559, 0.3333333333333333703, 0.3219752754296894559, 0.3333333333333333703, 0.3219752754296894559, 0.3333333333333333703, 0.3219752754296894559, 0.3333333333333333703, 0.3219752754296894559, 0.3333333333333333703, 0.3219752754296894559, 0.3333333333333333703, 0.3219752754296894559, 0.3333333333333333703, 0.3219752754296894559, 0.3333333333333333703, 0.3219752754296894559, 0.3333333333333333703, 0.3219752754296894559, 0.3333333333333333703, 0.3219752754296894559, 0.3333333333333333703, 0.3219752754296894559, 0.3333333333333333703, 0.3219752754296894559, 0.3333333333333333703, 0.3219752754296894559, 0.3333333333333333703, 0.3219752754296894559, 0.3333333333333333703, 0.3219752754296894559, 0.3333333333333333703, 0.3219752754296894559, 0.3333333333333333703, 0.3219752754296894559, 0.3333333333333333703, 0.3219752754296894559, 0.3333333333333333703, 0.3219752754296894559, 0.3333333333333333703, 0.3219752754296894559, 0.3333333333333333703, 0.3219752754296894559, 0.3333333333333333703, 0.3219752754296894559, 0.3333333333333333703, 0.3219752754296894559, 0.3333333333333333703, 0.3219752754296894559, 0.3333333333333333703, 0.3219752754296894559, 0.3333333333333333703, 0.3219752754296894559, 0.3333333333333333703, 0.3219752754296894559, 0.3333333333333333703, 0.3219752754296894559, 0.3333333333333333703, 0.3219752754296894559, 0.3333333333333333703, 0.3219752754296894559, 0.3333333333333333703, 0.3219752754296894559, 0.3333333333333333703, 0.3219752754296894559, 0.3333333333333333703, 0.3219752754296894559, 0.3333333333333333703, 0.3219752754296894559, 0.3333333333333333703, 0.3219752754296894559, 0.3333333333333333703, 0.3219752754296894559, 0.3333333333333333703, 0.3219752754296894559, 0.3333333333333333703, 0.3219752754296894559, 0.3333333333333333703, 0.3219752754296894559, 0.3333333333333333703, 0.3219752754296894559, 0.3333333333333333703, 0.3219752754296894559, 0.3333333333333333703, 0.3219752754296894559, 0.3333333333333333703, 0.3219752754296894559, 0.3333333333333333703, 0.3219752754296894559, 0.3333333333333333703, 0.3219752754296894559, 0.3333333333333333703, 0.3219752754296894559, 0.3333333333333333703, 0.3219752754296894559, 0.3333333333333333703, 0.3219752754296894559, 0.3333333333333333703, 0.3219752754296894559, 0.3333333333333333703, 0.3219752754296894559, 0.3333333333333333703, 0.3219752754296894559, 0.3333333333333333703, 0.3219752754296894559, 0.3333333333333333703, 0.3219752754296894559, 0.3333333333333333703, 0.3219752754296894559, 0.3333333333333333703, 0.3219752754296894559, 0.3333333333333333703, 0.3219752754296894559, 0.3333333333333333703, 0.3219752754296894559, 0.3333333333333333703, 0.3219752754296894559, 0.3333333333333333703, 0.3219752754296894559, 0.3333333333333333703, 0.3219752754296894559, 0.3333333333333333703, 0.3219752754296894559, 0.3333333333333333703, 0.3219752754296894559, 0.3333333333333333703, 0.3219752754296894559, 0.3333333333333333703, 0.3219752754296894559, 0.3333333333333333703, 0.3219752754296894559, 0.3333333333333333703, 0.3219752754296894559, 0.3333333333333333703, 0.3219752754296894559, 0.3333333333333333703, 0.3219752754296894559, 0.3333333333333333703, 0.3219752754296894559, 0.3333333333333333703, 0.3219752754296894559, 0.3333333333333333703, 0.3219752754296894559, 0.3333333333333333703, 0.3219752754296894559, 0.3333333333333333703, 0.3219752754296894559, 0.3333333333333333703, 0.3219752754296894559, 0.3333333333333333703, 0.3219752754296894559, 0.3333333333333333703, 0.3219752754296894559, 0.3333333333333333703, 0.3219752754296894559, 0.3333333333333333703, 0.3219752754296894559, 0.3333333333333333703, 0.3219752754296894559, 0.3333333333333333703, 0.3219752754296894559, 0.3333333333333333703, 0.3219752754296894559, 0.3333333333333333703, 0.3219752754296894559, 0.3333333333333333703, 0.3219752754296894559, 0.3333333333333333703, 0.3219752754296894559, 0.3333333333333333703, 0.3219752754296894559, 0.3333333333333333703, 0.3219752754296894559, 0.3333333333333333703, 0.3219752754296894559, 0.3333333333333333703, 0.3219752754296894559, 0.3333333333333333703, 0.3219752754296894559, 0.3333333333333333703, 0.3219752754296894559, 0.3333333333333333703, 0.3219752754296894559, 0.3333333333333333703, 0.3219752754296894559, 0.3333333333333333703, 0.3219752754296894559, 0.3333333333333333703, 0.3219752754296894559, 0.3333333333333333703, 0.3219752754296894559, 0.3333333333333333703, 0.3219752754296894559, 0.3333333333333333703, 0.3219752754296894559, 0.3333333333333333703, 0.3219752754296894559, 0.3333333333333333703, 0.3219752754296894559, 0.3333333333333333703, 0.3219752754296894559, 0.3333333333333333703, 0.3219752754296894559, 0.3333333333333333703, 0.3219752754296894559, 0.3333333333333333703, 0.3219752754296894559, 0.3333333333333333703, 0.3219752754296894559, 0.3333333333333333703, 0.3219752754296894559, 0.3333333333333333703, 0.3219752754296894559, 0.3333333333333333703, 0.3219752754296894559, 0.3333333333333333703, 0.3219752754296894559, 0.3333333333333333703, 0.3219752754296894559, 0.3333333333333333703, 0.3219752754296894559, 0.3333333333333333703, 0.3219752754296894559, 0.3333333333333333703, 0.3219752754296894559, 0.3333333333333333703, 0.3219752754296894559, 0.3333333333333333703, 0.3219752754296894559, 0.3333333333333333703, 0.3219752754296894559, 0.3333333333333333703, 0.3219752754296894559, 0.3333333333333333703, 0.3219752754296894559, 0.3333333333333333703, 0.3219752754296894559, 0.3333333333333333703, 0.3219752754296894559, 0.3333333333333333703, 0.3219752754296894559, 0.3333333333333333703, 0.3219752754296894559, 0.3333333333333333703, 0.3219752754296894559, 0.3333333333333333703, 0.3219752754296894559, 0.3333333333333333703, 0.3219752754296894559, 0.3333333333333333703, 0.3219752754296894559, 0.3333333333333333703, 0.3219752754296894559, 0.3333333333333333703, 0.3219752754296894559, 0.3333333333333333703, 0.3219752754296894559, 0.3333333333333333703, 0.3219752754296894559, 0.3333333333333333703, 0.3219752754296894559, 0.3333333333333333703, 0.3219752754296894559, 0.3333333333333333703, 0.3219752754296894559, 0.3333333333333333703, 0.3219752754296894559, 0.3333333333333333703, 0.3219752754296894559, 0.3333333333333333703, 0.3219752754296894559, 0.3333333333333333703, 0.3219752754296894559, 0.3333333333333333703, 0.3219752754296894559, 0.3333333333333333703, 0.3219752754296894559, 0.3333333333333333703, 0.3219752754296894559, 0.3333333333333333703, 0.3219752754296894559, 0.3333333333333333703, 0.3219752754296894559, 0.3333333333333333703, 0.3219752754296894559, 0.3333333333333333703, 0.3219752754296894559, 0.3333333333333333703, 0.3219752754296894559, 0.3333333333333333703, 0.3219752754296894559, 0.3333333333333333703, 0.3219752754296894559, 0.3333333333333333703, 0.3219752754296894559, 0.3333333333333333703, 0.3219752754296894559, 0.3333333333333333703, 0.3219752754296894559, 0.3333333333333333703, 0.3219752754296894559, 0.3333333333333333703, 0.3219752754296894559, 0.3333333333333333703, 0.3219752754296894559, 0.3333333333333333703, 0.3219752754296894559, 0.3333333333333333703, 0.3219752754296894559, 0.3333333333333333703, 0.3219752754296894559, 0.3333333333333333703, 0.3219752754296894559, 0.3333333333333333703, 0.3219752754296894559, 0.3333333333333333703, 0.3219752754296894559, 0.3333333333333333703, 0.3219752754296894559, 0.3333333333333333703, 0.3219752754296894559, 0.3333333333333333703, 0.3219752754296894559, 0.3333333333333333703, 0.3219752754296894559, 0.3333333333333333703, 0.3219752754296894559, 0.3333333333333333703, 0.3219752754296894559, 0.3333333333333333703, 0.3219752754296894559, 0.3333333333333333703, 0.3219752754296894559, 0.3333333333333333703, 0.3219752754296894559, 0.3333333333333333703, 0.3219752754296894559, 0.3333333333333333703, 0.3219752754296894559, 0.3333333333333333703, 0.3219752754296894559, 0.3333333333333333703, 0.3219752754296894559, 0.3333333333333333703, 0.3219752754296894559, 0.3333333333333333703, 0.3219752754296894559, 0.3333333333333333703, 0.3219752754296894559, 0.3333333333333333703, 0.3219752754296894559, 0.3333333333333333703, 0.3219752754296894559, 0.3333333333333333703, 0.3219752754296894559, 0.3333333333333333703, 0.3219752754296894559, 0.3333333333333333703, 0.3219752754296894559, 0.3333333333333333703, 0.3219752754296894559, 0.3333333333333333703, 0.3219752754296894559, 0.3333333333333333703, 0.3219752754296894559, 0.3333333333333333703, 0.3219752754296894559, 0.3333333333333333703, 0.3219752754296894559, 0.3333333333333333703, 0.3219752754296894559, 0.3333333333333333703, 0.3219752754296894559, 0.3333333333333333703, 0.3219752754296894559, 0.3333333333333333703, 0.3219752754296894559, 0.3333333333333333703, 0.3219752754296894559, 0.3333333333333333703, 0.3219752754296894559, 0.3333333333333333703, 0.3219752754296894559, 0.3333333333333333703, 0.3219752754296894559, 0.3333333333333333703, 0.3219752754296894559, 0.3333333333333333703, 0.3219752754296894559, 0.3333333333333333703, 0.3219752754296894559, 0.3333333333333333703, 0.3219752754296894559, 0.3333333333333333703, 0.3219752754296894559, 0.3333333333333333703, 0.3219752754296894559, 0.3333333333333333703, 0.3219752754296894559, 0.3333333333333333703, 0.3219752754296894559, 0.3333333333333333703, 0.3219752754296894559, 0.3333333333333333703, 0.3219752754296894559, 0.3333333333333333703, 0.3219752754296894559, 0.3333333333333333703, 0.3219752754296894559, 0.3333333333333333703, 0.3219752754296894559, 0.3333333333333333703, 0.3219752754296894559, 0.3333333333333333703, 0.3219752754296894559, 0.3333333333333333703, 0.3219752754296894559, 0.3333333333333333703, 0.3219752754296894559, 0.3333333333333333703, 0.3219752754296894559, 0.3333333333333333703, 0.3219752754296894559, 0.3333333333333333703, 0.3219752754296894559, 0.3333333333333333703, 0.3219752754296894559, 0.3333333333333333703, 0.3219752754296894559, 0.3333333333333333703, 0.3219752754296894559, 0.3333333333333333703, 0.3219752754296894559, 0.3333333333333333703, 0.3219752754296894559, 0.3333333333333333703, 0.3219752754296894559, 0.3333333333333333703, 0.3219752754296894559, 0.3333333333333333703, 0.3219752754296894559, 0.3333333333333333703, 0.3219752754296894559, 0.3333333333333333703, 0.3219752754296894559, 0.3333333333333333703, 0.3219752754296894559, 0.3333333333333333703),
 ( 0.3333333333333333703, 0.3219752754296894559, 0.3333333333333333703, 0.3219752754296894559, 0.3333333333333333703, 0.3219752754296894559, 0.3333333333333333703, 0.3219752754296894559, 0.3333333333333333703, 0.3219752754296894559, 0.3333333333333333703, 0.3219752754296894559, 0.3333333333333333703, 0.3219752754296894559, 0.3333333333333333703, 0.3219752754296894559, 0.3333333333333333703, 0.3219752754296894559, 0.3333333333333333703, 0.3219752754296894559, 0.3333333333333333703, 0.3219752754296894559, 0.3333333333333333703, 0.3219752754296894559, 0.3333333333333333703, 0.3219752754296894559, 0.3333333333333333703, 0.3219752754296894559, 0.3333333333333333703, 0.3219752754296894559, 0.3333333333333333703, 0.3219752754296894559, 0.3333333333333333703, 0.3219752754296894559, 0.3333333333333333703, 0.3219752754296894559, 0.3333333333333333703, 0.3219752754296894559, 0.3333333333333333703, 0.3219752754296894559, 0.3333333333333333703, 0.3219752754296894559, 0.3333333333333333703, 0.3219752754296894559, 0.3333333333333333703, 0.3219752754296894559, 0.3333333333333333703, 0.3219752754296894559, 0.3333333333333333703, 0.3219752754296894559, 0.3333333333333333703, 0.3219752754296894559, 0.3333333333333333703, 0.3219752754296894559, 0.3333333333333333703, 0.3219752754296894559, 0.3333333333333333703, 0.3219752754296894559, 0.3333333333333333703, 0.3219752754296894559, 0.3333333333333333703, 0.3219752754296894559, 0.3333333333333333703, 0.3219752754296894559, 0.3333333333333333703, 0.3219752754296894559, 0.3333333333333333703, 0.3219752754296894559, 0.3333333333333333703, 0.3219752754296894559, 0.3333333333333333703, 0.3219752754296894559, 0.3333333333333333703, 0.3219752754296894559, 0.3333333333333333703, 0.3219752754296894559, 0.3333333333333333703, 0.3219752754296894559, 0.3333333333333333703, 0.3219752754296894559, 0.3333333333333333703, 0.3219752754296894559, 0.3333333333333333703, 0.3219752754296894559, 0.3333333333333333703, 0.3219752754296894559, 0.3333333333333333703, 0.3219752754296894559, 0.3333333333333333703, 0.3219752754296894559, 0.3333333333333333703, 0.3219752754296894559, 0.3333333333333333703, 0.3219752754296894559, 0.3333333333333333703, 0.3219752754296894559, 0.3333333333333333703, 0.3219752754296894559, 0.3333333333333333703, 0.3219752754296894559, 0.3333333333333333703, 0.3219752754296894559, 0.3333333333333333703, 0.3219752754296894559, 0.3333333333333333703, 0.3219752754296894559, 0.3333333333333333703, 0.3219752754296894559, 0.3333333333333333703, 0.3219752754296894559, 0.3333333333333333703, 0.3219752754296894559, 0.3333333333333333703, 0.3219752754296894559, 0.3333333333333333703, 0.3219752754296894559, 0.3333333333333333703, 0.3219752754296894559, 0.3333333333333333703, 0.3219752754296894559, 0.3333333333333333703, 0.3219752754296894559, 0.3333333333333333703, 0.3219752754296894559, 0.3333333333333333703, 0.3219752754296894559, 0.3333333333333333703, 0.3219752754296894559, 0.3333333333333333703, 0.3219752754296894559, 0.3333333333333333703, 0.3219752754296894559, 0.3333333333333333703, 0.3219752754296894559, 0.3333333333333333703, 0.3219752754296894559, 0.3333333333333333703, 0.3219752754296894559, 0.3333333333333333703, 0.3219752754296894559, 0.3333333333333333703, 0.3219752754296894559, 0.3333333333333333703, 0.3219752754296894559, 0.3333333333333333703, 0.3219752754296894559, 0.3333333333333333703, 0.3219752754296894559, 0.3333333333333333703, 0.3219752754296894559, 0.3333333333333333703, 0.3219752754296894559, 0.3333333333333333703, 0.3219752754296894559, 0.3333333333333333703, 0.3219752754296894559, 0.3333333333333333703, 0.3219752754296894559, 0.3333333333333333703, 0.3219752754296894559, 0.3333333333333333703, 0.3219752754296894559, 0.3333333333333333703, 0.3219752754296894559, 0.3333333333333333703, 0.3219752754296894559, 0.3333333333333333703, 0.3219752754296894559, 0.3333333333333333703, 0.3219752754296894559, 0.3333333333333333703, 0.3219752754296894559, 0.3333333333333333703, 0.3219752754296894559, 0.3333333333333333703, 0.3219752754296894559, 0.3333333333333333703, 0.3219752754296894559, 0.3333333333333333703, 0.3219752754296894559, 0.3333333333333333703, 0.3219752754296894559, 0.3333333333333333703, 0.3219752754296894559, 0.3333333333333333703, 0.3219752754296894559, 0.3333333333333333703, 0.3219752754296894559, 0.3333333333333333703, 0.3219752754296894559, 0.3333333333333333703, 0.3219752754296894559, 0.3333333333333333703, 0.3219752754296894559, 0.3333333333333333703, 0.3219752754296894559, 0.3333333333333333703, 0.3219752754296894559, 0.3333333333333333703, 0.3219752754296894559, 0.3333333333333333703, 0.3219752754296894559, 0.3333333333333333703, 0.3219752754296894559, 0.3333333333333333703, 0.3219752754296894559, 0.3333333333333333703, 0.3219752754296894559, 0.3333333333333333703, 0.3219752754296894559, 0.3333333333333333703, 0.3219752754296894559, 0.3333333333333333703, 0.3219752754296894559, 0.3333333333333333703, 0.3219752754296894559, 0.3333333333333333703, 0.3219752754296894559, 0.3333333333333333703, 0.3219752754296894559, 0.3333333333333333703, 0.3219752754296894559, 0.3333333333333333703, 0.3219752754296894559, 0.3333333333333333703, 0.3219752754296894559, 0.3333333333333333703, 0.3219752754296894559, 0.3333333333333333703, 0.3219752754296894559, 0.3333333333333333703, 0.3219752754296894559, 0.3333333333333333703, 0.3219752754296894559, 0.3333333333333333703, 0.3219752754296894559, 0.3333333333333333703, 0.3219752754296894559, 0.3333333333333333703, 0.3219752754296894559, 0.3333333333333333703, 0.3219752754296894559, 0.3333333333333333703, 0.3219752754296894559, 0.3333333333333333703, 0.3219752754296894559, 0.3333333333333333703, 0.3219752754296894559, 0.3333333333333333703, 0.3219752754296894559, 0.3333333333333333703, 0.3219752754296894559, 0.3333333333333333703, 0.3219752754296894559, 0.3333333333333333703, 0.3219752754296894559, 0.3333333333333333703, 0.3219752754296894559, 0.3333333333333333703, 0.3219752754296894559, 0.3333333333333333703, 0.3219752754296894559, 0.3333333333333333703, 0.3219752754296894559, 0.3333333333333333703, 0.3219752754296894559, 0.3333333333333333703, 0.3219752754296894559, 0.3333333333333333703, 0.3219752754296894559, 0.3333333333333333703, 0.3219752754296894559, 0.3333333333333333703, 0.3219752754296894559, 0.3333333333333333703, 0.3219752754296894559, 0.3333333333333333703, 0.3219752754296894559, 0.3333333333333333703, 0.3219752754296894559, 0.3333333333333333703, 0.3219752754296894559, 0.3333333333333333703, 0.3219752754296894559, 0.3333333333333333703, 0.3219752754296894559, 0.3333333333333333703, 0.3219752754296894559, 0.3333333333333333703, 0.3219752754296894559, 0.3333333333333333703, 0.3219752754296894559, 0.3333333333333333703, 0.3219752754296894559, 0.3333333333333333703, 0.3219752754296894559, 0.3333333333333333703, 0.3219752754296894559, 0.3333333333333333703, 0.3219752754296894559, 0.3333333333333333703, 0.3219752754296894559, 0.3333333333333333703, 0.3219752754296894559, 0.3333333333333333703, 0.3219752754296894559, 0.3333333333333333703, 0.3219752754296894559, 0.3333333333333333703, 0.3219752754296894559, 0.3333333333333333703, 0.3219752754296894559, 0.3333333333333333703, 0.3219752754296894559, 0.3333333333333333703, 0.3219752754296894559, 0.3333333333333333703, 0.3219752754296894559, 0.3333333333333333703, 0.3219752754296894559, 0.3333333333333333703, 0.3219752754296894559, 0.3333333333333333703, 0.3219752754296894559, 0.3333333333333333703, 0.3219752754296894559, 0.3333333333333333703, 0.3219752754296894559, 0.3333333333333333703, 0.3219752754296894559, 0.3333333333333333703, 0.3219752754296894559, 0.3333333333333333703, 0.3219752754296894559, 0.3333333333333333703, 0.3219752754296894559, 0.3333333333333333703, 0.3219752754296894559, 0.3333333333333333703, 0.3219752754296894559, 0.3333333333333333703, 0.3219752754296894559, 0.3333333333333333703, 0.3219752754296894559, 0.3333333333333333703, 0.3219752754296894559, 0.3333333333333333703, 0.3219752754296894559, 0.3333333333333333703, 0.3219752754296894559, 0.3333333333333333703, 0.3219752754296894559, 0.3333333333333333703, 0.3219752754296894559, 0.3333333333333333703, 0.3219752754296894559, 0.3333333333333333703, 0.3219752754296894559, 0.3333333333333333703, 0.3219752754296894559, 0.3333333333333333703, 0.3219752754296894559, 0.3333333333333333703, 0.3219752754296894559, 0.3333333333333333703, 0.3219752754296894559, 0.3333333333333333703, 0.3219752754296894559, 0.3333333333333333703, 0.3219752754296894559, 0.3333333333333333703, 0.3219752754296894559, 0.3333333333333333703, 0.3219752754296894559, 0.3333333333333333703, 0.3219752754296894559, 0.3333333333333333703, 0.3219752754296894559, 0.3333333333333333703, 0.3219752754296894559, 0.3333333333333333703, 0.3219752754296894559, 0.3333333333333333703, 0.3219752754296894559, 0.3333333333333333703, 0.3219752754296894559, 0.3333333333333333703, 0.3219752754296894559, 0.3333333333333333703, 0.3219752754296894559, 0.3333333333333333703, 0.3219752754296894559, 0.3333333333333333703, 0.3219752754296894559, 0.3333333333333333703, 0.3219752754296894559, 0.3333333333333333703, 0.3219752754296894559, 0.3333333333333333703, 0.3219752754296894559, 0.3333333333333333703, 0.3219752754296894559, 0.3333333333333333703, 0.3219752754296894559, 0.3333333333333333703, 0.3219752754296894559, 0.3333333333333333703, 0.3219752754296894559, 0.3333333333333333703, 0.3219752754296894559, 0.3333333333333333703, 0.3219752754296894559, 0.3333333333333333703, 0.3219752754296894559, 0.3333333333333333703, 0.3219752754296894559, 0.3333333333333333703, 0.3219752754296894559, 0.3333333333333333703, 0.3219752754296894559, 0.3333333333333333703, 0.3219752754296894559, 0.3333333333333333703, 0.3219752754296894559, 0.3333333333333333703, 0.3219752754296894559, 0.3333333333333333703, 0.3219752754296894559, 0.3333333333333333703, 0.3219752754296894559, 0.3333333333333333703, 0.3219752754296894559, 0.3333333333333333703, 0.3219752754296894559, 0.3333333333333333703, 0.3219752754296894559, 0.3333333333333333703, 0.3219752754296894559, 0.3333333333333333703, 0.3219752754296894559, 0.3333333333333333703, 0.3219752754296894559, 0.3333333333333333703, 0.3219752754296894559, 0.3333333333333333703, 0.3219752754296894559, 0.3333333333333333703, 0.3219752754296894559, 0.3333333333333333703, 0.3219752754296894559, 0.3333333333333333703, 0.3219752754296894559, 0.3333333333333333703, 0.3219752754296894559, 0.3333333333333333703, 0.3219752754296894559, 0.3333333333333333703),
 ( 1.000000000000000000, 0.9659258262890683122, 1.000000000000000000, 0.9659258262890683122, 1.000000000000000000, 0.9659258262890683122, 1.000000000000000000, 0.9659258262890683122, 1.000000000000000000, 0.9659258262890683122, 1.000000000000000000, 0.9659258262890683122, 1.000000000000000000, 0.9659258262890683122, 1.000000000000000000, 0.9659258262890683122, 1.000000000000000000, 0.9659258262890683122, 1.000000000000000000, 0.9659258262890683122, 1.000000000000000000, 0.9659258262890683122, 1.000000000000000000, 0.9659258262890683122, 1.000000000000000000, 0.9659258262890683122, 1.000000000000000000, 0.9659258262890683122, 1.000000000000000000, 0.9659258262890683122, 1.000000000000000000, 0.9659258262890683122, 1.000000000000000000, 0.9659258262890683122, 1.000000000000000000, 0.9659258262890683122, 1.000000000000000000, 0.9659258262890683122, 1.000000000000000000, 0.9659258262890683122, 1.000000000000000000, 0.9659258262890683122, 1.000000000000000000, 0.9659258262890683122, 1.000000000000000000, 0.9659258262890683122, 1.000000000000000000, 0.9659258262890683122, 1.000000000000000000, 0.9659258262890683122, 1.000000000000000000, 0.9659258262890683122, 1.000000000000000000, 0.9659258262890683122, 1.000000000000000000, 0.9659258262890683122, 1.000000000000000000, 0.9659258262890683122, 1.000000000000000000, 0.9659258262890683122, 1.000000000000000000, 0.9659258262890683122, 1.000000000000000000, 0.9659258262890683122, 1.000000000000000000, 0.9659258262890683122, 1.000000000000000000, 0.9659258262890683122, 1.000000000000000000, 0.9659258262890683122, 1.000000000000000000, 0.9659258262890683122, 1.000000000000000000, 0.9659258262890683122, 1.000000000000000000, 0.9659258262890683122, 1.000000000000000000, 0.9659258262890683122, 1.000000000000000000, 0.9659258262890683122, 1.000000000000000000, 0.9659258262890683122, 1.000000000000000000, 0.9659258262890683122, 1.000000000000000000, 0.9659258262890683122, 1.000000000000000000, 0.9659258262890683122, 1.000000000000000000, 0.9659258262890683122, 1.000000000000000000, 0.9659258262890683122, 1.000000000000000000, 0.9659258262890683122, 1.000000000000000000, 0.9659258262890683122, 1.000000000000000000, 0.9659258262890683122, 1.000000000000000000, 0.9659258262890683122, 1.000000000000000000, 0.9659258262890683122, 1.000000000000000000, 0.9659258262890683122, 1.000000000000000000, 0.9659258262890683122, 1.000000000000000000, 0.9659258262890683122, 1.000000000000000000, 0.9659258262890683122, 1.000000000000000000, 0.9659258262890683122, 1.000000000000000000, 0.9659258262890683122, 1.000000000000000000, 0.9659258262890683122, 1.000000000000000000, 0.9659258262890683122, 1.000000000000000000, 0.9659258262890683122, 1.000000000000000000, 0.9659258262890683122, 1.000000000000000000, 0.9659258262890683122, 1.000000000000000000, 0.9659258262890683122, 1.000000000000000000, 0.9659258262890683122, 1.000000000000000000, 0.9659258262890683122, 1.000000000000000000, 0.9659258262890683122, 1.000000000000000000, 0.9659258262890683122, 1.000000000000000000, 0.9659258262890683122, 1.000000000000000000, 0.9659258262890683122, 1.000000000000000000, 0.9659258262890683122, 1.000000000000000000, 0.9659258262890683122, 1.000000000000000000, 0.9659258262890683122, 1.000000000000000000, 0.9659258262890683122, 1.000000000000000000, 0.9659258262890683122, 1.000000000000000000, 0.9659258262890683122, 1.000000000000000000, 0.9659258262890683122, 1.000000000000000000, 0.9659258262890683122, 1.000000000000000000, 0.9659258262890683122, 1.000000000000000000, 0.9659258262890683122, 1.000000000000000000, 0.9659258262890683122, 1.000000000000000000, 0.9659258262890683122, 1.000000000000000000, 0.9659258262890683122, 1.000000000000000000, 0.9659258262890683122, 1.000000000000000000, 0.9659258262890683122, 1.000000000000000000, 0.9659258262890683122, 1.000000000000000000, 0.9659258262890683122, 1.000000000000000000, 0.9659258262890683122, 1.000000000000000000, 0.9659258262890683122, 1.000000000000000000, 0.9659258262890683122, 1.000000000000000000, 0.9659258262890683122, 1.000000000000000000, 0.9659258262890683122, 1.000000000000000000, 0.9659258262890683122, 1.000000000000000000, 0.9659258262890683122, 1.000000000000000000, 0.9659258262890683122, 1.000000000000000000, 0.9659258262890683122, 1.000000000000000000, 0.9659258262890683122, 1.000000000000000000, 0.9659258262890683122, 1.000000000000000000, 0.9659258262890683122, 1.000000000000000000, 0.9659258262890683122, 1.000000000000000000, 0.9659258262890683122, 1.000000000000000000, 0.9659258262890683122, 1.000000000000000000, 0.9659258262890683122, 1.000000000000000000, 0.9659258262890683122, 1.000000000000000000, 0.9659258262890683122, 1.000000000000000000, 0.9659258262890683122, 1.000000000000000000, 0.9659258262890683122, 1.000000000000000000, 0.9659258262890683122, 1.000000000000000000, 0.9659258262890683122, 1.000000000000000000, 0.9659258262890683122, 1.000000000000000000, 0.9659258262890683122, 1.000000000000000000, 0.9659258262890683122, 1.000000000000000000, 0.9659258262890683122, 1.000000000000000000, 0.9659258262890683122, 1.000000000000000000, 0.9659258262890683122, 1.000000000000000000, 0.9659258262890683122, 1.000000000000000000, 0.9659258262890683122, 1.000000000000000000, 0.9659258262890683122, 1.000000000000000000, 0.9659258262890683122, 1.000000000000000000, 0.9659258262890683122, 1.000000000000000000, 0.9659258262890683122, 1.000000000000000000, 0.9659258262890683122, 1.000000000000000000, 0.9659258262890683122, 1.000000000000000000, 0.9659258262890683122, 1.000000000000000000, 0.9659258262890683122, 1.000000000000000000, 0.9659258262890683122, 1.000000000000000000, 0.9659258262890683122, 1.000000000000000000, 0.9659258262890683122, 1.000000000000000000, 0.9659258262890683122, 1.000000000000000000, 0.9659258262890683122, 1.000000000000000000, 0.9659258262890683122, 1.000000000000000000, 0.9659258262890683122, 1.000000000000000000, 0.9659258262890683122, 1.000000000000000000, 0.9659258262890683122, 1.000000000000000000, 0.9659258262890683122, 1.000000000000000000, 0.9659258262890683122, 1.000000000000000000, 0.9659258262890683122, 1.000000000000000000, 0.9659258262890683122, 1.000000000000000000, 0.9659258262890683122, 1.000000000000000000, 0.9659258262890683122, 1.000000000000000000, 0.9659258262890683122, 1.000000000000000000, 0.9659258262890683122, 1.000000000000000000, 0.9659258262890683122, 1.000000000000000000, 0.9659258262890683122, 1.000000000000000000, 0.9659258262890683122, 1.000000000000000000, 0.9659258262890683122, 1.000000000000000000, 0.9659258262890683122, 1.000000000000000000, 0.9659258262890683122, 1.000000000000000000, 0.9659258262890683122, 1.000000000000000000, 0.9659258262890683122, 1.000000000000000000, 0.9659258262890683122, 1.000000000000000000, 0.9659258262890683122, 1.000000000000000000, 0.9659258262890683122, 1.000000000000000000, 0.9659258262890683122, 1.000000000000000000, 0.9659258262890683122, 1.000000000000000000, 0.9659258262890683122, 1.000000000000000000, 0.9659258262890683122, 1.000000000000000000, 0.9659258262890683122, 1.000000000000000000, 0.9659258262890683122, 1.000000000000000000, 0.9659258262890683122, 1.000000000000000000, 0.9659258262890683122, 1.000000000000000000, 0.9659258262890683122, 1.000000000000000000, 0.9659258262890683122, 1.000000000000000000, 0.9659258262890683122, 1.000000000000000000, 0.9659258262890683122, 1.000000000000000000, 0.9659258262890683122, 1.000000000000000000, 0.9659258262890683122, 1.000000000000000000, 0.9659258262890683122, 1.000000000000000000, 0.9659258262890683122, 1.000000000000000000, 0.9659258262890683122, 1.000000000000000000, 0.9659258262890683122, 1.000000000000000000, 0.9659258262890683122, 1.000000000000000000, 0.9659258262890683122, 1.000000000000000000, 0.9659258262890683122, 1.000000000000000000, 0.9659258262890683122, 1.000000000000000000, 0.9659258262890683122, 1.000000000000000000, 0.9659258262890683122, 1.000000000000000000, 0.9659258262890683122, 1.000000000000000000, 0.9659258262890683122, 1.000000000000000000, 0.9659258262890683122, 1.000000000000000000, 0.9659258262890683122, 1.000000000000000000, 0.9659258262890683122, 1.000000000000000000, 0.9659258262890683122, 1.000000000000000000, 0.9659258262890683122, 1.000000000000000000, 0.9659258262890683122, 1.000000000000000000, 0.9659258262890683122, 1.000000000000000000, 0.9659258262890683122, 1.000000000000000000, 0.9659258262890683122, 1.000000000000000000, 0.9659258262890683122, 1.000000000000000000, 0.9659258262890683122, 1.000000000000000000, 0.9659258262890683122, 1.000000000000000000, 0.9659258262890683122, 1.000000000000000000, 0.9659258262890683122, 1.000000000000000000, 0.9659258262890683122, 1.000000000000000000, 0.9659258262890683122, 1.000000000000000000, 0.9659258262890683122, 1.000000000000000000, 0.9659258262890683122, 1.000000000000000000, 0.9659258262890683122, 1.000000000000000000, 0.9659258262890683122, 1.000000000000000000, 0.9659258262890683122, 1.000000000000000000, 0.9659258262890683122, 1.000000000000000000, 0.9659258262890683122, 1.000000000000000000, 0.9659258262890683122, 1.000000000000000000, 0.9659258262890683122, 1.000000000000000000, 0.9659258262890683122, 1.000000000000000000, 0.9659258262890683122, 1.000000000000000000, 0.9659258262890683122, 1.000000000000000000, 0.9659258262890683122, 1.000000000000000000, 0.9659258262890683122, 1.000000000000000000, 0.9659258262890683122, 1.000000000000000000, 0.9659258262890683122, 1.000000000000000000, 0.9659258262890683122, 1.000000000000000000, 0.9659258262890683122, 1.000000000000000000, 0.9659258262890683122, 1.000000000000000000, 0.9659258262890683122, 1.000000000000000000, 0.9659258262890683122, 1.000000000000000000, 0.9659258262890683122, 1.000000000000000000, 0.9659258262890683122, 1.000000000000000000, 0.9659258262890683122, 1.000000000000000000, 0.9659258262890683122, 1.000000000000000000, 0.9659258262890683122, 1.000000000000000000, 0.9659258262890683122, 1.000000000000000000, 0.9659258262890683122, 1.000000000000000000, 0.9659258262890683122, 1.000000000000000000, 0.9659258262890683122, 1.000000000000000000, 0.9659258262890683122, 1.000000000000000000, 0.9659258262890683122, 1.000000000000000000, 0.9659258262890683122, 1.000000000000000000, 0.9659258262890683122, 1.000000000000000000),
 ( 0.3333333333333333703, 0.3219752754296894559, 0.3333333333333333703, 0.3219752754296894559, 0.3333333333333333703, 0.3219752754296894559, 0.3333333333333333703, 0.3219752754296894559, 0.3333333333333333703, 0.3219752754296894559, 0.3333333333333333703, 0.3219752754296894559, 0.3333333333333333703, 0.3219752754296894559, 0.3333333333333333703, 0.3219752754296894559, 0.3333333333333333703, 0.3219752754296894559, 0.3333333333333333703, 0.3219752754296894559, 0.3333333333333333703, 0.3219752754296894559, 0.3333333333333333703, 0.3219752754296894559, 0.3333333333333333703, 0.3219752754296894559, 0.3333333333333333703, 0.3219752754296894559, 0.3333333333333333703, 0.3219752754296894559, 0.3333333333333333703, 0.3219752754296894559, 0.3333333333333333703, 0.3219752754296894559, 0.3333333333333333703, 0.3219752754296894559, 0.3333333333333333703, 0.3219752754296894559, 0.3333333333333333703, 0.3219752754296894559, 0.3333333333333333703, 0.3219752754296894559, 0.3333333333333333703, 0.3219752754296894559, 0.3333333333333333703, 0.3219752754296894559, 0.3333333333333333703, 0.3219752754296894559, 0.3333333333333333703, 0.3219752754296894559, 0.3333333333333333703, 0.3219752754296894559, 0.3333333333333333703, 0.3219752754296894559, 0.3333333333333333703, 0.3219752754296894559, 0.3333333333333333703, 0.3219752754296894559, 0.3333333333333333703, 0.3219752754296894559, 0.3333333333333333703, 0.3219752754296894559, 0.3333333333333333703, 0.3219752754296894559, 0.3333333333333333703, 0.3219752754296894559, 0.3333333333333333703, 0.3219752754296894559, 0.3333333333333333703, 0.3219752754296894559, 0.3333333333333333703, 0.3219752754296894559, 0.3333333333333333703, 0.3219752754296894559, 0.3333333333333333703, 0.3219752754296894559, 0.3333333333333333703, 0.3219752754296894559, 0.3333333333333333703, 0.3219752754296894559, 0.3333333333333333703, 0.3219752754296894559, 0.3333333333333333703, 0.3219752754296894559, 0.3333333333333333703, 0.3219752754296894559, 0.3333333333333333703, 0.3219752754296894559, 0.3333333333333333703, 0.3219752754296894559, 0.3333333333333333703, 0.3219752754296894559, 0.3333333333333333703, 0.3219752754296894559, 0.3333333333333333703, 0.3219752754296894559, 0.3333333333333333703, 0.3219752754296894559, 0.3333333333333333703, 0.3219752754296894559, 0.3333333333333333703, 0.3219752754296894559, 0.3333333333333333703, 0.3219752754296894559, 0.3333333333333333703, 0.3219752754296894559, 0.3333333333333333703, 0.3219752754296894559, 0.3333333333333333703, 0.3219752754296894559, 0.3333333333333333703, 0.3219752754296894559, 0.3333333333333333703, 0.3219752754296894559, 0.3333333333333333703, 0.3219752754296894559, 0.3333333333333333703, 0.3219752754296894559, 0.3333333333333333703, 0.3219752754296894559, 0.3333333333333333703, 0.3219752754296894559, 0.3333333333333333703, 0.3219752754296894559, 0.3333333333333333703, 0.3219752754296894559, 0.3333333333333333703, 0.3219752754296894559, 0.3333333333333333703, 0.3219752754296894559, 0.3333333333333333703, 0.3219752754296894559, 0.3333333333333333703, 0.3219752754296894559, 0.3333333333333333703, 0.3219752754296894559, 0.3333333333333333703, 0.3219752754296894559, 0.3333333333333333703, 0.3219752754296894559, 0.3333333333333333703, 0.3219752754296894559, 0.3333333333333333703, 0.3219752754296894559, 0.3333333333333333703, 0.3219752754296894559, 0.3333333333333333703, 0.3219752754296894559, 0.3333333333333333703, 0.3219752754296894559, 0.3333333333333333703, 0.3219752754296894559, 0.3333333333333333703, 0.3219752754296894559, 0.3333333333333333703, 0.3219752754296894559, 0.3333333333333333703, 0.3219752754296894559, 0.3333333333333333703, 0.3219752754296894559, 0.3333333333333333703, 0.3219752754296894559, 0.3333333333333333703, 0.3219752754296894559, 0.3333333333333333703, 0.3219752754296894559, 0.3333333333333333703, 0.3219752754296894559, 0.3333333333333333703, 0.3219752754296894559, 0.3333333333333333703, 0.3219752754296894559, 0.3333333333333333703, 0.3219752754296894559, 0.3333333333333333703, 0.3219752754296894559, 0.3333333333333333703, 0.3219752754296894559, 0.3333333333333333703, 0.3219752754296894559, 0.3333333333333333703, 0.3219752754296894559, 0.3333333333333333703, 0.3219752754296894559, 0.3333333333333333703, 0.3219752754296894559, 0.3333333333333333703, 0.3219752754296894559, 0.3333333333333333703, 0.3219752754296894559, 0.3333333333333333703, 0.3219752754296894559, 0.3333333333333333703, 0.3219752754296894559, 0.3333333333333333703, 0.3219752754296894559, 0.3333333333333333703, 0.3219752754296894559, 0.3333333333333333703, 0.3219752754296894559, 0.3333333333333333703, 0.3219752754296894559, 0.3333333333333333703, 0.3219752754296894559, 0.3333333333333333703, 0.3219752754296894559, 0.3333333333333333703, 0.3219752754296894559, 0.3333333333333333703, 0.3219752754296894559, 0.3333333333333333703, 0.3219752754296894559, 0.3333333333333333703, 0.3219752754296894559, 0.3333333333333333703, 0.3219752754296894559, 0.3333333333333333703, 0.3219752754296894559, 0.3333333333333333703, 0.3219752754296894559, 0.3333333333333333703, 0.3219752754296894559, 0.3333333333333333703, 0.3219752754296894559, 0.3333333333333333703, 0.3219752754296894559, 0.3333333333333333703, 0.3219752754296894559, 0.3333333333333333703, 0.3219752754296894559, 0.3333333333333333703, 0.3219752754296894559, 0.3333333333333333703, 0.3219752754296894559, 0.3333333333333333703, 0.3219752754296894559, 0.3333333333333333703, 0.3219752754296894559, 0.3333333333333333703, 0.3219752754296894559, 0.3333333333333333703, 0.3219752754296894559, 0.3333333333333333703, 0.3219752754296894559, 0.3333333333333333703, 0.3219752754296894559, 0.3333333333333333703, 0.3219752754296894559, 0.3333333333333333703, 0.3219752754296894559, 0.3333333333333333703, 0.3219752754296894559, 0.3333333333333333703, 0.3219752754296894559, 0.3333333333333333703, 0.3219752754296894559, 0.3333333333333333703, 0.3219752754296894559, 0.3333333333333333703, 0.3219752754296894559, 0.3333333333333333703, 0.3219752754296894559, 0.3333333333333333703, 0.3219752754296894559, 0.3333333333333333703, 0.3219752754296894559, 0.3333333333333333703, 0.3219752754296894559, 0.3333333333333333703, 0.3219752754296894559, 0.3333333333333333703, 0.3219752754296894559, 0.3333333333333333703, 0.3219752754296894559, 0.3333333333333333703, 0.3219752754296894559, 0.3333333333333333703, 0.3219752754296894559, 0.3333333333333333703, 0.3219752754296894559, 0.3333333333333333703, 0.3219752754296894559, 0.3333333333333333703, 0.3219752754296894559, 0.3333333333333333703, 0.3219752754296894559, 0.3333333333333333703, 0.3219752754296894559, 0.3333333333333333703, 0.3219752754296894559, 0.3333333333333333703, 0.3219752754296894559, 0.3333333333333333703, 0.3219752754296894559, 0.3333333333333333703, 0.3219752754296894559, 0.3333333333333333703, 0.3219752754296894559, 0.3333333333333333703, 0.3219752754296894559, 0.3333333333333333703, 0.3219752754296894559, 0.3333333333333333703, 0.3219752754296894559, 0.3333333333333333703, 0.3219752754296894559, 0.3333333333333333703, 0.3219752754296894559, 0.3333333333333333703, 0.3219752754296894559, 0.3333333333333333703, 0.3219752754296894559, 0.3333333333333333703, 0.3219752754296894559, 0.3333333333333333703, 0.3219752754296894559, 0.3333333333333333703, 0.3219752754296894559, 0.3333333333333333703, 0.3219752754296894559, 0.3333333333333333703, 0.3219752754296894559, 0.3333333333333333703, 0.3219752754296894559, 0.3333333333333333703, 0.3219752754296894559, 0.3333333333333333703, 0.3219752754296894559, 0.3333333333333333703, 0.3219752754296894559, 0.3333333333333333703, 0.3219752754296894559, 0.3333333333333333703, 0.3219752754296894559, 0.3333333333333333703, 0.3219752754296894559, 0.3333333333333333703, 0.3219752754296894559, 0.3333333333333333703, 0.3219752754296894559, 0.3333333333333333703, 0.3219752754296894559, 0.3333333333333333703, 0.3219752754296894559, 0.3333333333333333703, 0.3219752754296894559, 0.3333333333333333703, 0.3219752754296894559, 0.3333333333333333703, 0.3219752754296894559, 0.3333333333333333703, 0.3219752754296894559, 0.3333333333333333703, 0.3219752754296894559, 0.3333333333333333703, 0.3219752754296894559, 0.3333333333333333703, 0.3219752754296894559, 0.3333333333333333703, 0.3219752754296894559, 0.3333333333333333703, 0.3219752754296894559, 0.3333333333333333703, 0.3219752754296894559, 0.3333333333333333703, 0.3219752754296894559, 0.3333333333333333703, 0.3219752754296894559, 0.3333333333333333703, 0.3219752754296894559, 0.3333333333333333703, 0.3219752754296894559, 0.3333333333333333703, 0.3219752754296894559, 0.3333333333333333703, 0.3219752754296894559, 0.3333333333333333703, 0.3219752754296894559, 0.3333333333333333703, 0.3219752754296894559, 0.3333333333333333703, 0.3219752754296894559, 0.3333333333333333703, 0.3219752754296894559, 0.3333333333333333703, 0.3219752754296894559, 0.3333333333333333703, 0.3219752754296894559, 0.3333333333333333703, 0.3219752754296894559, 0.3333333333333333703, 0.3219752754296894559, 0.3333333333333333703, 0.3219752754296894559, 0.3333333333333333703, 0.3219752754296894559, 0.3333333333333333703, 0.3219752754296894559, 0.3333333333333333703, 0.3219752754296894559, 0.3333333333333333703, 0.3219752754296894559, 0.3333333333333333703, 0.3219752754296894559, 0.3333333333333333703, 0.3219752754296894559, 0.3333333333333333703, 0.3219752754296894559, 0.3333333333333333703, 0.3219752754296894559, 0.3333333333333333703, 0.3219752754296894559, 0.3333333333333333703, 0.3219752754296894559, 0.3333333333333333703, 0.3219752754296894559, 0.3333333333333333703, 0.3219752754296894559, 0.3333333333333333703, 0.3219752754296894559, 0.3333333333333333703, 0.3219752754296894559, 0.3333333333333333703, 0.3219752754296894559, 0.3333333333333333703, 0.3219752754296894559, 0.3333333333333333703, 0.3219752754296894559, 0.3333333333333333703, 0.3219752754296894559, 0.3333333333333333703, 0.3219752754296894559, 0.3333333333333333703, 0.3219752754296894559, 0.3333333333333333703, 0.3219752754296894559, 0.3333333333333333703, 0.3219752754296894559, 0.3333333333333333703, 0.3219752754296894559, 0.3333333333333333703, 0.3219752754296894559, 0.3333333333333333703, 0.3219752754296894559, 0.3333333333333333703, 0.3219752754296894559, 0.3333333333333333703, 0.3219752754296894559, 0.3333333333333333703, 0.3219752754296894559, 0.3333333333333333703, 0.3219752754296894559, 0.3333333333333333703, 0.3219752754296894559, 0.3333333333333333703, 0.3219752754296894559, 0.3333333333333333703),
 ( 0.3333333333333333703, 0.3219752754296894559, 0.3333333333333333703, 0.3219752754296894559, 0.3333333333333333703, 0.3219752754296894559, 0.3333333333333333703, 0.3219752754296894559, 0.3333333333333333703, 0.3219752754296894559, 0.3333333333333333703, 0.3219752754296894559, 0.3333333333333333703, 0.3219752754296894559, 0.3333333333333333703, 0.3219752754296894559, 0.3333333333333333703, 0.3219752754296894559, 0.3333333333333333703, 0.3219752754296894559, 0.3333333333333333703, 0.3219752754296894559, 0.3333333333333333703, 0.3219752754296894559, 0.3333333333333333703, 0.3219752754296894559, 0.3333333333333333703, 0.3219752754296894559, 0.3333333333333333703, 0.3219752754296894559, 0.3333333333333333703, 0.3219752754296894559, 0.3333333333333333703, 0.3219752754296894559, 0.3333333333333333703, 0.3219752754296894559, 0.3333333333333333703, 0.3219752754296894559, 0.3333333333333333703, 0.3219752754296894559, 0.3333333333333333703, 0.3219752754296894559, 0.3333333333333333703, 0.3219752754296894559, 0.3333333333333333703, 0.3219752754296894559, 0.3333333333333333703, 0.3219752754296894559, 0.3333333333333333703, 0.3219752754296894559, 0.3333333333333333703, 0.3219752754296894559, 0.3333333333333333703, 0.3219752754296894559, 0.3333333333333333703, 0.3219752754296894559, 0.3333333333333333703, 0.3219752754296894559, 0.3333333333333333703, 0.3219752754296894559, 0.3333333333333333703, 0.3219752754296894559, 0.3333333333333333703, 0.3219752754296894559, 0.3333333333333333703, 0.3219752754296894559, 0.3333333333333333703, 0.3219752754296894559, 0.3333333333333333703, 0.3219752754296894559, 0.3333333333333333703, 0.3219752754296894559, 0.3333333333333333703, 0.3219752754296894559, 0.3333333333333333703, 0.3219752754296894559, 0.3333333333333333703, 0.3219752754296894559, 0.3333333333333333703, 0.3219752754296894559, 0.3333333333333333703, 0.3219752754296894559, 0.3333333333333333703, 0.3219752754296894559, 0.3333333333333333703, 0.3219752754296894559, 0.3333333333333333703, 0.3219752754296894559, 0.3333333333333333703, 0.3219752754296894559, 0.3333333333333333703, 0.3219752754296894559, 0.3333333333333333703, 0.3219752754296894559, 0.3333333333333333703, 0.3219752754296894559, 0.3333333333333333703, 0.3219752754296894559, 0.3333333333333333703, 0.3219752754296894559, 0.3333333333333333703, 0.3219752754296894559, 0.3333333333333333703, 0.3219752754296894559, 0.3333333333333333703, 0.3219752754296894559, 0.3333333333333333703, 0.3219752754296894559, 0.3333333333333333703, 0.3219752754296894559, 0.3333333333333333703, 0.3219752754296894559, 0.3333333333333333703, 0.3219752754296894559, 0.3333333333333333703, 0.3219752754296894559, 0.3333333333333333703, 0.3219752754296894559, 0.3333333333333333703, 0.3219752754296894559, 0.3333333333333333703, 0.3219752754296894559, 0.3333333333333333703, 0.3219752754296894559, 0.3333333333333333703, 0.3219752754296894559, 0.3333333333333333703, 0.3219752754296894559, 0.3333333333333333703, 0.3219752754296894559, 0.3333333333333333703, 0.3219752754296894559, 0.3333333333333333703, 0.3219752754296894559, 0.3333333333333333703, 0.3219752754296894559, 0.3333333333333333703, 0.3219752754296894559, 0.3333333333333333703, 0.3219752754296894559, 0.3333333333333333703, 0.3219752754296894559, 0.3333333333333333703, 0.3219752754296894559, 0.3333333333333333703, 0.3219752754296894559, 0.3333333333333333703, 0.3219752754296894559, 0.3333333333333333703, 0.3219752754296894559, 0.3333333333333333703, 0.3219752754296894559, 0.3333333333333333703, 0.3219752754296894559, 0.3333333333333333703, 0.3219752754296894559, 0.3333333333333333703, 0.3219752754296894559, 0.3333333333333333703, 0.3219752754296894559, 0.3333333333333333703, 0.3219752754296894559, 0.3333333333333333703, 0.3219752754296894559, 0.3333333333333333703, 0.3219752754296894559, 0.3333333333333333703, 0.3219752754296894559, 0.3333333333333333703, 0.3219752754296894559, 0.3333333333333333703, 0.3219752754296894559, 0.3333333333333333703, 0.3219752754296894559, 0.3333333333333333703, 0.3219752754296894559, 0.3333333333333333703, 0.3219752754296894559, 0.3333333333333333703, 0.3219752754296894559, 0.3333333333333333703, 0.3219752754296894559, 0.3333333333333333703, 0.3219752754296894559, 0.3333333333333333703, 0.3219752754296894559, 0.3333333333333333703, 0.3219752754296894559, 0.3333333333333333703, 0.3219752754296894559, 0.3333333333333333703, 0.3219752754296894559, 0.3333333333333333703, 0.3219752754296894559, 0.3333333333333333703, 0.3219752754296894559, 0.3333333333333333703, 0.3219752754296894559, 0.3333333333333333703, 0.3219752754296894559, 0.3333333333333333703, 0.3219752754296894559, 0.3333333333333333703, 0.3219752754296894559, 0.3333333333333333703, 0.3219752754296894559, 0.3333333333333333703, 0.3219752754296894559, 0.3333333333333333703, 0.3219752754296894559, 0.3333333333333333703, 0.3219752754296894559, 0.3333333333333333703, 0.3219752754296894559, 0.3333333333333333703, 0.3219752754296894559, 0.3333333333333333703, 0.3219752754296894559, 0.3333333333333333703, 0.3219752754296894559, 0.3333333333333333703, 0.3219752754296894559, 0.3333333333333333703, 0.3219752754296894559, 0.3333333333333333703, 0.3219752754296894559, 0.3333333333333333703, 0.3219752754296894559, 0.3333333333333333703, 0.3219752754296894559, 0.3333333333333333703, 0.3219752754296894559, 0.3333333333333333703, 0.3219752754296894559, 0.3333333333333333703, 0.3219752754296894559, 0.3333333333333333703, 0.3219752754296894559, 0.3333333333333333703, 0.3219752754296894559, 0.3333333333333333703, 0.3219752754296894559, 0.3333333333333333703, 0.3219752754296894559, 0.3333333333333333703, 0.3219752754296894559, 0.3333333333333333703, 0.3219752754296894559, 0.3333333333333333703, 0.3219752754296894559, 0.3333333333333333703, 0.3219752754296894559, 0.3333333333333333703, 0.3219752754296894559, 0.3333333333333333703, 0.3219752754296894559, 0.3333333333333333703, 0.3219752754296894559, 0.3333333333333333703, 0.3219752754296894559, 0.3333333333333333703, 0.3219752754296894559, 0.3333333333333333703, 0.3219752754296894559, 0.3333333333333333703, 0.3219752754296894559, 0.3333333333333333703, 0.3219752754296894559, 0.3333333333333333703, 0.3219752754296894559, 0.3333333333333333703, 0.3219752754296894559, 0.3333333333333333703, 0.3219752754296894559, 0.3333333333333333703, 0.3219752754296894559, 0.3333333333333333703, 0.3219752754296894559, 0.3333333333333333703, 0.3219752754296894559, 0.3333333333333333703, 0.3219752754296894559, 0.3333333333333333703, 0.3219752754296894559, 0.3333333333333333703, 0.3219752754296894559, 0.3333333333333333703, 0.3219752754296894559, 0.3333333333333333703, 0.3219752754296894559, 0.3333333333333333703, 0.3219752754296894559, 0.3333333333333333703, 0.3219752754296894559, 0.3333333333333333703, 0.3219752754296894559, 0.3333333333333333703, 0.3219752754296894559, 0.3333333333333333703, 0.3219752754296894559, 0.3333333333333333703, 0.3219752754296894559, 0.3333333333333333703, 0.3219752754296894559, 0.3333333333333333703, 0.3219752754296894559, 0.3333333333333333703, 0.3219752754296894559, 0.3333333333333333703, 0.3219752754296894559, 0.3333333333333333703, 0.3219752754296894559, 0.3333333333333333703, 0.3219752754296894559, 0.3333333333333333703, 0.3219752754296894559, 0.3333333333333333703, 0.3219752754296894559, 0.3333333333333333703, 0.3219752754296894559, 0.3333333333333333703, 0.3219752754296894559, 0.3333333333333333703, 0.3219752754296894559, 0.3333333333333333703, 0.3219752754296894559, 0.3333333333333333703, 0.3219752754296894559, 0.3333333333333333703, 0.3219752754296894559, 0.3333333333333333703, 0.3219752754296894559, 0.3333333333333333703, 0.3219752754296894559, 0.3333333333333333703, 0.3219752754296894559, 0.3333333333333333703, 0.3219752754296894559, 0.3333333333333333703, 0.3219752754296894559, 0.3333333333333333703, 0.3219752754296894559, 0.3333333333333333703, 0.3219752754296894559, 0.3333333333333333703, 0.3219752754296894559, 0.3333333333333333703, 0.3219752754296894559, 0.3333333333333333703, 0.3219752754296894559, 0.3333333333333333703, 0.3219752754296894559, 0.3333333333333333703, 0.3219752754296894559, 0.3333333333333333703, 0.3219752754296894559, 0.3333333333333333703, 0.3219752754296894559, 0.3333333333333333703, 0.3219752754296894559, 0.3333333333333333703, 0.3219752754296894559, 0.3333333333333333703, 0.3219752754296894559, 0.3333333333333333703, 0.3219752754296894559, 0.3333333333333333703, 0.3219752754296894559, 0.3333333333333333703, 0.3219752754296894559, 0.3333333333333333703, 0.3219752754296894559, 0.3333333333333333703, 0.3219752754296894559, 0.3333333333333333703, 0.3219752754296894559, 0.3333333333333333703, 0.3219752754296894559, 0.3333333333333333703, 0.3219752754296894559, 0.3333333333333333703, 0.3219752754296894559, 0.3333333333333333703, 0.3219752754296894559, 0.3333333333333333703, 0.3219752754296894559, 0.3333333333333333703, 0.3219752754296894559, 0.3333333333333333703, 0.3219752754296894559, 0.3333333333333333703, 0.3219752754296894559, 0.3333333333333333703, 0.3219752754296894559, 0.3333333333333333703, 0.3219752754296894559, 0.3333333333333333703, 0.3219752754296894559, 0.3333333333333333703, 0.3219752754296894559, 0.3333333333333333703, 0.3219752754296894559, 0.3333333333333333703, 0.3219752754296894559, 0.3333333333333333703, 0.3219752754296894559, 0.3333333333333333703, 0.3219752754296894559, 0.3333333333333333703, 0.3219752754296894559, 0.3333333333333333703, 0.3219752754296894559, 0.3333333333333333703, 0.3219752754296894559, 0.3333333333333333703, 0.3219752754296894559, 0.3333333333333333703, 0.3219752754296894559, 0.3333333333333333703, 0.3219752754296894559, 0.3333333333333333703, 0.3219752754296894559, 0.3333333333333333703, 0.3219752754296894559, 0.3333333333333333703, 0.3219752754296894559, 0.3333333333333333703, 0.3219752754296894559, 0.3333333333333333703, 0.3219752754296894559, 0.3333333333333333703, 0.3219752754296894559, 0.3333333333333333703, 0.3219752754296894559, 0.3333333333333333703, 0.3219752754296894559, 0.3333333333333333703, 0.3219752754296894559, 0.3333333333333333703, 0.3219752754296894559, 0.3333333333333333703, 0.3219752754296894559, 0.3333333333333333703, 0.3219752754296894559, 0.3333333333333333703, 0.3219752754296894559, 0.3333333333333333703, 0.3219752754296894559, 0.3333333333333333703, 0.3219752754296894559, 0.3333333333333333703, 0.3219752754296894559, 0.3333333333333333703, 0.3219752754296894559, 0.3333333333333333703, 0.3219752754296894559, 0.3333333333333333703),
 ( 1.000000000000000000, 0.9659258262890683122, 1.000000000000000000, 0.9659258262890683122, 1.000000000000000000, 0.9659258262890683122, 1.000000000000000000, 0.9659258262890683122, 1.000000000000000000, 0.9659258262890683122, 1.000000000000000000, 0.9659258262890683122, 1.000000000000000000, 0.9659258262890683122, 1.000000000000000000, 0.9659258262890683122, 1.000000000000000000, 0.9659258262890683122, 1.000000000000000000, 0.9659258262890683122, 1.000000000000000000, 0.9659258262890683122, 1.000000000000000000, 0.9659258262890683122, 1.000000000000000000, 0.9659258262890683122, 1.000000000000000000, 0.9659258262890683122, 1.000000000000000000, 0.9659258262890683122, 1.000000000000000000, 0.9659258262890683122, 1.000000000000000000, 0.9659258262890683122, 1.000000000000000000, 0.9659258262890683122, 1.000000000000000000, 0.9659258262890683122, 1.000000000000000000, 0.9659258262890683122, 1.000000000000000000, 0.9659258262890683122, 1.000000000000000000, 0.9659258262890683122, 1.000000000000000000, 0.9659258262890683122, 1.000000000000000000, 0.9659258262890683122, 1.000000000000000000, 0.9659258262890683122, 1.000000000000000000, 0.9659258262890683122, 1.000000000000000000, 0.9659258262890683122, 1.000000000000000000, 0.9659258262890683122, 1.000000000000000000, 0.9659258262890683122, 1.000000000000000000, 0.9659258262890683122, 1.000000000000000000, 0.9659258262890683122, 1.000000000000000000, 0.9659258262890683122, 1.000000000000000000, 0.9659258262890683122, 1.000000000000000000, 0.9659258262890683122, 1.000000000000000000, 0.9659258262890683122, 1.000000000000000000, 0.9659258262890683122, 1.000000000000000000, 0.9659258262890683122, 1.000000000000000000, 0.9659258262890683122, 1.000000000000000000, 0.9659258262890683122, 1.000000000000000000, 0.9659258262890683122, 1.000000000000000000, 0.9659258262890683122, 1.000000000000000000, 0.9659258262890683122, 1.000000000000000000, 0.9659258262890683122, 1.000000000000000000, 0.9659258262890683122, 1.000000000000000000, 0.9659258262890683122, 1.000000000000000000, 0.9659258262890683122, 1.000000000000000000, 0.9659258262890683122, 1.000000000000000000, 0.9659258262890683122, 1.000000000000000000, 0.9659258262890683122, 1.000000000000000000, 0.9659258262890683122, 1.000000000000000000, 0.9659258262890683122, 1.000000000000000000, 0.9659258262890683122, 1.000000000000000000, 0.9659258262890683122, 1.000000000000000000, 0.9659258262890683122, 1.000000000000000000, 0.9659258262890683122, 1.000000000000000000, 0.9659258262890683122, 1.000000000000000000, 0.9659258262890683122, 1.000000000000000000, 0.9659258262890683122, 1.000000000000000000, 0.9659258262890683122, 1.000000000000000000, 0.9659258262890683122, 1.000000000000000000, 0.9659258262890683122, 1.000000000000000000, 0.9659258262890683122, 1.000000000000000000, 0.9659258262890683122, 1.000000000000000000, 0.9659258262890683122, 1.000000000000000000, 0.9659258262890683122, 1.000000000000000000, 0.9659258262890683122, 1.000000000000000000, 0.9659258262890683122, 1.000000000000000000, 0.9659258262890683122, 1.000000000000000000, 0.9659258262890683122, 1.000000000000000000, 0.9659258262890683122, 1.000000000000000000, 0.9659258262890683122, 1.000000000000000000, 0.9659258262890683122, 1.000000000000000000, 0.9659258262890683122, 1.000000000000000000, 0.9659258262890683122, 1.000000000000000000, 0.9659258262890683122, 1.000000000000000000, 0.9659258262890683122, 1.000000000000000000, 0.9659258262890683122, 1.000000000000000000, 0.9659258262890683122, 1.000000000000000000, 0.9659258262890683122, 1.000000000000000000, 0.9659258262890683122, 1.000000000000000000, 0.9659258262890683122, 1.000000000000000000, 0.9659258262890683122, 1.000000000000000000, 0.9659258262890683122, 1.000000000000000000, 0.9659258262890683122, 1.000000000000000000, 0.9659258262890683122, 1.000000000000000000, 0.9659258262890683122, 1.000000000000000000, 0.9659258262890683122, 1.000000000000000000, 0.9659258262890683122, 1.000000000000000000, 0.9659258262890683122, 1.000000000000000000, 0.9659258262890683122, 1.000000000000000000, 0.9659258262890683122, 1.000000000000000000, 0.9659258262890683122, 1.000000000000000000, 0.9659258262890683122, 1.000000000000000000, 0.9659258262890683122, 1.000000000000000000, 0.9659258262890683122, 1.000000000000000000, 0.9659258262890683122, 1.000000000000000000, 0.9659258262890683122, 1.000000000000000000, 0.9659258262890683122, 1.000000000000000000, 0.9659258262890683122, 1.000000000000000000, 0.9659258262890683122, 1.000000000000000000, 0.9659258262890683122, 1.000000000000000000, 0.9659258262890683122, 1.000000000000000000, 0.9659258262890683122, 1.000000000000000000, 0.9659258262890683122, 1.000000000000000000, 0.9659258262890683122, 1.000000000000000000, 0.9659258262890683122, 1.000000000000000000, 0.9659258262890683122, 1.000000000000000000, 0.9659258262890683122, 1.000000000000000000, 0.9659258262890683122, 1.000000000000000000, 0.9659258262890683122, 1.000000000000000000, 0.9659258262890683122, 1.000000000000000000, 0.9659258262890683122, 1.000000000000000000, 0.9659258262890683122, 1.000000000000000000, 0.9659258262890683122, 1.000000000000000000, 0.9659258262890683122, 1.000000000000000000, 0.9659258262890683122, 1.000000000000000000, 0.9659258262890683122, 1.000000000000000000, 0.9659258262890683122, 1.000000000000000000, 0.9659258262890683122, 1.000000000000000000, 0.9659258262890683122, 1.000000000000000000, 0.9659258262890683122, 1.000000000000000000, 0.9659258262890683122, 1.000000000000000000, 0.9659258262890683122, 1.000000000000000000, 0.9659258262890683122, 1.000000000000000000, 0.9659258262890683122, 1.000000000000000000, 0.9659258262890683122, 1.000000000000000000, 0.9659258262890683122, 1.000000000000000000, 0.9659258262890683122, 1.000000000000000000, 0.9659258262890683122, 1.000000000000000000, 0.9659258262890683122, 1.000000000000000000, 0.9659258262890683122, 1.000000000000000000, 0.9659258262890683122, 1.000000000000000000, 0.9659258262890683122, 1.000000000000000000, 0.9659258262890683122, 1.000000000000000000, 0.9659258262890683122, 1.000000000000000000, 0.9659258262890683122, 1.000000000000000000, 0.9659258262890683122, 1.000000000000000000, 0.9659258262890683122, 1.000000000000000000, 0.9659258262890683122, 1.000000000000000000, 0.9659258262890683122, 1.000000000000000000, 0.9659258262890683122, 1.000000000000000000, 0.9659258262890683122, 1.000000000000000000, 0.9659258262890683122, 1.000000000000000000, 0.9659258262890683122, 1.000000000000000000, 0.9659258262890683122, 1.000000000000000000, 0.9659258262890683122, 1.000000000000000000, 0.9659258262890683122, 1.000000000000000000, 0.9659258262890683122, 1.000000000000000000, 0.9659258262890683122, 1.000000000000000000, 0.9659258262890683122, 1.000000000000000000, 0.9659258262890683122, 1.000000000000000000, 0.9659258262890683122, 1.000000000000000000, 0.9659258262890683122, 1.000000000000000000, 0.9659258262890683122, 1.000000000000000000, 0.9659258262890683122, 1.000000000000000000, 0.9659258262890683122, 1.000000000000000000, 0.9659258262890683122, 1.000000000000000000, 0.9659258262890683122, 1.000000000000000000, 0.9659258262890683122, 1.000000000000000000, 0.9659258262890683122, 1.000000000000000000, 0.9659258262890683122, 1.000000000000000000, 0.9659258262890683122, 1.000000000000000000, 0.9659258262890683122, 1.000000000000000000, 0.9659258262890683122, 1.000000000000000000, 0.9659258262890683122, 1.000000000000000000, 0.9659258262890683122, 1.000000000000000000, 0.9659258262890683122, 1.000000000000000000, 0.9659258262890683122, 1.000000000000000000, 0.9659258262890683122, 1.000000000000000000, 0.9659258262890683122, 1.000000000000000000, 0.9659258262890683122, 1.000000000000000000, 0.9659258262890683122, 1.000000000000000000, 0.9659258262890683122, 1.000000000000000000, 0.9659258262890683122, 1.000000000000000000, 0.9659258262890683122, 1.000000000000000000, 0.9659258262890683122, 1.000000000000000000, 0.9659258262890683122, 1.000000000000000000, 0.9659258262890683122, 1.000000000000000000, 0.9659258262890683122, 1.000000000000000000, 0.9659258262890683122, 1.000000000000000000, 0.9659258262890683122, 1.000000000000000000, 0.9659258262890683122, 1.000000000000000000, 0.9659258262890683122, 1.000000000000000000, 0.9659258262890683122, 1.000000000000000000, 0.9659258262890683122, 1.000000000000000000, 0.9659258262890683122, 1.000000000000000000, 0.9659258262890683122, 1.000000000000000000, 0.9659258262890683122, 1.000000000000000000, 0.9659258262890683122, 1.000000000000000000, 0.9659258262890683122, 1.000000000000000000, 0.9659258262890683122, 1.000000000000000000, 0.9659258262890683122, 1.000000000000000000, 0.9659258262890683122, 1.000000000000000000, 0.9659258262890683122, 1.000000000000000000, 0.9659258262890683122, 1.000000000000000000, 0.9659258262890683122, 1.000000000000000000, 0.9659258262890683122, 1.000000000000000000, 0.9659258262890683122, 1.000000000000000000, 0.9659258262890683122, 1.000000000000000000, 0.9659258262890683122, 1.000000000000000000, 0.9659258262890683122, 1.000000000000000000, 0.9659258262890683122, 1.000000000000000000, 0.9659258262890683122, 1.000000000000000000, 0.9659258262890683122, 1.000000000000000000, 0.9659258262890683122, 1.000000000000000000, 0.9659258262890683122, 1.000000000000000000, 0.9659258262890683122, 1.000000000000000000, 0.9659258262890683122, 1.000000000000000000, 0.9659258262890683122, 1.000000000000000000, 0.9659258262890683122, 1.000000000000000000, 0.9659258262890683122, 1.000000000000000000, 0.9659258262890683122, 1.000000000000000000, 0.9659258262890683122, 1.000000000000000000, 0.9659258262890683122, 1.000000000000000000, 0.9659258262890683122, 1.000000000000000000, 0.9659258262890683122, 1.000000000000000000, 0.9659258262890683122, 1.000000000000000000, 0.9659258262890683122, 1.000000000000000000, 0.9659258262890683122, 1.000000000000000000, 0.9659258262890683122, 1.000000000000000000, 0.9659258262890683122, 1.000000000000000000, 0.9659258262890683122, 1.000000000000000000, 0.9659258262890683122, 1.000000000000000000, 0.9659258262890683122, 1.000000000000000000, 0.9659258262890683122, 1.000000000000000000, 0.9659258262890683122, 1.000000000000000000, 0.9659258262890683122, 1.000000000000000000, 0.9659258262890683122, 1.000000000000000000) ) ) 
 REPRESENTATION_ITEM ( '' )  SURFACE ( )  );
#69769=CARTESIAN_POINT ( 'NONE',  ( -5.823673210054431948, 21.52544592524334988, 72.70942372801901854 ) ) ;
#69770=CARTESIAN_POINT ( 'NONE',  ( 16.53943276465976808, 0.05219959533934440121, 46.25109039468567573 ) ) ;
#69771=CARTESIAN_POINT ( 'NONE',  ( -5.153800228976328057, -19.02544592524343514, 77.29057627198099567 ) ) ;
#69772=CARTESIAN_POINT ( 'NONE',  ( 19.05341960407617918, -5.049401038297876454, 106.0427570613523471 ) ) ;
#69773=CARTESIAN_POINT ( 'NONE',  ( 16.53943276465976808, 0.05219959533934440121, 86.25109039468568994 ) ) ;
#69774=CARTESIAN_POINT ( 'NONE',  ( -9.474510206698720793, -16.51473224551083518, 89.58442372801900433 ) ) ;
#69775=CARTESIAN_POINT ( 'NONE',  ( 19.02544592524343514, -5.153800228976328945, 58.54057627198102409 ) ) ;
#69776=CARTESIAN_POINT ( 'NONE',  ( 5.719274019375991003, -21.55341960407610458, 92.70724293864770971 ) ) ;
#69777=CARTESIAN_POINT ( 'NONE',  ( -12.06949235617756955, 12.14591786802309770, 95.62390960531436690 ) ) ;
#69778=CARTESIAN_POINT ( 'NONE',  ( 13.89961937509957401, 13.97604488694547697, 91.87609039468567573 ) ) ;
#69779=CARTESIAN_POINT ( 'NONE',  ( -4.483927247898782831, 16.52544592524335698, 62.70942372801902565 ) ) ;
#69780=CARTESIAN_POINT ( 'NONE',  ( 17.48847506799971185, -5.747544572773693794, 63.32697437843280852 ) ) ;
#69781=CARTESIAN_POINT ( 'NONE',  ( -13.97604488694547697, 13.89961937509957934, 68.12609039468563310 ) ) ;
#69782=CARTESIAN_POINT ( 'NONE',  ( -16.52544592524342804, 4.483927247898546575, 26.04057627198103475 ) ) ;
#69783=CARTESIAN_POINT ( 'NONE',  ( 14.29746914071049879, -8.314922557960816363, 83.33224293864769550 ) ) ;
#69784=CARTESIAN_POINT ( 'NONE',  ( 13.97604488694548053, -13.89961937509957401, 25.62609039468566507 ) ) ;
#69785=CARTESIAN_POINT ( 'NONE',  ( -17.26058549869106429, 6.457015423128171783, 38.62254162523935008 ) ) ;
#69786=CARTESIAN_POINT ( 'NONE',  ( 10.81492255796106328, -18.62759615963255655, 20.41775706135234714 ) ) ;
#69787=CARTESIAN_POINT ( 'NONE',  ( -19.02544592524342804, 5.153800228976336051, 116.0405762719810383 ) ) ;
#69788=CARTESIAN_POINT ( 'NONE',  ( 19.03943276465977164, -0.05219959533909143690, 83.74890960531436690 ) ) ;
#69789=CARTESIAN_POINT ( 'NONE',  ( -18.62759615963255300, -10.81492255796106328, 99.16775706135234714 ) ) ;
#69790=CARTESIAN_POINT ( 'NONE',  ( -13.89961937509977652, 13.97604488694528158, 75.62390960531438111 ) ) ;
#69791=CARTESIAN_POINT ( 'NONE',  ( 10.81492255796078972, 18.62759615963270932, 49.58224293864769550 ) ) ;
#69792=CARTESIAN_POINT ( 'NONE',  ( 4.483927247898545687, 16.52544592524342804, 79.79057627198102409 ) ) ;
#69793=CARTESIAN_POINT ( 'NONE',  ( -19.05341960407611168, -5.049401038298163336, 56.45724293864768129 ) ) ;
#69795=CARTESIAN_POINT ( 'NONE',  ( -12.14591786802309592, -12.06949235617757132, 106.8739096053143811 ) ) ;
#69796=CARTESIAN_POINT ( 'NONE',  ( 15.80617190586769283, -15.72974639402175789, 25.62609039468567929 ) ) ;
#69797=CARTESIAN_POINT ( 'NONE',  ( 21.55341960407619695, -5.719274019375665929, 56.04275706135235424 ) ) ;
#69798=CARTESIAN_POINT ( 'NONE',  ( 9.474510206698971260, -16.51473224551069308, 42.91557627198103120 ) ) ;
#69799=CARTESIAN_POINT ( 'NONE',  ( -12.14591786802326823, 12.06949235617739902, 83.12609039468568994 ) ) ;
#69800=CARTESIAN_POINT ( 'NONE',  ( -10.81492255796078084, -18.62759615963271287, 112.0822429386477097 ) ) ;
#69801=CARTESIAN_POINT ( 'NONE',  ( -0.05219959533907301413, -21.53943276465977519, 112.4989096053143669 ) ) ;
#69802=CARTESIAN_POINT ( 'NONE',  ( 19.03943276465977164, 0.05219959533936151252, 46.25109039468566863 ) ) ;
#69803=CARTESIAN_POINT ( 'NONE',  ( -13.89961937509977652, 13.97604488694528158, 60.62390960531436690 ) ) ;
#69804=CARTESIAN_POINT ( 'NONE',  ( -13.97604488694547697, 13.89961937509957934, 38.12609039468566152 ) ) ;
#69805=CARTESIAN_POINT ( 'NONE',  ( 21.53943276465977519, 0.05219959533937863772, 71.25109039468568994 ) ) ;
#69807=CARTESIAN_POINT ( 'NONE',  ( 18.62759615963271287, -10.81492255796078972, 68.33224293864769550 ) ) ;
#69808=CARTESIAN_POINT ( 'NONE',  ( 14.29746914071049879, -8.314922557960816363, 33.33224293864769550 ) ) ;
#69809=CARTESIAN_POINT ( 'NONE',  ( 15.80617190586769283, -15.72974639402175789, 95.62609039468568994 ) ) ;
#69810=CARTESIAN_POINT ( 'NONE',  ( -15.80617190586768217, 15.72974639402176855, 108.1260903946856757 ) ) ;
#69811=CARTESIAN_POINT ( 'NONE',  ( -14.29746914071049879, 8.314922557960819915, 55.83224293864770260 ) ) ;
#69812=CARTESIAN_POINT ( 'NONE',  ( -12.06949235617756955, 12.14591786802309770, 105.6239096053143669 ) ) ;
#69813=CARTESIAN_POINT ( 'NONE',  ( 19.03943276465977164, 0.05219959533936151252, 61.25109039468566863 ) ) ;
#69814=CARTESIAN_POINT ( 'NONE',  ( 4.379528057220339221, -16.55341960407611168, 22.70724293864769194 ) ) ;
#69815=CARTESIAN_POINT ( 'NONE',  ( -15.80617190586768217, 15.72974639402176855, 63.12609039468568994 ) ) ;
#69816=CARTESIAN_POINT ( 'NONE',  ( 16.51473224551069308, 9.474510206698969483, 74.16557627198103830 ) ) ;
#69817=CARTESIAN_POINT ( 'NONE',  ( -0.05219959533936034679, 19.03943276465977164, 42.50109039468566152 ) ) ;
#69818=CARTESIAN_POINT ( 'NONE',  ( 21.55341960407610458, 5.719274019375980345, 48.95724293864770971 ) ) ;
#69819=CARTESIAN_POINT ( 'NONE',  ( 21.55341960407619695, -5.719274019375665929, 41.04275706135236135 ) ) ;
#69820=CARTESIAN_POINT ( 'NONE',  ( 0.05219959533907565091, 21.53943276465977519, 104.9989096053143669 ) ) ;
#69821=CARTESIAN_POINT ( 'NONE',  ( -9.564922557961040184, 16.46253265017147172, 97.91775706135233293 ) ) ;
#69822=CARTESIAN_POINT ( 'NONE',  ( 8.314922557961029526, -14.29746914071037800, 65.41775706135234714 ) ) ;
#69824=CARTESIAN_POINT ( 'NONE',  ( 15.72974639402199770, -15.80617190586745480, 98.12390960531436690 ) ) ;
#69825=CARTESIAN_POINT ( 'NONE',  ( -12.06949235617756955, 12.14591786802309770, 90.62390960531436690 ) ) ;
#69827=CARTESIAN_POINT ( 'NONE',  ( 8.314922557961029526, -14.29746914071037800, 20.41775706135234714 ) ) ;
#69828=CARTESIAN_POINT ( 'NONE',  ( 21.52544592524344225, -5.823673210054117533, 43.54057627198103830 ) ) ;
#69829=CARTESIAN_POINT ( 'NONE',  ( 16.55341960407618274, -4.379528057220086978, 91.04275706135236135 ) ) ;
#69830=CARTESIAN_POINT ( 'NONE',  ( -5.153800228976328057, -19.02544592524343514, 22.29057627198102765 ) ) ;
#69831=CARTESIAN_POINT ( 'NONE',  ( -12.06949235617739369, -12.14591786802326823, 59.37609039468568284 ) ) ;
#69832=CARTESIAN_POINT ( 'NONE',  ( 21.53943276465977519, 0.05219959533937863772, 26.25109039468567573 ) ) ;
#69833=CARTESIAN_POINT ( 'NONE',  ( 5.823673210054125526, 21.52544592524343514, 49.79057627198102409 ) ) ;
#69834=CARTESIAN_POINT ( 'NONE',  ( 14.34966873604972726, -8.224510206698740333, 90.83442372801901854 ) ) ;
#69835=CARTESIAN_POINT ( 'NONE',  ( 9.474510206698971260, -16.51473224551069308, 102.9155762719810241 ) ) ;
#69836=CARTESIAN_POINT ( 'NONE',  ( -18.62759615963255300, -10.81492255796106328, 74.16775706135231871 ) ) ;
#69837=CARTESIAN_POINT ( 'NONE',  ( 0.05219959533907565091, 21.53943276465977519, 44.99890960531435979 ) ) ;
#69838=CARTESIAN_POINT ( 'NONE',  ( 10.81492255796078972, 18.62759615963270932, 34.58224293864770260 ) ) ;
#69839=VERTEX_POINT ( 'NONE', #157397 ) ;
#69840=CARTESIAN_POINT ( 'NONE',  ( -13.89961937509957401, -13.97604488694547875, 49.37609039468567573 ) ) ;
#69841=CARTESIAN_POINT ( 'NONE',  ( 8.314922557961029526, -14.29746914071037800, 65.41775706135234714 ) ) ;
#69842=CARTESIAN_POINT ( 'NONE',  ( 21.53943276465977519, -0.05219959533907433946, 33.74890960531436690 ) ) ;
#69844=CARTESIAN_POINT ( 'NONE',  ( -19.05341960407611168, -5.049401038298163336, 91.45724293864766707 ) ) ;
#69845=CARTESIAN_POINT ( 'NONE',  ( -4.379528057220086978, -16.55341960407618274, 109.7927570613523613 ) ) ;
#69847=CARTESIAN_POINT ( 'NONE',  ( -4.379528057220328563, 16.55341960407611168, 105.2072429386477097 ) ) ;
#69848=CARTESIAN_POINT ( 'NONE',  ( -5.823673210054116645, -21.52544592524344225, 42.29057627198103120 ) ) ;
#69849=CARTESIAN_POINT ( 'NONE',  ( 9.564922557960805705, 16.46253265017160317, 44.58224293864769550 ) ) ;
#69850=CARTESIAN_POINT ( 'NONE',  ( 14.29746914071037800, 8.314922557961029526, 81.66775706135236135 ) ) ;
#69851=CARTESIAN_POINT ( 'NONE',  ( 15.72974639402176855, 15.80617190586768217, 31.87609039468567929 ) ) ;
#69852=CARTESIAN_POINT ( 'NONE',  ( -13.97604488694547697, 13.89961937509957934, 88.12609039468563310 ) ) ;
#69853=CARTESIAN_POINT ( 'NONE',  ( -8.224510206698948167, 14.34966873604960824, 85.41557627198102409 ) ) ;
#69854=CARTESIAN_POINT ( 'NONE',  ( 5.153800228976335163, 19.02544592524342804, 59.79057627198100988 ) ) ;
#69855=CIRCLE ( 'NONE', #102193, 2.000000000000001776 ) ;
#69856=CARTESIAN_POINT ( 'NONE',  ( -5.049401038298153566, 19.05341960407611168, 25.20724293864768484 ) ) ;
#69857=CARTESIAN_POINT ( 'NONE',  ( -5.719274019375665041, -21.55341960407619695, 104.7927570613523898 ) ) ;
#69858=CARTESIAN_POINT ( 'NONE',  ( 0.05219959533909260263, 19.03943276465977164, 79.99890960531436690 ) ) ;
#69859=CARTESIAN_POINT ( 'NONE',  ( -8.224510206698735004, -14.34966873604973081, 59.58442372801901854 ) ) ;
#69860=CARTESIAN_POINT ( 'NONE',  ( -15.80617190586768217, 15.72974639402176855, 98.12609039468570415 ) ) ;
#69861=CARTESIAN_POINT ( 'NONE',  ( -0.05219959533907301413, -21.53943276465977519, 47.49890960531435979 ) ) ;
#69862=CARTESIAN_POINT ( 'NONE',  ( -12.14591786802326823, 12.06949235617739902, 78.12609039468570415 ) ) ;
#69863=CARTESIAN_POINT ( 'NONE',  ( 16.51473224551083163, -9.474510206698727899, 45.83442372801900433 ) ) ;
#69864=CARTESIAN_POINT ( 'NONE',  ( -19.02544592524334988, -5.153800228976617603, 63.95942372801899012 ) ) ;
#69866=CARTESIAN_POINT ( 'NONE',  ( -18.67979575497193778, 10.72451020669871902, 68.33442372801900433 ) ) ;
#69867=CARTESIAN_POINT ( 'NONE',  ( -16.51473224551069308, -9.474510206698971260, 66.66557627198102409 ) ) ;
#69868=CARTESIAN_POINT ( 'NONE',  ( 13.89961937509978007, -13.97604488694527269, 58.12390960531435979 ) ) ;
#69869=CARTESIAN_POINT ( 'NONE',  ( -16.51473224551082808, 9.474510206698731452, 58.33442372801900433 ) ) ;
#69871=CARTESIAN_POINT ( 'NONE',  ( -13.97604488694527625, -13.89961937509977652, 91.87390960531432427 ) ) ;
#69872=CARTESIAN_POINT ( 'NONE',  ( -8.224510206698948167, 14.34966873604960824, 50.41557627198103120 ) ) ;
#69873=CARTESIAN_POINT ( 'NONE',  ( 21.53943276465977519, -0.05219959533907433946, 48.74890960531435979 ) ) ;
#69874=DIRECTION ( 'NONE',  ( -0.000000000000000000, 1.000000000000000000, 0.000000000000000000 ) ) ;
#69875=CARTESIAN_POINT ( 'NONE',  ( 19.05341960407617918, -5.049401038297876454, 21.04275706135232582 ) ) ;
#69877=CARTESIAN_POINT ( 'NONE',  ( 0.05219959533909260263, 19.03943276465977164, 44.99890960531435979 ) ) ;
#69878=CARTESIAN_POINT ( 'NONE',  ( 18.22780087662121673, 5.500000000000056843, 83.98459894673892734 ) ) ;
#69881=CARTESIAN_POINT ( 'NONE',  ( 14.34966873604972726, -8.224510206698740333, 60.83442372801901854 ) ) ;
#69882=CARTESIAN_POINT ( 'NONE',  ( -21.55341960407610458, -5.719274019375992779, 86.45724293864770971 ) ) ;
#69883=CARTESIAN_POINT ( 'NONE',  ( 8.314922557960818139, 14.29746914071049879, 59.58224293864770260 ) ) ;
#69884=CARTESIAN_POINT ( 'NONE',  ( -13.97604488694527625, -13.89961937509977652, 46.87390960531435979 ) ) ;
#69886=CARTESIAN_POINT ( 'NONE',  ( 15.72974639402176855, 15.80617190586768217, 36.87609039468568994 ) ) ;
#69887=CARTESIAN_POINT ( 'NONE',  ( -5.153800228976607833, 19.02544592524334988, 47.70942372801900433 ) ) ;
#69888=CARTESIAN_POINT ( 'NONE',  ( 19.05341960407611168, 5.049401038298154454, 38.95724293864767418 ) ) ;
#69889=CARTESIAN_POINT ( 'NONE',  ( -10.72451020669870658, -18.67979575497194134, 89.58442372801901854 ) ) ;
#69891=CARTESIAN_POINT ( 'NONE',  ( -17.72696623605160582, 5.499999999999857003, 48.59811031808417425 ) ) ;
#69892=ORIENTED_EDGE ( 'NONE', *, *, #138165, .F. ) ;
#69893=CARTESIAN_POINT ( 'NONE',  ( -16.53943276465976808, 0.05219959533911058130, 36.24890960531435979 ) ) ;
#69895=CARTESIAN_POINT ( 'NONE',  ( 10.81492255796078972, 18.62759615963270932, 34.58224293864770260 ) ) ;
#69898=CARTESIAN_POINT ( 'NONE',  ( -19.03943276465977164, 0.05219959533909376836, 91.24890960531436690 ) ) ;
#69899=CARTESIAN_POINT ( 'NONE',  ( 8.224510206698953496, -14.34966873604960469, 82.91557627198103830 ) ) ;
#69900=CARTESIAN_POINT ( 'NONE',  ( 8.314922557961029526, -14.29746914071037800, 30.41775706135234358 ) ) ;
#69901=CARTESIAN_POINT ( 'NONE',  ( -4.483927247898782831, 16.52544592524335698, 112.7094237280190328 ) ) ;
#69904=CARTESIAN_POINT ( 'NONE',  ( -5.153800228976328057, -19.02544592524343514, 52.29057627198100988 ) ) ;
#69905=CARTESIAN_POINT ( 'NONE',  ( -9.474510206698964154, 16.51473224551069663, 80.41557627198103830 ) ) ;
#69906=CARTESIAN_POINT ( 'NONE',  ( 21.55341960407610458, 5.719274019375980345, 93.95724293864770971 ) ) ;
#69907=CARTESIAN_POINT ( 'NONE',  ( 14.29746914071049879, -8.314922557960816363, 23.33224293864769194 ) ) ;
#69908=CARTESIAN_POINT ( 'NONE',  ( -5.153800228976328057, -19.02544592524343514, 107.2905762719810383 ) ) ;
#69909=CARTESIAN_POINT ( 'NONE',  ( 19.03943276465977164, 0.05219959533936151252, 76.25109039468566152 ) ) ;
#69910=CARTESIAN_POINT ( 'NONE',  ( -21.52544592524334988, -5.823673210054445271, 103.9594237280190185 ) ) ;
#69911=CARTESIAN_POINT ( 'NONE',  ( 21.52544592524344225, -5.823673210054117533, 93.54057627198103830 ) ) ;
#69912=CARTESIAN_POINT ( 'NONE',  ( 15.80617190586746368, 15.72974639402197994, 34.37390960531435979 ) ) ;
#69913=CARTESIAN_POINT ( 'NONE',  ( 9.474510206698971260, -16.51473224551069308, 67.91557627198102409 ) ) ;
#69914=CARTESIAN_POINT ( 'NONE',  ( 0.05219959533934541429, -16.53943276465976808, 110.0010903946856757 ) ) ;
#69915=CARTESIAN_POINT ( 'NONE',  ( -5.153800228976328057, -19.02544592524343514, 72.29057627198102409 ) ) ;
#69916=VERTEX_POINT ( 'NONE', #111878 ) ;
#69918=CARTESIAN_POINT ( 'NONE',  ( 5.153800228976615827, -19.02544592524334988, 30.20942372801900433 ) ) ;
#69919=CARTESIAN_POINT ( 'NONE',  ( -14.34966873604960291, -8.224510206698953496, 91.66557627198103830 ) ) ;
#69920=CARTESIAN_POINT ( 'NONE',  ( -18.67979575497193778, 10.72451020669871902, 28.33442372801902209 ) ) ;
#69922=CARTESIAN_POINT ( 'NONE',  ( 10.81492255796078972, 18.62759615963270932, 69.58224293864769550 ) ) ;
#69923=CARTESIAN_POINT ( 'NONE',  ( 4.483927247898790824, -16.52544592524335698, 95.20942372801903275 ) ) ;
#69924=CARTESIAN_POINT ( 'NONE',  ( -16.51473224551069308, -9.474510206698971260, 26.66557627198103120 ) ) ;
#69925=CARTESIAN_POINT ( 'NONE',  ( 19.03943276465977164, -0.05219959533909143690, 78.74890960531436690 ) ) ;
#69928=CARTESIAN_POINT ( 'NONE',  ( -14.34966873604960291, -8.224510206698953496, 36.66557627198103120 ) ) ;
#69930=CARTESIAN_POINT ( 'NONE',  ( -5.719274019375665041, -21.55341960407619695, 64.79275706135234714 ) ) ;
#69931=CARTESIAN_POINT ( 'NONE',  ( -0.05219959533909027116, -19.03943276465977164, 107.4989096053143527 ) ) ;
#69932=CARTESIAN_POINT ( 'NONE',  ( 21.55341960407619695, -5.719274019375665929, 91.04275706135236135 ) ) ;
#69933=CARTESIAN_POINT ( 'NONE',  ( -5.049401038298153566, 19.05341960407611168, 45.20724293864769550 ) ) ;
#69934=CARTESIAN_POINT ( 'NONE',  ( -5.153800228976328057, -19.02544592524343514, 57.29057627198103120 ) ) ;
#69936=CARTESIAN_POINT ( 'NONE',  ( -5.823673210054431948, 21.52544592524334988, 97.70942372801904696 ) ) ;
#69937=CARTESIAN_POINT ( 'NONE',  ( -0.05219959533934338120, 16.53943276465976808, 67.50109039468568994 ) ) ;
#69938=CARTESIAN_POINT ( 'NONE',  ( -21.55341960407619339, 5.719274019375674811, 88.54275706135236135 ) ) ;
#69939=CARTESIAN_POINT ( 'NONE',  ( 18.67979575497178502, 10.72451020669898547, 24.16557627198103120 ) ) ;
#69940=CARTESIAN_POINT ( 'NONE',  ( -19.03943276465977164, -0.05219959533935918106, 93.75109039468566152 ) ) ;
#69941=CARTESIAN_POINT ( 'NONE',  ( 10.81492255796106328, -18.62759615963255655, 60.41775706135235424 ) ) ;
#69942=CARTESIAN_POINT ( 'NONE',  ( -8.224510206698735004, -14.34966873604973081, 34.58442372801900433 ) ) ;
#69943=CARTESIAN_POINT ( 'NONE',  ( 5.719274019375991003, -21.55341960407610458, 87.70724293864769550 ) ) ;
#69944=CARTESIAN_POINT ( 'NONE',  ( -19.05341960407617563, 5.049401038297882671, 83.54275706135233293 ) ) ;
#69945=CARTESIAN_POINT ( 'NONE',  ( -5.049401038298153566, 19.05341960407611168, 65.20724293864765286 ) ) ;
#69946=CARTESIAN_POINT ( 'NONE',  ( 13.89961937509957401, 13.97604488694547697, 96.87609039468566152 ) ) ;
#69947=CARTESIAN_POINT ( 'NONE',  ( -5.049401038297874678, -19.05341960407617918, 104.7927570613523471 ) ) ;
#69948=CARTESIAN_POINT ( 'NONE',  ( 16.55341960407611168, 4.379528057220329451, 48.95724293864770971 ) ) ;
#69949=CARTESIAN_POINT ( 'NONE',  ( -19.05341960407617563, 5.049401038297882671, 83.54275706135233293 ) ) ;
#69950=CARTESIAN_POINT ( 'NONE',  ( -16.53943276465976808, -0.05219959533934237506, 58.75109039468568994 ) ) ;
#69951=CARTESIAN_POINT ( 'NONE',  ( -5.153800228976607833, 19.02544592524334988, 42.70942372801901143 ) ) ;
#69952=CARTESIAN_POINT ( 'NONE',  ( 19.05341960407611168, 5.049401038298154454, 38.95724293864767418 ) ) ;
#69953=CARTESIAN_POINT ( 'NONE',  ( 5.049401038298161559, -19.05341960407611168, 52.70724293864767418 ) ) ;
#69954=CARTESIAN_POINT ( 'NONE',  ( -16.52544592524335698, -4.483927247898792601, 53.95942372801900433 ) ) ;
#69957=CARTESIAN_POINT ( 'NONE',  ( 5.153800228976335163, 19.02544592524342804, 109.7905762719810099 ) ) ;
#69958=CARTESIAN_POINT ( 'NONE',  ( -19.02544592524342804, 5.153800228976336051, 26.04057627198103120 ) ) ;
#69960=CARTESIAN_POINT ( 'NONE',  ( -19.03943276465977164, -0.05219959533935918106, 98.75109039468567573 ) ) ;
#69961=CARTESIAN_POINT ( 'NONE',  ( -15.72974639402197994, 15.80617190586746368, 40.62390960531435269 ) ) ;
#69962=CARTESIAN_POINT ( 'NONE',  ( -19.05341960407617563, 5.049401038297882671, 33.54275706135231871 ) ) ;
#69963=CARTESIAN_POINT ( 'NONE',  ( -16.51473224551082808, 9.474510206698731452, 113.3344237280190043 ) ) ;
#69964=CARTESIAN_POINT ( 'NONE',  ( -13.89961937509977652, 13.97604488694528158, 35.62390960531435269 ) ) ;
#69965=CARTESIAN_POINT ( 'NONE',  ( 0.05219959533909260263, 19.03943276465977164, 44.99890960531435979 ) ) ;
#69966=CARTESIAN_POINT ( 'NONE',  ( -0.05219959533907301413, -21.53943276465977519, 67.49890960531436690 ) ) ;
#69967=CARTESIAN_POINT ( 'NONE',  ( 9.474510206698971260, -16.51473224551069308, 102.9155762719810241 ) ) ;
#69968=CARTESIAN_POINT ( 'NONE',  ( 19.03943276465977164, -0.05219959533909143690, 38.74890960531436690 ) ) ;
#69970=CARTESIAN_POINT ( 'NONE',  ( -16.46253265017146816, -9.564922557961047289, 89.16775706135234714 ) ) ;
#69971=CARTESIAN_POINT ( 'NONE',  ( -16.53943276465976808, 0.05219959533911058130, 51.24890960531436690 ) ) ;
#69972=CARTESIAN_POINT ( 'NONE',  ( 10.72451020669898902, -18.67979575497178502, 47.91557627198102409 ) ) ;
#69973=CARTESIAN_POINT ( 'NONE',  ( -21.52544592524334988, -5.823673210054445271, 108.9594237280190185 ) ) ;
#69974=CARTESIAN_POINT ( 'NONE',  ( -18.67979575497178146, -10.72451020669898902, 96.66557627198102409 ) ) ;
#69975=CARTESIAN_POINT ( 'NONE',  ( 21.52544592524334988, 5.823673210054432836, 66.45942372801903275 ) ) ;
#69976=CARTESIAN_POINT ( 'NONE',  ( -15.72974639402176322, -15.80617190586768395, 79.37609039468567573 ) ) ;
#69977=CARTESIAN_POINT ( 'NONE',  ( -16.46253265017160317, 9.564922557960807481, 110.8322429386476955 ) ) ;
#69978=CARTESIAN_POINT ( 'NONE',  ( -4.483927247898782831, 16.52544592524335698, 102.7094237280190185 ) ) ;
#69979=CARTESIAN_POINT ( 'NONE',  ( -5.719274019375665041, -21.55341960407619695, 59.79275706135234714 ) ) ;
#69980=CARTESIAN_POINT ( 'NONE',  ( -13.89961937509977652, 13.97604488694528158, 70.62390960531432427 ) ) ;
#69981=CARTESIAN_POINT ( 'NONE',  ( 9.474510206698729675, 16.51473224551082808, 32.08442372801900433 ) ) ;
#69982=CARTESIAN_POINT ( 'NONE',  ( -15.72974639402176322, -15.80617190586768395, 34.37609039468568284 ) ) ;
#69983=CARTESIAN_POINT ( 'NONE',  ( 16.46253265017160672, -9.564922557960803928, 73.33224293864769550 ) ) ;
#69984=CARTESIAN_POINT ( 'NONE',  ( 14.34966873604960469, 8.224510206698951720, 79.16557627198103830 ) ) ;
#69985=CARTESIAN_POINT ( 'NONE',  ( 16.55341960407611168, 4.379528057220329451, 43.95724293864769550 ) ) ;
#69986=CARTESIAN_POINT ( 'NONE',  ( -10.81492255796078084, -18.62759615963271287, 52.08224293864768839 ) ) ;
#69987=CARTESIAN_POINT ( 'NONE',  ( 9.474510206698971260, -16.51473224551069308, 67.91557627198102409 ) ) ;
#69988=CARTESIAN_POINT ( 'NONE',  ( 18.62759615963271287, -10.81492255796078972, 68.33224293864769550 ) ) ;
#69989=CARTESIAN_POINT ( 'NONE',  ( 9.564922557961047289, -16.46253265017146816, 60.41775706135233293 ) ) ;
#69990=CARTESIAN_POINT ( 'NONE',  ( 5.153800228976617603, -19.02544592524335343, 20.20942372801899722 ) ) ;
#69991=CARTESIAN_POINT ( 'NONE',  ( 4.379528057220339221, -16.55341960407611168, 57.70724293864770260 ) ) ;
#69992=CARTESIAN_POINT ( 'NONE',  ( 0.05219959533907565091, 21.53943276465977519, 39.99890960531436690 ) ) ;
#69995=CARTESIAN_POINT ( 'NONE',  ( -16.52544592524335698, -4.483927247898792601, 83.95942372801900433 ) ) ;
#69997=CARTESIAN_POINT ( 'NONE',  ( 5.049401038297881783, 19.05341960407617563, 82.29275706135229029 ) ) ;
#69998=CARTESIAN_POINT ( 'NONE',  ( 12.14591786802309770, 12.06949235617756955, 54.37390960531435979 ) ) ;
#69999=CARTESIAN_POINT ( 'NONE',  ( -9.564922557960796823, -16.46253265017161027, 47.08224293864769550 ) ) ;
#70000=CARTESIAN_POINT ( 'NONE',  ( -12.06949235617756955, 12.14591786802309770, 45.62390960531436690 ) ) ;
#70001=CARTESIAN_POINT ( 'NONE',  ( 16.51473224551069308, 9.474510206698969483, 89.16557627198103830 ) ) ;
#70002=CARTESIAN_POINT ( 'NONE',  ( -9.564922557960796823, -16.46253265017161027, 47.08224293864769550 ) ) ;
#70003=CARTESIAN_POINT ( 'NONE',  ( 21.52544592524334988, 5.823673210054432836, 61.45942372801901854 ) ) ;
#70004=CARTESIAN_POINT ( 'NONE',  ( 16.46253265017160672, -9.564922557960803928, 68.33224293864770971 ) ) ;
#70005=CARTESIAN_POINT ( 'NONE',  ( 19.02544592524343514, -5.153800228976328945, 23.54057627198102054 ) ) ;
#70006=CARTESIAN_POINT ( 'NONE',  ( 5.049401038298161559, -19.05341960407611168, 77.70724293864765286 ) ) ;
#70008=CARTESIAN_POINT ( 'NONE',  ( -21.52544592524343514, 5.823673210054127303, 46.04057627198103830 ) ) ;
#70009=CARTESIAN_POINT ( 'NONE',  ( -9.474510206698964154, 16.51473224551069663, 55.41557627198103120 ) ) ;
#70010=CARTESIAN_POINT ( 'NONE',  ( -18.62759615963270932, 10.81492255796079327, 50.83224293864770971 ) ) ;
#70011=CARTESIAN_POINT ( 'NONE',  ( -5.049401038297874678, -19.05341960407617918, 79.79275706135233293 ) ) ;
#70012=CARTESIAN_POINT ( 'NONE',  ( 0.05219959533934541429, -16.53943276465976808, 100.0010903946857042 ) ) ;
#70013=CARTESIAN_POINT ( 'NONE',  ( -13.97604488694547697, 13.89961937509957934, 38.12609039468566152 ) ) ;
#70014=CARTESIAN_POINT ( 'NONE',  ( 16.53943276465976808, 0.05219959533934440121, 66.25109039468567573 ) ) ;
#70015=CARTESIAN_POINT ( 'NONE',  ( 8.224510206698742110, 14.34966873604972548, 82.08442372801901854 ) ) ;
#70016=FACE_OUTER_BOUND ( 'NONE', #16194, .T. ) ;
#70017=CARTESIAN_POINT ( 'NONE',  ( 4.483927247898790824, -16.52544592524335698, 65.20942372801901854 ) ) ;
#70018=CARTESIAN_POINT ( 'NONE',  ( 0.05219959533909260263, 19.03943276465977164, 114.9989096053143669 ) ) ;
#70019=CARTESIAN_POINT ( 'NONE',  ( 19.02544592524343514, -5.153800228976328945, 28.54057627198102409 ) ) ;
#70020=CARTESIAN_POINT ( 'NONE',  ( -8.224510206698735004, -14.34966873604973081, 44.58442372801901854 ) ) ;
#70021=CARTESIAN_POINT ( 'NONE',  ( 19.03943276465977164, -0.05219959533909143690, 43.74890960531435979 ) ) ;
#70022=CARTESIAN_POINT ( 'NONE',  ( -15.80617190586768217, 15.72974639402176855, 43.12609039468568284 ) ) ;
#70023=CARTESIAN_POINT ( 'NONE',  ( 4.483927247898790824, -16.52544592524335698, 40.20942372801901854 ) ) ;
#70024=CARTESIAN_POINT ( 'NONE',  ( -0.05219959533934338120, 16.53943276465976808, 102.5010903946856899 ) ) ;
#70026=CARTESIAN_POINT ( 'NONE',  ( 15.80617190586769283, -15.72974639402175789, 110.6260903946857042 ) ) ;
#70027=CARTESIAN_POINT ( 'NONE',  ( 0.05219959533936267826, -19.03943276465977164, 105.0010903946856615 ) ) ;
#70028=CARTESIAN_POINT ( 'NONE',  ( -5.049401038297874678, -19.05341960407617918, 64.79275706135233293 ) ) ;
#70029=CARTESIAN_POINT ( 'NONE',  ( 4.379528057220339221, -16.55341960407611168, 67.70724293864769550 ) ) ;
#70030=CARTESIAN_POINT ( 'NONE',  ( 16.51473224551069308, 9.474510206698969483, 44.16557627198103120 ) ) ;
#70031=CARTESIAN_POINT ( 'NONE',  ( -9.564922557961040184, 16.46253265017147172, 62.91775706135233293 ) ) ;
#70032=CARTESIAN_POINT ( 'NONE',  ( 17.31728774477212696, -6.344390552233678982, 58.31906651689306642 ) ) ;
#70033=CARTESIAN_POINT ( 'NONE',  ( 18.62759615963255655, 10.81492255796105972, 66.66775706135234714 ) ) ;
#70034=CARTESIAN_POINT ( 'NONE',  ( 14.34966873604972726, -8.224510206698740333, 40.83442372801901854 ) ) ;
#70035=CARTESIAN_POINT ( 'NONE',  ( 17.49999999999999289, 5.622605283950886879, 38.81207310596112592 ) ) ;
#70036=CARTESIAN_POINT ( 'NONE',  ( -15.80617190586745835, -15.72974639402198527, 21.87390960531436690 ) ) ;
#70037=CARTESIAN_POINT ( 'NONE',  ( -13.97604488694547697, 13.89961937509957934, 103.1260903946856473 ) ) ;
#70038=CARTESIAN_POINT ( 'NONE',  ( -13.97604488694527625, -13.89961937509977652, 111.8739096053143243 ) ) ;
#70039=FACE_OUTER_BOUND ( 'NONE', #140806, .T. ) ;
#70040=CARTESIAN_POINT ( 'NONE',  ( -0.05219959533909027116, -19.03943276465977164, 27.49890960531435624 ) ) ;
#70041=CARTESIAN_POINT ( 'NONE',  ( 21.55341960407619695, -5.719274019375665929, 111.0427570613523613 ) ) ;
#70042=CARTESIAN_POINT ( 'NONE',  ( 9.474510206698971260, -16.51473224551069308, 52.91557627198102409 ) ) ;
#70044=CARTESIAN_POINT ( 'NONE',  ( -10.72451020669870658, -18.67979575497194134, 59.58442372801901854 ) ) ;
#70045=CARTESIAN_POINT ( 'NONE',  ( 21.52544592524334988, 5.823673210054432836, 96.45942372801901854 ) ) ;
#70046=CARTESIAN_POINT ( 'NONE',  ( 16.52544592524342804, -4.483927247898539470, 23.54057627198102765 ) ) ;
#70047=CARTESIAN_POINT ( 'NONE',  ( -16.51473224551069308, -9.474510206698971260, 31.66557627198102054 ) ) ;
#70048=CARTESIAN_POINT ( 'NONE',  ( -5.049401038298153566, 19.05341960407611168, 75.20724293864769550 ) ) ;
#70049=CARTESIAN_POINT ( 'NONE',  ( 10.72451020669871369, 18.67979575497193778, 57.08442372801901854 ) ) ;
#70050=CARTESIAN_POINT ( 'NONE',  ( -5.049401038298153566, 19.05341960407611168, 40.20724293864768839 ) ) ;
#70051=CARTESIAN_POINT ( 'NONE',  ( -5.823673210054431948, 21.52544592524334988, 52.70942372801902565 ) ) ;
#70052=CARTESIAN_POINT ( 'NONE',  ( 9.564922557961047289, -16.46253265017146816, 80.41775706135234714 ) ) ;
#70053=CARTESIAN_POINT ( 'NONE',  ( 16.51473224551069308, 9.474510206698969483, 99.16557627198102409 ) ) ;
#70054=CARTESIAN_POINT ( 'NONE',  ( -16.55341960407611168, -4.379528057220339221, 111.4572429386476813 ) ) ;
#70055=CARTESIAN_POINT ( 'NONE',  ( -21.52544592524343514, 5.823673210054127303, 106.0405762719810525 ) ) ;
#70056=CARTESIAN_POINT ( 'NONE',  ( 19.02544592524334988, 5.153800228976608722, 31.45942372801900433 ) ) ;
#70057=CARTESIAN_POINT ( 'NONE',  ( 4.379528057220339221, -16.55341960407611168, 92.70724293864770971 ) ) ;
#70058=CARTESIAN_POINT ( 'NONE',  ( 19.02544592524343514, -5.153800228976328945, 48.54057627198103120 ) ) ;
#70059=CARTESIAN_POINT ( 'NONE',  ( -5.049401038297874678, -19.05341960407617918, 94.79275706135230450 ) ) ;
#70060=CARTESIAN_POINT ( 'NONE',  ( 16.55341960407611168, 4.379528057220329451, 58.95724293864770971 ) ) ;
#70061=CARTESIAN_POINT ( 'NONE',  ( 5.719274019375673035, 21.55341960407619339, 107.2927570613523471 ) ) ;
#70062=CARTESIAN_POINT ( 'NONE',  ( -13.89961937509977652, 13.97604488694528158, 100.6239096053143669 ) ) ;
#70063=CARTESIAN_POINT ( 'NONE',  ( -19.03943276465977164, -0.05219959533935918106, 93.75109039468566152 ) ) ;
#70064=CARTESIAN_POINT ( 'NONE',  ( 18.67979575497178502, 10.72451020669898547, 94.16557627198103830 ) ) ;
#70065=CARTESIAN_POINT ( 'NONE',  ( 15.80617190586769283, -15.72974639402175789, 50.62609039468568994 ) ) ;
#70066=CARTESIAN_POINT ( 'NONE',  ( 12.14591786802327356, -12.06949235617739191, 45.62609039468567573 ) ) ;
#70067=CARTESIAN_POINT ( 'NONE',  ( -8.224510206698735004, -14.34966873604973081, 109.5844237280190328 ) ) ;
#70068=CARTESIAN_POINT ( 'NONE',  ( 12.14591786802327356, -12.06949235617739191, 45.62609039468567573 ) ) ;
#70069=CARTESIAN_POINT ( 'NONE',  ( -5.719274019375665041, -21.55341960407619695, 49.79275706135234714 ) ) ;
#70070=CARTESIAN_POINT ( 'NONE',  ( 21.55341960407610458, 5.719274019375980345, 38.95724293864768839 ) ) ;
#70071=CARTESIAN_POINT ( 'NONE',  ( 19.03943276465977164, -0.05219959533909143690, 33.74890960531435979 ) ) ;
#70073=CARTESIAN_POINT ( 'NONE',  ( 14.29746914071037800, 8.314922557961029526, 66.66775706135234714 ) ) ;
#70074=CARTESIAN_POINT ( 'NONE',  ( 15.72974639402199770, -15.80617190586745480, 83.12390960531436690 ) ) ;
#70075=CARTESIAN_POINT ( 'NONE',  ( 14.34966873604960469, 8.224510206698951720, 34.16557627198102409 ) ) ;
#70076=CARTESIAN_POINT ( 'NONE',  ( -12.14591786802326823, 12.06949235617739902, 63.12609039468568994 ) ) ;
#70077=CARTESIAN_POINT ( 'NONE',  ( 13.89961937509977652, -13.97604488694527269, 63.12390960531435979 ) ) ;
#70078=CARTESIAN_POINT ( 'NONE',  ( 13.97604488694548053, -13.89961937509957401, 95.62609039468563310 ) ) ;
#70079=CARTESIAN_POINT ( 'NONE',  ( 5.823673210054125526, 21.52544592524343514, 79.79057627198102409 ) ) ;
#70080=CARTESIAN_POINT ( 'NONE',  ( -16.55341960407611168, -4.379528057220339221, 31.45724293864769550 ) ) ;
#70081=VERTEX_POINT ( 'NONE', #95709 ) ;
#70083=CARTESIAN_POINT ( 'NONE',  ( -15.72974639402197994, 15.80617190586746368, 70.62390960531436690 ) ) ;
#70084=CARTESIAN_POINT ( 'NONE',  ( -16.52544592524335698, -4.483927247898792601, 108.9594237280190185 ) ) ;
#70085=ORIENTED_EDGE ( 'NONE', *, *, #122826, .F. ) ;
#70086=CARTESIAN_POINT ( 'NONE',  ( 17.49999999999999645, -5.099703775203614065, 103.2332118591204448 ) ) ;
#70087=CARTESIAN_POINT ( 'NONE',  ( -0.05219959533907301413, -21.53943276465977519, 92.49890960531436690 ) ) ;
#70088=CARTESIAN_POINT ( 'NONE',  ( 18.62759615963271287, -10.81492255796078972, 108.3322429386477097 ) ) ;
#70089=CARTESIAN_POINT ( 'NONE',  ( -16.52544592524342804, 4.483927247898546575, 31.04057627198102409 ) ) ;
#70090=CARTESIAN_POINT ( 'NONE',  ( -16.55341960407617563, 4.379528057220093196, 28.54275706135234358 ) ) ;
#70091=CARTESIAN_POINT ( 'NONE',  ( 16.51473224551069308, 9.474510206698969483, 39.16557627198103120 ) ) ;
#70092=CARTESIAN_POINT ( 'NONE',  ( -9.474510206698964154, 16.51473224551069663, 65.41557627198102409 ) ) ;
#70094=CARTESIAN_POINT ( 'NONE',  ( -5.823673210054116645, -21.52544592524344225, 27.29057627198103120 ) ) ;
#70096=CARTESIAN_POINT ( 'NONE',  ( 9.564922557961047289, -16.46253265017146816, 110.4177570613523471 ) ) ;
#70097=CARTESIAN_POINT ( 'NONE',  ( 16.46253265017146816, 9.564922557961045513, 41.66775706135234003 ) ) ;
#70098=CARTESIAN_POINT ( 'NONE',  ( -15.72974639402197994, 15.80617190586746368, 85.62390960531436690 ) ) ;
#70099=CARTESIAN_POINT ( 'NONE',  ( -4.379528057220086978, -16.55341960407618274, 109.7927570613523613 ) ) ;
#70100=CARTESIAN_POINT ( 'NONE',  ( 10.81492255796078972, 18.62759615963270932, 39.58224293864769550 ) ) ;
#70101=CARTESIAN_POINT ( 'NONE',  ( 5.823673210054125526, 21.52544592524343514, 84.79057627198102409 ) ) ;
#70102=CARTESIAN_POINT ( 'NONE',  ( 16.46253265017146816, 9.564922557961045513, 101.6677570613523329 ) ) ;
#70103=CARTESIAN_POINT ( 'NONE',  ( 13.89961937509977652, -13.97604488694527269, 103.1239096053143527 ) ) ;
#70104=CARTESIAN_POINT ( 'NONE',  ( -21.53943276465977519, -0.05219959533937600094, 78.75109039468568994 ) ) ;
#70105=CARTESIAN_POINT ( 'NONE',  ( 9.474510206698971260, -16.51473224551069308, 77.91557627198103830 ) ) ;
#70106=CARTESIAN_POINT ( 'NONE',  ( 16.53943276465976808, -0.05219959533910856209, 98.74890960531438111 ) ) ;
#70108=CARTESIAN_POINT ( 'NONE',  ( 9.564922557960805705, 16.46253265017160317, 69.58224293864770971 ) ) ;
#70109=CARTESIAN_POINT ( 'NONE',  ( 4.483927247898545687, 16.52544592524342804, 84.79057627198102409 ) ) ;
#70111=CARTESIAN_POINT ( 'NONE',  ( 5.049401038297881783, 19.05341960407617563, 107.2927570613523187 ) ) ;
#70113=CARTESIAN_POINT ( 'NONE',  ( 19.03943276465977164, -0.05219959533909143690, 53.74890960531436690 ) ) ;
#70114=CARTESIAN_POINT ( 'NONE',  ( -5.823673210054431948, 21.52544592524334988, 87.70942372801901854 ) ) ;
#70115=CARTESIAN_POINT ( 'NONE',  ( -19.05341960407611168, -5.049401038298163336, 96.45724293864769550 ) ) ;
#70116=CARTESIAN_POINT ( 'NONE',  ( -14.34966873604972548, 8.224510206698743886, 83.33442372801903275 ) ) ;
#70118=CARTESIAN_POINT ( 'NONE',  ( -19.02544592524334988, -5.153800228976617603, 53.95942372801898301 ) ) ;
#70119=CARTESIAN_POINT ( 'NONE',  ( 10.81492255796106328, -18.62759615963255655, 100.4177570613523471 ) ) ;
#70122=CARTESIAN_POINT ( 'NONE',  ( -16.55341960407617563, 4.379528057220093196, 108.5427570613523756 ) ) ;
#70124=CARTESIAN_POINT ( 'NONE',  ( 8.314922557961029526, -14.29746914071037800, 90.41775706135236135 ) ) ;
#70126=CARTESIAN_POINT ( 'NONE',  ( 4.483927247898790824, -16.52544592524335698, 65.20942372801901854 ) ) ;
#70128=CARTESIAN_POINT ( 'NONE',  ( -10.81492255796105439, 18.62759615963255655, 77.91775706135231871 ) ) ;
#70129=CARTESIAN_POINT ( 'NONE',  ( -9.474510206698720793, -16.51473224551083518, 89.58442372801900433 ) ) ;
#70130=CARTESIAN_POINT ( 'NONE',  ( -13.89961937509957401, -13.97604488694547875, 44.37609039468566863 ) ) ;
#70131=CARTESIAN_POINT ( 'NONE',  ( -16.51473224551069308, -9.474510206698971260, 61.66557627198103120 ) ) ;
#70132=CARTESIAN_POINT ( 'NONE',  ( -16.51473224551069308, -9.474510206698971260, 61.66557627198103120 ) ) ;
#70134=CARTESIAN_POINT ( 'NONE',  ( -21.53943276465977519, 0.05219959533907696930, 76.24890960531435269 ) ) ;
#70136=CARTESIAN_POINT ( 'NONE',  ( -18.62759615963270932, 10.81492255796079327, 40.83224293864769550 ) ) ;
#70137=CARTESIAN_POINT ( 'NONE',  ( -13.89961937509977652, 13.97604488694528158, 35.62390960531435269 ) ) ;
#70138=CARTESIAN_POINT ( 'NONE',  ( -4.483927247898782831, 16.52544592524335698, 67.70942372801901854 ) ) ;
#70140=CARTESIAN_POINT ( 'NONE',  ( -21.53943276465977519, -0.05219959533937600094, 33.75109039468568284 ) ) ;
#70141=CARTESIAN_POINT ( 'NONE',  ( 14.34966873604960469, 8.224510206698951720, 64.16557627198102409 ) ) ;
#70143=CARTESIAN_POINT ( 'NONE',  ( -8.314922557961024197, 14.29746914071037800, 27.91775706135234358 ) ) ;
#70144=CARTESIAN_POINT ( 'NONE',  ( 13.97604488694548053, -13.89961937509957401, 55.62609039468566863 ) ) ;
#70146=CARTESIAN_POINT ( 'NONE',  ( 12.06949235617757843, -12.14591786802309237, 58.12390960531435979 ) ) ;
#70147=CARTESIAN_POINT ( 'NONE',  ( -10.81492255796105439, 18.62759615963255655, 32.91775706135234714 ) ) ;
#70149=CARTESIAN_POINT ( 'NONE',  ( -21.55341960407610458, -5.719274019375992779, 71.45724293864769550 ) ) ;
#70150=CARTESIAN_POINT ( 'NONE',  ( 19.03943276465977164, -0.05219959533909143690, 98.74890960531436690 ) ) ;
#70151=CARTESIAN_POINT ( 'NONE',  ( -8.314922557960811034, -14.29746914071050412, 72.08224293864769550 ) ) ;
#70153=LINE ( 'NONE', #10488, #76388 ) ;
#70154=CARTESIAN_POINT ( 'NONE',  ( -5.049401038297874678, -19.05341960407617918, 74.79275706135231871 ) ) ;
#70155=CARTESIAN_POINT ( 'NONE',  ( -21.52544592524334988, -5.823673210054445271, 23.95942372801901143 ) ) ;
#70156=CARTESIAN_POINT ( 'NONE',  ( -19.02544592524342804, 5.153800228976336051, 56.04057627198100988 ) ) ;
#70157=CARTESIAN_POINT ( 'NONE',  ( 13.89961937509957401, 13.97604488694547697, 41.87609039468566152 ) ) ;
#70158=CARTESIAN_POINT ( 'NONE',  ( 13.89961937509977652, -13.97604488694527269, 33.12390960531434558 ) ) ;
#70159=CARTESIAN_POINT ( 'NONE',  ( 5.823673210054444382, -21.52544592524334988, 60.20942372801902565 ) ) ;
#70162=CARTESIAN_POINT ( 'NONE',  ( -4.483927247898539470, -16.52544592524342804, 47.29057627198103120 ) ) ;
#70163=CARTESIAN_POINT ( 'NONE',  ( 16.46253265017160672, -9.564922557960803928, 68.33224293864770971 ) ) ;
#70164=CARTESIAN_POINT ( 'NONE',  ( -5.719274019375978568, 21.55341960407610458, 85.20724293864770971 ) ) ;
#70165=CARTESIAN_POINT ( 'NONE',  ( -5.153800228976328057, -19.02544592524343514, 62.29057627198100988 ) ) ;
#70167=CARTESIAN_POINT ( 'NONE',  ( -10.81492255796078084, -18.62759615963271287, 72.08224293864769550 ) ) ;
#70169=CARTESIAN_POINT ( 'NONE',  ( 5.823673210054444382, -21.52544592524334988, 105.2094237280190328 ) ) ;
#70170=FACE_OUTER_BOUND ( 'NONE', #191446, .T. ) ;
#70171=CARTESIAN_POINT ( 'NONE',  ( 16.53943276465976808, 0.05219959533934440121, 91.25109039468568994 ) ) ;
#70172=CARTESIAN_POINT ( 'NONE',  ( -12.14591786802309592, -12.06949235617757132, 76.87390960531439532 ) ) ;
#70173=CARTESIAN_POINT ( 'NONE',  ( -13.97604488694547697, 13.89961937509957934, 98.12609039468566152 ) ) ;
#70175=CARTESIAN_POINT ( 'NONE',  ( -21.55341960407619339, 5.719274019375674811, 23.54275706135235424 ) ) ;
#70176=CARTESIAN_POINT ( 'NONE',  ( 19.02544592524334988, 5.153800228976608722, 46.45942372801899012 ) ) ;
#70177=CARTESIAN_POINT ( 'NONE',  ( 4.379528057220092307, 16.55341960407617563, 97.29275706135234714 ) ) ;
#70178=CARTESIAN_POINT ( 'NONE',  ( 13.89961937509957401, 13.97604488694547697, 36.87609039468565442 ) ) ;
#70179=CARTESIAN_POINT ( 'NONE',  ( 9.564922557960805705, 16.46253265017160317, 89.58224293864769550 ) ) ;
#70180=CARTESIAN_POINT ( 'NONE',  ( 15.72974639402199770, -15.80617190586745480, 58.12390960531435979 ) ) ;
#70182=CARTESIAN_POINT ( 'NONE',  ( -0.05219959533909027116, -19.03943276465977164, 22.49890960531436690 ) ) ;
#70183=CARTESIAN_POINT ( 'NONE',  ( 21.55341960407619695, -5.719274019375665929, 111.0427570613523613 ) ) ;
#70184=CARTESIAN_POINT ( 'NONE',  ( 16.53943276465976808, 0.05219959533934440121, 76.25109039468568994 ) ) ;
#70185=CARTESIAN_POINT ( 'NONE',  ( 10.72451020669871369, 18.67979575497193778, 32.08442372801901854 ) ) ;
#70186=CARTESIAN_POINT ( 'NONE',  ( -16.52544592524335698, -4.483927247898792601, 33.95942372801901143 ) ) ;
#70187=CARTESIAN_POINT ( 'NONE',  ( 16.51473224551069308, 9.474510206698969483, 99.16557627198102409 ) ) ;
#70188=CARTESIAN_POINT ( 'NONE',  ( -16.46253265017160317, 9.564922557960807481, 35.83224293864768839 ) ) ;
#70189=CARTESIAN_POINT ( 'NONE',  ( -19.03943276465977164, 0.05219959533909376836, 61.24890960531436690 ) ) ;
#70191=CARTESIAN_POINT ( 'NONE',  ( 16.55341960407618274, -4.379528057220086978, 51.04275706135234714 ) ) ;
#70192=CARTESIAN_POINT ( 'NONE',  ( 14.34966873604960469, 8.224510206698951720, 99.16557627198100988 ) ) ;
#70193=CARTESIAN_POINT ( 'NONE',  ( 0.05219959533934541429, -16.53943276465976808, 95.00109039468568994 ) ) ;
#70194=CARTESIAN_POINT ( 'NONE',  ( -10.72451020669870658, -18.67979575497194134, 49.58442372801901143 ) ) ;
#70195=CARTESIAN_POINT ( 'NONE',  ( 5.049401038298161559, -19.05341960407611168, 72.70724293864768129 ) ) ;
#70196=CARTESIAN_POINT ( 'NONE',  ( -0.05219959533909027116, -19.03943276465977164, 67.49890960531436690 ) ) ;
#70197=CARTESIAN_POINT ( 'NONE',  ( -16.51473224551069308, -9.474510206698971260, 101.6655762719810241 ) ) ;
#70198=CARTESIAN_POINT ( 'NONE',  ( -0.05219959533910754901, -16.53943276465976808, 32.49890960531435979 ) ) ;
#70199=CARTESIAN_POINT ( 'NONE',  ( 4.483927247898790824, -16.52544592524335698, 105.2094237280190328 ) ) ;
#70201=CARTESIAN_POINT ( 'NONE',  ( 19.02544592524334988, 5.153800228976608722, 41.45942372801900433 ) ) ;
#70202=CARTESIAN_POINT ( 'NONE',  ( -9.474510206698964154, 16.51473224551069663, 110.4155762719810383 ) ) ;
#70203=CARTESIAN_POINT ( 'NONE',  ( 13.97604488694527802, 13.89961937509977652, 69.37390960531436690 ) ) ;
#70204=CARTESIAN_POINT ( 'NONE',  ( -19.05341960407617563, 5.049401038297882671, 38.54275706135233293 ) ) ;
#70206=CARTESIAN_POINT ( 'NONE',  ( -16.18388926212241330, -7.379444403734410685, 65.43953151366150678 ) ) ;
#70207=CARTESIAN_POINT ( 'NONE',  ( 16.52544592524335698, 4.483927247898782831, 36.45942372801901143 ) ) ;
#70208=CARTESIAN_POINT ( 'NONE',  ( 13.97604488694548053, -13.89961937509957401, 75.62609039468564731 ) ) ;
#70209=CARTESIAN_POINT ( 'NONE',  ( -12.14591786802326823, 12.06949235617739902, 53.12609039468568284 ) ) ;
#70211=CARTESIAN_POINT ( 'NONE',  ( -16.51473224551069308, -9.474510206698971260, 96.66557627198102409 ) ) ;
#70212=CARTESIAN_POINT ( 'NONE',  ( -5.719274019375978568, 21.55341960407610458, 110.2072429386477239 ) ) ;
#70213=CARTESIAN_POINT ( 'NONE',  ( -16.51473224551082808, 9.474510206698731452, 83.33442372801899012 ) ) ;
#70214=CARTESIAN_POINT ( 'NONE',  ( -0.05219959533909027116, -19.03943276465977164, 102.4989096053143669 ) ) ;
#70215=CARTESIAN_POINT ( 'NONE',  ( -9.474510206698964154, 16.51473224551069663, 35.41557627198102409 ) ) ;
#70216=CARTESIAN_POINT ( 'NONE',  ( 16.51473224551069308, 9.474510206698969483, 74.16557627198103830 ) ) ;
#70217=CARTESIAN_POINT ( 'NONE',  ( -0.05219959533910754901, -16.53943276465976808, 47.49890960531435979 ) ) ;
#70218=CARTESIAN_POINT ( 'NONE',  ( -0.05219959533909027116, -19.03943276465977164, 32.49890960531435979 ) ) ;
#70219=CARTESIAN_POINT ( 'NONE',  ( -19.02544592524334988, -5.153800228976617603, 53.95942372801898301 ) ) ;
#70220=CARTESIAN_POINT ( 'NONE',  ( -8.314922557960811034, -14.29746914071050412, 87.08224293864769550 ) ) ;
#70221=CARTESIAN_POINT ( 'NONE',  ( 5.049401038297881783, 19.05341960407617563, 22.29275706135233648 ) ) ;
#70222=CARTESIAN_POINT ( 'NONE',  ( 19.05341960407611168, 5.049401038298154454, 48.95724293864768129 ) ) ;
#70223=CARTESIAN_POINT ( 'NONE',  ( -0.05219959533907301413, -21.53943276465977519, 52.49890960531435979 ) ) ;
#70224=CARTESIAN_POINT ( 'NONE',  ( -12.14591786802309592, -12.06949235617757132, 56.87390960531436690 ) ) ;
#70225=CARTESIAN_POINT ( 'NONE',  ( -16.51473224551082808, 9.474510206698731452, 28.33442372801900433 ) ) ;
#70226=CARTESIAN_POINT ( 'NONE',  ( -19.03943276465977164, 0.05219959533909376836, 101.2489096053143669 ) ) ;
#70227=CARTESIAN_POINT ( 'NONE',  ( 19.03943276465977164, -0.05219959533909143690, 108.7489096053143527 ) ) ;
#70228=CARTESIAN_POINT ( 'NONE',  ( -5.153800228976328057, -19.02544592524343514, 42.29057627198101699 ) ) ;
#70229=CARTESIAN_POINT ( 'NONE',  ( -16.46253265017160317, 9.564922557960807481, 30.83224293864769550 ) ) ;
#70230=CARTESIAN_POINT ( 'NONE',  ( -16.55341960407611168, -4.379528057220339221, 91.45724293864769550 ) ) ;
#70231=CARTESIAN_POINT ( 'NONE',  ( 21.53943276465977519, -0.05219959533907433946, 98.74890960531438111 ) ) ;
#70232=CARTESIAN_POINT ( 'NONE',  ( 19.02544592524343514, -5.153800228976328945, 98.54057627198100988 ) ) ;
#70233=CARTESIAN_POINT ( 'NONE',  ( -10.81492255796078084, -18.62759615963271287, 107.0822429386476955 ) ) ;
#70234=CARTESIAN_POINT ( 'NONE',  ( -16.51473224551069308, -9.474510206698971260, 106.6655762719810383 ) ) ;
#70236=CARTESIAN_POINT ( 'NONE',  ( -0.05219959533910754901, -16.53943276465976808, 107.4989096053143669 ) ) ;
#70237=CARTESIAN_POINT ( 'NONE',  ( 16.51473224551069308, 9.474510206698969483, 74.16557627198103830 ) ) ;
#70238=CARTESIAN_POINT ( 'NONE',  ( -21.52544592524343514, 5.823673210054127303, 86.04057627198102409 ) ) ;
#70239=CARTESIAN_POINT ( 'NONE',  ( 17.12812012977027365, -6.668231424565973064, 106.1405124067685506 ) ) ;
#70241=CARTESIAN_POINT ( 'NONE',  ( 18.67979575497178502, 10.72451020669898547, 34.16557627198102409 ) ) ;
#70242=CARTESIAN_POINT ( 'NONE',  ( 18.22780087662122384, -5.500000000000022204, 66.01540105326107266 ) ) ;
#70243=CARTESIAN_POINT ( 'NONE',  ( 14.29746914071037800, 8.314922557961029526, 36.66775706135234714 ) ) ;
#70244=CARTESIAN_POINT ( 'NONE',  ( 8.314922557960818139, 14.29746914071049879, 89.58224293864768129 ) ) ;
#70246=CARTESIAN_POINT ( 'NONE',  ( -19.02544592524342804, 5.153800228976336051, 56.04057627198100988 ) ) ;
#70247=CARTESIAN_POINT ( 'NONE',  ( -8.224510206698948167, 14.34966873604960824, 75.41557627198102409 ) ) ;
#70248=CARTESIAN_POINT ( 'NONE',  ( -15.80617190586745835, -15.72974639402198527, 26.87390960531435979 ) ) ;
#70249=CARTESIAN_POINT ( 'NONE',  ( -16.53943276465976808, 0.05219959533911058130, 61.24890960531435979 ) ) ;
#70250=CARTESIAN_POINT ( 'NONE',  ( 14.29746914071037800, 8.314922557961029526, 26.66775706135235424 ) ) ;
#70251=CARTESIAN_POINT ( 'NONE',  ( -15.72974639402176322, -15.80617190586768395, 74.37609039468568994 ) ) ;
#70252=CARTESIAN_POINT ( 'NONE',  ( 16.20579543436678449, -7.371946100355083686, 76.93479165828125588 ) ) ;
#70253=CARTESIAN_POINT ( 'NONE',  ( 0.05219959533909260263, 19.03943276465977164, 114.9989096053143669 ) ) ;
#70254=CARTESIAN_POINT ( 'NONE',  ( 16.53943276465976808, 0.05219959533934440121, 86.25109039468568994 ) ) ;
#70255=CARTESIAN_POINT ( 'NONE',  ( 16.46253265017160672, -9.564922557960803928, 33.33224293864770260 ) ) ;
#70256=CARTESIAN_POINT ( 'NONE',  ( 13.97604488694527802, 13.89961937509977652, 84.37390960531433848 ) ) ;
#70257=CARTESIAN_POINT ( 'NONE',  ( 21.55341960407610458, 5.719274019375980345, 88.95724293864769550 ) ) ;
#70258=CARTESIAN_POINT ( 'NONE',  ( -12.14591786802326823, 12.06949235617739902, 23.12609039468567573 ) ) ;
#70259=CARTESIAN_POINT ( 'NONE',  ( -4.379528057220328563, 16.55341960407611168, 45.20724293864769550 ) ) ;
#70260=CARTESIAN_POINT ( 'NONE',  ( 5.719274019375673035, 21.55341960407619339, 72.29275706135236135 ) ) ;
#70261=CARTESIAN_POINT ( 'NONE',  ( 16.55341960407618274, -4.379528057220086978, 106.0427570613523471 ) ) ;
#70262=CARTESIAN_POINT ( 'NONE',  ( 19.02544592524343514, -5.153800228976328945, 113.5405762719810241 ) ) ;
#70264=CARTESIAN_POINT ( 'NONE',  ( -12.14591786802326823, 12.06949235617739902, 108.1260903946856757 ) ) ;
#70265=CARTESIAN_POINT ( 'NONE',  ( 14.34966873604972726, -8.224510206698740333, 65.83442372801900433 ) ) ;
#70266=CARTESIAN_POINT ( 'NONE',  ( -5.153800228976328057, -19.02544592524343514, 77.29057627198099567 ) ) ;
#70268=CARTESIAN_POINT ( 'NONE',  ( -0.05219959533909027116, -19.03943276465977164, 82.49890960531436690 ) ) ;
#70269=CARTESIAN_POINT ( 'NONE',  ( -21.52544592524334988, -5.823673210054445271, 73.95942372801901854 ) ) ;
#70270=CARTESIAN_POINT ( 'NONE',  ( -12.06949235617739369, -12.14591786802326823, 69.37609039468567573 ) ) ;
#70271=CARTESIAN_POINT ( 'NONE',  ( 16.55341960407611168, 4.379528057220329451, 63.95724293864770260 ) ) ;
#70272=CARTESIAN_POINT ( 'NONE',  ( -5.049401038298153566, 19.05341960407611168, 50.20724293864770260 ) ) ;
#70274=CARTESIAN_POINT ( 'NONE',  ( 0.05219959533936267826, -19.03943276465977164, 105.0010903946856615 ) ) ;
#70275=CARTESIAN_POINT ( 'NONE',  ( 14.34966873604960469, 8.224510206698951720, 109.1655762719810383 ) ) ;
#70276=CARTESIAN_POINT ( 'NONE',  ( 0.05219959533909260263, 19.03943276465977164, 74.99890960531435269 ) ) ;
#70277=CARTESIAN_POINT ( 'NONE',  ( 16.55341960407618274, -4.379528057220086978, 21.04275706135234714 ) ) ;
#70279=CARTESIAN_POINT ( 'NONE',  ( -15.72974639402176322, -15.80617190586768395, 99.37609039468568994 ) ) ;
#70280=CARTESIAN_POINT ( 'NONE',  ( 16.52544592524335698, 4.483927247898782831, 76.45942372801901854 ) ) ;
#70281=CARTESIAN_POINT ( 'NONE',  ( 9.474510206698729675, 16.51473224551082808, 87.08442372801900433 ) ) ;
#70282=CARTESIAN_POINT ( 'NONE',  ( 19.02544592524343514, -5.153800228976328945, 23.54057627198102054 ) ) ;
#70283=CARTESIAN_POINT ( 'NONE',  ( 4.483927247898790824, -16.52544592524335698, 70.20942372801904696 ) ) ;
#70285=CARTESIAN_POINT ( 'NONE',  ( 5.153800228976615827, -19.02544592524334988, 60.20942372801899012 ) ) ;
#70286=CARTESIAN_POINT ( 'NONE',  ( -21.52544592524334988, -5.823673210054445271, 93.95942372801903275 ) ) ;
#70287=CARTESIAN_POINT ( 'NONE',  ( -5.153800228976328057, -19.02544592524343514, 32.29057627198102409 ) ) ;
#70288=CARTESIAN_POINT ( 'NONE',  ( 19.02544592524343514, -5.153800228976328945, 78.54057627198099567 ) ) ;
#70289=CARTESIAN_POINT ( 'NONE',  ( 16.52544592524342804, -4.483927247898539470, 78.54057627198103830 ) ) ;
#70290=CARTESIAN_POINT ( 'NONE',  ( -21.52544592524334988, -5.823673210054445271, 83.95942372801900433 ) ) ;
#70291=CARTESIAN_POINT ( 'NONE',  ( -0.05219959533936034679, 19.03943276465977164, 52.50109039468566863 ) ) ;
#70292=CARTESIAN_POINT ( 'NONE',  ( 19.03943276465977164, 0.05219959533936151252, 36.25109039468567573 ) ) ;
#70293=CARTESIAN_POINT ( 'NONE',  ( -0.05219959533907301413, -21.53943276465977519, 32.49890960531435979 ) ) ;
#70294=CARTESIAN_POINT ( 'NONE',  ( -0.05219959533937732626, 21.53943276465977519, 102.5010903946856899 ) ) ;
#70295=CARTESIAN_POINT ( 'NONE',  ( -19.05341960407611168, -5.049401038298163336, 81.45724293864769550 ) ) ;
#70296=CARTESIAN_POINT ( 'NONE',  ( 18.62759615963255655, 10.81492255796105972, 86.66775706135234714 ) ) ;
#70297=CARTESIAN_POINT ( 'NONE',  ( -10.81492255796078084, -18.62759615963271287, 57.08224293864769550 ) ) ;
#70298=CARTESIAN_POINT ( 'NONE',  ( 0.05219959533909260263, 19.03943276465977164, 89.99890960531436690 ) ) ;
#70299=CARTESIAN_POINT ( 'NONE',  ( -9.474510206698720793, -16.51473224551083518, 69.58442372801901854 ) ) ;
#70300=CARTESIAN_POINT ( 'NONE',  ( 16.51473224551069308, 9.474510206698969483, 89.16557627198103830 ) ) ;
#70301=CARTESIAN_POINT ( 'NONE',  ( 19.03943276465977164, 0.05219959533936151252, 91.25109039468566152 ) ) ;
#70302=CARTESIAN_POINT ( 'NONE',  ( 16.52544592524335698, 4.483927247898782831, 36.45942372801901143 ) ) ;
#70303=CARTESIAN_POINT ( 'NONE',  ( 4.379528057220339221, -16.55341960407611168, 97.70724293864772392 ) ) ;
#70304=CARTESIAN_POINT ( 'NONE',  ( 5.153800228976335163, 19.02544592524342804, 74.79057627198103830 ) ) ;
#70305=CARTESIAN_POINT ( 'NONE',  ( -0.05219959533907301413, -21.53943276465977519, 62.49890960531436690 ) ) ;
#70306=CARTESIAN_POINT ( 'NONE',  ( 4.483927247898790824, -16.52544592524335698, 30.20942372801902565 ) ) ;
#70307=CARTESIAN_POINT ( 'NONE',  ( -5.823673210054431948, 21.52544592524334988, 32.70942372801900433 ) ) ;
#70308=CARTESIAN_POINT ( 'NONE',  ( 15.80617190586769283, -15.72974639402175789, 85.62609039468568994 ) ) ;
#70309=CARTESIAN_POINT ( 'NONE',  ( 4.483927247898790824, -16.52544592524335698, 80.20942372801901854 ) ) ;
#70310=CARTESIAN_POINT ( 'NONE',  ( 13.89961937509977652, -13.97604488694527269, 78.12390960531433848 ) ) ;
#70311=CARTESIAN_POINT ( 'NONE',  ( 8.314922557960818139, 14.29746914071049879, 79.58224293864769550 ) ) ;
#70312=CARTESIAN_POINT ( 'NONE',  ( 8.314922557961029526, -14.29746914071037800, 100.4177570613523471 ) ) ;
#70313=CARTESIAN_POINT ( 'NONE',  ( -16.46253265017146816, -9.564922557961047289, 49.16775706135233293 ) ) ;
#70314=EDGE_CURVE ( 'NONE', #93191, #45948, #167116, .T. ) ;
#70316=CARTESIAN_POINT ( 'NONE',  ( -0.05219959533937732626, 21.53943276465977519, 27.50109039468567929 ) ) ;
#70317=CARTESIAN_POINT ( 'NONE',  ( 12.06949235617757843, -12.14591786802309237, 83.12390960531436690 ) ) ;
#70318=CARTESIAN_POINT ( 'NONE',  ( -19.03943276465977164, 0.05219959533909376836, 96.24890960531436690 ) ) ;
#70319=CARTESIAN_POINT ( 'NONE',  ( 16.53943276465976808, 0.05219959533934440121, 101.2510903946856757 ) ) ;
#70320=CARTESIAN_POINT ( 'NONE',  ( 21.53943276465977519, 0.05219959533937863772, 71.25109039468568994 ) ) ;
#70321=CARTESIAN_POINT ( 'NONE',  ( 14.34966873604972726, -8.224510206698740333, 45.83442372801901854 ) ) ;
#70322=CARTESIAN_POINT ( 'NONE',  ( 10.81492255796106328, -18.62759615963255655, 40.41775706135234714 ) ) ;
#70323=CARTESIAN_POINT ( 'NONE',  ( 4.483927247898545687, 16.52544592524342804, 69.79057627198102409 ) ) ;
#70324=ORIENTED_EDGE ( 'NONE', *, *, #150999, .T. ) ;
#70325=CARTESIAN_POINT ( 'NONE',  ( 10.72451020669898902, -18.67979575497178502, 112.9155762719810383 ) ) ;
#70326=CARTESIAN_POINT ( 'NONE',  ( 17.50000000000000355, -5.499999999999992006, 26.21769037696436300 ) ) ;
#70327=CARTESIAN_POINT ( 'NONE',  ( -16.53943276465976808, 0.05219959533911058130, 46.24890960531435979 ) ) ;
#70328=CARTESIAN_POINT ( 'NONE',  ( 9.564922557960805705, 16.46253265017160317, 24.58224293864769194 ) ) ;
#70329=CARTESIAN_POINT ( 'NONE',  ( -18.67979575497178146, -10.72451020669898902, 31.66557627198102054 ) ) ;
#70330=CARTESIAN_POINT ( 'NONE',  ( 8.314922557960818139, 14.29746914071049879, 74.58224293864768129 ) ) ;
#70331=CARTESIAN_POINT ( 'NONE',  ( -0.05219959533907301413, -21.53943276465977519, 82.49890960531436690 ) ) ;
#70332=CARTESIAN_POINT ( 'NONE',  ( 16.51473224551069308, 9.474510206698969483, 79.16557627198103830 ) ) ;
#70333=CARTESIAN_POINT ( 'NONE',  ( 9.564922557960805705, 16.46253265017160317, 39.58224293864768839 ) ) ;
#70334=CARTESIAN_POINT ( 'NONE',  ( 9.474510206698729675, 16.51473224551082808, 77.08442372801900433 ) ) ;
#70335=CARTESIAN_POINT ( 'NONE',  ( 18.67979575497194134, -10.72451020669871369, 50.83442372801901143 ) ) ;
#70336=CARTESIAN_POINT ( 'NONE',  ( -15.72974639402197994, 15.80617190586746368, 60.62390960531437401 ) ) ;
#70337=CARTESIAN_POINT ( 'NONE',  ( 19.02544592524343514, -5.153800228976328945, 33.54057627198102409 ) ) ;
#70338=CARTESIAN_POINT ( 'NONE',  ( 0.05219959533909260263, 19.03943276465977164, 74.99890960531435269 ) ) ;
#70339=ORIENTED_EDGE ( 'NONE', *, *, #46382, .T. ) ;
#70340=CARTESIAN_POINT ( 'NONE',  ( 8.314922557961029526, -14.29746914071037800, 55.41775706135234714 ) ) ;
#70341=CARTESIAN_POINT ( 'NONE',  ( 21.52544592524334988, 5.823673210054432836, 36.45942372801901143 ) ) ;
#70342=CARTESIAN_POINT ( 'NONE',  ( -21.55341960407619339, 5.719274019375674811, 58.54275706135235424 ) ) ;
#70343=CARTESIAN_POINT ( 'NONE',  ( 19.03943276465977164, -0.05219959533909143690, 108.7489096053143527 ) ) ;
#70344=CARTESIAN_POINT ( 'NONE',  ( -21.53943276465977519, 0.05219959533907696930, 91.24890960531436690 ) ) ;
#70345=CARTESIAN_POINT ( 'NONE',  ( 5.823673210054444382, -21.52544592524334988, 25.20942372801901854 ) ) ;
#70346=CARTESIAN_POINT ( 'NONE',  ( 4.483927247898790824, -16.52544592524335698, 45.20942372801901854 ) ) ;
#70347=CARTESIAN_POINT ( 'NONE',  ( -5.719274019375978568, 21.55341960407610458, 45.20724293864769550 ) ) ;
#70348=CARTESIAN_POINT ( 'NONE',  ( -9.474510206698720793, -16.51473224551083518, 19.58442372801899722 ) ) ;
#70349=CARTESIAN_POINT ( 'NONE',  ( 19.02544592524343514, -5.153800228976328945, 53.54057627198102409 ) ) ;
#70350=CARTESIAN_POINT ( 'NONE',  ( -19.03943276465977164, 0.05219959533909376836, 116.2489096053143669 ) ) ;
#70351=CARTESIAN_POINT ( 'NONE',  ( -19.05341960407611168, -5.049401038298163336, 91.45724293864766707 ) ) ;
#70352=CARTESIAN_POINT ( 'NONE',  ( -13.97604488694547520, 13.89961937509957934, 53.12609039468566152 ) ) ;
#70353=CARTESIAN_POINT ( 'NONE',  ( 0.05219959533936267826, -19.03943276465977164, 70.00109039468566152 ) ) ;
#70354=CARTESIAN_POINT ( 'NONE',  ( -21.52544592524343514, 5.823673210054127303, 46.04057627198103830 ) ) ;
#70355=CARTESIAN_POINT ( 'NONE',  ( 4.379528057220339221, -16.55341960407611168, 22.70724293864769194 ) ) ;
#70356=CARTESIAN_POINT ( 'NONE',  ( 5.049401038297881783, 19.05341960407617563, 87.29275706135234714 ) ) ;
#70357=CARTESIAN_POINT ( 'NONE',  ( 16.46253265017160672, -9.564922557960803928, 23.33224293864769194 ) ) ;
#70358=CARTESIAN_POINT ( 'NONE',  ( 18.62759615963255655, 10.81492255796105972, 111.6677570613523613 ) ) ;
#70359=CARTESIAN_POINT ( 'NONE',  ( -5.153800228976607833, 19.02544592524334988, 92.70942372801901854 ) ) ;
#70360=CARTESIAN_POINT ( 'NONE',  ( -19.03943276465977164, -0.05219959533935918106, 38.75109039468566152 ) ) ;
#70362=CARTESIAN_POINT ( 'NONE',  ( -5.153800228976328057, -19.02544592524343514, 52.29057627198100988 ) ) ;
#70363=CARTESIAN_POINT ( 'NONE',  ( 4.483927247898545687, 16.52544592524342804, 64.79057627198103830 ) ) ;
#70364=CARTESIAN_POINT ( 'NONE',  ( 19.03943276465977164, -0.05219959533909143690, 33.74890960531435979 ) ) ;
#70365=CARTESIAN_POINT ( 'NONE',  ( 8.314922557960818139, 14.29746914071049879, 34.58224293864770260 ) ) ;
#70366=CARTESIAN_POINT ( 'NONE',  ( 18.22780087662122384, -5.500000000000022204, 56.01540105326107977 ) ) ;
#70367=CARTESIAN_POINT ( 'NONE',  ( -4.483927247898782831, 16.52544592524335698, 102.7094237280190185 ) ) ;
#70368=CARTESIAN_POINT ( 'NONE',  ( 16.46253265017160672, -9.564922557960803928, 63.33224293864769550 ) ) ;
#70369=CARTESIAN_POINT ( 'NONE',  ( 9.564922557961047289, -16.46253265017146816, 20.41775706135233293 ) ) ;
#70370=CARTESIAN_POINT ( 'NONE',  ( -4.483927247898782831, 16.52544592524335698, 27.70942372801901854 ) ) ;
#70371=CARTESIAN_POINT ( 'NONE',  ( 21.55341960407610458, 5.719274019375980345, 48.95724293864770971 ) ) ;
#70372=CARTESIAN_POINT ( 'NONE',  ( 21.55341960407619695, -5.719274019375665929, 106.0427570613523471 ) ) ;
#70373=ORIENTED_EDGE ( 'NONE', *, *, #11302, .F. ) ;
#70374=CARTESIAN_POINT ( 'NONE',  ( -19.05341960407611168, -5.049401038298163336, 61.45724293864769550 ) ) ;
#70375=CARTESIAN_POINT ( 'NONE',  ( -19.02544592524342804, 5.153800228976336051, 111.0405762719810099 ) ) ;
#70376=CARTESIAN_POINT ( 'NONE',  ( -9.564922557960796823, -16.46253265017161027, 102.0822429386477097 ) ) ;
#70378=CARTESIAN_POINT ( 'NONE',  ( -15.80617190586768217, 15.72974639402176855, 28.12609039468568284 ) ) ;
#70379=CARTESIAN_POINT ( 'NONE',  ( -16.52544592524342804, 4.483927247898546575, 91.04057627198103830 ) ) ;
#70380=CARTESIAN_POINT ( 'NONE',  ( 15.72974639402199770, -15.80617190586745480, 83.12390960531436690 ) ) ;
#70381=CARTESIAN_POINT ( 'NONE',  ( -5.153800228976328057, -19.02544592524343514, 62.29057627198100988 ) ) ;
#70382=CARTESIAN_POINT ( 'NONE',  ( 9.564922557960805705, 16.46253265017160317, 69.58224293864770971 ) ) ;
#70383=CARTESIAN_POINT ( 'NONE',  ( 15.72974639402199770, -15.80617190586745480, 113.1239096053143953 ) ) ;
#70385=CARTESIAN_POINT ( 'NONE',  ( 19.02544592524343514, -5.153800228976328945, 68.54057627198103830 ) ) ;
#70387=CARTESIAN_POINT ( 'NONE',  ( 8.224510206698953496, -14.34966873604960469, 107.9155762719810241 ) ) ;
#70389=CARTESIAN_POINT ( 'NONE',  ( 9.474510206698971260, -16.51473224551069308, 67.91557627198102409 ) ) ;
#70390=CARTESIAN_POINT ( 'NONE',  ( 19.05341960407617918, -5.049401038297876454, 91.04275706135234714 ) ) ;
#70391=CARTESIAN_POINT ( 'NONE',  ( 14.34966873604960469, 8.224510206698951720, 99.16557627198100988 ) ) ;
#70392=CARTESIAN_POINT ( 'NONE',  ( -15.80617190586768217, 15.72974639402176855, 68.12609039468567573 ) ) ;
#70393=CARTESIAN_POINT ( 'NONE',  ( 13.89961937509977652, -13.97604488694527269, 43.12390960531434558 ) ) ;
#70394=CARTESIAN_POINT ( 'NONE',  ( -21.55341960407619339, 5.719274019375674811, 33.54275706135234714 ) ) ;
#70395=CARTESIAN_POINT ( 'NONE',  ( -0.05219959533907301413, -21.53943276465977519, 107.4989096053143669 ) ) ;
#70397=CARTESIAN_POINT ( 'NONE',  ( -5.153800228976328057, -19.02544592524343514, 72.29057627198102409 ) ) ;
#70399=CARTESIAN_POINT ( 'NONE',  ( -16.46253265017146816, -9.564922557961047289, 104.1677570613523329 ) ) ;
#70400=CARTESIAN_POINT ( 'NONE',  ( 0.05219959533907565091, 21.53943276465977519, 34.99890960531435979 ) ) ;
#70401=CARTESIAN_POINT ( 'NONE',  ( 18.62759615963255655, 10.81492255796105972, 66.66775706135234714 ) ) ;
#70402=CARTESIAN_POINT ( 'NONE',  ( -16.46253265017160317, 9.564922557960807481, 90.83224293864769550 ) ) ;
#70403=CARTESIAN_POINT ( 'NONE',  ( -13.97604488694547697, 13.89961937509957934, 78.12609039468567573 ) ) ;
#70404=CARTESIAN_POINT ( 'NONE',  ( -9.474510206698964154, 16.51473224551069663, 50.41557627198102409 ) ) ;
#70405=CARTESIAN_POINT ( 'NONE',  ( 13.89961937509977652, -13.97604488694527269, 68.12390960531436690 ) ) ;
#70406=CARTESIAN_POINT ( 'NONE',  ( -4.379528057220328563, 16.55341960407611168, 90.20724293864770971 ) ) ;
#70407=CARTESIAN_POINT ( 'NONE',  ( 9.474510206698971260, -16.51473224551069308, 97.91557627198102409 ) ) ;
#70408=CARTESIAN_POINT ( 'NONE',  ( -14.34966873604960291, -8.224510206698953496, 86.66557627198102409 ) ) ;
#70409=CARTESIAN_POINT ( 'NONE',  ( 19.05341960407611168, 5.049401038298154454, 93.95724293864769550 ) ) ;
#70410=EDGE_CURVE ( 'NONE', #183245, #67326, #56426, .T. ) ;
#70411=CARTESIAN_POINT ( 'NONE',  ( 0.05219959533910956823, 16.53943276465976808, 39.99890960531436690 ) ) ;
#70412=CARTESIAN_POINT ( 'NONE',  ( -9.564922557960796823, -16.46253265017161027, 32.08224293864769550 ) ) ;
#70414=CARTESIAN_POINT ( 'NONE',  ( -0.05219959533937732626, 21.53943276465977519, 57.50109039468568994 ) ) ;
#70415=CARTESIAN_POINT ( 'NONE',  ( 19.05341960407617918, -5.049401038297876454, 86.04275706135233293 ) ) ;
#70416=CARTESIAN_POINT ( 'NONE',  ( 12.14591786802309770, 12.06949235617756955, 44.37390960531435979 ) ) ;
#70417=CARTESIAN_POINT ( 'NONE',  ( -10.72451020669898014, 18.67979575497178502, 95.41557627198102409 ) ) ;
#70418=CARTESIAN_POINT ( 'NONE',  ( 10.72451020669898902, -18.67979575497178502, 27.91557627198103830 ) ) ;
#70419=CARTESIAN_POINT ( 'NONE',  ( 14.29746914071049879, -8.314922557960816363, 88.33224293864769550 ) ) ;
#70420=CARTESIAN_POINT ( 'NONE',  ( 9.474510206698971260, -16.51473224551069308, 57.91557627198103120 ) ) ;
#70421=CARTESIAN_POINT ( 'NONE',  ( 14.29746914071049879, -8.314922557960816363, 23.33224293864769194 ) ) ;
#70423=CARTESIAN_POINT ( 'NONE',  ( -12.06949235617739369, -12.14591786802326823, 99.37609039468568994 ) ) ;
#70424=CARTESIAN_POINT ( 'NONE',  ( 12.06949235617739724, 12.14591786802326823, 76.87609039468567573 ) ) ;
#70425=CARTESIAN_POINT ( 'NONE',  ( 9.564922557961047289, -16.46253265017146816, 25.41775706135234003 ) ) ;
#70426=CARTESIAN_POINT ( 'NONE',  ( -19.03943276465977164, 0.05219959533909376836, 101.2489096053143669 ) ) ;
#70427=CARTESIAN_POINT ( 'NONE',  ( 0.05219959533909260263, 19.03943276465977164, 74.99890960531435269 ) ) ;
#70428=CARTESIAN_POINT ( 'NONE',  ( -19.03943276465977164, 0.05219959533909376836, 31.24890960531435979 ) ) ;
#70429=CARTESIAN_POINT ( 'NONE',  ( 16.52544592524342804, -4.483927247898539470, 48.54057627198103120 ) ) ;
#70430=CARTESIAN_POINT ( 'NONE',  ( -13.97604488694527625, -13.89961937509977652, 101.8739096053143811 ) ) ;
#70431=CARTESIAN_POINT ( 'NONE',  ( 10.72451020669898902, -18.67979575497178502, 42.91557627198103120 ) ) ;
#70432=CARTESIAN_POINT ( 'NONE',  ( 16.55341960407611168, 4.379528057220329451, 78.95724293864769550 ) ) ;
#70433=CARTESIAN_POINT ( 'NONE',  ( -0.05219959533934338120, 16.53943276465976808, 27.50109039468567929 ) ) ;
#70434=CARTESIAN_POINT ( 'NONE',  ( -0.05219959533910754901, -16.53943276465976808, 67.49890960531436690 ) ) ;
#70436=CARTESIAN_POINT ( 'NONE',  ( 19.03943276465977164, 0.05219959533936151252, 66.25109039468567573 ) ) ;
#70437=CARTESIAN_POINT ( 'NONE',  ( 19.05341960407611168, 5.049401038298154454, 103.9572429386476671 ) ) ;
#70438=CARTESIAN_POINT ( 'NONE',  ( -5.153800228976607833, 19.02544592524334988, 77.70942372801900433 ) ) ;
#70439=CARTESIAN_POINT ( 'NONE',  ( -17.58332526062528345, -7.635886036038592728, 39.07665040441535353 ) ) ;
#70440=CARTESIAN_POINT ( 'NONE',  ( -16.51473224551082808, 9.474510206698731452, 113.3344237280190043 ) ) ;
#70441=CARTESIAN_POINT ( 'NONE',  ( 14.34966873604972726, -8.224510206698740333, 105.8344237280190328 ) ) ;
#70442=CARTESIAN_POINT ( 'NONE',  ( -5.153800228976328057, -19.02544592524343514, 37.29057627198102409 ) ) ;
#70443=CARTESIAN_POINT ( 'NONE',  ( -5.719274019375978568, 21.55341960407610458, 35.20724293864768839 ) ) ;
#70444=CARTESIAN_POINT ( 'NONE',  ( 10.81492255796106328, -18.62759615963255655, 60.41775706135235424 ) ) ;
#70446=CARTESIAN_POINT ( 'NONE',  ( -8.224510206698735004, -14.34966873604973081, 24.58442372801901499 ) ) ;
#70447=CARTESIAN_POINT ( 'NONE',  ( 17.49999999999985079, 3.193340300986046820, 22.66536441064387475 ) ) ;
#70448=CARTESIAN_POINT ( 'NONE',  ( -5.049401038298153566, 19.05341960407611168, 70.20724293864769550 ) ) ;
#70450=CARTESIAN_POINT ( 'NONE',  ( -16.51473224551069308, -9.474510206698971260, 21.66557627198102765 ) ) ;
#70451=CARTESIAN_POINT ( 'NONE',  ( 12.14591786802309770, 12.06949235617756955, 84.37390960531438111 ) ) ;
#70452=CARTESIAN_POINT ( 'NONE',  ( -9.474510206698964154, 16.51473224551069663, 70.41557627198102409 ) ) ;
#70453=CARTESIAN_POINT ( 'NONE',  ( -16.46253265017160317, 9.564922557960807481, 90.83224293864769550 ) ) ;
#70455=CARTESIAN_POINT ( 'NONE',  ( -9.564922557961040184, 16.46253265017147172, 87.91775706135233293 ) ) ;
#70456=CARTESIAN_POINT ( 'NONE',  ( 5.719274019375991003, -21.55341960407610458, 62.70724293864769550 ) ) ;
#70457=CARTESIAN_POINT ( 'NONE',  ( 16.51473224551069308, 9.474510206698969483, 24.16557627198102765 ) ) ;
#70458=CARTESIAN_POINT ( 'NONE',  ( -16.51473224551082808, 9.474510206698731452, 53.33442372801900433 ) ) ;
#70459=CARTESIAN_POINT ( 'NONE',  ( -19.03943276465977164, 0.05219959533909376836, 61.24890960531436690 ) ) ;
#70460=CARTESIAN_POINT ( 'NONE',  ( 16.46253265017160672, -9.564922557960803928, 88.33224293864769550 ) ) ;
#70462=CARTESIAN_POINT ( 'NONE',  ( -15.72974639402197994, 15.80617190586746368, 100.6239096053143811 ) ) ;
#70463=CARTESIAN_POINT ( 'NONE',  ( -12.14591786802309592, -12.06949235617757132, 91.87390960531436690 ) ) ;
#70464=CARTESIAN_POINT ( 'NONE',  ( -16.46253265017160317, 9.564922557960807481, 85.83224293864769550 ) ) ;
#70465=CARTESIAN_POINT ( 'NONE',  ( -19.05341960407617563, 5.049401038297882671, 58.54275706135234003 ) ) ;
#70466=CARTESIAN_POINT ( 'NONE',  ( 5.823673210054125526, 21.52544592524343514, 94.79057627198105251 ) ) ;
#70467=CARTESIAN_POINT ( 'NONE',  ( 21.55341960407610458, 5.719274019375980345, 68.95724293864769550 ) ) ;
#70468=CARTESIAN_POINT ( 'NONE',  ( 4.483927247898545687, 16.52544592524342804, 34.79057627198103120 ) ) ;
#70469=CARTESIAN_POINT ( 'NONE',  ( -15.80617190586768217, 15.72974639402176855, 98.12609039468570415 ) ) ;
#70470=CARTESIAN_POINT ( 'NONE',  ( 12.14591786802327356, -12.06949235617739191, 60.62609039468567573 ) ) ;
#70471=CARTESIAN_POINT ( 'NONE',  ( -19.05341960407611168, -5.049401038298163336, 81.45724293864769550 ) ) ;
#70472=CARTESIAN_POINT ( 'NONE',  ( 13.89961937509977652, -13.97604488694527269, 28.12390960531435624 ) ) ;
#70473=CARTESIAN_POINT ( 'NONE',  ( -21.53943276465977519, -0.05219959533937600094, 33.75109039468568284 ) ) ;
#70474=CARTESIAN_POINT ( 'NONE',  ( -21.52544592524334988, -5.823673210054445271, 48.95942372801902565 ) ) ;
#70475=CARTESIAN_POINT ( 'NONE',  ( -9.564922557960796823, -16.46253265017161027, 47.08224293864769550 ) ) ;
#70476=CARTESIAN_POINT ( 'NONE',  ( -5.719274019375978568, 21.55341960407610458, 115.2072429386476955 ) ) ;
#70477=CARTESIAN_POINT ( 'NONE',  ( 13.97604488694548053, -13.89961937509957401, 70.62609039468567573 ) ) ;
#70478=CARTESIAN_POINT ( 'NONE',  ( -16.46253265017146816, -9.564922557961047289, 74.16775706135234714 ) ) ;
#70479=CARTESIAN_POINT ( 'NONE',  ( 9.564922557960805705, 16.46253265017160317, 29.58224293864769550 ) ) ;
#70480=CARTESIAN_POINT ( 'NONE',  ( -16.53943276465976808, -0.05219959533934237506, 78.75109039468568994 ) ) ;
#70481=CARTESIAN_POINT ( 'NONE',  ( 9.474510206698971260, -16.51473224551069308, 47.91557627198102409 ) ) ;
#70483=CARTESIAN_POINT ( 'NONE',  ( -13.97604488694527625, -13.89961937509977652, 96.87390960531433848 ) ) ;
#70484=CARTESIAN_POINT ( 'NONE',  ( 19.05341960407611168, 5.049401038298154454, 38.95724293864767418 ) ) ;
#70485=CARTESIAN_POINT ( 'NONE',  ( 21.53943276465977519, -0.05219959533907433946, 68.74890960531435269 ) ) ;
#70486=CARTESIAN_POINT ( 'NONE',  ( 14.34966873604972726, -8.224510206698740333, 55.83442372801901854 ) ) ;
#70487=CARTESIAN_POINT ( 'NONE',  ( -18.62759615963255300, -10.81492255796106328, 109.1677570613523613 ) ) ;
#70488=CARTESIAN_POINT ( 'NONE',  ( 0.05219959533909260263, 19.03943276465977164, 54.99890960531435979 ) ) ;
#70489=CARTESIAN_POINT ( 'NONE',  ( 12.06949235617757843, -12.14591786802309237, 33.12390960531435979 ) ) ;
#70490=CARTESIAN_POINT ( 'NONE',  ( 14.29746914071049879, -8.314922557960816363, 68.33224293864769550 ) ) ;
#70491=CARTESIAN_POINT ( 'NONE',  ( -19.03943276465977164, 0.05219959533909376836, 76.24890960531435269 ) ) ;
#70492=CARTESIAN_POINT ( 'NONE',  ( -0.05219959533937732626, 21.53943276465977519, 42.50109039468567573 ) ) ;
#70493=CARTESIAN_POINT ( 'NONE',  ( 5.049401038298161559, -19.05341960407611168, 87.70724293864769550 ) ) ;
#70494=CARTESIAN_POINT ( 'NONE',  ( 0.05219959533937995610, -21.53943276465977519, 100.0010903946857042 ) ) ;
#70495=CARTESIAN_POINT ( 'NONE',  ( 4.379528057220092307, 16.55341960407617563, 67.29275706135234714 ) ) ;
#70496=CARTESIAN_POINT ( 'NONE',  ( -19.05341960407611168, -5.049401038298163336, 111.4572429386476671 ) ) ;
#70497=CARTESIAN_POINT ( 'NONE',  ( 5.823673210054125526, 21.52544592524343514, 94.79057627198105251 ) ) ;
#70498=CARTESIAN_POINT ( 'NONE',  ( 0.05219959533910956823, 16.53943276465976808, 49.99890960531437401 ) ) ;
#70499=CARTESIAN_POINT ( 'NONE',  ( 19.03943276465977164, -0.05219959533909143690, 43.74890960531435979 ) ) ;
#70500=CARTESIAN_POINT ( 'NONE',  ( -8.224510206698735004, -14.34966873604973081, 54.58442372801901143 ) ) ;
#70501=CARTESIAN_POINT ( 'NONE',  ( 12.06949235617757843, -12.14591786802309237, 63.12390960531435979 ) ) ;
#70502=CARTESIAN_POINT ( 'NONE',  ( 19.05341960407611168, 5.049401038298154454, 113.9572429386477097 ) ) ;
#70503=CARTESIAN_POINT ( 'NONE',  ( 18.62759615963271287, -10.81492255796078972, 38.33224293864768839 ) ) ;
#70504=CARTESIAN_POINT ( 'NONE',  ( 13.89961937509957401, 13.97604488694547697, 26.87609039468566507 ) ) ;
#70505=CARTESIAN_POINT ( 'NONE',  ( -4.379528057220328563, 16.55341960407611168, 95.20724293864769550 ) ) ;
#70506=CARTESIAN_POINT ( 'NONE',  ( 0.05219959533909260263, 19.03943276465977164, 109.9989096053143669 ) ) ;
#70508=CARTESIAN_POINT ( 'NONE',  ( 4.379528057220092307, 16.55341960407617563, 52.29275706135236135 ) ) ;
#70509=CARTESIAN_POINT ( 'NONE',  ( 16.51473224551069308, 9.474510206698969483, 59.16557627198102409 ) ) ;
#70511=CARTESIAN_POINT ( 'NONE',  ( 9.474510206698729675, 16.51473224551082808, 52.08442372801900433 ) ) ;
#70512=CARTESIAN_POINT ( 'NONE',  ( -14.29746914071037622, -8.314922557961029526, 99.16775706135234714 ) ) ;
#70513=CARTESIAN_POINT ( 'NONE',  ( -16.51473224551082808, 9.474510206698731452, 98.33442372801900433 ) ) ;
#70514=CARTESIAN_POINT ( 'NONE',  ( 5.823673210054444382, -21.52544592524334988, 65.20942372801901854 ) ) ;
#70515=CARTESIAN_POINT ( 'NONE',  ( 0.05219959533909260263, 19.03943276465977164, 74.99890960531435269 ) ) ;
#70516=CARTESIAN_POINT ( 'NONE',  ( -5.719274019375978568, 21.55341960407610458, 95.20724293864769550 ) ) ;
#70517=CARTESIAN_POINT ( 'NONE',  ( -8.224510206698948167, 14.34966873604960824, 110.4155762719810383 ) ) ;
#70518=CARTESIAN_POINT ( 'NONE',  ( -13.89961937509957401, -13.97604488694547875, 79.37609039468567573 ) ) ;
#70519=CARTESIAN_POINT ( 'NONE',  ( 15.72974639402199770, -15.80617190586745480, 73.12390960531436690 ) ) ;
#70520=CARTESIAN_POINT ( 'NONE',  ( -13.97604488694547697, 13.89961937509957934, 38.12609039468566152 ) ) ;
#70521=CARTESIAN_POINT ( 'NONE',  ( 19.01529144963337004, 5.500000000000029310, 98.73431955728440812 ) ) ;
#70522=CARTESIAN_POINT ( 'NONE',  ( -15.72974639402197994, 15.80617190586746368, 90.62390960531436690 ) ) ;
#70523=CARTESIAN_POINT ( 'NONE',  ( -19.25663599770061651, 5.499999999999450218, 53.99419308057203182 ) ) ;
#70524=CARTESIAN_POINT ( 'NONE',  ( -19.05341960407611168, -5.049401038298163336, 66.45724293864769550 ) ) ;
#70526=CARTESIAN_POINT ( 'NONE',  ( 12.14591786802327356, -12.06949235617739191, 25.62609039468567929 ) ) ;
#70528=CARTESIAN_POINT ( 'NONE',  ( 16.46253265017160672, -9.564922557960803928, 48.33224293864769550 ) ) ;
#70529=CARTESIAN_POINT ( 'NONE',  ( -19.05341960407611168, -5.049401038298163336, 111.4572429386476671 ) ) ;
#70530=CARTESIAN_POINT ( 'NONE',  ( -10.81492255796078084, -18.62759615963271287, 102.0822429386476955 ) ) ;
#70531=CARTESIAN_POINT ( 'NONE',  ( -0.05219959533910754901, -16.53943276465976808, 52.49890960531435979 ) ) ;
#70532=CARTESIAN_POINT ( 'NONE',  ( -5.719274019375665041, -21.55341960407619695, 74.79275706135234714 ) ) ;
#70533=CARTESIAN_POINT ( 'NONE',  ( 14.34966873604972726, -8.224510206698740333, 30.83442372801902209 ) ) ;
#70534=CARTESIAN_POINT ( 'NONE',  ( -16.46253265017146816, -9.564922557961047289, 34.16775706135233293 ) ) ;
#70535=CARTESIAN_POINT ( 'NONE',  ( 12.06949235617757843, -12.14591786802309237, 33.12390960531435979 ) ) ;
#70536=CARTESIAN_POINT ( 'NONE',  ( 21.55341960407619695, -5.719274019375665929, 41.04275706135236135 ) ) ;
#70537=CARTESIAN_POINT ( 'NONE',  ( -0.05219959533907301413, -21.53943276465977519, 112.4989096053143669 ) ) ;
#70538=CARTESIAN_POINT ( 'NONE',  ( 12.06949235617757843, -12.14591786802309237, 43.12390960531435269 ) ) ;
#70539=CARTESIAN_POINT ( 'NONE',  ( 16.51473224551083163, -9.474510206698727899, 100.8344237280190043 ) ) ;
#70541=CARTESIAN_POINT ( 'NONE',  ( 0.05219959533936267826, -19.03943276465977164, 70.00109039468566152 ) ) ;
#70542=CARTESIAN_POINT ( 'NONE',  ( 5.719274019375673035, 21.55341960407619339, 67.29275706135234714 ) ) ;
#70543=CARTESIAN_POINT ( 'NONE',  ( -5.049401038297874678, -19.05341960407617918, 49.79275706135231871 ) ) ;
#70544=CARTESIAN_POINT ( 'NONE',  ( 0.05219959533909260263, 19.03943276465977164, 24.99890960531435269 ) ) ;
#70545=CARTESIAN_POINT ( 'NONE',  ( 21.53943276465977519, -0.05219959533907433946, 43.74890960531435979 ) ) ;
#70546=CARTESIAN_POINT ( 'NONE',  ( 8.314922557960818139, 14.29746914071049879, 54.58224293864769550 ) ) ;
#70548=CARTESIAN_POINT ( 'NONE',  ( 5.823673210054444382, -21.52544592524334988, 110.2094237280190185 ) ) ;
#70549=CARTESIAN_POINT ( 'NONE',  ( 4.379528057220092307, 16.55341960407617563, 87.29275706135236135 ) ) ;
#70550=CARTESIAN_POINT ( 'NONE',  ( 8.314922557960818139, 14.29746914071049879, 34.58224293864770260 ) ) ;
#70551=CARTESIAN_POINT ( 'NONE',  ( -15.72974639402176322, -15.80617190586768395, 69.37609039468567573 ) ) ;
#70552=CARTESIAN_POINT ( 'NONE',  ( -10.72451020669870658, -18.67979575497194134, 84.58442372801903275 ) ) ;
#70553=CARTESIAN_POINT ( 'NONE',  ( -10.81492255796078084, -18.62759615963271287, 82.08224293864768129 ) ) ;
#70554=CARTESIAN_POINT ( 'NONE',  ( 16.46253265017160672, -9.564922557960803928, 38.33224293864768839 ) ) ;
#70555=CARTESIAN_POINT ( 'NONE',  ( 21.53943276465977519, 0.05219959533937863772, 61.25109039468567573 ) ) ;
#70556=CARTESIAN_POINT ( 'NONE',  ( 13.89961937509977652, -13.97604488694527269, 38.12390960531436690 ) ) ;
#70557=CARTESIAN_POINT ( 'NONE',  ( 13.97604488694527802, 13.89961937509977652, 49.37390960531434558 ) ) ;
#70558=CARTESIAN_POINT ( 'NONE',  ( -16.55341960407611168, -4.379528057220339221, 86.45724293864770971 ) ) ;
#70559=CARTESIAN_POINT ( 'NONE',  ( 9.564922557960805705, 16.46253265017160317, 94.58224293864769550 ) ) ;
#70560=CARTESIAN_POINT ( 'NONE',  ( -16.52544592524342804, 4.483927247898546575, 41.04057627198103120 ) ) ;
#70561=CARTESIAN_POINT ( 'NONE',  ( 12.14591786802309770, 12.06949235617756955, 114.3739096053143527 ) ) ;
#70562=CARTESIAN_POINT ( 'NONE',  ( -18.67979575497178146, -10.72451020669898902, 76.66557627198103830 ) ) ;
#70563=CARTESIAN_POINT ( 'NONE',  ( 5.823673210054125526, 21.52544592524343514, 114.7905762719810383 ) ) ;
#70565=CARTESIAN_POINT ( 'NONE',  ( -13.97604488694527625, -13.89961937509977652, 81.87390960531436690 ) ) ;
#70566=CARTESIAN_POINT ( 'NONE',  ( 14.34966873604972726, -8.224510206698740333, 20.83442372801901143 ) ) ;
#70567=CARTESIAN_POINT ( 'NONE',  ( 10.81492255796078972, 18.62759615963270932, 74.58224293864768129 ) ) ;
#70568=CARTESIAN_POINT ( 'NONE',  ( 21.55341960407619695, -5.719274019375665929, 96.04275706135236135 ) ) ;
#70569=CARTESIAN_POINT ( 'NONE',  ( -16.46253265017160317, 9.564922557960807481, 75.83224293864769550 ) ) ;
#70570=CARTESIAN_POINT ( 'NONE',  ( 10.81492255796106328, -18.62759615963255655, 35.41775706135234003 ) ) ;
#70571=CARTESIAN_POINT ( 'NONE',  ( -15.80617190586745835, -15.72974639402198527, 21.87390960531436690 ) ) ;
#70572=CARTESIAN_POINT ( 'NONE',  ( -8.224510206698735004, -14.34966873604973081, 84.58442372801903275 ) ) ;
#70573=CARTESIAN_POINT ( 'NONE',  ( 15.72974639402176855, 15.80617190586768217, 66.87609039468568994 ) ) ;
#70574=CARTESIAN_POINT ( 'NONE',  ( -21.55341960407619339, 5.719274019375674811, 103.5427570613523613 ) ) ;
#70575=CARTESIAN_POINT ( 'NONE',  ( 14.34966873604972726, -8.224510206698740333, 80.83442372801901854 ) ) ;
#70576=CARTESIAN_POINT ( 'NONE',  ( -21.53943276465977519, -0.05219959533937600094, 23.75109039468567929 ) ) ;
#70577=CARTESIAN_POINT ( 'NONE',  ( 9.474510206698971260, -16.51473224551069308, 22.91557627198102765 ) ) ;
#70578=CARTESIAN_POINT ( 'NONE',  ( 0.05219959533937995610, -21.53943276465977519, 95.00109039468568994 ) ) ;
#70579=CARTESIAN_POINT ( 'NONE',  ( 5.049401038298161559, -19.05341960407611168, 87.70724293864769550 ) ) ;
#70580=CARTESIAN_POINT ( 'NONE',  ( -15.72974639402197994, 15.80617190586746368, 85.62390960531436690 ) ) ;
#70581=CARTESIAN_POINT ( 'NONE',  ( 19.05341960407617918, -5.049401038297876454, 56.04275706135234714 ) ) ;
#70583=CARTESIAN_POINT ( 'NONE',  ( 21.53943276465977519, -0.05219959533907433946, 53.74890960531437401 ) ) ;
#70584=CARTESIAN_POINT ( 'NONE',  ( 9.564922557960805705, 16.46253265017160317, 89.58224293864769550 ) ) ;
#70585=CARTESIAN_POINT ( 'NONE',  ( -0.05219959533910754901, -16.53943276465976808, 52.49890960531435979 ) ) ;
#70587=CARTESIAN_POINT ( 'NONE',  ( -19.02544592524334988, -5.153800228976617603, 83.95942372801901854 ) ) ;
#70588=AXIS2_PLACEMENT_3D ( 'NONE', #93550, #13740, #183598 ) ;
#70590=CARTESIAN_POINT ( 'NONE',  ( -19.05341960407617563, 5.049401038297882671, 113.5427570613523471 ) ) ;
#70591=CARTESIAN_POINT ( 'NONE',  ( 21.55341960407610458, 5.719274019375980345, 78.95724293864769550 ) ) ;
#70592=CARTESIAN_POINT ( 'NONE',  ( -12.14591786802309592, -12.06949235617757132, 66.87390960531436690 ) ) ;
#70593=CARTESIAN_POINT ( 'NONE',  ( -19.03943276465977164, 0.05219959533909376836, 96.24890960531436690 ) ) ;
#70594=CARTESIAN_POINT ( 'NONE',  ( 12.06949235617739724, 12.14591786802326823, 41.87609039468568284 ) ) ;
#70595=CARTESIAN_POINT ( 'NONE',  ( 16.46253265017160672, -9.564922557960803928, 58.33224293864769550 ) ) ;
#70596=CARTESIAN_POINT ( 'NONE',  ( -18.67979575497178146, -10.72451020669898902, 111.6655762719810525 ) ) ;
#70597=CARTESIAN_POINT ( 'NONE',  ( 13.89961937509957401, 13.97604488694547697, 86.87609039468567573 ) ) ;
#70598=CARTESIAN_POINT ( 'NONE',  ( -13.97604488694527625, -13.89961937509977652, 96.87390960531433848 ) ) ;
#70599=( BOUNDED_CURVE ( )  B_SPLINE_CURVE ( 2, ( #162723, #24228, #85879, #39378, #146541, #102053, #118229, #54546, #177910, #103052, #9052, #52539, #194083 ),
 .UNSPECIFIED., .F., .F. ) 
 B_SPLINE_CURVE_WITH_KNOTS ( ( 3, 2, 2, 2, 2, 2, 3 ),
 ( 0.2656340109859774423, 0.2675438596491228060, 0.2719298245614035214, 0.2763157894736842368, 0.2807017543859648967, 0.2850877192982456121, 0.2870432477834812812 ),
 .UNSPECIFIED. ) 
 CURVE ( )  GEOMETRIC_REPRESENTATION_ITEM ( )  RATIONAL_B_SPLINE_CURVE ( ( 0.9832469066685285419, 0.9851625545550100060, 1.000000000000000000, 0.9659258262890683122, 1.000000000000000000, 0.9659258262890683122, 1.000000000000000000, 0.9659258262890683122, 1.000000000000000000, 0.9659258262890683122, 1.000000000000000000, 0.9848076720550082985, 0.9831626618144002627 ) ) 
 REPRESENTATION_ITEM ( '' )  );
#70600=CARTESIAN_POINT ( 'NONE',  ( 13.89961937509977652, -13.97604488694527269, 78.12390960531433848 ) ) ;
#70601=CARTESIAN_POINT ( 'NONE',  ( -10.72451020669898014, 18.67979575497178502, 80.41557627198103830 ) ) ;
#70602=CARTESIAN_POINT ( 'NONE',  ( -9.564922557960796823, -16.46253265017161027, 47.08224293864769550 ) ) ;
#70604=CARTESIAN_POINT ( 'NONE',  ( 4.379528057220339221, -16.55341960407611168, 52.70724293864769550 ) ) ;
#70605=CARTESIAN_POINT ( 'NONE',  ( -9.564922557960796823, -16.46253265017161027, 97.08224293864769550 ) ) ;
#70607=CARTESIAN_POINT ( 'NONE',  ( 9.474510206698729675, 16.51473224551082808, 67.08442372801900433 ) ) ;
#70608=CARTESIAN_POINT ( 'NONE',  ( 10.72451020669898902, -18.67979575497178502, 92.91557627198103830 ) ) ;
#70609=CARTESIAN_POINT ( 'NONE',  ( -5.049401038297874678, -19.05341960407617918, 44.79275706135232582 ) ) ;
#70610=CARTESIAN_POINT ( 'NONE',  ( -9.564922557960796823, -16.46253265017161027, 97.08224293864769550 ) ) ;
#70612=CARTESIAN_POINT ( 'NONE',  ( 5.719274019375991003, -21.55341960407610458, 42.70724293864770260 ) ) ;
#70613=CARTESIAN_POINT ( 'NONE',  ( 13.97604488694527802, 13.89961937509977652, 69.37390960531436690 ) ) ;
#70614=CARTESIAN_POINT ( 'NONE',  ( 18.67979575497194134, -10.72451020669871369, 65.83442372801900433 ) ) ;
#70615=CARTESIAN_POINT ( 'NONE',  ( -16.46253265017160317, 9.564922557960807481, 35.83224293864768839 ) ) ;
#70617=CARTESIAN_POINT ( 'NONE',  ( 4.483927247898545687, 16.52544592524342804, 74.79057627198105251 ) ) ;
#70619=CARTESIAN_POINT ( 'NONE',  ( 16.52544592524335698, 4.483927247898782831, 26.45942372801901854 ) ) ;
#70620=CARTESIAN_POINT ( 'NONE',  ( 15.72974639402176855, 15.80617190586768217, 56.87609039468568994 ) ) ;
#70621=ORIENTED_EDGE ( 'NONE', *, *, #59834, .F. ) ;
#70623=CARTESIAN_POINT ( 'NONE',  ( -0.05219959533936034679, 19.03943276465977164, 67.50109039468566152 ) ) ;
#70625=CARTESIAN_POINT ( 'NONE',  ( -21.53943276465977519, 0.05219959533907696930, 116.2489096053143669 ) ) ;
#70626=CARTESIAN_POINT ( 'NONE',  ( 13.97604488694527802, 13.89961937509977652, 54.37390960531435979 ) ) ;
#70628=CARTESIAN_POINT ( 'NONE',  ( 19.05341960407617918, -5.049401038297876454, 26.04275706135233293 ) ) ;
#70629=CARTESIAN_POINT ( 'NONE',  ( 19.05341960407611168, 5.049401038298154454, 43.95724293864769550 ) ) ;
#70630=CARTESIAN_POINT ( 'NONE',  ( 10.81492255796106328, -18.62759615963255655, 110.4177570613523756 ) ) ;
#70631=CARTESIAN_POINT ( 'NONE',  ( 12.06949235617739724, 12.14591786802326823, 86.87609039468568994 ) ) ;
#70633=CARTESIAN_POINT ( 'NONE',  ( 16.51473224551069308, 9.474510206698969483, 99.16557627198102409 ) ) ;
#70634=CARTESIAN_POINT ( 'NONE',  ( -21.53943276465977519, -0.05219959533937600094, 68.75109039468568994 ) ) ;
#70636=CARTESIAN_POINT ( 'NONE',  ( -19.03943276465977164, 0.05219959533909376836, 116.2489096053143669 ) ) ;
#70638=CARTESIAN_POINT ( 'NONE',  ( -12.14591786802326823, 12.06949235617739902, 53.12609039468568284 ) ) ;
#70639=CARTESIAN_POINT ( 'NONE',  ( -18.62759615963255300, -10.81492255796106328, 69.16775706135234714 ) ) ;
#70640=CARTESIAN_POINT ( 'NONE',  ( 5.823673210054444382, -21.52544592524334988, 100.2094237280190043 ) ) ;
#70642=CARTESIAN_POINT ( 'NONE',  ( -16.53943276465976808, -0.05219959533934237506, 38.75109039468567573 ) ) ;
#70643=CARTESIAN_POINT ( 'NONE',  ( 13.89961937509977652, -13.97604488694527269, 83.12390960531436690 ) ) ;
#70644=CARTESIAN_POINT ( 'NONE',  ( -19.02544592524342804, 5.153800228976336051, 111.0405762719810099 ) ) ;
#70646=CARTESIAN_POINT ( 'NONE',  ( 16.88567814943166212, 6.947325034625596807, 43.79001122652586986 ) ) ;
#70647=CARTESIAN_POINT ( 'NONE',  ( 13.97604488694527802, 13.89961937509977652, 39.37390960531435269 ) ) ;
#70648=CARTESIAN_POINT ( 'NONE',  ( 10.81492255796078972, 18.62759615963270932, 49.58224293864769550 ) ) ;
#70649=CARTESIAN_POINT ( 'NONE',  ( -16.52544592524335698, -4.483927247898792601, 108.9594237280190185 ) ) ;
#70650=CARTESIAN_POINT ( 'NONE',  ( -4.379528057220328563, 16.55341960407611168, 85.20724293864770971 ) ) ;
#70651=CARTESIAN_POINT ( 'NONE',  ( -16.51473224551069308, -9.474510206698971260, 76.66557627198103830 ) ) ;
#70652=CARTESIAN_POINT ( 'NONE',  ( -10.81492255796105439, 18.62759615963255655, 107.9177570613523471 ) ) ;
#70653=CARTESIAN_POINT ( 'NONE',  ( 8.314922557961029526, -14.29746914071037800, 20.41775706135234714 ) ) ;
#70654=CARTESIAN_POINT ( 'NONE',  ( -14.29746914071049879, 8.314922557960819915, 85.83224293864768129 ) ) ;
#70655=CARTESIAN_POINT ( 'NONE',  ( 10.81492255796106328, -18.62759615963255655, 35.41775706135234003 ) ) ;
#70656=CARTESIAN_POINT ( 'NONE',  ( 5.823673210054125526, 21.52544592524343514, 69.79057627198102409 ) ) ;
#70657=CARTESIAN_POINT ( 'NONE',  ( 13.89961937509957401, 13.97604488694547697, 56.87609039468564731 ) ) ;
#70659=CARTESIAN_POINT ( 'NONE',  ( -0.05219959533909027116, -19.03943276465977164, 92.49890960531436690 ) ) ;
#70660=CARTESIAN_POINT ( 'NONE',  ( -0.05219959533910754901, -16.53943276465976808, 62.49890960531436690 ) ) ;
#70661=CARTESIAN_POINT ( 'NONE',  ( -12.06949235617756955, 12.14591786802309770, 50.62390960531435979 ) ) ;
#70662=CARTESIAN_POINT ( 'NONE',  ( 14.29746914071037800, 8.314922557961029526, 111.6677570613523613 ) ) ;
#70663=CARTESIAN_POINT ( 'NONE',  ( 5.153800228976615827, -19.02544592524334988, 70.20942372801899012 ) ) ;
#70665=CARTESIAN_POINT ( 'NONE',  ( -5.823673210054116645, -21.52544592524344225, 27.29057627198103120 ) ) ;
#70666=CARTESIAN_POINT ( 'NONE',  ( 4.379528057220339221, -16.55341960407611168, 87.70724293864769550 ) ) ;
#70668=CARTESIAN_POINT ( 'NONE',  ( -9.564922557960796823, -16.46253265017161027, 42.08224293864769550 ) ) ;
#70669=CARTESIAN_POINT ( 'NONE',  ( 5.719274019375991003, -21.55341960407610458, 42.70724293864770260 ) ) ;
#70670=CARTESIAN_POINT ( 'NONE',  ( -9.474510206698964154, 16.51473224551069663, 25.41557627198103120 ) ) ;
#70671=CARTESIAN_POINT ( 'NONE',  ( -12.06949235617739369, -12.14591786802326823, 64.37609039468568994 ) ) ;
#70672=CARTESIAN_POINT ( 'NONE',  ( 9.564922557960805705, 16.46253265017160317, 64.58224293864769550 ) ) ;
#70673=CARTESIAN_POINT ( 'NONE',  ( 5.153800228976615827, -19.02544592524334988, 40.20942372801898301 ) ) ;
#70674=CARTESIAN_POINT ( 'NONE',  ( -18.67979575497193778, 10.72451020669871902, 53.33442372801901854 ) ) ;
#70676=CARTESIAN_POINT ( 'NONE',  ( 15.72974639402199770, -15.80617190586745480, 38.12390960531436690 ) ) ;
#70677=CARTESIAN_POINT ( 'NONE',  ( 8.314922557960818139, 14.29746914071049879, 99.58224293864770971 ) ) ;
#70678=CARTESIAN_POINT ( 'NONE',  ( -9.564922557961040184, 16.46253265017147172, 92.91775706135233293 ) ) ;
#70681=CARTESIAN_POINT ( 'NONE',  ( 21.53943276465977519, -0.05219959533907433946, 48.74890960531435979 ) ) ;
#70682=CARTESIAN_POINT ( 'NONE',  ( -5.153800228976328057, -19.02544592524343514, 27.29057627198103120 ) ) ;
#70683=CARTESIAN_POINT ( 'NONE',  ( -15.72974639402176322, -15.80617190586768395, 89.37609039468568994 ) ) ;
#70684=CARTESIAN_POINT ( 'NONE',  ( -14.29746914071049879, 8.314922557960819915, 45.83224293864769550 ) ) ;
#70685=CARTESIAN_POINT ( 'NONE',  ( -14.34966873604972548, 8.224510206698743886, 58.33442372801901143 ) ) ;
#70686=CARTESIAN_POINT ( 'NONE',  ( -16.55341960407611168, -4.379528057220339221, 56.45724293864768839 ) ) ;
#70687=CARTESIAN_POINT ( 'NONE',  ( 15.72974639402199770, -15.80617190586745480, 88.12390960531436690 ) ) ;
#70688=CARTESIAN_POINT ( 'NONE',  ( -18.62759615963270932, 10.81492255796079327, 70.83224293864770971 ) ) ;
#70690=CARTESIAN_POINT ( 'NONE',  ( -0.05219959533936034679, 19.03943276465977164, 87.50109039468567573 ) ) ;
#70691=CARTESIAN_POINT ( 'NONE',  ( 15.80617190586746368, 15.72974639402197994, 24.37390960531435979 ) ) ;
#70692=CARTESIAN_POINT ( 'NONE',  ( -5.049401038298153566, 19.05341960407611168, 65.20724293864765286 ) ) ;
#70693=CARTESIAN_POINT ( 'NONE',  ( -16.51473224551069308, -9.474510206698971260, 36.66557627198102409 ) ) ;
#70695=CARTESIAN_POINT ( 'NONE',  ( -8.314922557961024197, 14.29746914071037800, 87.91775706135234714 ) ) ;
#70696=CARTESIAN_POINT ( 'NONE',  ( 0.05219959533937995610, -21.53943276465977519, 25.00109039468567218 ) ) ;
#70697=CARTESIAN_POINT ( 'NONE',  ( -9.564922557960796823, -16.46253265017161027, 67.08224293864769550 ) ) ;
#70698=CARTESIAN_POINT ( 'NONE',  ( -18.67979575497193778, 10.72451020669871902, 53.33442372801901854 ) ) ;
#70699=CARTESIAN_POINT ( 'NONE',  ( -5.049401038298153566, 19.05341960407611168, 90.20724293864766707 ) ) ;
#70702=CARTESIAN_POINT ( 'NONE',  ( -21.52544592524334988, -5.823673210054445271, 43.95942372801902565 ) ) ;
#70703=CARTESIAN_POINT ( 'NONE',  ( -19.05341960407611168, -5.049401038298163336, 26.45724293864769550 ) ) ;
#70704=CARTESIAN_POINT ( 'NONE',  ( -9.564922557960796823, -16.46253265017161027, 107.0822429386476955 ) ) ;
#70705=CARTESIAN_POINT ( 'NONE',  ( -0.05219959533936034679, 19.03943276465977164, 47.50109039468566863 ) ) ;
#70706=CARTESIAN_POINT ( 'NONE',  ( -15.80617190586745835, -15.72974639402198527, 106.8739096053143811 ) ) ;
#70707=CARTESIAN_POINT ( 'NONE',  ( -19.05341960407617563, 5.049401038297882671, 48.54275706135233293 ) ) ;
#70708=CARTESIAN_POINT ( 'NONE',  ( 16.51473224551083163, -9.474510206698727899, 45.83442372801900433 ) ) ;
#70709=CARTESIAN_POINT ( 'NONE',  ( 16.53943276465976808, 0.05219959533934440121, 111.2510903946856899 ) ) ;
#70711=ORIENTED_EDGE ( 'NONE', *, *, #44529, .T. ) ;
#70712=CARTESIAN_POINT ( 'NONE',  ( -19.02544592524342804, 5.153800228976336051, 76.04057627198102409 ) ) ;
#70713=CARTESIAN_POINT ( 'NONE',  ( 5.719274019375673035, 21.55341960407619339, 82.29275706135234714 ) ) ;
#70714=CARTESIAN_POINT ( 'NONE',  ( -5.719274019375665041, -21.55341960407619695, 94.79275706135234714 ) ) ;
#70716=CARTESIAN_POINT ( 'NONE',  ( -16.51473224551069308, -9.474510206698971260, 96.66557627198102409 ) ) ;
#70717=CARTESIAN_POINT ( 'NONE',  ( -21.53943276465977519, -0.05219959533937600094, 73.75109039468567573 ) ) ;
#70718=CARTESIAN_POINT ( 'NONE',  ( -8.224510206698735004, -14.34966873604973081, 19.58442372801901143 ) ) ;
#70719=CARTESIAN_POINT ( 'NONE',  ( 9.474510206698971260, -16.51473224551069308, 77.91557627198103830 ) ) ;
#70720=CARTESIAN_POINT ( 'NONE',  ( 0.05219959533909260263, 19.03943276465977164, 114.9989096053143669 ) ) ;
#70722=CARTESIAN_POINT ( 'NONE',  ( 19.03943276465977164, -0.05219959533909143690, 88.74890960531436690 ) ) ;
#70724=CARTESIAN_POINT ( 'NONE',  ( 9.564922557960805705, 16.46253265017160317, 84.58224293864769550 ) ) ;
#70725=CARTESIAN_POINT ( 'NONE',  ( 16.46253265017160672, -9.564922557960803928, 63.33224293864769550 ) ) ;
#70726=CARTESIAN_POINT ( 'NONE',  ( -10.81492255796078084, -18.62759615963271287, 107.0822429386476955 ) ) ;
#70727=CARTESIAN_POINT ( 'NONE',  ( 12.14591786802327356, -12.06949235617739191, 105.6260903946856899 ) ) ;
#70729=CARTESIAN_POINT ( 'NONE',  ( 19.03943276465977164, 0.05219959533936151252, 56.25109039468566863 ) ) ;
#70730=CARTESIAN_POINT ( 'NONE',  ( 16.51473224551069308, 9.474510206698969483, 94.16557627198103830 ) ) ;
#70731=CARTESIAN_POINT ( 'NONE',  ( 4.379528057220339221, -16.55341960407611168, 87.70724293864769550 ) ) ;
#70732=CARTESIAN_POINT ( 'NONE',  ( 9.564922557960805705, 16.46253265017160317, 24.58224293864769194 ) ) ;
#70733=CARTESIAN_POINT ( 'NONE',  ( -15.80617190586745835, -15.72974639402198527, 31.87390960531435979 ) ) ;
#70734=CARTESIAN_POINT ( 'NONE',  ( 21.52544592524344225, -5.823673210054117533, 23.54057627198102765 ) ) ;
#70735=CARTESIAN_POINT ( 'NONE',  ( 16.53943276465976808, -0.05219959533910856209, 98.74890960531438111 ) ) ;
#70737=CARTESIAN_POINT ( 'NONE',  ( -19.02544592524334988, -5.153800228976617603, 38.95942372801900433 ) ) ;
#70738=CARTESIAN_POINT ( 'NONE',  ( -4.483927247898782831, 16.52544592524335698, 107.7094237280190328 ) ) ;
#70739=CARTESIAN_POINT ( 'NONE',  ( 5.049401038298161559, -19.05341960407611168, 82.70724293864770971 ) ) ;
#70740=CARTESIAN_POINT ( 'NONE',  ( -18.62759615963255300, -10.81492255796106328, 69.16775706135234714 ) ) ;
#70741=CARTESIAN_POINT ( 'NONE',  ( 21.52544592524344225, -5.823673210054117533, 43.54057627198103830 ) ) ;
#70742=CARTESIAN_POINT ( 'NONE',  ( -5.719274019375665041, -21.55341960407619695, 34.79275706135235424 ) ) ;
#70743=CARTESIAN_POINT ( 'NONE',  ( -18.67979575497178146, -10.72451020669898902, 86.66557627198102409 ) ) ;
#70744=CARTESIAN_POINT ( 'NONE',  ( -4.379528057220328563, 16.55341960407611168, 105.2072429386477097 ) ) ;
#70745=CARTESIAN_POINT ( 'NONE',  ( -0.05219959533936034679, 19.03943276465977164, 67.50109039468566152 ) ) ;
#70746=CARTESIAN_POINT ( 'NONE',  ( -16.46253265017160317, 9.564922557960807481, 50.83224293864770260 ) ) ;
#70747=CARTESIAN_POINT ( 'NONE',  ( 19.02544592524343514, -5.153800228976328945, 98.54057627198100988 ) ) ;
#70748=CARTESIAN_POINT ( 'NONE',  ( -5.153800228976328057, -19.02544592524343514, 97.29057627198099567 ) ) ;
#70749=CARTESIAN_POINT ( 'NONE',  ( 16.52544592524342804, -4.483927247898539470, 113.5405762719810383 ) ) ;
#70750=CARTESIAN_POINT ( 'NONE',  ( -14.29746914071049879, 8.314922557960819915, 45.83224293864769550 ) ) ;
#70751=CARTESIAN_POINT ( 'NONE',  ( -0.05219959533934338120, 16.53943276465976808, 37.50109039468568284 ) ) ;
#70752=CARTESIAN_POINT ( 'NONE',  ( 10.81492255796106328, -18.62759615963255655, 105.4177570613523613 ) ) ;
#70753=SPHERICAL_SURFACE ( 'NONE', #175277, 2.000000000000000000 ) ;
#70754=CARTESIAN_POINT ( 'NONE',  ( 14.29746914071049879, -8.314922557960816363, 23.33224293864769194 ) ) ;
#70755=CARTESIAN_POINT ( 'NONE',  ( 18.62759615963255655, 10.81492255796105972, 26.66775706135235424 ) ) ;
#70756=CARTESIAN_POINT ( 'NONE',  ( 16.51473224551069308, 9.474510206698969483, 104.1655762719810241 ) ) ;
#70757=CARTESIAN_POINT ( 'NONE',  ( 16.55341960407618274, -4.379528057220086978, 111.0427570613523613 ) ) ;
#70758=CARTESIAN_POINT ( 'NONE',  ( -16.55341960407617563, 4.379528057220093196, 93.54275706135234714 ) ) ;
#70759=CARTESIAN_POINT ( 'NONE',  ( 12.14591786802327356, -12.06949235617739191, 30.62609039468567929 ) ) ;
#70760=CARTESIAN_POINT ( 'NONE',  ( -13.89961937509977652, 13.97604488694528158, 45.62390960531433848 ) ) ;
#70761=CARTESIAN_POINT ( 'NONE',  ( -12.06949235617756955, 12.14591786802309770, 105.6239096053143669 ) ) ;
#70762=CARTESIAN_POINT ( 'NONE',  ( -18.62759615963270932, 10.81492255796079327, 115.8322429386477097 ) ) ;
#70763=CARTESIAN_POINT ( 'NONE',  ( -5.049401038298153566, 19.05341960407611168, 35.20724293864768839 ) ) ;
#70764=CARTESIAN_POINT ( 'NONE',  ( -19.05341960407611168, -5.049401038298163336, 111.4572429386476671 ) ) ;
#70765=CARTESIAN_POINT ( 'NONE',  ( 21.53943276465977519, 0.05219959533937863772, 26.25109039468567573 ) ) ;
#70766=CARTESIAN_POINT ( 'NONE',  ( 13.97604488694527802, 13.89961937509977652, 34.37390960531436690 ) ) ;
#70767=CARTESIAN_POINT ( 'NONE',  ( -19.02544592524342804, 5.153800228976336051, 106.0405762719810241 ) ) ;
#70769=CARTESIAN_POINT ( 'NONE',  ( -5.049401038298153566, 19.05341960407611168, 100.2072429386476955 ) ) ;
#70770=CARTESIAN_POINT ( 'NONE',  ( 10.81492255796106328, -18.62759615963255655, 45.41775706135234003 ) ) ;
#70771=CARTESIAN_POINT ( 'NONE',  ( 12.14591786802309770, 12.06949235617756955, 89.37390960531435269 ) ) ;
#70772=CARTESIAN_POINT ( 'NONE',  ( 16.51473224551069308, 9.474510206698969483, 94.16557627198103830 ) ) ;
#70774=CARTESIAN_POINT ( 'NONE',  ( -14.34966873604972548, 8.224510206698743886, 68.33442372801900433 ) ) ;
#70775=CARTESIAN_POINT ( 'NONE',  ( -21.55341960407619339, 5.719274019375674811, 83.54275706135234714 ) ) ;
#70776=CARTESIAN_POINT ( 'NONE',  ( 16.53943276465976808, 0.05219959533934440121, 36.25109039468567573 ) ) ;
#70777=CARTESIAN_POINT ( 'NONE',  ( 5.049401038298161559, -19.05341960407611168, 77.70724293864765286 ) ) ;
#70779=CARTESIAN_POINT ( 'NONE',  ( 19.02544592524334988, 5.153800228976608722, 106.4594237280190185 ) ) ;
#70780=CARTESIAN_POINT ( 'NONE',  ( 14.34966873604972726, -8.224510206698740333, 75.83442372801900433 ) ) ;
#70781=CARTESIAN_POINT ( 'NONE',  ( 19.03943276465977164, 0.05219959533936151252, 91.25109039468566152 ) ) ;
#70782=CARTESIAN_POINT ( 'NONE',  ( -9.474510206698964154, 16.51473224551069663, 65.41557627198102409 ) ) ;
#70783=CARTESIAN_POINT ( 'NONE',  ( 10.81492255796078972, 18.62759615963270932, 89.58224293864768129 ) ) ;
#70784=CARTESIAN_POINT ( 'NONE',  ( -16.53943276465976808, 0.05219959533911058130, 96.24890960531435269 ) ) ;
#70785=CARTESIAN_POINT ( 'NONE',  ( -16.51473224551082808, 9.474510206698731452, 88.33442372801900433 ) ) ;
#70786=CARTESIAN_POINT ( 'NONE',  ( -16.53943276465976808, -0.05219959533934237506, 53.75109039468568994 ) ) ;
#70788=CARTESIAN_POINT ( 'NONE',  ( -13.97604488694547697, 13.89961937509957934, 63.12609039468566152 ) ) ;
#70789=CARTESIAN_POINT ( 'NONE',  ( -12.14591786802309592, -12.06949235617757132, 36.87390960531435979 ) ) ;
#70790=CARTESIAN_POINT ( 'NONE',  ( 12.14591786802309770, 12.06949235617756955, 74.37390960531436690 ) ) ;
#70791=CARTESIAN_POINT ( 'NONE',  ( 19.03943276465977164, 0.05219959533936151252, 26.25109039468566507 ) ) ;
#70792=CARTESIAN_POINT ( 'NONE',  ( -16.61371651742640410, 7.165104196375922108, 38.85415069992971127 ) ) ;
#70793=CARTESIAN_POINT ( 'NONE',  ( 21.52544592524334988, 5.823673210054432836, 21.45942372801901499 ) ) ;
#70795=CARTESIAN_POINT ( 'NONE',  ( -9.564922557960796823, -16.46253265017161027, 77.08224293864769550 ) ) ;
#70796=CARTESIAN_POINT ( 'NONE',  ( 21.52544592524334988, 5.823673210054432836, 96.45942372801901854 ) ) ;
#70797=CARTESIAN_POINT ( 'NONE',  ( -9.564922557960796823, -16.46253265017161027, 77.08224293864769550 ) ) ;
#70798=CARTESIAN_POINT ( 'NONE',  ( 10.81492255796078972, 18.62759615963270932, 44.58224293864769550 ) ) ;
#70799=CARTESIAN_POINT ( 'NONE',  ( -14.34966873604960291, -8.224510206698953496, 81.66557627198103830 ) ) ;
#70800=CARTESIAN_POINT ( 'NONE',  ( -19.02544592524342804, 5.153800228976336051, 61.04057627198103120 ) ) ;
#70801=CARTESIAN_POINT ( 'NONE',  ( -8.314922557960811034, -14.29746914071050412, 112.0822429386477097 ) ) ;
#70802=CARTESIAN_POINT ( 'NONE',  ( 5.823673210054444382, -21.52544592524334988, 20.20942372801900788 ) ) ;
#70803=CARTESIAN_POINT ( 'NONE',  ( -5.719274019375665041, -21.55341960407619695, 64.79275706135234714 ) ) ;
#70804=CARTESIAN_POINT ( 'NONE',  ( -13.97604488694527625, -13.89961937509977652, 46.87390960531435979 ) ) ;
#70805=CARTESIAN_POINT ( 'NONE',  ( -8.224510206698735004, -14.34966873604973081, 69.58442372801900433 ) ) ;
#70807=CARTESIAN_POINT ( 'NONE',  ( -18.62759615963270932, 10.81492255796079327, 115.8322429386477097 ) ) ;
#70808=CARTESIAN_POINT ( 'NONE',  ( 21.52544592524344225, -5.823673210054117533, 108.5405762719810241 ) ) ;
#70809=CARTESIAN_POINT ( 'NONE',  ( -13.97604488694547697, 13.89961937509957934, 33.12609039468566863 ) ) ;
#70810=CARTESIAN_POINT ( 'NONE',  ( 16.51473224551069308, 9.474510206698969483, 59.16557627198102409 ) ) ;
#70812=CARTESIAN_POINT ( 'NONE',  ( 15.80617190586769283, -15.72974639402175789, 65.62609039468568994 ) ) ;
#70813=CARTESIAN_POINT ( 'NONE',  ( 18.62759615963271287, -10.81492255796078972, 53.33224293864769550 ) ) ;
#70814=CARTESIAN_POINT ( 'NONE',  ( 8.314922557960818139, 14.29746914071049879, 39.58224293864769550 ) ) ;
#70815=CARTESIAN_POINT ( 'NONE',  ( -5.719274019375665041, -21.55341960407619695, 74.79275706135234714 ) ) ;
#70816=CARTESIAN_POINT ( 'NONE',  ( 10.81492255796106328, -18.62759615963255655, 110.4177570613523756 ) ) ;
#70817=CARTESIAN_POINT ( 'NONE',  ( 16.55341960407611168, 4.379528057220329451, 58.95724293864770971 ) ) ;
#70818=CARTESIAN_POINT ( 'NONE',  ( 12.14591786802309770, 12.06949235617756955, 99.37390960531436690 ) ) ;
#70819=CARTESIAN_POINT ( 'NONE',  ( -16.51473224551082808, 9.474510206698731452, 58.33442372801900433 ) ) ;
#70820=CARTESIAN_POINT ( 'NONE',  ( 12.06949235617757843, -12.14591786802309237, 28.12390960531435979 ) ) ;
#70821=CARTESIAN_POINT ( 'NONE',  ( -18.62759615963255300, -10.81492255796106328, 69.16775706135234714 ) ) ;
#70822=CARTESIAN_POINT ( 'NONE',  ( 13.89961937509977652, -13.97604488694527269, 78.12390960531433848 ) ) ;
#70823=CARTESIAN_POINT ( 'NONE',  ( 5.153800228976615827, -19.02544592524334988, 35.20942372801899722 ) ) ;
#70824=CARTESIAN_POINT ( 'NONE',  ( -18.62759615963270932, 10.81492255796079327, 40.83224293864769550 ) ) ;
#70825=CARTESIAN_POINT ( 'NONE',  ( 21.52544592524334988, 5.823673210054432836, 36.45942372801901143 ) ) ;
#70827=CARTESIAN_POINT ( 'NONE',  ( -5.823673210054116645, -21.52544592524344225, 87.29057627198103830 ) ) ;
#70828=CARTESIAN_POINT ( 'NONE',  ( -13.89961937509957401, -13.97604488694547875, 104.3760903946856757 ) ) ;
#70829=CARTESIAN_POINT ( 'NONE',  ( 14.29746914071037800, 8.314922557961029526, 56.66775706135235424 ) ) ;
#70831=CARTESIAN_POINT ( 'NONE',  ( -15.72974639402197994, 15.80617190586746368, 90.62390960531436690 ) ) ;
#70832=CARTESIAN_POINT ( 'NONE',  ( 8.314922557960818139, 14.29746914071049879, 84.58224293864769550 ) ) ;
#70833=CARTESIAN_POINT ( 'NONE',  ( -17.26058549869091507, -6.457015423128549259, 101.3774583747607210 ) ) ;
#70834=CARTESIAN_POINT ( 'NONE',  ( 9.474510206698729675, 16.51473224551082808, 112.0844237280190043 ) ) ;
#70835=CARTESIAN_POINT ( 'NONE',  ( -18.67979575497178146, -10.72451020669898902, 51.66557627198102409 ) ) ;
#70836=CARTESIAN_POINT ( 'NONE',  ( 12.14591786802327356, -12.06949235617739191, 90.62609039468567573 ) ) ;
#70837=DIRECTION ( 'NONE',  ( -1.000000000000000000, 0.000000000000000000, 0.000000000000000000 ) ) ;
#70838=CARTESIAN_POINT ( 'NONE',  ( -0.05219959533934338120, 16.53943276465976808, 47.50109039468568994 ) ) ;
#70839=CARTESIAN_POINT ( 'NONE',  ( -18.62759615963255300, -10.81492255796106328, 29.16775706135234003 ) ) ;
#70840=CARTESIAN_POINT ( 'NONE',  ( -15.80617190586745835, -15.72974639402198527, 41.87390960531435979 ) ) ;
#70841=CARTESIAN_POINT ( 'NONE',  ( 8.224510206698742110, 14.34966873604972548, 87.08442372801901854 ) ) ;
#70842=CARTESIAN_POINT ( 'NONE',  ( -9.474510206698964154, 16.51473224551069663, 95.41557627198102409 ) ) ;
#70843=CARTESIAN_POINT ( 'NONE',  ( 0.05219959533937995610, -21.53943276465977519, 75.00109039468568994 ) ) ;
#70844=CARTESIAN_POINT ( 'NONE',  ( -21.55341960407610458, -5.719274019375992779, 36.45724293864768839 ) ) ;
#70845=CARTESIAN_POINT ( 'NONE',  ( 16.46253265017160672, -9.564922557960803928, 113.3322429386476955 ) ) ;
#70846=CARTESIAN_POINT ( 'NONE',  ( -19.02544592524334988, -5.153800228976617603, 53.95942372801898301 ) ) ;
#70847=CARTESIAN_POINT ( 'NONE',  ( 14.34966873604972726, -8.224510206698740333, 70.83442372801901854 ) ) ;
#70848=CARTESIAN_POINT ( 'NONE',  ( 15.72974639402199770, -15.80617190586745480, 23.12390960531436335 ) ) ;
#70850=CARTESIAN_POINT ( 'NONE',  ( -16.51473224551069308, -9.474510206698971260, 86.66557627198102409 ) ) ;
#70851=CARTESIAN_POINT ( 'NONE',  ( -12.14591786802326823, 12.06949235617739902, 103.1260903946856757 ) ) ;
#70852=CARTESIAN_POINT ( 'NONE',  ( -17.97058386085788229, -5.499999999999976019, 79.00390968646219392 ) ) ;
#70853=CARTESIAN_POINT ( 'NONE',  ( -16.53943276465976808, 0.05219959533911058130, 91.24890960531436690 ) ) ;
#70854=CARTESIAN_POINT ( 'NONE',  ( 21.53943276465977519, -0.05219959533907433946, 43.74890960531435979 ) ) ;
#70855=CARTESIAN_POINT ( 'NONE',  ( -19.05341960407611168, -5.049401038298163336, 36.45724293864766707 ) ) ;
#70856=CARTESIAN_POINT ( 'NONE',  ( -14.34966873604972548, 8.224510206698743886, 83.33442372801903275 ) ) ;
#70857=CARTESIAN_POINT ( 'NONE',  ( 15.80617190586769283, -15.72974639402175789, 35.62609039468568994 ) ) ;
#70858=CARTESIAN_POINT ( 'NONE',  ( 9.564922557961047289, -16.46253265017146816, 95.41775706135233293 ) ) ;
#70859=CARTESIAN_POINT ( 'NONE',  ( 4.379528057220339221, -16.55341960407611168, 87.70724293864769550 ) ) ;
#70860=CARTESIAN_POINT ( 'NONE',  ( 5.153800228976335163, 19.02544592524342804, 54.79057627198103120 ) ) ;
#70862=CARTESIAN_POINT ( 'NONE',  ( 19.02544592524343514, -5.153800228976328945, 23.54057627198102054 ) ) ;
#70863=CARTESIAN_POINT ( 'NONE',  ( 10.81492255796106328, -18.62759615963255655, 105.4177570613523613 ) ) ;
#70864=CARTESIAN_POINT ( 'NONE',  ( 13.89961937509977652, -13.97604488694527269, 83.12390960531436690 ) ) ;
#70865=CARTESIAN_POINT ( 'NONE',  ( -14.29746914071037622, -8.314922557961029526, 59.16775706135234714 ) ) ;
#70866=CARTESIAN_POINT ( 'NONE',  ( -10.72451020669870658, -18.67979575497194134, 94.58442372801901854 ) ) ;
#70867=CARTESIAN_POINT ( 'NONE',  ( 8.224510206698742110, 14.34966873604972548, 77.08442372801901854 ) ) ;
#70868=CARTESIAN_POINT ( 'NONE',  ( 5.153800228976615827, -19.02544592524334988, 55.20942372801899722 ) ) ;
#70869=CARTESIAN_POINT ( 'NONE',  ( 0.05219959533936267826, -19.03943276465977164, 65.00109039468567573 ) ) ;
#70871=CARTESIAN_POINT ( 'NONE',  ( 0.05219959533937995610, -21.53943276465977519, 65.00109039468568994 ) ) ;
#70872=CARTESIAN_POINT ( 'NONE',  ( 19.02544592524343514, -5.153800228976328945, 63.54057627198103830 ) ) ;
#70873=CARTESIAN_POINT ( 'NONE',  ( -13.97604488694527625, -13.89961937509977652, 26.87390960531434558 ) ) ;
#70874=CARTESIAN_POINT ( 'NONE',  ( -16.46253265017146816, -9.564922557961047289, 59.16775706135233293 ) ) ;
#70876=CARTESIAN_POINT ( 'NONE',  ( -9.564922557960796823, -16.46253265017161027, 87.08224293864769550 ) ) ;
#70877=CARTESIAN_POINT ( 'NONE',  ( -16.53943276465976808, 0.05219959533911058130, 36.24890960531435979 ) ) ;
#70878=CARTESIAN_POINT ( 'NONE',  ( -0.05219959533907301413, -21.53943276465977519, 47.49890960531435979 ) ) ;
#70880=CARTESIAN_POINT ( 'NONE',  ( -15.80617190586768217, 15.72974639402176855, 108.1260903946856757 ) ) ;
#70881=CARTESIAN_POINT ( 'NONE',  ( -16.29526858892875296, -7.335722546920122156, 80.79670597800208043 ) ) ;
#70882=CARTESIAN_POINT ( 'NONE',  ( -16.51473224551069308, -9.474510206698971260, 31.66557627198102054 ) ) ;
#70883=CARTESIAN_POINT ( 'NONE',  ( 16.51473224551069308, 9.474510206698969483, 24.16557627198102765 ) ) ;
#70885=CARTESIAN_POINT ( 'NONE',  ( -5.719274019375665041, -21.55341960407619695, 69.79275706135234714 ) ) ;
#70887=CARTESIAN_POINT ( 'NONE',  ( -8.314922557961024197, 14.29746914071037800, 62.91775706135236135 ) ) ;
#70888=CARTESIAN_POINT ( 'NONE',  ( -15.72974639402197994, 15.80617190586746368, 85.62390960531436690 ) ) ;
#70889=CARTESIAN_POINT ( 'NONE',  ( 4.379528057220339221, -16.55341960407611168, 57.70724293864770260 ) ) ;
#70890=CARTESIAN_POINT ( 'NONE',  ( 16.51473224551069308, 9.474510206698969483, 34.16557627198102409 ) ) ;
#70891=CARTESIAN_POINT ( 'NONE',  ( 0.05219959533909260263, 19.03943276465977164, 114.9989096053143669 ) ) ;
#70892=CARTESIAN_POINT ( 'NONE',  ( -15.72974639402176322, -15.80617190586768395, 39.37609039468567573 ) ) ;
#70893=CARTESIAN_POINT ( 'NONE',  ( -13.89961937509957401, -13.97604488694547875, 44.37609039468566863 ) ) ;
#70894=CARTESIAN_POINT ( 'NONE',  ( 13.89961937509977652, -13.97604488694527269, 28.12390960531435624 ) ) ;
#70895=CARTESIAN_POINT ( 'NONE',  ( 18.67979575497194134, -10.72451020669871369, 85.83442372801901854 ) ) ;
#70896=CARTESIAN_POINT ( 'NONE',  ( -5.153800228976328057, -19.02544592524343514, 22.29057627198102765 ) ) ;
#70897=CARTESIAN_POINT ( 'NONE',  ( 12.06949235617757843, -12.14591786802309237, 38.12390960531436690 ) ) ;
#70899=CARTESIAN_POINT ( 'NONE',  ( -10.72451020669898014, 18.67979575497178502, 45.41557627198103830 ) ) ;
#70901=CARTESIAN_POINT ( 'NONE',  ( 0.05219959533909260263, 19.03943276465977164, 94.99890960531436690 ) ) ;
#70902=CARTESIAN_POINT ( 'NONE',  ( 4.483927247898545687, 16.52544592524342804, 89.79057627198103830 ) ) ;
#70903=CARTESIAN_POINT ( 'NONE',  ( 12.14591786802327356, -12.06949235617739191, 30.62609039468567929 ) ) ;
#70904=CARTESIAN_POINT ( 'NONE',  ( -10.81492255796078084, -18.62759615963271287, 62.08224293864769550 ) ) ;
#70906=CARTESIAN_POINT ( 'NONE',  ( -13.97604488694527625, -13.89961937509977652, 36.87390960531436690 ) ) ;
#70907=CARTESIAN_POINT ( 'NONE',  ( 9.564922557960805705, 16.46253265017160317, 79.58224293864769550 ) ) ;
#70908=CARTESIAN_POINT ( 'NONE',  ( 18.67979575497178502, 10.72451020669898547, 94.16557627198103830 ) ) ;
#70909=CARTESIAN_POINT ( 'NONE',  ( -0.05219959533910754901, -16.53943276465976808, 27.49890960531435269 ) ) ;
#70910=CARTESIAN_POINT ( 'NONE',  ( 16.46253265017160672, -9.564922557960803928, 98.33224293864769550 ) ) ;
#70911=CARTESIAN_POINT ( 'NONE',  ( -13.89961937509957401, -13.97604488694547875, 84.37609039468567573 ) ) ;
#70912=CARTESIAN_POINT ( 'NONE',  ( -21.53943276465977519, -0.05219959533937600094, 108.7510903946857042 ) ) ;
#70913=CARTESIAN_POINT ( 'NONE',  ( 10.72451020669898902, -18.67979575497178502, 82.91557627198103830 ) ) ;
#70914=CARTESIAN_POINT ( 'NONE',  ( 21.52544592524344225, -5.823673210054117533, 33.54057627198102409 ) ) ;
#70915=CARTESIAN_POINT ( 'NONE',  ( -5.049401038298153566, 19.05341960407611168, 55.20724293864769550 ) ) ;
#70916=CARTESIAN_POINT ( 'NONE',  ( -8.314922557960811034, -14.29746914071050412, 27.08224293864769550 ) ) ;
#70917=CARTESIAN_POINT ( 'NONE',  ( 13.89961937509977652, -13.97604488694527269, 73.12390960531436690 ) ) ;
#70920=CARTESIAN_POINT ( 'NONE',  ( -9.474510206698720793, -16.51473224551083518, 29.58442372801900433 ) ) ;
#70921=CARTESIAN_POINT ( 'NONE',  ( 16.55341960407611168, 4.379528057220329451, 83.95724293864770971 ) ) ;
#70922=CARTESIAN_POINT ( 'NONE',  ( -10.72451020669870658, -18.67979575497194134, 19.58442372801901143 ) ) ;
#70924=CARTESIAN_POINT ( 'NONE',  ( 21.53943276465977519, -0.05219959533907433946, 53.74890960531437401 ) ) ;
#70925=CARTESIAN_POINT ( 'NONE',  ( -0.05219959533934338120, 16.53943276465976808, 87.50109039468568994 ) ) ;
#70926=CARTESIAN_POINT ( 'NONE',  ( -8.224510206698948167, 14.34966873604960824, 115.4155762719810241 ) ) ;
#70927=CARTESIAN_POINT ( 'NONE',  ( -5.049401038298153566, 19.05341960407611168, 70.20724293864769550 ) ) ;
#70929=CARTESIAN_POINT ( 'NONE',  ( 16.52544592524342804, -4.483927247898539470, 23.54057627198102765 ) ) ;
#70930=CARTESIAN_POINT ( 'NONE',  ( -21.52544592524334988, -5.823673210054445271, 63.95942372801901854 ) ) ;
#70931=CARTESIAN_POINT ( 'NONE',  ( 19.02544592524343514, -5.153800228976328945, 113.5405762719810241 ) ) ;
#70932=CARTESIAN_POINT ( 'NONE',  ( 10.81492255796106328, -18.62759615963255655, 95.41775706135234714 ) ) ;
#70933=CARTESIAN_POINT ( 'NONE',  ( -16.51473224551069308, -9.474510206698971260, 41.66557627198103120 ) ) ;
#70934=CARTESIAN_POINT ( 'NONE',  ( 13.89961937509977652, -13.97604488694527269, 48.12390960531435979 ) ) ;
#70936=CARTESIAN_POINT ( 'NONE',  ( 21.52544592524334988, 5.823673210054432836, 101.4594237280190185 ) ) ;
#70937=CARTESIAN_POINT ( 'NONE',  ( 12.14591786802327356, -12.06949235617739191, 65.62609039468568994 ) ) ;
#70938=CARTESIAN_POINT ( 'NONE',  ( -0.05219959533937732626, 21.53943276465977519, 82.50109039468568994 ) ) ;
#70939=CARTESIAN_POINT ( 'NONE',  ( -0.05219959533907301413, -21.53943276465977519, 27.49890960531435269 ) ) ;
#70940=CARTESIAN_POINT ( 'NONE',  ( -16.46253265017146816, -9.564922557961047289, 99.16775706135233293 ) ) ;
#70941=CARTESIAN_POINT ( 'NONE',  ( -18.62759615963255300, -10.81492255796106328, 49.16775706135234003 ) ) ;
#70942=CARTESIAN_POINT ( 'NONE',  ( 16.52544592524335698, 4.483927247898782831, 36.45942372801901143 ) ) ;
#70943=CARTESIAN_POINT ( 'NONE',  ( 19.02544592524334988, 5.153800228976608722, 81.45942372801897591 ) ) ;
#70944=CARTESIAN_POINT ( 'NONE',  ( -19.02544592524342804, 5.153800228976336051, 71.04057627198099567 ) ) ;
#70945=CARTESIAN_POINT ( 'NONE',  ( -16.46253265017146816, -9.564922557961047289, 99.16775706135233293 ) ) ;
#70946=CARTESIAN_POINT ( 'NONE',  ( 9.564922557961047289, -16.46253265017146816, 95.41775706135233293 ) ) ;
#70947=CARTESIAN_POINT ( 'NONE',  ( 8.314922557960818139, 14.29746914071049879, 54.58224293864769550 ) ) ;
#70948=CARTESIAN_POINT ( 'NONE',  ( -19.03943276465977164, -0.05219959533935918106, 73.75109039468566152 ) ) ;
#70949=CARTESIAN_POINT ( 'NONE',  ( -12.14591786802326823, 12.06949235617739902, 58.12609039468568994 ) ) ;
#70950=CARTESIAN_POINT ( 'NONE',  ( -19.03943276465977164, -0.05219959533935918106, 23.75109039468566152 ) ) ;
#70951=CARTESIAN_POINT ( 'NONE',  ( 5.153800228976335163, 19.02544592524342804, 34.79057627198102409 ) ) ;
#70952=CARTESIAN_POINT ( 'NONE',  ( -16.51473224551069308, -9.474510206698971260, 36.66557627198102409 ) ) ;
#70953=CARTESIAN_POINT ( 'NONE',  ( 14.34966873604972726, -8.224510206698740333, 60.83442372801901854 ) ) ;
#70955=EDGE_CURVE ( 'NONE', #40791, #53699, #125901, .T. ) ;
#70957=CARTESIAN_POINT ( 'NONE',  ( 5.049401038298161559, -19.05341960407611168, 102.7072429386476955 ) ) ;
#70958=CARTESIAN_POINT ( 'NONE',  ( -17.49999999999999645, 5.499999999999997335, 120.0000000000000142 ) ) ;
#70960=CARTESIAN_POINT ( 'NONE',  ( -16.46253265017146816, -9.564922557961047289, 104.1677570613523329 ) ) ;
#70962=CARTESIAN_POINT ( 'NONE',  ( 15.80617190586746368, 15.72974639402197994, 34.37390960531435979 ) ) ;
#70963=CARTESIAN_POINT ( 'NONE',  ( -9.474510206698720793, -16.51473224551083518, 29.58442372801900433 ) ) ;
#70964=CARTESIAN_POINT ( 'NONE',  ( -12.06949235617739369, -12.14591786802326823, 19.37609039468568639 ) ) ;
#70965=CARTESIAN_POINT ( 'NONE',  ( 13.97604488694527802, 13.89961937509977652, 29.37390960531435979 ) ) ;
#70966=CARTESIAN_POINT ( 'NONE',  ( -13.97604488694527625, -13.89961937509977652, 56.87390960531434558 ) ) ;
#70967=CARTESIAN_POINT ( 'NONE',  ( -21.53943276465977519, 0.05219959533907696930, 76.24890960531435269 ) ) ;
#70968=CARTESIAN_POINT ( 'NONE',  ( 5.049401038298161559, -19.05341960407611168, 102.7072429386476955 ) ) ;
#70969=CARTESIAN_POINT ( 'NONE',  ( -9.474510206698964154, 16.51473224551069663, 35.41557627198102409 ) ) ;
#70971=CARTESIAN_POINT ( 'NONE',  ( 16.51473224551083163, -9.474510206698727899, 85.83442372801900433 ) ) ;
#70972=CARTESIAN_POINT ( 'NONE',  ( 16.52544592524342804, -4.483927247898539470, 48.54057627198103120 ) ) ;
#70973=CARTESIAN_POINT ( 'NONE',  ( 5.719274019375991003, -21.55341960407610458, 27.70724293864769905 ) ) ;
#70974=CARTESIAN_POINT ( 'NONE',  ( -15.72974639402176322, -15.80617190586768395, 104.3760903946856899 ) ) ;
#70975=CARTESIAN_POINT ( 'NONE',  ( -18.62759615963270932, 10.81492255796079327, 100.8322429386477097 ) ) ;
#70976=CARTESIAN_POINT ( 'NONE',  ( -21.55341960407619339, 5.719274019375674811, 68.54275706135234714 ) ) ;
#70977=CARTESIAN_POINT ( 'NONE',  ( -0.05219959533937732626, 21.53943276465977519, 77.50109039468567573 ) ) ;
#70978=CARTESIAN_POINT ( 'NONE',  ( -19.05341960407611168, -5.049401038298163336, 106.4572429386476955 ) ) ;
#70979=CARTESIAN_POINT ( 'NONE',  ( 16.52544592524335698, 4.483927247898782831, 111.4594237280190328 ) ) ;
#70980=CARTESIAN_POINT ( 'NONE',  ( -0.05219959533937732626, 21.53943276465977519, 62.50109039468568284 ) ) ;
#70981=CARTESIAN_POINT ( 'NONE',  ( -13.97604488694527625, -13.89961937509977652, 56.87390960531434558 ) ) ;
#70982=CARTESIAN_POINT ( 'NONE',  ( 0.05219959533936267826, -19.03943276465977164, 40.00109039468566152 ) ) ;
#70983=CARTESIAN_POINT ( 'NONE',  ( 5.823673210054444382, -21.52544592524334988, 30.20942372801902565 ) ) ;
#70984=CARTESIAN_POINT ( 'NONE',  ( -0.05219959533909027116, -19.03943276465977164, 72.49890960531435269 ) ) ;
#70985=CARTESIAN_POINT ( 'NONE',  ( 4.379528057220339221, -16.55341960407611168, 77.70724293864770971 ) ) ;
#70986=CARTESIAN_POINT ( 'NONE',  ( 0.05219959533910956823, 16.53943276465976808, 49.99890960531437401 ) ) ;
#70987=CARTESIAN_POINT ( 'NONE',  ( -5.719274019375978568, 21.55341960407610458, 60.20724293864768839 ) ) ;
#70988=CARTESIAN_POINT ( 'NONE',  ( 9.474510206698971260, -16.51473224551069308, 57.91557627198103120 ) ) ;
#70989=CARTESIAN_POINT ( 'NONE',  ( 15.72974639402199770, -15.80617190586745480, 78.12390960531436690 ) ) ;
#70990=CARTESIAN_POINT ( 'NONE',  ( 9.474510206698729675, 16.51473224551082808, 57.08442372801900433 ) ) ;
#70991=CARTESIAN_POINT ( 'NONE',  ( -19.02544592524335343, -5.153800228976618492, 18.95942372801899367 ) ) ;
#70992=CARTESIAN_POINT ( 'NONE',  ( 0.05219959533910956823, 16.53943276465976808, 59.99890960531436690 ) ) ;
#70993=CARTESIAN_POINT ( 'NONE',  ( -10.81492255796078084, -18.62759615963271287, 37.08224293864768129 ) ) ;
#70997=CARTESIAN_POINT ( 'NONE',  ( 16.55341960407618274, -4.379528057220086978, 81.04275706135236135 ) ) ;
#70999=CARTESIAN_POINT ( 'NONE',  ( -19.03943276465977164, -0.05219959533935918106, 88.75109039468567573 ) ) ;
#71000=CARTESIAN_POINT ( 'NONE',  ( 14.29746914071049879, -8.314922557960816363, 48.33224293864770260 ) ) ;
#71002=CARTESIAN_POINT ( 'NONE',  ( -16.51473224551069308, -9.474510206698971260, 46.66557627198102409 ) ) ;
#71003=CARTESIAN_POINT ( 'NONE',  ( -4.379528057220328563, 16.55341960407611168, 40.20724293864769550 ) ) ;
#71004=CARTESIAN_POINT ( 'NONE',  ( 16.51473224551069308, 9.474510206698969483, 94.16557627198103830 ) ) ;
#71005=CARTESIAN_POINT ( 'NONE',  ( 13.97604488694527802, 13.89961937509977652, 54.37390960531435979 ) ) ;
#71006=CARTESIAN_POINT ( 'NONE',  ( -15.80617190586768217, 15.72974639402176855, 58.12609039468568994 ) ) ;
#71007=CARTESIAN_POINT ( 'NONE',  ( -9.564922557960796823, -16.46253265017161027, 77.08224293864769550 ) ) ;
#71008=CARTESIAN_POINT ( 'NONE',  ( -19.02544592524342804, 5.153800228976336051, 31.04057627198102409 ) ) ;
#71009=CARTESIAN_POINT ( 'NONE',  ( 9.474510206698971260, -16.51473224551069308, 77.91557627198103830 ) ) ;
#71010=CARTESIAN_POINT ( 'NONE',  ( 5.823673210054125526, 21.52544592524343514, 49.79057627198102409 ) ) ;
#71011=CARTESIAN_POINT ( 'NONE',  ( -9.474510206698964154, 16.51473224551069663, 40.41557627198103120 ) ) ;
#71012=CARTESIAN_POINT ( 'NONE',  ( -18.67979575497178146, -10.72451020669898902, 36.66557627198103120 ) ) ;
#71013=CARTESIAN_POINT ( 'NONE',  ( 14.34966873604972726, -8.224510206698740333, 110.8344237280190043 ) ) ;
#71014=CARTESIAN_POINT ( 'NONE',  ( -0.05219959533936034679, 19.03943276465977164, 22.50109039468566152 ) ) ;
#71015=CARTESIAN_POINT ( 'NONE',  ( -4.379528057220086978, -16.55341960407618274, 44.79275706135234714 ) ) ;
#71016=CARTESIAN_POINT ( 'NONE',  ( 16.53943276465976808, 0.05219959533934440121, 81.25109039468568994 ) ) ;
#71018=CARTESIAN_POINT ( 'NONE',  ( 14.34966873604972726, -8.224510206698740333, 70.83442372801901854 ) ) ;
#71019=CARTESIAN_POINT ( 'NONE',  ( -18.67979575497178146, -10.72451020669898902, 31.66557627198102054 ) ) ;
#71020=CARTESIAN_POINT ( 'NONE',  ( -19.02544592524342804, 5.153800228976336051, 31.04057627198102409 ) ) ;
#71021=CARTESIAN_POINT ( 'NONE',  ( -14.29746914071037622, -8.314922557961029526, 44.16775706135234714 ) ) ;
#71022=CARTESIAN_POINT ( 'NONE',  ( -19.05341960407611168, -5.049401038298163336, 46.45724293864768129 ) ) ;
#71023=CARTESIAN_POINT ( 'NONE',  ( 15.80617190586769283, -15.72974639402175789, 45.62609039468567573 ) ) ;
#71024=CARTESIAN_POINT ( 'NONE',  ( 16.55341960407618274, -4.379528057220086978, 41.04275706135236135 ) ) ;
#71025=CARTESIAN_POINT ( 'NONE',  ( -0.05219959533934338120, 16.53943276465976808, 97.50109039468567573 ) ) ;
#71027=CARTESIAN_POINT ( 'NONE',  ( 21.55341960407619695, -5.719274019375665929, 96.04275706135236135 ) ) ;
#71028=CARTESIAN_POINT ( 'NONE',  ( -19.05341960407617563, 5.049401038297882671, 93.54275706135234714 ) ) ;
#71029=CARTESIAN_POINT ( 'NONE',  ( -13.89961937509957401, -13.97604488694547875, 49.37609039468567573 ) ) ;
#71030=CARTESIAN_POINT ( 'NONE',  ( -14.29746914071049879, 8.314922557960819915, 75.83224293864769550 ) ) ;
#71031=CARTESIAN_POINT ( 'NONE',  ( 13.97604488694527802, 13.89961937509977652, 24.37390960531435624 ) ) ;
#71032=CARTESIAN_POINT ( 'NONE',  ( -0.05219959533936034679, 19.03943276465977164, 62.50109039468566863 ) ) ;
#71033=CARTESIAN_POINT ( 'NONE',  ( 16.18388926212238133, 7.379444403734545688, 77.93953151366154941 ) ) ;
#71034=CARTESIAN_POINT ( 'NONE',  ( -0.05219959533937732626, 21.53943276465977519, 57.50109039468568994 ) ) ;
#71035=CARTESIAN_POINT ( 'NONE',  ( -8.224510206698735004, -14.34966873604973081, 29.58442372801901854 ) ) ;
#71037=CARTESIAN_POINT ( 'NONE',  ( 5.823673210054125526, 21.52544592524343514, 24.79057627198103120 ) ) ;
#71038=CARTESIAN_POINT ( 'NONE',  ( 5.049401038297881783, 19.05341960407617563, 102.2927570613523045 ) ) ;
#71039=CARTESIAN_POINT ( 'NONE',  ( -13.89961937509977652, 13.97604488694528158, 110.6239096053143243 ) ) ;
#71041=CARTESIAN_POINT ( 'NONE',  ( -4.379528057220328563, 16.55341960407611168, 115.2072429386476955 ) ) ;
#71042=CARTESIAN_POINT ( 'NONE',  ( 10.81492255796106328, -18.62759615963255655, 110.4177570613523756 ) ) ;
#71043=CARTESIAN_POINT ( 'NONE',  ( 19.05341960407611168, 5.049401038298154454, 58.95724293864768129 ) ) ;
#71044=CARTESIAN_POINT ( 'NONE',  ( -5.719274019375665041, -21.55341960407619695, 59.79275706135234714 ) ) ;
#71045=CARTESIAN_POINT ( 'NONE',  ( 5.719274019375673035, 21.55341960407619339, 107.2927570613523471 ) ) ;
#71046=CARTESIAN_POINT ( 'NONE',  ( -16.53943276465976808, -0.05219959533934237506, 98.75109039468568994 ) ) ;
#71048=CARTESIAN_POINT ( 'NONE',  ( -16.46253265017160317, 9.564922557960807481, 80.83224293864769550 ) ) ;
#71049=CARTESIAN_POINT ( 'NONE',  ( -21.52544592524334988, -5.823673210054445271, 53.95942372801900433 ) ) ;
#71050=CARTESIAN_POINT ( 'NONE',  ( -18.67979575497193778, 10.72451020669871902, 58.33442372801901143 ) ) ;
#71051=CARTESIAN_POINT ( 'NONE',  ( 0.05219959533936267826, -19.03943276465977164, 75.00109039468566152 ) ) ;
#71052=CARTESIAN_POINT ( 'NONE',  ( 19.03943276465977164, -0.05219959533909143690, 108.7489096053143527 ) ) ;
#71053=CARTESIAN_POINT ( 'NONE',  ( 16.51473224551069308, 9.474510206698969483, 24.16557627198102765 ) ) ;
#71054=CARTESIAN_POINT ( 'NONE',  ( 21.55341960407610458, 5.719274019375980345, 93.95724293864770971 ) ) ;
#71055=CARTESIAN_POINT ( 'NONE',  ( 5.049401038297881783, 19.05341960407617563, 27.29275706135232937 ) ) ;
#71056=CARTESIAN_POINT ( 'NONE',  ( 8.314922557960818139, 14.29746914071049879, 99.58224293864770971 ) ) ;
#71057=CARTESIAN_POINT ( 'NONE',  ( 0.05219959533909260263, 19.03943276465977164, 49.99890960531435979 ) ) ;
#71058=CARTESIAN_POINT ( 'NONE',  ( -13.97604488694547697, 13.89961937509957934, 103.1260903946856473 ) ) ;
#71059=CARTESIAN_POINT ( 'NONE',  ( -14.29746914071049879, 8.314922557960819915, 65.83224293864769550 ) ) ;
#71060=CARTESIAN_POINT ( 'NONE',  ( -18.62759615963255300, -10.81492255796106328, 109.1677570613523613 ) ) ;
#71061=CARTESIAN_POINT ( 'NONE',  ( 19.03943276465977164, -0.05219959533909143690, 98.74890960531436690 ) ) ;
#71062=CARTESIAN_POINT ( 'NONE',  ( -13.89961937509957401, -13.97604488694547875, 74.37609039468566152 ) ) ;
#71063=CARTESIAN_POINT ( 'NONE',  ( -0.05219959533907301413, -21.53943276465977519, 82.49890960531436690 ) ) ;
#71064=CARTESIAN_POINT ( 'NONE',  ( 15.80617190586769283, -15.72974639402175789, 40.62609039468567573 ) ) ;
#71065=CARTESIAN_POINT ( 'NONE',  ( -0.05219959533934338120, 16.53943276465976808, 42.50109039468567573 ) ) ;
#71066=CARTESIAN_POINT ( 'NONE',  ( -12.14591786802326823, 12.06949235617739902, 98.12609039468570415 ) ) ;
#71067=CARTESIAN_POINT ( 'NONE',  ( -4.483927247898782831, 16.52544592524335698, 37.70942372801900433 ) ) ;
#71068=CARTESIAN_POINT ( 'NONE',  ( 15.72974639402176855, 15.80617190586768217, 31.87609039468567929 ) ) ;
#71069=CARTESIAN_POINT ( 'NONE',  ( 21.55341960407610458, 5.719274019375980345, 43.95724293864769550 ) ) ;
#71070=CARTESIAN_POINT ( 'NONE',  ( -13.97604488694527625, -13.89961937509977652, 31.87390960531435979 ) ) ;
#71072=CARTESIAN_POINT ( 'NONE',  ( 16.55341960407618274, -4.379528057220086978, 56.04275706135235424 ) ) ;
#71073=CARTESIAN_POINT ( 'NONE',  ( 15.80617190586746368, 15.72974639402197994, 89.37390960531435269 ) ) ;
#71074=CARTESIAN_POINT ( 'NONE',  ( -16.55341960407611168, -4.379528057220339221, 36.45724293864768839 ) ) ;
#71075=CARTESIAN_POINT ( 'NONE',  ( -8.224510206698735004, -14.34966873604973081, 44.58442372801901854 ) ) ;
#71076=CARTESIAN_POINT ( 'NONE',  ( -19.05341960407611168, -5.049401038298163336, 56.45724293864768129 ) ) ;
#71077=CARTESIAN_POINT ( 'NONE',  ( -9.474510206698720793, -16.51473224551083518, 89.58442372801900433 ) ) ;
#71078=CARTESIAN_POINT ( 'NONE',  ( -5.719274019375978568, 21.55341960407610458, 85.20724293864770971 ) ) ;
#71079=CARTESIAN_POINT ( 'NONE',  ( -16.52544592524342804, 4.483927247898546575, 36.04057627198102409 ) ) ;
#71080=ORIENTED_EDGE ( 'NONE', *, *, #122412, .F. ) ;
#71082=CARTESIAN_POINT ( 'NONE',  ( 21.55341960407610458, 5.719274019375980345, 58.95724293864770971 ) ) ;
#71083=CARTESIAN_POINT ( 'NONE',  ( -16.55341960407617563, 4.379528057220093196, 108.5427570613523756 ) ) ;
#71085=CARTESIAN_POINT ( 'NONE',  ( 19.39056639909673763, 5.500000000000049738, 88.28948781074345220 ) ) ;
#71086=CARTESIAN_POINT ( 'NONE',  ( -0.05219959533907301413, -21.53943276465977519, 87.49890960531436690 ) ) ;
#71087=CARTESIAN_POINT ( 'NONE',  ( -12.06949235617756955, 12.14591786802309770, 25.62390960531435624 ) ) ;
#71088=CARTESIAN_POINT ( 'NONE',  ( -16.53943276465976808, -0.05219959533934237506, 38.75109039468567573 ) ) ;
#71089=CARTESIAN_POINT ( 'NONE',  ( -19.03943276465977164, 0.05219959533909376836, 41.24890960531435269 ) ) ;
#71090=CARTESIAN_POINT ( 'NONE',  ( 5.049401038298161559, -19.05341960407611168, 67.70724293864769550 ) ) ;
#71092=CARTESIAN_POINT ( 'NONE',  ( 18.62759615963271287, -10.81492255796078972, 28.33224293864769550 ) ) ;
#71094=CARTESIAN_POINT ( 'NONE',  ( 14.34966873604972726, -8.224510206698740333, 105.8344237280190328 ) ) ;
#71095=CARTESIAN_POINT ( 'NONE',  ( -16.46253265017146816, -9.564922557961047289, 109.1677570613523471 ) ) ;
#71096=CARTESIAN_POINT ( 'NONE',  ( 0.05219959533936267826, -19.03943276465977164, 40.00109039468566152 ) ) ;
#71097=CARTESIAN_POINT ( 'NONE',  ( -15.80617190586745835, -15.72974639402198527, 86.87390960531438111 ) ) ;
#71098=CARTESIAN_POINT ( 'NONE',  ( -0.05219959533910754901, -16.53943276465976808, 27.49890960531435269 ) ) ;
#71099=CARTESIAN_POINT ( 'NONE',  ( -15.80617190586745835, -15.72974639402198527, 51.87390960531437401 ) ) ;
#71100=CARTESIAN_POINT ( 'NONE',  ( -21.55341960407610458, -5.719274019375992779, 76.45724293864769550 ) ) ;
#71101=CARTESIAN_POINT ( 'NONE',  ( -19.02544592524334988, -5.153800228976617603, 103.9594237280190043 ) ) ;
#71102=CARTESIAN_POINT ( 'NONE',  ( 9.474510206698971260, -16.51473224551069308, 107.9155762719810383 ) ) ;
#71103=CARTESIAN_POINT ( 'NONE',  ( -18.62759615963255300, -10.81492255796106328, 69.16775706135234714 ) ) ;
#71104=CARTESIAN_POINT ( 'NONE',  ( 16.51473224551069308, 9.474510206698969483, 59.16557627198102409 ) ) ;
#71106=CARTESIAN_POINT ( 'NONE',  ( -16.55341960407611168, -4.379528057220339221, 96.45724293864770971 ) ) ;
#71108=CARTESIAN_POINT ( 'NONE',  ( -5.049401038298153566, 19.05341960407611168, 75.20724293864769550 ) ) ;
#71109=CARTESIAN_POINT ( 'NONE',  ( -16.52544592524342804, 4.483927247898546575, 96.04057627198102409 ) ) ;
#71110=ORIENTED_EDGE ( 'NONE', *, *, #80930, .T. ) ;
#71111=CARTESIAN_POINT ( 'NONE',  ( -19.02544592524334988, -5.153800228976617603, 88.95942372801897591 ) ) ;
#71112=CARTESIAN_POINT ( 'NONE',  ( 17.12812012977029852, -6.668231424565925991, 81.14051240676860743 ) ) ;
#71113=CARTESIAN_POINT ( 'NONE',  ( 13.97604488694527802, 13.89961937509977652, 54.37390960531435979 ) ) ;
#71115=CARTESIAN_POINT ( 'NONE',  ( 5.823673210054444382, -21.52544592524334988, 85.20942372801901854 ) ) ;
#71116=CARTESIAN_POINT ( 'NONE',  ( 5.153800228976335163, 19.02544592524342804, 94.79057627198103830 ) ) ;
#71117=CARTESIAN_POINT ( 'NONE',  ( -16.55341960407617563, 4.379528057220093196, 63.54275706135234003 ) ) ;
#71119=CARTESIAN_POINT ( 'NONE',  ( -19.05341960407617563, 5.049401038297882671, 43.54275706135232582 ) ) ;
#71120=CARTESIAN_POINT ( 'NONE',  ( 21.55341960407619695, -5.719274019375665929, 101.0427570613523756 ) ) ;
#71123=CARTESIAN_POINT ( 'NONE',  ( -8.314922557961024197, 14.29746914071037800, 97.91775706135236135 ) ) ;
#71125=CARTESIAN_POINT ( 'NONE',  ( -16.52544592524335698, -4.483927247898792601, 98.95942372801903275 ) ) ;
#71127=CARTESIAN_POINT ( 'NONE',  ( 8.224510206698742110, 14.34966873604972548, 62.08442372801901143 ) ) ;
#71129=CARTESIAN_POINT ( 'NONE',  ( -5.719274019375665041, -21.55341960407619695, 79.79275706135236135 ) ) ;
#71130=CARTESIAN_POINT ( 'NONE',  ( -19.03943276465977164, -0.05219959533935918106, 93.75109039468566152 ) ) ;
#71131=CARTESIAN_POINT ( 'NONE',  ( -5.153800228976607833, 19.02544592524334988, 32.70942372801899722 ) ) ;
#71132=CARTESIAN_POINT ( 'NONE',  ( -5.153800228976328057, -19.02544592524343514, 72.29057627198102409 ) ) ;
#71133=CARTESIAN_POINT ( 'NONE',  ( 0.05219959533909260263, 19.03943276465977164, 54.99890960531435979 ) ) ;
#71134=CARTESIAN_POINT ( 'NONE',  ( 16.30887417027163622, -7.330987202194335417, 22.64566514850552181 ) ) ;
#71135=CARTESIAN_POINT ( 'NONE',  ( 10.81492255796078972, 18.62759615963270932, 74.58224293864768129 ) ) ;
#71137=CARTESIAN_POINT ( 'NONE',  ( 0.05219959533907565091, 21.53943276465977519, 39.99890960531436690 ) ) ;
#71138=CARTESIAN_POINT ( 'NONE',  ( 9.564922557960805705, 16.46253265017160317, 29.58224293864769550 ) ) ;
#71139=CARTESIAN_POINT ( 'NONE',  ( 16.52544592524335698, 4.483927247898782831, 66.45942372801903275 ) ) ;
#71141=CARTESIAN_POINT ( 'NONE',  ( 18.67979575497194134, -10.72451020669871369, 25.83442372801901499 ) ) ;
#71142=CARTESIAN_POINT ( 'NONE',  ( -4.379528057220328563, 16.55341960407611168, 65.20724293864768129 ) ) ;
#71144=CARTESIAN_POINT ( 'NONE',  ( 12.06949235617739724, 12.14591786802326823, 26.87609039468567218 ) ) ;
#71145=CARTESIAN_POINT ( 'NONE',  ( -19.02544592524334988, -5.153800228976617603, 53.95942372801898301 ) ) ;
#71146=CARTESIAN_POINT ( 'NONE',  ( -12.14591786802309592, -12.06949235617757132, 51.87390960531437401 ) ) ;
#71147=CARTESIAN_POINT ( 'NONE',  ( 15.72974639402176855, 15.80617190586768217, 21.87609039468567573 ) ) ;
#71149=CARTESIAN_POINT ( 'NONE',  ( 10.72451020669898902, -18.67979575497178502, 72.91557627198103830 ) ) ;
#71150=CARTESIAN_POINT ( 'NONE',  ( -13.97604488694527625, -13.89961937509977652, 101.8739096053143811 ) ) ;
#71151=CARTESIAN_POINT ( 'NONE',  ( -14.29746914071049879, 8.314922557960819915, 65.83224293864769550 ) ) ;
#71152=CARTESIAN_POINT ( 'NONE',  ( -16.46253265017160317, 9.564922557960807481, 115.8322429386477097 ) ) ;
#71154=CARTESIAN_POINT ( 'NONE',  ( 19.02544592524334988, 5.153800228976608722, 66.45942372801899012 ) ) ;
#71155=CARTESIAN_POINT ( 'NONE',  ( 21.55341960407610458, 5.719274019375980345, 113.9572429386477239 ) ) ;
#71156=CARTESIAN_POINT ( 'NONE',  ( 19.03943276465977164, -0.05219959533909143690, 53.74890960531436690 ) ) ;
#71157=CARTESIAN_POINT ( 'NONE',  ( -16.51473224551082808, 9.474510206698731452, 48.33442372801900433 ) ) ;
#71158=CARTESIAN_POINT ( 'NONE',  ( 0.05219959533909260263, 19.03943276465977164, 34.99890960531435979 ) ) ;
#71159=CARTESIAN_POINT ( 'NONE',  ( 18.67979575497194134, -10.72451020669871369, 65.83442372801900433 ) ) ;
#71162=CARTESIAN_POINT ( 'NONE',  ( -12.14591786802309592, -12.06949235617757132, 36.87390960531435979 ) ) ;
#71163=CARTESIAN_POINT ( 'NONE',  ( 5.153800228976335163, 19.02544592524342804, 59.79057627198100988 ) ) ;
#71164=CARTESIAN_POINT ( 'NONE',  ( -10.81492255796078084, -18.62759615963271287, 72.08224293864769550 ) ) ;
#71165=CARTESIAN_POINT ( 'NONE',  ( -19.03943276465977164, 0.05219959533909376836, 61.24890960531436690 ) ) ;
#71167=CARTESIAN_POINT ( 'NONE',  ( -21.52544592524343514, 5.823673210054127303, 66.04057627198103830 ) ) ;
#71169=CARTESIAN_POINT ( 'NONE',  ( -0.05219959533937732626, 21.53943276465977519, 102.5010903946856899 ) ) ;
#71171=CARTESIAN_POINT ( 'NONE',  ( 14.29746914071037800, 8.314922557961029526, 101.6677570613523613 ) ) ;
#71172=CARTESIAN_POINT ( 'NONE',  ( 4.483927247898545687, 16.52544592524342804, 79.79057627198102409 ) ) ;
#71173=CARTESIAN_POINT ( 'NONE',  ( -5.049401038297874678, -19.05341960407617918, 89.79275706135230450 ) ) ;
#71175=CARTESIAN_POINT ( 'NONE',  ( 0.05219959533936267826, -19.03943276465977164, 45.00109039468566863 ) ) ;
#71176=CARTESIAN_POINT ( 'NONE',  ( 16.53943276465976808, 0.05219959533934440121, 106.2510903946856757 ) ) ;
#71177=CARTESIAN_POINT ( 'NONE',  ( 16.46253265017146816, 9.564922557961045513, 31.66775706135232937 ) ) ;
#71178=CARTESIAN_POINT ( 'NONE',  ( 5.153800228976335163, 19.02544592524342804, 94.79057627198103830 ) ) ;
#71179=CARTESIAN_POINT ( 'NONE',  ( 21.52544592524344225, -5.823673210054117533, 63.54057627198103830 ) ) ;
#71181=CARTESIAN_POINT ( 'NONE',  ( -13.97604488694527625, -13.89961937509977652, 21.87390960531435979 ) ) ;
#71182=CARTESIAN_POINT ( 'NONE',  ( 18.62759615963255655, 10.81492255796105972, 91.66775706135234714 ) ) ;
#71183=CARTESIAN_POINT ( 'NONE',  ( 14.34966873604972726, -8.224510206698740333, 70.83442372801901854 ) ) ;
#71184=CARTESIAN_POINT ( 'NONE',  ( -5.719274019375665041, -21.55341960407619695, 29.79275706135234358 ) ) ;
#71185=CARTESIAN_POINT ( 'NONE',  ( 14.29746914071037800, 8.314922557961029526, 36.66775706135234714 ) ) ;
#71186=CARTESIAN_POINT ( 'NONE',  ( -9.474510206698964154, 16.51473224551069663, 110.4155762719810383 ) ) ;
#71187=CARTESIAN_POINT ( 'NONE',  ( 13.97604488694527802, 13.89961937509977652, 34.37390960531436690 ) ) ;
#71188=CARTESIAN_POINT ( 'NONE',  ( 9.474510206698971260, -16.51473224551069308, 47.91557627198102409 ) ) ;
#71189=CARTESIAN_POINT ( 'NONE',  ( 12.06949235617739724, 12.14591786802326823, 51.87609039468568284 ) ) ;
#71190=CARTESIAN_POINT ( 'NONE',  ( -12.14591786802309592, -12.06949235617757132, 91.87390960531436690 ) ) ;
#71191=CARTESIAN_POINT ( 'NONE',  ( 4.379528057220092307, 16.55341960407617563, 97.29275706135234714 ) ) ;
#71192=CARTESIAN_POINT ( 'NONE',  ( 21.53943276465977519, 0.05219959533937863772, 41.25109039468568284 ) ) ;
#71193=CARTESIAN_POINT ( 'NONE',  ( 9.564922557960805705, 16.46253265017160317, 84.58224293864769550 ) ) ;
#71194=CARTESIAN_POINT ( 'NONE',  ( -5.153800228976328057, -19.02544592524343514, 62.29057627198100988 ) ) ;
#71195=CARTESIAN_POINT ( 'NONE',  ( -16.51473224551069308, -9.474510206698971260, 81.66557627198103830 ) ) ;
#71196=CARTESIAN_POINT ( 'NONE',  ( 8.314922557960818139, 14.29746914071049879, 34.58224293864770260 ) ) ;
#71197=CARTESIAN_POINT ( 'NONE',  ( -16.55341960407617563, 4.379528057220093196, 103.5427570613523613 ) ) ;
#71200=CARTESIAN_POINT ( 'NONE',  ( -13.89961937509957401, -13.97604488694547875, 39.37609039468566152 ) ) ;
#71201=CARTESIAN_POINT ( 'NONE',  ( 5.049401038298161559, -19.05341960407611168, 112.7072429386476813 ) ) ;
#71202=CARTESIAN_POINT ( 'NONE',  ( -9.564922557960796823, -16.46253265017161027, 57.08224293864769550 ) ) ;
#71203=CARTESIAN_POINT ( 'NONE',  ( 5.049401038297881783, 19.05341960407617563, 37.29275706135232582 ) ) ;
#71205=CARTESIAN_POINT ( 'NONE',  ( 8.314922557961029526, -14.29746914071037800, 40.41775706135234714 ) ) ;
#71206=CARTESIAN_POINT ( 'NONE',  ( -5.153800228976607833, 19.02544592524334988, 77.70942372801900433 ) ) ;
#71207=CARTESIAN_POINT ( 'NONE',  ( 8.314922557961029526, -14.29746914071037800, 55.41775706135234714 ) ) ;
#71208=CARTESIAN_POINT ( 'NONE',  ( -16.46253265017160317, 9.564922557960807481, 115.8322429386477097 ) ) ;
#71209=CARTESIAN_POINT ( 'NONE',  ( -9.474510206698964154, 16.51473224551069663, 90.41557627198103830 ) ) ;
#71210=CARTESIAN_POINT ( 'NONE',  ( -15.80617190586745835, -15.72974639402198527, 106.8739096053143811 ) ) ;
#71211=CARTESIAN_POINT ( 'NONE',  ( -19.05341960407617563, 5.049401038297882671, 83.54275706135233293 ) ) ;
#71212=CARTESIAN_POINT ( 'NONE',  ( 19.05341960407611168, 5.049401038298154454, 103.9572429386476671 ) ) ;
#71213=CARTESIAN_POINT ( 'NONE',  ( 19.02544592524343514, -5.153800228976328945, 38.54057627198103120 ) ) ;
#71214=CARTESIAN_POINT ( 'NONE',  ( -9.474510206698964154, 16.51473224551069663, 70.41557627198102409 ) ) ;
#71215=CARTESIAN_POINT ( 'NONE',  ( 14.29746914071049879, -8.314922557960816363, 38.33224293864768839 ) ) ;
#71216=CARTESIAN_POINT ( 'NONE',  ( -0.05219959533909027116, -19.03943276465977164, 42.49890960531435269 ) ) ;
#71217=CARTESIAN_POINT ( 'NONE',  ( 5.153800228976615827, -19.02544592524334988, 50.20942372801897591 ) ) ;
#71218=CARTESIAN_POINT ( 'NONE',  ( 4.483927247898545687, 16.52544592524342804, 89.79057627198103830 ) ) ;
#71219=CARTESIAN_POINT ( 'NONE',  ( -18.67979575497193778, 10.72451020669871902, 108.3344237280190185 ) ) ;
#71220=CARTESIAN_POINT ( 'NONE',  ( -5.153800228976328057, -19.02544592524343514, 47.29057627198102409 ) ) ;
#71221=CARTESIAN_POINT ( 'NONE',  ( 21.52544592524344225, -5.823673210054117533, 53.54057627198103120 ) ) ;
#71222=CARTESIAN_POINT ( 'NONE',  ( -8.314922557960811034, -14.29746914071050412, 52.08224293864768839 ) ) ;
#71223=CARTESIAN_POINT ( 'NONE',  ( -5.719274019375665041, -21.55341960407619695, 99.79275706135234714 ) ) ;
#71224=CARTESIAN_POINT ( 'NONE',  ( 13.89961937509977652, -13.97604488694527269, 113.1239096053143527 ) ) ;
#71225=CARTESIAN_POINT ( 'NONE',  ( -16.51473224551069308, -9.474510206698971260, 101.6655762719810241 ) ) ;
#71226=CARTESIAN_POINT ( 'NONE',  ( 13.97604488694527802, 13.89961937509977652, 34.37390960531436690 ) ) ;
#71227=CARTESIAN_POINT ( 'NONE',  ( -19.03943276465977164, 0.05219959533909376836, 26.24890960531435624 ) ) ;
#71228=CARTESIAN_POINT ( 'NONE',  ( 16.55341960407611168, 4.379528057220329451, 88.95724293864769550 ) ) ;
#71229=CARTESIAN_POINT ( 'NONE',  ( 15.72974639402199770, -15.80617190586745480, 98.12390960531436690 ) ) ;
#71230=CARTESIAN_POINT ( 'NONE',  ( 5.153800228976335163, 19.02544592524342804, 104.7905762719809957 ) ) ;
#71231=CARTESIAN_POINT ( 'NONE',  ( -18.67979575497178146, -10.72451020669898902, 111.6655762719810525 ) ) ;
#71232=CARTESIAN_POINT ( 'NONE',  ( -13.89961937509977652, 13.97604488694528158, 85.62390960531433848 ) ) ;
#71234=CARTESIAN_POINT ( 'NONE',  ( 14.29746914071049879, -8.314922557960816363, 98.33224293864769550 ) ) ;
#71235=CARTESIAN_POINT ( 'NONE',  ( -19.05341960407611168, -5.049401038298163336, 71.45724293864766707 ) ) ;
#71236=CARTESIAN_POINT ( 'NONE',  ( -15.72974639402197994, 15.80617190586746368, 75.62390960531439532 ) ) ;
#71239=CARTESIAN_POINT ( 'NONE',  ( 10.72451020669898902, -18.67979575497178502, 27.91557627198103830 ) ) ;
#71240=CARTESIAN_POINT ( 'NONE',  ( 18.56453257813360835, -5.500000000000033751, 68.49000423690685579 ) ) ;
#71241=CARTESIAN_POINT ( 'NONE',  ( -8.314922557961024197, 14.29746914071037800, 37.91775706135235424 ) ) ;
#71242=CARTESIAN_POINT ( 'NONE',  ( 12.14591786802309770, 12.06949235617756955, 89.37390960531435269 ) ) ;
#71244=CARTESIAN_POINT ( 'NONE',  ( 9.564922557960805705, 16.46253265017160317, 94.58224293864769550 ) ) ;
#71245=CARTESIAN_POINT ( 'NONE',  ( -5.049401038298153566, 19.05341960407611168, 45.20724293864769550 ) ) ;
#71246=CARTESIAN_POINT ( 'NONE',  ( -8.314922557960811034, -14.29746914071050412, 82.08224293864768129 ) ) ;
#71247=CARTESIAN_POINT ( 'NONE',  ( 21.53943276465977519, -0.05219959533907433946, 38.74890960531435979 ) ) ;
#71248=CARTESIAN_POINT ( 'NONE',  ( 12.14591786802309770, 12.06949235617756955, 54.37390960531435979 ) ) ;
#71249=CARTESIAN_POINT ( 'NONE',  ( 19.05341960407617918, -5.049401038297876454, 111.0427570613523329 ) ) ;
#71250=CARTESIAN_POINT ( 'NONE',  ( -10.72451020669870658, -18.67979575497194134, 79.58442372801903275 ) ) ;
#71252=CARTESIAN_POINT ( 'NONE',  ( -15.80617190586745835, -15.72974639402198527, 21.87390960531436690 ) ) ;
#71253=CARTESIAN_POINT ( 'NONE',  ( -14.29746914071037622, -8.314922557961029526, 89.16775706135236135 ) ) ;
#71254=CARTESIAN_POINT ( 'NONE',  ( -19.05341960407611168, -5.049401038298163336, 26.45724293864769550 ) ) ;
#71255=CARTESIAN_POINT ( 'NONE',  ( -5.049401038298153566, 19.05341960407611168, 80.20724293864769550 ) ) ;
#71256=CARTESIAN_POINT ( 'NONE',  ( -21.55341960407610458, -5.719274019375992779, 96.45724293864770971 ) ) ;
#71257=CARTESIAN_POINT ( 'NONE',  ( 8.314922557961029526, -14.29746914071037800, 25.41775706135235779 ) ) ;
#71258=CARTESIAN_POINT ( 'NONE',  ( -16.55341960407611168, -4.379528057220339221, 46.45724293864769550 ) ) ;
#71259=CARTESIAN_POINT ( 'NONE',  ( -18.62759615963255300, -10.81492255796106328, 74.16775706135231871 ) ) ;
#71260=CARTESIAN_POINT ( 'NONE',  ( 8.224510206698742110, 14.34966873604972548, 92.08442372801901854 ) ) ;
#71261=CARTESIAN_POINT ( 'NONE',  ( 10.72451020669898902, -18.67979575497178502, 22.91557627198102765 ) ) ;
#71264=CARTESIAN_POINT ( 'NONE',  ( -4.379528057220086978, -16.55341960407618274, 109.7927570613523613 ) ) ;
#71265=CARTESIAN_POINT ( 'NONE',  ( -16.52544592524335698, -4.483927247898792601, 63.95942372801901854 ) ) ;
#71266=CARTESIAN_POINT ( 'NONE',  ( -5.049401038298153566, 19.05341960407611168, 70.20724293864769550 ) ) ;
#71267=CARTESIAN_POINT ( 'NONE',  ( -19.03943276465977164, 0.05219959533909376836, 91.24890960531436690 ) ) ;
#71268=CARTESIAN_POINT ( 'NONE',  ( 18.67979575497194134, -10.72451020669871369, 65.83442372801900433 ) ) ;
#71269=CARTESIAN_POINT ( 'NONE',  ( -16.55341960407617563, 4.379528057220093196, 78.54275706135236135 ) ) ;
#71270=CARTESIAN_POINT ( 'NONE',  ( -8.314922557960811034, -14.29746914071050412, 42.08224293864769550 ) ) ;
#71271=CARTESIAN_POINT ( 'NONE',  ( 19.03943276465977164, -0.05219959533909143690, 58.74890960531435979 ) ) ;
#71272=CARTESIAN_POINT ( 'NONE',  ( 16.51473224551069308, 9.474510206698969483, 44.16557627198103120 ) ) ;
#71274=CARTESIAN_POINT ( 'NONE',  ( -16.51473224551082808, 9.474510206698731452, 108.3344237280190043 ) ) ;
#71275=CARTESIAN_POINT ( 'NONE',  ( -16.52544592524342804, 4.483927247898546575, 116.0405762719810383 ) ) ;
#71276=CARTESIAN_POINT ( 'NONE',  ( 9.564922557960805705, 16.46253265017160317, 69.58224293864770971 ) ) ;
#71277=CARTESIAN_POINT ( 'NONE',  ( 16.46253265017146816, 9.564922557961045513, 101.6677570613523329 ) ) ;
#71279=CARTESIAN_POINT ( 'NONE',  ( -0.05219959533937732626, 21.53943276465977519, 97.50109039468567573 ) ) ;
#71280=CARTESIAN_POINT ( 'NONE',  ( 8.314922557961029526, -14.29746914071037800, 70.41775706135236135 ) ) ;
#71281=CARTESIAN_POINT ( 'NONE',  ( 13.97604488694548053, -13.89961937509957401, 95.62609039468563310 ) ) ;
#71282=CARTESIAN_POINT ( 'NONE',  ( 21.52544592524344225, -5.823673210054117533, 63.54057627198103830 ) ) ;
#71283=CARTESIAN_POINT ( 'NONE',  ( 12.06949235617739724, 12.14591786802326823, 51.87609039468568284 ) ) ;
#71285=CARTESIAN_POINT ( 'NONE',  ( 19.05341960407617918, -5.049401038297876454, 56.04275706135234714 ) ) ;
#71286=CARTESIAN_POINT ( 'NONE',  ( 18.67979575497194134, -10.72451020669871369, 90.83442372801901854 ) ) ;
#71287=CARTESIAN_POINT ( 'NONE',  ( -5.049401038298153566, 19.05341960407611168, 25.20724293864768484 ) ) ;
#71288=CARTESIAN_POINT ( 'NONE',  ( 9.564922557960805705, 16.46253265017160317, 64.58224293864769550 ) ) ;
#71289=CARTESIAN_POINT ( 'NONE',  ( 12.14591786802309770, 12.06949235617756955, 64.37390960531435269 ) ) ;
#71292=CARTESIAN_POINT ( 'NONE',  ( -15.80617190586768217, 15.72974639402176855, 93.12609039468568994 ) ) ;
#71293=CARTESIAN_POINT ( 'NONE',  ( -16.51473224551082808, 9.474510206698731452, 43.33442372801900433 ) ) ;
#71294=CARTESIAN_POINT ( 'NONE',  ( -9.474510206698720793, -16.51473224551083518, 24.58442372801900078 ) ) ;
#71295=CARTESIAN_POINT ( 'NONE',  ( 5.823673210054125526, 21.52544592524343514, 24.79057627198103120 ) ) ;
#71296=CARTESIAN_POINT ( 'NONE',  ( -15.80617190586768217, 15.72974639402176855, 103.1260903946856757 ) ) ;
#71297=CARTESIAN_POINT ( 'NONE',  ( -19.03943276465977164, 0.05219959533909376836, 76.24890960531435269 ) ) ;
#71298=CARTESIAN_POINT ( 'NONE',  ( 21.55341960407619695, -5.719274019375665929, 91.04275706135236135 ) ) ;
#71299=CARTESIAN_POINT ( 'NONE',  ( 15.72974639402199770, -15.80617190586745480, 53.12390960531436690 ) ) ;
#71300=CARTESIAN_POINT ( 'NONE',  ( 5.049401038298161559, -19.05341960407611168, 77.70724293864765286 ) ) ;
#71301=CARTESIAN_POINT ( 'NONE',  ( 16.46253265017146816, 9.564922557961045513, 81.66775706135233293 ) ) ;
#71302=CARTESIAN_POINT ( 'NONE',  ( -19.05341960407611168, -5.049401038298163336, 41.45724293864769550 ) ) ;
#71303=CARTESIAN_POINT ( 'NONE',  ( 19.03943276465977164, -0.05219959533909143690, 83.74890960531436690 ) ) ;
#71304=CARTESIAN_POINT ( 'NONE',  ( -5.153800228976607833, 19.02544592524334988, 87.70942372801897591 ) ) ;
#71305=CARTESIAN_POINT ( 'NONE',  ( -16.55341960407617563, 4.379528057220093196, 48.54275706135234714 ) ) ;
#71306=CARTESIAN_POINT ( 'NONE',  ( 16.53943276465976808, -0.05219959533910856209, 103.7489096053143669 ) ) ;
#71307=CARTESIAN_POINT ( 'NONE',  ( 19.03943276465977164, -0.05219959533909143690, 68.74890960531436690 ) ) ;
#71308=CARTESIAN_POINT ( 'NONE',  ( 5.823673210054125526, 21.52544592524343514, 44.79057627198103120 ) ) ;
#71309=CARTESIAN_POINT ( 'NONE',  ( -5.153800228976607833, 19.02544592524334988, 112.7094237280190043 ) ) ;
#71310=CARTESIAN_POINT ( 'NONE',  ( -21.53943276465977519, -0.05219959533937600094, 33.75109039468568284 ) ) ;
#71311=CARTESIAN_POINT ( 'NONE',  ( 15.80617190586769283, -15.72974639402175789, 90.62609039468567573 ) ) ;
#71312=CARTESIAN_POINT ( 'NONE',  ( -14.29746914071037622, -8.314922557961029526, 89.16775706135236135 ) ) ;
#71313=CARTESIAN_POINT ( 'NONE',  ( 16.46253265017160672, -9.564922557960803928, 73.33224293864769550 ) ) ;
#71314=CARTESIAN_POINT ( 'NONE',  ( 12.06949235617739724, 12.14591786802326823, 101.8760903946857042 ) ) ;
#71315=CARTESIAN_POINT ( 'NONE',  ( 5.049401038297881783, 19.05341960407617563, 52.29275706135234003 ) ) ;
#71316=CARTESIAN_POINT ( 'NONE',  ( -5.823673210054431948, 21.52544592524334988, 32.70942372801900433 ) ) ;
#71317=CARTESIAN_POINT ( 'NONE',  ( 14.29746914071049879, -8.314922557960816363, 78.33224293864770971 ) ) ;
#71318=CARTESIAN_POINT ( 'NONE',  ( -16.51473224551069308, -9.474510206698971260, 96.66557627198102409 ) ) ;
#71319=CARTESIAN_POINT ( 'NONE',  ( 4.483927247898790824, -16.52544592524335698, 105.2094237280190328 ) ) ;
#71320=CARTESIAN_POINT ( 'NONE',  ( -21.55341960407619339, 5.719274019375674811, 78.54275706135236135 ) ) ;
#71321=CARTESIAN_POINT ( 'NONE',  ( 16.52544592524335698, 4.483927247898782831, 36.45942372801901143 ) ) ;
#71322=CARTESIAN_POINT ( 'NONE',  ( 21.53943276465977519, 0.05219959533937863772, 31.25109039468568639 ) ) ;
#71323=CARTESIAN_POINT ( 'NONE',  ( 8.224510206698953496, -14.34966873604960469, 72.91557627198103830 ) ) ;
#71324=EDGE_CURVE ( 'NONE', #88586, #4577, #27098, .T. ) ;
#71326=CARTESIAN_POINT ( 'NONE',  ( 18.62759615963271287, -10.81492255796078972, 103.3322429386476955 ) ) ;
#71327=CARTESIAN_POINT ( 'NONE',  ( -12.14591786802309592, -12.06949235617757132, 56.87390960531436690 ) ) ;
#71328=CARTESIAN_POINT ( 'NONE',  ( 13.97604488694527802, 13.89961937509977652, 24.37390960531435624 ) ) ;
#71329=CARTESIAN_POINT ( 'NONE',  ( 0.05219959533907565091, 21.53943276465977519, 24.99890960531435624 ) ) ;
#71330=CARTESIAN_POINT ( 'NONE',  ( 5.719274019375673035, 21.55341960407619339, 52.29275706135236135 ) ) ;
#71331=CARTESIAN_POINT ( 'NONE',  ( 8.314922557960818139, 14.29746914071049879, 59.58224293864770260 ) ) ;
#71332=CARTESIAN_POINT ( 'NONE',  ( 21.55341960407610458, 5.719274019375980345, 83.95724293864770971 ) ) ;
#71333=CARTESIAN_POINT ( 'NONE',  ( -13.89961937509977652, 13.97604488694528158, 70.62390960531432427 ) ) ;
#71334=CARTESIAN_POINT ( 'NONE',  ( -19.05341960407611168, -5.049401038298163336, 31.45724293864769550 ) ) ;
#71335=CARTESIAN_POINT ( 'NONE',  ( -13.89961937509957401, -13.97604488694547875, 79.37609039468567573 ) ) ;
#71336=CARTESIAN_POINT ( 'NONE',  ( -21.53943276465977519, -0.05219959533937600094, 53.75109039468568994 ) ) ;
#71337=CARTESIAN_POINT ( 'NONE',  ( 10.72451020669898902, -18.67979575497178502, 62.91557627198102409 ) ) ;
#71338=CARTESIAN_POINT ( 'NONE',  ( 19.03943276465977164, -0.05219959533909143690, 38.74890960531436690 ) ) ;
#71339=CARTESIAN_POINT ( 'NONE',  ( -0.05219959533909027116, -19.03943276465977164, 72.49890960531435269 ) ) ;
#71341=CARTESIAN_POINT ( 'NONE',  ( 8.314922557961029526, -14.29746914071037800, 45.41775706135234003 ) ) ;
#71342=CARTESIAN_POINT ( 'NONE',  ( 0.05219959533937995610, -21.53943276465977519, 35.00109039468568284 ) ) ;
#71343=CARTESIAN_POINT ( 'NONE',  ( 15.80617190586769283, -15.72974639402175789, 65.62609039468568994 ) ) ;
#71344=CARTESIAN_POINT ( 'NONE',  ( 9.564922557960805705, 16.46253265017160317, 99.58224293864770971 ) ) ;
#71345=CARTESIAN_POINT ( 'NONE',  ( 21.55341960407610458, 5.719274019375980345, 83.95724293864770971 ) ) ;
#71346=CARTESIAN_POINT ( 'NONE',  ( 21.53943276465977519, 0.05219959533937863772, 26.25109039468567573 ) ) ;
#71347=CARTESIAN_POINT ( 'NONE',  ( 8.224510206698742110, 14.34966873604972548, 47.08442372801901854 ) ) ;
#71348=CARTESIAN_POINT ( 'NONE',  ( -5.719274019375978568, 21.55341960407610458, 50.20724293864769550 ) ) ;
#71349=CARTESIAN_POINT ( 'NONE',  ( -9.474510206698720793, -16.51473224551083518, 24.58442372801900078 ) ) ;
#71350=CARTESIAN_POINT ( 'NONE',  ( 16.46253265017160672, -9.564922557960803928, 53.33224293864768839 ) ) ;
#71351=CARTESIAN_POINT ( 'NONE',  ( -5.153800228976328057, -19.02544592524343514, 112.2905762719810099 ) ) ;
#71352=CARTESIAN_POINT ( 'NONE',  ( -5.153800228976328057, -19.02544592524343514, 92.29057627198099567 ) ) ;
#71354=CARTESIAN_POINT ( 'NONE',  ( -16.46253265017146816, -9.564922557961047289, 74.16775706135234714 ) ) ;
#71355=CARTESIAN_POINT ( 'NONE',  ( 18.67979575497178502, 10.72451020669898547, 49.16557627198102409 ) ) ;
#71356=CARTESIAN_POINT ( 'NONE',  ( 16.52544592524342804, -4.483927247898539470, 28.54057627198103120 ) ) ;
#71357=CARTESIAN_POINT ( 'NONE',  ( -9.474510206698720793, -16.51473224551083518, 79.58442372801899012 ) ) ;
#71359=CARTESIAN_POINT ( 'NONE',  ( -9.564922557961040184, 16.46253265017147172, 22.91775706135233648 ) ) ;
#71360=CARTESIAN_POINT ( 'NONE',  ( -9.474510206698720793, -16.51473224551083518, 84.58442372801900433 ) ) ;
#71361=CARTESIAN_POINT ( 'NONE',  ( 16.51473224551083163, -9.474510206698727899, 45.83442372801900433 ) ) ;
#71362=CARTESIAN_POINT ( 'NONE',  ( 16.88567814943159817, 6.947325034625697171, 108.7900112265258912 ) ) ;
#71363=CARTESIAN_POINT ( 'NONE',  ( 16.46253265017160672, -9.564922557960803928, 58.33224293864769550 ) ) ;
#71364=CARTESIAN_POINT ( 'NONE',  ( -4.379528057220328563, 16.55341960407611168, 50.20724293864769550 ) ) ;
#71365=CARTESIAN_POINT ( 'NONE',  ( 19.03943276465977164, -0.05219959533909143690, 28.74890960531435624 ) ) ;
#71366=CARTESIAN_POINT ( 'NONE',  ( -4.483927247898539470, -16.52544592524342804, 42.29057627198103120 ) ) ;
#71368=CARTESIAN_POINT ( 'NONE',  ( 14.29746914071037800, 8.314922557961029526, 111.6677570613523613 ) ) ;
#71369=CARTESIAN_POINT ( 'NONE',  ( -5.049401038298153566, 19.05341960407611168, 45.20724293864769550 ) ) ;
#71370=CARTESIAN_POINT ( 'NONE',  ( -16.46253265017146816, -9.564922557961047289, 19.16775706135233293 ) ) ;
#71371=CARTESIAN_POINT ( 'NONE',  ( -16.55341960407617563, 4.379528057220093196, 38.54275706135234714 ) ) ;
#71372=CARTESIAN_POINT ( 'NONE',  ( 18.62759615963271287, -10.81492255796078972, 33.33224293864769550 ) ) ;
#71373=CARTESIAN_POINT ( 'NONE',  ( 5.823673210054444382, -21.52544592524334988, 90.20942372801903275 ) ) ;
#71375=CARTESIAN_POINT ( 'NONE',  ( 16.46253265017160672, -9.564922557960803928, 63.33224293864769550 ) ) ;
#71376=CARTESIAN_POINT ( 'NONE',  ( -5.049401038298153566, 19.05341960407611168, 105.2072429386476671 ) ) ;
#71377=CARTESIAN_POINT ( 'NONE',  ( 16.46253265017160672, -9.564922557960803928, 93.33224293864769550 ) ) ;
#71379=CARTESIAN_POINT ( 'NONE',  ( 0.05219959533937995610, -21.53943276465977519, 30.00109039468568284 ) ) ;
#71380=CARTESIAN_POINT ( 'NONE',  ( 16.52544592524342804, -4.483927247898539470, 83.54057627198102409 ) ) ;
#71381=CARTESIAN_POINT ( 'NONE',  ( -0.05219959533907301413, -21.53943276465977519, 77.49890960531433848 ) ) ;
#71382=CARTESIAN_POINT ( 'NONE',  ( -19.05341960407611168, -5.049401038298163336, 71.45724293864766707 ) ) ;
#71383=CARTESIAN_POINT ( 'NONE',  ( -16.46253265017160317, 9.564922557960807481, 70.83224293864770971 ) ) ;
#71384=CARTESIAN_POINT ( 'NONE',  ( -18.62759615963270932, 10.81492255796079327, 115.8322429386477097 ) ) ;
#71386=CARTESIAN_POINT ( 'NONE',  ( -19.03943276465977164, 0.05219959533909376836, 71.24890960531435269 ) ) ;
#71387=CARTESIAN_POINT ( 'NONE',  ( 16.55341960407611168, 4.379528057220329451, 103.9572429386476813 ) ) ;
#71389=CARTESIAN_POINT ( 'NONE',  ( 0.05219959533909260263, 19.03943276465977164, 59.99890960531436690 ) ) ;
#71390=CARTESIAN_POINT ( 'NONE',  ( -5.049401038297874678, -19.05341960407617918, 89.79275706135230450 ) ) ;
#71391=CARTESIAN_POINT ( 'NONE',  ( -8.224510206698948167, 14.34966873604960824, 95.41557627198102409 ) ) ;
#71392=CARTESIAN_POINT ( 'NONE',  ( 10.72451020669871369, 18.67979575497193778, 77.08442372801901854 ) ) ;
#71393=CARTESIAN_POINT ( 'NONE',  ( -16.46253265017160317, 9.564922557960807481, 55.83224293864769550 ) ) ;
#71394=CARTESIAN_POINT ( 'NONE',  ( -10.72451020669870658, -18.67979575497194134, 24.58442372801901499 ) ) ;
#71395=CARTESIAN_POINT ( 'NONE',  ( -16.53943276465976808, 0.05219959533911058130, 96.24890960531435269 ) ) ;
#71397=CARTESIAN_POINT ( 'NONE',  ( 19.02544592524343514, -5.153800228976328945, 68.54057627198103830 ) ) ;
#71398=CARTESIAN_POINT ( 'NONE',  ( 16.21995358207305316, 7.366697692864170754, 112.5644899848783496 ) ) ;
#71399=CARTESIAN_POINT ( 'NONE',  ( -9.564922557961040184, 16.46253265017147172, 107.9177570613523471 ) ) ;
#71400=CARTESIAN_POINT ( 'NONE',  ( -5.823673210054116645, -21.52544592524344225, 32.29057627198102409 ) ) ;
#71401=CARTESIAN_POINT ( 'NONE',  ( 18.62759615963255655, 10.81492255796105972, 51.66775706135234714 ) ) ;
#71402=CARTESIAN_POINT ( 'NONE',  ( -9.474510206698964154, 16.51473224551069663, 90.41557627198103830 ) ) ;
#71403=CARTESIAN_POINT ( 'NONE',  ( 16.51473224551083163, -9.474510206698727899, 85.83442372801900433 ) ) ;
#71404=CARTESIAN_POINT ( 'NONE',  ( 19.03943276465977164, -0.05219959533909143690, 68.74890960531436690 ) ) ;
#71405=CARTESIAN_POINT ( 'NONE',  ( 4.379528057220339221, -16.55341960407611168, 82.70724293864770971 ) ) ;
#71406=CARTESIAN_POINT ( 'NONE',  ( -5.153800228976328057, -19.02544592524343514, 102.2905762719810383 ) ) ;
#71407=CARTESIAN_POINT ( 'NONE',  ( 12.14591786802309770, 12.06949235617756955, 94.37390960531436690 ) ) ;
#71408=CARTESIAN_POINT ( 'NONE',  ( 19.02544592524343514, -5.153800228976328945, 93.54057627198102409 ) ) ;
#71409=CARTESIAN_POINT ( 'NONE',  ( -12.06949235617756955, 12.14591786802309770, 45.62390960531436690 ) ) ;
#71410=CARTESIAN_POINT ( 'NONE',  ( -19.05341960407611168, -5.049401038298163336, 21.45724293864768839 ) ) ;
#71412=CARTESIAN_POINT ( 'NONE',  ( 18.62759615963255655, 10.81492255796105972, 61.66775706135235424 ) ) ;
#71413=CARTESIAN_POINT ( 'NONE',  ( -9.564922557961040184, 16.46253265017147172, 77.91775706135234714 ) ) ;
#71414=CARTESIAN_POINT ( 'NONE',  ( 4.379528057220339221, -16.55341960407611168, 52.70724293864769550 ) ) ;
#71415=CARTESIAN_POINT ( 'NONE',  ( -15.80617190586745835, -15.72974639402198527, 96.87390960531436690 ) ) ;
#71416=CARTESIAN_POINT ( 'NONE',  ( 15.80617190586746368, 15.72974639402197994, 34.37390960531435979 ) ) ;
#71417=CARTESIAN_POINT ( 'NONE',  ( 4.379528057220339221, -16.55341960407611168, 82.70724293864770971 ) ) ;
#71418=CARTESIAN_POINT ( 'NONE',  ( 5.049401038298161559, -19.05341960407611168, 52.70724293864767418 ) ) ;
#71419=CARTESIAN_POINT ( 'NONE',  ( 0.05219959533910956823, 16.53943276465976808, 29.99890960531435979 ) ) ;
#71420=CARTESIAN_POINT ( 'NONE',  ( -14.29746914071037622, -8.314922557961029526, 89.16775706135236135 ) ) ;
#71421=CARTESIAN_POINT ( 'NONE',  ( 14.34966873604972726, -8.224510206698740333, 75.83442372801900433 ) ) ;
#71422=CARTESIAN_POINT ( 'NONE',  ( 19.03943276465977164, 0.05219959533936151252, 26.25109039468566507 ) ) ;
#71423=CARTESIAN_POINT ( 'NONE',  ( 0.05219959533909260263, 19.03943276465977164, 89.99890960531436690 ) ) ;
#71424=CARTESIAN_POINT ( 'NONE',  ( -9.474510206698964154, 16.51473224551069663, 75.41557627198103830 ) ) ;
#71425=CARTESIAN_POINT ( 'NONE',  ( 14.29746914071037800, 8.314922557961029526, 81.66775706135236135 ) ) ;
#71426=CARTESIAN_POINT ( 'NONE',  ( 0.05219959533909260263, 19.03943276465977164, 34.99890960531435979 ) ) ;
#71427=CARTESIAN_POINT ( 'NONE',  ( -16.53943276465976808, 0.05219959533911058130, 51.24890960531436690 ) ) ;
#71428=CARTESIAN_POINT ( 'NONE',  ( 19.03943276465977164, -0.05219959533909143690, 113.7489096053143669 ) ) ;
#71429=CARTESIAN_POINT ( 'NONE',  ( 5.049401038298161559, -19.05341960407611168, 102.7072429386476955 ) ) ;
#71430=CARTESIAN_POINT ( 'NONE',  ( 0.05219959533907565091, 21.53943276465977519, 39.99890960531436690 ) ) ;
#71431=CARTESIAN_POINT ( 'NONE',  ( -16.55341960407611168, -4.379528057220339221, 76.45724293864769550 ) ) ;
#71432=CARTESIAN_POINT ( 'NONE',  ( 16.53943276465976808, 0.05219959533934440121, 21.25109039468567218 ) ) ;
#71434=CARTESIAN_POINT ( 'NONE',  ( -8.314922557960811034, -14.29746914071050412, 72.08224293864769550 ) ) ;
#71436=CARTESIAN_POINT ( 'NONE',  ( -13.97604488694547697, 13.89961937509957934, 58.12609039468566863 ) ) ;
#71437=CARTESIAN_POINT ( 'NONE',  ( 16.51473224551069308, 9.474510206698969483, 109.1655762719810383 ) ) ;
#71438=CARTESIAN_POINT ( 'NONE',  ( -9.474510206698720793, -16.51473224551083518, 79.58442372801899012 ) ) ;
#71439=CARTESIAN_POINT ( 'NONE',  ( 16.46253265017146816, 9.564922557961045513, 106.6677570613523471 ) ) ;
#71440=CARTESIAN_POINT ( 'NONE',  ( -8.314922557961024197, 14.29746914071037800, 92.91775706135236135 ) ) ;
#71441=CARTESIAN_POINT ( 'NONE',  ( 0.05219959533909260263, 19.03943276465977164, 34.99890960531435979 ) ) ;
#71442=CARTESIAN_POINT ( 'NONE',  ( 15.80617190586746368, 15.72974639402197994, 29.37390960531435269 ) ) ;
#71443=CARTESIAN_POINT ( 'NONE',  ( -10.72451020669870658, -18.67979575497194134, 54.58442372801901143 ) ) ;
#71444=CARTESIAN_POINT ( 'NONE',  ( -19.03943276465977164, -0.05219959533935918106, 113.7510903946856757 ) ) ;
#71445=CARTESIAN_POINT ( 'NONE',  ( 9.564922557961047289, -16.46253265017146816, 55.41775706135234003 ) ) ;
#71446=CARTESIAN_POINT ( 'NONE',  ( 13.89961937509977652, -13.97604488694527269, 68.12390960531436690 ) ) ;
#71447=CARTESIAN_POINT ( 'NONE',  ( -5.049401038298153566, 19.05341960407611168, 115.2072429386477097 ) ) ;
#71448=CARTESIAN_POINT ( 'NONE',  ( -14.29746914071049879, 8.314922557960819915, 80.83224293864769550 ) ) ;
#71449=CARTESIAN_POINT ( 'NONE',  ( 13.89961937509977652, -13.97604488694527269, 73.12390960531436690 ) ) ;
#71450=CARTESIAN_POINT ( 'NONE',  ( -5.049401038298153566, 19.05341960407611168, 85.20724293864766707 ) ) ;
#71452=CARTESIAN_POINT ( 'NONE',  ( 16.51473224551083163, -9.474510206698727899, 90.83442372801900433 ) ) ;
#71453=CARTESIAN_POINT ( 'NONE',  ( 15.80617190586746368, 15.72974639402197994, 59.37390960531436690 ) ) ;
#71454=CARTESIAN_POINT ( 'NONE',  ( 0.05219959533909260263, 19.03943276465977164, 34.99890960531435979 ) ) ;
#71455=CARTESIAN_POINT ( 'NONE',  ( -16.51473224551082808, 9.474510206698731452, 63.33442372801900433 ) ) ;
#71456=CARTESIAN_POINT ( 'NONE',  ( -16.51473224551069308, -9.474510206698971260, 51.66557627198102409 ) ) ;
#71457=CARTESIAN_POINT ( 'NONE',  ( -19.05341960407611168, -5.049401038298163336, 86.45724293864769550 ) ) ;
#71459=CARTESIAN_POINT ( 'NONE',  ( -15.80617190586745835, -15.72974639402198527, 91.87390960531436690 ) ) ;
#71460=CARTESIAN_POINT ( 'NONE',  ( 8.314922557960818139, 14.29746914071049879, 99.58224293864770971 ) ) ;
#71461=CARTESIAN_POINT ( 'NONE',  ( -19.02544592524334988, -5.153800228976617603, 53.95942372801898301 ) ) ;
#71462=CARTESIAN_POINT ( 'NONE',  ( -5.823673210054116645, -21.52544592524344225, 87.29057627198103830 ) ) ;
#71463=CARTESIAN_POINT ( 'NONE',  ( 18.67979575497178502, 10.72451020669898547, 74.16557627198102409 ) ) ;
#71464=CARTESIAN_POINT ( 'NONE',  ( 16.53943276465976808, -0.05219959533910856209, 33.74890960531436690 ) ) ;
#71465=CARTESIAN_POINT ( 'NONE',  ( -10.81492255796105439, 18.62759615963255655, 102.9177570613523756 ) ) ;
#71466=CARTESIAN_POINT ( 'NONE',  ( 0.05219959533934541429, -16.53943276465976808, 50.00109039468568994 ) ) ;
#71467=CARTESIAN_POINT ( 'NONE',  ( 13.89961937509977652, -13.97604488694527269, 83.12390960531436690 ) ) ;
#71468=CARTESIAN_POINT ( 'NONE',  ( -19.03943276465977164, 0.05219959533909376836, 26.24890960531435624 ) ) ;
#71469=CARTESIAN_POINT ( 'NONE',  ( -15.80617190586768217, 15.72974639402176855, 38.12609039468567573 ) ) ;
#71470=CARTESIAN_POINT ( 'NONE',  ( 15.80617190586769283, -15.72974639402175789, 60.62609039468567573 ) ) ;
#71471=CARTESIAN_POINT ( 'NONE',  ( 16.51473224551069308, 9.474510206698969483, 54.16557627198103120 ) ) ;
#71472=CARTESIAN_POINT ( 'NONE',  ( 0.05219959533907565091, 21.53943276465977519, 114.9989096053143669 ) ) ;
#71473=CARTESIAN_POINT ( 'NONE',  ( -5.153800228976607833, 19.02544592524334988, 57.70942372801899012 ) ) ;
#71474=CARTESIAN_POINT ( 'NONE',  ( -16.51473224551082808, 9.474510206698731452, 68.33442372801900433 ) ) ;
#71475=CARTESIAN_POINT ( 'NONE',  ( -12.14591786802326823, 12.06949235617739902, 33.12609039468569705 ) ) ;
#71477=CARTESIAN_POINT ( 'NONE',  ( -14.29746914071037622, -8.314922557961029526, 74.16775706135231871 ) ) ;
#71478=CARTESIAN_POINT ( 'NONE',  ( 19.02544592524343514, -5.153800228976328945, 43.54057627198103120 ) ) ;
#71480=CARTESIAN_POINT ( 'NONE',  ( 9.474510206698971260, -16.51473224551069308, 92.91557627198103830 ) ) ;
#71481=CARTESIAN_POINT ( 'NONE',  ( 16.55341960407611168, 4.379528057220329451, 113.9572429386477239 ) ) ;
#71482=CARTESIAN_POINT ( 'NONE',  ( -21.53943276465977519, 0.05219959533907696930, 76.24890960531435269 ) ) ;
#71483=CARTESIAN_POINT ( 'NONE',  ( -0.05219959533934338120, 16.53943276465976808, 62.50109039468568284 ) ) ;
#71484=CARTESIAN_POINT ( 'NONE',  ( -21.52544592524334988, -5.823673210054445271, 108.9594237280190185 ) ) ;
#71485=CARTESIAN_POINT ( 'NONE',  ( -9.474510206698964154, 16.51473224551069663, 45.41557627198103120 ) ) ;
#71486=CARTESIAN_POINT ( 'NONE',  ( -16.53943276465976808, 0.05219959533911058130, 26.24890960531435624 ) ) ;
#71487=CARTESIAN_POINT ( 'NONE',  ( -0.05219959533910754901, -16.53943276465976808, 62.49890960531436690 ) ) ;
#71488=CARTESIAN_POINT ( 'NONE',  ( -16.46253265017160317, 9.564922557960807481, 70.83224293864770971 ) ) ;
#71489=CARTESIAN_POINT ( 'NONE',  ( -0.05219959533937732626, 21.53943276465977519, 32.50109039468568284 ) ) ;
#71490=CARTESIAN_POINT ( 'NONE',  ( 5.049401038298161559, -19.05341960407611168, 77.70724293864765286 ) ) ;
#71491=CARTESIAN_POINT ( 'NONE',  ( 5.719274019375673035, 21.55341960407619339, 82.29275706135234714 ) ) ;
#71492=CARTESIAN_POINT ( 'NONE',  ( -16.55341960407617563, 4.379528057220093196, 63.54275706135234003 ) ) ;
#71493=CARTESIAN_POINT ( 'NONE',  ( 9.564922557960805705, 16.46253265017160317, 104.5822429386476955 ) ) ;
#71494=CARTESIAN_POINT ( 'NONE',  ( 4.483927247898545687, 16.52544592524342804, 44.79057627198103120 ) ) ;
#71495=CARTESIAN_POINT ( 'NONE',  ( -13.97604488694527625, -13.89961937509977652, 21.87390960531435979 ) ) ;
#71496=CARTESIAN_POINT ( 'NONE',  ( 16.55341960407618274, -4.379528057220086978, 51.04275706135234714 ) ) ;
#71497=CARTESIAN_POINT ( 'NONE',  ( 8.314922557960818139, 14.29746914071049879, 54.58224293864769550 ) ) ;
#71498=CARTESIAN_POINT ( 'NONE',  ( 16.46253265017160672, -9.564922557960803928, 113.3322429386476955 ) ) ;
#71499=CARTESIAN_POINT ( 'NONE',  ( -10.72451020669898014, 18.67979575497178502, 30.41557627198101699 ) ) ;
#71500=CARTESIAN_POINT ( 'NONE',  ( 0.05219959533936267826, -19.03943276465977164, 20.00109039468567218 ) ) ;
#71501=CARTESIAN_POINT ( 'NONE',  ( -14.34966873604960291, -8.224510206698953496, 91.66557627198103830 ) ) ;
#71502=CARTESIAN_POINT ( 'NONE',  ( -13.89961937509977652, 13.97604488694528158, 90.62390960531432427 ) ) ;
#71504=CARTESIAN_POINT ( 'NONE',  ( -4.483927247898782831, 16.52544592524335698, 57.70942372801901143 ) ) ;
#71505=CARTESIAN_POINT ( 'NONE',  ( 19.03943276465977164, -0.05219959533909143690, 58.74890960531435979 ) ) ;
#71507=CARTESIAN_POINT ( 'NONE',  ( -0.05219959533936034679, 19.03943276465977164, 42.50109039468566152 ) ) ;
#71508=CARTESIAN_POINT ( 'NONE',  ( 0.05219959533934541429, -16.53943276465976808, 80.00109039468568994 ) ) ;
#71509=CARTESIAN_POINT ( 'NONE',  ( -19.03943276465977164, -0.05219959533935918106, 98.75109039468567573 ) ) ;
#71510=CARTESIAN_POINT ( 'NONE',  ( 10.81492255796106328, -18.62759615963255655, 70.41775706135236135 ) ) ;
#71511=CARTESIAN_POINT ( 'NONE',  ( 9.474510206698971260, -16.51473224551069308, 72.91557627198102409 ) ) ;
#71512=CARTESIAN_POINT ( 'NONE',  ( 5.823673210054125526, 21.52544592524343514, 89.79057627198103830 ) ) ;
#71513=CARTESIAN_POINT ( 'NONE',  ( 16.52544592524342804, -4.483927247898539470, 98.54057627198105251 ) ) ;
#71514=CARTESIAN_POINT ( 'NONE',  ( 5.049401038297881783, 19.05341960407617563, 67.29275706135234714 ) ) ;
#71515=CARTESIAN_POINT ( 'NONE',  ( -18.67979575497178146, -10.72451020669898902, 61.66557627198103120 ) ) ;
#71516=CARTESIAN_POINT ( 'NONE',  ( 19.05341960407617918, -5.049401038297876454, 36.04275706135234003 ) ) ;
#71517=FACE_BOUND ( 'NONE', #186012, .T. ) ;
#71518=CARTESIAN_POINT ( 'NONE',  ( -18.67979575497178146, -10.72451020669898902, 96.66557627198102409 ) ) ;
#71519=CARTESIAN_POINT ( 'NONE',  ( -19.46398650005389541, 5.499999999999947597, 55.18269651486371430 ) ) ;
#71520=CARTESIAN_POINT ( 'NONE',  ( 0.05219959533909260263, 19.03943276465977164, 69.99890960531435269 ) ) ;
#71521=CARTESIAN_POINT ( 'NONE',  ( -5.153800228976328057, -19.02544592524343514, 92.29057627198102409 ) ) ;
#71522=CARTESIAN_POINT ( 'NONE',  ( 9.564922557961047289, -16.46253265017146816, 110.4177570613523471 ) ) ;
#71524=CARTESIAN_POINT ( 'NONE',  ( -9.564922557960796823, -16.46253265017161027, 42.08224293864769550 ) ) ;
#71525=CARTESIAN_POINT ( 'NONE',  ( -19.02544592524342804, 5.153800228976336051, 116.0405762719810383 ) ) ;
#71526=CARTESIAN_POINT ( 'NONE',  ( -15.80617190586745835, -15.72974639402198527, 86.87390960531438111 ) ) ;
#71527=CARTESIAN_POINT ( 'NONE',  ( -16.52544592524342804, 4.483927247898546575, 46.04057627198103830 ) ) ;
#71528=CARTESIAN_POINT ( 'NONE',  ( 5.823673210054444382, -21.52544592524334988, 70.20942372801904696 ) ) ;
#71530=CARTESIAN_POINT ( 'NONE',  ( -14.29746914071037622, -8.314922557961029526, 29.16775706135234003 ) ) ;
#71531=CARTESIAN_POINT ( 'NONE',  ( -5.049401038297874678, -19.05341960407617918, 29.79275706135232227 ) ) ;
#71532=CARTESIAN_POINT ( 'NONE',  ( 16.53943276465976808, -0.05219959533910856209, 28.74890960531435624 ) ) ;
#71533=CARTESIAN_POINT ( 'NONE',  ( -15.72974639402197994, 15.80617190586746368, 115.6239096053143669 ) ) ;
#71534=CARTESIAN_POINT ( 'NONE',  ( -4.483927247898539470, -16.52544592524342804, 52.29057627198102409 ) ) ;
#71535=CARTESIAN_POINT ( 'NONE',  ( 13.97604488694548053, -13.89961937509957401, 100.6260903946856615 ) ) ;
#71536=CARTESIAN_POINT ( 'NONE',  ( 9.564922557961047289, -16.46253265017146816, 65.41775706135233293 ) ) ;
#71537=CARTESIAN_POINT ( 'NONE',  ( -21.55341960407619339, 5.719274019375674811, 73.54275706135234714 ) ) ;
#71538=CARTESIAN_POINT ( 'NONE',  ( -9.564922557961040184, 16.46253265017147172, 52.91775706135233293 ) ) ;
#71539=CARTESIAN_POINT ( 'NONE',  ( -0.05219959533910754901, -16.53943276465976808, 112.4989096053143669 ) ) ;
#71540=CARTESIAN_POINT ( 'NONE',  ( -5.719274019375978568, 21.55341960407610458, 50.20724293864769550 ) ) ;
#71541=CARTESIAN_POINT ( 'NONE',  ( 16.52544592524342804, -4.483927247898539470, 43.54057627198103830 ) ) ;
#71542=CARTESIAN_POINT ( 'NONE',  ( -18.09918380851992481, -5.500000000000039968, 51.48618307335613054 ) ) ;
#71543=CARTESIAN_POINT ( 'NONE',  ( 10.72451020669871369, 18.67979575497193778, 112.0844237280190185 ) ) ;
#71544=CARTESIAN_POINT ( 'NONE',  ( 12.14591786802327356, -12.06949235617739191, 90.62609039468567573 ) ) ;
#71545=CARTESIAN_POINT ( 'NONE',  ( -16.55341960407611168, -4.379528057220339221, 36.45724293864768839 ) ) ;
#71546=CARTESIAN_POINT ( 'NONE',  ( 0.05219959533937995610, -21.53943276465977519, 75.00109039468568994 ) ) ;
#71547=CARTESIAN_POINT ( 'NONE',  ( 18.62759615963255655, 10.81492255796105972, 71.66775706135234714 ) ) ;
#71548=CARTESIAN_POINT ( 'NONE',  ( 10.72451020669898902, -18.67979575497178502, 77.91557627198102409 ) ) ;
#71550=CARTESIAN_POINT ( 'NONE',  ( -13.97604488694527625, -13.89961937509977652, 36.87390960531436690 ) ) ;
#71551=CARTESIAN_POINT ( 'NONE',  ( -15.80617190586768217, 15.72974639402176855, 53.12609039468568284 ) ) ;
#71552=CARTESIAN_POINT ( 'NONE',  ( 13.97604488694527802, 13.89961937509977652, 39.37390960531435269 ) ) ;
#71553=CARTESIAN_POINT ( 'NONE',  ( -0.05219959533909027116, -19.03943276465977164, 47.49890960531435979 ) ) ;
#71554=CARTESIAN_POINT ( 'NONE',  ( 16.52544592524342804, -4.483927247898539470, 93.54057627198103830 ) ) ;
#71555=CARTESIAN_POINT ( 'NONE',  ( -16.51473224551069308, -9.474510206698971260, 81.66557627198103830 ) ) ;
#71556=CARTESIAN_POINT ( 'NONE',  ( -16.55341960407611168, -4.379528057220339221, 46.45724293864769550 ) ) ;
#71557=CARTESIAN_POINT ( 'NONE',  ( -0.05219959533910754901, -16.53943276465976808, 102.4989096053143811 ) ) ;
#71558=CARTESIAN_POINT ( 'NONE',  ( -18.67979575497178146, -10.72451020669898902, 66.66557627198102409 ) ) ;
#71559=CARTESIAN_POINT ( 'NONE',  ( -0.05219959533937732626, 21.53943276465977519, 27.50109039468567929 ) ) ;
#71561=CARTESIAN_POINT ( 'NONE',  ( 13.97604488694527802, 13.89961937509977652, 84.37390960531433848 ) ) ;
#71562=CARTESIAN_POINT ( 'NONE',  ( 16.52544592524335698, 4.483927247898782831, 21.45942372801901499 ) ) ;
#71563=CARTESIAN_POINT ( 'NONE',  ( -10.81492255796078084, -18.62759615963271287, 77.08224293864769550 ) ) ;
#71564=CARTESIAN_POINT ( 'NONE',  ( 10.81492255796106328, -18.62759615963255655, 100.4177570613523471 ) ) ;
#71565=CARTESIAN_POINT ( 'NONE',  ( 19.03943276465977164, -0.05219959533909143690, 83.74890960531436690 ) ) ;
#71566=CARTESIAN_POINT ( 'NONE',  ( -21.53943276465977519, -0.05219959533937600094, 18.75109039468568639 ) ) ;
#71567=CARTESIAN_POINT ( 'NONE',  ( -16.46253265017160317, 9.564922557960807481, 110.8322429386476955 ) ) ;
#71568=CARTESIAN_POINT ( 'NONE',  ( 14.34966873604972726, -8.224510206698740333, 90.83442372801901854 ) ) ;
#71569=CARTESIAN_POINT ( 'NONE',  ( -18.62759615963255300, -10.81492255796106328, 69.16775706135234714 ) ) ;
#71570=CARTESIAN_POINT ( 'NONE',  ( -10.72451020669870658, -18.67979575497194134, 99.58442372801900433 ) ) ;
#71571=CARTESIAN_POINT ( 'NONE',  ( 12.06949235617739724, 12.14591786802326823, 66.87609039468568994 ) ) ;
#71572=CARTESIAN_POINT ( 'NONE',  ( -10.72451020669870658, -18.67979575497194134, 29.58442372801901854 ) ) ;
#71573=CARTESIAN_POINT ( 'NONE',  ( -18.67979575497193778, 10.72451020669871902, 93.33442372801901854 ) ) ;
#71574=CARTESIAN_POINT ( 'NONE',  ( 16.46253265017160672, -9.564922557960803928, 98.33224293864769550 ) ) ;
#71575=CARTESIAN_POINT ( 'NONE',  ( -21.52544592524343514, 5.823673210054127303, 91.04057627198103830 ) ) ;
#71576=CARTESIAN_POINT ( 'NONE',  ( 9.564922557961047289, -16.46253265017146816, 65.41775706135233293 ) ) ;
#71578=CARTESIAN_POINT ( 'NONE',  ( 15.72974639402199770, -15.80617190586745480, 58.12390960531435979 ) ) ;
#71579=CARTESIAN_POINT ( 'NONE',  ( 19.02544592524343514, -5.153800228976328945, 88.54057627198102409 ) ) ;
#71580=CARTESIAN_POINT ( 'NONE',  ( -16.53943276465976808, 0.05219959533911058130, 36.24890960531435979 ) ) ;
#71582=CARTESIAN_POINT ( 'NONE',  ( 16.46253265017146816, 9.564922557961045513, 71.66775706135233293 ) ) ;
#71584=CARTESIAN_POINT ( 'NONE',  ( -0.05219959533936034679, 19.03943276465977164, 107.5010903946856615 ) ) ;
#71585=CARTESIAN_POINT ( 'NONE',  ( -21.53943276465977519, 0.05219959533907696930, 81.24890960531436690 ) ) ;
#71586=CARTESIAN_POINT ( 'NONE',  ( 8.224510206698953496, -14.34966873604960469, 67.91557627198102409 ) ) ;
#71587=CARTESIAN_POINT ( 'NONE',  ( -9.474510206698964154, 16.51473224551069663, 95.41557627198102409 ) ) ;
#71588=CARTESIAN_POINT ( 'NONE',  ( -4.379528057220086978, -16.55341960407618274, 24.79275706135235779 ) ) ;
#71589=CARTESIAN_POINT ( 'NONE',  ( 16.51473224551069308, 9.474510206698969483, 64.16557627198102409 ) ) ;
#71590=CARTESIAN_POINT ( 'NONE',  ( -15.80617190586745835, -15.72974639402198527, 111.8739096053143669 ) ) ;
#71591=CARTESIAN_POINT ( 'NONE',  ( -19.03943276465977164, -0.05219959533935918106, 78.75109039468567573 ) ) ;
#71592=CARTESIAN_POINT ( 'NONE',  ( -9.474510206698964154, 16.51473224551069663, 95.41557627198102409 ) ) ;
#71593=CARTESIAN_POINT ( 'NONE',  ( 5.153800228976335163, 19.02544592524342804, 69.79057627198103830 ) ) ;
#71594=CARTESIAN_POINT ( 'NONE',  ( -5.823673210054116645, -21.52544592524344225, 72.29057627198102409 ) ) ;
#71595=CARTESIAN_POINT ( 'NONE',  ( -5.153800228976328057, -19.02544592524343514, 42.29057627198101699 ) ) ;
#71597=CARTESIAN_POINT ( 'NONE',  ( 0.05219959533910956823, 16.53943276465976808, 49.99890960531437401 ) ) ;
#71598=CARTESIAN_POINT ( 'NONE',  ( -13.89961937509977652, 13.97604488694528158, 100.6239096053143669 ) ) ;
#71600=CARTESIAN_POINT ( 'NONE',  ( 9.474510206698729675, 16.51473224551082808, 62.08442372801899722 ) ) ;
#71601=CARTESIAN_POINT ( 'NONE',  ( 18.67979575497178502, 10.72451020669898547, 84.16557627198103830 ) ) ;
#71602=CARTESIAN_POINT ( 'NONE',  ( -16.46253265017146816, -9.564922557961047289, 49.16775706135233293 ) ) ;
#71603=CARTESIAN_POINT ( 'NONE',  ( 5.049401038298161559, -19.05341960407611168, 102.7072429386476955 ) ) ;
#71605=CARTESIAN_POINT ( 'NONE',  ( 15.80617190586746368, 15.72974639402197994, 44.37390960531435979 ) ) ;
#71606=CARTESIAN_POINT ( 'NONE',  ( 19.05341960407611168, 5.049401038298154454, 78.95724293864769550 ) ) ;
#71607=CARTESIAN_POINT ( 'NONE',  ( 0.05219959533937995610, -21.53943276465977519, 65.00109039468568994 ) ) ;
#71608=CARTESIAN_POINT ( 'NONE',  ( -16.51473224551069308, -9.474510206698971260, 41.66557627198103120 ) ) ;
#71609=CARTESIAN_POINT ( 'NONE',  ( -10.72451020669898014, 18.67979575497178502, 115.4155762719810241 ) ) ;
#71611=CARTESIAN_POINT ( 'NONE',  ( -15.80617190586768217, 15.72974639402176855, 58.12609039468568994 ) ) ;
#71613=CARTESIAN_POINT ( 'NONE',  ( 19.05341960407611168, 5.049401038298154454, 113.9572429386477097 ) ) ;
#71614=CARTESIAN_POINT ( 'NONE',  ( -13.97604488694547697, 13.89961937509957934, 68.12609039468563310 ) ) ;
#71615=CIRCLE ( 'NONE', #103950, 1.250000000000006439 ) ;
#71617=CARTESIAN_POINT ( 'NONE',  ( -18.67979575497178146, -10.72451020669898902, 111.6655762719810525 ) ) ;
#71618=CARTESIAN_POINT ( 'NONE',  ( 19.05341960407611168, 5.049401038298154454, 63.95724293864769550 ) ) ;
#71619=CARTESIAN_POINT ( 'NONE',  ( -4.483927247898782831, 16.52544592524335698, 37.70942372801900433 ) ) ;
#71621=CARTESIAN_POINT ( 'NONE',  ( -18.67979575497193778, 10.72451020669871902, 98.33442372801901854 ) ) ;
#71622=CARTESIAN_POINT ( 'NONE',  ( -5.153800228976328057, -19.02544592524343514, 37.29057627198102409 ) ) ;
#71623=CARTESIAN_POINT ( 'NONE',  ( 15.80617190586769283, -15.72974639402175789, 110.6260903946857042 ) ) ;
#71624=CARTESIAN_POINT ( 'NONE',  ( -8.314922557961024197, 14.29746914071037800, 87.91775706135234714 ) ) ;
#71625=CARTESIAN_POINT ( 'NONE',  ( -0.05219959533909027116, -19.03943276465977164, 92.49890960531436690 ) ) ;
#71626=CARTESIAN_POINT ( 'NONE',  ( 10.81492255796106328, -18.62759615963255655, 55.41775706135234714 ) ) ;
#71628=CARTESIAN_POINT ( 'NONE',  ( -19.02544592524342804, 5.153800228976336051, 116.0405762719810383 ) ) ;
#71630=CARTESIAN_POINT ( 'NONE',  ( -14.34966873604972548, 8.224510206698743886, 53.33442372801901854 ) ) ;
#71631=CARTESIAN_POINT ( 'NONE',  ( 15.80617190586769283, -15.72974639402175789, 70.62609039468567573 ) ) ;
#71632=CARTESIAN_POINT ( 'NONE',  ( 15.72974639402176855, 15.80617190586768217, 106.8760903946856899 ) ) ;
#71634=CARTESIAN_POINT ( 'NONE',  ( 16.55341960407618274, -4.379528057220086978, 26.04275706135235779 ) ) ;
#71635=CARTESIAN_POINT ( 'NONE',  ( 13.97604488694527802, 13.89961937509977652, 89.37390960531436690 ) ) ;
#71636=CARTESIAN_POINT ( 'NONE',  ( 13.97604488694527802, 13.89961937509977652, 109.3739096053143669 ) ) ;
#71637=ORIENTED_EDGE ( 'NONE', *, *, #85633, .T. ) ;
#71638=CARTESIAN_POINT ( 'NONE',  ( 16.18388926212241685, 7.379444403734403579, 42.93953151366154231 ) ) ;
#71639=CARTESIAN_POINT ( 'NONE',  ( -12.06949235617756955, 12.14591786802309770, 115.6239096053143669 ) ) ;
#71640=CARTESIAN_POINT ( 'NONE',  ( -18.62759615963270932, 10.81492255796079327, 40.83224293864769550 ) ) ;
#71641=CARTESIAN_POINT ( 'NONE',  ( -16.53943276465976808, -0.05219959533934237506, 108.7510903946857042 ) ) ;
#71642=CARTESIAN_POINT ( 'NONE',  ( 4.379528057220339221, -16.55341960407611168, 87.70724293864769550 ) ) ;
#71643=CARTESIAN_POINT ( 'NONE',  ( 5.153800228976335163, 19.02544592524342804, 64.79057627198100988 ) ) ;
#71644=CARTESIAN_POINT ( 'NONE',  ( -5.823673210054431948, 21.52544592524334988, 87.70942372801901854 ) ) ;
#71645=CARTESIAN_POINT ( 'NONE',  ( 4.483927247898790824, -16.52544592524335698, 30.20942372801902565 ) ) ;
#71646=CARTESIAN_POINT ( 'NONE',  ( 16.52544592524342804, -4.483927247898539470, 88.54057627198103830 ) ) ;
#71647=CARTESIAN_POINT ( 'NONE',  ( -21.53943276465977519, -0.05219959533937600094, 38.75109039468567573 ) ) ;
#71648=CARTESIAN_POINT ( 'NONE',  ( -18.67979575497178146, -10.72451020669898902, 76.66557627198103830 ) ) ;
#71649=CARTESIAN_POINT ( 'NONE',  ( -9.474510206698720793, -16.51473224551083518, 34.58442372801899722 ) ) ;
#71651=CARTESIAN_POINT ( 'NONE',  ( -0.05219959533909027116, -19.03943276465977164, 97.49890960531436690 ) ) ;
#71652=CARTESIAN_POINT ( 'NONE',  ( 16.53943276465976808, -0.05219959533910856209, 68.74890960531435269 ) ) ;
#71653=CARTESIAN_POINT ( 'NONE',  ( 14.34966873604960469, 8.224510206698951720, 54.16557627198103120 ) ) ;
#71654=CARTESIAN_POINT ( 'NONE',  ( -14.34966873604960291, -8.224510206698953496, 21.66557627198102409 ) ) ;
#71655=CARTESIAN_POINT ( 'NONE',  ( 9.564922557961047289, -16.46253265017146816, 70.41775706135233293 ) ) ;
#71656=CARTESIAN_POINT ( 'NONE',  ( 19.39056639909672342, 5.500000000000042633, 53.28948781074348773 ) ) ;
#71657=CARTESIAN_POINT ( 'NONE',  ( -16.46253265017160317, 9.564922557960807481, 115.8322429386477097 ) ) ;
#71658=CARTESIAN_POINT ( 'NONE',  ( 16.52544592524342804, -4.483927247898539470, 83.54057627198102409 ) ) ;
#71660=CARTESIAN_POINT ( 'NONE',  ( 13.97604488694527802, 13.89961937509977652, 44.37390960531435269 ) ) ;
#71661=CARTESIAN_POINT ( 'NONE',  ( 21.53943276465977519, -0.05219959533907433946, 48.74890960531435979 ) ) ;
#71662=CARTESIAN_POINT ( 'NONE',  ( -15.80617190586745835, -15.72974639402198527, 86.87390960531438111 ) ) ;
#71663=CARTESIAN_POINT ( 'NONE',  ( 12.14591786802309770, 12.06949235617756955, 114.3739096053143527 ) ) ;
#71664=CARTESIAN_POINT ( 'NONE',  ( -14.34966873604972548, 8.224510206698743886, 63.33442372801900433 ) ) ;
#71665=CARTESIAN_POINT ( 'NONE',  ( -19.02544592524342804, 5.153800228976336051, 51.04057627198103120 ) ) ;
#71666=CARTESIAN_POINT ( 'NONE',  ( 0.05219959533936267826, -19.03943276465977164, 40.00109039468566152 ) ) ;
#71667=CARTESIAN_POINT ( 'NONE',  ( 21.55341960407619695, -5.719274019375665929, 56.04275706135235424 ) ) ;
#71668=CARTESIAN_POINT ( 'NONE',  ( 12.14591786802309770, 12.06949235617756955, 109.3739096053143811 ) ) ;
#71669=CARTESIAN_POINT ( 'NONE',  ( 9.564922557961047289, -16.46253265017146816, 85.41775706135233293 ) ) ;
#71671=CARTESIAN_POINT ( 'NONE',  ( 17.50000000000000000, 5.499999999999997335, 36.70309617465829177 ) ) ;
#71672=CARTESIAN_POINT ( 'NONE',  ( -0.05219959533907301413, -21.53943276465977519, 52.49890960531435979 ) ) ;
#71673=CARTESIAN_POINT ( 'NONE',  ( 16.51473224551069308, 9.474510206698969483, 29.16557627198103475 ) ) ;
#71674=CARTESIAN_POINT ( 'NONE',  ( -10.72451020669870658, -18.67979575497194134, 79.58442372801903275 ) ) ;
#71675=CARTESIAN_POINT ( 'NONE',  ( 16.55341960407611168, 4.379528057220329451, 28.95724293864769905 ) ) ;
#71676=CARTESIAN_POINT ( 'NONE',  ( 16.53943276465976808, 0.05219959533934440121, 56.25109039468568284 ) ) ;
#71677=CARTESIAN_POINT ( 'NONE',  ( 8.314922557960818139, 14.29746914071049879, 44.58224293864769550 ) ) ;
#71678=CARTESIAN_POINT ( 'NONE',  ( -10.72451020669898014, 18.67979575497178502, 75.41557627198102409 ) ) ;
#71679=CARTESIAN_POINT ( 'NONE',  ( -21.55341960407610458, -5.719274019375992779, 81.45724293864769550 ) ) ;
#71680=CARTESIAN_POINT ( 'NONE',  ( -18.22780087662122028, 5.500000000000031086, 68.51540105326107266 ) ) ;
#71681=CARTESIAN_POINT ( 'NONE',  ( 0.05219959533936267826, -19.03943276465977164, 85.00109039468567573 ) ) ;
#71682=CARTESIAN_POINT ( 'NONE',  ( -0.05219959533909027116, -19.03943276465977164, 112.4989096053143669 ) ) ;
#71684=CARTESIAN_POINT ( 'NONE',  ( 16.46253265017160672, -9.564922557960803928, 43.33224293864769550 ) ) ;
#71685=CARTESIAN_POINT ( 'NONE',  ( -16.46253265017160317, 9.564922557960807481, 35.83224293864768839 ) ) ;
#71686=CARTESIAN_POINT ( 'NONE',  ( -17.97161686093728150, 5.499999999999980460, 75.99637206859166838 ) ) ;
#71688=CARTESIAN_POINT ( 'NONE',  ( -14.29746914071037622, -8.314922557961029526, 89.16775706135236135 ) ) ;
#71689=CARTESIAN_POINT ( 'NONE',  ( -21.55341960407610458, -5.719274019375992779, 106.4572429386477097 ) ) ;
#71690=CARTESIAN_POINT ( 'NONE',  ( 16.46253265017160672, -9.564922557960803928, 68.33224293864770971 ) ) ;
#71691=CARTESIAN_POINT ( 'NONE',  ( 10.72451020669871369, 18.67979575497193778, 47.08442372801901854 ) ) ;
#71692=CARTESIAN_POINT ( 'NONE',  ( -5.049401038298153566, 19.05341960407611168, 100.2072429386476955 ) ) ;
#71695=CARTESIAN_POINT ( 'NONE',  ( 21.52544592524334988, 5.823673210054432836, 36.45942372801901143 ) ) ;
#71696=CARTESIAN_POINT ( 'NONE',  ( 16.51473224551069308, 9.474510206698969483, 114.1655762719810241 ) ) ;
#71697=CARTESIAN_POINT ( 'NONE',  ( 9.564922557960805705, 16.46253265017160317, 104.5822429386476955 ) ) ;
#71698=CARTESIAN_POINT ( 'NONE',  ( 16.51473224551083163, -9.474510206698727899, 35.83442372801899722 ) ) ;
#71699=CARTESIAN_POINT ( 'NONE',  ( 15.72974639402176855, 15.80617190586768217, 21.87609039468567573 ) ) ;
#71700=CARTESIAN_POINT ( 'NONE',  ( -13.89961937509957401, -13.97604488694547875, 44.37609039468566863 ) ) ;
#71701=CARTESIAN_POINT ( 'NONE',  ( 19.03943276465977164, 0.05219959533936151252, 51.25109039468567573 ) ) ;
#71702=CARTESIAN_POINT ( 'NONE',  ( -12.06949235617739369, -12.14591786802326823, 89.37609039468568994 ) ) ;
#71703=CARTESIAN_POINT ( 'NONE',  ( 13.97604488694527802, 13.89961937509977652, 114.3739096053143669 ) ) ;
#71704=CARTESIAN_POINT ( 'NONE',  ( 13.89961937509977652, -13.97604488694527269, 73.12390960531436690 ) ) ;
#71705=CARTESIAN_POINT ( 'NONE',  ( 21.52544592524334988, 5.823673210054432836, 76.45942372801901854 ) ) ;
#71706=CARTESIAN_POINT ( 'NONE',  ( -15.72974639402176322, -15.80617190586768395, 89.37609039468568994 ) ) ;
#71708=CARTESIAN_POINT ( 'NONE',  ( -9.564922557960796823, -16.46253265017161027, 87.08224293864769550 ) ) ;
#71709=CARTESIAN_POINT ( 'NONE',  ( -15.80617190586768217, 15.72974639402176855, 68.12609039468567573 ) ) ;
#71710=CARTESIAN_POINT ( 'NONE',  ( 19.05341960407617918, -5.049401038297876454, 106.0427570613523471 ) ) ;
#71711=CARTESIAN_POINT ( 'NONE',  ( 13.89961937509977652, -13.97604488694527269, 63.12390960531435979 ) ) ;
#71712=CARTESIAN_POINT ( 'NONE',  ( -16.46253265017160317, 9.564922557960807481, 115.8322429386477097 ) ) ;
#71713=CARTESIAN_POINT ( 'NONE',  ( -19.02544592524342804, 5.153800228976336051, 76.04057627198102409 ) ) ;
#71715=CARTESIAN_POINT ( 'NONE',  ( 19.05341960407611168, 5.049401038298154454, 68.95724293864769550 ) ) ;
#71716=CARTESIAN_POINT ( 'NONE',  ( -13.89961937509977652, 13.97604488694528158, 55.62390960531434558 ) ) ;
#71717=CARTESIAN_POINT ( 'NONE',  ( 15.72974639402199770, -15.80617190586745480, 108.1239096053143811 ) ) ;
#71718=CARTESIAN_POINT ( 'NONE',  ( 8.314922557961029526, -14.29746914071037800, 105.4177570613523613 ) ) ;
#71720=CARTESIAN_POINT ( 'NONE',  ( -16.51473224551082808, 9.474510206698731452, 63.33442372801900433 ) ) ;
#71721=CARTESIAN_POINT ( 'NONE',  ( -5.049401038298153566, 19.05341960407611168, 90.20724293864766707 ) ) ;
#71722=CARTESIAN_POINT ( 'NONE',  ( 8.224510206698953496, -14.34966873604960469, 67.91557627198102409 ) ) ;
#71723=CARTESIAN_POINT ( 'NONE',  ( 16.55341960407611168, 4.379528057220329451, 103.9572429386476813 ) ) ;
#71724=CARTESIAN_POINT ( 'NONE',  ( -5.823673210054116645, -21.52544592524344225, 27.29057627198103120 ) ) ;
#71725=CARTESIAN_POINT ( 'NONE',  ( 10.81492255796078972, 18.62759615963270932, 29.58224293864769905 ) ) ;
#71726=CARTESIAN_POINT ( 'NONE',  ( -8.224510206698948167, 14.34966873604960824, 90.41557627198103830 ) ) ;
#71727=CARTESIAN_POINT ( 'NONE',  ( -16.51473224551069308, -9.474510206698971260, 81.66557627198103830 ) ) ;
#71728=CARTESIAN_POINT ( 'NONE',  ( 5.049401038297881783, 19.05341960407617563, 27.29275706135232937 ) ) ;
#71729=CARTESIAN_POINT ( 'NONE',  ( 8.224510206698742110, 14.34966873604972548, 102.0844237280190185 ) ) ;
#71730=CARTESIAN_POINT ( 'NONE',  ( 19.05341960407611168, 5.049401038298154454, 93.95724293864769550 ) ) ;
#71731=CARTESIAN_POINT ( 'NONE',  ( -18.67979575497193778, 10.72451020669871902, 48.33442372801902565 ) ) ;
#71732=CARTESIAN_POINT ( 'NONE',  ( 0.05219959533907565091, 21.53943276465977519, 49.99890960531437401 ) ) ;
#71733=CARTESIAN_POINT ( 'NONE',  ( 18.62759615963255655, 10.81492255796105972, 26.66775706135235424 ) ) ;
#71734=CARTESIAN_POINT ( 'NONE',  ( 21.55341960407610458, 5.719274019375980345, 78.95724293864769550 ) ) ;
#71735=CARTESIAN_POINT ( 'NONE',  ( 16.55341960407611168, 4.379528057220329451, 98.95724293864770971 ) ) ;
#71736=CARTESIAN_POINT ( 'NONE',  ( -13.97604488694547697, 13.89961937509957934, 53.12609039468565442 ) ) ;
#71737=CARTESIAN_POINT ( 'NONE',  ( -19.03943276465977164, 0.05219959533909376836, 41.24890960531435269 ) ) ;
#71738=CARTESIAN_POINT ( 'NONE',  ( 19.02544592524343514, -5.153800228976328945, 93.54057627198102409 ) ) ;
#71739=CARTESIAN_POINT ( 'NONE',  ( 9.474510206698971260, -16.51473224551069308, 92.91557627198103830 ) ) ;
#71740=CARTESIAN_POINT ( 'NONE',  ( -8.224510206698948167, 14.34966873604960824, 110.4155762719810383 ) ) ;
#71741=CARTESIAN_POINT ( 'NONE',  ( 12.14591786802309770, 12.06949235617756955, 44.37390960531435979 ) ) ;
#71742=CARTESIAN_POINT ( 'NONE',  ( 16.52544592524335698, 4.483927247898782831, 36.45942372801901143 ) ) ;
#71743=CARTESIAN_POINT ( 'NONE',  ( -10.72451020669870658, -18.67979575497194134, 104.5844237280190185 ) ) ;
#71745=CARTESIAN_POINT ( 'NONE',  ( 14.34966873604972726, -8.224510206698740333, 110.8344237280190043 ) ) ;
#71746=CARTESIAN_POINT ( 'NONE',  ( 15.80617190586769283, -15.72974639402175789, 30.62609039468567929 ) ) ;
#71747=CARTESIAN_POINT ( 'NONE',  ( 13.89961937509977652, -13.97604488694527269, 108.1239096053143669 ) ) ;
#71749=CARTESIAN_POINT ( 'NONE',  ( 8.224510206698742110, 14.34966873604972548, 57.08442372801901854 ) ) ;
#71750=CARTESIAN_POINT ( 'NONE',  ( -16.53943276465976808, 0.05219959533911058130, 21.24890960531436690 ) ) ;
#71751=B_SPLINE_CURVE_WITH_KNOTS ( 'NONE', 3,
 ( #154478, #136332, #47309, #170645, #198006, #93791, #199994, #92790, #139300, #155471, #122141, #106969, #16963, #1782, #61461, #63460, #90803, #91785, #125136, #153479, #107959, #14975, #186834, #76635, #48302, #109959, #28187, #138313, #152486, #184818, #169646, #4568 ),
 .UNSPECIFIED., .F., .F.,
 ( 4, 2, 2, 2, 2, 2, 2, 2, 2, 2, 2, 2, 2, 2, 2, 4 ),
 ( 2.711112516444420852E-17, 0.0003712461730036998968, 0.0007424923460073726885, 0.001113738519011045480, 0.001484984692014718272, 0.002227477038022064072, 0.002598723211025740984, 0.002969969384029417896, 0.003341215557033094374, 0.003712461730036770852, 0.004083707903040447763, 0.004454954076044124675, 0.004826200249047800719, 0.005197446422051477631, 0.005568692595055154543, 0.005939938768058831454 ),
 .UNSPECIFIED. ) ;
#71752=CARTESIAN_POINT ( 'NONE',  ( 0.05219959533934541429, -16.53943276465976808, 90.00109039468567573 ) ) ;
#71753=CARTESIAN_POINT ( 'NONE',  ( 12.14591786802327356, -12.06949235617739191, 25.62609039468567929 ) ) ;
#71754=CARTESIAN_POINT ( 'NONE',  ( 5.049401038298161559, -19.05341960407611168, 42.70724293864767418 ) ) ;
#71755=CARTESIAN_POINT ( 'NONE',  ( -0.05219959533910754901, -16.53943276465976808, 112.4989096053143669 ) ) ;
#71756=CARTESIAN_POINT ( 'NONE',  ( -21.53943276465977519, 0.05219959533907696930, 116.2489096053143669 ) ) ;
#71757=CARTESIAN_POINT ( 'NONE',  ( -19.05341960407611168, -5.049401038298163336, 36.45724293864766707 ) ) ;
#71758=CARTESIAN_POINT ( 'NONE',  ( 0.05219959533909260263, 19.03943276465977164, 104.9989096053143669 ) ) ;
#71759=CARTESIAN_POINT ( 'NONE',  ( -10.81492255796105439, 18.62759615963255655, 27.91775706135234358 ) ) ;
#71760=CARTESIAN_POINT ( 'NONE',  ( 9.474510206698971260, -16.51473224551069308, 22.91557627198102765 ) ) ;
#71761=CARTESIAN_POINT ( 'NONE',  ( -5.049401038298153566, 19.05341960407611168, 105.2072429386476671 ) ) ;
#71762=CARTESIAN_POINT ( 'NONE',  ( 16.18388926212238843, -7.379444403734509272, 112.0604684863385074 ) ) ;
#71763=CARTESIAN_POINT ( 'NONE',  ( -16.46253265017160317, 9.564922557960807481, 100.8322429386477097 ) ) ;
#71764=CARTESIAN_POINT ( 'NONE',  ( 5.719274019375673035, 21.55341960407619339, 52.29275706135236135 ) ) ;
#71765=CARTESIAN_POINT ( 'NONE',  ( 16.53943276465976808, -0.05219959533910856209, 93.74890960531436690 ) ) ;
#71766=CARTESIAN_POINT ( 'NONE',  ( -9.564922557960796823, -16.46253265017161027, 97.08224293864769550 ) ) ;
#71767=CARTESIAN_POINT ( 'NONE',  ( 18.10062525802553424, -5.500000000000022204, 96.01383468041922242 ) ) ;
#71768=CARTESIAN_POINT ( 'NONE',  ( 14.29746914071037800, 8.314922557961029526, 66.66775706135234714 ) ) ;
#71769=CARTESIAN_POINT ( 'NONE',  ( 5.823673210054444382, -21.52544592524334988, 85.20942372801901854 ) ) ;
#71770=CARTESIAN_POINT ( 'NONE',  ( -16.52544592524335698, -4.483927247898792601, 38.95942372801901854 ) ) ;
#71771=CARTESIAN_POINT ( 'NONE',  ( 16.51473224551069308, 9.474510206698969483, 84.16557627198102409 ) ) ;
#71772=CARTESIAN_POINT ( 'NONE',  ( -4.379528057220086978, -16.55341960407618274, 19.79275706135235069 ) ) ;
#71773=CARTESIAN_POINT ( 'NONE',  ( 12.14591786802327356, -12.06949235617739191, 65.62609039468568994 ) ) ;
#71774=CARTESIAN_POINT ( 'NONE',  ( 16.51473224551083163, -9.474510206698727899, 20.83442372801899722 ) ) ;
#71775=CARTESIAN_POINT ( 'NONE',  ( -19.03943276465977164, -0.05219959533935918106, 88.75109039468567573 ) ) ;
#71776=CARTESIAN_POINT ( 'NONE',  ( 13.97604488694527802, 13.89961937509977652, 69.37390960531436690 ) ) ;
#71777=CARTESIAN_POINT ( 'NONE',  ( -21.52544592524343514, 5.823673210054127303, 81.04057627198102409 ) ) ;
#71778=CARTESIAN_POINT ( 'NONE',  ( -8.314922557960811034, -14.29746914071050412, 87.08224293864769550 ) ) ;
#71779=CARTESIAN_POINT ( 'NONE',  ( 19.05341960407617918, -5.049401038297876454, 96.04275706135231871 ) ) ;
#71780=CARTESIAN_POINT ( 'NONE',  ( -8.314922557961024197, 14.29746914071037800, 57.91775706135234714 ) ) ;
#71782=CARTESIAN_POINT ( 'NONE',  ( 19.05341960407617918, -5.049401038297876454, 61.04275706135232582 ) ) ;
#71783=CARTESIAN_POINT ( 'NONE',  ( -4.483927247898539470, -16.52544592524342804, 32.29057627198102409 ) ) ;
#71784=CARTESIAN_POINT ( 'NONE',  ( -8.314922557960811034, -14.29746914071050412, 77.08224293864769550 ) ) ;
#71785=CARTESIAN_POINT ( 'NONE',  ( -5.719274019375665041, -21.55341960407619695, 109.7927570613523613 ) ) ;
#71786=CARTESIAN_POINT ( 'NONE',  ( -16.20579543436696568, 7.371946100355090792, 39.43479165828050270 ) ) ;
#71787=CARTESIAN_POINT ( 'NONE',  ( 21.55341960407619695, -5.719274019375665929, 21.04275706135234714 ) ) ;
#71789=CARTESIAN_POINT ( 'NONE',  ( 5.153800228976335163, 19.02544592524342804, 104.7905762719809957 ) ) ;
#71790=CARTESIAN_POINT ( 'NONE',  ( 16.51473224551069308, 9.474510206698969483, 84.16557627198102409 ) ) ;
#71791=CARTESIAN_POINT ( 'NONE',  ( -18.67979575497193778, 10.72451020669871902, 93.33442372801901854 ) ) ;
#71792=CARTESIAN_POINT ( 'NONE',  ( 9.564922557960805705, 16.46253265017160317, 74.58224293864769550 ) ) ;
#71793=CARTESIAN_POINT ( 'NONE',  ( 18.62759615963271287, -10.81492255796078972, 43.33224293864769550 ) ) ;
#71794=CARTESIAN_POINT ( 'NONE',  ( 4.483927247898545687, 16.52544592524342804, 74.79057627198105251 ) ) ;
#71795=CARTESIAN_POINT ( 'NONE',  ( 16.51473224551069308, 9.474510206698969483, 39.16557627198103120 ) ) ;
#71796=CARTESIAN_POINT ( 'NONE',  ( -12.14591786802309592, -12.06949235617757132, 91.87390960531436690 ) ) ;
#71797=CARTESIAN_POINT ( 'NONE',  ( 21.52544592524344225, -5.823673210054117533, 113.5405762719810383 ) ) ;
#71798=CARTESIAN_POINT ( 'NONE',  ( -10.72451020669870658, -18.67979575497194134, 59.58442372801901854 ) ) ;
#71799=CARTESIAN_POINT ( 'NONE',  ( 9.474510206698971260, -16.51473224551069308, 27.91557627198103120 ) ) ;
#71800=CARTESIAN_POINT ( 'NONE',  ( -16.52544592524335698, -4.483927247898792601, 58.95942372801902565 ) ) ;
#71801=CARTESIAN_POINT ( 'NONE',  ( 18.67979575497194134, -10.72451020669871369, 20.83442372801901143 ) ) ;
#71802=CARTESIAN_POINT ( 'NONE',  ( -0.05219959533907301413, -21.53943276465977519, 107.4989096053143669 ) ) ;
#71803=CARTESIAN_POINT ( 'NONE',  ( 13.97604488694548053, -13.89961937509957401, 40.62609039468564731 ) ) ;
#71804=CARTESIAN_POINT ( 'NONE',  ( 19.05341960407611168, 5.049401038298154454, 48.95724293864768129 ) ) ;
#71805=FACE_OUTER_BOUND ( 'NONE', #197279, .T. ) ;
#71806=CARTESIAN_POINT ( 'NONE',  ( -21.55341960407619339, 5.719274019375674811, 68.54275706135234714 ) ) ;
#71807=CARTESIAN_POINT ( 'NONE',  ( 18.62759615963271287, -10.81492255796078972, 58.33224293864768839 ) ) ;
#71808=CARTESIAN_POINT ( 'NONE',  ( 16.53943276465976808, -0.05219959533910856209, 33.74890960531436690 ) ) ;
#71809=CARTESIAN_POINT ( 'NONE',  ( -15.80617190586768217, 15.72974639402176855, 78.12609039468570415 ) ) ;
#71810=CARTESIAN_POINT ( 'NONE',  ( 15.80617190586769283, -15.72974639402175789, 110.6260903946857042 ) ) ;
#71811=CARTESIAN_POINT ( 'NONE',  ( 16.52544592524342804, -4.483927247898539470, 53.54057627198103120 ) ) ;
#71812=CARTESIAN_POINT ( 'NONE',  ( 4.379528057220339221, -16.55341960407611168, 107.7072429386476955 ) ) ;
#71813=CARTESIAN_POINT ( 'NONE',  ( 13.89961937509957401, 13.97604488694547697, 46.87609039468565442 ) ) ;
#71814=CARTESIAN_POINT ( 'NONE',  ( -8.314922557961024197, 14.29746914071037800, 102.9177570613523756 ) ) ;
#71815=CARTESIAN_POINT ( 'NONE',  ( -5.823673210054431948, 21.52544592524334988, 67.70942372801901854 ) ) ;
#71816=CARTESIAN_POINT ( 'NONE',  ( -13.89961937509977652, 13.97604488694528158, 55.62390960531434558 ) ) ;
#71817=CARTESIAN_POINT ( 'NONE',  ( -5.153800228976607833, 19.02544592524334988, 32.70942372801899722 ) ) ;
#71818=CARTESIAN_POINT ( 'NONE',  ( 21.55341960407610458, 5.719274019375980345, 38.95724293864768839 ) ) ;
#71819=CARTESIAN_POINT ( 'NONE',  ( 15.80617190586769283, -15.72974639402175789, 30.62609039468567929 ) ) ;
#71820=CARTESIAN_POINT ( 'NONE',  ( 5.719274019375991003, -21.55341960407610458, 82.70724293864770971 ) ) ;
#71821=CARTESIAN_POINT ( 'NONE',  ( 9.564922557961047289, -16.46253265017146816, 80.41775706135234714 ) ) ;
#71822=CARTESIAN_POINT ( 'NONE',  ( -8.314922557961024197, 14.29746914071037800, 47.91775706135234714 ) ) ;
#71823=CARTESIAN_POINT ( 'NONE',  ( 17.50000000000050449, -4.380085919831727459, 36.54968126928942240 ) ) ;
#71824=CARTESIAN_POINT ( 'NONE',  ( -5.823673210054116645, -21.52544592524344225, 87.29057627198103830 ) ) ;
#71825=CARTESIAN_POINT ( 'NONE',  ( 16.53943276465976808, -0.05219959533910856209, 73.74890960531433848 ) ) ;
#71827=CARTESIAN_POINT ( 'NONE',  ( -16.52544592524335698, -4.483927247898792601, 18.95942372801901143 ) ) ;
#71828=CARTESIAN_POINT ( 'NONE',  ( -5.719274019375978568, 21.55341960407610458, 45.20724293864769550 ) ) ;
#71829=CARTESIAN_POINT ( 'NONE',  ( -16.53943276465976808, -0.05219959533934237506, 78.75109039468568994 ) ) ;
#71830=CARTESIAN_POINT ( 'NONE',  ( 22.00000000000000000, -5.510910596163089556E-15, 42.49999999999999289 ) ) ;
#71831=CARTESIAN_POINT ( 'NONE',  ( 12.06949235617739724, 12.14591786802326823, 51.87609039468568284 ) ) ;
#71832=CARTESIAN_POINT ( 'NONE',  ( -10.81492255796105439, 18.62759615963255655, 27.91775706135234358 ) ) ;
#71833=CARTESIAN_POINT ( 'NONE',  ( -21.52544592524343514, 5.823673210054127303, 46.04057627198103830 ) ) ;
#71834=CARTESIAN_POINT ( 'NONE',  ( -14.34966873604972548, 8.224510206698743886, 68.33442372801900433 ) ) ;
#71835=CARTESIAN_POINT ( 'NONE',  ( -19.05341960407611168, -5.049401038298163336, 101.4572429386476955 ) ) ;
#71836=CARTESIAN_POINT ( 'NONE',  ( -5.823673210054431948, 21.52544592524334988, 62.70942372801902565 ) ) ;
#71837=CARTESIAN_POINT ( 'NONE',  ( -16.46253265017160317, 9.564922557960807481, 30.83224293864769550 ) ) ;
#71838=CARTESIAN_POINT ( 'NONE',  ( -5.823673210054116645, -21.52544592524344225, 37.29057627198102409 ) ) ;
#71839=CARTESIAN_POINT ( 'NONE',  ( -21.52544592524343514, 5.823673210054127303, 26.04057627198103475 ) ) ;
#71840=ORIENTED_EDGE ( 'NONE', *, *, #100439, .F. ) ;
#71841=CARTESIAN_POINT ( 'NONE',  ( 9.474510206698729675, 16.51473224551082808, 37.08442372801899722 ) ) ;
#71842=CARTESIAN_POINT ( 'NONE',  ( 16.55341960407618274, -4.379528057220086978, 56.04275706135235424 ) ) ;
#71843=CARTESIAN_POINT ( 'NONE',  ( 5.049401038298161559, -19.05341960407611168, 112.7072429386476813 ) ) ;
#71844=VERTEX_POINT ( 'NONE', #92959 ) ;
#71845=CARTESIAN_POINT ( 'NONE',  ( -5.153800228976328057, -19.02544592524343514, 82.29057627198103830 ) ) ;
#71846=CARTESIAN_POINT ( 'NONE',  ( 4.483927247898790824, -16.52544592524335698, 95.20942372801903275 ) ) ;
#71848=CARTESIAN_POINT ( 'NONE',  ( -8.224510206698948167, 14.34966873604960824, 90.41557627198103830 ) ) ;
#71849=CARTESIAN_POINT ( 'NONE',  ( 5.823673210054125526, 21.52544592524343514, 54.79057627198104541 ) ) ;
#71850=CARTESIAN_POINT ( 'NONE',  ( -5.153800228976328057, -19.02544592524343514, 32.29057627198102409 ) ) ;
#71851=CARTESIAN_POINT ( 'NONE',  ( -12.06949235617739369, -12.14591786802326823, 79.37609039468567573 ) ) ;
#71852=CARTESIAN_POINT ( 'NONE',  ( 10.81492255796106328, -18.62759615963255655, 35.41775706135234003 ) ) ;
#71853=CARTESIAN_POINT ( 'NONE',  ( 19.05341960407617918, -5.049401038297876454, 91.04275706135234714 ) ) ;
#71854=CARTESIAN_POINT ( 'NONE',  ( -13.89961937509977652, 13.97604488694528158, 45.62390960531433848 ) ) ;
#71855=CARTESIAN_POINT ( 'NONE',  ( -5.153800228976328057, -19.02544592524343514, 107.2905762719810383 ) ) ;
#71856=CARTESIAN_POINT ( 'NONE',  ( 18.62759615963255655, 10.81492255796105972, 101.6677570613523613 ) ) ;
#71857=CARTESIAN_POINT ( 'NONE',  ( 19.05341960407611168, 5.049401038298154454, 78.95724293864769550 ) ) ;
#71858=CARTESIAN_POINT ( 'NONE',  ( 12.06949235617739724, 12.14591786802326823, 66.87609039468568994 ) ) ;
#71859=CARTESIAN_POINT ( 'NONE',  ( -10.81492255796105439, 18.62759615963255655, 92.91775706135236135 ) ) ;
#71860=CARTESIAN_POINT ( 'NONE',  ( -5.049401038297874678, -19.05341960407617918, 49.79275706135231871 ) ) ;
#71861=CARTESIAN_POINT ( 'NONE',  ( -19.03943276465977164, -0.05219959533935918106, 63.75109039468566863 ) ) ;
#71863=CARTESIAN_POINT ( 'NONE',  ( -18.67979575497193778, 10.72451020669871902, 63.33442372801900433 ) ) ;
#71864=CARTESIAN_POINT ( 'NONE',  ( -19.05341960407611168, -5.049401038298163336, 66.45724293864769550 ) ) ;
#71865=CARTESIAN_POINT ( 'NONE',  ( 15.50000000000000178, -5.500000000000000888, 22.00000000000000711 ) ) ;
#71866=CARTESIAN_POINT ( 'NONE',  ( -5.049401038297874678, -19.05341960407617918, 54.79275706135234003 ) ) ;
#71867=FACE_OUTER_BOUND ( 'NONE', #5882, .T. ) ;
#71868=CARTESIAN_POINT ( 'NONE',  ( -0.05219959533909027116, -19.03943276465977164, 82.49890960531436690 ) ) ;
#71869=CARTESIAN_POINT ( 'NONE',  ( -14.29746914071049879, 8.314922557960819915, 40.83224293864769550 ) ) ;
#71870=CARTESIAN_POINT ( 'NONE',  ( 10.72451020669898902, -18.67979575497178502, 37.91557627198102409 ) ) ;
#71871=CARTESIAN_POINT ( 'NONE',  ( -18.09918380851993192, -5.500000000000014211, 96.48618307335613054 ) ) ;
#71872=CARTESIAN_POINT ( 'NONE',  ( 5.049401038297881783, 19.05341960407617563, 22.29275706135233648 ) ) ;
#71874=CARTESIAN_POINT ( 'NONE',  ( 5.049401038298161559, -19.05341960407611168, 42.70724293864767418 ) ) ;
#71875=CARTESIAN_POINT ( 'NONE',  ( 9.564922557960805705, 16.46253265017160317, 29.58224293864769550 ) ) ;
#71877=CARTESIAN_POINT ( 'NONE',  ( 15.80617190586769283, -15.72974639402175789, 70.62609039468567573 ) ) ;
#71879=CARTESIAN_POINT ( 'NONE',  ( 16.55341960407618274, -4.379528057220086978, 66.04275706135236135 ) ) ;
#71880=CARTESIAN_POINT ( 'NONE',  ( 10.81492255796078972, 18.62759615963270932, 79.58224293864769550 ) ) ;
#71881=CARTESIAN_POINT ( 'NONE',  ( 16.55341960407611168, 4.379528057220329451, 48.95724293864770971 ) ) ;
#71882=CARTESIAN_POINT ( 'NONE',  ( -5.153800228976328057, -19.02544592524343514, 27.29057627198103120 ) ) ;
#71883=CARTESIAN_POINT ( 'NONE',  ( -9.564922557960796823, -16.46253265017161027, 107.0822429386476955 ) ) ;
#71884=CARTESIAN_POINT ( 'NONE',  ( 21.52544592524334988, 5.823673210054432836, 31.45942372801901854 ) ) ;
#71885=CARTESIAN_POINT ( 'NONE',  ( -9.474510206698720793, -16.51473224551083518, 49.58442372801899722 ) ) ;
#71886=CARTESIAN_POINT ( 'NONE',  ( 0.05219959533909260263, 19.03943276465977164, 29.99890960531435979 ) ) ;
#71887=CARTESIAN_POINT ( 'NONE',  ( 15.72974639402176855, 15.80617190586768217, 86.87609039468568994 ) ) ;
#71888=CARTESIAN_POINT ( 'NONE',  ( 17.26058549869090086, -6.457015423128600773, 31.12254162523932166 ) ) ;
#71889=CARTESIAN_POINT ( 'NONE',  ( 12.06949235617757843, -12.14591786802309237, 33.12390960531435979 ) ) ;
#71890=CARTESIAN_POINT ( 'NONE',  ( 17.50000000000000000, 3.345213924137398820, 112.9123137690565528 ) ) ;
#71891=CARTESIAN_POINT ( 'NONE',  ( -15.72974639402197994, 15.80617190586746368, 45.62390960531436690 ) ) ;
#71893=CARTESIAN_POINT ( 'NONE',  ( 19.03943276465977164, -0.05219959533909143690, 93.74890960531435269 ) ) ;
#71894=CARTESIAN_POINT ( 'NONE',  ( 4.379528057220339221, -16.55341960407611168, 87.70724293864769550 ) ) ;
#71895=CARTESIAN_POINT ( 'NONE',  ( -19.03943276465977164, -0.05219959533935918106, 108.7510903946856615 ) ) ;
#71896=CARTESIAN_POINT ( 'NONE',  ( 5.719274019375991003, -21.55341960407610458, 57.70724293864770260 ) ) ;
#71898=CARTESIAN_POINT ( 'NONE',  ( 16.51473224551069308, 9.474510206698969483, 34.16557627198102409 ) ) ;
#71899=CARTESIAN_POINT ( 'NONE',  ( -16.51473224551069308, -9.474510206698971260, 81.66557627198103830 ) ) ;
#71900=CARTESIAN_POINT ( 'NONE',  ( 10.81492255796078972, 18.62759615963270932, 94.58224293864769550 ) ) ;
#71901=CARTESIAN_POINT ( 'NONE',  ( 4.483927247898790824, -16.52544592524335698, 105.2094237280190328 ) ) ;
#71902=CARTESIAN_POINT ( 'NONE',  ( -13.97604488694527625, -13.89961937509977652, 106.8739096053143669 ) ) ;
#71903=CARTESIAN_POINT ( 'NONE',  ( -19.02544592524334988, -5.153800228976617603, 73.95942372801900433 ) ) ;
#71904=CARTESIAN_POINT ( 'NONE',  ( -10.72451020669870658, -18.67979575497194134, 94.58442372801901854 ) ) ;
#71905=CARTESIAN_POINT ( 'NONE',  ( -18.67979575497178146, -10.72451020669898902, 76.66557627198103830 ) ) ;
#71906=CARTESIAN_POINT ( 'NONE',  ( 15.72974639402199770, -15.80617190586745480, 38.12390960531436690 ) ) ;
#71907=CARTESIAN_POINT ( 'NONE',  ( 13.89961937509977652, -13.97604488694527269, 48.12390960531435979 ) ) ;
#71908=CARTESIAN_POINT ( 'NONE',  ( -16.55341960407617563, 4.379528057220093196, 108.5427570613523756 ) ) ;
#71909=CARTESIAN_POINT ( 'NONE',  ( -0.05219959533909027116, -19.03943276465977164, 67.49890960531436690 ) ) ;
#71910=ORIENTED_EDGE ( 'NONE', *, *, #194452, .F. ) ;
#71912=CARTESIAN_POINT ( 'NONE',  ( -13.97604488694547697, 13.89961937509957934, 33.12609039468566863 ) ) ;
#71913=CARTESIAN_POINT ( 'NONE',  ( -12.06949235617756955, 12.14591786802309770, 75.62390960531439532 ) ) ;
#71914=CARTESIAN_POINT ( 'NONE',  ( 10.81492255796106328, -18.62759615963255655, 25.41775706135235779 ) ) ;
#71916=CARTESIAN_POINT ( 'NONE',  ( -15.80617190586745835, -15.72974639402198527, 56.87390960531436690 ) ) ;
#71917=ADVANCED_FACE ( 'NONE', ( #49455 ), #111117, .T. ) ;
#71918=CARTESIAN_POINT ( 'NONE',  ( 16.55341960407618274, -4.379528057220086978, 96.04275706135236135 ) ) ;
#71919=CARTESIAN_POINT ( 'NONE',  ( -12.06949235617756955, 12.14591786802309770, 105.6239096053143669 ) ) ;
#71920=CARTESIAN_POINT ( 'NONE',  ( 16.51473224551069308, 9.474510206698969483, 79.16557627198103830 ) ) ;
#71921=CARTESIAN_POINT ( 'NONE',  ( 8.224510206698953496, -14.34966873604960469, 32.91557627198102409 ) ) ;
#71922=ORIENTED_EDGE ( 'NONE', *, *, #62447, .F. ) ;
#71923=CARTESIAN_POINT ( 'NONE',  ( -18.62759615963255300, -10.81492255796106328, 44.16775706135234714 ) ) ;
#71924=CARTESIAN_POINT ( 'NONE',  ( -5.153800228976328057, -19.02544592524343514, 107.2905762719810383 ) ) ;
#71925=CARTESIAN_POINT ( 'NONE',  ( -15.72974639402176322, -15.80617190586768395, 79.37609039468567573 ) ) ;
#71926=CARTESIAN_POINT ( 'NONE',  ( -9.474510206698964154, 16.51473224551069663, 30.41557627198102054 ) ) ;
#71927=CARTESIAN_POINT ( 'NONE',  ( 5.049401038298161559, -19.05341960407611168, 32.70724293864768129 ) ) ;
#71929=CARTESIAN_POINT ( 'NONE',  ( 10.72451020669871369, 18.67979575497193778, 92.08442372801901854 ) ) ;
#71930=CARTESIAN_POINT ( 'NONE',  ( 16.55341960407618274, -4.379528057220086978, 46.04275706135234714 ) ) ;
#71931=CARTESIAN_POINT ( 'NONE',  ( -10.81492255796105439, 18.62759615963255655, 72.91775706135234714 ) ) ;
#71932=CARTESIAN_POINT ( 'NONE',  ( 9.474510206698971260, -16.51473224551069308, 107.9155762719810383 ) ) ;
#71933=CARTESIAN_POINT ( 'NONE',  ( -13.97604488694547697, 13.89961937509957934, 98.12609039468566152 ) ) ;
#71934=CARTESIAN_POINT ( 'NONE',  ( 0.05219959533937995610, -21.53943276465977519, 60.00109039468568284 ) ) ;
#71935=CARTESIAN_POINT ( 'NONE',  ( -12.14591786802326823, 12.06949235617739902, 23.12609039468567573 ) ) ;
#71936=CARTESIAN_POINT ( 'NONE',  ( 9.564922557961047289, -16.46253265017146816, 80.41775706135234714 ) ) ;
#71937=CARTESIAN_POINT ( 'NONE',  ( -19.03943276465977164, 0.05219959533909376836, 46.24890960531435979 ) ) ;
#71938=CARTESIAN_POINT ( 'NONE',  ( 16.46253265017146816, 9.564922557961045513, 101.6677570613523329 ) ) ;
#71939=CARTESIAN_POINT ( 'NONE',  ( 16.53943276465976808, -0.05219959533910856209, 23.74890960531435269 ) ) ;
#71940=CARTESIAN_POINT ( 'NONE',  ( -19.03943276465977164, -0.05219959533935918106, 83.75109039468567573 ) ) ;
#71941=CARTESIAN_POINT ( 'NONE',  ( 4.379528057220339221, -16.55341960407611168, 47.70724293864770260 ) ) ;
#71942=CARTESIAN_POINT ( 'NONE',  ( 16.46253265017146816, 9.564922557961045513, 61.66775706135234003 ) ) ;
#71943=CARTESIAN_POINT ( 'NONE',  ( -4.379528057220086978, -16.55341960407618274, 64.79275706135234714 ) ) ;
#71944=CARTESIAN_POINT ( 'NONE',  ( 16.46253265017146816, 9.564922557961045513, 21.66775706135233648 ) ) ;
#71945=CARTESIAN_POINT ( 'NONE',  ( 5.049401038298161559, -19.05341960407611168, 22.70724293864769194 ) ) ;
#71946=CARTESIAN_POINT ( 'NONE',  ( 16.46253265017160672, -9.564922557960803928, 38.33224293864768839 ) ) ;
#71947=CARTESIAN_POINT ( 'NONE',  ( 4.483927247898790824, -16.52544592524335698, 55.20942372801902565 ) ) ;
#71948=LINE ( 'NONE', #137591, #69234 ) ;
#71950=CARTESIAN_POINT ( 'NONE',  ( 19.05341960407611168, 5.049401038298154454, 88.95724293864769550 ) ) ;
#71951=CARTESIAN_POINT ( 'NONE',  ( -13.89961937509957401, -13.97604488694547697, 84.37609039468567573 ) ) ;
#71953=CARTESIAN_POINT ( 'NONE',  ( -19.03943276465977164, -0.05219959533935918106, 103.7510903946856757 ) ) ;
#71954=CARTESIAN_POINT ( 'NONE',  ( -18.62759615963270932, 10.81492255796079327, 35.83224293864768839 ) ) ;
#71955=CARTESIAN_POINT ( 'NONE',  ( 0.05219959533936267826, -19.03943276465977164, 25.00109039468566152 ) ) ;
#71956=CARTESIAN_POINT ( 'NONE',  ( 19.02544592524334988, 5.153800228976608722, 111.4594237280190043 ) ) ;
#71957=CARTESIAN_POINT ( 'NONE',  ( 16.55341960407611168, 4.379528057220329451, 108.9572429386476955 ) ) ;
#71958=CARTESIAN_POINT ( 'NONE',  ( 9.564922557960805705, 16.46253265017160317, 34.58224293864770260 ) ) ;
#71959=CARTESIAN_POINT ( 'NONE',  ( -18.62759615963270932, 10.81492255796079327, 70.83224293864770971 ) ) ;
#71960=CARTESIAN_POINT ( 'NONE',  ( -13.89961937509977652, 13.97604488694528158, 30.62390960531435269 ) ) ;
#71962=CARTESIAN_POINT ( 'NONE',  ( 19.03943276465977164, 0.05219959533936151252, 81.25109039468567573 ) ) ;
#71963=CARTESIAN_POINT ( 'NONE',  ( 16.52544592524342804, -4.483927247898539470, 53.54057627198103120 ) ) ;
#71964=CARTESIAN_POINT ( 'NONE',  ( -5.823673210054116645, -21.52544592524344225, 27.29057627198103120 ) ) ;
#71965=CARTESIAN_POINT ( 'NONE',  ( 18.67979575497194134, -10.72451020669871369, 90.83442372801901854 ) ) ;
#71966=CARTESIAN_POINT ( 'NONE',  ( 21.55341960407610458, 5.719274019375980345, 83.95724293864770971 ) ) ;
#71967=CARTESIAN_POINT ( 'NONE',  ( -15.80617190586768217, 15.72974639402176855, 78.12609039468570415 ) ) ;
#71968=CARTESIAN_POINT ( 'NONE',  ( 21.52544592524334988, 5.823673210054432836, 66.45942372801903275 ) ) ;
#71969=CARTESIAN_POINT ( 'NONE',  ( -19.03943276465977164, 0.05219959533909376836, 116.2489096053143669 ) ) ;
#71970=CARTESIAN_POINT ( 'NONE',  ( 16.53943276465976808, 0.05219959533934440121, 111.2510903946856899 ) ) ;
#71971=CARTESIAN_POINT ( 'NONE',  ( 21.55341960407619695, -5.719274019375665929, 61.04275706135234714 ) ) ;
#71972=CARTESIAN_POINT ( 'NONE',  ( -9.564922557960796823, -16.46253265017161027, 57.08224293864769550 ) ) ;
#71973=CARTESIAN_POINT ( 'NONE',  ( 18.62759615963255655, 10.81492255796105972, 36.66775706135234714 ) ) ;
#71974=CARTESIAN_POINT ( 'NONE',  ( 5.049401038298161559, -19.05341960407611168, 72.70724293864768129 ) ) ;
#71975=CARTESIAN_POINT ( 'NONE',  ( 4.483927247898545687, 16.52544592524342804, 79.79057627198102409 ) ) ;
#71976=CARTESIAN_POINT ( 'NONE',  ( -14.29746914071049879, 8.314922557960819915, 50.83224293864770971 ) ) ;
#71977=CARTESIAN_POINT ( 'NONE',  ( 15.72974639402199770, -15.80617190586745480, 58.12390960531435979 ) ) ;
#71978=CARTESIAN_POINT ( 'NONE',  ( 13.89961937509977652, -13.97604488694527269, 48.12390960531435979 ) ) ;
#71979=CARTESIAN_POINT ( 'NONE',  ( -10.81492255796078084, -18.62759615963271287, 62.08224293864769550 ) ) ;
#71980=CARTESIAN_POINT ( 'NONE',  ( 9.474510206698729675, 16.51473224551082808, 52.08442372801900433 ) ) ;
#71981=CARTESIAN_POINT ( 'NONE',  ( 13.97604488694548053, -13.89961937509957401, 20.62609039468567218 ) ) ;
#71982=CARTESIAN_POINT ( 'NONE',  ( -4.483927247898539470, -16.52544592524342804, 67.29057627198103830 ) ) ;
#71983=CARTESIAN_POINT ( 'NONE',  ( -18.62759615963270932, 10.81492255796079327, 45.83224293864769550 ) ) ;
#71986=CARTESIAN_POINT ( 'NONE',  ( 4.379528057220092307, 16.55341960407617563, 87.29275706135236135 ) ) ;
#71989=CARTESIAN_POINT ( 'NONE',  ( 9.474510206698729675, 16.51473224551082808, 87.08442372801900433 ) ) ;
#71990=CARTESIAN_POINT ( 'NONE',  ( 14.34966873604960469, 8.224510206698951720, 59.16557627198103120 ) ) ;
#71992=CARTESIAN_POINT ( 'NONE',  ( 0.05219959533909260263, 19.03943276465977164, 49.99890960531435979 ) ) ;
#71993=CARTESIAN_POINT ( 'NONE',  ( 4.483927247898545687, 16.52544592524342804, 44.79057627198103120 ) ) ;
#71994=CARTESIAN_POINT ( 'NONE',  ( -16.46253265017160317, 9.564922557960807481, 90.83224293864769550 ) ) ;
#71995=CARTESIAN_POINT ( 'NONE',  ( 19.03943276465977164, -0.05219959533909143690, 48.74890960531435979 ) ) ;
#71996=CARTESIAN_POINT ( 'NONE',  ( -15.72974639402176322, -15.80617190586768395, 54.37609039468568994 ) ) ;
#71997=CARTESIAN_POINT ( 'NONE',  ( 19.03943276465977164, -0.05219959533909143690, 78.74890960531436690 ) ) ;
#71998=CARTESIAN_POINT ( 'NONE',  ( -13.89961937509977652, 13.97604488694528158, 25.62390960531434558 ) ) ;
#71999=CARTESIAN_POINT ( 'NONE',  ( 16.51473224551069308, 9.474510206698969483, 64.16557627198102409 ) ) ;
#72000=CARTESIAN_POINT ( 'NONE',  ( 18.62759615963271287, -10.81492255796078972, 43.33224293864769550 ) ) ;
#72001=CARTESIAN_POINT ( 'NONE',  ( 0.05219959533909260263, 19.03943276465977164, 34.99890960531435979 ) ) ;
#72002=CARTESIAN_POINT ( 'NONE',  ( 5.719274019375991003, -21.55341960407610458, 47.70724293864770260 ) ) ;
#72003=B_SPLINE_CURVE_WITH_KNOTS ( 'NONE', 3,
 ( #151446, #105918, #163622, #150458, #165619, #148450, #44261, #41276, #196960, #102938, #27118, #136265, #26117, #195976, #180802, #182778, #10941, #117103, #29099, #178798, #72614, #197940 ),
 .UNSPECIFIED., .F., .F.,
 ( 4, 2, 2, 2, 2, 2, 2, 2, 2, 2, 4 ),
 ( 0.000000000000000000, 0.001309639967555287438, 0.001964459951332926061, 0.002291869943221736157, 0.002455574939166141855, 0.002619279935110547120, 0.002782984931054952819, 0.002946689926999358517, 0.003274099918888195501, 0.003928919902665849520, 0.005238559870221154088 ),
 .UNSPECIFIED. ) ;
#72004=CARTESIAN_POINT ( 'NONE',  ( -16.55341960407617563, 4.379528057220093196, 103.5427570613523613 ) ) ;
#72005=CARTESIAN_POINT ( 'NONE',  ( 5.153800228976615827, -19.02544592524334988, 20.20942372801899722 ) ) ;
#72006=CARTESIAN_POINT ( 'NONE',  ( 12.06949235617739724, 12.14591786802326823, 41.87609039468568284 ) ) ;
#72007=CARTESIAN_POINT ( 'NONE',  ( -12.06949235617739369, -12.14591786802326823, 79.37609039468567573 ) ) ;
#72009=CARTESIAN_POINT ( 'NONE',  ( -14.29746914071037622, -8.314922557961029526, 64.16775706135234714 ) ) ;
#72010=CARTESIAN_POINT ( 'NONE',  ( -8.224510206698735004, -14.34966873604973081, 59.58442372801901854 ) ) ;
#72011=CARTESIAN_POINT ( 'NONE',  ( -0.05219959533909027116, -19.03943276465977164, 112.4989096053143669 ) ) ;
#72012=CARTESIAN_POINT ( 'NONE',  ( 5.049401038298161559, -19.05341960407611168, 32.70724293864768129 ) ) ;
#72013=CARTESIAN_POINT ( 'NONE',  ( -8.314922557961024197, 14.29746914071037800, 32.91775706135234714 ) ) ;
#72014=CARTESIAN_POINT ( 'NONE',  ( 13.89961937509977652, -13.97604488694527269, 53.12390960531434558 ) ) ;
#72015=CARTESIAN_POINT ( 'NONE',  ( -0.05219959533937732626, 21.53943276465977519, 32.50109039468568284 ) ) ;
#72016=CARTESIAN_POINT ( 'NONE',  ( 16.53943276465976808, 0.05219959533934440121, 41.25109039468568284 ) ) ;
#72017=CARTESIAN_POINT ( 'NONE',  ( -8.314922557961024197, 14.29746914071037800, 92.91775706135236135 ) ) ;
#72018=CARTESIAN_POINT ( 'NONE',  ( 18.22780087662121673, 5.500000000000056843, 58.98459894673892023 ) ) ;
#72019=CARTESIAN_POINT ( 'NONE',  ( -5.719274019375665041, -21.55341960407619695, 99.79275706135234714 ) ) ;
#72020=CARTESIAN_POINT ( 'NONE',  ( 5.049401038297881783, 19.05341960407617563, 92.29275706135234714 ) ) ;
#72021=CARTESIAN_POINT ( 'NONE',  ( -13.89961937509957401, -13.97604488694547875, 59.37609039468566863 ) ) ;
#72022=CARTESIAN_POINT ( 'NONE',  ( -0.05219959533910754901, -16.53943276465976808, 62.49890960531436690 ) ) ;
#72023=CARTESIAN_POINT ( 'NONE',  ( 13.97604488694527802, 13.89961937509977652, 29.37390960531435979 ) ) ;
#72024=CARTESIAN_POINT ( 'NONE',  ( -9.474510206698720793, -16.51473224551083518, 64.58442372801900433 ) ) ;
#72026=CARTESIAN_POINT ( 'NONE',  ( -0.05219959533937732626, 21.53943276465977519, 67.50109039468568994 ) ) ;
#72027=CARTESIAN_POINT ( 'NONE',  ( 12.14591786802327356, -12.06949235617739191, 25.62609039468567929 ) ) ;
#72028=CARTESIAN_POINT ( 'NONE',  ( 16.20579543436677383, 7.371946100355107667, 83.06520834171875833 ) ) ;
#72029=CARTESIAN_POINT ( 'NONE',  ( -0.05219959533907301413, -21.53943276465977519, 27.49890960531435269 ) ) ;
#72030=CARTESIAN_POINT ( 'NONE',  ( 16.46253265017146816, 9.564922557961045513, 111.6677570613523329 ) ) ;
#72033=CARTESIAN_POINT ( 'NONE',  ( -19.02544592524342804, 5.153800228976336051, 26.04057627198103120 ) ) ;
#72034=CARTESIAN_POINT ( 'NONE',  ( -10.81492255796105439, 18.62759615963255655, 107.9177570613523471 ) ) ;
#72035=CARTESIAN_POINT ( 'NONE',  ( 16.46253265017160672, -9.564922557960803928, 43.33224293864769550 ) ) ;
#72036=CARTESIAN_POINT ( 'NONE',  ( -18.62759615963255300, -10.81492255796106328, 64.16775706135234714 ) ) ;
#72037=CARTESIAN_POINT ( 'NONE',  ( 5.823673210054444382, -21.52544592524334988, 105.2094237280190328 ) ) ;
#72038=CARTESIAN_POINT ( 'NONE',  ( -12.06949235617739369, -12.14591786802326823, 104.3760903946856899 ) ) ;
#72039=CARTESIAN_POINT ( 'NONE',  ( -19.05341960407611168, -5.049401038298163336, 81.45724293864769550 ) ) ;
#72040=CARTESIAN_POINT ( 'NONE',  ( -15.80617190586768217, 15.72974639402176855, 58.12609039468568994 ) ) ;
#72041=CARTESIAN_POINT ( 'NONE',  ( -0.05219959533937732626, 21.53943276465977519, 57.50109039468568994 ) ) ;
#72042=CARTESIAN_POINT ( 'NONE',  ( -13.97604488694547697, 13.89961937509957934, 73.12609039468568994 ) ) ;
#72043=CARTESIAN_POINT ( 'NONE',  ( 9.564922557960805705, 16.46253265017160317, 109.5822429386476955 ) ) ;
#72044=CARTESIAN_POINT ( 'NONE',  ( -16.46253265017160317, 9.564922557960807481, 25.83224293864769194 ) ) ;
#72045=CARTESIAN_POINT ( 'NONE',  ( -15.80617190586745835, -15.72974639402198527, 96.87390960531436690 ) ) ;
#72046=CARTESIAN_POINT ( 'NONE',  ( 19.02544592524334988, 5.153800228976608722, 26.45942372801899722 ) ) ;
#72047=CARTESIAN_POINT ( 'NONE',  ( -12.06949235617756955, 12.14591786802309770, 100.6239096053143811 ) ) ;
#72048=CARTESIAN_POINT ( 'NONE',  ( 13.89961937509977652, -13.97604488694527269, 48.12390960531435979 ) ) ;
#72049=CARTESIAN_POINT ( 'NONE',  ( 13.97604488694548053, -13.89961937509957401, 80.62609039468567573 ) ) ;
#72050=CARTESIAN_POINT ( 'NONE',  ( 4.483927247898545687, 16.52544592524342804, 59.79057627198103120 ) ) ;
#72051=CARTESIAN_POINT ( 'NONE',  ( -10.81492255796105439, 18.62759615963255655, 102.9177570613523756 ) ) ;
#72052=CARTESIAN_POINT ( 'NONE',  ( -5.049401038298153566, 19.05341960407611168, 110.2072429386476671 ) ) ;
#72053=CARTESIAN_POINT ( 'NONE',  ( 13.89961937509957401, 13.97604488694547697, 76.87609039468566152 ) ) ;
#72054=CARTESIAN_POINT ( 'NONE',  ( 0.05219959533907565091, 21.53943276465977519, 74.99890960531435269 ) ) ;
#72055=CARTESIAN_POINT ( 'NONE',  ( 15.72974639402176855, 15.80617190586768217, 36.87609039468568994 ) ) ;
#72056=CARTESIAN_POINT ( 'NONE',  ( 14.34966873604972726, -8.224510206698740333, 30.83442372801902209 ) ) ;
#72057=CARTESIAN_POINT ( 'NONE',  ( -14.34966873604972548, 8.224510206698743886, 88.33442372801901854 ) ) ;
#72058=CARTESIAN_POINT ( 'NONE',  ( -8.314922557961024197, 14.29746914071037800, 42.91775706135235424 ) ) ;
#72059=CARTESIAN_POINT ( 'NONE',  ( 5.719274019375673035, 21.55341960407619339, 42.29275706135235424 ) ) ;
#72060=CARTESIAN_POINT ( 'NONE',  ( 18.62759615963271287, -10.81492255796078972, 43.33224293864769550 ) ) ;
#72061=CARTESIAN_POINT ( 'NONE',  ( 5.153800228976335163, 19.02544592524342804, 34.79057627198102409 ) ) ;
#72063=CARTESIAN_POINT ( 'NONE',  ( 16.53943276465976808, 0.05219959533934440121, 66.25109039468567573 ) ) ;
#72065=CARTESIAN_POINT ( 'NONE',  ( 21.52544592524344225, -5.823673210054117533, 88.54057627198103830 ) ) ;
#72066=CARTESIAN_POINT ( 'NONE',  ( 16.55341960407611168, 4.379528057220329451, 43.95724293864769550 ) ) ;
#72067=CARTESIAN_POINT ( 'NONE',  ( -8.224510206698735004, -14.34966873604973081, 49.58442372801901143 ) ) ;
#72068=CARTESIAN_POINT ( 'NONE',  ( 13.97604488694527802, 13.89961937509977652, 54.37390960531435979 ) ) ;
#72069=CARTESIAN_POINT ( 'NONE',  ( -16.53943276465976808, -0.05219959533934237506, 88.75109039468567573 ) ) ;
#72070=CARTESIAN_POINT ( 'NONE',  ( -19.03943276465977164, -0.05219959533935918106, 83.75109039468567573 ) ) ;
#72071=CARTESIAN_POINT ( 'NONE',  ( 21.53943276465977519, -0.05219959533907433946, 88.74890960531436690 ) ) ;
#72072=CARTESIAN_POINT ( 'NONE',  ( 8.314922557960818139, 14.29746914071049879, 29.58224293864769905 ) ) ;
#72075=CARTESIAN_POINT ( 'NONE',  ( 5.823673210054125526, 21.52544592524343514, 54.79057627198104541 ) ) ;
#72076=VERTEX_POINT ( 'NONE', #173808 ) ;
#72077=CARTESIAN_POINT ( 'NONE',  ( -4.483927247898782831, 16.52544592524335698, 102.7094237280190185 ) ) ;
#72078=ORIENTED_EDGE ( 'NONE', *, *, #81519, .F. ) ;
#72079=CARTESIAN_POINT ( 'NONE',  ( 21.55341960407610458, 5.719274019375980345, 28.95724293864769905 ) ) ;
#72081=CARTESIAN_POINT ( 'NONE',  ( -21.52544592524343514, 5.823673210054127303, 91.04057627198103830 ) ) ;
#72082=CARTESIAN_POINT ( 'NONE',  ( -14.34966873604960291, -8.224510206698953496, 26.66557627198103475 ) ) ;
#72083=CARTESIAN_POINT ( 'NONE',  ( 4.379528057220092307, 16.55341960407617563, 37.29275706135235424 ) ) ;
#72084=CARTESIAN_POINT ( 'NONE',  ( 9.564922557960805705, 16.46253265017160317, 29.58224293864769550 ) ) ;
#72085=CARTESIAN_POINT ( 'NONE',  ( 8.314922557961029526, -14.29746914071037800, 30.41775706135234358 ) ) ;
#72086=CARTESIAN_POINT ( 'NONE',  ( -9.564922557960796823, -16.46253265017161027, 57.08224293864769550 ) ) ;
#72088=CARTESIAN_POINT ( 'NONE',  ( 5.153800228976335163, 19.02544592524342804, 109.7905762719810099 ) ) ;
#72089=CARTESIAN_POINT ( 'NONE',  ( 19.05341960407611168, 5.049401038298154454, 113.9572429386477097 ) ) ;
#72090=CARTESIAN_POINT ( 'NONE',  ( 12.06949235617739724, 12.14591786802326823, 101.8760903946857042 ) ) ;
#72091=CARTESIAN_POINT ( 'NONE',  ( -0.05219959533936034679, 19.03943276465977164, 87.50109039468567573 ) ) ;
#72092=CARTESIAN_POINT ( 'NONE',  ( 5.153800228976615827, -19.02544592524334988, 40.20942372801898301 ) ) ;
#72093=CARTESIAN_POINT ( 'NONE',  ( 0.05219959533907565091, 21.53943276465977519, 89.99890960531438111 ) ) ;
#72095=CARTESIAN_POINT ( 'NONE',  ( -14.34966873604960291, -8.224510206698953496, 21.66557627198102409 ) ) ;
#72096=AXIS2_PLACEMENT_3D ( 'NONE', #6544, #115744, #177431 ) ;
#72097=CARTESIAN_POINT ( 'NONE',  ( -15.72974639402197994, 15.80617190586746368, 35.62390960531437401 ) ) ;
#72098=CARTESIAN_POINT ( 'NONE',  ( 5.153800228976615827, -19.02544592524334988, 105.2094237280190185 ) ) ;
#72099=CARTESIAN_POINT ( 'NONE',  ( 13.97604488694527802, 13.89961937509977652, 109.3739096053143669 ) ) ;
#72100=CARTESIAN_POINT ( 'NONE',  ( 18.67979575497194134, -10.72451020669871369, 65.83442372801900433 ) ) ;
#72101=CARTESIAN_POINT ( 'NONE',  ( 0.05219959533909260263, 19.03943276465977164, 59.99890960531436690 ) ) ;
#72102=CARTESIAN_POINT ( 'NONE',  ( -8.224510206698948167, 14.34966873604960824, 95.41557627198102409 ) ) ;
#72104=CARTESIAN_POINT ( 'NONE',  ( 14.34966873604960469, 8.224510206698951720, 84.16557627198103830 ) ) ;
#72106=CARTESIAN_POINT ( 'NONE',  ( -13.89961937509957401, -13.97604488694547875, 94.37609039468566152 ) ) ;
#72108=CARTESIAN_POINT ( 'NONE',  ( -13.89961937509977652, 13.97604488694528158, 65.62390960531436690 ) ) ;
#72109=CARTESIAN_POINT ( 'NONE',  ( 16.36317988757097552, -7.306389748694710917, 71.59789608363172420 ) ) ;
#72110=CARTESIAN_POINT ( 'NONE',  ( 9.564922557960805705, 16.46253265017160317, 79.58224293864769550 ) ) ;
#72111=CARTESIAN_POINT ( 'NONE',  ( -16.46253265017160317, 9.564922557960807481, 100.8322429386477097 ) ) ;
#72112=CARTESIAN_POINT ( 'NONE',  ( 12.06949235617739724, 12.14591786802326823, 66.87609039468568994 ) ) ;
#72113=CARTESIAN_POINT ( 'NONE',  ( -17.13100169013299734, -6.664070546373170423, 49.23210164300151348 ) ) ;
#72115=CARTESIAN_POINT ( 'NONE',  ( 9.564922557961047289, -16.46253265017146816, 40.41775706135234003 ) ) ;
#72116=CARTESIAN_POINT ( 'NONE',  ( 15.80617190586769283, -15.72974639402175789, 95.62609039468568994 ) ) ;
#72118=CARTESIAN_POINT ( 'NONE',  ( -5.153800228976328057, -19.02544592524343514, 107.2905762719810383 ) ) ;
#72119=CARTESIAN_POINT ( 'NONE',  ( 16.53943276465976808, 0.05219959533934440121, 96.25109039468568994 ) ) ;
#72121=CARTESIAN_POINT ( 'NONE',  ( 12.06949235617739724, 12.14591786802326823, 96.87609039468568994 ) ) ;
#72123=CARTESIAN_POINT ( 'NONE',  ( -16.52544592524335698, -4.483927247898792601, 68.95942372801901854 ) ) ;
#72125=CARTESIAN_POINT ( 'NONE',  ( -18.62759615963255300, -10.81492255796106328, 84.16775706135234714 ) ) ;
#72126=CARTESIAN_POINT ( 'NONE',  ( -16.51473224551082808, 9.474510206698731452, 83.33442372801899012 ) ) ;
#72127=CARTESIAN_POINT ( 'NONE',  ( 16.46253265017146816, 9.564922557961045513, 21.66775706135233648 ) ) ;
#72128=CARTESIAN_POINT ( 'NONE',  ( -19.05341960407611168, -5.049401038298163336, 61.45724293864769550 ) ) ;
#72129=CARTESIAN_POINT ( 'NONE',  ( 19.05341960407611168, 5.049401038298154454, 43.95724293864769550 ) ) ;
#72131=CARTESIAN_POINT ( 'NONE',  ( 10.81492255796078972, 18.62759615963270932, 84.58224293864769550 ) ) ;
#72132=CARTESIAN_POINT ( 'NONE',  ( 18.62759615963271287, -10.81492255796078972, 38.33224293864768839 ) ) ;
#72133=CARTESIAN_POINT ( 'NONE',  ( 0.05219959533909260263, 19.03943276465977164, 29.99890960531435979 ) ) ;
#72134=CARTESIAN_POINT ( 'NONE',  ( 16.53943276465976808, 0.05219959533934440121, 56.25109039468568284 ) ) ;
#72136=CARTESIAN_POINT ( 'NONE',  ( -15.80617190586768217, 15.72974639402176855, 38.12609039468567573 ) ) ;
#72137=CARTESIAN_POINT ( 'NONE',  ( -16.53943276465976808, 0.05219959533911058130, 56.24890960531436690 ) ) ;
#72139=CARTESIAN_POINT ( 'NONE',  ( -12.14591786802326823, 12.06949235617739902, 23.12609039468567573 ) ) ;
#72140=CARTESIAN_POINT ( 'NONE',  ( -19.02544592524334988, -5.153800228976617603, 43.95942372801899012 ) ) ;
#72141=CARTESIAN_POINT ( 'NONE',  ( 12.14591786802309770, 12.06949235617756955, 64.37390960531435269 ) ) ;
#72142=CARTESIAN_POINT ( 'NONE',  ( -21.53943276465977519, -0.05219959533937600094, 18.75109039468568639 ) ) ;
#72144=CARTESIAN_POINT ( 'NONE',  ( 15.72974639402199770, -15.80617190586745480, 73.12390960531436690 ) ) ;
#72145=CARTESIAN_POINT ( 'NONE',  ( -19.05341960407611168, -5.049401038298163336, 86.45724293864769550 ) ) ;
#72146=CARTESIAN_POINT ( 'NONE',  ( -0.05219959533910754901, -16.53943276465976808, 67.49890960531436690 ) ) ;
#72147=CARTESIAN_POINT ( 'NONE',  ( 16.46253265017160672, -9.564922557960803928, 98.33224293864769550 ) ) ;
#72148=CARTESIAN_POINT ( 'NONE',  ( -18.22780087662119541, 5.500000000000102141, 46.01763182126894947 ) ) ;
#72149=CARTESIAN_POINT ( 'NONE',  ( -13.89961937509957401, -13.97604488694547875, 74.37609039468566152 ) ) ;
#72150=CARTESIAN_POINT ( 'NONE',  ( -0.05219959533907301413, -21.53943276465977519, 112.4989096053143669 ) ) ;
#72151=CARTESIAN_POINT ( 'NONE',  ( 9.474510206698971260, -16.51473224551069308, 62.91557627198102409 ) ) ;
#72152=CARTESIAN_POINT ( 'NONE',  ( -9.474510206698720793, -16.51473224551083518, 44.58442372801900433 ) ) ;
#72153=CARTESIAN_POINT ( 'NONE',  ( 0.05219959533909260263, 19.03943276465977164, 24.99890960531435269 ) ) ;
#72155=CARTESIAN_POINT ( 'NONE',  ( 18.62759615963255655, 10.81492255796105972, 66.66775706135234714 ) ) ;
#72156=CARTESIAN_POINT ( 'NONE',  ( -16.61371651742604172, -7.165104196376156587, 71.14584930007008268 ) ) ;
#72157=CARTESIAN_POINT ( 'NONE',  ( 8.314922557960818139, 14.29746914071049879, 39.58224293864769550 ) ) ;
#72158=CARTESIAN_POINT ( 'NONE',  ( -13.97604488694527625, -13.89961937509977652, 56.87390960531434558 ) ) ;
#72159=CARTESIAN_POINT ( 'NONE',  ( 21.55341960407610458, 5.719274019375980345, 68.95724293864769550 ) ) ;
#72161=CARTESIAN_POINT ( 'NONE',  ( -16.46253265017160317, 9.564922557960807481, 60.83224293864769550 ) ) ;
#72163=CARTESIAN_POINT ( 'NONE',  ( -0.05219959533907301413, -21.53943276465977519, 72.49890960531435269 ) ) ;
#72165=CARTESIAN_POINT ( 'NONE',  ( 21.52544592524334988, 5.823673210054432836, 106.4594237280190328 ) ) ;
#72167=CARTESIAN_POINT ( 'NONE',  ( -16.52544592524335698, -4.483927247898792601, 98.95942372801903275 ) ) ;
#72168=CARTESIAN_POINT ( 'NONE',  ( 16.52544592524342804, -4.483927247898539470, 78.54057627198103830 ) ) ;
#72169=CARTESIAN_POINT ( 'NONE',  ( -5.049401038298153566, 19.05341960407611168, 65.20724293864765286 ) ) ;
#72171=CARTESIAN_POINT ( 'NONE',  ( -19.02544592524334988, -5.153800228976617603, 33.95942372801897591 ) ) ;
#72172=CARTESIAN_POINT ( 'NONE',  ( 14.29746914071037800, 8.314922557961029526, 86.66775706135234714 ) ) ;
#72174=CARTESIAN_POINT ( 'NONE',  ( 13.97604488694548053, -13.89961937509957401, 35.62609039468567573 ) ) ;
#72175=CARTESIAN_POINT ( 'NONE',  ( 16.46253265017160672, -9.564922557960803928, 93.33224293864769550 ) ) ;
#72176=CARTESIAN_POINT ( 'NONE',  ( -5.719274019375978568, 21.55341960407610458, 55.20724293864770260 ) ) ;
#72178=CARTESIAN_POINT ( 'NONE',  ( -5.153800228976328057, -19.02544592524343514, 27.29057627198103120 ) ) ;
#72179=CARTESIAN_POINT ( 'NONE',  ( -15.80617190586768217, 15.72974639402176855, 98.12609039468570415 ) ) ;
#72180=CARTESIAN_POINT ( 'NONE',  ( 14.29746914071037800, 8.314922557961029526, 61.66775706135235424 ) ) ;
#72181=CARTESIAN_POINT ( 'NONE',  ( -21.53943276465977519, -0.05219959533937600094, 28.75109039468567929 ) ) ;
#72182=CARTESIAN_POINT ( 'NONE',  ( -16.52544592524335698, -4.483927247898792601, 23.95942372801901143 ) ) ;
#72183=CARTESIAN_POINT ( 'NONE',  ( 5.049401038298161559, -19.05341960407611168, 97.70724293864766707 ) ) ;
#72184=CARTESIAN_POINT ( 'NONE',  ( -19.05341960407611168, -5.049401038298163336, 41.45724293864769550 ) ) ;
#72185=CARTESIAN_POINT ( 'NONE',  ( -19.05341960407611168, -5.049401038298163336, 51.45724293864770260 ) ) ;
#72186=CARTESIAN_POINT ( 'NONE',  ( 4.379528057220092307, 16.55341960407617563, 37.29275706135235424 ) ) ;
#72187=CARTESIAN_POINT ( 'NONE',  ( -8.224510206698948167, 14.34966873604960824, 95.41557627198102409 ) ) ;
#72188=CARTESIAN_POINT ( 'NONE',  ( 16.55341960407618274, -4.379528057220086978, 101.0427570613523756 ) ) ;
#72189=CARTESIAN_POINT ( 'NONE',  ( -10.72451020669870658, -18.67979575497194134, 44.58442372801901854 ) ) ;
#72190=CARTESIAN_POINT ( 'NONE',  ( 0.05219959533909260263, 19.03943276465977164, 74.99890960531435269 ) ) ;
#72191=CARTESIAN_POINT ( 'NONE',  ( -19.02544592524342804, 5.153800228976336051, 46.04057627198101699 ) ) ;
#72192=CARTESIAN_POINT ( 'NONE',  ( -19.05341960407611168, -5.049401038298163336, 86.45724293864769550 ) ) ;
#72194=CARTESIAN_POINT ( 'NONE',  ( 14.29746914071049879, -8.314922557960816363, 33.33224293864769550 ) ) ;
#72195=CARTESIAN_POINT ( 'NONE',  ( 8.224510206698742110, 14.34966873604972548, 97.08442372801904696 ) ) ;
#72197=CARTESIAN_POINT ( 'NONE',  ( -19.05341960407617563, 5.049401038297882671, 43.54275706135232582 ) ) ;
#72198=CARTESIAN_POINT ( 'NONE',  ( 13.97604488694527802, 13.89961937509977652, 114.3739096053143669 ) ) ;
#72199=CARTESIAN_POINT ( 'NONE',  ( 19.02544592524343514, -5.153800228976328945, 53.54057627198102409 ) ) ;
#72200=CARTESIAN_POINT ( 'NONE',  ( 16.46253265017146816, 9.564922557961045513, 21.66775706135233648 ) ) ;
#72202=CARTESIAN_POINT ( 'NONE',  ( 4.379528057220092307, 16.55341960407617563, 37.29275706135235424 ) ) ;
#72203=CARTESIAN_POINT ( 'NONE',  ( 0.05219959533936267826, -19.03943276465977164, 75.00109039468566152 ) ) ;
#72204=CARTESIAN_POINT ( 'NONE',  ( 8.314922557961029526, -14.29746914071037800, 50.41775706135235424 ) ) ;
#72205=CARTESIAN_POINT ( 'NONE',  ( -9.474510206698964154, 16.51473224551069663, 115.4155762719810241 ) ) ;
#72206=CARTESIAN_POINT ( 'NONE',  ( 5.153800228976335163, 19.02544592524342804, 79.79057627198102409 ) ) ;
#72207=CARTESIAN_POINT ( 'NONE',  ( 21.52544592524334988, 5.823673210054432836, 21.45942372801901499 ) ) ;
#72208=CARTESIAN_POINT ( 'NONE',  ( -13.97604488694547697, 13.89961937509957934, 83.12609039468564731 ) ) ;
#72209=CARTESIAN_POINT ( 'NONE',  ( -5.049401038298153566, 19.05341960407611168, 105.2072429386476671 ) ) ;
#72210=CARTESIAN_POINT ( 'NONE',  ( -9.474510206698964154, 16.51473224551069663, 30.41557627198102054 ) ) ;
#72211=CARTESIAN_POINT ( 'NONE',  ( 0.05219959533909260263, 19.03943276465977164, 74.99890960531435269 ) ) ;
#72212=CARTESIAN_POINT ( 'NONE',  ( 16.53943276465976808, -0.05219959533910856209, 28.74890960531435624 ) ) ;
#72213=CARTESIAN_POINT ( 'NONE',  ( 5.153800228976335163, 19.02544592524342804, 34.79057627198102409 ) ) ;
#72214=CARTESIAN_POINT ( 'NONE',  ( -19.05341960407617563, 5.049401038297882671, 53.54275706135231871 ) ) ;
#72215=CARTESIAN_POINT ( 'NONE',  ( -12.14591786802309592, -12.06949235617757132, 76.87390960531439532 ) ) ;
#72216=CARTESIAN_POINT ( 'NONE',  ( 9.474510206698729675, 16.51473224551082808, 22.08442372801899722 ) ) ;
#72217=CARTESIAN_POINT ( 'NONE',  ( -5.049401038298153566, 19.05341960407611168, 50.20724293864770260 ) ) ;
#72218=CARTESIAN_POINT ( 'NONE',  ( 10.72451020669898902, -18.67979575497178502, 52.91557627198103830 ) ) ;
#72219=CARTESIAN_POINT ( 'NONE',  ( -16.53943276465976808, 0.05219959533911058130, 51.24890960531436690 ) ) ;
#72220=CARTESIAN_POINT ( 'NONE',  ( 15.80617190586769283, -15.72974639402175789, 100.6260903946857184 ) ) ;
#72221=CARTESIAN_POINT ( 'NONE',  ( 9.564922557960805705, 16.46253265017160317, 94.58224293864769550 ) ) ;
#72222=CARTESIAN_POINT ( 'NONE',  ( 13.97604488694527802, 13.89961937509977652, 114.3739096053143669 ) ) ;
#72223=CARTESIAN_POINT ( 'NONE',  ( -19.05341960407611168, -5.049401038298163336, 41.45724293864769550 ) ) ;
#72224=CARTESIAN_POINT ( 'NONE',  ( -8.224510206698948167, 14.34966873604960824, 115.4155762719810241 ) ) ;
#72225=CARTESIAN_POINT ( 'NONE',  ( 8.314922557960818139, 14.29746914071049879, 89.58224293864768129 ) ) ;
#72226=CARTESIAN_POINT ( 'NONE',  ( -21.53943276465977519, 0.05219959533907696930, 101.2489096053143669 ) ) ;
#72227=CARTESIAN_POINT ( 'NONE',  ( -13.89961937509977652, 13.97604488694528158, 85.62390960531433848 ) ) ;
#72228=CARTESIAN_POINT ( 'NONE',  ( 0.05219959533907565091, 21.53943276465977519, 114.9989096053143669 ) ) ;
#72229=CARTESIAN_POINT ( 'NONE',  ( -5.049401038298153566, 19.05341960407611168, 95.20724293864770971 ) ) ;
#72231=CARTESIAN_POINT ( 'NONE',  ( 12.14591786802309770, 12.06949235617756955, 104.3739096053143669 ) ) ;
#72232=CARTESIAN_POINT ( 'NONE',  ( 5.049401038298161559, -19.05341960407611168, 72.70724293864768129 ) ) ;
#72233=CARTESIAN_POINT ( 'NONE',  ( 0.05219959533907565091, 21.53943276465977519, 79.99890960531435269 ) ) ;
#72235=CARTESIAN_POINT ( 'NONE',  ( -18.62759615963270932, 10.81492255796079327, 25.83224293864769194 ) ) ;
#72237=CARTESIAN_POINT ( 'NONE',  ( -16.53943276465976808, -0.05219959533934237506, 33.75109039468568284 ) ) ;
#72238=CARTESIAN_POINT ( 'NONE',  ( -14.29746914071049879, 8.314922557960819915, 100.8322429386477097 ) ) ;
#72239=CARTESIAN_POINT ( 'NONE',  ( -17.49999999999999645, -5.500000000000000000, 111.2823096230356725 ) ) ;
#72240=CARTESIAN_POINT ( 'NONE',  ( 5.049401038298161559, -19.05341960407611168, 82.70724293864770971 ) ) ;
#72241=CARTESIAN_POINT ( 'NONE',  ( 19.03943276465977164, -0.05219959533909143690, 43.74890960531435979 ) ) ;
#72242=CARTESIAN_POINT ( 'NONE',  ( 16.55341960407611168, 4.379528057220329451, 73.95724293864769550 ) ) ;
#72243=CARTESIAN_POINT ( 'NONE',  ( -21.52544592524343514, 5.823673210054127303, 36.04057627198102409 ) ) ;
#72244=CARTESIAN_POINT ( 'NONE',  ( 16.52544592524342804, -4.483927247898539470, 53.54057627198103120 ) ) ;
#72245=CARTESIAN_POINT ( 'NONE',  ( -19.05341960407617563, 5.049401038297882671, 108.5427570613523187 ) ) ;
#72246=CARTESIAN_POINT ( 'NONE',  ( 15.72974639402176855, 15.80617190586768217, 71.87609039468568994 ) ) ;
#72248=CARTESIAN_POINT ( 'NONE',  ( 5.153800228976335163, 19.02544592524342804, 109.7905762719810099 ) ) ;
#72249=CARTESIAN_POINT ( 'NONE',  ( -4.483927247898782831, 16.52544592524335698, 87.70942372801901854 ) ) ;
#72250=CARTESIAN_POINT ( 'NONE',  ( -17.40805194821983548, 6.112264579160783917, 95.83371272510609629 ) ) ;
#72251=CARTESIAN_POINT ( 'NONE',  ( 5.049401038298161559, -19.05341960407611168, 72.70724293864768129 ) ) ;
#72252=CARTESIAN_POINT ( 'NONE',  ( 15.80617190586746368, 15.72974639402197994, 79.37390960531436690 ) ) ;
#72253=CARTESIAN_POINT ( 'NONE',  ( -8.224510206698735004, -14.34966873604973081, 24.58442372801901499 ) ) ;
#72254=CARTESIAN_POINT ( 'NONE',  ( -8.314922557960811034, -14.29746914071050412, 52.08224293864768839 ) ) ;
#72255=CARTESIAN_POINT ( 'NONE',  ( -5.719274019375665041, -21.55341960407619695, 74.79275706135234714 ) ) ;
#72256=CARTESIAN_POINT ( 'NONE',  ( -12.06949235617739369, -12.14591786802326823, 84.37609039468570415 ) ) ;
#72257=CARTESIAN_POINT ( 'NONE',  ( -21.52544592524343514, 5.823673210054127303, 26.04057627198103475 ) ) ;
#72258=CARTESIAN_POINT ( 'NONE',  ( -19.03943276465977164, 0.05219959533909376836, 116.2489096053143669 ) ) ;
#72260=CARTESIAN_POINT ( 'NONE',  ( 0.05219959533934541429, -16.53943276465976808, 110.0010903946856757 ) ) ;
#72261=CARTESIAN_POINT ( 'NONE',  ( -4.379528057220086978, -16.55341960407618274, 54.79275706135235424 ) ) ;
#72262=CARTESIAN_POINT ( 'NONE',  ( 13.89961937509977652, -13.97604488694527269, 78.12390960531433848 ) ) ;
#72264=CARTESIAN_POINT ( 'NONE',  ( 13.97604488694527802, 13.89961937509977652, 84.37390960531433848 ) ) ;
#72265=CARTESIAN_POINT ( 'NONE',  ( -18.67979575497193778, 10.72451020669871902, 73.33442372801901854 ) ) ;
#72266=CARTESIAN_POINT ( 'NONE',  ( -14.34966873604972548, 8.224510206698743886, 73.33442372801901854 ) ) ;
#72267=CARTESIAN_POINT ( 'NONE',  ( -0.05219959533910754901, -16.53943276465976808, 52.49890960531435979 ) ) ;
#72268=CARTESIAN_POINT ( 'NONE',  ( 19.03943276465977164, -0.05219959533909143690, 48.74890960531435979 ) ) ;
#72269=CARTESIAN_POINT ( 'NONE',  ( 13.97604488694527802, 13.89961937509977652, 49.37390960531434558 ) ) ;
#72270=ORIENTED_EDGE ( 'NONE', *, *, #115041, .F. ) ;
#72271=CARTESIAN_POINT ( 'NONE',  ( 13.97604488694548053, -13.89961937509957401, 90.62609039468567573 ) ) ;
#72272=CARTESIAN_POINT ( 'NONE',  ( 16.52544592524342804, -4.483927247898539470, 93.54057627198103830 ) ) ;
#72273=CARTESIAN_POINT ( 'NONE',  ( 13.97604488694527802, 13.89961937509977652, 59.37390960531434558 ) ) ;
#72274=CARTESIAN_POINT ( 'NONE',  ( -16.46253265017146816, -9.564922557961047289, 94.16775706135233293 ) ) ;
#72276=CARTESIAN_POINT ( 'NONE',  ( -18.62759615963255300, -10.81492255796106328, 109.1677570613523613 ) ) ;
#72277=CARTESIAN_POINT ( 'NONE',  ( 12.06949235617739724, 12.14591786802326823, 66.87609039468568994 ) ) ;
#72278=CARTESIAN_POINT ( 'NONE',  ( -5.153800228976607833, 19.02544592524334988, 87.70942372801897591 ) ) ;
#72279=CARTESIAN_POINT ( 'NONE',  ( 21.52544592524344225, -5.823673210054117533, 68.54057627198103830 ) ) ;
#72280=CARTESIAN_POINT ( 'NONE',  ( -0.05219959533934338120, 16.53943276465976808, 52.50109039468567573 ) ) ;
#72282=CARTESIAN_POINT ( 'NONE',  ( -19.02544592524334988, -5.153800228976617603, 53.95942372801898301 ) ) ;
#72283=CARTESIAN_POINT ( 'NONE',  ( -21.55341960407619339, 5.719274019375674811, 98.54275706135234714 ) ) ;
#72284=CARTESIAN_POINT ( 'NONE',  ( -16.53943276465976808, 0.05219959533911058130, 111.2489096053143669 ) ) ;
#72285=CARTESIAN_POINT ( 'NONE',  ( -19.02544592524342804, 5.153800228976336051, 66.04057627198103830 ) ) ;
#72286=CARTESIAN_POINT ( 'NONE',  ( -16.52544592524342804, 4.483927247898546575, 61.04057627198103120 ) ) ;
#72287=CARTESIAN_POINT ( 'NONE',  ( -5.823673210054431948, 21.52544592524334988, 87.70942372801901854 ) ) ;
#72288=CARTESIAN_POINT ( 'NONE',  ( 5.049401038297881783, 19.05341960407617563, 52.29275706135234003 ) ) ;
#72289=CARTESIAN_POINT ( 'NONE',  ( -13.97604488694547697, 13.89961937509957934, 28.12609039468565797 ) ) ;
#72290=CARTESIAN_POINT ( 'NONE',  ( -10.81492255796078084, -18.62759615963271287, 27.08224293864769550 ) ) ;
#72291=CARTESIAN_POINT ( 'NONE',  ( 10.81492255796106328, -18.62759615963255655, 100.4177570613523471 ) ) ;
#72292=CARTESIAN_POINT ( 'NONE',  ( 16.51473224551069308, 9.474510206698969483, 79.16557627198103830 ) ) ;
#72293=CARTESIAN_POINT ( 'NONE',  ( -18.67979575497193778, 10.72451020669871902, 98.33442372801901854 ) ) ;
#72294=CARTESIAN_POINT ( 'NONE',  ( 21.53943276465977519, -0.05219959533907433946, 53.74890960531437401 ) ) ;
#72295=CARTESIAN_POINT ( 'NONE',  ( 13.97604488694527802, 13.89961937509977652, 89.37390960531436690 ) ) ;
#72296=CARTESIAN_POINT ( 'NONE',  ( 9.564922557961047289, -16.46253265017146816, 60.41775706135233293 ) ) ;
#72297=CARTESIAN_POINT ( 'NONE',  ( -9.564922557960796823, -16.46253265017161027, 42.08224293864769550 ) ) ;
#72298=CARTESIAN_POINT ( 'NONE',  ( 19.03943276465977164, -0.05219959533909143690, 88.74890960531436690 ) ) ;
#72299=EDGE_CURVE ( 'NONE', #29646, #44580, #3071, .T. ) ;
#72300=CARTESIAN_POINT ( 'NONE',  ( 19.05341960407617918, -5.049401038297876454, 86.04275706135233293 ) ) ;
#72301=CARTESIAN_POINT ( 'NONE',  ( 12.14591786802327356, -12.06949235617739191, 45.62609039468567573 ) ) ;
#72302=CARTESIAN_POINT ( 'NONE',  ( -8.224510206698948167, 14.34966873604960824, 100.4155762719810241 ) ) ;
#72303=CARTESIAN_POINT ( 'NONE',  ( -19.03943276465977164, 0.05219959533909376836, 71.24890960531435269 ) ) ;
#72304=CARTESIAN_POINT ( 'NONE',  ( -18.62759615963270932, 10.81492255796079327, 50.83224293864770971 ) ) ;
#72305=CARTESIAN_POINT ( 'NONE',  ( -19.02544592524334988, -5.153800228976617603, 108.9594237280189759 ) ) ;
#72306=CARTESIAN_POINT ( 'NONE',  ( -18.67979575497193778, 10.72451020669871902, 23.33442372801901499 ) ) ;
#72307=CARTESIAN_POINT ( 'NONE',  ( 21.52544592524334988, 5.823673210054432836, 76.45942372801901854 ) ) ;
#72308=CARTESIAN_POINT ( 'NONE',  ( -4.483927247898782831, 16.52544592524335698, 77.70942372801900433 ) ) ;
#72310=CARTESIAN_POINT ( 'NONE',  ( -5.153800228976328057, -19.02544592524343514, 72.29057627198102409 ) ) ;
#72311=CARTESIAN_POINT ( 'NONE',  ( 4.483927247898790824, -16.52544592524335698, 100.2094237280190043 ) ) ;
#72312=CARTESIAN_POINT ( 'NONE',  ( -13.89961937509957401, -13.97604488694547875, 44.37609039468566863 ) ) ;
#72313=CARTESIAN_POINT ( 'NONE',  ( 5.823673210054444382, -21.52544592524334988, 35.20942372801901854 ) ) ;
#72315=CARTESIAN_POINT ( 'NONE',  ( -4.379528057220328563, 16.55341960407611168, 85.20724293864770971 ) ) ;
#72316=CARTESIAN_POINT ( 'NONE',  ( -13.89961937509977652, 13.97604488694528158, 105.6239096053143527 ) ) ;
#72317=CARTESIAN_POINT ( 'NONE',  ( -16.53943276465976808, -0.05219959533934237506, 88.75109039468567573 ) ) ;
#72318=CARTESIAN_POINT ( 'NONE',  ( -15.72974639402176322, -15.80617190586768395, 69.37609039468567573 ) ) ;
#72319=CARTESIAN_POINT ( 'NONE',  ( -16.53943276465976808, -0.05219959533934237506, 33.75109039468568284 ) ) ;
#72320=CARTESIAN_POINT ( 'NONE',  ( 15.72974639402176855, 15.80617190586768217, 31.87609039468567929 ) ) ;
#72321=CARTESIAN_POINT ( 'NONE',  ( 14.34966873604960469, 8.224510206698951720, 74.16557627198102409 ) ) ;
#72323=CARTESIAN_POINT ( 'NONE',  ( -18.67979575497178146, -10.72451020669898902, 96.66557627198102409 ) ) ;
#72324=CARTESIAN_POINT ( 'NONE',  ( 8.314922557960818139, 14.29746914071049879, 54.58224293864769550 ) ) ;
#72325=ORIENTED_EDGE ( 'NONE', *, *, #172057, .T. ) ;
#72326=CARTESIAN_POINT ( 'NONE',  ( 0.05219959533909260263, 19.03943276465977164, 29.99890960531435979 ) ) ;
#72327=CARTESIAN_POINT ( 'NONE',  ( 5.823673210054125526, 21.52544592524343514, 34.79057627198103120 ) ) ;
#72328=CARTESIAN_POINT ( 'NONE',  ( -0.05219959533937732626, 21.53943276465977519, 32.50109039468568284 ) ) ;
#72329=CARTESIAN_POINT ( 'NONE',  ( -16.53943276465976808, 0.05219959533911058130, 66.24890960531436690 ) ) ;
#72331=CARTESIAN_POINT ( 'NONE',  ( 21.55341960407610458, 5.719274019375980345, 68.95724293864769550 ) ) ;
#72332=CARTESIAN_POINT ( 'NONE',  ( 9.564922557960805705, 16.46253265017160317, 74.58224293864769550 ) ) ;
#72333=CARTESIAN_POINT ( 'NONE',  ( -19.02544592524342804, 5.153800228976336051, 26.04057627198103120 ) ) ;
#72334=CARTESIAN_POINT ( 'NONE',  ( -13.89961937509957401, -13.97604488694547875, 84.37609039468567573 ) ) ;
#72335=CARTESIAN_POINT ( 'NONE',  ( 10.81492255796078972, 18.62759615963270932, 59.58224293864770260 ) ) ;
#72336=CARTESIAN_POINT ( 'NONE',  ( -19.05341960407611168, -5.049401038298163336, 41.45724293864769550 ) ) ;
#72337=CARTESIAN_POINT ( 'NONE',  ( 19.05341960407611168, 5.049401038298154454, 73.95724293864768129 ) ) ;
#72339=CARTESIAN_POINT ( 'NONE',  ( -8.224510206698735004, -14.34966873604973081, 54.58442372801901143 ) ) ;
#72340=CARTESIAN_POINT ( 'NONE',  ( 5.719274019375673035, 21.55341960407619339, 27.29275706135234358 ) ) ;
#72342=CARTESIAN_POINT ( 'NONE',  ( -21.55341960407619339, 5.719274019375674811, 53.54275706135234714 ) ) ;
#72343=CARTESIAN_POINT ( 'NONE',  ( 13.89961937509977652, -13.97604488694527269, 98.12390960531433848 ) ) ;
#72344=CARTESIAN_POINT ( 'NONE',  ( 10.81492255796078972, 18.62759615963270932, 69.58224293864769550 ) ) ;
#72345=CARTESIAN_POINT ( 'NONE',  ( 15.80617190586746368, 15.72974639402197994, 114.3739096053143527 ) ) ;
#72346=CARTESIAN_POINT ( 'NONE',  ( 0.05219959533934541429, -16.53943276465976808, 50.00109039468568994 ) ) ;
#72347=CARTESIAN_POINT ( 'NONE',  ( 18.67979575497178502, 10.72451020669898547, 49.16557627198102409 ) ) ;
#72348=CARTESIAN_POINT ( 'NONE',  ( -21.55341960407619339, 5.719274019375674811, 108.5427570613523756 ) ) ;
#72349=CARTESIAN_POINT ( 'NONE',  ( -16.46253265017160317, 9.564922557960807481, 55.83224293864769550 ) ) ;
#72350=CARTESIAN_POINT ( 'NONE',  ( -13.89961937509977652, 13.97604488694528158, 110.6239096053143243 ) ) ;
#72351=CARTESIAN_POINT ( 'NONE',  ( -16.46253265017160317, 9.564922557960807481, 75.83224293864769550 ) ) ;
#72353=CARTESIAN_POINT ( 'NONE',  ( -19.03943276465977164, -0.05219959533935918106, 73.75109039468566152 ) ) ;
#72354=CARTESIAN_POINT ( 'NONE',  ( -13.89961937509957401, -13.97604488694547875, 19.37609039468566507 ) ) ;
#72355=CARTESIAN_POINT ( 'NONE',  ( -15.72974639402197994, 15.80617190586746368, 40.62390960531435269 ) ) ;
#72356=CARTESIAN_POINT ( 'NONE',  ( -0.05219959533934338120, 16.53943276465976808, 102.5010903946856899 ) ) ;
#72357=CARTESIAN_POINT ( 'NONE',  ( -9.564922557961040184, 16.46253265017147172, 82.91775706135233293 ) ) ;
#72358=CARTESIAN_POINT ( 'NONE',  ( -17.49999999999999645, 5.624438216177593652, 60.81670344914646620 ) ) ;
#72359=CARTESIAN_POINT ( 'NONE',  ( 16.51473224551083163, -9.474510206698727899, 25.83442372801900078 ) ) ;
#72360=CARTESIAN_POINT ( 'NONE',  ( -19.03943276465977164, -0.05219959533935918106, 83.75109039468567573 ) ) ;
#72361=CARTESIAN_POINT ( 'NONE',  ( 5.153800228976615827, -19.02544592524334988, 45.20942372801901143 ) ) ;
#72362=CARTESIAN_POINT ( 'NONE',  ( -17.48847506799968698, -5.747544572773811034, 44.17302562156721280 ) ) ;
#72363=CARTESIAN_POINT ( 'NONE',  ( -19.02544592524342804, 5.153800228976336051, 41.04057627198103120 ) ) ;
#72364=CARTESIAN_POINT ( 'NONE',  ( -0.05219959533910754901, -16.53943276465976808, 52.49890960531435979 ) ) ;
#72365=CARTESIAN_POINT ( 'NONE',  ( -19.03943276465977164, 0.05219959533909376836, 36.24890960531436690 ) ) ;
#72366=CARTESIAN_POINT ( 'NONE',  ( 0.05219959533910956823, 16.53943276465976808, 44.99890960531435979 ) ) ;
#72367=CARTESIAN_POINT ( 'NONE',  ( 17.97182807773875979, -5.499999999999868550, 46.03038844047287625 ) ) ;
#72368=CARTESIAN_POINT ( 'NONE',  ( -12.14591786802309592, -12.06949235617757132, 21.87390960531436690 ) ) ;
#72369=CARTESIAN_POINT ( 'NONE',  ( -9.474510206698964154, 16.51473224551069663, 55.41557627198103120 ) ) ;
#72370=CARTESIAN_POINT ( 'NONE',  ( 5.049401038297881783, 19.05341960407617563, 27.29275706135232937 ) ) ;
#72371=CARTESIAN_POINT ( 'NONE',  ( -0.05219959533934338120, 16.53943276465976808, 37.50109039468568284 ) ) ;
#72372=CARTESIAN_POINT ( 'NONE',  ( 18.67979575497178502, 10.72451020669898547, 39.16557627198102409 ) ) ;
#72373=CARTESIAN_POINT ( 'NONE',  ( 5.719274019375673035, 21.55341960407619339, 97.29275706135234714 ) ) ;
#72374=ORIENTED_EDGE ( 'NONE', *, *, #155151, .F. ) ;
#72375=CARTESIAN_POINT ( 'NONE',  ( -16.51473224551069308, -9.474510206698971260, 111.6655762719810383 ) ) ;
#72376=CARTESIAN_POINT ( 'NONE',  ( -16.46253265017160317, 9.564922557960807481, 100.8322429386477097 ) ) ;
#72378=CARTESIAN_POINT ( 'NONE',  ( -21.52544592524334988, -5.823673210054445271, 18.95942372801901143 ) ) ;
#72379=CARTESIAN_POINT ( 'NONE',  ( -14.34966873604960291, -8.224510206698953496, 76.66557627198103830 ) ) ;
#72380=CARTESIAN_POINT ( 'NONE',  ( -10.81492255796078084, -18.62759615963271287, 77.08224293864769550 ) ) ;
#72381=CARTESIAN_POINT ( 'NONE',  ( -19.03943276465977164, 0.05219959533909376836, 66.24890960531436690 ) ) ;
#72382=CARTESIAN_POINT ( 'NONE',  ( 16.51473224551069308, 9.474510206698969483, 79.16557627198103830 ) ) ;
#72383=CARTESIAN_POINT ( 'NONE',  ( -18.67979575497178146, -10.72451020669898902, 106.6655762719810383 ) ) ;
#72385=CARTESIAN_POINT ( 'NONE',  ( -16.46253265017160317, 9.564922557960807481, 55.83224293864769550 ) ) ;
#72387=CARTESIAN_POINT ( 'NONE',  ( 4.379528057220339221, -16.55341960407611168, 102.7072429386476955 ) ) ;
#72389=CARTESIAN_POINT ( 'NONE',  ( 13.89961937509977652, -13.97604488694527269, 58.12390960531436690 ) ) ;
#72390=CARTESIAN_POINT ( 'NONE',  ( 16.46253265017146816, 9.564922557961045513, 86.66775706135233293 ) ) ;
#72391=CARTESIAN_POINT ( 'NONE',  ( 14.29746914071049879, -8.314922557960816363, 98.33224293864769550 ) ) ;
#72392=CARTESIAN_POINT ( 'NONE',  ( 10.81492255796106328, -18.62759615963255655, 60.41775706135235424 ) ) ;
#72393=CARTESIAN_POINT ( 'NONE',  ( 9.564922557960805705, 16.46253265017160317, 54.58224293864769550 ) ) ;
#72394=CARTESIAN_POINT ( 'NONE',  ( 18.67979575497194134, -10.72451020669871369, 20.83442372801901143 ) ) ;
#72395=CARTESIAN_POINT ( 'NONE',  ( -14.34966873604960291, -8.224510206698953496, 101.6655762719810383 ) ) ;
#72397=CARTESIAN_POINT ( 'NONE',  ( -0.05219959533909027116, -19.03943276465977164, 77.49890960531435269 ) ) ;
#72399=CARTESIAN_POINT ( 'NONE',  ( -5.153800228976607833, 19.02544592524334988, 107.7094237280189759 ) ) ;
#72400=CARTESIAN_POINT ( 'NONE',  ( -21.55341960407610458, -5.719274019375992779, 31.45724293864769550 ) ) ;
#72401=CARTESIAN_POINT ( 'NONE',  ( -15.80617190586768217, 15.72974639402176855, 48.12609039468568284 ) ) ;
#72402=CARTESIAN_POINT ( 'NONE',  ( -19.03943276465977164, 0.05219959533909376836, 91.24890960531436690 ) ) ;
#72403=CARTESIAN_POINT ( 'NONE',  ( -13.89961937509957401, -13.97604488694547875, 89.37609039468563310 ) ) ;
#72404=CARTESIAN_POINT ( 'NONE',  ( -19.03943276465977164, 0.05219959533909376836, 66.24890960531436690 ) ) ;
#72405=CARTESIAN_POINT ( 'NONE',  ( -12.06949235617756955, 12.14591786802309770, 85.62390960531436690 ) ) ;
#72406=CARTESIAN_POINT ( 'NONE',  ( -5.153800228976328057, -19.02544592524343514, 107.2905762719810383 ) ) ;
#72407=CARTESIAN_POINT ( 'NONE',  ( -12.06949235617756955, 12.14591786802309770, 75.62390960531439532 ) ) ;
#72408=CARTESIAN_POINT ( 'NONE',  ( 13.89961937509977652, -13.97604488694527269, 98.12390960531433848 ) ) ;
#72409=CARTESIAN_POINT ( 'NONE',  ( 13.97604488694548053, -13.89961937509957401, 50.62609039468566152 ) ) ;
#72410=CARTESIAN_POINT ( 'NONE',  ( -19.05341960407611168, -5.049401038298163336, 46.45724293864768129 ) ) ;
#72411=CARTESIAN_POINT ( 'NONE',  ( 8.314922557960818139, 14.29746914071049879, 39.58224293864769550 ) ) ;
#72412=CARTESIAN_POINT ( 'NONE',  ( -5.153800228976328057, -19.02544592524343514, 27.29057627198103120 ) ) ;
#72413=ORIENTED_EDGE ( 'NONE', *, *, #173531, .F. ) ;
#72414=CARTESIAN_POINT ( 'NONE',  ( 18.67979575497194134, -10.72451020669871369, 50.83442372801901143 ) ) ;
#72415=CARTESIAN_POINT ( 'NONE',  ( 19.02544592524334988, 5.153800228976608722, 76.45942372801897591 ) ) ;
#72416=CARTESIAN_POINT ( 'NONE',  ( 16.55341960407611168, 4.379528057220329451, 48.95724293864770971 ) ) ;
#72417=CARTESIAN_POINT ( 'NONE',  ( -5.719274019375978568, 21.55341960407610458, 100.2072429386476955 ) ) ;
#72418=CARTESIAN_POINT ( 'NONE',  ( 18.67979575497178502, 10.72451020669898547, 39.16557627198102409 ) ) ;
#72419=CARTESIAN_POINT ( 'NONE',  ( -4.379528057220328563, 16.55341960407611168, 80.20724293864769550 ) ) ;
#72420=CARTESIAN_POINT ( 'NONE',  ( 19.03943276465977164, -0.05219959533909143690, 48.74890960531435979 ) ) ;
#72421=CARTESIAN_POINT ( 'NONE',  ( -14.34966873604972548, 8.224510206698743886, 113.3344237280190328 ) ) ;
#72422=CARTESIAN_POINT ( 'NONE',  ( 8.224510206698742110, 14.34966873604972548, 87.08442372801901854 ) ) ;
#72423=CARTESIAN_POINT ( 'NONE',  ( 4.483927247898790824, -16.52544592524335698, 65.20942372801901854 ) ) ;
#72424=CARTESIAN_POINT ( 'NONE',  ( 19.02544592524334988, 5.153800228976608722, 26.45942372801899722 ) ) ;
#72425=CARTESIAN_POINT ( 'NONE',  ( -13.89961937509977652, 13.97604488694528158, 95.62390960531436690 ) ) ;
#72426=CARTESIAN_POINT ( 'NONE',  ( 9.564922557960805705, 16.46253265017160317, 79.58224293864769550 ) ) ;
#72427=CARTESIAN_POINT ( 'NONE',  ( -8.314922557961024197, 14.29746914071037800, 72.91775706135234714 ) ) ;
#72428=CARTESIAN_POINT ( 'NONE',  ( -13.89961937509977652, 13.97604488694528158, 35.62390960531435269 ) ) ;
#72429=CARTESIAN_POINT ( 'NONE',  ( 4.379528057220339221, -16.55341960407611168, 52.70724293864769550 ) ) ;
#72430=CARTESIAN_POINT ( 'NONE',  ( 16.51473224551069308, 9.474510206698969483, 114.1655762719810241 ) ) ;
#72431=CARTESIAN_POINT ( 'NONE',  ( 19.03943276465977164, -0.05219959533909143690, 108.7489096053143527 ) ) ;
#72432=CARTESIAN_POINT ( 'NONE',  ( -15.72974639402197994, 15.80617190586746368, 30.62390960531436335 ) ) ;
#72435=CARTESIAN_POINT ( 'NONE',  ( 4.379528057220339221, -16.55341960407611168, 72.70724293864769550 ) ) ;
#72436=CARTESIAN_POINT ( 'NONE',  ( -12.06949235617756955, 12.14591786802309770, 70.62390960531436690 ) ) ;
#72439=CARTESIAN_POINT ( 'NONE',  ( -19.05341960407617563, 5.049401038297882671, 68.54275706135230450 ) ) ;
#72440=CARTESIAN_POINT ( 'NONE',  ( 13.97604488694527802, 13.89961937509977652, 84.37390960531433848 ) ) ;
#72441=CARTESIAN_POINT ( 'NONE',  ( 0.05219959533936267826, -19.03943276465977164, 75.00109039468566152 ) ) ;
#72442=CARTESIAN_POINT ( 'NONE',  ( -5.049401038297874678, -19.05341960407618274, 94.79275706135233293 ) ) ;
#72443=CARTESIAN_POINT ( 'NONE',  ( -12.06949235617739369, -12.14591786802326823, 19.37609039468568639 ) ) ;
#72444=CARTESIAN_POINT ( 'NONE',  ( 16.53943276465976808, 0.05219959533934440121, 96.25109039468568994 ) ) ;
#72446=CARTESIAN_POINT ( 'NONE',  ( 16.51473224551069308, 9.474510206698969483, 39.16557627198103120 ) ) ;
#72447=CARTESIAN_POINT ( 'NONE',  ( -0.05219959533909027116, -19.03943276465977164, 112.4989096053143669 ) ) ;
#72448=CARTESIAN_POINT ( 'NONE',  ( -5.719274019375665041, -21.55341960407619695, 54.79275706135235424 ) ) ;
#72449=CARTESIAN_POINT ( 'NONE',  ( -16.52544592524335698, -4.483927247898792601, 23.95942372801901143 ) ) ;
#72451=CARTESIAN_POINT ( 'NONE',  ( -13.97604488694527625, -13.89961937509977652, 76.87390960531433848 ) ) ;
#72452=CARTESIAN_POINT ( 'NONE',  ( -19.02544592524342804, 5.153800228976336051, 116.0405762719810383 ) ) ;
#72453=CARTESIAN_POINT ( 'NONE',  ( -4.483927247898539470, -16.52544592524342804, 77.29057627198102409 ) ) ;
#72454=CARTESIAN_POINT ( 'NONE',  ( 9.564922557960805705, 16.46253265017160317, 74.58224293864769550 ) ) ;
#72456=CARTESIAN_POINT ( 'NONE',  ( 13.89961937509977652, -13.97604488694527269, 73.12390960531436690 ) ) ;
#72458=CARTESIAN_POINT ( 'NONE',  ( -16.51473224551082808, 9.474510206698731452, 93.33442372801900433 ) ) ;
#72459=CARTESIAN_POINT ( 'NONE',  ( 18.62759615963271287, -10.81492255796078972, 68.33224293864769550 ) ) ;
#72460=CARTESIAN_POINT ( 'NONE',  ( -5.049401038298153566, 19.05341960407611168, 35.20724293864768839 ) ) ;
#72461=CARTESIAN_POINT ( 'NONE',  ( 9.474510206698729675, 16.51473224551082808, 62.08442372801899722 ) ) ;
#72462=CARTESIAN_POINT ( 'NONE',  ( 19.02544592524343514, -5.153800228976328945, 53.54057627198102409 ) ) ;
#72463=CARTESIAN_POINT ( 'NONE',  ( -13.97604488694527625, -13.89961937509977652, 91.87390960531432427 ) ) ;
#72466=CARTESIAN_POINT ( 'NONE',  ( 5.823673210054125526, 21.52544592524343514, 89.79057627198103830 ) ) ;
#72467=CARTESIAN_POINT ( 'NONE',  ( -12.06949235617756955, 12.14591786802309770, 95.62390960531436690 ) ) ;
#72468=CARTESIAN_POINT ( 'NONE',  ( 9.474510206698729675, 16.51473224551082808, 52.08442372801900433 ) ) ;
#72469=CARTESIAN_POINT ( 'NONE',  ( -15.72974639402197994, 15.80617190586746368, 85.62390960531436690 ) ) ;
#72470=CARTESIAN_POINT ( 'NONE',  ( -15.80617190586745835, -15.72974639402198527, 71.87390960531438111 ) ) ;
#72471=CARTESIAN_POINT ( 'NONE',  ( 12.06949235617757843, -12.14591786802309237, 38.12390960531436690 ) ) ;
#72472=CARTESIAN_POINT ( 'NONE',  ( 5.823673210054444382, -21.52544592524334988, 110.2094237280190185 ) ) ;
#72473=CARTESIAN_POINT ( 'NONE',  ( -16.46253265017160317, 9.564922557960807481, 75.83224293864769550 ) ) ;
#72474=CARTESIAN_POINT ( 'NONE',  ( -9.474510206698964154, 16.51473224551069663, 35.41557627198102409 ) ) ;
#72476=CARTESIAN_POINT ( 'NONE',  ( 15.80617190586769283, -15.72974639402175789, 35.62609039468568994 ) ) ;
#72477=CARTESIAN_POINT ( 'NONE',  ( -15.80617190586768217, 15.72974639402176855, 58.12609039468568994 ) ) ;
#72478=CARTESIAN_POINT ( 'NONE',  ( -19.05341960407611168, -5.049401038298163336, 41.45724293864769550 ) ) ;
#72479=CARTESIAN_POINT ( 'NONE',  ( -0.05219959533937732626, 21.53943276465977519, 22.50109039468567573 ) ) ;
#72480=CARTESIAN_POINT ( 'NONE',  ( -5.049401038297874678, -19.05341960407617918, 54.79275706135234003 ) ) ;
#72481=CARTESIAN_POINT ( 'NONE',  ( 9.474510206698971260, -16.51473224551069308, 37.91557627198102409 ) ) ;
#72482=CARTESIAN_POINT ( 'NONE',  ( -16.55341960407617563, 4.379528057220093196, 23.54275706135235424 ) ) ;
#72483=CARTESIAN_POINT ( 'NONE',  ( -13.89961937509977652, 13.97604488694528158, 25.62390960531434558 ) ) ;
#72484=CARTESIAN_POINT ( 'NONE',  ( -16.55341960407617563, 4.379528057220093196, 73.54275706135234714 ) ) ;
#72485=CARTESIAN_POINT ( 'NONE',  ( -19.05341960407611168, -5.049401038298163336, 41.45724293864769550 ) ) ;
#72487=CARTESIAN_POINT ( 'NONE',  ( -16.46253265017160317, 9.564922557960807481, 80.83224293864769550 ) ) ;
#72488=CARTESIAN_POINT ( 'NONE',  ( -16.51473224551069308, -9.474510206698971260, 31.66557627198102054 ) ) ;
#72489=CARTESIAN_POINT ( 'NONE',  ( -21.52544592524343514, 5.823673210054127303, 76.04057627198102409 ) ) ;
#72490=CARTESIAN_POINT ( 'NONE',  ( 16.55341960407618274, -4.379528057220086978, 41.04275706135236135 ) ) ;
#72491=CARTESIAN_POINT ( 'NONE',  ( 5.049401038297881783, 19.05341960407617563, 22.29275706135233648 ) ) ;
#72492=CARTESIAN_POINT ( 'NONE',  ( 0.05219959533909260263, 19.03943276465977164, 44.99890960531435979 ) ) ;
#72493=CARTESIAN_POINT ( 'NONE',  ( -16.55341960407611168, -4.379528057220339221, 26.45724293864768839 ) ) ;
#72494=CARTESIAN_POINT ( 'NONE',  ( 12.14591786802309770, 12.06949235617756955, 74.37390960531436690 ) ) ;
#72495=CARTESIAN_POINT ( 'NONE',  ( -9.474510206698964154, 16.51473224551069663, 65.41557627198102409 ) ) ;
#72496=CARTESIAN_POINT ( 'NONE',  ( 21.55341960407619695, -5.719274019375665929, 111.0427570613523613 ) ) ;
#72497=CARTESIAN_POINT ( 'NONE',  ( 5.719274019375673035, 21.55341960407619339, 27.29275706135234358 ) ) ;
#72498=CARTESIAN_POINT ( 'NONE',  ( -13.97604488694527625, -13.89961937509977652, 76.87390960531433848 ) ) ;
#72499=CARTESIAN_POINT ( 'NONE',  ( -15.72974639402176322, -15.80617190586768395, 84.37609039468570415 ) ) ;
#72500=CARTESIAN_POINT ( 'NONE',  ( -4.379528057220086978, -16.55341960407618274, 59.79275706135234714 ) ) ;
#72501=CARTESIAN_POINT ( 'NONE',  ( -8.314922557961024197, 14.29746914071037800, 22.91775706135235069 ) ) ;
#72502=CARTESIAN_POINT ( 'NONE',  ( -16.53943276465976808, 0.05219959533911058130, 91.24890960531436690 ) ) ;
#72503=CARTESIAN_POINT ( 'NONE',  ( 13.89961937509977652, -13.97604488694527269, 108.1239096053143669 ) ) ;
#72504=CARTESIAN_POINT ( 'NONE',  ( -16.53943276465976808, 0.05219959533911058130, 36.24890960531435979 ) ) ;
#72505=CARTESIAN_POINT ( 'NONE',  ( 0.05219959533909260263, 19.03943276465977164, 24.99890960531435269 ) ) ;
#72506=CARTESIAN_POINT ( 'NONE',  ( -16.52544592524335698, -4.483927247898792601, 48.95942372801902565 ) ) ;
#72507=CARTESIAN_POINT ( 'NONE',  ( 14.29746914071049879, -8.314922557960816363, 53.33224293864769550 ) ) ;
#72508=CARTESIAN_POINT ( 'NONE',  ( -8.224510206698735004, -14.34966873604973081, 99.58442372801900433 ) ) ;
#72509=CARTESIAN_POINT ( 'NONE',  ( 9.564922557960805705, 16.46253265017160317, 114.5822429386476955 ) ) ;
#72510=CARTESIAN_POINT ( 'NONE',  ( -21.52544592524343514, 5.823673210054127303, 31.04057627198102409 ) ) ;
#72511=CARTESIAN_POINT ( 'NONE',  ( -13.89961937509957401, -13.97604488694547875, 19.37609039468566507 ) ) ;
#72512=CARTESIAN_POINT ( 'NONE',  ( 8.224510206698953496, -14.34966873604960469, 82.91557627198103830 ) ) ;
#72513=CARTESIAN_POINT ( 'NONE',  ( 0.05219959533909260263, 19.03943276465977164, 99.99890960531436690 ) ) ;
#72515=CARTESIAN_POINT ( 'NONE',  ( 12.14591786802327356, -12.06949235617739191, 40.62609039468567573 ) ) ;
#72516=CARTESIAN_POINT ( 'NONE',  ( -19.02544592524342804, 5.153800228976336051, 56.04057627198100988 ) ) ;
#72518=CARTESIAN_POINT ( 'NONE',  ( 16.51473224551083163, -9.474510206698727899, 50.83442372801899722 ) ) ;
#72519=CARTESIAN_POINT ( 'NONE',  ( 16.46253265017160672, -9.564922557960803928, 43.33224293864769550 ) ) ;
#72520=CARTESIAN_POINT ( 'NONE',  ( -12.06949235617739369, -12.14591786802326823, 74.37609039468568994 ) ) ;
#72521=CARTESIAN_POINT ( 'NONE',  ( -5.153800228976607833, 19.02544592524334988, 92.70942372801901854 ) ) ;
#72522=CARTESIAN_POINT ( 'NONE',  ( 5.049401038298161559, -19.05341960407611168, 62.70724293864769550 ) ) ;
#72523=CARTESIAN_POINT ( 'NONE',  ( 15.72974639402199770, -15.80617190586745480, 88.12390960531436690 ) ) ;
#72524=CARTESIAN_POINT ( 'NONE',  ( -14.34966873604960291, -8.224510206698953496, 96.66557627198102409 ) ) ;
#72525=CARTESIAN_POINT ( 'NONE',  ( -13.89961937509957401, -13.97604488694547875, 74.37609039468566152 ) ) ;
#72526=CARTESIAN_POINT ( 'NONE',  ( 10.72451020669898902, -18.67979575497178502, 57.91557627198103120 ) ) ;
#72527=CARTESIAN_POINT ( 'NONE',  ( 5.049401038297881783, 19.05341960407617563, 42.29275706135234003 ) ) ;
#72528=CARTESIAN_POINT ( 'NONE',  ( 9.564922557960805705, 16.46253265017160317, 114.5822429386476955 ) ) ;
#72529=CARTESIAN_POINT ( 'NONE',  ( -0.05219959533907301413, -21.53943276465977519, 92.49890960531436690 ) ) ;
#72530=CARTESIAN_POINT ( 'NONE',  ( -19.52837319214027900, 5.499999999999901412, 54.60471352585540217 ) ) ;
#72531=CARTESIAN_POINT ( 'NONE',  ( 19.03943276465977164, 0.05219959533936151252, 106.2510903946856615 ) ) ;
#72532=CARTESIAN_POINT ( 'NONE',  ( -17.97058386085786452, -5.500000000000008882, 99.00390968646219392 ) ) ;
#72534=CARTESIAN_POINT ( 'NONE',  ( -12.14591786802326823, 12.06949235617739902, 23.12609039468567573 ) ) ;
#72535=CARTESIAN_POINT ( 'NONE',  ( -19.03943276465977164, 0.05219959533909376836, 46.24890960531435979 ) ) ;
#72536=CARTESIAN_POINT ( 'NONE',  ( 5.049401038298161559, -19.05341960407611168, 112.7072429386476813 ) ) ;
#72537=CARTESIAN_POINT ( 'NONE',  ( 21.55341960407610458, 5.719274019375980345, 83.95724293864770971 ) ) ;
#72538=CARTESIAN_POINT ( 'NONE',  ( 10.81492255796106328, -18.62759615963255655, 65.41775706135234714 ) ) ;
#72539=CARTESIAN_POINT ( 'NONE',  ( 19.05341960407617918, -5.049401038297876454, 111.0427570613523329 ) ) ;
#72540=CARTESIAN_POINT ( 'NONE',  ( 13.89961937509957401, 13.97604488694547697, 26.87609039468566507 ) ) ;
#72541=CARTESIAN_POINT ( 'NONE',  ( -16.53943276465976808, 0.05219959533911058130, 26.24890960531435624 ) ) ;
#72542=CARTESIAN_POINT ( 'NONE',  ( 21.55341960407610458, 5.719274019375980345, 103.9572429386476813 ) ) ;
#72543=CARTESIAN_POINT ( 'NONE',  ( -14.29746914071049879, 8.314922557960819915, 55.83224293864770260 ) ) ;
#72544=CARTESIAN_POINT ( 'NONE',  ( 5.049401038297881783, 19.05341960407617563, 92.29275706135234714 ) ) ;
#72545=CARTESIAN_POINT ( 'NONE',  ( 0.05219959533936267826, -19.03943276465977164, 60.00109039468566863 ) ) ;
#72546=CARTESIAN_POINT ( 'NONE',  ( 15.80617190586769283, -15.72974639402175789, 75.62609039468567573 ) ) ;
#72547=CARTESIAN_POINT ( 'NONE',  ( 0.05219959533936267826, -19.03943276465977164, 40.00109039468566152 ) ) ;
#72548=CARTESIAN_POINT ( 'NONE',  ( -13.97604488694527625, -13.89961937509977652, 21.87390960531435979 ) ) ;
#72549=CARTESIAN_POINT ( 'NONE',  ( -10.81492255796078084, -18.62759615963271287, 47.08224293864770260 ) ) ;
#72550=CARTESIAN_POINT ( 'NONE',  ( -4.483927247898539470, -16.52544592524342804, 37.29057627198102409 ) ) ;
#72551=CARTESIAN_POINT ( 'NONE',  ( -21.52544592524334988, -5.823673210054445271, 108.9594237280190185 ) ) ;
#72552=CARTESIAN_POINT ( 'NONE',  ( 14.34966873604972726, -8.224510206698740333, 75.83442372801900433 ) ) ;
#72553=CARTESIAN_POINT ( 'NONE',  ( 4.483927247898545687, 16.52544592524342804, 34.79057627198103120 ) ) ;
#72554=CARTESIAN_POINT ( 'NONE',  ( 5.719274019375673035, 21.55341960407619339, 72.29275706135236135 ) ) ;
#72555=CARTESIAN_POINT ( 'NONE',  ( 21.52544592524334988, 5.823673210054432836, 61.45942372801901854 ) ) ;
#72557=CARTESIAN_POINT ( 'NONE',  ( -10.72451020669898014, 18.67979575497178502, 65.41557627198102409 ) ) ;
#72559=EDGE_LOOP ( 'NONE', ( #117642, #196272 ) ) ;
#72560=CARTESIAN_POINT ( 'NONE',  ( 0.05219959533909260263, 19.03943276465977164, 34.99890960531435979 ) ) ;
#72561=CARTESIAN_POINT ( 'NONE',  ( 5.823673210054444382, -21.52544592524334988, 40.20942372801901854 ) ) ;
#72562=CARTESIAN_POINT ( 'NONE',  ( -13.97604488694527625, -13.89961937509977652, 26.87390960531434558 ) ) ;
#72563=CARTESIAN_POINT ( 'NONE',  ( -9.564922557960796823, -16.46253265017161027, 42.08224293864769550 ) ) ;
#72564=CARTESIAN_POINT ( 'NONE',  ( -4.483927247898539470, -16.52544592524342804, 92.29057627198103830 ) ) ;
#72565=CARTESIAN_POINT ( 'NONE',  ( 19.05341960407611168, 5.049401038298154454, 78.95724293864769550 ) ) ;
#72566=CARTESIAN_POINT ( 'NONE',  ( 8.314922557960818139, 14.29746914071049879, 34.58224293864770260 ) ) ;
#72567=CARTESIAN_POINT ( 'NONE',  ( -12.06949235617756955, 12.14591786802309770, 100.6239096053143811 ) ) ;
#72568=CARTESIAN_POINT ( 'NONE',  ( 21.55341960407610458, 5.719274019375980345, 63.95724293864770260 ) ) ;
#72569=CARTESIAN_POINT ( 'NONE',  ( -10.72451020669898014, 18.67979575497178502, 110.4155762719810383 ) ) ;
#72570=CARTESIAN_POINT ( 'NONE',  ( 19.05341960407611168, 5.049401038298154454, 113.9572429386477097 ) ) ;
#72571=CARTESIAN_POINT ( 'NONE',  ( 0.05219959533909260263, 19.03943276465977164, 59.99890960531436690 ) ) ;
#72572=CARTESIAN_POINT ( 'NONE',  ( 12.14591786802327356, -12.06949235617739191, 25.62609039468567929 ) ) ;
#72573=CARTESIAN_POINT ( 'NONE',  ( -15.80617190586745835, -15.72974639402198527, 51.87390960531437401 ) ) ;
#72575=CARTESIAN_POINT ( 'NONE',  ( 18.67979575497194134, -10.72451020669871369, 90.83442372801901854 ) ) ;
#72576=CARTESIAN_POINT ( 'NONE',  ( -9.564922557960796823, -16.46253265017161027, 77.08224293864769550 ) ) ;
#72577=CARTESIAN_POINT ( 'NONE',  ( -21.52544592524343514, 5.823673210054127303, 116.0405762719810383 ) ) ;
#72578=CARTESIAN_POINT ( 'NONE',  ( -9.564922557960796823, -16.46253265017161027, 112.0822429386476955 ) ) ;
#72579=CARTESIAN_POINT ( 'NONE',  ( 16.53943276465976808, 0.05219959533934440121, 91.25109039468568994 ) ) ;
#72580=CARTESIAN_POINT ( 'NONE',  ( 10.72451020669871369, 18.67979575497193778, 77.08442372801901854 ) ) ;
#72581=CARTESIAN_POINT ( 'NONE',  ( -21.55341960407619339, 5.719274019375674811, 98.54275706135234714 ) ) ;
#72582=CARTESIAN_POINT ( 'NONE',  ( 4.379528057220092307, 16.55341960407617563, 62.29275706135236845 ) ) ;
#72583=CARTESIAN_POINT ( 'NONE',  ( 5.823673210054444382, -21.52544592524334988, 30.20942372801902565 ) ) ;
#72584=CARTESIAN_POINT ( 'NONE',  ( -19.05341960407611168, -5.049401038298163336, 111.4572429386476671 ) ) ;
#72585=CARTESIAN_POINT ( 'NONE',  ( 21.52544592524334988, 5.823673210054432836, 86.45942372801901854 ) ) ;
#72586=CARTESIAN_POINT ( 'NONE',  ( 16.51473224551069308, 9.474510206698969483, 94.16557627198103830 ) ) ;
#72587=CARTESIAN_POINT ( 'NONE',  ( 18.67979575497178502, 10.72451020669898547, 89.16557627198102409 ) ) ;
#72588=CARTESIAN_POINT ( 'NONE',  ( 5.049401038297881783, 19.05341960407617563, 47.29275706135231161 ) ) ;
#72589=CARTESIAN_POINT ( 'NONE',  ( 15.80617190586746368, 15.72974639402197994, 59.37390960531436690 ) ) ;
#72590=CARTESIAN_POINT ( 'NONE',  ( 9.564922557960805705, 16.46253265017160317, 99.58224293864770971 ) ) ;
#72591=CARTESIAN_POINT ( 'NONE',  ( 8.224510206698953496, -14.34966873604960469, 32.91557627198102409 ) ) ;
#72593=CARTESIAN_POINT ( 'NONE',  ( 13.97604488694548053, -13.89961937509957401, 65.62609039468567573 ) ) ;
#72595=CARTESIAN_POINT ( 'NONE',  ( 5.153800228976615827, -19.02544592524334988, 105.2094237280190185 ) ) ;
#72596=CARTESIAN_POINT ( 'NONE',  ( -21.55341960407610458, -5.719274019375992779, 91.45724293864769550 ) ) ;
#72597=CARTESIAN_POINT ( 'NONE',  ( 8.314922557960818139, 14.29746914071049879, 54.58224293864769550 ) ) ;
#72598=CARTESIAN_POINT ( 'NONE',  ( -4.379528057220086978, -16.55341960407618274, 34.79275706135235424 ) ) ;
#72599=CARTESIAN_POINT ( 'NONE',  ( 9.564922557960805705, 16.46253265017160317, 49.58224293864770260 ) ) ;
#72600=CARTESIAN_POINT ( 'NONE',  ( 21.53943276465977519, -0.05219959533907433946, 113.7489096053143527 ) ) ;
#72601=CARTESIAN_POINT ( 'NONE',  ( 9.564922557961047289, -16.46253265017146816, 90.41775706135234714 ) ) ;
#72602=CARTESIAN_POINT ( 'NONE',  ( 19.03943276465977164, -0.05219959533909143690, 88.74890960531436690 ) ) ;
#72603=CARTESIAN_POINT ( 'NONE',  ( -9.564922557960796823, -16.46253265017161027, 72.08224293864770971 ) ) ;
#72604=CARTESIAN_POINT ( 'NONE',  ( -21.55341960407610458, -5.719274019375992779, 76.45724293864769550 ) ) ;
#72605=CARTESIAN_POINT ( 'NONE',  ( 19.05341960407611168, 5.049401038298154454, 48.95724293864768129 ) ) ;
#72607=CARTESIAN_POINT ( 'NONE',  ( 8.314922557960818139, 14.29746914071049879, 54.58224293864769550 ) ) ;
#72608=CARTESIAN_POINT ( 'NONE',  ( -0.05219959533909027116, -19.03943276465977164, 87.49890960531436690 ) ) ;
#72610=CARTESIAN_POINT ( 'NONE',  ( -9.564922557961040184, 16.46253265017147172, 62.91775706135233293 ) ) ;
#72611=CARTESIAN_POINT ( 'NONE',  ( -18.62759615963270932, 10.81492255796079327, 75.83224293864769550 ) ) ;
#72612=CARTESIAN_POINT ( 'NONE',  ( -5.153800228976607833, 19.02544592524334988, 32.70942372801899722 ) ) ;
#72613=CARTESIAN_POINT ( 'NONE',  ( -13.97604488694527625, -13.89961937509977652, 101.8739096053143811 ) ) ;
#72614=CARTESIAN_POINT ( 'NONE',  ( -17.49999999999999645, 5.076555817581247965, 113.8204850795022907 ) ) ;
#72615=CARTESIAN_POINT ( 'NONE',  ( -5.823673210054116645, -21.52544592524344225, 42.29057627198103120 ) ) ;
#72617=CARTESIAN_POINT ( 'NONE',  ( 19.05341960407611168, 5.049401038298154454, 73.95724293864768129 ) ) ;
#72618=CARTESIAN_POINT ( 'NONE',  ( 0.05219959533937995610, -21.53943276465977519, 60.00109039468568284 ) ) ;
#72619=CARTESIAN_POINT ( 'NONE',  ( 19.05341960407611168, 5.049401038298154454, 23.95724293864769194 ) ) ;
#72620=CARTESIAN_POINT ( 'NONE',  ( -21.52544592524343514, 5.823673210054127303, 116.0405762719810383 ) ) ;
#72622=CARTESIAN_POINT ( 'NONE',  ( -10.81492255796105439, 18.62759615963255655, 47.91775706135234714 ) ) ;
#72624=CARTESIAN_POINT ( 'NONE',  ( -5.153800228976328057, -19.02544592524343514, 97.29057627198099567 ) ) ;
#72625=CARTESIAN_POINT ( 'NONE',  ( -0.05219959533936034679, 19.03943276465977164, 72.50109039468566152 ) ) ;
#72627=CARTESIAN_POINT ( 'NONE',  ( -5.823673210054116645, -21.52544592524344225, 107.2905762719810525 ) ) ;
#72628=CARTESIAN_POINT ( 'NONE',  ( 9.474510206698971260, -16.51473224551069308, 57.91557627198103120 ) ) ;
#72629=CARTESIAN_POINT ( 'NONE',  ( -14.34966873604972548, 8.224510206698743886, 33.33442372801900433 ) ) ;
#72631=CARTESIAN_POINT ( 'NONE',  ( 5.719274019375673035, 21.55341960407619339, 97.29275706135234714 ) ) ;
#72632=CARTESIAN_POINT ( 'NONE',  ( 19.02544592524343514, -5.153800228976328945, 43.54057627198103120 ) ) ;
#72633=CARTESIAN_POINT ( 'NONE',  ( -18.67979575497193778, 10.72451020669871902, 103.3344237280190043 ) ) ;
#72634=CARTESIAN_POINT ( 'NONE',  ( 9.474510206698971260, -16.51473224551069308, 82.91557627198103830 ) ) ;
#72635=CARTESIAN_POINT ( 'NONE',  ( -21.53943276465977519, -0.05219959533937600094, 53.75109039468568994 ) ) ;
#72637=CARTESIAN_POINT ( 'NONE',  ( -16.51473224551069308, -9.474510206698971260, 111.6655762719810383 ) ) ;
#72639=CARTESIAN_POINT ( 'NONE',  ( 8.224510206698742110, 14.34966873604972548, 47.08442372801901854 ) ) ;
#72640=CARTESIAN_POINT ( 'NONE',  ( -0.05219959533937732626, 21.53943276465977519, 67.50109039468568994 ) ) ;
#72641=CARTESIAN_POINT ( 'NONE',  ( -10.72451020669870658, -18.67979575497194134, 94.58442372801901854 ) ) ;
#72643=CARTESIAN_POINT ( 'NONE',  ( 14.29746914071037800, 8.314922557961029526, 21.66775706135235069 ) ) ;
#72644=CARTESIAN_POINT ( 'NONE',  ( 16.51473224551069308, 9.474510206698969483, 84.16557627198102409 ) ) ;
#72645=CARTESIAN_POINT ( 'NONE',  ( 0.05219959533909260263, 19.03943276465977164, 114.9989096053143669 ) ) ;
#72646=VERTEX_POINT ( 'NONE', #166611 ) ;
#72648=CARTESIAN_POINT ( 'NONE',  ( 8.314922557960818139, 14.29746914071049879, 114.5822429386477097 ) ) ;
#72649=CARTESIAN_POINT ( 'NONE',  ( 18.62759615963271287, -10.81492255796078972, 43.33224293864769550 ) ) ;
#72650=CARTESIAN_POINT ( 'NONE',  ( 14.29746914071037800, 8.314922557961029526, 91.66775706135234714 ) ) ;
#72651=CARTESIAN_POINT ( 'NONE',  ( -14.34966873604960291, -8.224510206698953496, 81.66557627198103830 ) ) ;
#72652=CARTESIAN_POINT ( 'NONE',  ( 19.03943276465977164, -0.05219959533909143690, 63.74890960531435979 ) ) ;
#72653=CARTESIAN_POINT ( 'NONE',  ( 5.823673210054444382, -21.52544592524334988, 85.20942372801901854 ) ) ;
#72655=CARTESIAN_POINT ( 'NONE',  ( -19.05341960407617563, 5.049401038297882671, 113.5427570613523471 ) ) ;
#72656=CARTESIAN_POINT ( 'NONE',  ( 14.34966873604960469, 8.224510206698951720, 84.16557627198103830 ) ) ;
#72657=CARTESIAN_POINT ( 'NONE',  ( 5.823673210054444382, -21.52544592524334988, 40.20942372801901854 ) ) ;
#72658=CARTESIAN_POINT ( 'NONE',  ( -5.719274019375978568, 21.55341960407610458, 75.20724293864769550 ) ) ;
#72659=CARTESIAN_POINT ( 'NONE',  ( -19.03943276465977164, -0.05219959533935918106, 43.75109039468566863 ) ) ;
#72660=CARTESIAN_POINT ( 'NONE',  ( 17.59860650958989936, 7.585241751807028088, 44.07662985737508166 ) ) ;
#72661=CARTESIAN_POINT ( 'NONE',  ( 9.474510206698971260, -16.51473224551069308, 77.91557627198103830 ) ) ;
#72662=CARTESIAN_POINT ( 'NONE',  ( 16.52544592524342804, -4.483927247898539470, 68.54057627198103830 ) ) ;
#72663=CARTESIAN_POINT ( 'NONE',  ( -16.53943276465976808, 0.05219959533911058130, 36.24890960531435979 ) ) ;
#72664=CARTESIAN_POINT ( 'NONE',  ( 16.52544592524335698, 4.483927247898782831, 106.4594237280190328 ) ) ;
#72665=CARTESIAN_POINT ( 'NONE',  ( -19.03943276465977164, -0.05219959533935918106, 68.75109039468566152 ) ) ;
#72666=CARTESIAN_POINT ( 'NONE',  ( 17.31728774477273447, 6.344390552232407998, 46.68093348310681279 ) ) ;
#72667=CARTESIAN_POINT ( 'NONE',  ( -9.474510206698964154, 16.51473224551069663, 115.4155762719810241 ) ) ;
#72668=CARTESIAN_POINT ( 'NONE',  ( -16.55341960407611168, -4.379528057220339221, 91.45724293864769550 ) ) ;
#72670=CARTESIAN_POINT ( 'NONE',  ( -19.05341960407611168, -5.049401038298163336, 46.45724293864768129 ) ) ;
#72671=CARTESIAN_POINT ( 'NONE',  ( -18.62759615963270932, 10.81492255796079327, 45.83224293864769550 ) ) ;
#72672=CARTESIAN_POINT ( 'NONE',  ( 21.52544592524344225, -5.823673210054117533, 68.54057627198103830 ) ) ;
#72673=CARTESIAN_POINT ( 'NONE',  ( -13.97604488694527625, -13.89961937509977652, 21.87390960531435979 ) ) ;
#72674=CARTESIAN_POINT ( 'NONE',  ( -4.379528057220086978, -16.55341960407618274, 59.79275706135234714 ) ) ;
#72675=CARTESIAN_POINT ( 'NONE',  ( -13.89961937509977652, 13.97604488694528158, 50.62390960531435979 ) ) ;
#72677=CARTESIAN_POINT ( 'NONE',  ( -21.55341960407619339, 5.719274019375674811, 53.54275706135234714 ) ) ;
#72678=CARTESIAN_POINT ( 'NONE',  ( 0.05219959533910956823, 16.53943276465976808, 99.99890960531436690 ) ) ;
#72680=CARTESIAN_POINT ( 'NONE',  ( 13.89961937509957401, 13.97604488694547697, 91.87609039468567573 ) ) ;
#72683=CARTESIAN_POINT ( 'NONE',  ( -21.52544592524343514, 5.823673210054127303, 51.04057627198103120 ) ) ;
#72684=CARTESIAN_POINT ( 'NONE',  ( 17.49999999999999645, -5.624438216177594541, 68.31670344914645909 ) ) ;
#72685=CARTESIAN_POINT ( 'NONE',  ( -18.62759615963255300, -10.81492255796106328, 79.16775706135234714 ) ) ;
#72686=CARTESIAN_POINT ( 'NONE',  ( 14.34966873604972726, -8.224510206698740333, 55.83442372801901854 ) ) ;
#72687=CARTESIAN_POINT ( 'NONE',  ( -12.14591786802309592, -12.06949235617757132, 36.87390960531435979 ) ) ;
#72688=CARTESIAN_POINT ( 'NONE',  ( 18.67979575497178502, 10.72451020669898547, 74.16557627198102409 ) ) ;
#72689=CARTESIAN_POINT ( 'NONE',  ( -15.72974639402197994, 15.80617190586746368, 75.62390960531439532 ) ) ;
#72691=CARTESIAN_POINT ( 'NONE',  ( -19.05341960407617563, 5.049401038297882671, 88.54275706135230450 ) ) ;
#72692=CARTESIAN_POINT ( 'NONE',  ( 13.97604488694527802, 13.89961937509977652, 109.3739096053143669 ) ) ;
#72693=CARTESIAN_POINT ( 'NONE',  ( 0.05219959533909260263, 19.03943276465977164, 54.99890960531435979 ) ) ;
#72694=CARTESIAN_POINT ( 'NONE',  ( 16.53943276465976808, -0.05219959533910856209, 113.7489096053143527 ) ) ;
#72697=ORIENTED_EDGE ( 'NONE', *, *, #143807, .T. ) ;
#72699=CARTESIAN_POINT ( 'NONE',  ( -16.52544592524335698, -4.483927247898792601, 88.95942372801901854 ) ) ;
#72700=CARTESIAN_POINT ( 'NONE',  ( 5.823673210054125526, 21.52544592524343514, 104.7905762719810241 ) ) ;
#72701=CARTESIAN_POINT ( 'NONE',  ( -5.049401038298153566, 19.05341960407611168, 65.20724293864765286 ) ) ;
#72702=CARTESIAN_POINT ( 'NONE',  ( -15.80617190586768217, 15.72974639402176855, 38.12609039468567573 ) ) ;
#72703=CARTESIAN_POINT ( 'NONE',  ( -19.05341960407611168, -5.049401038298163336, 96.45724293864769550 ) ) ;
#72706=ORIENTED_EDGE ( 'NONE', *, *, #86027, .T. ) ;
#72707=CARTESIAN_POINT ( 'NONE',  ( 21.53943276465977519, 0.05219959533937863772, 31.25109039468568639 ) ) ;
#72708=CARTESIAN_POINT ( 'NONE',  ( -0.05219959533909027116, -19.03943276465977164, 22.49890960531436690 ) ) ;
#72709=CARTESIAN_POINT ( 'NONE',  ( -19.02544592524334988, -5.153800228976617603, 88.95942372801897591 ) ) ;
#72710=CARTESIAN_POINT ( 'NONE',  ( 19.03943276465977164, 0.05219959533936151252, 41.25109039468566152 ) ) ;
#72711=CARTESIAN_POINT ( 'NONE',  ( -18.62759615963255300, -10.81492255796106328, 19.16775706135234714 ) ) ;
#72712=CARTESIAN_POINT ( 'NONE',  ( -19.02544592524334988, -5.153800228976617603, 38.95942372801900433 ) ) ;
#72713=CARTESIAN_POINT ( 'NONE',  ( -16.46253265017146816, -9.564922557961047289, 44.16775706135232582 ) ) ;
#72714=CARTESIAN_POINT ( 'NONE',  ( 14.29746914071037800, 8.314922557961029526, 91.66775706135234714 ) ) ;
#72716=CARTESIAN_POINT ( 'NONE',  ( 16.46253265017160672, -9.564922557960803928, 68.33224293864770971 ) ) ;
#72717=MECHANICAL_DESIGN_GEOMETRIC_PRESENTATION_REPRESENTATION('',(#179239),#108182);
#72718=CARTESIAN_POINT ( 'NONE',  ( 18.67979575497194134, -10.72451020669871369, 75.83442372801900433 ) ) ;
#72719=CARTESIAN_POINT ( 'NONE',  ( -0.05219959533937732626, 21.53943276465977519, 92.50109039468567573 ) ) ;
#72721=CARTESIAN_POINT ( 'NONE',  ( 0.05219959533909260263, 19.03943276465977164, 84.99890960531436690 ) ) ;
#72722=CARTESIAN_POINT ( 'NONE',  ( -5.823673210054431948, 21.52544592524334988, 62.70942372801902565 ) ) ;
#72723=CARTESIAN_POINT ( 'NONE',  ( -13.97604488694547697, 13.89961937509957934, 103.1260903946856473 ) ) ;
#72724=CARTESIAN_POINT ( 'NONE',  ( -13.89961937509977652, 13.97604488694528158, 65.62390960531436690 ) ) ;
#72725=CARTESIAN_POINT ( 'NONE',  ( -10.81492255796078084, -18.62759615963271287, 22.08224293864769194 ) ) ;
#72726=CARTESIAN_POINT ( 'NONE',  ( 9.564922557960805705, 16.46253265017160317, 74.58224293864769550 ) ) ;
#72728=CARTESIAN_POINT ( 'NONE',  ( -16.51473224551069308, -9.474510206698971260, 61.66557627198103120 ) ) ;
#72729=CARTESIAN_POINT ( 'NONE',  ( -9.564922557960796823, -16.46253265017161027, 47.08224293864769550 ) ) ;
#72730=CARTESIAN_POINT ( 'NONE',  ( 21.52544592524344225, -5.823673210054117533, 113.5405762719810383 ) ) ;
#72731=CARTESIAN_POINT ( 'NONE',  ( 14.34966873604972726, -8.224510206698740333, 95.83442372801903275 ) ) ;
#72732=CARTESIAN_POINT ( 'NONE',  ( -18.56399227203345603, -5.499999999999827693, 38.97830131249903474 ) ) ;
#72733=AXIS2_PLACEMENT_3D ( 'NONE', #59317, #75484, #120986 ) ;
#72735=CARTESIAN_POINT ( 'NONE',  ( 5.049401038297881783, 19.05341960407617563, 62.29275706135234003 ) ) ;
#72736=CARTESIAN_POINT ( 'NONE',  ( -13.97604488694527625, -13.89961937509977652, 76.87390960531433848 ) ) ;
#72737=CARTESIAN_POINT ( 'NONE',  ( -16.52544592524342804, 4.483927247898546575, 71.04057627198103830 ) ) ;
#72738=CARTESIAN_POINT ( 'NONE',  ( 16.52544592524342804, -4.483927247898539470, 103.5405762719810383 ) ) ;
#72740=CARTESIAN_POINT ( 'NONE',  ( 15.72974639402199770, -15.80617190586745480, 38.12390960531436690 ) ) ;
#72741=( BOUNDED_CURVE ( )  B_SPLINE_CURVE ( 2, ( #152839, #107321, #185173, #61811, #137672, #76990, #88189, #45670, #184188, #149873, #14333, #123481, #75998 ),
 .UNSPECIFIED., .F., .F. ) 
 B_SPLINE_CURVE_WITH_KNOTS ( ( 3, 2, 2, 2, 2, 2, 3 ),
 ( 0.6603708530912405505, 0.6622807017543859143, 0.6666666666666666297, 0.6710526315789473450, 0.6754385964912280604, 0.6798245614035087758, 0.6817800898887445005 ),
 .UNSPECIFIED. ) 
 CURVE ( )  GEOMETRIC_REPRESENTATION_ITEM ( )  RATIONAL_B_SPLINE_CURVE ( ( 0.9832469066685283199, 0.9851625545550095620, 1.000000000000000000, 0.9659258262890683122, 1.000000000000000000, 0.9659258262890683122, 1.000000000000000000, 0.9659258262890683122, 1.000000000000000000, 0.9659258262890683122, 1.000000000000000000, 0.9848076720550078544, 0.9831626618144001517 ) ) 
 REPRESENTATION_ITEM ( '' )  );
#72742=CARTESIAN_POINT ( 'NONE',  ( 5.153800228976335163, 19.02544592524342804, 109.7905762719810099 ) ) ;
#72743=CARTESIAN_POINT ( 'NONE',  ( -4.483927247898539470, -16.52544592524342804, 97.29057627198105251 ) ) ;
#72744=CARTESIAN_POINT ( 'NONE',  ( -13.97604488694527625, -13.89961937509977830, 81.87390960531436690 ) ) ;
#72745=CARTESIAN_POINT ( 'NONE',  ( 19.02544592524334988, 5.153800228976608722, 26.45942372801899722 ) ) ;
#72746=CARTESIAN_POINT ( 'NONE',  ( -16.52544592524335698, -4.483927247898792601, 103.9594237280190185 ) ) ;
#72747=CARTESIAN_POINT ( 'NONE',  ( -0.05219959533909027116, -19.03943276465977164, 87.49890960531436690 ) ) ;
#72748=CARTESIAN_POINT ( 'NONE',  ( 18.62759615963255655, 10.81492255796105972, 46.66775706135234714 ) ) ;
#72749=CARTESIAN_POINT ( 'NONE',  ( 5.719274019375991003, -21.55341960407610458, 37.70724293864769550 ) ) ;
#72750=CARTESIAN_POINT ( 'NONE',  ( -15.80617190586745835, -15.72974639402198527, 111.8739096053143669 ) ) ;
#72751=CARTESIAN_POINT ( 'NONE',  ( -10.72451020669898014, 18.67979575497178502, 75.41557627198102409 ) ) ;
#72752=CARTESIAN_POINT ( 'NONE',  ( -12.06949235617756955, 12.14591786802309770, 90.62390960531436690 ) ) ;
#72753=CARTESIAN_POINT ( 'NONE',  ( -19.02544592524334988, -5.153800228976617603, 58.95942372801900433 ) ) ;
#72754=CARTESIAN_POINT ( 'NONE',  ( -13.89961937509977652, 13.97604488694528158, 30.62390960531435269 ) ) ;
#72755=CARTESIAN_POINT ( 'NONE',  ( 13.89961937509977652, -13.97604488694527269, 98.12390960531433848 ) ) ;
#72756=CARTESIAN_POINT ( 'NONE',  ( -19.05341960407611168, -5.049401038298163336, 91.45724293864766707 ) ) ;
#72757=CARTESIAN_POINT ( 'NONE',  ( 16.52544592524342804, -4.483927247898539470, 108.5405762719810241 ) ) ;
#72758=CARTESIAN_POINT ( 'NONE',  ( -14.29746914071049879, 8.314922557960819915, 25.83224293864769194 ) ) ;
#72759=CARTESIAN_POINT ( 'NONE',  ( 16.55341960407618274, -4.379528057220086978, 41.04275706135236135 ) ) ;
#72760=CARTESIAN_POINT ( 'NONE',  ( -18.62759615963255300, -10.81492255796106328, 104.1677570613523471 ) ) ;
#72762=CARTESIAN_POINT ( 'NONE',  ( -13.97604488694527625, -13.89961937509977652, 101.8739096053143811 ) ) ;
#72763=CARTESIAN_POINT ( 'NONE',  ( 16.53943276465976808, -0.05219959533910856209, 23.74890960531435269 ) ) ;
#72764=CARTESIAN_POINT ( 'NONE',  ( 18.62759615963255655, 10.81492255796105972, 36.66775706135234714 ) ) ;
#72765=CARTESIAN_POINT ( 'NONE',  ( -13.89961937509977652, 13.97604488694528158, 45.62390960531433848 ) ) ;
#72766=CARTESIAN_POINT ( 'NONE',  ( 16.55341960407618274, -4.379528057220086978, 51.04275706135234714 ) ) ;
#72767=CARTESIAN_POINT ( 'NONE',  ( 16.52544592524335698, 4.483927247898782831, 111.4594237280190328 ) ) ;
#72768=CARTESIAN_POINT ( 'NONE',  ( -16.53943276465976808, -0.05219959533934237506, 98.75109039468568994 ) ) ;
#72769=CARTESIAN_POINT ( 'NONE',  ( -16.46253265017146816, -9.564922557961047289, 104.1677570613523329 ) ) ;
#72770=CARTESIAN_POINT ( 'NONE',  ( 9.564922557960805705, 16.46253265017160317, 39.58224293864768839 ) ) ;
#72771=CARTESIAN_POINT ( 'NONE',  ( 16.52544592524342804, -4.483927247898539470, 93.54057627198103830 ) ) ;
#72772=CARTESIAN_POINT ( 'NONE',  ( -10.72451020669898014, 18.67979575497178502, 105.4155762719810383 ) ) ;
#72773=CARTESIAN_POINT ( 'NONE',  ( -0.05219959533909027116, -19.03943276465977164, 37.49890960531436690 ) ) ;
#72774=CARTESIAN_POINT ( 'NONE',  ( -16.51473224551069308, -9.474510206698971260, 101.6655762719810241 ) ) ;
#72775=CARTESIAN_POINT ( 'NONE',  ( 5.719274019375673035, 21.55341960407619339, 27.29275706135234358 ) ) ;
#72777=CARTESIAN_POINT ( 'NONE',  ( 9.474510206698971260, -16.51473224551069308, 102.9155762719810241 ) ) ;
#72779=CARTESIAN_POINT ( 'NONE',  ( -19.02544592524342804, 5.153800228976336051, 91.04057627198100988 ) ) ;
#72780=CARTESIAN_POINT ( 'NONE',  ( -5.719274019375665041, -21.55341960407619695, 34.79275706135235424 ) ) ;
#72781=CARTESIAN_POINT ( 'NONE',  ( -12.14591786802309592, -12.06949235617757132, 96.87390960531436690 ) ) ;
#72782=CARTESIAN_POINT ( 'NONE',  ( 19.03943276465977164, -0.05219959533909143690, 93.74890960531435269 ) ) ;
#72783=CARTESIAN_POINT ( 'NONE',  ( 16.51473224551083163, -9.474510206698727899, 25.83442372801900078 ) ) ;
#72784=CARTESIAN_POINT ( 'NONE',  ( -12.06949235617739369, -12.14591786802326823, 59.37609039468568284 ) ) ;
#72785=CARTESIAN_POINT ( 'NONE',  ( -21.53943276465977519, -0.05219959533937600094, 73.75109039468567573 ) ) ;
#72786=CARTESIAN_POINT ( 'NONE',  ( 8.314922557961029526, -14.29746914071037800, 45.41775706135234003 ) ) ;
#72787=CARTESIAN_POINT ( 'NONE',  ( -19.02544592524342804, 5.153800228976336051, 86.04057627198103830 ) ) ;
#72788=CARTESIAN_POINT ( 'NONE',  ( -16.46253265017146816, -9.564922557961047289, 89.16775706135234714 ) ) ;
#72789=CARTESIAN_POINT ( 'NONE',  ( -8.314922557961024197, 14.29746914071037800, 72.91775706135234714 ) ) ;
#72790=CARTESIAN_POINT ( 'NONE',  ( 10.72451020669871369, 18.67979575497193778, 107.0844237280190043 ) ) ;
#72791=CARTESIAN_POINT ( 'NONE',  ( 13.89961937509957401, 13.97604488694547697, 96.87609039468566152 ) ) ;
#72792=CARTESIAN_POINT ( 'NONE',  ( 9.474510206698971260, -16.51473224551069308, 67.91557627198102409 ) ) ;
#72793=CARTESIAN_POINT ( 'NONE',  ( 5.719274019375991003, -21.55341960407610458, 77.70724293864770971 ) ) ;
#72794=CARTESIAN_POINT ( 'NONE',  ( -14.29746914071049879, 8.314922557960819915, 85.83224293864768129 ) ) ;
#72795=CARTESIAN_POINT ( 'NONE',  ( 5.153800228976615827, -19.02544592524334988, 90.20942372801900433 ) ) ;
#72796=CARTESIAN_POINT ( 'NONE',  ( 12.14591786802327356, -12.06949235617739191, 65.62609039468568994 ) ) ;
#72798=CARTESIAN_POINT ( 'NONE',  ( 16.51473224551083163, -9.474510206698727899, 60.83442372801900433 ) ) ;
#72799=CARTESIAN_POINT ( 'NONE',  ( 12.06949235617757843, -12.14591786802309237, 23.12390960531436335 ) ) ;
#72800=CARTESIAN_POINT ( 'NONE',  ( 12.06949235617757843, -12.14591786802309237, 83.12390960531436690 ) ) ;
#72801=CARTESIAN_POINT ( 'NONE',  ( -16.46253265017146816, -9.564922557961047289, 19.16775706135233293 ) ) ;
#72802=CARTESIAN_POINT ( 'NONE',  ( -17.44279575226786250, 5.990770900253883369, 40.83557567514318265 ) ) ;
#72803=CARTESIAN_POINT ( 'NONE',  ( -21.52544592524334988, -5.823673210054445271, 18.95942372801901143 ) ) ;
#72804=CARTESIAN_POINT ( 'NONE',  ( 9.474510206698971260, -16.51473224551069308, 97.91557627198102409 ) ) ;
#72805=CARTESIAN_POINT ( 'NONE',  ( -5.049401038298153566, 19.05341960407611168, 80.20724293864769550 ) ) ;
#72806=CARTESIAN_POINT ( 'NONE',  ( -21.52544592524334988, -5.823673210054445271, 88.95942372801901854 ) ) ;
#72807=CARTESIAN_POINT ( 'NONE',  ( -16.51473224551069308, -9.474510206698971260, 66.66557627198102409 ) ) ;
#72808=CARTESIAN_POINT ( 'NONE',  ( 21.53943276465977519, -0.05219959533907433946, 28.74890960531435624 ) ) ;
#72810=CARTESIAN_POINT ( 'NONE',  ( 14.29746914071049879, -8.314922557960816363, 78.33224293864770971 ) ) ;
#72811=CARTESIAN_POINT ( 'NONE',  ( -16.46253265017160317, 9.564922557960807481, 40.83224293864769550 ) ) ;
#72812=CARTESIAN_POINT ( 'NONE',  ( -0.05219959533910754901, -16.53943276465976808, 102.4989096053143811 ) ) ;
#72813=CARTESIAN_POINT ( 'NONE',  ( 5.823673210054125526, 21.52544592524343514, 104.7905762719810241 ) ) ;
#72814=CARTESIAN_POINT ( 'NONE',  ( 18.67979575497194134, -10.72451020669871369, 60.83442372801901854 ) ) ;
#72815=CARTESIAN_POINT ( 'NONE',  ( -9.474510206698964154, 16.51473224551069663, 30.41557627198102054 ) ) ;
#72816=CARTESIAN_POINT ( 'NONE',  ( -8.224510206698735004, -14.34966873604973081, 64.58442372801900433 ) ) ;
#72817=CARTESIAN_POINT ( 'NONE',  ( -15.80617190586745835, -15.72974639402198527, 106.8739096053143811 ) ) ;
#72818=CARTESIAN_POINT ( 'NONE',  ( -5.823673210054116645, -21.52544592524344225, 112.2905762719810241 ) ) ;
#72819=CARTESIAN_POINT ( 'NONE',  ( 13.97604488694548053, -13.89961937509957401, 45.62609039468566863 ) ) ;
#72820=CARTESIAN_POINT ( 'NONE',  ( 5.049401038298161559, -19.05341960407611168, 47.70724293864770260 ) ) ;
#72821=CARTESIAN_POINT ( 'NONE',  ( -17.72696623605158806, 5.500000000000047962, 83.59811031808415294 ) ) ;
#72822=CARTESIAN_POINT ( 'NONE',  ( -0.05219959533937732626, 21.53943276465977519, 62.50109039468568284 ) ) ;
#72823=CARTESIAN_POINT ( 'NONE',  ( 15.80617190586746368, 15.72974639402197994, 54.37390960531435979 ) ) ;
#72824=CARTESIAN_POINT ( 'NONE',  ( -14.34966873604960291, -8.224510206698953496, 31.66557627198102054 ) ) ;
#72825=CARTESIAN_POINT ( 'NONE',  ( -0.05219959533937732626, 21.53943276465977519, 72.50109039468568994 ) ) ;
#72826=CARTESIAN_POINT ( 'NONE',  ( 18.62759615963255655, 10.81492255796105972, 111.6677570613523613 ) ) ;
#72827=CARTESIAN_POINT ( 'NONE',  ( 0.05219959533910956823, 16.53943276465976808, 54.99890960531435269 ) ) ;
#72828=CARTESIAN_POINT ( 'NONE',  ( 0.05219959533910956823, 16.53943276465976808, 104.9989096053143669 ) ) ;
#72829=CARTESIAN_POINT ( 'NONE',  ( -9.474510206698720793, -16.51473224551083518, 39.58442372801899722 ) ) ;
#72830=CARTESIAN_POINT ( 'NONE',  ( -14.34966873604972548, 8.224510206698743886, 98.33442372801901854 ) ) ;
#72831=CARTESIAN_POINT ( 'NONE',  ( 0.05219959533937995610, -21.53943276465977519, 65.00109039468568994 ) ) ;
#72832=CARTESIAN_POINT ( 'NONE',  ( 19.05341960407611168, 5.049401038298154454, 58.95724293864768129 ) ) ;
#72833=CARTESIAN_POINT ( 'NONE',  ( -16.46253265017146816, -9.564922557961047289, 34.16775706135233293 ) ) ;
#72834=CARTESIAN_POINT ( 'NONE',  ( 18.67979575497178502, 10.72451020669898547, 39.16557627198102409 ) ) ;
#72835=CARTESIAN_POINT ( 'NONE',  ( -21.52544592524334988, -5.823673210054445271, 28.95942372801902209 ) ) ;
#72836=CARTESIAN_POINT ( 'NONE',  ( -10.81492255796078084, -18.62759615963271287, 82.08224293864768129 ) ) ;
#72837=CARTESIAN_POINT ( 'NONE',  ( 0.05219959533936267826, -19.03943276465977164, 90.00109039468567573 ) ) ;
#72838=CARTESIAN_POINT ( 'NONE',  ( 12.14591786802327356, -12.06949235617739191, 50.62609039468568994 ) ) ;
#72839=CARTESIAN_POINT ( 'NONE',  ( 17.50000000000050093, -3.947464652946276242, 36.72413553410236631 ) ) ;
#72840=CARTESIAN_POINT ( 'NONE',  ( -0.05219959533907301413, -21.53943276465977519, 97.49890960531436690 ) ) ;
#72841=CARTESIAN_POINT ( 'NONE',  ( -16.52544592524335698, -4.483927247898792601, 83.95942372801900433 ) ) ;
#72842=CARTESIAN_POINT ( 'NONE',  ( -16.53943276465976808, 0.05219959533911058130, 76.24890960531435269 ) ) ;
#72843=CARTESIAN_POINT ( 'NONE',  ( -17.44270441346515454, -5.991230190323027394, 101.3633507926422794 ) ) ;
#72844=CARTESIAN_POINT ( 'NONE',  ( -0.05219959533934338120, 16.53943276465976808, 27.50109039468567929 ) ) ;
#72846=CARTESIAN_POINT ( 'NONE',  ( 15.80617190586746368, 15.72974639402197994, 39.37390960531436690 ) ) ;
#72847=CARTESIAN_POINT ( 'NONE',  ( 4.379528057220092307, 16.55341960407617563, 72.29275706135236135 ) ) ;
#72848=CARTESIAN_POINT ( 'NONE',  ( -16.55341960407617563, 4.379528057220093196, 53.54275706135234714 ) ) ;
#72849=CARTESIAN_POINT ( 'NONE',  ( 10.72451020669871369, 18.67979575497193778, 32.08442372801901854 ) ) ;
#72850=CARTESIAN_POINT ( 'NONE',  ( 18.67979575497178502, 10.72451020669898547, 49.16557627198102409 ) ) ;
#72851=CARTESIAN_POINT ( 'NONE',  ( 12.14591786802327356, -12.06949235617739191, 75.62609039468567573 ) ) ;
#72852=CARTESIAN_POINT ( 'NONE',  ( -5.153800228976328057, -19.02544592524343514, 82.29057627198103830 ) ) ;
#72853=CARTESIAN_POINT ( 'NONE',  ( -5.823673210054431948, 21.52544592524334988, 57.70942372801901143 ) ) ;
#72854=CARTESIAN_POINT ( 'NONE',  ( 9.474510206698971260, -16.51473224551069308, 32.91557627198102409 ) ) ;
#72855=CARTESIAN_POINT ( 'NONE',  ( -10.81492255796078084, -18.62759615963271287, 42.08224293864769550 ) ) ;
#72856=CARTESIAN_POINT ( 'NONE',  ( -18.62759615963270932, 10.81492255796079327, 25.83224293864769194 ) ) ;
#72857=ORIENTED_EDGE ( 'NONE', *, *, #67133, .T. ) ;
#72858=CARTESIAN_POINT ( 'NONE',  ( 0.05219959533936267826, -19.03943276465977164, 45.00109039468566863 ) ) ;
#72859=CARTESIAN_POINT ( 'NONE',  ( -12.14591786802326823, 12.06949235617739902, 48.12609039468568284 ) ) ;
#72860=CARTESIAN_POINT ( 'NONE',  ( 13.89961937509977652, -13.97604488694527269, 108.1239096053143669 ) ) ;
#72861=ORIENTED_EDGE ( 'NONE', *, *, #62108, .F. ) ;
#72862=CARTESIAN_POINT ( 'NONE',  ( -0.05219959533909027116, -19.03943276465977164, 82.49890960531436690 ) ) ;
#72863=CARTESIAN_POINT ( 'NONE',  ( -16.53943276465976808, -0.05219959533934237506, 103.7510903946857042 ) ) ;
#72865=CARTESIAN_POINT ( 'NONE',  ( 16.53943276465976808, -0.05219959533910856209, 98.74890960531438111 ) ) ;
#72866=CARTESIAN_POINT ( 'NONE',  ( -10.81492255796078084, -18.62759615963271287, 32.08224293864769550 ) ) ;
#72867=CARTESIAN_POINT ( 'NONE',  ( -16.51473224551069308, -9.474510206698971260, 26.66557627198103120 ) ) ;
#72868=CARTESIAN_POINT ( 'NONE',  ( -14.29746914071037622, -8.314922557961029526, 84.16775706135234714 ) ) ;
#72869=CARTESIAN_POINT ( 'NONE',  ( 18.62759615963255655, 10.81492255796105972, 21.66775706135235069 ) ) ;
#72870=CARTESIAN_POINT ( 'NONE',  ( -9.474510206698720793, -16.51473224551083518, 74.58442372801900433 ) ) ;
#72871=CARTESIAN_POINT ( 'NONE',  ( -5.049401038298153566, 19.05341960407611168, 35.20724293864768839 ) ) ;
#72873=CARTESIAN_POINT ( 'NONE',  ( -0.05219959533909027116, -19.03943276465977164, 112.4989096053143669 ) ) ;
#72874=CARTESIAN_POINT ( 'NONE',  ( 21.55341960407619695, -5.719274019375665929, 106.0427570613523471 ) ) ;
#72875=CARTESIAN_POINT ( 'NONE',  ( 19.03943276465977164, -0.05219959533909143690, 63.74890960531435979 ) ) ;
#72876=CARTESIAN_POINT ( 'NONE',  ( 16.55341960407618274, -4.379528057220086978, 46.04275706135234714 ) ) ;
#72877=CARTESIAN_POINT ( 'NONE',  ( 21.52544592524334988, 5.823673210054432836, 86.45942372801901854 ) ) ;
#72878=CARTESIAN_POINT ( 'NONE',  ( -0.05219959533936034679, 19.03943276465977164, 47.50109039468566863 ) ) ;
#72879=CARTESIAN_POINT ( 'NONE',  ( 9.564922557961047289, -16.46253265017146816, 55.41775706135234003 ) ) ;
#72880=ORIENTED_EDGE ( 'NONE', *, *, #166372, .F. ) ;
#72881=CARTESIAN_POINT ( 'NONE',  ( -21.55341960407619339, 5.719274019375674811, 48.54275706135234714 ) ) ;
#72882=DIRECTION ( 'NONE',  ( -1.000000000000000000, 0.000000000000000000, 0.000000000000000000 ) ) ;
#72883=CARTESIAN_POINT ( 'NONE',  ( 13.89961937509957401, 13.97604488694547697, 46.87609039468565442 ) ) ;
#72884=CARTESIAN_POINT ( 'NONE',  ( -19.05341960407611168, -5.049401038298163336, 96.45724293864769550 ) ) ;
#72885=CARTESIAN_POINT ( 'NONE',  ( 5.049401038298161559, -19.05341960407611168, 77.70724293864765286 ) ) ;
#72886=CARTESIAN_POINT ( 'NONE',  ( 4.379528057220339221, -16.55341960407611168, 32.70724293864770260 ) ) ;
#72887=CARTESIAN_POINT ( 'NONE',  ( 5.823673210054125526, 21.52544592524343514, 29.79057627198102409 ) ) ;
#72891=CARTESIAN_POINT ( 'NONE',  ( -5.153800228976607833, 19.02544592524334988, 22.70942372801899012 ) ) ;
#72893=CARTESIAN_POINT ( 'NONE',  ( 16.46253265017160672, -9.564922557960803928, 43.33224293864769550 ) ) ;
#72894=CARTESIAN_POINT ( 'NONE',  ( 16.46253265017160672, -9.564922557960803928, 23.33224293864769194 ) ) ;
#72897=CARTESIAN_POINT ( 'NONE',  ( -0.05219959533934338120, 16.53943276465976808, 67.50109039468568994 ) ) ;
#72898=CARTESIAN_POINT ( 'NONE',  ( 18.67979575497178502, 10.72451020669898547, 89.16557627198102409 ) ) ;
#72899=CARTESIAN_POINT ( 'NONE',  ( 16.55341960407611168, 4.379528057220329451, 53.95724293864770260 ) ) ;
#72900=CARTESIAN_POINT ( 'NONE',  ( 19.05341960407611168, 5.049401038298154454, 28.95724293864769550 ) ) ;
#72901=CARTESIAN_POINT ( 'NONE',  ( 9.474510206698971260, -16.51473224551069308, 112.9155762719810383 ) ) ;
#72902=CARTESIAN_POINT ( 'NONE',  ( 10.72451020669871369, 18.67979575497193778, 32.08442372801901854 ) ) ;
#72903=CARTESIAN_POINT ( 'NONE',  ( 19.02544592524334988, 5.153800228976608722, 36.45942372801900433 ) ) ;
#72904=CARTESIAN_POINT ( 'NONE',  ( -13.97604488694527625, -13.89961937509977652, 36.87390960531436690 ) ) ;
#72905=CARTESIAN_POINT ( 'NONE',  ( -18.62759615963255300, -10.81492255796106328, 79.16775706135234714 ) ) ;
#72907=CARTESIAN_POINT ( 'NONE',  ( -4.379528057220328563, 16.55341960407611168, 25.20724293864769550 ) ) ;
#72909=CARTESIAN_POINT ( 'NONE',  ( 5.719274019375991003, -21.55341960407610458, 47.70724293864770260 ) ) ;
#72910=CARTESIAN_POINT ( 'NONE',  ( 0.05219959533910956823, 16.53943276465976808, 109.9989096053143527 ) ) ;
#72912=CARTESIAN_POINT ( 'NONE',  ( -19.02544592524342804, 5.153800228976336051, 86.04057627198103830 ) ) ;
#72913=CARTESIAN_POINT ( 'NONE',  ( 14.34966873604960469, 8.224510206698951720, 79.16557627198103830 ) ) ;
#72914=CARTESIAN_POINT ( 'NONE',  ( -19.02544592524334988, -5.153800228976617603, 103.9594237280190043 ) ) ;
#72916=CARTESIAN_POINT ( 'NONE',  ( 15.80617190586746368, 15.72974639402197994, 69.37390960531436690 ) ) ;
#72918=CARTESIAN_POINT ( 'NONE',  ( 19.02544592524343514, -5.153800228976328945, 28.54057627198102409 ) ) ;
#72919=CARTESIAN_POINT ( 'NONE',  ( -13.89961937509977652, 13.97604488694528158, 90.62390960531432427 ) ) ;
#72920=CARTESIAN_POINT ( 'NONE',  ( 18.62759615963271287, -10.81492255796078972, 93.33224293864769550 ) ) ;
#72921=CARTESIAN_POINT ( 'NONE',  ( 14.29746914071037800, 8.314922557961029526, 101.6677570613523613 ) ) ;
#72922=CARTESIAN_POINT ( 'NONE',  ( 5.049401038298161559, -19.05341960407611168, 92.70724293864769550 ) ) ;
#72923=CARTESIAN_POINT ( 'NONE',  ( 19.05341960407617918, -5.049401038297876454, 86.04275706135233293 ) ) ;
#72924=CARTESIAN_POINT ( 'NONE',  ( 18.62759615963255655, 10.81492255796105972, 96.66775706135234714 ) ) ;
#72925=CARTESIAN_POINT ( 'NONE',  ( 15.72974639402199770, -15.80617190586745480, 83.12390960531436690 ) ) ;
#72926=CARTESIAN_POINT ( 'NONE',  ( 15.80617190586746368, 15.72974639402197994, 39.37390960531436690 ) ) ;
#72927=CARTESIAN_POINT ( 'NONE',  ( 5.153800228976335163, 19.02544592524342804, 49.79057627198100988 ) ) ;
#72928=CARTESIAN_POINT ( 'NONE',  ( -4.483927247898539470, -16.52544592524342804, 27.29057627198103120 ) ) ;
#72929=CARTESIAN_POINT ( 'NONE',  ( 19.05341960407611168, 5.049401038298154454, 63.95724293864769550 ) ) ;
#72931=CARTESIAN_POINT ( 'NONE',  ( 13.97604488694548053, -13.89961937509957401, 25.62609039468566507 ) ) ;
#72932=CARTESIAN_POINT ( 'NONE',  ( -8.314922557960811034, -14.29746914071050412, 77.08224293864769550 ) ) ;
#72933=CARTESIAN_POINT ( 'NONE',  ( -18.67979575497178146, -10.72451020669898902, 111.6655762719810525 ) ) ;
#72935=CARTESIAN_POINT ( 'NONE',  ( -10.72451020669898014, 18.67979575497178502, 55.41557627198102409 ) ) ;
#72936=CARTESIAN_POINT ( 'NONE',  ( 16.52544592524335698, 4.483927247898782831, 91.45942372801901854 ) ) ;
#72937=CARTESIAN_POINT ( 'NONE',  ( -16.52544592524342804, 4.483927247898546575, 101.0405762719810383 ) ) ;
#72938=CARTESIAN_POINT ( 'NONE',  ( 5.153800228976335163, 19.02544592524342804, 59.79057627198100988 ) ) ;
#72940=CARTESIAN_POINT ( 'NONE',  ( -14.29746914071049879, 8.314922557960819915, 35.83224293864768839 ) ) ;
#72941=CARTESIAN_POINT ( 'NONE',  ( 21.55341960407619695, -5.719274019375665929, 41.04275706135236135 ) ) ;
#72942=CARTESIAN_POINT ( 'NONE',  ( -13.89961937509977652, 13.97604488694528158, 110.6239096053143243 ) ) ;
#72943=CARTESIAN_POINT ( 'NONE',  ( -18.62759615963255300, -10.81492255796106328, 79.16775706135234714 ) ) ;
#72944=CARTESIAN_POINT ( 'NONE',  ( -13.97604488694527625, -13.89961937509977652, 26.87390960531434558 ) ) ;
#72945=CARTESIAN_POINT ( 'NONE',  ( -5.049401038298153566, 19.05341960407611168, 40.20724293864768839 ) ) ;
#72947=CARTESIAN_POINT ( 'NONE',  ( 15.80617190586769283, -15.72974639402175789, 90.62609039468567573 ) ) ;
#72948=CARTESIAN_POINT ( 'NONE',  ( -16.52544592524335698, -4.483927247898792601, 43.95942372801902565 ) ) ;
#72949=CARTESIAN_POINT ( 'NONE',  ( 18.62759615963255655, 10.81492255796105972, 71.66775706135234714 ) ) ;
#72950=CARTESIAN_POINT ( 'NONE',  ( -0.05219959533909027116, -19.03943276465977164, 107.4989096053143527 ) ) ;
#72951=CARTESIAN_POINT ( 'NONE',  ( 9.474510206698729675, 16.51473224551082808, 87.08442372801900433 ) ) ;
#72952=CARTESIAN_POINT ( 'NONE',  ( -10.72451020669870658, -18.67979575497194134, 54.58442372801901143 ) ) ;
#72953=CARTESIAN_POINT ( 'NONE',  ( 19.02544592524334988, 5.153800228976608722, 111.4594237280190043 ) ) ;
#72955=CARTESIAN_POINT ( 'NONE',  ( -13.97604488694547697, 13.89961937509957934, 83.12609039468564731 ) ) ;
#72956=CARTESIAN_POINT ( 'NONE',  ( 19.05341960407611168, 5.049401038298154454, 53.95724293864770260 ) ) ;
#72957=CARTESIAN_POINT ( 'NONE',  ( -19.02544592524334988, -5.153800228976617603, 83.95942372801901854 ) ) ;
#72958=CARTESIAN_POINT ( 'NONE',  ( -14.34966873604972548, 8.224510206698743886, 113.3344237280190328 ) ) ;
#72959=CARTESIAN_POINT ( 'NONE',  ( 19.03943276465977164, 0.05219959533936151252, 91.25109039468566152 ) ) ;
#72960=CARTESIAN_POINT ( 'NONE',  ( -14.34966873604960291, -8.224510206698953496, 36.66557627198103120 ) ) ;
#72961=CARTESIAN_POINT ( 'NONE',  ( -9.564922557961040184, 16.46253265017147172, 67.91775706135233293 ) ) ;
#72962=CARTESIAN_POINT ( 'NONE',  ( 16.52544592524335698, 4.483927247898782831, 46.45942372801901854 ) ) ;
#72963=CARTESIAN_POINT ( 'NONE',  ( -9.564922557961040184, 16.46253265017147172, 27.91775706135232582 ) ) ;
#72964=CARTESIAN_POINT ( 'NONE',  ( 0.05219959533910956823, 16.53943276465976808, 114.9989096053143669 ) ) ;
#72965=CARTESIAN_POINT ( 'NONE',  ( 9.564922557960805705, 16.46253265017160317, 39.58224293864768839 ) ) ;
#72966=CARTESIAN_POINT ( 'NONE',  ( -16.52544592524335698, -4.483927247898792601, 43.95942372801902565 ) ) ;
#72969=CARTESIAN_POINT ( 'NONE',  ( -16.51473224551069308, -9.474510206698971260, 86.66557627198102409 ) ) ;
#72970=CARTESIAN_POINT ( 'NONE',  ( 17.66907692000856400, -2.165031582821545175, 102.5000000000000000 ) ) ;
#72971=ORIENTED_EDGE ( 'NONE', *, *, #80196, .T. ) ;
#72972=CARTESIAN_POINT ( 'NONE',  ( -16.51473224551082808, 9.474510206698731452, 93.33442372801900433 ) ) ;
#72973=CARTESIAN_POINT ( 'NONE',  ( -18.67979575497178146, -10.72451020669898902, 26.66557627198103475 ) ) ;
#72974=CARTESIAN_POINT ( 'NONE',  ( 16.51473224551083163, -9.474510206698727899, 25.83442372801900078 ) ) ;
#72975=CARTESIAN_POINT ( 'NONE',  ( -5.049401038297874678, -19.05341960407617918, 104.7927570613523471 ) ) ;
#72976=CARTESIAN_POINT ( 'NONE',  ( 16.53943276465976808, -0.05219959533910856209, 108.7489096053143669 ) ) ;
#72977=CARTESIAN_POINT ( 'NONE',  ( 5.153800228976335163, 19.02544592524342804, 34.79057627198102409 ) ) ;
#72978=CARTESIAN_POINT ( 'NONE',  ( 15.72974639402199770, -15.80617190586745480, 68.12390960531436690 ) ) ;
#72979=CARTESIAN_POINT ( 'NONE',  ( -0.05219959533909027116, -19.03943276465977164, 37.49890960531436690 ) ) ;
#72981=CARTESIAN_POINT ( 'NONE',  ( -16.46253265017146816, -9.564922557961047289, 74.16775706135234714 ) ) ;
#72982=CARTESIAN_POINT ( 'NONE',  ( 16.53943276465976808, -0.05219959533910856209, 58.74890960531436690 ) ) ;
#72983=CARTESIAN_POINT ( 'NONE',  ( 10.81492255796078972, 18.62759615963270932, 34.58224293864770260 ) ) ;
#72984=CARTESIAN_POINT ( 'NONE',  ( 15.80617190586769283, -15.72974639402175789, 90.62609039468567573 ) ) ;
#72985=CARTESIAN_POINT ( 'NONE',  ( 15.80617190586746368, 15.72974639402197994, 84.37390960531438111 ) ) ;
#72986=CARTESIAN_POINT ( 'NONE',  ( 5.719274019375673035, 21.55341960407619339, 77.29275706135234714 ) ) ;
#72987=CARTESIAN_POINT ( 'NONE',  ( -18.67979575497193778, 10.72451020669871902, 58.33442372801901143 ) ) ;
#72988=CARTESIAN_POINT ( 'NONE',  ( 19.05341960407611168, 5.049401038298154454, 98.95724293864766707 ) ) ;
#72989=CARTESIAN_POINT ( 'NONE',  ( -14.34966873604972548, 8.224510206698743886, 88.33442372801901854 ) ) ;
#72990=CARTESIAN_POINT ( 'NONE',  ( -10.81492255796105439, 18.62759615963255655, 62.91775706135236135 ) ) ;
#72991=CARTESIAN_POINT ( 'NONE',  ( 13.97604488694527802, 13.89961937509977652, 59.37390960531434558 ) ) ;
#72992=CARTESIAN_POINT ( 'NONE',  ( 21.52544592524334988, 5.823673210054432836, 36.45942372801901143 ) ) ;
#72993=CARTESIAN_POINT ( 'NONE',  ( 9.564922557960805705, 16.46253265017160317, 69.58224293864770971 ) ) ;
#72994=CARTESIAN_POINT ( 'NONE',  ( 4.483927247898545687, 16.52544592524342804, 64.79057627198103830 ) ) ;
#72995=CARTESIAN_POINT ( 'NONE',  ( 8.224510206698953496, -14.34966873604960469, 27.91557627198103830 ) ) ;
#72996=CARTESIAN_POINT ( 'NONE',  ( 18.62759615963271287, -10.81492255796078972, 48.33224293864770260 ) ) ;
#72998=CARTESIAN_POINT ( 'NONE',  ( -5.153800228976328057, -19.02544592524343514, 47.29057627198102409 ) ) ;
#72999=CARTESIAN_POINT ( 'NONE',  ( -0.05219959533907301413, -21.53943276465977519, 52.49890960531435979 ) ) ;
#73000=CARTESIAN_POINT ( 'NONE',  ( 16.51473224551083163, -9.474510206698727899, 55.83442372801899722 ) ) ;
#73002=CARTESIAN_POINT ( 'NONE',  ( 8.224510206698953496, -14.34966873604960469, 62.91557627198102409 ) ) ;
#73003=CARTESIAN_POINT ( 'NONE',  ( 21.52544592524344225, -5.823673210054117533, 38.54057627198103120 ) ) ;
#73004=ORIENTED_EDGE ( 'NONE', *, *, #146462, .T. ) ;
#73005=DIRECTION ( 'NONE',  ( 0.000000000000000000, 0.000000000000000000, -1.000000000000000000 ) ) ;
#73006=CARTESIAN_POINT ( 'NONE',  ( 0.05219959533934541429, -16.53943276465976808, 80.00109039468568994 ) ) ;
#73007=CARTESIAN_POINT ( 'NONE',  ( -9.564922557961040184, 16.46253265017147172, 87.91775706135233293 ) ) ;
#73008=CARTESIAN_POINT ( 'NONE',  ( -14.29746914071049879, 8.314922557960819915, 60.83224293864769550 ) ) ;
#73010=CARTESIAN_POINT ( 'NONE',  ( 9.564922557960805705, 16.46253265017160317, 54.58224293864769550 ) ) ;
#73011=CARTESIAN_POINT ( 'NONE',  ( -0.05219959533910754901, -16.53943276465976808, 37.49890960531436690 ) ) ;
#73012=CARTESIAN_POINT ( 'NONE',  ( -13.97604488694527625, -13.89961937509977652, 51.87390960531436690 ) ) ;
#73013=CARTESIAN_POINT ( 'NONE',  ( 19.02544592524343514, -5.153800228976328945, 78.54057627198099567 ) ) ;
#73014=CARTESIAN_POINT ( 'NONE',  ( -5.049401038298153566, 19.05341960407611168, 40.20724293864768839 ) ) ;
#73015=CARTESIAN_POINT ( 'NONE',  ( -21.52544592524334988, -5.823673210054445271, 48.95942372801902565 ) ) ;
#73016=CARTESIAN_POINT ( 'NONE',  ( 9.474510206698971260, -16.51473224551069308, 67.91557627198102409 ) ) ;
#73017=CARTESIAN_POINT ( 'NONE',  ( -9.474510206698964154, 16.51473224551069663, 25.41557627198103120 ) ) ;
#73018=CARTESIAN_POINT ( 'NONE',  ( 16.51473224551069308, 9.474510206698969483, 54.16557627198103120 ) ) ;
#73019=CARTESIAN_POINT ( 'NONE',  ( 10.81492255796078972, 18.62759615963270932, 49.58224293864769550 ) ) ;
#73020=CARTESIAN_POINT ( 'NONE',  ( 13.97604488694527802, 13.89961937509977652, 29.37390960531435979 ) ) ;
#73021=CARTESIAN_POINT ( 'NONE',  ( 18.67979575497178502, 10.72451020669898547, 44.16557627198103120 ) ) ;
#73022=CARTESIAN_POINT ( 'NONE',  ( 4.379528057220092307, 16.55341960407617563, 107.2927570613523471 ) ) ;
#73023=CARTESIAN_POINT ( 'NONE',  ( 13.97604488694548053, -13.89961937509957401, 25.62609039468566507 ) ) ;
#73024=CARTESIAN_POINT ( 'NONE',  ( 0.05219959533934541429, -16.53943276465976808, 50.00109039468568994 ) ) ;
#73025=CARTESIAN_POINT ( 'NONE',  ( -8.314922557961024197, 14.29746914071037800, 82.91775706135234714 ) ) ;
#73027=CARTESIAN_POINT ( 'NONE',  ( 0.05219959533934541429, -16.53943276465976808, 70.00109039468568994 ) ) ;
#73028=CARTESIAN_POINT ( 'NONE',  ( -4.483927247898782831, 16.52544592524335698, 57.70942372801901143 ) ) ;
#73029=CARTESIAN_POINT ( 'NONE',  ( -13.89961937509977652, 13.97604488694528158, 105.6239096053143527 ) ) ;
#73030=CARTESIAN_POINT ( 'NONE',  ( 16.53943276465976808, 0.05219959533934440121, 36.25109039468567573 ) ) ;
#73031=CARTESIAN_POINT ( 'NONE',  ( 13.89961937509977652, -13.97604488694527269, 33.12390960531434558 ) ) ;
#73032=CARTESIAN_POINT ( 'NONE',  ( 5.719274019375673035, 21.55341960407619339, 32.29275706135235424 ) ) ;
#73033=CARTESIAN_POINT ( 'NONE',  ( -16.52544592524335698, -4.483927247898792601, 38.95942372801901854 ) ) ;
#73034=CARTESIAN_POINT ( 'NONE',  ( -12.06949235617739369, -12.14591786802326823, 104.3760903946856899 ) ) ;
#73036=CARTESIAN_POINT ( 'NONE',  ( 15.72974639402176855, 15.80617190586768217, 106.8760903946856899 ) ) ;
#73037=CARTESIAN_POINT ( 'NONE',  ( -9.564922557961040184, 16.46253265017147172, 97.91775706135233293 ) ) ;
#73038=CARTESIAN_POINT ( 'NONE',  ( -12.14591786802309592, -12.06949235617757132, 61.87390960531436690 ) ) ;
#73039=CARTESIAN_POINT ( 'NONE',  ( 13.89961937509977652, -13.97604488694527269, 23.12390960531436335 ) ) ;
#73040=CARTESIAN_POINT ( 'NONE',  ( -0.05219959533936034679, 19.03943276465977164, 57.50109039468566863 ) ) ;
#73042=CARTESIAN_POINT ( 'NONE',  ( -18.67979575497193778, 10.72451020669871902, 63.33442372801900433 ) ) ;
#73043=CARTESIAN_POINT ( 'NONE',  ( -12.14591786802326823, 12.06949235617739902, 33.12609039468569705 ) ) ;
#73044=CARTESIAN_POINT ( 'NONE',  ( 16.21995358207306737, 7.366697692864124569, 82.56448998487843483 ) ) ;
#73045=CARTESIAN_POINT ( 'NONE',  ( -16.46253265017160317, 9.564922557960807481, 115.8322429386477097 ) ) ;
#73046=CARTESIAN_POINT ( 'NONE',  ( 13.89961937509957401, 13.97604488694547697, 111.8760903946856757 ) ) ;
#73049=CARTESIAN_POINT ( 'NONE',  ( -12.06949235617756955, 12.14591786802309770, 115.6239096053143669 ) ) ;
#73050=CARTESIAN_POINT ( 'NONE',  ( 5.823673210054444382, -21.52544592524334988, 105.2094237280190328 ) ) ;
#73051=CARTESIAN_POINT ( 'NONE',  ( 13.89961937509977652, -13.97604488694527269, 43.12390960531434558 ) ) ;
#73053=CARTESIAN_POINT ( 'NONE',  ( 18.67979575497194134, -10.72451020669871369, 55.83442372801901854 ) ) ;
#73054=CARTESIAN_POINT ( 'NONE',  ( 18.67979575497194134, -10.72451020669871369, 100.8344237280190185 ) ) ;
#73055=CARTESIAN_POINT ( 'NONE',  ( 0.05219959533934541429, -16.53943276465976808, 105.0010903946856757 ) ) ;
#73056=CARTESIAN_POINT ( 'NONE',  ( -13.97604488694527625, -13.89961937509977652, 76.87390960531433848 ) ) ;
#73057=CARTESIAN_POINT ( 'NONE',  ( -21.55341960407619339, 5.719274019375674811, 43.54275706135235424 ) ) ;
#73058=CARTESIAN_POINT ( 'NONE',  ( -10.81492255796105439, 18.62759615963255655, 57.91775706135234714 ) ) ;
#73059=CARTESIAN_POINT ( 'NONE',  ( 19.02544592524334988, 5.153800228976608722, 81.45942372801897591 ) ) ;
#73060=CARTESIAN_POINT ( 'NONE',  ( 16.46253265017160672, -9.564922557960803928, 98.33224293864769550 ) ) ;
#73061=CARTESIAN_POINT ( 'NONE',  ( 14.34966873604960469, 8.224510206698951720, 104.1655762719810241 ) ) ;
#73062=CARTESIAN_POINT ( 'NONE',  ( -5.823673210054116645, -21.52544592524344225, 97.29057627198105251 ) ) ;
#73063=CARTESIAN_POINT ( 'NONE',  ( -5.049401038297874678, -19.05341960407617918, 24.79275706135233648 ) ) ;
#73064=CARTESIAN_POINT ( 'NONE',  ( -16.52544592524342804, 4.483927247898546575, 96.04057627198102409 ) ) ;
#73065=CARTESIAN_POINT ( 'NONE',  ( -5.153800228976328057, -19.02544592524343514, 47.29057627198102409 ) ) ;
#73066=CARTESIAN_POINT ( 'NONE',  ( 16.46253265017146816, 9.564922557961045513, 81.66775706135233293 ) ) ;
#73067=CARTESIAN_POINT ( 'NONE',  ( 16.53943276465976808, -0.05219959533910856209, 43.74890960531435979 ) ) ;
#73068=CARTESIAN_POINT ( 'NONE',  ( -18.67979575497193778, 10.72451020669871902, 113.3344237280190328 ) ) ;
#73069=CARTESIAN_POINT ( 'NONE',  ( -19.02544592524342804, 5.153800228976336051, 111.0405762719810099 ) ) ;
#73070=CARTESIAN_POINT ( 'NONE',  ( 0.05219959533936267826, -19.03943276465977164, 80.00109039468567573 ) ) ;
#73071=CARTESIAN_POINT ( 'NONE',  ( 21.53943276465977519, -0.05219959533907433946, 83.74890960531435269 ) ) ;
#73072=CARTESIAN_POINT ( 'NONE',  ( -0.05219959533937732626, 21.53943276465977519, 27.50109039468567929 ) ) ;
#73073=CARTESIAN_POINT ( 'NONE',  ( -12.06949235617739369, -12.14591786802326823, 34.37609039468568284 ) ) ;
#73074=CARTESIAN_POINT ( 'NONE',  ( -12.06949235617739369, -12.14591786802326823, 89.37609039468568994 ) ) ;
#73075=CARTESIAN_POINT ( 'NONE',  ( -19.02544592524342804, 5.153800228976336051, 26.04057627198103120 ) ) ;
#73076=CARTESIAN_POINT ( 'NONE',  ( 10.81492255796106328, -18.62759615963255655, 30.41775706135234358 ) ) ;
#73077=CARTESIAN_POINT ( 'NONE',  ( -15.72974639402197994, 15.80617190586746368, 45.62390960531436690 ) ) ;
#73078=CARTESIAN_POINT ( 'NONE',  ( -12.06949235617756955, 12.14591786802309770, 110.6239096053143669 ) ) ;
#73080=CARTESIAN_POINT ( 'NONE',  ( -12.14591786802326823, 12.06949235617739902, 63.12609039468568994 ) ) ;
#73081=EDGE_CURVE ( 'NONE', #17083, #132603, #186462, .T. ) ;
#73082=CARTESIAN_POINT ( 'NONE',  ( 12.06949235617757843, -12.14591786802309237, 88.12390960531436690 ) ) ;
#73083=CARTESIAN_POINT ( 'NONE',  ( 18.62759615963271287, -10.81492255796078972, 73.33224293864769550 ) ) ;
#73084=CARTESIAN_POINT ( 'NONE',  ( 8.224510206698742110, 14.34966873604972548, 112.0844237280190185 ) ) ;
#73085=CARTESIAN_POINT ( 'NONE',  ( -14.34966873604972548, 8.224510206698743886, 53.33442372801901854 ) ) ;
#73086=CARTESIAN_POINT ( 'NONE',  ( -19.03943276465977164, 0.05219959533909376836, 56.24890960531435979 ) ) ;
#73087=CARTESIAN_POINT ( 'NONE',  ( 8.224510206698742110, 14.34966873604972548, 87.08442372801901854 ) ) ;
#73088=CARTESIAN_POINT ( 'NONE',  ( 16.46253265017146816, 9.564922557961045513, 86.66775706135233293 ) ) ;
#73089=CARTESIAN_POINT ( 'NONE',  ( 18.67979575497178502, 10.72451020669898547, 84.16557627198103830 ) ) ;
#73090=CARTESIAN_POINT ( 'NONE',  ( 16.55341960407618274, -4.379528057220086978, 106.0427570613523471 ) ) ;
#73093=CARTESIAN_POINT ( 'NONE',  ( 0.05219959533907565091, 21.53943276465977519, 59.99890960531436690 ) ) ;
#73094=CARTESIAN_POINT ( 'NONE',  ( -12.06949235617739369, -12.14591786802326823, 89.37609039468568994 ) ) ;
#73096=CARTESIAN_POINT ( 'NONE',  ( -5.823673210054116645, -21.52544592524344225, 32.29057627198102409 ) ) ;
#73097=CARTESIAN_POINT ( 'NONE',  ( -18.56453257813363678, 5.500000000000057732, 75.99000423690684158 ) ) ;
#73098=CARTESIAN_POINT ( 'NONE',  ( 5.823673210054125526, 21.52544592524343514, 84.79057627198102409 ) ) ;
#73099=AXIS2_PLACEMENT_3D ( 'NONE', #77101, #152943, #1241 ) ;
#73100=CARTESIAN_POINT ( 'NONE',  ( -12.06949235617756955, 12.14591786802309770, 30.62390960531436335 ) ) ;
#73101=CARTESIAN_POINT ( 'NONE',  ( -4.483927247898782831, 16.52544592524335698, 32.70942372801900433 ) ) ;
#73102=CARTESIAN_POINT ( 'NONE',  ( 0.05219959533909260263, 19.03943276465977164, 39.99890960531436690 ) ) ;
#73103=CARTESIAN_POINT ( 'NONE',  ( -8.224510206698735004, -14.34966873604973081, 24.58442372801901499 ) ) ;
#73105=CARTESIAN_POINT ( 'NONE',  ( -0.05219959533909027116, -19.03943276465977164, 52.49890960531436690 ) ) ;
#73107=CARTESIAN_POINT ( 'NONE',  ( -9.564922557960796823, -16.46253265017161027, 107.0822429386476955 ) ) ;
#73108=CARTESIAN_POINT ( 'NONE',  ( 16.46253265017160672, -9.564922557960803928, 103.3322429386476955 ) ) ;
#73109=CARTESIAN_POINT ( 'NONE',  ( -8.224510206698735004, -14.34966873604973081, 99.58442372801900433 ) ) ;
#73110=CARTESIAN_POINT ( 'NONE',  ( -16.51473224551082808, 9.474510206698731452, 98.33442372801900433 ) ) ;
#73111=CARTESIAN_POINT ( 'NONE',  ( 13.89961937509957401, 13.97604488694547697, 41.87609039468566152 ) ) ;
#73112=CARTESIAN_POINT ( 'NONE',  ( -15.80617190586745835, -15.72974639402198527, 71.87390960531438111 ) ) ;
#73113=CARTESIAN_POINT ( 'NONE',  ( -4.483927247898782831, 16.52544592524335698, 102.7094237280190185 ) ) ;
#73114=B_SPLINE_CURVE_WITH_KNOTS ( 'NONE', 3,
 ( #105974, #42334, #89818, #165673, #27172, #58483 ),
 .UNSPECIFIED., .F., .F.,
 ( 4, 2, 4 ),
 ( 0.003239945802372203986, 0.003620412082092052709, 0.004000878361811900999 ),
 .UNSPECIFIED. ) ;
#73115=CARTESIAN_POINT ( 'NONE',  ( 18.67979575497178502, 10.72451020669898547, 34.16557627198102409 ) ) ;
#73116=CARTESIAN_POINT ( 'NONE',  ( 16.46253265017146816, 9.564922557961045513, 96.66775706135233293 ) ) ;
#73117=CARTESIAN_POINT ( 'NONE',  ( 0.05219959533909260263, 19.03943276465977164, 49.99890960531435979 ) ) ;
#73118=CARTESIAN_POINT ( 'NONE',  ( -5.153800228976328057, -19.02544592524343514, 102.2905762719810383 ) ) ;
#73119=CARTESIAN_POINT ( 'NONE',  ( 15.72974639402176855, 15.80617190586768217, 66.87609039468568994 ) ) ;
#73120=CARTESIAN_POINT ( 'NONE',  ( -9.564922557960796823, -16.46253265017161027, 67.08224293864769550 ) ) ;
#73121=CARTESIAN_POINT ( 'NONE',  ( 0.05219959533910956823, 16.53943276465976808, 104.9989096053143669 ) ) ;
#73122=CARTESIAN_POINT ( 'NONE',  ( -17.44270441346519007, -5.991230190322947458, 86.36335079264233627 ) ) ;
#73123=CARTESIAN_POINT ( 'NONE',  ( 16.55341960407611168, 4.379528057220329451, 83.95724293864770971 ) ) ;
#73124=CARTESIAN_POINT ( 'NONE',  ( -15.80617190586745835, -15.72974639402198527, 76.87390960531439532 ) ) ;
#73126=CARTESIAN_POINT ( 'NONE',  ( -5.153800228976607833, 19.02544592524334988, 87.70942372801897591 ) ) ;
#73127=CARTESIAN_POINT ( 'NONE',  ( 17.50000000000001066, -5.622605283950866450, 81.18792689403893803 ) ) ;
#73128=CARTESIAN_POINT ( 'NONE',  ( 13.97604488694527802, 13.89961937509977652, 64.37390960531436690 ) ) ;
#73130=CARTESIAN_POINT ( 'NONE',  ( -0.05219959533909027116, -19.03943276465977164, 72.49890960531435269 ) ) ;
#73131=CARTESIAN_POINT ( 'NONE',  ( 19.02544592524343514, -5.153800228976328945, 88.54057627198102409 ) ) ;
#73132=CARTESIAN_POINT ( 'NONE',  ( -14.34966873604972548, 8.224510206698743886, 58.33442372801901143 ) ) ;
#73133=CARTESIAN_POINT ( 'NONE',  ( -16.62475595723696742, -7.163666690055265462, 49.47286648189535185 ) ) ;
#73134=CARTESIAN_POINT ( 'NONE',  ( 16.46253265017146816, 9.564922557961045513, 41.66775706135234003 ) ) ;
#73136=CARTESIAN_POINT ( 'NONE',  ( -9.474510206698964154, 16.51473224551069663, 110.4155762719810383 ) ) ;
#73137=CARTESIAN_POINT ( 'NONE',  ( -14.34966873604972548, 8.224510206698743886, 98.33442372801901854 ) ) ;
#73139=CARTESIAN_POINT ( 'NONE',  ( 0.05219959533934541429, -16.53943276465976808, 95.00109039468568994 ) ) ;
#73140=CARTESIAN_POINT ( 'NONE',  ( -17.49999999999999645, 5.622605283950868227, 28.68792689403889895 ) ) ;
#73141=CARTESIAN_POINT ( 'NONE',  ( -4.483927247898782831, 16.52544592524335698, 67.70942372801901854 ) ) ;
#73143=CARTESIAN_POINT ( 'NONE',  ( -21.53943276465977519, -0.05219959533937600094, 73.75109039468567573 ) ) ;
#73144=CARTESIAN_POINT ( 'NONE',  ( -9.474510206698720793, -16.51473224551083518, 74.58442372801900433 ) ) ;
#73145=CARTESIAN_POINT ( 'NONE',  ( 13.89961937509957401, 13.97604488694547697, 26.87609039468566507 ) ) ;
#73146=CARTESIAN_POINT ( 'NONE',  ( 19.02544592524343514, -5.153800228976328945, 63.54057627198103830 ) ) ;
#73147=CARTESIAN_POINT ( 'NONE',  ( -9.564922557960796823, -16.46253265017161027, 42.08224293864769550 ) ) ;
#73149=CARTESIAN_POINT ( 'NONE',  ( 21.55341960407610458, 5.719274019375980345, 83.95724293864770971 ) ) ;
#73150=CARTESIAN_POINT ( 'NONE',  ( -10.72451020669898014, 18.67979575497178502, 35.41557627198102409 ) ) ;
#73151=CARTESIAN_POINT ( 'NONE',  ( -16.51473224551069308, -9.474510206698971260, 36.66557627198102409 ) ) ;
#73152=CARTESIAN_POINT ( 'NONE',  ( -16.52544592524335698, -4.483927247898792601, 48.95942372801902565 ) ) ;
#73155=CARTESIAN_POINT ( 'NONE',  ( 10.72451020669871369, 18.67979575497193778, 32.08442372801901854 ) ) ;
#73156=CARTESIAN_POINT ( 'NONE',  ( -14.34966873604960291, -8.224510206698953496, 56.66557627198103830 ) ) ;
#73158=CARTESIAN_POINT ( 'NONE',  ( -8.224510206698735004, -14.34966873604973081, 29.58442372801901854 ) ) ;
#73159=CARTESIAN_POINT ( 'NONE',  ( 16.51473224551083163, -9.474510206698727899, 35.83442372801899722 ) ) ;
#73160=CARTESIAN_POINT ( 'NONE',  ( -12.14591786802309592, -12.06949235617757132, 61.87390960531436690 ) ) ;
#73161=CARTESIAN_POINT ( 'NONE',  ( -18.62759615963270932, 10.81492255796079327, 110.8322429386476955 ) ) ;
#73163=CARTESIAN_POINT ( 'NONE',  ( -5.823673210054116645, -21.52544592524344225, 82.29057627198103830 ) ) ;
#73164=CARTESIAN_POINT ( 'NONE',  ( -19.02544592524342804, 5.153800228976336051, 96.04057627198103830 ) ) ;
#73165=CARTESIAN_POINT ( 'NONE',  ( -16.55341960407611168, -4.379528057220339221, 66.45724293864768129 ) ) ;
#73166=CARTESIAN_POINT ( 'NONE',  ( 9.564922557960805705, 16.46253265017160317, 99.58224293864770971 ) ) ;
#73168=CARTESIAN_POINT ( 'NONE',  ( 16.46253265017146816, 9.564922557961045513, 71.66775706135233293 ) ) ;
#73169=CARTESIAN_POINT ( 'NONE',  ( -21.55341960407610458, -5.719274019375992779, 101.4572429386476955 ) ) ;
#73170=CARTESIAN_POINT ( 'NONE',  ( 19.05341960407611168, 5.049401038298154454, 58.95724293864768129 ) ) ;
#73171=CARTESIAN_POINT ( 'NONE',  ( 19.03943276465977164, 0.05219959533936151252, 46.25109039468566863 ) ) ;
#73172=CARTESIAN_POINT ( 'NONE',  ( 14.34966873604960469, 8.224510206698951720, 114.1655762719810383 ) ) ;
#73173=CARTESIAN_POINT ( 'NONE',  ( -21.55341960407619339, 5.719274019375674811, 58.54275706135235424 ) ) ;
#73174=CARTESIAN_POINT ( 'NONE',  ( -17.12812012977030562, -6.668231424565919774, 71.35948759323142099 ) ) ;
#73175=CARTESIAN_POINT ( 'NONE',  ( 4.483927247898545687, 16.52544592524342804, 44.79057627198103120 ) ) ;
#73176=CARTESIAN_POINT ( 'NONE',  ( -19.02544592524342804, 5.153800228976336051, 51.04057627198103120 ) ) ;
#73177=CARTESIAN_POINT ( 'NONE',  ( -5.049401038298153566, 19.05341960407611168, 115.2072429386477097 ) ) ;
#73178=CARTESIAN_POINT ( 'NONE',  ( -18.62759615963270932, 10.81492255796079327, 70.83224293864770971 ) ) ;
#73180=CARTESIAN_POINT ( 'NONE',  ( 9.564922557960805705, 16.46253265017160317, 49.58224293864770260 ) ) ;
#73181=CARTESIAN_POINT ( 'NONE',  ( -15.72974639402197994, 15.80617190586746368, 65.62390960531436690 ) ) ;
#73183=CARTESIAN_POINT ( 'NONE',  ( 0.05219959533937995610, -21.53943276465977519, 90.00109039468567573 ) ) ;
#73185=CARTESIAN_POINT ( 'NONE',  ( 16.53943276465976808, 0.05219959533934440121, 96.25109039468568994 ) ) ;
#73186=CARTESIAN_POINT ( 'NONE',  ( 16.53943276465976808, -0.05219959533910856209, 88.74890960531436690 ) ) ;
#73187=CARTESIAN_POINT ( 'NONE',  ( 19.02544592524343514, -5.153800228976328945, 73.54057627198103830 ) ) ;
#73189=CARTESIAN_POINT ( 'NONE',  ( 5.153800228976615827, -19.02544592524334988, 40.20942372801898301 ) ) ;
#73190=CARTESIAN_POINT ( 'NONE',  ( 8.224510206698742110, 14.34966873604972548, 82.08442372801901854 ) ) ;
#73191=CARTESIAN_POINT ( 'NONE',  ( -19.05341960407617563, 5.049401038297882671, 23.54275706135233648 ) ) ;
#73192=CARTESIAN_POINT ( 'NONE',  ( 16.46253265017160672, -9.564922557960803928, 83.33224293864768129 ) ) ;
#73193=CARTESIAN_POINT ( 'NONE',  ( 0.05219959533907565091, 21.53943276465977519, 44.99890960531435979 ) ) ;
#73195=CARTESIAN_POINT ( 'NONE',  ( -21.52544592524334988, -5.823673210054445271, 98.95942372801903275 ) ) ;
#73196=CARTESIAN_POINT ( 'NONE',  ( -14.34966873604972548, 8.224510206698743886, 58.33442372801901143 ) ) ;
#73197=CARTESIAN_POINT ( 'NONE',  ( 21.52544592524344225, -5.823673210054117533, 108.5405762719810241 ) ) ;
#73198=CARTESIAN_POINT ( 'NONE',  ( 8.224510206698742110, 14.34966873604972548, 37.08442372801901143 ) ) ;
#73199=CARTESIAN_POINT ( 'NONE',  ( 13.97604488694527802, 13.89961937509977652, 89.37390960531436690 ) ) ;
#73200=CARTESIAN_POINT ( 'NONE',  ( 9.564922557960805705, 16.46253265017160317, 34.58224293864770260 ) ) ;
#73201=CARTESIAN_POINT ( 'NONE',  ( -0.05219959533909027116, -19.03943276465977164, 47.49890960531435979 ) ) ;
#73202=CARTESIAN_POINT ( 'NONE',  ( -16.55341960407617563, 4.379528057220093196, 28.54275706135234358 ) ) ;
#73203=CARTESIAN_POINT ( 'NONE',  ( 8.314922557960818139, 14.29746914071049879, 79.58224293864769550 ) ) ;
#73204=CARTESIAN_POINT ( 'NONE',  ( -8.314922557961024197, 14.29746914071037800, 92.91775706135236135 ) ) ;
#73205=CARTESIAN_POINT ( 'NONE',  ( 15.72974639402176855, 15.80617190586768217, 41.87609039468568284 ) ) ;
#73206=CARTESIAN_POINT ( 'NONE',  ( -16.51473224551069308, -9.474510206698971260, 71.66557627198102409 ) ) ;
#73207=CARTESIAN_POINT ( 'NONE',  ( 5.049401038298161559, -19.05341960407611168, 57.70724293864769550 ) ) ;
#73208=CARTESIAN_POINT ( 'NONE',  ( -13.89961937509977652, 13.97604488694528158, 85.62390960531433848 ) ) ;
#73209=CARTESIAN_POINT ( 'NONE',  ( -12.06949235617756955, 12.14591786802309770, 30.62390960531436335 ) ) ;
#73210=CARTESIAN_POINT ( 'NONE',  ( 4.483927247898790824, -16.52544592524335698, 90.20942372801903275 ) ) ;
#73211=ORIENTED_EDGE ( 'NONE', *, *, #187522, .F. ) ;
#73212=CARTESIAN_POINT ( 'NONE',  ( 9.564922557961047289, -16.46253265017146816, 25.41775706135234003 ) ) ;
#73213=CARTESIAN_POINT ( 'NONE',  ( -19.05341960407611168, -5.049401038298163336, 96.45724293864769550 ) ) ;
#73214=CARTESIAN_POINT ( 'NONE',  ( 9.474510206698971260, -16.51473224551069308, 47.91557627198102409 ) ) ;
#73216=CARTESIAN_POINT ( 'NONE',  ( 16.53943276465976808, 0.05219959533934440121, 41.25109039468568284 ) ) ;
#73217=CARTESIAN_POINT ( 'NONE',  ( -5.049401038297874678, -19.05341960407617918, 74.79275706135231871 ) ) ;
#73218=CARTESIAN_POINT ( 'NONE',  ( 16.55341960407618274, -4.379528057220086978, 56.04275706135235424 ) ) ;
#73220=CARTESIAN_POINT ( 'NONE',  ( 5.153800228976335163, 19.02544592524342804, 74.79057627198103830 ) ) ;
#73221=CARTESIAN_POINT ( 'NONE',  ( -21.52544592524334988, -5.823673210054445271, 18.95942372801901143 ) ) ;
#73222=CARTESIAN_POINT ( 'NONE',  ( -19.03943276465977164, -0.05219959533935918106, 63.75109039468566863 ) ) ;
#73223=CARTESIAN_POINT ( 'NONE',  ( 19.05341960407611168, 5.049401038298154454, 108.9572429386477097 ) ) ;
#73224=CARTESIAN_POINT ( 'NONE',  ( 9.564922557960805705, 16.46253265017160317, 34.58224293864770260 ) ) ;
#73225=CARTESIAN_POINT ( 'NONE',  ( -5.153800228976328057, -19.02544592524343514, 82.29057627198103830 ) ) ;
#73226=CARTESIAN_POINT ( 'NONE',  ( -16.52544592524342804, 4.483927247898546575, 41.04057627198103120 ) ) ;
#73227=CARTESIAN_POINT ( 'NONE',  ( -5.049401038298153566, 19.05341960407611168, 70.20724293864769550 ) ) ;
#73228=CARTESIAN_POINT ( 'NONE',  ( 9.474510206698729675, 16.51473224551082808, 37.08442372801899722 ) ) ;
#73229=CARTESIAN_POINT ( 'NONE',  ( 12.14591786802309770, 12.06949235617756955, 79.37390960531436690 ) ) ;
#73230=CARTESIAN_POINT ( 'NONE',  ( 16.46253265017146816, 9.564922557961045513, 21.66775706135233648 ) ) ;
#73231=CARTESIAN_POINT ( 'NONE',  ( 19.02544592524343514, -5.153800228976328945, 48.54057627198103120 ) ) ;
#73232=CARTESIAN_POINT ( 'NONE',  ( -8.224510206698948167, 14.34966873604960824, 35.41557627198102409 ) ) ;
#73233=CARTESIAN_POINT ( 'NONE',  ( 5.719274019375673035, 21.55341960407619339, 107.2927570613523471 ) ) ;
#73234=CARTESIAN_POINT ( 'NONE',  ( 0.05219959533909260263, 19.03943276465977164, 89.99890960531436690 ) ) ;
#73235=CARTESIAN_POINT ( 'NONE',  ( -16.46253265017160317, 9.564922557960807481, 105.8322429386476955 ) ) ;
#73236=CARTESIAN_POINT ( 'NONE',  ( -5.049401038298153566, 19.05341960407611168, 45.20724293864769550 ) ) ;
#73237=CARTESIAN_POINT ( 'NONE',  ( 13.89961937509977652, -13.97604488694527269, 28.12390960531435624 ) ) ;
#73238=CARTESIAN_POINT ( 'NONE',  ( -0.05219959533910754901, -16.53943276465976808, 82.49890960531436690 ) ) ;
#73239=CARTESIAN_POINT ( 'NONE',  ( 10.72451020669898902, -18.67979575497178502, 102.9155762719810383 ) ) ;
#73240=CARTESIAN_POINT ( 'NONE',  ( 9.564922557960805705, 16.46253265017160317, 94.58224293864769550 ) ) ;
#73241=CARTESIAN_POINT ( 'NONE',  ( 5.719274019375991003, -21.55341960407610458, 92.70724293864770971 ) ) ;
#73242=CARTESIAN_POINT ( 'NONE',  ( 13.89961937509977652, -13.97604488694527269, 93.12390960531436690 ) ) ;
#73243=DIRECTION ( 'NONE',  ( -0.000000000000000000, 0.000000000000000000, 1.000000000000000000 ) ) ;
#73244=CARTESIAN_POINT ( 'NONE',  ( -16.52544592524342804, 4.483927247898546575, 101.0405762719810383 ) ) ;
#73246=CARTESIAN_POINT ( 'NONE',  ( -9.564922557960796823, -16.46253265017161027, 67.08224293864769550 ) ) ;
#73247=CARTESIAN_POINT ( 'NONE',  ( 18.62759615963271287, -10.81492255796078972, 73.33224293864769550 ) ) ;
#73249=CARTESIAN_POINT ( 'NONE',  ( 5.719274019375991003, -21.55341960407610458, 22.70724293864769194 ) ) ;
#73251=CARTESIAN_POINT ( 'NONE',  ( -16.53943276465976808, -0.05219959533934237506, 38.75109039468567573 ) ) ;
#73252=CARTESIAN_POINT ( 'NONE',  ( -0.05219959533910754901, -16.53943276465976808, 97.49890960531436690 ) ) ;
#73254=CARTESIAN_POINT ( 'NONE',  ( -5.153800228976328057, -19.02544592524343514, 92.29057627198099567 ) ) ;
#73255=CARTESIAN_POINT ( 'NONE',  ( 5.153800228976335163, 19.02544592524342804, 49.79057627198100988 ) ) ;
#73256=CARTESIAN_POINT ( 'NONE',  ( 4.379528057220339221, -16.55341960407611168, 77.70724293864770971 ) ) ;
#73258=CARTESIAN_POINT ( 'NONE',  ( -5.823673210054116645, -21.52544592524344225, 22.29057627198102765 ) ) ;
#73259=CARTESIAN_POINT ( 'NONE',  ( 12.06949235617757843, -12.14591786802309237, 58.12390960531435979 ) ) ;
#73260=CARTESIAN_POINT ( 'NONE',  ( 19.03943276465977164, 0.05219959533936151252, 96.25109039468567573 ) ) ;
#73261=CARTESIAN_POINT ( 'NONE',  ( -5.719274019375665041, -21.55341960407619695, 59.79275706135234714 ) ) ;
#73263=CARTESIAN_POINT ( 'NONE',  ( -9.564922557960796823, -16.46253265017161027, 102.0822429386477097 ) ) ;
#73264=CARTESIAN_POINT ( 'NONE',  ( -8.224510206698735004, -14.34966873604973081, 89.58442372801901854 ) ) ;
#73265=LINE ( 'NONE', #167250, #129122 ) ;
#73266=CARTESIAN_POINT ( 'NONE',  ( 16.46253265017160672, -9.564922557960803928, 78.33224293864769550 ) ) ;
#73267=CARTESIAN_POINT ( 'NONE',  ( 18.62759615963271287, -10.81492255796078972, 83.33224293864769550 ) ) ;
#73268=CARTESIAN_POINT ( 'NONE',  ( 9.474510206698729675, 16.51473224551082808, 112.0844237280190043 ) ) ;
#73269=CARTESIAN_POINT ( 'NONE',  ( 8.224510206698953496, -14.34966873604960469, 57.91557627198103120 ) ) ;
#73270=CARTESIAN_POINT ( 'NONE',  ( -5.719274019375665041, -21.55341960407619695, 64.79275706135234714 ) ) ;
#73271=CARTESIAN_POINT ( 'NONE',  ( 12.14591786802327356, -12.06949235617739191, 80.62609039468567573 ) ) ;
#73272=CARTESIAN_POINT ( 'NONE',  ( -15.80617190586745835, -15.72974639402198527, 26.87390960531435979 ) ) ;
#73273=CARTESIAN_POINT ( 'NONE',  ( 13.89961937509978007, -13.97604488694527269, 113.1239096053143669 ) ) ;
#73275=CARTESIAN_POINT ( 'NONE',  ( -8.314922557961024197, 14.29746914071037800, 107.9177570613523471 ) ) ;
#73276=CARTESIAN_POINT ( 'NONE',  ( 16.52544592524335698, 4.483927247898782831, 66.45942372801903275 ) ) ;
#73277=CARTESIAN_POINT ( 'NONE',  ( 13.97604488694527802, 13.89961937509977652, 69.37390960531436690 ) ) ;
#73278=CARTESIAN_POINT ( 'NONE',  ( 19.03943276465977164, -0.05219959533909143690, 83.74890960531436690 ) ) ;
#73279=CARTESIAN_POINT ( 'NONE',  ( -21.55341960407619339, 5.719274019375674811, 78.54275706135236135 ) ) ;
#73280=CARTESIAN_POINT ( 'NONE',  ( -4.379528057220086978, -16.55341960407618274, 79.79275706135236135 ) ) ;
#73281=CARTESIAN_POINT ( 'NONE',  ( 12.06949235617757843, -12.14591786802309237, 53.12390960531436690 ) ) ;
#73282=CARTESIAN_POINT ( 'NONE',  ( 5.049401038298161559, -19.05341960407611168, 52.70724293864767418 ) ) ;
#73283=CARTESIAN_POINT ( 'NONE',  ( -19.05341960407611168, -5.049401038298163336, 51.45724293864770260 ) ) ;
#73284=CARTESIAN_POINT ( 'NONE',  ( 8.314922557961029526, -14.29746914071037800, 45.41775706135234003 ) ) ;
#73285=ORIENTED_EDGE ( 'NONE', *, *, #20112, .T. ) ;
#73286=CARTESIAN_POINT ( 'NONE',  ( 16.51473224551083163, -9.474510206698727899, 100.8344237280190043 ) ) ;
#73287=CARTESIAN_POINT ( 'NONE',  ( -4.379528057220328563, 16.55341960407611168, 100.2072429386476955 ) ) ;
#73288=CARTESIAN_POINT ( 'NONE',  ( -13.89961937509977652, 13.97604488694528158, 60.62390960531436690 ) ) ;
#73289=CARTESIAN_POINT ( 'NONE',  ( 13.97604488694548053, -13.89961937509957401, 105.6260903946856757 ) ) ;
#73291=CARTESIAN_POINT ( 'NONE',  ( -21.53943276465977519, -0.05219959533937600094, 103.7510903946857042 ) ) ;
#73292=CARTESIAN_POINT ( 'NONE',  ( -16.53943276465976808, -0.05219959533934237506, 63.75109039468568284 ) ) ;
#73294=CARTESIAN_POINT ( 'NONE',  ( -21.52544592524343514, 5.823673210054127303, 66.04057627198103830 ) ) ;
#73295=CARTESIAN_POINT ( 'NONE',  ( 4.379528057220092307, 16.55341960407617563, 47.29275706135234003 ) ) ;
#73297=CARTESIAN_POINT ( 'NONE',  ( -5.153800228976607833, 19.02544592524334988, 47.70942372801900433 ) ) ;
#73298=CARTESIAN_POINT ( 'NONE',  ( -9.564922557960796823, -16.46253265017161027, 87.08224293864769550 ) ) ;
#73299=CARTESIAN_POINT ( 'NONE',  ( 13.97604488694527802, 13.89961937509977652, 24.37390960531435624 ) ) ;
#73300=CARTESIAN_POINT ( 'NONE',  ( 19.03943276465977164, -0.05219959533909143690, 58.74890960531435979 ) ) ;
#73301=CARTESIAN_POINT ( 'NONE',  ( -14.34966873604960291, -8.224510206698953496, 61.66557627198103120 ) ) ;
#73302=CARTESIAN_POINT ( 'NONE',  ( -5.823673210054431948, 21.52544592524334988, 72.70942372801901854 ) ) ;
#73303=CARTESIAN_POINT ( 'NONE',  ( -16.46253265017146816, -9.564922557961047289, 49.16775706135233293 ) ) ;
#73304=CARTESIAN_POINT ( 'NONE',  ( -19.05341960407617563, 5.049401038297882671, 28.54275706135232937 ) ) ;
#73305=CARTESIAN_POINT ( 'NONE',  ( -19.02544592524342804, 5.153800228976336051, 51.04057627198103120 ) ) ;
#73306=CARTESIAN_POINT ( 'NONE',  ( 10.81492255796078972, 18.62759615963270932, 29.58224293864769905 ) ) ;
#73307=CARTESIAN_POINT ( 'NONE',  ( 10.72451020669871369, 18.67979575497193778, 102.0844237280190185 ) ) ;
#73308=CARTESIAN_POINT ( 'NONE',  ( 19.03943276465977164, -0.05219959533909143690, 63.74890960531435979 ) ) ;
#73309=CARTESIAN_POINT ( 'NONE',  ( -0.05219959533937732626, 21.53943276465977519, 97.50109039468567573 ) ) ;
#73310=CARTESIAN_POINT ( 'NONE',  ( 10.81492255796078972, 18.62759615963270932, 34.58224293864770260 ) ) ;
#73311=CARTESIAN_POINT ( 'NONE',  ( -5.153800228976328057, -19.02544592524343514, 82.29057627198103830 ) ) ;
#73312=CARTESIAN_POINT ( 'NONE',  ( -16.46253265017146816, -9.564922557961047289, 64.16775706135233293 ) ) ;
#73313=CARTESIAN_POINT ( 'NONE',  ( 19.03943276465977164, -0.05219959533909143690, 38.74890960531436690 ) ) ;
#73314=CARTESIAN_POINT ( 'NONE',  ( -19.05341960407611168, -5.049401038298163336, 86.45724293864769550 ) ) ;
#73315=CARTESIAN_POINT ( 'NONE',  ( 14.34966873604972726, -8.224510206698740333, 30.83442372801902209 ) ) ;
#73316=CARTESIAN_POINT ( 'NONE',  ( -16.53943276465976808, 0.05219959533911058130, 86.24890960531436690 ) ) ;
#73317=CARTESIAN_POINT ( 'NONE',  ( -13.97604488694527625, -13.89961937509977652, 66.87390960531436690 ) ) ;
#73318=CARTESIAN_POINT ( 'NONE',  ( -15.72974639402197994, 15.80617190586746368, 45.62390960531436690 ) ) ;
#73319=CARTESIAN_POINT ( 'NONE',  ( -12.06949235617739369, -12.14591786802326823, 19.37609039468568639 ) ) ;
#73320=CARTESIAN_POINT ( 'NONE',  ( 21.52544592524334988, 5.823673210054432836, 26.45942372801901854 ) ) ;
#73321=CARTESIAN_POINT ( 'NONE',  ( 18.67979575497194134, -10.72451020669871369, 65.83442372801900433 ) ) ;
#73322=CARTESIAN_POINT ( 'NONE',  ( -16.55341960407617563, 4.379528057220093196, 73.54275706135234714 ) ) ;
#73323=CARTESIAN_POINT ( 'NONE',  ( 14.34966873604972726, -8.224510206698740333, 65.83442372801900433 ) ) ;
#73324=CARTESIAN_POINT ( 'NONE',  ( 9.474510206698971260, -16.51473224551069308, 57.91557627198103120 ) ) ;
#73325=CARTESIAN_POINT ( 'NONE',  ( -16.52544592524335698, -4.483927247898792601, 98.95942372801903275 ) ) ;
#73326=CARTESIAN_POINT ( 'NONE',  ( 19.03943276465977164, 0.05219959533936151252, 41.25109039468566152 ) ) ;
#73327=CARTESIAN_POINT ( 'NONE',  ( -21.53943276465977519, -0.05219959533937600094, 28.75109039468567929 ) ) ;
#73328=CARTESIAN_POINT ( 'NONE',  ( -4.483927247898539470, -16.52544592524342804, 62.29057627198102409 ) ) ;
#73329=CARTESIAN_POINT ( 'NONE',  ( -13.97604488694527625, -13.89961937509977652, 96.87390960531433848 ) ) ;
#73330=CARTESIAN_POINT ( 'NONE',  ( 16.55341960407618274, -4.379528057220086978, 91.04275706135236135 ) ) ;
#73331=CARTESIAN_POINT ( 'NONE',  ( -10.81492255796105439, 18.62759615963255655, 77.91775706135231871 ) ) ;
#73332=CARTESIAN_POINT ( 'NONE',  ( -14.34966873604972548, 8.224510206698743886, 33.33442372801900433 ) ) ;
#73333=CARTESIAN_POINT ( 'NONE',  ( -15.80617190586768217, 15.72974639402176855, 23.12609039468567573 ) ) ;
#73334=CARTESIAN_POINT ( 'NONE',  ( -12.14591786802309592, -12.06949235617757132, 56.87390960531436690 ) ) ;
#73336=CARTESIAN_POINT ( 'NONE',  ( 15.72974639402199770, -15.80617190586745480, 98.12390960531436690 ) ) ;
#73337=CARTESIAN_POINT ( 'NONE',  ( 8.224510206698953496, -14.34966873604960469, 42.91557627198103120 ) ) ;
#73338=ORIENTED_EDGE ( 'NONE', *, *, #166372, .T. ) ;
#73339=CARTESIAN_POINT ( 'NONE',  ( 16.46253265017160672, -9.564922557960803928, 23.33224293864769194 ) ) ;
#73340=CARTESIAN_POINT ( 'NONE',  ( 21.53943276465977519, -0.05219959533907433946, 33.74890960531436690 ) ) ;
#73341=CARTESIAN_POINT ( 'NONE',  ( 21.53943276465977519, 0.05219959533937863772, 41.25109039468568284 ) ) ;
#73342=CARTESIAN_POINT ( 'NONE',  ( -4.379528057220328563, 16.55341960407611168, 70.20724293864769550 ) ) ;
#73343=CARTESIAN_POINT ( 'NONE',  ( -18.62759615963270932, 10.81492255796079327, 60.83224293864769550 ) ) ;
#73344=CARTESIAN_POINT ( 'NONE',  ( 19.02544592524343514, -5.153800228976328945, 73.54057627198103830 ) ) ;
#73345=CARTESIAN_POINT ( 'NONE',  ( 16.46253265017160672, -9.564922557960803928, 23.33224293864769194 ) ) ;
#73346=CARTESIAN_POINT ( 'NONE',  ( -9.564922557961040184, 16.46253265017147172, 82.91775706135233293 ) ) ;
#73348=CARTESIAN_POINT ( 'NONE',  ( -21.53943276465977519, 0.05219959533907696930, 46.24890960531435979 ) ) ;
#73349=CARTESIAN_POINT ( 'NONE',  ( 9.564922557960805705, 16.46253265017160317, 39.58224293864768839 ) ) ;
#73350=CARTESIAN_POINT ( 'NONE',  ( 16.51473224551069308, 9.474510206698969483, 74.16557627198103830 ) ) ;
#73352=CARTESIAN_POINT ( 'NONE',  ( 4.379528057220092307, 16.55341960407617563, 37.29275706135235424 ) ) ;
#73353=CARTESIAN_POINT ( 'NONE',  ( -0.05219959533907301413, -21.53943276465977519, 112.4989096053143669 ) ) ;
#73354=CARTESIAN_POINT ( 'NONE',  ( -8.314922557960811034, -14.29746914071050412, 42.08224293864769550 ) ) ;
#73355=CARTESIAN_POINT ( 'NONE',  ( 13.89961937509977652, -13.97604488694527269, 103.1239096053143527 ) ) ;
#73356=CARTESIAN_POINT ( 'NONE',  ( -18.62759615963270932, 10.81492255796079327, 75.83224293864769550 ) ) ;
#73357=CARTESIAN_POINT ( 'NONE',  ( 10.72451020669898902, -18.67979575497178502, 107.9155762719810241 ) ) ;
#73358=CARTESIAN_POINT ( 'NONE',  ( 12.06949235617739724, 12.14591786802326823, 56.87609039468568994 ) ) ;
#73360=CARTESIAN_POINT ( 'NONE',  ( 21.52544592524344225, -5.823673210054117533, 53.54057627198103120 ) ) ;
#73361=CARTESIAN_POINT ( 'NONE',  ( -5.719274019375665041, -21.55341960407619695, 99.79275706135234714 ) ) ;
#73362=CARTESIAN_POINT ( 'NONE',  ( 5.049401038298161559, -19.05341960407611168, 57.70724293864769550 ) ) ;
#73363=CARTESIAN_POINT ( 'NONE',  ( 19.05341960407611168, 5.049401038298154454, 103.9572429386476671 ) ) ;
#73364=CARTESIAN_POINT ( 'NONE',  ( -16.46253265017160317, 9.564922557960807481, 80.83224293864769550 ) ) ;
#73366=CARTESIAN_POINT ( 'NONE',  ( 19.03943276465977164, 0.05219959533936151252, 51.25109039468567573 ) ) ;
#73367=CARTESIAN_POINT ( 'NONE',  ( 21.52544592524334988, 5.823673210054432836, 111.4594237280190328 ) ) ;
#73368=CARTESIAN_POINT ( 'NONE',  ( 15.80617190586746368, 15.72974639402197994, 34.37390960531435979 ) ) ;
#73369=CARTESIAN_POINT ( 'NONE',  ( -12.14591786802326823, 12.06949235617739902, 103.1260903946856757 ) ) ;
#73370=CARTESIAN_POINT ( 'NONE',  ( -5.049401038297874678, -19.05341960407617918, 84.79275706135233293 ) ) ;
#73371=CARTESIAN_POINT ( 'NONE',  ( -17.12812012977025944, 6.668231424566050336, 58.64051240676859322 ) ) ;
#73372=CARTESIAN_POINT ( 'NONE',  ( 0.05219959533909260263, 19.03943276465977164, 104.9989096053143669 ) ) ;
#73373=CARTESIAN_POINT ( 'NONE',  ( -5.049401038297874678, -19.05341960407617918, 79.79275706135233293 ) ) ;
#73374=CARTESIAN_POINT ( 'NONE',  ( 13.89961937509957401, 13.97604488694547697, 46.87609039468565442 ) ) ;
#73375=CARTESIAN_POINT ( 'NONE',  ( 17.50000000000000000, 5.499999999999992895, 71.70309617465829888 ) ) ;
#73376=CARTESIAN_POINT ( 'NONE',  ( -0.05219959533909027116, -19.03943276465977164, 47.49890960531435979 ) ) ;
#73377=CARTESIAN_POINT ( 'NONE',  ( 12.06949235617757843, -12.14591786802309237, 53.12390960531436690 ) ) ;
#73378=CARTESIAN_POINT ( 'NONE',  ( 19.03943276465977164, -0.05219959533909143690, 38.74890960531436690 ) ) ;
#73379=CARTESIAN_POINT ( 'NONE',  ( -14.29746914071049879, 8.314922557960819915, 35.83224293864768839 ) ) ;
#73381=CARTESIAN_POINT ( 'NONE',  ( 4.483927247898790824, -16.52544592524335698, 105.2094237280190328 ) ) ;
#73382=CARTESIAN_POINT ( 'NONE',  ( 19.05341960407611168, 5.049401038298154454, 53.95724293864770260 ) ) ;
#73383=CARTESIAN_POINT ( 'NONE',  ( -21.53943276465977519, -0.05219959533937600094, 113.7510903946856757 ) ) ;
#73384=CARTESIAN_POINT ( 'NONE',  ( -14.29746914071037622, -8.314922557961029526, 29.16775706135234003 ) ) ;
#73385=CARTESIAN_POINT ( 'NONE',  ( -21.55341960407610458, -5.719274019375992779, 36.45724293864768839 ) ) ;
#73386=CARTESIAN_POINT ( 'NONE',  ( 18.62759615963255655, 10.81492255796105972, 86.66775706135234714 ) ) ;
#73388=CARTESIAN_POINT ( 'NONE',  ( 5.153800228976335163, 19.02544592524342804, 99.79057627198102409 ) ) ;
#73389=CARTESIAN_POINT ( 'NONE',  ( -19.02544592524342804, 5.153800228976336051, 86.04057627198103830 ) ) ;
#73391=CARTESIAN_POINT ( 'NONE',  ( -15.72974639402197994, 15.80617190586746368, 105.6239096053143669 ) ) ;
#73393=CARTESIAN_POINT ( 'NONE',  ( -4.483927247898539470, -16.52544592524342804, 77.29057627198102409 ) ) ;
#73394=CARTESIAN_POINT ( 'NONE',  ( 21.55341960407610458, 5.719274019375980345, 68.95724293864769550 ) ) ;
#73395=CARTESIAN_POINT ( 'NONE',  ( 19.03943276465977164, -0.05219959533909143690, 73.74890960531435269 ) ) ;
#73396=CARTESIAN_POINT ( 'NONE',  ( -0.05219959533907301413, -21.53943276465977519, 97.49890960531436690 ) ) ;
#73398=CARTESIAN_POINT ( 'NONE',  ( 9.564922557960805705, 16.46253265017160317, 64.58224293864769550 ) ) ;
#73399=CARTESIAN_POINT ( 'NONE',  ( 16.52544592524342804, -4.483927247898539470, 93.54057627198103830 ) ) ;
#73401=CARTESIAN_POINT ( 'NONE',  ( -19.03943276465977164, 0.05219959533909376836, 66.24890960531436690 ) ) ;
#73402=CARTESIAN_POINT ( 'NONE',  ( -9.474510206698720793, -16.51473224551083518, 74.58442372801900433 ) ) ;
#73403=CARTESIAN_POINT ( 'NONE',  ( 12.06949235617757843, -12.14591786802309237, 98.12390960531436690 ) ) ;
#73404=CARTESIAN_POINT ( 'NONE',  ( -5.823673210054431948, 21.52544592524334988, 62.70942372801902565 ) ) ;
#73405=CARTESIAN_POINT ( 'NONE',  ( 19.05341960407611168, 5.049401038298154454, 53.95724293864770260 ) ) ;
#73406=CARTESIAN_POINT ( 'NONE',  ( -5.719274019375665041, -21.55341960407619695, 19.79275706135235069 ) ) ;
#73407=CARTESIAN_POINT ( 'NONE',  ( -8.224510206698948167, 14.34966873604960824, 100.4155762719810241 ) ) ;
#73409=CARTESIAN_POINT ( 'NONE',  ( 9.564922557960805705, 16.46253265017160317, 59.58224293864769550 ) ) ;
#73411=CARTESIAN_POINT ( 'NONE',  ( 13.97604488694548053, -13.89961937509957401, 105.6260903946856757 ) ) ;
#73412=CARTESIAN_POINT ( 'NONE',  ( -9.564922557960796823, -16.46253265017161027, 112.0822429386476955 ) ) ;
#73413=CARTESIAN_POINT ( 'NONE',  ( 21.55341960407619695, -5.719274019375665929, 51.04275706135234714 ) ) ;
#73414=CARTESIAN_POINT ( 'NONE',  ( -5.049401038298153566, 19.05341960407611168, 95.20724293864770971 ) ) ;
#73415=CARTESIAN_POINT ( 'NONE',  ( -19.05341960407617563, 5.049401038297882671, 83.54275706135233293 ) ) ;
#73416=CARTESIAN_POINT ( 'NONE',  ( -16.51473224551069308, -9.474510206698971260, 61.66557627198103120 ) ) ;
#73417=CARTESIAN_POINT ( 'NONE',  ( 4.379528057220339221, -16.55341960407611168, 77.70724293864770971 ) ) ;
#73418=CARTESIAN_POINT ( 'NONE',  ( -9.474510206698964154, 16.51473224551069663, 95.41557627198102409 ) ) ;
#73419=CARTESIAN_POINT ( 'NONE',  ( 4.379528057220339221, -16.55341960407611168, 77.70724293864770971 ) ) ;
#73420=CARTESIAN_POINT ( 'NONE',  ( 13.97604488694527802, 13.89961937509977652, 79.37390960531435269 ) ) ;
#73421=CARTESIAN_POINT ( 'NONE',  ( 9.474510206698729675, 16.51473224551082808, 32.08442372801900433 ) ) ;
#73422=CARTESIAN_POINT ( 'NONE',  ( -16.51473224551069308, -9.474510206698971260, 51.66557627198102409 ) ) ;
#73423=CARTESIAN_POINT ( 'NONE',  ( -4.483927247898539470, -16.52544592524342804, 47.29057627198103120 ) ) ;
#73424=CARTESIAN_POINT ( 'NONE',  ( 5.049401038298161559, -19.05341960407611168, 32.70724293864768129 ) ) ;
#73425=EDGE_LOOP ( 'NONE', ( #86497, #144164 ) ) ;
#73426=CARTESIAN_POINT ( 'NONE',  ( -10.81492255796105439, 18.62759615963255655, 42.91775706135235424 ) ) ;
#73427=CARTESIAN_POINT ( 'NONE',  ( 16.51473224551083163, -9.474510206698727899, 75.83442372801900433 ) ) ;
#73428=CARTESIAN_POINT ( 'NONE',  ( -8.314922557960811034, -14.29746914071050412, 42.08224293864769550 ) ) ;
#73429=CARTESIAN_POINT ( 'NONE',  ( 15.80617190586746368, 15.72974639402197994, 94.37390960531436690 ) ) ;
#73430=CARTESIAN_POINT ( 'NONE',  ( 10.72451020669898902, -18.67979575497178502, 32.91557627198102409 ) ) ;
#73431=CARTESIAN_POINT ( 'NONE',  ( 14.34966873604960469, 8.224510206698951720, 74.16557627198102409 ) ) ;
#73432=CARTESIAN_POINT ( 'NONE',  ( -19.05341960407611168, -5.049401038298163336, 36.45724293864766707 ) ) ;
#73433=CARTESIAN_POINT ( 'NONE',  ( 0.05219959533934541429, -16.53943276465976808, 105.0010903946856757 ) ) ;
#73434=CARTESIAN_POINT ( 'NONE',  ( -8.224510206698735004, -14.34966873604973081, 64.58442372801900433 ) ) ;
#73435=CARTESIAN_POINT ( 'NONE',  ( 13.89961937509957401, 13.97604488694547697, 31.87609039468566863 ) ) ;
#73436=CARTESIAN_POINT ( 'NONE',  ( 19.05341960407611168, 5.049401038298154454, 98.95724293864766707 ) ) ;
#73437=CARTESIAN_POINT ( 'NONE',  ( -16.51473224551069308, -9.474510206698971260, 76.66557627198103830 ) ) ;
#73438=CARTESIAN_POINT ( 'NONE',  ( 4.379528057220092307, 16.55341960407617563, 72.29275706135236135 ) ) ;
#73439=CARTESIAN_POINT ( 'NONE',  ( -16.51473224551069308, -9.474510206698971260, 41.66557627198103120 ) ) ;
#73440=CARTESIAN_POINT ( 'NONE',  ( 14.29746914071049879, -8.314922557960816363, 53.33224293864769550 ) ) ;
#73441=CARTESIAN_POINT ( 'NONE',  ( -0.05219959533909027116, -19.03943276465977164, 107.4989096053143527 ) ) ;
#73442=CARTESIAN_POINT ( 'NONE',  ( -19.03943276465977164, 0.05219959533909376836, 96.24890960531436690 ) ) ;
#73443=CARTESIAN_POINT ( 'NONE',  ( 18.67979575497178502, 10.72451020669898547, 24.16557627198103120 ) ) ;
#73444=CARTESIAN_POINT ( 'NONE',  ( -14.34966873604960291, -8.224510206698953496, 71.66557627198100988 ) ) ;
#73445=CARTESIAN_POINT ( 'NONE',  ( -12.14591786802309592, -12.06949235617757132, 71.87390960531438111 ) ) ;
#73446=CARTESIAN_POINT ( 'NONE',  ( 8.224510206698742110, 14.34966873604972548, 57.08442372801901854 ) ) ;
#73448=CARTESIAN_POINT ( 'NONE',  ( 5.049401038297881783, 19.05341960407617563, 67.29275706135234714 ) ) ;
#73449=CARTESIAN_POINT ( 'NONE',  ( 9.564922557960805705, 16.46253265017160317, 84.58224293864769550 ) ) ;
#73450=CARTESIAN_POINT ( 'NONE',  ( 9.564922557961047289, -16.46253265017146816, 60.41775706135233293 ) ) ;
#73451=CARTESIAN_POINT ( 'NONE',  ( 0.05219959533936267826, -19.03943276465977164, 40.00109039468566152 ) ) ;
#73452=CARTESIAN_POINT ( 'NONE',  ( 0.05219959533934541429, -16.53943276465976808, 20.00109039468568639 ) ) ;
#73453=CARTESIAN_POINT ( 'NONE',  ( 16.52544592524335698, 4.483927247898782831, 101.4594237280190185 ) ) ;
#73454=CARTESIAN_POINT ( 'NONE',  ( -16.51473224551069308, -9.474510206698971260, 36.66557627198102409 ) ) ;
#73455=CARTESIAN_POINT ( 'NONE',  ( 18.67979575497178502, 10.72451020669898547, 24.16557627198103120 ) ) ;
#73456=CARTESIAN_POINT ( 'NONE',  ( -21.52544592524334988, -5.823673210054445271, 58.95942372801902565 ) ) ;
#73457=CARTESIAN_POINT ( 'NONE',  ( 13.89961937509957401, 13.97604488694547697, 106.8760903946856757 ) ) ;
#73459=CARTESIAN_POINT ( 'NONE',  ( 19.03943276465977164, -0.05219959533909143690, 73.74890960531435269 ) ) ;
#73460=CARTESIAN_POINT ( 'NONE',  ( -16.51473224551069308, -9.474510206698971260, 111.6655762719810383 ) ) ;
#73461=CARTESIAN_POINT ( 'NONE',  ( 0.05219959533910956823, 16.53943276465976808, 74.99890960531435269 ) ) ;
#73462=CARTESIAN_POINT ( 'NONE',  ( 9.474510206698971260, -16.51473224551069308, 82.91557627198103830 ) ) ;
#73464=CARTESIAN_POINT ( 'NONE',  ( 19.03943276465977164, -0.05219959533909143690, 73.74890960531435269 ) ) ;
#73465=CARTESIAN_POINT ( 'NONE',  ( 13.89961937509957401, 13.97604488694547697, 76.87609039468566152 ) ) ;
#73466=CARTESIAN_POINT ( 'NONE',  ( 15.72974639402199770, -15.80617190586745480, 63.12390960531435979 ) ) ;
#73467=CARTESIAN_POINT ( 'NONE',  ( -16.53943276465976808, 0.05219959533911058130, 116.2489096053143669 ) ) ;
#73468=CARTESIAN_POINT ( 'NONE',  ( 19.05341960407617918, -5.049401038297876454, 61.04275706135232582 ) ) ;
#73469=CARTESIAN_POINT ( 'NONE',  ( 9.564922557960805705, 16.46253265017160317, 54.58224293864769550 ) ) ;
#73470=CARTESIAN_POINT ( 'NONE',  ( 19.02544592524343514, -5.153800228976328945, 93.54057627198102409 ) ) ;
#73472=CARTESIAN_POINT ( 'NONE',  ( 21.53943276465977519, -0.05219959533907433946, 83.74890960531435269 ) ) ;
#73473=CARTESIAN_POINT ( 'NONE',  ( 12.06949235617757843, -12.14591786802309237, 98.12390960531436690 ) ) ;
#73474=CARTESIAN_POINT ( 'NONE',  ( 9.474510206698729675, 16.51473224551082808, 42.08442372801900433 ) ) ;
#73475=CARTESIAN_POINT ( 'NONE',  ( 5.719274019375991003, -21.55341960407610458, 77.70724293864770971 ) ) ;
#73476=CARTESIAN_POINT ( 'NONE',  ( -18.62759615963270932, 10.81492255796079327, 65.83224293864769550 ) ) ;
#73477=CARTESIAN_POINT ( 'NONE',  ( 12.14591786802309770, 12.06949235617756955, 39.37390960531436690 ) ) ;
#73478=CARTESIAN_POINT ( 'NONE',  ( 21.55341960407619695, -5.719274019375665929, 111.0427570613523613 ) ) ;
#73479=CARTESIAN_POINT ( 'NONE',  ( 5.153800228976335163, 19.02544592524342804, 84.79057627198099567 ) ) ;
#73480=CARTESIAN_POINT ( 'NONE',  ( -5.049401038298153566, 19.05341960407611168, 30.20724293864768839 ) ) ;
#73482=CARTESIAN_POINT ( 'NONE',  ( -10.81492255796105439, 18.62759615963255655, 42.91775706135235424 ) ) ;
#73483=CARTESIAN_POINT ( 'NONE',  ( 21.55341960407619695, -5.719274019375665929, 36.04275706135234714 ) ) ;
#73484=CARTESIAN_POINT ( 'NONE',  ( 9.564922557960805705, 16.46253265017160317, 49.58224293864770260 ) ) ;
#73485=CARTESIAN_POINT ( 'NONE',  ( -18.67979575497193778, 10.72451020669871902, 23.33442372801901499 ) ) ;
#73486=CARTESIAN_POINT ( 'NONE',  ( 5.049401038297881783, 19.05341960407617563, 57.29275706135231871 ) ) ;
#73487=CARTESIAN_POINT ( 'NONE',  ( -19.02544592524342804, 5.153800228976336051, 31.04057627198102409 ) ) ;
#73488=CARTESIAN_POINT ( 'NONE',  ( 16.55341960407618274, -4.379528057220086978, 31.04275706135234714 ) ) ;
#73489=CARTESIAN_POINT ( 'NONE',  ( -9.564922557960796823, -16.46253265017161027, 32.08224293864769550 ) ) ;
#73490=CARTESIAN_POINT ( 'NONE',  ( 16.52544592524335698, 4.483927247898782831, 76.45942372801901854 ) ) ;
#73491=CARTESIAN_POINT ( 'NONE',  ( 19.03943276465977164, -0.05219959533909143690, 43.74890960531435979 ) ) ;
#73493=CARTESIAN_POINT ( 'NONE',  ( -9.474510206698964154, 16.51473224551069663, 80.41557627198103830 ) ) ;
#73494=CARTESIAN_POINT ( 'NONE',  ( 19.02544592524343514, -5.153800228976328945, 28.54057627198102409 ) ) ;
#73496=CARTESIAN_POINT ( 'NONE',  ( -18.67979575497178146, -10.72451020669898902, 71.66557627198100988 ) ) ;
#73497=CARTESIAN_POINT ( 'NONE',  ( 8.314922557961029526, -14.29746914071037800, 45.41775706135234003 ) ) ;
#73498=CARTESIAN_POINT ( 'NONE',  ( 15.72974639402176855, 15.80617190586768217, 96.87609039468568994 ) ) ;
#73499=CARTESIAN_POINT ( 'NONE',  ( 5.153800228976335163, 19.02544592524342804, 34.79057627198102409 ) ) ;
#73500=CARTESIAN_POINT ( 'NONE',  ( -8.314922557960811034, -14.29746914071050412, 27.08224293864769550 ) ) ;
#73501=CARTESIAN_POINT ( 'NONE',  ( -8.224510206698948167, 14.34966873604960824, 65.41557627198102409 ) ) ;
#73502=CARTESIAN_POINT ( 'NONE',  ( 19.03943276465977164, -0.05219959533909143690, 63.74890960531435979 ) ) ;
#73503=CARTESIAN_POINT ( 'NONE',  ( -18.62759615963255300, -10.81492255796106328, 104.1677570613523471 ) ) ;
#73504=CARTESIAN_POINT ( 'NONE',  ( -15.80617190586768217, 15.72974639402176855, 23.12609039468567573 ) ) ;
#73505=CARTESIAN_POINT ( 'NONE',  ( -19.02544592524342804, 5.153800228976336051, 81.04057627198103830 ) ) ;
#73506=CARTESIAN_POINT ( 'NONE',  ( -18.67979575497193778, 10.72451020669871902, 88.33442372801901854 ) ) ;
#73507=CARTESIAN_POINT ( 'NONE',  ( 8.314922557961029526, -14.29746914071037800, 55.41775706135234714 ) ) ;
#73508=CARTESIAN_POINT ( 'NONE',  ( 8.314922557961029526, -14.29746914071037800, 25.41775706135235779 ) ) ;
#73509=CARTESIAN_POINT ( 'NONE',  ( -8.314922557960811034, -14.29746914071050412, 92.08224293864769550 ) ) ;
#73510=CARTESIAN_POINT ( 'NONE',  ( 21.55341960407619695, -5.719274019375665929, 96.04275706135236135 ) ) ;
#73512=CARTESIAN_POINT ( 'NONE',  ( 16.55341960407611168, 4.379528057220329451, 28.95724293864769905 ) ) ;
#73513=CARTESIAN_POINT ( 'NONE',  ( 13.97604488694527802, 13.89961937509977652, 29.37390960531435979 ) ) ;
#73514=CARTESIAN_POINT ( 'NONE',  ( -12.14591786802326823, 12.06949235617739902, 53.12609039468568284 ) ) ;
#73515=CARTESIAN_POINT ( 'NONE',  ( 14.34966873604960469, 8.224510206698951720, 54.16557627198103120 ) ) ;
#73516=CARTESIAN_POINT ( 'NONE',  ( 8.224510206698742110, 14.34966873604972548, 97.08442372801904696 ) ) ;
#73517=CARTESIAN_POINT ( 'NONE',  ( 9.474510206698971260, -16.51473224551069308, 112.9155762719810383 ) ) ;
#73518=CARTESIAN_POINT ( 'NONE',  ( -15.72974639402197994, 15.80617190586746368, 35.62390960531437401 ) ) ;
#73519=CARTESIAN_POINT ( 'NONE',  ( -19.02544592524334988, -5.153800228976617603, 18.95942372801899722 ) ) ;
#73520=CARTESIAN_POINT ( 'NONE',  ( 12.06949235617757843, -12.14591786802309237, 93.12390960531436690 ) ) ;
#73521=CARTESIAN_POINT ( 'NONE',  ( 19.05341960407611168, 5.049401038298154454, 98.95724293864766707 ) ) ;
#73523=CARTESIAN_POINT ( 'NONE',  ( 14.34966873604972726, -8.224510206698740333, 40.83442372801901854 ) ) ;
#73524=CARTESIAN_POINT ( 'NONE',  ( -19.02544592524342804, 5.153800228976336051, 36.04057627198100988 ) ) ;
#73525=CARTESIAN_POINT ( 'NONE',  ( -16.53943276465976808, -0.05219959533934237506, 48.75109039468568284 ) ) ;
#73527=CARTESIAN_POINT ( 'NONE',  ( -9.474510206698720793, -16.51473224551083518, 54.58442372801899722 ) ) ;
#73528=CARTESIAN_POINT ( 'NONE',  ( 5.153800228976335163, 19.02544592524342804, 39.79057627198100988 ) ) ;
#73529=CARTESIAN_POINT ( 'NONE',  ( -0.05219959533934338120, 16.53943276465976808, 82.50109039468568994 ) ) ;
#73530=CARTESIAN_POINT ( 'NONE',  ( -9.564922557961040184, 16.46253265017147172, 97.91775706135233293 ) ) ;
#73531=CARTESIAN_POINT ( 'NONE',  ( 19.03943276465977164, 0.05219959533936151252, 26.25109039468566507 ) ) ;
#73532=CARTESIAN_POINT ( 'NONE',  ( 16.51473224551069308, 9.474510206698969483, 59.16557627198102409 ) ) ;
#73533=CARTESIAN_POINT ( 'NONE',  ( 16.52544592524342804, -4.483927247898539470, 93.54057627198103830 ) ) ;
#73534=CARTESIAN_POINT ( 'NONE',  ( 13.89961937509957401, 13.97604488694547697, 66.87609039468567573 ) ) ;
#73535=CARTESIAN_POINT ( 'NONE',  ( -10.72451020669898014, 18.67979575497178502, 65.41557627198102409 ) ) ;
#73536=CARTESIAN_POINT ( 'NONE',  ( 0.05219959533936267826, -19.03943276465977164, 35.00109039468566863 ) ) ;
#73537=CARTESIAN_POINT ( 'NONE',  ( 13.97604488694527802, 13.89961937509977652, 104.3739096053143385 ) ) ;
#73538=CARTESIAN_POINT ( 'NONE',  ( -21.52544592524343514, 5.823673210054127303, 91.04057627198103830 ) ) ;
#73539=CARTESIAN_POINT ( 'NONE',  ( -16.88567814943162659, 6.947325034625692730, 83.70998877347415146 ) ) ;
#73540=CARTESIAN_POINT ( 'NONE',  ( -16.51473224551082808, 9.474510206698731452, 98.33442372801900433 ) ) ;
#73541=CARTESIAN_POINT ( 'NONE',  ( -17.49999999999999645, -5.499999999999992895, 99.20309617465831309 ) ) ;
#73542=CARTESIAN_POINT ( 'NONE',  ( -8.314922557961024197, 14.29746914071037800, 22.91775706135235069 ) ) ;
#73543=CARTESIAN_POINT ( 'NONE',  ( -0.05219959533909027116, -19.03943276465977164, 52.49890960531436690 ) ) ;
#73544=CARTESIAN_POINT ( 'NONE',  ( 19.05341960407611168, 5.049401038298154454, 108.9572429386477097 ) ) ;
#73545=CARTESIAN_POINT ( 'NONE',  ( 15.72974639402199770, -15.80617190586745480, 93.12390960531436690 ) ) ;
#73546=CARTESIAN_POINT ( 'NONE',  ( 21.53943276465977519, 0.05219959533937863772, 56.25109039468568284 ) ) ;
#73547=CARTESIAN_POINT ( 'NONE',  ( -16.51473224551082808, 9.474510206698731452, 108.3344237280190043 ) ) ;
#73548=CARTESIAN_POINT ( 'NONE',  ( 19.02544592524334988, 5.153800228976608722, 21.45942372801899012 ) ) ;
#73549=CARTESIAN_POINT ( 'NONE',  ( 16.52544592524335698, 4.483927247898782831, 106.4594237280190328 ) ) ;
#73550=CARTESIAN_POINT ( 'NONE',  ( -5.719274019375978568, 21.55341960407610458, 105.2072429386477097 ) ) ;
#73551=CARTESIAN_POINT ( 'NONE',  ( -16.52544592524342804, 4.483927247898546575, 51.04057627198103120 ) ) ;
#73552=CARTESIAN_POINT ( 'NONE',  ( -19.02544592524334988, -5.153800228976617603, 78.95942372801900433 ) ) ;
#73553=CARTESIAN_POINT ( 'NONE',  ( 13.89961937509957401, 13.97604488694547697, 56.87609039468564731 ) ) ;
#73554=CARTESIAN_POINT ( 'NONE',  ( -5.719274019375665041, -21.55341960407619695, 74.79275706135234714 ) ) ;
#73555=CARTESIAN_POINT ( 'NONE',  ( -9.474510206698720793, -16.51473224551083518, 34.58442372801899722 ) ) ;
#73556=CARTESIAN_POINT ( 'NONE',  ( 5.049401038298161559, -19.05341960407611168, 27.70724293864769550 ) ) ;
#73557=CARTESIAN_POINT ( 'NONE',  ( -21.52544592524343514, 5.823673210054127303, 41.04057627198103120 ) ) ;
#73558=CARTESIAN_POINT ( 'NONE',  ( -16.52544592524342804, 4.483927247898546575, 31.04057627198102409 ) ) ;
#73559=CARTESIAN_POINT ( 'NONE',  ( 21.52544592524334988, 5.823673210054432836, 106.4594237280190328 ) ) ;
#73560=CARTESIAN_POINT ( 'NONE',  ( 12.06949235617739724, 12.14591786802326823, 76.87609039468567573 ) ) ;
#73561=CARTESIAN_POINT ( 'NONE',  ( -4.483927247898539470, -16.52544592524342804, 42.29057627198103120 ) ) ;
#73562=CARTESIAN_POINT ( 'NONE',  ( 5.823673210054444382, -21.52544592524334988, 65.20942372801901854 ) ) ;
#73563=CARTESIAN_POINT ( 'NONE',  ( -21.55341960407619339, 5.719274019375674811, 63.54275706135234003 ) ) ;
#73564=CARTESIAN_POINT ( 'NONE',  ( -5.823673210054116645, -21.52544592524344225, 67.29057627198103830 ) ) ;
#73566=CARTESIAN_POINT ( 'NONE',  ( 5.049401038298161559, -19.05341960407611168, 27.70724293864769550 ) ) ;
#73567=CARTESIAN_POINT ( 'NONE',  ( -15.80617190586768217, 15.72974639402176855, 48.12609039468568284 ) ) ;
#73568=CARTESIAN_POINT ( 'NONE',  ( -9.474510206698964154, 16.51473224551069663, 25.41557627198103120 ) ) ;
#73569=CARTESIAN_POINT ( 'NONE',  ( 16.46253265017160672, -9.564922557960803928, 43.33224293864769550 ) ) ;
#73570=CARTESIAN_POINT ( 'NONE',  ( 4.379528057220339221, -16.55341960407611168, 92.70724293864770971 ) ) ;
#73571=CARTESIAN_POINT ( 'NONE',  ( 19.05341960407611168, 5.049401038298154454, 88.95724293864769550 ) ) ;
#73572=CARTESIAN_POINT ( 'NONE',  ( -0.05219959533910754901, -16.53943276465976808, 27.49890960531435269 ) ) ;
#73573=CARTESIAN_POINT ( 'NONE',  ( -4.483927247898539470, -16.52544592524342804, 102.2905762719810383 ) ) ;
#73574=CARTESIAN_POINT ( 'NONE',  ( 0.05219959533907565091, 21.53943276465977519, 69.99890960531435269 ) ) ;
#73575=CARTESIAN_POINT ( 'NONE',  ( -0.05219959533907301413, -21.53943276465977519, 102.4989096053143811 ) ) ;
#73576=CARTESIAN_POINT ( 'NONE',  ( 19.03943276465977164, -0.05219959533909143690, 108.7489096053143527 ) ) ;
#73577=CARTESIAN_POINT ( 'NONE',  ( 13.89961937509977652, -13.97604488694527269, 68.12390960531436690 ) ) ;
#73578=CARTESIAN_POINT ( 'NONE',  ( 14.29746914071037800, 8.314922557961029526, 26.66775706135235424 ) ) ;
#73579=EDGE_CURVE ( 'NONE', #197846, #24501, #118770, .T. ) ;
#73580=CARTESIAN_POINT ( 'NONE',  ( 21.55341960407610458, 5.719274019375980345, 58.95724293864770971 ) ) ;
#73581=CARTESIAN_POINT ( 'NONE',  ( -0.05219959533937732626, 21.53943276465977519, 87.50109039468568994 ) ) ;
#73582=CARTESIAN_POINT ( 'NONE',  ( 9.564922557960805705, 16.46253265017160317, 79.58224293864769550 ) ) ;
#73583=CARTESIAN_POINT ( 'NONE',  ( -21.53943276465977519, 0.05219959533907696930, 21.24890960531436690 ) ) ;
#73584=CARTESIAN_POINT ( 'NONE',  ( -12.14591786802326823, 12.06949235617739902, 73.12609039468567573 ) ) ;
#73585=CARTESIAN_POINT ( 'NONE',  ( 15.80617190586769283, -15.72974639402175789, 70.62609039468567573 ) ) ;
#73586=CARTESIAN_POINT ( 'NONE',  ( 18.67979575497194134, -10.72451020669871369, 95.83442372801903275 ) ) ;
#73587=CARTESIAN_POINT ( 'NONE',  ( -4.483927247898782831, 16.52544592524335698, 62.70942372801902565 ) ) ;
#73588=CARTESIAN_POINT ( 'NONE',  ( 10.81492255796106328, -18.62759615963255655, 20.41775706135234714 ) ) ;
#73589=CARTESIAN_POINT ( 'NONE',  ( 16.51473224551069308, 9.474510206698969483, 24.16557627198102765 ) ) ;
#73590=CARTESIAN_POINT ( 'NONE',  ( 0.05219959533907565091, 21.53943276465977519, 94.99890960531436690 ) ) ;
#73591=CARTESIAN_POINT ( 'NONE',  ( -16.51473224551082808, 9.474510206698731452, 53.33442372801900433 ) ) ;
#73592=CARTESIAN_POINT ( 'NONE',  ( 18.67979575497178502, 10.72451020669898547, 59.16557627198103120 ) ) ;
#73593=CARTESIAN_POINT ( 'NONE',  ( -19.05341960407611168, -5.049401038298163336, 96.45724293864769550 ) ) ;
#73594=CARTESIAN_POINT ( 'NONE',  ( 12.06949235617757843, -12.14591786802309237, 38.12390960531436690 ) ) ;
#73595=CARTESIAN_POINT ( 'NONE',  ( 17.50000000000000000, 5.499999999999992895, 91.70309617465828467 ) ) ;
#73596=CARTESIAN_POINT ( 'NONE',  ( -19.20446147854526231, -5.500000000000010658, 79.38999695167677828 ) ) ;
#73597=CARTESIAN_POINT ( 'NONE',  ( -19.03943276465977164, -0.05219959533935918106, 113.7510903946856757 ) ) ;
#73598=CARTESIAN_POINT ( 'NONE',  ( 15.72974639402199770, -15.80617190586745480, 73.12390960531436690 ) ) ;
#73599=CARTESIAN_POINT ( 'NONE',  ( -8.224510206698948167, 14.34966873604960824, 45.41557627198103830 ) ) ;
#73600=CARTESIAN_POINT ( 'NONE',  ( -0.05219959533934338120, 16.53943276465976808, 27.50109039468567929 ) ) ;
#73601=CARTESIAN_POINT ( 'NONE',  ( -19.03943276465977164, 0.05219959533909376836, 51.24890960531436690 ) ) ;
#73602=CARTESIAN_POINT ( 'NONE',  ( -21.52544592524343514, 5.823673210054127303, 111.0405762719810525 ) ) ;
#73603=CARTESIAN_POINT ( 'NONE',  ( 13.89961937509957401, 13.97604488694547697, 81.87609039468564731 ) ) ;
#73605=CARTESIAN_POINT ( 'NONE',  ( -16.46253265017160317, 9.564922557960807481, 80.83224293864769550 ) ) ;
#73606=CARTESIAN_POINT ( 'NONE',  ( -5.049401038298153566, 19.05341960407611168, 70.20724293864769550 ) ) ;
#73607=CARTESIAN_POINT ( 'NONE',  ( 21.53943276465977519, -0.05219959533907433946, 73.74890960531433848 ) ) ;
#73608=CARTESIAN_POINT ( 'NONE',  ( 19.05341960407611168, 5.049401038298154454, 33.95724293864769550 ) ) ;
#73610=CARTESIAN_POINT ( 'NONE',  ( -8.314922557960811034, -14.29746914071050412, 57.08224293864769550 ) ) ;
#73611=CARTESIAN_POINT ( 'NONE',  ( -19.02544592524342804, 5.153800228976336051, 91.04057627198100988 ) ) ;
#73613=CARTESIAN_POINT ( 'NONE',  ( 16.51473224551083163, -9.474510206698727899, 60.83442372801900433 ) ) ;
#73614=CARTESIAN_POINT ( 'NONE',  ( 15.80617190586746368, 15.72974639402197994, 79.37390960531436690 ) ) ;
#73615=CARTESIAN_POINT ( 'NONE',  ( 9.564922557961047289, -16.46253265017146816, 30.41775706135232937 ) ) ;
#73616=CARTESIAN_POINT ( 'NONE',  ( -0.05219959533909027116, -19.03943276465977164, 92.49890960531436690 ) ) ;
#73617=DIRECTION ( 'NONE',  ( 6.716189716306310304E-15, -0.9991276842514723588, 0.04175967627138119781 ) ) ;
#73618=CARTESIAN_POINT ( 'NONE',  ( 10.72451020669898902, -18.67979575497178502, 32.91557627198102409 ) ) ;
#73620=CARTESIAN_POINT ( 'NONE',  ( -13.89961937509977652, 13.97604488694528158, 75.62390960531438111 ) ) ;
#73621=CARTESIAN_POINT ( 'NONE',  ( -21.52544592524334988, -5.823673210054445271, 53.95942372801900433 ) ) ;
#73622=CARTESIAN_POINT ( 'NONE',  ( 9.564922557960805705, 16.46253265017160317, 24.58224293864769194 ) ) ;
#73623=CARTESIAN_POINT ( 'NONE',  ( 15.80617190586746368, 15.72974639402197994, 109.3739096053143811 ) ) ;
#73625=CARTESIAN_POINT ( 'NONE',  ( -0.05219959533937732626, 21.53943276465977519, 37.50109039468568284 ) ) ;
#73627=CARTESIAN_POINT ( 'NONE',  ( -16.51473224551069308, -9.474510206698971260, 96.66557627198102409 ) ) ;
#73629=CARTESIAN_POINT ( 'NONE',  ( -21.55341960407610458, -5.719274019375992779, 101.4572429386476955 ) ) ;
#73630=CARTESIAN_POINT ( 'NONE',  ( -16.51473224551069308, -9.474510206698971260, 66.66557627198102409 ) ) ;
#73631=CARTESIAN_POINT ( 'NONE',  ( -14.29746914071037622, -8.314922557961029526, 19.16775706135234714 ) ) ;
#73633=CARTESIAN_POINT ( 'NONE',  ( -15.72974639402176322, -15.80617190586768395, 104.3760903946856899 ) ) ;
#73634=CARTESIAN_POINT ( 'NONE',  ( 13.97604488694527802, 13.89961937509977652, 39.37390960531435269 ) ) ;
#73635=CARTESIAN_POINT ( 'NONE',  ( -5.823673210054431948, 21.52544592524334988, 97.70942372801904696 ) ) ;
#73636=CARTESIAN_POINT ( 'NONE',  ( 19.03943276465977164, -0.05219959533909143690, 93.74890960531435269 ) ) ;
#73637=CARTESIAN_POINT ( 'NONE',  ( 5.719274019375673035, 21.55341960407619339, 62.29275706135236845 ) ) ;
#73641=CARTESIAN_POINT ( 'NONE',  ( -4.379528057220086978, -16.55341960407618274, 54.79275706135235424 ) ) ;
#73642=CARTESIAN_POINT ( 'NONE',  ( -14.34966873604972548, 8.224510206698743886, 68.33442372801900433 ) ) ;
#73643=CARTESIAN_POINT ( 'NONE',  ( 5.823673210054444382, -21.52544592524334988, 60.20942372801902565 ) ) ;
#73644=CARTESIAN_POINT ( 'NONE',  ( -21.55341960407619339, 5.719274019375674811, 88.54275706135236135 ) ) ;
#73646=CARTESIAN_POINT ( 'NONE',  ( -12.06949235617739369, -12.14591786802326823, 29.37609039468568284 ) ) ;
#73647=CARTESIAN_POINT ( 'NONE',  ( 16.46253265017160672, -9.564922557960803928, 78.33224293864769550 ) ) ;
#73648=CARTESIAN_POINT ( 'NONE',  ( -9.564922557960796823, -16.46253265017161027, 92.08224293864769550 ) ) ;
#73649=CARTESIAN_POINT ( 'NONE',  ( 16.81555441253550498, 7.025013491695491830, 41.86314554665747778 ) ) ;
#73650=CARTESIAN_POINT ( 'NONE',  ( -19.03943276465977164, 0.05219959533909376836, 31.24890960531435979 ) ) ;
#73651=CARTESIAN_POINT ( 'NONE',  ( 21.53943276465977519, -0.05219959533907433946, 48.74890960531435979 ) ) ;
#73652=CARTESIAN_POINT ( 'NONE',  ( -16.52544592524335698, -4.483927247898792601, 88.95942372801901854 ) ) ;
#73653=CARTESIAN_POINT ( 'NONE',  ( 12.14591786802309770, 12.06949235617756955, 84.37390960531438111 ) ) ;
#73654=CARTESIAN_POINT ( 'NONE',  ( -0.05219959533909027116, -19.03943276465977164, 72.49890960531435269 ) ) ;
#73655=CARTESIAN_POINT ( 'NONE',  ( 18.67979575497194134, -10.72451020669871369, 85.83442372801901854 ) ) ;
#73657=CARTESIAN_POINT ( 'NONE',  ( -16.53943276465976808, -0.05219959533934237506, 28.75109039468567929 ) ) ;
#73658=CARTESIAN_POINT ( 'NONE',  ( -12.06949235617756955, 12.14591786802309770, 70.62390960531436690 ) ) ;
#73659=CARTESIAN_POINT ( 'NONE',  ( -5.823673210054431948, 21.52544592524334988, 47.70942372801902565 ) ) ;
#73660=CARTESIAN_POINT ( 'NONE',  ( -21.53943276465977519, 0.05219959533907696930, 76.24890960531435269 ) ) ;
#73661=CARTESIAN_POINT ( 'NONE',  ( -13.89961937509957401, -13.97604488694547875, 44.37609039468566863 ) ) ;
#73662=CARTESIAN_POINT ( 'NONE',  ( 5.153800228976335163, 19.02544592524342804, 44.79057627198103120 ) ) ;
#73663=CARTESIAN_POINT ( 'NONE',  ( -19.05341960407611168, -5.049401038298163336, 81.45724293864769550 ) ) ;
#73664=CARTESIAN_POINT ( 'NONE',  ( -12.06949235617756955, 12.14591786802309770, 45.62390960531436690 ) ) ;
#73665=CARTESIAN_POINT ( 'NONE',  ( 16.55341960407611168, 4.379528057220329451, 28.95724293864769905 ) ) ;
#73666=CARTESIAN_POINT ( 'NONE',  ( -12.14591786802309592, -12.06949235617757132, 21.87390960531436690 ) ) ;
#73667=CARTESIAN_POINT ( 'NONE',  ( -9.564922557961040184, 16.46253265017147172, 62.91775706135233293 ) ) ;
#73669=CARTESIAN_POINT ( 'NONE',  ( 10.81492255796078972, 18.62759615963270932, 29.58224293864769905 ) ) ;
#73670=CARTESIAN_POINT ( 'NONE',  ( 16.53943276465976808, -0.05219959533910856209, 93.74890960531436690 ) ) ;
#73672=CARTESIAN_POINT ( 'NONE',  ( -9.474510206698964154, 16.51473224551069663, 45.41557627198103120 ) ) ;
#73673=CARTESIAN_POINT ( 'NONE',  ( -21.55341960407610458, -5.719274019375992779, 31.45724293864769550 ) ) ;
#73674=CARTESIAN_POINT ( 'NONE',  ( -18.67979575497178146, -10.72451020669898902, 66.66557627198102409 ) ) ;
#73675=CARTESIAN_POINT ( 'NONE',  ( 13.89961937509977652, -13.97604488694527269, 23.12390960531436335 ) ) ;
#73676=CARTESIAN_POINT ( 'NONE',  ( -0.05219959533934338120, 16.53943276465976808, 62.50109039468568284 ) ) ;
#73677=CARTESIAN_POINT ( 'NONE',  ( 9.474510206698971260, -16.51473224551069308, 52.91557627198102409 ) ) ;
#73678=CARTESIAN_POINT ( 'NONE',  ( -0.05219959533937732626, 21.53943276465977519, 52.50109039468567573 ) ) ;
#73680=CARTESIAN_POINT ( 'NONE',  ( 4.483927247898545687, 16.52544592524342804, 99.79057627198103830 ) ) ;
#73682=CARTESIAN_POINT ( 'NONE',  ( 19.05341960407617918, -5.049401038297876454, 96.04275706135231871 ) ) ;
#73684=CARTESIAN_POINT ( 'NONE',  ( -18.22780087662123805, 5.499999999999981348, 71.01763182126894947 ) ) ;
#73685=CARTESIAN_POINT ( 'NONE',  ( 18.67979575497178502, 10.72451020669898547, 29.16557627198103120 ) ) ;
#73687=CARTESIAN_POINT ( 'NONE',  ( 18.67979575497194134, -10.72451020669871369, 75.83442372801900433 ) ) ;
#73688=VERTEX_POINT ( 'NONE', #184264 ) ;
#73689=CARTESIAN_POINT ( 'NONE',  ( -12.06949235617739369, -12.14591786802326823, 59.37609039468568284 ) ) ;
#73690=CARTESIAN_POINT ( 'NONE',  ( 16.52544592524342804, -4.483927247898539470, 43.54057627198103830 ) ) ;
#73691=CARTESIAN_POINT ( 'NONE',  ( 18.62759615963271287, -10.81492255796078972, 68.33224293864769550 ) ) ;
#73692=CARTESIAN_POINT ( 'NONE',  ( -10.81492255796078084, -18.62759615963271287, 62.08224293864769550 ) ) ;
#73693=DIRECTION ( 'NONE',  ( 0.000000000000000000, 0.000000000000000000, -1.000000000000000000 ) ) ;
#73694=CARTESIAN_POINT ( 'NONE',  ( -5.153800228976607833, 19.02544592524334988, 82.70942372801897591 ) ) ;
#73695=CARTESIAN_POINT ( 'NONE',  ( 5.719274019375991003, -21.55341960407610458, 22.70724293864769194 ) ) ;
#73696=CARTESIAN_POINT ( 'NONE',  ( -19.02544592524342804, 5.153800228976336051, 51.04057627198103120 ) ) ;
#73697=CARTESIAN_POINT ( 'NONE',  ( 19.02544592524343514, -5.153800228976328945, 23.54057627198102054 ) ) ;
#73699=CARTESIAN_POINT ( 'NONE',  ( -19.03943276465977164, 0.05219959533909376836, 111.2489096053143669 ) ) ;
#73701=CARTESIAN_POINT ( 'NONE',  ( -16.55341960407617563, 4.379528057220093196, 73.54275706135234714 ) ) ;
#73702=CARTESIAN_POINT ( 'NONE',  ( -18.67979575497178146, -10.72451020669898902, 106.6655762719810383 ) ) ;
#73703=CARTESIAN_POINT ( 'NONE',  ( -5.153800228976328057, -19.02544592524343514, 67.29057627198102409 ) ) ;
#73704=CARTESIAN_POINT ( 'NONE',  ( -21.55341960407619339, 5.719274019375674811, 43.54275706135235424 ) ) ;
#73705=CARTESIAN_POINT ( 'NONE',  ( -0.05219959533909027116, -19.03943276465977164, 102.4989096053143669 ) ) ;
#73708=CARTESIAN_POINT ( 'NONE',  ( -5.823673210054431948, 21.52544592524334988, 32.70942372801900433 ) ) ;
#73709=CARTESIAN_POINT ( 'NONE',  ( -9.474510206698964154, 16.51473224551069663, 25.41557627198103120 ) ) ;
#73710=CARTESIAN_POINT ( 'NONE',  ( -5.153800228976607833, 19.02544592524334988, 82.70942372801897591 ) ) ;
#73711=CARTESIAN_POINT ( 'NONE',  ( -13.97604488694547697, 13.89961937509957934, 38.12609039468566152 ) ) ;
#73712=CARTESIAN_POINT ( 'NONE',  ( -10.81492255796078084, -18.62759615963271287, 112.0822429386477097 ) ) ;
#73713=CARTESIAN_POINT ( 'NONE',  ( -19.05341960407617563, 5.049401038297882671, 33.54275706135231871 ) ) ;
#73714=CARTESIAN_POINT ( 'NONE',  ( -5.153800228976607833, 19.02544592524334988, 52.70942372801900433 ) ) ;
#73715=CARTESIAN_POINT ( 'NONE',  ( -14.34966873604972548, 8.224510206698743886, 98.33442372801901854 ) ) ;
#73717=CARTESIAN_POINT ( 'NONE',  ( 19.02544592524343514, -5.153800228976328945, 73.54057627198103830 ) ) ;
#73718=CARTESIAN_POINT ( 'NONE',  ( -5.823673210054431948, 21.52544592524334988, 82.70942372801900433 ) ) ;
#73719=CARTESIAN_POINT ( 'NONE',  ( -15.80617190586768217, 15.72974639402176855, 93.12609039468568994 ) ) ;
#73720=CARTESIAN_POINT ( 'NONE',  ( 17.50000000000000000, 5.499999999999997335, 26.70309617465829888 ) ) ;
#73721=CARTESIAN_POINT ( 'NONE',  ( 9.564922557960805705, 16.46253265017160317, 94.58224293864769550 ) ) ;
#73722=CARTESIAN_POINT ( 'NONE',  ( -21.53943276465977519, -0.05219959533937600094, 58.75109039468568994 ) ) ;
#73723=CARTESIAN_POINT ( 'NONE',  ( 19.03943276465977164, 0.05219959533936151252, 106.2510903946856615 ) ) ;
#73724=CARTESIAN_POINT ( 'NONE',  ( -0.05219959533909027116, -19.03943276465977164, 62.49890960531435979 ) ) ;
#73725=CARTESIAN_POINT ( 'NONE',  ( -16.46253265017160317, 9.564922557960807481, 110.8322429386476955 ) ) ;
#73726=CARTESIAN_POINT ( 'NONE',  ( -5.049401038298153566, 19.05341960407611168, 85.20724293864766707 ) ) ;
#73727=CARTESIAN_POINT ( 'NONE',  ( -17.50000000000002132, -5.499999999999948486, 91.28230962303565832 ) ) ;
#73728=CARTESIAN_POINT ( 'NONE',  ( 19.02544592524343514, -5.153800228976328945, 68.54057627198103830 ) ) ;
#73729=CARTESIAN_POINT ( 'NONE',  ( -19.03943276465977164, 0.05219959533909376836, 46.24890960531435979 ) ) ;
#73730=CARTESIAN_POINT ( 'NONE',  ( -5.823673210054116645, -21.52544592524344225, 112.2905762719810241 ) ) ;
#73731=CARTESIAN_POINT ( 'NONE',  ( -0.05219959533934338120, 16.53943276465976808, 82.50109039468568994 ) ) ;
#73733=CARTESIAN_POINT ( 'NONE',  ( -9.474510206698720793, -16.51473224551083518, 49.58442372801899722 ) ) ;
#73734=CARTESIAN_POINT ( 'NONE',  ( 19.05341960407611168, 5.049401038298154454, 73.95724293864768129 ) ) ;
#73735=CARTESIAN_POINT ( 'NONE',  ( 12.06949235617757843, -12.14591786802309237, 73.12390960531436690 ) ) ;
#73736=CARTESIAN_POINT ( 'NONE',  ( 0.05219959533910956823, 16.53943276465976808, 109.9989096053143527 ) ) ;
#73737=CARTESIAN_POINT ( 'NONE',  ( -9.564922557960796823, -16.46253265017161027, 112.0822429386476955 ) ) ;
#73739=CARTESIAN_POINT ( 'NONE',  ( -16.51473224551069308, -9.474510206698971260, 106.6655762719810383 ) ) ;
#73740=CARTESIAN_POINT ( 'NONE',  ( 12.14591786802309770, 12.06949235617756955, 74.37390960531436690 ) ) ;
#73741=CARTESIAN_POINT ( 'NONE',  ( 16.51473224551069308, 9.474510206698969483, 114.1655762719810241 ) ) ;
#73742=CARTESIAN_POINT ( 'NONE',  ( 0.05219959533936267826, -19.03943276465977164, 35.00109039468566863 ) ) ;
#73743=CARTESIAN_POINT ( 'NONE',  ( -8.314922557961024197, 14.29746914071037800, 102.9177570613523756 ) ) ;
#73744=CARTESIAN_POINT ( 'NONE',  ( 19.02544592524343514, -5.153800228976328945, 88.54057627198102409 ) ) ;
#73745=CARTESIAN_POINT ( 'NONE',  ( 5.719274019375673035, 21.55341960407619339, 57.29275706135234714 ) ) ;
#73746=CARTESIAN_POINT ( 'NONE',  ( 21.52544592524344225, -5.823673210054117533, 48.54057627198103120 ) ) ;
#73747=CARTESIAN_POINT ( 'NONE',  ( -10.81492255796078084, -18.62759615963271287, 112.0822429386477097 ) ) ;
#73748=CARTESIAN_POINT ( 'NONE',  ( -5.823673210054116645, -21.52544592524344225, 67.29057627198103830 ) ) ;
#73749=CARTESIAN_POINT ( 'NONE',  ( 14.29746914071049879, -8.314922557960816363, 88.33224293864769550 ) ) ;
#73750=CARTESIAN_POINT ( 'NONE',  ( -9.474510206698720793, -16.51473224551083518, 54.58442372801899722 ) ) ;
#73751=CARTESIAN_POINT ( 'NONE',  ( -13.89961937509977652, 13.97604488694528158, 25.62390960531434558 ) ) ;
#73752=CARTESIAN_POINT ( 'NONE',  ( -9.474510206698964154, 16.51473224551069663, 80.41557627198103830 ) ) ;
#73753=CARTESIAN_POINT ( 'NONE',  ( -19.02544592524342804, 5.153800228976336051, 86.04057627198103830 ) ) ;
#73754=CARTESIAN_POINT ( 'NONE',  ( -8.224510206698948167, 14.34966873604960824, 100.4155762719810241 ) ) ;
#73755=ORIENTED_EDGE ( 'NONE', *, *, #123102, .T. ) ;
#73756=CARTESIAN_POINT ( 'NONE',  ( -4.483927247898539470, -16.52544592524342804, 27.29057627198103120 ) ) ;
#73757=CARTESIAN_POINT ( 'NONE',  ( 8.314922557961029526, -14.29746914071037800, 40.41775706135234714 ) ) ;
#73758=CARTESIAN_POINT ( 'NONE',  ( 5.823673210054444382, -21.52544592524334988, 105.2094237280190328 ) ) ;
#73759=CARTESIAN_POINT ( 'NONE',  ( -19.02544592524342804, 5.153800228976336051, 96.04057627198103830 ) ) ;
#73760=CARTESIAN_POINT ( 'NONE',  ( -21.55341960407619339, 5.719274019375674811, 38.54275706135234714 ) ) ;
#73761=CARTESIAN_POINT ( 'NONE',  ( 19.03943276465977164, -0.05219959533909143690, 48.74890960531435979 ) ) ;
#73762=CARTESIAN_POINT ( 'NONE',  ( 0.05219959533934541429, -16.53943276465976808, 40.00109039468567573 ) ) ;
#73763=CARTESIAN_POINT ( 'NONE',  ( -5.049401038297874678, -19.05341960407617918, 104.7927570613523471 ) ) ;
#73764=CARTESIAN_POINT ( 'NONE',  ( -9.474510206698964154, 16.51473224551069663, 40.41557627198103120 ) ) ;
#73765=CARTESIAN_POINT ( 'NONE',  ( -8.314922557960811034, -14.29746914071050412, 97.08224293864770971 ) ) ;
#73766=CARTESIAN_POINT ( 'NONE',  ( -15.72974639402197994, 15.80617190586746368, 105.6239096053143669 ) ) ;
#73767=CARTESIAN_POINT ( 'NONE',  ( 16.51473224551083163, -9.474510206698727899, 75.83442372801900433 ) ) ;
#73768=CARTESIAN_POINT ( 'NONE',  ( -16.51473224551069308, -9.474510206698971260, 31.66557627198102054 ) ) ;
#73769=CARTESIAN_POINT ( 'NONE',  ( 9.474510206698971260, -16.51473224551069308, 92.91557627198103830 ) ) ;
#73770=CARTESIAN_POINT ( 'NONE',  ( 21.55341960407619695, -5.719274019375665929, 36.04275706135234714 ) ) ;
#73772=CARTESIAN_POINT ( 'NONE',  ( -5.153800228976328057, -19.02544592524343514, 97.29057627198099567 ) ) ;
#73774=CARTESIAN_POINT ( 'NONE',  ( 19.05341960407611168, 5.049401038298154454, 88.95724293864769550 ) ) ;
#73775=CARTESIAN_POINT ( 'NONE',  ( -0.05219959533937732626, 21.53943276465977519, 37.50109039468568284 ) ) ;
#73776=CARTESIAN_POINT ( 'NONE',  ( -8.314922557960811034, -14.29746914071050412, 87.08224293864769550 ) ) ;
#73777=CARTESIAN_POINT ( 'NONE',  ( 13.89961937509977652, -13.97604488694527269, 93.12390960531436690 ) ) ;
#73778=CARTESIAN_POINT ( 'NONE',  ( 0.05219959533936267826, -19.03943276465977164, 25.00109039468566152 ) ) ;
#73779=CARTESIAN_POINT ( 'NONE',  ( -16.52544592524335698, -4.483927247898792601, 53.95942372801900433 ) ) ;
#73780=CARTESIAN_POINT ( 'NONE',  ( -15.72974639402176322, -15.80617190586768395, 74.37609039468568994 ) ) ;
#73782=CARTESIAN_POINT ( 'NONE',  ( 12.06949235617739724, 12.14591786802326823, 26.87609039468567218 ) ) ;
#73783=CARTESIAN_POINT ( 'NONE',  ( -19.05341960407611168, -5.049401038298163336, 66.45724293864769550 ) ) ;
#73784=CARTESIAN_POINT ( 'NONE',  ( -19.05341960407617563, 5.049401038297882671, 98.54275706135233293 ) ) ;
#73785=CARTESIAN_POINT ( 'NONE',  ( -0.05219959533934338120, 16.53943276465976808, 72.50109039468568994 ) ) ;
#73786=CARTESIAN_POINT ( 'NONE',  ( 9.564922557961047289, -16.46253265017146816, 20.41775706135233293 ) ) ;
#73787=CARTESIAN_POINT ( 'NONE',  ( -13.89961937509957401, -13.97604488694547875, 74.37609039468566152 ) ) ;
#73788=CARTESIAN_POINT ( 'NONE',  ( -5.049401038298153566, 19.05341960407611168, 60.20724293864768129 ) ) ;
#73789=CARTESIAN_POINT ( 'NONE',  ( 21.52544592524344225, -5.823673210054117533, 78.54057627198103830 ) ) ;
#73790=CARTESIAN_POINT ( 'NONE',  ( -14.29746914071049879, 8.314922557960819915, 75.83224293864769550 ) ) ;
#73791=CARTESIAN_POINT ( 'NONE',  ( 5.049401038297881783, 19.05341960407617563, 82.29275706135229029 ) ) ;
#73792=CARTESIAN_POINT ( 'NONE',  ( 16.29526858892873165, -7.335722546920202092, 61.70329402199800484 ) ) ;
#73793=CARTESIAN_POINT ( 'NONE',  ( 16.46253265017146816, 9.564922557961045513, 51.66775706135233293 ) ) ;
#73794=CARTESIAN_POINT ( 'NONE',  ( -0.05219959533934338120, 16.53943276465976808, 112.5010903946857042 ) ) ;
#73795=CARTESIAN_POINT ( 'NONE',  ( 0.05219959533910956823, 16.53943276465976808, 74.99890960531435269 ) ) ;
#73796=CARTESIAN_POINT ( 'NONE',  ( -13.89961937509957401, -13.97604488694547875, 24.37609039468565442 ) ) ;
#73798=CARTESIAN_POINT ( 'NONE',  ( -21.53943276465977519, 0.05219959533907696930, 111.2489096053143669 ) ) ;
#73799=CARTESIAN_POINT ( 'NONE',  ( -19.03943276465977164, 0.05219959533909376836, 101.2489096053143669 ) ) ;
#73800=CARTESIAN_POINT ( 'NONE',  ( 16.51473224551069308, 9.474510206698969483, 74.16557627198103830 ) ) ;
#73801=CARTESIAN_POINT ( 'NONE',  ( 0.05219959533937995610, -21.53943276465977519, 80.00109039468568994 ) ) ;
#73802=CARTESIAN_POINT ( 'NONE',  ( -5.153800228976328057, -19.02544592524343514, 57.29057627198103120 ) ) ;
#73803=ORIENTED_EDGE ( 'NONE', *, *, #164773, .T. ) ;
#73804=CARTESIAN_POINT ( 'NONE',  ( 16.46253265017160672, -9.564922557960803928, 43.33224293864769550 ) ) ;
#73805=CARTESIAN_POINT ( 'NONE',  ( -10.72451020669898014, 18.67979575497178502, 25.41557627198103120 ) ) ;
#73806=CARTESIAN_POINT ( 'NONE',  ( -14.29746914071049879, 8.314922557960819915, 80.83224293864769550 ) ) ;
#73807=CARTESIAN_POINT ( 'NONE',  ( -16.51473224551069308, -9.474510206698971260, 41.66557627198103120 ) ) ;
#73808=CARTESIAN_POINT ( 'NONE',  ( -4.483927247898539470, -16.52544592524342804, 102.2905762719810383 ) ) ;
#73809=CARTESIAN_POINT ( 'NONE',  ( 15.72974639402199770, -15.80617190586745480, 103.1239096053143811 ) ) ;
#73811=B_SPLINE_CURVE_WITH_KNOTS ( 'NONE', 3,
 ( #141531, #112189, #35347, #140533, #172877, #63701 ),
 .UNSPECIFIED., .F., .F.,
 ( 4, 2, 4 ),
 ( 0.000000000000000000, 0.0003837532665634976444, 0.0007675065331269952888 ),
 .UNSPECIFIED. ) ;
#73812=CARTESIAN_POINT ( 'NONE',  ( -21.55341960407619339, 5.719274019375674811, 48.54275706135234714 ) ) ;
#73813=CARTESIAN_POINT ( 'NONE',  ( -13.89961937509977652, 13.97604488694528158, 35.62390960531435269 ) ) ;
#73814=CARTESIAN_POINT ( 'NONE',  ( 12.06949235617739724, 12.14591786802326823, 61.87609039468568284 ) ) ;
#73815=CARTESIAN_POINT ( 'NONE',  ( -18.67979575497178146, -10.72451020669898902, 106.6655762719810383 ) ) ;
#73816=CARTESIAN_POINT ( 'NONE',  ( 15.80617190586746368, 15.72974639402197994, 99.37390960531436690 ) ) ;
#73817=CARTESIAN_POINT ( 'NONE',  ( 19.02544592524334988, 5.153800228976608722, 36.45942372801900433 ) ) ;
#73818=CARTESIAN_POINT ( 'NONE',  ( -19.05341960407611168, -5.049401038298163336, 46.45724293864768129 ) ) ;
#73819=CARTESIAN_POINT ( 'NONE',  ( 19.02544592524343514, -5.153800228976328945, 113.5405762719810241 ) ) ;
#73820=CARTESIAN_POINT ( 'NONE',  ( -21.52544592524334988, -5.823673210054445271, 58.95942372801902565 ) ) ;
#73821=CARTESIAN_POINT ( 'NONE',  ( -10.81492255796078084, -18.62759615963271287, 52.08224293864768839 ) ) ;
#73822=CARTESIAN_POINT ( 'NONE',  ( -8.314922557960811034, -14.29746914071050412, 37.08224293864768129 ) ) ;
#73823=CARTESIAN_POINT ( 'NONE',  ( -21.53943276465977519, -0.05219959533937600094, 73.75109039468567573 ) ) ;
#73824=CARTESIAN_POINT ( 'NONE',  ( 15.72974639402176855, 15.80617190586768217, 111.8760903946856615 ) ) ;
#73825=CARTESIAN_POINT ( 'NONE',  ( -16.51473224551082808, 9.474510206698731452, 48.33442372801900433 ) ) ;
#73826=CARTESIAN_POINT ( 'NONE',  ( -12.14591786802326823, 12.06949235617739902, 98.12609039468570415 ) ) ;
#73827=CARTESIAN_POINT ( 'NONE',  ( -18.67979575497193778, 10.72451020669871902, 53.33442372801901854 ) ) ;
#73828=CARTESIAN_POINT ( 'NONE',  ( -5.049401038298153566, 19.05341960407611168, 55.20724293864769550 ) ) ;
#73829=CARTESIAN_POINT ( 'NONE',  ( -13.97604488694547697, 13.89961937509957934, 28.12609039468565797 ) ) ;
#73830=CARTESIAN_POINT ( 'NONE',  ( -15.72974639402197994, 15.80617190586746368, 35.62390960531437401 ) ) ;
#73831=CARTESIAN_POINT ( 'NONE',  ( 18.67979575497194134, -10.72451020669871369, 35.83442372801901143 ) ) ;
#73832=CARTESIAN_POINT ( 'NONE',  ( 5.719274019375991003, -21.55341960407610458, 92.70724293864770971 ) ) ;
#73833=CARTESIAN_POINT ( 'NONE',  ( -9.474510206698720793, -16.51473224551083518, 84.58442372801900433 ) ) ;
#73834=CARTESIAN_POINT ( 'NONE',  ( -8.224510206698735004, -14.34966873604973081, 59.58442372801901854 ) ) ;
#73836=CARTESIAN_POINT ( 'NONE',  ( -10.81492255796078084, -18.62759615963271287, 87.08224293864769550 ) ) ;
#73837=CARTESIAN_POINT ( 'NONE',  ( -12.14591786802326823, 12.06949235617739902, 78.12609039468570415 ) ) ;
#73838=CARTESIAN_POINT ( 'NONE',  ( -16.53943276465976808, 0.05219959533911058130, 81.24890960531436690 ) ) ;
#73839=CARTESIAN_POINT ( 'NONE',  ( -16.79531203550646978, -7.028104445595615424, 101.2524498822044450 ) ) ;
#73840=CARTESIAN_POINT ( 'NONE',  ( -13.97604488694547697, 13.89961937509957934, 103.1260903946856473 ) ) ;
#73841=CARTESIAN_POINT ( 'NONE',  ( 5.823673210054125526, 21.52544592524343514, 29.79057627198102409 ) ) ;
#73843=CARTESIAN_POINT ( 'NONE',  ( 4.483927247898790824, -16.52544592524335698, 50.20942372801901854 ) ) ;
#73844=CARTESIAN_POINT ( 'NONE',  ( -10.72451020669870658, -18.67979575497194134, 24.58442372801901499 ) ) ;
#73845=CARTESIAN_POINT ( 'NONE',  ( -10.81492255796078084, -18.62759615963271287, 47.08224293864770260 ) ) ;
#73846=CARTESIAN_POINT ( 'NONE',  ( 16.52544592524335698, 4.483927247898782831, 66.45942372801903275 ) ) ;
#73847=CARTESIAN_POINT ( 'NONE',  ( 16.51473224551069308, 9.474510206698969483, 79.16557627198103830 ) ) ;
#73848=CARTESIAN_POINT ( 'NONE',  ( -21.53943276465977519, -0.05219959533937600094, 58.75109039468568994 ) ) ;
#73849=CARTESIAN_POINT ( 'NONE',  ( -9.474510206698964154, 16.51473224551069663, 30.41557627198102054 ) ) ;
#73851=CARTESIAN_POINT ( 'NONE',  ( 21.52544592524344225, -5.823673210054117533, 28.54057627198103120 ) ) ;
#73853=CARTESIAN_POINT ( 'NONE',  ( -13.97604488694547697, 13.89961937509957934, 38.12609039468566152 ) ) ;
#73854=CARTESIAN_POINT ( 'NONE',  ( -8.314922557961024197, 14.29746914071037800, 57.91775706135234714 ) ) ;
#73855=CARTESIAN_POINT ( 'NONE',  ( -15.80617190586745835, -15.72974639402198527, 21.87390960531436690 ) ) ;
#73857=CARTESIAN_POINT ( 'NONE',  ( -9.564922557960796823, -16.46253265017161027, 77.08224293864769550 ) ) ;
#73858=CARTESIAN_POINT ( 'NONE',  ( -16.55341960407617563, 4.379528057220093196, 103.5427570613523613 ) ) ;
#73860=CARTESIAN_POINT ( 'NONE',  ( 8.224510206698953496, -14.34966873604960469, 97.91557627198103830 ) ) ;
#73861=CARTESIAN_POINT ( 'NONE',  ( -18.62759615963270932, 10.81492255796079327, 40.83224293864769550 ) ) ;
#73862=CARTESIAN_POINT ( 'NONE',  ( 13.89961937509977652, -13.97604488694527269, 38.12390960531436690 ) ) ;
#73863=CARTESIAN_POINT ( 'NONE',  ( -14.29746914071037622, -8.314922557961029526, 74.16775706135231871 ) ) ;
#73864=CARTESIAN_POINT ( 'NONE',  ( 15.80617190586769283, -15.72974639402175789, 20.62609039468568639 ) ) ;
#73865=CARTESIAN_POINT ( 'NONE',  ( -19.03943276465977164, -0.05219959533935918106, 78.75109039468567573 ) ) ;
#73866=CARTESIAN_POINT ( 'NONE',  ( 5.049401038298161559, -19.05341960407611168, 37.70724293864768839 ) ) ;
#73867=CARTESIAN_POINT ( 'NONE',  ( -19.03943276465977164, 0.05219959533909376836, 111.2489096053143669 ) ) ;
#73868=CARTESIAN_POINT ( 'NONE',  ( 21.53943276465977519, 0.05219959533937863772, 86.25109039468568994 ) ) ;
#73869=CARTESIAN_POINT ( 'NONE',  ( 19.03943276465977164, -0.05219959533909143690, 58.74890960531435979 ) ) ;
#73870=CARTESIAN_POINT ( 'NONE',  ( 12.14591786802327356, -12.06949235617739191, 50.62609039468568994 ) ) ;
#73871=CARTESIAN_POINT ( 'NONE',  ( 15.72974639402176855, 15.80617190586768217, 76.87609039468567573 ) ) ;
#73872=CARTESIAN_POINT ( 'NONE',  ( -16.46253265017146816, -9.564922557961047289, 44.16775706135232582 ) ) ;
#73873=CARTESIAN_POINT ( 'NONE',  ( -19.02544592524334988, -5.153800228976617603, 53.95942372801898301 ) ) ;
#73875=CARTESIAN_POINT ( 'NONE',  ( 21.53943276465977519, 0.05219959533937863772, 56.25109039468568284 ) ) ;
#73876=CARTESIAN_POINT ( 'NONE',  ( 19.03943276465977164, -0.05219959533909143690, 23.74890960531435269 ) ) ;
#73877=CARTESIAN_POINT ( 'NONE',  ( 16.46253265017146816, 9.564922557961045513, 41.66775706135234003 ) ) ;
#73878=CARTESIAN_POINT ( 'NONE',  ( 13.97604488694527802, 13.89961937509977652, 104.3739096053143385 ) ) ;
#73879=CARTESIAN_POINT ( 'NONE',  ( 19.02544592524343514, -5.153800228976328945, 83.54057627198100988 ) ) ;
#73880=CARTESIAN_POINT ( 'NONE',  ( 0.05219959533910956823, 16.53943276465976808, 39.99890960531436690 ) ) ;
#73881=CARTESIAN_POINT ( 'NONE',  ( 5.719274019375991003, -21.55341960407610458, 37.70724293864769550 ) ) ;
#73884=CARTESIAN_POINT ( 'NONE',  ( 21.55341960407619695, -5.719274019375665929, 96.04275706135236135 ) ) ;
#73886=CARTESIAN_POINT ( 'NONE',  ( 9.564922557960805705, 16.46253265017160317, 39.58224293864768839 ) ) ;
#73887=CARTESIAN_POINT ( 'NONE',  ( 9.474510206698971260, -16.51473224551069308, 107.9155762719810383 ) ) ;
#73889=CARTESIAN_POINT ( 'NONE',  ( 4.379528057220092307, 16.55341960407617563, 57.29275706135234714 ) ) ;
#73890=CARTESIAN_POINT ( 'NONE',  ( 5.719274019375991003, -21.55341960407610458, 77.70724293864770971 ) ) ;
#73891=CARTESIAN_POINT ( 'NONE',  ( -16.53943276465976808, 0.05219959533911058130, 41.24890960531435269 ) ) ;
#73892=CARTESIAN_POINT ( 'NONE',  ( 13.89961937509977652, -13.97604488694527269, 33.12390960531434558 ) ) ;
#73893=CARTESIAN_POINT ( 'NONE',  ( 5.049401038298161559, -19.05341960407611168, 112.7072429386476813 ) ) ;
#73894=CARTESIAN_POINT ( 'NONE',  ( 0.05219959533937995610, -21.53943276465977519, 30.00109039468568284 ) ) ;
#73895=CARTESIAN_POINT ( 'NONE',  ( -13.97604488694547697, 13.89961937509957934, 33.12609039468566863 ) ) ;
#73896=CARTESIAN_POINT ( 'NONE',  ( 13.97604488694527802, 13.89961937509977652, 39.37390960531435269 ) ) ;
#73897=CARTESIAN_POINT ( 'NONE',  ( -18.62759615963255300, -10.81492255796106328, 84.16775706135234714 ) ) ;
#73899=CARTESIAN_POINT ( 'NONE',  ( 12.14591786802309770, 12.06949235617756955, 24.37390960531435979 ) ) ;
#73901=CARTESIAN_POINT ( 'NONE',  ( 15.72974639402199770, -15.80617190586745480, 23.12390960531436335 ) ) ;
#73902=CARTESIAN_POINT ( 'NONE',  ( -14.29746914071049879, 8.314922557960819915, 105.8322429386476955 ) ) ;
#73904=CARTESIAN_POINT ( 'NONE',  ( -16.46253265017160317, 9.564922557960807481, 85.83224293864769550 ) ) ;
#73905=CARTESIAN_POINT ( 'NONE',  ( -4.483927247898539470, -16.52544592524342804, 72.29057627198102409 ) ) ;
#73906=CARTESIAN_POINT ( 'NONE',  ( 13.97604488694548053, -13.89961937509957401, 100.6260903946856615 ) ) ;
#73907=CARTESIAN_POINT ( 'NONE',  ( -5.823673210054116645, -21.52544592524344225, 67.29057627198103830 ) ) ;
#73908=ORIENTED_EDGE ( 'NONE', *, *, #588, .T. ) ;
#73909=CARTESIAN_POINT ( 'NONE',  ( -19.05341960407611168, -5.049401038298163336, 36.45724293864766707 ) ) ;
#73910=CARTESIAN_POINT ( 'NONE',  ( 16.46253265017160672, -9.564922557960803928, 88.33224293864769550 ) ) ;
#73911=CARTESIAN_POINT ( 'NONE',  ( -5.823673210054116645, -21.52544592524344225, 87.29057627198103830 ) ) ;
#73912=CARTESIAN_POINT ( 'NONE',  ( -14.29746914071037622, -8.314922557961029526, 99.16775706135234714 ) ) ;
#73913=CARTESIAN_POINT ( 'NONE',  ( 19.05341960407611168, 5.049401038298154454, 83.95724293864766707 ) ) ;
#73914=CARTESIAN_POINT ( 'NONE',  ( -16.51473224551082808, 9.474510206698731452, 68.33442372801900433 ) ) ;
#73915=CARTESIAN_POINT ( 'NONE',  ( 18.62759615963255655, 10.81492255796105972, 101.6677570613523613 ) ) ;
#73916=CARTESIAN_POINT ( 'NONE',  ( 18.62759615963271287, -10.81492255796078972, 78.33224293864770971 ) ) ;
#73917=CARTESIAN_POINT ( 'NONE',  ( -10.72451020669898014, 18.67979575497178502, 35.41557627198102409 ) ) ;
#73918=CARTESIAN_POINT ( 'NONE',  ( 16.46253265017160672, -9.564922557960803928, 48.33224293864769550 ) ) ;
#73919=CARTESIAN_POINT ( 'NONE',  ( -16.53943276465976808, 0.05219959533911058130, 26.24890960531435624 ) ) ;
#73920=CARTESIAN_POINT ( 'NONE',  ( -9.564922557960796823, -16.46253265017161027, 62.08224293864769550 ) ) ;
#73922=CARTESIAN_POINT ( 'NONE',  ( 0.05219959533936267826, -19.03943276465977164, 20.00109039468567218 ) ) ;
#73923=CARTESIAN_POINT ( 'NONE',  ( -16.52544592524342804, 4.483927247898546575, 76.04057627198102409 ) ) ;
#73925=CARTESIAN_POINT ( 'NONE',  ( -18.62759615963270932, 10.81492255796079327, 110.8322429386476955 ) ) ;
#73926=CARTESIAN_POINT ( 'NONE',  ( 18.62759615963271287, -10.81492255796078972, 108.3322429386477097 ) ) ;
#73928=CARTESIAN_POINT ( 'NONE',  ( -5.719274019375978568, 21.55341960407610458, 65.20724293864768129 ) ) ;
#73929=CARTESIAN_POINT ( 'NONE',  ( -4.379528057220086978, -16.55341960407618274, 99.79275706135234714 ) ) ;
#73930=CARTESIAN_POINT ( 'NONE',  ( 16.52544592524342804, -4.483927247898539470, 103.5405762719810383 ) ) ;
#73931=CARTESIAN_POINT ( 'NONE',  ( -19.02544592524342804, 5.153800228976336051, 66.04057627198103830 ) ) ;
#73933=CARTESIAN_POINT ( 'NONE',  ( -14.29746914071037622, -8.314922557961029526, 109.1677570613523613 ) ) ;
#73934=CARTESIAN_POINT ( 'NONE',  ( -5.823673210054431948, 21.52544592524334988, 52.70942372801902565 ) ) ;
#73935=CARTESIAN_POINT ( 'NONE',  ( 13.97604488694527802, 13.89961937509977652, 104.3739096053143385 ) ) ;
#73936=CARTESIAN_POINT ( 'NONE',  ( 10.72451020669871369, 18.67979575497193778, 82.08442372801901854 ) ) ;
#73937=CARTESIAN_POINT ( 'NONE',  ( -13.89961937509977652, 13.97604488694528158, 25.62390960531434558 ) ) ;
#73938=CARTESIAN_POINT ( 'NONE',  ( -19.02544592524342804, 5.153800228976336051, 41.04057627198103120 ) ) ;
#73939=VERTEX_POINT ( 'NONE', #166127 ) ;
#73940=CARTESIAN_POINT ( 'NONE',  ( -15.72974639402176322, -15.80617190586768395, 84.37609039468570415 ) ) ;
#73941=CARTESIAN_POINT ( 'NONE',  ( 10.72451020669871369, 18.67979575497193778, 67.08442372801901854 ) ) ;
#73942=CARTESIAN_POINT ( 'NONE',  ( 9.564922557960805705, 16.46253265017160317, 109.5822429386476955 ) ) ;
#73943=CARTESIAN_POINT ( 'NONE',  ( 13.89961937509957401, 13.97604488694547697, 81.87609039468564731 ) ) ;
#73944=CARTESIAN_POINT ( 'NONE',  ( 21.53943276465977519, 0.05219959533937863772, 51.25109039468568994 ) ) ;
#73945=CARTESIAN_POINT ( 'NONE',  ( -4.379528057220086978, -16.55341960407618274, 24.79275706135235779 ) ) ;
#73946=CARTESIAN_POINT ( 'NONE',  ( 13.89961937509957401, 13.97604488694547697, 76.87609039468566152 ) ) ;
#73947=CARTESIAN_POINT ( 'NONE',  ( 5.153800228976335163, 19.02544592524342804, 49.79057627198100988 ) ) ;
#73948=CARTESIAN_POINT ( 'NONE',  ( -5.153800228976607833, 19.02544592524334988, 77.70942372801900433 ) ) ;
#73949=CARTESIAN_POINT ( 'NONE',  ( 12.06949235617739724, 12.14591786802326823, 111.8760903946856615 ) ) ;
#73951=CARTESIAN_POINT ( 'NONE',  ( -13.97604488694547697, 13.89961937509957934, 88.12609039468563310 ) ) ;
#73952=CARTESIAN_POINT ( 'NONE',  ( -4.379528057220328563, 16.55341960407611168, 40.20724293864769550 ) ) ;
#73953=CARTESIAN_POINT ( 'NONE',  ( -9.474510206698720793, -16.51473224551083518, 69.58442372801901854 ) ) ;
#73954=CARTESIAN_POINT ( 'NONE',  ( -16.55341960407617563, 4.379528057220093196, 43.54275706135235424 ) ) ;
#73955=CARTESIAN_POINT ( 'NONE',  ( -0.05219959533936034679, 19.03943276465977164, 22.50109039468566152 ) ) ;
#73956=CARTESIAN_POINT ( 'NONE',  ( -13.97604488694527625, -13.89961937509977652, 36.87390960531436690 ) ) ;
#73957=CARTESIAN_POINT ( 'NONE',  ( -17.49999999999999645, -5.499999999999992895, 64.20309617465829888 ) ) ;
#73958=CARTESIAN_POINT ( 'NONE',  ( 0.05219959533934541429, -16.53943276465976808, 40.00109039468567573 ) ) ;
#73961=CARTESIAN_POINT ( 'NONE',  ( -19.02544592524342804, 5.153800228976336051, 96.04057627198103830 ) ) ;
#73962=CARTESIAN_POINT ( 'NONE',  ( 16.51473224551083163, -9.474510206698727899, 85.83442372801900433 ) ) ;
#73964=CARTESIAN_POINT ( 'NONE',  ( 19.02544592524334988, 5.153800228976608722, 101.4594237280189759 ) ) ;
#73965=CARTESIAN_POINT ( 'NONE',  ( 18.67979575497178502, 10.72451020669898547, 24.16557627198103120 ) ) ;
#73966=CARTESIAN_POINT ( 'NONE',  ( -15.80617190586768217, 15.72974639402176855, 113.1260903946856899 ) ) ;
#73967=CARTESIAN_POINT ( 'NONE',  ( -19.03943276465977164, -0.05219959533935918106, 108.7510903946856615 ) ) ;
#73968=CARTESIAN_POINT ( 'NONE',  ( -12.14591786802309592, -12.06949235617757132, 111.8739096053143669 ) ) ;
#73969=CARTESIAN_POINT ( 'NONE',  ( -16.46253265017160317, 9.564922557960807481, 30.83224293864769550 ) ) ;
#73970=CARTESIAN_POINT ( 'NONE',  ( 5.719274019375991003, -21.55341960407610458, 62.70724293864769550 ) ) ;
#73971=CARTESIAN_POINT ( 'NONE',  ( -13.97604488694527625, -13.89961937509977652, 36.87390960531436690 ) ) ;
#73973=CARTESIAN_POINT ( 'NONE',  ( 13.89961937509957401, 13.97604488694547697, 76.87609039468566152 ) ) ;
#73974=CARTESIAN_POINT ( 'NONE',  ( -8.314922557960811034, -14.29746914071050412, 47.08224293864770260 ) ) ;
#73975=CARTESIAN_POINT ( 'NONE',  ( 21.55341960407610458, 5.719274019375980345, 28.95724293864769905 ) ) ;
#73976=CARTESIAN_POINT ( 'NONE',  ( -21.52544592524334988, -5.823673210054445271, 93.95942372801903275 ) ) ;
#73977=CARTESIAN_POINT ( 'NONE',  ( -18.62759615963270932, 10.81492255796079327, 90.83224293864769550 ) ) ;
#73978=CARTESIAN_POINT ( 'NONE',  ( -21.53943276465977519, -0.05219959533937600094, 63.75109039468568284 ) ) ;
#73979=CARTESIAN_POINT ( 'NONE',  ( 15.72974639402176855, 15.80617190586768217, 66.87609039468568994 ) ) ;
#73980=CARTESIAN_POINT ( 'NONE',  ( 9.564922557960805705, 16.46253265017160317, 99.58224293864770971 ) ) ;
#73981=CARTESIAN_POINT ( 'NONE',  ( -0.05219959533934338120, 16.53943276465976808, 97.50109039468567573 ) ) ;
#73982=CARTESIAN_POINT ( 'NONE',  ( -5.823673210054431948, 21.52544592524334988, 62.70942372801902565 ) ) ;
#73983=CARTESIAN_POINT ( 'NONE',  ( 16.51473224551069308, 9.474510206698969483, 54.16557627198103120 ) ) ;
#73984=CARTESIAN_POINT ( 'NONE',  ( -0.05219959533909027116, -19.03943276465977164, 22.49890960531436690 ) ) ;
#73985=CARTESIAN_POINT ( 'NONE',  ( -9.474510206698964154, 16.51473224551069663, 55.41557627198103120 ) ) ;
#73986=CARTESIAN_POINT ( 'NONE',  ( 16.55341960407611168, 4.379528057220329451, 63.95724293864770260 ) ) ;
#73987=CARTESIAN_POINT ( 'NONE',  ( -8.314922557960811034, -14.29746914071050412, 37.08224293864768129 ) ) ;
#73988=CARTESIAN_POINT ( 'NONE',  ( -15.72974639402197994, 15.80617190586746368, 40.62390960531435269 ) ) ;
#73989=CARTESIAN_POINT ( 'NONE',  ( -19.05341960407611168, -5.049401038298163336, 46.45724293864768129 ) ) ;
#73990=CARTESIAN_POINT ( 'NONE',  ( 5.823673210054125526, 21.52544592524343514, 59.79057627198103120 ) ) ;
#73991=CARTESIAN_POINT ( 'NONE',  ( 19.05341960407617918, -5.049401038297876454, 51.04275706135231871 ) ) ;
#73993=CARTESIAN_POINT ( 'NONE',  ( 12.06949235617757843, -12.14591786802309237, 48.12390960531436690 ) ) ;
#73994=CARTESIAN_POINT ( 'NONE',  ( 21.53943276465977519, -0.05219959533907433946, 23.74890960531435269 ) ) ;
#73996=CARTESIAN_POINT ( 'NONE',  ( 16.38665767535054130, 7.295008042176128527, 102.2359913578545303 ) ) ;
#73997=CARTESIAN_POINT ( 'NONE',  ( -12.14591786802326823, 12.06949235617739902, 83.12609039468568994 ) ) ;
#73998=CARTESIAN_POINT ( 'NONE',  ( 5.153800228976615827, -19.02544592524334988, 70.20942372801899012 ) ) ;
#73999=CARTESIAN_POINT ( 'NONE',  ( 0.05219959533910956823, 16.53943276465976808, 59.99890960531436690 ) ) ;
#74001=CARTESIAN_POINT ( 'NONE',  ( 12.14591786802309770, 12.06949235617756955, 34.37390960531435979 ) ) ;
#74002=CARTESIAN_POINT ( 'NONE',  ( -9.474510206698964154, 16.51473224551069663, 55.41557627198103120 ) ) ;
#74003=CARTESIAN_POINT ( 'NONE',  ( -9.564922557960796823, -16.46253265017161027, 77.08224293864769550 ) ) ;
#74004=CARTESIAN_POINT ( 'NONE',  ( -9.474510206698964154, 16.51473224551069663, 35.41557627198102409 ) ) ;
#74005=CARTESIAN_POINT ( 'NONE',  ( -5.719274019375665041, -21.55341960407619695, 39.79275706135235424 ) ) ;
#74006=CARTESIAN_POINT ( 'NONE',  ( -5.153800228976328057, -19.02544592524343514, 72.29057627198102409 ) ) ;
#74007=CARTESIAN_POINT ( 'NONE',  ( 19.02544592524343514, -5.153800228976328945, 58.54057627198102409 ) ) ;
#74008=CARTESIAN_POINT ( 'NONE',  ( -10.72451020669898014, 18.67979575497178502, 30.41557627198101699 ) ) ;
#74010=CARTESIAN_POINT ( 'NONE',  ( -0.05219959533909027116, -19.03943276465977164, 37.49890960531436690 ) ) ;
#74011=CARTESIAN_POINT ( 'NONE',  ( 5.823673210054125526, 21.52544592524343514, 44.79057627198103120 ) ) ;
#74012=CARTESIAN_POINT ( 'NONE',  ( -0.05219959533934338120, 16.53943276465976808, 92.50109039468567573 ) ) ;
#74013=CARTESIAN_POINT ( 'NONE',  ( 13.89961937509957401, 13.97604488694547697, 21.87609039468566152 ) ) ;
#74014=CARTESIAN_POINT ( 'NONE',  ( 16.53943276465976808, 0.05219959533934440121, 51.25109039468568994 ) ) ;
#74015=CARTESIAN_POINT ( 'NONE',  ( 14.29746914071037800, 8.314922557961029526, 76.66775706135234714 ) ) ;
#74017=CARTESIAN_POINT ( 'NONE',  ( 8.224510206698742110, 14.34966873604972548, 62.08442372801901143 ) ) ;
#74018=CARTESIAN_POINT ( 'NONE',  ( -16.53943276465976808, -0.05219959533934237506, 43.75109039468568284 ) ) ;
#74019=CARTESIAN_POINT ( 'NONE',  ( 16.51473224551069308, 9.474510206698969483, 114.1655762719810241 ) ) ;
#74020=CARTESIAN_POINT ( 'NONE',  ( -12.06949235617739369, -12.14591786802326823, 24.37609039468567573 ) ) ;
#74021=CARTESIAN_POINT ( 'NONE',  ( 9.474510206698971260, -16.51473224551069308, 37.91557627198102409 ) ) ;
#74022=CARTESIAN_POINT ( 'NONE',  ( 15.80617190586769283, -15.72974639402175789, 25.62609039468567929 ) ) ;
#74023=CARTESIAN_POINT ( 'NONE',  ( -0.05219959533934338120, 16.53943276465976808, 37.50109039468568284 ) ) ;
#74024=CARTESIAN_POINT ( 'NONE',  ( -8.224510206698735004, -14.34966873604973081, 94.58442372801901854 ) ) ;
#74026=CARTESIAN_POINT ( 'NONE',  ( 10.72451020669871369, 18.67979575497193778, 102.0844237280190185 ) ) ;
#74027=CARTESIAN_POINT ( 'NONE',  ( -9.564922557961040184, 16.46253265017147172, 92.91775706135233293 ) ) ;
#74028=CARTESIAN_POINT ( 'NONE',  ( 0.05219959533910956823, 16.53943276465976808, 59.99890960531436690 ) ) ;
#74029=CARTESIAN_POINT ( 'NONE',  ( -16.52544592524342804, 4.483927247898546575, 116.0405762719810383 ) ) ;
#74030=CARTESIAN_POINT ( 'NONE',  ( -9.474510206698720793, -16.51473224551083518, 59.58442372801900433 ) ) ;
#74031=CARTESIAN_POINT ( 'NONE',  ( 16.21995358207306026, 7.366697692864119240, 77.56448998487844904 ) ) ;
#74032=CARTESIAN_POINT ( 'NONE',  ( -5.719274019375665041, -21.55341960407619695, 54.79275706135235424 ) ) ;
#74033=CARTESIAN_POINT ( 'NONE',  ( 16.55341960407618274, -4.379528057220086978, 31.04275706135234714 ) ) ;
#74035=CARTESIAN_POINT ( 'NONE',  ( -19.02544592524342804, 5.153800228976336051, 116.0405762719810383 ) ) ;
#74036=CARTESIAN_POINT ( 'NONE',  ( -0.05219959533907301413, -21.53943276465977519, 72.49890960531435269 ) ) ;
#74037=CARTESIAN_POINT ( 'NONE',  ( 19.03943276465977164, 0.05219959533936151252, 106.2510903946856615 ) ) ;
#74038=CARTESIAN_POINT ( 'NONE',  ( -16.46253265017160317, 9.564922557960807481, 100.8322429386477097 ) ) ;
#74040=CARTESIAN_POINT ( 'NONE',  ( 19.02544592524343514, -5.153800228976328945, 23.54057627198102054 ) ) ;
#74041=CARTESIAN_POINT ( 'NONE',  ( -18.62759615963255300, -10.81492255796106328, 89.16775706135236135 ) ) ;
#74042=CARTESIAN_POINT ( 'NONE',  ( -9.564922557960796823, -16.46253265017161027, 42.08224293864769550 ) ) ;
#74043=CARTESIAN_POINT ( 'NONE',  ( -21.55341960407619339, 5.719274019375674811, 53.54275706135234714 ) ) ;
#74044=CARTESIAN_POINT ( 'NONE',  ( -18.62759615963255300, -10.81492255796106328, 94.16775706135237556 ) ) ;
#74045=CARTESIAN_POINT ( 'NONE',  ( 14.29746914071037800, 8.314922557961029526, 101.6677570613523613 ) ) ;
#74046=CARTESIAN_POINT ( 'NONE',  ( -5.153800228976328057, -19.02544592524343514, 82.29057627198103830 ) ) ;
#74047=CARTESIAN_POINT ( 'NONE',  ( -0.05219959533937732626, 21.53943276465977519, 42.50109039468567573 ) ) ;
#74048=CARTESIAN_POINT ( 'NONE',  ( -21.55341960407619339, 5.719274019375674811, 38.54275706135234714 ) ) ;
#74049=CARTESIAN_POINT ( 'NONE',  ( 9.474510206698729675, 16.51473224551082808, 77.08442372801900433 ) ) ;
#74050=CARTESIAN_POINT ( 'NONE',  ( -9.474510206698964154, 16.51473224551069663, 90.41557627198103830 ) ) ;
#74051=CARTESIAN_POINT ( 'NONE',  ( -8.314922557960811034, -14.29746914071050412, 107.0822429386476955 ) ) ;
#74052=CARTESIAN_POINT ( 'NONE',  ( -18.62759615963270932, 10.81492255796079327, 95.83224293864770971 ) ) ;
#74053=CARTESIAN_POINT ( 'NONE',  ( -16.53943276465976808, 0.05219959533911058130, 81.24890960531436690 ) ) ;
#74054=CARTESIAN_POINT ( 'NONE',  ( 13.89961937509957401, 13.97604488694547697, 21.87609039468566152 ) ) ;
#74055=CARTESIAN_POINT ( 'NONE',  ( -4.483927247898539470, -16.52544592524342804, 97.29057627198105251 ) ) ;
#74056=CARTESIAN_POINT ( 'NONE',  ( 16.51473224551069308, 9.474510206698969483, 54.16557627198103120 ) ) ;
#74057=CARTESIAN_POINT ( 'NONE',  ( -9.564922557961040184, 16.46253265017147172, 87.91775706135233293 ) ) ;
#74058=CARTESIAN_POINT ( 'NONE',  ( -16.53943276465976808, 0.05219959533911058130, 46.24890960531435979 ) ) ;
#74059=CARTESIAN_POINT ( 'NONE',  ( -21.55341960407619339, 5.719274019375674811, 113.5427570613523756 ) ) ;
#74060=CARTESIAN_POINT ( 'NONE',  ( -0.05219959533909027116, -19.03943276465977164, 102.4989096053143669 ) ) ;
#74061=CARTESIAN_POINT ( 'NONE',  ( 16.51473224551083163, -9.474510206698727899, 75.83442372801900433 ) ) ;
#74062=CARTESIAN_POINT ( 'NONE',  ( 5.823673210054125526, 21.52544592524343514, 84.79057627198102409 ) ) ;
#74063=CARTESIAN_POINT ( 'NONE',  ( -18.67979575497193778, 10.72451020669871902, 33.33442372801900433 ) ) ;
#74064=CARTESIAN_POINT ( 'NONE',  ( 4.379528057220092307, 16.55341960407617563, 32.29275706135235424 ) ) ;
#74065=CARTESIAN_POINT ( 'NONE',  ( -4.483927247898782831, 16.52544592524335698, 92.70942372801901854 ) ) ;
#74066=CARTESIAN_POINT ( 'NONE',  ( 5.049401038298161559, -19.05341960407611168, 22.70724293864769194 ) ) ;
#74067=CARTESIAN_POINT ( 'NONE',  ( 15.72974639402176855, 15.80617190586768217, 41.87609039468568284 ) ) ;
#74068=CARTESIAN_POINT ( 'NONE',  ( -19.03943276465977164, 0.05219959533909376836, 26.24890960531435624 ) ) ;
#74070=CARTESIAN_POINT ( 'NONE',  ( 12.14591786802327356, -12.06949235617739191, 50.62609039468568994 ) ) ;
#74071=CARTESIAN_POINT ( 'NONE',  ( -16.52544592524342804, 4.483927247898546575, 81.04057627198102409 ) ) ;
#74072=CARTESIAN_POINT ( 'NONE',  ( 15.80617190586746368, 15.72974639402197994, 74.37390960531436690 ) ) ;
#74073=CARTESIAN_POINT ( 'NONE',  ( 16.52544592524342804, -4.483927247898539470, 28.54057627198103120 ) ) ;
#74074=CARTESIAN_POINT ( 'NONE',  ( -16.52544592524335698, -4.483927247898792601, 53.95942372801900433 ) ) ;
#74075=CARTESIAN_POINT ( 'NONE',  ( -19.02544592524342804, 5.153800228976336051, 46.04057627198101699 ) ) ;
#74076=CARTESIAN_POINT ( 'NONE',  ( -8.224510206698735004, -14.34966873604973081, 99.58442372801900433 ) ) ;
#74077=CARTESIAN_POINT ( 'NONE',  ( 5.153800228976615827, -19.02544592524334988, 90.20942372801900433 ) ) ;
#74078=CARTESIAN_POINT ( 'NONE',  ( -18.67979575497178146, -10.72451020669898902, 81.66557627198103830 ) ) ;
#74079=CARTESIAN_POINT ( 'NONE',  ( 4.379528057220092307, 16.55341960407617563, 107.2927570613523471 ) ) ;
#74081=CARTESIAN_POINT ( 'NONE',  ( 13.89961937509977652, -13.97604488694527269, 113.1239096053143527 ) ) ;
#74083=CARTESIAN_POINT ( 'NONE',  ( -18.62759615963270932, 10.81492255796079327, 65.83224293864769550 ) ) ;
#74085=CARTESIAN_POINT ( 'NONE',  ( -4.483927247898782831, 16.52544592524335698, 97.70942372801904696 ) ) ;
#74087=CARTESIAN_POINT ( 'NONE',  ( -0.05219959533907301413, -21.53943276465977519, 32.49890960531435979 ) ) ;
#74088=CARTESIAN_POINT ( 'NONE',  ( 17.50000000000003553, 4.049696124445888223, 108.3196032933406201 ) ) ;
#74089=CARTESIAN_POINT ( 'NONE',  ( -21.52544592524343514, 5.823673210054127303, 81.04057627198102409 ) ) ;
#74090=CARTESIAN_POINT ( 'NONE',  ( 0.05219959533910956823, 16.53943276465976808, 24.99890960531435624 ) ) ;
#74091=CARTESIAN_POINT ( 'NONE',  ( 4.379528057220092307, 16.55341960407617563, 22.29275706135235069 ) ) ;
#74092=CARTESIAN_POINT ( 'NONE',  ( 9.474510206698971260, -16.51473224551069308, 32.91557627198102409 ) ) ;
#74093=CARTESIAN_POINT ( 'NONE',  ( 16.55341960407618274, -4.379528057220086978, 31.04275706135234714 ) ) ;
#74094=CARTESIAN_POINT ( 'NONE',  ( -9.564922557960796823, -16.46253265017161027, 47.08224293864769550 ) ) ;
#74096=CARTESIAN_POINT ( 'NONE',  ( 0.05219959533909260263, 19.03943276465977164, 109.9989096053143669 ) ) ;
#74097=CARTESIAN_POINT ( 'NONE',  ( -5.153800228976328057, -19.02544592524343514, 102.2905762719810383 ) ) ;
#74098=CARTESIAN_POINT ( 'NONE',  ( -16.52544592524335698, -4.483927247898792601, 93.95942372801903275 ) ) ;
#74099=CARTESIAN_POINT ( 'NONE',  ( 19.02544592524334988, 5.153800228976608722, 86.45942372801900433 ) ) ;
#74100=CARTESIAN_POINT ( 'NONE',  ( 13.89961937509957401, 13.97604488694547697, 31.87609039468566863 ) ) ;
#74101=CARTESIAN_POINT ( 'NONE',  ( -0.05219959533907301413, -21.53943276465977519, 77.49890960531433848 ) ) ;
#74102=CARTESIAN_POINT ( 'NONE',  ( -16.52544592524335698, -4.483927247898792601, 103.9594237280190185 ) ) ;
#74103=CARTESIAN_POINT ( 'NONE',  ( 5.823673210054125526, 21.52544592524343514, 34.79057627198103120 ) ) ;
#74104=CARTESIAN_POINT ( 'NONE',  ( 0.05219959533936267826, -19.03943276465977164, 100.0010903946856757 ) ) ;
#74105=CARTESIAN_POINT ( 'NONE',  ( -13.89961937509977652, 13.97604488694528158, 45.62390960531433848 ) ) ;
#74106=CARTESIAN_POINT ( 'NONE',  ( -16.51473224551069308, -9.474510206698971260, 86.66557627198102409 ) ) ;
#74107=CARTESIAN_POINT ( 'NONE',  ( 5.823673210054444382, -21.52544592524334988, 65.20942372801901854 ) ) ;
#74108=CARTESIAN_POINT ( 'NONE',  ( 0.05219959533909260263, 19.03943276465977164, 54.99890960531435979 ) ) ;
#74109=CARTESIAN_POINT ( 'NONE',  ( 12.14591786802309770, 12.06949235617756955, 99.37390960531436690 ) ) ;
#74111=CARTESIAN_POINT ( 'NONE',  ( 8.314922557960818139, 14.29746914071049879, 84.58224293864769550 ) ) ;
#74112=CARTESIAN_POINT ( 'NONE',  ( -10.72451020669898014, 18.67979575497178502, 70.41557627198102409 ) ) ;
#74113=CARTESIAN_POINT ( 'NONE',  ( 19.02544592524334988, 5.153800228976608722, 91.45942372801900433 ) ) ;
#74114=CARTESIAN_POINT ( 'NONE',  ( 17.26058549869093284, -6.457015423128480869, 81.12254162523936429 ) ) ;
#74115=CARTESIAN_POINT ( 'NONE',  ( -19.05341960407611168, -5.049401038298163336, 56.45724293864768129 ) ) ;
#74116=CARTESIAN_POINT ( 'NONE',  ( 19.02544592524343514, -5.153800228976328945, 78.54057627198099567 ) ) ;
#74117=CARTESIAN_POINT ( 'NONE',  ( -16.46253265017160317, 9.564922557960807481, 80.83224293864769550 ) ) ;
#74118=CARTESIAN_POINT ( 'NONE',  ( -16.53943276465976808, -0.05219959533934237506, 68.75109039468568994 ) ) ;
#74119=CARTESIAN_POINT ( 'NONE',  ( -17.05587630539785238, -6.762274262135719027, 49.25819690962688213 ) ) ;
#74120=CARTESIAN_POINT ( 'NONE',  ( 5.153800228976615827, -19.02544592524334988, 40.20942372801898301 ) ) ;
#74122=CARTESIAN_POINT ( 'NONE',  ( -19.03943276465977164, 0.05219959533909376836, 111.2489096053143669 ) ) ;
#74123=CARTESIAN_POINT ( 'NONE',  ( 4.379528057220092307, 16.55341960407617563, 102.2927570613523613 ) ) ;
#74125=CARTESIAN_POINT ( 'NONE',  ( -16.52544592524335698, -4.483927247898792601, 78.95942372801901854 ) ) ;
#74127=CARTESIAN_POINT ( 'NONE',  ( 12.14591786802327356, -12.06949235617739191, 60.62609039468567573 ) ) ;
#74128=CARTESIAN_POINT ( 'NONE',  ( -18.22780087662123805, 5.499999999999981348, 76.01763182126894947 ) ) ;
#74129=CARTESIAN_POINT ( 'NONE',  ( 18.62759615963255655, 10.81492255796105972, 71.66775706135234714 ) ) ;
#74130=CARTESIAN_POINT ( 'NONE',  ( 13.97604488694548053, -13.89961937509957401, 70.62609039468567573 ) ) ;
#74131=CARTESIAN_POINT ( 'NONE',  ( -9.564922557961040184, 16.46253265017147172, 22.91775706135233648 ) ) ;
#74132=CARTESIAN_POINT ( 'NONE',  ( 16.51473224551069308, 9.474510206698969483, 49.16557627198102409 ) ) ;
#74133=CARTESIAN_POINT ( 'NONE',  ( -13.89961937509977652, 13.97604488694528158, 40.62390960531435979 ) ) ;
#74134=CARTESIAN_POINT ( 'NONE',  ( 16.20063489777861676, -7.373262058553140541, 22.00000000000000711 ) ) ;
#74135=CARTESIAN_POINT ( 'NONE',  ( -18.67979575497178146, -10.72451020669898902, 71.66557627198100988 ) ) ;
#74136=CARTESIAN_POINT ( 'NONE',  ( 5.823673210054125526, 21.52544592524343514, 29.79057627198102409 ) ) ;
#74137=CARTESIAN_POINT ( 'NONE',  ( -5.153800228976328057, -19.02544592524343514, 22.29057627198102765 ) ) ;
#74138=CARTESIAN_POINT ( 'NONE',  ( -0.05219959533934338120, 16.53943276465976808, 52.50109039468567573 ) ) ;
#74140=CARTESIAN_POINT ( 'NONE',  ( 18.67979575497194134, -10.72451020669871369, 35.83442372801901143 ) ) ;
#74141=CARTESIAN_POINT ( 'NONE',  ( 14.29746914071049879, -8.314922557960816363, 48.33224293864770260 ) ) ;
#74143=CARTESIAN_POINT ( 'NONE',  ( 8.224510206698742110, 14.34966873604972548, 22.08442372801901143 ) ) ;
#74144=CARTESIAN_POINT ( 'NONE',  ( 9.564922557961047289, -16.46253265017146816, 35.41775706135233293 ) ) ;
#74145=CARTESIAN_POINT ( 'NONE',  ( -16.52544592524342804, 4.483927247898546575, 46.04057627198103830 ) ) ;
#74146=CARTESIAN_POINT ( 'NONE',  ( -21.53943276465977519, -0.05219959533937600094, 23.75109039468567929 ) ) ;
#74148=CARTESIAN_POINT ( 'NONE',  ( -5.719274019375978568, 21.55341960407610458, 75.20724293864769550 ) ) ;
#74149=CARTESIAN_POINT ( 'NONE',  ( -13.97604488694527625, -13.89961937509977652, 91.87390960531432427 ) ) ;
#74150=CARTESIAN_POINT ( 'NONE',  ( 4.379528057220339221, -16.55341960407611168, 57.70724293864770260 ) ) ;
#74151=CARTESIAN_POINT ( 'NONE',  ( -13.89961937509977652, 13.97604488694528158, 105.6239096053143527 ) ) ;
#74154=CARTESIAN_POINT ( 'NONE',  ( -9.474510206698720793, -16.51473224551083518, 59.58442372801900433 ) ) ;
#74155=CARTESIAN_POINT ( 'NONE',  ( 21.52544592524344225, -5.823673210054117533, 103.5405762719810383 ) ) ;
#74156=CARTESIAN_POINT ( 'NONE',  ( 19.02544592524343514, -5.153800228976328945, 38.54057627198103120 ) ) ;
#74157=CARTESIAN_POINT ( 'NONE',  ( 8.314922557960818139, 14.29746914071049879, 109.5822429386476955 ) ) ;
#74158=CARTESIAN_POINT ( 'NONE',  ( -18.62759615963255300, -10.81492255796106328, 54.16775706135235424 ) ) ;
#74160=CARTESIAN_POINT ( 'NONE',  ( 8.314922557960818139, 14.29746914071049879, 44.58224293864769550 ) ) ;
#74161=CARTESIAN_POINT ( 'NONE',  ( 19.02544592524343514, -5.153800228976328945, 43.54057627198103120 ) ) ;
#74162=CARTESIAN_POINT ( 'NONE',  ( 5.049401038298161559, -19.05341960407611168, 102.7072429386476955 ) ) ;
#74163=CARTESIAN_POINT ( 'NONE',  ( 21.55341960407610458, 5.719274019375980345, 78.95724293864769550 ) ) ;
#74165=CARTESIAN_POINT ( 'NONE',  ( -19.02544592524342804, 5.153800228976336051, 51.04057627198103120 ) ) ;
#74167=CARTESIAN_POINT ( 'NONE',  ( -21.53943276465977519, 0.05219959533907696930, 66.24890960531436690 ) ) ;
#74169=CARTESIAN_POINT ( 'NONE',  ( 5.719274019375673035, 21.55341960407619339, 92.29275706135236135 ) ) ;
#74170=CARTESIAN_POINT ( 'NONE',  ( -17.49999999999999645, 5.499999999999985789, 38.71769037696434879 ) ) ;
#74171=CARTESIAN_POINT ( 'NONE',  ( 0.05219959533934541429, -16.53943276465976808, 80.00109039468568994 ) ) ;
#74172=CARTESIAN_POINT ( 'NONE',  ( -4.379528057220328563, 16.55341960407611168, 80.20724293864769550 ) ) ;
#74173=CARTESIAN_POINT ( 'NONE',  ( 16.51473224551069308, 9.474510206698969483, 69.16557627198102409 ) ) ;
#74174=ORIENTED_EDGE ( 'NONE', *, *, #27973, .T. ) ;
#74175=CARTESIAN_POINT ( 'NONE',  ( 0.05219959533936267826, -19.03943276465977164, 30.00109039468566863 ) ) ;
#74176=CARTESIAN_POINT ( 'NONE',  ( -16.55341960407617563, 4.379528057220093196, 88.54275706135236135 ) ) ;
#74177=CARTESIAN_POINT ( 'NONE',  ( 21.53943276465977519, 0.05219959533937863772, 106.2510903946856757 ) ) ;
#74178=CARTESIAN_POINT ( 'NONE',  ( -9.474510206698964154, 16.51473224551069663, 75.41557627198103830 ) ) ;
#74179=CARTESIAN_POINT ( 'NONE',  ( -18.62759615963270932, 10.81492255796079327, 45.83224293864769550 ) ) ;
#74180=CARTESIAN_POINT ( 'NONE',  ( 10.81492255796106328, -18.62759615963255655, 90.41775706135236135 ) ) ;
#74181=CARTESIAN_POINT ( 'NONE',  ( 14.29746914071037800, 8.314922557961029526, 56.66775706135235424 ) ) ;
#74182=CARTESIAN_POINT ( 'NONE',  ( 10.72451020669898902, -18.67979575497178502, 112.9155762719810383 ) ) ;
#74183=CARTESIAN_POINT ( 'NONE',  ( 9.474510206698729675, 16.51473224551082808, 112.0844237280190043 ) ) ;
#74184=CARTESIAN_POINT ( 'NONE',  ( -19.02544592524342804, 5.153800228976336051, 91.04057627198100988 ) ) ;
#74185=CARTESIAN_POINT ( 'NONE',  ( -12.14591786802326823, 12.06949235617739902, 33.12609039468569705 ) ) ;
#74186=CARTESIAN_POINT ( 'NONE',  ( -16.46253265017160317, 9.564922557960807481, 55.83224293864769550 ) ) ;
#74188=CARTESIAN_POINT ( 'NONE',  ( 12.06949235617739724, 12.14591786802326823, 36.87609039468568994 ) ) ;
#74189=CARTESIAN_POINT ( 'NONE',  ( -8.224510206698948167, 14.34966873604960824, 75.41557627198102409 ) ) ;
#74190=CARTESIAN_POINT ( 'NONE',  ( -14.29746914071037622, -8.314922557961029526, 84.16775706135234714 ) ) ;
#74191=CARTESIAN_POINT ( 'NONE',  ( -5.823673210054431948, 21.52544592524334988, 42.70942372801901854 ) ) ;
#74192=CARTESIAN_POINT ( 'NONE',  ( 13.97604488694527802, 13.89961937509977652, 59.37390960531434558 ) ) ;
#74193=CARTESIAN_POINT ( 'NONE',  ( 16.51473224551069308, 9.474510206698969483, 79.16557627198103830 ) ) ;
#74194=CARTESIAN_POINT ( 'NONE',  ( 14.34966873604972726, -8.224510206698740333, 90.83442372801901854 ) ) ;
#74197=CARTESIAN_POINT ( 'NONE',  ( -9.564922557961040184, 16.46253265017147172, 27.91775706135232582 ) ) ;
#74198=CARTESIAN_POINT ( 'NONE',  ( -9.474510206698964154, 16.51473224551069663, 100.4155762719810241 ) ) ;
#74199=CARTESIAN_POINT ( 'NONE',  ( 16.51473224551069308, 9.474510206698969483, 49.16557627198102409 ) ) ;
#74200=CARTESIAN_POINT ( 'NONE',  ( -19.05341960407611168, -5.049401038298163336, 111.4572429386476671 ) ) ;
#74201=CARTESIAN_POINT ( 'NONE',  ( 0.05219959533934541429, -16.53943276465976808, 45.00109039468568284 ) ) ;
#74202=CARTESIAN_POINT ( 'NONE',  ( -16.46253265017146816, -9.564922557961047289, 59.16775706135233293 ) ) ;
#74203=CARTESIAN_POINT ( 'NONE',  ( 0.05219959533934541429, -16.53943276465976808, 60.00109039468568284 ) ) ;
#74205=CARTESIAN_POINT ( 'NONE',  ( 19.02544592524343514, -5.153800228976328945, 83.54057627198100988 ) ) ;
#74206=CARTESIAN_POINT ( 'NONE',  ( 18.62759615963271287, -10.81492255796078972, 108.3322429386477097 ) ) ;
#74207=CARTESIAN_POINT ( 'NONE',  ( 13.89961937509957401, 13.97604488694547697, 61.87609039468566863 ) ) ;
#74208=CARTESIAN_POINT ( 'NONE',  ( -5.153800228976328057, -19.02544592524343514, 97.29057627198099567 ) ) ;
#74209=CARTESIAN_POINT ( 'NONE',  ( 5.049401038298161559, -19.05341960407611168, 22.70724293864769194 ) ) ;
#74211=CARTESIAN_POINT ( 'NONE',  ( -16.51473224551069308, -9.474510206698971260, 76.66557627198103830 ) ) ;
#74212=CARTESIAN_POINT ( 'NONE',  ( -16.53943276465976808, 0.05219959533911058130, 36.24890960531435979 ) ) ;
#74213=CARTESIAN_POINT ( 'NONE',  ( 9.564922557960805705, 16.46253265017160317, 24.58224293864769194 ) ) ;
#74214=CARTESIAN_POINT ( 'NONE',  ( -9.474510206698720793, -16.51473224551083518, 44.58442372801900433 ) ) ;
#74215=CARTESIAN_POINT ( 'NONE',  ( 4.483927247898545687, 16.52544592524342804, 69.79057627198102409 ) ) ;
#74216=CARTESIAN_POINT ( 'NONE',  ( 15.80617190586769283, -15.72974639402175789, 100.6260903946857184 ) ) ;
#74217=CARTESIAN_POINT ( 'NONE',  ( -0.05219959533909027116, -19.03943276465977164, 37.49890960531436690 ) ) ;
#74218=CARTESIAN_POINT ( 'NONE',  ( -8.314922557960811034, -14.29746914071050412, 37.08224293864768129 ) ) ;
#74219=CARTESIAN_POINT ( 'NONE',  ( -21.53943276465977519, -0.05219959533937600094, 98.75109039468568994 ) ) ;
#74220=CARTESIAN_POINT ( 'NONE',  ( 5.153800228976335163, 19.02544592524342804, 99.79057627198102409 ) ) ;
#74221=CARTESIAN_POINT ( 'NONE',  ( 5.153800228976335163, 19.02544592524342804, 89.79057627198102409 ) ) ;
#74222=CARTESIAN_POINT ( 'NONE',  ( -19.02544592524342804, 5.153800228976336051, 41.04057627198103120 ) ) ;
#74223=CARTESIAN_POINT ( 'NONE',  ( 14.34966873604960469, 8.224510206698951720, 104.1655762719810241 ) ) ;
#74224=CARTESIAN_POINT ( 'NONE',  ( 8.314922557960818139, 14.29746914071049879, 74.58224293864768129 ) ) ;
#74225=CARTESIAN_POINT ( 'NONE',  ( -21.53943276465977519, 0.05219959533907696930, 86.24890960531436690 ) ) ;
#74226=CARTESIAN_POINT ( 'NONE',  ( -9.474510206698964154, 16.51473224551069663, 85.41557627198102409 ) ) ;
#74227=CARTESIAN_POINT ( 'NONE',  ( -18.67979575497178146, -10.72451020669898902, 101.6655762719810383 ) ) ;
#74228=CARTESIAN_POINT ( 'NONE',  ( -5.153800228976328057, -19.02544592524343514, 92.29057627198099567 ) ) ;
#74229=CARTESIAN_POINT ( 'NONE',  ( -19.34837522270365540, -5.499999999999852562, 90.86337684832578532 ) ) ;
#74230=CARTESIAN_POINT ( 'NONE',  ( 14.34966873604960469, 8.224510206698951720, 99.16557627198100988 ) ) ;
#74231=CARTESIAN_POINT ( 'NONE',  ( 9.564922557960805705, 16.46253265017160317, 74.58224293864769550 ) ) ;
#74232=CARTESIAN_POINT ( 'NONE',  ( 15.72974639402199770, -15.80617190586745480, 83.12390960531436690 ) ) ;
#74234=CARTESIAN_POINT ( 'NONE',  ( -21.55341960407610458, -5.719274019375992779, 31.45724293864769550 ) ) ;
#74236=CARTESIAN_POINT ( 'NONE',  ( -19.03943276465977164, -0.05219959533935918106, 113.7510903946856757 ) ) ;
#74237=CARTESIAN_POINT ( 'NONE',  ( -14.34966873604960291, -8.224510206698953496, 96.66557627198102409 ) ) ;
#74238=CARTESIAN_POINT ( 'NONE',  ( -16.52216118717208815, -7.221426719304519182, 96.07599021046995347 ) ) ;
#74239=CARTESIAN_POINT ( 'NONE',  ( -9.564922557960796823, -16.46253265017161027, 82.08224293864768129 ) ) ;
#74240=CARTESIAN_POINT ( 'NONE',  ( 16.46253265017160672, -9.564922557960803928, 43.33224293864769550 ) ) ;
#74241=CARTESIAN_POINT ( 'NONE',  ( -14.29746914071049879, 8.314922557960819915, 85.83224293864768129 ) ) ;
#74242=CARTESIAN_POINT ( 'NONE',  ( -16.51473224551069308, -9.474510206698971260, 111.6655762719810383 ) ) ;
#74243=CARTESIAN_POINT ( 'NONE',  ( 4.379528057220339221, -16.55341960407611168, 57.70724293864770260 ) ) ;
#74244=CARTESIAN_POINT ( 'NONE',  ( 16.51473224551083163, -9.474510206698727899, 100.8344237280190043 ) ) ;
#74245=CARTESIAN_POINT ( 'NONE',  ( 5.823673210054444382, -21.52544592524334988, 65.20942372801901854 ) ) ;
#74247=CARTESIAN_POINT ( 'NONE',  ( 16.51473224551069308, 9.474510206698969483, 94.16557627198103830 ) ) ;
#74248=CARTESIAN_POINT ( 'NONE',  ( 10.81492255796078972, 18.62759615963270932, 84.58224293864769550 ) ) ;
#74249=CARTESIAN_POINT ( 'NONE',  ( 8.314922557961029526, -14.29746914071037800, 90.41775706135236135 ) ) ;
#74250=CARTESIAN_POINT ( 'NONE',  ( -5.153800228976328057, -19.02544592524343514, 22.29057627198102765 ) ) ;
#74251=CARTESIAN_POINT ( 'NONE',  ( 5.153800228976335163, 19.02544592524342804, 74.79057627198103830 ) ) ;
#74252=CARTESIAN_POINT ( 'NONE',  ( 15.72974639402199770, -15.80617190586745480, 83.12390960531436690 ) ) ;
#74253=CARTESIAN_POINT ( 'NONE',  ( 9.474510206698729675, 16.51473224551082808, 107.0844237280190043 ) ) ;
#74254=CARTESIAN_POINT ( 'NONE',  ( -14.29746914071049879, 8.314922557960819915, 50.83224293864770971 ) ) ;
#74255=CARTESIAN_POINT ( 'NONE',  ( 21.52544592524334988, 5.823673210054432836, 56.45942372801902565 ) ) ;
#74256=CARTESIAN_POINT ( 'NONE',  ( -14.34966873604972548, 8.224510206698743886, 83.33442372801903275 ) ) ;
#74257=CARTESIAN_POINT ( 'NONE',  ( -10.81492255796078084, -18.62759615963271287, 22.08224293864769194 ) ) ;
#74258=CARTESIAN_POINT ( 'NONE',  ( -9.474510206698964154, 16.51473224551069663, 110.4155762719810383 ) ) ;
#74259=CARTESIAN_POINT ( 'NONE',  ( 18.22780087662119897, -5.500000000000096811, 58.51763182126894947 ) ) ;
#74260=CARTESIAN_POINT ( 'NONE',  ( -12.14591786802326823, 12.06949235617739902, 103.1260903946856757 ) ) ;
#74261=CARTESIAN_POINT ( 'NONE',  ( -12.06949235617739369, -12.14591786802326823, 64.37609039468568994 ) ) ;
#74262=CARTESIAN_POINT ( 'NONE',  ( 5.049401038298161559, -19.05341960407611168, 52.70724293864767418 ) ) ;
#74263=CARTESIAN_POINT ( 'NONE',  ( 5.153800228976335163, 19.02544592524342804, 69.79057627198103830 ) ) ;
#74264=CARTESIAN_POINT ( 'NONE',  ( 16.53943276465976808, 0.05219959533934440121, 76.25109039468568994 ) ) ;
#74265=CARTESIAN_POINT ( 'NONE',  ( -16.53943276465976808, 0.05219959533911058130, 51.24890960531436690 ) ) ;
#74266=CARTESIAN_POINT ( 'NONE',  ( 16.51473224551069308, 9.474510206698969483, 59.16557627198102409 ) ) ;
#74267=CARTESIAN_POINT ( 'NONE',  ( -13.97604488694527625, -13.89961937509977652, 46.87390960531435979 ) ) ;
#74268=CARTESIAN_POINT ( 'NONE',  ( 14.34966873604972726, -8.224510206698740333, 35.83442372801901143 ) ) ;
#74270=CARTESIAN_POINT ( 'NONE',  ( 9.474510206698729675, 16.51473224551082808, 92.08442372801900433 ) ) ;
#74271=CARTESIAN_POINT ( 'NONE',  ( -4.379528057220328563, 16.55341960407611168, 95.20724293864769550 ) ) ;
#74272=CARTESIAN_POINT ( 'NONE',  ( -19.02544592524342804, 5.153800228976336051, 61.04057627198103120 ) ) ;
#74273=CARTESIAN_POINT ( 'NONE',  ( -16.46253265017146816, -9.564922557961047289, 99.16775706135233293 ) ) ;
#74275=CARTESIAN_POINT ( 'NONE',  ( -5.719274019375665041, -21.55341960407619695, 109.7927570613523613 ) ) ;
#74276=CARTESIAN_POINT ( 'NONE',  ( -14.34966873604972548, 8.224510206698743886, 73.33442372801901854 ) ) ;
#74278=CARTESIAN_POINT ( 'NONE',  ( -10.81492255796078084, -18.62759615963271287, 62.08224293864769550 ) ) ;
#74279=CARTESIAN_POINT ( 'NONE',  ( -16.53943276465976808, -0.05219959533934237506, 53.75109039468568994 ) ) ;
#74280=CARTESIAN_POINT ( 'NONE',  ( -16.51473224551069308, -9.474510206698971260, 31.66557627198102054 ) ) ;
#74281=CARTESIAN_POINT ( 'NONE',  ( -16.51473224551082808, 9.474510206698731452, 38.33442372801899722 ) ) ;
#74282=CARTESIAN_POINT ( 'NONE',  ( -16.46253265017160317, 9.564922557960807481, 90.83224293864769550 ) ) ;
#74283=CARTESIAN_POINT ( 'NONE',  ( 16.55341960407611168, 4.379528057220329451, 113.9572429386477239 ) ) ;
#74284=CARTESIAN_POINT ( 'NONE',  ( 0.05219959533909260263, 19.03943276465977164, 69.99890960531435269 ) ) ;
#74285=CARTESIAN_POINT ( 'NONE',  ( -15.72974639402176322, -15.80617190586768395, 79.37609039468567573 ) ) ;
#74286=EDGE_CURVE ( 'NONE', #142306, #189322, #193231, .T. ) ;
#74287=CARTESIAN_POINT ( 'NONE',  ( -9.564922557961040184, 16.46253265017147172, 52.91775706135233293 ) ) ;
#74288=CARTESIAN_POINT ( 'NONE',  ( 13.97604488694548053, -13.89961937509957401, 25.62609039468566507 ) ) ;
#74289=CARTESIAN_POINT ( 'NONE',  ( 19.03943276465977164, -0.05219959533909143690, 58.74890960531435979 ) ) ;
#74290=CARTESIAN_POINT ( 'NONE',  ( 16.46253265017160672, -9.564922557960803928, 113.3322429386476955 ) ) ;
#74291=CARTESIAN_POINT ( 'NONE',  ( -18.62759615963255300, -10.81492255796106328, 84.16775706135234714 ) ) ;
#74292=CARTESIAN_POINT ( 'NONE',  ( -19.02544592524342804, 5.153800228976336051, 61.04057627198103120 ) ) ;
#74293=CARTESIAN_POINT ( 'NONE',  ( -10.72451020669870658, -18.67979575497194134, 94.58442372801901854 ) ) ;
#74294=CARTESIAN_POINT ( 'NONE',  ( -15.80617190586745835, -15.72974639402198527, 31.87390960531435979 ) ) ;
#74295=CARTESIAN_POINT ( 'NONE',  ( -16.51473224551069308, -9.474510206698971260, 86.66557627198102409 ) ) ;
#74296=CARTESIAN_POINT ( 'NONE',  ( -21.53943276465977519, -0.05219959533937600094, 43.75109039468568284 ) ) ;
#74297=CARTESIAN_POINT ( 'NONE',  ( 16.46253265017146816, 9.564922557961045513, 56.66775706135233293 ) ) ;
#74298=CARTESIAN_POINT ( 'NONE',  ( -19.02544592524342804, 5.153800228976336051, 36.04057627198100988 ) ) ;
#74299=CARTESIAN_POINT ( 'NONE',  ( -19.03943276465977164, 0.05219959533909376836, 91.24890960531436690 ) ) ;
#74300=CARTESIAN_POINT ( 'NONE',  ( 12.14591786802327356, -12.06949235617739191, 25.62609039468567929 ) ) ;
#74301=CARTESIAN_POINT ( 'NONE',  ( 0.05219959533910956823, 16.53943276465976808, 94.99890960531436690 ) ) ;
#74302=CARTESIAN_POINT ( 'NONE',  ( 16.51473224551069308, 9.474510206698969483, 74.16557627198103830 ) ) ;
#74304=CARTESIAN_POINT ( 'NONE',  ( 5.823673210054125526, 21.52544592524343514, 54.79057627198104541 ) ) ;
#74306=CARTESIAN_POINT ( 'NONE',  ( -16.51473224551082808, 9.474510206698731452, 113.3344237280190043 ) ) ;
#74307=CARTESIAN_POINT ( 'NONE',  ( 0.05219959533937995610, -21.53943276465977519, 20.00109039468568639 ) ) ;
#74308=CARTESIAN_POINT ( 'NONE',  ( -21.52544592524334988, -5.823673210054445271, 73.95942372801901854 ) ) ;
#74309=CARTESIAN_POINT ( 'NONE',  ( -16.53943276465976808, -0.05219959533934237506, 63.75109039468568284 ) ) ;
#74310=CARTESIAN_POINT ( 'NONE',  ( -12.06949235617739369, -12.14591786802326823, 64.37609039468568994 ) ) ;
#74311=CARTESIAN_POINT ( 'NONE',  ( -19.03943276465977164, 0.05219959533909376836, 61.24890960531436690 ) ) ;
#74312=CARTESIAN_POINT ( 'NONE',  ( -14.34966873604972548, 8.224510206698743886, 98.33442372801901854 ) ) ;
#74313=CARTESIAN_POINT ( 'NONE',  ( -5.153800228976607833, 19.02544592524334988, 47.70942372801900433 ) ) ;
#74314=CARTESIAN_POINT ( 'NONE',  ( 10.81492255796078972, 18.62759615963270932, 114.5822429386477097 ) ) ;
#74315=CARTESIAN_POINT ( 'NONE',  ( -8.224510206698948167, 14.34966873604960824, 60.41557627198102409 ) ) ;
#74316=CARTESIAN_POINT ( 'NONE',  ( -19.05341960407611168, -5.049401038298163336, 91.45724293864766707 ) ) ;
#74317=CARTESIAN_POINT ( 'NONE',  ( 8.314922557961029526, -14.29746914071037800, 90.41775706135236135 ) ) ;
#74318=CARTESIAN_POINT ( 'NONE',  ( -10.72451020669870658, -18.67979575497194134, 64.58442372801900433 ) ) ;
#74319=CARTESIAN_POINT ( 'NONE',  ( 16.55341960407618274, -4.379528057220086978, 31.04275706135234714 ) ) ;
#74320=CARTESIAN_POINT ( 'NONE',  ( 10.81492255796106328, -18.62759615963255655, 30.41775706135234358 ) ) ;
#74321=CARTESIAN_POINT ( 'NONE',  ( 8.224510206698953496, -14.34966873604960469, 57.91557627198103120 ) ) ;
#74323=CARTESIAN_POINT ( 'NONE',  ( -0.05219959533907301413, -21.53943276465977519, 102.4989096053143811 ) ) ;
#74324=CARTESIAN_POINT ( 'NONE',  ( 0.05219959533910956823, 16.53943276465976808, 39.99890960531436690 ) ) ;
#74327=CARTESIAN_POINT ( 'NONE',  ( 18.67979575497178502, 10.72451020669898547, 34.16557627198102409 ) ) ;
#74328=CARTESIAN_POINT ( 'NONE',  ( -15.80617190586768217, 15.72974639402176855, 38.12609039468567573 ) ) ;
#74329=CARTESIAN_POINT ( 'NONE',  ( -12.06949235617756955, 12.14591786802309770, 70.62390960531436690 ) ) ;
#74331=CARTESIAN_POINT ( 'NONE',  ( -21.52544592524343514, 5.823673210054127303, 71.04057627198103830 ) ) ;
#74332=CARTESIAN_POINT ( 'NONE',  ( -13.89961937509977652, 13.97604488694528158, 80.62390960531436690 ) ) ;
#74333=CARTESIAN_POINT ( 'NONE',  ( 9.474510206698971260, -16.51473224551069308, 27.91557627198103120 ) ) ;
#74334=CARTESIAN_POINT ( 'NONE',  ( 16.51473224551083163, -9.474510206698727899, 65.83442372801900433 ) ) ;
#74335=CARTESIAN_POINT ( 'NONE',  ( 21.53943276465977519, -0.05219959533907433946, 48.74890960531435979 ) ) ;
#74336=CARTESIAN_POINT ( 'NONE',  ( 19.05341960407611168, 5.049401038298154454, 63.95724293864769550 ) ) ;
#74337=CARTESIAN_POINT ( 'NONE',  ( -14.34966873604972548, 8.224510206698743886, 38.33442372801900433 ) ) ;
#74338=CARTESIAN_POINT ( 'NONE',  ( 10.81492255796078972, 18.62759615963270932, 109.5822429386476955 ) ) ;
#74339=CARTESIAN_POINT ( 'NONE',  ( -16.52544592524342804, 4.483927247898546575, 51.04057627198103120 ) ) ;
#74340=CARTESIAN_POINT ( 'NONE',  ( 5.153800228976335163, 19.02544592524342804, 104.7905762719809957 ) ) ;
#74341=CARTESIAN_POINT ( 'NONE',  ( 18.67979575497178502, 10.72451020669898547, 69.16557627198102409 ) ) ;
#74342=CARTESIAN_POINT ( 'NONE',  ( 15.72974639402199770, -15.80617190586745480, 108.1239096053143811 ) ) ;
#74343=CARTESIAN_POINT ( 'NONE',  ( 16.53943276465976808, 0.05219959533934440121, 41.25109039468568284 ) ) ;
#74344=CARTESIAN_POINT ( 'NONE',  ( 10.72451020669898902, -18.67979575497178502, 42.91557627198103120 ) ) ;
#74345=CARTESIAN_POINT ( 'NONE',  ( 21.55341960407619695, -5.719274019375665929, 96.04275706135236135 ) ) ;
#74346=CARTESIAN_POINT ( 'NONE',  ( -19.02544592524342804, 5.153800228976336051, 41.04057627198103120 ) ) ;
#74347=CARTESIAN_POINT ( 'NONE',  ( 19.03943276465977164, -0.05219959533909143690, 93.74890960531435269 ) ) ;
#74348=CARTESIAN_POINT ( 'NONE',  ( -19.03943276465977164, 0.05219959533909376836, 76.24890960531435269 ) ) ;
#74349=CARTESIAN_POINT ( 'NONE',  ( 17.31728774477213406, -6.344390552233679870, 88.31906651689307353 ) ) ;
#74350=CARTESIAN_POINT ( 'NONE',  ( -0.05219959533936034679, 19.03943276465977164, 52.50109039468566863 ) ) ;
#74351=CARTESIAN_POINT ( 'NONE',  ( -18.62759615963255300, -10.81492255796106328, 109.1677570613523613 ) ) ;
#74352=CARTESIAN_POINT ( 'NONE',  ( -10.72451020669898014, 18.67979575497178502, 35.41557627198102409 ) ) ;
#74353=CARTESIAN_POINT ( 'NONE',  ( -8.224510206698735004, -14.34966873604973081, 109.5844237280190328 ) ) ;
#74354=CARTESIAN_POINT ( 'NONE',  ( 13.97604488694548053, -13.89961937509957401, 90.62609039468567573 ) ) ;
#74356=CARTESIAN_POINT ( 'NONE',  ( 0.05219959533936267826, -19.03943276465977164, 90.00109039468567573 ) ) ;
#74357=CARTESIAN_POINT ( 'NONE',  ( 13.97604488694548053, -13.89961937509957401, 50.62609039468566152 ) ) ;
#74358=CARTESIAN_POINT ( 'NONE',  ( -16.38665767535053064, -7.295008042176048590, 44.73599135785455871 ) ) ;
#74359=CARTESIAN_POINT ( 'NONE',  ( -16.46253265017160317, 9.564922557960807481, 40.83224293864769550 ) ) ;
#74360=CARTESIAN_POINT ( 'NONE',  ( 4.483927247898545687, 16.52544592524342804, 49.79057627198102409 ) ) ;
#74361=CARTESIAN_POINT ( 'NONE',  ( -17.31728774477273802, -6.344390552232371583, 109.1809334831068412 ) ) ;
#74362=CARTESIAN_POINT ( 'NONE',  ( 4.483927247898545687, 16.52544592524342804, 24.79057627198103120 ) ) ;
#74364=CARTESIAN_POINT ( 'NONE',  ( -8.224510206698735004, -14.34966873604973081, 94.58442372801901854 ) ) ;
#74365=CARTESIAN_POINT ( 'NONE',  ( 0.05219959533909260263, 19.03943276465977164, 54.99890960531435979 ) ) ;
#74366=CARTESIAN_POINT ( 'NONE',  ( -18.67979575497193778, 10.72451020669871902, 103.3344237280190043 ) ) ;
#74367=CARTESIAN_POINT ( 'NONE',  ( -4.483927247898782831, 16.52544592524335698, 22.70942372801901499 ) ) ;
#74368=CARTESIAN_POINT ( 'NONE',  ( 5.719274019375991003, -21.55341960407610458, 37.70724293864769550 ) ) ;
#74369=CARTESIAN_POINT ( 'NONE',  ( -21.55341960407619339, 5.719274019375674811, 98.54275706135234714 ) ) ;
#74370=ORIENTED_EDGE ( 'NONE', *, *, #169635, .T. ) ;
#74371=CARTESIAN_POINT ( 'NONE',  ( 16.51473224551069308, 9.474510206698969483, 99.16557627198102409 ) ) ;
#74372=CARTESIAN_POINT ( 'NONE',  ( 0.05219959533909260263, 19.03943276465977164, 84.99890960531436690 ) ) ;
#74374=CARTESIAN_POINT ( 'NONE',  ( 21.55341960407610458, 5.719274019375980345, 103.9572429386476813 ) ) ;
#74375=CARTESIAN_POINT ( 'NONE',  ( -14.34966873604960291, -8.224510206698953496, 81.66557627198103830 ) ) ;
#74376=CARTESIAN_POINT ( 'NONE',  ( -5.823673210054116645, -21.52544592524344225, 77.29057627198102409 ) ) ;
#74377=CARTESIAN_POINT ( 'NONE',  ( 5.153800228976335163, 19.02544592524342804, 54.79057627198103120 ) ) ;
#74378=CARTESIAN_POINT ( 'NONE',  ( -18.62759615963270932, 10.81492255796079327, 95.83224293864770971 ) ) ;
#74379=ORIENTED_EDGE ( 'NONE', *, *, #153559, .F. ) ;
#74380=CARTESIAN_POINT ( 'NONE',  ( -9.474510206698964154, 16.51473224551069663, 65.41557627198102409 ) ) ;
#74381=CARTESIAN_POINT ( 'NONE',  ( 16.52544592524342804, -4.483927247898539470, 98.54057627198105251 ) ) ;
#74383=CARTESIAN_POINT ( 'NONE',  ( 16.51473224551069308, 9.474510206698969483, 69.16557627198102409 ) ) ;
#74384=CARTESIAN_POINT ( 'NONE',  ( -0.05219959533936034679, 19.03943276465977164, 82.50109039468567573 ) ) ;
#74385=CARTESIAN_POINT ( 'NONE',  ( -14.29746914071049879, 8.314922557960819915, 90.83224293864769550 ) ) ;
#74386=CARTESIAN_POINT ( 'NONE',  ( 21.52544592524334988, 5.823673210054432836, 61.45942372801901854 ) ) ;
#74387=CARTESIAN_POINT ( 'NONE',  ( 19.05341960407611168, 5.049401038298154454, 48.95724293864768129 ) ) ;
#74388=CARTESIAN_POINT ( 'NONE',  ( 18.62759615963271287, -10.81492255796078972, 113.3322429386476955 ) ) ;
#74389=CARTESIAN_POINT ( 'NONE',  ( -12.14591786802309592, -12.06949235617757132, 106.8739096053143811 ) ) ;
#74391=CARTESIAN_POINT ( 'NONE',  ( 16.51473224551069308, 9.474510206698969483, 59.16557627198102409 ) ) ;
#74393=CARTESIAN_POINT ( 'NONE',  ( -5.153800228976607833, 19.02544592524334988, 112.7094237280190043 ) ) ;
#74394=CARTESIAN_POINT ( 'NONE',  ( -19.03943276465977164, 0.05219959533909376836, 106.2489096053143669 ) ) ;
#74395=CARTESIAN_POINT ( 'NONE',  ( -18.62759615963255300, -10.81492255796106328, 54.16775706135235424 ) ) ;
#74396=CARTESIAN_POINT ( 'NONE',  ( 19.05341960407611168, 5.049401038298154454, 98.95724293864766707 ) ) ;
#74397=CARTESIAN_POINT ( 'NONE',  ( -13.97604488694547697, 13.89961937509957934, 88.12609039468563310 ) ) ;
#74398=CARTESIAN_POINT ( 'NONE',  ( 9.564922557960805705, 16.46253265017160317, 64.58224293864769550 ) ) ;
#74399=CARTESIAN_POINT ( 'NONE',  ( -12.14591786802309592, -12.06949235617757132, 76.87390960531439532 ) ) ;
#74400=CARTESIAN_POINT ( 'NONE',  ( -4.379528057220328563, 16.55341960407611168, 85.20724293864770971 ) ) ;
#74401=CARTESIAN_POINT ( 'NONE',  ( -5.153800228976328057, -19.02544592524343514, 87.29057627198103830 ) ) ;
#74402=CARTESIAN_POINT ( 'NONE',  ( 4.379528057220339221, -16.55341960407611168, 72.70724293864769550 ) ) ;
#74403=CARTESIAN_POINT ( 'NONE',  ( 19.05341960407611168, 5.049401038298154454, 83.95724293864766707 ) ) ;
#74404=CARTESIAN_POINT ( 'NONE',  ( 19.03943276465977164, 0.05219959533936151252, 26.25109039468566507 ) ) ;
#74405=CARTESIAN_POINT ( 'NONE',  ( 0.05219959533909260263, 19.03943276465977164, 54.99890960531435979 ) ) ;
#74406=CARTESIAN_POINT ( 'NONE',  ( 0.05219959533910956823, 16.53943276465976808, 34.99890960531435979 ) ) ;
#74407=CARTESIAN_POINT ( 'NONE',  ( -19.05341960407611168, -5.049401038298163336, 26.45724293864769550 ) ) ;
#74409=CARTESIAN_POINT ( 'NONE',  ( -21.52544592524334988, -5.823673210054445271, 48.95942372801902565 ) ) ;
#74410=CARTESIAN_POINT ( 'NONE',  ( -19.05341960407617563, 5.049401038297882671, 78.54275706135233293 ) ) ;
#74411=CARTESIAN_POINT ( 'NONE',  ( 8.314922557960818139, 14.29746914071049879, 34.58224293864770260 ) ) ;
#74412=CARTESIAN_POINT ( 'NONE',  ( 5.719274019375991003, -21.55341960407610458, 92.70724293864770971 ) ) ;
#74413=CARTESIAN_POINT ( 'NONE',  ( -15.80617190586745835, -15.72974639402198527, 36.87390960531435979 ) ) ;
#74414=CARTESIAN_POINT ( 'NONE',  ( -14.29746914071049879, 8.314922557960819915, 65.83224293864769550 ) ) ;
#74415=CARTESIAN_POINT ( 'NONE',  ( 16.46253265017160672, -9.564922557960803928, 48.33224293864769550 ) ) ;
#74416=CARTESIAN_POINT ( 'NONE',  ( 16.52544592524335698, 4.483927247898782831, 96.45942372801901854 ) ) ;
#74417=CARTESIAN_POINT ( 'NONE',  ( 16.53943276465976808, 0.05219959533934440121, 76.25109039468568994 ) ) ;
#74418=CARTESIAN_POINT ( 'NONE',  ( 5.823673210054125526, 21.52544592524343514, 39.79057627198103830 ) ) ;
#74419=CARTESIAN_POINT ( 'NONE',  ( -5.049401038297874678, -19.05341960407617918, 24.79275706135233648 ) ) ;
#74420=CARTESIAN_POINT ( 'NONE',  ( 16.51473224551069308, 9.474510206698969483, 89.16557627198103830 ) ) ;
#74421=CARTESIAN_POINT ( 'NONE',  ( -0.05219959533934338120, 16.53943276465976808, 67.50109039468568994 ) ) ;
#74422=CARTESIAN_POINT ( 'NONE',  ( -16.53943276465976808, 0.05219959533911058130, 116.2489096053143669 ) ) ;
#74423=CARTESIAN_POINT ( 'NONE',  ( 8.314922557960818139, 14.29746914071049879, 34.58224293864770260 ) ) ;
#74424=CARTESIAN_POINT ( 'NONE',  ( -13.89961937509977652, 13.97604488694528158, 100.6239096053143669 ) ) ;
#74425=CARTESIAN_POINT ( 'NONE',  ( -9.564922557960796823, -16.46253265017161027, 97.08224293864769550 ) ) ;
#74426=CARTESIAN_POINT ( 'NONE',  ( 0.05219959533907565091, 21.53943276465977519, 29.99890960531435979 ) ) ;
#74427=CARTESIAN_POINT ( 'NONE',  ( -16.52544592524342804, 4.483927247898546575, 71.04057627198103830 ) ) ;
#74428=CARTESIAN_POINT ( 'NONE',  ( 16.55341960407611168, 4.379528057220329451, 53.95724293864770260 ) ) ;
#74429=CARTESIAN_POINT ( 'NONE',  ( -16.53943276465976808, -0.05219959533934237506, 58.75109039468568994 ) ) ;
#74431=CARTESIAN_POINT ( 'NONE',  ( 16.51473224551083163, -9.474510206698727899, 50.83442372801899722 ) ) ;
#74432=CARTESIAN_POINT ( 'NONE',  ( 5.153800228976335163, 19.02544592524342804, 89.79057627198102409 ) ) ;
#74433=CARTESIAN_POINT ( 'NONE',  ( 5.049401038297881783, 19.05341960407617563, 72.29275706135234714 ) ) ;
#74435=CARTESIAN_POINT ( 'NONE',  ( 16.46253265017146816, 9.564922557961045513, 56.66775706135233293 ) ) ;
#74436=CARTESIAN_POINT ( 'NONE',  ( 19.02544592524334988, 5.153800228976608722, 111.4594237280190043 ) ) ;
#74437=CARTESIAN_POINT ( 'NONE',  ( 4.483927247898790824, -16.52544592524335698, 90.20942372801903275 ) ) ;
#74439=CARTESIAN_POINT ( 'NONE',  ( -13.97604488694527625, -13.89961937509977652, 41.87390960531435979 ) ) ;
#74440=CARTESIAN_POINT ( 'NONE',  ( -9.564922557960796823, -16.46253265017161027, 112.0822429386476955 ) ) ;
#74441=CARTESIAN_POINT ( 'NONE',  ( -18.62759615963255300, -10.81492255796106328, 59.16775706135234714 ) ) ;
#74442=CARTESIAN_POINT ( 'NONE',  ( -9.564922557961040184, 16.46253265017147172, 97.91775706135233293 ) ) ;
#74444=CARTESIAN_POINT ( 'NONE',  ( -19.02544592524342804, 5.153800228976336051, 61.04057627198103120 ) ) ;
#74446=CARTESIAN_POINT ( 'NONE',  ( -16.46253265017160317, 9.564922557960807481, 110.8322429386476955 ) ) ;
#74447=CARTESIAN_POINT ( 'NONE',  ( -8.224510206698948167, 14.34966873604960824, 80.41557627198103830 ) ) ;
#74448=CARTESIAN_POINT ( 'NONE',  ( 13.97604488694527802, 13.89961937509977652, 64.37390960531436690 ) ) ;
#74449=CARTESIAN_POINT ( 'NONE',  ( -9.564922557960796823, -16.46253265017161027, 72.08224293864770971 ) ) ;
#74450=CARTESIAN_POINT ( 'NONE',  ( 9.474510206698729675, 16.51473224551082808, 72.08442372801900433 ) ) ;
#74451=CARTESIAN_POINT ( 'NONE',  ( -15.80617190586745835, -15.72974639402198527, 61.87390960531436690 ) ) ;
#74452=CARTESIAN_POINT ( 'NONE',  ( 0.05219959533910956823, 16.53943276465976808, 109.9989096053143527 ) ) ;
#74453=CARTESIAN_POINT ( 'NONE',  ( 19.05341960407617918, -5.049401038297876454, 56.04275706135234714 ) ) ;
#74454=CARTESIAN_POINT ( 'NONE',  ( 5.049401038298161559, -19.05341960407611168, 62.70724293864769550 ) ) ;
#74455=CARTESIAN_POINT ( 'NONE',  ( 9.564922557960805705, 16.46253265017160317, 89.58224293864769550 ) ) ;
#74456=CARTESIAN_POINT ( 'NONE',  ( 5.719274019375991003, -21.55341960407610458, 92.70724293864770971 ) ) ;
#74457=CARTESIAN_POINT ( 'NONE',  ( 16.52544592524342804, -4.483927247898539470, 83.54057627198102409 ) ) ;
#74458=CARTESIAN_POINT ( 'NONE',  ( 13.89961937509957401, 13.97604488694547697, 51.87609039468566863 ) ) ;
#74459=CARTESIAN_POINT ( 'NONE',  ( -10.81492255796078084, -18.62759615963271287, 82.08224293864768129 ) ) ;
#74460=CARTESIAN_POINT ( 'NONE',  ( -21.55341960407610458, -5.719274019375992779, 56.45724293864768839 ) ) ;
#74461=CARTESIAN_POINT ( 'NONE',  ( 14.34966873604960469, 8.224510206698951720, 39.16557627198102409 ) ) ;
#74462=CARTESIAN_POINT ( 'NONE',  ( 21.55341960407619695, -5.719274019375665929, 91.04275706135236135 ) ) ;
#74463=CARTESIAN_POINT ( 'NONE',  ( -16.46253265017160317, 9.564922557960807481, 85.83224293864769550 ) ) ;
#74464=CARTESIAN_POINT ( 'NONE',  ( -19.05341960407611168, -5.049401038298163336, 21.45724293864768839 ) ) ;
#74466=CARTESIAN_POINT ( 'NONE',  ( -15.72974639402176322, -15.80617190586768395, 29.37609039468568284 ) ) ;
#74467=CARTESIAN_POINT ( 'NONE',  ( -15.72974639402176322, -15.80617190586768395, 34.37609039468568284 ) ) ;
#74468=CARTESIAN_POINT ( 'NONE',  ( -19.03943276465977164, 0.05219959533909376836, 51.24890960531436690 ) ) ;
#74469=CARTESIAN_POINT ( 'NONE',  ( 21.52544592524334988, 5.823673210054432836, 26.45942372801901854 ) ) ;
#74470=CARTESIAN_POINT ( 'NONE',  ( -13.89961937509957401, -13.97604488694547875, 64.37609039468567573 ) ) ;
#74472=CARTESIAN_POINT ( 'NONE',  ( -19.03943276465977164, 0.05219959533909376836, 41.24890960531435269 ) ) ;
#74473=CARTESIAN_POINT ( 'NONE',  ( 4.379528057220092307, 16.55341960407617563, 22.29275706135235069 ) ) ;
#74474=CARTESIAN_POINT ( 'NONE',  ( -19.05341960407611168, -5.049401038298163336, 31.45724293864769550 ) ) ;
#74475=CARTESIAN_POINT ( 'NONE',  ( 12.14591786802327356, -12.06949235617739191, 70.62609039468567573 ) ) ;
#74476=CARTESIAN_POINT ( 'NONE',  ( -19.02544592524342804, 5.153800228976336051, 41.04057627198103120 ) ) ;
#74478=CARTESIAN_POINT ( 'NONE',  ( 19.03943276465977164, -0.05219959533909143690, 88.74890960531436690 ) ) ;
#74479=CARTESIAN_POINT ( 'NONE',  ( -12.06949235617756955, 12.14591786802309770, 115.6239096053143669 ) ) ;
#74480=CARTESIAN_POINT ( 'NONE',  ( -15.80617190586745835, -15.72974639402198527, 61.87390960531436690 ) ) ;
#74481=CARTESIAN_POINT ( 'NONE',  ( -16.52544592524335698, -4.483927247898792601, 53.95942372801900433 ) ) ;
#74482=CARTESIAN_POINT ( 'NONE',  ( 5.823673210054444382, -21.52544592524334988, 100.2094237280190043 ) ) ;
#74483=CARTESIAN_POINT ( 'NONE',  ( 0.05219959533909260263, 19.03943276465977164, 39.99890960531436690 ) ) ;
#74484=CARTESIAN_POINT ( 'NONE',  ( -8.224510206698948167, 14.34966873604960824, 35.41557627198102409 ) ) ;
#74485=CARTESIAN_POINT ( 'NONE',  ( 16.55341960407611168, 4.379528057220329451, 63.95724293864770260 ) ) ;
#74486=CARTESIAN_POINT ( 'NONE',  ( -19.02544592524342804, 5.153800228976336051, 71.04057627198099567 ) ) ;
#74487=CARTESIAN_POINT ( 'NONE',  ( -18.67979575497193778, 10.72451020669871902, 113.3344237280190328 ) ) ;
#74488=CARTESIAN_POINT ( 'NONE',  ( 18.62759615963255655, 10.81492255796105972, 26.66775706135235424 ) ) ;
#74489=CARTESIAN_POINT ( 'NONE',  ( -5.153800228976328057, -19.02544592524343514, 82.29057627198103830 ) ) ;
#74490=CARTESIAN_POINT ( 'NONE',  ( 5.823673210054444382, -21.52544592524334988, 90.20942372801903275 ) ) ;
#74491=CARTESIAN_POINT ( 'NONE',  ( 4.483927247898790824, -16.52544592524335698, 50.20942372801901854 ) ) ;
#74492=CARTESIAN_POINT ( 'NONE',  ( 14.34966873604972726, -8.224510206698740333, 35.83442372801901143 ) ) ;
#74493=CARTESIAN_POINT ( 'NONE',  ( -16.55341960407611168, -4.379528057220339221, 86.45724293864770971 ) ) ;
#74494=CARTESIAN_POINT ( 'NONE',  ( -21.55341960407619339, 5.719274019375674811, 98.54275706135234714 ) ) ;
#74495=CARTESIAN_POINT ( 'NONE',  ( -8.224510206698948167, 14.34966873604960824, 40.41557627198103120 ) ) ;
#74496=CARTESIAN_POINT ( 'NONE',  ( 13.89961937509977652, -13.97604488694527269, 28.12390960531435624 ) ) ;
#74497=CARTESIAN_POINT ( 'NONE',  ( -12.14591786802326823, 12.06949235617739902, 48.12609039468568284 ) ) ;
#74498=CARTESIAN_POINT ( 'NONE',  ( 4.379528057220339221, -16.55341960407611168, 57.70724293864770260 ) ) ;
#74499=CARTESIAN_POINT ( 'NONE',  ( 0.05219959533934541429, -16.53943276465976808, 95.00109039468568994 ) ) ;
#74500=CARTESIAN_POINT ( 'NONE',  ( 21.52544592524344225, -5.823673210054117533, 23.54057627198102765 ) ) ;
#74501=CARTESIAN_POINT ( 'NONE',  ( 19.02544592524343514, -5.153800228976328945, 108.5405762719810383 ) ) ;
#74502=CARTESIAN_POINT ( 'NONE',  ( 0.05219959533937995610, -21.53943276465977519, 110.0010903946856757 ) ) ;
#74503=CARTESIAN_POINT ( 'NONE',  ( -8.314922557960811034, -14.29746914071050412, 92.08224293864769550 ) ) ;
#74504=CARTESIAN_POINT ( 'NONE',  ( 9.564922557960805705, 16.46253265017160317, 94.58224293864769550 ) ) ;
#74506=CARTESIAN_POINT ( 'NONE',  ( 12.14591786802327356, -12.06949235617739191, 35.62609039468568994 ) ) ;
#74507=CARTESIAN_POINT ( 'NONE',  ( -9.564922557960796823, -16.46253265017161027, 47.08224293864769550 ) ) ;
#74508=CARTESIAN_POINT ( 'NONE',  ( 8.314922557961029526, -14.29746914071037800, 50.41775706135235424 ) ) ;
#74510=CARTESIAN_POINT ( 'NONE',  ( -19.03943276465977164, -0.05219959533935918106, 43.75109039468566863 ) ) ;
#74511=CARTESIAN_POINT ( 'NONE',  ( 9.474510206698971260, -16.51473224551069308, 42.91557627198103120 ) ) ;
#74512=CARTESIAN_POINT ( 'NONE',  ( 0.05219959533934541429, -16.53943276465976808, 85.00109039468568994 ) ) ;
#74513=CARTESIAN_POINT ( 'NONE',  ( -16.46253265017146816, -9.564922557961047289, 79.16775706135234714 ) ) ;
#74514=CARTESIAN_POINT ( 'NONE',  ( -19.05341960407617563, 5.049401038297882671, 28.54275706135232937 ) ) ;
#74515=CARTESIAN_POINT ( 'NONE',  ( -9.474510206698964154, 16.51473224551069663, 65.41557627198102409 ) ) ;
#74516=CARTESIAN_POINT ( 'NONE',  ( 14.34966873604960469, 8.224510206698951720, 104.1655762719810241 ) ) ;
#74518=CARTESIAN_POINT ( 'NONE',  ( -9.564922557961040184, 16.46253265017147172, 62.91775706135233293 ) ) ;
#74519=CARTESIAN_POINT ( 'NONE',  ( 21.55341960407610458, 5.719274019375980345, 63.95724293864770260 ) ) ;
#74520=CARTESIAN_POINT ( 'NONE',  ( 9.474510206698729675, 16.51473224551082808, 32.08442372801900433 ) ) ;
#74521=CARTESIAN_POINT ( 'NONE',  ( -5.049401038298153566, 19.05341960407611168, 105.2072429386476671 ) ) ;
#74522=CARTESIAN_POINT ( 'NONE',  ( -15.80617190586745835, -15.72974639402198527, 76.87390960531439532 ) ) ;
#74523=CARTESIAN_POINT ( 'NONE',  ( -16.79531203550646623, 7.028104445595604766, 83.74755011779558345 ) ) ;
#74524=CARTESIAN_POINT ( 'NONE',  ( -0.05219959533936034679, 19.03943276465977164, 107.5010903946856615 ) ) ;
#74525=CARTESIAN_POINT ( 'NONE',  ( -17.72560187377284180, -5.500000000000007105, 99.07814504131322053 ) ) ;
#74526=CARTESIAN_POINT ( 'NONE',  ( -16.53943276465976808, -0.05219959533934237506, 33.75109039468568284 ) ) ;
#74527=CARTESIAN_POINT ( 'NONE',  ( 13.89961937509977652, -13.97604488694527269, 28.12390960531435624 ) ) ;
#74528=CARTESIAN_POINT ( 'NONE',  ( -5.153800228976328057, -19.02544592524343514, 112.2905762719810099 ) ) ;
#74529=CARTESIAN_POINT ( 'NONE',  ( -18.67979575497178146, -10.72451020669898902, 86.66557627198102409 ) ) ;
#74530=CARTESIAN_POINT ( 'NONE',  ( -5.823673210054431948, 21.52544592524334988, 62.70942372801902565 ) ) ;
#74531=CARTESIAN_POINT ( 'NONE',  ( 9.474510206698729675, 16.51473224551082808, 112.0844237280190043 ) ) ;
#74532=CARTESIAN_POINT ( 'NONE',  ( -13.89961937509957401, -13.97604488694547875, 19.37609039468566507 ) ) ;
#74533=CARTESIAN_POINT ( 'NONE',  ( -16.55341960407617563, 4.379528057220093196, 103.5427570613523613 ) ) ;
#74534=CARTESIAN_POINT ( 'NONE',  ( -21.53943276465977519, 0.05219959533907696930, 101.2489096053143669 ) ) ;
#74535=CARTESIAN_POINT ( 'NONE',  ( 16.55341960407611168, 4.379528057220329451, 53.95724293864770260 ) ) ;
#74536=CARTESIAN_POINT ( 'NONE',  ( -13.97604488694547697, 13.89961937509957934, 83.12609039468564731 ) ) ;
#74537=CARTESIAN_POINT ( 'NONE',  ( 13.97604488694548053, -13.89961937509957401, 55.62609039468566863 ) ) ;
#74538=CARTESIAN_POINT ( 'NONE',  ( 10.72451020669871369, 18.67979575497193778, 57.08442372801901854 ) ) ;
#74539=CARTESIAN_POINT ( 'NONE',  ( -13.89961937509957401, -13.97604488694547875, 34.37609039468566863 ) ) ;
#74540=CARTESIAN_POINT ( 'NONE',  ( -8.224510206698948167, 14.34966873604960824, 100.4155762719810241 ) ) ;
#74541=CARTESIAN_POINT ( 'NONE',  ( 5.719274019375991003, -21.55341960407610458, 47.70724293864770260 ) ) ;
#74542=CARTESIAN_POINT ( 'NONE',  ( 12.14591786802309770, 12.06949235617756955, 39.37390960531436690 ) ) ;
#74543=CARTESIAN_POINT ( 'NONE',  ( -5.823673210054431948, 21.52544592524334988, 102.7094237280190185 ) ) ;
#74544=CARTESIAN_POINT ( 'NONE',  ( 16.53943276465976808, 0.05219959533934440121, 66.25109039468567573 ) ) ;
#74545=CARTESIAN_POINT ( 'NONE',  ( -0.05219959533910754901, -16.53943276465976808, 32.49890960531435979 ) ) ;
#74546=CARTESIAN_POINT ( 'NONE',  ( -5.719274019375665041, -21.55341960407619695, 64.79275706135234714 ) ) ;
#74547=CARTESIAN_POINT ( 'NONE',  ( -10.81492255796105439, 18.62759615963255655, 62.91775706135236135 ) ) ;
#74548=CARTESIAN_POINT ( 'NONE',  ( 18.67979575497178502, 10.72451020669898547, 69.16557627198102409 ) ) ;
#74549=CARTESIAN_POINT ( 'NONE',  ( 21.52544592524334988, 5.823673210054432836, 46.45942372801901854 ) ) ;
#74550=CARTESIAN_POINT ( 'NONE',  ( 5.153800228976335163, 19.02544592524342804, 24.79057627198102765 ) ) ;
#74551=CARTESIAN_POINT ( 'NONE',  ( 13.89961937509977652, -13.97604488694527269, 38.12390960531436690 ) ) ;
#74552=CARTESIAN_POINT ( 'NONE',  ( -8.224510206698948167, 14.34966873604960824, 80.41557627198103830 ) ) ;
#74553=CARTESIAN_POINT ( 'NONE',  ( -19.05341960407611168, -5.049401038298163336, 91.45724293864766707 ) ) ;
#74554=CARTESIAN_POINT ( 'NONE',  ( -16.55341960407617563, 4.379528057220093196, 113.5427570613523756 ) ) ;
#74555=CARTESIAN_POINT ( 'NONE',  ( -0.05219959533910754901, -16.53943276465976808, 97.49890960531436690 ) ) ;
#74556=CARTESIAN_POINT ( 'NONE',  ( -21.55341960407610458, -5.719274019375992779, 71.45724293864769550 ) ) ;
#74557=CARTESIAN_POINT ( 'NONE',  ( -18.67979575497178146, -10.72451020669898902, 111.6655762719810525 ) ) ;
#74558=CARTESIAN_POINT ( 'NONE',  ( -16.51473224551069308, -9.474510206698971260, 111.6655762719810383 ) ) ;
#74559=CARTESIAN_POINT ( 'NONE',  ( 0.05219959533909260263, 19.03943276465977164, 69.99890960531435269 ) ) ;
#74560=CARTESIAN_POINT ( 'NONE',  ( 13.97604488694548053, -13.89961937509957401, 100.6260903946856615 ) ) ;
#74561=CARTESIAN_POINT ( 'NONE',  ( 21.52544592524344225, -5.823673210054117533, 58.54057627198103120 ) ) ;
#74562=CARTESIAN_POINT ( 'NONE',  ( -5.823673210054431948, 21.52544592524334988, 87.70942372801901854 ) ) ;
#74563=CARTESIAN_POINT ( 'NONE',  ( 5.153800228976335163, 19.02544592524342804, 64.79057627198100988 ) ) ;
#74564=CARTESIAN_POINT ( 'NONE',  ( 13.97604488694527802, 13.89961937509977652, 99.37390960531436690 ) ) ;
#74565=CARTESIAN_POINT ( 'NONE',  ( 8.224510206698742110, 14.34966873604972548, 72.08442372801899012 ) ) ;
#74566=CARTESIAN_POINT ( 'NONE',  ( 10.72451020669871369, 18.67979575497193778, 62.08442372801901143 ) ) ;
#74567=CARTESIAN_POINT ( 'NONE',  ( -21.52544592524334988, -5.823673210054445271, 93.95942372801903275 ) ) ;
#74568=CARTESIAN_POINT ( 'NONE',  ( 21.55341960407610458, 5.719274019375980345, 113.9572429386477239 ) ) ;
#74569=CARTESIAN_POINT ( 'NONE',  ( 15.80617190586746368, 15.72974639402197994, 84.37390960531438111 ) ) ;
#74570=CARTESIAN_POINT ( 'NONE',  ( 19.05341960407617918, -5.049401038297876454, 41.04275706135233293 ) ) ;
#74571=CARTESIAN_POINT ( 'NONE',  ( -21.52544592524343514, 5.823673210054127303, 36.04057627198102409 ) ) ;
#74572=CARTESIAN_POINT ( 'NONE',  ( 19.02544592524343514, -5.153800228976328945, 83.54057627198100988 ) ) ;
#74573=CARTESIAN_POINT ( 'NONE',  ( -14.29746914071049879, 8.314922557960819915, 35.83224293864768839 ) ) ;
#74574=CARTESIAN_POINT ( 'NONE',  ( -17.49999999999999645, 5.499999999999992895, 63.71769037696435589 ) ) ;
#74576=CARTESIAN_POINT ( 'NONE',  ( 13.89961937509957401, 13.97604488694547697, 96.87609039468566152 ) ) ;
#74577=CARTESIAN_POINT ( 'NONE',  ( -21.55341960407610458, -5.719274019375992779, 66.45724293864768129 ) ) ;
#74578=CARTESIAN_POINT ( 'NONE',  ( -12.06949235617756955, 12.14591786802309770, 50.62390960531435979 ) ) ;
#74579=CARTESIAN_POINT ( 'NONE',  ( 16.52544592524335698, 4.483927247898782831, 36.45942372801901143 ) ) ;
#74580=CARTESIAN_POINT ( 'NONE',  ( -19.02544592524342804, 5.153800228976336051, 51.04057627198103120 ) ) ;
#74581=CARTESIAN_POINT ( 'NONE',  ( 15.72974639402199770, -15.80617190586745480, 108.1239096053143811 ) ) ;
#74582=CARTESIAN_POINT ( 'NONE',  ( 5.153800228976615827, -19.02544592524334988, 85.20942372801900433 ) ) ;
#74583=CARTESIAN_POINT ( 'NONE',  ( -13.89961937509977652, 13.97604488694528158, 75.62390960531438111 ) ) ;
#74584=CARTESIAN_POINT ( 'NONE',  ( -4.483927247898539470, -16.52544592524342804, 92.29057627198103830 ) ) ;
#74585=CARTESIAN_POINT ( 'NONE',  ( 13.97604488694527802, 13.89961937509977652, 79.37390960531435269 ) ) ;
#74586=CARTESIAN_POINT ( 'NONE',  ( -5.719274019375978568, 21.55341960407610458, 80.20724293864769550 ) ) ;
#74587=CARTESIAN_POINT ( 'NONE',  ( 16.46253265017160672, -9.564922557960803928, 28.33224293864769550 ) ) ;
#74589=CARTESIAN_POINT ( 'NONE',  ( 12.14591786802309770, 12.06949235617756955, 59.37390960531436690 ) ) ;
#74590=CARTESIAN_POINT ( 'NONE',  ( 13.89961937509977652, -13.97604488694527269, 93.12390960531436690 ) ) ;
#74592=CARTESIAN_POINT ( 'NONE',  ( -13.89961937509957401, -13.97604488694547875, 49.37609039468567573 ) ) ;
#74593=CARTESIAN_POINT ( 'NONE',  ( 14.29746914071037800, 8.314922557961029526, 56.66775706135235424 ) ) ;
#74594=CARTESIAN_POINT ( 'NONE',  ( 5.823673210054125526, 21.52544592524343514, 74.79057627198105251 ) ) ;
#74595=CARTESIAN_POINT ( 'NONE',  ( 5.153800228976615827, -19.02544592524334988, 40.20942372801898301 ) ) ;
#74596=CARTESIAN_POINT ( 'NONE',  ( 5.153800228976335163, 19.02544592524342804, 84.79057627198099567 ) ) ;
#74598=CARTESIAN_POINT ( 'NONE',  ( -21.52544592524343514, 5.823673210054127303, 31.04057627198102409 ) ) ;
#74600=CARTESIAN_POINT ( 'NONE',  ( -5.153800228976328057, -19.02544592524343514, 72.29057627198102409 ) ) ;
#74601=CARTESIAN_POINT ( 'NONE',  ( 21.55341960407619695, -5.719274019375665929, 46.04275706135234714 ) ) ;
#74602=CARTESIAN_POINT ( 'NONE',  ( -14.29746914071049879, 8.314922557960819915, 115.8322429386477097 ) ) ;
#74603=CARTESIAN_POINT ( 'NONE',  ( -21.53943276465977519, -0.05219959533937600094, 18.75109039468568639 ) ) ;
#74604=CARTESIAN_POINT ( 'NONE',  ( 19.02544592524343514, -5.153800228976328945, 98.54057627198100988 ) ) ;
#74606=CARTESIAN_POINT ( 'NONE',  ( -18.62759615963255300, -10.81492255796106328, 34.16775706135234714 ) ) ;
#74608=CARTESIAN_POINT ( 'NONE',  ( -19.03943276465977164, 0.05219959533909376836, 106.2489096053143669 ) ) ;
#74611=CARTESIAN_POINT ( 'NONE',  ( 18.67979575497178502, 10.72451020669898547, 114.1655762719810383 ) ) ;
#74612=CARTESIAN_POINT ( 'NONE',  ( 13.97604488694527802, 13.89961937509977652, 49.37390960531434558 ) ) ;
#74613=CARTESIAN_POINT ( 'NONE',  ( -8.224510206698735004, -14.34966873604973081, 29.58442372801901854 ) ) ;
#74615=CARTESIAN_POINT ( 'NONE',  ( 15.72974639402176855, 15.80617190586768217, 101.8760903946857042 ) ) ;
#74616=CARTESIAN_POINT ( 'NONE',  ( 19.03943276465977164, -0.05219959533909143690, 48.74890960531435979 ) ) ;
#74617=CARTESIAN_POINT ( 'NONE',  ( -10.81492255796105439, 18.62759615963255655, 92.91775706135236135 ) ) ;
#74618=CARTESIAN_POINT ( 'NONE',  ( -13.89961937509977652, 13.97604488694528158, 95.62390960531436690 ) ) ;
#74619=CARTESIAN_POINT ( 'NONE',  ( -15.72974639402176322, -15.80617190586768395, 59.37609039468568284 ) ) ;
#74621=CARTESIAN_POINT ( 'NONE',  ( -16.46253265017160317, 9.564922557960807481, 95.83224293864769550 ) ) ;
#74622=CARTESIAN_POINT ( 'NONE',  ( -17.49999999999999289, 3.345213924137299788, 29.58768623094355732 ) ) ;
#74623=CARTESIAN_POINT ( 'NONE',  ( -0.05219959533934338120, 16.53943276465976808, 52.50109039468567573 ) ) ;
#74624=CARTESIAN_POINT ( 'NONE',  ( -4.483927247898782831, 16.52544592524335698, 62.70942372801902565 ) ) ;
#74625=CARTESIAN_POINT ( 'NONE',  ( 10.72451020669871369, 18.67979575497193778, 52.08442372801901854 ) ) ;
#74626=CARTESIAN_POINT ( 'NONE',  ( 10.72451020669871369, 18.67979575497193778, 92.08442372801901854 ) ) ;
#74628=CARTESIAN_POINT ( 'NONE',  ( -14.29746914071037622, -8.314922557961029526, 29.16775706135234003 ) ) ;
#74629=CARTESIAN_POINT ( 'NONE',  ( 13.97604488694527802, 13.89961937509977652, 79.37390960531435269 ) ) ;
#74630=CARTESIAN_POINT ( 'NONE',  ( 9.474510206698971260, -16.51473224551069308, 102.9155762719810241 ) ) ;
#74633=CARTESIAN_POINT ( 'NONE',  ( 13.89961937509977652, -13.97604488694527269, 23.12390960531436335 ) ) ;
#74634=CARTESIAN_POINT ( 'NONE',  ( -10.72451020669898014, 18.67979575497178502, 35.41557627198102409 ) ) ;
#74635=CARTESIAN_POINT ( 'NONE',  ( 8.224510206698742110, 14.34966873604972548, 97.08442372801904696 ) ) ;
#74636=CARTESIAN_POINT ( 'NONE',  ( 8.224510206698953496, -14.34966873604960469, 67.91557627198102409 ) ) ;
#74637=CARTESIAN_POINT ( 'NONE',  ( 19.02544592524343514, -5.153800228976328945, 68.54057627198103830 ) ) ;
#74638=CARTESIAN_POINT ( 'NONE',  ( 10.72451020669871369, 18.67979575497193778, 97.08442372801904696 ) ) ;
#74639=FACE_OUTER_BOUND ( 'NONE', #63649, .T. ) ;
#74640=CARTESIAN_POINT ( 'NONE',  ( 16.52544592524335698, 4.483927247898782831, 26.45942372801901854 ) ) ;
#74641=CARTESIAN_POINT ( 'NONE',  ( 8.314922557960818139, 14.29746914071049879, 79.58224293864769550 ) ) ;
#74642=CARTESIAN_POINT ( 'NONE',  ( 15.72974639402176855, 15.80617190586768217, 21.87609039468567573 ) ) ;
#74643=CARTESIAN_POINT ( 'NONE',  ( -0.05219959533907301413, -21.53943276465977519, 77.49890960531433848 ) ) ;
#74644=CARTESIAN_POINT ( 'NONE',  ( 5.049401038297881783, 19.05341960407617563, 37.29275706135232582 ) ) ;
#74646=CARTESIAN_POINT ( 'NONE',  ( 0.05219959533909260263, 19.03943276465977164, 84.99890960531436690 ) ) ;
#74647=CARTESIAN_POINT ( 'NONE',  ( 16.55341960407611168, 4.379528057220329451, 43.95724293864769550 ) ) ;
#74648=CARTESIAN_POINT ( 'NONE',  ( 4.379528057220339221, -16.55341960407611168, 37.70724293864769550 ) ) ;
#74649=CARTESIAN_POINT ( 'NONE',  ( 16.55341960407611168, 4.379528057220329451, 23.95724293864769550 ) ) ;
#74650=CARTESIAN_POINT ( 'NONE',  ( 19.05341960407617918, -5.049401038297876454, 61.04275706135232582 ) ) ;
#74651=CARTESIAN_POINT ( 'NONE',  ( 18.56101223717332616, 5.499999999999941380, 53.94978406935679516 ) ) ;
#74652=CARTESIAN_POINT ( 'NONE',  ( -19.02544592524342804, 5.153800228976336051, 101.0405762719810241 ) ) ;
#74653=CARTESIAN_POINT ( 'NONE',  ( 16.55341960407611168, 4.379528057220329451, 68.95724293864769550 ) ) ;
#74654=CARTESIAN_POINT ( 'NONE',  ( 19.17291183240699581, -5.500000000000061284, 38.15094504727040459 ) ) ;
#74655=CARTESIAN_POINT ( 'NONE',  ( -5.153800228976328057, -19.02544592524343514, 27.29057627198103120 ) ) ;
#74656=CARTESIAN_POINT ( 'NONE',  ( -18.67979575497178146, -10.72451020669898902, 41.66557627198103120 ) ) ;
#74657=CARTESIAN_POINT ( 'NONE',  ( -5.823673210054116645, -21.52544592524344225, 72.29057627198102409 ) ) ;
#74658=CARTESIAN_POINT ( 'NONE',  ( 4.483927247898545687, 16.52544592524342804, 109.7905762719810383 ) ) ;
#74659=CARTESIAN_POINT ( 'NONE',  ( -16.55341960407617563, 4.379528057220093196, 63.54275706135234003 ) ) ;
#74660=CARTESIAN_POINT ( 'NONE',  ( -16.46253265017160317, 9.564922557960807481, 40.83224293864769550 ) ) ;
#74661=CARTESIAN_POINT ( 'NONE',  ( 0.05219959533937995610, -21.53943276465977519, 60.00109039468568284 ) ) ;
#74663=CARTESIAN_POINT ( 'NONE',  ( 16.55341960407611168, 4.379528057220329451, 103.9572429386476813 ) ) ;
#74664=CARTESIAN_POINT ( 'NONE',  ( 17.05116617787826527, -6.768360034955669846, 36.15675553259198693 ) ) ;
#74666=CARTESIAN_POINT ( 'NONE',  ( -0.05219959533907301413, -21.53943276465977519, 37.49890960531436690 ) ) ;
#74668=CARTESIAN_POINT ( 'NONE',  ( -15.72974639402176322, -15.80617190586768395, 74.37609039468568994 ) ) ;
#74670=CARTESIAN_POINT ( 'NONE',  ( 16.52544592524335698, 4.483927247898782831, 61.45942372801901854 ) ) ;
#74671=CARTESIAN_POINT ( 'NONE',  ( 16.53943276465976808, -0.05219959533910856209, 38.74890960531435979 ) ) ;
#74672=CARTESIAN_POINT ( 'NONE',  ( -5.823673210054116645, -21.52544592524344225, 62.29057627198102409 ) ) ;
#74673=CARTESIAN_POINT ( 'NONE',  ( 21.55341960407610458, 5.719274019375980345, 58.95724293864770971 ) ) ;
#74675=CARTESIAN_POINT ( 'NONE',  ( -9.564922557961040184, 16.46253265017147172, 87.91775706135233293 ) ) ;
#74676=CARTESIAN_POINT ( 'NONE',  ( 0.05219959533907565091, 21.53943276465977519, 24.99890960531435624 ) ) ;
#74677=CARTESIAN_POINT ( 'NONE',  ( -19.03943276465977164, 0.05219959533909376836, 46.24890960531435979 ) ) ;
#74678=CARTESIAN_POINT ( 'NONE',  ( 19.03943276465977164, -0.05219959533909143690, 23.74890960531435269 ) ) ;
#74682=CARTESIAN_POINT ( 'NONE',  ( -16.52544592524335698, -4.483927247898792601, 68.95942372801901854 ) ) ;
#74683=CARTESIAN_POINT ( 'NONE',  ( 21.55341960407610458, 5.719274019375980345, 103.9572429386476813 ) ) ;
#74684=CARTESIAN_POINT ( 'NONE',  ( -13.97604488694527625, -13.89961937509977652, 61.87390960531435979 ) ) ;
#74685=CARTESIAN_POINT ( 'NONE',  ( -0.05219959533937732626, 21.53943276465977519, 37.50109039468568284 ) ) ;
#74686=CARTESIAN_POINT ( 'NONE',  ( -0.05219959533909027116, -19.03943276465977164, 97.49890960531436690 ) ) ;
#74688=ORIENTED_EDGE ( 'NONE', *, *, #67133, .F. ) ;
#74689=CARTESIAN_POINT ( 'NONE',  ( 15.80617190586769283, -15.72974639402175789, 30.62609039468567929 ) ) ;
#74690=CARTESIAN_POINT ( 'NONE',  ( -19.05341960407611168, -5.049401038298163336, 106.4572429386476955 ) ) ;
#74691=CARTESIAN_POINT ( 'NONE',  ( 16.51473224551083163, -9.474510206698727899, 85.83442372801900433 ) ) ;
#74692=EDGE_CURVE ( 'NONE', #8743, #92102, #137705, .T. ) ;
#74693=CARTESIAN_POINT ( 'NONE',  ( -13.97604488694547697, 13.89961937509957934, 43.12609039468566152 ) ) ;
#74694=CARTESIAN_POINT ( 'NONE',  ( 15.80617190586746368, 15.72974639402197994, 94.37390960531436690 ) ) ;
#74695=CARTESIAN_POINT ( 'NONE',  ( 19.03943276465977164, 0.05219959533936151252, 36.25109039468567573 ) ) ;
#74696=CARTESIAN_POINT ( 'NONE',  ( 5.153800228976615827, -19.02544592524334988, 50.20942372801897591 ) ) ;
#74697=CARTESIAN_POINT ( 'NONE',  ( -0.05219959533934338120, 16.53943276465976808, 97.50109039468567573 ) ) ;
#74699=VERTEX_POINT ( 'NONE', #8201 ) ;
#74700=CARTESIAN_POINT ( 'NONE',  ( -19.05341960407611168, -5.049401038298163336, 66.45724293864769550 ) ) ;
#74701=CARTESIAN_POINT ( 'NONE',  ( -21.55341960407619339, 5.719274019375674811, 83.54275706135234714 ) ) ;
#74702=CARTESIAN_POINT ( 'NONE',  ( 10.81492255796106328, -18.62759615963255655, 75.41775706135233293 ) ) ;
#74704=CARTESIAN_POINT ( 'NONE',  ( 9.474510206698971260, -16.51473224551069308, 87.91557627198102409 ) ) ;
#74705=CARTESIAN_POINT ( 'NONE',  ( 15.80617190586769283, -15.72974639402175789, 55.62609039468568284 ) ) ;
#74706=CARTESIAN_POINT ( 'NONE',  ( 0.05219959533936267826, -19.03943276465977164, 100.0010903946856757 ) ) ;
#74708=CARTESIAN_POINT ( 'NONE',  ( -5.153800228976328057, -19.02544592524343514, 67.29057627198102409 ) ) ;
#74709=CARTESIAN_POINT ( 'NONE',  ( -13.97604488694527625, -13.89961937509977652, 106.8739096053143669 ) ) ;
#74710=CARTESIAN_POINT ( 'NONE',  ( 5.153800228976335163, 19.02544592524342804, 84.79057627198099567 ) ) ;
#74711=CARTESIAN_POINT ( 'NONE',  ( 17.50000000000000000, -3.456093896842488800, 22.00000000000000711 ) ) ;
#74712=CARTESIAN_POINT ( 'NONE',  ( -16.46253265017160317, 9.564922557960807481, 60.83224293864769550 ) ) ;
#74713=CARTESIAN_POINT ( 'NONE',  ( -16.46253265017160317, 9.564922557960807481, 55.83224293864769550 ) ) ;
#74714=CARTESIAN_POINT ( 'NONE',  ( -5.719274019375978568, 21.55341960407610458, 95.20724293864769550 ) ) ;
#74715=CARTESIAN_POINT ( 'NONE',  ( -16.52544592524335698, -4.483927247898792601, 88.95942372801901854 ) ) ;
#74716=FACE_OUTER_BOUND ( 'NONE', #182787, .T. ) ;
#74717=CARTESIAN_POINT ( 'NONE',  ( -9.474510206698720793, -16.51473224551083518, 44.58442372801900433 ) ) ;
#74718=CARTESIAN_POINT ( 'NONE',  ( -19.05341960407611168, -5.049401038298163336, 76.45724293864769550 ) ) ;
#74719=CARTESIAN_POINT ( 'NONE',  ( 16.53943276465976808, -0.05219959533910856209, 68.74890960531435269 ) ) ;
#74720=CARTESIAN_POINT ( 'NONE',  ( 8.314922557960818139, 14.29746914071049879, 114.5822429386477097 ) ) ;
#74721=CARTESIAN_POINT ( 'NONE',  ( -5.823673210054116645, -21.52544592524344225, 22.29057627198102765 ) ) ;
#74722=CARTESIAN_POINT ( 'NONE',  ( -19.03943276465977164, 0.05219959533909376836, 101.2489096053143669 ) ) ;
#74723=CARTESIAN_POINT ( 'NONE',  ( -4.379528057220328563, 16.55341960407611168, 85.20724293864770971 ) ) ;
#74724=CARTESIAN_POINT ( 'NONE',  ( 13.89961937509957401, 13.97604488694547697, 26.87609039468566507 ) ) ;
#74725=CARTESIAN_POINT ( 'NONE',  ( 16.53943276465976808, 0.05219959533934440121, 91.25109039468568994 ) ) ;
#74726=CARTESIAN_POINT ( 'NONE',  ( 5.153800228976335163, 19.02544592524342804, 79.79057627198102409 ) ) ;
#74727=CARTESIAN_POINT ( 'NONE',  ( -21.53943276465977519, -0.05219959533937600094, 53.75109039468568994 ) ) ;
#74728=CARTESIAN_POINT ( 'NONE',  ( 18.62759615963271287, -10.81492255796078972, 48.33224293864770260 ) ) ;
#74729=CARTESIAN_POINT ( 'NONE',  ( -0.05219959533937732626, 21.53943276465977519, 22.50109039468567573 ) ) ;
#74730=CARTESIAN_POINT ( 'NONE',  ( -18.62759615963270932, 10.81492255796079327, 70.83224293864770971 ) ) ;
#74731=CARTESIAN_POINT ( 'NONE',  ( 8.224510206698953496, -14.34966873604960469, 92.91557627198103830 ) ) ;
#74732=CARTESIAN_POINT ( 'NONE',  ( 0.05219959533936267826, -19.03943276465977164, 55.00109039468566863 ) ) ;
#74733=CARTESIAN_POINT ( 'NONE',  ( 13.89961937509977652, -13.97604488694527269, 38.12390960531436690 ) ) ;
#74734=( BOUNDED_CURVE ( )  B_SPLINE_CURVE ( 2, ( #157118, #21585, #83243, #66089, #125780, #187482, #189456, #48949, #50934, #172284, #18614, #80261, #8423 ),
 .UNSPECIFIED., .F., .T. ) 
 B_SPLINE_CURVE_WITH_KNOTS ( ( 3, 2, 2, 2, 2, 2, 3 ),
 ( 0.5287462259007293941, 0.5307017543859648967, 0.5350877192982456121, 0.5394736842105263275, 0.5438596491228070429, 0.5482456140350877583, 0.5501554626982332330 ),
 .UNSPECIFIED. ) 
 CURVE ( )  GEOMETRIC_REPRESENTATION_ITEM ( )  RATIONAL_B_SPLINE_CURVE ( ( 0.9831626618144007068, 0.9848076720550096308, 1.000000000000000000, 0.9659258262890683122, 1.000000000000000000, 0.9659258262890683122, 1.000000000000000000, 0.9659258262890683122, 1.000000000000000000, 0.9659258262890683122, 1.000000000000000000, 0.9851625545550091179, 0.9832469066685282089 ) ) 
 REPRESENTATION_ITEM ( '' )  );
#74735=CARTESIAN_POINT ( 'NONE',  ( -9.564922557960796823, -16.46253265017161027, 87.08224293864769550 ) ) ;
#74736=CARTESIAN_POINT ( 'NONE',  ( 16.46253265017160672, -9.564922557960803928, 88.33224293864769550 ) ) ;
#74737=CARTESIAN_POINT ( 'NONE',  ( -16.52544592524342804, 4.483927247898546575, 96.04057627198102409 ) ) ;
#74738=CARTESIAN_POINT ( 'NONE',  ( 16.55341960407611168, 4.379528057220329451, 28.95724293864769905 ) ) ;
#74739=CARTESIAN_POINT ( 'NONE',  ( -4.483927247898782831, 16.52544592524335698, 32.70942372801900433 ) ) ;
#74740=CARTESIAN_POINT ( 'NONE',  ( -18.62759615963255300, -10.81492255796106328, 89.16775706135236135 ) ) ;
#74741=CARTESIAN_POINT ( 'NONE',  ( 19.03943276465977164, -0.05219959533909143690, 103.7489096053143669 ) ) ;
#74742=CARTESIAN_POINT ( 'NONE',  ( 10.72451020669871369, 18.67979575497193778, 22.08442372801901143 ) ) ;
#74743=CARTESIAN_POINT ( 'NONE',  ( -13.97604488694527625, -13.89961937509977652, 41.87390960531435979 ) ) ;
#74744=CARTESIAN_POINT ( 'NONE',  ( 8.314922557961029526, -14.29746914071037800, 50.41775706135235424 ) ) ;
#74745=CARTESIAN_POINT ( 'NONE',  ( 16.46253265017146816, 9.564922557961045513, 101.6677570613523329 ) ) ;
#74746=CARTESIAN_POINT ( 'NONE',  ( 9.474510206698971260, -16.51473224551069308, 37.91557627198102409 ) ) ;
#74747=CARTESIAN_POINT ( 'NONE',  ( 14.29746914071049879, -8.314922557960816363, 98.33224293864769550 ) ) ;
#74748=CARTESIAN_POINT ( 'NONE',  ( -10.72451020669898014, 18.67979575497178502, 110.4155762719810383 ) ) ;
#74749=CARTESIAN_POINT ( 'NONE',  ( 16.46253265017146816, 9.564922557961045513, 81.66775706135233293 ) ) ;
#74750=CARTESIAN_POINT ( 'NONE',  ( -16.51473224551069308, -9.474510206698971260, 21.66557627198102765 ) ) ;
#74751=CARTESIAN_POINT ( 'NONE',  ( -9.474510206698964154, 16.51473224551069663, 85.41557627198102409 ) ) ;
#74752=CARTESIAN_POINT ( 'NONE',  ( 5.719274019375991003, -21.55341960407610458, 112.7072429386476955 ) ) ;
#74753=CARTESIAN_POINT ( 'NONE',  ( -13.89961937509977652, 13.97604488694528158, 25.62390960531434558 ) ) ;
#74754=CARTESIAN_POINT ( 'NONE',  ( -16.51473224551069308, -9.474510206698971260, 86.66557627198102409 ) ) ;
#74755=CARTESIAN_POINT ( 'NONE',  ( 16.21995358207305671, -7.366697692864175195, 112.4355100151216504 ) ) ;
#74757=CARTESIAN_POINT ( 'NONE',  ( 19.03943276465977164, -0.05219959533909143690, 83.74890960531436690 ) ) ;
#74758=CARTESIAN_POINT ( 'NONE',  ( -5.823673210054431948, 21.52544592524334988, 37.70942372801900433 ) ) ;
#74759=CARTESIAN_POINT ( 'NONE',  ( -4.379528057220328563, 16.55341960407611168, 75.20724293864769550 ) ) ;
#74760=CARTESIAN_POINT ( 'NONE',  ( -19.02544592524342804, 5.153800228976336051, 101.0405762719810241 ) ) ;
#74761=CARTESIAN_POINT ( 'NONE',  ( 9.474510206698729675, 16.51473224551082808, 27.08442372801900433 ) ) ;
#74762=CARTESIAN_POINT ( 'NONE',  ( 0.05219959533934541429, -16.53943276465976808, 45.00109039468568284 ) ) ;
#74763=CARTESIAN_POINT ( 'NONE',  ( 18.62759615963255655, 10.81492255796105972, 61.66775706135235424 ) ) ;
#74764=CARTESIAN_POINT ( 'NONE',  ( 14.29746914071037800, 8.314922557961029526, 31.66775706135234358 ) ) ;
#74765=CARTESIAN_POINT ( 'NONE',  ( 16.51473224551069308, 9.474510206698969483, 69.16557627198102409 ) ) ;
#74766=CARTESIAN_POINT ( 'NONE',  ( -13.89961937509957401, -13.97604488694547875, 99.37609039468567573 ) ) ;
#74767=CARTESIAN_POINT ( 'NONE',  ( 16.52544592524335698, 4.483927247898782831, 66.45942372801903275 ) ) ;
#74768=CARTESIAN_POINT ( 'NONE',  ( 10.81492255796106328, -18.62759615963255655, 105.4177570613523613 ) ) ;
#74769=CARTESIAN_POINT ( 'NONE',  ( 19.03943276465977164, 0.05219959533936151252, 81.25109039468567573 ) ) ;
#74770=CARTESIAN_POINT ( 'NONE',  ( 16.46253265017160672, -9.564922557960803928, 53.33224293864768839 ) ) ;
#74771=CARTESIAN_POINT ( 'NONE',  ( 15.80617190586746368, 15.72974639402197994, 84.37390960531438111 ) ) ;
#74772=CARTESIAN_POINT ( 'NONE',  ( 14.34966873604960469, 8.224510206698951720, 74.16557627198102409 ) ) ;
#74773=CARTESIAN_POINT ( 'NONE',  ( -9.564922557961040184, 16.46253265017147172, 72.91775706135233293 ) ) ;
#74775=CARTESIAN_POINT ( 'NONE',  ( -13.89961937509957401, -13.97604488694547875, 59.37609039468566863 ) ) ;
#74776=CARTESIAN_POINT ( 'NONE',  ( -16.53943276465976808, 0.05219959533911058130, 21.24890960531436690 ) ) ;
#74777=CARTESIAN_POINT ( 'NONE',  ( 16.53943276465976808, -0.05219959533910856209, 63.74890960531435979 ) ) ;
#74778=CARTESIAN_POINT ( 'NONE',  ( -5.719274019375665041, -21.55341960407619695, 104.7927570613523898 ) ) ;
#74780=CARTESIAN_POINT ( 'NONE',  ( -10.81492255796078084, -18.62759615963271287, 102.0822429386476955 ) ) ;
#74781=CARTESIAN_POINT ( 'NONE',  ( -16.46253265017160317, 9.564922557960807481, 60.83224293864769550 ) ) ;
#74782=CARTESIAN_POINT ( 'NONE',  ( -10.81492255796105439, 18.62759615963255655, 82.91775706135234714 ) ) ;
#74783=CARTESIAN_POINT ( 'NONE',  ( -19.02544592524342804, 5.153800228976336051, 66.04057627198103830 ) ) ;
#74784=CARTESIAN_POINT ( 'NONE',  ( -19.05341960407611168, -5.049401038298163336, 21.45724293864768839 ) ) ;
#74785=CARTESIAN_POINT ( 'NONE',  ( 21.55341960407610458, 5.719274019375980345, 33.95724293864769550 ) ) ;
#74786=CARTESIAN_POINT ( 'NONE',  ( -4.483927247898539470, -16.52544592524342804, 67.29057627198103830 ) ) ;
#74787=CARTESIAN_POINT ( 'NONE',  ( 5.153800228976335163, 19.02544592524342804, 39.79057627198100988 ) ) ;
#74788=CARTESIAN_POINT ( 'NONE',  ( -16.55341960407611168, -4.379528057220339221, 96.45724293864770971 ) ) ;
#74789=CARTESIAN_POINT ( 'NONE',  ( 21.52544592524344225, -5.823673210054117533, 108.5405762719810241 ) ) ;
#74790=CARTESIAN_POINT ( 'NONE',  ( -10.81492255796105439, 18.62759615963255655, 47.91775706135234714 ) ) ;
#74791=CARTESIAN_POINT ( 'NONE',  ( 0.05219959533909260263, 19.03943276465977164, 34.99890960531435979 ) ) ;
#74792=CARTESIAN_POINT ( 'NONE',  ( -4.379528057220086978, -16.55341960407618274, 69.79275706135234714 ) ) ;
#74793=CARTESIAN_POINT ( 'NONE',  ( -5.823673210054116645, -21.52544592524344225, 107.2905762719810525 ) ) ;
#74794=CARTESIAN_POINT ( 'NONE',  ( 18.62759615963271287, -10.81492255796078972, 103.3322429386476955 ) ) ;
#74795=CARTESIAN_POINT ( 'NONE',  ( 16.46253265017146816, 9.564922557961045513, 26.66775706135234003 ) ) ;
#74796=CARTESIAN_POINT ( 'NONE',  ( -16.51473224551069308, -9.474510206698971260, 56.66557627198103120 ) ) ;
#74797=CARTESIAN_POINT ( 'NONE',  ( -17.97182807773870650, 5.500000000000046185, 83.53038844047284783 ) ) ;
#74798=CARTESIAN_POINT ( 'NONE',  ( -5.823673210054431948, 21.52544592524334988, 57.70942372801901143 ) ) ;
#74799=CARTESIAN_POINT ( 'NONE',  ( -18.62759615963270932, 10.81492255796079327, 50.83224293864770971 ) ) ;
#74800=CARTESIAN_POINT ( 'NONE',  ( -16.52544592524342804, 4.483927247898546575, 26.04057627198103475 ) ) ;
#74801=CARTESIAN_POINT ( 'NONE',  ( -18.62759615963255300, -10.81492255796106328, 79.16775706135234714 ) ) ;
#74802=CARTESIAN_POINT ( 'NONE',  ( -0.05219959533937732626, 21.53943276465977519, 97.50109039468567573 ) ) ;
#74803=CARTESIAN_POINT ( 'NONE',  ( -16.46253265017146816, -9.564922557961047289, 39.16775706135234003 ) ) ;
#74804=CARTESIAN_POINT ( 'NONE',  ( 4.379528057220092307, 16.55341960407617563, 107.2927570613523471 ) ) ;
#74805=CARTESIAN_POINT ( 'NONE',  ( 15.72974639402176855, 15.80617190586768217, 51.87609039468568284 ) ) ;
#74807=CARTESIAN_POINT ( 'NONE',  ( -9.564922557960796823, -16.46253265017161027, 62.08224293864769550 ) ) ;
#74808=CARTESIAN_POINT ( 'NONE',  ( -19.02544592524334988, -5.153800228976617603, 18.95942372801899722 ) ) ;
#74809=CARTESIAN_POINT ( 'NONE',  ( 21.55341960407610458, 5.719274019375980345, 33.95724293864769550 ) ) ;
#74810=CARTESIAN_POINT ( 'NONE',  ( 15.80617190586769283, -15.72974639402175789, 35.62609039468568994 ) ) ;
#74811=CARTESIAN_POINT ( 'NONE',  ( 10.81492255796078972, 18.62759615963270932, 84.58224293864769550 ) ) ;
#74812=CARTESIAN_POINT ( 'NONE',  ( 19.03943276465977164, 0.05219959533936151252, 91.25109039468566152 ) ) ;
#74813=CARTESIAN_POINT ( 'NONE',  ( -8.224510206698735004, -14.34966873604973081, 54.58442372801901143 ) ) ;
#74814=CARTESIAN_POINT ( 'NONE',  ( 17.50000000000000000, 5.500000000000013323, 63.78230962303565832 ) ) ;
#74815=CARTESIAN_POINT ( 'NONE',  ( -15.72974639402197994, 15.80617190586746368, 85.62390960531436690 ) ) ;
#74816=CARTESIAN_POINT ( 'NONE',  ( 16.55341960407618274, -4.379528057220086978, 71.04275706135234714 ) ) ;
#74817=CARTESIAN_POINT ( 'NONE',  ( -0.05219959533910754901, -16.53943276465976808, 72.49890960531435269 ) ) ;
#74819=CARTESIAN_POINT ( 'NONE',  ( 16.51473224551083163, -9.474510206698727899, 100.8344237280190043 ) ) ;
#74820=CARTESIAN_POINT ( 'NONE',  ( -10.81492255796078084, -18.62759615963271287, 37.08224293864768129 ) ) ;
#74823=CARTESIAN_POINT ( 'NONE',  ( 14.29746914071037800, 8.314922557961029526, 36.66775706135234714 ) ) ;
#74824=CARTESIAN_POINT ( 'NONE',  ( 18.62759615963271287, -10.81492255796078972, 108.3322429386477097 ) ) ;
#74825=CARTESIAN_POINT ( 'NONE',  ( -10.72451020669898014, 18.67979575497178502, 30.41557627198101699 ) ) ;
#74826=CARTESIAN_POINT ( 'NONE',  ( 16.53943276465976808, 0.05219959533934440121, 71.25109039468568994 ) ) ;
#74827=CARTESIAN_POINT ( 'NONE',  ( 9.474510206698971260, -16.51473224551069308, 87.91557627198102409 ) ) ;
#74828=CARTESIAN_POINT ( 'NONE',  ( -0.05219959533937732626, 21.53943276465977519, 62.50109039468568284 ) ) ;
#74829=CARTESIAN_POINT ( 'NONE',  ( -5.153800228976328057, -19.02544592524343514, 32.29057627198102409 ) ) ;
#74830=CARTESIAN_POINT ( 'NONE',  ( -15.80617190586745835, -15.72974639402198527, 21.87390960531436690 ) ) ;
#74831=CARTESIAN_POINT ( 'NONE',  ( 13.97604488694548053, -13.89961937509957401, 40.62609039468564731 ) ) ;
#74832=CARTESIAN_POINT ( 'NONE',  ( -12.14591786802326823, 12.06949235617739902, 53.12609039468568284 ) ) ;
#74833=CARTESIAN_POINT ( 'NONE',  ( -5.719274019375978568, 21.55341960407610458, 25.20724293864769550 ) ) ;
#74834=CARTESIAN_POINT ( 'NONE',  ( 19.05341960407611168, 5.049401038298154454, 73.95724293864768129 ) ) ;
#74835=CARTESIAN_POINT ( 'NONE',  ( 14.34966873604972726, -8.224510206698740333, 100.8344237280190185 ) ) ;
#74836=CARTESIAN_POINT ( 'NONE',  ( -4.483927247898539470, -16.52544592524342804, 92.29057627198103830 ) ) ;
#74837=CARTESIAN_POINT ( 'NONE',  ( -21.55341960407610458, -5.719274019375992779, 36.45724293864768839 ) ) ;
#74838=CARTESIAN_POINT ( 'NONE',  ( -5.049401038298153566, 19.05341960407611168, 30.20724293864768839 ) ) ;
#74839=CARTESIAN_POINT ( 'NONE',  ( -12.06949235617739369, -12.14591786802326823, 64.37609039468568994 ) ) ;
#74840=CARTESIAN_POINT ( 'NONE',  ( -15.72974639402176322, -15.80617190586768395, 19.37609039468568639 ) ) ;
#74841=CARTESIAN_POINT ( 'NONE',  ( -16.51473224551082808, 9.474510206698731452, 83.33442372801899012 ) ) ;
#74842=CARTESIAN_POINT ( 'NONE',  ( -19.03943276465977164, 0.05219959533909376836, 46.24890960531435979 ) ) ;
#74843=CARTESIAN_POINT ( 'NONE',  ( -5.823673210054116645, -21.52544592524344225, 67.29057627198103830 ) ) ;
#74844=CARTESIAN_POINT ( 'NONE',  ( 13.97604488694527802, 13.89961937509977652, 109.3739096053143669 ) ) ;
#74845=CARTESIAN_POINT ( 'NONE',  ( -5.719274019375665041, -21.55341960407619695, 94.79275706135234714 ) ) ;
#74846=CARTESIAN_POINT ( 'NONE',  ( -5.049401038298153566, 19.05341960407611168, 65.20724293864765286 ) ) ;
#74847=CARTESIAN_POINT ( 'NONE',  ( 14.29746914071037800, 8.314922557961029526, 51.66775706135234714 ) ) ;
#74848=CARTESIAN_POINT ( 'NONE',  ( -5.049401038298153566, 19.05341960407611168, 65.20724293864765286 ) ) ;
#74849=CARTESIAN_POINT ( 'NONE',  ( -21.55341960407619339, 5.719274019375674811, 83.54275706135234714 ) ) ;
#74850=CARTESIAN_POINT ( 'NONE',  ( -13.97604488694547697, 13.89961937509957934, 38.12609039468566152 ) ) ;
#74852=CARTESIAN_POINT ( 'NONE',  ( -16.46253265017146816, -9.564922557961047289, 59.16775706135233293 ) ) ;
#74854=CARTESIAN_POINT ( 'NONE',  ( 21.52544592524334988, 5.823673210054432836, 56.45942372801902565 ) ) ;
#74856=CARTESIAN_POINT ( 'NONE',  ( 16.46253265017146816, 9.564922557961045513, 51.66775706135233293 ) ) ;
#74857=CARTESIAN_POINT ( 'NONE',  ( 16.46253265017160672, -9.564922557960803928, 103.3322429386476955 ) ) ;
#74858=CARTESIAN_POINT ( 'NONE',  ( -19.02544592524342804, 5.153800228976336051, 76.04057627198102409 ) ) ;
#74859=CARTESIAN_POINT ( 'NONE',  ( -16.52544592524342804, 4.483927247898546575, 36.04057627198102409 ) ) ;
#74860=CARTESIAN_POINT ( 'NONE',  ( 18.62759615963271287, -10.81492255796078972, 33.33224293864769550 ) ) ;
#74863=CARTESIAN_POINT ( 'NONE',  ( 10.81492255796106328, -18.62759615963255655, 100.4177570613523471 ) ) ;
#74865=CARTESIAN_POINT ( 'NONE',  ( 13.89961937509977652, -13.97604488694527269, 33.12390960531434558 ) ) ;
#74866=CARTESIAN_POINT ( 'NONE',  ( -0.05219959533909027116, -19.03943276465977164, 112.4989096053143669 ) ) ;
#74868=CARTESIAN_POINT ( 'NONE',  ( 4.483927247898790824, -16.52544592524335698, 50.20942372801901854 ) ) ;
#74869=CARTESIAN_POINT ( 'NONE',  ( -10.81492255796078084, -18.62759615963271287, 72.08224293864769550 ) ) ;
#74870=CARTESIAN_POINT ( 'NONE',  ( -16.53943276465976808, 0.05219959533911058130, 46.24890960531435979 ) ) ;
#74871=CARTESIAN_POINT ( 'NONE',  ( -5.049401038298153566, 19.05341960407611168, 30.20724293864768839 ) ) ;
#74872=CARTESIAN_POINT ( 'NONE',  ( 16.46253265017160672, -9.564922557960803928, 103.3322429386476955 ) ) ;
#74873=CARTESIAN_POINT ( 'NONE',  ( 5.719274019375673035, 21.55341960407619339, 27.29275706135234358 ) ) ;
#74874=CARTESIAN_POINT ( 'NONE',  ( -9.474510206698720793, -16.51473224551083518, 39.58442372801899722 ) ) ;
#74875=CARTESIAN_POINT ( 'NONE',  ( -12.14591786802309592, -12.06949235617757132, 111.8739096053143669 ) ) ;
#74876=CARTESIAN_POINT ( 'NONE',  ( 10.81492255796106328, -18.62759615963255655, 75.41775706135233293 ) ) ;
#74877=CARTESIAN_POINT ( 'NONE',  ( 16.62475595723696031, -7.163666690055223718, 33.02713351810466236 ) ) ;
#74878=CARTESIAN_POINT ( 'NONE',  ( 12.14591786802309770, 12.06949235617756955, 34.37390960531435979 ) ) ;
#74879=CARTESIAN_POINT ( 'NONE',  ( 17.49999999999999645, 4.013004640162542991, 112.0539427900559417 ) ) ;
#74880=CARTESIAN_POINT ( 'NONE',  ( 21.52544592524344225, -5.823673210054117533, 28.54057627198103120 ) ) ;
#74881=CARTESIAN_POINT ( 'NONE',  ( 4.483927247898545687, 16.52544592524342804, 94.79057627198105251 ) ) ;
#74882=CARTESIAN_POINT ( 'NONE',  ( -17.49999999999999645, -5.500000000000000888, 39.20309617465829177 ) ) ;
#74883=CARTESIAN_POINT ( 'NONE',  ( -19.02544592524342804, 5.153800228976336051, 81.04057627198103830 ) ) ;
#74884=CARTESIAN_POINT ( 'NONE',  ( -12.14591786802309592, -12.06949235617757132, 76.87390960531439532 ) ) ;
#74885=CARTESIAN_POINT ( 'NONE',  ( 19.03943276465977164, 0.05219959533936151252, 101.2510903946856757 ) ) ;
#74886=CARTESIAN_POINT ( 'NONE',  ( 15.80617190586746368, 15.72974639402197994, 64.37390960531435269 ) ) ;
#74888=CARTESIAN_POINT ( 'NONE',  ( 19.03943276465977164, -0.05219959533909143690, 38.74890960531436690 ) ) ;
#74889=CARTESIAN_POINT ( 'NONE',  ( -5.153800228976328057, -19.02544592524343514, 77.29057627198099567 ) ) ;
#74890=CARTESIAN_POINT ( 'NONE',  ( 5.823673210054125526, 21.52544592524343514, 69.79057627198102409 ) ) ;
#74891=CARTESIAN_POINT ( 'NONE',  ( 16.52544592524335698, 4.483927247898782831, 106.4594237280190328 ) ) ;
#74892=CARTESIAN_POINT ( 'NONE',  ( 19.03943276465977164, -0.05219959533909143690, 83.74890960531436690 ) ) ;
#74893=CARTESIAN_POINT ( 'NONE',  ( -19.02544592524334988, -5.153800228976617603, 68.95942372801896170 ) ) ;
#74894=CARTESIAN_POINT ( 'NONE',  ( -15.72974639402176322, -15.80617190586768395, 94.37609039468568994 ) ) ;
#74895=CARTESIAN_POINT ( 'NONE',  ( -5.719274019375978568, 21.55341960407610458, 75.20724293864769550 ) ) ;
#74896=CARTESIAN_POINT ( 'NONE',  ( 15.80617190586746368, 15.72974639402197994, 24.37390960531435979 ) ) ;
#74897=CARTESIAN_POINT ( 'NONE',  ( -5.153800228976328057, -19.02544592524343514, 52.29057627198100988 ) ) ;
#74898=CARTESIAN_POINT ( 'NONE',  ( 0.05219959533934541429, -16.53943276465976808, 95.00109039468568994 ) ) ;
#74899=CARTESIAN_POINT ( 'NONE',  ( -5.049401038298153566, 19.05341960407611168, 65.20724293864765286 ) ) ;
#74901=CARTESIAN_POINT ( 'NONE',  ( 5.823673210054444382, -21.52544592524334988, 110.2094237280190185 ) ) ;
#74902=CARTESIAN_POINT ( 'NONE',  ( 14.29746914071049879, -8.314922557960816363, 73.33224293864769550 ) ) ;
#74903=CARTESIAN_POINT ( 'NONE',  ( 21.53943276465977519, -0.05219959533907433946, 103.7489096053143669 ) ) ;
#74904=CARTESIAN_POINT ( 'NONE',  ( -0.05219959533907301413, -21.53943276465977519, 102.4989096053143811 ) ) ;
#74906=CARTESIAN_POINT ( 'NONE',  ( 5.823673210054125526, 21.52544592524343514, 64.79057627198103830 ) ) ;
#74907=CARTESIAN_POINT ( 'NONE',  ( 16.55341960407618274, -4.379528057220086978, 81.04275706135236135 ) ) ;
#74908=CARTESIAN_POINT ( 'NONE',  ( -4.483927247898539470, -16.52544592524342804, 102.2905762719810383 ) ) ;
#74909=CARTESIAN_POINT ( 'NONE',  ( -5.049401038298153566, 19.05341960407611168, 60.20724293864768129 ) ) ;
#74911=CARTESIAN_POINT ( 'NONE',  ( -16.53943276465976808, -0.05219959533934237506, 113.7510903946856757 ) ) ;
#74912=CARTESIAN_POINT ( 'NONE',  ( 0.05219959533937995610, -21.53943276465977519, 50.00109039468568994 ) ) ;
#74913=CARTESIAN_POINT ( 'NONE',  ( -9.474510206698964154, 16.51473224551069663, 100.4155762719810241 ) ) ;
#74914=CARTESIAN_POINT ( 'NONE',  ( -5.823673210054431948, 21.52544592524334988, 77.70942372801900433 ) ) ;
#74915=CARTESIAN_POINT ( 'NONE',  ( 5.153800228976335163, 19.02544592524342804, 24.79057627198102765 ) ) ;
#74916=CARTESIAN_POINT ( 'NONE',  ( 9.564922557960805705, 16.46253265017160317, 34.58224293864770260 ) ) ;
#74917=ORIENTED_EDGE ( 'NONE', *, *, #79855, .T. ) ;
#74918=CARTESIAN_POINT ( 'NONE',  ( 18.62759615963255655, 10.81492255796105972, 76.66775706135234714 ) ) ;
#74919=CARTESIAN_POINT ( 'NONE',  ( -13.89961937509977652, 13.97604488694528158, 100.6239096053143669 ) ) ;
#74920=CARTESIAN_POINT ( 'NONE',  ( 9.564922557961047289, -16.46253265017146816, 85.41775706135233293 ) ) ;
#74921=CARTESIAN_POINT ( 'NONE',  ( 0.05219959533937995610, -21.53943276465977519, 45.00109039468568284 ) ) ;
#74922=CARTESIAN_POINT ( 'NONE',  ( 16.55341960407618274, -4.379528057220086978, 26.04275706135235779 ) ) ;
#74923=CARTESIAN_POINT ( 'NONE',  ( -19.02544592524334988, -5.153800228976617603, 68.95942372801896170 ) ) ;
#74924=CARTESIAN_POINT ( 'NONE',  ( 13.97604488694527802, 13.89961937509977652, 49.37390960531434558 ) ) ;
#74925=CARTESIAN_POINT ( 'NONE',  ( 0.05219959533936267826, -19.03943276465977164, 85.00109039468567573 ) ) ;
#74926=CARTESIAN_POINT ( 'NONE',  ( 14.34966873604960469, 8.224510206698951720, 29.16557627198103120 ) ) ;
#74927=CARTESIAN_POINT ( 'NONE',  ( -9.564922557961040184, 16.46253265017147172, 87.91775706135233293 ) ) ;
#74928=CARTESIAN_POINT ( 'NONE',  ( 14.29746914071049879, -8.314922557960816363, 38.33224293864768839 ) ) ;
#74929=CARTESIAN_POINT ( 'NONE',  ( 0.05219959533936267826, -19.03943276465977164, 70.00109039468566152 ) ) ;
#74930=CARTESIAN_POINT ( 'NONE',  ( 12.14591786802327356, -12.06949235617739191, 50.62609039468568994 ) ) ;
#74931=CARTESIAN_POINT ( 'NONE',  ( -19.03943276465977164, -0.05219959533935918106, 18.75109039468567218 ) ) ;
#74932=CARTESIAN_POINT ( 'NONE',  ( 19.02544592524343514, -5.153800228976328945, 38.54057627198103120 ) ) ;
#74933=CARTESIAN_POINT ( 'NONE',  ( -17.26058549869088310, -6.457015423128632747, 66.37745837476067834 ) ) ;
#74934=CARTESIAN_POINT ( 'NONE',  ( 16.55341960407618274, -4.379528057220086978, 51.04275706135234714 ) ) ;
#74937=CARTESIAN_POINT ( 'NONE',  ( -5.049401038298153566, 19.05341960407611168, 90.20724293864766707 ) ) ;
#74938=CARTESIAN_POINT ( 'NONE',  ( -15.49999999999999822, -5.500000000000000888, 118.0000000000000142 ) ) ;
#74940=CARTESIAN_POINT ( 'NONE',  ( 13.97604488694548053, -13.89961937509957401, 80.62609039468567573 ) ) ;
#74941=CARTESIAN_POINT ( 'NONE',  ( -18.62759615963270932, 10.81492255796079327, 25.83224293864769194 ) ) ;
#74942=CARTESIAN_POINT ( 'NONE',  ( -19.02544592524334988, -5.153800228976617603, 23.95942372801900078 ) ) ;
#74943=CARTESIAN_POINT ( 'NONE',  ( 19.05341960407617918, -5.049401038297876454, 101.0427570613523045 ) ) ;
#74944=CARTESIAN_POINT ( 'NONE',  ( -9.564922557960796823, -16.46253265017161027, 22.08224293864768839 ) ) ;
#74945=CARTESIAN_POINT ( 'NONE',  ( 5.049401038298161559, -19.05341960407611168, 32.70724293864768129 ) ) ;
#74946=CARTESIAN_POINT ( 'NONE',  ( -15.80617190586745835, -15.72974639402198527, 56.87390960531436690 ) ) ;
#74947=CARTESIAN_POINT ( 'NONE',  ( -12.06949235617756955, 12.14591786802309770, 115.6239096053143669 ) ) ;
#74948=CYLINDRICAL_SURFACE ( 'NONE', #30657, 2.500000000000002220 ) ;
#74949=CARTESIAN_POINT ( 'NONE',  ( 5.049401038297881783, 19.05341960407617563, 77.29275706135231871 ) ) ;
#74950=CARTESIAN_POINT ( 'NONE',  ( 14.34966873604960469, 8.224510206698951720, 44.16557627198103120 ) ) ;
#74951=CARTESIAN_POINT ( 'NONE',  ( 21.53943276465977519, -0.05219959533907433946, 28.74890960531435624 ) ) ;
#74952=CARTESIAN_POINT ( 'NONE',  ( 15.72974639402176855, 15.80617190586768217, 96.87609039468568994 ) ) ;
#74953=CARTESIAN_POINT ( 'NONE',  ( 18.62759615963271287, -10.81492255796078972, 88.33224293864769550 ) ) ;
#74954=CARTESIAN_POINT ( 'NONE',  ( -0.05219959533937732626, 21.53943276465977519, 52.50109039468567573 ) ) ;
#74955=CARTESIAN_POINT ( 'NONE',  ( 10.81492255796106328, -18.62759615963255655, 65.41775706135234714 ) ) ;
#74957=CARTESIAN_POINT ( 'NONE',  ( 19.02544592524343514, -5.153800228976328945, 93.54057627198102409 ) ) ;
#74958=CARTESIAN_POINT ( 'NONE',  ( -14.29746914071037622, -8.314922557961029526, 99.16775706135234714 ) ) ;
#74959=CARTESIAN_POINT ( 'NONE',  ( 15.80617190586769283, -15.72974639402175789, 55.62609039468568284 ) ) ;
#74960=CARTESIAN_POINT ( 'NONE',  ( 14.34966873604960469, 8.224510206698951720, 114.1655762719810383 ) ) ;
#74961=CARTESIAN_POINT ( 'NONE',  ( -16.55341960407611168, -4.379528057220339221, 61.45724293864770260 ) ) ;
#74962=CARTESIAN_POINT ( 'NONE',  ( 4.379528057220339221, -16.55341960407611168, 37.70724293864769550 ) ) ;
#74963=CARTESIAN_POINT ( 'NONE',  ( 10.81492255796078972, 18.62759615963270932, 44.58224293864769550 ) ) ;
#74964=CARTESIAN_POINT ( 'NONE',  ( 5.049401038298161559, -19.05341960407611168, 52.70724293864767418 ) ) ;
#74965=CARTESIAN_POINT ( 'NONE',  ( 18.62759615963271287, -10.81492255796078972, 58.33224293864768839 ) ) ;
#74966=CARTESIAN_POINT ( 'NONE',  ( 19.05341960407617918, -5.049401038297876454, 46.04275706135233293 ) ) ;
#74967=CARTESIAN_POINT ( 'NONE',  ( -16.62475595723695676, -7.163666690055263686, 39.47286648189535896 ) ) ;
#74968=CARTESIAN_POINT ( 'NONE',  ( -4.483927247898539470, -16.52544592524342804, 52.29057627198102409 ) ) ;
#74969=CARTESIAN_POINT ( 'NONE',  ( -15.80617190586745835, -15.72974639402198527, 21.87390960531436690 ) ) ;
#74973=CARTESIAN_POINT ( 'NONE',  ( -14.34966873604972548, 8.224510206698743886, 73.33442372801901854 ) ) ;
#74974=CARTESIAN_POINT ( 'NONE',  ( 13.97604488694548053, -13.89961937509957401, 80.62609039468567573 ) ) ;
#74975=CARTESIAN_POINT ( 'NONE',  ( -16.53943276465976808, 0.05219959533911058130, 36.24890960531435979 ) ) ;
#74977=CARTESIAN_POINT ( 'NONE',  ( -8.314922557960811034, -14.29746914071050412, 22.08224293864769194 ) ) ;
#74978=CARTESIAN_POINT ( 'NONE',  ( -19.03943276465977164, 0.05219959533909376836, 46.24890960531435979 ) ) ;
#74979=CARTESIAN_POINT ( 'NONE',  ( 0.05219959533909260263, 19.03943276465977164, 69.99890960531435269 ) ) ;
#74980=CARTESIAN_POINT ( 'NONE',  ( 19.03943276465977164, -0.05219959533909143690, 33.74890960531435979 ) ) ;
#74981=CARTESIAN_POINT ( 'NONE',  ( -18.67979575497193778, 10.72451020669871902, 48.33442372801902565 ) ) ;
#74982=CARTESIAN_POINT ( 'NONE',  ( 9.474510206698971260, -16.51473224551069308, 57.91557627198103120 ) ) ;
#74984=CARTESIAN_POINT ( 'NONE',  ( 9.564922557960805705, 16.46253265017160317, 59.58224293864769550 ) ) ;
#74985=CARTESIAN_POINT ( 'NONE',  ( 10.81492255796078972, 18.62759615963270932, 39.58224293864769550 ) ) ;
#74986=CARTESIAN_POINT ( 'NONE',  ( 19.02544592524343514, -5.153800228976328945, 33.54057627198102409 ) ) ;
#74987=CARTESIAN_POINT ( 'NONE',  ( -18.62759615963270932, 10.81492255796079327, 35.83224293864768839 ) ) ;
#74988=CARTESIAN_POINT ( 'NONE',  ( 4.379528057220092307, 16.55341960407617563, 87.29275706135236135 ) ) ;
#74989=CARTESIAN_POINT ( 'NONE',  ( 0.05219959533937995610, -21.53943276465977519, 100.0010903946857042 ) ) ;
#74990=CARTESIAN_POINT ( 'NONE',  ( -4.379528057220086978, -16.55341960407618274, 64.79275706135234714 ) ) ;
#74991=CARTESIAN_POINT ( 'NONE',  ( -16.46253265017160317, 9.564922557960807481, 105.8322429386476955 ) ) ;
#74992=CARTESIAN_POINT ( 'NONE',  ( 12.14591786802327356, -12.06949235617739191, 55.62609039468568284 ) ) ;
#74993=CARTESIAN_POINT ( 'NONE',  ( 16.52544592524335698, 4.483927247898782831, 36.45942372801901143 ) ) ;
#74994=CARTESIAN_POINT ( 'NONE',  ( 13.97604488694527802, 13.89961937509977652, 104.3739096053143385 ) ) ;
#74995=CARTESIAN_POINT ( 'NONE',  ( -16.52544592524335698, -4.483927247898792601, 28.95942372801902209 ) ) ;
#74996=CARTESIAN_POINT ( 'NONE',  ( 5.049401038298161559, -19.05341960407611168, 32.70724293864768129 ) ) ;
#74997=CARTESIAN_POINT ( 'NONE',  ( -10.72451020669870658, -18.67979575497194134, 24.58442372801901499 ) ) ;
#74998=CARTESIAN_POINT ( 'NONE',  ( 16.53943276465976808, 0.05219959533934440121, 21.25109039468567218 ) ) ;
#74999=CARTESIAN_POINT ( 'NONE',  ( 8.314922557961029526, -14.29746914071037800, 90.41775706135236135 ) ) ;
#75001=CARTESIAN_POINT ( 'NONE',  ( -21.55341960407619339, 5.719274019375674811, 98.54275706135234714 ) ) ;
#75002=CARTESIAN_POINT ( 'NONE',  ( 19.05341960407617918, -5.049401038297876454, 91.04275706135234714 ) ) ;
#75003=CARTESIAN_POINT ( 'NONE',  ( 0.05219959533910956823, 16.53943276465976808, 54.99890960531435269 ) ) ;
#75004=CARTESIAN_POINT ( 'NONE',  ( 14.29746914071049879, -8.314922557960816363, 103.3322429386476955 ) ) ;
#75005=CARTESIAN_POINT ( 'NONE',  ( 9.564922557961047289, -16.46253265017146816, 45.41775706135232582 ) ) ;
#75007=CARTESIAN_POINT ( 'NONE',  ( 15.72974639402176855, 15.80617190586768217, 51.87609039468568284 ) ) ;
#75008=CARTESIAN_POINT ( 'NONE',  ( 16.52544592524335698, 4.483927247898782831, 31.45942372801901854 ) ) ;
#75009=CARTESIAN_POINT ( 'NONE',  ( 17.12812012977029141, 6.668231424565952636, 83.85948759323147783 ) ) ;
#75010=CARTESIAN_POINT ( 'NONE',  ( -19.03943276465977164, 0.05219959533909376836, 111.2489096053143669 ) ) ;
#75011=CARTESIAN_POINT ( 'NONE',  ( 18.62759615963271287, -10.81492255796078972, 68.33224293864769550 ) ) ;
#75012=CARTESIAN_POINT ( 'NONE',  ( -9.474510206698720793, -16.51473224551083518, 94.58442372801900433 ) ) ;
#75013=CARTESIAN_POINT ( 'NONE',  ( -9.564922557960796823, -16.46253265017161027, 102.0822429386477097 ) ) ;
#75015=CARTESIAN_POINT ( 'NONE',  ( -16.55341960407611168, -4.379528057220339221, 111.4572429386476813 ) ) ;
#75016=CARTESIAN_POINT ( 'NONE',  ( -21.53943276465977519, -0.05219959533937600094, 98.75109039468568994 ) ) ;
#75017=CARTESIAN_POINT ( 'NONE',  ( -0.05219959533909027116, -19.03943276465977164, 47.49890960531435979 ) ) ;
#75018=CARTESIAN_POINT ( 'NONE',  ( -5.719274019375665041, -21.55341960407619695, 54.79275706135235424 ) ) ;
#75019=CARTESIAN_POINT ( 'NONE',  ( 0.05219959533937995610, -21.53943276465977519, 85.00109039468568994 ) ) ;
#75020=CARTESIAN_POINT ( 'NONE',  ( 8.314922557961029526, -14.29746914071037800, 110.4177570613523756 ) ) ;
#75021=CARTESIAN_POINT ( 'NONE',  ( -5.153800228976328057, -19.02544592524343514, 67.29057627198102409 ) ) ;
#75022=CARTESIAN_POINT ( 'NONE',  ( -15.80617190586768217, 15.72974639402176855, 38.12609039468567573 ) ) ;
#75023=CARTESIAN_POINT ( 'NONE',  ( -21.52544592524334988, -5.823673210054445271, 33.95942372801901143 ) ) ;
#75024=CARTESIAN_POINT ( 'NONE',  ( 13.89961937509957401, 13.97604488694547697, 71.87609039468567573 ) ) ;
#75025=CARTESIAN_POINT ( 'NONE',  ( 16.46253265017160672, -9.564922557960803928, 93.33224293864769550 ) ) ;
#75026=CARTESIAN_POINT ( 'NONE',  ( 14.34966873604960469, 8.224510206698951720, 109.1655762719810383 ) ) ;
#75027=CARTESIAN_POINT ( 'NONE',  ( -21.55341960407610458, -5.719274019375992779, 96.45724293864770971 ) ) ;
#75028=CARTESIAN_POINT ( 'NONE',  ( 12.14591786802309770, 12.06949235617756955, 69.37390960531436690 ) ) ;
#75029=CARTESIAN_POINT ( 'NONE',  ( 5.719274019375673035, 21.55341960407619339, 112.2927570613523471 ) ) ;
#75030=CARTESIAN_POINT ( 'NONE',  ( 12.06949235617757843, -12.14591786802309237, 88.12390960531436690 ) ) ;
#75031=CARTESIAN_POINT ( 'NONE',  ( 5.049401038298161559, -19.05341960407611168, 42.70724293864767418 ) ) ;
#75032=CARTESIAN_POINT ( 'NONE',  ( 19.02544592524334988, 5.153800228976608722, 81.45942372801897591 ) ) ;
#75033=CARTESIAN_POINT ( 'NONE',  ( 14.29746914071049879, -8.314922557960816363, 48.33224293864770260 ) ) ;
#75034=CARTESIAN_POINT ( 'NONE',  ( -21.52544592524334988, -5.823673210054445271, 98.95942372801903275 ) ) ;
#75035=CARTESIAN_POINT ( 'NONE',  ( 19.02544592524343514, -5.153800228976328945, 93.54057627198102409 ) ) ;
#75036=CARTESIAN_POINT ( 'NONE',  ( -19.03943276465977164, -0.05219959533935918106, 68.75109039468566152 ) ) ;
#75037=CARTESIAN_POINT ( 'NONE',  ( -10.81492255796078084, -18.62759615963271287, 77.08224293864769550 ) ) ;
#75038=CARTESIAN_POINT ( 'NONE',  ( 5.719274019375673035, 21.55341960407619339, 27.29275706135234358 ) ) ;
#75039=CARTESIAN_POINT ( 'NONE',  ( -16.53943276465976808, -0.05219959533934237506, 23.75109039468567929 ) ) ;
#75040=CARTESIAN_POINT ( 'NONE',  ( 16.53943276465976808, 0.05219959533934440121, 96.25109039468568994 ) ) ;
#75041=CARTESIAN_POINT ( 'NONE',  ( 19.05341960407611168, 5.049401038298154454, 23.95724293864769194 ) ) ;
#75042=CARTESIAN_POINT ( 'NONE',  ( -0.05219959533937732626, 21.53943276465977519, 42.50109039468567573 ) ) ;
#75043=CARTESIAN_POINT ( 'NONE',  ( 5.049401038298161559, -19.05341960407611168, 27.70724293864769550 ) ) ;
#75045=CARTESIAN_POINT ( 'NONE',  ( 0.05219959533934541429, -16.53943276465976808, 45.00109039468568284 ) ) ;
#75046=CARTESIAN_POINT ( 'NONE',  ( 4.483927247898545687, 16.52544592524342804, 74.79057627198105251 ) ) ;
#75047=CARTESIAN_POINT ( 'NONE',  ( 18.67979575497178502, 10.72451020669898547, 69.16557627198102409 ) ) ;
#75048=CARTESIAN_POINT ( 'NONE',  ( -16.53943276465976808, 0.05219959533911058130, 26.24890960531435624 ) ) ;
#75049=CARTESIAN_POINT ( 'NONE',  ( 8.314922557961029526, -14.29746914071037800, 55.41775706135234714 ) ) ;
#75050=CARTESIAN_POINT ( 'NONE',  ( -9.564922557960796823, -16.46253265017161027, 47.08224293864769550 ) ) ;
#75051=CARTESIAN_POINT ( 'NONE',  ( -14.29746914071037622, -8.314922557961029526, 99.16775706135234714 ) ) ;
#75052=CARTESIAN_POINT ( 'NONE',  ( 16.51473224551083163, -9.474510206698727899, 80.83442372801899012 ) ) ;
#75053=CARTESIAN_POINT ( 'NONE',  ( 15.72974639402199770, -15.80617190586745480, 68.12390960531436690 ) ) ;
#75054=CARTESIAN_POINT ( 'NONE',  ( 4.379528057220092307, 16.55341960407617563, 112.2927570613523471 ) ) ;
#75057=CARTESIAN_POINT ( 'NONE',  ( 0.05219959533907565091, 21.53943276465977519, 64.99890960531435269 ) ) ;
#75059=CARTESIAN_POINT ( 'NONE',  ( 14.29746914071037800, 8.314922557961029526, 91.66775706135234714 ) ) ;
#75061=CARTESIAN_POINT ( 'NONE',  ( 5.049401038298161559, -19.05341960407611168, 107.7072429386476955 ) ) ;
#75063=CARTESIAN_POINT ( 'NONE',  ( 5.823673210054125526, 21.52544592524343514, 69.79057627198102409 ) ) ;
#75064=CARTESIAN_POINT ( 'NONE',  ( 14.34966873604972726, -8.224510206698740333, 105.8344237280190328 ) ) ;
#75065=CARTESIAN_POINT ( 'NONE',  ( -16.53943276465976808, -0.05219959533934237506, 18.75109039468568639 ) ) ;
#75066=CARTESIAN_POINT ( 'NONE',  ( -5.153800228976328057, -19.02544592524343514, 22.29057627198102765 ) ) ;
#75067=CARTESIAN_POINT ( 'NONE',  ( -12.06949235617739369, -12.14591786802326823, 29.37609039468568284 ) ) ;
#75068=CARTESIAN_POINT ( 'NONE',  ( 13.97604488694527802, 13.89961937509977652, 59.37390960531434558 ) ) ;
#75070=CARTESIAN_POINT ( 'NONE',  ( 13.97604488694527802, 13.89961937509977652, 99.37390960531436690 ) ) ;
#75071=CARTESIAN_POINT ( 'NONE',  ( -16.53943276465976808, -0.05219959533934237506, 93.75109039468567573 ) ) ;
#75072=CARTESIAN_POINT ( 'NONE',  ( -9.564922557961040184, 16.46253265017147172, 87.91775706135233293 ) ) ;
#75073=CARTESIAN_POINT ( 'NONE',  ( -13.89961937509957401, -13.97604488694547875, 19.37609039468566507 ) ) ;
#75074=CARTESIAN_POINT ( 'NONE',  ( 10.81492255796078972, 18.62759615963270932, 69.58224293864769550 ) ) ;
#75075=CARTESIAN_POINT ( 'NONE',  ( -16.52544592524335698, -4.483927247898792601, 93.95942372801903275 ) ) ;
#75076=CARTESIAN_POINT ( 'NONE',  ( 16.51473224551083163, -9.474510206698727899, 90.83442372801900433 ) ) ;
#75077=CARTESIAN_POINT ( 'NONE',  ( -16.51473224551069308, -9.474510206698971260, 51.66557627198102409 ) ) ;
#75078=CARTESIAN_POINT ( 'NONE',  ( -16.51473224551069308, -9.474510206698971260, 96.66557627198102409 ) ) ;
#75079=CARTESIAN_POINT ( 'NONE',  ( -18.62759615963255300, -10.81492255796106328, 64.16775706135234714 ) ) ;
#75080=CARTESIAN_POINT ( 'NONE',  ( -13.89961937509977652, 13.97604488694528158, 65.62390960531436690 ) ) ;
#75081=CARTESIAN_POINT ( 'NONE',  ( -8.224510206698948167, 14.34966873604960824, 90.41557627198103830 ) ) ;
#75082=CARTESIAN_POINT ( 'NONE',  ( -17.13100169013300444, -6.664070546373138448, 84.23210164300149927 ) ) ;
#75083=CARTESIAN_POINT ( 'NONE',  ( -14.34966873604960291, -8.224510206698953496, 81.66557627198103830 ) ) ;
#75084=CARTESIAN_POINT ( 'NONE',  ( 5.823673210054125526, 21.52544592524343514, 79.79057627198102409 ) ) ;
#75087=CARTESIAN_POINT ( 'NONE',  ( 5.153800228976615827, -19.02544592524334988, 40.20942372801898301 ) ) ;
#75088=CARTESIAN_POINT ( 'NONE',  ( 17.44279575226788026, -5.990770900253884257, 73.33557567514321818 ) ) ;
#75089=CARTESIAN_POINT ( 'NONE',  ( 13.97604488694527802, 13.89961937509977652, 74.37390960531436690 ) ) ;
#75090=CARTESIAN_POINT ( 'NONE',  ( -5.049401038298153566, 19.05341960407611168, 85.20724293864766707 ) ) ;
#75091=CARTESIAN_POINT ( 'NONE',  ( 16.52544592524335698, 4.483927247898782831, 61.45942372801901854 ) ) ;
#75093=CARTESIAN_POINT ( 'NONE',  ( -19.05341960407617563, 5.049401038297882671, 48.54275706135233293 ) ) ;
#75094=CARTESIAN_POINT ( 'NONE',  ( 16.85867132384987244, 6.968984503517829054, 21.84742265313312259 ) ) ;
#75095=CARTESIAN_POINT ( 'NONE',  ( 19.02544592524343514, -5.153800228976328945, 113.5405762719810241 ) ) ;
#75096=CARTESIAN_POINT ( 'NONE',  ( 8.224510206698742110, 14.34966873604972548, 87.08442372801901854 ) ) ;
#75098=CARTESIAN_POINT ( 'NONE',  ( 12.14591786802327356, -12.06949235617739191, 75.62609039468567573 ) ) ;
#75100=CARTESIAN_POINT ( 'NONE',  ( -12.14591786802326823, 12.06949235617739902, 48.12609039468568284 ) ) ;
#75102=CARTESIAN_POINT ( 'NONE',  ( 18.62759615963255655, 10.81492255796105972, 61.66775706135235424 ) ) ;
#75103=CARTESIAN_POINT ( 'NONE',  ( 13.97604488694548053, -13.89961937509957401, 80.62609039468567573 ) ) ;
#75104=CARTESIAN_POINT ( 'NONE',  ( 13.97604488694548053, -13.89961937509957401, 20.62609039468567573 ) ) ;
#75105=CARTESIAN_POINT ( 'NONE',  ( -16.51473224551069308, -9.474510206698971260, 51.66557627198102409 ) ) ;
#75106=CARTESIAN_POINT ( 'NONE',  ( 9.564922557960805705, 16.46253265017160317, 39.58224293864768839 ) ) ;
#75108=CARTESIAN_POINT ( 'NONE',  ( 15.72974639402199770, -15.80617190586745480, 63.12390960531435979 ) ) ;
#75109=CARTESIAN_POINT ( 'NONE',  ( -13.89961937509977652, 13.97604488694528158, 115.6239096053143669 ) ) ;
#75110=CARTESIAN_POINT ( 'NONE',  ( 14.29746914071049879, -8.314922557960816363, 113.3322429386476955 ) ) ;
#75111=CARTESIAN_POINT ( 'NONE',  ( -14.29746914071037622, -8.314922557961029526, 49.16775706135234003 ) ) ;
#75112=ORIENTED_EDGE ( 'NONE', *, *, #38764, .F. ) ;
#75113=CARTESIAN_POINT ( 'NONE',  ( -5.719274019375978568, 21.55341960407610458, 115.2072429386476955 ) ) ;
#75114=CARTESIAN_POINT ( 'NONE',  ( -14.29746914071049879, 8.314922557960819915, 55.83224293864770260 ) ) ;
#75116=CARTESIAN_POINT ( 'NONE',  ( -19.02544592524334988, -5.153800228976617603, 108.9594237280189759 ) ) ;
#75117=CARTESIAN_POINT ( 'NONE',  ( -13.97604488694547697, 13.89961937509957934, 38.12609039468566152 ) ) ;
#75118=CARTESIAN_POINT ( 'NONE',  ( 4.483927247898545687, 16.52544592524342804, 39.79057627198103830 ) ) ;
#75119=CARTESIAN_POINT ( 'NONE',  ( 21.52544592524334988, 5.823673210054432836, 21.45942372801901499 ) ) ;
#75120=CARTESIAN_POINT ( 'NONE',  ( 17.48853670773242186, 5.747243402303175763, 33.83328700250010002 ) ) ;
#75121=CARTESIAN_POINT ( 'NONE',  ( 15.72974639402199770, -15.80617190586745480, 58.12390960531435979 ) ) ;
#75122=CARTESIAN_POINT ( 'NONE',  ( -13.97604488694527625, -13.89961937509977652, 86.87390960531436690 ) ) ;
#75123=CARTESIAN_POINT ( 'NONE',  ( -4.483927247898539470, -16.52544592524342804, 57.29057627198103120 ) ) ;
#75124=CARTESIAN_POINT ( 'NONE',  ( 13.97604488694527802, 13.89961937509977652, 109.3739096053143669 ) ) ;
#75126=CARTESIAN_POINT ( 'NONE',  ( -19.02544592524334988, -5.153800228976617603, 48.95942372801900433 ) ) ;
#75127=CARTESIAN_POINT ( 'NONE',  ( 21.55341960407610458, 5.719274019375980345, 103.9572429386476813 ) ) ;
#75128=CARTESIAN_POINT ( 'NONE',  ( 0.05219959533909260263, 19.03943276465977164, 49.99890960531435979 ) ) ;
#75129=CARTESIAN_POINT ( 'NONE',  ( -14.29746914071049879, 8.314922557960819915, 110.8322429386476955 ) ) ;
#75130=CARTESIAN_POINT ( 'NONE',  ( 21.53943276465977519, 0.05219959533937863772, 46.25109039468567573 ) ) ;
#75132=CARTESIAN_POINT ( 'NONE',  ( 0.05219959533910956823, 16.53943276465976808, 29.99890960531435979 ) ) ;
#75133=CARTESIAN_POINT ( 'NONE',  ( -9.564922557960796823, -16.46253265017161027, 47.08224293864769550 ) ) ;
#75134=CARTESIAN_POINT ( 'NONE',  ( 16.51473224551069308, 9.474510206698969483, 104.1655762719810241 ) ) ;
#75135=CARTESIAN_POINT ( 'NONE',  ( 18.62759615963271287, -10.81492255796078972, 73.33224293864769550 ) ) ;
#75137=B_SPLINE_CURVE_WITH_KNOTS ( 'NONE', 3,
 ( #168006, #14319, #46648, #76975, #75984, #137657, #199344, #45655, #30483, #138646, #15316, #169988, #93131, #79966, #20272, #52607, #68774, #65781, #97100, #82936, #141635, #36431, #95128, #51611, #112290, #173980, #33470, #129435, #144614, #48648, #188159, #3125 ),
 .UNSPECIFIED., .F., .F.,
 ( 4, 2, 2, 2, 2, 2, 2, 2, 2, 2, 2, 2, 2, 2, 2, 4 ),
 ( 1.638340482224582059E-15, 0.0003712461730052129009, 0.0007424923460087874639, 0.001113738519012362135, 0.001484984692015936698, 0.002227477038023092330, 0.002598723211026670362, 0.002969969384030248395, 0.003341215557033825993, 0.003712461730037403592, 0.004083707903040982058, 0.004454954076044560091, 0.004826200249048137256, 0.005197446422051715288, 0.005568692595055293321, 0.005939938768058871353 ),
 .UNSPECIFIED. ) ;
#75138=CARTESIAN_POINT ( 'NONE',  ( -9.474510206698964154, 16.51473224551069663, 40.41557627198103120 ) ) ;
#75139=CARTESIAN_POINT ( 'NONE',  ( -21.53943276465977519, 0.05219959533907696930, 56.24890960531436690 ) ) ;
#75140=CARTESIAN_POINT ( 'NONE',  ( 21.55341960407619695, -5.719274019375665929, 91.04275706135236135 ) ) ;
#75142=CARTESIAN_POINT ( 'NONE',  ( -14.29746914071037622, -8.314922557961029526, 79.16775706135234714 ) ) ;
#75143=CARTESIAN_POINT ( 'NONE',  ( -8.224510206698948167, 14.34966873604960824, 65.41557627198102409 ) ) ;
#75144=CARTESIAN_POINT ( 'NONE',  ( 5.153800228976335163, 19.02544592524342804, 74.79057627198103830 ) ) ;
#75146=CARTESIAN_POINT ( 'NONE',  ( -5.153800228976607833, 19.02544592524334988, 27.70942372801899722 ) ) ;
#75147=CARTESIAN_POINT ( 'NONE',  ( -8.224510206698735004, -14.34966873604973081, 89.58442372801901854 ) ) ;
#75148=CARTESIAN_POINT ( 'NONE',  ( -19.03943276465977164, -0.05219959533935918106, 23.75109039468566152 ) ) ;
#75149=CARTESIAN_POINT ( 'NONE',  ( -5.153800228976328057, -19.02544592524343514, 72.29057627198102409 ) ) ;
#75150=CARTESIAN_POINT ( 'NONE',  ( 18.62759615963271287, -10.81492255796078972, 48.33224293864770260 ) ) ;
#75151=CARTESIAN_POINT ( 'NONE',  ( 16.53943276465976808, 0.05219959533934440121, 31.25109039468568639 ) ) ;
#75152=CARTESIAN_POINT ( 'NONE',  ( 21.52544592524334988, 5.823673210054432836, 81.45942372801900433 ) ) ;
#75153=CARTESIAN_POINT ( 'NONE',  ( -14.34966873604972548, 8.224510206698743886, 63.33442372801900433 ) ) ;
#75154=CARTESIAN_POINT ( 'NONE',  ( -5.823673210054116645, -21.52544592524344225, 112.2905762719810241 ) ) ;
#75155=CARTESIAN_POINT ( 'NONE',  ( 8.224510206698742110, 14.34966873604972548, 22.08442372801901143 ) ) ;
#75156=CARTESIAN_POINT ( 'NONE',  ( 9.564922557960805705, 16.46253265017160317, 94.58224293864769550 ) ) ;
#75157=CARTESIAN_POINT ( 'NONE',  ( -16.55341960407617563, 4.379528057220093196, 28.54275706135234358 ) ) ;
#75158=CARTESIAN_POINT ( 'NONE',  ( 19.03943276465977164, -0.05219959533909143690, 53.74890960531436690 ) ) ;
#75159=CARTESIAN_POINT ( 'NONE',  ( 0.05219959533934541429, -16.53943276465976808, 35.00109039468568284 ) ) ;
#75160=CARTESIAN_POINT ( 'NONE',  ( -8.314922557960811034, -14.29746914071050412, 82.08224293864768129 ) ) ;
#75161=CARTESIAN_POINT ( 'NONE',  ( 16.53943276465976808, 0.05219959533934440121, 86.25109039468568994 ) ) ;
#75162=CARTESIAN_POINT ( 'NONE',  ( 0.05219959533937995610, -21.53943276465977519, 25.00109039468567218 ) ) ;
#75163=CARTESIAN_POINT ( 'NONE',  ( 0.05219959533909260263, 19.03943276465977164, 64.99890960531436690 ) ) ;
#75164=CARTESIAN_POINT ( 'NONE',  ( -13.97604488694527625, -13.89961937509977652, 76.87390960531433848 ) ) ;
#75165=CARTESIAN_POINT ( 'NONE',  ( -16.52544592524335698, -4.483927247898792601, 88.95942372801901854 ) ) ;
#75167=ORIENTED_EDGE ( 'NONE', *, *, #132905, .T. ) ;
#75169=CARTESIAN_POINT ( 'NONE',  ( 16.51473224551083163, -9.474510206698727899, 30.83442372801900433 ) ) ;
#75170=CARTESIAN_POINT ( 'NONE',  ( 9.474510206698971260, -16.51473224551069308, 97.91557627198102409 ) ) ;
#75171=CARTESIAN_POINT ( 'NONE',  ( -5.049401038298153566, 19.05341960407611168, 55.20724293864769550 ) ) ;
#75172=CARTESIAN_POINT ( 'NONE',  ( -16.46253265017160317, 9.564922557960807481, 115.8322429386477097 ) ) ;
#75173=CARTESIAN_POINT ( 'NONE',  ( -0.05219959533934338120, 16.53943276465976808, 32.50109039468568284 ) ) ;
#75174=CARTESIAN_POINT ( 'NONE',  ( -13.89961937509957401, -13.97604488694547875, 54.37609039468565442 ) ) ;
#75175=CARTESIAN_POINT ( 'NONE',  ( 8.314922557961029526, -14.29746914071037800, 40.41775706135234714 ) ) ;
#75176=CARTESIAN_POINT ( 'NONE',  ( -5.153800228976328057, -19.02544592524343514, 107.2905762719810383 ) ) ;
#75177=CARTESIAN_POINT ( 'NONE',  ( -19.05341960407611168, -5.049401038298163336, 71.45724293864766707 ) ) ;
#75178=CARTESIAN_POINT ( 'NONE',  ( -21.53943276465977519, 0.05219959533907696930, 101.2489096053143669 ) ) ;
#75179=CARTESIAN_POINT ( 'NONE',  ( 5.153800228976615827, -19.02544592524334988, 70.20942372801899012 ) ) ;
#75180=CARTESIAN_POINT ( 'NONE',  ( -16.51473224551069308, -9.474510206698971260, 86.66557627198102409 ) ) ;
#75182=CARTESIAN_POINT ( 'NONE',  ( 19.02544592524343514, -5.153800228976328945, 58.54057627198102409 ) ) ;
#75183=CARTESIAN_POINT ( 'NONE',  ( -14.29746914071049879, 8.314922557960819915, 40.83224293864769550 ) ) ;
#75184=CARTESIAN_POINT ( 'NONE',  ( -16.46253265017160317, 9.564922557960807481, 25.83224293864769194 ) ) ;
#75185=CARTESIAN_POINT ( 'NONE',  ( -16.51473224551082808, 9.474510206698731452, 43.33442372801900433 ) ) ;
#75186=CARTESIAN_POINT ( 'NONE',  ( -14.34966873604960291, -8.224510206698953496, 76.66557627198103830 ) ) ;
#75187=CARTESIAN_POINT ( 'NONE',  ( 21.52544592524334988, 5.823673210054432836, 96.45942372801901854 ) ) ;
#75188=CARTESIAN_POINT ( 'NONE',  ( 9.564922557960805705, 16.46253265017160317, 39.58224293864768839 ) ) ;
#75189=CARTESIAN_POINT ( 'NONE',  ( -12.06949235617739369, -12.14591786802326823, 54.37609039468568994 ) ) ;
#75191=CARTESIAN_POINT ( 'NONE',  ( 12.14591786802309770, 12.06949235617756955, 39.37390960531436690 ) ) ;
#75192=CARTESIAN_POINT ( 'NONE',  ( -18.62759615963255300, -10.81492255796106328, 104.1677570613523471 ) ) ;
#75193=CARTESIAN_POINT ( 'NONE',  ( 5.049401038298161559, -19.05341960407611168, 92.70724293864769550 ) ) ;
#75194=CARTESIAN_POINT ( 'NONE',  ( 5.049401038298161559, -19.05341960407611168, 97.70724293864766707 ) ) ;
#75195=CARTESIAN_POINT ( 'NONE',  ( -13.97604488694527625, -13.89961937509977652, 21.87390960531435979 ) ) ;
#75196=CARTESIAN_POINT ( 'NONE',  ( -16.55341960407611168, -4.379528057220339221, 106.4572429386477097 ) ) ;
#75197=CARTESIAN_POINT ( 'NONE',  ( -12.14591786802309592, -12.06949235617757132, 71.87390960531438111 ) ) ;
#75198=CARTESIAN_POINT ( 'NONE',  ( 10.81492255796078972, 18.62759615963270932, 79.58224293864769550 ) ) ;
#75199=CARTESIAN_POINT ( 'NONE',  ( 5.153800228976335163, 19.02544592524342804, 89.79057627198102409 ) ) ;
#75200=CARTESIAN_POINT ( 'NONE',  ( 15.72974639402199770, -15.80617190586745480, 93.12390960531436690 ) ) ;
#75201=CARTESIAN_POINT ( 'NONE',  ( 5.153800228976335163, 19.02544592524342804, 94.79057627198103830 ) ) ;
#75202=CARTESIAN_POINT ( 'NONE',  ( -19.39056639909674473, -5.499999999999968026, 90.78948781074345220 ) ) ;
#75203=CARTESIAN_POINT ( 'NONE',  ( -14.34966873604960291, -8.224510206698953496, 91.66557627198103830 ) ) ;
#75204=CARTESIAN_POINT ( 'NONE',  ( 13.89961937509977652, -13.97604488694527269, 58.12390960531436690 ) ) ;
#75205=CARTESIAN_POINT ( 'NONE',  ( -15.72974639402197994, 15.80617190586746368, 70.62390960531436690 ) ) ;
#75206=CARTESIAN_POINT ( 'NONE',  ( 17.05116617787827948, -6.768360034955676952, 26.15675553259199759 ) ) ;
#75207=CARTESIAN_POINT ( 'NONE',  ( -16.55341960407611168, -4.379528057220339221, 21.45724293864769550 ) ) ;
#75209=CARTESIAN_POINT ( 'NONE',  ( 8.314922557961029526, -14.29746914071037800, 25.41775706135235779 ) ) ;
#75210=CARTESIAN_POINT ( 'NONE',  ( -14.34966873604960291, -8.224510206698953496, 76.66557627198103830 ) ) ;
#75211=CARTESIAN_POINT ( 'NONE',  ( -18.09918380851992481, -5.500000000000039968, 46.48618307335612343 ) ) ;
#75212=CARTESIAN_POINT ( 'NONE',  ( 9.474510206698971260, -16.51473224551069308, 77.91557627198103830 ) ) ;
#75213=CARTESIAN_POINT ( 'NONE',  ( -19.03943276465977164, 0.05219959533909376836, 41.24890960531435269 ) ) ;
#75214=CARTESIAN_POINT ( 'NONE',  ( -4.483927247898539470, -16.52544592524342804, 67.29057627198103830 ) ) ;
#75215=CARTESIAN_POINT ( 'NONE',  ( 13.89961937509977652, -13.97604488694527269, 113.1239096053143527 ) ) ;
#75216=CARTESIAN_POINT ( 'NONE',  ( -19.02544592524334988, -5.153800228976617603, 98.95942372801900433 ) ) ;
#75217=CARTESIAN_POINT ( 'NONE',  ( 18.67979575497194134, -10.72451020669871369, 60.83442372801901854 ) ) ;
#75218=CARTESIAN_POINT ( 'NONE',  ( -9.474510206698964154, 16.51473224551069663, 95.41557627198102409 ) ) ;
#75219=CARTESIAN_POINT ( 'NONE',  ( 0.05219959533907565091, 21.53943276465977519, 79.99890960531435269 ) ) ;
#75220=CARTESIAN_POINT ( 'NONE',  ( -16.52544592524335698, -4.483927247898792601, 73.95942372801901854 ) ) ;
#75221=CARTESIAN_POINT ( 'NONE',  ( 5.153800228976335163, 19.02544592524342804, 24.79057627198102765 ) ) ;
#75222=CARTESIAN_POINT ( 'NONE',  ( 0.05219959533909260263, 19.03943276465977164, 69.99890960531435269 ) ) ;
#75223=CARTESIAN_POINT ( 'NONE',  ( 5.719274019375991003, -21.55341960407610458, 87.70724293864769550 ) ) ;
#75224=CARTESIAN_POINT ( 'NONE',  ( -0.05219959533936034679, 19.03943276465977164, 102.5010903946856757 ) ) ;
#75226=CARTESIAN_POINT ( 'NONE',  ( 4.379528057220339221, -16.55341960407611168, 42.70724293864770260 ) ) ;
#75227=CARTESIAN_POINT ( 'NONE',  ( -15.72974639402176322, -15.80617190586768395, 64.37609039468568994 ) ) ;
#75228=CARTESIAN_POINT ( 'NONE',  ( 12.14591786802327356, -12.06949235617739191, 90.62609039468567573 ) ) ;
#75229=CARTESIAN_POINT ( 'NONE',  ( 5.153800228976335163, 19.02544592524342804, 109.7905762719810099 ) ) ;
#75230=CARTESIAN_POINT ( 'NONE',  ( 16.51473224551069308, 9.474510206698969483, 104.1655762719810241 ) ) ;
#75232=CARTESIAN_POINT ( 'NONE',  ( -4.379528057220086978, -16.55341960407618274, 94.79275706135234714 ) ) ;
#75233=CARTESIAN_POINT ( 'NONE',  ( 16.55341960407618274, -4.379528057220086978, 51.04275706135234714 ) ) ;
#75234=CARTESIAN_POINT ( 'NONE',  ( 9.564922557960805705, 16.46253265017160317, 54.58224293864769550 ) ) ;
#75235=CARTESIAN_POINT ( 'NONE',  ( 5.153800228976335163, 19.02544592524342804, 74.79057627198103830 ) ) ;
#75236=CARTESIAN_POINT ( 'NONE',  ( -18.62759615963255300, -10.81492255796106328, 69.16775706135234714 ) ) ;
#75237=CARTESIAN_POINT ( 'NONE',  ( -4.483927247898782831, 16.52544592524335698, 67.70942372801901854 ) ) ;
#75238=CARTESIAN_POINT ( 'NONE',  ( -16.55341960407611168, -4.379528057220339221, 46.45724293864769550 ) ) ;
#75239=CARTESIAN_POINT ( 'NONE',  ( -19.02544592524342804, 5.153800228976336051, 46.04057627198101699 ) ) ;
#75240=CARTESIAN_POINT ( 'NONE',  ( 19.02544592524343514, -5.153800228976328945, 53.54057627198102409 ) ) ;
#75241=CARTESIAN_POINT ( 'NONE',  ( 8.224510206698742110, 14.34966873604972548, 37.08442372801901143 ) ) ;
#75242=CARTESIAN_POINT ( 'NONE',  ( -9.474510206698720793, -16.51473224551083518, 89.58442372801900433 ) ) ;
#75243=CARTESIAN_POINT ( 'NONE',  ( -16.53943276465976808, 0.05219959533911058130, 91.24890960531436690 ) ) ;
#75244=CARTESIAN_POINT ( 'NONE',  ( 19.03943276465977164, -0.05219959533909143690, 68.74890960531436690 ) ) ;
#75245=CARTESIAN_POINT ( 'NONE',  ( 19.03943276465977164, 0.05219959533936151252, 101.2510903946856757 ) ) ;
#75247=CARTESIAN_POINT ( 'NONE',  ( 21.53943276465977519, 0.05219959533937863772, 91.25109039468568994 ) ) ;
#75248=CARTESIAN_POINT ( 'NONE',  ( 16.55341960407618274, -4.379528057220086978, 61.04275706135234714 ) ) ;
#75250=CARTESIAN_POINT ( 'NONE',  ( -0.05219959533907301413, -21.53943276465977519, 47.49890960531435979 ) ) ;
#75251=CARTESIAN_POINT ( 'NONE',  ( 0.05219959533934541429, -16.53943276465976808, 55.00109039468568284 ) ) ;
#75252=CARTESIAN_POINT ( 'NONE',  ( 17.58332526062526568, -7.635886036038552760, 38.42334959558466778 ) ) ;
#75253=CARTESIAN_POINT ( 'NONE',  ( 13.89961937509957401, 13.97604488694547697, 41.87609039468566152 ) ) ;
#75254=CARTESIAN_POINT ( 'NONE',  ( -19.03943276465977164, 0.05219959533909376836, 86.24890960531436690 ) ) ;
#75255=CARTESIAN_POINT ( 'NONE',  ( -9.564922557960796823, -16.46253265017161027, 22.08224293864768839 ) ) ;
#75256=CARTESIAN_POINT ( 'NONE',  ( -5.153800228976328057, -19.02544592524343514, 62.29057627198100988 ) ) ;
#75258=CARTESIAN_POINT ( 'NONE',  ( -18.67979575497193778, 10.72451020669871902, 78.33442372801901854 ) ) ;
#75259=CARTESIAN_POINT ( 'NONE',  ( -18.39639308325436673, -5.500000000000040856, 56.48252246182197212 ) ) ;
#75260=CARTESIAN_POINT ( 'NONE',  ( -19.03943276465977164, -0.05219959533935918106, 38.75109039468566152 ) ) ;
#75261=CARTESIAN_POINT ( 'NONE',  ( -5.153800228976607833, 19.02544592524334988, 27.70942372801899722 ) ) ;
#75262=CARTESIAN_POINT ( 'NONE',  ( -4.379528057220328563, 16.55341960407611168, 50.20724293864769550 ) ) ;
#75263=CARTESIAN_POINT ( 'NONE',  ( 19.03943276465977164, -0.05219959533909143690, 53.74890960531436690 ) ) ;
#75264=CARTESIAN_POINT ( 'NONE',  ( 21.55341960407610458, 5.719274019375980345, 23.95724293864769550 ) ) ;
#75265=CARTESIAN_POINT ( 'NONE',  ( -21.55341960407619339, 5.719274019375674811, 78.54275706135236135 ) ) ;
#75266=CARTESIAN_POINT ( 'NONE',  ( 5.049401038298161559, -19.05341960407611168, 67.70724293864769550 ) ) ;
#75268=CARTESIAN_POINT ( 'NONE',  ( 21.53943276465977519, 0.05219959533937863772, 76.25109039468568994 ) ) ;
#75269=CARTESIAN_POINT ( 'NONE',  ( 21.52544592524344225, -5.823673210054117533, 33.54057627198102409 ) ) ;
#75270=CARTESIAN_POINT ( 'NONE',  ( -5.823673210054431948, 21.52544592524334988, 42.70942372801901854 ) ) ;
#75271=CARTESIAN_POINT ( 'NONE',  ( -19.05341960407617563, 5.049401038297882671, 63.54275706135234003 ) ) ;
#75272=CARTESIAN_POINT ( 'NONE',  ( -5.049401038298153566, 19.05341960407611168, 45.20724293864769550 ) ) ;
#75273=CARTESIAN_POINT ( 'NONE',  ( 9.474510206698971260, -16.51473224551069308, 82.91557627198103830 ) ) ;
#75274=CARTESIAN_POINT ( 'NONE',  ( 12.06949235617739724, 12.14591786802326823, 31.87609039468567929 ) ) ;
#75275=CARTESIAN_POINT ( 'NONE',  ( -4.483927247898539470, -16.52544592524342804, 82.29057627198103830 ) ) ;
#75276=CARTESIAN_POINT ( 'NONE',  ( -19.05341960407611168, -5.049401038298163336, 51.45724293864770260 ) ) ;
#75277=CARTESIAN_POINT ( 'NONE',  ( 21.53943276465977519, -0.05219959533907433946, 48.74890960531435979 ) ) ;
#75278=CARTESIAN_POINT ( 'NONE',  ( 14.34966873604972726, -8.224510206698740333, 20.83442372801901143 ) ) ;
#75279=CARTESIAN_POINT ( 'NONE',  ( 15.80617190586769283, -15.72974639402175789, 25.62609039468567929 ) ) ;
#75280=CARTESIAN_POINT ( 'NONE',  ( 10.72451020669871369, 18.67979575497193778, 77.08442372801901854 ) ) ;
#75281=CARTESIAN_POINT ( 'NONE',  ( 12.14591786802327356, -12.06949235617739191, 75.62609039468567573 ) ) ;
#75282=CARTESIAN_POINT ( 'NONE',  ( -8.224510206698735004, -14.34966873604973081, 64.58442372801900433 ) ) ;
#75283=CARTESIAN_POINT ( 'NONE',  ( -5.153800228976328057, -19.02544592524343514, 57.29057627198103120 ) ) ;
#75284=CARTESIAN_POINT ( 'NONE',  ( -16.53943276465976808, -0.05219959533934237506, 88.75109039468567573 ) ) ;
#75285=CARTESIAN_POINT ( 'NONE',  ( -13.97604488694547697, 13.89961937509957934, 48.12609039468566863 ) ) ;
#75286=CARTESIAN_POINT ( 'NONE',  ( -21.55341960407619339, 5.719274019375674811, 23.54275706135235424 ) ) ;
#75287=CARTESIAN_POINT ( 'NONE',  ( -8.314922557960811034, -14.29746914071050412, 62.08224293864769550 ) ) ;
#75288=CARTESIAN_POINT ( 'NONE',  ( 9.474510206698971260, -16.51473224551069308, 82.91557627198103830 ) ) ;
#75289=CARTESIAN_POINT ( 'NONE',  ( 8.314922557961029526, -14.29746914071037800, 95.41775706135234714 ) ) ;
#75290=CARTESIAN_POINT ( 'NONE',  ( -21.55341960407619339, 5.719274019375674811, 58.54275706135235424 ) ) ;
#75291=CARTESIAN_POINT ( 'NONE',  ( -14.29746914071037622, -8.314922557961029526, 29.16775706135234003 ) ) ;
#75292=CARTESIAN_POINT ( 'NONE',  ( -15.72974639402197994, 15.80617190586746368, 105.6239096053143669 ) ) ;
#75293=CARTESIAN_POINT ( 'NONE',  ( -8.224510206698948167, 14.34966873604960824, 55.41557627198102409 ) ) ;
#75295=CARTESIAN_POINT ( 'NONE',  ( -15.72974639402197994, 15.80617190586746368, 95.62390960531436690 ) ) ;
#75296=CARTESIAN_POINT ( 'NONE',  ( 0.05219959533910956823, 16.53943276465976808, 44.99890960531435979 ) ) ;
#75299=CARTESIAN_POINT ( 'NONE',  ( -9.474510206698964154, 16.51473224551069663, 115.4155762719810241 ) ) ;
#75300=CARTESIAN_POINT ( 'NONE',  ( -18.67979575497193778, 10.72451020669871902, 43.33442372801901143 ) ) ;
#75301=CARTESIAN_POINT ( 'NONE',  ( -12.14591786802309592, -12.06949235617757132, 61.87390960531436690 ) ) ;
#75302=CARTESIAN_POINT ( 'NONE',  ( -9.474510206698964154, 16.51473224551069663, 60.41557627198102409 ) ) ;
#75303=CARTESIAN_POINT ( 'NONE',  ( -13.89961937509977652, 13.97604488694528158, 30.62390960531435269 ) ) ;
#75304=CARTESIAN_POINT ( 'NONE',  ( 5.049401038297881783, 19.05341960407617563, 67.29275706135234714 ) ) ;
#75305=CARTESIAN_POINT ( 'NONE',  ( -5.823673210054116645, -21.52544592524344225, 42.29057627198103120 ) ) ;
#75307=CARTESIAN_POINT ( 'NONE',  ( 5.153800228976335163, 19.02544592524342804, 64.79057627198100988 ) ) ;
#75308=CARTESIAN_POINT ( 'NONE',  ( 14.29746914071037800, 8.314922557961029526, 36.66775706135234714 ) ) ;
#75309=CARTESIAN_POINT ( 'NONE',  ( 5.823673210054125526, 21.52544592524343514, 109.7905762719810383 ) ) ;
#75310=CARTESIAN_POINT ( 'NONE',  ( -16.52544592524342804, 4.483927247898546575, 41.04057627198103120 ) ) ;
#75311=ORIENTED_EDGE ( 'NONE', *, *, #114623, .F. ) ;
#75312=CARTESIAN_POINT ( 'NONE',  ( -5.153800228976328057, -19.02544592524343514, 92.29057627198099567 ) ) ;
#75313=CARTESIAN_POINT ( 'NONE',  ( 0.05219959533907565091, 21.53943276465977519, 69.99890960531435269 ) ) ;
#75314=CARTESIAN_POINT ( 'NONE',  ( 15.72974639402199770, -15.80617190586745480, 113.1239096053143953 ) ) ;
#75315=CARTESIAN_POINT ( 'NONE',  ( 8.314922557961029526, -14.29746914071037800, 40.41775706135234714 ) ) ;
#75316=CARTESIAN_POINT ( 'NONE',  ( 15.80617190586746368, 15.72974639402197994, 34.37390960531435979 ) ) ;
#75317=CARTESIAN_POINT ( 'NONE',  ( 5.719274019375673035, 21.55341960407619339, 107.2927570613523471 ) ) ;
#75318=CARTESIAN_POINT ( 'NONE',  ( 19.02544592524343514, -5.153800228976328945, 103.5405762719809957 ) ) ;
#75319=CARTESIAN_POINT ( 'NONE',  ( -5.153800228976328057, -19.02544592524343514, 47.29057627198102409 ) ) ;
#75320=CARTESIAN_POINT ( 'NONE',  ( 13.97604488694527802, 13.89961937509977652, 94.37390960531436690 ) ) ;
#75321=CARTESIAN_POINT ( 'NONE',  ( -5.153800228976328057, -19.02544592524343514, 77.29057627198099567 ) ) ;
#75322=CARTESIAN_POINT ( 'NONE',  ( 16.18388926212248791, -7.379444403734420455, 87.06046848633769741 ) ) ;
#75324=CARTESIAN_POINT ( 'NONE',  ( 9.474510206698729675, 16.51473224551082808, 57.08442372801900433 ) ) ;
#75325=CARTESIAN_POINT ( 'NONE',  ( 0.05219959533936267826, -19.03943276465977164, 20.00109039468567218 ) ) ;
#75326=CARTESIAN_POINT ( 'NONE',  ( 10.81492255796078972, 18.62759615963270932, 34.58224293864770260 ) ) ;
#75327=CARTESIAN_POINT ( 'NONE',  ( 12.14591786802327356, -12.06949235617739191, 110.6260903946857042 ) ) ;
#75328=CARTESIAN_POINT ( 'NONE',  ( -19.03943276465977164, -0.05219959533935918106, 78.75109039468567573 ) ) ;
#75329=CARTESIAN_POINT ( 'NONE',  ( 13.97604488694527802, 13.89961937509977830, 39.37390960531435979 ) ) ;
#75330=CARTESIAN_POINT ( 'NONE',  ( -16.51473224551082808, 9.474510206698731452, 83.33442372801899012 ) ) ;
#75331=CARTESIAN_POINT ( 'NONE',  ( -19.05341960407617563, 5.049401038297882671, 33.54275706135231871 ) ) ;
#75332=CARTESIAN_POINT ( 'NONE',  ( 16.79531203550646623, 7.028104445595620753, 108.7524498822044023 ) ) ;
#75333=CARTESIAN_POINT ( 'NONE',  ( -5.049401038298153566, 19.05341960407611168, 40.20724293864768839 ) ) ;
#75334=CARTESIAN_POINT ( 'NONE',  ( 4.483927247898545687, 16.52544592524342804, 54.79057627198104541 ) ) ;
#75335=CARTESIAN_POINT ( 'NONE',  ( -19.05341960407611168, -5.049401038298163336, 21.45724293864768839 ) ) ;
#75336=CARTESIAN_POINT ( 'NONE',  ( -16.55341960407611168, -4.379528057220339221, 21.45724293864769550 ) ) ;
#75337=CARTESIAN_POINT ( 'NONE',  ( 18.22780087662122384, -5.500000000000022204, 46.01540105326107266 ) ) ;
#75338=CARTESIAN_POINT ( 'NONE',  ( 8.224510206698742110, 14.34966873604972548, 97.08442372801904696 ) ) ;
#75339=CARTESIAN_POINT ( 'NONE',  ( -19.03943276465977164, 0.05219959533909376836, 56.24890960531435979 ) ) ;
#75340=CARTESIAN_POINT ( 'NONE',  ( -18.62759615963255300, -10.81492255796106328, 109.1677570613523613 ) ) ;
#75341=CARTESIAN_POINT ( 'NONE',  ( 12.14591786802327356, -12.06949235617739191, 20.62609039468568639 ) ) ;
#75342=CARTESIAN_POINT ( 'NONE',  ( 21.52544592524334988, 5.823673210054432836, 91.45942372801901854 ) ) ;
#75344=CARTESIAN_POINT ( 'NONE',  ( -9.474510206698964154, 16.51473224551069663, 95.41557627198102409 ) ) ;
#75345=CARTESIAN_POINT ( 'NONE',  ( 19.03943276465977164, -0.05219959533909143690, 88.74890960531436690 ) ) ;
#75347=CARTESIAN_POINT ( 'NONE',  ( 21.55341960407610458, 5.719274019375980345, 113.9572429386477239 ) ) ;
#75348=CARTESIAN_POINT ( 'NONE',  ( 14.34966873604960469, 8.224510206698951720, 79.16557627198103830 ) ) ;
#75349=CARTESIAN_POINT ( 'NONE',  ( 15.80617190586746368, 15.72974639402197994, 74.37390960531436690 ) ) ;
#75350=CARTESIAN_POINT ( 'NONE',  ( -16.46253265017160317, 9.564922557960807481, 65.83224293864769550 ) ) ;
#75351=CARTESIAN_POINT ( 'NONE',  ( 10.81492255796078972, 18.62759615963270932, 99.58224293864770971 ) ) ;
#75352=CARTESIAN_POINT ( 'NONE',  ( -4.379528057220086978, -16.55341960407618274, 89.79275706135236135 ) ) ;
#75353=ORIENTED_EDGE ( 'NONE', *, *, #8545, .T. ) ;
#75354=CARTESIAN_POINT ( 'NONE',  ( -13.97604488694527625, -13.89961937509977652, 66.87390960531436690 ) ) ;
#75355=CARTESIAN_POINT ( 'NONE',  ( -16.53943276465976808, 0.05219959533911058130, 86.24890960531436690 ) ) ;
#75356=CARTESIAN_POINT ( 'NONE',  ( 17.50000000000000000, 5.500000000000001776, 33.78230962303567253 ) ) ;
#75357=CARTESIAN_POINT ( 'NONE',  ( 16.46253265017160672, -9.564922557960803928, 48.33224293864769550 ) ) ;
#75358=CARTESIAN_POINT ( 'NONE',  ( 16.51473224551083163, -9.474510206698727899, 75.83442372801900433 ) ) ;
#75359=CARTESIAN_POINT ( 'NONE',  ( 14.34966873604960469, 8.224510206698951720, 79.16557627198103830 ) ) ;
#75360=CARTESIAN_POINT ( 'NONE',  ( 21.52544592524334988, 5.823673210054432836, 56.45942372801902565 ) ) ;
#75361=CARTESIAN_POINT ( 'NONE',  ( -13.97604488694527625, -13.89961937509977652, 36.87390960531436690 ) ) ;
#75362=CARTESIAN_POINT ( 'NONE',  ( -21.52544592524343514, 5.823673210054127303, 116.0405762719810383 ) ) ;
#75363=CARTESIAN_POINT ( 'NONE',  ( -12.14591786802309592, -12.06949235617757132, 101.8739096053143811 ) ) ;
#75365=CARTESIAN_POINT ( 'NONE',  ( -13.97604488694527625, -13.89961937509977652, 61.87390960531435979 ) ) ;
#75366=CARTESIAN_POINT ( 'NONE',  ( 19.19724070472090105, 5.500000000000154543, 48.56193348274384647 ) ) ;
#75367=CARTESIAN_POINT ( 'NONE',  ( 13.97604488694548053, -13.89961937509957401, 100.6260903946856615 ) ) ;
#75368=CARTESIAN_POINT ( 'NONE',  ( 0.05219959533909260263, 19.03943276465977164, 109.9989096053143669 ) ) ;
#75369=CARTESIAN_POINT ( 'NONE',  ( 21.55341960407619695, -5.719274019375665929, 46.04275706135234714 ) ) ;
#75370=CARTESIAN_POINT ( 'NONE',  ( 19.03943276465977164, -0.05219959533909143690, 83.74890960531436690 ) ) ;
#75371=CARTESIAN_POINT ( 'NONE',  ( -13.89961937509957401, -13.97604488694547875, 74.37609039468566152 ) ) ;
#75372=CARTESIAN_POINT ( 'NONE',  ( 5.049401038298161559, -19.05341960407611168, 57.70724293864769550 ) ) ;
#75373=CARTESIAN_POINT ( 'NONE',  ( -0.05219959533910754901, -16.53943276465976808, 82.49890960531436690 ) ) ;
#75374=CARTESIAN_POINT ( 'NONE',  ( -4.483927247898539470, -16.52544592524342804, 67.29057627198103830 ) ) ;
#75375=CARTESIAN_POINT ( 'NONE',  ( -0.05219959533909027116, -19.03943276465977164, 87.49890960531436690 ) ) ;
#75376=CARTESIAN_POINT ( 'NONE',  ( 16.52544592524342804, -4.483927247898539470, 73.54057627198102409 ) ) ;
#75377=CARTESIAN_POINT ( 'NONE',  ( -9.474510206698964154, 16.51473224551069663, 80.41557627198103830 ) ) ;
#75378=CARTESIAN_POINT ( 'NONE',  ( 19.02544592524334988, 5.153800228976608722, 31.45942372801900433 ) ) ;
#75379=CARTESIAN_POINT ( 'NONE',  ( -13.97604488694527625, -13.89961937509977652, 46.87390960531435979 ) ) ;
#75380=CARTESIAN_POINT ( 'NONE',  ( -14.34966873604960291, -8.224510206698953496, 31.66557627198102054 ) ) ;
#75381=CARTESIAN_POINT ( 'NONE',  ( -19.03943276465977164, 0.05219959533909376836, 21.24890960531436335 ) ) ;
#75382=ORIENTED_EDGE ( 'NONE', *, *, #137500, .F. ) ;
#75383=CARTESIAN_POINT ( 'NONE',  ( 15.80617190586769283, -15.72974639402175789, 40.62609039468567573 ) ) ;
#75384=CARTESIAN_POINT ( 'NONE',  ( 9.474510206698729675, 16.51473224551082808, 62.08442372801899722 ) ) ;
#75385=CARTESIAN_POINT ( 'NONE',  ( 16.52544592524342804, -4.483927247898539470, 33.54057627198102409 ) ) ;
#75386=CARTESIAN_POINT ( 'NONE',  ( -5.719274019375978568, 21.55341960407610458, 80.20724293864769550 ) ) ;
#75387=CARTESIAN_POINT ( 'NONE',  ( -15.72974639402197994, 15.80617190586746368, 25.62390960531435624 ) ) ;
#75388=CARTESIAN_POINT ( 'NONE',  ( 8.314922557960818139, 14.29746914071049879, 64.58224293864769550 ) ) ;
#75389=CARTESIAN_POINT ( 'NONE',  ( 19.02544592524343514, -5.153800228976328945, 43.54057627198103120 ) ) ;
#75390=CARTESIAN_POINT ( 'NONE',  ( -5.049401038297874678, -19.05341960407617918, 44.79275706135232582 ) ) ;
#75391=CARTESIAN_POINT ( 'NONE',  ( 16.53943276465976808, 0.05219959533934440121, 106.2510903946856757 ) ) ;
#75392=CARTESIAN_POINT ( 'NONE',  ( 4.379528057220092307, 16.55341960407617563, 62.29275706135236845 ) ) ;
#75393=CARTESIAN_POINT ( 'NONE',  ( -10.81492255796078084, -18.62759615963271287, 32.08224293864769550 ) ) ;
#75394=CARTESIAN_POINT ( 'NONE',  ( -21.53943276465977519, -0.05219959533937600094, 103.7510903946857042 ) ) ;
#75395=CARTESIAN_POINT ( 'NONE',  ( 0.05219959533909260263, 19.03943276465977164, 94.99890960531436690 ) ) ;
#75396=CARTESIAN_POINT ( 'NONE',  ( -12.14591786802326823, 12.06949235617739902, 73.12609039468567573 ) ) ;
#75397=CARTESIAN_POINT ( 'NONE',  ( -19.02544592524342804, 5.153800228976336051, 26.04057627198103120 ) ) ;
#75399=CARTESIAN_POINT ( 'NONE',  ( -16.53943276465976808, 0.05219959533911058130, 36.24890960531435979 ) ) ;
#75400=CARTESIAN_POINT ( 'NONE',  ( 19.02544592524343514, -5.153800228976328945, 98.54057627198100988 ) ) ;
#75401=CARTESIAN_POINT ( 'NONE',  ( -5.153800228976328057, -19.02544592524343514, 97.29057627198099567 ) ) ;
#75402=CARTESIAN_POINT ( 'NONE',  ( -18.67979575497178146, -10.72451020669898902, 21.66557627198102409 ) ) ;
#75403=CARTESIAN_POINT ( 'NONE',  ( 0.05219959533910956823, 16.53943276465976808, 69.99890960531435269 ) ) ;
#75404=CARTESIAN_POINT ( 'NONE',  ( -0.05219959533910754901, -16.53943276465976808, 37.49890960531436690 ) ) ;
#75406=CARTESIAN_POINT ( 'NONE',  ( -12.06949235617756955, 12.14591786802309770, 55.62390960531436690 ) ) ;
#75407=EDGE_LOOP ( 'NONE', ( #17697, #124592, #195444, #186083 ) ) ;
#75408=CARTESIAN_POINT ( 'NONE',  ( 16.52544592524335698, 4.483927247898782831, 56.45942372801902565 ) ) ;
#75409=CARTESIAN_POINT ( 'NONE',  ( 19.05341960407617918, -5.049401038297876454, 56.04275706135234714 ) ) ;
#75410=CARTESIAN_POINT ( 'NONE',  ( 9.474510206698971260, -16.51473224551069308, 82.91557627198103830 ) ) ;
#75411=CARTESIAN_POINT ( 'NONE',  ( 13.89961937509957401, 13.97604488694547697, 71.87609039468567573 ) ) ;
#75413=CARTESIAN_POINT ( 'NONE',  ( 16.51473224551083163, -9.474510206698727899, 50.83442372801899722 ) ) ;
#75414=CARTESIAN_POINT ( 'NONE',  ( 13.97604488694548053, -13.89961937509957401, 95.62609039468563310 ) ) ;
#75415=CARTESIAN_POINT ( 'NONE',  ( -16.55341960407617563, 4.379528057220093196, 98.54275706135234714 ) ) ;
#75417=CARTESIAN_POINT ( 'NONE',  ( 9.564922557960805705, 16.46253265017160317, 24.58224293864769194 ) ) ;
#75418=CARTESIAN_POINT ( 'NONE',  ( 5.719274019375991003, -21.55341960407610458, 22.70724293864769194 ) ) ;
#75419=CARTESIAN_POINT ( 'NONE',  ( 15.80617190586769283, -15.72974639402175789, 45.62609039468567573 ) ) ;
#75420=CARTESIAN_POINT ( 'NONE',  ( 16.46253265017146816, 9.564922557961045513, 106.6677570613523471 ) ) ;
#75421=CARTESIAN_POINT ( 'NONE',  ( 17.49999999999999645, -4.013004640162614933, 107.9460572099440725 ) ) ;
#75422=CARTESIAN_POINT ( 'NONE',  ( 5.049401038298161559, -19.05341960407611168, 57.70724293864769550 ) ) ;
#75424=CARTESIAN_POINT ( 'NONE',  ( -8.314922557960811034, -14.29746914071050412, 77.08224293864769550 ) ) ;
#75425=CARTESIAN_POINT ( 'NONE',  ( -9.474510206698964154, 16.51473224551069663, 65.41557627198102409 ) ) ;
#75426=CARTESIAN_POINT ( 'NONE',  ( -19.05341960407611168, -5.049401038298163336, 76.45724293864769550 ) ) ;
#75427=CARTESIAN_POINT ( 'NONE',  ( -9.474510206698720793, -16.51473224551083518, 79.58442372801899012 ) ) ;
#75428=CARTESIAN_POINT ( 'NONE',  ( -18.67979575497178146, -10.72451020669898902, 51.66557627198102409 ) ) ;
#75429=CARTESIAN_POINT ( 'NONE',  ( 16.53943276465976808, -0.05219959533910856209, 108.7489096053143669 ) ) ;
#75430=CARTESIAN_POINT ( 'NONE',  ( -9.474510206698720793, -16.51473224551083518, 39.58442372801899722 ) ) ;
#75431=CARTESIAN_POINT ( 'NONE',  ( 5.153800228976335163, 19.02544592524342804, 79.79057627198102409 ) ) ;
#75432=CARTESIAN_POINT ( 'NONE',  ( -5.823673210054116645, -21.52544592524344225, 72.29057627198102409 ) ) ;
#75433=CARTESIAN_POINT ( 'NONE',  ( -16.55341960407611168, -4.379528057220339221, 86.45724293864770971 ) ) ;
#75434=CARTESIAN_POINT ( 'NONE',  ( -9.564922557961040184, 16.46253265017147172, 42.91775706135234003 ) ) ;
#75435=CARTESIAN_POINT ( 'NONE',  ( 5.823673210054125526, 21.52544592524343514, 74.79057627198105251 ) ) ;
#75436=CARTESIAN_POINT ( 'NONE',  ( -10.72451020669898014, 18.67979575497178502, 65.41557627198102409 ) ) ;
#75437=CARTESIAN_POINT ( 'NONE',  ( 10.72451020669898902, -18.67979575497178502, 37.91557627198102409 ) ) ;
#75438=CARTESIAN_POINT ( 'NONE',  ( 21.52544592524334988, 5.823673210054432836, 96.45942372801901854 ) ) ;
#75439=CARTESIAN_POINT ( 'NONE',  ( -16.46253265017160317, 9.564922557960807481, 70.83224293864770971 ) ) ;
#75440=CARTESIAN_POINT ( 'NONE',  ( 13.97604488694527802, 13.89961937509977652, 24.37390960531435624 ) ) ;
#75441=CARTESIAN_POINT ( 'NONE',  ( 18.62759615963255655, 10.81492255796105972, 31.66775706135234358 ) ) ;
#75442=CARTESIAN_POINT ( 'NONE',  ( -18.62759615963255300, -10.81492255796106328, 44.16775706135234714 ) ) ;
#75443=CARTESIAN_POINT ( 'NONE',  ( -13.97604488694527625, -13.89961937509977652, 31.87390960531435979 ) ) ;
#75444=CARTESIAN_POINT ( 'NONE',  ( 18.67979575497178502, 10.72451020669898547, 109.1655762719810383 ) ) ;
#75445=CARTESIAN_POINT ( 'NONE',  ( -19.03943276465977164, -0.05219959533935918106, 58.75109039468566863 ) ) ;
#75446=CARTESIAN_POINT ( 'NONE',  ( -0.05219959533909027116, -19.03943276465977164, 42.49890960531435269 ) ) ;
#75447=CARTESIAN_POINT ( 'NONE',  ( 16.53943276465976808, 0.05219959533934440121, 26.25109039468567573 ) ) ;
#75449=CARTESIAN_POINT ( 'NONE',  ( 12.14591786802327356, -12.06949235617739191, 55.62609039468568284 ) ) ;
#75450=CARTESIAN_POINT ( 'NONE',  ( 9.564922557960805705, 16.46253265017160317, 34.58224293864770260 ) ) ;
#75452=CARTESIAN_POINT ( 'NONE',  ( 16.46253265017160672, -9.564922557960803928, 83.33224293864768129 ) ) ;
#75453=CARTESIAN_POINT ( 'NONE',  ( 0.05219959533910956823, 16.53943276465976808, 114.9989096053143669 ) ) ;
#75454=CARTESIAN_POINT ( 'NONE',  ( -0.05219959533907301413, -21.53943276465977519, 62.49890960531436690 ) ) ;
#75455=CARTESIAN_POINT ( 'NONE',  ( 4.483927247898790824, -16.52544592524335698, 50.20942372801901854 ) ) ;
#75456=CARTESIAN_POINT ( 'NONE',  ( 10.81492255796106328, -18.62759615963255655, 105.4177570613523613 ) ) ;
#75457=CARTESIAN_POINT ( 'NONE',  ( -19.03943276465977164, 0.05219959533909376836, 41.24890960531435269 ) ) ;
#75458=CARTESIAN_POINT ( 'NONE',  ( 4.379528057220339221, -16.55341960407611168, 22.70724293864769194 ) ) ;
#75459=CARTESIAN_POINT ( 'NONE',  ( 4.483927247898545687, 16.52544592524342804, 54.79057627198104541 ) ) ;
#75460=CARTESIAN_POINT ( 'NONE',  ( -9.564922557960796823, -16.46253265017161027, 67.08224293864769550 ) ) ;
#75461=CARTESIAN_POINT ( 'NONE',  ( 18.67979575497194134, -10.72451020669871369, 105.8344237280190328 ) ) ;
#75462=CARTESIAN_POINT ( 'NONE',  ( 0.05219959533937995610, -21.53943276465977519, 25.00109039468567218 ) ) ;
#75464=CARTESIAN_POINT ( 'NONE',  ( 10.81492255796106328, -18.62759615963255655, 80.41775706135234714 ) ) ;
#75465=CARTESIAN_POINT ( 'NONE',  ( 16.52544592524335698, 4.483927247898782831, 46.45942372801901854 ) ) ;
#75466=CARTESIAN_POINT ( 'NONE',  ( -16.52544592524335698, -4.483927247898792601, 23.95942372801901143 ) ) ;
#75467=CARTESIAN_POINT ( 'NONE',  ( 12.14591786802309770, 12.06949235617756955, 79.37390960531436690 ) ) ;
#75468=CARTESIAN_POINT ( 'NONE',  ( -21.53943276465977519, -0.05219959533937600094, 93.75109039468567573 ) ) ;
#75469=CARTESIAN_POINT ( 'NONE',  ( -12.06949235617756955, 12.14591786802309770, 35.62390960531437401 ) ) ;
#75470=CARTESIAN_POINT ( 'NONE',  ( -17.26058549869090086, 6.457015423128545706, 113.6225416252393501 ) ) ;
#75471=CARTESIAN_POINT ( 'NONE',  ( 12.06949235617739724, 12.14591786802326823, 41.87609039468568284 ) ) ;
#75472=CARTESIAN_POINT ( 'NONE',  ( 16.52544592524342804, -4.483927247898539470, 53.54057627198103120 ) ) ;
#75473=CARTESIAN_POINT ( 'NONE',  ( -12.14591786802326823, 12.06949235617739902, 93.12609039468568994 ) ) ;
#75474=CARTESIAN_POINT ( 'NONE',  ( 19.05341960407611168, 5.049401038298154454, 98.95724293864766707 ) ) ;
#75475=CARTESIAN_POINT ( 'NONE',  ( 9.564922557960805705, 16.46253265017160317, 114.5822429386476955 ) ) ;
#75476=CARTESIAN_POINT ( 'NONE',  ( -18.62759615963255300, -10.81492255796106328, 109.1677570613523613 ) ) ;
#75477=CARTESIAN_POINT ( 'NONE',  ( 4.379528057220339221, -16.55341960407611168, 82.70724293864770971 ) ) ;
#75478=CARTESIAN_POINT ( 'NONE',  ( 5.153800228976335163, 19.02544592524342804, 99.79057627198102409 ) ) ;
#75479=ORIENTED_EDGE ( 'NONE', *, *, #35102, .T. ) ;
#75480=CARTESIAN_POINT ( 'NONE',  ( 16.55341960407618274, -4.379528057220086978, 36.04275706135234714 ) ) ;
#75481=CARTESIAN_POINT ( 'NONE',  ( -5.049401038298153566, 19.05341960407611168, 40.20724293864768839 ) ) ;
#75482=CARTESIAN_POINT ( 'NONE',  ( 5.153800228976335163, 19.02544592524342804, 104.7905762719809957 ) ) ;
#75483=CARTESIAN_POINT ( 'NONE',  ( 14.34966873604972726, -8.224510206698740333, 40.83442372801901854 ) ) ;
#75484=DIRECTION ( 'NONE',  ( 0.000000000000000000, 0.000000000000000000, -1.000000000000000000 ) ) ;
#75485=CARTESIAN_POINT ( 'NONE',  ( -5.153800228976607833, 19.02544592524334988, 37.70942372801899722 ) ) ;
#75486=CARTESIAN_POINT ( 'NONE',  ( -19.03943276465977164, 0.05219959533909376836, 41.24890960531435269 ) ) ;
#75487=CARTESIAN_POINT ( 'NONE',  ( -16.53943276465976808, -0.05219959533934237506, 83.75109039468568994 ) ) ;
#75488=CARTESIAN_POINT ( 'NONE',  ( -19.02544592524334988, -5.153800228976617603, 78.95942372801900433 ) ) ;
#75489=CARTESIAN_POINT ( 'NONE',  ( 13.89961937509957401, 13.97604488694547697, 31.87609039468566863 ) ) ;
#75490=CARTESIAN_POINT ( 'NONE',  ( -5.049401038298153566, 19.05341960407611168, 55.20724293864769550 ) ) ;
#75491=CARTESIAN_POINT ( 'NONE',  ( -14.34966873604960291, -8.224510206698953496, 101.6655762719810383 ) ) ;
#75492=CARTESIAN_POINT ( 'NONE',  ( 16.46253265017146816, 9.564922557961045513, 71.66775706135233293 ) ) ;
#75493=CARTESIAN_POINT ( 'NONE',  ( 21.52544592524344225, -5.823673210054117533, 68.54057627198103830 ) ) ;
#75494=CARTESIAN_POINT ( 'NONE',  ( 19.02544592524334988, 5.153800228976608722, 21.45942372801899012 ) ) ;
#75495=CARTESIAN_POINT ( 'NONE',  ( 13.97604488694527802, 13.89961937509977652, 109.3739096053143669 ) ) ;
#75496=CARTESIAN_POINT ( 'NONE',  ( -5.823673210054116645, -21.52544592524344225, 72.29057627198102409 ) ) ;
#75497=CARTESIAN_POINT ( 'NONE',  ( -13.97604488694527625, -13.89961937509977652, 111.8739096053143243 ) ) ;
#75498=CARTESIAN_POINT ( 'NONE',  ( 19.05341960407617918, -5.049401038297876454, 101.0427570613523045 ) ) ;
#75499=CARTESIAN_POINT ( 'NONE',  ( -13.97604488694547520, 13.89961937509957934, 98.12609039468566152 ) ) ;
#75500=CARTESIAN_POINT ( 'NONE',  ( 14.29746914071037800, 8.314922557961029526, 21.66775706135235069 ) ) ;
#75501=CARTESIAN_POINT ( 'NONE',  ( 5.153800228976335163, 19.02544592524342804, 29.79057627198102409 ) ) ;
#75502=CARTESIAN_POINT ( 'NONE',  ( 9.474510206698971260, -16.51473224551069308, 102.9155762719810241 ) ) ;
#75503=CARTESIAN_POINT ( 'NONE',  ( 5.719274019375991003, -21.55341960407610458, 87.70724293864769550 ) ) ;
#75505=CARTESIAN_POINT ( 'NONE',  ( 15.72974639402176855, 15.80617190586768217, 61.87609039468568284 ) ) ;
#75506=CARTESIAN_POINT ( 'NONE',  ( -16.46253265017146816, -9.564922557961047289, 104.1677570613523329 ) ) ;
#75507=CARTESIAN_POINT ( 'NONE',  ( -21.55341960407619339, 5.719274019375674811, 113.5427570613523756 ) ) ;
#75508=CARTESIAN_POINT ( 'NONE',  ( 12.06949235617757843, -12.14591786802309237, 23.12390960531436335 ) ) ;
#75509=CARTESIAN_POINT ( 'NONE',  ( -18.62759615963270932, 10.81492255796079327, 105.8322429386476955 ) ) ;
#75510=CARTESIAN_POINT ( 'NONE',  ( 12.06949235617757843, -12.14591786802309237, 38.12390960531436690 ) ) ;
#75511=CARTESIAN_POINT ( 'NONE',  ( -9.474510206698720793, -16.51473224551083518, 84.58442372801900433 ) ) ;
#75512=CARTESIAN_POINT ( 'NONE',  ( -13.89961937509957401, -13.97604488694547875, 54.37609039468565442 ) ) ;
#75513=CARTESIAN_POINT ( 'NONE',  ( -21.53943276465977519, -0.05219959533937600094, 58.75109039468568994 ) ) ;
#75514=CARTESIAN_POINT ( 'NONE',  ( 13.97604488694548053, -13.89961937509957401, 45.62609039468566863 ) ) ;
#75515=CARTESIAN_POINT ( 'NONE',  ( 14.34966873604960469, 8.224510206698951720, 104.1655762719810241 ) ) ;
#75516=CARTESIAN_POINT ( 'NONE',  ( 18.67979575497178502, 10.72451020669898547, 29.16557627198103120 ) ) ;
#75517=CARTESIAN_POINT ( 'NONE',  ( -8.314922557960811034, -14.29746914071050412, 37.08224293864768129 ) ) ;
#75518=CARTESIAN_POINT ( 'NONE',  ( -10.81492255796105439, 18.62759615963255655, 92.91775706135236135 ) ) ;
#75519=CARTESIAN_POINT ( 'NONE',  ( -8.314922557961024197, 14.29746914071037800, 67.91775706135234714 ) ) ;
#75520=CARTESIAN_POINT ( 'NONE',  ( -0.05219959533910754901, -16.53943276465976808, 27.49890960531435269 ) ) ;
#75521=CARTESIAN_POINT ( 'NONE',  ( 15.72974639402176855, 15.80617190586768217, 66.87609039468568994 ) ) ;
#75522=CARTESIAN_POINT ( 'NONE',  ( -21.52544592524334988, -5.823673210054445271, 68.95942372801901854 ) ) ;
#75523=CARTESIAN_POINT ( 'NONE',  ( -10.81492255796078084, -18.62759615963271287, 72.08224293864769550 ) ) ;
#75524=ORIENTED_EDGE ( 'NONE', *, *, #122751, .F. ) ;
#75525=CARTESIAN_POINT ( 'NONE',  ( 0.05219959533909260263, 19.03943276465977164, 29.99890960531435979 ) ) ;
#75526=CARTESIAN_POINT ( 'NONE',  ( -21.52544592524334988, -5.823673210054445271, 43.95942372801902565 ) ) ;
#75527=CARTESIAN_POINT ( 'NONE',  ( -12.06949235617756955, 12.14591786802309770, 115.6239096053143669 ) ) ;
#75528=CARTESIAN_POINT ( 'NONE',  ( -16.51473224551069308, -9.474510206698971260, 41.66557627198103120 ) ) ;
#75529=CARTESIAN_POINT ( 'NONE',  ( 8.224510206698953496, -14.34966873604960469, 82.91557627198103830 ) ) ;
#75530=CARTESIAN_POINT ( 'NONE',  ( 16.46253265017160672, -9.564922557960803928, 83.33224293864768129 ) ) ;
#75531=CARTESIAN_POINT ( 'NONE',  ( 0.05219959533910956823, 16.53943276465976808, 29.99890960531435979 ) ) ;
#75532=CARTESIAN_POINT ( 'NONE',  ( 18.62759615963271287, -10.81492255796078972, 73.33224293864769550 ) ) ;
#75533=CARTESIAN_POINT ( 'NONE',  ( -21.52544592524343514, 5.823673210054127303, 111.0405762719810525 ) ) ;
#75535=CARTESIAN_POINT ( 'NONE',  ( -5.153800228976328057, -19.02544592524343514, 67.29057627198102409 ) ) ;
#75536=CARTESIAN_POINT ( 'NONE',  ( 16.51473224551083163, -9.474510206698727899, 105.8344237280190043 ) ) ;
#75537=CARTESIAN_POINT ( 'NONE',  ( 18.67979575497178502, 10.72451020669898547, 59.16557627198103120 ) ) ;
#75538=CARTESIAN_POINT ( 'NONE',  ( 21.53943276465977519, 0.05219959533937863772, 76.25109039468568994 ) ) ;
#75539=CARTESIAN_POINT ( 'NONE',  ( -16.46253265017160317, 9.564922557960807481, 60.83224293864769550 ) ) ;
#75541=CARTESIAN_POINT ( 'NONE',  ( 9.474510206698971260, -16.51473224551069308, 92.91557627198103830 ) ) ;
#75542=CARTESIAN_POINT ( 'NONE',  ( 8.314922557961029526, -14.29746914071037800, 80.41775706135234714 ) ) ;
#75543=CARTESIAN_POINT ( 'NONE',  ( 0.05219959533937995610, -21.53943276465977519, 60.00109039468568284 ) ) ;
#75544=CARTESIAN_POINT ( 'NONE',  ( -5.823673210054431948, 21.52544592524334988, 82.70942372801900433 ) ) ;
#75545=CARTESIAN_POINT ( 'NONE',  ( 5.823673210054125526, 21.52544592524343514, 109.7905762719810383 ) ) ;
#75546=CARTESIAN_POINT ( 'NONE',  ( 15.80617190586746368, 15.72974639402197994, 79.37390960531436690 ) ) ;
#75547=CARTESIAN_POINT ( 'NONE',  ( 5.049401038297881783, 19.05341960407617563, 42.29275706135234003 ) ) ;
#75548=CARTESIAN_POINT ( 'NONE',  ( 15.80617190586746368, 15.72974639402197994, 39.37390960531436690 ) ) ;
#75549=CARTESIAN_POINT ( 'NONE',  ( 19.05341960407611168, 5.049401038298154454, 83.95724293864766707 ) ) ;
#75550=CARTESIAN_POINT ( 'NONE',  ( -8.314922557960811034, -14.29746914071050412, 32.08224293864769550 ) ) ;
#75554=CARTESIAN_POINT ( 'NONE',  ( 9.564922557961047289, -16.46253265017146816, 90.41775706135234714 ) ) ;
#75555=CARTESIAN_POINT ( 'NONE',  ( 15.72974639402199770, -15.80617190586745480, 68.12390960531436690 ) ) ;
#75556=CARTESIAN_POINT ( 'NONE',  ( 12.06949235617757843, -12.14591786802309237, 58.12390960531435979 ) ) ;
#75557=CARTESIAN_POINT ( 'NONE',  ( 14.29746914071037800, 8.314922557961029526, 26.66775706135235424 ) ) ;
#75558=CARTESIAN_POINT ( 'NONE',  ( -19.03943276465977164, 0.05219959533909376836, 41.24890960531435269 ) ) ;
#75559=CARTESIAN_POINT ( 'NONE',  ( 5.823673210054125526, 21.52544592524343514, 104.7905762719810241 ) ) ;
#75560=CARTESIAN_POINT ( 'NONE',  ( -16.51473224551082808, 9.474510206698731452, 73.33442372801900433 ) ) ;
#75561=CARTESIAN_POINT ( 'NONE',  ( -5.153800228976328057, -19.02544592524343514, 87.29057627198103830 ) ) ;
#75562=CARTESIAN_POINT ( 'NONE',  ( 16.52544592524342804, -4.483927247898539470, 83.54057627198102409 ) ) ;
#75563=CARTESIAN_POINT ( 'NONE',  ( -0.05219959533909027116, -19.03943276465977164, 62.49890960531435979 ) ) ;
#75564=CARTESIAN_POINT ( 'NONE',  ( 0.05219959533910956823, 16.53943276465976808, 64.99890960531435269 ) ) ;
#75565=CARTESIAN_POINT ( 'NONE',  ( -13.97604488694527625, -13.89961937509977652, 36.87390960531436690 ) ) ;
#75566=CARTESIAN_POINT ( 'NONE',  ( -17.13361728884595081, -5.330296506332817152, 20.84482979903667754 ) ) ;
#75567=CARTESIAN_POINT ( 'NONE',  ( -16.52544592524342804, 4.483927247898546575, 46.04057627198103830 ) ) ;
#75568=CARTESIAN_POINT ( 'NONE',  ( 9.564922557960805705, 16.46253265017160317, 94.58224293864769550 ) ) ;
#75570=CARTESIAN_POINT ( 'NONE',  ( -16.51473224551082808, 9.474510206698731452, 58.33442372801900433 ) ) ;
#75571=CARTESIAN_POINT ( 'NONE',  ( -12.14591786802326823, 12.06949235617739902, 63.12609039468568994 ) ) ;
#75572=CARTESIAN_POINT ( 'NONE',  ( 15.72974639402199770, -15.80617190586745480, 78.12390960531436690 ) ) ;
#75573=CARTESIAN_POINT ( 'NONE',  ( 19.03943276465977164, 0.05219959533936151252, 36.25109039468567573 ) ) ;
#75574=CARTESIAN_POINT ( 'NONE',  ( 0.05219959533909260263, 19.03943276465977164, 84.99890960531436690 ) ) ;
#75576=CARTESIAN_POINT ( 'NONE',  ( -0.05219959533907301413, -21.53943276465977519, 22.49890960531436335 ) ) ;
#75577=CARTESIAN_POINT ( 'NONE',  ( -16.51473224551069308, -9.474510206698971260, 61.66557627198103120 ) ) ;
#75578=CARTESIAN_POINT ( 'NONE',  ( -18.62759615963255300, -10.81492255796106328, 54.16775706135235424 ) ) ;
#75579=CARTESIAN_POINT ( 'NONE',  ( -8.224510206698948167, 14.34966873604960824, 115.4155762719810241 ) ) ;
#75580=CARTESIAN_POINT ( 'NONE',  ( -5.719274019375665041, -21.55341960407619695, 19.79275706135235069 ) ) ;
#75581=CARTESIAN_POINT ( 'NONE',  ( 13.89961937509977652, -13.97604488694527269, 98.12390960531433848 ) ) ;
#75583=CARTESIAN_POINT ( 'NONE',  ( -18.62759615963255300, -10.81492255796106328, 39.16775706135235424 ) ) ;
#75585=CARTESIAN_POINT ( 'NONE',  ( 19.02544592524343514, -5.153800228976328945, 103.5405762719809957 ) ) ;
#75587=CARTESIAN_POINT ( 'NONE',  ( -21.55341960407610458, -5.719274019375992779, 106.4572429386477097 ) ) ;
#75588=CARTESIAN_POINT ( 'NONE',  ( 19.02544592524343514, -5.153800228976328945, 53.54057627198102409 ) ) ;
#75589=CARTESIAN_POINT ( 'NONE',  ( -16.53943276465976808, -0.05219959533934237506, 23.75109039468567929 ) ) ;
#75591=CARTESIAN_POINT ( 'NONE',  ( -18.62759615963255300, -10.81492255796106328, 99.16775706135234714 ) ) ;
#75592=CARTESIAN_POINT ( 'NONE',  ( 5.049401038298161559, -19.05341960407611168, 32.70724293864768129 ) ) ;
#75593=CARTESIAN_POINT ( 'NONE',  ( 0.05219959533937995610, -21.53943276465977519, 95.00109039468568994 ) ) ;
#75594=CARTESIAN_POINT ( 'NONE',  ( -13.97604488694527625, -13.89961937509977652, 86.87390960531436690 ) ) ;
#75595=CARTESIAN_POINT ( 'NONE',  ( 0.05219959533937995610, -21.53943276465977519, 55.00109039468568284 ) ) ;
#75597=CARTESIAN_POINT ( 'NONE',  ( 13.97604488694527802, 13.89961937509977652, 94.37390960531436690 ) ) ;
#75599=CARTESIAN_POINT ( 'NONE',  ( 14.29746914071037800, 8.314922557961029526, 41.66775706135235424 ) ) ;
#75600=CARTESIAN_POINT ( 'NONE',  ( 12.06949235617739724, 12.14591786802326823, 71.87609039468568994 ) ) ;
#75601=CARTESIAN_POINT ( 'NONE',  ( -10.72451020669870658, -18.67979575497194134, 54.58442372801901143 ) ) ;
#75602=CARTESIAN_POINT ( 'NONE',  ( -15.80617190586768217, 15.72974639402176855, 83.12609039468568994 ) ) ;
#75604=CARTESIAN_POINT ( 'NONE',  ( -13.97604488694547697, 13.89961937509957934, 113.1260903946856757 ) ) ;
#75605=CARTESIAN_POINT ( 'NONE',  ( 5.049401038298161559, -19.05341960407611168, 77.70724293864765286 ) ) ;
#75606=CARTESIAN_POINT ( 'NONE',  ( 5.049401038298161559, -19.05341960407611168, 92.70724293864769550 ) ) ;
#75607=CARTESIAN_POINT ( 'NONE',  ( -8.224510206698948167, 14.34966873604960824, 115.4155762719810241 ) ) ;
#75608=CARTESIAN_POINT ( 'NONE',  ( -21.52544592524343514, 5.823673210054127303, 26.04057627198103475 ) ) ;
#75609=CARTESIAN_POINT ( 'NONE',  ( -4.483927247898782831, 16.52544592524335698, 92.70942372801901854 ) ) ;
#75610=CARTESIAN_POINT ( 'NONE',  ( 8.314922557960818139, 14.29746914071049879, 64.58224293864769550 ) ) ;
#75611=CARTESIAN_POINT ( 'NONE',  ( -13.89961937509977652, 13.97604488694528158, 60.62390960531436690 ) ) ;
#75612=CARTESIAN_POINT ( 'NONE',  ( -0.05219959533937732626, 21.53943276465977519, 92.50109039468567573 ) ) ;
#75614=CARTESIAN_POINT ( 'NONE',  ( 19.05341960407617918, -5.049401038297876454, 111.0427570613523329 ) ) ;
#75615=CARTESIAN_POINT ( 'NONE',  ( -12.06949235617756955, 12.14591786802309770, 80.62390960531438111 ) ) ;
#75616=CARTESIAN_POINT ( 'NONE',  ( 21.55341960407619695, -5.719274019375665929, 31.04275706135234714 ) ) ;
#75617=CARTESIAN_POINT ( 'NONE',  ( 5.823673210054125526, 21.52544592524343514, 59.79057627198103120 ) ) ;
#75618=CARTESIAN_POINT ( 'NONE',  ( -13.89961937509957401, -13.97604488694547875, 39.37609039468566152 ) ) ;
#75620=CARTESIAN_POINT ( 'NONE',  ( -9.474510206698964154, 16.51473224551069663, 80.41557627198103830 ) ) ;
#75621=CARTESIAN_POINT ( 'NONE',  ( 16.52544592524342804, -4.483927247898539470, 53.54057627198103120 ) ) ;
#75623=CARTESIAN_POINT ( 'NONE',  ( 4.483927247898545687, 16.52544592524342804, 34.79057627198103120 ) ) ;
#75624=CARTESIAN_POINT ( 'NONE',  ( 8.224510206698742110, 14.34966873604972548, 97.08442372801904696 ) ) ;
#75625=CARTESIAN_POINT ( 'NONE',  ( 16.46253265017146816, 9.564922557961045513, 56.66775706135233293 ) ) ;
#75627=CARTESIAN_POINT ( 'NONE',  ( 0.05219959533909260263, 19.03943276465977164, 99.99890960531436690 ) ) ;
#75629=CARTESIAN_POINT ( 'NONE',  ( -12.06949235617756955, 12.14591786802309770, 80.62390960531438111 ) ) ;
#75630=CARTESIAN_POINT ( 'NONE',  ( -0.05219959533936034679, 19.03943276465977164, 47.50109039468566863 ) ) ;
#75631=CARTESIAN_POINT ( 'NONE',  ( -16.46253265017160317, 9.564922557960807481, 30.83224293864769550 ) ) ;
#75632=CARTESIAN_POINT ( 'NONE',  ( -21.55341960407610458, -5.719274019375992779, 36.45724293864768839 ) ) ;
#75633=CARTESIAN_POINT ( 'NONE',  ( 21.52544592524344225, -5.823673210054117533, 73.54057627198102409 ) ) ;
#75634=CARTESIAN_POINT ( 'NONE',  ( -16.53943276465976808, 0.05219959533911058130, 106.2489096053143811 ) ) ;
#75635=CARTESIAN_POINT ( 'NONE',  ( 4.379528057220092307, 16.55341960407617563, 47.29275706135234003 ) ) ;
#75636=CARTESIAN_POINT ( 'NONE',  ( -9.564922557960796823, -16.46253265017161027, 47.08224293864769550 ) ) ;
#75637=CARTESIAN_POINT ( 'NONE',  ( -0.05219959533937732626, 21.53943276465977519, 42.50109039468567573 ) ) ;
#75638=CARTESIAN_POINT ( 'NONE',  ( -16.52544592524342804, 4.483927247898546575, 86.04057627198102409 ) ) ;
#75641=CARTESIAN_POINT ( 'NONE',  ( 18.62759615963271287, -10.81492255796078972, 33.33224293864769550 ) ) ;
#75644=CARTESIAN_POINT ( 'NONE',  ( -14.34966873604972548, 8.224510206698743886, 38.33442372801900433 ) ) ;
#75645=CARTESIAN_POINT ( 'NONE',  ( 8.314922557960818139, 14.29746914071049879, 49.58224293864769550 ) ) ;
#75646=CARTESIAN_POINT ( 'NONE',  ( 10.72451020669898902, -18.67979575497178502, 67.91557627198102409 ) ) ;
#75647=CARTESIAN_POINT ( 'NONE',  ( 18.67979575497178502, 10.72451020669898547, 64.16557627198102409 ) ) ;
#75649=CARTESIAN_POINT ( 'NONE',  ( -16.51473224551069308, -9.474510206698971260, 41.66557627198103120 ) ) ;
#75650=CARTESIAN_POINT ( 'NONE',  ( -16.46253265017160317, 9.564922557960807481, 105.8322429386476955 ) ) ;
#75651=CARTESIAN_POINT ( 'NONE',  ( -9.474510206698964154, 16.51473224551069663, 50.41557627198102409 ) ) ;
#75652=CARTESIAN_POINT ( 'NONE',  ( 16.53943276465976808, -0.05219959533910856209, 108.7489096053143669 ) ) ;
#75654=CARTESIAN_POINT ( 'NONE',  ( -5.049401038298153566, 19.05341960407611168, 115.2072429386477097 ) ) ;
#75657=CARTESIAN_POINT ( 'NONE',  ( -8.224510206698735004, -14.34966873604973081, 69.58442372801900433 ) ) ;
#75658=CARTESIAN_POINT ( 'NONE',  ( 5.823673210054125526, 21.52544592524343514, 109.7905762719810383 ) ) ;
#75659=CARTESIAN_POINT ( 'NONE',  ( -16.51473224551069308, -9.474510206698971260, 51.66557627198102409 ) ) ;
#75660=CARTESIAN_POINT ( 'NONE',  ( 21.52544592524334988, 5.823673210054432836, 41.45942372801901143 ) ) ;
#75661=CARTESIAN_POINT ( 'NONE',  ( -0.05219959533909027116, -19.03943276465977164, 87.49890960531436690 ) ) ;
#75664=CARTESIAN_POINT ( 'NONE',  ( 21.55341960407619695, -5.719274019375665929, 31.04275706135234714 ) ) ;
#75665=CARTESIAN_POINT ( 'NONE',  ( -0.05219959533909027116, -19.03943276465977164, 107.4989096053143527 ) ) ;
#75666=CARTESIAN_POINT ( 'NONE',  ( -0.05219959533936034679, 19.03943276465977164, 87.50109039468567573 ) ) ;
#75667=CARTESIAN_POINT ( 'NONE',  ( 0.05219959533936267826, -19.03943276465977164, 45.00109039468566863 ) ) ;
#75668=CARTESIAN_POINT ( 'NONE',  ( -21.55341960407610458, -5.719274019375992779, 106.4572429386477097 ) ) ;
#75669=CARTESIAN_POINT ( 'NONE',  ( -19.05341960407617563, 5.049401038297882671, 28.54275706135232937 ) ) ;
#75670=CARTESIAN_POINT ( 'NONE',  ( 5.049401038297881783, 19.05341960407617563, 32.29275706135233293 ) ) ;
#75671=CARTESIAN_POINT ( 'NONE',  ( 8.314922557961029526, -14.29746914071037800, 90.41775706135236135 ) ) ;
#75672=FACE_OUTER_BOUND ( 'NONE', #136094, .T. ) ;
#75673=CARTESIAN_POINT ( 'NONE',  ( -19.02544592524342804, 5.153800228976336051, 56.04057627198100988 ) ) ;
#75674=CARTESIAN_POINT ( 'NONE',  ( -21.53943276465977519, -0.05219959533937600094, 63.75109039468568284 ) ) ;
#75675=CARTESIAN_POINT ( 'NONE',  ( 5.719274019375673035, 21.55341960407619339, 87.29275706135236135 ) ) ;
#75676=CARTESIAN_POINT ( 'NONE',  ( 9.564922557960805705, 16.46253265017160317, 79.58224293864769550 ) ) ;
#75677=CARTESIAN_POINT ( 'NONE',  ( -5.719274019375665041, -21.55341960407619695, 59.79275706135234714 ) ) ;
#75678=CARTESIAN_POINT ( 'NONE',  ( 13.89961937509957401, 13.97604488694547697, 96.87609039468566152 ) ) ;
#75679=CARTESIAN_POINT ( 'NONE',  ( -19.02544592524342804, 5.153800228976336051, 61.04057627198103120 ) ) ;
#75680=CARTESIAN_POINT ( 'NONE',  ( 19.03943276465977164, -0.05219959533909143690, 93.74890960531435269 ) ) ;
#75681=CARTESIAN_POINT ( 'NONE',  ( 13.97604488694527802, 13.89961937509977652, 79.37390960531435269 ) ) ;
#75683=CARTESIAN_POINT ( 'NONE',  ( 19.05341960407611168, 5.049401038298154454, 63.95724293864769550 ) ) ;
#75684=CARTESIAN_POINT ( 'NONE',  ( 21.55341960407610458, 5.719274019375980345, 93.95724293864770971 ) ) ;
#75685=CARTESIAN_POINT ( 'NONE',  ( 0.05219959533934541429, -16.53943276465976808, 85.00109039468568994 ) ) ;
#75687=CARTESIAN_POINT ( 'NONE',  ( -9.564922557961040184, 16.46253265017147172, 42.91775706135234003 ) ) ;
#75688=CARTESIAN_POINT ( 'NONE',  ( 5.153800228976335163, 19.02544592524342804, 74.79057627198103830 ) ) ;
#75689=CARTESIAN_POINT ( 'NONE',  ( -16.55341960407611168, -4.379528057220339221, 71.45724293864769550 ) ) ;
#75690=CARTESIAN_POINT ( 'NONE',  ( -12.14591786802309592, -12.06949235617757132, 106.8739096053143811 ) ) ;
#75691=CARTESIAN_POINT ( 'NONE',  ( 15.80617190586746368, 15.72974639402197994, 24.37390960531435979 ) ) ;
#75692=CARTESIAN_POINT ( 'NONE',  ( 9.564922557960805705, 16.46253265017160317, 104.5822429386476955 ) ) ;
#75694=CARTESIAN_POINT ( 'NONE',  ( 5.153800228976615827, -19.02544592524334988, 25.20942372801900433 ) ) ;
#75695=CARTESIAN_POINT ( 'NONE',  ( -14.29746914071037622, -8.314922557961029526, 89.16775706135236135 ) ) ;
#75696=CARTESIAN_POINT ( 'NONE',  ( -13.97604488694527625, -13.89961937509977652, 76.87390960531433848 ) ) ;
#75697=CARTESIAN_POINT ( 'NONE',  ( -5.719274019375665041, -21.55341960407619695, 54.79275706135235424 ) ) ;
#75698=CARTESIAN_POINT ( 'NONE',  ( -15.80617190586745835, -15.72974639402198527, 31.87390960531435979 ) ) ;
#75699=CARTESIAN_POINT ( 'NONE',  ( -10.81492255796105439, 18.62759615963255655, 22.91775706135235069 ) ) ;
#75700=CARTESIAN_POINT ( 'NONE',  ( 5.823673210054125526, 21.52544592524343514, 74.79057627198105251 ) ) ;
#75701=CARTESIAN_POINT ( 'NONE',  ( 0.05219959533910956823, 16.53943276465976808, 89.99890960531438111 ) ) ;
#75702=CARTESIAN_POINT ( 'NONE',  ( 5.049401038297881783, 19.05341960407617563, 57.29275706135231871 ) ) ;
#75704=CARTESIAN_POINT ( 'NONE',  ( -16.46253265017160317, 9.564922557960807481, 30.83224293864769550 ) ) ;
#75705=CARTESIAN_POINT ( 'NONE',  ( 13.89961937509977652, -13.97604488694527269, 78.12390960531433848 ) ) ;
#75706=CARTESIAN_POINT ( 'NONE',  ( 13.89961937509977652, -13.97604488694527269, 83.12390960531436690 ) ) ;
#75708=CARTESIAN_POINT ( 'NONE',  ( -14.29746914071049879, 8.314922557960819915, 100.8322429386477097 ) ) ;
#75710=CARTESIAN_POINT ( 'NONE',  ( -4.483927247898539470, -16.52544592524342804, 32.29057627198102409 ) ) ;
#75711=CARTESIAN_POINT ( 'NONE',  ( -8.224510206698735004, -14.34966873604973081, 24.58442372801901499 ) ) ;
#75712=CARTESIAN_POINT ( 'NONE',  ( -15.72974639402176322, -15.80617190586768395, 89.37609039468568994 ) ) ;
#75713=CARTESIAN_POINT ( 'NONE',  ( 19.05341960407611168, 5.049401038298154454, 103.9572429386476671 ) ) ;
#75714=CARTESIAN_POINT ( 'NONE',  ( 5.719274019375991003, -21.55341960407610458, 112.7072429386476955 ) ) ;
#75715=CARTESIAN_POINT ( 'NONE',  ( 16.51473224551069308, 9.474510206698969483, 39.16557627198103120 ) ) ;
#75716=CARTESIAN_POINT ( 'NONE',  ( -14.29746914071037622, -8.314922557961029526, 44.16775706135234714 ) ) ;
#75718=CARTESIAN_POINT ( 'NONE',  ( 5.049401038297881783, 19.05341960407617563, 112.2927570613523471 ) ) ;
#75720=CARTESIAN_POINT ( 'NONE',  ( -19.03943276465977164, 0.05219959533909376836, 31.24890960531435979 ) ) ;
#75721=CARTESIAN_POINT ( 'NONE',  ( -8.224510206698948167, 14.34966873604960824, 100.4155762719810241 ) ) ;
#75722=CARTESIAN_POINT ( 'NONE',  ( 15.80617190586746368, 15.72974639402197994, 109.3739096053143811 ) ) ;
#75723=CARTESIAN_POINT ( 'NONE',  ( 5.049401038297881783, 19.05341960407617563, 62.29275706135234003 ) ) ;
#75725=CARTESIAN_POINT ( 'NONE',  ( 15.80617190586769283, -15.72974639402175789, 25.62609039468567929 ) ) ;
#75727=CARTESIAN_POINT ( 'NONE',  ( -19.02544592524342804, 5.153800228976336051, 86.04057627198103830 ) ) ;
#75730=CARTESIAN_POINT ( 'NONE',  ( 0.05219959533909260263, 19.03943276465977164, 79.99890960531436690 ) ) ;
#75731=CARTESIAN_POINT ( 'NONE',  ( -18.67979575497193778, 10.72451020669871902, 38.33442372801900433 ) ) ;
#75732=CARTESIAN_POINT ( 'NONE',  ( 14.29746914071049879, -8.314922557960816363, 83.33224293864769550 ) ) ;
#75733=CARTESIAN_POINT ( 'NONE',  ( -9.564922557960796823, -16.46253265017161027, 82.08224293864768129 ) ) ;
#75734=CARTESIAN_POINT ( 'NONE',  ( -0.05219959533934338120, 16.53943276465976808, 47.50109039468568994 ) ) ;
#75735=CARTESIAN_POINT ( 'NONE',  ( -16.46253265017146816, -9.564922557961047289, 54.16775706135234003 ) ) ;
#75736=CARTESIAN_POINT ( 'NONE',  ( -5.719274019375665041, -21.55341960407619695, 59.79275706135234714 ) ) ;
#75737=CARTESIAN_POINT ( 'NONE',  ( -8.224510206698735004, -14.34966873604973081, 24.58442372801901499 ) ) ;
#75738=CARTESIAN_POINT ( 'NONE',  ( -5.049401038298153566, 19.05341960407611168, 70.20724293864769550 ) ) ;
#75739=CARTESIAN_POINT ( 'NONE',  ( 9.564922557961047289, -16.46253265017146816, 95.41775706135233293 ) ) ;
#75740=CARTESIAN_POINT ( 'NONE',  ( 12.06949235617739724, 12.14591786802326823, 56.87609039468568994 ) ) ;
#75741=CARTESIAN_POINT ( 'NONE',  ( -0.05219959533937732626, 21.53943276465977519, 102.5010903946856899 ) ) ;
#75742=CARTESIAN_POINT ( 'NONE',  ( 19.02544592524334988, 5.153800228976608722, 81.45942372801897591 ) ) ;
#75743=CARTESIAN_POINT ( 'NONE',  ( -16.46253265017160317, 9.564922557960807481, 45.83224293864769550 ) ) ;
#75744=CARTESIAN_POINT ( 'NONE',  ( 15.80617190586746368, 15.72974639402197994, 64.37390960531435269 ) ) ;
#75745=CARTESIAN_POINT ( 'NONE',  ( -8.314922557960811034, -14.29746914071050412, 77.08224293864769550 ) ) ;
#75746=CARTESIAN_POINT ( 'NONE',  ( -0.05219959533936034679, 19.03943276465977164, 72.50109039468566152 ) ) ;
#75747=CARTESIAN_POINT ( 'NONE',  ( 17.44270441346518652, -5.991230190322998972, 61.13664920735772768 ) ) ;
#75748=CARTESIAN_POINT ( 'NONE',  ( -9.474510206698720793, -16.51473224551083518, 49.58442372801899722 ) ) ;
#75749=CARTESIAN_POINT ( 'NONE',  ( 0.05219959533910956823, 16.53943276465976808, 24.99890960531435624 ) ) ;
#75750=CARTESIAN_POINT ( 'NONE',  ( -14.29746914071049879, 8.314922557960819915, 60.83224293864769550 ) ) ;
#75751=CARTESIAN_POINT ( 'NONE',  ( 18.62759615963255655, 10.81492255796105972, 96.66775706135234714 ) ) ;
#75753=CARTESIAN_POINT ( 'NONE',  ( -15.72974639402197994, 15.80617190586746368, 110.6239096053143669 ) ) ;
#75754=CARTESIAN_POINT ( 'NONE',  ( 19.05341960407611168, 5.049401038298154454, 68.95724293864769550 ) ) ;
#75755=CARTESIAN_POINT ( 'NONE',  ( -5.823673210054431948, 21.52544592524334988, 87.70942372801901854 ) ) ;
#75756=CARTESIAN_POINT ( 'NONE',  ( -9.474510206698964154, 16.51473224551069663, 65.41557627198102409 ) ) ;
#75758=CARTESIAN_POINT ( 'NONE',  ( 12.06949235617757843, -12.14591786802309237, 113.1239096053143953 ) ) ;
#75759=CARTESIAN_POINT ( 'NONE',  ( -5.719274019375978568, 21.55341960407610458, 35.20724293864768839 ) ) ;
#75760=CARTESIAN_POINT ( 'NONE',  ( 16.53943276465976808, -0.05219959533910856209, 73.74890960531433848 ) ) ;
#75761=CARTESIAN_POINT ( 'NONE',  ( 9.474510206698971260, -16.51473224551069308, 42.91557627198103120 ) ) ;
#75762=CARTESIAN_POINT ( 'NONE',  ( 8.314922557960818139, 14.29746914071049879, 94.58224293864769550 ) ) ;
#75764=CARTESIAN_POINT ( 'NONE',  ( -21.52544592524343514, 5.823673210054127303, 106.0405762719810525 ) ) ;
#75765=CARTESIAN_POINT ( 'NONE',  ( 10.81492255796106328, -18.62759615963255655, 45.41775706135234003 ) ) ;
#75766=CARTESIAN_POINT ( 'NONE',  ( -9.474510206698964154, 16.51473224551069663, 35.41557627198102409 ) ) ;
#75767=CARTESIAN_POINT ( 'NONE',  ( 14.34966873604972726, -8.224510206698740333, 45.83442372801901854 ) ) ;
#75768=CARTESIAN_POINT ( 'NONE',  ( 21.52544592524344225, -5.823673210054117533, 98.54057627198105251 ) ) ;
#75769=CARTESIAN_POINT ( 'NONE',  ( 15.72974639402199770, -15.80617190586745480, 98.12390960531436690 ) ) ;
#75770=CARTESIAN_POINT ( 'NONE',  ( 5.153800228976615827, -19.02544592524334988, 25.20942372801900433 ) ) ;
#75771=CARTESIAN_POINT ( 'NONE',  ( -13.97604488694527625, -13.89961937509977652, 51.87390960531436690 ) ) ;
#75772=CARTESIAN_POINT ( 'NONE',  ( 19.02544592524343514, -5.153800228976328945, 108.5405762719810383 ) ) ;
#75773=CARTESIAN_POINT ( 'NONE',  ( 5.719274019375673035, 21.55341960407619339, 52.29275706135236135 ) ) ;
#75774=CARTESIAN_POINT ( 'NONE',  ( 5.719274019375991003, -21.55341960407610458, 47.70724293864770260 ) ) ;
#75775=CARTESIAN_POINT ( 'NONE',  ( 16.52544592524335698, 4.483927247898782831, 111.4594237280190328 ) ) ;
#75776=CARTESIAN_POINT ( 'NONE',  ( -15.80617190586768217, 15.72974639402176855, 63.12609039468568994 ) ) ;
#75777=CARTESIAN_POINT ( 'NONE',  ( -15.72974639402176322, -15.80617190586768395, 94.37609039468568994 ) ) ;
#75778=CARTESIAN_POINT ( 'NONE',  ( -13.89961937509957401, -13.97604488694547875, 44.37609039468566863 ) ) ;
#75779=CARTESIAN_POINT ( 'NONE',  ( 4.483927247898790824, -16.52544592524335698, 105.2094237280190328 ) ) ;
#75780=CARTESIAN_POINT ( 'NONE',  ( 5.719274019375673035, 21.55341960407619339, 57.29275706135234714 ) ) ;
#75781=CARTESIAN_POINT ( 'NONE',  ( -16.46253265017160317, 9.564922557960807481, 55.83224293864769550 ) ) ;
#75782=CARTESIAN_POINT ( 'NONE',  ( 0.05219959533937995610, -21.53943276465977519, 110.0010903946856757 ) ) ;
#75783=CARTESIAN_POINT ( 'NONE',  ( -15.72974639402197994, 15.80617190586746368, 25.62390960531435624 ) ) ;
#75784=CARTESIAN_POINT ( 'NONE',  ( -21.52544592524343514, 5.823673210054127303, 111.0405762719810525 ) ) ;
#75785=CARTESIAN_POINT ( 'NONE',  ( 5.823673210054125526, 21.52544592524343514, 74.79057627198105251 ) ) ;
#75786=CARTESIAN_POINT ( 'NONE',  ( -14.29746914071037622, -8.314922557961029526, 44.16775706135234714 ) ) ;
#75788=CARTESIAN_POINT ( 'NONE',  ( 21.55341960407610458, 5.719274019375980345, 78.95724293864769550 ) ) ;
#75789=CARTESIAN_POINT ( 'NONE',  ( -14.34966873604972548, 8.224510206698743886, 68.33442372801900433 ) ) ;
#75790=CARTESIAN_POINT ( 'NONE',  ( -16.53943276465976808, 0.05219959533911058130, 71.24890960531435269 ) ) ;
#75792=CARTESIAN_POINT ( 'NONE',  ( -9.474510206698720793, -16.51473224551083518, 109.5844237280190043 ) ) ;
#75793=CARTESIAN_POINT ( 'NONE',  ( -10.72451020669898014, 18.67979575497178502, 40.41557627198103120 ) ) ;
#75794=CARTESIAN_POINT ( 'NONE',  ( 0.05219959533909260263, 19.03943276465977164, 94.99890960531436690 ) ) ;
#75795=CARTESIAN_POINT ( 'NONE',  ( 8.314922557961029526, -14.29746914071037800, 35.41775706135234003 ) ) ;
#75796=CARTESIAN_POINT ( 'NONE',  ( -10.72451020669898014, 18.67979575497178502, 105.4155762719810383 ) ) ;
#75797=CARTESIAN_POINT ( 'NONE',  ( -21.52544592524343514, 5.823673210054127303, 31.04057627198102409 ) ) ;
#75798=CARTESIAN_POINT ( 'NONE',  ( -4.379528057220086978, -16.55341960407618274, 64.79275706135234714 ) ) ;
#75799=CARTESIAN_POINT ( 'NONE',  ( 13.89961937509977652, -13.97604488694527269, 88.12390960531438111 ) ) ;
#75800=CARTESIAN_POINT ( 'NONE',  ( -18.67979575497193778, 10.72451020669871902, 58.33442372801901143 ) ) ;
#75801=CARTESIAN_POINT ( 'NONE',  ( 13.89961937509977652, -13.97604488694527269, 33.12390960531434558 ) ) ;
#75802=CARTESIAN_POINT ( 'NONE',  ( -15.72974639402197994, 15.80617190586746368, 30.62390960531436335 ) ) ;
#75804=CARTESIAN_POINT ( 'NONE',  ( -19.02544592524334988, -5.153800228976617603, 33.95942372801897591 ) ) ;
#75805=CARTESIAN_POINT ( 'NONE',  ( 16.53943276465976808, 0.05219959533934440121, 56.25109039468568284 ) ) ;
#75806=CARTESIAN_POINT ( 'NONE',  ( -16.51473224551069308, -9.474510206698971260, 101.6655762719810241 ) ) ;
#75807=CARTESIAN_POINT ( 'NONE',  ( -18.62759615963270932, 10.81492255796079327, 100.8322429386477097 ) ) ;
#75808=CARTESIAN_POINT ( 'NONE',  ( 16.46253265017160672, -9.564922557960803928, 68.33224293864770971 ) ) ;
#75809=CARTESIAN_POINT ( 'NONE',  ( -17.13100169013300444, 6.664070546373152659, 25.76789835699850073 ) ) ;
#75811=CARTESIAN_POINT ( 'NONE',  ( -14.34966873604960291, -8.224510206698953496, 86.66557627198102409 ) ) ;
#75812=CARTESIAN_POINT ( 'NONE',  ( -5.823673210054116645, -21.52544592524344225, 32.29057627198102409 ) ) ;
#75813=CARTESIAN_POINT ( 'NONE',  ( -16.31925111598457789, 7.325300261831451998, 35.16424538967250868 ) ) ;
#75814=CARTESIAN_POINT ( 'NONE',  ( -14.29746914071037622, -8.314922557961029526, 69.16775706135234714 ) ) ;
#75815=CARTESIAN_POINT ( 'NONE',  ( -5.719274019375978568, 21.55341960407610458, 115.2072429386476955 ) ) ;
#75816=CARTESIAN_POINT ( 'NONE',  ( 9.564922557961047289, -16.46253265017146816, 75.41775706135234714 ) ) ;
#75817=CARTESIAN_POINT ( 'NONE',  ( -9.564922557960796823, -16.46253265017161027, 37.08224293864768839 ) ) ;
#75818=CARTESIAN_POINT ( 'NONE',  ( 21.55341960407610458, 5.719274019375980345, 63.95724293864770260 ) ) ;
#75819=CARTESIAN_POINT ( 'NONE',  ( -0.05219959533909027116, -19.03943276465977164, 97.49890960531436690 ) ) ;
#75820=CARTESIAN_POINT ( 'NONE',  ( 15.72974639402176855, 15.80617190586768217, 96.87609039468568994 ) ) ;
#75821=CARTESIAN_POINT ( 'NONE',  ( -19.02544592524342804, 5.153800228976336051, 66.04057627198103830 ) ) ;
#75823=CARTESIAN_POINT ( 'NONE',  ( -14.29746914071037622, -8.314922557961029526, 44.16775706135234714 ) ) ;
#75824=CARTESIAN_POINT ( 'NONE',  ( 19.03943276465977164, -0.05219959533909143690, 53.74890960531436690 ) ) ;
#75825=CARTESIAN_POINT ( 'NONE',  ( 0.05219959533937995610, -21.53943276465977519, 75.00109039468568994 ) ) ;
#75826=CARTESIAN_POINT ( 'NONE',  ( -9.564922557961040184, 16.46253265017147172, 42.91775706135234003 ) ) ;
#75827=CARTESIAN_POINT ( 'NONE',  ( -16.46253265017146816, -9.564922557961047289, 54.16775706135234003 ) ) ;
#75828=CARTESIAN_POINT ( 'NONE',  ( 5.823673210054444382, -21.52544592524334988, 50.20942372801901854 ) ) ;
#75830=CARTESIAN_POINT ( 'NONE',  ( -13.97604488694547697, 13.89961937509957934, 48.12609039468566863 ) ) ;
#75831=CARTESIAN_POINT ( 'NONE',  ( -5.153800228976328057, -19.02544592524343514, 102.2905762719810383 ) ) ;
#75832=CARTESIAN_POINT ( 'NONE',  ( -13.89961937509977652, 13.97604488694528158, 75.62390960531438111 ) ) ;
#75833=CARTESIAN_POINT ( 'NONE',  ( 0.05219959533910956823, 16.53943276465976808, 29.99890960531435979 ) ) ;
#75834=CARTESIAN_POINT ( 'NONE',  ( -18.62759615963270932, 10.81492255796079327, 30.83224293864770260 ) ) ;
#75835=CARTESIAN_POINT ( 'NONE',  ( 18.62759615963255655, 10.81492255796105972, 101.6677570613523613 ) ) ;
#75838=CARTESIAN_POINT ( 'NONE',  ( -5.719274019375665041, -21.55341960407619695, 99.79275706135234714 ) ) ;
#75841=CARTESIAN_POINT ( 'NONE',  ( 5.049401038298161559, -19.05341960407611168, 27.70724293864769550 ) ) ;
#75842=CARTESIAN_POINT ( 'NONE',  ( -13.97604488694527625, -13.89961937509977652, 111.8739096053143243 ) ) ;
#75845=CARTESIAN_POINT ( 'NONE',  ( -8.314922557961024197, 14.29746914071037800, 52.91775706135235424 ) ) ;
#75846=CARTESIAN_POINT ( 'NONE',  ( -5.719274019375978568, 21.55341960407610458, 70.20724293864769550 ) ) ;
#75847=CARTESIAN_POINT ( 'NONE',  ( -12.14591786802309592, -12.06949235617757132, 41.87390960531435979 ) ) ;
#75848=CARTESIAN_POINT ( 'NONE',  ( 4.379528057220339221, -16.55341960407611168, 112.7072429386476955 ) ) ;
#75849=CARTESIAN_POINT ( 'NONE',  ( 13.89961937509977652, -13.97604488694527269, 113.1239096053143527 ) ) ;
#75850=CARTESIAN_POINT ( 'NONE',  ( 16.46253265017146816, 9.564922557961045513, 41.66775706135234003 ) ) ;
#75851=CARTESIAN_POINT ( 'NONE',  ( 14.29746914071049879, -8.314922557960816363, 113.3322429386476955 ) ) ;
#75852=CARTESIAN_POINT ( 'NONE',  ( -10.81492255796105439, 18.62759615963255655, 67.91775706135234714 ) ) ;
#75854=CARTESIAN_POINT ( 'NONE',  ( 0.05219959533910956823, 16.53943276465976808, 24.99890960531435624 ) ) ;
#75856=CARTESIAN_POINT ( 'NONE',  ( 21.53943276465977519, -0.05219959533907433946, 28.74890960531435624 ) ) ;
#75857=CARTESIAN_POINT ( 'NONE',  ( 16.55341960407611168, 4.379528057220329451, 83.95724293864770971 ) ) ;
#75860=CARTESIAN_POINT ( 'NONE',  ( -13.97604488694527625, -13.89961937509977652, 81.87390960531436690 ) ) ;
#75861=CARTESIAN_POINT ( 'NONE',  ( 14.34966873604960469, 8.224510206698951720, 69.16557627198102409 ) ) ;
#75862=CARTESIAN_POINT ( 'NONE',  ( 9.564922557961047289, -16.46253265017146816, 105.4177570613523471 ) ) ;
#75863=CARTESIAN_POINT ( 'NONE',  ( -15.72974639402197994, 15.80617190586746368, 50.62390960531435979 ) ) ;
#75865=CARTESIAN_POINT ( 'NONE',  ( 16.53943276465976808, -0.05219959533910856209, 108.7489096053143669 ) ) ;
#75866=CARTESIAN_POINT ( 'NONE',  ( -19.05341960407611168, -5.049401038298163336, 76.45724293864769550 ) ) ;
#75867=CARTESIAN_POINT ( 'NONE',  ( -21.55341960407610458, -5.719274019375992779, 76.45724293864769550 ) ) ;
#75868=CARTESIAN_POINT ( 'NONE',  ( -16.55341960407617563, 4.379528057220093196, 103.5427570613523613 ) ) ;
#75869=CARTESIAN_POINT ( 'NONE',  ( -19.05341960407611168, -5.049401038298163336, 81.45724293864769550 ) ) ;
#75870=CARTESIAN_POINT ( 'NONE',  ( 19.03943276465977164, 0.05219959533936151252, 66.25109039468567573 ) ) ;
#75871=CARTESIAN_POINT ( 'NONE',  ( 0.05219959533937995610, -21.53943276465977519, 90.00109039468567573 ) ) ;
#75872=CARTESIAN_POINT ( 'NONE',  ( 15.80617190586746368, 15.72974639402197994, 69.37390960531436690 ) ) ;
#75873=CARTESIAN_POINT ( 'NONE',  ( 15.80617190586746368, 15.72974639402197994, 29.37390960531435269 ) ) ;
#75874=CARTESIAN_POINT ( 'NONE',  ( -5.049401038298153566, 19.05341960407611168, 35.20724293864768839 ) ) ;
#75875=CARTESIAN_POINT ( 'NONE',  ( -16.53943276465976808, -0.05219959533934237506, 103.7510903946857042 ) ) ;
#75876=CARTESIAN_POINT ( 'NONE',  ( 13.97604488694527802, 13.89961937509977652, 59.37390960531434558 ) ) ;
#75877=CARTESIAN_POINT ( 'NONE',  ( 8.224510206698742110, 14.34966873604972548, 22.08442372801901143 ) ) ;
#75879=CARTESIAN_POINT ( 'NONE',  ( -15.80617190586768217, 15.72974639402176855, 108.1260903946856757 ) ) ;
#75880=CARTESIAN_POINT ( 'NONE',  ( -16.55341960407611168, -4.379528057220339221, 76.45724293864769550 ) ) ;
#75882=CARTESIAN_POINT ( 'NONE',  ( 15.80617190586746368, 15.72974639402197994, 114.3739096053143527 ) ) ;
#75883=CARTESIAN_POINT ( 'NONE',  ( -0.05219959533907301413, -21.53943276465977519, 107.4989096053143669 ) ) ;
#75885=CARTESIAN_POINT ( 'NONE',  ( 5.823673210054125526, 21.52544592524343514, 39.79057627198103830 ) ) ;
#75886=CARTESIAN_POINT ( 'NONE',  ( -4.483927247898782831, 16.52544592524335698, 82.70942372801900433 ) ) ;
#75887=CARTESIAN_POINT ( 'NONE',  ( 8.314922557960818139, 14.29746914071049879, 99.58224293864770971 ) ) ;
#75888=CARTESIAN_POINT ( 'NONE',  ( -16.51473224551069308, -9.474510206698971260, 56.66557627198103120 ) ) ;
#75890=CARTESIAN_POINT ( 'NONE',  ( -0.05219959533910754901, -16.53943276465976808, 22.49890960531436335 ) ) ;
#75892=CARTESIAN_POINT ( 'NONE',  ( 18.62759615963255655, 10.81492255796105972, 41.66775706135235424 ) ) ;
#75893=CARTESIAN_POINT ( 'NONE',  ( 5.153800228976335163, 19.02544592524342804, 94.79057627198103830 ) ) ;
#75894=CARTESIAN_POINT ( 'NONE',  ( 15.72974639402176855, 15.80617190586768217, 76.87609039468567573 ) ) ;
#75895=CARTESIAN_POINT ( 'NONE',  ( 0.05219959533909260263, 19.03943276465977164, 34.99890960531435979 ) ) ;
#75896=CARTESIAN_POINT ( 'NONE',  ( -19.05341960407611168, -5.049401038298163336, 21.45724293864768839 ) ) ;
#75899=CARTESIAN_POINT ( 'NONE',  ( 15.80617190586769283, -15.72974639402175789, 70.62609039468567573 ) ) ;
#75900=CARTESIAN_POINT ( 'NONE',  ( -16.51473224551069308, -9.474510206698971260, 101.6655762719810241 ) ) ;
#75901=CARTESIAN_POINT ( 'NONE',  ( -19.02544592524334988, -5.153800228976617603, 73.95942372801900433 ) ) ;
#75902=CARTESIAN_POINT ( 'NONE',  ( -0.05219959533937732626, 21.53943276465977519, 47.50109039468568994 ) ) ;
#75903=CARTESIAN_POINT ( 'NONE',  ( -8.224510206698735004, -14.34966873604973081, 19.58442372801901143 ) ) ;
#75904=CARTESIAN_POINT ( 'NONE',  ( 19.02544592524334988, 5.153800228976608722, 66.45942372801899012 ) ) ;
#75905=CARTESIAN_POINT ( 'NONE',  ( 0.05219959533909260263, 19.03943276465977164, 39.99890960531436690 ) ) ;
#75906=CARTESIAN_POINT ( 'NONE',  ( -9.564922557961040184, 16.46253265017147172, 87.91775706135233293 ) ) ;
#75907=AXIS2_PLACEMENT_3D ( 'NONE', #22129, #145459, #188254 ) ;
#75908=CARTESIAN_POINT ( 'NONE',  ( 12.06949235617757843, -12.14591786802309237, 23.12390960531436335 ) ) ;
#75909=CARTESIAN_POINT ( 'NONE',  ( 5.049401038297881783, 19.05341960407617563, 82.29275706135229029 ) ) ;
#75910=CARTESIAN_POINT ( 'NONE',  ( 14.34966873604960469, 8.224510206698951720, 34.16557627198102409 ) ) ;
#75911=CARTESIAN_POINT ( 'NONE',  ( 19.03943276465977164, 0.05219959533936151252, 66.25109039468567573 ) ) ;
#75912=CARTESIAN_POINT ( 'NONE',  ( -21.52544592524334988, -5.823673210054445271, 108.9594237280190185 ) ) ;
#75913=CARTESIAN_POINT ( 'NONE',  ( 9.564922557961047289, -16.46253265017146816, 30.41775706135232937 ) ) ;
#75914=CARTESIAN_POINT ( 'NONE',  ( 19.05341960407611168, 5.049401038298154454, 28.95724293864769550 ) ) ;
#75915=CARTESIAN_POINT ( 'NONE',  ( -16.88567814943164436, -6.947325034625593254, 66.29001122652586275 ) ) ;
#75916=CARTESIAN_POINT ( 'NONE',  ( -4.483927247898782831, 16.52544592524335698, 47.70942372801902565 ) ) ;
#75919=CARTESIAN_POINT ( 'NONE',  ( 9.474510206698971260, -16.51473224551069308, 87.91557627198102409 ) ) ;
#75922=CARTESIAN_POINT ( 'NONE',  ( -13.89961937509957401, -13.97604488694547875, 89.37609039468563310 ) ) ;
#75923=CARTESIAN_POINT ( 'NONE',  ( -10.72451020669898014, 18.67979575497178502, 25.41557627198103120 ) ) ;
#75924=CARTESIAN_POINT ( 'NONE',  ( 13.97604488694548053, -13.89961937509957401, 20.62609039468567573 ) ) ;
#75925=CARTESIAN_POINT ( 'NONE',  ( -0.05219959533936034679, 19.03943276465977164, 102.5010903946856757 ) ) ;
#75926=CARTESIAN_POINT ( 'NONE',  ( 8.224510206698953496, -14.34966873604960469, 107.9155762719810241 ) ) ;
#75927=CARTESIAN_POINT ( 'NONE',  ( 5.153800228976335163, 19.02544592524342804, 29.79057627198102409 ) ) ;
#75928=CARTESIAN_POINT ( 'NONE',  ( -10.81492255796078084, -18.62759615963271287, 57.08224293864769550 ) ) ;
#75929=CARTESIAN_POINT ( 'NONE',  ( -18.67979575497178146, -10.72451020669898902, 46.66557627198102409 ) ) ;
#75930=CARTESIAN_POINT ( 'NONE',  ( -5.049401038298153566, 19.05341960407611168, 25.20724293864768484 ) ) ;
#75932=CARTESIAN_POINT ( 'NONE',  ( -5.049401038297874678, -19.05341960407617918, 74.79275706135231871 ) ) ;
#75933=CARTESIAN_POINT ( 'NONE',  ( -8.314922557960811034, -14.29746914071050412, 37.08224293864768129 ) ) ;
#75934=CARTESIAN_POINT ( 'NONE',  ( -15.80617190586745835, -15.72974639402198527, 21.87390960531436690 ) ) ;
#75935=CARTESIAN_POINT ( 'NONE',  ( -10.72451020669870658, -18.67979575497194134, 89.58442372801901854 ) ) ;
#75936=CARTESIAN_POINT ( 'NONE',  ( -15.72974639402197994, 15.80617190586746368, 80.62390960531438111 ) ) ;
#75937=CARTESIAN_POINT ( 'NONE',  ( 18.62759615963255655, 10.81492255796105972, 56.66775706135235424 ) ) ;
#75938=CARTESIAN_POINT ( 'NONE',  ( -10.81492255796105439, 18.62759615963255655, 67.91775706135234714 ) ) ;
#75939=CARTESIAN_POINT ( 'NONE',  ( 13.89961937509977652, -13.97604488694527269, 98.12390960531433848 ) ) ;
#75940=CARTESIAN_POINT ( 'NONE',  ( -16.53943276465976808, -0.05219959533934237506, 93.75109039468567573 ) ) ;
#75941=CARTESIAN_POINT ( 'NONE',  ( -21.53943276465977519, -0.05219959533937600094, 53.75109039468568994 ) ) ;
#75942=CARTESIAN_POINT ( 'NONE',  ( -19.02544592524342804, 5.153800228976336051, 26.04057627198103120 ) ) ;
#75945=CARTESIAN_POINT ( 'NONE',  ( -12.06949235617756955, 12.14591786802309770, 65.62390960531436690 ) ) ;
#75946=CARTESIAN_POINT ( 'NONE',  ( -8.224510206698948167, 14.34966873604960824, 35.41557627198102409 ) ) ;
#75947=CARTESIAN_POINT ( 'NONE',  ( 13.97604488694527802, 13.89961937509977652, 69.37390960531436690 ) ) ;
#75948=CARTESIAN_POINT ( 'NONE',  ( 16.51473224551069308, 9.474510206698969483, 54.16557627198103120 ) ) ;
#75949=CARTESIAN_POINT ( 'NONE',  ( 5.823673210054125526, 21.52544592524343514, 54.79057627198104541 ) ) ;
#75950=CARTESIAN_POINT ( 'NONE',  ( 9.474510206698729675, 16.51473224551082808, 37.08442372801899722 ) ) ;
#75952=CARTESIAN_POINT ( 'NONE',  ( 14.29746914071049879, -8.314922557960816363, 53.33224293864769550 ) ) ;
#75953=CARTESIAN_POINT ( 'NONE',  ( -9.474510206698964154, 16.51473224551069663, 115.4155762719810241 ) ) ;
#75956=CARTESIAN_POINT ( 'NONE',  ( 16.55341960407618274, -4.379528057220086978, 66.04275706135236135 ) ) ;
#75957=CARTESIAN_POINT ( 'NONE',  ( 0.05219959533936267826, -19.03943276465977164, 80.00109039468567573 ) ) ;
#75958=CARTESIAN_POINT ( 'NONE',  ( 16.55341960407611168, 4.379528057220329451, 43.95724293864769550 ) ) ;
#75960=CARTESIAN_POINT ( 'NONE',  ( -16.55341960407617563, 4.379528057220093196, 113.5427570613523756 ) ) ;
#75961=CARTESIAN_POINT ( 'NONE',  ( 9.564922557960805705, 16.46253265017160317, 54.58224293864769550 ) ) ;
#75963=CARTESIAN_POINT ( 'NONE',  ( -5.049401038298153566, 19.05341960407611168, 75.20724293864769550 ) ) ;
#75964=CARTESIAN_POINT ( 'NONE',  ( -16.46253265017160317, 9.564922557960807481, 45.83224293864769550 ) ) ;
#75965=CARTESIAN_POINT ( 'NONE',  ( -10.81492255796105439, 18.62759615963255655, 47.91775706135234714 ) ) ;
#75966=CARTESIAN_POINT ( 'NONE',  ( 19.02544592524343514, -5.153800228976328945, 53.54057627198102409 ) ) ;
#75968=CARTESIAN_POINT ( 'NONE',  ( 9.474510206698971260, -16.51473224551069308, 62.91557627198102409 ) ) ;
#75969=CARTESIAN_POINT ( 'NONE',  ( -21.52544592524343514, 5.823673210054127303, 36.04057627198102409 ) ) ;
#75970=CARTESIAN_POINT ( 'NONE',  ( 13.97604488694527802, 13.89961937509977652, 24.37390960531435624 ) ) ;
#75971=CARTESIAN_POINT ( 'NONE',  ( 21.53943276465977519, -0.05219959533907433946, 28.74890960531435624 ) ) ;
#75972=CARTESIAN_POINT ( 'NONE',  ( -14.29746914071037622, -8.314922557961029526, 94.16775706135237556 ) ) ;
#75973=CARTESIAN_POINT ( 'NONE',  ( -18.62759615963255300, -10.81492255796106328, 104.1677570613523471 ) ) ;
#75974=CARTESIAN_POINT ( 'NONE',  ( 16.52544592524335698, 4.483927247898782831, 61.45942372801901854 ) ) ;
#75975=CARTESIAN_POINT ( 'NONE',  ( -19.02544592524342804, 5.153800228976336051, 106.0405762719810241 ) ) ;
#75976=CARTESIAN_POINT ( 'NONE',  ( 4.379528057220092307, 16.55341960407617563, 52.29275706135236135 ) ) ;
#75977=CARTESIAN_POINT ( 'NONE',  ( -8.314922557961024197, 14.29746914071037800, 42.91775706135235424 ) ) ;
#75978=CARTESIAN_POINT ( 'NONE',  ( 9.564922557960805705, 16.46253265017160317, 109.5822429386476955 ) ) ;
#75979=CARTESIAN_POINT ( 'NONE',  ( 16.55341960407618274, -4.379528057220086978, 26.04275706135235779 ) ) ;
#75980=CARTESIAN_POINT ( 'NONE',  ( -9.564922557960796823, -16.46253265017161027, 32.08224293864769550 ) ) ;
#75981=CARTESIAN_POINT ( 'NONE',  ( -15.72974639402197994, 15.80617190586746368, 105.6239096053143669 ) ) ;
#75982=CARTESIAN_POINT ( 'NONE',  ( -16.52544592524335698, -4.483927247898792601, 18.95942372801901143 ) ) ;
#75983=CARTESIAN_POINT ( 'NONE',  ( 12.14591786802327356, -12.06949235617739191, 85.62609039468568994 ) ) ;
#75984=CARTESIAN_POINT ( 'NONE',  ( -17.40805194821984259, 6.112264579160790134, 45.83371272510608918 ) ) ;
#75985=CARTESIAN_POINT ( 'NONE',  ( -10.72451020669870658, -18.67979575497194134, 89.58442372801901854 ) ) ;
#75986=CARTESIAN_POINT ( 'NONE',  ( -9.474510206698720793, -16.51473224551083518, 79.58442372801899012 ) ) ;
#75987=CARTESIAN_POINT ( 'NONE',  ( -12.06949235617756955, 12.14591786802309770, 60.62390960531437401 ) ) ;
#75988=CARTESIAN_POINT ( 'NONE',  ( 8.314922557960818139, 14.29746914071049879, 104.5822429386477097 ) ) ;
#75989=CARTESIAN_POINT ( 'NONE',  ( 5.049401038297881783, 19.05341960407617563, 52.29275706135234003 ) ) ;
#75990=CARTESIAN_POINT ( 'NONE',  ( 17.50000000000001421, -5.622605283950835364, 56.18792689403892382 ) ) ;
#75991=CARTESIAN_POINT ( 'NONE',  ( -21.55341960407619339, 5.719274019375674811, 53.54275706135234714 ) ) ;
#75992=CARTESIAN_POINT ( 'NONE',  ( -16.46253265017146816, -9.564922557961047289, 104.1677570613523329 ) ) ;
#75993=CARTESIAN_POINT ( 'NONE',  ( -17.49999999999999645, 5.499999999999997335, 120.0000000000000142 ) ) ;
#75994=CARTESIAN_POINT ( 'NONE',  ( -19.03943276465977164, 0.05219959533909376836, 106.2489096053143669 ) ) ;
#75995=CARTESIAN_POINT ( 'NONE',  ( -5.823673210054116645, -21.52544592524344225, 72.29057627198102409 ) ) ;
#75996=CARTESIAN_POINT ( 'NONE',  ( -16.51473224551082808, 9.474510206698731452, 93.33442372801900433 ) ) ;
#75997=CARTESIAN_POINT ( 'NONE',  ( -9.474510206698964154, 16.51473224551069663, 105.4155762719810383 ) ) ;
#75998=CARTESIAN_POINT ( 'NONE',  ( -18.22780087662126647, -5.499999999999827693, 48.98236817873107185 ) ) ;
#75999=CARTESIAN_POINT ( 'NONE',  ( 16.55341960407611168, 4.379528057220329451, 108.9572429386476955 ) ) ;
#76000=CARTESIAN_POINT ( 'NONE',  ( 15.80617190586769283, -15.72974639402175789, 90.62609039468567573 ) ) ;
#76001=CARTESIAN_POINT ( 'NONE',  ( -19.02544592524342804, 5.153800228976336051, 41.04057627198103120 ) ) ;
#76003=CARTESIAN_POINT ( 'NONE',  ( 5.719274019375673035, 21.55341960407619339, 57.29275706135234714 ) ) ;
#76004=CARTESIAN_POINT ( 'NONE',  ( -15.72974639402176322, -15.80617190586768395, 89.37609039468568994 ) ) ;
#76005=CARTESIAN_POINT ( 'NONE',  ( 0.05219959533934541429, -16.53943276465976808, 95.00109039468568994 ) ) ;
#76006=CARTESIAN_POINT ( 'NONE',  ( 15.72974639402176855, 15.80617190586768217, 41.87609039468568284 ) ) ;
#76007=CARTESIAN_POINT ( 'NONE',  ( -18.67979575497193778, 10.72451020669871902, 43.33442372801901143 ) ) ;
#76008=CARTESIAN_POINT ( 'NONE',  ( 13.97604488694548053, -13.89961937509957401, 65.62609039468567573 ) ) ;
#76009=CARTESIAN_POINT ( 'NONE',  ( -9.474510206698964154, 16.51473224551069663, 95.41557627198102409 ) ) ;
#76010=CARTESIAN_POINT ( 'NONE',  ( 12.14591786802309770, 12.06949235617756955, 104.3739096053143669 ) ) ;
#76011=CARTESIAN_POINT ( 'NONE',  ( -10.81492255796078084, -18.62759615963271287, 82.08224293864768129 ) ) ;
#76012=CARTESIAN_POINT ( 'NONE',  ( 8.224510206698953496, -14.34966873604960469, 67.91557627198102409 ) ) ;
#76013=CARTESIAN_POINT ( 'NONE',  ( -18.62759615963255300, -10.81492255796106328, 99.16775706135234714 ) ) ;
#76014=CARTESIAN_POINT ( 'NONE',  ( 16.52544592524342804, -4.483927247898539470, 78.54057627198103830 ) ) ;
#76015=CARTESIAN_POINT ( 'NONE',  ( -16.46253265017160317, 9.564922557960807481, 40.83224293864769550 ) ) ;
#76016=CARTESIAN_POINT ( 'NONE',  ( -19.02544592524334988, -5.153800228976617603, 83.95942372801901854 ) ) ;
#76017=CARTESIAN_POINT ( 'NONE',  ( -12.06949235617756955, 12.14591786802309770, 50.62390960531435979 ) ) ;
#76018=CARTESIAN_POINT ( 'NONE',  ( -21.53943276465977519, -0.05219959533937600094, 93.75109039468567573 ) ) ;
#76019=CARTESIAN_POINT ( 'NONE',  ( -16.46253265017160317, 9.564922557960807481, 85.83224293864769550 ) ) ;
#76020=CARTESIAN_POINT ( 'NONE',  ( 16.46253265017146816, 9.564922557961045513, 61.66775706135234003 ) ) ;
#76021=CARTESIAN_POINT ( 'NONE',  ( 18.67979575497178502, 10.72451020669898547, 69.16557627198102409 ) ) ;
#76022=CARTESIAN_POINT ( 'NONE',  ( -18.62759615963255300, -10.81492255796106328, 24.16775706135235424 ) ) ;
#76023=CARTESIAN_POINT ( 'NONE',  ( 4.379528057220092307, 16.55341960407617563, 27.29275706135234358 ) ) ;
#76024=CARTESIAN_POINT ( 'NONE',  ( -16.55341960407617563, 4.379528057220093196, 73.54275706135234714 ) ) ;
#76025=CARTESIAN_POINT ( 'NONE',  ( -0.05219959533909027116, -19.03943276465977164, 27.49890960531435624 ) ) ;
#76026=CARTESIAN_POINT ( 'NONE',  ( 18.67979575497178502, 10.72451020669898547, 114.1655762719810383 ) ) ;
#76027=CARTESIAN_POINT ( 'NONE',  ( -8.314922557960811034, -14.29746914071050412, 112.0822429386477097 ) ) ;
#76029=CARTESIAN_POINT ( 'NONE',  ( 16.52544592524335698, 4.483927247898782831, 51.45942372801901854 ) ) ;
#76030=CARTESIAN_POINT ( 'NONE',  ( 16.53943276465976808, -0.05219959533910856209, 73.74890960531433848 ) ) ;
#76031=CARTESIAN_POINT ( 'NONE',  ( -0.05219959533907301413, -21.53943276465977519, 77.49890960531433848 ) ) ;
#76033=CARTESIAN_POINT ( 'NONE',  ( -16.55341960407611168, -4.379528057220339221, 21.45724293864769550 ) ) ;
#76034=CARTESIAN_POINT ( 'NONE',  ( 14.34966873604972726, -8.224510206698740333, 40.83442372801901854 ) ) ;
#76035=CARTESIAN_POINT ( 'NONE',  ( -0.05219959533909027116, -19.03943276465977164, 42.49890960531435269 ) ) ;
#76036=CARTESIAN_POINT ( 'NONE',  ( -8.224510206698735004, -14.34966873604973081, 79.58442372801903275 ) ) ;
#76037=CARTESIAN_POINT ( 'NONE',  ( -5.153800228976607833, 19.02544592524334988, 72.70942372801900433 ) ) ;
#76038=CARTESIAN_POINT ( 'NONE',  ( -21.52544592524343514, 5.823673210054127303, 76.04057627198102409 ) ) ;
#76039=CARTESIAN_POINT ( 'NONE',  ( -16.53943276465976808, -0.05219959533934237506, 113.7510903946856757 ) ) ;
#76042=CARTESIAN_POINT ( 'NONE',  ( 0.05219959533907565091, 21.53943276465977519, 44.99890960531435979 ) ) ;
#76044=CARTESIAN_POINT ( 'NONE',  ( 14.29746914071037800, 8.314922557961029526, 96.66775706135234714 ) ) ;
#76046=CARTESIAN_POINT ( 'NONE',  ( 9.564922557960805705, 16.46253265017160317, 114.5822429386476955 ) ) ;
#76048=CARTESIAN_POINT ( 'NONE',  ( 0.05219959533907565091, 21.53943276465977519, 74.99890960531435269 ) ) ;
#76049=CARTESIAN_POINT ( 'NONE',  ( 8.224510206698742110, 14.34966873604972548, 107.0844237280190043 ) ) ;
#76050=CARTESIAN_POINT ( 'NONE',  ( 5.719274019375673035, 21.55341960407619339, 57.29275706135234714 ) ) ;
#76051=CARTESIAN_POINT ( 'NONE',  ( -9.564922557961040184, 16.46253265017147172, 112.9177570613523329 ) ) ;
#76052=CARTESIAN_POINT ( 'NONE',  ( 9.474510206698971260, -16.51473224551069308, 22.91557627198102765 ) ) ;
#76053=CARTESIAN_POINT ( 'NONE',  ( -14.34966873604972548, 8.224510206698743886, 23.33442372801901499 ) ) ;
#76054=CARTESIAN_POINT ( 'NONE',  ( -19.03943276465977164, 0.05219959533909376836, 56.24890960531435979 ) ) ;
#76056=CARTESIAN_POINT ( 'NONE',  ( -0.05219959533909027116, -19.03943276465977164, 107.4989096053143527 ) ) ;
#76058=CARTESIAN_POINT ( 'NONE',  ( 12.06949235617739724, 12.14591786802326823, 91.87609039468568994 ) ) ;
#76059=CARTESIAN_POINT ( 'NONE',  ( -19.03943276465977164, -0.05219959533935918106, 93.75109039468566152 ) ) ;
#76060=CARTESIAN_POINT ( 'NONE',  ( -5.049401038297874678, -19.05341960407617918, 24.79275706135233648 ) ) ;
#76061=CARTESIAN_POINT ( 'NONE',  ( 15.80617190586746368, 15.72974639402197994, 69.37390960531436690 ) ) ;
#76062=CARTESIAN_POINT ( 'NONE',  ( 12.06949235617739724, 12.14591786802326823, 96.87609039468568994 ) ) ;
#76063=CARTESIAN_POINT ( 'NONE',  ( 13.89961937509957401, 13.97604488694547697, 96.87609039468566152 ) ) ;
#76064=CARTESIAN_POINT ( 'NONE',  ( 0.05219959533909260263, 19.03943276465977164, 54.99890960531435979 ) ) ;
#76065=CARTESIAN_POINT ( 'NONE',  ( 13.97604488694527802, 13.89961937509977652, 94.37390960531436690 ) ) ;
#76066=CARTESIAN_POINT ( 'NONE',  ( -5.823673210054431948, 21.52544592524334988, 52.70942372801902565 ) ) ;
#76067=CARTESIAN_POINT ( 'NONE',  ( -19.05341960407611168, -5.049401038298163336, 46.45724293864768129 ) ) ;
#76068=CARTESIAN_POINT ( 'NONE',  ( -12.06949235617756955, 12.14591786802309770, 65.62390960531436690 ) ) ;
#76069=CARTESIAN_POINT ( 'NONE',  ( -18.62759615963270932, 10.81492255796079327, 75.83224293864769550 ) ) ;
#76071=CARTESIAN_POINT ( 'NONE',  ( 13.89961937509957401, 13.97604488694547697, 46.87609039468565442 ) ) ;
#76073=CARTESIAN_POINT ( 'NONE',  ( 16.46253265017160672, -9.564922557960803928, 73.33224293864769550 ) ) ;
#76074=CARTESIAN_POINT ( 'NONE',  ( -13.89961937509977652, 13.97604488694528158, 90.62390960531432427 ) ) ;
#76075=CARTESIAN_POINT ( 'NONE',  ( -4.483927247898782831, 16.52544592524335698, 57.70942372801901143 ) ) ;
#76077=CARTESIAN_POINT ( 'NONE',  ( 19.03943276465977164, 0.05219959533936151252, 36.25109039468567573 ) ) ;
#76078=CARTESIAN_POINT ( 'NONE',  ( 18.22780087662123805, -5.499999999999976019, 93.51763182126896368 ) ) ;
#76079=CARTESIAN_POINT ( 'NONE',  ( -8.314922557961024197, 14.29746914071037800, 92.91775706135236135 ) ) ;
#76081=CARTESIAN_POINT ( 'NONE',  ( -16.53943276465976808, -0.05219959533934237506, 78.75109039468568994 ) ) ;
#76082=CARTESIAN_POINT ( 'NONE',  ( 16.53943276465976808, 0.05219959533934440121, 56.25109039468568284 ) ) ;
#76083=CARTESIAN_POINT ( 'NONE',  ( 19.02544592524343514, -5.153800228976328945, 53.54057627198102409 ) ) ;
#76084=CARTESIAN_POINT ( 'NONE',  ( -13.89961937509977830, 13.97604488694528158, 75.62390960531436690 ) ) ;
#76085=CARTESIAN_POINT ( 'NONE',  ( -10.81492255796105439, 18.62759615963255655, 62.91775706135236135 ) ) ;
#76086=CARTESIAN_POINT ( 'NONE',  ( -13.89961937509957401, -13.97604488694547875, 74.37609039468566152 ) ) ;
#76087=CARTESIAN_POINT ( 'NONE',  ( 18.62759615963255655, 10.81492255796105972, 111.6677570613523613 ) ) ;
#76089=CARTESIAN_POINT ( 'NONE',  ( 9.474510206698971260, -16.51473224551069308, 57.91557627198103120 ) ) ;
#76090=CARTESIAN_POINT ( 'NONE',  ( -0.05219959533909027116, -19.03943276465977164, 37.49890960531436690 ) ) ;
#76092=CARTESIAN_POINT ( 'NONE',  ( -10.81492255796078084, -18.62759615963271287, 72.08224293864769550 ) ) ;
#76093=CARTESIAN_POINT ( 'NONE',  ( -13.89961937509977652, 13.97604488694528158, 110.6239096053143243 ) ) ;
#76094=CARTESIAN_POINT ( 'NONE',  ( 16.52544592524342804, -4.483927247898539470, 113.5405762719810383 ) ) ;
#76095=CARTESIAN_POINT ( 'NONE',  ( 0.05219959533934541429, -16.53943276465976808, 45.00109039468568284 ) ) ;
#76096=CARTESIAN_POINT ( 'NONE',  ( 8.314922557960818139, 14.29746914071049879, 34.58224293864770260 ) ) ;
#76097=ORIENTED_EDGE ( 'NONE', *, *, #125462, .T. ) ;
#76098=CARTESIAN_POINT ( 'NONE',  ( -5.719274019375978568, 21.55341960407610458, 110.2072429386477239 ) ) ;
#76099=CARTESIAN_POINT ( 'NONE',  ( 0.05219959533910956823, 16.53943276465976808, 49.99890960531437401 ) ) ;
#76101=CARTESIAN_POINT ( 'NONE',  ( -19.03943276465977164, -0.05219959533935918106, 113.7510903946856757 ) ) ;
#76102=CARTESIAN_POINT ( 'NONE',  ( -16.51473224551082808, 9.474510206698731452, 38.33442372801899722 ) ) ;
#76103=CARTESIAN_POINT ( 'NONE',  ( -12.06949235617756955, 12.14591786802309770, 45.62390960531436690 ) ) ;
#76104=CARTESIAN_POINT ( 'NONE',  ( -15.72974639402197994, 15.80617190586746368, 105.6239096053143669 ) ) ;
#76106=CARTESIAN_POINT ( 'NONE',  ( 5.719274019375991003, -21.55341960407610458, 57.70724293864770260 ) ) ;
#76107=CARTESIAN_POINT ( 'NONE',  ( 13.89961937509977652, -13.97604488694527269, 73.12390960531436690 ) ) ;
#76108=CARTESIAN_POINT ( 'NONE',  ( 12.06949235617757843, -12.14591786802309237, 48.12390960531436690 ) ) ;
#76109=CARTESIAN_POINT ( 'NONE',  ( 19.03943276465977164, -0.05219959533909143690, 103.7489096053143669 ) ) ;
#76111=CARTESIAN_POINT ( 'NONE',  ( 9.564922557961047289, -16.46253265017146816, 55.41775706135234003 ) ) ;
#76112=CARTESIAN_POINT ( 'NONE',  ( 15.72974639402199770, -15.80617190586745480, 93.12390960531436690 ) ) ;
#76113=CARTESIAN_POINT ( 'NONE',  ( -9.474510206698964154, 16.51473224551069663, 45.41557627198103120 ) ) ;
#76114=CARTESIAN_POINT ( 'NONE',  ( 16.53943276465976808, -0.05219959533910856209, 113.7489096053143527 ) ) ;
#76115=CARTESIAN_POINT ( 'NONE',  ( 18.67979575497194134, -10.72451020669871369, 55.83442372801901854 ) ) ;
#76117=CARTESIAN_POINT ( 'NONE',  ( -8.224510206698948167, 14.34966873604960824, 25.41557627198103120 ) ) ;
#76118=CARTESIAN_POINT ( 'NONE',  ( 0.05219959533909260263, 19.03943276465977164, 54.99890960531435979 ) ) ;
#76119=CARTESIAN_POINT ( 'NONE',  ( -13.89961937509977652, 13.97604488694528158, 100.6239096053143669 ) ) ;
#76120=CARTESIAN_POINT ( 'NONE',  ( -21.53943276465977519, 0.05219959533907696930, 66.24890960531436690 ) ) ;
#76122=CARTESIAN_POINT ( 'NONE',  ( 13.89961937509977652, -13.97604488694527269, 43.12390960531434558 ) ) ;
#76123=CARTESIAN_POINT ( 'NONE',  ( 10.81492255796078972, 18.62759615963270932, 54.58224293864769550 ) ) ;
#76124=CARTESIAN_POINT ( 'NONE',  ( 10.72451020669871369, 18.67979575497193778, 82.08442372801901854 ) ) ;
#76126=CARTESIAN_POINT ( 'NONE',  ( -16.53943276465976808, -0.05219959533934237506, 88.75109039468567573 ) ) ;
#76127=CARTESIAN_POINT ( 'NONE',  ( 8.314922557960818139, 14.29746914071049879, 69.58224293864769550 ) ) ;
#76128=CARTESIAN_POINT ( 'NONE',  ( 14.34966873604972726, -8.224510206698740333, 85.83442372801901854 ) ) ;
#76129=CARTESIAN_POINT ( 'NONE',  ( -19.03943276465977164, 0.05219959533909376836, 71.24890960531435269 ) ) ;
#76130=VERTEX_POINT ( 'NONE', #47509 ) ;
#76131=CARTESIAN_POINT ( 'NONE',  ( 19.05341960407617918, -5.049401038297876454, 31.04275706135232227 ) ) ;
#76132=CARTESIAN_POINT ( 'NONE',  ( -0.05219959533934338120, 16.53943276465976808, 87.50109039468568994 ) ) ;
#76133=CARTESIAN_POINT ( 'NONE',  ( 19.05341960407617918, -5.049401038297876454, 21.04275706135232582 ) ) ;
#76134=CARTESIAN_POINT ( 'NONE',  ( 19.03943276465977164, -0.05219959533909143690, 78.74890960531436690 ) ) ;
#76135=CARTESIAN_POINT ( 'NONE',  ( -18.67979575497178146, -10.72451020669898902, 41.66557627198103120 ) ) ;
#76136=CARTESIAN_POINT ( 'NONE',  ( -14.34966873604972548, 8.224510206698743886, 23.33442372801901499 ) ) ;
#76137=CARTESIAN_POINT ( 'NONE',  ( -0.05219959533937732626, 21.53943276465977519, 77.50109039468567573 ) ) ;
#76138=CARTESIAN_POINT ( 'NONE',  ( 4.379528057220092307, 16.55341960407617563, 62.29275706135236845 ) ) ;
#76139=CARTESIAN_POINT ( 'NONE',  ( -15.72974639402197994, 15.80617190586746368, 110.6239096053143669 ) ) ;
#76140=CARTESIAN_POINT ( 'NONE',  ( 9.474510206698729675, 16.51473224551082808, 107.0844237280190043 ) ) ;
#76141=CARTESIAN_POINT ( 'NONE',  ( -0.05219959533909027116, -19.03943276465977164, 92.49890960531436690 ) ) ;
#76142=CARTESIAN_POINT ( 'NONE',  ( 8.314922557961029526, -14.29746914071037800, 30.41775706135234358 ) ) ;
#76143=CARTESIAN_POINT ( 'NONE',  ( 13.89961937509977652, -13.97604488694527269, 38.12390960531436690 ) ) ;
#76144=CARTESIAN_POINT ( 'NONE',  ( 12.06949235617739724, 12.14591786802326823, 21.87609039468567573 ) ) ;
#76145=CARTESIAN_POINT ( 'NONE',  ( 14.34966873604960469, 8.224510206698951720, 84.16557627198103830 ) ) ;
#76146=CARTESIAN_POINT ( 'NONE',  ( -0.05219959533934338120, 16.53943276465976808, 82.50109039468568994 ) ) ;
#76147=CARTESIAN_POINT ( 'NONE',  ( -21.55341960407619339, 5.719274019375674811, 23.54275706135235424 ) ) ;
#76148=CARTESIAN_POINT ( 'NONE',  ( -9.564922557960796823, -16.46253265017161027, 67.08224293864769550 ) ) ;
#76149=CARTESIAN_POINT ( 'NONE',  ( 13.97604488694527802, 13.89961937509977652, 69.37390960531436690 ) ) ;
#76150=CARTESIAN_POINT ( 'NONE',  ( 14.29746914071037800, 8.314922557961029526, 91.66775706135234714 ) ) ;
#76152=EDGE_LOOP ( 'NONE', ( #87533, #156483, #87543 ) ) ;
#76154=CARTESIAN_POINT ( 'NONE',  ( 13.97604488694548053, -13.89961937509957401, 35.62609039468567573 ) ) ;
#76155=EDGE_CURVE ( 'NONE', #89992, #106494, #46029, .T. ) ;
#76156=CARTESIAN_POINT ( 'NONE',  ( -19.05341960407611168, -5.049401038298163336, 51.45724293864770260 ) ) ;
#76157=CARTESIAN_POINT ( 'NONE',  ( -19.02544592524342804, 5.153800228976336051, 111.0405762719810099 ) ) ;
#76159=CARTESIAN_POINT ( 'NONE',  ( 16.53943276465976808, 0.05219959533934440121, 26.25109039468567573 ) ) ;
#76160=CARTESIAN_POINT ( 'NONE',  ( -19.02544592524334988, -5.153800228976617603, 53.95942372801898301 ) ) ;
#76161=CARTESIAN_POINT ( 'NONE',  ( 4.379528057220092307, 16.55341960407617563, 47.29275706135234003 ) ) ;
#76162=CARTESIAN_POINT ( 'NONE',  ( 0.05219959533909260263, 19.03943276465977164, 99.99890960531436690 ) ) ;
#76163=CARTESIAN_POINT ( 'NONE',  ( 16.51473224551069308, 9.474510206698969483, 74.16557627198103830 ) ) ;
#76164=CARTESIAN_POINT ( 'NONE',  ( 21.55341960407610458, 5.719274019375980345, 103.9572429386476813 ) ) ;
#76165=CARTESIAN_POINT ( 'NONE',  ( -9.564922557961040184, 16.46253265017147172, 67.91775706135233293 ) ) ;
#76166=CARTESIAN_POINT ( 'NONE',  ( -9.474510206698964154, 16.51473224551069663, 85.41557627198102409 ) ) ;
#76168=CARTESIAN_POINT ( 'NONE',  ( 9.564922557960805705, 16.46253265017160317, 59.58224293864769550 ) ) ;
#76169=CARTESIAN_POINT ( 'NONE',  ( 14.29746914071049879, -8.314922557960816363, 23.33224293864769194 ) ) ;
#76170=CARTESIAN_POINT ( 'NONE',  ( 5.049401038298161559, -19.05341960407611168, 27.70724293864769550 ) ) ;
#76171=CARTESIAN_POINT ( 'NONE',  ( -5.153800228976607833, 19.02544592524334988, 37.70942372801899722 ) ) ;
#76172=CARTESIAN_POINT ( 'NONE',  ( -12.06949235617756955, 12.14591786802309770, 75.62390960531439532 ) ) ;
#76173=CARTESIAN_POINT ( 'NONE',  ( 0.05219959533937995610, -21.53943276465977519, 95.00109039468568994 ) ) ;
#76174=CARTESIAN_POINT ( 'NONE',  ( 13.89961937509977652, -13.97604488694527269, 43.12390960531434558 ) ) ;
#76175=CARTESIAN_POINT ( 'NONE',  ( -16.53943276465976808, -0.05219959533934237506, 48.75109039468568284 ) ) ;
#76176=CARTESIAN_POINT ( 'NONE',  ( -12.06949235617756955, 12.14591786802309770, 45.62390960531436690 ) ) ;
#76177=CARTESIAN_POINT ( 'NONE',  ( 21.53943276465977519, 0.05219959533937863772, 91.25109039468568994 ) ) ;
#76178=CARTESIAN_POINT ( 'NONE',  ( -0.05219959533909027116, -19.03943276465977164, 97.49890960531436690 ) ) ;
#76179=CARTESIAN_POINT ( 'NONE',  ( 13.89961937509977652, -13.97604488694527269, 98.12390960531433848 ) ) ;
#76180=CARTESIAN_POINT ( 'NONE',  ( -0.05219959533910754901, -16.53943276465976808, 107.4989096053143669 ) ) ;
#76181=CARTESIAN_POINT ( 'NONE',  ( 14.29746914071049879, -8.314922557960816363, 68.33224293864769550 ) ) ;
#76182=CARTESIAN_POINT ( 'NONE',  ( 5.719274019375991003, -21.55341960407610458, 77.70724293864770971 ) ) ;
#76183=CARTESIAN_POINT ( 'NONE',  ( 19.03943276465977164, -0.05219959533909143690, 93.74890960531435269 ) ) ;
#76184=CARTESIAN_POINT ( 'NONE',  ( 5.823673210054125526, 21.52544592524343514, 104.7905762719810241 ) ) ;
#76185=CARTESIAN_POINT ( 'NONE',  ( 5.049401038297881783, 19.05341960407617563, 72.29275706135234714 ) ) ;
#76187=CARTESIAN_POINT ( 'NONE',  ( -19.53091890409953990, -5.499999999999944933, 90.06097431831425126 ) ) ;
#76188=CARTESIAN_POINT ( 'NONE',  ( 8.314922557960818139, 14.29746914071049879, 89.58224293864768129 ) ) ;
#76189=CARTESIAN_POINT ( 'NONE',  ( 19.02544592524343514, -5.153800228976328945, 53.54057627198102409 ) ) ;
#76190=CARTESIAN_POINT ( 'NONE',  ( -0.05219959533907301413, -21.53943276465977519, 67.49890960531436690 ) ) ;
#76191=CARTESIAN_POINT ( 'NONE',  ( 19.50973618000807619, 5.499999999999992895, 102.5000000000000142 ) ) ;
#76192=CARTESIAN_POINT ( 'NONE',  ( 16.52544592524335698, 4.483927247898782831, 106.4594237280190328 ) ) ;
#76194=CARTESIAN_POINT ( 'NONE',  ( -14.34966873604972548, 8.224510206698743886, 23.33442372801901499 ) ) ;
#76195=CARTESIAN_POINT ( 'NONE',  ( -0.05219959533910754901, -16.53943276465976808, 87.49890960531436690 ) ) ;
#76197=CARTESIAN_POINT ( 'NONE',  ( -5.049401038298153566, 19.05341960407611168, 70.20724293864769550 ) ) ;
#76198=CARTESIAN_POINT ( 'NONE',  ( -9.564922557960796823, -16.46253265017161027, 37.08224293864768839 ) ) ;
#76199=CARTESIAN_POINT ( 'NONE',  ( -14.34966873604960291, -8.224510206698953496, 66.66557627198102409 ) ) ;
#76200=CARTESIAN_POINT ( 'NONE',  ( -21.52544592524343514, 5.823673210054127303, 26.04057627198103475 ) ) ;
#76201=CARTESIAN_POINT ( 'NONE',  ( 9.474510206698729675, 16.51473224551082808, 97.08442372801900433 ) ) ;
#76202=CARTESIAN_POINT ( 'NONE',  ( -13.89961937509977652, 13.97604488694528158, 100.6239096053143669 ) ) ;
#76203=CARTESIAN_POINT ( 'NONE',  ( -18.62759615963270932, 10.81492255796079327, 80.83224293864769550 ) ) ;
#76204=CARTESIAN_POINT ( 'NONE',  ( -4.483927247898782831, 16.52544592524335698, 77.70942372801900433 ) ) ;
#76205=CARTESIAN_POINT ( 'NONE',  ( -16.46253265017146816, -9.564922557961047289, 109.1677570613523471 ) ) ;
#76206=CARTESIAN_POINT ( 'NONE',  ( -16.51473224551069308, -9.474510206698971260, 56.66557627198103120 ) ) ;
#76207=CARTESIAN_POINT ( 'NONE',  ( 15.80617190586746368, 15.72974639402197994, 64.37390960531435269 ) ) ;
#76208=CARTESIAN_POINT ( 'NONE',  ( -5.153800228976607833, 19.02544592524334988, 102.7094237280189759 ) ) ;
#76209=CARTESIAN_POINT ( 'NONE',  ( 14.29746914071049879, -8.314922557960816363, 43.33224293864769550 ) ) ;
#76210=CARTESIAN_POINT ( 'NONE',  ( 18.62759615963255655, 10.81492255796105972, 61.66775706135235424 ) ) ;
#76212=CARTESIAN_POINT ( 'NONE',  ( 0.05219959533934541429, -16.53943276465976808, 75.00109039468568994 ) ) ;
#76213=CARTESIAN_POINT ( 'NONE',  ( -16.46253265017160317, 9.564922557960807481, 100.8322429386477097 ) ) ;
#76214=CARTESIAN_POINT ( 'NONE',  ( -9.564922557960796823, -16.46253265017161027, 107.0822429386476955 ) ) ;
#76216=CARTESIAN_POINT ( 'NONE',  ( -16.52544592524335698, -4.483927247898792601, 98.95942372801903275 ) ) ;
#76217=CARTESIAN_POINT ( 'NONE',  ( -16.52544592524335698, -4.483927247898792601, 43.95942372801902565 ) ) ;
#76218=CARTESIAN_POINT ( 'NONE',  ( 19.03943276465977164, -0.05219959533909143690, 53.74890960531436690 ) ) ;
#76219=CARTESIAN_POINT ( 'NONE',  ( 9.474510206698971260, -16.51473224551069308, 72.91557627198102409 ) ) ;
#76220=CARTESIAN_POINT ( 'NONE',  ( 21.52544592524334988, 5.823673210054432836, 66.45942372801903275 ) ) ;
#76221=CARTESIAN_POINT ( 'NONE',  ( 16.55341960407618274, -4.379528057220086978, 61.04275706135234714 ) ) ;
#76222=CARTESIAN_POINT ( 'NONE',  ( -12.06949235617756955, 12.14591786802309770, 30.62390960531436335 ) ) ;
#76223=CARTESIAN_POINT ( 'NONE',  ( 9.564922557960805705, 16.46253265017160317, 39.58224293864768839 ) ) ;
#76224=CARTESIAN_POINT ( 'NONE',  ( 16.51473224551069308, 9.474510206698969483, 34.16557627198102409 ) ) ;
#76225=CARTESIAN_POINT ( 'NONE',  ( -14.29746914071037622, -8.314922557961029526, 34.16775706135234714 ) ) ;
#76226=CARTESIAN_POINT ( 'NONE',  ( 9.564922557961047289, -16.46253265017146816, 100.4177570613523329 ) ) ;
#76227=CARTESIAN_POINT ( 'NONE',  ( -14.34966873604960291, -8.224510206698953496, 101.6655762719810383 ) ) ;
#76228=CARTESIAN_POINT ( 'NONE',  ( 5.153800228976335163, 19.02544592524342804, 49.79057627198100988 ) ) ;
#76229=CARTESIAN_POINT ( 'NONE',  ( 13.97604488694548053, -13.89961937509957401, 85.62609039468568994 ) ) ;
#76231=CARTESIAN_POINT ( 'NONE',  ( 10.72451020669871369, 18.67979575497193778, 92.08442372801901854 ) ) ;
#76232=CARTESIAN_POINT ( 'NONE',  ( -12.14591786802326823, 12.06949235617739902, 58.12609039468568994 ) ) ;
#76233=CARTESIAN_POINT ( 'NONE',  ( -18.22780087662126647, -5.499999999999827693, 48.98236817873107185 ) ) ;
#76234=CARTESIAN_POINT ( 'NONE',  ( -10.81492255796078084, -18.62759615963271287, 52.08224293864768839 ) ) ;
#76235=CARTESIAN_POINT ( 'NONE',  ( 12.14591786802327356, -12.06949235617739191, 35.62609039468568994 ) ) ;
#76236=CARTESIAN_POINT ( 'NONE',  ( -18.39635199886970796, 5.499999999999980460, 71.01967076360004683 ) ) ;
#76237=CARTESIAN_POINT ( 'NONE',  ( -19.05341960407617563, 5.049401038297882671, 38.54275706135233293 ) ) ;
#76239=CARTESIAN_POINT ( 'NONE',  ( 19.05341960407611168, 5.049401038298154454, 93.95724293864769550 ) ) ;
#76240=CARTESIAN_POINT ( 'NONE',  ( -5.153800228976328057, -19.02544592524343514, 57.29057627198103120 ) ) ;
#76242=CARTESIAN_POINT ( 'NONE',  ( 5.719274019375673035, 21.55341960407619339, 77.29275706135234714 ) ) ;
#76243=CARTESIAN_POINT ( 'NONE',  ( -15.49999999999999822, 0.000000000000000000, 120.0000000000000142 ) ) ;
#76244=CARTESIAN_POINT ( 'NONE',  ( 0.05219959533936267826, -19.03943276465977164, 35.00109039468566863 ) ) ;
#76245=CARTESIAN_POINT ( 'NONE',  ( 19.05341960407617918, -5.049401038297876454, 21.04275706135232582 ) ) ;
#76246=CARTESIAN_POINT ( 'NONE',  ( -16.52544592524342804, 4.483927247898546575, 51.04057627198103120 ) ) ;
#76247=CARTESIAN_POINT ( 'NONE',  ( -19.03943276465977164, 0.05219959533909376836, 56.24890960531435979 ) ) ;
#76248=CARTESIAN_POINT ( 'NONE',  ( -9.474510206698964154, 16.51473224551069663, 110.4155762719810383 ) ) ;
#76249=CARTESIAN_POINT ( 'NONE',  ( 18.62759615963255655, 10.81492255796105972, 86.66775706135234714 ) ) ;
#76250=CARTESIAN_POINT ( 'NONE',  ( 9.564922557960805705, 16.46253265017160317, 69.58224293864770971 ) ) ;
#76251=CARTESIAN_POINT ( 'NONE',  ( 15.80617190586769283, -15.72974639402175789, 75.62609039468567573 ) ) ;
#76252=CARTESIAN_POINT ( 'NONE',  ( 21.53943276465977519, -0.05219959533907433946, 33.74890960531436690 ) ) ;
#76253=CARTESIAN_POINT ( 'NONE',  ( -21.53943276465977519, -0.05219959533937600094, 33.75109039468568284 ) ) ;
#76254=CARTESIAN_POINT ( 'NONE',  ( -19.02544592524334988, -5.153800228976617603, 63.95942372801899012 ) ) ;
#76255=CARTESIAN_POINT ( 'NONE',  ( 13.97604488694527802, 13.89961937509977652, 24.37390960531435624 ) ) ;
#76256=CARTESIAN_POINT ( 'NONE',  ( -16.46253265017160317, 9.564922557960807481, 70.83224293864770971 ) ) ;
#76257=CARTESIAN_POINT ( 'NONE',  ( 16.53943276465976808, 0.05219959533934440121, 31.25109039468568639 ) ) ;
#76258=CARTESIAN_POINT ( 'NONE',  ( -16.52544592524342804, 4.483927247898546575, 86.04057627198102409 ) ) ;
#76259=CARTESIAN_POINT ( 'NONE',  ( -16.51473224551069308, -9.474510206698971260, 61.66557627198103120 ) ) ;
#76260=CARTESIAN_POINT ( 'NONE',  ( 5.823673210054125526, 21.52544592524343514, 39.79057627198103830 ) ) ;
#76261=CARTESIAN_POINT ( 'NONE',  ( -9.474510206698720793, -16.51473224551083518, 104.5844237280190043 ) ) ;
#76262=CARTESIAN_POINT ( 'NONE',  ( -10.72451020669898014, 18.67979575497178502, 115.4155762719810241 ) ) ;
#76263=CARTESIAN_POINT ( 'NONE',  ( 21.53943276465977519, 0.05219959533937863772, 76.25109039468568994 ) ) ;
#76264=CARTESIAN_POINT ( 'NONE',  ( -4.379528057220086978, -16.55341960407618274, 74.79275706135234714 ) ) ;
#76265=CARTESIAN_POINT ( 'NONE',  ( -16.53943276465976808, -0.05219959533934237506, 68.75109039468568994 ) ) ;
#76267=CARTESIAN_POINT ( 'NONE',  ( -13.97604488694527625, -13.89961937509977652, 66.87390960531436690 ) ) ;
#76268=CARTESIAN_POINT ( 'NONE',  ( -4.379528057220086978, -16.55341960407618274, 84.79275706135234714 ) ) ;
#76269=CARTESIAN_POINT ( 'NONE',  ( 9.474510206698729675, 16.51473224551082808, 42.08442372801900433 ) ) ;
#76270=CARTESIAN_POINT ( 'NONE',  ( 10.72451020669898902, -18.67979575497178502, 112.9155762719810383 ) ) ;
#76271=CARTESIAN_POINT ( 'NONE',  ( 12.14591786802309770, 12.06949235617756955, 69.37390960531436690 ) ) ;
#76272=CARTESIAN_POINT ( 'NONE',  ( 9.564922557960805705, 16.46253265017160317, 79.58224293864769550 ) ) ;
#76273=CARTESIAN_POINT ( 'NONE',  ( 4.483927247898790824, -16.52544592524335698, 85.20942372801901854 ) ) ;
#76274=CARTESIAN_POINT ( 'NONE',  ( 0.05219959533937995610, -21.53943276465977519, 65.00109039468568994 ) ) ;
#76275=CARTESIAN_POINT ( 'NONE',  ( -5.153800228976607833, 19.02544592524334988, 112.7094237280190043 ) ) ;
#76276=CARTESIAN_POINT ( 'NONE',  ( 15.80617190586769283, -15.72974639402175789, 20.62609039468568639 ) ) ;
#76277=CARTESIAN_POINT ( 'NONE',  ( -8.314922557960811034, -14.29746914071050412, 57.08224293864769550 ) ) ;
#76279=CARTESIAN_POINT ( 'NONE',  ( 21.53943276465977519, -0.05219959533907433946, 93.74890960531436690 ) ) ;
#76280=CARTESIAN_POINT ( 'NONE',  ( -12.06949235617756955, 12.14591786802309770, 40.62390960531435269 ) ) ;
#76281=EDGE_LOOP ( 'NONE', ( #155101, #39000, #195471, #107189, #70085, #185308, #187235, #45625, #158910, #95189, #191607, #150012, #43000, #93816, #79614, #164129, #40581, #104497, #8715, #133354, #161342, #97212, #46799, #199114, #146668, #175736, #104197, #27593, #92497, #66947, #112957, #57741, #26848, #89146, #26150, #29668, #106611, #42599, #156165, #160852, #7819, #36577, #153120, #155544, #101396, #69615, #124388, #98881, #47428, #42183, #151350, #56446, #68359, #36753, #1663, #75382 ) ) ;
#76283=CARTESIAN_POINT ( 'NONE',  ( 10.81492255796078972, 18.62759615963270932, 109.5822429386476955 ) ) ;
#76284=CARTESIAN_POINT ( 'NONE',  ( 5.153800228976335163, 19.02544592524342804, 109.7905762719810099 ) ) ;
#76285=CARTESIAN_POINT ( 'NONE',  ( 21.55341960407619695, -5.719274019375665929, 31.04275706135234714 ) ) ;
#76286=CARTESIAN_POINT ( 'NONE',  ( -16.55341960407611168, -4.379528057220339221, 51.45724293864770260 ) ) ;
#76287=CARTESIAN_POINT ( 'NONE',  ( -19.05341960407611168, -5.049401038298163336, 56.45724293864768129 ) ) ;
#76289=B_SPLINE_CURVE_WITH_KNOTS ( 'NONE', 3,
 ( #119144, #151469, #152445, #133295, #121107, #103964 ),
 .UNSPECIFIED., .F., .F.,
 ( 4, 2, 4 ),
 ( 0.003989672132298028098, 0.004372778065220453078, 0.004755883998142877191 ),
 .UNSPECIFIED. ) ;
#76290=CARTESIAN_POINT ( 'NONE',  ( 9.474510206698729675, 16.51473224551082808, 62.08442372801899722 ) ) ;
#76291=CARTESIAN_POINT ( 'NONE',  ( 5.153800228976335163, 19.02544592524342804, 89.79057627198102409 ) ) ;
#76292=CARTESIAN_POINT ( 'NONE',  ( 18.67979575497178502, 10.72451020669898547, 54.16557627198103120 ) ) ;
#76294=CARTESIAN_POINT ( 'NONE',  ( -9.564922557960796823, -16.46253265017161027, 57.08224293864769550 ) ) ;
#76295=CARTESIAN_POINT ( 'NONE',  ( 16.53943276465976808, 0.05219959533934440121, 41.25109039468568284 ) ) ;
#76296=CARTESIAN_POINT ( 'NONE',  ( -19.03943276465977164, -0.05219959533935918106, 68.75109039468566152 ) ) ;
#76297=CARTESIAN_POINT ( 'NONE',  ( -21.55341960407610458, -5.719274019375992779, 111.4572429386476813 ) ) ;
#76298=CARTESIAN_POINT ( 'NONE',  ( -12.14591786802309592, -12.06949235617757132, 51.87390960531437401 ) ) ;
#76300=CARTESIAN_POINT ( 'NONE',  ( 0.05219959533909260263, 19.03943276465977164, 84.99890960531436690 ) ) ;
#76301=CARTESIAN_POINT ( 'NONE',  ( 18.67979575497178502, 10.72451020669898547, 74.16557627198102409 ) ) ;
#76302=CARTESIAN_POINT ( 'NONE',  ( 21.55341960407610458, 5.719274019375980345, 103.9572429386476813 ) ) ;
#76303=CARTESIAN_POINT ( 'NONE',  ( 16.52544592524335698, 4.483927247898782831, 36.45942372801901143 ) ) ;
#76304=CARTESIAN_POINT ( 'NONE',  ( 10.81492255796078972, 18.62759615963270932, 34.58224293864770260 ) ) ;
#76305=CARTESIAN_POINT ( 'NONE',  ( 18.67979575497194134, -10.72451020669871369, 100.8344237280190185 ) ) ;
#76306=CARTESIAN_POINT ( 'NONE',  ( -19.02544592524342804, 5.153800228976336051, 91.04057627198100988 ) ) ;
#76307=CARTESIAN_POINT ( 'NONE',  ( -19.02544592524342804, 5.153800228976336051, 46.04057627198101699 ) ) ;
#76308=CARTESIAN_POINT ( 'NONE',  ( -19.05341960407611168, -5.049401038298163336, 101.4572429386476955 ) ) ;
#76309=CARTESIAN_POINT ( 'NONE',  ( -13.97604488694527625, -13.89961937509977652, 71.87390960531433848 ) ) ;
#76310=CARTESIAN_POINT ( 'NONE',  ( 16.52544592524335698, 4.483927247898782831, 21.45942372801901499 ) ) ;
#76312=CARTESIAN_POINT ( 'NONE',  ( -19.03943276465977164, -0.05219959533935918106, 53.75109039468566863 ) ) ;
#76313=CARTESIAN_POINT ( 'NONE',  ( -5.719274019375665041, -21.55341960407619695, 104.7927570613523898 ) ) ;
#76314=CARTESIAN_POINT ( 'NONE',  ( 5.823673210054125526, 21.52544592524343514, 34.79057627198103120 ) ) ;
#76315=CARTESIAN_POINT ( 'NONE',  ( 4.379528057220092307, 16.55341960407617563, 102.2927570613523613 ) ) ;
#76317=CARTESIAN_POINT ( 'NONE',  ( -16.46253265017146816, -9.564922557961047289, 74.16775706135234714 ) ) ;
#76318=CARTESIAN_POINT ( 'NONE',  ( 5.049401038297881783, 19.05341960407617563, 27.29275706135232937 ) ) ;
#76320=CARTESIAN_POINT ( 'NONE',  ( -16.46253265017160317, 9.564922557960807481, 45.83224293864769550 ) ) ;
#76321=CARTESIAN_POINT ( 'NONE',  ( -14.34966873604960291, -8.224510206698953496, 41.66557627198103120 ) ) ;
#76323=CARTESIAN_POINT ( 'NONE',  ( -16.79531203550645202, -7.028104445595626082, 111.2524498822044023 ) ) ;
#76324=CARTESIAN_POINT ( 'NONE',  ( 12.06949235617757843, -12.14591786802309237, 33.12390960531435979 ) ) ;
#76326=CARTESIAN_POINT ( 'NONE',  ( -4.483927247898782831, 16.52544592524335698, 92.70942372801901854 ) ) ;
#76327=CARTESIAN_POINT ( 'NONE',  ( 5.153800228976335163, 19.02544592524342804, 34.79057627198102409 ) ) ;
#76328=CARTESIAN_POINT ( 'NONE',  ( -5.823673210054431948, 21.52544592524334988, 112.7094237280190328 ) ) ;
#76329=CARTESIAN_POINT ( 'NONE',  ( -16.53943276465976808, -0.05219959533934237506, 18.75109039468568639 ) ) ;
#76330=CARTESIAN_POINT ( 'NONE',  ( -15.72974639402176322, -15.80617190586768395, 84.37609039468570415 ) ) ;
#76332=CARTESIAN_POINT ( 'NONE',  ( 19.02544592524334988, 5.153800228976608722, 71.45942372801900433 ) ) ;
#76333=CARTESIAN_POINT ( 'NONE',  ( -19.02544592524342804, 5.153800228976336051, 96.04057627198103830 ) ) ;
#76334=CARTESIAN_POINT ( 'NONE',  ( -9.564922557960796823, -16.46253265017161027, 87.08224293864769550 ) ) ;
#76337=CARTESIAN_POINT ( 'NONE',  ( 5.823673210054125526, 21.52544592524343514, 114.7905762719810383 ) ) ;
#76339=CARTESIAN_POINT ( 'NONE',  ( 0.05219959533910956823, 16.53943276465976808, 69.99890960531435269 ) ) ;
#76340=CARTESIAN_POINT ( 'NONE',  ( -0.05219959533907301413, -21.53943276465977519, 57.49890960531435979 ) ) ;
#76341=CARTESIAN_POINT ( 'NONE',  ( -19.02544592524342804, 5.153800228976336051, 66.04057627198103830 ) ) ;
#76342=CARTESIAN_POINT ( 'NONE',  ( 18.67979575497178502, 10.72451020669898547, 94.16557627198103830 ) ) ;
#76343=CARTESIAN_POINT ( 'NONE',  ( -14.29746914071037622, -8.314922557961029526, 84.16775706135234714 ) ) ;
#76344=ORIENTED_EDGE ( 'NONE', *, *, #104192, .T. ) ;
#76345=CARTESIAN_POINT ( 'NONE',  ( -13.97604488694527625, -13.89961937509977652, 56.87390960531434558 ) ) ;
#76346=CARTESIAN_POINT ( 'NONE',  ( -0.05219959533910754901, -16.53943276465976808, 92.49890960531436690 ) ) ;
#76348=CARTESIAN_POINT ( 'NONE',  ( -13.89961937509977652, 13.97604488694528158, 45.62390960531433848 ) ) ;
#76349=CARTESIAN_POINT ( 'NONE',  ( -13.97604488694547697, 13.89961937509957934, 83.12609039468564731 ) ) ;
#76350=CARTESIAN_POINT ( 'NONE',  ( 16.52544592524342804, -4.483927247898539470, 78.54057627198103830 ) ) ;
#76351=CARTESIAN_POINT ( 'NONE',  ( 10.81492255796106328, -18.62759615963255655, 55.41775706135234714 ) ) ;
#76352=CARTESIAN_POINT ( 'NONE',  ( -19.02544592524342804, 5.153800228976336051, 41.04057627198103120 ) ) ;
#76353=CARTESIAN_POINT ( 'NONE',  ( -10.72451020669898014, 18.67979575497178502, 105.4155762719810383 ) ) ;
#76354=B_SPLINE_CURVE_WITH_KNOTS ( 'NONE', 3,
 ( #194487, #196498, #57968, #10469, #151954, #42801, #147982, #27649, #103470, #165149, #59932, #44776, #40797, #71134, #104463, #105450, #26640, #74134 ),
 .UNSPECIFIED., .F., .F.,
 ( 4, 2, 2, 2, 2, 2, 2, 2, 4 ),
 ( 9.540979117872439019E-18, 0.0003942454150793282125, 0.0007884908301586468840, 0.001182736245237965556, 0.001576981660317284227, 0.001971227075396602899, 0.002365472490475921570, 0.002759717905555240242, 0.003153963320634558913 ),
 .UNSPECIFIED. ) ;
#76355=CARTESIAN_POINT ( 'NONE',  ( -8.314922557960811034, -14.29746914071050412, 87.08224293864769550 ) ) ;
#76356=CARTESIAN_POINT ( 'NONE',  ( 18.09918380851993192, 5.500000000000009770, 93.98618307335613054 ) ) ;
#76357=CARTESIAN_POINT ( 'NONE',  ( 19.05341960407611168, 5.049401038298154454, 63.95724293864769550 ) ) ;
#76358=CARTESIAN_POINT ( 'NONE',  ( 18.87255363501902394, 5.499999999999941380, 48.82513748171827217 ) ) ;
#76359=CARTESIAN_POINT ( 'NONE',  ( -19.03943276465977164, -0.05219959533935918106, 98.75109039468567573 ) ) ;
#76360=CARTESIAN_POINT ( 'NONE',  ( -0.05219959533909027116, -19.03943276465977164, 112.4989096053143669 ) ) ;
#76361=CARTESIAN_POINT ( 'NONE',  ( 5.719274019375673035, 21.55341960407619339, 37.29275706135235424 ) ) ;
#76362=CARTESIAN_POINT ( 'NONE',  ( 19.02544592524343514, -5.153800228976328945, 78.54057627198099567 ) ) ;
#76363=CARTESIAN_POINT ( 'NONE',  ( 9.564922557961047289, -16.46253265017146816, 65.41775706135233293 ) ) ;
#76364=CARTESIAN_POINT ( 'NONE',  ( -9.564922557960796823, -16.46253265017161027, 57.08224293864769550 ) ) ;
#76365=CARTESIAN_POINT ( 'NONE',  ( -16.55341960407611168, -4.379528057220339221, 81.45724293864769550 ) ) ;
#76366=CARTESIAN_POINT ( 'NONE',  ( 8.224510206698953496, -14.34966873604960469, 72.91557627198103830 ) ) ;
#76367=CARTESIAN_POINT ( 'NONE',  ( -16.51473224551069308, -9.474510206698971260, 91.66557627198103830 ) ) ;
#76368=CARTESIAN_POINT ( 'NONE',  ( 8.314922557960818139, 14.29746914071049879, 84.58224293864769550 ) ) ;
#76369=CARTESIAN_POINT ( 'NONE',  ( 13.97604488694527802, 13.89961937509977652, 89.37390960531436690 ) ) ;
#76370=CARTESIAN_POINT ( 'NONE',  ( -16.46253265017146816, -9.564922557961047289, 34.16775706135233293 ) ) ;
#76371=CARTESIAN_POINT ( 'NONE',  ( -5.153800228976328057, -19.02544592524343514, 32.29057627198102409 ) ) ;
#76372=CARTESIAN_POINT ( 'NONE',  ( 16.52544592524342804, -4.483927247898539470, 28.54057627198103120 ) ) ;
#76373=CARTESIAN_POINT ( 'NONE',  ( 4.483927247898545687, 16.52544592524342804, 104.7905762719810241 ) ) ;
#76375=CARTESIAN_POINT ( 'NONE',  ( -15.80617190586768217, 15.72974639402176855, 38.12609039468567573 ) ) ;
#76376=CARTESIAN_POINT ( 'NONE',  ( 16.46253265017146816, 9.564922557961045513, 71.66775706135233293 ) ) ;
#76377=CARTESIAN_POINT ( 'NONE',  ( -0.05219959533910754901, -16.53943276465976808, 32.49890960531435979 ) ) ;
#76378=CARTESIAN_POINT ( 'NONE',  ( -21.52544592524343514, 5.823673210054127303, 91.04057627198103830 ) ) ;
#76379=CARTESIAN_POINT ( 'NONE',  ( -15.80617190586745835, -15.72974639402198527, 26.87390960531435979 ) ) ;
#76380=CARTESIAN_POINT ( 'NONE',  ( 14.29746914071049879, -8.314922557960816363, 73.33224293864769550 ) ) ;
#76381=CARTESIAN_POINT ( 'NONE',  ( 9.564922557960805705, 16.46253265017160317, 44.58224293864769550 ) ) ;
#76382=CARTESIAN_POINT ( 'NONE',  ( -16.46253265017146816, -9.564922557961047289, 24.16775706135233648 ) ) ;
#76383=CARTESIAN_POINT ( 'NONE',  ( -4.483927247898782831, 16.52544592524335698, 102.7094237280190185 ) ) ;
#76384=CARTESIAN_POINT ( 'NONE',  ( -8.314922557961024197, 14.29746914071037800, 57.91775706135234714 ) ) ;
#76385=CARTESIAN_POINT ( 'NONE',  ( -5.719274019375978568, 21.55341960407610458, 40.20724293864769550 ) ) ;
#76386=CARTESIAN_POINT ( 'NONE',  ( -15.80617190586768217, 15.72974639402176855, 108.1260903946856757 ) ) ;
#76387=CARTESIAN_POINT ( 'NONE',  ( -5.049401038298153566, 19.05341960407611168, 80.20724293864769550 ) ) ;
#76388=VECTOR ( 'NONE', #38818, 1000.000000000000000 ) ;
#76389=CARTESIAN_POINT ( 'NONE',  ( 16.52544592524335698, 4.483927247898782831, 76.45942372801901854 ) ) ;
#76390=CARTESIAN_POINT ( 'NONE',  ( -13.89961937509977652, 13.97604488694528158, 25.62390960531434558 ) ) ;
#76391=CARTESIAN_POINT ( 'NONE',  ( 16.52544592524342804, -4.483927247898539470, 38.54057627198103120 ) ) ;
#76392=CARTESIAN_POINT ( 'NONE',  ( -13.89961937509977652, 13.97604488694528158, 105.6239096053143527 ) ) ;
#76393=CARTESIAN_POINT ( 'NONE',  ( 0.05219959533909260263, 19.03943276465977164, 94.99890960531436690 ) ) ;
#76394=CARTESIAN_POINT ( 'NONE',  ( -15.80617190586745835, -15.72974639402198527, 31.87390960531435979 ) ) ;
#76395=CARTESIAN_POINT ( 'NONE',  ( -8.224510206698948167, 14.34966873604960824, 55.41557627198102409 ) ) ;
#76396=CARTESIAN_POINT ( 'NONE',  ( 16.53943276465976808, -0.05219959533910856209, 38.74890960531435979 ) ) ;
#76398=CARTESIAN_POINT ( 'NONE',  ( 14.29746914071049879, -8.314922557960816363, 58.33224293864768839 ) ) ;
#76399=CARTESIAN_POINT ( 'NONE',  ( -12.14591786802326823, 12.06949235617739902, 38.12609039468567573 ) ) ;
#76401=CARTESIAN_POINT ( 'NONE',  ( -0.05219959533936034679, 19.03943276465977164, 47.50109039468566863 ) ) ;
#76402=CARTESIAN_POINT ( 'NONE',  ( -9.474510206698964154, 16.51473224551069663, 90.41557627198103830 ) ) ;
#76403=CARTESIAN_POINT ( 'NONE',  ( 19.02544592524334988, 5.153800228976608722, 61.45942372801900433 ) ) ;
#76405=CARTESIAN_POINT ( 'NONE',  ( -19.03943276465977164, -0.05219959533935918106, 53.75109039468566863 ) ) ;
#76406=CARTESIAN_POINT ( 'NONE',  ( -9.474510206698720793, -16.51473224551083518, 99.58442372801900433 ) ) ;
#76407=CARTESIAN_POINT ( 'NONE',  ( 16.55341960407618274, -4.379528057220086978, 76.04275706135237556 ) ) ;
#76409=CARTESIAN_POINT ( 'NONE',  ( 19.05341960407611168, 5.049401038298154454, 23.95724293864769194 ) ) ;
#76410=CARTESIAN_POINT ( 'NONE',  ( 21.53943276465977519, -0.05219959533907433946, 23.74890960531435269 ) ) ;
#76411=CARTESIAN_POINT ( 'NONE',  ( -0.05219959533937732626, 21.53943276465977519, 37.50109039468568284 ) ) ;
#76412=CARTESIAN_POINT ( 'NONE',  ( -16.46253265017146816, -9.564922557961047289, 99.16775706135233293 ) ) ;
#76413=CARTESIAN_POINT ( 'NONE',  ( 17.49999999999999289, -3.237210098469628150, 107.2123698737954243 ) ) ;
#76414=CARTESIAN_POINT ( 'NONE',  ( -0.05219959533909027116, -19.03943276465977164, 57.49890960531435979 ) ) ;
#76415=CARTESIAN_POINT ( 'NONE',  ( 9.474510206698971260, -16.51473224551069308, 107.9155762719810383 ) ) ;
#76416=CARTESIAN_POINT ( 'NONE',  ( -8.224510206698948167, 14.34966873604960824, 65.41557627198102409 ) ) ;
#76417=CARTESIAN_POINT ( 'NONE',  ( -16.46253265017160317, 9.564922557960807481, 60.83224293864769550 ) ) ;
#76418=CARTESIAN_POINT ( 'NONE',  ( 9.474510206698971260, -16.51473224551069308, 77.91557627198103830 ) ) ;
#76419=CARTESIAN_POINT ( 'NONE',  ( 0.05219959533936267826, -19.03943276465977164, 80.00109039468567573 ) ) ;
#76420=CARTESIAN_POINT ( 'NONE',  ( -10.81492255796078084, -18.62759615963271287, 57.08224293864769550 ) ) ;
#76421=CARTESIAN_POINT ( 'NONE',  ( -0.05219959533910754901, -16.53943276465976808, 107.4989096053143669 ) ) ;
#76422=CARTESIAN_POINT ( 'NONE',  ( 9.474510206698729675, 16.51473224551082808, 47.08442372801900433 ) ) ;
#76423=CARTESIAN_POINT ( 'NONE',  ( -19.02544592524342804, 5.153800228976336051, 86.04057627198103830 ) ) ;
#76424=CARTESIAN_POINT ( 'NONE',  ( -21.53943276465977519, 0.05219959533907696930, 71.24890960531435269 ) ) ;
#76425=CARTESIAN_POINT ( 'NONE',  ( 0.05219959533910956823, 16.53943276465976808, 79.99890960531435269 ) ) ;
#76426=CARTESIAN_POINT ( 'NONE',  ( 16.46253265017146816, 9.564922557961045513, 41.66775706135234003 ) ) ;
#76427=CARTESIAN_POINT ( 'NONE',  ( 21.55341960407610458, 5.719274019375980345, 78.95724293864769550 ) ) ;
#76428=CARTESIAN_POINT ( 'NONE',  ( 15.80617190586746368, 15.72974639402197994, 59.37390960531436690 ) ) ;
#76429=CARTESIAN_POINT ( 'NONE',  ( 10.72451020669898902, -18.67979575497178502, 42.91557627198103120 ) ) ;
#76430=CARTESIAN_POINT ( 'NONE',  ( 18.67979575497194134, -10.72451020669871369, 85.83442372801901854 ) ) ;
#76431=CARTESIAN_POINT ( 'NONE',  ( 9.474510206698971260, -16.51473224551069308, 62.91557627198102409 ) ) ;
#76432=CARTESIAN_POINT ( 'NONE',  ( 8.224510206698953496, -14.34966873604960469, 112.9155762719810383 ) ) ;
#76433=CARTESIAN_POINT ( 'NONE',  ( -10.72451020669870658, -18.67979575497194134, 19.58442372801901143 ) ) ;
#76434=CARTESIAN_POINT ( 'NONE',  ( -17.60691670004650788, -5.500000000000068390, 49.13333313366439370 ) ) ;
#76435=CARTESIAN_POINT ( 'NONE',  ( -10.81492255796105439, 18.62759615963255655, 37.91775706135235424 ) ) ;
#76436=CARTESIAN_POINT ( 'NONE',  ( -9.474510206698964154, 16.51473224551069663, 40.41557627198103120 ) ) ;
#76437=CARTESIAN_POINT ( 'NONE',  ( 18.62759615963271287, -10.81492255796078972, 103.3322429386476955 ) ) ;
#76438=CARTESIAN_POINT ( 'NONE',  ( -13.97604488694547697, 13.89961937509957934, 53.12609039468565442 ) ) ;
#76439=CARTESIAN_POINT ( 'NONE',  ( -5.153800228976328057, -19.02544592524343514, 42.29057627198101699 ) ) ;
#76441=CARTESIAN_POINT ( 'NONE',  ( 16.21926038945174398, -7.366295777783752996, 21.89088085486532620 ) ) ;
#76442=CARTESIAN_POINT ( 'NONE',  ( -14.29746914071037622, -8.314922557961029526, 54.16775706135235424 ) ) ;
#76443=CARTESIAN_POINT ( 'NONE',  ( 5.049401038298161559, -19.05341960407611168, 27.70724293864769550 ) ) ;
#76445=CARTESIAN_POINT ( 'NONE',  ( -13.89961937509977652, 13.97604488694528158, 80.62390960531436690 ) ) ;
#76446=CARTESIAN_POINT ( 'NONE',  ( -16.52544592524342804, 4.483927247898546575, 106.0405762719810525 ) ) ;
#76447=CARTESIAN_POINT ( 'NONE',  ( 10.81492255796078972, 18.62759615963270932, 54.58224293864769550 ) ) ;
#76448=CARTESIAN_POINT ( 'NONE',  ( -4.483927247898782831, 16.52544592524335698, 47.70942372801902565 ) ) ;
#76449=CARTESIAN_POINT ( 'NONE',  ( -10.72451020669870658, -18.67979575497194134, 99.58442372801900433 ) ) ;
#76450=CARTESIAN_POINT ( 'NONE',  ( -13.89961937509977652, 13.97604488694528158, 30.62390960531435269 ) ) ;
#76451=CARTESIAN_POINT ( 'NONE',  ( -16.55341960407611168, -4.379528057220339221, 21.45724293864769550 ) ) ;
#76452=CARTESIAN_POINT ( 'NONE',  ( -8.224510206698948167, 14.34966873604960824, 50.41557627198103120 ) ) ;
#76453=CARTESIAN_POINT ( 'NONE',  ( -19.03943276465977164, 0.05219959533909376836, 56.24890960531435979 ) ) ;
#76454=CARTESIAN_POINT ( 'NONE',  ( -0.05219959533937732626, 21.53943276465977519, 112.5010903946857042 ) ) ;
#76455=CARTESIAN_POINT ( 'NONE',  ( -18.62759615963255300, -10.81492255796106328, 19.16775706135234714 ) ) ;
#76456=CARTESIAN_POINT ( 'NONE',  ( 5.823673210054444382, -21.52544592524334988, 75.20942372801901854 ) ) ;
#76457=CARTESIAN_POINT ( 'NONE',  ( 8.314922557961029526, -14.29746914071037800, 50.41775706135235424 ) ) ;
#76458=CARTESIAN_POINT ( 'NONE',  ( 16.52544592524335698, 4.483927247898782831, 31.45942372801901854 ) ) ;
#76460=CARTESIAN_POINT ( 'NONE',  ( -0.05219959533910754901, -16.53943276465976808, 72.49890960531435269 ) ) ;
#76461=CARTESIAN_POINT ( 'NONE',  ( -21.55341960407619339, 5.719274019375674811, 93.54275706135234714 ) ) ;
#76462=CARTESIAN_POINT ( 'NONE',  ( 4.483927247898545687, 16.52544592524342804, 39.79057627198103830 ) ) ;
#76463=CARTESIAN_POINT ( 'NONE',  ( -17.49999999999999645, 5.499999999999997335, 115.7969038253417438 ) ) ;
#76464=CARTESIAN_POINT ( 'NONE',  ( -14.29746914071037622, -8.314922557961029526, 39.16775706135235424 ) ) ;
#76465=CARTESIAN_POINT ( 'NONE',  ( -0.05219959533910754901, -16.53943276465976808, 42.49890960531435979 ) ) ;
#76466=CARTESIAN_POINT ( 'NONE',  ( 14.29746914071037800, 8.314922557961029526, 91.66775706135234714 ) ) ;
#76467=CARTESIAN_POINT ( 'NONE',  ( -13.89961937509977652, 13.97604488694528158, 100.6239096053143669 ) ) ;
#76468=CARTESIAN_POINT ( 'NONE',  ( -16.46253265017160317, 9.564922557960807481, 115.8322429386477097 ) ) ;
#76469=CARTESIAN_POINT ( 'NONE',  ( 15.72974639402176855, 15.80617190586768217, 96.87609039468568994 ) ) ;
#76470=CARTESIAN_POINT ( 'NONE',  ( -8.314922557961024197, 14.29746914071037800, 97.91775706135236135 ) ) ;
#76471=CARTESIAN_POINT ( 'NONE',  ( -0.05219959533910754901, -16.53943276465976808, 72.49890960531435269 ) ) ;
#76472=CARTESIAN_POINT ( 'NONE',  ( 19.02544592524343514, -5.153800228976328945, 83.54057627198100988 ) ) ;
#76473=EDGE_LOOP ( 'NONE', ( #165939, #102501, #1727, #123156 ) ) ;
#76474=CARTESIAN_POINT ( 'NONE',  ( 0.05219959533934541429, -16.53943276465976808, 45.00109039468568284 ) ) ;
#76475=CARTESIAN_POINT ( 'NONE',  ( -0.05219959533909027116, -19.03943276465977164, 37.49890960531436690 ) ) ;
#76476=CARTESIAN_POINT ( 'NONE',  ( -5.049401038298153566, 19.05341960407611168, 90.20724293864766707 ) ) ;
#76477=CARTESIAN_POINT ( 'NONE',  ( 14.29746914071037800, 8.314922557961029526, 36.66775706135234714 ) ) ;
#76479=CARTESIAN_POINT ( 'NONE',  ( -5.153800228976607833, 19.02544592524334988, 32.70942372801899722 ) ) ;
#76480=CARTESIAN_POINT ( 'NONE',  ( -16.52544592524335698, -4.483927247898792601, 93.95942372801903275 ) ) ;
#76481=CARTESIAN_POINT ( 'NONE',  ( -5.049401038298153566, 19.05341960407611168, 30.20724293864768839 ) ) ;
#76482=CARTESIAN_POINT ( 'NONE',  ( 12.06949235617739724, 12.14591786802326823, 81.87609039468568994 ) ) ;
#76483=CARTESIAN_POINT ( 'NONE',  ( 14.29746914071037800, 8.314922557961029526, 66.66775706135234714 ) ) ;
#76484=CARTESIAN_POINT ( 'NONE',  ( 0.05219959533936267826, -19.03943276465977164, 85.00109039468567573 ) ) ;
#76485=CARTESIAN_POINT ( 'NONE',  ( 0.05219959533936267826, -19.03943276465977164, 30.00109039468566863 ) ) ;
#76486=CARTESIAN_POINT ( 'NONE',  ( -16.51473224551069308, -9.474510206698971260, 56.66557627198103120 ) ) ;
#76487=CARTESIAN_POINT ( 'NONE',  ( 8.224510206698953496, -14.34966873604960469, 87.91557627198103830 ) ) ;
#76489=CARTESIAN_POINT ( 'NONE',  ( 0.05219959533936267826, -19.03943276465977164, 60.00109039468566863 ) ) ;
#76490=CARTESIAN_POINT ( 'NONE',  ( -5.823673210054116645, -21.52544592524344225, 47.29057627198103120 ) ) ;
#76491=CARTESIAN_POINT ( 'NONE',  ( 0.05219959533936267826, -19.03943276465977164, 25.00109039468566152 ) ) ;
#76492=CARTESIAN_POINT ( 'NONE',  ( -16.51473224551069308, -9.474510206698971260, 106.6655762719810383 ) ) ;
#76493=CARTESIAN_POINT ( 'NONE',  ( -5.719274019375978568, 21.55341960407610458, 80.20724293864769550 ) ) ;
#76494=CARTESIAN_POINT ( 'NONE',  ( 16.51473224551069308, 9.474510206698969483, 104.1655762719810241 ) ) ;
#76496=CARTESIAN_POINT ( 'NONE',  ( 9.474510206698729675, 16.51473224551082808, 102.0844237280190043 ) ) ;
#76497=CARTESIAN_POINT ( 'NONE',  ( 0.05219959533909260263, 19.03943276465977164, 109.9989096053143669 ) ) ;
#76498=CARTESIAN_POINT ( 'NONE',  ( -9.564922557961040184, 16.46253265017147172, 102.9177570613523329 ) ) ;
#76499=CARTESIAN_POINT ( 'NONE',  ( 16.46253265017160672, -9.564922557960803928, 38.33224293864768839 ) ) ;
#76500=CARTESIAN_POINT ( 'NONE',  ( -16.51473224551069308, -9.474510206698971260, 96.66557627198102409 ) ) ;
#76501=CARTESIAN_POINT ( 'NONE',  ( -21.55341960407610458, -5.719274019375992779, 81.45724293864769550 ) ) ;
#76502=CARTESIAN_POINT ( 'NONE',  ( -4.379528057220086978, -16.55341960407618274, 64.79275706135234714 ) ) ;
#76503=CARTESIAN_POINT ( 'NONE',  ( 18.62759615963255655, 10.81492255796105972, 66.66775706135234714 ) ) ;
#76504=CARTESIAN_POINT ( 'NONE',  ( 19.02544592524334988, 5.153800228976608722, 111.4594237280190043 ) ) ;
#76505=CARTESIAN_POINT ( 'NONE',  ( 5.719274019375673035, 21.55341960407619339, 112.2927570613523471 ) ) ;
#76506=CARTESIAN_POINT ( 'NONE',  ( 0.05219959533934541429, -16.53943276465976808, 105.0010903946856757 ) ) ;
#76507=CARTESIAN_POINT ( 'NONE',  ( -18.67979575497178146, -10.72451020669898902, 101.6655762719810383 ) ) ;
#76508=CARTESIAN_POINT ( 'NONE',  ( 0.05219959533910956823, 16.53943276465976808, 39.99890960531436690 ) ) ;
#76509=CARTESIAN_POINT ( 'NONE',  ( -9.474510206698720793, -16.51473224551083518, 79.58442372801899012 ) ) ;
#76510=CARTESIAN_POINT ( 'NONE',  ( 15.80617190586769283, -15.72974639402175789, 60.62609039468567573 ) ) ;
#76511=CARTESIAN_POINT ( 'NONE',  ( -5.153800228976607833, 19.02544592524334988, 37.70942372801899722 ) ) ;
#76512=CARTESIAN_POINT ( 'NONE',  ( -8.314922557960811034, -14.29746914071050412, 102.0822429386476955 ) ) ;
#76513=CARTESIAN_POINT ( 'NONE',  ( -21.53943276465977519, 0.05219959533907696930, 26.24890960531435624 ) ) ;
#76514=CARTESIAN_POINT ( 'NONE',  ( -12.06949235617756955, 12.14591786802309770, 35.62390960531437401 ) ) ;
#76515=CARTESIAN_POINT ( 'NONE',  ( -18.67979575497193778, 10.72451020669871902, 98.33442372801901854 ) ) ;
#76516=CARTESIAN_POINT ( 'NONE',  ( 16.55341960407618274, -4.379528057220086978, 76.04275706135237556 ) ) ;
#76517=CARTESIAN_POINT ( 'NONE',  ( -16.55341960407611168, -4.379528057220339221, 26.45724293864768839 ) ) ;
#76518=CARTESIAN_POINT ( 'NONE',  ( -21.53943276465977519, -0.05219959533937600094, 58.75109039468568994 ) ) ;
#76519=CARTESIAN_POINT ( 'NONE',  ( -0.05219959533937732626, 21.53943276465977519, 52.50109039468567573 ) ) ;
#76520=ORIENTED_EDGE ( 'NONE', *, *, #60120, .F. ) ;
#76521=CARTESIAN_POINT ( 'NONE',  ( -0.05219959533909027116, -19.03943276465977164, 27.49890960531435624 ) ) ;
#76522=CARTESIAN_POINT ( 'NONE',  ( -21.55341960407619339, 5.719274019375674811, 38.54275706135234714 ) ) ;
#76523=CARTESIAN_POINT ( 'NONE',  ( -13.89961937509977652, 13.97604488694528158, 25.62390960531434558 ) ) ;
#76524=CARTESIAN_POINT ( 'NONE',  ( 19.02544592524343514, -5.153800228976328945, 38.54057627198103120 ) ) ;
#76525=CARTESIAN_POINT ( 'NONE',  ( -12.14591786802309592, -12.06949235617757132, 81.87390960531435269 ) ) ;
#76526=CARTESIAN_POINT ( 'NONE',  ( 19.05341960407611168, 5.049401038298154454, 73.95724293864768129 ) ) ;
#76527=CARTESIAN_POINT ( 'NONE',  ( 12.14591786802309770, 12.06949235617756955, 29.37390960531435269 ) ) ;
#76528=CARTESIAN_POINT ( 'NONE',  ( 15.72974639402199770, -15.80617190586745480, 58.12390960531435979 ) ) ;
#76529=CARTESIAN_POINT ( 'NONE',  ( 16.53943276465976808, -0.05219959533910856209, 93.74890960531436690 ) ) ;
#76531=CARTESIAN_POINT ( 'NONE',  ( 10.72451020669898902, -18.67979575497178502, 112.9155762719810383 ) ) ;
#76532=CARTESIAN_POINT ( 'NONE',  ( 9.474510206698971260, -16.51473224551069308, 107.9155762719810383 ) ) ;
#76533=CARTESIAN_POINT ( 'NONE',  ( -5.049401038298153566, 19.05341960407611168, 70.20724293864769550 ) ) ;
#76534=CARTESIAN_POINT ( 'NONE',  ( 19.02544592524334988, 5.153800228976608722, 106.4594237280190185 ) ) ;
#76535=CARTESIAN_POINT ( 'NONE',  ( 21.52544592524344225, -5.823673210054117533, 53.54057627198103120 ) ) ;
#76536=CARTESIAN_POINT ( 'NONE',  ( 21.55341960407619695, -5.719274019375665929, 81.04275706135236135 ) ) ;
#76537=CARTESIAN_POINT ( 'NONE',  ( -19.05341960407611168, -5.049401038298163336, 66.45724293864769550 ) ) ;
#76538=CARTESIAN_POINT ( 'NONE',  ( 5.153800228976335163, 19.02544592524342804, 104.7905762719809957 ) ) ;
#76539=CARTESIAN_POINT ( 'NONE',  ( 12.06949235617739724, 12.14591786802326823, 81.87609039468568994 ) ) ;
#76540=CARTESIAN_POINT ( 'NONE',  ( 10.81492255796106328, -18.62759615963255655, 55.41775706135234714 ) ) ;
#76541=CARTESIAN_POINT ( 'NONE',  ( 15.72974639402176855, 15.80617190586768217, 81.87609039468568994 ) ) ;
#76542=CARTESIAN_POINT ( 'NONE',  ( 10.81492255796078972, 18.62759615963270932, 109.5822429386476955 ) ) ;
#76543=CARTESIAN_POINT ( 'NONE',  ( -12.14591786802326823, 12.06949235617739902, 83.12609039468568994 ) ) ;
#76544=CARTESIAN_POINT ( 'NONE',  ( -5.719274019375978568, 21.55341960407610458, 70.20724293864769550 ) ) ;
#76545=CARTESIAN_POINT ( 'NONE',  ( 16.51473224551083163, -9.474510206698727899, 45.83442372801900433 ) ) ;
#76546=CARTESIAN_POINT ( 'NONE',  ( 0.05219959533907565091, 21.53943276465977519, 39.99890960531436690 ) ) ;
#76547=CARTESIAN_POINT ( 'NONE',  ( 0.05219959533909260263, 19.03943276465977164, 74.99890960531435269 ) ) ;
#76548=CARTESIAN_POINT ( 'NONE',  ( -4.483927247898782831, 16.52544592524335698, 112.7094237280190328 ) ) ;
#76549=CARTESIAN_POINT ( 'NONE',  ( -17.48853670773241831, 5.747243402303156223, 63.66671299749991420 ) ) ;
#76550=CARTESIAN_POINT ( 'NONE',  ( 0.05219959533909260263, 19.03943276465977164, 114.9989096053143669 ) ) ;
#76551=CARTESIAN_POINT ( 'NONE',  ( 18.22780087662122739, 5.500000000000000888, 81.48236817873103632 ) ) ;
#76552=CARTESIAN_POINT ( 'NONE',  ( -19.05341960407617563, 5.049401038297882671, 93.54275706135234714 ) ) ;
#76553=CARTESIAN_POINT ( 'NONE',  ( 15.80617190586746368, 15.72974639402197994, 74.37390960531436690 ) ) ;
#76554=CARTESIAN_POINT ( 'NONE',  ( 16.53943276465976808, -0.05219959533910856209, 53.74890960531437401 ) ) ;
#76555=CARTESIAN_POINT ( 'NONE',  ( 12.14591786802327356, -12.06949235617739191, 20.62609039468568639 ) ) ;
#76556=CARTESIAN_POINT ( 'NONE',  ( -13.97604488694527625, -13.89961937509977652, 26.87390960531434558 ) ) ;
#76557=CARTESIAN_POINT ( 'NONE',  ( -10.81492255796078084, -18.62759615963271287, 97.08224293864770971 ) ) ;
#76558=CARTESIAN_POINT ( 'NONE',  ( -13.97604488694547697, 13.89961937509957934, 68.12609039468563310 ) ) ;
#76559=CARTESIAN_POINT ( 'NONE',  ( 19.03943276465977164, -0.05219959533909143690, 78.74890960531436690 ) ) ;
#76560=CARTESIAN_POINT ( 'NONE',  ( -0.05219959533910754901, -16.53943276465976808, 77.49890960531433848 ) ) ;
#76562=CARTESIAN_POINT ( 'NONE',  ( 9.474510206698971260, -16.51473224551069308, 57.91557627198103120 ) ) ;
#76563=CARTESIAN_POINT ( 'NONE',  ( -14.29746914071049879, 8.314922557960819915, 60.83224293864769550 ) ) ;
#76564=CARTESIAN_POINT ( 'NONE',  ( -5.049401038298153566, 19.05341960407611168, 30.20724293864768839 ) ) ;
#76566=CARTESIAN_POINT ( 'NONE',  ( 14.34966873604960469, 8.224510206698951720, 39.16557627198102409 ) ) ;
#76567=CARTESIAN_POINT ( 'NONE',  ( -19.05341960407611168, -5.049401038298163336, 86.45724293864769550 ) ) ;
#76569=CARTESIAN_POINT ( 'NONE',  ( -13.97604488694547697, 13.89961937509957934, 48.12609039468566863 ) ) ;
#76570=CARTESIAN_POINT ( 'NONE',  ( 12.06949235617739724, 12.14591786802326823, 66.87609039468568994 ) ) ;
#76571=CARTESIAN_POINT ( 'NONE',  ( -18.62759615963270932, 10.81492255796079327, 70.83224293864770971 ) ) ;
#76572=CARTESIAN_POINT ( 'NONE',  ( -0.05219959533936034679, 19.03943276465977164, 37.50109039468567573 ) ) ;
#76573=CARTESIAN_POINT ( 'NONE',  ( -19.03943276465977164, 0.05219959533909376836, 86.24890960531436690 ) ) ;
#76575=CARTESIAN_POINT ( 'NONE',  ( 0.05219959533907565091, 21.53943276465977519, 24.99890960531435624 ) ) ;
#76576=CARTESIAN_POINT ( 'NONE',  ( -13.89961937509977652, 13.97604488694528158, 55.62390960531434558 ) ) ;
#76577=CARTESIAN_POINT ( 'NONE',  ( 18.62759615963255655, 10.81492255796105972, 46.66775706135234714 ) ) ;
#76578=CARTESIAN_POINT ( 'NONE',  ( 14.34966873604960469, 8.224510206698951720, 104.1655762719810241 ) ) ;
#76579=CARTESIAN_POINT ( 'NONE',  ( 0.05219959533907565091, 21.53943276465977519, 99.99890960531436690 ) ) ;
#76580=CARTESIAN_POINT ( 'NONE',  ( 19.02544592524343514, -5.153800228976328945, 88.54057627198102409 ) ) ;
#76582=CARTESIAN_POINT ( 'NONE',  ( -15.80617190586768217, 15.72974639402176855, 43.12609039468568284 ) ) ;
#76584=CARTESIAN_POINT ( 'NONE',  ( 16.46253265017160672, -9.564922557960803928, 103.3322429386476955 ) ) ;
#76585=CARTESIAN_POINT ( 'NONE',  ( 9.564922557960805705, 16.46253265017160317, 89.58224293864769550 ) ) ;
#76586=CARTESIAN_POINT ( 'NONE',  ( -15.80617190586745835, -15.72974639402198527, 91.87390960531436690 ) ) ;
#76587=CARTESIAN_POINT ( 'NONE',  ( 19.05341960407611168, 5.049401038298154454, 43.95724293864769550 ) ) ;
#76588=CARTESIAN_POINT ( 'NONE',  ( 16.53943276465976808, 0.05219959533934440121, 21.25109039468567218 ) ) ;
#76590=CARTESIAN_POINT ( 'NONE',  ( -16.51473224551069308, -9.474510206698971260, 26.66557627198103120 ) ) ;
#76591=CARTESIAN_POINT ( 'NONE',  ( 10.72451020669871369, 18.67979575497193778, 102.0844237280190185 ) ) ;
#76592=CARTESIAN_POINT ( 'NONE',  ( -0.05219959533909027116, -19.03943276465977164, 82.49890960531436690 ) ) ;
#76593=CARTESIAN_POINT ( 'NONE',  ( 5.719274019375673035, 21.55341960407619339, 42.29275706135235424 ) ) ;
#76595=CARTESIAN_POINT ( 'NONE',  ( 16.51473224551069308, 9.474510206698969483, 94.16557627198103830 ) ) ;
#76597=CARTESIAN_POINT ( 'NONE',  ( 14.29746914071037800, 8.314922557961029526, 36.66775706135234714 ) ) ;
#76598=CARTESIAN_POINT ( 'NONE',  ( -12.14591786802326823, 12.06949235617739902, 68.12609039468567573 ) ) ;
#76599=CARTESIAN_POINT ( 'NONE',  ( -21.53943276465977519, -0.05219959533937600094, 63.75109039468568284 ) ) ;
#76600=CARTESIAN_POINT ( 'NONE',  ( -21.52544592524334988, -5.823673210054445271, 73.95942372801901854 ) ) ;
#76602=CARTESIAN_POINT ( 'NONE',  ( 16.53943276465976808, 0.05219959533934440121, 21.25109039468567218 ) ) ;
#76603=CARTESIAN_POINT ( 'NONE',  ( 13.97604488694527802, 13.89961937509977652, 74.37390960531436690 ) ) ;
#76604=CARTESIAN_POINT ( 'NONE',  ( 9.564922557960805705, 16.46253265017160317, 104.5822429386476955 ) ) ;
#76605=CARTESIAN_POINT ( 'NONE',  ( 4.483927247898545687, 16.52544592524342804, 109.7905762719810383 ) ) ;
#76606=CARTESIAN_POINT ( 'NONE',  ( 10.81492255796078972, 18.62759615963270932, 29.58224293864769905 ) ) ;
#76607=CARTESIAN_POINT ( 'NONE',  ( -16.55341960407617563, 4.379528057220093196, 88.54275706135236135 ) ) ;
#76608=CARTESIAN_POINT ( 'NONE',  ( 8.314922557960818139, 14.29746914071049879, 74.58224293864768129 ) ) ;
#76609=CARTESIAN_POINT ( 'NONE',  ( -0.05219959533909027116, -19.03943276465977164, 52.49890960531436690 ) ) ;
#76610=CARTESIAN_POINT ( 'NONE',  ( 5.823673210054444382, -21.52544592524334988, 75.20942372801901854 ) ) ;
#76612=CARTESIAN_POINT ( 'NONE',  ( 13.97604488694548053, -13.89961937509957401, 100.6260903946856615 ) ) ;
#76613=CARTESIAN_POINT ( 'NONE',  ( 0.05219959533910956823, 16.53943276465976808, 74.99890960531435269 ) ) ;
#76614=CARTESIAN_POINT ( 'NONE',  ( 18.62759615963255655, 10.81492255796105972, 26.66775706135235424 ) ) ;
#76615=CARTESIAN_POINT ( 'NONE',  ( -5.823673210054116645, -21.52544592524344225, 62.29057627198102409 ) ) ;
#76616=CARTESIAN_POINT ( 'NONE',  ( -17.44279575226825330, -5.990770900252416098, 104.1644243248568387 ) ) ;
#76618=CARTESIAN_POINT ( 'NONE',  ( 19.02544592524343514, -5.153800228976328945, 78.54057627198099567 ) ) ;
#76619=CARTESIAN_POINT ( 'NONE',  ( -8.224510206698948167, 14.34966873604960824, 50.41557627198103120 ) ) ;
#76620=CARTESIAN_POINT ( 'NONE',  ( -14.34966873604960291, -8.224510206698953496, 41.66557627198103120 ) ) ;
#76621=CARTESIAN_POINT ( 'NONE',  ( -8.314922557961024197, 14.29746914071037800, 102.9177570613523756 ) ) ;
#76622=CARTESIAN_POINT ( 'NONE',  ( 9.474510206698729675, 16.51473224551082808, 47.08442372801900433 ) ) ;
#76624=CARTESIAN_POINT ( 'NONE',  ( -16.46253265017160317, 9.564922557960807481, 110.8322429386476955 ) ) ;
#76625=CARTESIAN_POINT ( 'NONE',  ( 12.06949235617757843, -12.14591786802309237, 68.12390960531436690 ) ) ;
#76626=CARTESIAN_POINT ( 'NONE',  ( -13.97604488694547697, 13.89961937509957934, 48.12609039468566863 ) ) ;
#76627=CARTESIAN_POINT ( 'NONE',  ( 13.97604488694527802, 13.89961937509977652, 34.37390960531436690 ) ) ;
#76628=CARTESIAN_POINT ( 'NONE',  ( 10.81492255796078972, 18.62759615963270932, 34.58224293864770260 ) ) ;
#76629=CARTESIAN_POINT ( 'NONE',  ( -21.52544592524343514, 5.823673210054127303, 61.04057627198103120 ) ) ;
#76630=CARTESIAN_POINT ( 'NONE',  ( 8.224510206698953496, -14.34966873604960469, 102.9155762719810383 ) ) ;
#76631=CARTESIAN_POINT ( 'NONE',  ( -8.314922557961024197, 14.29746914071037800, 47.91775706135234714 ) ) ;
#76632=CARTESIAN_POINT ( 'NONE',  ( 10.72451020669871369, 18.67979575497193778, 47.08442372801901854 ) ) ;
#76633=CARTESIAN_POINT ( 'NONE',  ( 12.06949235617757843, -12.14591786802309237, 98.12390960531436690 ) ) ;
#76634=CARTESIAN_POINT ( 'NONE',  ( 16.38665767535054840, -7.295008042176023721, 37.76400864214549102 ) ) ;
#76635=CARTESIAN_POINT ( 'NONE',  ( -17.05116617787826527, 6.768360034955678728, 48.65675553259197983 ) ) ;
#76636=CARTESIAN_POINT ( 'NONE',  ( -21.52544592524343514, 5.823673210054127303, 31.04057627198102409 ) ) ;
#76639=CARTESIAN_POINT ( 'NONE',  ( 16.53943276465976808, 0.05219959533934440121, 46.25109039468567573 ) ) ;
#76640=CARTESIAN_POINT ( 'NONE',  ( 14.29746914071049879, -8.314922557960816363, 28.33224293864769550 ) ) ;
#76641=CARTESIAN_POINT ( 'NONE',  ( -0.05219959533907301413, -21.53943276465977519, 67.49890960531436690 ) ) ;
#76642=CARTESIAN_POINT ( 'NONE',  ( -5.049401038297874678, -19.05341960407617918, 89.79275706135230450 ) ) ;
#76643=CARTESIAN_POINT ( 'NONE',  ( -21.55341960407610458, -5.719274019375992779, 66.45724293864768129 ) ) ;
#76645=CARTESIAN_POINT ( 'NONE',  ( 4.379528057220092307, 16.55341960407617563, 47.29275706135234003 ) ) ;
#76646=CARTESIAN_POINT ( 'NONE',  ( 16.46253265017160672, -9.564922557960803928, 33.33224293864770260 ) ) ;
#76647=CARTESIAN_POINT ( 'NONE',  ( 9.474510206698971260, -16.51473224551069308, 107.9155762719810383 ) ) ;
#76649=CARTESIAN_POINT ( 'NONE',  ( 13.97604488694527802, 13.89961937509977652, 39.37390960531435269 ) ) ;
#76650=CARTESIAN_POINT ( 'NONE',  ( -16.53943276465976808, 0.05219959533911058130, 116.2489096053143669 ) ) ;
#76652=CARTESIAN_POINT ( 'NONE',  ( 16.46253265017160672, -9.564922557960803928, 113.3322429386476955 ) ) ;
#76653=CARTESIAN_POINT ( 'NONE',  ( -0.05219959533934338120, 16.53943276465976808, 67.50109039468568994 ) ) ;
#76654=CARTESIAN_POINT ( 'NONE',  ( 21.52544592524344225, -5.823673210054117533, 93.54057627198103830 ) ) ;
#76655=CARTESIAN_POINT ( 'NONE',  ( -16.51473224551069308, -9.474510206698971260, 56.66557627198103120 ) ) ;
#76656=CARTESIAN_POINT ( 'NONE',  ( -21.55341960407619339, 5.719274019375674811, 33.54275706135234714 ) ) ;
#76657=CARTESIAN_POINT ( 'NONE',  ( -16.51473224551069308, -9.474510206698971260, 86.66557627198102409 ) ) ;
#76658=CARTESIAN_POINT ( 'NONE',  ( 16.46253265017160672, -9.564922557960803928, 113.3322429386476955 ) ) ;
#76660=CARTESIAN_POINT ( 'NONE',  ( -21.52544592524334988, -5.823673210054445271, 18.95942372801901143 ) ) ;
#76661=CARTESIAN_POINT ( 'NONE',  ( 9.564922557960805705, 16.46253265017160317, 24.58224293864769194 ) ) ;
#76662=CARTESIAN_POINT ( 'NONE',  ( -9.474510206698964154, 16.51473224551069663, 100.4155762719810241 ) ) ;
#76663=CARTESIAN_POINT ( 'NONE',  ( 0.05219959533936267826, -19.03943276465977164, 95.00109039468567573 ) ) ;
#76664=CARTESIAN_POINT ( 'NONE',  ( 19.05341960407617918, -5.049401038297876454, 26.04275706135233293 ) ) ;
#76665=CARTESIAN_POINT ( 'NONE',  ( -0.05219959533907301413, -21.53943276465977519, 102.4989096053143811 ) ) ;
#76666=CARTESIAN_POINT ( 'NONE',  ( -5.153800228976607833, 19.02544592524334988, 32.70942372801899722 ) ) ;
#76667=CARTESIAN_POINT ( 'NONE',  ( 4.379528057220092307, 16.55341960407617563, 82.29275706135234714 ) ) ;
#76668=CARTESIAN_POINT ( 'NONE',  ( -5.049401038298153566, 19.05341960407611168, 105.2072429386476671 ) ) ;
#76669=ORIENTED_EDGE ( 'NONE', *, *, #78822, .T. ) ;
#76670=CARTESIAN_POINT ( 'NONE',  ( 9.564922557960805705, 16.46253265017160317, 54.58224293864769550 ) ) ;
#76672=CARTESIAN_POINT ( 'NONE',  ( 5.719274019375673035, 21.55341960407619339, 62.29275706135236845 ) ) ;
#76673=CARTESIAN_POINT ( 'NONE',  ( -18.62759615963255300, -10.81492255796106328, 79.16775706135234714 ) ) ;
#76675=CARTESIAN_POINT ( 'NONE',  ( 0.05219959533909260263, 19.03943276465977164, 74.99890960531435269 ) ) ;
#76676=CARTESIAN_POINT ( 'NONE',  ( 5.823673210054444382, -21.52544592524334988, 50.20942372801901854 ) ) ;
#76677=CARTESIAN_POINT ( 'NONE',  ( 9.564922557961047289, -16.46253265017146816, 90.41775706135234714 ) ) ;
#76678=CARTESIAN_POINT ( 'NONE',  ( 16.46253265017160672, -9.564922557960803928, 48.33224293864769550 ) ) ;
#76679=CARTESIAN_POINT ( 'NONE',  ( -16.46253265017160317, 9.564922557960807481, 100.8322429386477097 ) ) ;
#76680=CARTESIAN_POINT ( 'NONE',  ( 13.97604488694527802, 13.89961937509977652, 64.37390960531436690 ) ) ;
#76681=CARTESIAN_POINT ( 'NONE',  ( 17.50000000000009237, -3.443395144217226367, 22.69309096419004845 ) ) ;
#76682=CARTESIAN_POINT ( 'NONE',  ( -16.51473224551069308, -9.474510206698971260, 56.66557627198103120 ) ) ;
#76683=CARTESIAN_POINT ( 'NONE',  ( -21.53943276465977519, 0.05219959533907696930, 101.2489096053143669 ) ) ;
#76684=CARTESIAN_POINT ( 'NONE',  ( -12.06949235617739369, -12.14591786802326823, 84.37609039468570415 ) ) ;
#76686=CARTESIAN_POINT ( 'NONE',  ( 13.97604488694548053, -13.89961937509957401, 45.62609039468566863 ) ) ;
#76687=CARTESIAN_POINT ( 'NONE',  ( 9.474510206698971260, -16.51473224551069308, 67.91557627198102409 ) ) ;
#76688=CARTESIAN_POINT ( 'NONE',  ( 4.379528057220339221, -16.55341960407611168, 62.70724293864769550 ) ) ;
#76689=CARTESIAN_POINT ( 'NONE',  ( 12.06949235617757843, -12.14591786802309237, 93.12390960531436690 ) ) ;
#76690=CARTESIAN_POINT ( 'NONE',  ( 19.05341960407611168, 5.049401038298154454, 113.9572429386477097 ) ) ;
#76691=CARTESIAN_POINT ( 'NONE',  ( -9.564922557960796823, -16.46253265017161027, 102.0822429386477097 ) ) ;
#76692=CARTESIAN_POINT ( 'NONE',  ( -19.03943276465977164, 0.05219959533909376836, 111.2489096053143669 ) ) ;
#76693=CARTESIAN_POINT ( 'NONE',  ( -15.80617190586768217, 15.72974639402176855, 113.1260903946856899 ) ) ;
#76694=CARTESIAN_POINT ( 'NONE',  ( 14.29746914071037800, 8.314922557961029526, 86.66775706135234714 ) ) ;
#76695=CARTESIAN_POINT ( 'NONE',  ( -5.049401038298153566, 19.05341960407611168, 80.20724293864769550 ) ) ;
#76697=CARTESIAN_POINT ( 'NONE',  ( 21.55341960407619695, -5.719274019375665929, 46.04275706135234714 ) ) ;
#76698=CARTESIAN_POINT ( 'NONE',  ( 15.72974639402199770, -15.80617190586745480, 28.12390960531435979 ) ) ;
#76699=CARTESIAN_POINT ( 'NONE',  ( -21.52544592524343514, 5.823673210054127303, 116.0405762719810383 ) ) ;
#76700=CARTESIAN_POINT ( 'NONE',  ( 21.55341960407610458, 5.719274019375980345, 73.95724293864769550 ) ) ;
#76701=CARTESIAN_POINT ( 'NONE',  ( 12.06949235617757843, -12.14591786802309237, 88.12390960531436690 ) ) ;
#76702=CARTESIAN_POINT ( 'NONE',  ( -0.05219959533936034679, 19.03943276465977164, 42.50109039468566152 ) ) ;
#76703=CARTESIAN_POINT ( 'NONE',  ( -5.153800228976328057, -19.02544592524343514, 32.29057627198102409 ) ) ;
#76704=CARTESIAN_POINT ( 'NONE',  ( -0.05219959533909027116, -19.03943276465977164, 77.49890960531435269 ) ) ;
#76705=CARTESIAN_POINT ( 'NONE',  ( -19.05341960407611168, -5.049401038298163336, 76.45724293864769550 ) ) ;
#76707=CARTESIAN_POINT ( 'NONE',  ( 16.55341960407611168, 4.379528057220329451, 98.95724293864770971 ) ) ;
#76709=CARTESIAN_POINT ( 'NONE',  ( 14.34966873604960469, 8.224510206698951720, 34.16557627198102409 ) ) ;
#76710=CARTESIAN_POINT ( 'NONE',  ( -8.314922557961024197, 14.29746914071037800, 32.91775706135234714 ) ) ;
#76711=CARTESIAN_POINT ( 'NONE',  ( -0.05219959533937732626, 21.53943276465977519, 92.50109039468567573 ) ) ;
#76712=CARTESIAN_POINT ( 'NONE',  ( -19.05341960407611168, -5.049401038298163336, 101.4572429386476955 ) ) ;
#76713=CARTESIAN_POINT ( 'NONE',  ( -21.55341960407619339, 5.719274019375674811, 23.54275706135235424 ) ) ;
#76714=CARTESIAN_POINT ( 'NONE',  ( -16.46253265017160317, 9.564922557960807481, 40.83224293864769550 ) ) ;
#76715=CARTESIAN_POINT ( 'NONE',  ( -8.224510206698735004, -14.34966873604973081, 34.58442372801900433 ) ) ;
#76716=CARTESIAN_POINT ( 'NONE',  ( 0.05219959533936267826, -19.03943276465977164, 110.0010903946856757 ) ) ;
#76717=CARTESIAN_POINT ( 'NONE',  ( -18.67979575497178146, -10.72451020669898902, 101.6655762719810383 ) ) ;
#76718=CARTESIAN_POINT ( 'NONE',  ( 19.02544592524334988, 5.153800228976608722, 71.45942372801900433 ) ) ;
#76720=CARTESIAN_POINT ( 'NONE',  ( 5.823673210054125526, 21.52544592524343514, 114.7905762719810383 ) ) ;
#76721=CARTESIAN_POINT ( 'NONE',  ( 13.89961937509978007, -13.97604488694527269, 73.12390960531436690 ) ) ;
#76722=CARTESIAN_POINT ( 'NONE',  ( 19.05341960407611168, 5.049401038298154454, 93.95724293864769550 ) ) ;
#76724=B_SPLINE_CURVE_WITH_KNOTS ( 'NONE', 3,
 ( #82250, #68099, #143941, #7418, #175290, #129751, #37769, #193463, #99431, #22609, #84255, #54940, #145937, #177307, #69102, #130768, #192460, #53943, #135784, #134796, #136753, #28612, #10447, #167111, #71112, #74114, #196477, #86270, #121578, #179311, #73127, #181301 ),
 .UNSPECIFIED., .F., .F.,
 ( 4, 2, 2, 2, 2, 2, 2, 2, 2, 2, 2, 2, 2, 2, 2, 4 ),
 ( 2.281672496420497865E-17, 0.0003712461730036837964, 0.0007424923460073447161, 0.001113738519011005582, 0.001484984692014666664, 0.002227477038022000321, 0.002598723211025685039, 0.002969969384029369323, 0.003341215557033053608, 0.003712461730036737458, 0.004083707903040420875, 0.004454954076044104726, 0.004826200249047788576, 0.005197446422051473294, 0.005568692595055157145, 0.005939938768058841863 ),
 .UNSPECIFIED. ) ;
#76725=CARTESIAN_POINT ( 'NONE',  ( -16.51473224551069308, -9.474510206698971260, 81.66557627198103830 ) ) ;
#76726=CARTESIAN_POINT ( 'NONE',  ( 15.72974639402176855, 15.80617190586768217, 31.87609039468567929 ) ) ;
#76727=CARTESIAN_POINT ( 'NONE',  ( 16.53943276465976808, -0.05219959533910856209, 73.74890960531433848 ) ) ;
#76728=CARTESIAN_POINT ( 'NONE',  ( 13.89961937509977652, -13.97604488694527269, 83.12390960531436690 ) ) ;
#76729=CARTESIAN_POINT ( 'NONE',  ( 12.14591786802327356, -12.06949235617739191, 55.62609039468568284 ) ) ;
#76730=CARTESIAN_POINT ( 'NONE',  ( 13.97604488694548053, -13.89961937509957401, 60.62609039468564731 ) ) ;
#76731=CARTESIAN_POINT ( 'NONE',  ( 21.52544592524334988, 5.823673210054432836, 66.45942372801903275 ) ) ;
#76732=CARTESIAN_POINT ( 'NONE',  ( -16.52544592524335698, -4.483927247898792601, 23.95942372801901143 ) ) ;
#76733=CARTESIAN_POINT ( 'NONE',  ( -16.46253265017160317, 9.564922557960807481, 65.83224293864769550 ) ) ;
#76734=CARTESIAN_POINT ( 'NONE',  ( 19.05341960407617918, -5.049401038297876454, 96.04275706135231871 ) ) ;
#76735=CARTESIAN_POINT ( 'NONE',  ( 0.05219959533934541429, -16.53943276465976808, 60.00109039468568284 ) ) ;
#76736=CARTESIAN_POINT ( 'NONE',  ( -21.55341960407619339, 5.719274019375674811, 93.54275706135234714 ) ) ;
#76738=CARTESIAN_POINT ( 'NONE',  ( -9.564922557961040184, 16.46253265017147172, 82.91775706135233293 ) ) ;
#76739=CARTESIAN_POINT ( 'NONE',  ( 5.049401038298161559, -19.05341960407611168, 52.70724293864767418 ) ) ;
#76740=CARTESIAN_POINT ( 'NONE',  ( -5.823673210054116645, -21.52544592524344225, 72.29057627198102409 ) ) ;
#76741=CARTESIAN_POINT ( 'NONE',  ( 4.379528057220339221, -16.55341960407611168, 72.70724293864769550 ) ) ;
#76742=CARTESIAN_POINT ( 'NONE',  ( -16.51473224551082808, 9.474510206698731452, 78.33442372801900433 ) ) ;
#76744=CARTESIAN_POINT ( 'NONE',  ( 0.05219959533936267826, -19.03943276465977164, 45.00109039468566863 ) ) ;
#76745=CARTESIAN_POINT ( 'NONE',  ( -8.224510206698948167, 14.34966873604960824, 25.41557627198103120 ) ) ;
#76746=CARTESIAN_POINT ( 'NONE',  ( 12.14591786802309770, 12.06949235617756955, 64.37390960531435269 ) ) ;
#76747=CARTESIAN_POINT ( 'NONE',  ( 15.80617190586769283, -15.72974639402175789, 105.6260903946856899 ) ) ;
#76749=CARTESIAN_POINT ( 'NONE',  ( -15.80617190586745835, -15.72974639402198527, 111.8739096053143669 ) ) ;
#76750=CARTESIAN_POINT ( 'NONE',  ( -13.97604488694527625, -13.89961937509977652, 61.87390960531435979 ) ) ;
#76751=CARTESIAN_POINT ( 'NONE',  ( 0.05219959533937995610, -21.53943276465977519, 85.00109039468568994 ) ) ;
#76752=CARTESIAN_POINT ( 'NONE',  ( -13.97604488694527625, -13.89961937509977652, 61.87390960531435979 ) ) ;
#76753=CARTESIAN_POINT ( 'NONE',  ( -9.474510206698964154, 16.51473224551069663, 30.41557627198102054 ) ) ;
#76754=CARTESIAN_POINT ( 'NONE',  ( 0.05219959533907565091, 21.53943276465977519, 29.99890960531435979 ) ) ;
#76755=CARTESIAN_POINT ( 'NONE',  ( -16.55341960407611168, -4.379528057220339221, 71.45724293864769550 ) ) ;
#76756=CARTESIAN_POINT ( 'NONE',  ( 0.05219959533909260263, 19.03943276465977164, 34.99890960531435979 ) ) ;
#76757=CARTESIAN_POINT ( 'NONE',  ( -14.29746914071049879, 8.314922557960819915, 85.83224293864768129 ) ) ;
#76759=CARTESIAN_POINT ( 'NONE',  ( -0.05219959533907301413, -21.53943276465977519, 97.49890960531436690 ) ) ;
#76760=CARTESIAN_POINT ( 'NONE',  ( 5.823673210054444382, -21.52544592524334988, 45.20942372801901854 ) ) ;
#76763=CARTESIAN_POINT ( 'NONE',  ( 14.34966873604972726, -8.224510206698740333, 55.83442372801901854 ) ) ;
#76764=CARTESIAN_POINT ( 'NONE',  ( -21.52544592524343514, 5.823673210054127303, 101.0405762719810383 ) ) ;
#76765=CARTESIAN_POINT ( 'NONE',  ( 16.51473224551083163, -9.474510206698727899, 30.83442372801900433 ) ) ;
#76766=CARTESIAN_POINT ( 'NONE',  ( -5.049401038298153566, 19.05341960407611168, 40.20724293864768839 ) ) ;
#76767=CARTESIAN_POINT ( 'NONE',  ( -16.51473224551069308, -9.474510206698971260, 101.6655762719810241 ) ) ;
#76768=CARTESIAN_POINT ( 'NONE',  ( 18.67979575497194134, -10.72451020669871369, 60.83442372801901854 ) ) ;
#76769=CARTESIAN_POINT ( 'NONE',  ( -15.72974639402197994, 15.80617190586746368, 40.62390960531435269 ) ) ;
#76770=CARTESIAN_POINT ( 'NONE',  ( 14.29746914071037800, 8.314922557961029526, 111.6677570613523613 ) ) ;
#76771=CARTESIAN_POINT ( 'NONE',  ( -5.823673210054431948, 21.52544592524334988, 62.70942372801902565 ) ) ;
#76772=CARTESIAN_POINT ( 'NONE',  ( -5.823673210054431948, 21.52544592524334988, 97.70942372801904696 ) ) ;
#76773=CARTESIAN_POINT ( 'NONE',  ( 0.05219959533936267826, -19.03943276465977164, 30.00109039468566863 ) ) ;
#76774=CARTESIAN_POINT ( 'NONE',  ( -0.05219959533934338120, 16.53943276465976808, 92.50109039468567573 ) ) ;
#76775=CARTESIAN_POINT ( 'NONE',  ( -21.52544592524334988, -5.823673210054445271, 53.95942372801900433 ) ) ;
#76776=CARTESIAN_POINT ( 'NONE',  ( -19.02544592524342804, 5.153800228976336051, 46.04057627198101699 ) ) ;
#76777=CARTESIAN_POINT ( 'NONE',  ( -10.81492255796105439, 18.62759615963255655, 112.9177570613523329 ) ) ;
#76778=CARTESIAN_POINT ( 'NONE',  ( 19.03943276465977164, -0.05219959533909143690, 113.7489096053143669 ) ) ;
#76780=CARTESIAN_POINT ( 'NONE',  ( -5.719274019375978568, 21.55341960407610458, 110.2072429386477239 ) ) ;
#76781=CARTESIAN_POINT ( 'NONE',  ( 21.55341960407610458, 5.719274019375980345, 68.95724293864769550 ) ) ;
#76782=CARTESIAN_POINT ( 'NONE',  ( 14.34966873604972726, -8.224510206698740333, 40.83442372801901854 ) ) ;
#76783=LINE ( 'NONE', #125285, #67649 ) ;
#76784=CARTESIAN_POINT ( 'NONE',  ( 5.823673210054125526, 21.52544592524343514, 74.79057627198105251 ) ) ;
#76785=CARTESIAN_POINT ( 'NONE',  ( 4.379528057220092307, 16.55341960407617563, 67.29275706135234714 ) ) ;
#76786=CARTESIAN_POINT ( 'NONE',  ( -12.14591786802309592, -12.06949235617757132, 61.87390960531436690 ) ) ;
#76788=CARTESIAN_POINT ( 'NONE',  ( 13.97604488694548053, -13.89961937509957401, 110.6260903946856615 ) ) ;
#76789=CARTESIAN_POINT ( 'NONE',  ( 21.52544592524344225, -5.823673210054117533, 38.54057627198103120 ) ) ;
#76791=CARTESIAN_POINT ( 'NONE',  ( 8.224510206698742110, 14.34966873604972548, 42.08442372801901854 ) ) ;
#76792=CARTESIAN_POINT ( 'NONE',  ( -10.72451020669898014, 18.67979575497178502, 110.4155762719810383 ) ) ;
#76793=CARTESIAN_POINT ( 'NONE',  ( -10.72451020669898014, 18.67979575497178502, 35.41557627198102409 ) ) ;
#76794=CARTESIAN_POINT ( 'NONE',  ( -16.52544592524335698, -4.483927247898792601, 58.95942372801902565 ) ) ;
#76795=CARTESIAN_POINT ( 'NONE',  ( 16.46253265017160672, -9.564922557960803928, 78.33224293864769550 ) ) ;
#76796=CARTESIAN_POINT ( 'NONE',  ( -15.80617190586768217, 15.72974639402176855, 43.12609039468568284 ) ) ;
#76797=CARTESIAN_POINT ( 'NONE',  ( -19.03943276465977164, -0.05219959533935918106, 108.7510903946856615 ) ) ;
#76798=CARTESIAN_POINT ( 'NONE',  ( -10.72451020669898014, 18.67979575497178502, 25.41557627198103120 ) ) ;
#76799=ORIENTED_EDGE ( 'NONE', *, *, #99588, .T. ) ;
#76800=CARTESIAN_POINT ( 'NONE',  ( -19.05341960407617563, 5.049401038297882671, 28.54275706135232937 ) ) ;
#76801=CARTESIAN_POINT ( 'NONE',  ( -0.05219959533934338120, 16.53943276465976808, 37.50109039468568284 ) ) ;
#76802=CARTESIAN_POINT ( 'NONE',  ( -13.89961937509977652, 13.97604488694528158, 95.62390960531436690 ) ) ;
#76803=CARTESIAN_POINT ( 'NONE',  ( 15.80617190586746368, 15.72974639402197994, 109.3739096053143811 ) ) ;
#76804=CARTESIAN_POINT ( 'NONE',  ( 16.51473224551069308, 9.474510206698969483, 74.16557627198103830 ) ) ;
#76806=CARTESIAN_POINT ( 'NONE',  ( -16.53943276465976808, 0.05219959533911058130, 81.24890960531436690 ) ) ;
#76807=CARTESIAN_POINT ( 'NONE',  ( -5.719274019375978568, 21.55341960407610458, 40.20724293864769550 ) ) ;
#76809=CARTESIAN_POINT ( 'NONE',  ( 0.05219959533934541429, -16.53943276465976808, 65.00109039468568994 ) ) ;
#76810=CARTESIAN_POINT ( 'NONE',  ( -18.67979575497178146, -10.72451020669898902, 106.6655762719810383 ) ) ;
#76811=CARTESIAN_POINT ( 'NONE',  ( 16.51473224551083163, -9.474510206698727899, 80.83442372801899012 ) ) ;
#76812=CARTESIAN_POINT ( 'NONE',  ( 19.03943276465977164, -0.05219959533909143690, 33.74890960531435979 ) ) ;
#76813=CARTESIAN_POINT ( 'NONE',  ( 18.67979575497178502, 10.72451020669898547, 69.16557627198102409 ) ) ;
#76814=CARTESIAN_POINT ( 'NONE',  ( -19.05341960407611168, -5.049401038298163336, 96.45724293864769550 ) ) ;
#76815=CARTESIAN_POINT ( 'NONE',  ( 15.80617190586769283, -15.72974639402175789, 95.62609039468568994 ) ) ;
#76816=CARTESIAN_POINT ( 'NONE',  ( -16.46253265017160317, 9.564922557960807481, 60.83224293864769550 ) ) ;
#76817=CARTESIAN_POINT ( 'NONE',  ( -14.34966873604972548, 8.224510206698743886, 43.33442372801901143 ) ) ;
#76818=CARTESIAN_POINT ( 'NONE',  ( 13.97604488694527802, 13.89961937509977652, 54.37390960531435979 ) ) ;
#76819=CARTESIAN_POINT ( 'NONE',  ( -10.72451020669870658, -18.67979575497194134, 79.58442372801903275 ) ) ;
#76821=CARTESIAN_POINT ( 'NONE',  ( -19.02544592524334988, -5.153800228976617603, 43.95942372801899012 ) ) ;
#76822=CARTESIAN_POINT ( 'NONE',  ( -9.474510206698720793, -16.51473224551083518, 59.58442372801900433 ) ) ;
#76823=CARTESIAN_POINT ( 'NONE',  ( -5.823673210054431948, 21.52544592524334988, 52.70942372801902565 ) ) ;
#76825=CARTESIAN_POINT ( 'NONE',  ( 13.89961937509957401, 13.97604488694547697, 41.87609039468566152 ) ) ;
#76826=CARTESIAN_POINT ( 'NONE',  ( -9.564922557960796823, -16.46253265017161027, 97.08224293864769550 ) ) ;
#76827=CARTESIAN_POINT ( 'NONE',  ( -16.51473224551069308, -9.474510206698971260, 66.66557627198102409 ) ) ;
#76828=CARTESIAN_POINT ( 'NONE',  ( 12.06949235617739724, 12.14591786802326823, 111.8760903946856615 ) ) ;
#76829=CARTESIAN_POINT ( 'NONE',  ( 21.55341960407610458, 5.719274019375980345, 23.95724293864769550 ) ) ;
#76830=CARTESIAN_POINT ( 'NONE',  ( 10.81492255796106328, -18.62759615963255655, 90.41775706135236135 ) ) ;
#76832=CARTESIAN_POINT ( 'NONE',  ( 16.88567814943164791, 6.947325034625594142, 58.79001122652586275 ) ) ;
#76833=CARTESIAN_POINT ( 'NONE',  ( -10.81492255796105439, 18.62759615963255655, 102.9177570613523756 ) ) ;
#76835=CARTESIAN_POINT ( 'NONE',  ( 16.55341960407611168, 4.379528057220329451, 113.9572429386477239 ) ) ;
#76838=CARTESIAN_POINT ( 'NONE',  ( 8.314922557961029526, -14.29746914071037800, 55.41775706135234714 ) ) ;
#76839=CARTESIAN_POINT ( 'NONE',  ( 0.05219959533907565091, 21.53943276465977519, 69.99890960531435269 ) ) ;
#76840=CARTESIAN_POINT ( 'NONE',  ( -0.05219959533910754901, -16.53943276465976808, 42.49890960531435979 ) ) ;
#76841=CARTESIAN_POINT ( 'NONE',  ( -4.379528057220328563, 16.55341960407611168, 105.2072429386477097 ) ) ;
#76842=CARTESIAN_POINT ( 'NONE',  ( -19.05341960407611168, -5.049401038298163336, 96.45724293864769550 ) ) ;
#76843=CARTESIAN_POINT ( 'NONE',  ( 16.46253265017146816, 9.564922557961045513, 31.66775706135232937 ) ) ;
#76844=CARTESIAN_POINT ( 'NONE',  ( 8.224510206698953496, -14.34966873604960469, 112.9155762719810383 ) ) ;
#76845=CARTESIAN_POINT ( 'NONE',  ( -18.67979575497193778, 10.72451020669871902, 73.33442372801901854 ) ) ;
#76846=CARTESIAN_POINT ( 'NONE',  ( -13.97604488694527625, -13.89961937509977830, 96.87390960531435269 ) ) ;
#76847=CARTESIAN_POINT ( 'NONE',  ( -8.314922557961024197, 14.29746914071037800, 112.9177570613523329 ) ) ;
#76848=CARTESIAN_POINT ( 'NONE',  ( 17.58332526062524437, 7.635886036038643354, 66.57665040441534643 ) ) ;
#76849=CARTESIAN_POINT ( 'NONE',  ( 21.55341960407610458, 5.719274019375980345, 28.95724293864769905 ) ) ;
#76850=CARTESIAN_POINT ( 'NONE',  ( 8.224510206698953496, -14.34966873604960469, 92.91557627198103830 ) ) ;
#76851=CARTESIAN_POINT ( 'NONE',  ( -9.474510206698720793, -16.51473224551083518, 54.58442372801899722 ) ) ;
#76852=CARTESIAN_POINT ( 'NONE',  ( -13.89961937509977652, 13.97604488694528158, 75.62390960531438111 ) ) ;
#76853=CARTESIAN_POINT ( 'NONE',  ( 8.224510206698953496, -14.34966873604960469, 72.91557627198103830 ) ) ;
#76854=CARTESIAN_POINT ( 'NONE',  ( 19.03943276465977164, 0.05219959533936151252, 86.25109039468567573 ) ) ;
#76855=CARTESIAN_POINT ( 'NONE',  ( 21.55341960407610458, 5.719274019375980345, 43.95724293864769550 ) ) ;
#76857=CARTESIAN_POINT ( 'NONE',  ( -0.05219959533909027116, -19.03943276465977164, 22.49890960531436690 ) ) ;
#76858=CARTESIAN_POINT ( 'NONE',  ( -17.49999999999999645, -5.500000000000005329, 31.28230962303567253 ) ) ;
#76860=CARTESIAN_POINT ( 'NONE',  ( -5.153800228976328057, -19.02544592524343514, 67.29057627198102409 ) ) ;
#76861=CARTESIAN_POINT ( 'NONE',  ( -10.81492255796078084, -18.62759615963271287, 77.08224293864769550 ) ) ;
#76862=CARTESIAN_POINT ( 'NONE',  ( 8.314922557961029526, -14.29746914071037800, 90.41775706135236135 ) ) ;
#76863=CARTESIAN_POINT ( 'NONE',  ( -9.564922557960796823, -16.46253265017161027, 92.08224293864769550 ) ) ;
#76864=CARTESIAN_POINT ( 'NONE',  ( -19.05341960407617563, 5.049401038297882671, 73.54275706135233293 ) ) ;
#76865=CARTESIAN_POINT ( 'NONE',  ( 18.62759615963255655, 10.81492255796105972, 86.66775706135234714 ) ) ;
#76866=CARTESIAN_POINT ( 'NONE',  ( -5.823673210054116645, -21.52544592524344225, 57.29057627198103120 ) ) ;
#76867=CARTESIAN_POINT ( 'NONE',  ( -10.72451020669898014, 18.67979575497178502, 30.41557627198101699 ) ) ;
#76868=CARTESIAN_POINT ( 'NONE',  ( 9.474510206698971260, -16.51473224551069308, 32.91557627198102409 ) ) ;
#76869=CARTESIAN_POINT ( 'NONE',  ( -0.05219959533934338120, 16.53943276465976808, 102.5010903946856899 ) ) ;
#76870=CARTESIAN_POINT ( 'NONE',  ( -5.049401038298153566, 19.05341960407611168, 45.20724293864769550 ) ) ;
#76871=CARTESIAN_POINT ( 'NONE',  ( -13.97604488694547697, 13.89961937509957934, 113.1260903946856757 ) ) ;
#76872=CARTESIAN_POINT ( 'NONE',  ( 17.31728774477272736, 6.344390552232407110, 51.68093348310683410 ) ) ;
#76873=CARTESIAN_POINT ( 'NONE',  ( -10.81492255796105439, 18.62759615963255655, 107.9177570613523471 ) ) ;
#76874=CARTESIAN_POINT ( 'NONE',  ( -14.34966873604960291, -8.224510206698953496, 56.66557627198103830 ) ) ;
#76875=CARTESIAN_POINT ( 'NONE',  ( 18.62759615963271287, -10.81492255796078972, 103.3322429386476955 ) ) ;
#76876=CARTESIAN_POINT ( 'NONE',  ( -21.55341960407610458, -5.719274019375992779, 106.4572429386477097 ) ) ;
#76878=CARTESIAN_POINT ( 'NONE',  ( 21.53943276465977519, -0.05219959533907433946, 43.74890960531435979 ) ) ;
#76879=CARTESIAN_POINT ( 'NONE',  ( 4.483927247898790824, -16.52544592524335698, 75.20942372801901854 ) ) ;
#76880=CARTESIAN_POINT ( 'NONE',  ( 4.379528057220339221, -16.55341960407611168, 92.70724293864770971 ) ) ;
#76881=CARTESIAN_POINT ( 'NONE',  ( 19.05341960407611168, 5.049401038298154454, 53.95724293864770260 ) ) ;
#76883=CARTESIAN_POINT ( 'NONE',  ( -4.483927247898782831, 16.52544592524335698, 107.7094237280190328 ) ) ;
#76884=CARTESIAN_POINT ( 'NONE',  ( 21.53943276465977519, 0.05219959533937863772, 36.25109039468567573 ) ) ;
#76885=CARTESIAN_POINT ( 'NONE',  ( -5.049401038298153566, 19.05341960407611168, 95.20724293864770971 ) ) ;
#76886=CARTESIAN_POINT ( 'NONE',  ( -15.80617190586768217, 15.72974639402176855, 63.12609039468568994 ) ) ;
#76888=CARTESIAN_POINT ( 'NONE',  ( -19.03943276465977164, 0.05219959533909376836, 21.24890960531436335 ) ) ;
#76890=CARTESIAN_POINT ( 'NONE',  ( 5.823673210054444382, -21.52544592524334988, 60.20942372801902565 ) ) ;
#76891=CARTESIAN_POINT ( 'NONE',  ( -9.474510206698964154, 16.51473224551069663, 45.41557627198103120 ) ) ;
#76892=CARTESIAN_POINT ( 'NONE',  ( -9.474510206698964154, 16.51473224551069663, 95.41557627198102409 ) ) ;
#76893=CARTESIAN_POINT ( 'NONE',  ( -19.05341960407617563, 5.049401038297882671, 68.54275706135230450 ) ) ;
#76894=CARTESIAN_POINT ( 'NONE',  ( 21.55341960407619695, -5.719274019375665929, 36.04275706135234714 ) ) ;
#76895=CARTESIAN_POINT ( 'NONE',  ( 13.89961937509957401, 13.97604488694547697, 106.8760903946856757 ) ) ;
#76896=CARTESIAN_POINT ( 'NONE',  ( -16.51473224551082808, 9.474510206698731452, 78.33442372801900433 ) ) ;
#76897=CARTESIAN_POINT ( 'NONE',  ( -9.564922557960796823, -16.46253265017161027, 42.08224293864769550 ) ) ;
#76898=CARTESIAN_POINT ( 'NONE',  ( -19.02544592524334988, -5.153800228976617603, 78.95942372801900433 ) ) ;
#76899=CARTESIAN_POINT ( 'NONE',  ( -8.224510206698735004, -14.34966873604973081, 99.58442372801900433 ) ) ;
#76900=CARTESIAN_POINT ( 'NONE',  ( 5.049401038297881783, 19.05341960407617563, 72.29275706135234714 ) ) ;
#76901=CARTESIAN_POINT ( 'NONE',  ( -14.29746914071049879, 8.314922557960819915, 40.83224293864769550 ) ) ;
#76902=CARTESIAN_POINT ( 'NONE',  ( -16.51473224551082808, 9.474510206698731452, 48.33442372801900433 ) ) ;
#76903=CARTESIAN_POINT ( 'NONE',  ( 18.67979575497194134, -10.72451020669871369, 100.8344237280190185 ) ) ;
#76904=CARTESIAN_POINT ( 'NONE',  ( -13.97604488694547697, 13.89961937509957934, 28.12609039468565797 ) ) ;
#76905=CARTESIAN_POINT ( 'NONE',  ( 5.153800228976335163, 19.02544592524342804, 34.79057627198102409 ) ) ;
#76906=CARTESIAN_POINT ( 'NONE',  ( 15.72974639402176855, 15.80617190586768217, 86.87609039468568994 ) ) ;
#76907=CARTESIAN_POINT ( 'NONE',  ( 14.34966873604972726, -8.224510206698740333, 40.83442372801901854 ) ) ;
#76908=CARTESIAN_POINT ( 'NONE',  ( -0.05219959533909027116, -19.03943276465977164, 87.49890960531436690 ) ) ;
#76910=CARTESIAN_POINT ( 'NONE',  ( -16.46253265017160317, 9.564922557960807481, 80.83224293864769550 ) ) ;
#76911=LINE ( 'NONE', #141572, #32936 ) ;
#76913=CARTESIAN_POINT ( 'NONE',  ( -5.049401038297874678, -19.05341960407617918, 84.79275706135233293 ) ) ;
#76914=CARTESIAN_POINT ( 'NONE',  ( -21.55341960407610458, -5.719274019375992779, 21.45724293864769550 ) ) ;
#76915=CARTESIAN_POINT ( 'NONE',  ( 5.823673210054444382, -21.52544592524334988, 110.2094237280190185 ) ) ;
#76916=CARTESIAN_POINT ( 'NONE',  ( 5.153800228976615827, -19.02544592524334988, 95.20942372801897591 ) ) ;
#76917=CARTESIAN_POINT ( 'NONE',  ( -8.314922557960811034, -14.29746914071050412, 102.0822429386476955 ) ) ;
#76918=CARTESIAN_POINT ( 'NONE',  ( 5.049401038298161559, -19.05341960407611168, 22.70724293864769194 ) ) ;
#76919=CARTESIAN_POINT ( 'NONE',  ( -21.53943276465977519, 0.05219959533907696930, 61.24890960531435979 ) ) ;
#76920=CARTESIAN_POINT ( 'NONE',  ( 21.55341960407610458, 5.719274019375980345, 48.95724293864770971 ) ) ;
#76921=CARTESIAN_POINT ( 'NONE',  ( -14.29746914071049879, 8.314922557960819915, 115.8322429386477097 ) ) ;
#76923=CARTESIAN_POINT ( 'NONE',  ( 13.97604488694548053, -13.89961937509957401, 75.62609039468564731 ) ) ;
#76924=CARTESIAN_POINT ( 'NONE',  ( -16.55341960407611168, -4.379528057220339221, 46.45724293864769550 ) ) ;
#76926=CARTESIAN_POINT ( 'NONE',  ( -21.53943276465977519, 0.05219959533907696930, 21.24890960531436690 ) ) ;
#76928=CARTESIAN_POINT ( 'NONE',  ( 0.05219959533937995610, -21.53943276465977519, 85.00109039468568994 ) ) ;
#76929=CARTESIAN_POINT ( 'NONE',  ( 18.67979575497178502, 10.72451020669898547, 74.16557627198102409 ) ) ;
#76930=CARTESIAN_POINT ( 'NONE',  ( 5.823673210054444382, -21.52544592524334988, 65.20942372801901854 ) ) ;
#76931=CARTESIAN_POINT ( 'NONE',  ( -15.80617190586768217, 15.72974639402176855, 48.12609039468568284 ) ) ;
#76932=CARTESIAN_POINT ( 'NONE',  ( -0.05219959533909027116, -19.03943276465977164, 82.49890960531436690 ) ) ;
#76933=CARTESIAN_POINT ( 'NONE',  ( 16.55341960407618274, -4.379528057220086978, 96.04275706135236135 ) ) ;
#76934=CARTESIAN_POINT ( 'NONE',  ( -12.14591786802309592, -12.06949235617757132, 111.8739096053143669 ) ) ;
#76936=CARTESIAN_POINT ( 'NONE',  ( -8.224510206698948167, 14.34966873604960824, 65.41557627198102409 ) ) ;
#76937=CARTESIAN_POINT ( 'NONE',  ( -14.34966873604960291, -8.224510206698953496, 31.66557627198102054 ) ) ;
#76938=CARTESIAN_POINT ( 'NONE',  ( 5.153800228976335163, 19.02544592524342804, 64.79057627198100988 ) ) ;
#76939=CARTESIAN_POINT ( 'NONE',  ( 19.03943276465977164, -0.05219959533909143690, 38.74890960531436690 ) ) ;
#76940=CARTESIAN_POINT ( 'NONE',  ( -18.62759615963270932, 10.81492255796079327, 40.83224293864769550 ) ) ;
#76941=CARTESIAN_POINT ( 'NONE',  ( -5.153800228976607833, 19.02544592524334988, 32.70942372801899722 ) ) ;
#76943=CARTESIAN_POINT ( 'NONE',  ( 16.52544592524342804, -4.483927247898539470, 48.54057627198103120 ) ) ;
#76944=CARTESIAN_POINT ( 'NONE',  ( -18.67979575497178146, -10.72451020669898902, 26.66557627198103475 ) ) ;
#76945=DIRECTION ( 'NONE',  ( 0.000000000000000000, 0.000000000000000000, 1.000000000000000000 ) ) ;
#76946=CARTESIAN_POINT ( 'NONE',  ( -4.483927247898782831, 16.52544592524335698, 77.70942372801900433 ) ) ;
#76947=CARTESIAN_POINT ( 'NONE',  ( 9.564922557961047289, -16.46253265017146816, 80.41775706135234714 ) ) ;
#76949=CARTESIAN_POINT ( 'NONE',  ( -12.06949235617756955, 12.14591786802309770, 45.62390960531436690 ) ) ;
#76950=CARTESIAN_POINT ( 'NONE',  ( 16.21995358207308158, -7.366697692864041969, 52.43551001512160781 ) ) ;
#76951=CARTESIAN_POINT ( 'NONE',  ( 4.379528057220339221, -16.55341960407611168, 27.70724293864769905 ) ) ;
#76952=CARTESIAN_POINT ( 'NONE',  ( 19.03943276465977164, -0.05219959533909143690, 48.74890960531435979 ) ) ;
#76953=CARTESIAN_POINT ( 'NONE',  ( 0.05219959533909260263, 19.03943276465977164, 79.99890960531436690 ) ) ;
#76954=CARTESIAN_POINT ( 'NONE',  ( 16.51473224551069308, 9.474510206698969483, 44.16557627198103120 ) ) ;
#76955=CARTESIAN_POINT ( 'NONE',  ( 18.62759615963255655, 10.81492255796105972, 41.66775706135235424 ) ) ;
#76956=CARTESIAN_POINT ( 'NONE',  ( 19.03943276465977164, -0.05219959533909143690, 58.74890960531435979 ) ) ;
#76958=CARTESIAN_POINT ( 'NONE',  ( -13.97604488694527625, -13.89961937509977652, 46.87390960531435979 ) ) ;
#76959=CARTESIAN_POINT ( 'NONE',  ( -21.53943276465977519, 0.05219959533907696930, 41.24890960531435269 ) ) ;
#76960=CARTESIAN_POINT ( 'NONE',  ( 18.62759615963255655, 10.81492255796105972, 71.66775706135234714 ) ) ;
#76961=CARTESIAN_POINT ( 'NONE',  ( 12.14591786802309770, 12.06949235617756955, 114.3739096053143527 ) ) ;
#76962=CARTESIAN_POINT ( 'NONE',  ( -5.719274019375978568, 21.55341960407610458, 25.20724293864769550 ) ) ;
#76963=CARTESIAN_POINT ( 'NONE',  ( -0.05219959533934338120, 16.53943276465976808, 97.50109039468567573 ) ) ;
#76964=CARTESIAN_POINT ( 'NONE',  ( -15.72974639402176322, -15.80617190586768395, 99.37609039468568994 ) ) ;
#76965=CARTESIAN_POINT ( 'NONE',  ( 14.34966873604972726, -8.224510206698740333, 65.83442372801900433 ) ) ;
#76966=CARTESIAN_POINT ( 'NONE',  ( -0.05219959533909027116, -19.03943276465977164, 112.4989096053143669 ) ) ;
#76967=CARTESIAN_POINT ( 'NONE',  ( 4.483927247898790824, -16.52544592524335698, 55.20942372801902565 ) ) ;
#76968=CARTESIAN_POINT ( 'NONE',  ( -14.29746914071037622, -8.314922557961029526, 39.16775706135235424 ) ) ;
#76969=CARTESIAN_POINT ( 'NONE',  ( -8.314922557961024197, 14.29746914071037800, 97.91775706135236135 ) ) ;
#76970=CARTESIAN_POINT ( 'NONE',  ( -21.53943276465977519, -0.05219959533937600094, 58.75109039468568994 ) ) ;
#76971=CARTESIAN_POINT ( 'NONE',  ( 14.29746914071037800, 8.314922557961029526, 26.66775706135235424 ) ) ;
#76972=CARTESIAN_POINT ( 'NONE',  ( -10.72451020669898014, 18.67979575497178502, 110.4155762719810383 ) ) ;
#76973=CARTESIAN_POINT ( 'NONE',  ( 16.55341960407618274, -4.379528057220086978, 21.04275706135234714 ) ) ;
#76974=CARTESIAN_POINT ( 'NONE',  ( -14.34966873604972548, 8.224510206698743886, 83.33442372801903275 ) ) ;
#76975=CARTESIAN_POINT ( 'NONE',  ( -17.44279575226787316, 5.990770900253887810, 45.83557567514318976 ) ) ;
#76976=CARTESIAN_POINT ( 'NONE',  ( 21.52544592524334988, 5.823673210054432836, 81.45942372801900433 ) ) ;
#76977=CARTESIAN_POINT ( 'NONE',  ( -19.05341960407617563, 5.049401038297882671, 88.54275706135230450 ) ) ;
#76978=CARTESIAN_POINT ( 'NONE',  ( 16.52544592524342804, -4.483927247898539470, 58.54057627198103120 ) ) ;
#76979=CARTESIAN_POINT ( 'NONE',  ( -8.224510206698948167, 14.34966873604960824, 40.41557627198103120 ) ) ;
#76980=CARTESIAN_POINT ( 'NONE',  ( -16.52544592524342804, 4.483927247898546575, 101.0405762719810383 ) ) ;
#76981=CARTESIAN_POINT ( 'NONE',  ( -5.049401038297874678, -19.05341960407617918, 49.79275706135231871 ) ) ;
#76983=CARTESIAN_POINT ( 'NONE',  ( 5.719274019375673035, 21.55341960407619339, 47.29275706135234003 ) ) ;
#76984=CARTESIAN_POINT ( 'NONE',  ( -5.153800228976607833, 19.02544592524334988, 107.7094237280189759 ) ) ;
#76986=CARTESIAN_POINT ( 'NONE',  ( 13.97604488694527802, 13.89961937509977652, 99.37390960531436690 ) ) ;
#76987=CARTESIAN_POINT ( 'NONE',  ( 21.53943276465977519, -0.05219959533907433946, 73.74890960531433848 ) ) ;
#76988=CARTESIAN_POINT ( 'NONE',  ( 13.89961937509957401, 13.97604488694547697, 96.87609039468566152 ) ) ;
#76989=CARTESIAN_POINT ( 'NONE',  ( -13.89961937509977652, 13.97604488694528158, 105.6239096053143527 ) ) ;
#76990=CARTESIAN_POINT ( 'NONE',  ( 5.153800228976617603, -19.02544592524335343, 50.20942372801899012 ) ) ;
#76991=CARTESIAN_POINT ( 'NONE',  ( 12.14591786802309770, 12.06949235617756955, 104.3739096053143669 ) ) ;
#76992=CARTESIAN_POINT ( 'NONE',  ( 10.81492255796106328, -18.62759615963255655, 95.41775706135234714 ) ) ;
#76993=CARTESIAN_POINT ( 'NONE',  ( -19.05341960407611168, -5.049401038298163336, 31.45724293864769550 ) ) ;
#76994=CARTESIAN_POINT ( 'NONE',  ( 15.72974639402176855, 15.80617190586768217, 46.87609039468568994 ) ) ;
#76995=CARTESIAN_POINT ( 'NONE',  ( 18.67979575497194134, -10.72451020669871369, 85.83442372801901854 ) ) ;
#76996=CARTESIAN_POINT ( 'NONE',  ( -4.483927247898782831, 16.52544592524335698, 87.70942372801901854 ) ) ;
#76997=CARTESIAN_POINT ( 'NONE',  ( -18.62759615963255300, -10.81492255796106328, 49.16775706135234003 ) ) ;
#76998=CARTESIAN_POINT ( 'NONE',  ( -10.81492255796105439, 18.62759615963255655, 37.91775706135235424 ) ) ;
#76999=CARTESIAN_POINT ( 'NONE',  ( 16.51473224551083163, -9.474510206698727899, 60.83442372801900433 ) ) ;
#77000=CARTESIAN_POINT ( 'NONE',  ( 16.51473224551069308, 9.474510206698969483, 89.16557627198103830 ) ) ;
#77001=CARTESIAN_POINT ( 'NONE',  ( 16.52544592524342804, -4.483927247898539470, 108.5405762719810241 ) ) ;
#77002=CARTESIAN_POINT ( 'NONE',  ( 10.72451020669898902, -18.67979575497178502, 77.91557627198102409 ) ) ;
#77003=CARTESIAN_POINT ( 'NONE',  ( -8.224510206698948167, 14.34966873604960824, 70.41557627198102409 ) ) ;
#77004=CARTESIAN_POINT ( 'NONE',  ( -10.72451020669870658, -18.67979575497194134, 104.5844237280190185 ) ) ;
#77005=CARTESIAN_POINT ( 'NONE',  ( 8.314922557960818139, 14.29746914071049879, 84.58224293864769550 ) ) ;
#77006=CARTESIAN_POINT ( 'NONE',  ( 5.049401038298161559, -19.05341960407611168, 32.70724293864768129 ) ) ;
#77007=CARTESIAN_POINT ( 'NONE',  ( -13.97604488694547697, 13.89961937509957934, 73.12609039468568994 ) ) ;
#77008=CARTESIAN_POINT ( 'NONE',  ( -0.05219959533910754901, -16.53943276465976808, 52.49890960531435979 ) ) ;
#77009=CARTESIAN_POINT ( 'NONE',  ( 21.53943276465977519, 0.05219959533937863772, 91.25109039468568994 ) ) ;
#77010=CARTESIAN_POINT ( 'NONE',  ( -16.46253265017160317, 9.564922557960807481, 95.83224293864769550 ) ) ;
#77011=CARTESIAN_POINT ( 'NONE',  ( 13.97604488694548053, -13.89961937509957401, 55.62609039468566863 ) ) ;
#77012=CARTESIAN_POINT ( 'NONE',  ( -18.62759615963270932, 10.81492255796079327, 70.83224293864770971 ) ) ;
#77013=CARTESIAN_POINT ( 'NONE',  ( -21.55341960407619339, 5.719274019375674811, 23.54275706135235424 ) ) ;
#77014=CARTESIAN_POINT ( 'NONE',  ( -9.564922557961040184, 16.46253265017147172, 112.9177570613523329 ) ) ;
#77015=CARTESIAN_POINT ( 'NONE',  ( -8.224510206698735004, -14.34966873604973081, 84.58442372801903275 ) ) ;
#77016=CARTESIAN_POINT ( 'NONE',  ( -0.05219959533909027116, -19.03943276465977164, 22.49890960531436690 ) ) ;
#77017=CARTESIAN_POINT ( 'NONE',  ( 0.05219959533937995610, -21.53943276465977519, 25.00109039468567218 ) ) ;
#77018=CARTESIAN_POINT ( 'NONE',  ( 12.14591786802309770, 12.06949235617756955, 114.3739096053143527 ) ) ;
#77020=CARTESIAN_POINT ( 'NONE',  ( 8.314922557961029526, -14.29746914071037800, 50.41775706135235424 ) ) ;
#77021=CARTESIAN_POINT ( 'NONE',  ( -4.379528057220328563, 16.55341960407611168, 80.20724293864769550 ) ) ;
#77022=CARTESIAN_POINT ( 'NONE',  ( 21.52544592524344225, -5.823673210054117533, 73.54057627198102409 ) ) ;
#77023=CARTESIAN_POINT ( 'NONE',  ( 14.34966873604960469, 8.224510206698951720, 29.16557627198103120 ) ) ;
#77024=CARTESIAN_POINT ( 'NONE',  ( -12.14591786802326823, 12.06949235617739902, 33.12609039468569705 ) ) ;
#77025=CARTESIAN_POINT ( 'NONE',  ( -9.474510206698964154, 16.51473224551069663, 40.41557627198103120 ) ) ;
#77026=CARTESIAN_POINT ( 'NONE',  ( -8.224510206698735004, -14.34966873604973081, 84.58442372801903275 ) ) ;
#77027=CARTESIAN_POINT ( 'NONE',  ( -19.02544592524334988, -5.153800228976617603, 73.95942372801900433 ) ) ;
#77028=CARTESIAN_POINT ( 'NONE',  ( -15.72974639402197994, 15.80617190586746368, 65.62390960531436690 ) ) ;
#77029=CARTESIAN_POINT ( 'NONE',  ( -0.05219959533934338120, 16.53943276465976808, 112.5010903946857042 ) ) ;
#77031=CARTESIAN_POINT ( 'NONE',  ( 21.52544592524334988, 5.823673210054432836, 86.45942372801901854 ) ) ;
#77032=CARTESIAN_POINT ( 'NONE',  ( -15.80617190586745835, -15.72974639402198527, 41.87390960531435979 ) ) ;
#77035=CARTESIAN_POINT ( 'NONE',  ( 12.06949235617739724, 12.14591786802326823, 96.87609039468568994 ) ) ;
#77036=CARTESIAN_POINT ( 'NONE',  ( 15.80617190586746368, 15.72974639402197994, 39.37390960531436690 ) ) ;
#77038=CARTESIAN_POINT ( 'NONE',  ( -13.97604488694527625, -13.89961937509977652, 106.8739096053143669 ) ) ;
#77040=CARTESIAN_POINT ( 'NONE',  ( -13.97604488694527625, -13.89961937509977652, 31.87390960531435979 ) ) ;
#77041=CARTESIAN_POINT ( 'NONE',  ( -21.53943276465977519, 0.05219959533907696930, 71.24890960531435269 ) ) ;
#77042=CARTESIAN_POINT ( 'NONE',  ( 4.379528057220092307, 16.55341960407617563, 102.2927570613523613 ) ) ;
#77043=CARTESIAN_POINT ( 'NONE',  ( -21.52544592524334988, -5.823673210054445271, 63.95942372801901854 ) ) ;
#77044=CARTESIAN_POINT ( 'NONE',  ( -8.314922557961024197, 14.29746914071037800, 22.91775706135235069 ) ) ;
#77045=CARTESIAN_POINT ( 'NONE',  ( -16.53943276465976808, 0.05219959533911058130, 116.2489096053143669 ) ) ;
#77046=CARTESIAN_POINT ( 'NONE',  ( 13.89961937509957401, 13.97604488694547697, 106.8760903946856757 ) ) ;
#77047=CARTESIAN_POINT ( 'NONE',  ( -16.46253265017160317, 9.564922557960807481, 35.83224293864768839 ) ) ;
#77049=CARTESIAN_POINT ( 'NONE',  ( 9.564922557960805705, 16.46253265017160317, 104.5822429386476955 ) ) ;
#77050=CARTESIAN_POINT ( 'NONE',  ( 4.379528057220092307, 16.55341960407617563, 92.29275706135236135 ) ) ;
#77051=CARTESIAN_POINT ( 'NONE',  ( 5.153800228976615827, -19.02544592524334988, 80.20942372801901854 ) ) ;
#77052=CARTESIAN_POINT ( 'NONE',  ( -13.89961937509957401, -13.97604488694547875, 24.37609039468565442 ) ) ;
#77053=CARTESIAN_POINT ( 'NONE',  ( -10.81492255796078084, -18.62759615963271287, 77.08224293864769550 ) ) ;
#77054=CARTESIAN_POINT ( 'NONE',  ( 16.52544592524335698, 4.483927247898782831, 86.45942372801901854 ) ) ;
#77055=CARTESIAN_POINT ( 'NONE',  ( -13.89961937509957401, -13.97604488694547875, 89.37609039468563310 ) ) ;
#77056=CARTESIAN_POINT ( 'NONE',  ( -16.46253265017160317, 9.564922557960807481, 50.83224293864770260 ) ) ;
#77057=CARTESIAN_POINT ( 'NONE',  ( 5.153800228976335163, 19.02544592524342804, 94.79057627198103830 ) ) ;
#77058=CARTESIAN_POINT ( 'NONE',  ( -21.55341960407619339, 5.719274019375674811, 48.54275706135234714 ) ) ;
#77059=CARTESIAN_POINT ( 'NONE',  ( 19.03943276465977164, -0.05219959533909143690, 48.74890960531435979 ) ) ;
#77060=CARTESIAN_POINT ( 'NONE',  ( -16.29526858892877783, -7.335722546920120379, 85.79670597800210885 ) ) ;
#77061=CARTESIAN_POINT ( 'NONE',  ( -13.97604488694527625, -13.89961937509977652, 111.8739096053143243 ) ) ;
#77062=CARTESIAN_POINT ( 'NONE',  ( -14.34966873604960291, -8.224510206698953496, 61.66557627198103120 ) ) ;
#77063=CARTESIAN_POINT ( 'NONE',  ( 5.823673210054125526, 21.52544592524343514, 69.79057627198102409 ) ) ;
#77064=LINE ( 'NONE', #50721, #54646 ) ;
#77065=CARTESIAN_POINT ( 'NONE',  ( -13.89961937509957401, -13.97604488694547875, 44.37609039468566863 ) ) ;
#77068=CARTESIAN_POINT ( 'NONE',  ( 5.049401038298161559, -19.05341960407611168, 67.70724293864769550 ) ) ;
#77069=CARTESIAN_POINT ( 'NONE',  ( 19.05341960407611168, 5.049401038298154454, 73.95724293864768129 ) ) ;
#77070=CARTESIAN_POINT ( 'NONE',  ( 14.34966873604972726, -8.224510206698740333, 45.83442372801901854 ) ) ;
#77071=CARTESIAN_POINT ( 'NONE',  ( -17.60779699588840330, -5.500000000000021316, 66.34981316670106821 ) ) ;
#77072=CARTESIAN_POINT ( 'NONE',  ( 16.51473224551083163, -9.474510206698727899, 25.83442372801900078 ) ) ;
#77074=CARTESIAN_POINT ( 'NONE',  ( -16.55341960407617563, 4.379528057220093196, 88.54275706135236135 ) ) ;
#77076=CARTESIAN_POINT ( 'NONE',  ( -12.06949235617739369, -12.14591786802326823, 84.37609039468570415 ) ) ;
#77077=( BOUNDED_CURVE ( )  B_SPLINE_CURVE ( 2, ( #25641, #196488, #7430, #117625, #87286, #181312, #130780, #192472, #9461, #149961, #53955, #115630, #180325 ),
 .UNSPECIFIED., .F., .T. ) 
 B_SPLINE_CURVE_WITH_KNOTS ( ( 3, 2, 2, 2, 2, 2, 3 ),
 ( 0.3972129583543985154, 0.3991228070175438791, 0.4035087719298245390, 0.4078947368421052544, 0.4122807017543859698, 0.4166666666666666852, 0.4186221951519023543 ),
 .UNSPECIFIED. ) 
 CURVE ( )  GEOMETRIC_REPRESENTATION_ITEM ( )  RATIONAL_B_SPLINE_CURVE ( ( 0.9832469066685285419, 0.9851625545550100060, 1.000000000000000000, 0.9659258262890683122, 1.000000000000000000, 0.9659258262890683122, 1.000000000000000000, 0.9659258262890683122, 1.000000000000000000, 0.9659258262890683122, 1.000000000000000000, 0.9848076720550081875, 0.9831626618144004848 ) ) 
 REPRESENTATION_ITEM ( '' )  );
#77078=CARTESIAN_POINT ( 'NONE',  ( -4.483927247898782831, 16.52544592524335698, 52.70942372801902565 ) ) ;
#77079=CARTESIAN_POINT ( 'NONE',  ( 9.474510206698729675, 16.51473224551082808, 27.08442372801900433 ) ) ;
#77080=CARTESIAN_POINT ( 'NONE',  ( -9.474510206698964154, 16.51473224551069663, 50.41557627198102409 ) ) ;
#77082=CARTESIAN_POINT ( 'NONE',  ( -5.719274019375665041, -21.55341960407619695, 64.79275706135234714 ) ) ;
#77083=CARTESIAN_POINT ( 'NONE',  ( 0.05219959533936267826, -19.03943276465977164, 80.00109039468567573 ) ) ;
#77084=CARTESIAN_POINT ( 'NONE',  ( -21.55341960407619339, 5.719274019375674811, 103.5427570613523613 ) ) ;
#77085=CARTESIAN_POINT ( 'NONE',  ( -9.564922557960796823, -16.46253265017161027, 37.08224293864768839 ) ) ;
#77087=CARTESIAN_POINT ( 'NONE',  ( -15.80617190586745835, -15.72974639402198527, 61.87390960531436690 ) ) ;
#77088=CARTESIAN_POINT ( 'NONE',  ( -5.823673210054116645, -21.52544592524344225, 22.29057627198102765 ) ) ;
#77089=CARTESIAN_POINT ( 'NONE',  ( -4.379528057220328563, 16.55341960407611168, 110.2072429386477239 ) ) ;
#77090=CARTESIAN_POINT ( 'NONE',  ( -14.34966873604972548, 8.224510206698743886, 33.33442372801900433 ) ) ;
#77091=CARTESIAN_POINT ( 'NONE',  ( -8.224510206698948167, 14.34966873604960824, 25.41557627198103120 ) ) ;
#77092=EDGE_LOOP ( 'NONE', ( #58102, #8490, #8225 ) ) ;
#77094=CARTESIAN_POINT ( 'NONE',  ( -21.52544592524334988, -5.823673210054445271, 18.95942372801901143 ) ) ;
#77095=CARTESIAN_POINT ( 'NONE',  ( -16.52544592524342804, 4.483927247898546575, 36.04057627198102409 ) ) ;
#77097=CARTESIAN_POINT ( 'NONE',  ( -13.89961937509957401, -13.97604488694547875, 104.3760903946856757 ) ) ;
#77098=CARTESIAN_POINT ( 'NONE',  ( -9.474510206698720793, -16.51473224551083518, 24.58442372801900078 ) ) ;
#77099=CARTESIAN_POINT ( 'NONE',  ( -14.34966873604960291, -8.224510206698953496, 41.66557627198103120 ) ) ;
#77100=CARTESIAN_POINT ( 'NONE',  ( 15.80617190586746368, 15.72974639402197994, 104.3739096053143669 ) ) ;
#77101=CARTESIAN_POINT ( 'NONE',  ( 22.00000000000000000, -5.510910596163089556E-15, 45.00000000000000000 ) ) ;
#77102=CARTESIAN_POINT ( 'NONE',  ( -10.72451020669898014, 18.67979575497178502, 60.41557627198102409 ) ) ;
#77103=CARTESIAN_POINT ( 'NONE',  ( -5.153800228976328057, -19.02544592524343514, 72.29057627198102409 ) ) ;
#77104=CARTESIAN_POINT ( 'NONE',  ( -4.379528057220328563, 16.55341960407611168, 50.20724293864769550 ) ) ;
#77105=CARTESIAN_POINT ( 'NONE',  ( 16.51473224551069308, 9.474510206698969483, 89.16557627198103830 ) ) ;
#77106=DIRECTION ( 'NONE',  ( 0.000000000000000000, 0.000000000000000000, -1.000000000000000000 ) ) ;
#77107=CARTESIAN_POINT ( 'NONE',  ( -19.05341960407617563, 5.049401038297882671, 53.54275706135231871 ) ) ;
#77108=CARTESIAN_POINT ( 'NONE',  ( 21.55341960407610458, 5.719274019375980345, 88.95724293864769550 ) ) ;
#77109=CARTESIAN_POINT ( 'NONE',  ( 5.049401038298161559, -19.05341960407611168, 47.70724293864770260 ) ) ;
#77110=CARTESIAN_POINT ( 'NONE',  ( -12.06949235617756955, 12.14591786802309770, 105.6239096053143669 ) ) ;
#77111=CARTESIAN_POINT ( 'NONE',  ( -5.823673210054431948, 21.52544592524334988, 47.70942372801902565 ) ) ;
#77113=CARTESIAN_POINT ( 'NONE',  ( -14.29746914071049879, 8.314922557960819915, 25.83224293864769194 ) ) ;
#77114=CARTESIAN_POINT ( 'NONE',  ( -16.46253265017160317, 9.564922557960807481, 45.83224293864769550 ) ) ;
#77115=CARTESIAN_POINT ( 'NONE',  ( -9.474510206698964154, 16.51473224551069663, 95.41557627198102409 ) ) ;
#77116=CARTESIAN_POINT ( 'NONE',  ( -18.62759615963270932, 10.81492255796079327, 55.83224293864770260 ) ) ;
#77117=CARTESIAN_POINT ( 'NONE',  ( -18.22780087662119541, 5.500000000000102141, 46.01763182126894947 ) ) ;
#77118=CARTESIAN_POINT ( 'NONE',  ( 16.46253265017160672, -9.564922557960803928, 48.33224293864769550 ) ) ;
#77119=CARTESIAN_POINT ( 'NONE',  ( -5.823673210054116645, -21.52544592524344225, 47.29057627198103120 ) ) ;
#77121=CARTESIAN_POINT ( 'NONE',  ( 0.05219959533937995610, -21.53943276465977519, 85.00109039468568994 ) ) ;
#77123=CARTESIAN_POINT ( 'NONE',  ( -12.14591786802326823, 12.06949235617739902, 88.12609039468570415 ) ) ;
#77124=CARTESIAN_POINT ( 'NONE',  ( -12.06949235617739369, -12.14591786802326823, 89.37609039468568994 ) ) ;
#77125=CARTESIAN_POINT ( 'NONE',  ( 16.51473224551069308, 9.474510206698969483, 59.16557627198102409 ) ) ;
#77126=CARTESIAN_POINT ( 'NONE',  ( 0.05219959533909260263, 19.03943276465977164, 59.99890960531436690 ) ) ;
#77128=CARTESIAN_POINT ( 'NONE',  ( 9.564922557961047289, -16.46253265017146816, 25.41775706135234003 ) ) ;
#77129=CARTESIAN_POINT ( 'NONE',  ( 0.05219959533934541429, -16.53943276465976808, 80.00109039468568994 ) ) ;
#77130=CARTESIAN_POINT ( 'NONE',  ( 10.72451020669871369, 18.67979575497193778, 107.0844237280190043 ) ) ;
#77131=CARTESIAN_POINT ( 'NONE',  ( 16.51473224551069308, 9.474510206698969483, 79.16557627198103830 ) ) ;
#77132=CARTESIAN_POINT ( 'NONE',  ( -18.67979575497178146, -10.72451020669898902, 51.66557627198102409 ) ) ;
#77133=CARTESIAN_POINT ( 'NONE',  ( 4.483927247898790824, -16.52544592524335698, 20.20942372801900788 ) ) ;
#77134=CARTESIAN_POINT ( 'NONE',  ( -21.55341960407619339, 5.719274019375674811, 83.54275706135234714 ) ) ;
#77135=CARTESIAN_POINT ( 'NONE',  ( -14.29746914071037622, -8.314922557961029526, 44.16775706135234714 ) ) ;
#77136=CARTESIAN_POINT ( 'NONE',  ( 10.72451020669898902, -18.67979575497178502, 107.9155762719810241 ) ) ;
#77137=CARTESIAN_POINT ( 'NONE',  ( 5.049401038297881783, 19.05341960407617563, 112.2927570613523471 ) ) ;
#77138=CARTESIAN_POINT ( 'NONE',  ( 19.02544592524343514, -5.153800228976328945, 73.54057627198103830 ) ) ;
#77139=CARTESIAN_POINT ( 'NONE',  ( 4.379528057220092307, 16.55341960407617563, 27.29275706135234358 ) ) ;
#77140=CARTESIAN_POINT ( 'NONE',  ( -19.03943276465977164, 0.05219959533909376836, 41.24890960531435269 ) ) ;
#77141=CARTESIAN_POINT ( 'NONE',  ( 16.55341960407618274, -4.379528057220086978, 21.04275706135234714 ) ) ;
#77142=CARTESIAN_POINT ( 'NONE',  ( 14.34966873604960469, 8.224510206698951720, 74.16557627198102409 ) ) ;
#77143=CARTESIAN_POINT ( 'NONE',  ( -4.379528057220086978, -16.55341960407618274, 89.79275706135236135 ) ) ;
#77144=CARTESIAN_POINT ( 'NONE',  ( -15.72974639402176322, -15.80617190586768395, 34.37609039468568284 ) ) ;
#77145=CARTESIAN_POINT ( 'NONE',  ( -19.02544592524342804, 5.153800228976336051, 66.04057627198103830 ) ) ;
#77146=CARTESIAN_POINT ( 'NONE',  ( 19.02544592524343514, -5.153800228976328945, 68.54057627198103830 ) ) ;
#77147=CARTESIAN_POINT ( 'NONE',  ( -16.55341960407617563, 4.379528057220093196, 83.54275706135234714 ) ) ;
#77151=CARTESIAN_POINT ( 'NONE',  ( 13.89961937509957401, 13.97604488694547697, 31.87609039468566863 ) ) ;
#77152=CARTESIAN_POINT ( 'NONE',  ( -19.05341960407611168, -5.049401038298163336, 31.45724293864769550 ) ) ;
#77153=CARTESIAN_POINT ( 'NONE',  ( 5.049401038298161559, -19.05341960407611168, 112.7072429386476813 ) ) ;
#77154=ORIENTED_EDGE ( 'NONE', *, *, #96372, .T. ) ;
#77155=CARTESIAN_POINT ( 'NONE',  ( -8.314922557961024197, 14.29746914071037800, 27.91775706135234358 ) ) ;
#77157=CARTESIAN_POINT ( 'NONE',  ( 5.049401038297881783, 19.05341960407617563, 52.29275706135234003 ) ) ;
#77158=CARTESIAN_POINT ( 'NONE',  ( -4.379528057220086978, -16.55341960407618274, 39.79275706135235424 ) ) ;
#77159=CARTESIAN_POINT ( 'NONE',  ( -19.02544592524342804, 5.153800228976336051, 101.0405762719810241 ) ) ;
#77160=CARTESIAN_POINT ( 'NONE',  ( 19.02544592524343514, -5.153800228976328945, 63.54057627198103830 ) ) ;
#77161=CARTESIAN_POINT ( 'NONE',  ( -5.823673210054116645, -21.52544592524344225, 102.2905762719810383 ) ) ;
#77162=CARTESIAN_POINT ( 'NONE',  ( -13.97604488694527625, -13.89961937509977652, 91.87390960531432427 ) ) ;
#77163=CARTESIAN_POINT ( 'NONE',  ( 16.46253265017160672, -9.564922557960803928, 23.33224293864769194 ) ) ;
#77164=CARTESIAN_POINT ( 'NONE',  ( -5.153800228976328057, -19.02544592524343514, 62.29057627198100988 ) ) ;
#77165=CARTESIAN_POINT ( 'NONE',  ( 4.379528057220092307, 16.55341960407617563, 112.2927570613523471 ) ) ;
#77166=CARTESIAN_POINT ( 'NONE',  ( -9.564922557960796823, -16.46253265017161027, 22.08224293864768839 ) ) ;
#77167=CARTESIAN_POINT ( 'NONE',  ( 16.46253265017146816, 9.564922557961045513, 36.66775706135233293 ) ) ;
#77168=CARTESIAN_POINT ( 'NONE',  ( 16.53943276465976808, -0.05219959533910856209, 63.74890960531435979 ) ) ;
#77169=CARTESIAN_POINT ( 'NONE',  ( -0.05219959533937732626, 21.53943276465977519, 102.5010903946856899 ) ) ;
#77170=CARTESIAN_POINT ( 'NONE',  ( 19.02544592524343514, -5.153800228976328945, 38.54057627198103120 ) ) ;
#77171=CARTESIAN_POINT ( 'NONE',  ( -12.14591786802326823, 12.06949235617739902, 58.12609039468568994 ) ) ;
#77172=CARTESIAN_POINT ( 'NONE',  ( -16.53943276465976808, 0.05219959533911058130, 41.24890960531435269 ) ) ;
#77173=CARTESIAN_POINT ( 'NONE',  ( 5.719274019375673035, 21.55341960407619339, 92.29275706135236135 ) ) ;
#77174=CARTESIAN_POINT ( 'NONE',  ( -5.049401038298153566, 19.05341960407611168, 75.20724293864769550 ) ) ;
#77175=CARTESIAN_POINT ( 'NONE',  ( 16.51473224551069308, 9.474510206698969483, 99.16557627198102409 ) ) ;
#77176=CARTESIAN_POINT ( 'NONE',  ( 14.29746914071049879, -8.314922557960816363, 108.3322429386477097 ) ) ;
#77177=CARTESIAN_POINT ( 'NONE',  ( 4.379528057220339221, -16.55341960407611168, 77.70724293864770971 ) ) ;
#77178=CARTESIAN_POINT ( 'NONE',  ( 0.05219959533907565091, 21.53943276465977519, 84.99890960531436690 ) ) ;
#77179=CARTESIAN_POINT ( 'NONE',  ( -5.049401038298153566, 19.05341960407611168, 75.20724293864769550 ) ) ;
#77180=CARTESIAN_POINT ( 'NONE',  ( 5.823673210054125526, 21.52544592524343514, 94.79057627198105251 ) ) ;
#77181=CARTESIAN_POINT ( 'NONE',  ( -0.05219959533936034679, 19.03943276465977164, 72.50109039468566152 ) ) ;
#77183=CARTESIAN_POINT ( 'NONE',  ( -8.224510206698948167, 14.34966873604960824, 90.41557627198103830 ) ) ;
#77184=CARTESIAN_POINT ( 'NONE',  ( 9.474510206698971260, -16.51473224551069308, 62.91557627198102409 ) ) ;
#77185=CARTESIAN_POINT ( 'NONE',  ( -18.62759615963270932, 10.81492255796079327, 65.83224293864769550 ) ) ;
#77187=CARTESIAN_POINT ( 'NONE',  ( -4.379528057220328563, 16.55341960407611168, 25.20724293864769550 ) ) ;
#77189=CARTESIAN_POINT ( 'NONE',  ( -5.049401038297874678, -19.05341960407617918, 109.7927570613523187 ) ) ;
#77191=CARTESIAN_POINT ( 'NONE',  ( -0.05219959533910754901, -16.53943276465976808, 82.49890960531436690 ) ) ;
#77192=CARTESIAN_POINT ( 'NONE',  ( 22.00000000000000000, -1.163414459189985801E-14, 95.00000000000000000 ) ) ;
#77193=CARTESIAN_POINT ( 'NONE',  ( -16.51473224551069308, -9.474510206698971260, 76.66557627198103830 ) ) ;
#77194=CARTESIAN_POINT ( 'NONE',  ( 9.564922557960805705, 16.46253265017160317, 34.58224293864770260 ) ) ;
#77195=CARTESIAN_POINT ( 'NONE',  ( 14.29746914071049879, -8.314922557960816363, 68.33224293864769550 ) ) ;
#77196=CARTESIAN_POINT ( 'NONE',  ( 13.97604488694527802, 13.89961937509977652, 109.3739096053143669 ) ) ;
#77197=CARTESIAN_POINT ( 'NONE',  ( 19.02544592524334988, 5.153800228976608722, 91.45942372801900433 ) ) ;
#77198=CARTESIAN_POINT ( 'NONE',  ( -16.51473224551069308, -9.474510206698971260, 96.66557627198102409 ) ) ;
#77199=CARTESIAN_POINT ( 'NONE',  ( -0.05219959533907301413, -21.53943276465977519, 77.49890960531433848 ) ) ;
#77200=CARTESIAN_POINT ( 'NONE',  ( 14.34966873604972726, -8.224510206698740333, 65.83442372801900433 ) ) ;
#77201=CARTESIAN_POINT ( 'NONE',  ( -17.48853670773245739, 5.747243402303007009, 93.66671299749994262 ) ) ;
#77202=CARTESIAN_POINT ( 'NONE',  ( -0.05219959533909027116, -19.03943276465977164, 57.49890960531435979 ) ) ;
#77203=CARTESIAN_POINT ( 'NONE',  ( -5.823673210054116645, -21.52544592524344225, 62.29057627198102409 ) ) ;
#77204=CARTESIAN_POINT ( 'NONE',  ( -13.97604488694547697, 13.89961937509957934, 108.1260903946856331 ) ) ;
#77205=CARTESIAN_POINT ( 'NONE',  ( 14.34966873604960469, 8.224510206698951720, 44.16557627198103120 ) ) ;
#77206=CARTESIAN_POINT ( 'NONE',  ( -10.81492255796105439, 18.62759615963255655, 47.91775706135234714 ) ) ;
#77208=CARTESIAN_POINT ( 'NONE',  ( -16.55341960407617563, 4.379528057220093196, 78.54275706135236135 ) ) ;
#77209=CARTESIAN_POINT ( 'NONE',  ( -0.05219959533909027116, -19.03943276465977164, 107.4989096053143527 ) ) ;
#77210=CARTESIAN_POINT ( 'NONE',  ( -5.153800228976328057, -19.02544592524343514, 102.2905762719810241 ) ) ;
#77211=CARTESIAN_POINT ( 'NONE',  ( -19.03943276465977164, -1.327063459122257427E-13, 115.0000000000000142 ) ) ;
#77212=CARTESIAN_POINT ( 'NONE',  ( 14.29746914071037800, 8.314922557961029526, 91.66775706135234714 ) ) ;
#77213=CARTESIAN_POINT ( 'NONE',  ( -16.55341960407617563, 4.379528057220093196, 53.54275706135234714 ) ) ;
#77214=CARTESIAN_POINT ( 'NONE',  ( -0.05219959533909027116, -19.03943276465977164, 52.49890960531436690 ) ) ;
#77215=CARTESIAN_POINT ( 'NONE',  ( -0.05219959533909027116, -19.03943276465977164, 72.49890960531435269 ) ) ;
#77216=CARTESIAN_POINT ( 'NONE',  ( 21.53943276465977519, 0.05219959533937863772, 51.25109039468568994 ) ) ;
#77217=CARTESIAN_POINT ( 'NONE',  ( -0.05219959533934338120, 16.53943276465976808, 67.50109039468568994 ) ) ;
#77218=CARTESIAN_POINT ( 'NONE',  ( 16.55341960407611168, 4.379528057220329451, 33.95724293864769550 ) ) ;
#77219=CARTESIAN_POINT ( 'NONE',  ( 19.05341960407611168, 5.049401038298154454, 43.95724293864769550 ) ) ;
#77220=CARTESIAN_POINT ( 'NONE',  ( -16.46253265017160317, 9.564922557960807481, 30.83224293864769550 ) ) ;
#77221=CARTESIAN_POINT ( 'NONE',  ( -12.06949235617739369, -12.14591786802326823, 29.37609039468568284 ) ) ;
#77222=CARTESIAN_POINT ( 'NONE',  ( 19.02544592524334988, 5.153800228976608722, 76.45942372801897591 ) ) ;
#77223=CARTESIAN_POINT ( 'NONE',  ( 14.29746914071049879, -8.314922557960816363, 88.33224293864769550 ) ) ;
#77224=CARTESIAN_POINT ( 'NONE',  ( -19.03943276465977164, 0.05219959533909376836, 46.24890960531435979 ) ) ;
#77225=CARTESIAN_POINT ( 'NONE',  ( 5.049401038297881783, 19.05341960407617563, 87.29275706135234714 ) ) ;
#77227=CARTESIAN_POINT ( 'NONE',  ( -15.72974639402176322, -15.80617190586768395, 84.37609039468570415 ) ) ;
#77228=CARTESIAN_POINT ( 'NONE',  ( -16.53943276465976808, -0.05219959533934237506, 48.75109039468568284 ) ) ;
#77229=PLANE ( 'NONE',  #192291 ) ;
#77230=CARTESIAN_POINT ( 'NONE',  ( 21.52544592524344225, -5.823673210054117533, 53.54057627198103120 ) ) ;
#77231=CARTESIAN_POINT ( 'NONE',  ( -16.53943276465976808, -0.05219959533934237506, 33.75109039468568284 ) ) ;
#77232=CARTESIAN_POINT ( 'NONE',  ( 9.564922557960805705, 16.46253265017160317, 34.58224293864770260 ) ) ;
#77233=CARTESIAN_POINT ( 'NONE',  ( 5.049401038297881783, 19.05341960407617563, 42.29275706135234003 ) ) ;
#77234=CARTESIAN_POINT ( 'NONE',  ( 16.51473224551069308, 9.474510206698969483, 79.16557627198103830 ) ) ;
#77235=CARTESIAN_POINT ( 'NONE',  ( -5.153800228976328057, -19.02544592524343514, 47.29057627198102409 ) ) ;
#77237=CARTESIAN_POINT ( 'NONE',  ( 10.72451020669871369, 18.67979575497193778, 72.08442372801899012 ) ) ;
#77239=CARTESIAN_POINT ( 'NONE',  ( 9.564922557961047289, -16.46253265017146816, 30.41775706135232937 ) ) ;
#77240=CARTESIAN_POINT ( 'NONE',  ( -15.72974639402176322, -15.80617190586768395, 104.3760903946856899 ) ) ;
#77241=CARTESIAN_POINT ( 'NONE',  ( 16.53943276465976808, -0.05219959533910856209, 43.74890960531435979 ) ) ;
#77242=CARTESIAN_POINT ( 'NONE',  ( 5.153800228976335163, 19.02544592524342804, 44.79057627198103830 ) ) ;
#77243=CARTESIAN_POINT ( 'NONE',  ( -13.97604488694527625, -13.89961937509977652, 101.8739096053143811 ) ) ;
#77244=CARTESIAN_POINT ( 'NONE',  ( 15.80617190586769283, -15.72974639402175789, 85.62609039468568994 ) ) ;
#77245=CARTESIAN_POINT ( 'NONE',  ( 9.474510206698971260, -16.51473224551069308, 57.91557627198103120 ) ) ;
#77246=CARTESIAN_POINT ( 'NONE',  ( 5.719274019375673035, 21.55341960407619339, 82.29275706135234714 ) ) ;
#77247=CARTESIAN_POINT ( 'NONE',  ( -21.55341960407610458, -5.719274019375992779, 36.45724293864768839 ) ) ;
#77248=CARTESIAN_POINT ( 'NONE',  ( 10.72451020669871369, 18.67979575497193778, 32.08442372801901854 ) ) ;
#77249=CARTESIAN_POINT ( 'NONE',  ( 0.05219959533936267826, -19.03943276465977164, 55.00109039468566863 ) ) ;
#77250=CARTESIAN_POINT ( 'NONE',  ( 9.474510206698971260, -16.51473224551069308, 22.91557627198102765 ) ) ;
#77251=CARTESIAN_POINT ( 'NONE',  ( 0.05219959533909260263, 19.03943276465977164, 79.99890960531436690 ) ) ;
#77252=CARTESIAN_POINT ( 'NONE',  ( -4.379528057220086978, -16.55341960407618274, 34.79275706135235424 ) ) ;
#77253=CARTESIAN_POINT ( 'NONE',  ( 14.29746914071049879, -8.314922557960816363, 93.33224293864769550 ) ) ;
#77254=CARTESIAN_POINT ( 'NONE',  ( 13.89961937509977652, -13.97604488694527269, 58.12390960531436690 ) ) ;
#77255=CARTESIAN_POINT ( 'NONE',  ( 21.55341960407610458, 5.719274019375980345, 33.95724293864769550 ) ) ;
#77256=CARTESIAN_POINT ( 'NONE',  ( 9.474510206698729675, 16.51473224551082808, 102.0844237280190043 ) ) ;
#77257=CARTESIAN_POINT ( 'NONE',  ( -15.72974639402197994, 15.80617190586746368, 105.6239096053143669 ) ) ;
#77258=CARTESIAN_POINT ( 'NONE',  ( -18.62759615963255300, -10.81492255796106328, 59.16775706135234714 ) ) ;
#77259=CARTESIAN_POINT ( 'NONE',  ( 16.53943276465976808, 0.05219959533934440121, 66.25109039468567573 ) ) ;
#77260=CARTESIAN_POINT ( 'NONE',  ( 4.379528057220092307, 16.55341960407617563, 72.29275706135236135 ) ) ;
#77261=CARTESIAN_POINT ( 'NONE',  ( -0.05219959533909027116, -19.03943276465977164, 62.49890960531435979 ) ) ;
#77262=CARTESIAN_POINT ( 'NONE',  ( 12.14591786802327356, -12.06949235617739191, 90.62609039468567573 ) ) ;
#77263=CARTESIAN_POINT ( 'NONE',  ( 0.05219959533907565091, 21.53943276465977519, 114.9989096053143669 ) ) ;
#77264=CARTESIAN_POINT ( 'NONE',  ( 4.483927247898545687, 16.52544592524342804, 69.79057627198102409 ) ) ;
#77265=CARTESIAN_POINT ( 'NONE',  ( -9.474510206698964154, 16.51473224551069663, 80.41557627198103830 ) ) ;
#77266=CARTESIAN_POINT ( 'NONE',  ( 14.34966873604972726, -8.224510206698740333, 70.83442372801901854 ) ) ;
#77267=CARTESIAN_POINT ( 'NONE',  ( -21.55341960407619339, 5.719274019375674811, 63.54275706135234003 ) ) ;
#77268=CARTESIAN_POINT ( 'NONE',  ( 0.05219959533936267826, -19.03943276465977164, 110.0010903946856757 ) ) ;
#77269=CARTESIAN_POINT ( 'NONE',  ( -10.72451020669898014, 18.67979575497178502, 115.4155762719810241 ) ) ;
#77270=CARTESIAN_POINT ( 'NONE',  ( -16.53943276465976808, 0.05219959533911058130, 61.24890960531435979 ) ) ;
#77272=CARTESIAN_POINT ( 'NONE',  ( -16.20579543436679160, 7.371946100355093456, 69.43479165828128430 ) ) ;
#77273=CARTESIAN_POINT ( 'NONE',  ( -5.719274019375978568, 21.55341960407610458, 85.20724293864770971 ) ) ;
#77274=CARTESIAN_POINT ( 'NONE',  ( 4.483927247898545687, 16.52544592524342804, 34.79057627198103120 ) ) ;
#77277=CARTESIAN_POINT ( 'NONE',  ( 15.72974639402176855, 15.80617190586768217, 21.87609039468567573 ) ) ;
#77278=CARTESIAN_POINT ( 'NONE',  ( -19.05341960407611168, -5.049401038298163336, 106.4572429386476955 ) ) ;
#77279=CARTESIAN_POINT ( 'NONE',  ( 10.81492255796106328, -18.62759615963255655, 25.41775706135235779 ) ) ;
#77280=CARTESIAN_POINT ( 'NONE',  ( -14.29746914071049879, 8.314922557960819915, 45.83224293864769550 ) ) ;
#77281=CARTESIAN_POINT ( 'NONE',  ( 16.52544592524335698, 4.483927247898782831, 61.45942372801901854 ) ) ;
#77282=CARTESIAN_POINT ( 'NONE',  ( 19.05341960407611168, 5.049401038298154454, 58.95724293864768129 ) ) ;
#77283=CARTESIAN_POINT ( 'NONE',  ( -5.049401038297874678, -19.05341960407617918, 59.79275706135231871 ) ) ;
#77284=CARTESIAN_POINT ( 'NONE',  ( -9.564922557960796823, -16.46253265017161027, 82.08224293864768129 ) ) ;
#77285=CARTESIAN_POINT ( 'NONE',  ( 15.80617190586746368, 15.72974639402197994, 44.37390960531435979 ) ) ;
#77287=CARTESIAN_POINT ( 'NONE',  ( 16.46253265017160672, -9.564922557960803928, 53.33224293864768839 ) ) ;
#77288=CARTESIAN_POINT ( 'NONE',  ( -4.379528057220086978, -16.55341960407618274, 34.79275706135235424 ) ) ;
#77289=CARTESIAN_POINT ( 'NONE',  ( 19.03943276465977164, 0.05219959533936151252, 66.25109039468567573 ) ) ;
#77290=CARTESIAN_POINT ( 'NONE',  ( 10.81492255796078972, 18.62759615963270932, 114.5822429386477097 ) ) ;
#77291=CARTESIAN_POINT ( 'NONE',  ( 12.06949235617757843, -12.14591786802309237, 53.12390960531436690 ) ) ;
#77292=CARTESIAN_POINT ( 'NONE',  ( 13.97604488694527802, 13.89961937509977652, 94.37390960531436690 ) ) ;
#77293=CARTESIAN_POINT ( 'NONE',  ( -15.72974639402197994, 15.80617190586746368, 60.62390960531437401 ) ) ;
#77294=CARTESIAN_POINT ( 'NONE',  ( -10.72451020669898014, 18.67979575497178502, 95.41557627198102409 ) ) ;
#77295=CARTESIAN_POINT ( 'NONE',  ( -12.14591786802326823, 12.06949235617739902, 33.12609039468569705 ) ) ;
#77297=CARTESIAN_POINT ( 'NONE',  ( -0.05219959533907301413, -21.53943276465977519, 32.49890960531435979 ) ) ;
#77298=CARTESIAN_POINT ( 'NONE',  ( 18.67979575497194134, -10.72451020669871369, 90.83442372801901854 ) ) ;
#77299=CARTESIAN_POINT ( 'NONE',  ( 13.97604488694527802, 13.89961937509977652, 84.37390960531433848 ) ) ;
#77301=CARTESIAN_POINT ( 'NONE',  ( -0.05219959533909027116, -19.03943276465977164, 37.49890960531436690 ) ) ;
#77302=CARTESIAN_POINT ( 'NONE',  ( -19.03943276465977164, 0.05219959533909376836, 101.2489096053143669 ) ) ;
#77303=CARTESIAN_POINT ( 'NONE',  ( 14.34966873604960469, 8.224510206698951720, 104.1655762719810241 ) ) ;
#77304=CARTESIAN_POINT ( 'NONE',  ( -19.02544592524342804, 5.153800228976336051, 61.04057627198103120 ) ) ;
#77305=CARTESIAN_POINT ( 'NONE',  ( 16.55341960407618274, -4.379528057220086978, 21.04275706135234714 ) ) ;
#77306=CARTESIAN_POINT ( 'NONE',  ( 17.50000000000001776, 3.850315288878741526, 33.23370869396553928 ) ) ;
#77307=CARTESIAN_POINT ( 'NONE',  ( -18.67979575497193778, 10.72451020669871902, 98.33442372801901854 ) ) ;
#77308=CARTESIAN_POINT ( 'NONE',  ( -10.81492255796078084, -18.62759615963271287, 27.08224293864769550 ) ) ;
#77309=CARTESIAN_POINT ( 'NONE',  ( -16.53943276465976808, -0.05219959533934237506, 88.75109039468567573 ) ) ;
#77312=CARTESIAN_POINT ( 'NONE',  ( -16.46253265017146816, -9.564922557961047289, 64.16775706135233293 ) ) ;
#77313=CARTESIAN_POINT ( 'NONE',  ( -16.51473224551082808, 9.474510206698731452, 28.33442372801900433 ) ) ;
#77315=CARTESIAN_POINT ( 'NONE',  ( -9.474510206698964154, 16.51473224551069663, 30.41557627198102054 ) ) ;
#77316=CARTESIAN_POINT ( 'NONE',  ( -4.379528057220328563, 16.55341960407611168, 35.20724293864768839 ) ) ;
#77317=CARTESIAN_POINT ( 'NONE',  ( -17.05587630539786304, -6.762274262135681724, 109.2581969096268466 ) ) ;
#77318=CARTESIAN_POINT ( 'NONE',  ( -16.52544592524342804, 4.483927247898546575, 31.04057627198102409 ) ) ;
#77320=CARTESIAN_POINT ( 'NONE',  ( 0.05219959533934541429, -16.53943276465976808, 95.00109039468568994 ) ) ;
#77321=CARTESIAN_POINT ( 'NONE',  ( 13.89961937509977652, -13.97604488694527269, 33.12390960531434558 ) ) ;
#77322=CARTESIAN_POINT ( 'NONE',  ( 15.72974639402176855, 15.80617190586768217, 111.8760903946856615 ) ) ;
#77323=CARTESIAN_POINT ( 'NONE',  ( -5.153800228976607833, 19.02544592524334988, 112.7094237280190043 ) ) ;
#77324=CARTESIAN_POINT ( 'NONE',  ( -21.53943276465977519, -0.05219959533937600094, 78.75109039468568994 ) ) ;
#77325=CARTESIAN_POINT ( 'NONE',  ( 19.03943276465977164, 0.05219959533936151252, 56.25109039468566863 ) ) ;
#77326=CARTESIAN_POINT ( 'NONE',  ( -9.474510206698964154, 16.51473224551069663, 90.41557627198103830 ) ) ;
#77327=CARTESIAN_POINT ( 'NONE',  ( 16.46253265017160672, -9.564922557960803928, 78.33224293864769550 ) ) ;
#77328=CARTESIAN_POINT ( 'NONE',  ( -18.87075004821571866, 5.499999999999899636, 38.67408112101045958 ) ) ;
#77329=CARTESIAN_POINT ( 'NONE',  ( -21.53943276465977519, 0.05219959533907696930, 91.24890960531436690 ) ) ;
#77331=CARTESIAN_POINT ( 'NONE',  ( 4.483927247898545687, 16.52544592524342804, 64.79057627198103830 ) ) ;
#77332=CARTESIAN_POINT ( 'NONE',  ( -15.80617190586745835, -15.72974639402198527, 56.87390960531436690 ) ) ;
#77333=CARTESIAN_POINT ( 'NONE',  ( -5.049401038298153566, 19.05341960407611168, 55.20724293864769550 ) ) ;
#77334=CARTESIAN_POINT ( 'NONE',  ( 18.62759615963271287, -10.81492255796078972, 83.33224293864769550 ) ) ;
#77335=CARTESIAN_POINT ( 'NONE',  ( 12.06949235617739724, 12.14591786802326823, 96.87609039468568994 ) ) ;
#77337=CARTESIAN_POINT ( 'NONE',  ( 9.474510206698971260, -16.51473224551069308, 47.91557627198102409 ) ) ;
#77339=CARTESIAN_POINT ( 'NONE',  ( 16.52544592524342804, -4.483927247898539470, 88.54057627198103830 ) ) ;
#77341=CARTESIAN_POINT ( 'NONE',  ( 5.153800228976335163, 19.02544592524342804, 44.79057627198103830 ) ) ;
#77342=CARTESIAN_POINT ( 'NONE',  ( 19.02544592524343514, -5.153800228976328945, 23.54057627198102054 ) ) ;
#77343=CARTESIAN_POINT ( 'NONE',  ( 5.049401038297881783, 19.05341960407617563, 67.29275706135234714 ) ) ;
#77344=CARTESIAN_POINT ( 'NONE',  ( 4.379528057220339221, -16.55341960407611168, 87.70724293864769550 ) ) ;
#77345=CARTESIAN_POINT ( 'NONE',  ( -15.80617190586768217, 15.72974639402176855, 48.12609039468568284 ) ) ;
#77346=CARTESIAN_POINT ( 'NONE',  ( -16.51473224551069308, -9.474510206698971260, 36.66557627198102409 ) ) ;
#77347=CARTESIAN_POINT ( 'NONE',  ( -21.55341960407610458, -5.719274019375992779, 101.4572429386476955 ) ) ;
#77348=CARTESIAN_POINT ( 'NONE',  ( 12.14591786802309770, 12.06949235617756955, 84.37390960531438111 ) ) ;
#77350=CARTESIAN_POINT ( 'NONE',  ( 9.564922557960805705, 16.46253265017160317, 64.58224293864769550 ) ) ;
#77352=CARTESIAN_POINT ( 'NONE',  ( -19.02544592524334988, -5.153800228976617603, 98.95942372801900433 ) ) ;
#77353=CARTESIAN_POINT ( 'NONE',  ( 18.62759615963271287, -10.81492255796078972, 23.33224293864769194 ) ) ;
#77354=CARTESIAN_POINT ( 'NONE',  ( 5.719274019375673035, 21.55341960407619339, 32.29275706135235424 ) ) ;
#77355=CARTESIAN_POINT ( 'NONE',  ( -9.564922557960796823, -16.46253265017161027, 77.08224293864769550 ) ) ;
#77356=CARTESIAN_POINT ( 'NONE',  ( -16.51473224551082808, 9.474510206698731452, 63.33442372801900433 ) ) ;
#77357=CARTESIAN_POINT ( 'NONE',  ( -16.51473224551069308, -9.474510206698971260, 51.66557627198102409 ) ) ;
#77358=CARTESIAN_POINT ( 'NONE',  ( 14.29746914071049879, -8.314922557960816363, 78.33224293864770971 ) ) ;
#77359=CARTESIAN_POINT ( 'NONE',  ( -16.52544592524342804, 4.483927247898546575, 71.04057627198103830 ) ) ;
#77360=CARTESIAN_POINT ( 'NONE',  ( 13.97604488694527802, 13.89961937509977652, 94.37390960531436690 ) ) ;
#77361=CARTESIAN_POINT ( 'NONE',  ( -21.53943276465977519, 0.05219959533907696930, 106.2489096053143811 ) ) ;
#77362=CARTESIAN_POINT ( 'NONE',  ( 19.02544592524343514, -5.153800228976328945, 83.54057627198100988 ) ) ;
#77363=CARTESIAN_POINT ( 'NONE',  ( -9.474510206698720793, -16.51473224551083518, 29.58442372801900433 ) ) ;
#77364=CARTESIAN_POINT ( 'NONE',  ( -19.02544592524342804, 5.153800228976336051, 31.04057627198102409 ) ) ;
#77365=CARTESIAN_POINT ( 'NONE',  ( 14.34966873604960469, 8.224510206698951720, 29.16557627198103120 ) ) ;
#77366=CARTESIAN_POINT ( 'NONE',  ( 16.55341960407611168, 4.379528057220329451, 108.9572429386476955 ) ) ;
#77368=CARTESIAN_POINT ( 'NONE',  ( -18.62759615963255300, -10.81492255796106328, 34.16775706135234714 ) ) ;
#77369=CARTESIAN_POINT ( 'NONE',  ( -13.97604488694547697, 13.89961937509957934, 73.12609039468568994 ) ) ;
#77370=CARTESIAN_POINT ( 'NONE',  ( -16.52544592524342804, 4.483927247898546575, 31.04057627198102409 ) ) ;
#77371=CARTESIAN_POINT ( 'NONE',  ( 0.05219959533907565091, 21.53943276465977519, 89.99890960531438111 ) ) ;
#77372=CARTESIAN_POINT ( 'NONE',  ( -0.05219959533907301413, -21.53943276465977519, 22.49890960531436335 ) ) ;
#77373=CARTESIAN_POINT ( 'NONE',  ( -8.314922557960811034, -14.29746914071050412, 67.08224293864770971 ) ) ;
#77374=CARTESIAN_POINT ( 'NONE',  ( 16.51473224551069308, 9.474510206698969483, 24.16557627198102765 ) ) ;
#77375=CARTESIAN_POINT ( 'NONE',  ( 9.474510206698729675, 16.51473224551082808, 22.08442372801899722 ) ) ;
#77376=CARTESIAN_POINT ( 'NONE',  ( 16.55341960407618274, -4.379528057220086978, 101.0427570613523756 ) ) ;
#77377=CARTESIAN_POINT ( 'NONE',  ( -16.55341960407617563, 4.379528057220093196, 58.54275706135235424 ) ) ;
#77378=CARTESIAN_POINT ( 'NONE',  ( 5.049401038298161559, -19.05341960407611168, 112.7072429386476813 ) ) ;
#77379=CARTESIAN_POINT ( 'NONE',  ( -0.05219959533937732626, 21.53943276465977519, 107.5010903946856899 ) ) ;
#77380=CARTESIAN_POINT ( 'NONE',  ( 9.564922557960805705, 16.46253265017160317, 84.58224293864769550 ) ) ;
#77381=CARTESIAN_POINT ( 'NONE',  ( 4.483927247898790824, -16.52544592524335698, 60.20942372801902565 ) ) ;
#77382=CARTESIAN_POINT ( 'NONE',  ( 8.224510206698953496, -14.34966873604960469, 112.9155762719810383 ) ) ;
#77383=CARTESIAN_POINT ( 'NONE',  ( -14.34966873604960291, -8.224510206698953496, 36.66557627198103120 ) ) ;
#77385=CARTESIAN_POINT ( 'NONE',  ( -19.02544592524342804, 5.153800228976336051, 111.0405762719810099 ) ) ;
#77386=CARTESIAN_POINT ( 'NONE',  ( 19.05341960407611168, 5.049401038298154454, 93.95724293864769550 ) ) ;
#77387=CARTESIAN_POINT ( 'NONE',  ( -19.05341960407611168, -5.049401038298163336, 111.4572429386476671 ) ) ;
#77388=CARTESIAN_POINT ( 'NONE',  ( -4.483927247898539470, -16.52544592524342804, 57.29057627198103120 ) ) ;
#77389=CARTESIAN_POINT ( 'NONE',  ( 4.483927247898545687, 16.52544592524342804, 39.79057627198103830 ) ) ;
#77390=CARTESIAN_POINT ( 'NONE',  ( -12.14591786802309592, -12.06949235617757132, 51.87390960531437401 ) ) ;
#77391=CARTESIAN_POINT ( 'NONE',  ( -4.379528057220086978, -16.55341960407618274, 44.79275706135234714 ) ) ;
#77393=CARTESIAN_POINT ( 'NONE',  ( 9.474510206698729675, 16.51473224551082808, 52.08442372801900433 ) ) ;
#77394=CARTESIAN_POINT ( 'NONE',  ( 9.474510206698971260, -16.51473224551069308, 77.91557627198103830 ) ) ;
#77395=CARTESIAN_POINT ( 'NONE',  ( -9.474510206698720793, -16.51473224551083518, 64.58442372801900433 ) ) ;
#77397=CARTESIAN_POINT ( 'NONE',  ( -16.51473224551082808, 9.474510206698731452, 58.33442372801900433 ) ) ;
#77398=CARTESIAN_POINT ( 'NONE',  ( -5.153800228976607833, 19.02544592524334988, 102.7094237280189759 ) ) ;
#77399=CARTESIAN_POINT ( 'NONE',  ( 14.29746914071037800, 8.314922557961029526, 81.66775706135236135 ) ) ;
#77401=CARTESIAN_POINT ( 'NONE',  ( -0.05219959533909027116, -19.03943276465977164, 32.49890960531435979 ) ) ;
#77402=CARTESIAN_POINT ( 'NONE',  ( 19.03943276465977164, -0.05219959533909143690, 98.74890960531436690 ) ) ;
#77403=CARTESIAN_POINT ( 'NONE',  ( 15.72974639402176855, 15.80617190586768217, 46.87609039468568994 ) ) ;
#77404=CARTESIAN_POINT ( 'NONE',  ( -19.02544592524334988, -5.153800228976617603, 103.9594237280190043 ) ) ;
#77405=CARTESIAN_POINT ( 'NONE',  ( 17.50000000000000355, -3.209263204892577548, 107.2619682560627581 ) ) ;
#77406=CARTESIAN_POINT ( 'NONE',  ( 13.97604488694527802, 13.89961937509977652, 64.37390960531436690 ) ) ;
#77407=CARTESIAN_POINT ( 'NONE',  ( 5.049401038298161559, -19.05341960407611168, 102.7072429386476955 ) ) ;
#77408=CARTESIAN_POINT ( 'NONE',  ( -4.483927247898539470, -16.52544592524342804, 62.29057627198102409 ) ) ;
#77409=CARTESIAN_POINT ( 'NONE',  ( 13.97604488694527802, 13.89961937509977652, 59.37390960531434558 ) ) ;
#77410=CARTESIAN_POINT ( 'NONE',  ( 0.05219959533909260263, 19.03943276465977164, 59.99890960531436690 ) ) ;
#77411=CARTESIAN_POINT ( 'NONE',  ( -16.46253265017146816, -9.564922557961047289, 84.16775706135233293 ) ) ;
#77412=CARTESIAN_POINT ( 'NONE',  ( -5.823673210054116645, -21.52544592524344225, 57.29057627198103120 ) ) ;
#77413=CARTESIAN_POINT ( 'NONE',  ( 14.34966873604960469, 8.224510206698951720, 114.1655762719810383 ) ) ;
#77414=CARTESIAN_POINT ( 'NONE',  ( 16.46253265017146816, 9.564922557961045513, 46.66775706135233293 ) ) ;
#77415=CARTESIAN_POINT ( 'NONE',  ( 5.153800228976335163, 19.02544592524342804, 84.79057627198099567 ) ) ;
#77416=CARTESIAN_POINT ( 'NONE',  ( 15.72974639402199770, -15.80617190586745480, 83.12390960531436690 ) ) ;
#77417=CARTESIAN_POINT ( 'NONE',  ( 8.314922557960818139, 14.29746914071049879, 79.58224293864769550 ) ) ;
#77418=CARTESIAN_POINT ( 'NONE',  ( -19.05341960407617563, 5.049401038297882671, 38.54275706135233293 ) ) ;
#77419=CARTESIAN_POINT ( 'NONE',  ( 5.823673210054125526, 21.52544592524343514, 59.79057627198103120 ) ) ;
#77420=CARTESIAN_POINT ( 'NONE',  ( -5.719274019375978568, 21.55341960407610458, 45.20724293864769550 ) ) ;
#77421=CARTESIAN_POINT ( 'NONE',  ( -15.80617190586768217, 15.72974639402176855, 93.12609039468568994 ) ) ;
#77422=CARTESIAN_POINT ( 'NONE',  ( 19.03943276465977164, -0.05219959533909143690, 68.74890960531436690 ) ) ;
#77423=CARTESIAN_POINT ( 'NONE',  ( 4.379528057220339221, -16.55341960407611168, 112.7072429386476955 ) ) ;
#77424=CARTESIAN_POINT ( 'NONE',  ( -0.05219959533937732626, 21.53943276465977519, 32.50109039468568284 ) ) ;
#77427=CARTESIAN_POINT ( 'NONE',  ( 5.823673210054444382, -21.52544592524334988, 45.20942372801901854 ) ) ;
#77428=CARTESIAN_POINT ( 'NONE',  ( -5.153800228976328057, -19.02544592524343514, 37.29057627198102409 ) ) ;
#77429=CARTESIAN_POINT ( 'NONE',  ( -15.80617190586745835, -15.72974639402198527, 101.8739096053143811 ) ) ;
#77430=CARTESIAN_POINT ( 'NONE',  ( 13.89961937509957401, 13.97604488694547697, 46.87609039468565442 ) ) ;
#77431=CARTESIAN_POINT ( 'NONE',  ( 19.03943276465977164, -0.05219959533909143690, 23.74890960531435269 ) ) ;
#77433=CARTESIAN_POINT ( 'NONE',  ( 8.224510206698742110, 14.34966873604972548, 62.08442372801901143 ) ) ;
#77434=CARTESIAN_POINT ( 'NONE',  ( 9.564922557960805705, 16.46253265017160317, 24.58224293864769194 ) ) ;
#77436=CARTESIAN_POINT ( 'NONE',  ( -19.02544592524342804, 5.153800228976336051, 76.04057627198102409 ) ) ;
#77437=CARTESIAN_POINT ( 'NONE',  ( -8.224510206698948167, 14.34966873604960824, 105.4155762719810383 ) ) ;
#77438=CARTESIAN_POINT ( 'NONE',  ( 21.52544592524344225, -5.823673210054117533, 63.54057627198103830 ) ) ;
#77439=CARTESIAN_POINT ( 'NONE',  ( -16.52544592524335698, -4.483927247898792601, 33.95942372801901143 ) ) ;
#77440=CARTESIAN_POINT ( 'NONE',  ( -21.55341960407619339, 5.719274019375674811, 98.54275706135234714 ) ) ;
#77442=CARTESIAN_POINT ( 'NONE',  ( -0.05219959533934338120, 16.53943276465976808, 112.5010903946857042 ) ) ;
#77443=CARTESIAN_POINT ( 'NONE',  ( 14.34966873604960469, 8.224510206698951720, 49.16557627198102409 ) ) ;
#77445=CARTESIAN_POINT ( 'NONE',  ( -9.474510206698964154, 16.51473224551069663, 45.41557627198103120 ) ) ;
#77446=CARTESIAN_POINT ( 'NONE',  ( -21.53943276465977519, -0.05219959533937600094, 98.75109039468568994 ) ) ;
#77447=CARTESIAN_POINT ( 'NONE',  ( -10.81492255796078084, -18.62759615963271287, 107.0822429386476955 ) ) ;
#77448=CARTESIAN_POINT ( 'NONE',  ( 10.81492255796106328, -18.62759615963255655, 70.41775706135236135 ) ) ;
#77449=CARTESIAN_POINT ( 'NONE',  ( 14.29746914071037800, 8.314922557961029526, 51.66775706135234714 ) ) ;
#77450=CARTESIAN_POINT ( 'NONE',  ( 16.55341960407611168, 4.379528057220329451, 83.95724293864770971 ) ) ;
#77451=CARTESIAN_POINT ( 'NONE',  ( -5.823673210054431948, 21.52544592524334988, 97.70942372801904696 ) ) ;
#77452=CARTESIAN_POINT ( 'NONE',  ( -12.14591786802326823, 12.06949235617739902, 113.1260903946856899 ) ) ;
#77454=CARTESIAN_POINT ( 'NONE',  ( 16.53943276465976808, 0.05219959533934440121, 36.25109039468567573 ) ) ;
#77455=CARTESIAN_POINT ( 'NONE',  ( -16.55341960407611168, -4.379528057220339221, 46.45724293864769550 ) ) ;
#77456=CARTESIAN_POINT ( 'NONE',  ( -14.29746914071037622, -8.314922557961029526, 89.16775706135236135 ) ) ;
#77457=CARTESIAN_POINT ( 'NONE',  ( -19.03943276465977164, 0.05219959533909376836, 96.24890960531436690 ) ) ;
#77458=CARTESIAN_POINT ( 'NONE',  ( -5.153800228976328057, -19.02544592524343514, 112.2905762719810099 ) ) ;
#77459=CARTESIAN_POINT ( 'NONE',  ( -5.719274019375665041, -21.55341960407619695, 99.79275706135234714 ) ) ;
#77461=CARTESIAN_POINT ( 'NONE',  ( -0.05219959533934338120, 16.53943276465976808, 107.5010903946856899 ) ) ;
#77462=CARTESIAN_POINT ( 'NONE',  ( 16.52544592524342804, -4.483927247898539470, 68.54057627198103830 ) ) ;
#77463=CARTESIAN_POINT ( 'NONE',  ( -5.153800228976328057, -19.02544592524343514, 77.29057627198099567 ) ) ;
#77465=CARTESIAN_POINT ( 'NONE',  ( -14.34966873604972548, 8.224510206698743886, 33.33442372801900433 ) ) ;
#77466=CARTESIAN_POINT ( 'NONE',  ( 19.02544592524343514, -5.153800228976328945, 28.54057627198102409 ) ) ;
#77467=CARTESIAN_POINT ( 'NONE',  ( 19.03943276465977164, -0.05219959533909143690, 88.74890960531436690 ) ) ;
#77468=CARTESIAN_POINT ( 'NONE',  ( -14.29746914071037622, -8.314922557961029526, 29.16775706135234003 ) ) ;
#77470=CARTESIAN_POINT ( 'NONE',  ( 5.153800228976615827, -19.02544592524334988, 35.20942372801899722 ) ) ;
#77471=CARTESIAN_POINT ( 'NONE',  ( -8.314922557961024197, 14.29746914071037800, 92.91775706135236135 ) ) ;
#77472=CARTESIAN_POINT ( 'NONE',  ( 5.049401038298161559, -19.05341960407611168, 37.70724293864768839 ) ) ;
#77473=CARTESIAN_POINT ( 'NONE',  ( 0.05219959533934541429, -16.53943276465976808, 75.00109039468568994 ) ) ;
#77474=CARTESIAN_POINT ( 'NONE',  ( 8.314922557961029526, -14.29746914071037800, 60.41775706135235424 ) ) ;
#77475=CARTESIAN_POINT ( 'NONE',  ( -16.46253265017146816, -9.564922557961047289, 84.16775706135233293 ) ) ;
#77476=CARTESIAN_POINT ( 'NONE',  ( 16.46253265017146816, 9.564922557961045513, 31.66775706135232937 ) ) ;
#77477=CARTESIAN_POINT ( 'NONE',  ( 13.97604488694527802, 13.89961937509977652, 44.37390960531435269 ) ) ;
#77478=CARTESIAN_POINT ( 'NONE',  ( -16.53943276465976808, 0.05219959533911058130, 86.24890960531436690 ) ) ;
#77480=CARTESIAN_POINT ( 'NONE',  ( -5.049401038297874678, -19.05341960407617918, 59.79275706135231871 ) ) ;
#77481=CARTESIAN_POINT ( 'NONE',  ( -10.72451020669898014, 18.67979575497178502, 50.41557627198103120 ) ) ;
#77482=CARTESIAN_POINT ( 'NONE',  ( 5.049401038297881783, 19.05341960407617563, 27.29275706135232937 ) ) ;
#77483=CARTESIAN_POINT ( 'NONE',  ( -9.564922557960796823, -16.46253265017161027, 107.0822429386476955 ) ) ;
#77484=CARTESIAN_POINT ( 'NONE',  ( -0.05219959533907301413, -21.53943276465977519, 77.49890960531433848 ) ) ;
#77485=CARTESIAN_POINT ( 'NONE',  ( 5.153800228976335163, 19.02544592524342804, 114.7905762719810241 ) ) ;
#77486=CARTESIAN_POINT ( 'NONE',  ( 9.564922557961047289, -16.46253265017146816, 90.41775706135234714 ) ) ;
#77487=CARTESIAN_POINT ( 'NONE',  ( -17.49999999999999645, 3.471454075611712042, 109.4833258114436347 ) ) ;
#77488=CARTESIAN_POINT ( 'NONE',  ( 5.049401038297881783, 19.05341960407617563, 112.2927570613523471 ) ) ;
#77489=CARTESIAN_POINT ( 'NONE',  ( -16.51473224551069308, -9.474510206698971260, 31.66557627198102054 ) ) ;
#77490=CARTESIAN_POINT ( 'NONE',  ( 9.564922557960805705, 16.46253265017160317, 94.58224293864769550 ) ) ;
#77491=CARTESIAN_POINT ( 'NONE',  ( -10.81492255796078084, -18.62759615963271287, 72.08224293864769550 ) ) ;
#77492=CARTESIAN_POINT ( 'NONE',  ( -0.05219959533934338120, 16.53943276465976808, 47.50109039468568994 ) ) ;
#77493=CARTESIAN_POINT ( 'NONE',  ( 15.80617190586769283, -15.72974639402175789, 50.62609039468568994 ) ) ;
#77494=CARTESIAN_POINT ( 'NONE',  ( -13.97604488694547697, 13.89961937509957934, 88.12609039468563310 ) ) ;
#77495=CARTESIAN_POINT ( 'NONE',  ( 10.81492255796106328, -18.62759615963255655, 105.4177570613523613 ) ) ;
#77496=CARTESIAN_POINT ( 'NONE',  ( 16.55341960407618274, -4.379528057220086978, 111.0427570613523613 ) ) ;
#77497=CARTESIAN_POINT ( 'NONE',  ( -16.46253265017160317, 9.564922557960807481, 100.8322429386477097 ) ) ;
#77498=CARTESIAN_POINT ( 'NONE',  ( -4.379528057220328563, 16.55341960407611168, 85.20724293864770971 ) ) ;
#77499=CARTESIAN_POINT ( 'NONE',  ( 4.379528057220339221, -16.55341960407611168, 42.70724293864770260 ) ) ;
#77500=CARTESIAN_POINT ( 'NONE',  ( 19.03943276465977164, 0.05219959533936151252, 76.25109039468566152 ) ) ;
#77501=CARTESIAN_POINT ( 'NONE',  ( 21.53943276465977519, 0.05219959533937863772, 61.25109039468567573 ) ) ;
#77502=CARTESIAN_POINT ( 'NONE',  ( -19.02544592524334988, -5.153800228976617603, 23.95942372801900078 ) ) ;
#77503=CARTESIAN_POINT ( 'NONE',  ( 16.55341960407611168, 4.379528057220329451, 98.95724293864770971 ) ) ;
#77504=CARTESIAN_POINT ( 'NONE',  ( -15.72974639402197994, 15.80617190586746368, 25.62390960531435624 ) ) ;
#77505=CARTESIAN_POINT ( 'NONE',  ( -4.483927247898539470, -16.52544592524342804, 27.29057627198103120 ) ) ;
#77506=CARTESIAN_POINT ( 'NONE',  ( 0.05219959533937995610, -21.53943276465977519, 100.0010903946857042 ) ) ;
#77507=CARTESIAN_POINT ( 'NONE',  ( -16.53943276465976808, -0.05219959533934237506, 63.75109039468568284 ) ) ;
#77508=CARTESIAN_POINT ( 'NONE',  ( -8.314922557960811034, -14.29746914071050412, 22.08224293864769194 ) ) ;
#77509=CARTESIAN_POINT ( 'NONE',  ( -5.823673210054431948, 21.52544592524334988, 57.70942372801901143 ) ) ;
#77510=CARTESIAN_POINT ( 'NONE',  ( 0.05219959533937995610, -21.53943276465977519, 55.00109039468568284 ) ) ;
#77512=CARTESIAN_POINT ( 'NONE',  ( -16.51473224551069308, -9.474510206698971260, 61.66557627198103120 ) ) ;
#77513=CARTESIAN_POINT ( 'NONE',  ( 10.72451020669871369, 18.67979575497193778, 27.08442372801901854 ) ) ;
#77514=CARTESIAN_POINT ( 'NONE',  ( 4.379528057220339221, -16.55341960407611168, 102.7072429386476955 ) ) ;
#77515=CARTESIAN_POINT ( 'NONE',  ( 9.564922557960805705, 16.46253265017160317, 29.58224293864769550 ) ) ;
#77516=CARTESIAN_POINT ( 'NONE',  ( 4.483927247898545687, 16.52544592524342804, 74.79057627198105251 ) ) ;
#77517=CARTESIAN_POINT ( 'NONE',  ( 16.46253265017160672, -9.564922557960803928, 68.33224293864770971 ) ) ;
#77518=CARTESIAN_POINT ( 'NONE',  ( -16.53943276465976808, 0.05219959533911058130, 26.24890960531435624 ) ) ;
#77519=CARTESIAN_POINT ( 'NONE',  ( -18.62759615963270932, 10.81492255796079327, 55.83224293864770260 ) ) ;
#77520=CARTESIAN_POINT ( 'NONE',  ( 8.224510206698953496, -14.34966873604960469, 92.91557627198103830 ) ) ;
#77521=CARTESIAN_POINT ( 'NONE',  ( -0.05219959533907301413, -21.53943276465977519, 92.49890960531436690 ) ) ;
#77522=CARTESIAN_POINT ( 'NONE',  ( -9.474510206698964154, 16.51473224551069663, 95.41557627198102409 ) ) ;
#77523=CARTESIAN_POINT ( 'NONE',  ( -19.05341960407611168, -5.049401038298163336, 51.45724293864770260 ) ) ;
#77524=CARTESIAN_POINT ( 'NONE',  ( -13.97604488694547697, 13.89961937509957934, 103.1260903946856473 ) ) ;
#77525=CARTESIAN_POINT ( 'NONE',  ( 5.719274019375991003, -21.55341960407610458, 42.70724293864770260 ) ) ;
#77526=CARTESIAN_POINT ( 'NONE',  ( 18.67979575497194134, -10.72451020669871369, 80.83442372801901854 ) ) ;
#77527=CARTESIAN_POINT ( 'NONE',  ( -19.03943276465977164, 0.05219959533909376836, 66.24890960531436690 ) ) ;
#77528=CARTESIAN_POINT ( 'NONE',  ( -9.564922557960796823, -16.46253265017161027, 102.0822429386477097 ) ) ;
#77529=CARTESIAN_POINT ( 'NONE',  ( -8.314922557961024197, 14.29746914071037800, 82.91775706135234714 ) ) ;
#77530=CARTESIAN_POINT ( 'NONE',  ( -5.823673210054431948, 21.52544592524334988, 62.70942372801902565 ) ) ;
#77531=CARTESIAN_POINT ( 'NONE',  ( 5.823673210054444382, -21.52544592524334988, 90.20942372801903275 ) ) ;
#77532=CARTESIAN_POINT ( 'NONE',  ( 21.55341960407619695, -5.719274019375665929, 21.04275706135234714 ) ) ;
#77533=CARTESIAN_POINT ( 'NONE',  ( -18.62759615963255300, -10.81492255796106328, 44.16775706135234714 ) ) ;
#77534=CARTESIAN_POINT ( 'NONE',  ( 12.06949235617739724, 12.14591786802326823, 76.87609039468567573 ) ) ;
#77535=CARTESIAN_POINT ( 'NONE',  ( 21.55341960407610458, 5.719274019375980345, 78.95724293864769550 ) ) ;
#77536=CARTESIAN_POINT ( 'NONE',  ( 9.474510206698729675, 16.51473224551082808, 27.08442372801900433 ) ) ;
#77537=CARTESIAN_POINT ( 'NONE',  ( 18.67979575497178502, 10.72451020669898547, 44.16557627198103120 ) ) ;
#77538=CARTESIAN_POINT ( 'NONE',  ( -9.564922557960796823, -16.46253265017161027, 87.08224293864769550 ) ) ;
#77539=CARTESIAN_POINT ( 'NONE',  ( -16.52544592524342804, 4.483927247898546575, 26.04057627198103475 ) ) ;
#77541=CARTESIAN_POINT ( 'NONE',  ( 16.46253265017160672, -9.564922557960803928, 98.33224293864769550 ) ) ;
#77542=DIRECTION ( 'NONE',  ( 0.000000000000000000, 0.000000000000000000, -1.000000000000000000 ) ) ;
#77543=CARTESIAN_POINT ( 'NONE',  ( 5.049401038297881783, 19.05341960407617563, 97.29275706135233293 ) ) ;
#77544=CARTESIAN_POINT ( 'NONE',  ( -5.719274019375978568, 21.55341960407610458, 70.20724293864769550 ) ) ;
#77545=CARTESIAN_POINT ( 'NONE',  ( 14.34966873604960469, 8.224510206698951720, 34.16557627198102409 ) ) ;
#77546=CARTESIAN_POINT ( 'NONE',  ( -16.51473224551082808, 9.474510206698731452, 108.3344237280190043 ) ) ;
#77547=CARTESIAN_POINT ( 'NONE',  ( -19.03943276465977164, 0.05219959533909376836, 36.24890960531436690 ) ) ;
#77548=CARTESIAN_POINT ( 'NONE',  ( -13.97604488694547697, 13.89961937509957934, 108.1260903946856331 ) ) ;
#77549=CARTESIAN_POINT ( 'NONE',  ( -21.53943276465977519, 0.05219959533907696930, 101.2489096053143669 ) ) ;
#77550=CARTESIAN_POINT ( 'NONE',  ( -19.02544592524334988, -5.153800228976617603, 73.95942372801900433 ) ) ;
#77551=CARTESIAN_POINT ( 'NONE',  ( -12.06949235617739369, -12.14591786802326823, 79.37609039468567573 ) ) ;
#77552=CARTESIAN_POINT ( 'NONE',  ( 5.153800228976335163, 19.02544592524342804, 84.79057627198099567 ) ) ;
#77553=CARTESIAN_POINT ( 'NONE',  ( 16.53943276465976808, -0.05219959533910856209, 73.74890960531433848 ) ) ;
#77554=CARTESIAN_POINT ( 'NONE',  ( 13.97604488694527802, 13.89961937509977652, 64.37390960531436690 ) ) ;
#77555=CARTESIAN_POINT ( 'NONE',  ( 0.05219959533910956823, 16.53943276465976808, 69.99890960531435269 ) ) ;
#77556=CARTESIAN_POINT ( 'NONE',  ( -16.46253265017160317, 9.564922557960807481, 35.83224293864768839 ) ) ;
#77558=CARTESIAN_POINT ( 'NONE',  ( -0.05219959533910754901, -16.53943276465976808, 47.49890960531435979 ) ) ;
#77559=CARTESIAN_POINT ( 'NONE',  ( -13.89961937509977652, 13.97604488694528158, 80.62390960531436690 ) ) ;
#77561=CARTESIAN_POINT ( 'NONE',  ( 19.02544592524334988, 5.153800228976608722, 46.45942372801899012 ) ) ;
#77562=CARTESIAN_POINT ( 'NONE',  ( -16.52544592524335698, -4.483927247898792601, 63.95942372801901854 ) ) ;
#77563=CARTESIAN_POINT ( 'NONE',  ( 10.81492255796078972, 18.62759615963270932, 64.58224293864769550 ) ) ;
#77564=CARTESIAN_POINT ( 'NONE',  ( 13.97604488694548053, -13.89961937509957401, 25.62609039468566507 ) ) ;
#77565=CARTESIAN_POINT ( 'NONE',  ( -19.03943276465977164, 0.05219959533909376836, 91.24890960531436690 ) ) ;
#77567=CARTESIAN_POINT ( 'NONE',  ( -10.81492255796078084, -18.62759615963271287, 27.08224293864769550 ) ) ;
#77568=CARTESIAN_POINT ( 'NONE',  ( 13.97604488694527802, 13.89961937509977652, 59.37390960531434558 ) ) ;
#77569=CARTESIAN_POINT ( 'NONE',  ( 10.72451020669871369, 18.67979575497193778, 47.08442372801901854 ) ) ;
#77570=CARTESIAN_POINT ( 'NONE',  ( 14.29746914071049879, -8.314922557960816363, 108.3322429386477097 ) ) ;
#77571=CARTESIAN_POINT ( 'NONE',  ( -0.05219959533907301413, -21.53943276465977519, 102.4989096053143811 ) ) ;
#77572=CARTESIAN_POINT ( 'NONE',  ( -19.02544592524342804, 5.153800228976336051, 96.04057627198103830 ) ) ;
#77574=CARTESIAN_POINT ( 'NONE',  ( -10.81492255796105439, 18.62759615963255655, 32.91775706135234714 ) ) ;
#77576=CARTESIAN_POINT ( 'NONE',  ( -9.564922557960796823, -16.46253265017161027, 92.08224293864769550 ) ) ;
#77577=CARTESIAN_POINT ( 'NONE',  ( 18.22780087662123805, -5.499999999999976019, 83.51763182126894947 ) ) ;
#77578=CARTESIAN_POINT ( 'NONE',  ( 10.72451020669898902, -18.67979575497178502, 92.91557627198103830 ) ) ;
#77579=CARTESIAN_POINT ( 'NONE',  ( 13.89961937509977652, -13.97604488694527269, 53.12390960531434558 ) ) ;
#77580=CARTESIAN_POINT ( 'NONE',  ( 12.14591786802327356, -12.06949235617739191, 20.62609039468568639 ) ) ;
#77582=CARTESIAN_POINT ( 'NONE',  ( -5.049401038298153566, 19.05341960407611168, 30.20724293864768839 ) ) ;
#77583=CARTESIAN_POINT ( 'NONE',  ( 18.62759615963255655, 10.81492255796105972, 86.66775706135234714 ) ) ;
#77584=CARTESIAN_POINT ( 'NONE',  ( 5.153800228976335163, 19.02544592524342804, 69.79057627198103830 ) ) ;
#77585=CARTESIAN_POINT ( 'NONE',  ( 21.55341960407619695, -5.719274019375665929, 51.04275706135234714 ) ) ;
#77586=AXIS2_PLACEMENT_3D ( 'NONE', #10461, #136766, #13435 ) ;
#77587=CARTESIAN_POINT ( 'NONE',  ( 15.72974639402176855, 15.80617190586768217, 31.87609039468567929 ) ) ;
#77589=CARTESIAN_POINT ( 'NONE',  ( 13.89961937509977652, -13.97604488694527269, 103.1239096053143527 ) ) ;
#77591=CARTESIAN_POINT ( 'NONE',  ( -16.55341960407617563, 4.379528057220093196, 33.54275706135234714 ) ) ;
#77592=CARTESIAN_POINT ( 'NONE',  ( -16.55341960407617563, 4.379528057220093196, 68.54275706135234714 ) ) ;
#77593=CARTESIAN_POINT ( 'NONE',  ( 18.62759615963255655, 10.81492255796105972, 61.66775706135235424 ) ) ;
#77594=CARTESIAN_POINT ( 'NONE',  ( 10.72451020669871369, 18.67979575497193778, 82.08442372801901854 ) ) ;
#77596=CARTESIAN_POINT ( 'NONE',  ( 13.97604488694548053, -13.89961937509957401, 110.6260903946856615 ) ) ;
#77597=CARTESIAN_POINT ( 'NONE',  ( 19.03943276465977164, -0.05219959533909143690, 63.74890960531435979 ) ) ;
#77598=CARTESIAN_POINT ( 'NONE',  ( 16.51473224551069308, 9.474510206698969483, 104.1655762719810241 ) ) ;
#77599=CARTESIAN_POINT ( 'NONE',  ( 4.483927247898545687, 16.52544592524342804, 104.7905762719810241 ) ) ;
#77600=CARTESIAN_POINT ( 'NONE',  ( -14.29746914071049879, 8.314922557960819915, 100.8322429386477097 ) ) ;
#77601=CARTESIAN_POINT ( 'NONE',  ( 21.52544592524344225, -5.823673210054117533, 33.54057627198102409 ) ) ;
#77602=CARTESIAN_POINT ( 'NONE',  ( 12.14591786802327356, -12.06949235617739191, 85.62609039468568994 ) ) ;
#77603=CARTESIAN_POINT ( 'NONE',  ( -8.224510206698948167, 14.34966873604960824, 70.41557627198102409 ) ) ;
#77604=CARTESIAN_POINT ( 'NONE',  ( -5.049401038298153566, 19.05341960407611168, 50.20724293864770260 ) ) ;
#77605=CARTESIAN_POINT ( 'NONE',  ( 21.53943276465977519, 0.05219959533937863772, 71.25109039468568994 ) ) ;
#77606=CARTESIAN_POINT ( 'NONE',  ( 18.67979575497194134, -10.72451020669871369, 70.83442372801901854 ) ) ;
#77607=CARTESIAN_POINT ( 'NONE',  ( 19.02544592524334988, 5.153800228976608722, 111.4594237280190043 ) ) ;
#77608=CARTESIAN_POINT ( 'NONE',  ( -4.483927247898539470, -16.52544592524342804, 72.29057627198102409 ) ) ;
#77609=CARTESIAN_POINT ( 'NONE',  ( -21.55341960407619339, 5.719274019375674811, 23.54275706135235424 ) ) ;
#77610=CARTESIAN_POINT ( 'NONE',  ( -21.55341960407610458, -5.719274019375992779, 66.45724293864768129 ) ) ;
#77611=CARTESIAN_POINT ( 'NONE',  ( -17.05116617787824396, -6.768360034955828830, 106.3432444674080273 ) ) ;
#77613=CARTESIAN_POINT ( 'NONE',  ( 16.51473224551069308, 9.474510206698969483, 69.16557627198102409 ) ) ;
#77614=CARTESIAN_POINT ( 'NONE',  ( -4.483927247898539470, -16.52544592524342804, 52.29057627198102409 ) ) ;
#77616=CARTESIAN_POINT ( 'NONE',  ( 14.34966873604960469, 8.224510206698951720, 24.16557627198103120 ) ) ;
#77617=CARTESIAN_POINT ( 'NONE',  ( -14.34966873604972548, 8.224510206698743886, 103.3344237280190043 ) ) ;
#77618=CARTESIAN_POINT ( 'NONE',  ( 19.02544592524334988, 5.153800228976608722, 56.45942372801898301 ) ) ;
#77620=CARTESIAN_POINT ( 'NONE',  ( -13.97604488694527625, -13.89961937509977652, 106.8739096053143669 ) ) ;
#77621=CARTESIAN_POINT ( 'NONE',  ( -16.55341960407611168, -4.379528057220339221, 71.45724293864769550 ) ) ;
#77622=CARTESIAN_POINT ( 'NONE',  ( 9.564922557961047289, -16.46253265017146816, 50.41775706135233293 ) ) ;
#77623=CARTESIAN_POINT ( 'NONE',  ( 13.89961937509977652, -13.97604488694527269, 38.12390960531436690 ) ) ;
#77624=CARTESIAN_POINT ( 'NONE',  ( 15.80617190586746368, 15.72974639402197994, 39.37390960531436690 ) ) ;
#77625=CARTESIAN_POINT ( 'NONE',  ( 18.67979575497178502, 10.72451020669898547, 54.16557627198103120 ) ) ;
#77627=CARTESIAN_POINT ( 'NONE',  ( 16.52544592524342804, -4.483927247898539470, 93.54057627198103830 ) ) ;
#77628=CARTESIAN_POINT ( 'NONE',  ( -8.314922557961024197, 14.29746914071037800, 57.91775706135234714 ) ) ;
#77629=CARTESIAN_POINT ( 'NONE',  ( -8.224510206698948167, 14.34966873604960824, 90.41557627198103830 ) ) ;
#77630=CARTESIAN_POINT ( 'NONE',  ( 17.40805194822032931, -6.112264579159339739, 38.33371272510613181 ) ) ;
#77632=CARTESIAN_POINT ( 'NONE',  ( -5.719274019375978568, 21.55341960407610458, 30.20724293864769550 ) ) ;
#77635=CARTESIAN_POINT ( 'NONE',  ( 4.379528057220092307, 16.55341960407617563, 47.29275706135234003 ) ) ;
#77636=CARTESIAN_POINT ( 'NONE',  ( 4.483927247898545687, 16.52544592524342804, 29.79057627198102409 ) ) ;
#77637=CARTESIAN_POINT ( 'NONE',  ( -18.62759615963270932, 10.81492255796079327, 50.83224293864770971 ) ) ;
#77638=CARTESIAN_POINT ( 'NONE',  ( 16.46253265017146816, 9.564922557961045513, 86.66775706135233293 ) ) ;
#77639=CARTESIAN_POINT ( 'NONE',  ( 15.72974639402199770, -15.80617190586745480, 63.12390960531435979 ) ) ;
#77640=CARTESIAN_POINT ( 'NONE',  ( 18.67979575497194134, -10.72451020669871369, 75.83442372801900433 ) ) ;
#77642=CARTESIAN_POINT ( 'NONE',  ( -4.483927247898782831, 16.52544592524335698, 47.70942372801902565 ) ) ;
#77643=CARTESIAN_POINT ( 'NONE',  ( -13.97604488694527625, -13.89961937509977652, 31.87390960531435979 ) ) ;
#77644=CARTESIAN_POINT ( 'NONE',  ( -19.02544592524342804, 5.153800228976336051, 101.0405762719810241 ) ) ;
#77645=CARTESIAN_POINT ( 'NONE',  ( -9.474510206698964154, 16.51473224551069663, 35.41557627198102409 ) ) ;
#77646=CARTESIAN_POINT ( 'NONE',  ( 16.53943276465976808, -0.05219959533910856209, 103.7489096053143669 ) ) ;
#77648=FACE_BOUND ( 'NONE', #53633, .T. ) ;
#77650=CARTESIAN_POINT ( 'NONE',  ( -14.29746914071037622, -8.314922557961029526, 64.16775706135234714 ) ) ;
#77651=CARTESIAN_POINT ( 'NONE',  ( 0.05219959533907565091, 21.53943276465977519, 84.99890960531436690 ) ) ;
#77652=CARTESIAN_POINT ( 'NONE',  ( 16.46253265017160672, -9.564922557960803928, 53.33224293864768839 ) ) ;
#77653=CARTESIAN_POINT ( 'NONE',  ( -10.81492255796105439, 18.62759615963255655, 27.91775706135234358 ) ) ;
#77654=CARTESIAN_POINT ( 'NONE',  ( 13.97604488694527802, 13.89961937509977652, 89.37390960531436690 ) ) ;
#77657=CARTESIAN_POINT ( 'NONE',  ( -10.72451020669870658, -18.67979575497194134, 24.58442372801901499 ) ) ;
#77658=CARTESIAN_POINT ( 'NONE',  ( -9.564922557960796823, -16.46253265017161027, 22.08224293864768839 ) ) ;
#77659=CARTESIAN_POINT ( 'NONE',  ( 9.564922557960805705, 16.46253265017160317, 109.5822429386476955 ) ) ;
#77660=CARTESIAN_POINT ( 'NONE',  ( 5.049401038297881783, 19.05341960407617563, 72.29275706135234714 ) ) ;
#77661=CARTESIAN_POINT ( 'NONE',  ( 13.89961937509957401, 13.97604488694547697, 31.87609039468566863 ) ) ;
#77662=CARTESIAN_POINT ( 'NONE',  ( -15.72974639402197994, 15.80617190586746368, 100.6239096053143811 ) ) ;
#77663=CARTESIAN_POINT ( 'NONE',  ( 0.05219959533936267826, -19.03943276465977164, 30.00109039468566863 ) ) ;
#77664=CARTESIAN_POINT ( 'NONE',  ( 12.14591786802327356, -12.06949235617739191, 75.62609039468567573 ) ) ;
#77665=CARTESIAN_POINT ( 'NONE',  ( -13.97604488694527625, -13.89961937509977652, 106.8739096053143669 ) ) ;
#77666=CARTESIAN_POINT ( 'NONE',  ( -13.89961937509977652, 13.97604488694528158, 55.62390960531434558 ) ) ;
#77667=CARTESIAN_POINT ( 'NONE',  ( -10.72451020669870658, -18.67979575497194134, 69.58442372801900433 ) ) ;
#77668=CARTESIAN_POINT ( 'NONE',  ( 21.55341960407619695, -5.719274019375665929, 81.04275706135236135 ) ) ;
#77669=CARTESIAN_POINT ( 'NONE',  ( 16.51473224551069308, 9.474510206698969483, 69.16557627198102409 ) ) ;
#77670=CARTESIAN_POINT ( 'NONE',  ( -21.53943276465977519, -0.05219959533937600094, 48.75109039468568284 ) ) ;
#77671=CARTESIAN_POINT ( 'NONE',  ( -9.474510206698720793, -16.51473224551083518, 89.58442372801900433 ) ) ;
#77672=CARTESIAN_POINT ( 'NONE',  ( 13.97604488694527802, 13.89961937509977652, 49.37390960531434558 ) ) ;
#77673=CARTESIAN_POINT ( 'NONE',  ( -5.049401038298153566, 19.05341960407611168, 100.2072429386476955 ) ) ;
#77674=CARTESIAN_POINT ( 'NONE',  ( 19.02544592524343514, -5.153800228976328945, 68.54057627198103830 ) ) ;
#77675=CARTESIAN_POINT ( 'NONE',  ( -19.05341960407611168, -5.049401038298163336, 111.4572429386476671 ) ) ;
#77676=CARTESIAN_POINT ( 'NONE',  ( -5.153800228976328057, -19.02544592524343514, 57.29057627198103120 ) ) ;
#77677=CARTESIAN_POINT ( 'NONE',  ( -21.55341960407610458, -5.719274019375992779, 101.4572429386476955 ) ) ;
#77678=CARTESIAN_POINT ( 'NONE',  ( 4.483927247898790824, -16.52544592524335698, 70.20942372801904696 ) ) ;
#77679=VECTOR ( 'NONE', #30824, 1000.000000000000000 ) ;
#77681=CARTESIAN_POINT ( 'NONE',  ( -13.89961937509957401, -13.97604488694547875, 44.37609039468566863 ) ) ;
#77682=CARTESIAN_POINT ( 'NONE',  ( 5.153800228976335163, 19.02544592524342804, 59.79057627198100988 ) ) ;
#77683=CARTESIAN_POINT ( 'NONE',  ( -0.05219959533910754901, -16.53943276465976808, 57.49890960531435979 ) ) ;
#77684=CARTESIAN_POINT ( 'NONE',  ( 4.483927247898545687, 16.52544592524342804, 89.79057627198103830 ) ) ;
#77685=CARTESIAN_POINT ( 'NONE',  ( -19.02544592524342804, 5.153800228976336051, 111.0405762719810099 ) ) ;
#77686=CARTESIAN_POINT ( 'NONE',  ( -9.564922557960796823, -16.46253265017161027, 97.08224293864769550 ) ) ;
#77687=CARTESIAN_POINT ( 'NONE',  ( 9.564922557960805705, 16.46253265017160317, 104.5822429386476955 ) ) ;
#77688=CARTESIAN_POINT ( 'NONE',  ( -5.823673210054431948, 21.52544592524334988, 107.7094237280190328 ) ) ;
#77689=CARTESIAN_POINT ( 'NONE',  ( 12.06949235617739724, 12.14591786802326823, 96.87609039468568994 ) ) ;
#77690=CARTESIAN_POINT ( 'NONE',  ( 9.474510206698971260, -16.51473224551069308, 77.91557627198103830 ) ) ;
#77691=CARTESIAN_POINT ( 'NONE',  ( -0.05219959533937732626, 21.53943276465977519, 37.50109039468568284 ) ) ;
#77692=CARTESIAN_POINT ( 'NONE',  ( -15.80617190586745835, -15.72974639402198527, 36.87390960531435979 ) ) ;
#77693=CARTESIAN_POINT ( 'NONE',  ( -18.67979575497178146, -10.72451020669898902, 101.6655762719810383 ) ) ;
#77694=CARTESIAN_POINT ( 'NONE',  ( -0.05219959533910754901, -16.53943276465976808, 62.49890960531436690 ) ) ;
#77695=CARTESIAN_POINT ( 'NONE',  ( -19.03943276465977164, 0.05219959533909376836, 56.24890960531435979 ) ) ;
#77696=CARTESIAN_POINT ( 'NONE',  ( 12.06949235617757843, -12.14591786802309237, 83.12390960531436690 ) ) ;
#77697=CARTESIAN_POINT ( 'NONE',  ( 16.46253265017146816, 9.564922557961045513, 41.66775706135234003 ) ) ;
#77699=CARTESIAN_POINT ( 'NONE',  ( 16.53943276465976808, -0.05219959533910856209, 108.7489096053143669 ) ) ;
#77700=CARTESIAN_POINT ( 'NONE',  ( -5.049401038298153566, 19.05341960407611168, 80.20724293864769550 ) ) ;
#77701=CARTESIAN_POINT ( 'NONE',  ( -9.474510206698964154, 16.51473224551069663, 75.41557627198103830 ) ) ;
#77703=CARTESIAN_POINT ( 'NONE',  ( 12.14591786802309770, 12.06949235617756955, 94.37390960531436690 ) ) ;
#77705=CARTESIAN_POINT ( 'NONE',  ( 16.53943276465976808, 0.05219959533934440121, 101.2510903946856757 ) ) ;
#77706=CARTESIAN_POINT ( 'NONE',  ( 16.55341960407618274, -4.379528057220086978, 31.04275706135234714 ) ) ;
#77707=CARTESIAN_POINT ( 'NONE',  ( -21.53943276465977519, -0.05219959533937600094, 98.75109039468568994 ) ) ;
#77708=CARTESIAN_POINT ( 'NONE',  ( -19.03943276465977164, 0.05219959533909376836, 91.24890960531436690 ) ) ;
#77709=CARTESIAN_POINT ( 'NONE',  ( -5.823673210054431948, 21.52544592524334988, 22.70942372801901499 ) ) ;
#77710=CARTESIAN_POINT ( 'NONE',  ( 0.05219959533909260263, 19.03943276465977164, 24.99890960531435269 ) ) ;
#77711=CARTESIAN_POINT ( 'NONE',  ( 14.29746914071037800, 8.314922557961029526, 26.66775706135235424 ) ) ;
#77712=CARTESIAN_POINT ( 'NONE',  ( -13.97604488694547697, 13.89961937509957934, 93.12609039468566152 ) ) ;
#77713=CARTESIAN_POINT ( 'NONE',  ( 10.81492255796078972, 18.62759615963270932, 94.58224293864769550 ) ) ;
#77714=CARTESIAN_POINT ( 'NONE',  ( 9.564922557961047289, -16.46253265017146816, 70.41775706135233293 ) ) ;
#77716=CARTESIAN_POINT ( 'NONE',  ( 15.72974639402199770, -15.80617190586745480, 113.1239096053143953 ) ) ;
#77718=CARTESIAN_POINT ( 'NONE',  ( 13.89961937509977652, -13.97604488694527269, 93.12390960531436690 ) ) ;
#77719=CARTESIAN_POINT ( 'NONE',  ( 16.55341960407618274, -4.379528057220086978, 46.04275706135234714 ) ) ;
#77721=CARTESIAN_POINT ( 'NONE',  ( -19.02544592524334988, -5.153800228976617603, 58.95942372801900433 ) ) ;
#77722=CARTESIAN_POINT ( 'NONE',  ( 21.52544592524334988, 5.823673210054432836, 21.45942372801901499 ) ) ;
#77723=CARTESIAN_POINT ( 'NONE',  ( 8.314922557960818139, 14.29746914071049879, 79.58224293864769550 ) ) ;
#77724=CARTESIAN_POINT ( 'NONE',  ( -0.05219959533909027116, -19.03943276465977164, 87.49890960531436690 ) ) ;
#77725=CARTESIAN_POINT ( 'NONE',  ( 14.34966873604972726, -8.224510206698740333, 45.83442372801901854 ) ) ;
#77726=CARTESIAN_POINT ( 'NONE',  ( 9.474510206698729675, 16.51473224551082808, 57.08442372801900433 ) ) ;
#77727=CARTESIAN_POINT ( 'NONE',  ( 10.81492255796106328, -18.62759615963255655, 70.41775706135236135 ) ) ;
#77728=CARTESIAN_POINT ( 'NONE',  ( 14.34966873604972726, -8.224510206698740333, 30.83442372801902209 ) ) ;
#77729=CARTESIAN_POINT ( 'NONE',  ( -19.05341960407611168, -5.049401038298163336, 71.45724293864766707 ) ) ;
#77730=CARTESIAN_POINT ( 'NONE',  ( 19.03943276465977164, 0.05219959533936151252, 81.25109039468567573 ) ) ;
#77731=CARTESIAN_POINT ( 'NONE',  ( -16.52544592524335698, -4.483927247898792601, 58.95942372801902565 ) ) ;
#77732=CARTESIAN_POINT ( 'NONE',  ( 10.72451020669871369, 18.67979575497193778, 92.08442372801901854 ) ) ;
#77733=CARTESIAN_POINT ( 'NONE',  ( -19.03943276465977164, -0.05219959533935918106, 78.75109039468567573 ) ) ;
#77734=CARTESIAN_POINT ( 'NONE',  ( -16.46253265017160317, 9.564922557960807481, 50.83224293864770260 ) ) ;
#77735=CARTESIAN_POINT ( 'NONE',  ( 15.80617190586746368, 15.72974639402197994, 74.37390960531436690 ) ) ;
#77736=CARTESIAN_POINT ( 'NONE',  ( -14.34966873604960291, -8.224510206698953496, 81.66557627198103830 ) ) ;
#77737=CARTESIAN_POINT ( 'NONE',  ( -13.89961937509957401, -13.97604488694547875, 84.37609039468567573 ) ) ;
#77738=CARTESIAN_POINT ( 'NONE',  ( -18.22780087662123094, -5.499999999999984901, 71.48459894673891313 ) ) ;
#77739=CARTESIAN_POINT ( 'NONE',  ( 16.46253265017146816, 9.564922557961045513, 41.66775706135234003 ) ) ;
#77740=CARTESIAN_POINT ( 'NONE',  ( -12.14591786802326823, 12.06949235617739902, 98.12609039468570415 ) ) ;
#77741=CARTESIAN_POINT ( 'NONE',  ( 16.52544592524342804, -4.483927247898539470, 68.54057627198103830 ) ) ;
#77742=CARTESIAN_POINT ( 'NONE',  ( 18.67979575497194134, -10.72451020669871369, 100.8344237280190185 ) ) ;
#77744=CARTESIAN_POINT ( 'NONE',  ( 18.67979575497178502, 10.72451020669898547, 109.1655762719810383 ) ) ;
#77745=CARTESIAN_POINT ( 'NONE',  ( 19.05341960407611168, 5.049401038298154454, 58.95724293864768129 ) ) ;
#77746=CARTESIAN_POINT ( 'NONE',  ( 21.55341960407619695, -5.719274019375665929, 76.04275706135237556 ) ) ;
#77747=CARTESIAN_POINT ( 'NONE',  ( 16.51473224551069308, 9.474510206698969483, 54.16557627198103120 ) ) ;
#77749=CARTESIAN_POINT ( 'NONE',  ( 5.049401038298161559, -19.05341960407611168, 27.70724293864769550 ) ) ;
#77750=CARTESIAN_POINT ( 'NONE',  ( -21.55341960407610458, -5.719274019375992779, 21.45724293864769550 ) ) ;
#77751=CARTESIAN_POINT ( 'NONE',  ( -12.06949235617756955, 12.14591786802309770, 65.62390960531436690 ) ) ;
#77752=CARTESIAN_POINT ( 'NONE',  ( 13.97604488694527802, 13.89961937509977652, 24.37390960531435624 ) ) ;
#77753=CARTESIAN_POINT ( 'NONE',  ( 4.483927247898545687, 16.52544592524342804, 84.79057627198102409 ) ) ;
#77754=CARTESIAN_POINT ( 'NONE',  ( 5.719274019375991003, -21.55341960407610458, 92.70724293864770971 ) ) ;
#77755=CARTESIAN_POINT ( 'NONE',  ( 5.719274019375673035, 21.55341960407619339, 42.29275706135235424 ) ) ;
#77757=CARTESIAN_POINT ( 'NONE',  ( 4.379528057220092307, 16.55341960407617563, 47.29275706135234003 ) ) ;
#77758=CARTESIAN_POINT ( 'NONE',  ( 21.53943276465977519, -0.05219959533907433946, 103.7489096053143669 ) ) ;
#77759=CARTESIAN_POINT ( 'NONE',  ( 19.05341960407617918, -5.049401038297876454, 26.04275706135233293 ) ) ;
#77760=CARTESIAN_POINT ( 'NONE',  ( -19.05341960407611168, -5.049401038298163336, 111.4572429386476671 ) ) ;
#77761=CARTESIAN_POINT ( 'NONE',  ( 18.67979575497194134, -10.72451020669871369, 40.83442372801901854 ) ) ;
#77762=CARTESIAN_POINT ( 'NONE',  ( 5.823673210054125526, 21.52544592524343514, 49.79057627198102409 ) ) ;
#77763=CARTESIAN_POINT ( 'NONE',  ( -0.05219959533910754901, -16.53943276465976808, 27.49890960531435269 ) ) ;
#77764=CARTESIAN_POINT ( 'NONE',  ( 5.823673210054444382, -21.52544592524334988, 65.20942372801901854 ) ) ;
#77765=CARTESIAN_POINT ( 'NONE',  ( -21.53943276465977519, -0.05219959533937600094, 98.75109039468568994 ) ) ;
#77766=CARTESIAN_POINT ( 'NONE',  ( 9.564922557961047289, -16.46253265017146816, 25.41775706135234003 ) ) ;
#77767=CARTESIAN_POINT ( 'NONE',  ( 16.53943276465976808, 0.05219959533934440121, 91.25109039468568994 ) ) ;
#77768=CARTESIAN_POINT ( 'NONE',  ( 21.53943276465977519, 0.05219959533937863772, 51.25109039468568994 ) ) ;
#77769=CARTESIAN_POINT ( 'NONE',  ( -5.049401038298153566, 19.05341960407611168, 40.20724293864768839 ) ) ;
#77770=CARTESIAN_POINT ( 'NONE',  ( -0.05219959533937732626, 21.53943276465977519, 112.5010903946857042 ) ) ;
#77771=CARTESIAN_POINT ( 'NONE',  ( 18.67979575497178502, 10.72451020669898547, 24.16557627198103120 ) ) ;
#77772=CARTESIAN_POINT ( 'NONE',  ( 5.823673210054444382, -21.52544592524334988, 25.20942372801901854 ) ) ;
#77773=CARTESIAN_POINT ( 'NONE',  ( -21.52544592524343514, 5.823673210054127303, 76.04057627198102409 ) ) ;
#77774=CARTESIAN_POINT ( 'NONE',  ( 16.53943276465976808, 0.05219959533934440121, 41.25109039468568284 ) ) ;
#77775=CARTESIAN_POINT ( 'NONE',  ( 5.719274019375991003, -21.55341960407610458, 77.70724293864770971 ) ) ;
#77776=CARTESIAN_POINT ( 'NONE',  ( 16.53943276465976808, 0.05219959533934440121, 66.25109039468567573 ) ) ;
#77777=CARTESIAN_POINT ( 'NONE',  ( 16.52544592524342804, -4.483927247898539470, 63.54057627198103830 ) ) ;
#77779=CARTESIAN_POINT ( 'NONE',  ( 16.46253265017146816, 9.564922557961045513, 101.6677570613523329 ) ) ;
#77781=CARTESIAN_POINT ( 'NONE',  ( 12.14591786802327356, -12.06949235617739191, 40.62609039468567573 ) ) ;
#77782=CARTESIAN_POINT ( 'NONE',  ( -21.52544592524343514, 5.823673210054127303, 116.0405762719810383 ) ) ;
#77783=CARTESIAN_POINT ( 'NONE',  ( -5.823673210054116645, -21.52544592524344225, 37.29057627198102409 ) ) ;
#77784=CARTESIAN_POINT ( 'NONE',  ( 16.52544592524335698, 4.483927247898782831, 51.45942372801901854 ) ) ;
#77785=CARTESIAN_POINT ( 'NONE',  ( 5.049401038298161559, -19.05341960407611168, 72.70724293864768129 ) ) ;
#77786=CARTESIAN_POINT ( 'NONE',  ( -18.67979575497193778, 10.72451020669871902, 48.33442372801902565 ) ) ;
#77787=CARTESIAN_POINT ( 'NONE',  ( -19.02544592524334988, -5.153800228976617603, 108.9594237280189759 ) ) ;
#77788=CARTESIAN_POINT ( 'NONE',  ( 21.55341960407610458, 5.719274019375980345, 23.95724293864769550 ) ) ;
#77790=CARTESIAN_POINT ( 'NONE',  ( 5.049401038297881783, 19.05341960407617563, 32.29275706135233293 ) ) ;
#77791=CARTESIAN_POINT ( 'NONE',  ( 16.53943276465976808, 0.05219959533934440121, 36.25109039468567573 ) ) ;
#77792=CARTESIAN_POINT ( 'NONE',  ( 9.564922557960805705, 16.46253265017160317, 99.58224293864770971 ) ) ;
#77793=CARTESIAN_POINT ( 'NONE',  ( 18.67979575497178502, 10.72451020669898547, 109.1655762719810383 ) ) ;
#77794=CARTESIAN_POINT ( 'NONE',  ( -16.51473224551069308, -9.474510206698971260, 76.66557627198103830 ) ) ;
#77795=CARTESIAN_POINT ( 'NONE',  ( -17.26172910966779028, 6.454744622555852018, 25.80646908649224613 ) ) ;
#77796=CARTESIAN_POINT ( 'NONE',  ( -4.483927247898539470, -16.52544592524342804, 82.29057627198103830 ) ) ;
#77797=CARTESIAN_POINT ( 'NONE',  ( 10.72451020669898902, -18.67979575497178502, 22.91557627198102765 ) ) ;
#77799=CARTESIAN_POINT ( 'NONE',  ( -4.379528057220086978, -16.55341960407618274, 64.79275706135234714 ) ) ;
#77800=CARTESIAN_POINT ( 'NONE',  ( 18.67979575497178502, 10.72451020669898547, 104.1655762719810241 ) ) ;
#77801=CARTESIAN_POINT ( 'NONE',  ( -19.02544592524334988, -5.153800228976617603, 58.95942372801900433 ) ) ;
#77802=CARTESIAN_POINT ( 'NONE',  ( 10.72451020669898902, -18.67979575497178502, 32.91557627198102409 ) ) ;
#77803=CARTESIAN_POINT ( 'NONE',  ( -5.049401038298153566, 19.05341960407611168, 25.20724293864768484 ) ) ;
#77804=CARTESIAN_POINT ( 'NONE',  ( -10.81492255796078084, -18.62759615963271287, 72.08224293864769550 ) ) ;
#77805=CARTESIAN_POINT ( 'NONE',  ( 13.89961937509977652, -13.97604488694527269, 93.12390960531436690 ) ) ;
#77806=CARTESIAN_POINT ( 'NONE',  ( 18.62759615963255655, 10.81492255796105972, 91.66775706135234714 ) ) ;
#77807=CARTESIAN_POINT ( 'NONE',  ( 5.153800228976335163, 19.02544592524342804, 54.79057627198103120 ) ) ;
#77808=CARTESIAN_POINT ( 'NONE',  ( 8.224510206698742110, 14.34966873604972548, 32.08442372801901854 ) ) ;
#77809=CARTESIAN_POINT ( 'NONE',  ( 13.89961937509977652, -13.97604488694527269, 53.12390960531434558 ) ) ;
#77810=CARTESIAN_POINT ( 'NONE',  ( 21.55341960407619695, -5.719274019375665929, 86.04275706135236135 ) ) ;
#77811=ORIENTED_EDGE ( 'NONE', *, *, #66266, .T. ) ;
#77812=CARTESIAN_POINT ( 'NONE',  ( -0.05219959533936034679, 19.03943276465977164, 42.50109039468566152 ) ) ;
#77813=CARTESIAN_POINT ( 'NONE',  ( 16.46253265017146816, 9.564922557961045513, 41.66775706135234003 ) ) ;
#77814=CARTESIAN_POINT ( 'NONE',  ( 18.62759615963255655, 10.81492255796105972, 41.66775706135235424 ) ) ;
#77815=CARTESIAN_POINT ( 'NONE',  ( 5.153800228976335163, 19.02544592524342804, 54.79057627198103120 ) ) ;
#77816=CARTESIAN_POINT ( 'NONE',  ( 19.02544592524334988, 5.153800228976608722, 26.45942372801899722 ) ) ;
#77817=CARTESIAN_POINT ( 'NONE',  ( -19.03943276465977164, 0.05219959533909376836, 86.24890960531436690 ) ) ;
#77818=CARTESIAN_POINT ( 'NONE',  ( 16.51473224551069308, 9.474510206698969483, 64.16557627198102409 ) ) ;
#77819=CARTESIAN_POINT ( 'NONE',  ( -16.52544592524342804, 4.483927247898546575, 31.04057627198102409 ) ) ;
#77820=CARTESIAN_POINT ( 'NONE',  ( -9.564922557960796823, -16.46253265017161027, 112.0822429386476955 ) ) ;
#77821=CARTESIAN_POINT ( 'NONE',  ( -21.53943276465977519, -0.05219959533937600094, 83.75109039468568994 ) ) ;
#77823=CARTESIAN_POINT ( 'NONE',  ( 17.44270441346513323, 5.991230190323100224, 58.86335079264229364 ) ) ;
#77824=CARTESIAN_POINT ( 'NONE',  ( -21.52544592524334988, -5.823673210054445271, 93.95942372801903275 ) ) ;
#77826=CARTESIAN_POINT ( 'NONE',  ( -16.51473224551069308, -9.474510206698971260, 26.66557627198103120 ) ) ;
#77830=CARTESIAN_POINT ( 'NONE',  ( -12.06949235617739369, -12.14591786802326823, 54.37609039468568994 ) ) ;
#77831=CARTESIAN_POINT ( 'NONE',  ( 18.67979575497178502, 10.72451020669898547, 69.16557627198102409 ) ) ;
#77832=CARTESIAN_POINT ( 'NONE',  ( -16.52544592524342804, 4.483927247898546575, 36.04057627198102409 ) ) ;
#77833=CARTESIAN_POINT ( 'NONE',  ( 4.379528057220339221, -16.55341960407611168, 107.7072429386476955 ) ) ;
#77834=CARTESIAN_POINT ( 'NONE',  ( -5.049401038298153566, 19.05341960407611168, 90.20724293864766707 ) ) ;
#77835=CARTESIAN_POINT ( 'NONE',  ( -19.03943276465977164, -0.05219959533935918106, 23.75109039468566152 ) ) ;
#77836=CARTESIAN_POINT ( 'NONE',  ( -16.53943276465976808, 0.05219959533911058130, 116.2489096053143669 ) ) ;
#77837=CARTESIAN_POINT ( 'NONE',  ( 10.72451020669871369, 18.67979575497193778, 72.08442372801899012 ) ) ;
#77838=CARTESIAN_POINT ( 'NONE',  ( -19.02544592524342804, 5.153800228976336051, 111.0405762719810099 ) ) ;
#77839=CARTESIAN_POINT ( 'NONE',  ( 8.224510206698742110, 14.34966873604972548, 112.0844237280190185 ) ) ;
#77840=CARTESIAN_POINT ( 'NONE',  ( 19.03943276465977164, 0.05219959533936151252, 71.25109039468566152 ) ) ;
#77842=CARTESIAN_POINT ( 'NONE',  ( 13.89961937509977652, -13.97604488694527269, 108.1239096053143669 ) ) ;
#77843=CARTESIAN_POINT ( 'NONE',  ( 12.14591786802309770, 12.06949235617756955, 94.37390960531436690 ) ) ;
#77844=CARTESIAN_POINT ( 'NONE',  ( -0.05219959533936034679, 19.03943276465977164, 62.50109039468566863 ) ) ;
#77845=CARTESIAN_POINT ( 'NONE',  ( 0.05219959533909260263, 19.03943276465977164, 69.99890960531435269 ) ) ;
#77846=CARTESIAN_POINT ( 'NONE',  ( 14.29746914071049879, -8.314922557960816363, 68.33224293864769550 ) ) ;
#77847=CARTESIAN_POINT ( 'NONE',  ( 19.02544592524334988, 5.153800228976608722, 91.45942372801900433 ) ) ;
#77848=CARTESIAN_POINT ( 'NONE',  ( -18.67979575497178146, -10.72451020669898902, 46.66557627198102409 ) ) ;
#77850=CARTESIAN_POINT ( 'NONE',  ( -14.29746914071049879, 8.314922557960819915, 110.8322429386476955 ) ) ;
#77851=CARTESIAN_POINT ( 'NONE',  ( 9.564922557961047289, -16.46253265017146816, 100.4177570613523329 ) ) ;
#77852=CARTESIAN_POINT ( 'NONE',  ( -16.51473224551069308, -9.474510206698971260, 71.66557627198102409 ) ) ;
#77853=CARTESIAN_POINT ( 'NONE',  ( -21.52544592524343514, 5.823673210054127303, 71.04057627198103830 ) ) ;
#77854=CARTESIAN_POINT ( 'NONE',  ( 14.34966873604972726, -8.224510206698740333, 95.83442372801903275 ) ) ;
#77855=CARTESIAN_POINT ( 'NONE',  ( 13.89961937509977652, -13.97604488694527269, 68.12390960531436690 ) ) ;
#77856=CARTESIAN_POINT ( 'NONE',  ( -19.03943276465977164, -0.05219959533935918106, 63.75109039468566863 ) ) ;
#77857=CARTESIAN_POINT ( 'NONE',  ( -5.823673210054431948, 21.52544592524334988, 87.70942372801901854 ) ) ;
#77858=CARTESIAN_POINT ( 'NONE',  ( -5.823673210054116645, -21.52544592524344225, 67.29057627198103830 ) ) ;
#77859=CARTESIAN_POINT ( 'NONE',  ( 0.05219959533907565091, 21.53943276465977519, 24.99890960531435624 ) ) ;
#77860=CARTESIAN_POINT ( 'NONE',  ( 16.46253265017160672, -9.564922557960803928, 38.33224293864768839 ) ) ;
#77861=CARTESIAN_POINT ( 'NONE',  ( -14.34966873604972548, 8.224510206698743886, 98.33442372801901854 ) ) ;
#77862=CARTESIAN_POINT ( 'NONE',  ( -13.97604488694527625, -13.89961937509977652, 46.87390960531435979 ) ) ;
#77863=CARTESIAN_POINT ( 'NONE',  ( 16.52544592524335698, 4.483927247898782831, 21.45942372801901499 ) ) ;
#77864=CARTESIAN_POINT ( 'NONE',  ( -30.00000000000000000, -5.510910596163089556E-15, 45.00000000000000000 ) ) ;
#77865=CARTESIAN_POINT ( 'NONE',  ( 19.02544592524334988, 5.153800228976608722, 21.45942372801899012 ) ) ;
#77866=CARTESIAN_POINT ( 'NONE',  ( 0.05219959533910956823, 16.53943276465976808, 54.99890960531435269 ) ) ;
#77867=CARTESIAN_POINT ( 'NONE',  ( -18.67979575497178146, -10.72451020669898902, 101.6655762719810383 ) ) ;
#77868=CARTESIAN_POINT ( 'NONE',  ( 5.823673210054125526, 21.52544592524343514, 104.7905762719810241 ) ) ;
#77869=CARTESIAN_POINT ( 'NONE',  ( 16.79531203550648044, -7.028104445595601213, 96.24755011779556924 ) ) ;
#77870=CARTESIAN_POINT ( 'NONE',  ( 5.719274019375991003, -21.55341960407610458, 47.70724293864770260 ) ) ;
#77871=CARTESIAN_POINT ( 'NONE',  ( 4.379528057220092307, 16.55341960407617563, 82.29275706135234714 ) ) ;
#77872=CARTESIAN_POINT ( 'NONE',  ( -16.53943276465976808, 0.05219959533911058130, 86.24890960531436690 ) ) ;
#77873=CARTESIAN_POINT ( 'NONE',  ( -13.97604488694527625, -13.89961937509977652, 46.87390960531435979 ) ) ;
#77875=CARTESIAN_POINT ( 'NONE',  ( -8.314922557961024197, 14.29746914071037800, 107.9177570613523471 ) ) ;
#77876=CARTESIAN_POINT ( 'NONE',  ( -10.81492255796105439, 18.62759615963255655, 27.91775706135234358 ) ) ;
#77877=CARTESIAN_POINT ( 'NONE',  ( -13.97604488694527625, -13.89961937509977652, 101.8739096053143811 ) ) ;
#77878=CARTESIAN_POINT ( 'NONE',  ( 5.719274019375673035, 21.55341960407619339, 62.29275706135236845 ) ) ;
#77882=CARTESIAN_POINT ( 'NONE',  ( 10.81492255796106328, -18.62759615963255655, 60.41775706135235424 ) ) ;
#77883=CARTESIAN_POINT ( 'NONE',  ( -16.46253265017160317, 9.564922557960807481, 45.83224293864769550 ) ) ;
#77884=CARTESIAN_POINT ( 'NONE',  ( 17.60728821187776916, -5.500000000000036415, 58.36690927743609336 ) ) ;
#77885=CARTESIAN_POINT ( 'NONE',  ( 9.474510206698971260, -16.51473224551069308, 92.91557627198103830 ) ) ;
#77886=CARTESIAN_POINT ( 'NONE',  ( 16.51473224551083163, -9.474510206698727899, 65.83442372801900433 ) ) ;
#77887=CARTESIAN_POINT ( 'NONE',  ( 15.80617190586769283, -15.72974639402175789, 40.62609039468567573 ) ) ;
#77888=CARTESIAN_POINT ( 'NONE',  ( 9.564922557961047289, -16.46253265017146816, 105.4177570613523471 ) ) ;
#77889=CARTESIAN_POINT ( 'NONE',  ( -13.97604488694547697, 13.89961937509957934, 68.12609039468563310 ) ) ;
#77890=CARTESIAN_POINT ( 'NONE',  ( -13.89961937509977652, 13.97604488694528158, 35.62390960531435269 ) ) ;
#77891=CARTESIAN_POINT ( 'NONE',  ( -12.06949235617739369, -12.14591786802326823, 109.3760903946857042 ) ) ;
#77892=CARTESIAN_POINT ( 'NONE',  ( -9.564922557961040184, 16.46253265017147172, 77.91775706135234714 ) ) ;
#77893=CARTESIAN_POINT ( 'NONE',  ( -8.314922557960811034, -14.29746914071050412, 22.08224293864769194 ) ) ;
#77894=CARTESIAN_POINT ( 'NONE',  ( 9.564922557961047289, -16.46253265017146816, 45.41775706135232582 ) ) ;
#77895=CARTESIAN_POINT ( 'NONE',  ( 18.67979575497194134, -10.72451020669871369, 105.8344237280190328 ) ) ;
#77896=CARTESIAN_POINT ( 'NONE',  ( -19.05341960407617563, 5.049401038297882671, 23.54275706135233648 ) ) ;
#77898=CARTESIAN_POINT ( 'NONE',  ( -19.03943276465977164, 0.05219959533909376836, 31.24890960531435979 ) ) ;
#77899=CARTESIAN_POINT ( 'NONE',  ( 5.719274019375673035, 21.55341960407619339, 82.29275706135234714 ) ) ;
#77900=CARTESIAN_POINT ( 'NONE',  ( -8.314922557961024197, 14.29746914071037800, 27.91775706135234358 ) ) ;
#77901=CARTESIAN_POINT ( 'NONE',  ( -19.05341960407611168, -5.049401038298163336, 91.45724293864766707 ) ) ;
#77903=CARTESIAN_POINT ( 'NONE',  ( -13.89961937509977652, 13.97604488694528158, 75.62390960531438111 ) ) ;
#77904=CARTESIAN_POINT ( 'NONE',  ( -17.44279575226783763, 5.990770900254001496, 100.8355756751431898 ) ) ;
#77905=CARTESIAN_POINT ( 'NONE',  ( -16.51473224551082808, 9.474510206698731452, 78.33442372801900433 ) ) ;
#77906=CARTESIAN_POINT ( 'NONE',  ( -16.46253265017160317, 9.564922557960807481, 110.8322429386476955 ) ) ;
#77907=CARTESIAN_POINT ( 'NONE',  ( 0.05219959533937995610, -21.53943276465977519, 110.0010903946856757 ) ) ;
#77908=CARTESIAN_POINT ( 'NONE',  ( -8.314922557960811034, -14.29746914071050412, 92.08224293864769550 ) ) ;
#77909=CARTESIAN_POINT ( 'NONE',  ( -19.05341960407611168, -5.049401038298163336, 26.45724293864769550 ) ) ;
#77910=CARTESIAN_POINT ( 'NONE',  ( -21.55341960407610458, -5.719274019375992779, 61.45724293864770260 ) ) ;
#77911=CARTESIAN_POINT ( 'NONE',  ( 15.80617190586746368, 15.72974639402197994, 39.37390960531436690 ) ) ;
#77912=CARTESIAN_POINT ( 'NONE',  ( 14.29746914071049879, -8.314922557960816363, 113.3322429386476955 ) ) ;
#77914=CARTESIAN_POINT ( 'NONE',  ( -16.51473224551082808, 9.474510206698731452, 63.33442372801900433 ) ) ;
#77915=CARTESIAN_POINT ( 'NONE',  ( -14.34966873604960291, -8.224510206698953496, 46.66557627198102409 ) ) ;
#77916=CARTESIAN_POINT ( 'NONE',  ( -19.03943276465977164, 0.05219959533909376836, 116.2489096053143669 ) ) ;
#77917=CARTESIAN_POINT ( 'NONE',  ( 0.05219959533937995610, -21.53943276465977519, 75.00109039468568994 ) ) ;
#77918=CARTESIAN_POINT ( 'NONE',  ( 15.72974639402199770, -15.80617190586745480, 68.12390960531436690 ) ) ;
#77919=CARTESIAN_POINT ( 'NONE',  ( 10.72451020669871369, 18.67979575497193778, 57.08442372801901854 ) ) ;
#77920=CARTESIAN_POINT ( 'NONE',  ( 21.55341960407610458, 5.719274019375980345, 98.95724293864770971 ) ) ;
#77921=CARTESIAN_POINT ( 'NONE',  ( 21.53943276465977519, 0.05219959533937863772, 46.25109039468567573 ) ) ;
#77922=CARTESIAN_POINT ( 'NONE',  ( 9.474510206698971260, -16.51473224551069308, 77.91557627198103830 ) ) ;
#77923=CARTESIAN_POINT ( 'NONE',  ( 4.483927247898790824, -16.52544592524335698, 85.20942372801901854 ) ) ;
#77924=CARTESIAN_POINT ( 'NONE',  ( -0.05219959533909027116, -19.03943276465977164, 27.49890960531435624 ) ) ;
#77926=CARTESIAN_POINT ( 'NONE',  ( -12.06949235617756955, 12.14591786802309770, 60.62390960531437401 ) ) ;
#77927=CARTESIAN_POINT ( 'NONE',  ( 16.55341960407611168, 4.379528057220329451, 23.95724293864769550 ) ) ;
#77928=CARTESIAN_POINT ( 'NONE',  ( 13.89961937509977652, -13.97604488694527269, 63.12390960531435979 ) ) ;
#77929=CARTESIAN_POINT ( 'NONE',  ( 9.564922557960805705, 16.46253265017160317, 34.58224293864770260 ) ) ;
#77930=CARTESIAN_POINT ( 'NONE',  ( -15.72974639402197994, 15.80617190586746368, 45.62390960531436690 ) ) ;
#77931=CARTESIAN_POINT ( 'NONE',  ( -19.05341960407617563, 5.049401038297882671, 38.54275706135233293 ) ) ;
#77932=CARTESIAN_POINT ( 'NONE',  ( -17.44279575226822843, -5.990770900252486264, 39.16442432485683156 ) ) ;
#77933=CARTESIAN_POINT ( 'NONE',  ( 12.14591786802309770, 12.06949235617756955, 54.37390960531435979 ) ) ;
#77934=CARTESIAN_POINT ( 'NONE',  ( 10.72451020669898902, -18.67979575497178502, 32.91557627198102409 ) ) ;
#77936=CARTESIAN_POINT ( 'NONE',  ( 0.05219959533934541429, -16.53943276465976808, 70.00109039468568994 ) ) ;
#77937=CARTESIAN_POINT ( 'NONE',  ( 19.03943276465977164, 0.05219959533936151252, 76.25109039468566152 ) ) ;
#77938=CARTESIAN_POINT ( 'NONE',  ( -4.379528057220328563, 16.55341960407611168, 45.20724293864769550 ) ) ;
#77939=CARTESIAN_POINT ( 'NONE',  ( -19.25176906914648711, -5.499999999999851674, 75.99927264242275271 ) ) ;
#77940=CARTESIAN_POINT ( 'NONE',  ( 16.52544592524342804, -4.483927247898539470, 23.54057627198102765 ) ) ;
#77941=CARTESIAN_POINT ( 'NONE',  ( -19.03943276465977164, 0.05219959533909376836, 36.24890960531436690 ) ) ;
#77942=CARTESIAN_POINT ( 'NONE',  ( -16.51473224551069308, -9.474510206698971260, 56.66557627198103120 ) ) ;
#77943=CARTESIAN_POINT ( 'NONE',  ( -16.51473224551069308, -9.474510206698971260, 21.66557627198102765 ) ) ;
#77944=CARTESIAN_POINT ( 'NONE',  ( 5.823673210054444382, -21.52544592524334988, 30.20942372801902565 ) ) ;
#77945=CARTESIAN_POINT ( 'NONE',  ( -9.564922557960796823, -16.46253265017161027, 62.08224293864769550 ) ) ;
#77947=CARTESIAN_POINT ( 'NONE',  ( -19.05341960407611168, -5.049401038298163336, 41.45724293864769550 ) ) ;
#77948=CARTESIAN_POINT ( 'NONE',  ( -0.05219959533907301413, -21.53943276465977519, 37.49890960531436690 ) ) ;
#77949=CARTESIAN_POINT ( 'NONE',  ( 21.52544592524334988, 5.823673210054432836, 61.45942372801901854 ) ) ;
#77950=CARTESIAN_POINT ( 'NONE',  ( -13.97604488694527625, -13.89961937509977652, 21.87390960531435979 ) ) ;
#77951=CARTESIAN_POINT ( 'NONE',  ( -18.62759615963270932, 10.81492255796079327, 30.83224293864770260 ) ) ;
#77952=CARTESIAN_POINT ( 'NONE',  ( -16.55341960407617563, 4.379528057220093196, 88.54275706135236135 ) ) ;
#77953=CARTESIAN_POINT ( 'NONE',  ( 21.55341960407619695, -5.719274019375665929, 101.0427570613523756 ) ) ;
#77954=CARTESIAN_POINT ( 'NONE',  ( -8.224510206698735004, -14.34966873604973081, 69.58442372801900433 ) ) ;
#77955=CARTESIAN_POINT ( 'NONE',  ( 5.153800228976335163, 19.02544592524342804, 114.7905762719810241 ) ) ;
#77956=CARTESIAN_POINT ( 'NONE',  ( 16.53943276465976808, 0.05219959533934440121, 56.25109039468568284 ) ) ;
#77957=CARTESIAN_POINT ( 'NONE',  ( -16.52544592524335698, -4.483927247898792601, 38.95942372801901854 ) ) ;
#77958=CARTESIAN_POINT ( 'NONE',  ( 14.34966873604972726, -8.224510206698740333, 90.83442372801901854 ) ) ;
#77959=CARTESIAN_POINT ( 'NONE',  ( -18.67979575497193778, 10.72451020669871902, 53.33442372801901854 ) ) ;
#77960=CARTESIAN_POINT ( 'NONE',  ( 4.483927247898790824, -16.52544592524335698, 20.20942372801900788 ) ) ;
#77961=CARTESIAN_POINT ( 'NONE',  ( -21.52544592524343514, 5.823673210054127303, 106.0405762719810525 ) ) ;
#77962=CARTESIAN_POINT ( 'NONE',  ( 14.29746914071037800, 8.314922557961029526, 26.66775706135235424 ) ) ;
#77963=CARTESIAN_POINT ( 'NONE',  ( 8.224510206698742110, 14.34966873604972548, 92.08442372801901854 ) ) ;
#77965=CARTESIAN_POINT ( 'NONE',  ( -0.05219959533937732626, 21.53943276465977519, 92.50109039468567573 ) ) ;
#77966=CARTESIAN_POINT ( 'NONE',  ( 19.02544592524334988, 5.153800228976608722, 81.45942372801897591 ) ) ;
#77967=CARTESIAN_POINT ( 'NONE',  ( 16.55341960407611168, 4.379528057220329451, 63.95724293864770260 ) ) ;
#77968=CARTESIAN_POINT ( 'NONE',  ( 12.06949235617757843, -12.14591786802309237, 38.12390960531436690 ) ) ;
#77969=CARTESIAN_POINT ( 'NONE',  ( -12.06949235617756955, 12.14591786802309770, 110.6239096053143669 ) ) ;
#77970=CARTESIAN_POINT ( 'NONE',  ( 13.97604488694548053, -13.89961937509957401, 45.62609039468566863 ) ) ;
#77972=CARTESIAN_POINT ( 'NONE',  ( 5.823673210054444382, -21.52544592524334988, 50.20942372801901854 ) ) ;
#77973=CARTESIAN_POINT ( 'NONE',  ( 9.564922557961047289, -16.46253265017146816, 110.4177570613523471 ) ) ;
#77975=CARTESIAN_POINT ( 'NONE',  ( -16.46253265017160317, 9.564922557960807481, 100.8322429386477097 ) ) ;
#77976=CARTESIAN_POINT ( 'NONE',  ( -15.80617190586745835, -15.72974639402198527, 76.87390960531439532 ) ) ;
#77977=CARTESIAN_POINT ( 'NONE',  ( -9.564922557961040184, 16.46253265017147172, 92.91775706135233293 ) ) ;
#77978=CARTESIAN_POINT ( 'NONE',  ( -19.02544592524342804, 5.153800228976336051, 106.0405762719810241 ) ) ;
#77979=CARTESIAN_POINT ( 'NONE',  ( 0.05219959533907565091, 21.53943276465977519, 59.99890960531436690 ) ) ;
#77980=CARTESIAN_POINT ( 'NONE',  ( -8.224510206698948167, 14.34966873604960824, 105.4155762719810383 ) ) ;
#77981=CARTESIAN_POINT ( 'NONE',  ( -13.97604488694527625, -13.89961937509977652, 71.87390960531433848 ) ) ;
#77982=CARTESIAN_POINT ( 'NONE',  ( -13.89961937509977652, 13.97604488694528158, 35.62390960531435269 ) ) ;
#77983=CARTESIAN_POINT ( 'NONE',  ( 21.53943276465977519, 0.05219959533937863772, 36.25109039468567573 ) ) ;
#77984=CARTESIAN_POINT ( 'NONE',  ( 5.823673210054444382, -21.52544592524334988, 85.20942372801901854 ) ) ;
#77985=CARTESIAN_POINT ( 'NONE',  ( -16.52544592524335698, -4.483927247898792601, 83.95942372801900433 ) ) ;
#77986=CARTESIAN_POINT ( 'NONE',  ( 15.80617190586769283, -15.72974639402175789, 35.62609039468568994 ) ) ;
#77987=CARTESIAN_POINT ( 'NONE',  ( -18.67979575497193778, 10.72451020669871902, 38.33442372801900433 ) ) ;
#77988=CARTESIAN_POINT ( 'NONE',  ( 13.97604488694548053, -13.89961937509957401, 60.62609039468564731 ) ) ;
#77989=CARTESIAN_POINT ( 'NONE',  ( 9.564922557960805705, 16.46253265017160317, 79.58224293864769550 ) ) ;
#77990=CARTESIAN_POINT ( 'NONE',  ( 21.52544592524334988, 5.823673210054432836, 81.45942372801900433 ) ) ;
#77991=CARTESIAN_POINT ( 'NONE',  ( -18.62759615963270932, 10.81492255796079327, 85.83224293864768129 ) ) ;
#77992=CARTESIAN_POINT ( 'NONE',  ( 4.379528057220339221, -16.55341960407611168, 57.70724293864770260 ) ) ;
#77993=CARTESIAN_POINT ( 'NONE',  ( -18.67979575497193778, 10.72451020669871902, 108.3344237280190185 ) ) ;
#77994=CARTESIAN_POINT ( 'NONE',  ( 4.483927247898545687, 16.52544592524342804, 89.79057627198103830 ) ) ;
#77995=CARTESIAN_POINT ( 'NONE',  ( -19.05341960407611168, -5.049401038298163336, 41.45724293864769550 ) ) ;
#77996=CARTESIAN_POINT ( 'NONE',  ( 19.03943276465977164, 0.05219959533936151252, 66.25109039468567573 ) ) ;
#77997=CARTESIAN_POINT ( 'NONE',  ( -12.14591786802309592, -12.06949235617757132, 36.87390960531435979 ) ) ;
#77998=CARTESIAN_POINT ( 'NONE',  ( -5.719274019375665041, -21.55341960407619695, 89.79275706135236135 ) ) ;
#77999=CARTESIAN_POINT ( 'NONE',  ( 16.46253265017160672, -9.564922557960803928, 93.33224293864769550 ) ) ;
#78000=CARTESIAN_POINT ( 'NONE',  ( 19.02544592524334988, 5.153800228976608722, 61.45942372801900433 ) ) ;
#78001=CARTESIAN_POINT ( 'NONE',  ( -18.67979575497178146, -10.72451020669898902, 71.66557627198100988 ) ) ;
#78002=CARTESIAN_POINT ( 'NONE',  ( 0.05219959533937995610, -21.53943276465977519, 20.00109039468568639 ) ) ;
#78003=CARTESIAN_POINT ( 'NONE',  ( 13.89961937509957401, 13.97604488694547697, 106.8760903946856757 ) ) ;
#78004=CARTESIAN_POINT ( 'NONE',  ( -4.379528057220086978, -16.55341960407618274, 74.79275706135234714 ) ) ;
#78006=CARTESIAN_POINT ( 'NONE',  ( -10.81492255796105439, 18.62759615963255655, 27.91775706135234358 ) ) ;
#78007=CARTESIAN_POINT ( 'NONE',  ( -16.53943276465976808, 0.05219959533911058130, 106.2489096053143811 ) ) ;
#78009=CARTESIAN_POINT ( 'NONE',  ( -16.53943276465976808, -0.05219959533934237506, 43.75109039468568284 ) ) ;
#78010=CARTESIAN_POINT ( 'NONE',  ( -0.05219959533907301413, -21.53943276465977519, 57.49890960531435979 ) ) ;
#78011=CARTESIAN_POINT ( 'NONE',  ( -4.379528057220086978, -16.55341960407618274, 99.79275706135234714 ) ) ;
#78012=CARTESIAN_POINT ( 'NONE',  ( -12.06949235617739369, -12.14591786802326823, 39.37609039468567573 ) ) ;
#78013=CARTESIAN_POINT ( 'NONE',  ( -19.03943276465977164, 0.05219959533909376836, 51.24890960531436690 ) ) ;
#78014=CARTESIAN_POINT ( 'NONE',  ( -14.34966873604972548, 8.224510206698743886, 73.33442372801901854 ) ) ;
#78015=CARTESIAN_POINT ( 'NONE',  ( 9.474510206698729675, 16.51473224551082808, 67.08442372801900433 ) ) ;
#78016=CARTESIAN_POINT ( 'NONE',  ( -0.05219959533907301413, -21.53943276465977519, 67.49890960531436690 ) ) ;
#78017=CARTESIAN_POINT ( 'NONE',  ( -12.14591786802326823, 12.06949235617739902, 103.1260903946856757 ) ) ;
#78018=CARTESIAN_POINT ( 'NONE',  ( -5.823673210054431948, 21.52544592524334988, 87.70942372801901854 ) ) ;
#78019=CARTESIAN_POINT ( 'NONE',  ( -5.719274019375978568, 21.55341960407610458, 70.20724293864769550 ) ) ;
#78020=CARTESIAN_POINT ( 'NONE',  ( 21.55341960407610458, 5.719274019375980345, 53.95724293864770260 ) ) ;
#78021=VERTEX_POINT ( 'NONE', #136293 ) ;
#78022=CARTESIAN_POINT ( 'NONE',  ( -14.34966873604972548, 8.224510206698743886, 78.33442372801901854 ) ) ;
#78023=CARTESIAN_POINT ( 'NONE',  ( 21.52544592524344225, -5.823673210054117533, 48.54057627198103120 ) ) ;
#78024=ORIENTED_EDGE ( 'NONE', *, *, #62342, .T. ) ;
#78025=CARTESIAN_POINT ( 'NONE',  ( -15.80617190586745835, -15.72974639402198527, 21.87390960531436690 ) ) ;
#78027=CARTESIAN_POINT ( 'NONE',  ( -19.05341960407611168, -5.049401038298163336, 26.45724293864769550 ) ) ;
#78028=CARTESIAN_POINT ( 'NONE',  ( 10.72451020669898902, -18.67979575497178502, 72.91557627198103830 ) ) ;
#78029=CARTESIAN_POINT ( 'NONE',  ( -12.06949235617739369, -12.14591786802326823, 99.37609039468568994 ) ) ;
#78030=CARTESIAN_POINT ( 'NONE',  ( -18.67979575497193778, 10.72451020669871902, 43.33442372801901143 ) ) ;
#78031=CARTESIAN_POINT ( 'NONE',  ( -9.474510206698720793, -16.51473224551083518, 104.5844237280190043 ) ) ;
#78032=CARTESIAN_POINT ( 'NONE',  ( 16.55341960407611168, 4.379528057220329451, 113.9572429386477239 ) ) ;
#78033=CARTESIAN_POINT ( 'NONE',  ( 9.564922557961047289, -16.46253265017146816, 105.4177570613523471 ) ) ;
#78034=CARTESIAN_POINT ( 'NONE',  ( -16.51473224551069308, -9.474510206698971260, 36.66557627198102409 ) ) ;
#78036=CARTESIAN_POINT ( 'NONE',  ( 16.51473224551069308, 9.474510206698969483, 94.16557627198103830 ) ) ;
#78037=CARTESIAN_POINT ( 'NONE',  ( -4.379528057220086978, -16.55341960407618274, 69.79275706135234714 ) ) ;
#78038=CARTESIAN_POINT ( 'NONE',  ( -16.46253265017146816, -9.564922557961047289, 74.16775706135234714 ) ) ;
#78039=CARTESIAN_POINT ( 'NONE',  ( 13.89961937509957401, 13.97604488694547697, 21.87609039468566152 ) ) ;
#78040=CARTESIAN_POINT ( 'NONE',  ( 15.72974639402199770, -15.80617190586745480, 68.12390960531436690 ) ) ;
#78041=CARTESIAN_POINT ( 'NONE',  ( -0.05219959533934338120, 16.53943276465976808, 82.50109039468568994 ) ) ;
#78042=CARTESIAN_POINT ( 'NONE',  ( 13.89961937509957401, 13.97604488694547697, 81.87609039468564731 ) ) ;
#78043=CARTESIAN_POINT ( 'NONE',  ( 19.05341960407611168, 5.049401038298154454, 33.95724293864769550 ) ) ;
#78044=CARTESIAN_POINT ( 'NONE',  ( 9.474510206698971260, -16.51473224551069308, 92.91557627198103830 ) ) ;
#78045=CARTESIAN_POINT ( 'NONE',  ( 21.53943276465977519, 0.05219959533937863772, 46.25109039468567573 ) ) ;
#78046=CARTESIAN_POINT ( 'NONE',  ( -19.02544592524342804, 5.153800228976336051, 41.04057627198103120 ) ) ;
#78048=CARTESIAN_POINT ( 'NONE',  ( -19.02544592524342804, 5.153800228976336051, 106.0405762719810241 ) ) ;
#78049=CARTESIAN_POINT ( 'NONE',  ( 16.55341960407611168, 4.379528057220329451, 58.95724293864770971 ) ) ;
#78050=CARTESIAN_POINT ( 'NONE',  ( -15.80617190586745835, -15.72974639402198527, 56.87390960531436690 ) ) ;
#78052=CARTESIAN_POINT ( 'NONE',  ( -0.05219959533936034679, 19.03943276465977164, 47.50109039468566863 ) ) ;
#78053=CARTESIAN_POINT ( 'NONE',  ( -19.03943276465977164, 0.05219959533909376836, 61.24890960531436690 ) ) ;
#78054=CARTESIAN_POINT ( 'NONE',  ( 9.564922557960805705, 16.46253265017160317, 69.58224293864770971 ) ) ;
#78056=CARTESIAN_POINT ( 'NONE',  ( 16.52544592524335698, 4.483927247898782831, 56.45942372801902565 ) ) ;
#78057=CARTESIAN_POINT ( 'NONE',  ( -17.97214573761831247, -5.500000000000092371, 66.46970049038654338 ) ) ;
#78059=CARTESIAN_POINT ( 'NONE',  ( -12.06949235617739369, -12.14591786802326823, 94.37609039468568994 ) ) ;
#78061=CARTESIAN_POINT ( 'NONE',  ( 16.55341960407618274, -4.379528057220086978, 86.04275706135236135 ) ) ;
#78062=CARTESIAN_POINT ( 'NONE',  ( -16.53943276465976808, -0.05219959533934237506, 53.75109039468568994 ) ) ;
#78063=CARTESIAN_POINT ( 'NONE',  ( -19.05341960407617563, 5.049401038297882671, 28.54275706135232937 ) ) ;
#78064=CARTESIAN_POINT ( 'NONE',  ( 19.05341960407611168, 5.049401038298154454, 48.95724293864768129 ) ) ;
#78066=CARTESIAN_POINT ( 'NONE',  ( 5.719274019375673035, 21.55341960407619339, 52.29275706135236135 ) ) ;
#78067=CARTESIAN_POINT ( 'NONE',  ( 9.474510206698729675, 16.51473224551082808, 57.08442372801900433 ) ) ;
#78068=CARTESIAN_POINT ( 'NONE',  ( -13.89961937509957401, -13.97604488694547875, 19.37609039468566507 ) ) ;
#78069=CARTESIAN_POINT ( 'NONE',  ( 0.05219959533909260263, 19.03943276465977164, 24.99890960531435269 ) ) ;
#78071=CARTESIAN_POINT ( 'NONE',  ( 10.81492255796078972, 18.62759615963270932, 69.58224293864769550 ) ) ;
#78072=CARTESIAN_POINT ( 'NONE',  ( -15.80617190586745835, -15.72974639402198527, 21.87390960531436690 ) ) ;
#78073=CARTESIAN_POINT ( 'NONE',  ( -4.483927247898539470, -16.52544592524342804, 112.2905762719810241 ) ) ;
#78074=CARTESIAN_POINT ( 'NONE',  ( -16.52544592524335698, -4.483927247898792601, 33.95942372801901143 ) ) ;
#78075=CARTESIAN_POINT ( 'NONE',  ( -14.34966873604960291, -8.224510206698953496, 31.66557627198102054 ) ) ;
#78077=B_SPLINE_CURVE_WITH_KNOTS ( 'NONE', 3,
 ( #173405, #98520, #83357, #188577, #130867, #53022, #82350, #176396, #111719, #114703, #191545, #99529, #128858, #34876, #129846, #113689, #37870, #142047, #160213, #189571, #51043, #112705, #21703, #161211, #174397, #22706, #192557, #7514, #69199, #115714, #95547, #35867 ),
 .UNSPECIFIED., .F., .F.,
 ( 4, 2, 2, 2, 2, 2, 2, 2, 2, 2, 2, 2, 2, 2, 2, 4 ),
 ( 1.346507514538369135E-17, 0.0003712461730036979452, 0.0007424923460073824463, 0.001113738519011066947, 0.001484984692014751449, 0.002227477038022120451, 0.002598723211025787388, 0.002969969384029454759, 0.003341215557033121696, 0.003712461730036789500, 0.004083707903040457304, 0.004454954076044123808, 0.004826200249047792046, 0.005197446422051459416, 0.005568692595055126787, 0.005939938768058793291 ),
 .UNSPECIFIED. ) ;
#78078=CARTESIAN_POINT ( 'NONE',  ( -21.52544592524343514, 5.823673210054127303, 111.0405762719810525 ) ) ;
#78079=CARTESIAN_POINT ( 'NONE',  ( 8.314922557960818139, 14.29746914071049879, 39.58224293864769550 ) ) ;
#78082=CARTESIAN_POINT ( 'NONE',  ( -9.564922557961040184, 16.46253265017147172, 112.9177570613523329 ) ) ;
#78083=CARTESIAN_POINT ( 'NONE',  ( 13.97604488694548053, -13.89961937509957401, 25.62609039468566507 ) ) ;
#78084=CARTESIAN_POINT ( 'NONE',  ( -14.29746914071049879, 8.314922557960819915, 50.83224293864770971 ) ) ;
#78085=CARTESIAN_POINT ( 'NONE',  ( 0.05219959533907565091, 21.53943276465977519, 104.9989096053143669 ) ) ;
#78086=CARTESIAN_POINT ( 'NONE',  ( 16.88567814943164436, 6.947325034625594142, 33.79001122652586986 ) ) ;
#78087=CARTESIAN_POINT ( 'NONE',  ( -10.81492255796078084, -18.62759615963271287, 62.08224293864769550 ) ) ;
#78088=CARTESIAN_POINT ( 'NONE',  ( -16.46253265017160317, 9.564922557960807481, 80.83224293864769550 ) ) ;
#78089=CARTESIAN_POINT ( 'NONE',  ( -4.483927247898539470, -16.52544592524342804, 42.29057627198103120 ) ) ;
#78090=CARTESIAN_POINT ( 'NONE',  ( -9.474510206698964154, 16.51473224551069663, 85.41557627198102409 ) ) ;
#78092=CARTESIAN_POINT ( 'NONE',  ( 19.05341960407617918, -5.049401038297876454, 51.04275706135231871 ) ) ;
#78093=CARTESIAN_POINT ( 'NONE',  ( -15.72974639402197994, 15.80617190586746368, 95.62390960531436690 ) ) ;
#78094=CARTESIAN_POINT ( 'NONE',  ( -4.483927247898539470, -16.52544592524342804, 97.29057627198105251 ) ) ;
#78095=CARTESIAN_POINT ( 'NONE',  ( 15.80617190586769283, -15.72974639402175789, 45.62609039468567573 ) ) ;
#78097=CARTESIAN_POINT ( 'NONE',  ( 16.52544592524342804, -4.483927247898539470, 33.54057627198102409 ) ) ;
#78098=CARTESIAN_POINT ( 'NONE',  ( -9.564922557960796823, -16.46253265017161027, 37.08224293864768839 ) ) ;
#78099=CARTESIAN_POINT ( 'NONE',  ( -19.03943276465977164, 0.05219959533909376836, 101.2489096053143669 ) ) ;
#78100=CARTESIAN_POINT ( 'NONE',  ( -18.67979575497178146, -10.72451020669898902, 61.66557627198103120 ) ) ;
#78102=CARTESIAN_POINT ( 'NONE',  ( 19.05341960407611168, 5.049401038298154454, 33.95724293864769550 ) ) ;
#78103=CARTESIAN_POINT ( 'NONE',  ( 18.67979575497178502, 10.72451020669898547, 49.16557627198102409 ) ) ;
#78104=CARTESIAN_POINT ( 'NONE',  ( -21.55341960407619339, 5.719274019375674811, 73.54275706135234714 ) ) ;
#78106=CARTESIAN_POINT ( 'NONE',  ( 16.55341960407618274, -4.379528057220086978, 71.04275706135234714 ) ) ;
#78107=CARTESIAN_POINT ( 'NONE',  ( 19.03943276465977164, -0.05219959533909143690, 53.74890960531436690 ) ) ;
#78108=CARTESIAN_POINT ( 'NONE',  ( 16.51473224551069308, 9.474510206698969483, 64.16557627198102409 ) ) ;
#78110=CARTESIAN_POINT ( 'NONE',  ( 9.474510206698729675, 16.51473224551082808, 22.08442372801899722 ) ) ;
#78111=CARTESIAN_POINT ( 'NONE',  ( 4.483927247898790824, -16.52544592524335698, 80.20942372801901854 ) ) ;
#78112=CARTESIAN_POINT ( 'NONE',  ( 15.72974639402176855, 15.80617190586768217, 96.87609039468568994 ) ) ;
#78113=CARTESIAN_POINT ( 'NONE',  ( -13.97604488694527625, -13.89961937509977652, 81.87390960531436690 ) ) ;
#78114=CARTESIAN_POINT ( 'NONE',  ( -5.719274019375978568, 21.55341960407610458, 30.20724293864769550 ) ) ;
#78115=CARTESIAN_POINT ( 'NONE',  ( 19.02544592524334988, 5.153800228976608722, 106.4594237280190185 ) ) ;
#78116=CARTESIAN_POINT ( 'NONE',  ( -15.80617190586768217, 15.72974639402176855, 78.12609039468570415 ) ) ;
#78117=CARTESIAN_POINT ( 'NONE',  ( -8.314922557961024197, 14.29746914071037800, 52.91775706135235424 ) ) ;
#78118=CARTESIAN_POINT ( 'NONE',  ( 5.823673210054125526, 21.52544592524343514, 94.79057627198105251 ) ) ;
#78119=CARTESIAN_POINT ( 'NONE',  ( -8.224510206698735004, -14.34966873604973081, 19.58442372801901143 ) ) ;
#78120=CARTESIAN_POINT ( 'NONE',  ( -19.05341960407611168, -5.049401038298163336, 81.45724293864769550 ) ) ;
#78121=CARTESIAN_POINT ( 'NONE',  ( -16.52544592524335698, -4.483927247898792601, 23.95942372801901143 ) ) ;
#78122=CARTESIAN_POINT ( 'NONE',  ( -19.03943276465977164, 0.05219959533909376836, 36.24890960531436690 ) ) ;
#78123=CARTESIAN_POINT ( 'NONE',  ( -5.049401038297874678, -19.05341960407617918, 109.7927570613523187 ) ) ;
#78124=CARTESIAN_POINT ( 'NONE',  ( -16.53943276465976808, 0.05219959533911058130, 71.24890960531435269 ) ) ;
#78125=CARTESIAN_POINT ( 'NONE',  ( 14.29746914071037800, 8.314922557961029526, 71.66775706135234714 ) ) ;
#78127=CARTESIAN_POINT ( 'NONE',  ( -5.719274019375665041, -21.55341960407619695, 34.79275706135235424 ) ) ;
#78128=CARTESIAN_POINT ( 'NONE',  ( 16.46253265017160672, -9.564922557960803928, 53.33224293864768839 ) ) ;
#78129=CARTESIAN_POINT ( 'NONE',  ( -19.03943276465977164, 0.05219959533909376836, 71.24890960531435269 ) ) ;
#78130=CARTESIAN_POINT ( 'NONE',  ( 16.52544592524335698, 4.483927247898782831, 71.45942372801901854 ) ) ;
#78133=VERTEX_POINT ( 'NONE', #49254 ) ;
#78134=CARTESIAN_POINT ( 'NONE',  ( -15.80617190586768217, 15.72974639402176855, 113.1260903946856899 ) ) ;
#78135=CARTESIAN_POINT ( 'NONE',  ( -16.51473224551069308, -9.474510206698971260, 36.66557627198102409 ) ) ;
#78136=CARTESIAN_POINT ( 'NONE',  ( -19.02544592524342804, 5.153800228976336051, 116.0405762719810383 ) ) ;
#78138=CARTESIAN_POINT ( 'NONE',  ( -4.483927247898782831, 16.52544592524335698, 27.70942372801901854 ) ) ;
#78139=CARTESIAN_POINT ( 'NONE',  ( 13.97604488694548053, -13.89961937509957401, 60.62609039468564731 ) ) ;
#78140=CARTESIAN_POINT ( 'NONE',  ( 0.05219959533934541429, -16.53943276465976808, 40.00109039468567573 ) ) ;
#78141=CARTESIAN_POINT ( 'NONE',  ( -5.153800228976328057, -19.02544592524343514, 42.29057627198101699 ) ) ;
#78142=CARTESIAN_POINT ( 'NONE',  ( 5.049401038298161559, -19.05341960407611168, 112.7072429386476813 ) ) ;
#78143=CARTESIAN_POINT ( 'NONE',  ( -9.474510206698964154, 16.51473224551069663, 60.41557627198102409 ) ) ;
#78144=CARTESIAN_POINT ( 'NONE',  ( -10.81492255796078084, -18.62759615963271287, 102.0822429386476955 ) ) ;
#78145=CARTESIAN_POINT ( 'NONE',  ( 19.02544592524343514, -5.153800228976328945, 93.54057627198102409 ) ) ;
#78146=CARTESIAN_POINT ( 'NONE',  ( 9.474510206698971260, -16.51473224551069308, 27.91557627198103120 ) ) ;
#78147=CARTESIAN_POINT ( 'NONE',  ( 5.153800228976335163, 19.02544592524342804, 59.79057627198100988 ) ) ;
#78148=CARTESIAN_POINT ( 'NONE',  ( -8.314922557960811034, -14.29746914071050412, 22.08224293864769194 ) ) ;
#78150=CARTESIAN_POINT ( 'NONE',  ( -5.153800228976607833, 19.02544592524334988, 97.70942372801900433 ) ) ;
#78151=CARTESIAN_POINT ( 'NONE',  ( 13.97604488694548053, -13.89961937509957401, 30.62609039468566863 ) ) ;
#78152=CARTESIAN_POINT ( 'NONE',  ( -14.29746914071049879, 8.314922557960819915, 55.83224293864770260 ) ) ;
#78153=CARTESIAN_POINT ( 'NONE',  ( 5.719274019375673035, 21.55341960407619339, 97.29275706135234714 ) ) ;
#78154=CARTESIAN_POINT ( 'NONE',  ( -13.97604488694527625, -13.89961937509977652, 41.87390960531435979 ) ) ;
#78155=CARTESIAN_POINT ( 'NONE',  ( 12.14591786802309770, 12.06949235617756955, 29.37390960531435269 ) ) ;
#78156=CARTESIAN_POINT ( 'NONE',  ( 5.823673210054444382, -21.52544592524334988, 85.20942372801901854 ) ) ;
#78157=CARTESIAN_POINT ( 'NONE',  ( -16.51473224551069308, -9.474510206698971260, 76.66557627198103830 ) ) ;
#78158=CARTESIAN_POINT ( 'NONE',  ( 0.05219959533909260263, 19.03943276465977164, 94.99890960531436690 ) ) ;
#78159=CARTESIAN_POINT ( 'NONE',  ( 12.06949235617757843, -12.14591786802309237, 93.12390960531436690 ) ) ;
#78160=CARTESIAN_POINT ( 'NONE',  ( 14.29746914071049879, -8.314922557960816363, 73.33224293864769550 ) ) ;
#78161=CARTESIAN_POINT ( 'NONE',  ( -5.719274019375978568, 21.55341960407610458, 85.20724293864770971 ) ) ;
#78162=CARTESIAN_POINT ( 'NONE',  ( -13.89961937509977652, 13.97604488694528158, 80.62390960531436690 ) ) ;
#78163=CARTESIAN_POINT ( 'NONE',  ( -21.53943276465977519, 0.05219959533907696930, 81.24890960531436690 ) ) ;
#78164=CARTESIAN_POINT ( 'NONE',  ( 13.97604488694548053, -13.89961937509957401, 75.62609039468564731 ) ) ;
#78166=CARTESIAN_POINT ( 'NONE',  ( -4.483927247898539470, -16.52544592524342804, 92.29057627198103830 ) ) ;
#78167=CARTESIAN_POINT ( 'NONE',  ( 0.05219959533909260263, 19.03943276465977164, 54.99890960531435979 ) ) ;
#78168=CARTESIAN_POINT ( 'NONE',  ( 18.62759615963271287, -10.81492255796078972, 63.33224293864770260 ) ) ;
#78170=CARTESIAN_POINT ( 'NONE',  ( -8.224510206698948167, 14.34966873604960824, 25.41557627198103120 ) ) ;
#78171=CARTESIAN_POINT ( 'NONE',  ( -16.53943276465976808, -0.05219959533934237506, 18.75109039468568639 ) ) ;
#78172=CARTESIAN_POINT ( 'NONE',  ( -14.34966873604960291, -8.224510206698953496, 86.66557627198102409 ) ) ;
#78174=CARTESIAN_POINT ( 'NONE',  ( 5.049401038298161559, -19.05341960407611168, 72.70724293864768129 ) ) ;
#78175=CARTESIAN_POINT ( 'NONE',  ( -19.02544592524342804, 5.153800228976336051, 31.04057627198102409 ) ) ;
#78176=CARTESIAN_POINT ( 'NONE',  ( 8.314922557960818139, 14.29746914071049879, 64.58224293864769550 ) ) ;
#78177=CARTESIAN_POINT ( 'NONE',  ( -16.46253265017160317, 9.564922557960807481, 105.8322429386476955 ) ) ;
#78178=CARTESIAN_POINT ( 'NONE',  ( -9.474510206698720793, -16.51473224551083518, 84.58442372801900433 ) ) ;
#78179=CARTESIAN_POINT ( 'NONE',  ( 19.03943276465977164, -0.05219959533909143690, 83.74890960531436690 ) ) ;
#78180=CARTESIAN_POINT ( 'NONE',  ( -16.51473224551069308, -9.474510206698971260, 86.66557627198102409 ) ) ;
#78181=CARTESIAN_POINT ( 'NONE',  ( -5.719274019375978568, 21.55341960407610458, 80.20724293864769550 ) ) ;
#78182=CARTESIAN_POINT ( 'NONE',  ( 14.34966873604972726, -8.224510206698740333, 70.83442372801901854 ) ) ;
#78183=CARTESIAN_POINT ( 'NONE',  ( -19.05341960407617918, 5.049401038297883559, 113.5427570613523329 ) ) ;
#78184=CARTESIAN_POINT ( 'NONE',  ( -13.89961937509977652, 13.97604488694528158, 65.62390960531436690 ) ) ;
#78185=CARTESIAN_POINT ( 'NONE',  ( 5.719274019375991003, -21.55341960407610458, 67.70724293864769550 ) ) ;
#78186=CARTESIAN_POINT ( 'NONE',  ( 5.153800228976615827, -19.02544592524334988, 90.20942372801900433 ) ) ;
#78187=CARTESIAN_POINT ( 'NONE',  ( -4.483927247898539470, -16.52544592524342804, 32.29057627198102409 ) ) ;
#78188=CARTESIAN_POINT ( 'NONE',  ( 0.05219959533937995610, -21.53943276465977519, 40.00109039468567573 ) ) ;
#78190=CARTESIAN_POINT ( 'NONE',  ( -8.224510206698735004, -14.34966873604973081, 79.58442372801903275 ) ) ;
#78191=CARTESIAN_POINT ( 'NONE',  ( -13.97604488694527625, -13.89961937509977652, 101.8739096053143811 ) ) ;
#78193=DIRECTION ( 'NONE',  ( 0.000000000000000000, 0.04175967627138096189, 0.9991276842514722478 ) ) ;
#78194=CARTESIAN_POINT ( 'NONE',  ( 12.14591786802327356, -12.06949235617739191, 100.6260903946857184 ) ) ;
#78195=CARTESIAN_POINT ( 'NONE',  ( -0.05219959533934338120, 16.53943276465976808, 42.50109039468567573 ) ) ;
#78196=CARTESIAN_POINT ( 'NONE',  ( -9.564922557960796823, -16.46253265017161027, 57.08224293864769550 ) ) ;
#78197=CARTESIAN_POINT ( 'NONE',  ( -16.51473224551069308, -9.474510206698971260, 66.66557627198102409 ) ) ;
#78198=CARTESIAN_POINT ( 'NONE',  ( -18.62759615963255300, -10.81492255796106328, 49.16775706135234003 ) ) ;
#78199=CARTESIAN_POINT ( 'NONE',  ( -14.29746914071037622, -8.314922557961029526, 64.16775706135234714 ) ) ;
#78200=CARTESIAN_POINT ( 'NONE',  ( 12.14591786802309770, 12.06949235617756955, 39.37390960531436690 ) ) ;
#78201=CARTESIAN_POINT ( 'NONE',  ( -5.153800228976328057, -19.02544592524343514, 47.29057627198102409 ) ) ;
#78202=CARTESIAN_POINT ( 'NONE',  ( -19.03943276465977164, 0.05219959533909376836, 41.24890960531435269 ) ) ;
#78203=CARTESIAN_POINT ( 'NONE',  ( 16.53943276465976808, 0.05219959533934440121, 31.25109039468568639 ) ) ;
#78204=CARTESIAN_POINT ( 'NONE',  ( -0.05219959533936034679, 19.03943276465977164, 77.50109039468566152 ) ) ;
#78205=CARTESIAN_POINT ( 'NONE',  ( -16.53943276465976808, 0.05219959533911058130, 86.24890960531436690 ) ) ;
#78206=CARTESIAN_POINT ( 'NONE',  ( -16.51473224551069308, -9.474510206698971260, 56.66557627198103120 ) ) ;
#78207=CARTESIAN_POINT ( 'NONE',  ( 19.03943276465977164, 0.05219959533936151252, 86.25109039468567573 ) ) ;
#78209=CARTESIAN_POINT ( 'NONE',  ( -18.62759615963255300, -10.81492255796106328, 84.16775706135234714 ) ) ;
#78210=CARTESIAN_POINT ( 'NONE',  ( 12.14591786802327356, -12.06949235617739191, 55.62609039468568284 ) ) ;
#78211=CARTESIAN_POINT ( 'NONE',  ( -17.49999999999997158, 3.305555262949582129, 24.62517152156607736 ) ) ;
#78212=CARTESIAN_POINT ( 'NONE',  ( 21.55341960407610458, 5.719274019375980345, 53.95724293864770260 ) ) ;
#78213=CARTESIAN_POINT ( 'NONE',  ( 8.224510206698742110, 14.34966873604972548, 37.08442372801901143 ) ) ;
#78214=CARTESIAN_POINT ( 'NONE',  ( -17.49999999999999645, -5.500000000000000888, 22.00000000000000711 ) ) ;
#78215=CARTESIAN_POINT ( 'NONE',  ( -16.46253265017146816, -9.564922557961047289, 34.16775706135233293 ) ) ;
#78216=CARTESIAN_POINT ( 'NONE',  ( 16.51473224551069308, 9.474510206698969483, 74.16557627198103830 ) ) ;
#78217=CARTESIAN_POINT ( 'NONE',  ( -0.05219959533909027116, -19.03943276465977164, 57.49890960531435979 ) ) ;
#78219=CARTESIAN_POINT ( 'NONE',  ( -16.46253265017160317, 9.564922557960807481, 70.83224293864770971 ) ) ;
#78220=CARTESIAN_POINT ( 'NONE',  ( 17.50000000000000000, -5.076555817581248853, 111.3204850795022480 ) ) ;
#78221=CARTESIAN_POINT ( 'NONE',  ( -19.05341960407617563, 5.049401038297882671, 28.54275706135232937 ) ) ;
#78222=CARTESIAN_POINT ( 'NONE',  ( -21.53943276465977519, -0.05219959533937600094, 103.7510903946857042 ) ) ;
#78223=CARTESIAN_POINT ( 'NONE',  ( 16.53943276465976808, -0.05219959533910856209, 33.74890960531436690 ) ) ;
#78224=CARTESIAN_POINT ( 'NONE',  ( 5.153800228976335163, 19.02544592524342804, 49.79057627198100988 ) ) ;
#78225=CARTESIAN_POINT ( 'NONE',  ( 19.05341960407611168, 5.049401038298154454, 108.9572429386477097 ) ) ;
#78226=CARTESIAN_POINT ( 'NONE',  ( -21.55341960407619339, 5.719274019375674811, 83.54275706135234714 ) ) ;
#78227=CARTESIAN_POINT ( 'NONE',  ( 19.03943276465977164, -0.05219959533909143690, 48.74890960531435979 ) ) ;
#78229=CARTESIAN_POINT ( 'NONE',  ( 21.55341960407619695, -5.719274019375665929, 76.04275706135237556 ) ) ;
#78230=CARTESIAN_POINT ( 'NONE',  ( -10.81492255796078084, -18.62759615963271287, 22.08224293864769194 ) ) ;
#78231=CARTESIAN_POINT ( 'NONE',  ( 21.53943276465977519, 0.05219959533937863772, 26.25109039468567573 ) ) ;
#78232=CARTESIAN_POINT ( 'NONE',  ( 19.02544592524334988, 5.153800228976608722, 51.45942372801900433 ) ) ;
#78233=CARTESIAN_POINT ( 'NONE',  ( 19.05341960407611168, 5.049401038298154454, 33.95724293864769550 ) ) ;
#78234=CARTESIAN_POINT ( 'NONE',  ( -19.02544592524342804, 5.153800228976336051, 81.04057627198103830 ) ) ;
#78235=CARTESIAN_POINT ( 'NONE',  ( 5.153800228976615827, -19.02544592524334988, 110.2094237280189901 ) ) ;
#78236=CARTESIAN_POINT ( 'NONE',  ( 8.314922557960818139, 14.29746914071049879, 69.58224293864769550 ) ) ;
#78237=CARTESIAN_POINT ( 'NONE',  ( 21.52544592524344225, -5.823673210054117533, 38.54057627198103120 ) ) ;
#78238=CARTESIAN_POINT ( 'NONE',  ( 0.05219959533936267826, -19.03943276465977164, 95.00109039468567573 ) ) ;
#78239=CARTESIAN_POINT ( 'NONE',  ( 21.55341960407610458, 5.719274019375980345, 98.95724293864770971 ) ) ;
#78240=CARTESIAN_POINT ( 'NONE',  ( -21.53943276465977519, -0.05219959533937600094, 63.75109039468568284 ) ) ;
#78241=CARTESIAN_POINT ( 'NONE',  ( 12.14591786802327356, -12.06949235617739191, 55.62609039468568284 ) ) ;
#78242=CARTESIAN_POINT ( 'NONE',  ( -12.06949235617739369, -12.14591786802326823, 59.37609039468568284 ) ) ;
#78243=CARTESIAN_POINT ( 'NONE',  ( 19.05341960407611168, 5.049401038298154454, 43.95724293864769550 ) ) ;
#78244=CARTESIAN_POINT ( 'NONE',  ( 14.34966873604972726, -8.224510206698740333, 85.83442372801901854 ) ) ;
#78245=CARTESIAN_POINT ( 'NONE',  ( 18.67979575497178502, 10.72451020669898547, 114.1655762719810383 ) ) ;
#78246=CARTESIAN_POINT ( 'NONE',  ( 16.53943276465976808, -0.05219959533910856209, 53.74890960531437401 ) ) ;
#78247=CARTESIAN_POINT ( 'NONE',  ( -19.03943276465977164, 0.05219959533909376836, 86.24890960531436690 ) ) ;
#78248=CARTESIAN_POINT ( 'NONE',  ( -0.05219959533934338120, 16.53943276465976808, 77.50109039468567573 ) ) ;
#78249=CARTESIAN_POINT ( 'NONE',  ( -0.05219959533937732626, 21.53943276465977519, 62.50109039468568284 ) ) ;
#78250=CARTESIAN_POINT ( 'NONE',  ( -16.46253265017146816, -9.564922557961047289, 109.1677570613523471 ) ) ;
#78251=CARTESIAN_POINT ( 'NONE',  ( 5.719274019375991003, -21.55341960407610458, 112.7072429386476955 ) ) ;
#78252=CARTESIAN_POINT ( 'NONE',  ( -16.55341960407611168, -4.379528057220339221, 46.45724293864769550 ) ) ;
#78253=VERTEX_POINT ( 'NONE', #13936 ) ;
#78254=CARTESIAN_POINT ( 'NONE',  ( -16.38665767535054130, 7.295008042176037044, 75.26400864214548392 ) ) ;
#78255=CARTESIAN_POINT ( 'NONE',  ( 10.81492255796078972, 18.62759615963270932, 84.58224293864769550 ) ) ;
#78256=CARTESIAN_POINT ( 'NONE',  ( -16.53943276465976808, 0.05219959533911058130, 31.24890960531435979 ) ) ;
#78257=EDGE_LOOP ( 'NONE', ( #21422, #82768, #175288, #139458 ) ) ;
#78259=CARTESIAN_POINT ( 'NONE',  ( -21.55341960407619339, 5.719274019375674811, 23.54275706135235424 ) ) ;
#78260=CARTESIAN_POINT ( 'NONE',  ( 19.05341960407611168, 5.049401038298154454, 113.9572429386477097 ) ) ;
#78261=CARTESIAN_POINT ( 'NONE',  ( 15.72974639402176855, 15.80617190586768217, 21.87609039468567573 ) ) ;
#78262=CARTESIAN_POINT ( 'NONE',  ( -8.224510206698948167, 14.34966873604960824, 55.41557627198102409 ) ) ;
#78264=CARTESIAN_POINT ( 'NONE',  ( -16.53943276465976808, -0.05219959533934237506, 63.75109039468568284 ) ) ;
#78265=CARTESIAN_POINT ( 'NONE',  ( -13.97604488694527625, -13.89961937509977652, 56.87390960531434558 ) ) ;
#78266=CARTESIAN_POINT ( 'NONE',  ( 19.05341960407617918, -5.049401038297876454, 66.04275706135233293 ) ) ;
#78267=CARTESIAN_POINT ( 'NONE',  ( 9.564922557960805705, 16.46253265017160317, 84.58224293864769550 ) ) ;
#78268=CARTESIAN_POINT ( 'NONE',  ( 15.72974639402199770, -15.80617190586745480, 38.12390960531436690 ) ) ;
#78270=CARTESIAN_POINT ( 'NONE',  ( 0.05219959533909260263, 19.03943276465977164, 54.99890960531435979 ) ) ;
#78271=CARTESIAN_POINT ( 'NONE',  ( 8.314922557961029526, -14.29746914071037800, 25.41775706135235779 ) ) ;
#78272=CARTESIAN_POINT ( 'NONE',  ( -0.05219959533936034679, 19.03943276465977164, 67.50109039468566152 ) ) ;
#78273=CARTESIAN_POINT ( 'NONE',  ( 21.55341960407610458, 5.719274019375980345, 98.95724293864770971 ) ) ;
#78274=CARTESIAN_POINT ( 'NONE',  ( 16.55341960407611168, 4.379528057220329451, 38.95724293864768839 ) ) ;
#78275=CARTESIAN_POINT ( 'NONE',  ( 19.02544592524343514, -5.153800228976328945, 93.54057627198102409 ) ) ;
#78276=CARTESIAN_POINT ( 'NONE',  ( -18.62759615963270932, 10.81492255796079327, 55.83224293864770260 ) ) ;
#78277=CARTESIAN_POINT ( 'NONE',  ( -21.52544592524343514, 5.823673210054127303, 91.04057627198103830 ) ) ;
#78278=CARTESIAN_POINT ( 'NONE',  ( 12.14591786802327356, -12.06949235617739191, 40.62609039468567573 ) ) ;
#78279=CARTESIAN_POINT ( 'NONE',  ( -15.80617190586745835, -15.72974639402198527, 41.87390960531435979 ) ) ;
#78280=CARTESIAN_POINT ( 'NONE',  ( -5.719274019375665041, -21.55341960407619695, 89.79275706135236135 ) ) ;
#78281=CARTESIAN_POINT ( 'NONE',  ( -13.89961937509977652, 13.97604488694528158, 90.62390960531432427 ) ) ;
#78282=CARTESIAN_POINT ( 'NONE',  ( 5.049401038298161559, -19.05341960407611168, 27.70724293864769550 ) ) ;
#78283=CARTESIAN_POINT ( 'NONE',  ( -19.02544592524342804, 5.153800228976336051, 86.04057627198103830 ) ) ;
#78284=CARTESIAN_POINT ( 'NONE',  ( 16.55341960407611168, 4.379528057220329451, 108.9572429386476955 ) ) ;
#78285=CARTESIAN_POINT ( 'NONE',  ( -13.97604488694527625, -13.89961937509977652, 66.87390960531436690 ) ) ;
#78286=CARTESIAN_POINT ( 'NONE',  ( -4.379528057220086978, -16.55341960407618274, 19.79275706135235069 ) ) ;
#78287=CARTESIAN_POINT ( 'NONE',  ( 16.46253265017146816, 9.564922557961045513, 41.66775706135234003 ) ) ;
#78288=CARTESIAN_POINT ( 'NONE',  ( -10.72451020669870658, -18.67979575497194134, 94.58442372801901854 ) ) ;
#78289=CARTESIAN_POINT ( 'NONE',  ( 16.46253265017160672, -9.564922557960803928, 108.3322429386476955 ) ) ;
#78290=CARTESIAN_POINT ( 'NONE',  ( -8.314922557961024197, 14.29746914071037800, 87.91775706135234714 ) ) ;
#78292=CARTESIAN_POINT ( 'NONE',  ( -9.474510206698720793, -16.51473224551083518, 74.58442372801900433 ) ) ;
#78293=CARTESIAN_POINT ( 'NONE',  ( -16.51473224551082808, 9.474510206698731452, 33.33442372801899722 ) ) ;
#78295=CARTESIAN_POINT ( 'NONE',  ( -19.05341960407611168, -5.049401038298163336, 31.45724293864769550 ) ) ;
#78296=CARTESIAN_POINT ( 'NONE',  ( -12.06949235617756955, 12.14591786802309770, 30.62390960531436335 ) ) ;
#78297=CARTESIAN_POINT ( 'NONE',  ( 16.46253265017160672, -9.564922557960803928, 23.33224293864769194 ) ) ;
#78298=CARTESIAN_POINT ( 'NONE',  ( 14.29746914071049879, -8.314922557960816363, 28.33224293864769550 ) ) ;
#78299=CARTESIAN_POINT ( 'NONE',  ( -19.49671883438224995, -5.500000000000074607, 84.89279849105676590 ) ) ;
#78300=CARTESIAN_POINT ( 'NONE',  ( -16.53943276465976808, -0.05219959533934237506, 98.75109039468568994 ) ) ;
#78301=CARTESIAN_POINT ( 'NONE',  ( -5.153800228976328057, -19.02544592524343514, 42.29057627198101699 ) ) ;
#78303=CARTESIAN_POINT ( 'NONE',  ( 5.823673210054444382, -21.52544592524334988, 90.20942372801903275 ) ) ;
#78304=CARTESIAN_POINT ( 'NONE',  ( 12.14591786802327356, -12.06949235617739191, 25.62609039468567929 ) ) ;
#78305=CARTESIAN_POINT ( 'NONE',  ( -5.823673210054431948, 21.52544592524334988, 82.70942372801900433 ) ) ;
#78306=CARTESIAN_POINT ( 'NONE',  ( 16.46253265017146816, 9.564922557961045513, 46.66775706135233293 ) ) ;
#78307=CARTESIAN_POINT ( 'NONE',  ( -0.05219959533909027116, -19.03943276465977164, 87.49890960531436690 ) ) ;
#78308=CARTESIAN_POINT ( 'NONE',  ( 16.51473224551069308, 9.474510206698969483, 74.16557627198103830 ) ) ;
#78310=CARTESIAN_POINT ( 'NONE',  ( -16.52544592524342804, 4.483927247898546575, 71.04057627198103830 ) ) ;
#78311=CARTESIAN_POINT ( 'NONE',  ( 5.823673210054125526, 21.52544592524343514, 59.79057627198103120 ) ) ;
#78312=CARTESIAN_POINT ( 'NONE',  ( -19.03943276465977164, 0.05219959533909376836, 61.24890960531436690 ) ) ;
#78313=CARTESIAN_POINT ( 'NONE',  ( 15.80617190586746368, 15.72974639402197994, 79.37390960531436690 ) ) ;
#78314=CARTESIAN_POINT ( 'NONE',  ( -4.379528057220086978, -16.55341960407618274, 79.79275706135236135 ) ) ;
#78315=EDGE_CURVE ( 'NONE', #144387, #176032, #186652, .T. ) ;
#78316=VERTEX_POINT ( 'NONE', #137282 ) ;
#78317=CARTESIAN_POINT ( 'NONE',  ( -0.05219959533909027116, -19.03943276465977164, 52.49890960531436690 ) ) ;
#78318=CARTESIAN_POINT ( 'NONE',  ( -14.34966873604960291, -8.224510206698953496, 81.66557627198103830 ) ) ;
#78320=CARTESIAN_POINT ( 'NONE',  ( 19.02544592524343514, -5.153800228976328945, 53.54057627198102409 ) ) ;
#78321=CARTESIAN_POINT ( 'NONE',  ( -8.314922557960811034, -14.29746914071050412, 112.0822429386477097 ) ) ;
#78322=CARTESIAN_POINT ( 'NONE',  ( -13.89961937509957401, -13.97604488694547875, 64.37609039468567573 ) ) ;
#78323=CARTESIAN_POINT ( 'NONE',  ( 16.53943276465976808, -0.05219959533910856209, 83.74890960531435269 ) ) ;
#78324=CARTESIAN_POINT ( 'NONE',  ( 10.81492255796106328, -18.62759615963255655, 45.41775706135234003 ) ) ;
#78325=CARTESIAN_POINT ( 'NONE',  ( -5.153800228976328057, -19.02544592524343514, 42.29057627198101699 ) ) ;
#78326=CARTESIAN_POINT ( 'NONE',  ( 15.80617190586746368, 15.72974639402197994, 104.3739096053143669 ) ) ;
#78328=CARTESIAN_POINT ( 'NONE',  ( 8.314922557960818139, 14.29746914071049879, 89.58224293864768129 ) ) ;
#78330=CARTESIAN_POINT ( 'NONE',  ( -19.02544592524342804, 5.153800228976336051, 51.04057627198103120 ) ) ;
#78331=DIRECTION ( 'NONE',  ( 0.000000000000000000, 0.000000000000000000, -1.000000000000000000 ) ) ;
#78332=CARTESIAN_POINT ( 'NONE',  ( 0.05219959533936267826, -19.03943276465977164, 90.00109039468567573 ) ) ;
#78333=CARTESIAN_POINT ( 'NONE',  ( 16.51473224551069308, 9.474510206698969483, 104.1655762719810241 ) ) ;
#78334=CARTESIAN_POINT ( 'NONE',  ( 21.55341960407619695, -5.719274019375665929, 41.04275706135236135 ) ) ;
#78335=CARTESIAN_POINT ( 'NONE',  ( -13.89961937509977652, 13.97604488694528158, 80.62390960531436690 ) ) ;
#78336=CARTESIAN_POINT ( 'NONE',  ( -9.474510206698720793, -16.51473224551083518, 74.58442372801900433 ) ) ;
#78337=CARTESIAN_POINT ( 'NONE',  ( 16.51473224551069308, 9.474510206698969483, 49.16557627198102409 ) ) ;
#78338=CARTESIAN_POINT ( 'NONE',  ( -8.314922557960811034, -14.29746914071050412, 77.08224293864769550 ) ) ;
#78339=CARTESIAN_POINT ( 'NONE',  ( -16.55341960407611168, -4.379528057220339221, 61.45724293864770260 ) ) ;
#78340=CARTESIAN_POINT ( 'NONE',  ( 16.51473224551069308, 9.474510206698969483, 79.16557627198103830 ) ) ;
#78341=CARTESIAN_POINT ( 'NONE',  ( -5.823673210054116645, -21.52544592524344225, 107.2905762719810525 ) ) ;
#78342=CARTESIAN_POINT ( 'NONE',  ( -5.049401038298153566, 19.05341960407611168, 75.20724293864769550 ) ) ;
#78343=CARTESIAN_POINT ( 'NONE',  ( -19.02544592524334988, -5.153800228976617603, 18.95942372801899722 ) ) ;
#78344=CARTESIAN_POINT ( 'NONE',  ( -16.51473224551069308, -9.474510206698971260, 36.66557627198102409 ) ) ;
#78345=CARTESIAN_POINT ( 'NONE',  ( -16.55341960407611168, -4.379528057220339221, 36.45724293864768839 ) ) ;
#78346=CARTESIAN_POINT ( 'NONE',  ( -4.483927247898539470, -16.52544592524342804, 107.2905762719810525 ) ) ;
#78347=CARTESIAN_POINT ( 'NONE',  ( -16.51473224551082808, 9.474510206698731452, 103.3344237280190043 ) ) ;
#78349=CARTESIAN_POINT ( 'NONE',  ( 21.52544592524334988, 5.823673210054432836, 26.45942372801901854 ) ) ;
#78350=CARTESIAN_POINT ( 'NONE',  ( 5.153800228976615827, -19.02544592524334988, 65.20942372801900433 ) ) ;
#78351=CARTESIAN_POINT ( 'NONE',  ( 16.55341960407611168, 4.379528057220329451, 23.95724293864769550 ) ) ;
#78352=CARTESIAN_POINT ( 'NONE',  ( -15.80617190586745835, -15.72974639402198527, 81.87390960531435269 ) ) ;
#78353=CARTESIAN_POINT ( 'NONE',  ( 21.55341960407610458, 5.719274019375980345, 23.95724293864769550 ) ) ;
#78354=CARTESIAN_POINT ( 'NONE',  ( 4.379528057220339221, -16.55341960407611168, 52.70724293864769550 ) ) ;
#78355=CARTESIAN_POINT ( 'NONE',  ( -13.89961937509977652, 13.97604488694528158, 35.62390960531435269 ) ) ;
#78356=CARTESIAN_POINT ( 'NONE',  ( 19.05341960407617918, -5.049401038297876454, 21.04275706135232582 ) ) ;
#78357=CARTESIAN_POINT ( 'NONE',  ( -14.29746914071037622, -8.314922557961029526, 84.16775706135234714 ) ) ;
#78358=CARTESIAN_POINT ( 'NONE',  ( 14.34966873604972726, -8.224510206698740333, 55.83442372801901854 ) ) ;
#78359=CARTESIAN_POINT ( 'NONE',  ( -5.719274019375978568, 21.55341960407610458, 25.20724293864769550 ) ) ;
#78360=CARTESIAN_POINT ( 'NONE',  ( -15.72974639402176322, -15.80617190586768395, 104.3760903946856899 ) ) ;
#78361=CARTESIAN_POINT ( 'NONE',  ( 16.46253265017160672, -9.564922557960803928, 83.33224293864768129 ) ) ;
#78362=CARTESIAN_POINT ( 'NONE',  ( -16.55341960407617563, 4.379528057220093196, 63.54275706135234003 ) ) ;
#78363=CARTESIAN_POINT ( 'NONE',  ( -12.14591786802309592, -12.06949235617757132, 106.8739096053143811 ) ) ;
#78364=CARTESIAN_POINT ( 'NONE',  ( -4.379528057220328563, 16.55341960407611168, 35.20724293864768839 ) ) ;
#78365=CARTESIAN_POINT ( 'NONE',  ( -18.22780087662122028, 5.500000000000031086, 38.51540105326107266 ) ) ;
#78366=CARTESIAN_POINT ( 'NONE',  ( 15.72974639402176855, 15.80617190586768217, 71.87609039468568994 ) ) ;
#78367=CARTESIAN_POINT ( 'NONE',  ( -13.97604488694527625, -13.89961937509977652, 91.87390960531432427 ) ) ;
#78368=CARTESIAN_POINT ( 'NONE',  ( 13.89961937509977652, -13.97604488694527269, 73.12390960531436690 ) ) ;
#78369=CARTESIAN_POINT ( 'NONE',  ( 13.97604488694527802, 13.89961937509977652, 109.3739096053143669 ) ) ;
#78370=CARTESIAN_POINT ( 'NONE',  ( -16.55341960407611168, -4.379528057220339221, 61.45724293864770260 ) ) ;
#78371=CARTESIAN_POINT ( 'NONE',  ( -16.53943276465976808, 0.05219959533911058130, 31.24890960531435979 ) ) ;
#78372=CARTESIAN_POINT ( 'NONE',  ( -0.05219959533910754901, -16.53943276465976808, 57.49890960531435979 ) ) ;
#78373=CARTESIAN_POINT ( 'NONE',  ( -14.29746914071037622, -8.314922557961029526, 39.16775706135235424 ) ) ;
#78374=CARTESIAN_POINT ( 'NONE',  ( 17.49999999999999289, -3.565345528327872771, 31.92494486806480580 ) ) ;
#78375=CARTESIAN_POINT ( 'NONE',  ( -5.049401038297874678, -19.05341960407617918, 44.79275706135232582 ) ) ;
#78376=CARTESIAN_POINT ( 'NONE',  ( 9.564922557960805705, 16.46253265017160317, 69.58224293864770971 ) ) ;
#78377=CARTESIAN_POINT ( 'NONE',  ( 19.03943276465977164, 0.05219959533936151252, 46.25109039468566863 ) ) ;
#78378=CARTESIAN_POINT ( 'NONE',  ( 5.049401038297881783, 19.05341960407617563, 52.29275706135234003 ) ) ;
#78379=CARTESIAN_POINT ( 'NONE',  ( -9.474510206698720793, -16.51473224551083518, 104.5844237280190043 ) ) ;
#78380=CARTESIAN_POINT ( 'NONE',  ( -16.52544592524335698, -4.483927247898792601, 88.95942372801901854 ) ) ;
#78382=CARTESIAN_POINT ( 'NONE',  ( -5.049401038298153566, 19.05341960407611168, 25.20724293864768484 ) ) ;
#78383=CARTESIAN_POINT ( 'NONE',  ( 13.89961937509977652, -13.97604488694527269, 108.1239096053143669 ) ) ;
#78384=CARTESIAN_POINT ( 'NONE',  ( 18.62759615963255655, 10.81492255796105972, 36.66775706135234714 ) ) ;
#78385=CARTESIAN_POINT ( 'NONE',  ( -0.05219959533936034679, 19.03943276465977164, 92.50109039468566152 ) ) ;
#78387=CARTESIAN_POINT ( 'NONE',  ( -19.02544592524342804, 5.153800228976336051, 56.04057627198100988 ) ) ;
#78388=CARTESIAN_POINT ( 'NONE',  ( -19.03943276465977164, 0.05219959533909376836, 101.2489096053143669 ) ) ;
#78389=CARTESIAN_POINT ( 'NONE',  ( -8.224510206698948167, 14.34966873604960824, 55.41557627198102409 ) ) ;
#78390=CARTESIAN_POINT ( 'NONE',  ( -13.89961937509977652, 13.97604488694528158, 65.62390960531436690 ) ) ;
#78391=CARTESIAN_POINT ( 'NONE',  ( 16.51473224551069308, 9.474510206698969483, 59.16557627198102409 ) ) ;
#78392=CARTESIAN_POINT ( 'NONE',  ( -9.474510206698720793, -16.51473224551083518, 59.58442372801900433 ) ) ;
#78393=CARTESIAN_POINT ( 'NONE',  ( 5.823673210054125526, 21.52544592524343514, 54.79057627198104541 ) ) ;
#78394=CARTESIAN_POINT ( 'NONE',  ( -9.564922557961040184, 16.46253265017147172, 37.91775706135233293 ) ) ;
#78395=CARTESIAN_POINT ( 'NONE',  ( 9.564922557960805705, 16.46253265017160317, 74.58224293864769550 ) ) ;
#78396=CARTESIAN_POINT ( 'NONE',  ( -10.81492255796078084, -18.62759615963271287, 82.08224293864768129 ) ) ;
#78397=CARTESIAN_POINT ( 'NONE',  ( 8.314922557960818139, 14.29746914071049879, 74.58224293864768129 ) ) ;
#78398=CARTESIAN_POINT ( 'NONE',  ( 0.05219959533936267826, -19.03943276465977164, 30.00109039468566863 ) ) ;
#78399=CARTESIAN_POINT ( 'NONE',  ( 18.67979575497178502, 10.72451020669898547, 49.16557627198102409 ) ) ;
#78400=CARTESIAN_POINT ( 'NONE',  ( -5.719274019375978568, 21.55341960407610458, 40.20724293864769550 ) ) ;
#78401=CARTESIAN_POINT ( 'NONE',  ( 9.564922557960805705, 16.46253265017160317, 69.58224293864770971 ) ) ;
#78402=CARTESIAN_POINT ( 'NONE',  ( 16.46253265017160672, -9.564922557960803928, 53.33224293864768839 ) ) ;
#78403=CARTESIAN_POINT ( 'NONE',  ( 19.02544592524343514, -5.153800228976328945, 23.54057627198102054 ) ) ;
#78404=CARTESIAN_POINT ( 'NONE',  ( 5.719274019375673035, 21.55341960407619339, 22.29275706135235069 ) ) ;
#78406=CARTESIAN_POINT ( 'NONE',  ( 5.719274019375673035, 21.55341960407619339, 27.29275706135234358 ) ) ;
#78407=CARTESIAN_POINT ( 'NONE',  ( -5.049401038298153566, 19.05341960407611168, 35.20724293864768839 ) ) ;
#78408=CARTESIAN_POINT ( 'NONE',  ( 18.62759615963271287, -10.81492255796078972, 108.3322429386477097 ) ) ;
#78409=CARTESIAN_POINT ( 'NONE',  ( -19.03943276465977164, -0.05219959533935918106, 43.75109039468566863 ) ) ;
#78410=CARTESIAN_POINT ( 'NONE',  ( 9.474510206698971260, -16.51473224551069308, 27.91557627198103120 ) ) ;
#78411=CARTESIAN_POINT ( 'NONE',  ( -13.97604488694527625, -13.89961937509977652, 21.87390960531435979 ) ) ;
#78413=CARTESIAN_POINT ( 'NONE',  ( -4.379528057220086978, -16.55341960407618274, 64.79275706135234714 ) ) ;
#78414=CARTESIAN_POINT ( 'NONE',  ( 13.97604488694527802, 13.89961937509977652, 24.37390960531435624 ) ) ;
#78416=CARTESIAN_POINT ( 'NONE',  ( 9.564922557960805705, 16.46253265017160317, 74.58224293864769550 ) ) ;
#78417=CARTESIAN_POINT ( 'NONE',  ( -14.29746914071049879, 8.314922557960819915, 105.8322429386476955 ) ) ;
#78419=CARTESIAN_POINT ( 'NONE',  ( -21.52544592524343514, 5.823673210054127303, 66.04057627198103830 ) ) ;
#78420=CARTESIAN_POINT ( 'NONE',  ( 16.53943276465976808, -0.05219959533910856209, 73.74890960531433848 ) ) ;
#78421=CARTESIAN_POINT ( 'NONE',  ( -4.379528057220086978, -16.55341960407618274, 29.79275706135234358 ) ) ;
#78422=CARTESIAN_POINT ( 'NONE',  ( -15.80617190586768217, 15.72974639402176855, 88.12609039468570415 ) ) ;
#78424=CARTESIAN_POINT ( 'NONE',  ( -19.02544592524342804, 5.153800228976336051, 31.04057627198102409 ) ) ;
#78425=CARTESIAN_POINT ( 'NONE',  ( 16.53943276465976808, 0.05219959533934440121, 111.2510903946856899 ) ) ;
#78426=CARTESIAN_POINT ( 'NONE',  ( 14.34966873604960469, 8.224510206698951720, 54.16557627198103120 ) ) ;
#78427=CARTESIAN_POINT ( 'NONE',  ( 16.46253265017160672, -9.564922557960803928, 53.33224293864768839 ) ) ;
#78428=CARTESIAN_POINT ( 'NONE',  ( 21.52544592524334988, 5.823673210054432836, 101.4594237280190185 ) ) ;
#78429=CARTESIAN_POINT ( 'NONE',  ( -15.80617190586745835, -15.72974639402198527, 101.8739096053143811 ) ) ;
#78430=CARTESIAN_POINT ( 'NONE',  ( -10.72451020669870658, -18.67979575497194134, 74.58442372801901854 ) ) ;
#78431=CARTESIAN_POINT ( 'NONE',  ( -4.379528057220086978, -16.55341960407618274, 39.79275706135235424 ) ) ;
#78432=CARTESIAN_POINT ( 'NONE',  ( 4.483927247898545687, 16.52544592524342804, 84.79057627198102409 ) ) ;
#78433=CARTESIAN_POINT ( 'NONE',  ( 15.80617190586769283, -15.72974639402175789, 85.62609039468568994 ) ) ;
#78435=CARTESIAN_POINT ( 'NONE',  ( 14.29746914071049879, -8.314922557960816363, 23.33224293864769194 ) ) ;
#78436=CARTESIAN_POINT ( 'NONE',  ( -16.61371651742599198, 7.165104196376160139, 113.8541506999300026 ) ) ;
#78437=CARTESIAN_POINT ( 'NONE',  ( -8.314922557961024197, 14.29746914071037800, 42.91775706135235424 ) ) ;
#78438=CARTESIAN_POINT ( 'NONE',  ( -14.29746914071049879, 8.314922557960819915, 35.83224293864768839 ) ) ;
#78439=CARTESIAN_POINT ( 'NONE',  ( -8.314922557961024197, 14.29746914071037800, 92.91775706135236135 ) ) ;
#78440=CARTESIAN_POINT ( 'NONE',  ( -9.474510206698964154, 16.51473224551069663, 100.4155762719810241 ) ) ;
#78441=CARTESIAN_POINT ( 'NONE',  ( 5.153800228976335163, 19.02544592524342804, 114.7905762719810241 ) ) ;
#78442=CARTESIAN_POINT ( 'NONE',  ( 0.05219959533937995610, -21.53943276465977519, 105.0010903946856757 ) ) ;
#78443=CARTESIAN_POINT ( 'NONE',  ( -14.29746914071037622, -8.314922557961029526, 104.1677570613523471 ) ) ;
#78444=CARTESIAN_POINT ( 'NONE',  ( -14.34966873604960291, -8.224510206698953496, 71.66557627198100988 ) ) ;
#78445=CARTESIAN_POINT ( 'NONE',  ( -19.03943276465977164, 0.05219959533909376836, 81.24890960531436690 ) ) ;
#78447=CARTESIAN_POINT ( 'NONE',  ( 16.53943276465976808, 0.05219959533934440121, 26.25109039468567573 ) ) ;
#78448=CARTESIAN_POINT ( 'NONE',  ( 5.049401038298161559, -19.05341960407611168, 22.70724293864769194 ) ) ;
#78449=CARTESIAN_POINT ( 'NONE',  ( 13.97604488694527802, 13.89961937509977652, 94.37390960531436690 ) ) ;
#78450=CARTESIAN_POINT ( 'NONE',  ( -4.483927247898782831, 16.52544592524335698, 32.70942372801900433 ) ) ;
#78452=CARTESIAN_POINT ( 'NONE',  ( 19.03943276465977164, 0.05219959533936151252, 36.25109039468567573 ) ) ;
#78453=CARTESIAN_POINT ( 'NONE',  ( -0.05219959533934338120, 16.53943276465976808, 87.50109039468568994 ) ) ;
#78454=CARTESIAN_POINT ( 'NONE',  ( 9.474510206698729675, 16.51473224551082808, 102.0844237280190043 ) ) ;
#78455=CARTESIAN_POINT ( 'NONE',  ( 19.02544592524343514, -5.153800228976328945, 38.54057627198103120 ) ) ;
#78456=CARTESIAN_POINT ( 'NONE',  ( 4.483927247898790824, -16.52544592524335698, 85.20942372801901854 ) ) ;
#78457=CARTESIAN_POINT ( 'NONE',  ( -14.29746914071037622, -8.314922557961029526, 69.16775706135234714 ) ) ;
#78458=CARTESIAN_POINT ( 'NONE',  ( -0.05219959533936034679, 19.03943276465977164, 77.50109039468566152 ) ) ;
#78459=CARTESIAN_POINT ( 'NONE',  ( -9.474510206698720793, -16.51473224551083518, 19.58442372801899722 ) ) ;
#78460=CARTESIAN_POINT ( 'NONE',  ( -16.51473224551069308, -9.474510206698971260, 41.66557627198103120 ) ) ;
#78461=CARTESIAN_POINT ( 'NONE',  ( -0.05219959533909027116, -19.03943276465977164, 97.49890960531436690 ) ) ;
#78462=CARTESIAN_POINT ( 'NONE',  ( -14.29746914071049879, 8.314922557960819915, 80.83224293864769550 ) ) ;
#78463=CARTESIAN_POINT ( 'NONE',  ( 13.89961937509957401, 13.97604488694547697, 51.87609039468566863 ) ) ;
#78464=CARTESIAN_POINT ( 'NONE',  ( 18.67979575497178502, 10.72451020669898547, 49.16557627198102409 ) ) ;
#78465=CARTESIAN_POINT ( 'NONE',  ( 19.02544592524334988, 5.153800228976608722, 26.45942372801899722 ) ) ;
#78466=CARTESIAN_POINT ( 'NONE',  ( -19.03943276465977164, 0.05219959533909376836, 96.24890960531436690 ) ) ;
#78467=EDGE_CURVE ( 'NONE', #196449, #160325, #190701, .T. ) ;
#78468=CARTESIAN_POINT ( 'NONE',  ( 19.05341960407617918, -5.049401038297876454, 26.04275706135233293 ) ) ;
#78469=CARTESIAN_POINT ( 'NONE',  ( 5.823673210054125526, 21.52544592524343514, 74.79057627198105251 ) ) ;
#78470=CARTESIAN_POINT ( 'NONE',  ( 16.46253265017160672, -9.564922557960803928, 108.3322429386476955 ) ) ;
#78471=CARTESIAN_POINT ( 'NONE',  ( 13.89961937509957401, 13.97604488694547697, 81.87609039468564731 ) ) ;
#78472=FACE_OUTER_BOUND ( 'NONE', #9269, .T. ) ;
#78473=CARTESIAN_POINT ( 'NONE',  ( -16.52544592524335698, -4.483927247898792601, 18.95942372801901143 ) ) ;
#78475=CARTESIAN_POINT ( 'NONE',  ( 16.46253265017160672, -9.564922557960803928, 33.33224293864770260 ) ) ;
#78476=CARTESIAN_POINT ( 'NONE',  ( -19.03943276465977164, 0.05219959533909376836, 91.24890960531436690 ) ) ;
#78477=CARTESIAN_POINT ( 'NONE',  ( -5.719274019375978568, 21.55341960407610458, 70.20724293864769550 ) ) ;
#78478=CARTESIAN_POINT ( 'NONE',  ( 12.06949235617739724, 12.14591786802326823, 51.87609039468568284 ) ) ;
#78479=CARTESIAN_POINT ( 'NONE',  ( 10.81492255796106328, -18.62759615963255655, 45.41775706135234003 ) ) ;
#78480=CARTESIAN_POINT ( 'NONE',  ( 13.89961937509957401, 13.97604488694547697, 86.87609039468567573 ) ) ;
#78481=CARTESIAN_POINT ( 'NONE',  ( 21.52544592524334988, 5.823673210054432836, 96.45942372801901854 ) ) ;
#78482=CARTESIAN_POINT ( 'NONE',  ( 14.29746914071037800, 8.314922557961029526, 91.66775706135234714 ) ) ;
#78483=CARTESIAN_POINT ( 'NONE',  ( -9.474510206698964154, 16.51473224551069663, 95.41557627198102409 ) ) ;
#78484=CARTESIAN_POINT ( 'NONE',  ( -16.52544592524342804, 4.483927247898546575, 96.04057627198102409 ) ) ;
#78485=CARTESIAN_POINT ( 'NONE',  ( -16.53943276465976808, 0.05219959533911058130, 36.24890960531435979 ) ) ;
#78486=CARTESIAN_POINT ( 'NONE',  ( -19.03943276465977164, -0.05219959533935918106, 73.75109039468566152 ) ) ;
#78487=CARTESIAN_POINT ( 'NONE',  ( -5.823673210054431948, 21.52544592524334988, 62.70942372801902565 ) ) ;
#78488=CARTESIAN_POINT ( 'NONE',  ( -0.05219959533936034679, 19.03943276465977164, 22.50109039468566152 ) ) ;
#78489=CARTESIAN_POINT ( 'NONE',  ( -14.34966873604960291, -8.224510206698953496, 106.6655762719810383 ) ) ;
#78490=CARTESIAN_POINT ( 'NONE',  ( -10.81492255796078084, -18.62759615963271287, 37.08224293864768129 ) ) ;
#78491=CARTESIAN_POINT ( 'NONE',  ( 14.29746914071037800, 8.314922557961029526, 111.6677570613523613 ) ) ;
#78492=CARTESIAN_POINT ( 'NONE',  ( 21.52544592524334988, 5.823673210054432836, 96.45942372801901854 ) ) ;
#78493=CARTESIAN_POINT ( 'NONE',  ( -4.483927247898782831, 16.52544592524335698, 62.70942372801902565 ) ) ;
#78494=CARTESIAN_POINT ( 'NONE',  ( -16.53943276465976808, -0.05219959533934237506, 103.7510903946857042 ) ) ;
#78495=CARTESIAN_POINT ( 'NONE',  ( -15.80617190586768217, 15.72974639402176855, 53.12609039468568284 ) ) ;
#78496=CARTESIAN_POINT ( 'NONE',  ( -5.719274019375665041, -21.55341960407619695, 59.79275706135234714 ) ) ;
#78498=CARTESIAN_POINT ( 'NONE',  ( -5.719274019375665041, -21.55341960407619695, 29.79275706135234358 ) ) ;
#78499=CARTESIAN_POINT ( 'NONE',  ( -4.379528057220328563, 16.55341960407611168, 100.2072429386476955 ) ) ;
#78500=CARTESIAN_POINT ( 'NONE',  ( 19.03943276465977164, -0.05219959533909143690, 28.74890960531435624 ) ) ;
#78501=CARTESIAN_POINT ( 'NONE',  ( -14.29746914071049879, 8.314922557960819915, 85.83224293864768129 ) ) ;
#78502=CARTESIAN_POINT ( 'NONE',  ( -19.03943276465977164, 0.05219959533909376836, 66.24890960531436690 ) ) ;
#78503=CARTESIAN_POINT ( 'NONE',  ( 0.05219959533934541429, -16.53943276465976808, 110.0010903946856757 ) ) ;
#78504=CARTESIAN_POINT ( 'NONE',  ( -10.81492255796078084, -18.62759615963271287, 57.08224293864769550 ) ) ;
#78505=CARTESIAN_POINT ( 'NONE',  ( -16.55341960407611168, -4.379528057220339221, 86.45724293864770971 ) ) ;
#78506=CARTESIAN_POINT ( 'NONE',  ( -5.823673210054116645, -21.52544592524344225, 97.29057627198105251 ) ) ;
#78507=CARTESIAN_POINT ( 'NONE',  ( -16.51473224551069308, -9.474510206698971260, 96.66557627198102409 ) ) ;
#78508=CARTESIAN_POINT ( 'NONE',  ( -5.153800228976328057, -19.02544592524343514, 52.29057627198100988 ) ) ;
#78509=CARTESIAN_POINT ( 'NONE',  ( 13.89961937509957401, 13.97604488694547697, 111.8760903946856757 ) ) ;
#78510=CARTESIAN_POINT ( 'NONE',  ( 21.53943276465977519, -0.05219959533907433946, 38.74890960531435979 ) ) ;
#78511=CARTESIAN_POINT ( 'NONE',  ( 21.52544592524334988, 5.823673210054432836, 71.45942372801901854 ) ) ;
#78512=CARTESIAN_POINT ( 'NONE',  ( 19.02544592524343514, -5.153800228976328945, 68.54057627198103830 ) ) ;
#78513=CARTESIAN_POINT ( 'NONE',  ( 5.049401038298161559, -19.05341960407611168, 102.7072429386476955 ) ) ;
#78514=CARTESIAN_POINT ( 'NONE',  ( -14.29746914071037622, -8.314922557961029526, 59.16775706135234714 ) ) ;
#78515=CARTESIAN_POINT ( 'NONE',  ( -0.05219959533937732626, 21.53943276465977519, 42.50109039468567573 ) ) ;
#78516=CARTESIAN_POINT ( 'NONE',  ( -10.72451020669870658, -18.67979575497194134, 84.58442372801903275 ) ) ;
#78517=CARTESIAN_POINT ( 'NONE',  ( 10.72451020669898902, -18.67979575497178502, 97.91557627198103830 ) ) ;
#78518=CARTESIAN_POINT ( 'NONE',  ( -15.72974639402176322, -15.80617190586768395, 39.37609039468567573 ) ) ;
#78519=CARTESIAN_POINT ( 'NONE',  ( 8.314922557961029526, -14.29746914071037800, 80.41775706135234714 ) ) ;
#78520=CARTESIAN_POINT ( 'NONE',  ( -18.62759615963270932, 10.81492255796079327, 75.83224293864769550 ) ) ;
#78521=CARTESIAN_POINT ( 'NONE',  ( -16.46253265017146816, -9.564922557961047289, 39.16775706135234003 ) ) ;
#78522=CARTESIAN_POINT ( 'NONE',  ( 9.474510206698971260, -16.51473224551069308, 87.91557627198102409 ) ) ;
#78523=CARTESIAN_POINT ( 'NONE',  ( -8.314922557961024197, 14.29746914071037800, 112.9177570613523329 ) ) ;
#78524=CARTESIAN_POINT ( 'NONE',  ( -17.12812012977024168, 6.668231424566043231, 63.64051240676855770 ) ) ;
#78525=CARTESIAN_POINT ( 'NONE',  ( -19.03943276465977164, 0.05219959533909376836, 101.2489096053143669 ) ) ;
#78527=CARTESIAN_POINT ( 'NONE',  ( 19.03943276465977164, 0.05219959533936151252, 91.25109039468566152 ) ) ;
#78528=CARTESIAN_POINT ( 'NONE',  ( 18.62759615963271287, -10.81492255796078972, 53.33224293864769550 ) ) ;
#78529=CARTESIAN_POINT ( 'NONE',  ( 16.52544592524342804, -4.483927247898539470, 43.54057627198103830 ) ) ;
#78530=CARTESIAN_POINT ( 'NONE',  ( -8.314922557961024197, 14.29746914071037800, 22.91775706135235069 ) ) ;
#78531=CARTESIAN_POINT ( 'NONE',  ( -9.474510206698964154, 16.51473224551069663, 25.41557627198103120 ) ) ;
#78532=CARTESIAN_POINT ( 'NONE',  ( 19.05341960407617918, -5.049401038297876454, 111.0427570613523329 ) ) ;
#78533=CARTESIAN_POINT ( 'NONE',  ( 18.62759615963271287, -10.81492255796078972, 98.33224293864769550 ) ) ;
#78534=CARTESIAN_POINT ( 'NONE',  ( -19.03943276465977164, -0.05219959533935918106, 68.75109039468566152 ) ) ;
#78535=CARTESIAN_POINT ( 'NONE',  ( -16.55341960407617563, 4.379528057220093196, 78.54275706135236135 ) ) ;
#78536=CARTESIAN_POINT ( 'NONE',  ( -16.46253265017160317, 9.564922557960807481, 70.83224293864770971 ) ) ;
#78537=CARTESIAN_POINT ( 'NONE',  ( -16.52544592524342804, 4.483927247898546575, 71.04057627198103830 ) ) ;
#78538=CARTESIAN_POINT ( 'NONE',  ( -9.474510206698964154, 16.51473224551069663, 65.41557627198102409 ) ) ;
#78539=CARTESIAN_POINT ( 'NONE',  ( -16.53943276465976808, 0.05219959533911058130, 71.24890960531435269 ) ) ;
#78542=CARTESIAN_POINT ( 'NONE',  ( -14.29746914071049879, 8.314922557960819915, 35.83224293864768839 ) ) ;
#78543=CARTESIAN_POINT ( 'NONE',  ( 5.153800228976335163, 19.02544592524342804, 79.79057627198102409 ) ) ;
#78545=CARTESIAN_POINT ( 'NONE',  ( 9.474510206698729675, 16.51473224551082808, 57.08442372801900433 ) ) ;
#78546=CARTESIAN_POINT ( 'NONE',  ( 12.14591786802327356, -12.06949235617739191, 65.62609039468568994 ) ) ;
#78547=CARTESIAN_POINT ( 'NONE',  ( -21.55341960407610458, -5.719274019375992779, 61.45724293864770260 ) ) ;
#78548=CARTESIAN_POINT ( 'NONE',  ( -19.05341960407617563, 5.049401038297882671, 23.54275706135233648 ) ) ;
#78549=CARTESIAN_POINT ( 'NONE',  ( 19.03943276465977164, -0.05219959533909143690, 78.74890960531436690 ) ) ;
#78551=CARTESIAN_POINT ( 'NONE',  ( 19.05341960407611168, 5.049401038298154454, 113.9572429386477097 ) ) ;
#78552=CARTESIAN_POINT ( 'NONE',  ( 9.564922557960805705, 16.46253265017160317, 64.58224293864769550 ) ) ;
#78553=CARTESIAN_POINT ( 'NONE',  ( 21.53943276465977519, 0.05219959533937863772, 41.25109039468568284 ) ) ;
#78554=CARTESIAN_POINT ( 'NONE',  ( 16.53943276465976808, -0.05219959533910856209, 103.7489096053143669 ) ) ;
#78555=CARTESIAN_POINT ( 'NONE',  ( -21.55341960407610458, -5.719274019375992779, 96.45724293864770971 ) ) ;
#78556=CARTESIAN_POINT ( 'NONE',  ( 16.51473224551069308, 9.474510206698969483, 94.16557627198103830 ) ) ;
#78558=CARTESIAN_POINT ( 'NONE',  ( -10.81492255796105439, 18.62759615963255655, 27.91775706135234358 ) ) ;
#78561=CARTESIAN_POINT ( 'NONE',  ( 16.46253265017160672, -9.564922557960803928, 83.33224293864768129 ) ) ;
#78564=CARTESIAN_POINT ( 'NONE',  ( -5.719274019375978568, 21.55341960407610458, 100.2072429386476955 ) ) ;
#78565=CARTESIAN_POINT ( 'NONE',  ( 0.05219959533909260263, 19.03943276465977164, 44.99890960531435979 ) ) ;
#78566=CARTESIAN_POINT ( 'NONE',  ( -0.05219959533936034679, 19.03943276465977164, 107.5010903946856615 ) ) ;
#78568=CARTESIAN_POINT ( 'NONE',  ( 5.049401038298161559, -19.05341960407611168, 22.70724293864769194 ) ) ;
#78569=CARTESIAN_POINT ( 'NONE',  ( 18.67979575497194134, -10.72451020669871369, 80.83442372801901854 ) ) ;
#78570=CARTESIAN_POINT ( 'NONE',  ( -5.153800228976328057, -19.02544592524343514, 82.29057627198103830 ) ) ;
#78571=CARTESIAN_POINT ( 'NONE',  ( -15.80617190586768217, 15.72974639402176855, 43.12609039468568284 ) ) ;
#78572=CARTESIAN_POINT ( 'NONE',  ( 18.67979575497194134, -10.72451020669871369, 30.83442372801902209 ) ) ;
#78574=CARTESIAN_POINT ( 'NONE',  ( 13.97604488694527802, 13.89961937509977652, 84.37390960531433848 ) ) ;
#78576=CARTESIAN_POINT ( 'NONE',  ( 4.379528057220092307, 16.55341960407617563, 42.29275706135235424 ) ) ;
#78577=CARTESIAN_POINT ( 'NONE',  ( 21.55341960407610458, 5.719274019375980345, 43.95724293864769550 ) ) ;
#78578=CARTESIAN_POINT ( 'NONE',  ( 0.05219959533937995610, -21.53943276465977519, 40.00109039468567573 ) ) ;
#78579=CARTESIAN_POINT ( 'NONE',  ( 18.67979575497194134, -10.72451020669871369, 70.83442372801901854 ) ) ;
#78581=CARTESIAN_POINT ( 'NONE',  ( -19.02544592524334988, -5.153800228976617603, 108.9594237280189759 ) ) ;
#78582=CARTESIAN_POINT ( 'NONE',  ( -19.05341960407611168, -5.049401038298163336, 61.45724293864769550 ) ) ;
#78583=CARTESIAN_POINT ( 'NONE',  ( -19.05341960407611168, -5.049401038298163336, 81.45724293864769550 ) ) ;
#78584=CARTESIAN_POINT ( 'NONE',  ( -16.55341960407611168, -4.379528057220339221, 106.4572429386477097 ) ) ;
#78585=CARTESIAN_POINT ( 'NONE',  ( -12.06949235617756955, 12.14591786802309770, 105.6239096053143669 ) ) ;
#78586=CARTESIAN_POINT ( 'NONE',  ( 10.81492255796078972, 18.62759615963270932, 34.58224293864770260 ) ) ;
#78588=CARTESIAN_POINT ( 'NONE',  ( -12.06949235617739369, -12.14591786802326823, 79.37609039468567573 ) ) ;
#78589=CARTESIAN_POINT ( 'NONE',  ( 4.483927247898545687, 16.52544592524342804, 64.79057627198103830 ) ) ;
#78590=CARTESIAN_POINT ( 'NONE',  ( 19.05341960407611168, 5.049401038298154454, 58.95724293864768129 ) ) ;
#78591=CARTESIAN_POINT ( 'NONE',  ( 10.72451020669871369, 18.67979575497193778, 82.08442372801901854 ) ) ;
#78592=CARTESIAN_POINT ( 'NONE',  ( -18.62759615963255300, -10.81492255796106328, 69.16775706135234714 ) ) ;
#78593=CARTESIAN_POINT ( 'NONE',  ( 16.46253265017146816, 9.564922557961045513, 111.6677570613523329 ) ) ;
#78594=CARTESIAN_POINT ( 'NONE',  ( -16.55341960407611168, -4.379528057220339221, 56.45724293864768839 ) ) ;
#78595=CARTESIAN_POINT ( 'NONE',  ( 5.719274019375673035, 21.55341960407619339, 27.29275706135234358 ) ) ;
#78596=CARTESIAN_POINT ( 'NONE',  ( 5.823673210054125526, 21.52544592524343514, 64.79057627198103830 ) ) ;
#78597=CARTESIAN_POINT ( 'NONE',  ( 19.01529144963336648, 5.499999999999971578, 73.73431955728440812 ) ) ;
#78599=CARTESIAN_POINT ( 'NONE',  ( 0.05219959533909260263, 19.03943276465977164, 74.99890960531435269 ) ) ;
#78600=CARTESIAN_POINT ( 'NONE',  ( -8.224510206698948167, 14.34966873604960824, 30.41557627198101699 ) ) ;
#78601=CARTESIAN_POINT ( 'NONE',  ( -4.483927247898539470, -16.52544592524342804, 22.29057627198102765 ) ) ;
#78602=CARTESIAN_POINT ( 'NONE',  ( -4.483927247898782831, 16.52544592524335698, 92.70942372801901854 ) ) ;
#78603=CARTESIAN_POINT ( 'NONE',  ( -16.51473224551082808, 9.474510206698731452, 58.33442372801900433 ) ) ;
#78605=CARTESIAN_POINT ( 'NONE',  ( 9.474510206698971260, -16.51473224551069308, 102.9155762719810241 ) ) ;
#78606=CARTESIAN_POINT ( 'NONE',  ( 12.14591786802309770, 12.06949235617756955, 74.37390960531436690 ) ) ;
#78607=CARTESIAN_POINT ( 'NONE',  ( -19.02544592524334988, -5.153800228976617603, 48.95942372801900433 ) ) ;
#78608=CARTESIAN_POINT ( 'NONE',  ( -5.153800228976328057, -19.02544592524343514, 37.29057627198102409 ) ) ;
#78609=CARTESIAN_POINT ( 'NONE',  ( -19.03943276465977164, 0.05219959533909376836, 116.2489096053143669 ) ) ;
#78610=CARTESIAN_POINT ( 'NONE',  ( -10.72451020669898014, 18.67979575497178502, 50.41557627198103120 ) ) ;
#78611=ORIENTED_EDGE ( 'NONE', *, *, #154603, .T. ) ;
#78612=CARTESIAN_POINT ( 'NONE',  ( -16.52544592524342804, 4.483927247898546575, 96.04057627198102409 ) ) ;
#78613=CARTESIAN_POINT ( 'NONE',  ( -14.34966873604972548, 8.224510206698743886, 58.33442372801901143 ) ) ;
#78614=CARTESIAN_POINT ( 'NONE',  ( 8.224510206698953496, -14.34966873604960469, 92.91557627198103830 ) ) ;
#78617=CARTESIAN_POINT ( 'NONE',  ( -5.049401038298153566, 19.05341960407611168, 110.2072429386476671 ) ) ;
#78619=DIRECTION ( 'NONE',  ( 0.000000000000000000, -1.000000000000000000, 0.000000000000000000 ) ) ;
#78620=CARTESIAN_POINT ( 'NONE',  ( -16.52544592524335698, -4.483927247898792601, 43.95942372801902565 ) ) ;
#78621=CARTESIAN_POINT ( 'NONE',  ( 16.52544592524342804, -4.483927247898539470, 23.54057627198102765 ) ) ;
#78622=CARTESIAN_POINT ( 'NONE',  ( -15.80617190586745835, -15.72974639402198527, 56.87390960531436690 ) ) ;
#78623=CIRCLE ( 'NONE', #46310, 2.000000000000000000 ) ;
#78624=CARTESIAN_POINT ( 'NONE',  ( 16.51473224551083163, -9.474510206698727899, 80.83442372801899012 ) ) ;
#78625=CARTESIAN_POINT ( 'NONE',  ( -18.62759615963270932, 10.81492255796079327, 45.83224293864769550 ) ) ;
#78626=CARTESIAN_POINT ( 'NONE',  ( 18.67979575497194134, -10.72451020669871369, 80.83442372801901854 ) ) ;
#78628=CARTESIAN_POINT ( 'NONE',  ( -0.05219959533934338120, 16.53943276465976808, 47.50109039468568994 ) ) ;
#78629=CARTESIAN_POINT ( 'NONE',  ( 16.51473224551069308, 9.474510206698969483, 39.16557627198103120 ) ) ;
#78630=CARTESIAN_POINT ( 'NONE',  ( 0.05219959533909260263, 19.03943276465977164, 99.99890960531436690 ) ) ;
#78631=CARTESIAN_POINT ( 'NONE',  ( -19.02544592524342804, 5.153800228976336051, 41.04057627198103120 ) ) ;
#78632=CARTESIAN_POINT ( 'NONE',  ( 14.34966873604960469, 8.224510206698951720, 104.1655762719810241 ) ) ;
#78634=CARTESIAN_POINT ( 'NONE',  ( 16.51473224551069308, 9.474510206698969483, 99.16557627198102409 ) ) ;
#78636=CARTESIAN_POINT ( 'NONE',  ( -0.05219959533934338120, 16.53943276465976808, 52.50109039468567573 ) ) ;
#78637=CARTESIAN_POINT ( 'NONE',  ( 5.719274019375991003, -21.55341960407610458, 92.70724293864770971 ) ) ;
#78638=CARTESIAN_POINT ( 'NONE',  ( -13.97604488694527625, -13.89961937509977652, 51.87390960531436690 ) ) ;
#78639=CARTESIAN_POINT ( 'NONE',  ( 10.81492255796106328, -18.62759615963255655, 25.41775706135235779 ) ) ;
#78640=CARTESIAN_POINT ( 'NONE',  ( -5.153800228976328057, -19.02544592524343514, 82.29057627198103830 ) ) ;
#78643=CARTESIAN_POINT ( 'NONE',  ( -16.55341960407617563, 4.379528057220093196, 53.54275706135234714 ) ) ;
#78644=CARTESIAN_POINT ( 'NONE',  ( 18.67979575497194134, -10.72451020669871369, 20.83442372801901143 ) ) ;
#78645=CARTESIAN_POINT ( 'NONE',  ( 0.05219959533909260263, 19.03943276465977164, 29.99890960531435979 ) ) ;
#78646=CARTESIAN_POINT ( 'NONE',  ( 16.46253265017160672, -9.564922557960803928, 103.3322429386476955 ) ) ;
#78647=CARTESIAN_POINT ( 'NONE',  ( -9.564922557961040184, 16.46253265017147172, 72.91775706135233293 ) ) ;
#78648=CARTESIAN_POINT ( 'NONE',  ( 16.51473224551083163, -9.474510206698727899, 30.83442372801900433 ) ) ;
#78649=CARTESIAN_POINT ( 'NONE',  ( 21.53943276465977519, -0.05219959533907433946, 88.74890960531436690 ) ) ;
#78650=CARTESIAN_POINT ( 'NONE',  ( -9.564922557961040184, 16.46253265017147172, 32.91775706135233293 ) ) ;
#78651=CARTESIAN_POINT ( 'NONE',  ( 8.314922557961029526, -14.29746914071037800, 80.41775706135234714 ) ) ;
#78652=CARTESIAN_POINT ( 'NONE',  ( -0.05219959533909027116, -19.03943276465977164, 102.4989096053143669 ) ) ;
#78653=CARTESIAN_POINT ( 'NONE',  ( -5.153800228976328057, -19.02544592524343514, 62.29057627198100988 ) ) ;
#78654=CARTESIAN_POINT ( 'NONE',  ( 5.719274019375673035, 21.55341960407619339, 72.29275706135236135 ) ) ;
#78655=CARTESIAN_POINT ( 'NONE',  ( -0.05219959533937732626, 21.53943276465977519, 87.50109039468568994 ) ) ;
#78656=CARTESIAN_POINT ( 'NONE',  ( -16.51473224551069308, -9.474510206698971260, 71.66557627198102409 ) ) ;
#78657=CARTESIAN_POINT ( 'NONE',  ( -0.05219959533937732626, 21.53943276465977519, 52.50109039468567573 ) ) ;
#78658=CARTESIAN_POINT ( 'NONE',  ( -13.97604488694547697, 13.89961937509957934, 83.12609039468564731 ) ) ;
#78659=CARTESIAN_POINT ( 'NONE',  ( 19.03943276465977164, -0.05219959533909143690, 53.74890960531436690 ) ) ;
#78660=CARTESIAN_POINT ( 'NONE',  ( -13.97604488694527625, -13.89961937509977652, 101.8739096053143811 ) ) ;
#78661=CARTESIAN_POINT ( 'NONE',  ( -16.46253265017160317, 9.564922557960807481, 70.83224293864770971 ) ) ;
#78662=CARTESIAN_POINT ( 'NONE',  ( 16.51473224551069308, 9.474510206698969483, 114.1655762719810241 ) ) ;
#78663=CARTESIAN_POINT ( 'NONE',  ( 16.51473224551069308, 9.474510206698969483, 49.16557627198102409 ) ) ;
#78664=CARTESIAN_POINT ( 'NONE',  ( -15.80617190586745835, -15.72974639402198527, 96.87390960531436690 ) ) ;
#78665=CARTESIAN_POINT ( 'NONE',  ( 8.224510206698742110, 14.34966873604972548, 77.08442372801901854 ) ) ;
#78667=CARTESIAN_POINT ( 'NONE',  ( 19.05341960407617918, -5.049401038297876454, 31.04275706135232227 ) ) ;
#78668=ADVANCED_FACE ( 'NONE', ( #159397 ), #131406, .T. ) ;
#78669=CARTESIAN_POINT ( 'NONE',  ( -16.46253265017160317, 9.564922557960807481, 60.83224293864769550 ) ) ;
#78670=CARTESIAN_POINT ( 'NONE',  ( 16.53943276465976808, -0.05219959533910856209, 63.74890960531435979 ) ) ;
#78671=CARTESIAN_POINT ( 'NONE',  ( 12.06949235617757843, -12.14591786802309237, 88.12390960531436690 ) ) ;
#78672=CARTESIAN_POINT ( 'NONE',  ( 19.05341960407611168, 5.049401038298154454, 103.9572429386476671 ) ) ;
#78673=CARTESIAN_POINT ( 'NONE',  ( -13.97604488694527625, -13.89961937509977652, 91.87390960531432427 ) ) ;
#78674=CARTESIAN_POINT ( 'NONE',  ( -16.51473224551069308, -9.474510206698971260, 106.6655762719810383 ) ) ;
#78675=CARTESIAN_POINT ( 'NONE',  ( -10.72451020669870658, -18.67979575497194134, 109.5844237280190328 ) ) ;
#78676=CARTESIAN_POINT ( 'NONE',  ( -12.14591786802326823, 12.06949235617739902, 88.12609039468570415 ) ) ;
#78677=CARTESIAN_POINT ( 'NONE',  ( 0.05219959533937995610, -21.53943276465977519, 40.00109039468567573 ) ) ;
#78678=CARTESIAN_POINT ( 'NONE',  ( -18.67979575497178146, -10.72451020669898902, 31.66557627198102054 ) ) ;
#78679=CARTESIAN_POINT ( 'NONE',  ( -10.81492255796078084, -18.62759615963271287, 107.0822429386476955 ) ) ;
#78680=CARTESIAN_POINT ( 'NONE',  ( 0.05219959533910956823, 16.53943276465976808, 54.99890960531435269 ) ) ;
#78681=CARTESIAN_POINT ( 'NONE',  ( 9.474510206698971260, -16.51473224551069308, 52.91557627198102409 ) ) ;
#78682=CARTESIAN_POINT ( 'NONE',  ( -0.05219959533910754901, -16.53943276465976808, 87.49890960531436690 ) ) ;
#78683=CARTESIAN_POINT ( 'NONE',  ( 15.80617190586746368, 15.72974639402197994, 49.37390960531436690 ) ) ;
#78684=CARTESIAN_POINT ( 'NONE',  ( 5.049401038297881783, 19.05341960407617563, 42.29275706135234003 ) ) ;
#78685=CARTESIAN_POINT ( 'NONE',  ( 5.153800228976335163, 19.02544592524342804, 24.79057627198102765 ) ) ;
#78687=CARTESIAN_POINT ( 'NONE',  ( -16.55341960407617563, 4.379528057220093196, 73.54275706135234714 ) ) ;
#78688=CARTESIAN_POINT ( 'NONE',  ( 5.049401038298161559, -19.05341960407611168, 62.70724293864769550 ) ) ;
#78690=CARTESIAN_POINT ( 'NONE',  ( 12.14591786802309770, 12.06949235617756955, 89.37390960531435269 ) ) ;
#78691=CARTESIAN_POINT ( 'NONE',  ( 21.52544592524344225, -5.823673210054117533, 43.54057627198103830 ) ) ;
#78693=CARTESIAN_POINT ( 'NONE',  ( 12.06949235617739724, 12.14591786802326823, 106.8760903946856899 ) ) ;
#78694=CARTESIAN_POINT ( 'NONE',  ( -12.06949235617739369, -12.14591786802326823, 29.37609039468568284 ) ) ;
#78695=CARTESIAN_POINT ( 'NONE',  ( 10.72451020669871369, 18.67979575497193778, 97.08442372801904696 ) ) ;
#78696=CARTESIAN_POINT ( 'NONE',  ( 13.97604488694527802, 13.89961937509977652, 89.37390960531436690 ) ) ;
#78697=CARTESIAN_POINT ( 'NONE',  ( 18.67979575497178502, 10.72451020669898547, 114.1655762719810383 ) ) ;
#78698=CARTESIAN_POINT ( 'NONE',  ( 9.474510206698971260, -16.51473224551069308, 27.91557627198103120 ) ) ;
#78699=CARTESIAN_POINT ( 'NONE',  ( -8.314922557961024197, 14.29746914071037800, 27.91775706135234358 ) ) ;
#78700=CARTESIAN_POINT ( 'NONE',  ( -5.153800228976607833, 19.02544592524334988, 97.70942372801900433 ) ) ;
#78701=AXIS2_PLACEMENT_3D ( 'NONE', #136379, #30192, #91834 ) ;
#78702=CARTESIAN_POINT ( 'NONE',  ( 21.55341960407610458, 5.719274019375980345, 83.95724293864770971 ) ) ;
#78703=CARTESIAN_POINT ( 'NONE',  ( 9.474510206698729675, 16.51473224551082808, 67.08442372801900433 ) ) ;
#78704=LINE ( 'NONE', #79710, #92943 ) ;
#78705=CARTESIAN_POINT ( 'NONE',  ( -10.81492255796105439, 18.62759615963255655, 22.91775706135235069 ) ) ;
#78706=CARTESIAN_POINT ( 'NONE',  ( -5.153800228976328057, -19.02544592524343514, 72.29057627198102409 ) ) ;
#78707=CARTESIAN_POINT ( 'NONE',  ( 5.049401038298161559, -19.05341960407611168, 82.70724293864770971 ) ) ;
#78708=CARTESIAN_POINT ( 'NONE',  ( -8.224510206698735004, -14.34966873604973081, 39.58442372801901143 ) ) ;
#78710=CARTESIAN_POINT ( 'NONE',  ( -19.02544592524334988, -5.153800228976617603, 63.95942372801899012 ) ) ;
#78711=CARTESIAN_POINT ( 'NONE',  ( 18.67979575497194134, -10.72451020669871369, 20.83442372801901143 ) ) ;
#78712=CARTESIAN_POINT ( 'NONE',  ( 16.55341960407611168, 4.379528057220329451, 73.95724293864769550 ) ) ;
#78713=CARTESIAN_POINT ( 'NONE',  ( 13.97604488694527802, 13.89961937509977652, 84.37390960531433848 ) ) ;
#78714=CARTESIAN_POINT ( 'NONE',  ( -14.29746914071037622, -8.314922557961029526, 34.16775706135234714 ) ) ;
#78715=CARTESIAN_POINT ( 'NONE',  ( -19.05341960407617563, 5.049401038297882671, 48.54275706135233293 ) ) ;
#78716=CARTESIAN_POINT ( 'NONE',  ( 5.823673210054444382, -21.52544592524334988, 60.20942372801902565 ) ) ;
#78717=CARTESIAN_POINT ( 'NONE',  ( 5.153800228976615827, -19.02544592524334988, 105.2094237280190185 ) ) ;
#78718=CARTESIAN_POINT ( 'NONE',  ( 19.05341960407611168, 5.049401038298154454, 58.95724293864768129 ) ) ;
#78719=CARTESIAN_POINT ( 'NONE',  ( 16.46253265017146816, 9.564922557961045513, 76.66775706135234714 ) ) ;
#78720=CARTESIAN_POINT ( 'NONE',  ( 12.14591786802327356, -12.06949235617739191, 50.62609039468568994 ) ) ;
#78721=CARTESIAN_POINT ( 'NONE',  ( 18.62759615963255655, 10.81492255796105972, 96.66775706135234714 ) ) ;
#78722=CARTESIAN_POINT ( 'NONE',  ( 9.564922557961047289, -16.46253265017146816, 70.41775706135233293 ) ) ;
#78723=CARTESIAN_POINT ( 'NONE',  ( -19.03943276465977164, 0.05219959533909376836, 46.24890960531435979 ) ) ;
#78724=CARTESIAN_POINT ( 'NONE',  ( 0.05219959533907565091, 21.53943276465977519, 69.99890960531435269 ) ) ;
#78725=CARTESIAN_POINT ( 'NONE',  ( 12.14591786802309770, 12.06949235617756955, 69.37390960531436690 ) ) ;
#78726=CARTESIAN_POINT ( 'NONE',  ( -19.05341960407617563, 5.049401038297882671, 63.54275706135234003 ) ) ;
#78728=CARTESIAN_POINT ( 'NONE',  ( 13.97604488694548053, -13.89961937509957401, 40.62609039468564731 ) ) ;
#78729=CARTESIAN_POINT ( 'NONE',  ( 16.53943276465976808, 0.05219959533934440121, 96.25109039468568994 ) ) ;
#78730=CARTESIAN_POINT ( 'NONE',  ( -8.314922557960811034, -14.29746914071050412, 62.08224293864769550 ) ) ;
#78731=CARTESIAN_POINT ( 'NONE',  ( -10.81492255796105439, 18.62759615963255655, 97.91775706135236135 ) ) ;
#78733=CARTESIAN_POINT ( 'NONE',  ( 10.72451020669898902, -18.67979575497178502, 97.91557627198103830 ) ) ;
#78734=CARTESIAN_POINT ( 'NONE',  ( 9.474510206698971260, -16.51473224551069308, 52.91557627198102409 ) ) ;
#78735=CARTESIAN_POINT ( 'NONE',  ( 0.05219959533937995610, -21.53943276465977519, 75.00109039468568994 ) ) ;
#78736=CARTESIAN_POINT ( 'NONE',  ( -9.474510206698964154, 16.51473224551069663, 55.41557627198103120 ) ) ;
#78737=CARTESIAN_POINT ( 'NONE',  ( -9.564922557960796823, -16.46253265017161027, 67.08224293864769550 ) ) ;
#78738=CARTESIAN_POINT ( 'NONE',  ( 16.46253265017160672, -9.564922557960803928, 28.33224293864769550 ) ) ;
#78739=CARTESIAN_POINT ( 'NONE',  ( -9.564922557960796823, -16.46253265017161027, 107.0822429386476955 ) ) ;
#78740=CARTESIAN_POINT ( 'NONE',  ( 16.52544592524342804, -4.483927247898539470, 68.54057627198103830 ) ) ;
#78741=CARTESIAN_POINT ( 'NONE',  ( 19.05341960407611168, 5.049401038298154454, 33.95724293864769550 ) ) ;
#78742=CARTESIAN_POINT ( 'NONE',  ( -0.05219959533910754901, -16.53943276465976808, 82.49890960531436690 ) ) ;
#78743=CARTESIAN_POINT ( 'NONE',  ( -10.72451020669898014, 18.67979575497178502, 90.41557627198103830 ) ) ;
#78744=CARTESIAN_POINT ( 'NONE',  ( 18.62759615963255655, 10.81492255796105972, 31.66775706135234358 ) ) ;
#78746=CARTESIAN_POINT ( 'NONE',  ( 16.52544592524335698, 4.483927247898782831, 46.45942372801901854 ) ) ;
#78747=CARTESIAN_POINT ( 'NONE',  ( 21.52544592524344225, -5.823673210054117533, 83.54057627198102409 ) ) ;
#78748=CARTESIAN_POINT ( 'NONE',  ( 15.72974639402176855, 15.80617190586768217, 111.8760903946856615 ) ) ;
#78749=CARTESIAN_POINT ( 'NONE',  ( -19.03943276465977164, 0.05219959533909376836, 106.2489096053143669 ) ) ;
#78750=CARTESIAN_POINT ( 'NONE',  ( 10.81492255796106328, -18.62759615963255655, 45.41775706135234003 ) ) ;
#78751=CARTESIAN_POINT ( 'NONE',  ( 21.53943276465977519, -0.05219959533907433946, 48.74890960531435979 ) ) ;
#78752=CARTESIAN_POINT ( 'NONE',  ( 8.224510206698742110, 14.34966873604972548, 102.0844237280190185 ) ) ;
#78753=CARTESIAN_POINT ( 'NONE',  ( -10.81492255796105439, 18.62759615963255655, 62.91775706135236135 ) ) ;
#78754=CARTESIAN_POINT ( 'NONE',  ( 15.80617190586769283, -15.72974639402175789, 100.6260903946857184 ) ) ;
#78755=CARTESIAN_POINT ( 'NONE',  ( -9.474510206698720793, -16.51473224551083518, 34.58442372801899722 ) ) ;
#78756=CARTESIAN_POINT ( 'NONE',  ( 14.29746914071037800, 8.314922557961029526, 81.66775706135236135 ) ) ;
#78757=CARTESIAN_POINT ( 'NONE',  ( -15.80617190586768217, 15.72974639402176855, 43.12609039468568284 ) ) ;
#78758=CARTESIAN_POINT ( 'NONE',  ( -0.05219959533909027116, -19.03943276465977164, 47.49890960531435979 ) ) ;
#78759=CARTESIAN_POINT ( 'NONE',  ( -5.153800228976607833, 19.02544592524334988, 22.70942372801899012 ) ) ;
#78760=CARTESIAN_POINT ( 'NONE',  ( -21.53943276465977519, 0.05219959533907696930, 26.24890960531435624 ) ) ;
#78761=CARTESIAN_POINT ( 'NONE',  ( -10.81492255796078084, -18.62759615963271287, 112.0822429386477097 ) ) ;
#78762=CARTESIAN_POINT ( 'NONE',  ( -10.72451020669898014, 18.67979575497178502, 75.41557627198102409 ) ) ;
#78763=CARTESIAN_POINT ( 'NONE',  ( 0.05219959533934541429, -16.53943276465976808, 45.00109039468568284 ) ) ;
#78765=CARTESIAN_POINT ( 'NONE',  ( 10.72451020669898902, -18.67979575497178502, 77.91557627198102409 ) ) ;
#78766=CARTESIAN_POINT ( 'NONE',  ( 16.52544592524335698, 4.483927247898782831, 71.45942372801901854 ) ) ;
#78767=CARTESIAN_POINT ( 'NONE',  ( -16.52544592524342804, 4.483927247898546575, 61.04057627198103120 ) ) ;
#78769=CARTESIAN_POINT ( 'NONE',  ( 5.153800228976615827, -19.02544592524334988, 85.20942372801900433 ) ) ;
#78772=CARTESIAN_POINT ( 'NONE',  ( -16.52544592524335698, -4.483927247898792601, 43.95942372801902565 ) ) ;
#78773=CARTESIAN_POINT ( 'NONE',  ( -18.62759615963255300, -10.81492255796106328, 19.16775706135234714 ) ) ;
#78774=CARTESIAN_POINT ( 'NONE',  ( -21.55341960407610458, -5.719274019375992779, 81.45724293864769550 ) ) ;
#78775=CARTESIAN_POINT ( 'NONE',  ( -0.05219959533907301413, -21.53943276465977519, 22.49890960531436335 ) ) ;
#78776=CARTESIAN_POINT ( 'NONE',  ( 4.483927247898790824, -16.52544592524335698, 60.20942372801902565 ) ) ;
#78777=CARTESIAN_POINT ( 'NONE',  ( 5.049401038298161559, -19.05341960407611168, 77.70724293864765286 ) ) ;
#78778=CARTESIAN_POINT ( 'NONE',  ( -21.55341960407619339, 5.719274019375674811, 43.54275706135235424 ) ) ;
#78779=CARTESIAN_POINT ( 'NONE',  ( -9.474510206698720793, -16.51473224551083518, 109.5844237280190043 ) ) ;
#78780=CARTESIAN_POINT ( 'NONE',  ( -5.049401038298153566, 19.05341960407611168, 110.2072429386476671 ) ) ;
#78781=CARTESIAN_POINT ( 'NONE',  ( 9.474510206698729675, 16.51473224551082808, 32.08442372801900433 ) ) ;
#78782=CARTESIAN_POINT ( 'NONE',  ( -8.314922557961024197, 14.29746914071037800, 42.91775706135235424 ) ) ;
#78783=CARTESIAN_POINT ( 'NONE',  ( 19.02544592524343514, -5.153800228976328945, 98.54057627198100988 ) ) ;
#78784=CARTESIAN_POINT ( 'NONE',  ( 5.823673210054125526, 21.52544592524343514, 104.7905762719810241 ) ) ;
#78785=CARTESIAN_POINT ( 'NONE',  ( 19.03943276465977164, -0.05219959533909143690, 63.74890960531435979 ) ) ;
#78786=CARTESIAN_POINT ( 'NONE',  ( -16.20579543436682357, 7.371946100354950460, 24.43479165828125232 ) ) ;
#78787=CARTESIAN_POINT ( 'NONE',  ( 16.52544592524342804, -4.483927247898539470, 83.54057627198102409 ) ) ;
#78788=CARTESIAN_POINT ( 'NONE',  ( 5.153800228976335163, 19.02544592524342804, 114.7905762719810241 ) ) ;
#78789=CARTESIAN_POINT ( 'NONE',  ( -13.97604488694527625, -13.89961937509977652, 21.87390960531435979 ) ) ;
#78790=CARTESIAN_POINT ( 'NONE',  ( -5.823673210054116645, -21.52544592524344225, 102.2905762719810383 ) ) ;
#78791=CARTESIAN_POINT ( 'NONE',  ( 13.89961937509957401, 13.97604488694547697, 66.87609039468567573 ) ) ;
#78792=CARTESIAN_POINT ( 'NONE',  ( 5.719274019375991003, -21.55341960407610458, 37.70724293864769550 ) ) ;
#78793=CARTESIAN_POINT ( 'NONE',  ( 16.51473224551069308, 9.474510206698969483, 29.16557627198103475 ) ) ;
#78794=CARTESIAN_POINT ( 'NONE',  ( -21.55341960407610458, -5.719274019375992779, 61.45724293864770260 ) ) ;
#78796=CARTESIAN_POINT ( 'NONE',  ( 0.05219959533909260263, 19.03943276465977164, 99.99890960531436690 ) ) ;
#78797=CARTESIAN_POINT ( 'NONE',  ( 5.823673210054444382, -21.52544592524334988, 85.20942372801901854 ) ) ;
#78798=CARTESIAN_POINT ( 'NONE',  ( -9.564922557960796823, -16.46253265017161027, 57.08224293864769550 ) ) ;
#78799=CARTESIAN_POINT ( 'NONE',  ( -16.53943276465976808, 0.05219959533911058130, 91.24890960531436690 ) ) ;
#78800=CARTESIAN_POINT ( 'NONE',  ( 12.06949235617739724, 12.14591786802326823, 31.87609039468567929 ) ) ;
#78801=CARTESIAN_POINT ( 'NONE',  ( 5.049401038298161559, -19.05341960407611168, 62.70724293864769550 ) ) ;
#78802=CARTESIAN_POINT ( 'NONE',  ( 21.55341960407619695, -5.719274019375665929, 71.04275706135234714 ) ) ;
#78803=EDGE_LOOP ( 'NONE', ( #97445, #135756, #72697, #141795, #49687, #16460, #136839, #106521, #130568, #141693, #32373, #94044, #73338, #29884 ) ) ;
#78804=CARTESIAN_POINT ( 'NONE',  ( 0.05219959533936267826, -19.03943276465977164, 30.00109039468566863 ) ) ;
#78805=CARTESIAN_POINT ( 'NONE',  ( 16.51473224551083163, -9.474510206698727899, 45.83442372801900433 ) ) ;
#78807=CARTESIAN_POINT ( 'NONE',  ( 21.52544592524334988, 5.823673210054432836, 36.45942372801901143 ) ) ;
#78809=CARTESIAN_POINT ( 'NONE',  ( -19.02544592524334988, -5.153800228976617603, 33.95942372801897591 ) ) ;
#78810=CARTESIAN_POINT ( 'NONE',  ( -5.049401038298153566, 19.05341960407611168, 90.20724293864766707 ) ) ;
#78811=CARTESIAN_POINT ( 'NONE',  ( 9.564922557960805705, 16.46253265017160317, 69.58224293864770971 ) ) ;
#78812=CARTESIAN_POINT ( 'NONE',  ( 16.53943276465976808, -0.05219959533910856209, 23.74890960531435269 ) ) ;
#78813=CARTESIAN_POINT ( 'NONE',  ( -21.55341960407610458, -5.719274019375992779, 26.45724293864768839 ) ) ;
#78814=CARTESIAN_POINT ( 'NONE',  ( 21.55341960407619695, -5.719274019375665929, 81.04275706135236135 ) ) ;
#78817=CARTESIAN_POINT ( 'NONE',  ( -5.719274019375665041, -21.55341960407619695, 84.79275706135234714 ) ) ;
#78818=CARTESIAN_POINT ( 'NONE',  ( 16.29526858892873520, -7.335722546920258935, 41.70329402199793378 ) ) ;
#78819=CARTESIAN_POINT ( 'NONE',  ( -5.049401038298153566, 19.05341960407611168, 105.2072429386476671 ) ) ;
#78821=CARTESIAN_POINT ( 'NONE',  ( -5.719274019375978568, 21.55341960407610458, 65.20724293864768129 ) ) ;
#78822=EDGE_CURVE ( 'NONE', #128850, #196699, #22037, .T. ) ;
#78823=CARTESIAN_POINT ( 'NONE',  ( -16.53943276465976808, 0.05219959533911058130, 31.24890960531435979 ) ) ;
#78824=CARTESIAN_POINT ( 'NONE',  ( -12.06949235617756955, 12.14591786802309770, 110.6239096053143669 ) ) ;
#78825=CARTESIAN_POINT ( 'NONE',  ( 5.153800228976335163, 19.02544592524342804, 89.79057627198102409 ) ) ;
#78826=CARTESIAN_POINT ( 'NONE',  ( 16.46253265017146816, 9.564922557961045513, 21.66775706135233648 ) ) ;
#78827=CARTESIAN_POINT ( 'NONE',  ( -4.483927247898539470, -16.52544592524342804, 102.2905762719810383 ) ) ;
#78828=CARTESIAN_POINT ( 'NONE',  ( -15.80617190586768217, 15.72974639402176855, 68.12609039468567573 ) ) ;
#78829=CARTESIAN_POINT ( 'NONE',  ( -5.153800228976328057, -19.02544592524343514, 97.29057627198102409 ) ) ;
#78830=CARTESIAN_POINT ( 'NONE',  ( 16.55341960407618274, -4.379528057220086978, 111.0427570613523613 ) ) ;
#78831=CARTESIAN_POINT ( 'NONE',  ( 16.51473224551083163, -9.474510206698727899, 65.83442372801900433 ) ) ;
#78832=CARTESIAN_POINT ( 'NONE',  ( -17.50000000000000711, -5.500000000000025757, 51.28230962303570095 ) ) ;
#78833=CARTESIAN_POINT ( 'NONE',  ( 19.03943276465977164, -0.05219959533909143690, 103.7489096053143669 ) ) ;
#78834=CARTESIAN_POINT ( 'NONE',  ( 14.34966873604960469, 8.224510206698951720, 94.16557627198103830 ) ) ;
#78835=CARTESIAN_POINT ( 'NONE',  ( 9.564922557961047289, -16.46253265017146816, 60.41775706135233293 ) ) ;
#78836=CARTESIAN_POINT ( 'NONE',  ( 5.049401038298161559, -19.05341960407611168, 77.70724293864765286 ) ) ;
#78837=CARTESIAN_POINT ( 'NONE',  ( -12.14591786802309592, -12.06949235617757132, 56.87390960531436690 ) ) ;
#78838=CARTESIAN_POINT ( 'NONE',  ( -16.46253265017146816, -9.564922557961047289, 89.16775706135234714 ) ) ;
#78839=CARTESIAN_POINT ( 'NONE',  ( 18.67979575497178502, 10.72451020669898547, 49.16557627198102409 ) ) ;
#78841=CARTESIAN_POINT ( 'NONE',  ( -4.483927247898539470, -16.52544592524342804, 112.2905762719810241 ) ) ;
#78842=CARTESIAN_POINT ( 'NONE',  ( 18.22780087662122384, -5.500000000000022204, 101.0154010532610869 ) ) ;
#78843=CARTESIAN_POINT ( 'NONE',  ( 5.049401038298161559, -19.05341960407611168, 72.70724293864768129 ) ) ;
#78844=CARTESIAN_POINT ( 'NONE',  ( -0.05219959533907301413, -21.53943276465977519, 77.49890960531433848 ) ) ;
#78845=CARTESIAN_POINT ( 'NONE',  ( -0.05219959533934338120, 16.53943276465976808, 97.50109039468567573 ) ) ;
#78846=CARTESIAN_POINT ( 'NONE',  ( 0.05219959533909260263, 19.03943276465977164, 74.99890960531435269 ) ) ;
#78847=CARTESIAN_POINT ( 'NONE',  ( 13.97604488694548053, -13.89961937509957401, 50.62609039468566152 ) ) ;
#78848=CARTESIAN_POINT ( 'NONE',  ( -15.80617190586768217, 15.72974639402176855, 88.12609039468570415 ) ) ;
#78849=CARTESIAN_POINT ( 'NONE',  ( 18.67979575497178502, 10.72451020669898547, 59.16557627198103120 ) ) ;
#78850=CARTESIAN_POINT ( 'NONE',  ( -15.80617190586745835, -15.72974639402198527, 26.87390960531435979 ) ) ;
#78851=CARTESIAN_POINT ( 'NONE',  ( -5.153800228976328057, -19.02544592524343514, 37.29057627198102409 ) ) ;
#78852=CARTESIAN_POINT ( 'NONE',  ( -16.52544592524335698, -4.483927247898792601, 103.9594237280190185 ) ) ;
#78853=CARTESIAN_POINT ( 'NONE',  ( -12.06949235617739369, -12.14591786802326823, 24.37609039468567573 ) ) ;
#78855=CARTESIAN_POINT ( 'NONE',  ( -5.719274019375665041, -21.55341960407619695, 94.79275706135234714 ) ) ;
#78856=CARTESIAN_POINT ( 'NONE',  ( -14.34966873604960291, -8.224510206698953496, 61.66557627198103120 ) ) ;
#78857=CARTESIAN_POINT ( 'NONE',  ( 21.52544592524344225, -5.823673210054117533, 98.54057627198105251 ) ) ;
#78858=CARTESIAN_POINT ( 'NONE',  ( 15.80617190586746368, 15.72974639402197994, 89.37390960531435269 ) ) ;
#78860=CARTESIAN_POINT ( 'NONE',  ( -0.05219959533907301413, -21.53943276465977519, 42.49890960531435979 ) ) ;
#78861=CARTESIAN_POINT ( 'NONE',  ( 8.224510206698742110, 14.34966873604972548, 72.08442372801899012 ) ) ;
#78862=CARTESIAN_POINT ( 'NONE',  ( -14.34966873604960291, -8.224510206698953496, 91.66557627198103830 ) ) ;
#78863=CARTESIAN_POINT ( 'NONE',  ( 9.474510206698971260, -16.51473224551069308, 47.91557627198102409 ) ) ;
#78865=CARTESIAN_POINT ( 'NONE',  ( -8.224510206698735004, -14.34966873604973081, 99.58442372801900433 ) ) ;
#78866=CARTESIAN_POINT ( 'NONE',  ( 15.80617190586769283, -15.72974639402175789, 35.62609039468568994 ) ) ;
#78867=CARTESIAN_POINT ( 'NONE',  ( 13.89961937509977652, -13.97604488694527269, 98.12390960531433848 ) ) ;
#78868=CARTESIAN_POINT ( 'NONE',  ( -18.67979575497193778, 10.72451020669871902, 73.33442372801901854 ) ) ;
#78869=CARTESIAN_POINT ( 'NONE',  ( 16.46253265017160672, -9.564922557960803928, 23.33224293864769194 ) ) ;
#78870=CARTESIAN_POINT ( 'NONE',  ( -16.51473224551069308, -9.474510206698971260, 26.66557627198103120 ) ) ;
#78873=CARTESIAN_POINT ( 'NONE',  ( -15.80617190586768217, 15.72974639402176855, 63.12609039468568994 ) ) ;
#78874=CARTESIAN_POINT ( 'NONE',  ( -0.05219959533909027116, -19.03943276465977164, 47.49890960531435979 ) ) ;
#78875=CARTESIAN_POINT ( 'NONE',  ( -19.03943276465977164, 0.05219959533909376836, 116.2489096053143669 ) ) ;
#78876=CARTESIAN_POINT ( 'NONE',  ( -5.049401038298153566, 19.05341960407611168, 95.20724293864770971 ) ) ;
#78877=CARTESIAN_POINT ( 'NONE',  ( 16.46253265017146816, 9.564922557961045513, 66.66775706135233293 ) ) ;
#78878=CARTESIAN_POINT ( 'NONE',  ( 21.53943276465977519, 0.05219959533937863772, 41.25109039468568284 ) ) ;
#78879=CARTESIAN_POINT ( 'NONE',  ( 9.564922557961047289, -16.46253265017146816, 60.41775706135233293 ) ) ;
#78880=CARTESIAN_POINT ( 'NONE',  ( 16.46253265017160672, -9.564922557960803928, 33.33224293864770260 ) ) ;
#78881=CARTESIAN_POINT ( 'NONE',  ( 8.314922557961029526, -14.29746914071037800, 100.4177570613523471 ) ) ;
#78882=CARTESIAN_POINT ( 'NONE',  ( -19.05341960407617563, 5.049401038297882671, 73.54275706135233293 ) ) ;
#78883=CARTESIAN_POINT ( 'NONE',  ( 14.34966873604960469, 8.224510206698951720, 29.16557627198103120 ) ) ;
#78884=CARTESIAN_POINT ( 'NONE',  ( -9.474510206698720793, -16.51473224551083518, 49.58442372801899722 ) ) ;
#78885=CARTESIAN_POINT ( 'NONE',  ( 13.97604488694527802, 13.89961937509977652, 99.37390960531436690 ) ) ;
#78886=CARTESIAN_POINT ( 'NONE',  ( 5.823673210054444382, -21.52544592524334988, 110.2094237280190185 ) ) ;
#78887=CARTESIAN_POINT ( 'NONE',  ( -16.46253265017146816, -9.564922557961047289, 29.16775706135232937 ) ) ;
#78888=CARTESIAN_POINT ( 'NONE',  ( 19.03943276465977164, -0.05219959533909143690, 28.74890960531435624 ) ) ;
#78889=CARTESIAN_POINT ( 'NONE',  ( -10.81492255796105439, 18.62759615963255655, 92.91775706135236135 ) ) ;
#78890=CARTESIAN_POINT ( 'NONE',  ( -8.314922557961024197, 14.29746914071037800, 32.91775706135234714 ) ) ;
#78891=CARTESIAN_POINT ( 'NONE',  ( -13.89961937509977652, 13.97604488694528158, 95.62390960531436690 ) ) ;
#78893=CARTESIAN_POINT ( 'NONE',  ( 16.51473224551069308, 9.474510206698969483, 74.16557627198103830 ) ) ;
#78896=CARTESIAN_POINT ( 'NONE',  ( -5.049401038297874678, -19.05341960407617918, 89.79275706135230450 ) ) ;
#78897=CARTESIAN_POINT ( 'NONE',  ( 19.03943276465977164, -0.05219959533909143690, 108.7489096053143527 ) ) ;
#78898=CARTESIAN_POINT ( 'NONE',  ( -21.52544592524334988, -5.823673210054445271, 98.95942372801903275 ) ) ;
#78899=CARTESIAN_POINT ( 'NONE',  ( 14.29746914071049879, -8.314922557960816363, 103.3322429386476955 ) ) ;
#78900=CARTESIAN_POINT ( 'NONE',  ( -13.89961937509977652, 13.97604488694528158, 30.62390960531435269 ) ) ;
#78901=CARTESIAN_POINT ( 'NONE',  ( -21.53943276465977519, 0.05219959533907696930, 41.24890960531435269 ) ) ;
#78902=( GEOMETRIC_REPRESENTATION_CONTEXT ( 3 ) GLOBAL_UNCERTAINTY_ASSIGNED_CONTEXT ( ( #144963 ) ) GLOBAL_UNIT_ASSIGNED_CONTEXT ( ( #183092, #195283, #49536 ) ) REPRESENTATION_CONTEXT ( 'NONE', 'WORKASPACE' ) );
#78903=CARTESIAN_POINT ( 'NONE',  ( -21.52544592524343514, 5.823673210054127303, 31.04057627198102409 ) ) ;
#78904=CARTESIAN_POINT ( 'NONE',  ( 0.05219959533909260263, 19.03943276465977164, 24.99890960531435269 ) ) ;
#78906=CARTESIAN_POINT ( 'NONE',  ( -5.153800228976607833, 19.02544592524334988, 62.70942372801899722 ) ) ;
#78907=CARTESIAN_POINT ( 'NONE',  ( 14.29746914071049879, -8.314922557960816363, 38.33224293864768839 ) ) ;
#78908=CARTESIAN_POINT ( 'NONE',  ( 21.52544592524344225, -5.823673210054117533, 23.54057627198102765 ) ) ;
#78909=CARTESIAN_POINT ( 'NONE',  ( 10.72451020669871369, 18.67979575497193778, 82.08442372801901854 ) ) ;
#78910=CARTESIAN_POINT ( 'NONE',  ( -15.80617190586745835, -15.72974639402198527, 76.87390960531439532 ) ) ;
#78911=CARTESIAN_POINT ( 'NONE',  ( 15.80617190586769283, -15.72974639402175789, 50.62609039468568994 ) ) ;
#78912=CARTESIAN_POINT ( 'NONE',  ( -10.81492255796078084, -18.62759615963271287, 97.08224293864770971 ) ) ;
#78913=CARTESIAN_POINT ( 'NONE',  ( 18.62759615963255655, 10.81492255796105972, 56.66775706135235424 ) ) ;
#78914=CARTESIAN_POINT ( 'NONE',  ( -9.564922557960796823, -16.46253265017161027, 27.08224293864769550 ) ) ;
#78915=CARTESIAN_POINT ( 'NONE',  ( 9.564922557960805705, 16.46253265017160317, 84.58224293864769550 ) ) ;
#78916=CARTESIAN_POINT ( 'NONE',  ( 12.14591786802327356, -12.06949235617739191, 85.62609039468568994 ) ) ;
#78917=CARTESIAN_POINT ( 'NONE',  ( -8.314922557960811034, -14.29746914071050412, 107.0822429386476955 ) ) ;
#78918=CARTESIAN_POINT ( 'NONE',  ( 9.564922557960805705, 16.46253265017160317, 109.5822429386476955 ) ) ;
#78919=CARTESIAN_POINT ( 'NONE',  ( -16.55341960407611168, -4.379528057220339221, 56.45724293864768839 ) ) ;
#78920=CARTESIAN_POINT ( 'NONE',  ( -16.55341960407611168, -4.379528057220339221, 21.45724293864769550 ) ) ;
#78921=CARTESIAN_POINT ( 'NONE',  ( -9.474510206698964154, 16.51473224551069663, 60.41557627198102409 ) ) ;
#78922=CARTESIAN_POINT ( 'NONE',  ( -13.89961937509977652, 13.97604488694528158, 35.62390960531435269 ) ) ;
#78923=CARTESIAN_POINT ( 'NONE',  ( 21.53943276465977519, -0.05219959533907433946, 48.74890960531435979 ) ) ;
#78924=CARTESIAN_POINT ( 'NONE',  ( 0.05219959533936267826, -19.03943276465977164, 35.00109039468566863 ) ) ;
#78927=CARTESIAN_POINT ( 'NONE',  ( 4.379528057220339221, -16.55341960407611168, 42.70724293864770260 ) ) ;
#78928=CARTESIAN_POINT ( 'NONE',  ( 9.564922557960805705, 16.46253265017160317, 109.5822429386476955 ) ) ;
#78929=CARTESIAN_POINT ( 'NONE',  ( -5.719274019375665041, -21.55341960407619695, 54.79275706135235424 ) ) ;
#78931=CARTESIAN_POINT ( 'NONE',  ( 8.314922557961029526, -14.29746914071037800, 65.41775706135234714 ) ) ;
#78932=CARTESIAN_POINT ( 'NONE',  ( 0.05219959533936267826, -19.03943276465977164, 65.00109039468567573 ) ) ;
#78933=CARTESIAN_POINT ( 'NONE',  ( -14.29746914071049879, 8.314922557960819915, 35.83224293864768839 ) ) ;
#78934=CARTESIAN_POINT ( 'NONE',  ( 16.29526858892872454, -7.335722546920200315, 51.70329402199800484 ) ) ;
#78935=CARTESIAN_POINT ( 'NONE',  ( -12.06949235617756955, 12.14591786802309770, 25.62390960531435624 ) ) ;
#78936=CARTESIAN_POINT ( 'NONE',  ( 0.05219959533909260263, 19.03943276465977164, 44.99890960531435979 ) ) ;
#78937=CARTESIAN_POINT ( 'NONE',  ( 19.03943276465977164, -0.05219959533909143690, 58.74890960531435979 ) ) ;
#78938=CARTESIAN_POINT ( 'NONE',  ( -19.02544592524342804, 5.153800228976336051, 31.04057627198102409 ) ) ;
#78939=CARTESIAN_POINT ( 'NONE',  ( -0.05219959533937732626, 21.53943276465977519, 27.50109039468567929 ) ) ;
#78940=CARTESIAN_POINT ( 'NONE',  ( 19.03943276465977164, -0.05219959533909143690, 53.74890960531436690 ) ) ;
#78942=CARTESIAN_POINT ( 'NONE',  ( 5.153800228976335163, 19.02544592524342804, 44.79057627198103830 ) ) ;
#78943=CARTESIAN_POINT ( 'NONE',  ( 21.55341960407610458, 5.719274019375980345, 28.95724293864769905 ) ) ;
#78944=CARTESIAN_POINT ( 'NONE',  ( -21.52544592524334988, -5.823673210054445271, 53.95942372801900433 ) ) ;
#78945=CARTESIAN_POINT ( 'NONE',  ( -5.153800228976328057, -19.02544592524343514, 22.29057627198102765 ) ) ;
#78946=CARTESIAN_POINT ( 'NONE',  ( -15.72974639402197994, 15.80617190586746368, 30.62390960531436335 ) ) ;
#78947=CARTESIAN_POINT ( 'NONE',  ( -16.55341960407617563, 4.379528057220093196, 73.54275706135234714 ) ) ;
#78949=CARTESIAN_POINT ( 'NONE',  ( 15.80617190586769283, -15.72974639402175789, 105.6260903946856899 ) ) ;
#78950=CARTESIAN_POINT ( 'NONE',  ( 0.05219959533934541429, -16.53943276465976808, 70.00109039468568994 ) ) ;
#78951=CARTESIAN_POINT ( 'NONE',  ( 9.564922557960805705, 16.46253265017160317, 99.58224293864770971 ) ) ;
#78952=CARTESIAN_POINT ( 'NONE',  ( -16.55341960407617563, 4.379528057220093196, 48.54275706135234714 ) ) ;
#78953=CARTESIAN_POINT ( 'NONE',  ( -12.06949235617739369, -12.14591786802326823, 29.37609039468568284 ) ) ;
#78954=CARTESIAN_POINT ( 'NONE',  ( 4.379528057220092307, 16.55341960407617563, 97.29275706135234714 ) ) ;
#78955=CARTESIAN_POINT ( 'NONE',  ( -5.719274019375665041, -21.55341960407619695, 54.79275706135235424 ) ) ;
#78956=CARTESIAN_POINT ( 'NONE',  ( 9.564922557961047289, -16.46253265017146816, 105.4177570613523471 ) ) ;
#78957=CARTESIAN_POINT ( 'NONE',  ( 10.72451020669898902, -18.67979575497178502, 107.9155762719810241 ) ) ;
#78958=CARTESIAN_POINT ( 'NONE',  ( -14.34966873604960291, -8.224510206698953496, 106.6655762719810383 ) ) ;
#78959=CARTESIAN_POINT ( 'NONE',  ( -19.03943276465977164, -0.05219959533935918106, 113.7510903946856757 ) ) ;
#78960=CARTESIAN_POINT ( 'NONE',  ( 16.53943276465976808, 0.05219959533934440121, 86.25109039468568994 ) ) ;
#78962=CARTESIAN_POINT ( 'NONE',  ( 5.719274019375673035, 21.55341960407619339, 87.29275706135236135 ) ) ;
#78963=CARTESIAN_POINT ( 'NONE',  ( 0.05219959533936267826, -19.03943276465977164, 80.00109039468567573 ) ) ;
#78964=CARTESIAN_POINT ( 'NONE',  ( 12.14591786802309770, 12.06949235617756955, 44.37390960531435979 ) ) ;
#78965=CARTESIAN_POINT ( 'NONE',  ( 16.55341960407611168, 4.379528057220329451, 48.95724293864770971 ) ) ;
#78966=CARTESIAN_POINT ( 'NONE',  ( -16.53943276465976808, 0.05219959533911058130, 111.2489096053143669 ) ) ;
#78967=CARTESIAN_POINT ( 'NONE',  ( 9.474510206698729675, 16.51473224551082808, 42.08442372801900433 ) ) ;
#78968=CARTESIAN_POINT ( 'NONE',  ( 17.44270441346523626, -5.991230190322815119, 56.13664920735774899 ) ) ;
#78969=CARTESIAN_POINT ( 'NONE',  ( -5.823673210054431948, 21.52544592524334988, 32.70942372801900433 ) ) ;
#78970=CARTESIAN_POINT ( 'NONE',  ( 13.89961937509957401, 13.97604488694547697, 111.8760903946856757 ) ) ;
#78972=CARTESIAN_POINT ( 'NONE',  ( -5.153800228976328057, -19.02544592524343514, 107.2905762719810383 ) ) ;
#78973=CARTESIAN_POINT ( 'NONE',  ( -18.67979575497178146, -10.72451020669898902, 61.66557627198103120 ) ) ;
#78974=CARTESIAN_POINT ( 'NONE',  ( 9.564922557960805705, 16.46253265017160317, 84.58224293864769550 ) ) ;
#78975=CARTESIAN_POINT ( 'NONE',  ( 5.719274019375991003, -21.55341960407610458, 52.70724293864769550 ) ) ;
#78976=CARTESIAN_POINT ( 'NONE',  ( -14.34966873604960291, -8.224510206698953496, 106.6655762719810383 ) ) ;
#78977=CARTESIAN_POINT ( 'NONE',  ( 9.474510206698971260, -16.51473224551069308, 72.91557627198102409 ) ) ;
#78978=CARTESIAN_POINT ( 'NONE',  ( 13.97604488694527802, 13.89961937509977652, 34.37390960531436690 ) ) ;
#78979=CARTESIAN_POINT ( 'NONE',  ( -0.05219959533937732626, 21.53943276465977519, 32.50109039468568284 ) ) ;
#78980=CARTESIAN_POINT ( 'NONE',  ( -10.81492255796105439, 18.62759615963255655, 77.91775706135231871 ) ) ;
#78981=CARTESIAN_POINT ( 'NONE',  ( 16.53943276465976808, 0.05219959533934440121, 96.25109039468568994 ) ) ;
#78982=CARTESIAN_POINT ( 'NONE',  ( 18.67979575497194134, -10.72451020669871369, 25.83442372801901499 ) ) ;
#78983=CARTESIAN_POINT ( 'NONE',  ( -5.823673210054431948, 21.52544592524334988, 32.70942372801900433 ) ) ;
#78984=CARTESIAN_POINT ( 'NONE',  ( -5.049401038297874678, -19.05341960407617918, 59.79275706135231871 ) ) ;
#78985=CARTESIAN_POINT ( 'NONE',  ( 9.564922557960805705, 16.46253265017160317, 84.58224293864769550 ) ) ;
#78986=CARTESIAN_POINT ( 'NONE',  ( -0.05219959533937732626, 21.53943276465977519, 77.50109039468567573 ) ) ;
#78988=CARTESIAN_POINT ( 'NONE',  ( 15.72974639402199770, -15.80617190586745480, 83.12390960531436690 ) ) ;
#78989=CARTESIAN_POINT ( 'NONE',  ( 16.53943276465976808, -0.05219959533910856209, 63.74890960531435979 ) ) ;
#78990=CARTESIAN_POINT ( 'NONE',  ( -21.52544592524334988, -5.823673210054445271, 98.95942372801903275 ) ) ;
#78991=CARTESIAN_POINT ( 'NONE',  ( -8.224510206698948167, 14.34966873604960824, 85.41557627198102409 ) ) ;
#78992=CARTESIAN_POINT ( 'NONE',  ( -19.03943276465977164, 0.05219959533909376836, 41.24890960531435269 ) ) ;
#78993=CARTESIAN_POINT ( 'NONE',  ( -13.89961937509957401, -13.97604488694547875, 69.37609039468564731 ) ) ;
#78994=CARTESIAN_POINT ( 'NONE',  ( 4.483927247898545687, 16.52544592524342804, 34.79057627198103120 ) ) ;
#78995=CARTESIAN_POINT ( 'NONE',  ( -18.67979575497193778, 10.72451020669871902, 98.33442372801901854 ) ) ;
#78996=CARTESIAN_POINT ( 'NONE',  ( 13.97604488694527802, 13.89961937509977652, 94.37390960531436690 ) ) ;
#78997=CARTESIAN_POINT ( 'NONE',  ( 19.03943276465977164, 0.05219959533936151252, 66.25109039468567573 ) ) ;
#78998=CARTESIAN_POINT ( 'NONE',  ( -21.53943276465977519, 0.05219959533907696930, 71.24890960531435269 ) ) ;
#78999=CARTESIAN_POINT ( 'NONE',  ( -21.53943276465977519, -0.05219959533937600094, 18.75109039468568639 ) ) ;
#79000=CARTESIAN_POINT ( 'NONE',  ( 5.049401038297881783, 19.05341960407617563, 112.2927570613523471 ) ) ;
#79001=CARTESIAN_POINT ( 'NONE',  ( -12.14591786802326823, 12.06949235617739902, 83.12609039468568994 ) ) ;
#79003=CARTESIAN_POINT ( 'NONE',  ( -10.72451020669870658, -18.67979575497194134, 19.58442372801901143 ) ) ;
#79004=CARTESIAN_POINT ( 'NONE',  ( 16.52544592524342804, -4.483927247898539470, 108.5405762719810241 ) ) ;
#79006=CARTESIAN_POINT ( 'NONE',  ( -14.34966873604972548, 8.224510206698743886, 33.33442372801900433 ) ) ;
#79007=CARTESIAN_POINT ( 'NONE',  ( 10.72451020669898902, -18.67979575497178502, 62.91557627198102409 ) ) ;
#79008=CARTESIAN_POINT ( 'NONE',  ( 14.29746914071037800, 8.314922557961029526, 106.6677570613523756 ) ) ;
#79009=CARTESIAN_POINT ( 'NONE',  ( 14.29746914071037800, 8.314922557961029526, 36.66775706135234714 ) ) ;
#79010=CARTESIAN_POINT ( 'NONE',  ( -5.049401038298153566, 19.05341960407611168, 30.20724293864768839 ) ) ;
#79011=CARTESIAN_POINT ( 'NONE',  ( 16.53943276465976808, 0.05219959533934440121, 81.25109039468568994 ) ) ;
#79012=CARTESIAN_POINT ( 'NONE',  ( -19.03943276465977164, -0.05219959533935918106, 73.75109039468566152 ) ) ;
#79013=CARTESIAN_POINT ( 'NONE',  ( -5.823673210054116645, -21.52544592524344225, 72.29057627198102409 ) ) ;
#79014=CARTESIAN_POINT ( 'NONE',  ( -14.29746914071037622, -8.314922557961029526, 104.1677570613523471 ) ) ;
#79015=CARTESIAN_POINT ( 'NONE',  ( -0.05219959533937732626, 21.53943276465977519, 82.50109039468568994 ) ) ;
#79016=CARTESIAN_POINT ( 'NONE',  ( 5.719274019375991003, -21.55341960407610458, 62.70724293864769550 ) ) ;
#79017=CARTESIAN_POINT ( 'NONE',  ( 21.52544592524344225, -5.823673210054117533, 53.54057627198103120 ) ) ;
#79018=ORIENTED_EDGE ( 'NONE', *, *, #43792, .T. ) ;
#79019=CARTESIAN_POINT ( 'NONE',  ( -14.29746914071037622, -8.314922557961029526, 84.16775706135234714 ) ) ;
#79020=CARTESIAN_POINT ( 'NONE',  ( 10.81492255796078972, 18.62759615963270932, 49.58224293864769550 ) ) ;
#79022=CARTESIAN_POINT ( 'NONE',  ( 9.474510206698971260, -16.51473224551069308, 112.9155762719810383 ) ) ;
#79024=CARTESIAN_POINT ( 'NONE',  ( 16.51473224551069308, 9.474510206698969483, 29.16557627198103475 ) ) ;
#79025=CARTESIAN_POINT ( 'NONE',  ( -0.05219959533907301413, -21.53943276465977519, 62.49890960531436690 ) ) ;
#79026=CARTESIAN_POINT ( 'NONE',  ( -12.06949235617739369, -12.14591786802326823, 104.3760903946856899 ) ) ;
#79027=CARTESIAN_POINT ( 'NONE',  ( 10.81492255796106328, -18.62759615963255655, 40.41775706135234714 ) ) ;
#79028=CARTESIAN_POINT ( 'NONE',  ( -9.564922557961040184, 16.46253265017147172, 97.91775706135233293 ) ) ;
#79029=CARTESIAN_POINT ( 'NONE',  ( -16.52544592524342804, 4.483927247898546575, 116.0405762719810383 ) ) ;
#79030=CARTESIAN_POINT ( 'NONE',  ( -16.51473224551082808, 9.474510206698731452, 113.3344237280190043 ) ) ;
#79031=CARTESIAN_POINT ( 'NONE',  ( -16.51473224551069308, -9.474510206698971260, 46.66557627198102409 ) ) ;
#79034=CARTESIAN_POINT ( 'NONE',  ( 9.474510206698971260, -16.51473224551069308, 87.91557627198102409 ) ) ;
#79035=CARTESIAN_POINT ( 'NONE',  ( 4.483927247898790824, -16.52544592524335698, 75.20942372801901854 ) ) ;
#79036=CARTESIAN_POINT ( 'NONE',  ( -9.474510206698720793, -16.51473224551083518, 79.58442372801899012 ) ) ;
#79037=CARTESIAN_POINT ( 'NONE',  ( -0.05219959533936034679, 19.03943276465977164, 22.50109039468566152 ) ) ;
#79038=CARTESIAN_POINT ( 'NONE',  ( -21.52544592524343514, 5.823673210054127303, 66.04057627198103830 ) ) ;
#79039=CARTESIAN_POINT ( 'NONE',  ( 16.52544592524335698, 4.483927247898782831, 91.45942372801901854 ) ) ;
#79040=CARTESIAN_POINT ( 'NONE',  ( -13.89961937509957401, -13.97604488694547875, 84.37609039468567573 ) ) ;
#79041=CARTESIAN_POINT ( 'NONE',  ( 9.564922557960805705, 16.46253265017160317, 34.58224293864770260 ) ) ;
#79042=CARTESIAN_POINT ( 'NONE',  ( -13.97604488694527625, -13.89961937509977652, 81.87390960531436690 ) ) ;
#79044=CARTESIAN_POINT ( 'NONE',  ( 18.67979575497194134, -10.72451020669871369, 50.83442372801901143 ) ) ;
#79045=CARTESIAN_POINT ( 'NONE',  ( 19.02544592524343514, -5.153800228976328945, 53.54057627198102409 ) ) ;
#79046=CARTESIAN_POINT ( 'NONE',  ( -19.03943276465977164, -0.05219959533935918106, 68.75109039468566152 ) ) ;
#79048=CARTESIAN_POINT ( 'NONE',  ( 9.564922557960805705, 16.46253265017160317, 114.5822429386476955 ) ) ;
#79049=CARTESIAN_POINT ( 'NONE',  ( 0.05219959533910956823, 16.53943276465976808, 69.99890960531435269 ) ) ;
#79050=CARTESIAN_POINT ( 'NONE',  ( -10.81492255796078084, -18.62759615963271287, 62.08224293864769550 ) ) ;
#79051=CARTESIAN_POINT ( 'NONE',  ( 19.96322699617726570, -3.697860406115397680, 102.5000000000000568 ) ) ;
#79053=CARTESIAN_POINT ( 'NONE',  ( -19.02544592524334988, -5.153800228976617603, 28.95942372801900433 ) ) ;
#79054=CARTESIAN_POINT ( 'NONE',  ( -17.49999999999999645, 5.499999999999992895, 88.71769037696435589 ) ) ;
#79055=CARTESIAN_POINT ( 'NONE',  ( -9.564922557960796823, -16.46253265017161027, 67.08224293864769550 ) ) ;
#79056=CARTESIAN_POINT ( 'NONE',  ( 19.05341960407611168, 5.049401038298154454, 78.95724293864769550 ) ) ;
#79057=CARTESIAN_POINT ( 'NONE',  ( -0.05219959533934338120, 16.53943276465976808, 52.50109039468567573 ) ) ;
#79060=CARTESIAN_POINT ( 'NONE',  ( 4.483927247898790824, -16.52544592524335698, 90.20942372801903275 ) ) ;
#79062=CARTESIAN_POINT ( 'NONE',  ( 12.06949235617739724, 12.14591786802326823, 71.87609039468568994 ) ) ;
#79063=CARTESIAN_POINT ( 'NONE',  ( -12.14591786802326823, 12.06949235617739902, 43.12609039468568284 ) ) ;
#79064=CARTESIAN_POINT ( 'NONE',  ( 5.153800228976335163, 19.02544592524342804, 54.79057627198103120 ) ) ;
#79066=CARTESIAN_POINT ( 'NONE',  ( -21.52544592524334988, -5.823673210054445271, 53.95942372801900433 ) ) ;
#79067=CARTESIAN_POINT ( 'NONE',  ( 5.153800228976615827, -19.02544592524334988, 65.20942372801900433 ) ) ;
#79068=CARTESIAN_POINT ( 'NONE',  ( -18.62759615963255300, -10.81492255796106328, 109.1677570613523613 ) ) ;
#79069=CARTESIAN_POINT ( 'NONE',  ( -9.474510206698964154, 16.51473224551069663, 25.41557627198103120 ) ) ;
#79071=CARTESIAN_POINT ( 'NONE',  ( 10.72451020669898902, -18.67979575497178502, 52.91557627198103830 ) ) ;
#79072=AXIS2_PLACEMENT_3D ( 'NONE', #158135, #127784, #128776 ) ;
#79073=CARTESIAN_POINT ( 'NONE',  ( -5.153800228976328057, -19.02544592524343514, 112.2905762719810099 ) ) ;
#79074=CARTESIAN_POINT ( 'NONE',  ( -16.52544592524342804, 4.483927247898546575, 96.04057627198102409 ) ) ;
#79075=CARTESIAN_POINT ( 'NONE',  ( 4.483927247898790824, -16.52544592524335698, 40.20942372801901854 ) ) ;
#79076=CARTESIAN_POINT ( 'NONE',  ( -16.53943276465976808, 0.05219959533911058130, 31.24890960531435979 ) ) ;
#79077=ORIENTED_EDGE ( 'NONE', *, *, #100282, .F. ) ;
#79078=CARTESIAN_POINT ( 'NONE',  ( 15.72974639402176855, 15.80617190586768217, 21.87609039468567573 ) ) ;
#79079=CARTESIAN_POINT ( 'NONE',  ( -4.379528057220328563, 16.55341960407611168, 45.20724293864769550 ) ) ;
#79080=CARTESIAN_POINT ( 'NONE',  ( -5.153800228976328057, -19.02544592524343514, 112.2905762719810099 ) ) ;
#79081=CARTESIAN_POINT ( 'NONE',  ( 19.02544592524334988, 5.153800228976608722, 101.4594237280189759 ) ) ;
#79082=CARTESIAN_POINT ( 'NONE',  ( 16.51473224551083163, -9.474510206698727899, 30.83442372801900433 ) ) ;
#79083=CARTESIAN_POINT ( 'NONE',  ( 0.05219959533910956823, 16.53943276465976808, 34.99890960531435979 ) ) ;
#79084=CARTESIAN_POINT ( 'NONE',  ( 5.719274019375991003, -21.55341960407610458, 107.7072429386476955 ) ) ;
#79085=CARTESIAN_POINT ( 'NONE',  ( 15.80617190586746368, 15.72974639402197994, 59.37390960531436690 ) ) ;
#79086=CARTESIAN_POINT ( 'NONE',  ( 16.46253265017160672, -9.564922557960803928, 73.33224293864769550 ) ) ;
#79087=CARTESIAN_POINT ( 'NONE',  ( 4.483927247898545687, 16.52544592524342804, 44.79057627198103120 ) ) ;
#79088=CARTESIAN_POINT ( 'NONE',  ( -5.049401038298153566, 19.05341960407611168, 95.20724293864770971 ) ) ;
#79089=CARTESIAN_POINT ( 'NONE',  ( 18.56399227203345603, 5.499999999999817923, 56.47830131249901342 ) ) ;
#79090=CARTESIAN_POINT ( 'NONE',  ( 9.474510206698729675, 16.51473224551082808, 42.08442372801900433 ) ) ;
#79091=CARTESIAN_POINT ( 'NONE',  ( 5.823673210054125526, 21.52544592524343514, 89.79057627198103830 ) ) ;
#79092=CARTESIAN_POINT ( 'NONE',  ( 0.05219959533910956823, 16.53943276465976808, 94.99890960531436690 ) ) ;
#79093=CARTESIAN_POINT ( 'NONE',  ( -10.81492255796105439, 18.62759615963255655, 32.91775706135234714 ) ) ;
#79095=CARTESIAN_POINT ( 'NONE',  ( 0.05219959533910956823, 16.53943276465976808, 24.99890960531435624 ) ) ;
#79096=CARTESIAN_POINT ( 'NONE',  ( -16.46253265017160317, 9.564922557960807481, 30.83224293864769550 ) ) ;
#79097=CARTESIAN_POINT ( 'NONE',  ( 9.564922557960805705, 16.46253265017160317, 89.58224293864769550 ) ) ;
#79098=CARTESIAN_POINT ( 'NONE',  ( 18.62759615963271287, -10.81492255796078972, 63.33224293864770260 ) ) ;
#79100=CARTESIAN_POINT ( 'NONE',  ( -16.46253265017160317, 9.564922557960807481, 25.83224293864769194 ) ) ;
#79101=CARTESIAN_POINT ( 'NONE',  ( -0.05219959533907301413, -21.53943276465977519, 57.49890960531435979 ) ) ;
#79102=CARTESIAN_POINT ( 'NONE',  ( -18.67979575497193778, 10.72451020669871902, 68.33442372801900433 ) ) ;
#79104=CARTESIAN_POINT ( 'NONE',  ( -16.53943276465976808, -0.05219959533934237506, 63.75109039468568284 ) ) ;
#79105=CARTESIAN_POINT ( 'NONE',  ( -5.049401038298153566, 19.05341960407611168, 55.20724293864769550 ) ) ;
#79106=CARTESIAN_POINT ( 'NONE',  ( 19.05341960407611168, 5.049401038298154454, 68.95724293864769550 ) ) ;
#79108=CARTESIAN_POINT ( 'NONE',  ( 18.67979575497194134, -10.72451020669871369, 105.8344237280190328 ) ) ;
#79109=CARTESIAN_POINT ( 'NONE',  ( 14.29746914071037800, 8.314922557961029526, 71.66775706135234714 ) ) ;
#79110=CARTESIAN_POINT ( 'NONE',  ( 10.81492255796106328, -18.62759615963255655, 100.4177570613523471 ) ) ;
#79111=CARTESIAN_POINT ( 'NONE',  ( -19.05341960407611168, -5.049401038298163336, 61.45724293864769550 ) ) ;
#79112=CARTESIAN_POINT ( 'NONE',  ( 21.52544592524344225, -5.823673210054117533, 28.54057627198103120 ) ) ;
#79113=CARTESIAN_POINT ( 'NONE',  ( -16.51473224551082808, 9.474510206698731452, 103.3344237280190043 ) ) ;
#79114=CARTESIAN_POINT ( 'NONE',  ( -18.67979575497193778, 10.72451020669871902, 88.33442372801901854 ) ) ;
#79115=CARTESIAN_POINT ( 'NONE',  ( -12.14591786802326823, 12.06949235617739902, 43.12609039468568284 ) ) ;
#79117=CARTESIAN_POINT ( 'NONE',  ( 15.72974639402199770, -15.80617190586745480, 93.12390960531436690 ) ) ;
#79118=CARTESIAN_POINT ( 'NONE',  ( -5.153800228976607833, 19.02544592524334988, 102.7094237280189759 ) ) ;
#79119=CARTESIAN_POINT ( 'NONE',  ( -13.97604488694527625, -13.89961937509977652, 71.87390960531433848 ) ) ;
#79120=CARTESIAN_POINT ( 'NONE',  ( -19.02544592524334988, -5.153800228976617603, 108.9594237280189759 ) ) ;
#79121=CARTESIAN_POINT ( 'NONE',  ( -9.474510206698964154, 16.51473224551069663, 35.41557627198102409 ) ) ;
#79122=CARTESIAN_POINT ( 'NONE',  ( 4.379528057220092307, 16.55341960407617563, 22.29275706135235069 ) ) ;
#79123=CARTESIAN_POINT ( 'NONE',  ( 16.53943276465976808, -0.05219959533910856209, 63.74890960531435979 ) ) ;
#79124=CARTESIAN_POINT ( 'NONE',  ( -16.53943276465976808, -0.05219959533934237506, 78.75109039468568994 ) ) ;
#79125=CARTESIAN_POINT ( 'NONE',  ( 18.62759615963255655, 10.81492255796105972, 31.66775706135234358 ) ) ;
#79126=CARTESIAN_POINT ( 'NONE',  ( -5.049401038298153566, 19.05341960407611168, 45.20724293864769550 ) ) ;
#79127=CARTESIAN_POINT ( 'NONE',  ( -13.89961937509977652, 13.97604488694528158, 70.62390960531432427 ) ) ;
#79128=CARTESIAN_POINT ( 'NONE',  ( -8.224510206698735004, -14.34966873604973081, 69.58442372801900433 ) ) ;
#79132=CARTESIAN_POINT ( 'NONE',  ( 15.72974639402176855, 15.80617190586768217, 111.8760903946856615 ) ) ;
#79133=CARTESIAN_POINT ( 'NONE',  ( 16.51473224551069308, 9.474510206698969483, 39.16557627198103120 ) ) ;
#79134=CARTESIAN_POINT ( 'NONE',  ( -19.03943276465977164, 0.05219959533909376836, 96.24890960531436690 ) ) ;
#79136=CARTESIAN_POINT ( 'NONE',  ( -8.224510206698735004, -14.34966873604973081, 29.58442372801901854 ) ) ;
#79137=CARTESIAN_POINT ( 'NONE',  ( 19.02544592524334988, 5.153800228976608722, 41.45942372801900433 ) ) ;
#79138=CARTESIAN_POINT ( 'NONE',  ( 14.34966873604972726, -8.224510206698740333, 45.83442372801901854 ) ) ;
#79139=CARTESIAN_POINT ( 'NONE',  ( -5.153800228976328057, -19.02544592524343514, 47.29057627198102409 ) ) ;
#79140=CARTESIAN_POINT ( 'NONE',  ( -9.474510206698964154, 16.51473224551069663, 100.4155762719810241 ) ) ;
#79141=CARTESIAN_POINT ( 'NONE',  ( -13.89961937509977652, 13.97604488694528158, 65.62390960531436690 ) ) ;
#79142=CARTESIAN_POINT ( 'NONE',  ( 10.81492255796078972, 18.62759615963270932, 99.58224293864770971 ) ) ;
#79143=CARTESIAN_POINT ( 'NONE',  ( -9.474510206698964154, 16.51473224551069663, 80.41557627198103830 ) ) ;
#79144=CARTESIAN_POINT ( 'NONE',  ( 19.05341960407611168, 5.049401038298154454, 108.9572429386477097 ) ) ;
#79145=CARTESIAN_POINT ( 'NONE',  ( 13.89961937509977652, -13.97604488694527269, 68.12390960531436690 ) ) ;
#79147=CARTESIAN_POINT ( 'NONE',  ( -16.51473224551082808, 9.474510206698731452, 93.33442372801900433 ) ) ;
#79149=CARTESIAN_POINT ( 'NONE',  ( -5.049401038297874678, -19.05341960407617918, 19.79275706135233293 ) ) ;
#79150=CARTESIAN_POINT ( 'NONE',  ( 0.05219959533910956823, 16.53943276465976808, 64.99890960531435269 ) ) ;
#79151=CARTESIAN_POINT ( 'NONE',  ( 18.67979575497194134, -10.72451020669871369, 90.83442372801901854 ) ) ;
#79152=CARTESIAN_POINT ( 'NONE',  ( -13.97604488694527625, -13.89961937509977652, 21.87390960531435979 ) ) ;
#79153=CARTESIAN_POINT ( 'NONE',  ( -16.55341960407617563, 4.379528057220093196, 113.5427570613523756 ) ) ;
#79154=CARTESIAN_POINT ( 'NONE',  ( 15.80617190586769283, -15.72974639402175789, 95.62609039468568994 ) ) ;
#79155=CARTESIAN_POINT ( 'NONE',  ( -13.89961937509977652, 13.97604488694528158, 80.62390960531436690 ) ) ;
#79156=CARTESIAN_POINT ( 'NONE',  ( -5.719274019375665041, -21.55341960407619695, 49.79275706135234714 ) ) ;
#79157=CARTESIAN_POINT ( 'NONE',  ( -9.564922557960796823, -16.46253265017161027, 82.08224293864768129 ) ) ;
#79158=CARTESIAN_POINT ( 'NONE',  ( -4.379528057220328563, 16.55341960407611168, 95.20724293864769550 ) ) ;
#79159=CARTESIAN_POINT ( 'NONE',  ( -16.55341960407611168, -4.379528057220339221, 61.45724293864770260 ) ) ;
#79160=CARTESIAN_POINT ( 'NONE',  ( -18.67979575497178146, -10.72451020669898902, 71.66557627198100988 ) ) ;
#79161=CARTESIAN_POINT ( 'NONE',  ( 5.049401038298161559, -19.05341960407611168, 72.70724293864768129 ) ) ;
#79162=CARTESIAN_POINT ( 'NONE',  ( -15.72974639402197994, 15.80617190586746368, 90.62390960531436690 ) ) ;
#79164=CARTESIAN_POINT ( 'NONE',  ( 13.89961937509957401, 13.97604488694547697, 81.87609039468564731 ) ) ;
#79165=CARTESIAN_POINT ( 'NONE',  ( -18.22780087662124160, -5.499999999999927169, 88.98236817873107896 ) ) ;
#79166=CARTESIAN_POINT ( 'NONE',  ( -14.29746914071049879, 8.314922557960819915, 70.83224293864770971 ) ) ;
#79167=CARTESIAN_POINT ( 'NONE',  ( 13.97604488694527802, 13.89961937509977652, 54.37390960531435979 ) ) ;
#79168=CARTESIAN_POINT ( 'NONE',  ( 18.67979575497178502, 10.72451020669898547, 64.16557627198102409 ) ) ;
#79170=CARTESIAN_POINT ( 'NONE',  ( 8.224510206698742110, 14.34966873604972548, 107.0844237280190043 ) ) ;
#79172=CARTESIAN_POINT ( 'NONE',  ( 9.564922557961047289, -16.46253265017146816, 95.41775706135233293 ) ) ;
#79173=CARTESIAN_POINT ( 'NONE',  ( 8.314922557960818139, 14.29746914071049879, 84.58224293864769550 ) ) ;
#79175=CARTESIAN_POINT ( 'NONE',  ( 0.05219959533909260263, 19.03943276465977164, 79.99890960531436690 ) ) ;
#79176=CARTESIAN_POINT ( 'NONE',  ( -5.153800228976328057, -19.02544592524343514, 32.29057627198102409 ) ) ;
#79177=CARTESIAN_POINT ( 'NONE',  ( 0.05219959533910956823, 16.53943276465976808, 69.99890960531435269 ) ) ;
#79178=CARTESIAN_POINT ( 'NONE',  ( -16.51473224551069308, -9.474510206698971260, 96.66557627198102409 ) ) ;
#79179=CARTESIAN_POINT ( 'NONE',  ( -9.564922557961040184, 16.46253265017147172, 87.91775706135233293 ) ) ;
#79180=CARTESIAN_POINT ( 'NONE',  ( -19.03943276465977164, 0.05219959533909376836, 71.24890960531435269 ) ) ;
#79182=CARTESIAN_POINT ( 'NONE',  ( -13.89961937509977652, 13.97604488694528158, 90.62390960531432427 ) ) ;
#79183=CARTESIAN_POINT ( 'NONE',  ( 5.719274019375991003, -21.55341960407610458, 82.70724293864770971 ) ) ;
#79184=CARTESIAN_POINT ( 'NONE',  ( -0.05219959533934338120, 16.53943276465976808, 67.50109039468568994 ) ) ;
#79185=CARTESIAN_POINT ( 'NONE',  ( -9.474510206698720793, -16.51473224551083518, 109.5844237280190043 ) ) ;
#79186=CARTESIAN_POINT ( 'NONE',  ( 19.03943276465977164, -0.05219959533909143690, 63.74890960531435979 ) ) ;
#79187=CARTESIAN_POINT ( 'NONE',  ( -5.823673210054116645, -21.52544592524344225, 72.29057627198102409 ) ) ;
#79188=CARTESIAN_POINT ( 'NONE',  ( 5.153800228976615827, -19.02544592524334988, 95.20942372801897591 ) ) ;
#79189=CARTESIAN_POINT ( 'NONE',  ( -0.05219959533910754901, -16.53943276465976808, 37.49890960531436690 ) ) ;
#79190=CARTESIAN_POINT ( 'NONE',  ( 15.72974639402176855, 15.80617190586768217, 46.87609039468568994 ) ) ;
#79192=CARTESIAN_POINT ( 'NONE',  ( 18.22780087662122739, 5.500000000000000888, 71.48236817873106475 ) ) ;
#79193=CARTESIAN_POINT ( 'NONE',  ( 0.05219959533934541429, -16.53943276465976808, 70.00109039468568994 ) ) ;
#79194=CARTESIAN_POINT ( 'NONE',  ( 13.97604488694527802, 13.89961937509977652, 109.3739096053143669 ) ) ;
#79196=CARTESIAN_POINT ( 'NONE',  ( -17.31728774477275579, -6.344390552232334279, 34.18093348310681989 ) ) ;
#79197=CARTESIAN_POINT ( 'NONE',  ( 14.29746914071037800, 8.314922557961029526, 96.66775706135234714 ) ) ;
#79198=CARTESIAN_POINT ( 'NONE',  ( -0.05219959533934338120, 16.53943276465976808, 32.50109039468568284 ) ) ;
#79199=CARTESIAN_POINT ( 'NONE',  ( -16.51473224551069308, -9.474510206698971260, 51.66557627198102409 ) ) ;
#79200=CARTESIAN_POINT ( 'NONE',  ( -0.05219959533909027116, -19.03943276465977164, 47.49890960531435979 ) ) ;
#79201=CARTESIAN_POINT ( 'NONE',  ( -9.564922557960796823, -16.46253265017161027, 62.08224293864769550 ) ) ;
#79202=CARTESIAN_POINT ( 'NONE',  ( 0.05219959533937995610, -21.53943276465977519, 55.00109039468568284 ) ) ;
#79203=CARTESIAN_POINT ( 'NONE',  ( -14.34966873604972548, 8.224510206698743886, 68.33442372801900433 ) ) ;
#79204=CARTESIAN_POINT ( 'NONE',  ( -8.314922557960811034, -14.29746914071050412, 32.08224293864769550 ) ) ;
#79205=CARTESIAN_POINT ( 'NONE',  ( -9.474510206698964154, 16.51473224551069663, 40.41557627198103120 ) ) ;
#79206=CARTESIAN_POINT ( 'NONE',  ( -5.049401038298153566, 19.05341960407611168, 30.20724293864768839 ) ) ;
#79207=CARTESIAN_POINT ( 'NONE',  ( 8.314922557961029526, -14.29746914071037800, 25.41775706135235779 ) ) ;
#79208=CARTESIAN_POINT ( 'NONE',  ( 19.03943276465977164, 0.05219959533936151252, 81.25109039468567573 ) ) ;
#79209=CARTESIAN_POINT ( 'NONE',  ( -16.52544592524342804, 4.483927247898546575, 81.04057627198102409 ) ) ;
#79210=CARTESIAN_POINT ( 'NONE',  ( -19.03943276465977164, 0.05219959533909376836, 56.24890960531435979 ) ) ;
#79211=CARTESIAN_POINT ( 'NONE',  ( -9.474510206698720793, -16.51473224551083518, 89.58442372801900433 ) ) ;
#79213=CARTESIAN_POINT ( 'NONE',  ( -10.81492255796105439, 18.62759615963255655, 87.91775706135234714 ) ) ;
#79214=CARTESIAN_POINT ( 'NONE',  ( 14.34966873604972726, -8.224510206698740333, 50.83442372801901143 ) ) ;
#79215=CARTESIAN_POINT ( 'NONE',  ( 17.26058549869090086, 6.457015423128631859, 38.87745837476068544 ) ) ;
#79216=CARTESIAN_POINT ( 'NONE',  ( 21.55341960407610458, 5.719274019375980345, 43.95724293864769550 ) ) ;
#79217=CARTESIAN_POINT ( 'NONE',  ( 8.314922557961029526, -14.29746914071037800, 45.41775706135234003 ) ) ;
#79219=CARTESIAN_POINT ( 'NONE',  ( -19.05341960407617563, 5.049401038297882671, 23.54275706135233648 ) ) ;
#79220=CARTESIAN_POINT ( 'NONE',  ( -16.51473224551069308, -9.474510206698971260, 81.66557627198103830 ) ) ;
#79222=CARTESIAN_POINT ( 'NONE',  ( 5.049401038298161559, -19.05341960407611168, 52.70724293864767418 ) ) ;
#79225=CARTESIAN_POINT ( 'NONE',  ( -5.153800228976328057, -19.02544592524343514, 72.29057627198102409 ) ) ;
#79226=CARTESIAN_POINT ( 'NONE',  ( -19.39056639909671986, -5.500000000000052403, 55.78948781074346641 ) ) ;
#79227=CARTESIAN_POINT ( 'NONE',  ( -5.049401038297874678, -19.05341960407617918, 24.79275706135233648 ) ) ;
#79228=CARTESIAN_POINT ( 'NONE',  ( -19.03943276465977164, -0.05219959533935918106, 18.75109039468567218 ) ) ;
#79229=CARTESIAN_POINT ( 'NONE',  ( -8.224510206698948167, 14.34966873604960824, 35.41557627198102409 ) ) ;
#79230=CARTESIAN_POINT ( 'NONE',  ( -9.474510206698964154, 16.51473224551069663, 40.41557627198103120 ) ) ;
#79231=CARTESIAN_POINT ( 'NONE',  ( 19.02544592524343514, -5.153800228976328945, 108.5405762719810383 ) ) ;
#79232=CARTESIAN_POINT ( 'NONE',  ( -15.72974639402176322, -15.80617190586768395, 69.37609039468567573 ) ) ;
#79233=CARTESIAN_POINT ( 'NONE',  ( -19.05341960407611168, -5.049401038298163336, 46.45724293864768129 ) ) ;
#79234=CARTESIAN_POINT ( 'NONE',  ( 10.72451020669871369, 18.67979575497193778, 77.08442372801901854 ) ) ;
#79235=CARTESIAN_POINT ( 'NONE',  ( 15.80617190586746368, 15.72974639402197994, 29.37390960531435269 ) ) ;
#79236=CARTESIAN_POINT ( 'NONE',  ( 0.05219959533909260263, 19.03943276465977164, 34.99890960531435979 ) ) ;
#79237=CARTESIAN_POINT ( 'NONE',  ( 5.823673210054444382, -21.52544592524334988, 30.20942372801902565 ) ) ;
#79238=CARTESIAN_POINT ( 'NONE',  ( 9.474510206698729675, 16.51473224551082808, 47.08442372801900433 ) ) ;
#79239=CARTESIAN_POINT ( 'NONE',  ( 5.049401038298161559, -19.05341960407611168, 32.70724293864768129 ) ) ;
#79240=CARTESIAN_POINT ( 'NONE',  ( -9.564922557960796823, -16.46253265017161027, 72.08224293864770971 ) ) ;
#79241=CARTESIAN_POINT ( 'NONE',  ( 16.51473224551083163, -9.474510206698727899, 105.8344237280190043 ) ) ;
#79242=CARTESIAN_POINT ( 'NONE',  ( -12.14591786802309592, -12.06949235617757132, 76.87390960531439532 ) ) ;
#79243=CARTESIAN_POINT ( 'NONE',  ( 5.719274019375991003, -21.55341960407610458, 32.70724293864770260 ) ) ;
#79244=CARTESIAN_POINT ( 'NONE',  ( -0.05219959533936034679, 19.03943276465977164, 97.50109039468567573 ) ) ;
#79245=CARTESIAN_POINT ( 'NONE',  ( 21.53943276465977519, -0.05219959533907433946, 108.7489096053143669 ) ) ;
#79246=CARTESIAN_POINT ( 'NONE',  ( 10.72451020669871369, 18.67979575497193778, 62.08442372801901143 ) ) ;
#79247=CARTESIAN_POINT ( 'NONE',  ( -16.52544592524335698, -4.483927247898792601, 58.95942372801902565 ) ) ;
#79248=CARTESIAN_POINT ( 'NONE',  ( -4.379528057220086978, -16.55341960407618274, 49.79275706135234714 ) ) ;
#79249=CARTESIAN_POINT ( 'NONE',  ( 18.62759615963271287, -10.81492255796078972, 73.33224293864769550 ) ) ;
#79250=CARTESIAN_POINT ( 'NONE',  ( -13.89961937509977652, 13.97604488694528158, 45.62390960531433848 ) ) ;
#79251=CARTESIAN_POINT ( 'NONE',  ( -16.52544592524335698, -4.483927247898792601, 93.95942372801903275 ) ) ;
#79252=CARTESIAN_POINT ( 'NONE',  ( 5.719274019375991003, -21.55341960407610458, 97.70724293864772392 ) ) ;
#79253=CARTESIAN_POINT ( 'NONE',  ( 16.53943276465976808, -0.05219959533910856209, 58.74890960531436690 ) ) ;
#79254=CARTESIAN_POINT ( 'NONE',  ( -19.03943276465977164, 0.05219959533909376836, 71.24890960531435269 ) ) ;
#79255=CARTESIAN_POINT ( 'NONE',  ( -16.52544592524335698, -4.483927247898792601, 78.95942372801901854 ) ) ;
#79256=CARTESIAN_POINT ( 'NONE',  ( -9.564922557961040184, 16.46253265017147172, 112.9177570613523329 ) ) ;
#79257=CARTESIAN_POINT ( 'NONE',  ( -0.05219959533907301413, -21.53943276465977519, 112.4989096053143669 ) ) ;
#79258=CARTESIAN_POINT ( 'NONE',  ( -12.06949235617756955, 12.14591786802309770, 40.62390960531435269 ) ) ;
#79260=CARTESIAN_POINT ( 'NONE',  ( -16.31925111598456013, 7.325300261831604764, 75.16424538967253000 ) ) ;
#79261=CARTESIAN_POINT ( 'NONE',  ( 15.80617190586746368, 15.72974639402197994, 89.37390960531435269 ) ) ;
#79262=CARTESIAN_POINT ( 'NONE',  ( 8.314922557960818139, 14.29746914071049879, 29.58224293864769905 ) ) ;
#79263=EDGE_LOOP ( 'NONE', ( #22434, #80024, #37767, #105307, #173042, #26443, #11273, #75311, #124064, #153209, #151455, #130339, #43168, #81239, #62392, #40274, #2422, #30790, #148486, #100280, #149295, #121776, #41285, #175376, #147038, #79354, #35177, #3038, #183671, #115724, #41102, #172150, #46246, #45057, #59126, #123202, #22817, #28931, #107365, #75112, #91545 ) ) ;
#79265=CARTESIAN_POINT ( 'NONE',  ( -15.80617190586745835, -15.72974639402198527, 106.8739096053143811 ) ) ;
#79267=CARTESIAN_POINT ( 'NONE',  ( -19.03943276465977164, 0.05219959533909376836, 106.2489096053143669 ) ) ;
#79268=CARTESIAN_POINT ( 'NONE',  ( -21.52544592524343514, 5.823673210054127303, 116.0405762719810383 ) ) ;
#79269=CARTESIAN_POINT ( 'NONE',  ( 8.224510206698953496, -14.34966873604960469, 52.91557627198103830 ) ) ;
#79270=CARTESIAN_POINT ( 'NONE',  ( -12.06949235617739369, -12.14591786802326823, 54.37609039468568994 ) ) ;
#79271=CARTESIAN_POINT ( 'NONE',  ( 19.05341960407611168, 5.049401038298154454, 63.95724293864769550 ) ) ;
#79272=CARTESIAN_POINT ( 'NONE',  ( 13.89961937509957401, 13.97604488694547697, 51.87609039468566863 ) ) ;
#79273=CARTESIAN_POINT ( 'NONE',  ( -5.049401038298153566, 19.05341960407611168, 80.20724293864769550 ) ) ;
#79275=CARTESIAN_POINT ( 'NONE',  ( 15.72974639402199770, -15.80617190586745480, 33.12390960531435979 ) ) ;
#79277=CARTESIAN_POINT ( 'NONE',  ( -19.05341960407611168, -5.049401038298163336, 51.45724293864770260 ) ) ;
#79278=CARTESIAN_POINT ( 'NONE',  ( -8.224510206698735004, -14.34966873604973081, 19.58442372801901143 ) ) ;
#79279=CARTESIAN_POINT ( 'NONE',  ( 9.564922557961047289, -16.46253265017146816, 70.41775706135233293 ) ) ;
#79280=CARTESIAN_POINT ( 'NONE',  ( 5.823673210054125526, 21.52544592524343514, 104.7905762719810241 ) ) ;
#79281=CARTESIAN_POINT ( 'NONE',  ( -14.34966873604960291, -8.224510206698953496, 36.66557627198103120 ) ) ;
#79282=CARTESIAN_POINT ( 'NONE',  ( -16.51473224551069308, -9.474510206698971260, 81.66557627198103830 ) ) ;
#79283=CARTESIAN_POINT ( 'NONE',  ( 0.05219959533907565091, 21.53943276465977519, 64.99890960531435269 ) ) ;
#79284=CARTESIAN_POINT ( 'NONE',  ( -18.62759615963270932, 10.81492255796079327, 100.8322429386477097 ) ) ;
#79285=CARTESIAN_POINT ( 'NONE',  ( -4.379528057220086978, -16.55341960407618274, 29.79275706135234358 ) ) ;
#79286=CARTESIAN_POINT ( 'NONE',  ( 13.97604488694527802, 13.89961937509977652, 114.3739096053143669 ) ) ;
#79287=CARTESIAN_POINT ( 'NONE',  ( -5.823673210054431948, 21.52544592524334988, 92.70942372801901854 ) ) ;
#79288=CARTESIAN_POINT ( 'NONE',  ( -19.05341960407611168, -5.049401038298163336, 81.45724293864769550 ) ) ;
#79290=CARTESIAN_POINT ( 'NONE',  ( -5.153800228976328057, -19.02544592524343514, 32.29057627198102409 ) ) ;
#79291=CARTESIAN_POINT ( 'NONE',  ( -5.049401038298153566, 19.05341960407611168, 90.20724293864766707 ) ) ;
#79292=CARTESIAN_POINT ( 'NONE',  ( 4.379528057220339221, -16.55341960407611168, 102.7072429386476955 ) ) ;
#79293=CARTESIAN_POINT ( 'NONE',  ( 19.05341960407611168, 5.049401038298154454, 63.95724293864769550 ) ) ;
#79294=CARTESIAN_POINT ( 'NONE',  ( 0.05219959533934541429, -16.53943276465976808, 20.00109039468568639 ) ) ;
#79295=CARTESIAN_POINT ( 'NONE',  ( -13.97604488694547520, 13.89961937509957934, 43.12609039468566152 ) ) ;
#79296=CARTESIAN_POINT ( 'NONE',  ( 18.62759615963255655, 10.81492255796105972, 91.66775706135234714 ) ) ;
#79297=CARTESIAN_POINT ( 'NONE',  ( -5.153800228976328057, -19.02544592524343514, 107.2905762719810383 ) ) ;
#79298=CARTESIAN_POINT ( 'NONE',  ( -8.224510206698735004, -14.34966873604973081, 94.58442372801901854 ) ) ;
#79300=CARTESIAN_POINT ( 'NONE',  ( -19.05341960407617563, 5.049401038297882671, 68.54275706135230450 ) ) ;
#79301=CARTESIAN_POINT ( 'NONE',  ( 5.049401038297881783, 19.05341960407617563, 32.29275706135233293 ) ) ;
#79302=CARTESIAN_POINT ( 'NONE',  ( 22.00000000000000000, -1.163414459189985801E-14, 92.50000000000000000 ) ) ;
#79303=CARTESIAN_POINT ( 'NONE',  ( 16.46253265017160672, -9.564922557960803928, 28.33224293864769550 ) ) ;
#79304=CARTESIAN_POINT ( 'NONE',  ( -0.05219959533910754901, -16.53943276465976808, 42.49890960531435979 ) ) ;
#79305=LINE ( 'NONE', #175302, #195302 ) ;
#79306=CARTESIAN_POINT ( 'NONE',  ( 4.483927247898790824, -16.52544592524335698, 110.2094237280190185 ) ) ;
#79308=CARTESIAN_POINT ( 'NONE',  ( 12.14591786802327356, -12.06949235617739191, 85.62609039468568994 ) ) ;
#79309=CARTESIAN_POINT ( 'NONE',  ( 13.97604488694527802, 13.89961937509977652, 39.37390960531435269 ) ) ;
#79310=CARTESIAN_POINT ( 'NONE',  ( -5.823673210054431948, 21.52544592524334988, 87.70942372801901854 ) ) ;
#79311=CARTESIAN_POINT ( 'NONE',  ( -16.51473224551082808, 9.474510206698731452, 108.3344237280190043 ) ) ;
#79312=CARTESIAN_POINT ( 'NONE',  ( 21.53943276465977519, 0.05219959533937863772, 81.25109039468568994 ) ) ;
#79313=CARTESIAN_POINT ( 'NONE',  ( 19.03943276465977164, 0.05219959533936151252, 51.25109039468567573 ) ) ;
#79314=CARTESIAN_POINT ( 'NONE',  ( -13.89961937509977652, 13.97604488694528158, 95.62390960531436690 ) ) ;
#79315=CARTESIAN_POINT ( 'NONE',  ( -5.049401038298153566, 19.05341960407611168, 75.20724293864769550 ) ) ;
#79316=CARTESIAN_POINT ( 'NONE',  ( -19.35633801406906329, 5.499999999999779732, 39.13373818172762242 ) ) ;
#79317=CARTESIAN_POINT ( 'NONE',  ( -16.53943276465976808, 0.05219959533911058130, 71.24890960531435269 ) ) ;
#79318=CARTESIAN_POINT ( 'NONE',  ( 15.72974639402199770, -15.80617190586745480, 58.12390960531435979 ) ) ;
#79319=CARTESIAN_POINT ( 'NONE',  ( -19.05341960407611168, -5.049401038298163336, 41.45724293864769550 ) ) ;
#79320=CARTESIAN_POINT ( 'NONE',  ( 10.81492255796078972, 18.62759615963270932, 89.58224293864768129 ) ) ;
#79321=CARTESIAN_POINT ( 'NONE',  ( 16.52544592524335698, 4.483927247898782831, 71.45942372801901854 ) ) ;
#79322=EDGE_LOOP ( 'NONE', ( #60124, #114868, #134001, #36784, #185899, #22115, #151761, #91433 ) ) ;
#79323=CARTESIAN_POINT ( 'NONE',  ( 9.564922557960805705, 16.46253265017160317, 49.58224293864770260 ) ) ;
#79324=CARTESIAN_POINT ( 'NONE',  ( 8.314922557960818139, 14.29746914071049879, 79.58224293864769550 ) ) ;
#79326=CARTESIAN_POINT ( 'NONE',  ( 19.03943276465977164, -0.05219959533909143690, 48.74890960531435979 ) ) ;
#79327=CARTESIAN_POINT ( 'NONE',  ( 12.14591786802309770, 12.06949235617756955, 114.3739096053143527 ) ) ;
#79328=CARTESIAN_POINT ( 'NONE',  ( -9.564922557961040184, 16.46253265017147172, 72.91775706135233293 ) ) ;
#79329=CARTESIAN_POINT ( 'NONE',  ( -16.55341960407611168, -4.379528057220339221, 76.45724293864769550 ) ) ;
#79330=CARTESIAN_POINT ( 'NONE',  ( 15.72974639402176855, 15.80617190586768217, 46.87609039468568994 ) ) ;
#79331=CARTESIAN_POINT ( 'NONE',  ( -16.51473224551069308, -9.474510206698971260, 31.66557627198102054 ) ) ;
#79332=CARTESIAN_POINT ( 'NONE',  ( -18.67979575497178146, -10.72451020669898902, 106.6655762719810383 ) ) ;
#79334=CARTESIAN_POINT ( 'NONE',  ( 16.53943276465976808, -0.05219959533910856209, 88.74890960531436690 ) ) ;
#79336=CARTESIAN_POINT ( 'NONE',  ( 0.05219959533909260263, 19.03943276465977164, 44.99890960531435979 ) ) ;
#79337=CARTESIAN_POINT ( 'NONE',  ( 19.39720447994796260, 5.499999999999971578, 47.16317477297181426 ) ) ;
#79338=CARTESIAN_POINT ( 'NONE',  ( -19.03943276465977164, -0.05219959533935918106, 93.75109039468566152 ) ) ;
#79339=CARTESIAN_POINT ( 'NONE',  ( -5.049401038298153566, 19.05341960407611168, 105.2072429386476671 ) ) ;
#79340=CARTESIAN_POINT ( 'NONE',  ( 15.72974639402176855, 15.80617190586768217, 31.87609039468567929 ) ) ;
#79341=CARTESIAN_POINT ( 'NONE',  ( -13.89961937509977652, 13.97604488694528158, 85.62390960531433848 ) ) ;
#79342=CARTESIAN_POINT ( 'NONE',  ( 9.474510206698729675, 16.51473224551082808, 72.08442372801900433 ) ) ;
#79343=CARTESIAN_POINT ( 'NONE',  ( 19.05341960407611168, 5.049401038298154454, 43.95724293864769550 ) ) ;
#79344=CARTESIAN_POINT ( 'NONE',  ( -12.14591786802309592, -12.06949235617757132, 61.87390960531436690 ) ) ;
#79345=CARTESIAN_POINT ( 'NONE',  ( 4.483927247898545687, 16.52544592524342804, 69.79057627198102409 ) ) ;
#79346=CARTESIAN_POINT ( 'NONE',  ( -5.153800228976328057, -19.02544592524343514, 72.29057627198102409 ) ) ;
#79347=CARTESIAN_POINT ( 'NONE',  ( -15.72974639402197994, 15.80617190586746368, 105.6239096053143669 ) ) ;
#79348=CARTESIAN_POINT ( 'NONE',  ( 0.05219959533909260263, 19.03943276465977164, 64.99890960531436690 ) ) ;
#79349=CARTESIAN_POINT ( 'NONE',  ( -21.52544592524334988, -5.823673210054445271, 108.9594237280190185 ) ) ;
#79350=CARTESIAN_POINT ( 'NONE',  ( -19.05341960407611168, -5.049401038298163336, 41.45724293864769550 ) ) ;
#79351=CARTESIAN_POINT ( 'NONE',  ( -4.483927247898782831, 16.52544592524335698, 112.7094237280190328 ) ) ;
#79352=CARTESIAN_POINT ( 'NONE',  ( 16.53943276465976808, -0.05219959533910856209, 108.7489096053143669 ) ) ;
#79353=CARTESIAN_POINT ( 'NONE',  ( 5.049401038297881783, 19.05341960407617563, 107.2927570613523187 ) ) ;
#79354=ORIENTED_EDGE ( 'NONE', *, *, #73579, .F. ) ;
#79355=CARTESIAN_POINT ( 'NONE',  ( -10.72451020669870658, -18.67979575497194134, 24.58442372801901499 ) ) ;
#79356=CARTESIAN_POINT ( 'NONE',  ( 5.153800228976615827, -19.02544592524334988, 50.20942372801897591 ) ) ;
#79357=CARTESIAN_POINT ( 'NONE',  ( -12.06949235617739369, -12.14591786802326823, 109.3760903946857042 ) ) ;
#79358=CARTESIAN_POINT ( 'NONE',  ( 0.05219959533907565091, 21.53943276465977519, 74.99890960531435269 ) ) ;
#79359=CARTESIAN_POINT ( 'NONE',  ( -21.52544592524343514, 5.823673210054127303, 26.04057627198103475 ) ) ;
#79360=CARTESIAN_POINT ( 'NONE',  ( 16.53943276465976808, -0.05219959533910856209, 53.74890960531437401 ) ) ;
#79361=CARTESIAN_POINT ( 'NONE',  ( 9.564922557960805705, 16.46253265017160317, 29.58224293864769550 ) ) ;
#79362=CARTESIAN_POINT ( 'NONE',  ( -13.89961937509977652, 13.97604488694528158, 40.62390960531435979 ) ) ;
#79363=CARTESIAN_POINT ( 'NONE',  ( -9.564922557961040184, 16.46253265017147172, 32.91775706135233293 ) ) ;
#79364=CARTESIAN_POINT ( 'NONE',  ( 8.314922557961029526, -14.29746914071037800, 95.41775706135234714 ) ) ;
#79365=CARTESIAN_POINT ( 'NONE',  ( -0.05219959533934338120, 16.53943276465976808, 57.50109039468568994 ) ) ;
#79366=CARTESIAN_POINT ( 'NONE',  ( -16.46253265017160317, 9.564922557960807481, 115.8322429386477097 ) ) ;
#79367=CARTESIAN_POINT ( 'NONE',  ( 5.153800228976335163, 19.02544592524342804, 59.79057627198100988 ) ) ;
#79368=CARTESIAN_POINT ( 'NONE',  ( -21.52544592524334988, -5.823673210054445271, 108.9594237280190185 ) ) ;
#79369=CARTESIAN_POINT ( 'NONE',  ( -13.89961937509977652, 13.97604488694528158, 80.62390960531436690 ) ) ;
#79370=VECTOR ( 'NONE', #85780, 1000.000000000000000 ) ;
#79371=CARTESIAN_POINT ( 'NONE',  ( 8.224510206698742110, 14.34966873604972548, 67.08442372801901854 ) ) ;
#79372=CARTESIAN_POINT ( 'NONE',  ( 14.34966873604960469, 8.224510206698951720, 104.1655762719810241 ) ) ;
#79373=CARTESIAN_POINT ( 'NONE',  ( 16.55341960407611168, 4.379528057220329451, 23.95724293864769550 ) ) ;
#79374=CARTESIAN_POINT ( 'NONE',  ( -17.72517630440433933, 5.499999999999974243, 70.92175719257211597 ) ) ;
#79375=CARTESIAN_POINT ( 'NONE',  ( 18.62759615963255655, 10.81492255796105972, 76.66775706135234714 ) ) ;
#79376=CARTESIAN_POINT ( 'NONE',  ( -16.51473224551069308, -9.474510206698971260, 86.66557627198102409 ) ) ;
#79377=CARTESIAN_POINT ( 'NONE',  ( -13.97604488694527625, -13.89961937509977652, 71.87390960531433848 ) ) ;
#79378=CARTESIAN_POINT ( 'NONE',  ( 0.05219959533909260263, 19.03943276465977164, 104.9989096053143669 ) ) ;
#79379=CARTESIAN_POINT ( 'NONE',  ( 14.34966873604960469, 8.224510206698951720, 54.16557627198103120 ) ) ;
#79381=CARTESIAN_POINT ( 'NONE',  ( 0.05219959533934541429, -16.53943276465976808, 110.0010903946856757 ) ) ;
#79383=CARTESIAN_POINT ( 'NONE',  ( -12.14591786802309592, -12.06949235617757132, 36.87390960531435979 ) ) ;
#79384=CARTESIAN_POINT ( 'NONE',  ( -4.483927247898782831, 16.52544592524335698, 42.70942372801901854 ) ) ;
#79385=DIRECTION ( 'NONE',  ( -0.000000000000000000, -0.000000000000000000, 1.000000000000000000 ) ) ;
#79386=CARTESIAN_POINT ( 'NONE',  ( -9.474510206698720793, -16.51473224551083518, 39.58442372801899722 ) ) ;
#79387=CARTESIAN_POINT ( 'NONE',  ( 5.049401038298161559, -19.05341960407611168, 77.70724293864765286 ) ) ;
#79388=CARTESIAN_POINT ( 'NONE',  ( -9.564922557961040184, 16.46253265017147172, 52.91775706135233293 ) ) ;
#79390=CARTESIAN_POINT ( 'NONE',  ( -5.049401038297874678, -19.05341960407617918, 99.79275706135234714 ) ) ;
#79391=CARTESIAN_POINT ( 'NONE',  ( -8.224510206698735004, -14.34966873604973081, 84.58442372801903275 ) ) ;
#79392=CARTESIAN_POINT ( 'NONE',  ( 13.97604488694527802, 13.89961937509977652, 24.37390960531435624 ) ) ;
#79393=CARTESIAN_POINT ( 'NONE',  ( 9.564922557960805705, 16.46253265017160317, 99.58224293864770971 ) ) ;
#79394=CARTESIAN_POINT ( 'NONE',  ( -15.80617190586768217, 15.72974639402176855, 48.12609039468568284 ) ) ;
#79395=CARTESIAN_POINT ( 'NONE',  ( 13.89961937509957401, 13.97604488694547697, 86.87609039468567573 ) ) ;
#79396=CYLINDRICAL_SURFACE ( 'NONE', #86294, 2.000000000000001776 ) ;
#79397=CARTESIAN_POINT ( 'NONE',  ( 19.03943276465977164, -0.05219959533909143690, 43.74890960531435979 ) ) ;
#79398=CARTESIAN_POINT ( 'NONE',  ( -16.46253265017160317, 9.564922557960807481, 105.8322429386476955 ) ) ;
#79399=CARTESIAN_POINT ( 'NONE',  ( -4.483927247898539470, -16.52544592524342804, 67.29057627198103830 ) ) ;
#79400=CARTESIAN_POINT ( 'NONE',  ( -13.89961937509977652, 13.97604488694528158, 55.62390960531434558 ) ) ;
#79401=CARTESIAN_POINT ( 'NONE',  ( -5.049401038298153566, 19.05341960407611168, 65.20724293864765286 ) ) ;
#79402=CARTESIAN_POINT ( 'NONE',  ( -19.02544592524334988, -5.153800228976617603, 58.95942372801900433 ) ) ;
#79403=CARTESIAN_POINT ( 'NONE',  ( -16.51473224551082808, 9.474510206698731452, 43.33442372801900433 ) ) ;
#79404=CARTESIAN_POINT ( 'NONE',  ( -16.51473224551069308, -9.474510206698971260, 71.66557627198102409 ) ) ;
#79405=CARTESIAN_POINT ( 'NONE',  ( -21.53943276465977519, 0.05219959533907696930, 81.24890960531436690 ) ) ;
#79406=CARTESIAN_POINT ( 'NONE',  ( -8.224510206698948167, 14.34966873604960824, 70.41557627198102409 ) ) ;
#79407=CARTESIAN_POINT ( 'NONE',  ( -9.474510206698720793, -16.51473224551083518, 39.58442372801899722 ) ) ;
#79408=CARTESIAN_POINT ( 'NONE',  ( 10.81492255796078972, 18.62759615963270932, 49.58224293864769550 ) ) ;
#79410=CARTESIAN_POINT ( 'NONE',  ( 0.05219959533907565091, 21.53943276465977519, 39.99890960531436690 ) ) ;
#79411=CARTESIAN_POINT ( 'NONE',  ( 13.97604488694527802, 13.89961937509977652, 64.37390960531436690 ) ) ;
#79412=CARTESIAN_POINT ( 'NONE',  ( -9.564922557960796823, -16.46253265017161027, 42.08224293864769550 ) ) ;
#79413=CARTESIAN_POINT ( 'NONE',  ( -16.53943276465976808, 0.05219959533911058130, 101.2489096053143669 ) ) ;
#79414=CARTESIAN_POINT ( 'NONE',  ( -15.72974639402197994, 15.80617190586746368, 110.6239096053143669 ) ) ;
#79416=CARTESIAN_POINT ( 'NONE',  ( 0.05219959533937995610, -21.53943276465977519, 30.00109039468568284 ) ) ;
#79417=CARTESIAN_POINT ( 'NONE',  ( -19.02544592524342804, 5.153800228976336051, 36.04057627198100988 ) ) ;
#79418=CARTESIAN_POINT ( 'NONE',  ( -0.05219959533907301413, -21.53943276465977519, 112.4989096053143669 ) ) ;
#79419=CARTESIAN_POINT ( 'NONE',  ( 0.05219959533936267826, -19.03943276465977164, 45.00109039468566863 ) ) ;
#79420=CARTESIAN_POINT ( 'NONE',  ( 19.02544592524343514, -5.153800228976328945, 23.54057627198102054 ) ) ;
#79421=CARTESIAN_POINT ( 'NONE',  ( -5.153800228976328057, -19.02544592524343514, 27.29057627198103120 ) ) ;
#79422=CARTESIAN_POINT ( 'NONE',  ( 4.483927247898790824, -16.52544592524335698, 40.20942372801901854 ) ) ;
#79423=CARTESIAN_POINT ( 'NONE',  ( 19.02544592524343514, -5.153800228976328945, 28.54057627198102409 ) ) ;
#79425=CARTESIAN_POINT ( 'NONE',  ( -5.049401038298153566, 19.05341960407611168, 75.20724293864769550 ) ) ;
#79426=CARTESIAN_POINT ( 'NONE',  ( 16.53943276465976808, -0.05219959533910856209, 113.7489096053143527 ) ) ;
#79427=CARTESIAN_POINT ( 'NONE',  ( 5.719274019375991003, -21.55341960407610458, 52.70724293864769550 ) ) ;
#79428=CARTESIAN_POINT ( 'NONE',  ( -16.55341960407611168, -4.379528057220339221, 81.45724293864769550 ) ) ;
#79429=CARTESIAN_POINT ( 'NONE',  ( -14.29746914071037622, -8.314922557961029526, 29.16775706135234003 ) ) ;
#79430=CARTESIAN_POINT ( 'NONE',  ( 21.52544592524334988, 5.823673210054432836, 86.45942372801901854 ) ) ;
#79431=CARTESIAN_POINT ( 'NONE',  ( -19.03943276465977164, 0.05219959533909376836, 31.24890960531435979 ) ) ;
#79432=CARTESIAN_POINT ( 'NONE',  ( -16.55341960407617563, 4.379528057220093196, 113.5427570613523756 ) ) ;
#79433=CARTESIAN_POINT ( 'NONE',  ( -12.06949235617756955, 12.14591786802309770, 50.62390960531435979 ) ) ;
#79434=CARTESIAN_POINT ( 'NONE',  ( 13.97604488694527802, 13.89961937509977652, 54.37390960531435979 ) ) ;
#79435=CARTESIAN_POINT ( 'NONE',  ( 15.72974639402176855, 15.80617190586768217, 101.8760903946857042 ) ) ;
#79436=CARTESIAN_POINT ( 'NONE',  ( 5.719274019375991003, -21.55341960407610458, 112.7072429386476955 ) ) ;
#79437=CARTESIAN_POINT ( 'NONE',  ( -21.52544592524334988, -5.823673210054445271, 78.95942372801901854 ) ) ;
#79438=CARTESIAN_POINT ( 'NONE',  ( 8.314922557961029526, -14.29746914071037800, 35.41775706135234003 ) ) ;
#79439=CARTESIAN_POINT ( 'NONE',  ( -8.224510206698948167, 14.34966873604960824, 75.41557627198102409 ) ) ;
#79440=CARTESIAN_POINT ( 'NONE',  ( -10.81492255796105439, 18.62759615963255655, 87.91775706135234714 ) ) ;
#79441=EDGE_CURVE ( 'NONE', #6927, #115616, #141379, .T. ) ;
#79442=CARTESIAN_POINT ( 'NONE',  ( 14.34966873604972726, -8.224510206698740333, 110.8344237280190043 ) ) ;
#79443=CARTESIAN_POINT ( 'NONE',  ( -17.13100169013301510, 6.664070546373117132, 115.7678983569985292 ) ) ;
#79444=CARTESIAN_POINT ( 'NONE',  ( 16.55341960407618274, -4.379528057220086978, 41.04275706135236135 ) ) ;
#79445=CARTESIAN_POINT ( 'NONE',  ( -4.483927247898539470, -16.52544592524342804, 37.29057627198102409 ) ) ;
#79446=CARTESIAN_POINT ( 'NONE',  ( -0.05219959533934338120, 16.53943276465976808, 82.50109039468568994 ) ) ;
#79447=CARTESIAN_POINT ( 'NONE',  ( -5.049401038298153566, 19.05341960407611168, 95.20724293864770971 ) ) ;
#79448=CARTESIAN_POINT ( 'NONE',  ( -16.46253265017160317, 9.564922557960807481, 95.83224293864769550 ) ) ;
#79449=CARTESIAN_POINT ( 'NONE',  ( -18.67979575497193778, 10.72451020669871902, 103.3344237280190043 ) ) ;
#79450=CARTESIAN_POINT ( 'NONE',  ( 4.483927247898790824, -16.52544592524335698, 100.2094237280190043 ) ) ;
#79451=CARTESIAN_POINT ( 'NONE',  ( -12.14591786802309592, -12.06949235617757132, 71.87390960531438111 ) ) ;
#79452=CARTESIAN_POINT ( 'NONE',  ( -19.03943276465977164, 0.05219959533909376836, 86.24890960531436690 ) ) ;
#79455=CARTESIAN_POINT ( 'NONE',  ( -8.314922557961024197, 14.29746914071037800, 27.91775706135234358 ) ) ;
#79456=CARTESIAN_POINT ( 'NONE',  ( -13.89961937509977652, 13.97604488694528158, 30.62390960531435269 ) ) ;
#79457=CARTESIAN_POINT ( 'NONE',  ( -13.89961937509977652, 13.97604488694528158, 90.62390960531432427 ) ) ;
#79458=CARTESIAN_POINT ( 'NONE',  ( -12.14591786802326823, 12.06949235617739902, 38.12609039468567573 ) ) ;
#79460=CARTESIAN_POINT ( 'NONE',  ( 9.564922557961047289, -16.46253265017146816, 30.41775706135232937 ) ) ;
#79461=CARTESIAN_POINT ( 'NONE',  ( 0.05219959533934541429, -16.53943276465976808, 95.00109039468568994 ) ) ;
#79462=CARTESIAN_POINT ( 'NONE',  ( 19.02544592524334988, 5.153800228976608722, 101.4594237280189759 ) ) ;
#79463=CARTESIAN_POINT ( 'NONE',  ( 5.049401038298161559, -19.05341960407611168, 32.70724293864768129 ) ) ;
#79464=CARTESIAN_POINT ( 'NONE',  ( -12.14591786802326823, 12.06949235617739902, 78.12609039468570415 ) ) ;
#79465=CARTESIAN_POINT ( 'NONE',  ( -8.224510206698735004, -14.34966873604973081, 69.58442372801900433 ) ) ;
#79466=CARTESIAN_POINT ( 'NONE',  ( 9.474510206698971260, -16.51473224551069308, 22.91557627198102765 ) ) ;
#79467=CARTESIAN_POINT ( 'NONE',  ( -5.049401038297874678, -19.05341960407617918, 69.79275706135233293 ) ) ;
#79468=CARTESIAN_POINT ( 'NONE',  ( 15.72974639402176855, 15.80617190586768217, 106.8760903946856899 ) ) ;
#79469=CARTESIAN_POINT ( 'NONE',  ( -5.049401038298153566, 19.05341960407611168, 50.20724293864770260 ) ) ;
#79471=CARTESIAN_POINT ( 'NONE',  ( -16.51473224551069308, -9.474510206698971260, 91.66557627198103830 ) ) ;
#79472=CARTESIAN_POINT ( 'NONE',  ( -8.314922557960811034, -14.29746914071050412, 92.08224293864769550 ) ) ;
#79474=CARTESIAN_POINT ( 'NONE',  ( -19.02544592524334988, -5.153800228976617603, 58.95942372801900433 ) ) ;
#79475=CARTESIAN_POINT ( 'NONE',  ( -15.80617190586745835, -15.72974639402198527, 56.87390960531436690 ) ) ;
#79476=CARTESIAN_POINT ( 'NONE',  ( 21.52544592524334988, 5.823673210054432836, 106.4594237280190328 ) ) ;
#79477=CARTESIAN_POINT ( 'NONE',  ( -19.02544592524342804, 5.153800228976336051, 96.04057627198103830 ) ) ;
#79478=CARTESIAN_POINT ( 'NONE',  ( -9.474510206698720793, -16.51473224551083518, 24.58442372801900078 ) ) ;
#79479=CARTESIAN_POINT ( 'NONE',  ( -18.62759615963270932, 10.81492255796079327, 60.83224293864769550 ) ) ;
#79480=CARTESIAN_POINT ( 'NONE',  ( 0.05219959533909260263, 19.03943276465977164, 104.9989096053143669 ) ) ;
#79481=CARTESIAN_POINT ( 'NONE',  ( 19.03943276465977164, 0.05219959533936151252, 86.25109039468567573 ) ) ;
#79483=CARTESIAN_POINT ( 'NONE',  ( -5.049401038297874678, -19.05341960407617918, 104.7927570613523471 ) ) ;
#79484=CARTESIAN_POINT ( 'NONE',  ( -14.29746914071049879, 8.314922557960819915, 110.8322429386476955 ) ) ;
#79485=CARTESIAN_POINT ( 'NONE',  ( -5.049401038298153566, 19.05341960407611168, 100.2072429386476955 ) ) ;
#79486=CARTESIAN_POINT ( 'NONE',  ( -0.05219959533907301413, -21.53943276465977519, 77.49890960531433848 ) ) ;
#79487=CARTESIAN_POINT ( 'NONE',  ( 4.379528057220092307, 16.55341960407617563, 47.29275706135234003 ) ) ;
#79488=CARTESIAN_POINT ( 'NONE',  ( 10.72451020669871369, 18.67979575497193778, 42.08442372801901854 ) ) ;
#79489=CARTESIAN_POINT ( 'NONE',  ( 18.62759615963255655, 10.81492255796105972, 96.66775706135234714 ) ) ;
#79490=CARTESIAN_POINT ( 'NONE',  ( 8.314922557961029526, -14.29746914071037800, 95.41775706135234714 ) ) ;
#79491=CARTESIAN_POINT ( 'NONE',  ( 19.02544592524343514, -5.153800228976328945, 83.54057627198100988 ) ) ;
#79492=CARTESIAN_POINT ( 'NONE',  ( 16.55341960407611168, 4.379528057220329451, 88.95724293864769550 ) ) ;
#79493=CARTESIAN_POINT ( 'NONE',  ( -12.06949235617756955, 12.14591786802309770, 30.62390960531436335 ) ) ;
#79494=CARTESIAN_POINT ( 'NONE',  ( -19.02544592524334988, -5.153800228976617603, 63.95942372801899012 ) ) ;
#79495=CARTESIAN_POINT ( 'NONE',  ( 21.55341960407619695, -5.719274019375665929, 46.04275706135234714 ) ) ;
#79496=CARTESIAN_POINT ( 'NONE',  ( -9.474510206698720793, -16.51473224551083518, 29.58442372801900433 ) ) ;
#79497=CARTESIAN_POINT ( 'NONE',  ( 14.34966873604960469, 8.224510206698951720, 94.16557627198103830 ) ) ;
#79498=CARTESIAN_POINT ( 'NONE',  ( 9.474510206698971260, -16.51473224551069308, 112.9155762719810383 ) ) ;
#79499=CARTESIAN_POINT ( 'NONE',  ( 12.06949235617757843, -12.14591786802309237, 23.12390960531436335 ) ) ;
#79500=CARTESIAN_POINT ( 'NONE',  ( -18.67979575497193778, 10.72451020669871902, 88.33442372801901854 ) ) ;
#79501=CARTESIAN_POINT ( 'NONE',  ( -0.05219959533934338120, 16.53943276465976808, 57.50109039468568994 ) ) ;
#79502=CARTESIAN_POINT ( 'NONE',  ( 16.53943276465976808, 0.05219959533934440121, 106.2510903946856757 ) ) ;
#79503=CARTESIAN_POINT ( 'NONE',  ( 18.67979575497194134, -10.72451020669871369, 60.83442372801901854 ) ) ;
#79504=CARTESIAN_POINT ( 'NONE',  ( 5.823673210054444382, -21.52544592524334988, 30.20942372801902565 ) ) ;
#79505=CARTESIAN_POINT ( 'NONE',  ( -12.14591786802309592, -12.06949235617757132, 101.8739096053143811 ) ) ;
#79506=CARTESIAN_POINT ( 'NONE',  ( -16.51473224551069308, -9.474510206698971260, 21.66557627198102765 ) ) ;
#79507=CARTESIAN_POINT ( 'NONE',  ( 0.05219959533910956823, 16.53943276465976808, 59.99890960531436690 ) ) ;
#79508=CARTESIAN_POINT ( 'NONE',  ( 13.97604488694527802, 13.89961937509977652, 69.37390960531436690 ) ) ;
#79509=CARTESIAN_POINT ( 'NONE',  ( 16.55341960407618274, -4.379528057220086978, 111.0427570613523613 ) ) ;
#79510=CARTESIAN_POINT ( 'NONE',  ( 10.81492255796078972, 18.62759615963270932, 59.58224293864770260 ) ) ;
#79511=CARTESIAN_POINT ( 'NONE',  ( -16.55341960407611168, -4.379528057220339221, 96.45724293864770971 ) ) ;
#79513=CARTESIAN_POINT ( 'NONE',  ( -10.72451020669898014, 18.67979575497178502, 95.41557627198102409 ) ) ;
#79514=CARTESIAN_POINT ( 'NONE',  ( -9.474510206698964154, 16.51473224551069663, 105.4155762719810383 ) ) ;
#79515=CARTESIAN_POINT ( 'NONE',  ( 13.89961937509977652, -13.97604488694527269, 53.12390960531434558 ) ) ;
#79516=CARTESIAN_POINT ( 'NONE',  ( 16.51473224551083163, -9.474510206698727899, 90.83442372801900433 ) ) ;
#79517=CARTESIAN_POINT ( 'NONE',  ( 21.52544592524344225, -5.823673210054117533, 48.54057627198103120 ) ) ;
#79518=CARTESIAN_POINT ( 'NONE',  ( 10.72451020669871369, 18.67979575497193778, 62.08442372801901143 ) ) ;
#79519=CARTESIAN_POINT ( 'NONE',  ( -5.153800228976328057, -19.02544592524343514, 47.29057627198102409 ) ) ;
#79520=CARTESIAN_POINT ( 'NONE',  ( -0.05219959533909027116, -19.03943276465977164, 82.49890960531436690 ) ) ;
#79521=CARTESIAN_POINT ( 'NONE',  ( -8.314922557961024197, 14.29746914071037800, 67.91775706135234714 ) ) ;
#79522=CARTESIAN_POINT ( 'NONE',  ( 5.823673210054444382, -21.52544592524334988, 40.20942372801901854 ) ) ;
#79523=CARTESIAN_POINT ( 'NONE',  ( -21.55341960407619339, 5.719274019375674811, 88.54275706135236135 ) ) ;
#79524=CARTESIAN_POINT ( 'NONE',  ( 18.67979575497178502, 10.72451020669898547, 99.16557627198100988 ) ) ;
#79525=CARTESIAN_POINT ( 'NONE',  ( -10.81492255796105439, 18.62759615963255655, 37.91775706135235424 ) ) ;
#79526=CARTESIAN_POINT ( 'NONE',  ( 8.314922557961029526, -14.29746914071037800, 65.41775706135234714 ) ) ;
#79527=CARTESIAN_POINT ( 'NONE',  ( 18.62759615963271287, -10.81492255796078972, 73.33224293864769550 ) ) ;
#79528=CARTESIAN_POINT ( 'NONE',  ( 5.049401038297881783, 19.05341960407617563, 32.29275706135233293 ) ) ;
#79529=CARTESIAN_POINT ( 'NONE',  ( -0.05219959533909027116, -19.03943276465977164, 62.49890960531435979 ) ) ;
#79530=CARTESIAN_POINT ( 'NONE',  ( 16.52544592524335698, 4.483927247898782831, 111.4594237280190328 ) ) ;
#79531=CARTESIAN_POINT ( 'NONE',  ( -17.49999999999999645, -3.345213924137415251, 105.4123137690565670 ) ) ;
#79532=CARTESIAN_POINT ( 'NONE',  ( -5.049401038298153566, 19.05341960407611168, 105.2072429386476671 ) ) ;
#79534=CARTESIAN_POINT ( 'NONE',  ( 16.51473224551083163, -9.474510206698727899, 85.83442372801900433 ) ) ;
#79535=CARTESIAN_POINT ( 'NONE',  ( 10.81492255796078972, 18.62759615963270932, 54.58224293864769550 ) ) ;
#79536=CARTESIAN_POINT ( 'NONE',  ( 14.29746914071049879, -8.314922557960816363, 33.33224293864769550 ) ) ;
#79537=CARTESIAN_POINT ( 'NONE',  ( -0.05219959533936034679, 19.03943276465977164, 112.5010903946856757 ) ) ;
#79538=CARTESIAN_POINT ( 'NONE',  ( 16.51473224551069308, 9.474510206698969483, 29.16557627198103475 ) ) ;
#79539=CARTESIAN_POINT ( 'NONE',  ( -16.51473224551082808, 9.474510206698731452, 108.3344237280190043 ) ) ;
#79540=CARTESIAN_POINT ( 'NONE',  ( -5.719274019375978568, 21.55341960407610458, 95.20724293864769550 ) ) ;
#79541=CARTESIAN_POINT ( 'NONE',  ( 9.564922557961047289, -16.46253265017146816, 70.41775706135233293 ) ) ;
#79542=CARTESIAN_POINT ( 'NONE',  ( 14.34966873604972726, -8.224510206698740333, 75.83442372801900433 ) ) ;
#79543=CARTESIAN_POINT ( 'NONE',  ( -9.474510206698964154, 16.51473224551069663, 65.41557627198102409 ) ) ;
#79544=CARTESIAN_POINT ( 'NONE',  ( -12.14591786802309592, -12.06949235617757132, 76.87390960531439532 ) ) ;
#79545=CARTESIAN_POINT ( 'NONE',  ( 9.564922557960805705, 16.46253265017160317, 54.58224293864769550 ) ) ;
#79546=CARTESIAN_POINT ( 'NONE',  ( -12.14591786802309592, -12.06949235617757132, 61.87390960531436690 ) ) ;
#79547=CARTESIAN_POINT ( 'NONE',  ( 30.00000000000000000, 0.000000000000000000, 0.000000000000000000 ) ) ;
#79549=CARTESIAN_POINT ( 'NONE',  ( -8.314922557960811034, -14.29746914071050412, 37.08224293864768129 ) ) ;
#79550=CARTESIAN_POINT ( 'NONE',  ( 19.03943276465977164, -0.05219959533909143690, 78.74890960531436690 ) ) ;
#79552=CARTESIAN_POINT ( 'NONE',  ( -13.89961937509957401, -13.97604488694547875, 39.37609039468566152 ) ) ;
#79553=CARTESIAN_POINT ( 'NONE',  ( 16.52544592524335698, 4.483927247898782831, 51.45942372801901854 ) ) ;
#79555=CARTESIAN_POINT ( 'NONE',  ( -5.823673210054116645, -21.52544592524344225, 62.29057627198102409 ) ) ;
#79556=CARTESIAN_POINT ( 'NONE',  ( 16.46253265017146816, 9.564922557961045513, 21.66775706135233648 ) ) ;
#79557=CARTESIAN_POINT ( 'NONE',  ( 0.05219959533909260263, 19.03943276465977164, 69.99890960531435269 ) ) ;
#79559=CARTESIAN_POINT ( 'NONE',  ( -9.474510206698964154, 16.51473224551069663, 105.4155762719810383 ) ) ;
#79560=CARTESIAN_POINT ( 'NONE',  ( 0.05219959533937995610, -21.53943276465977519, 40.00109039468567573 ) ) ;
#79562=CARTESIAN_POINT ( 'NONE',  ( -16.53943276465976808, 0.05219959533911058130, 101.2489096053143669 ) ) ;
#79563=CARTESIAN_POINT ( 'NONE',  ( 21.52544592524344225, -5.823673210054117533, 98.54057627198105251 ) ) ;
#79564=CARTESIAN_POINT ( 'NONE',  ( -19.05341960407611168, -5.049401038298163336, 81.45724293864769550 ) ) ;
#79566=CARTESIAN_POINT ( 'NONE',  ( 15.80617190586769283, -15.72974639402175789, 20.62609039468568639 ) ) ;
#79567=ORIENTED_EDGE ( 'NONE', *, *, #34959, .T. ) ;
#79568=CARTESIAN_POINT ( 'NONE',  ( -16.51473224551069308, -9.474510206698971260, 91.66557627198103830 ) ) ;
#79569=CARTESIAN_POINT ( 'NONE',  ( 19.53037848336980531, -5.499999999999891642, 82.35532783611442653 ) ) ;
#79570=CARTESIAN_POINT ( 'NONE',  ( 5.153800228976335163, 19.02544592524342804, 29.79057627198102409 ) ) ;
#79571=CARTESIAN_POINT ( 'NONE',  ( 16.46253265017146816, 9.564922557961045513, 106.6677570613523471 ) ) ;
#79573=CARTESIAN_POINT ( 'NONE',  ( 4.379528057220339221, -16.55341960407611168, 112.7072429386476955 ) ) ;
#79574=CARTESIAN_POINT ( 'NONE',  ( -18.62759615963255300, -10.81492255796106328, 79.16775706135234714 ) ) ;
#79575=CARTESIAN_POINT ( 'NONE',  ( 9.564922557960805705, 16.46253265017160317, 79.58224293864769550 ) ) ;
#79576=CARTESIAN_POINT ( 'NONE',  ( -21.55341960407619339, 5.719274019375674811, 43.54275706135235424 ) ) ;
#79577=CARTESIAN_POINT ( 'NONE',  ( 15.80617190586769283, -15.72974639402175789, 25.62609039468567929 ) ) ;
#79579=CARTESIAN_POINT ( 'NONE',  ( -0.05219959533909027116, -19.03943276465977164, 92.49890960531436690 ) ) ;
#79581=CARTESIAN_POINT ( 'NONE',  ( 16.53943276465976808, 0.05219959533934440121, 46.25109039468567573 ) ) ;
#79582=CARTESIAN_POINT ( 'NONE',  ( -5.719274019375978568, 21.55341960407610458, 40.20724293864769550 ) ) ;
#79583=CARTESIAN_POINT ( 'NONE',  ( 21.55341960407619695, -5.719274019375665929, 71.04275706135234714 ) ) ;
#79584=DIRECTION ( 'NONE',  ( 0.000000000000000000, -1.000000000000000000, 0.000000000000000000 ) ) ;
#79585=CARTESIAN_POINT ( 'NONE',  ( 19.05341960407617918, -5.049401038297876454, 106.0427570613523471 ) ) ;
#79586=CARTESIAN_POINT ( 'NONE',  ( 9.564922557960805705, 16.46253265017160317, 54.58224293864769550 ) ) ;
#79587=CARTESIAN_POINT ( 'NONE',  ( 19.03943276465977164, -0.05219959533909143690, 78.74890960531436690 ) ) ;
#79588=CARTESIAN_POINT ( 'NONE',  ( -0.05219959533910754901, -16.53943276465976808, 112.4989096053143669 ) ) ;
#79589=CARTESIAN_POINT ( 'NONE',  ( 4.483927247898545687, 16.52544592524342804, 104.7905762719810241 ) ) ;
#79590=CARTESIAN_POINT ( 'NONE',  ( -19.05341960407611168, -5.049401038298163336, 106.4572429386476955 ) ) ;
#79591=CARTESIAN_POINT ( 'NONE',  ( -8.224510206698735004, -14.34966873604973081, 79.58442372801903275 ) ) ;
#79592=CARTESIAN_POINT ( 'NONE',  ( -14.29746914071049879, 8.314922557960819915, 60.83224293864769550 ) ) ;
#79593=CARTESIAN_POINT ( 'NONE',  ( 13.89961937509977652, -13.97604488694527269, 58.12390960531436690 ) ) ;
#79594=CARTESIAN_POINT ( 'NONE',  ( -10.81492255796105439, 18.62759615963255655, 77.91775706135231871 ) ) ;
#79595=CARTESIAN_POINT ( 'NONE',  ( 10.72451020669871369, 18.67979575497193778, 72.08442372801899012 ) ) ;
#79596=CARTESIAN_POINT ( 'NONE',  ( 5.153800228976615827, -19.02544592524334988, 110.2094237280189901 ) ) ;
#79597=CARTESIAN_POINT ( 'NONE',  ( -16.52544592524342804, 4.483927247898546575, 61.04057627198103120 ) ) ;
#79598=CARTESIAN_POINT ( 'NONE',  ( -18.62759615963270932, 10.81492255796079327, 110.8322429386476955 ) ) ;
#79599=CARTESIAN_POINT ( 'NONE',  ( 15.80617190586746368, 15.72974639402197994, 54.37390960531435979 ) ) ;
#79602=CARTESIAN_POINT ( 'NONE',  ( -9.564922557960796823, -16.46253265017161027, 67.08224293864769550 ) ) ;
#79603=CARTESIAN_POINT ( 'NONE',  ( 12.14591786802309770, 12.06949235617756955, 39.37390960531436690 ) ) ;
#79604=CARTESIAN_POINT ( 'NONE',  ( -8.314922557960811034, -14.29746914071050412, 27.08224293864769550 ) ) ;
#79605=CARTESIAN_POINT ( 'NONE',  ( -0.05219959533934338120, 16.53943276465976808, 102.5010903946856899 ) ) ;
#79606=CARTESIAN_POINT ( 'NONE',  ( -19.03943276465977164, -0.05219959533935918106, 58.75109039468566863 ) ) ;
#79608=CARTESIAN_POINT ( 'NONE',  ( -19.05341960407611168, -5.049401038298163336, 91.45724293864766707 ) ) ;
#79609=CARTESIAN_POINT ( 'NONE',  ( -8.314922557960811034, -14.29746914071050412, 62.08224293864769550 ) ) ;
#79610=B_SPLINE_CURVE_WITH_KNOTS ( 'NONE', 3,
 ( #89046, #57731, #197240, #58701, #106195, #11232, #163917, #149731, #151721, #13214, #74877, #152695, #10228, #182064, #12236, #133558, #91009, #88043, #55719, #119401, #134575, #41565, #25413, #87055, #121363, #71888, #136539, #44540, #167879, #198220, #29378, #14184 ),
 .UNSPECIFIED., .F., .F.,
 ( 4, 2, 2, 2, 2, 2, 2, 2, 2, 2, 2, 2, 2, 2, 2, 4 ),
 ( 8.673617379884035472E-18, 0.0003712461730036821701, 0.0007424923460073556665, 0.001113738519011029217, 0.001484984692014702659, 0.002227477038022057567, 0.002598723211025738382, 0.002969969384029419197, 0.003341215557033099578, 0.003712461730036780826, 0.004083707903040461641, 0.004454954076044142022, 0.004826200249047823271, 0.005197446422051503652, 0.005568692595055184900, 0.005939938768058865282 ),
 .UNSPECIFIED. ) ;
#79611=CARTESIAN_POINT ( 'NONE',  ( 18.09805431107520590, -5.500000000000095923, 48.51606229291890315 ) ) ;
#79612=CARTESIAN_POINT ( 'NONE',  ( -10.81492255796078084, -18.62759615963271287, 22.08224293864769194 ) ) ;
#79613=CARTESIAN_POINT ( 'NONE',  ( -18.62759615963270932, 10.81492255796079327, 50.83224293864770971 ) ) ;
#79614=ORIENTED_EDGE ( 'NONE', *, *, #138961, .F. ) ;
#79615=CARTESIAN_POINT ( 'NONE',  ( 12.14591786802309770, 12.06949235617756955, 94.37390960531436690 ) ) ;
#79616=CARTESIAN_POINT ( 'NONE',  ( -8.314922557961024197, 14.29746914071037800, 52.91775706135235424 ) ) ;
#79618=CARTESIAN_POINT ( 'NONE',  ( 12.06949235617757843, -12.14591786802309237, 78.12390960531436690 ) ) ;
#79620=CARTESIAN_POINT ( 'NONE',  ( -9.564922557961040184, 16.46253265017147172, 82.91775706135233293 ) ) ;
#79621=CARTESIAN_POINT ( 'NONE',  ( 9.564922557960805705, 16.46253265017160317, 109.5822429386476955 ) ) ;
#79624=CARTESIAN_POINT ( 'NONE',  ( -16.55341960407617563, 4.379528057220093196, 48.54275706135234714 ) ) ;
#79625=CARTESIAN_POINT ( 'NONE',  ( 12.14591786802309770, 12.06949235617756955, 29.37390960531435269 ) ) ;
#79626=CARTESIAN_POINT ( 'NONE',  ( -5.719274019375978568, 21.55341960407610458, 55.20724293864770260 ) ) ;
#79627=CARTESIAN_POINT ( 'NONE',  ( -5.049401038297874678, -19.05341960407617918, 84.79275706135233293 ) ) ;
#79628=CARTESIAN_POINT ( 'NONE',  ( -18.67979575497178146, -10.72451020669898902, 51.66557627198102409 ) ) ;
#79629=CARTESIAN_POINT ( 'NONE',  ( 0.05219959533937995610, -21.53943276465977519, 80.00109039468568994 ) ) ;
#79631=CARTESIAN_POINT ( 'NONE',  ( 14.29746914071037800, 8.314922557961029526, 31.66775706135234358 ) ) ;
#79632=CARTESIAN_POINT ( 'NONE',  ( 9.474510206698971260, -16.51473224551069308, 42.91557627198103120 ) ) ;
#79633=CARTESIAN_POINT ( 'NONE',  ( -5.049401038298153566, 19.05341960407611168, 100.2072429386476955 ) ) ;
#79634=CARTESIAN_POINT ( 'NONE',  ( -16.46253265017160317, 9.564922557960807481, 40.83224293864769550 ) ) ;
#79635=CARTESIAN_POINT ( 'NONE',  ( 4.483927247898545687, 16.52544592524342804, 104.7905762719810241 ) ) ;
#79637=CARTESIAN_POINT ( 'NONE',  ( 19.02544592524343514, -5.153800228976328945, 98.54057627198100988 ) ) ;
#79639=CARTESIAN_POINT ( 'NONE',  ( -8.314922557961024197, 14.29746914071037800, 52.91775706135235424 ) ) ;
#79640=CARTESIAN_POINT ( 'NONE',  ( -15.72974639402197994, 15.80617190586746368, 90.62390960531436690 ) ) ;
#79641=CARTESIAN_POINT ( 'NONE',  ( 5.049401038298161559, -19.05341960407611168, 42.70724293864767418 ) ) ;
#79642=CARTESIAN_POINT ( 'NONE',  ( 21.53943276465977519, 0.05219959533937863772, 26.25109039468567573 ) ) ;
#79643=CARTESIAN_POINT ( 'NONE',  ( 19.05341960407611168, 5.049401038298154454, 78.95724293864769550 ) ) ;
#79646=CARTESIAN_POINT ( 'NONE',  ( -8.224510206698735004, -14.34966873604973081, 49.58442372801901143 ) ) ;
#79647=CARTESIAN_POINT ( 'NONE',  ( -18.67979575497178146, -10.72451020669898902, 111.6655762719810525 ) ) ;
#79648=CARTESIAN_POINT ( 'NONE',  ( 16.53943276465976808, -0.05219959533910856209, 103.7489096053143669 ) ) ;
#79649=CARTESIAN_POINT ( 'NONE',  ( 9.474510206698971260, -16.51473224551069308, 97.91557627198102409 ) ) ;
#79650=CARTESIAN_POINT ( 'NONE',  ( -16.46253265017146816, -9.564922557961047289, 69.16775706135233293 ) ) ;
#79651=CARTESIAN_POINT ( 'NONE',  ( -19.05341960407617563, 5.049401038297882671, 33.54275706135231871 ) ) ;
#79652=CARTESIAN_POINT ( 'NONE',  ( 21.55341960407610458, 5.719274019375980345, 88.95724293864769550 ) ) ;
#79653=CARTESIAN_POINT ( 'NONE',  ( 19.02544592524334988, 5.153800228976608722, 21.45942372801899012 ) ) ;
#79654=CARTESIAN_POINT ( 'NONE',  ( -8.224510206698735004, -14.34966873604973081, 79.58442372801903275 ) ) ;
#79655=CARTESIAN_POINT ( 'NONE',  ( -5.049401038298153566, 19.05341960407611168, 100.2072429386476955 ) ) ;
#79656=CARTESIAN_POINT ( 'NONE',  ( 19.03943276465977164, -0.05219959533909143690, 58.74890960531435979 ) ) ;
#79658=CARTESIAN_POINT ( 'NONE',  ( 21.55341960407619695, -5.719274019375665929, 71.04275706135234714 ) ) ;
#79659=CARTESIAN_POINT ( 'NONE',  ( -0.05219959533937732626, 21.53943276465977519, 67.50109039468568994 ) ) ;
#79660=CARTESIAN_POINT ( 'NONE',  ( -19.05341960407611168, -5.049401038298163336, 76.45724293864769550 ) ) ;
#79661=CARTESIAN_POINT ( 'NONE',  ( -15.80617190586768217, 15.72974639402176855, 53.12609039468568284 ) ) ;
#79662=CARTESIAN_POINT ( 'NONE',  ( -13.97604488694547697, 13.89961937509957934, 93.12609039468566152 ) ) ;
#79663=CARTESIAN_POINT ( 'NONE',  ( -13.89961937509977652, 13.97604488694528158, 50.62390960531435979 ) ) ;
#79664=CARTESIAN_POINT ( 'NONE',  ( 0.05219959533909260263, 19.03943276465977164, 94.99890960531436690 ) ) ;
#79665=CARTESIAN_POINT ( 'NONE',  ( 13.97604488694527802, 13.89961937509977652, 69.37390960531436690 ) ) ;
#79667=CARTESIAN_POINT ( 'NONE',  ( 19.02544592524343514, -5.153800228976328945, 48.54057627198103120 ) ) ;
#79668=CARTESIAN_POINT ( 'NONE',  ( 18.67979575497178502, 10.72451020669898547, 89.16557627198102409 ) ) ;
#79669=CARTESIAN_POINT ( 'NONE',  ( 12.14591786802327356, -12.06949235617739191, 70.62609039468567573 ) ) ;
#79671=CARTESIAN_POINT ( 'NONE',  ( -9.474510206698720793, -16.51473224551083518, 29.58442372801900433 ) ) ;
#79672=CARTESIAN_POINT ( 'NONE',  ( -16.46253265017160317, 9.564922557960807481, 65.83224293864769550 ) ) ;
#79673=CARTESIAN_POINT ( 'NONE',  ( -16.53943276465976808, 0.05219959533911058130, 56.24890960531436690 ) ) ;
#79674=CARTESIAN_POINT ( 'NONE',  ( -16.53943276465976808, 0.05219959533911058130, 101.2489096053143669 ) ) ;
#79675=CARTESIAN_POINT ( 'NONE',  ( -9.564922557960796823, -16.46253265017161027, 97.08224293864769550 ) ) ;
#79676=CARTESIAN_POINT ( 'NONE',  ( -5.153800228976328057, -19.02544592524343514, 97.29057627198099567 ) ) ;
#79677=CARTESIAN_POINT ( 'NONE',  ( 21.55341960407619695, -5.719274019375665929, 51.04275706135234714 ) ) ;
#79678=CARTESIAN_POINT ( 'NONE',  ( 19.02544592524343514, -5.153800228976328945, 108.5405762719810383 ) ) ;
#79679=CARTESIAN_POINT ( 'NONE',  ( 5.153800228976615827, -19.02544592524334988, 20.20942372801899722 ) ) ;
#79680=CARTESIAN_POINT ( 'NONE',  ( -4.483927247898782831, 16.52544592524335698, 82.70942372801900433 ) ) ;
#79681=B_SPLINE_CURVE_WITH_KNOTS ( 'NONE', 3,
 ( #48391, #34206, #171728, #143348, #50379, #33216, #96849, #4836, #95869, #18056, #81665, #20023, #175701, #128186, #112039, #94876, #157552, #173727, #19045, #98836 ),
 .UNSPECIFIED., .F., .F.,
 ( 4, 2, 2, 2, 2, 2, 2, 2, 2, 4 ),
 ( 0.004000878361811959112, 0.004499404418915953392, 0.004997930476019946805, 0.005496456533123941085, 0.005994982590227935365, 0.006244245618779932505, 0.006493508647331928778, 0.006992034704435923058, 0.007490560761539916471, 0.007989086818643910751 ),
 .UNSPECIFIED. ) ;
#79682=CARTESIAN_POINT ( 'NONE',  ( 18.62759615963255655, 10.81492255796105972, 36.66775706135234714 ) ) ;
#79683=CARTESIAN_POINT ( 'NONE',  ( -5.823673210054116645, -21.52544592524344225, 37.29057627198102409 ) ) ;
#79684=CARTESIAN_POINT ( 'NONE',  ( 21.52544592524344225, -5.823673210054117533, 103.5405762719810383 ) ) ;
#79685=CARTESIAN_POINT ( 'NONE',  ( -14.34966873604960291, -8.224510206698953496, 56.66557627198103830 ) ) ;
#79686=CARTESIAN_POINT ( 'NONE',  ( 19.02544592524343514, -5.153800228976328945, 48.54057627198103120 ) ) ;
#79687=CARTESIAN_POINT ( 'NONE',  ( -14.29746914071049879, 8.314922557960819915, 80.83224293864769550 ) ) ;
#79688=CARTESIAN_POINT ( 'NONE',  ( 21.52544592524344225, -5.823673210054117533, 38.54057627198103120 ) ) ;
#79689=CARTESIAN_POINT ( 'NONE',  ( 9.564922557961047289, -16.46253265017146816, 40.41775706135234003 ) ) ;
#79690=CARTESIAN_POINT ( 'NONE',  ( 14.34966873604960469, 8.224510206698951720, 114.1655762719810383 ) ) ;
#79692=CARTESIAN_POINT ( 'NONE',  ( -14.34966873604972548, 8.224510206698743886, 68.33442372801900433 ) ) ;
#79693=CARTESIAN_POINT ( 'NONE',  ( 5.049401038298161559, -19.05341960407611168, 72.70724293864768129 ) ) ;
#79695=CARTESIAN_POINT ( 'NONE',  ( 4.483927247898545687, 16.52544592524342804, 89.79057627198103830 ) ) ;
#79696=CARTESIAN_POINT ( 'NONE',  ( 10.72451020669898902, -18.67979575497178502, 37.91557627198102409 ) ) ;
#79697=CARTESIAN_POINT ( 'NONE',  ( -4.483927247898782831, 16.52544592524335698, 107.7094237280190328 ) ) ;
#79698=CARTESIAN_POINT ( 'NONE',  ( -13.97604488694547697, 13.89961937509957934, 113.1260903946856757 ) ) ;
#79699=CARTESIAN_POINT ( 'NONE',  ( -21.52544592524334988, -5.823673210054445271, 78.95942372801901854 ) ) ;
#79700=CARTESIAN_POINT ( 'NONE',  ( -19.03943276465977164, 0.05219959533909376836, 86.24890960531436690 ) ) ;
#79701=CARTESIAN_POINT ( 'NONE',  ( -15.72974639402197994, 15.80617190586746368, 100.6239096053143811 ) ) ;
#79702=CARTESIAN_POINT ( 'NONE',  ( 14.34966873604972726, -8.224510206698740333, 60.83442372801901854 ) ) ;
#79703=CARTESIAN_POINT ( 'NONE',  ( -9.474510206698964154, 16.51473224551069663, 30.41557627198102054 ) ) ;
#79705=CARTESIAN_POINT ( 'NONE',  ( 4.379528057220092307, 16.55341960407617563, 27.29275706135234358 ) ) ;
#79707=CARTESIAN_POINT ( 'NONE',  ( -16.51473224551082808, 9.474510206698731452, 88.33442372801900433 ) ) ;
#79708=CARTESIAN_POINT ( 'NONE',  ( 18.67979575497178502, 10.72451020669898547, 89.16557627198102409 ) ) ;
#79709=CARTESIAN_POINT ( 'NONE',  ( -16.51473224551082808, 9.474510206698731452, 48.33442372801900433 ) ) ;
#79710=CARTESIAN_POINT ( 'NONE',  ( 17.50000000000000000, -7.500000000000000888, 102.5000000000000142 ) ) ;
#79711=CARTESIAN_POINT ( 'NONE',  ( -5.719274019375978568, 21.55341960407610458, 110.2072429386477239 ) ) ;
#79712=CARTESIAN_POINT ( 'NONE',  ( -17.59860650958991002, -7.585241751807008548, 71.57662985737509587 ) ) ;
#79713=CARTESIAN_POINT ( 'NONE',  ( -16.51473224551069308, -9.474510206698971260, 76.66557627198103830 ) ) ;
#79714=CARTESIAN_POINT ( 'NONE',  ( 0.05219959533934541429, -16.53943276465976808, 30.00109039468568284 ) ) ;
#79716=CARTESIAN_POINT ( 'NONE',  ( 16.51473224551083163, -9.474510206698727899, 55.83442372801899722 ) ) ;
#79717=CARTESIAN_POINT ( 'NONE',  ( 10.81492255796106328, -18.62759615963255655, 20.41775706135234714 ) ) ;
#79718=CARTESIAN_POINT ( 'NONE',  ( -14.34966873604960291, -8.224510206698953496, 61.66557627198103120 ) ) ;
#79719=CARTESIAN_POINT ( 'NONE',  ( -19.05341960407611168, -5.049401038298163336, 66.45724293864769550 ) ) ;
#79720=CARTESIAN_POINT ( 'NONE',  ( -12.14591786802326823, 12.06949235617739902, 38.12609039468567573 ) ) ;
#79721=CARTESIAN_POINT ( 'NONE',  ( 5.049401038297881783, 19.05341960407617563, 47.29275706135231161 ) ) ;
#79722=CARTESIAN_POINT ( 'NONE',  ( -5.719274019375665041, -21.55341960407619695, 49.79275706135234714 ) ) ;
#79723=CARTESIAN_POINT ( 'NONE',  ( -19.03943276465977164, -0.05219959533935918106, 113.7510903946856757 ) ) ;
#79724=CARTESIAN_POINT ( 'NONE',  ( 13.97604488694527802, 13.89961937509977652, 59.37390960531434558 ) ) ;
#79725=CARTESIAN_POINT ( 'NONE',  ( -16.51473224551082808, 9.474510206698731452, 88.33442372801900433 ) ) ;
#79726=CARTESIAN_POINT ( 'NONE',  ( -18.67979575497193778, 10.72451020669871902, 93.33442372801901854 ) ) ;
#79727=CARTESIAN_POINT ( 'NONE',  ( -9.564922557961040184, 16.46253265017147172, 67.91775706135233293 ) ) ;
#79728=CARTESIAN_POINT ( 'NONE',  ( 16.51473224551069308, 9.474510206698969483, 39.16557627198103120 ) ) ;
#79729=CARTESIAN_POINT ( 'NONE',  ( -18.62759615963270932, 10.81492255796079327, 75.83224293864769550 ) ) ;
#79730=CARTESIAN_POINT ( 'NONE',  ( 8.314922557960818139, 14.29746914071049879, 59.58224293864770260 ) ) ;
#79731=CARTESIAN_POINT ( 'NONE',  ( -5.049401038297874678, -19.05341960407617918, 64.79275706135233293 ) ) ;
#79732=CARTESIAN_POINT ( 'NONE',  ( -16.81555441253554051, -7.025013491695444756, 24.36314554665744225 ) ) ;
#79733=CARTESIAN_POINT ( 'NONE',  ( 0.05219959533936267826, -19.03943276465977164, 25.00109039468566152 ) ) ;
#79734=CARTESIAN_POINT ( 'NONE',  ( -0.05219959533934338120, 16.53943276465976808, 92.50109039468567573 ) ) ;
#79735=CARTESIAN_POINT ( 'NONE',  ( -16.55341960407611168, -4.379528057220339221, 56.45724293864768839 ) ) ;
#79736=CARTESIAN_POINT ( 'NONE',  ( 5.823673210054444382, -21.52544592524334988, 85.20942372801901854 ) ) ;
#79738=CARTESIAN_POINT ( 'NONE',  ( 10.81492255796078972, 18.62759615963270932, 99.58224293864770971 ) ) ;
#79739=CARTESIAN_POINT ( 'NONE',  ( 5.049401038298161559, -19.05341960407611168, 57.70724293864769550 ) ) ;
#79740=CARTESIAN_POINT ( 'NONE',  ( 0.05219959533937995610, -21.53943276465977519, 70.00109039468568994 ) ) ;
#79741=CARTESIAN_POINT ( 'NONE',  ( 13.97604488694527802, 13.89961937509977652, 49.37390960531434558 ) ) ;
#79743=CARTESIAN_POINT ( 'NONE',  ( -16.51473224551069308, -9.474510206698971260, 66.66557627198102409 ) ) ;
#79744=CARTESIAN_POINT ( 'NONE',  ( -4.379528057220328563, 16.55341960407611168, 100.2072429386476955 ) ) ;
#79745=CARTESIAN_POINT ( 'NONE',  ( 16.51473224551069308, 9.474510206698969483, 109.1655762719810383 ) ) ;
#79746=CARTESIAN_POINT ( 'NONE',  ( -12.14591786802309592, -12.06949235617757132, 51.87390960531437401 ) ) ;
#79747=CARTESIAN_POINT ( 'NONE',  ( 13.97604488694527802, 13.89961937509977652, 34.37390960531436690 ) ) ;
#79748=CARTESIAN_POINT ( 'NONE',  ( 14.29746914071049879, -8.314922557960816363, 78.33224293864770971 ) ) ;
#79749=CARTESIAN_POINT ( 'NONE',  ( 18.67979575497178502, 10.72451020669898547, 99.16557627198100988 ) ) ;
#79750=CARTESIAN_POINT ( 'NONE',  ( 5.823673210054444382, -21.52544592524334988, 30.20942372801902565 ) ) ;
#79752=CARTESIAN_POINT ( 'NONE',  ( -12.14591786802326823, 12.06949235617739902, 53.12609039468568284 ) ) ;
#79753=CARTESIAN_POINT ( 'NONE',  ( -5.719274019375978568, 21.55341960407610458, 80.20724293864769550 ) ) ;
#79754=CARTESIAN_POINT ( 'NONE',  ( -15.80617190586768217, 15.72974639402176855, 108.1260903946856757 ) ) ;
#79755=CARTESIAN_POINT ( 'NONE',  ( -19.02544592524342804, 5.153800228976336051, 106.0405762719810241 ) ) ;
#79756=CARTESIAN_POINT ( 'NONE',  ( -0.05219959533937732626, 21.53943276465977519, 37.50109039468568284 ) ) ;
#79757=CARTESIAN_POINT ( 'NONE',  ( -10.81492255796078084, -18.62759615963271287, 37.08224293864768129 ) ) ;
#79758=CARTESIAN_POINT ( 'NONE',  ( 8.224510206698742110, 14.34966873604972548, 97.08442372801904696 ) ) ;
#79759=CARTESIAN_POINT ( 'NONE',  ( 10.72451020669871369, 18.67979575497193778, 67.08442372801901854 ) ) ;
#79760=CARTESIAN_POINT ( 'NONE',  ( 10.81492255796106328, -18.62759615963255655, 85.41775706135236135 ) ) ;
#79761=CARTESIAN_POINT ( 'NONE',  ( -9.564922557961040184, 16.46253265017147172, 27.91775706135232582 ) ) ;
#79762=CARTESIAN_POINT ( 'NONE',  ( 12.14591786802327356, -12.06949235617739191, 90.62609039468567573 ) ) ;
#79763=CARTESIAN_POINT ( 'NONE',  ( 10.81492255796106328, -18.62759615963255655, 35.41775706135234003 ) ) ;
#79764=CARTESIAN_POINT ( 'NONE',  ( 0.05219959533909260263, 19.03943276465977164, 44.99890960531435979 ) ) ;
#79765=CARTESIAN_POINT ( 'NONE',  ( 10.81492255796106328, -18.62759615963255655, 105.4177570613523613 ) ) ;
#79766=CARTESIAN_POINT ( 'NONE',  ( 15.72974639402199770, -15.80617190586745480, 23.12390960531436335 ) ) ;
#79768=CARTESIAN_POINT ( 'NONE',  ( -10.72451020669870658, -18.67979575497194134, 24.58442372801901499 ) ) ;
#79769=CARTESIAN_POINT ( 'NONE',  ( 10.72451020669898902, -18.67979575497178502, 77.91557627198102409 ) ) ;
#79771=CARTESIAN_POINT ( 'NONE',  ( 5.823673210054125526, 21.52544592524343514, 69.79057627198102409 ) ) ;
#79772=CARTESIAN_POINT ( 'NONE',  ( -16.55341960407617563, 4.379528057220093196, 58.54275706135235424 ) ) ;
#79773=CARTESIAN_POINT ( 'NONE',  ( 16.55341960407611168, 4.379528057220329451, 58.95724293864770971 ) ) ;
#79775=CARTESIAN_POINT ( 'NONE',  ( 5.153800228976615827, -19.02544592524334988, 95.20942372801897591 ) ) ;
#79777=CARTESIAN_POINT ( 'NONE',  ( -16.55341960407617563, 4.379528057220093196, 23.54275706135235424 ) ) ;
#79778=CARTESIAN_POINT ( 'NONE',  ( 10.72451020669898902, -18.67979575497178502, 97.91557627198103830 ) ) ;
#79779=CARTESIAN_POINT ( 'NONE',  ( 21.52544592524344225, -5.823673210054117533, 78.54057627198103830 ) ) ;
#79780=CARTESIAN_POINT ( 'NONE',  ( 5.153800228976335163, 19.02544592524342804, 114.7905762719810241 ) ) ;
#79781=CARTESIAN_POINT ( 'NONE',  ( -16.53943276465976808, -0.05219959533934237506, 53.75109039468568994 ) ) ;
#79782=CARTESIAN_POINT ( 'NONE',  ( -13.89961937509977652, 13.97604488694528158, 65.62390960531436690 ) ) ;
#79783=CARTESIAN_POINT ( 'NONE',  ( -21.53943276465977519, -0.05219959533937600094, 38.75109039468567573 ) ) ;
#79784=CARTESIAN_POINT ( 'NONE',  ( 19.05341960407617918, -5.049401038297876454, 111.0427570613523329 ) ) ;
#79785=CARTESIAN_POINT ( 'NONE',  ( 13.89961937509977652, -13.97604488694527269, 103.1239096053143527 ) ) ;
#79786=CARTESIAN_POINT ( 'NONE',  ( 5.153800228976615827, -19.02544592524334988, 30.20942372801900433 ) ) ;
#79787=CARTESIAN_POINT ( 'NONE',  ( -5.049401038298153566, 19.05341960407611168, 105.2072429386476671 ) ) ;
#79788=CARTESIAN_POINT ( 'NONE',  ( 21.55341960407610458, 5.719274019375980345, 103.9572429386476813 ) ) ;
#79789=CARTESIAN_POINT ( 'NONE',  ( 16.46253265017160672, -9.564922557960803928, 63.33224293864769550 ) ) ;
#79791=CARTESIAN_POINT ( 'NONE',  ( -16.55341960407611168, -4.379528057220339221, 76.45724293864769550 ) ) ;
#79792=CARTESIAN_POINT ( 'NONE',  ( -9.474510206698964154, 16.51473224551069663, 110.4155762719810383 ) ) ;
#79793=CARTESIAN_POINT ( 'NONE',  ( 0.05219959533909260263, 19.03943276465977164, 24.99890960531435269 ) ) ;
#79794=CARTESIAN_POINT ( 'NONE',  ( -10.72451020669898014, 18.67979575497178502, 100.4155762719810241 ) ) ;
#79795=CARTESIAN_POINT ( 'NONE',  ( 19.02544592524334988, 5.153800228976608722, 66.45942372801899012 ) ) ;
#79796=CARTESIAN_POINT ( 'NONE',  ( 9.474510206698971260, -16.51473224551069308, 112.9155762719810383 ) ) ;
#79797=CARTESIAN_POINT ( 'NONE',  ( -19.02544592524342804, 5.153800228976336051, 31.04057627198102409 ) ) ;
#79798=CARTESIAN_POINT ( 'NONE',  ( -21.53943276465977519, 0.05219959533907696930, 56.24890960531436690 ) ) ;
#79800=CARTESIAN_POINT ( 'NONE',  ( 5.049401038298161559, -19.05341960407611168, 97.70724293864766707 ) ) ;
#79801=CARTESIAN_POINT ( 'NONE',  ( -5.823673210054431948, 21.52544592524334988, 72.70942372801901854 ) ) ;
#79802=CARTESIAN_POINT ( 'NONE',  ( 16.51473224551069308, 9.474510206698969483, 54.16557627198103120 ) ) ;
#79803=CARTESIAN_POINT ( 'NONE',  ( 12.06949235617757843, -12.14591786802309237, 88.12390960531436690 ) ) ;
#79804=CARTESIAN_POINT ( 'NONE',  ( -12.06949235617739369, -12.14591786802326823, 39.37609039468567573 ) ) ;
#79805=CARTESIAN_POINT ( 'NONE',  ( 18.62759615963255655, 10.81492255796105972, 61.66775706135235424 ) ) ;
#79807=CARTESIAN_POINT ( 'NONE',  ( 19.05341960407617918, -5.049401038297876454, 31.04275706135232227 ) ) ;
#79808=CARTESIAN_POINT ( 'NONE',  ( -19.03943276465977164, -0.05219959533935918106, 83.75109039468567573 ) ) ;
#79809=CARTESIAN_POINT ( 'NONE',  ( -19.05341960407617563, 5.049401038297882671, 38.54275706135233293 ) ) ;
#79811=CARTESIAN_POINT ( 'NONE',  ( -18.67979575497193778, 10.72451020669871902, 38.33442372801900433 ) ) ;
#79815=CARTESIAN_POINT ( 'NONE',  ( -5.153800228976607833, 19.02544592524334988, 32.70942372801899722 ) ) ;
#79816=CARTESIAN_POINT ( 'NONE',  ( -13.89961937509977652, 13.97604488694528158, 65.62390960531436690 ) ) ;
#79817=CARTESIAN_POINT ( 'NONE',  ( -16.55341960407617563, 4.379528057220093196, 113.5427570613523756 ) ) ;
#79818=CARTESIAN_POINT ( 'NONE',  ( 0.05219959533907565091, 21.53943276465977519, 24.99890960531435624 ) ) ;
#79819=CARTESIAN_POINT ( 'NONE',  ( -18.62759615963255300, -10.81492255796106328, 89.16775706135236135 ) ) ;
#79821=CARTESIAN_POINT ( 'NONE',  ( -17.50000000000002487, -3.805241302050037522, 34.62647527217417576 ) ) ;
#79822=CARTESIAN_POINT ( 'NONE',  ( 5.719274019375673035, 21.55341960407619339, 82.29275706135234714 ) ) ;
#79824=CARTESIAN_POINT ( 'NONE',  ( 9.564922557960805705, 16.46253265017160317, 99.58224293864770971 ) ) ;
#79827=CARTESIAN_POINT ( 'NONE',  ( -9.474510206698964154, 16.51473224551069663, 55.41557627198103120 ) ) ;
#79828=CARTESIAN_POINT ( 'NONE',  ( -18.62759615963270932, 10.81492255796079327, 50.83224293864770971 ) ) ;
#79829=CARTESIAN_POINT ( 'NONE',  ( -0.05219959533910754901, -16.53943276465976808, 27.49890960531435269 ) ) ;
#79830=CARTESIAN_POINT ( 'NONE',  ( 12.14591786802309770, 12.06949235617756955, 109.3739096053143811 ) ) ;
#79831=CARTESIAN_POINT ( 'NONE',  ( -13.89961937509977652, 13.97604488694528158, 90.62390960531432427 ) ) ;
#79832=CARTESIAN_POINT ( 'NONE',  ( 19.03943276465977164, 0.05219959533936151252, 21.25109039468565797 ) ) ;
#79833=CARTESIAN_POINT ( 'NONE',  ( -16.55341960407611168, -4.379528057220339221, 96.45724293864770971 ) ) ;
#79834=CARTESIAN_POINT ( 'NONE',  ( 5.823673210054444382, -21.52544592524334988, 65.20942372801901854 ) ) ;
#79835=CARTESIAN_POINT ( 'NONE',  ( 19.03943276465977164, -0.05219959533909143690, 113.7489096053143669 ) ) ;
#79836=CARTESIAN_POINT ( 'NONE',  ( 4.379528057220092307, 16.55341960407617563, 102.2927570613523613 ) ) ;
#79837=CARTESIAN_POINT ( 'NONE',  ( -5.049401038297874678, -19.05341960407617918, 64.79275706135233293 ) ) ;
#79839=CARTESIAN_POINT ( 'NONE',  ( 5.153800228976335163, 19.02544592524342804, 114.7905762719810241 ) ) ;
#79840=CARTESIAN_POINT ( 'NONE',  ( -4.483927247898539470, -16.52544592524342804, 82.29057627198103830 ) ) ;
#79841=CARTESIAN_POINT ( 'NONE',  ( -5.153800228976607833, 19.02544592524334988, 62.70942372801899722 ) ) ;
#79843=CARTESIAN_POINT ( 'NONE',  ( -5.049401038298153566, 19.05341960407611168, 60.20724293864768129 ) ) ;
#79844=CARTESIAN_POINT ( 'NONE',  ( -4.483927247898539470, -16.52544592524342804, 62.29057627198102409 ) ) ;
#79845=CARTESIAN_POINT ( 'NONE',  ( 5.049401038297881783, 19.05341960407617563, 87.29275706135234714 ) ) ;
#79846=CARTESIAN_POINT ( 'NONE',  ( -10.72451020669898014, 18.67979575497178502, 50.41557627198103120 ) ) ;
#79847=ORIENTED_EDGE ( 'NONE', *, *, #192729, .T. ) ;
#79848=CARTESIAN_POINT ( 'NONE',  ( 0.05219959533909260263, 19.03943276465977164, 24.99890960531435269 ) ) ;
#79849=CARTESIAN_POINT ( 'NONE',  ( -16.38665767535053064, -7.295008042176051255, 29.73599135785456227 ) ) ;
#79850=CARTESIAN_POINT ( 'NONE',  ( -13.89961937509977652, 13.97604488694528158, 60.62390960531436690 ) ) ;
#79851=CARTESIAN_POINT ( 'NONE',  ( 18.67979575497178502, 10.72451020669898547, 59.16557627198103120 ) ) ;
#79852=CARTESIAN_POINT ( 'NONE',  ( -14.34966873604972548, 8.224510206698743886, 88.33442372801901854 ) ) ;
#79853=CARTESIAN_POINT ( 'NONE',  ( 0.05219959533909260263, 19.03943276465977164, 69.99890960531435269 ) ) ;
#79854=CARTESIAN_POINT ( 'NONE',  ( -9.564922557961040184, 16.46253265017147172, 47.91775706135233293 ) ) ;
#79855=EDGE_CURVE ( 'NONE', #133811, #120648, #79681, .T. ) ;
#79856=CARTESIAN_POINT ( 'NONE',  ( 21.53943276465977519, 0.05219959533937863772, 81.25109039468568994 ) ) ;
#79857=CARTESIAN_POINT ( 'NONE',  ( 10.81492255796078972, 18.62759615963270932, 64.58224293864769550 ) ) ;
#79858=CARTESIAN_POINT ( 'NONE',  ( -16.51473224551069308, -9.474510206698971260, 101.6655762719810241 ) ) ;
#79859=CARTESIAN_POINT ( 'NONE',  ( 19.02544592524343514, -5.153800228976328945, 38.54057627198103120 ) ) ;
#79860=CARTESIAN_POINT ( 'NONE',  ( 14.34966873604972726, -8.224510206698740333, 90.83442372801901854 ) ) ;
#79861=CARTESIAN_POINT ( 'NONE',  ( 9.474510206698729675, 16.51473224551082808, 112.0844237280190043 ) ) ;
#79863=CARTESIAN_POINT ( 'NONE',  ( -15.72974639402176322, -15.80617190586768395, 99.37609039468568994 ) ) ;
#79864=CARTESIAN_POINT ( 'NONE',  ( -12.14591786802309592, -12.06949235617757132, 61.87390960531436690 ) ) ;
#79865=CARTESIAN_POINT ( 'NONE',  ( -8.314922557960811034, -14.29746914071050412, 67.08224293864770971 ) ) ;
#79866=CARTESIAN_POINT ( 'NONE',  ( 5.823673210054125526, 21.52544592524343514, 99.79057627198103830 ) ) ;
#79867=CARTESIAN_POINT ( 'NONE',  ( 21.55341960407610458, 5.719274019375980345, 83.95724293864770971 ) ) ;
#79868=CARTESIAN_POINT ( 'NONE',  ( 17.40861289039002457, -6.110651285853308856, 96.12767529172566583 ) ) ;
#79869=CARTESIAN_POINT ( 'NONE',  ( -18.67979575497178146, -10.72451020669898902, 51.66557627198102409 ) ) ;
#79870=CARTESIAN_POINT ( 'NONE',  ( -8.224510206698735004, -14.34966873604973081, 64.58442372801900433 ) ) ;
#79871=CARTESIAN_POINT ( 'NONE',  ( -16.53943276465976808, 0.05219959533911058130, 96.24890960531435269 ) ) ;
#79872=CARTESIAN_POINT ( 'NONE',  ( -16.51473224551069308, -9.474510206698971260, 46.66557627198102409 ) ) ;
#79874=CARTESIAN_POINT ( 'NONE',  ( -14.34966873604972548, 8.224510206698743886, 93.33442372801901854 ) ) ;
#79875=CARTESIAN_POINT ( 'NONE',  ( -18.67979575497193778, 10.72451020669871902, 38.33442372801900433 ) ) ;
#79876=CARTESIAN_POINT ( 'NONE',  ( -16.46253265017160317, 9.564922557960807481, 85.83224293864769550 ) ) ;
#79877=CARTESIAN_POINT ( 'NONE',  ( 21.53943276465977519, 0.05219959533937863772, 61.25109039468567573 ) ) ;
#79879=CARTESIAN_POINT ( 'NONE',  ( 5.153800228976335163, 19.02544592524342804, 29.79057627198102409 ) ) ;
#79881=CARTESIAN_POINT ( 'NONE',  ( 10.81492255796106328, -18.62759615963255655, 65.41775706135234714 ) ) ;
#79882=CARTESIAN_POINT ( 'NONE',  ( 5.049401038298161559, -19.05341960407611168, 32.70724293864768129 ) ) ;
#79883=CARTESIAN_POINT ( 'NONE',  ( -13.97604488694527625, -13.89961937509977652, 91.87390960531432427 ) ) ;
#79884=CARTESIAN_POINT ( 'NONE',  ( -13.97604488694547697, 13.89961937509957934, 68.12609039468563310 ) ) ;
#79885=CARTESIAN_POINT ( 'NONE',  ( -5.719274019375665041, -21.55341960407619695, 24.79275706135235779 ) ) ;
#79886=CARTESIAN_POINT ( 'NONE',  ( -5.049401038297874678, -19.05341960407617918, 54.79275706135234003 ) ) ;
#79887=CARTESIAN_POINT ( 'NONE',  ( -19.03943276465977164, 0.05219959533909376836, 36.24890960531436690 ) ) ;
#79888=CARTESIAN_POINT ( 'NONE',  ( -16.53943276465976808, -0.05219959533934237506, 98.75109039468568994 ) ) ;
#79889=CARTESIAN_POINT ( 'NONE',  ( -5.049401038297874678, -19.05341960407617918, 69.79275706135233293 ) ) ;
#79890=CARTESIAN_POINT ( 'NONE',  ( -16.55341960407611168, -4.379528057220339221, 26.45724293864768839 ) ) ;
#79891=CARTESIAN_POINT ( 'NONE',  ( -0.05219959533936034679, 19.03943276465977164, 52.50109039468566863 ) ) ;
#79892=CARTESIAN_POINT ( 'NONE',  ( 19.02544592524343514, -5.153800228976328945, 103.5405762719809957 ) ) ;
#79893=CARTESIAN_POINT ( 'NONE',  ( -21.53943276465977519, -0.05219959533937600094, 108.7510903946857042 ) ) ;
#79894=CARTESIAN_POINT ( 'NONE',  ( -5.823673210054431948, 21.52544592524334988, 112.7094237280190328 ) ) ;
#79895=CARTESIAN_POINT ( 'NONE',  ( 5.049401038298161559, -19.05341960407611168, 27.70724293864769550 ) ) ;
#79896=CARTESIAN_POINT ( 'NONE',  ( -5.719274019375665041, -21.55341960407619695, 89.79275706135236135 ) ) ;
#79897=CARTESIAN_POINT ( 'NONE',  ( -16.52544592524335698, -4.483927247898792601, 33.95942372801901143 ) ) ;
#79898=CARTESIAN_POINT ( 'NONE',  ( 13.89961937509977652, -13.97604488694527269, 93.12390960531436690 ) ) ;
#79900=CARTESIAN_POINT ( 'NONE',  ( 9.564922557960805705, 16.46253265017160317, 74.58224293864769550 ) ) ;
#79901=LINE ( 'NONE', #64737, #120105 ) ;
#79902=CARTESIAN_POINT ( 'NONE',  ( 5.153800228976615827, -19.02544592524334988, 65.20942372801900433 ) ) ;
#79903=CARTESIAN_POINT ( 'NONE',  ( -19.02544592524342804, 5.153800228976336051, 111.0405762719810099 ) ) ;
#79904=CARTESIAN_POINT ( 'NONE',  ( 18.67979575497194134, -10.72451020669871369, 95.83442372801903275 ) ) ;
#79905=CARTESIAN_POINT ( 'NONE',  ( 4.379528057220339221, -16.55341960407611168, 102.7072429386476955 ) ) ;
#79906=CARTESIAN_POINT ( 'NONE',  ( 21.55341960407610458, 5.719274019375980345, 48.95724293864770971 ) ) ;
#79907=CARTESIAN_POINT ( 'NONE',  ( 5.823673210054125526, 21.52544592524343514, 34.79057627198103120 ) ) ;
#79908=CARTESIAN_POINT ( 'NONE',  ( 4.483927247898545687, 16.52544592524342804, 109.7905762719810383 ) ) ;
#79910=CARTESIAN_POINT ( 'NONE',  ( -13.89961937509957401, -13.97604488694547875, 59.37609039468566863 ) ) ;
#79911=CARTESIAN_POINT ( 'NONE',  ( -12.14591786802326823, 12.06949235617739902, 113.1260903946856899 ) ) ;
#79912=CARTESIAN_POINT ( 'NONE',  ( 0.05219959533909260263, 19.03943276465977164, 114.9989096053143669 ) ) ;
#79913=CARTESIAN_POINT ( 'NONE',  ( 18.62759615963255655, 10.81492255796105972, 81.66775706135236135 ) ) ;
#79914=CARTESIAN_POINT ( 'NONE',  ( -15.72974639402197994, 15.80617190586746368, 70.62390960531436690 ) ) ;
#79915=CARTESIAN_POINT ( 'NONE',  ( 5.823673210054444382, -21.52544592524334988, 40.20942372801901854 ) ) ;
#79916=CARTESIAN_POINT ( 'NONE',  ( 0.05219959533907565091, 21.53943276465977519, 99.99890960531436690 ) ) ;
#79917=CARTESIAN_POINT ( 'NONE',  ( -21.53943276465977519, -0.05219959533937600094, 53.75109039468568994 ) ) ;
#79918=CARTESIAN_POINT ( 'NONE',  ( 9.474510206698971260, -16.51473224551069308, 32.91557627198102409 ) ) ;
#79919=CARTESIAN_POINT ( 'NONE',  ( -5.049401038298153566, 19.05341960407611168, 80.20724293864769550 ) ) ;
#79920=CARTESIAN_POINT ( 'NONE',  ( -4.483927247898782831, 16.52544592524335698, 82.70942372801900433 ) ) ;
#79921=CARTESIAN_POINT ( 'NONE',  ( -16.53943276465976808, 0.05219959533911058130, 101.2489096053143669 ) ) ;
#79922=CARTESIAN_POINT ( 'NONE',  ( -5.049401038298153566, 19.05341960407611168, 105.2072429386476671 ) ) ;
#79923=CARTESIAN_POINT ( 'NONE',  ( -12.14591786802309592, -12.06949235617757132, 51.87390960531437401 ) ) ;
#79924=CARTESIAN_POINT ( 'NONE',  ( 8.224510206698742110, 14.34966873604972548, 112.0844237280190185 ) ) ;
#79925=CARTESIAN_POINT ( 'NONE',  ( 5.153800228976335163, 19.02544592524342804, 59.79057627198100988 ) ) ;
#79926=CARTESIAN_POINT ( 'NONE',  ( -19.02544592524342804, 5.153800228976336051, 41.04057627198103120 ) ) ;
#79927=CARTESIAN_POINT ( 'NONE',  ( 10.72451020669898902, -18.67979575497178502, 47.91557627198102409 ) ) ;
#79928=CARTESIAN_POINT ( 'NONE',  ( 13.97604488694548053, -13.89961937509957401, 35.62609039468567573 ) ) ;
#79929=VECTOR ( 'NONE', #67173, 1000.000000000000000 ) ;
#79931=CARTESIAN_POINT ( 'NONE',  ( 0.05219959533910956823, 16.53943276465976808, 39.99890960531436690 ) ) ;
#79932=CARTESIAN_POINT ( 'NONE',  ( 19.05341960407611168, 5.049401038298154454, 103.9572429386476671 ) ) ;
#79933=CARTESIAN_POINT ( 'NONE',  ( 5.823673210054444382, -21.52544592524334988, 45.20942372801901854 ) ) ;
#79935=CARTESIAN_POINT ( 'NONE',  ( -9.564922557960796823, -16.46253265017161027, 112.0822429386476955 ) ) ;
#79936=CARTESIAN_POINT ( 'NONE',  ( -12.06949235617739369, -12.14591786802326823, 59.37609039468568284 ) ) ;
#79937=CARTESIAN_POINT ( 'NONE',  ( 0.05219959533936267826, -19.03943276465977164, 60.00109039468566863 ) ) ;
#79938=CARTESIAN_POINT ( 'NONE',  ( 12.06949235617757843, -12.14591786802309237, 33.12390960531435979 ) ) ;
#79939=CARTESIAN_POINT ( 'NONE',  ( -17.49999999999999645, 5.499999999999997335, 120.0000000000000142 ) ) ;
#79940=CARTESIAN_POINT ( 'NONE',  ( -0.05219959533934338120, 16.53943276465976808, 107.5010903946856899 ) ) ;
#79941=CARTESIAN_POINT ( 'NONE',  ( 16.51473224551069308, 9.474510206698969483, 34.16557627198102409 ) ) ;
#79942=CARTESIAN_POINT ( 'NONE',  ( 19.02544592524343514, -5.153800228976328945, 63.54057627198103830 ) ) ;
#79943=CARTESIAN_POINT ( 'NONE',  ( -19.05341960407611168, -5.049401038298163336, 31.45724293864769550 ) ) ;
#79944=CARTESIAN_POINT ( 'NONE',  ( -21.53943276465977519, -0.05219959533937600094, 28.75109039468567929 ) ) ;
#79945=CARTESIAN_POINT ( 'NONE',  ( -9.474510206698964154, 16.51473224551069663, 40.41557627198103120 ) ) ;
#79946=CARTESIAN_POINT ( 'NONE',  ( -0.05219959533909027116, -19.03943276465977164, 112.4989096053143669 ) ) ;
#79947=CARTESIAN_POINT ( 'NONE',  ( -5.153800228976328057, -19.02544592524343514, 47.29057627198102409 ) ) ;
#79948=CARTESIAN_POINT ( 'NONE',  ( 19.02544592524343514, -5.153800228976328945, 113.5405762719810241 ) ) ;
#79949=CARTESIAN_POINT ( 'NONE',  ( -0.05219959533937732626, 21.53943276465977519, 52.50109039468567573 ) ) ;
#79950=CARTESIAN_POINT ( 'NONE',  ( -16.53943276465976808, 0.05219959533911058130, 111.2489096053143669 ) ) ;
#79951=CARTESIAN_POINT ( 'NONE',  ( 21.52544592524344225, -5.823673210054117533, 28.54057627198103120 ) ) ;
#79952=CARTESIAN_POINT ( 'NONE',  ( 8.224510206698742110, 14.34966873604972548, 72.08442372801899012 ) ) ;
#79953=CARTESIAN_POINT ( 'NONE',  ( -21.55341960407619339, 5.719274019375674811, 98.54275706135234714 ) ) ;
#79955=CARTESIAN_POINT ( 'NONE',  ( 8.224510206698742110, 14.34966873604972548, 52.08442372801901854 ) ) ;
#79956=CARTESIAN_POINT ( 'NONE',  ( -5.049401038298153566, 19.05341960407611168, 90.20724293864766707 ) ) ;
#79957=CARTESIAN_POINT ( 'NONE',  ( 0.05219959533934541429, -16.53943276465976808, 45.00109039468568284 ) ) ;
#79958=CARTESIAN_POINT ( 'NONE',  ( -4.483927247898782831, 16.52544592524335698, 27.70942372801901854 ) ) ;
#79959=CARTESIAN_POINT ( 'NONE',  ( -14.29746914071037622, -8.314922557961029526, 99.16775706135234714 ) ) ;
#79960=CARTESIAN_POINT ( 'NONE',  ( -18.67979575497193778, 10.72451020669871902, 58.33442372801901143 ) ) ;
#79961=CARTESIAN_POINT ( 'NONE',  ( 5.153800228976615827, -19.02544592524334988, 105.2094237280190185 ) ) ;
#79962=CARTESIAN_POINT ( 'NONE',  ( -18.62759615963270932, 10.81492255796079327, 110.8322429386476955 ) ) ;
#79963=CARTESIAN_POINT ( 'NONE',  ( -4.483927247898539470, -16.52544592524342804, 102.2905762719810383 ) ) ;
#79964=CARTESIAN_POINT ( 'NONE',  ( 16.51473224551083163, -9.474510206698727899, 105.8344237280190043 ) ) ;
#79965=CARTESIAN_POINT ( 'NONE',  ( -4.483927247898782831, 16.52544592524335698, 77.70942372801900433 ) ) ;
#79966=CARTESIAN_POINT ( 'NONE',  ( -16.21995358207275473, 7.366697692864369706, 44.93551001512068410 ) ) ;
#79967=CARTESIAN_POINT ( 'NONE',  ( -19.02544592524334988, -5.153800228976617603, 78.95942372801900433 ) ) ;
#79969=CARTESIAN_POINT ( 'NONE',  ( -14.29746914071049879, 8.314922557960819915, 50.83224293864770971 ) ) ;
#79970=CARTESIAN_POINT ( 'NONE',  ( 4.483927247898545687, 16.52544592524342804, 39.79057627198103830 ) ) ;
#79971=CARTESIAN_POINT ( 'NONE',  ( 16.53943276465976808, -0.05219959533910856209, 98.74890960531438111 ) ) ;
#79972=CARTESIAN_POINT ( 'NONE',  ( -19.05341960407617563, 5.049401038297882671, 38.54275706135233293 ) ) ;
#79973=CARTESIAN_POINT ( 'NONE',  ( -18.39443945427639093, 5.500000000000031974, 88.51745347608650150 ) ) ;
#79974=CARTESIAN_POINT ( 'NONE',  ( 15.80617190586769283, -15.72974639402175789, 35.62609039468568994 ) ) ;
#79975=CARTESIAN_POINT ( 'NONE',  ( 5.153800228976615827, -19.02544592524334988, 100.2094237280190043 ) ) ;
#79977=CARTESIAN_POINT ( 'NONE',  ( 19.05341960407611168, 5.049401038298154454, 88.95724293864769550 ) ) ;
#79978=CARTESIAN_POINT ( 'NONE',  ( -16.46253265017160317, 9.564922557960807481, 95.83224293864769550 ) ) ;
#79979=CARTESIAN_POINT ( 'NONE',  ( 10.81492255796078972, 18.62759615963270932, 59.58224293864770260 ) ) ;
#79980=CARTESIAN_POINT ( 'NONE',  ( -4.483927247898539470, -16.52544592524342804, 92.29057627198103830 ) ) ;
#79981=CARTESIAN_POINT ( 'NONE',  ( 19.03943276465977164, -0.05219959533909143690, 68.74890960531436690 ) ) ;
#79982=CARTESIAN_POINT ( 'NONE',  ( 19.02544592524343514, -5.153800228976328945, 23.54057627198102054 ) ) ;
#79983=CARTESIAN_POINT ( 'NONE',  ( 21.52544592524334988, 5.823673210054432836, 41.45942372801901143 ) ) ;
#79984=CARTESIAN_POINT ( 'NONE',  ( 5.823673210054444382, -21.52544592524334988, 70.20942372801904696 ) ) ;
#79985=CARTESIAN_POINT ( 'NONE',  ( -12.14591786802326823, 12.06949235617739902, 93.12609039468568994 ) ) ;
#79986=CARTESIAN_POINT ( 'NONE',  ( -18.67979575497193778, 10.72451020669871902, 23.33442372801901499 ) ) ;
#79987=CARTESIAN_POINT ( 'NONE',  ( 21.55341960407619695, -5.719274019375665929, 21.04275706135234714 ) ) ;
#79988=CARTESIAN_POINT ( 'NONE',  ( 16.46253265017146816, 9.564922557961045513, 56.66775706135233293 ) ) ;
#79989=CARTESIAN_POINT ( 'NONE',  ( 0.05219959533909260263, 19.03943276465977164, 74.99890960531435269 ) ) ;
#79990=CARTESIAN_POINT ( 'NONE',  ( 21.53943276465977519, 0.05219959533937863772, 81.25109039468568994 ) ) ;
#79991=CARTESIAN_POINT ( 'NONE',  ( 10.81492255796078972, 18.62759615963270932, 89.58224293864768129 ) ) ;
#79992=CARTESIAN_POINT ( 'NONE',  ( 12.06949235617757843, -12.14591786802309237, 48.12390960531436690 ) ) ;
#79993=CARTESIAN_POINT ( 'NONE',  ( 21.52544592524334988, 5.823673210054432836, 101.4594237280190185 ) ) ;
#79994=CARTESIAN_POINT ( 'NONE',  ( -16.46253265017146816, -9.564922557961047289, 34.16775706135233293 ) ) ;
#79995=CARTESIAN_POINT ( 'NONE',  ( -12.06949235617756955, 12.14591786802309770, 75.62390960531439532 ) ) ;
#79996=CARTESIAN_POINT ( 'NONE',  ( 12.06949235617757843, -12.14591786802309237, 113.1239096053143953 ) ) ;
#79997=CARTESIAN_POINT ( 'NONE',  ( 16.51473224551083163, -9.474510206698727899, 75.83442372801900433 ) ) ;
#79998=CARTESIAN_POINT ( 'NONE',  ( 0.05219959533910956823, 16.53943276465976808, 39.99890960531436690 ) ) ;
#79999=CARTESIAN_POINT ( 'NONE',  ( -15.80617190586768217, 15.72974639402176855, 83.12609039468568994 ) ) ;
#80000=CARTESIAN_POINT ( 'NONE',  ( 5.049401038298161559, -19.05341960407611168, 77.70724293864765286 ) ) ;
#80001=CARTESIAN_POINT ( 'NONE',  ( 19.05341960407617918, -5.049401038297876454, 66.04275706135233293 ) ) ;
#80002=CARTESIAN_POINT ( 'NONE',  ( 0.05219959533907565091, 21.53943276465977519, 64.99890960531435269 ) ) ;
#80003=CARTESIAN_POINT ( 'NONE',  ( 0.05219959533907565091, 21.53943276465977519, 109.9989096053143527 ) ) ;
#80004=CARTESIAN_POINT ( 'NONE',  ( 19.03943276465977164, 0.05219959533936151252, 111.2510903946856757 ) ) ;
#80005=CARTESIAN_POINT ( 'NONE',  ( 14.34966873604972726, -8.224510206698740333, 80.83442372801901854 ) ) ;
#80007=CARTESIAN_POINT ( 'NONE',  ( -18.67979575497193778, 10.72451020669871902, 23.33442372801901499 ) ) ;
#80008=CARTESIAN_POINT ( 'NONE',  ( 8.224510206698953496, -14.34966873604960469, 102.9155762719810383 ) ) ;
#80010=CARTESIAN_POINT ( 'NONE',  ( 16.52544592524335698, 4.483927247898782831, 41.45942372801901143 ) ) ;
#80011=CARTESIAN_POINT ( 'NONE',  ( -10.81492255796078084, -18.62759615963271287, 57.08224293864769550 ) ) ;
#80012=CARTESIAN_POINT ( 'NONE',  ( -16.53943276465976808, -0.05219959533934237506, 98.75109039468568994 ) ) ;
#80013=CARTESIAN_POINT ( 'NONE',  ( 16.51473224551069308, 9.474510206698969483, 29.16557627198103475 ) ) ;
#80014=CARTESIAN_POINT ( 'NONE',  ( 0.05219959533934541429, -16.53943276465976808, 80.00109039468568994 ) ) ;
#80015=CARTESIAN_POINT ( 'NONE',  ( 0.05219959533936267826, -19.03943276465977164, 70.00109039468566152 ) ) ;
#80016=CARTESIAN_POINT ( 'NONE',  ( 10.72451020669871369, 18.67979575497193778, 37.08442372801901143 ) ) ;
#80017=CARTESIAN_POINT ( 'NONE',  ( -15.80617190586745835, -15.72974639402198527, 61.87390960531436690 ) ) ;
#80018=CARTESIAN_POINT ( 'NONE',  ( -4.483927247898782831, 16.52544592524335698, 92.70942372801901854 ) ) ;
#80019=CARTESIAN_POINT ( 'NONE',  ( 21.55341960407619695, -5.719274019375665929, 86.04275706135236135 ) ) ;
#80020=CARTESIAN_POINT ( 'NONE',  ( -10.72451020669898014, 18.67979575497178502, 50.41557627198103120 ) ) ;
#80021=CARTESIAN_POINT ( 'NONE',  ( 21.53943276465977519, -0.05219959533907433946, 43.74890960531435979 ) ) ;
#80022=CARTESIAN_POINT ( 'NONE',  ( -12.14591786802326823, 12.06949235617739902, 83.12609039468568994 ) ) ;
#80023=CARTESIAN_POINT ( 'NONE',  ( -21.55341960407610458, -5.719274019375992779, 51.45724293864770260 ) ) ;
#80024=ORIENTED_EDGE ( 'NONE', *, *, #117330, .F. ) ;
#80025=CARTESIAN_POINT ( 'NONE',  ( 0.05219959533909260263, 19.03943276465977164, 104.9989096053143669 ) ) ;
#80027=CARTESIAN_POINT ( 'NONE',  ( 19.03943276465977164, -0.05219959533909143690, 23.74890960531435269 ) ) ;
#80028=CARTESIAN_POINT ( 'NONE',  ( -15.80617190586745835, -15.72974639402198527, 66.87390960531436690 ) ) ;
#80029=CARTESIAN_POINT ( 'NONE',  ( -4.483927247898782831, 16.52544592524335698, 92.70942372801901854 ) ) ;
#80030=CARTESIAN_POINT ( 'NONE',  ( 18.62759615963255655, 10.81492255796105972, 46.66775706135234714 ) ) ;
#80031=CARTESIAN_POINT ( 'NONE',  ( -9.474510206698720793, -16.51473224551083518, 99.58442372801900433 ) ) ;
#80032=CARTESIAN_POINT ( 'NONE',  ( 14.29746914071049879, -8.314922557960816363, 103.3322429386476955 ) ) ;
#80033=CARTESIAN_POINT ( 'NONE',  ( 16.53943276465976808, 0.05219959533934440121, 21.25109039468567218 ) ) ;
#80034=CARTESIAN_POINT ( 'NONE',  ( 13.89961937509977652, -13.97604488694527269, 43.12390960531434558 ) ) ;
#80036=CARTESIAN_POINT ( 'NONE',  ( 19.03943276465977164, -0.05219959533909143690, 88.74890960531436690 ) ) ;
#80037=CARTESIAN_POINT ( 'NONE',  ( 16.52544592524335698, 4.483927247898782831, 81.45942372801900433 ) ) ;
#80038=CARTESIAN_POINT ( 'NONE',  ( 18.67979575497194134, -10.72451020669871369, 105.8344237280190328 ) ) ;
#80039=CARTESIAN_POINT ( 'NONE',  ( -21.55341960407610458, -5.719274019375992779, 61.45724293864770260 ) ) ;
#80040=CARTESIAN_POINT ( 'NONE',  ( 14.34966873604972726, -8.224510206698740333, 85.83442372801901854 ) ) ;
#80041=CARTESIAN_POINT ( 'NONE',  ( 0.05219959533936267826, -19.03943276465977164, 75.00109039468566152 ) ) ;
#80042=CARTESIAN_POINT ( 'NONE',  ( 0.05219959533909260263, 19.03943276465977164, 34.99890960531435979 ) ) ;
#80043=CARTESIAN_POINT ( 'NONE',  ( 19.02544592524343514, -5.153800228976328945, 83.54057627198100988 ) ) ;
#80044=CARTESIAN_POINT ( 'NONE',  ( -15.72974639402176322, -15.80617190586768395, 44.37609039468567573 ) ) ;
#80045=CARTESIAN_POINT ( 'NONE',  ( -9.564922557960796823, -16.46253265017161027, 47.08224293864769550 ) ) ;
#80046=CARTESIAN_POINT ( 'NONE',  ( -13.89961937509957401, -13.97604488694547875, 69.37609039468564731 ) ) ;
#80048=CARTESIAN_POINT ( 'NONE',  ( -13.89961937509977652, 13.97604488694528158, 115.6239096053143669 ) ) ;
#80049=CARTESIAN_POINT ( 'NONE',  ( 8.224510206698953496, -14.34966873604960469, 67.91557627198102409 ) ) ;
#80050=CARTESIAN_POINT ( 'NONE',  ( 5.719274019375991003, -21.55341960407610458, 62.70724293864769550 ) ) ;
#80052=CARTESIAN_POINT ( 'NONE',  ( 16.51473224551083163, -9.474510206698727899, 30.83442372801900433 ) ) ;
#80053=CARTESIAN_POINT ( 'NONE',  ( -9.564922557960796823, -16.46253265017161027, 62.08224293864769550 ) ) ;
#80054=CARTESIAN_POINT ( 'NONE',  ( -19.02544592524342804, 5.153800228976336051, 71.04057627198099567 ) ) ;
#80055=CARTESIAN_POINT ( 'NONE',  ( -14.29746914071037622, -8.314922557961029526, 54.16775706135235424 ) ) ;
#80058=CARTESIAN_POINT ( 'NONE',  ( -12.06949235617739369, -12.14591786802326823, 79.37609039468567573 ) ) ;
#80059=PLANE ( 'NONE',  #75907 ) ;
#80060=CARTESIAN_POINT ( 'NONE',  ( 4.379528057220092307, 16.55341960407617563, 62.29275706135236845 ) ) ;
#80061=CARTESIAN_POINT ( 'NONE',  ( 14.29746914071037800, 8.314922557961029526, 36.66775706135234714 ) ) ;
#80062=CARTESIAN_POINT ( 'NONE',  ( 13.89961937509977652, -13.97604488694527269, 53.12390960531434558 ) ) ;
#80064=CARTESIAN_POINT ( 'NONE',  ( -10.81492255796105439, 18.62759615963255655, 57.91775706135234714 ) ) ;
#80065=CARTESIAN_POINT ( 'NONE',  ( -5.153800228976607833, 19.02544592524334988, 62.70942372801899722 ) ) ;
#80066=CARTESIAN_POINT ( 'NONE',  ( -10.81492255796105439, 18.62759615963255655, 107.9177570613523471 ) ) ;
#80067=CARTESIAN_POINT ( 'NONE',  ( -9.474510206698964154, 16.51473224551069663, 30.41557627198102054 ) ) ;
#80068=CARTESIAN_POINT ( 'NONE',  ( 17.18050156595283795, 6.597016869166541397, 23.86958650019716544 ) ) ;
#80069=CARTESIAN_POINT ( 'NONE',  ( 18.62759615963271287, -10.81492255796078972, 53.33224293864769550 ) ) ;
#80070=AXIS2_PLACEMENT_3D ( 'NONE', #171888, #129340, #173890 ) ;
#80071=CARTESIAN_POINT ( 'NONE',  ( 9.474510206698971260, -16.51473224551069308, 107.9155762719810383 ) ) ;
#80072=CARTESIAN_POINT ( 'NONE',  ( -12.14591786802309592, -12.06949235617757132, 106.8739096053143811 ) ) ;
#80073=CARTESIAN_POINT ( 'NONE',  ( -4.483927247898782831, 16.52544592524335698, 42.70942372801901854 ) ) ;
#80074=CARTESIAN_POINT ( 'NONE',  ( -16.53943276465976808, 0.05219959533911058130, 26.24890960531435624 ) ) ;
#80076=CARTESIAN_POINT ( 'NONE',  ( -10.72451020669898014, 18.67979575497178502, 100.4155762719810241 ) ) ;
#80077=CARTESIAN_POINT ( 'NONE',  ( 12.14591786802309770, 12.06949235617756955, 44.37390960531435979 ) ) ;
#80078=CARTESIAN_POINT ( 'NONE',  ( -5.049401038298153566, 19.05341960407611168, 115.2072429386477097 ) ) ;
#80079=CARTESIAN_POINT ( 'NONE',  ( 19.03943276465977164, 0.05219959533936151252, 96.25109039468567573 ) ) ;
#80080=CARTESIAN_POINT ( 'NONE',  ( 16.51473224551083163, -9.474510206698727899, 25.83442372801900078 ) ) ;
#80081=CARTESIAN_POINT ( 'NONE',  ( -8.224510206698948167, 14.34966873604960824, 35.41557627198102409 ) ) ;
#80082=CARTESIAN_POINT ( 'NONE',  ( 21.55341960407610458, 5.719274019375980345, 103.9572429386476813 ) ) ;
#80083=CARTESIAN_POINT ( 'NONE',  ( -5.719274019375978568, 21.55341960407610458, 50.20724293864769550 ) ) ;
#80084=CARTESIAN_POINT ( 'NONE',  ( -16.46253265017160317, 9.564922557960807481, 75.83224293864769550 ) ) ;
#80085=CARTESIAN_POINT ( 'NONE',  ( -16.55341960407611168, -4.379528057220339221, 41.45724293864769550 ) ) ;
#80086=CARTESIAN_POINT ( 'NONE',  ( -19.05341960407611168, -5.049401038298163336, 91.45724293864766707 ) ) ;
#80088=CARTESIAN_POINT ( 'NONE',  ( 19.01533133064922154, -5.499999999999651834, 61.26586590595741200 ) ) ;
#80089=CARTESIAN_POINT ( 'NONE',  ( 9.564922557961047289, -16.46253265017146816, 35.41775706135233293 ) ) ;
#80090=CARTESIAN_POINT ( 'NONE',  ( -15.72974639402197994, 15.80617190586746368, 80.62390960531438111 ) ) ;
#80091=CARTESIAN_POINT ( 'NONE',  ( 12.14591786802309770, 12.06949235617756955, 104.3739096053143669 ) ) ;
#80092=CARTESIAN_POINT ( 'NONE',  ( 21.52544592524334988, 5.823673210054432836, 31.45942372801901854 ) ) ;
#80094=CARTESIAN_POINT ( 'NONE',  ( 12.14591786802327356, -12.06949235617739191, 110.6260903946857042 ) ) ;
#80095=CARTESIAN_POINT ( 'NONE',  ( -9.564922557960796823, -16.46253265017161027, 42.08224293864769550 ) ) ;
#80096=CARTESIAN_POINT ( 'NONE',  ( -0.05219959533909027116, -19.03943276465977164, 82.49890960531436690 ) ) ;
#80097=CARTESIAN_POINT ( 'NONE',  ( -9.564922557961040184, 16.46253265017147172, 92.91775706135233293 ) ) ;
#80098=CARTESIAN_POINT ( 'NONE',  ( 19.02544592524343514, -5.153800228976328945, 28.54057627198102409 ) ) ;
#80099=CARTESIAN_POINT ( 'NONE',  ( -8.224510206698948167, 14.34966873604960824, 45.41557627198103830 ) ) ;
#80100=CARTESIAN_POINT ( 'NONE',  ( 21.55341960407619695, -5.719274019375665929, 76.04275706135237556 ) ) ;
#80102=CARTESIAN_POINT ( 'NONE',  ( 0.05219959533934541429, -16.53943276465976808, 70.00109039468568994 ) ) ;
#80103=CARTESIAN_POINT ( 'NONE',  ( -16.51473224551069308, -9.474510206698971260, 61.66557627198103120 ) ) ;
#80104=CARTESIAN_POINT ( 'NONE',  ( 5.049401038298161559, -19.05341960407611168, 62.70724293864769550 ) ) ;
#80106=CARTESIAN_POINT ( 'NONE',  ( -0.05219959533937732626, 21.53943276465977519, 102.5010903946856899 ) ) ;
#80107=CARTESIAN_POINT ( 'NONE',  ( 0.05219959533934541429, -16.53943276465976808, 70.00109039468568994 ) ) ;
#80108=CARTESIAN_POINT ( 'NONE',  ( -10.72451020669870658, -18.67979575497194134, 99.58442372801900433 ) ) ;
#80109=CARTESIAN_POINT ( 'NONE',  ( 19.03943276465977164, -0.05219959533909143690, 68.74890960531436690 ) ) ;
#80110=CARTESIAN_POINT ( 'NONE',  ( 15.72974639402199770, -15.80617190586745480, 33.12390960531435979 ) ) ;
#80111=CARTESIAN_POINT ( 'NONE',  ( 13.89961937509957401, 13.97604488694547697, 106.8760903946856757 ) ) ;
#80112=CARTESIAN_POINT ( 'NONE',  ( 0.05219959533937995610, -21.53943276465977519, 75.00109039468568994 ) ) ;
#80113=CARTESIAN_POINT ( 'NONE',  ( -12.14591786802326823, 12.06949235617739902, 48.12609039468568284 ) ) ;
#80114=CARTESIAN_POINT ( 'NONE',  ( 10.81492255796078972, 18.62759615963270932, 99.58224293864770971 ) ) ;
#80115=CARTESIAN_POINT ( 'NONE',  ( -5.049401038297874678, -19.05341960407617918, 104.7927570613523471 ) ) ;
#80116=CARTESIAN_POINT ( 'NONE',  ( 19.05341960407611168, 5.049401038298154454, 83.95724293864766707 ) ) ;
#80117=CARTESIAN_POINT ( 'NONE',  ( -5.153800228976607833, 19.02544592524334988, 107.7094237280189759 ) ) ;
#80118=CARTESIAN_POINT ( 'NONE',  ( -12.14591786802326823, 12.06949235617739902, 23.12609039468567573 ) ) ;
#80119=CARTESIAN_POINT ( 'NONE',  ( 14.29746914071049879, -8.314922557960816363, 63.33224293864770260 ) ) ;
#80120=CARTESIAN_POINT ( 'NONE',  ( -8.314922557961024197, 14.29746914071037800, 67.91775706135234714 ) ) ;
#80121=CARTESIAN_POINT ( 'NONE',  ( -21.52544592524343514, 5.823673210054127303, 111.0405762719810525 ) ) ;
#80122=CARTESIAN_POINT ( 'NONE',  ( -19.03943276465977164, 0.05219959533909376836, 51.24890960531436690 ) ) ;
#80123=CARTESIAN_POINT ( 'NONE',  ( 0.05219959533909260263, 19.03943276465977164, 74.99890960531435269 ) ) ;
#80124=CARTESIAN_POINT ( 'NONE',  ( -12.06949235617739369, -12.14591786802326823, 69.37609039468567573 ) ) ;
#80126=ORIENTED_EDGE ( 'NONE', *, *, #106448, .T. ) ;
#80127=CARTESIAN_POINT ( 'NONE',  ( -18.62759615963255300, -10.81492255796106328, 109.1677570613523613 ) ) ;
#80128=CARTESIAN_POINT ( 'NONE',  ( -19.02544592524342804, 5.153800228976336051, 36.04057627198100988 ) ) ;
#80130=CARTESIAN_POINT ( 'NONE',  ( -16.53943276465976808, -0.05219959533934237506, 18.75109039468568639 ) ) ;
#80131=CARTESIAN_POINT ( 'NONE',  ( 19.03943276465977164, 0.05219959533936151252, 51.25109039468567573 ) ) ;
#80132=CARTESIAN_POINT ( 'NONE',  ( -16.52544592524335698, -4.483927247898792601, 23.95942372801901143 ) ) ;
#80133=CARTESIAN_POINT ( 'NONE',  ( -13.97604488694527625, -13.89961937509977652, 46.87390960531435979 ) ) ;
#80134=CARTESIAN_POINT ( 'NONE',  ( 9.474510206698971260, -16.51473224551069308, 67.91557627198102409 ) ) ;
#80135=CARTESIAN_POINT ( 'NONE',  ( 5.719274019375991003, -21.55341960407610458, 87.70724293864769550 ) ) ;
#80136=CARTESIAN_POINT ( 'NONE',  ( 5.153800228976335163, 19.02544592524342804, 109.7905762719810099 ) ) ;
#80137=CARTESIAN_POINT ( 'NONE',  ( 19.03943276465977164, -0.05219959533909143690, 43.74890960531435979 ) ) ;
#80138=CARTESIAN_POINT ( 'NONE',  ( -17.72696623605160582, 5.499999999999962697, 93.59811031808420978 ) ) ;
#80139=CARTESIAN_POINT ( 'NONE',  ( 19.02544592524334988, 5.153800228976608722, 96.45942372801897591 ) ) ;
#80140=CARTESIAN_POINT ( 'NONE',  ( -18.62759615963270932, 10.81492255796079327, 70.83224293864770971 ) ) ;
#80141=CARTESIAN_POINT ( 'NONE',  ( 5.049401038297881783, 19.05341960407617563, 27.29275706135232937 ) ) ;
#80142=CARTESIAN_POINT ( 'NONE',  ( -14.29746914071049879, 8.314922557960819915, 60.83224293864769550 ) ) ;
#80143=CARTESIAN_POINT ( 'NONE',  ( 15.80617190586769283, -15.72974639402175789, 85.62609039468568994 ) ) ;
#80144=CARTESIAN_POINT ( 'NONE',  ( -16.46253265017160317, 9.564922557960807481, 25.83224293864769194 ) ) ;
#80145=CARTESIAN_POINT ( 'NONE',  ( 0.05219959533910956823, 16.53943276465976808, 29.99890960531435979 ) ) ;
#80146=CARTESIAN_POINT ( 'NONE',  ( 21.55341960407619695, -5.719274019375665929, 96.04275706135236135 ) ) ;
#80147=CARTESIAN_POINT ( 'NONE',  ( 0.05219959533909260263, 19.03943276465977164, 74.99890960531435269 ) ) ;
#80148=CARTESIAN_POINT ( 'NONE',  ( 5.823673210054444382, -21.52544592524334988, 40.20942372801901854 ) ) ;
#80149=CARTESIAN_POINT ( 'NONE',  ( 0.05219959533909260263, 19.03943276465977164, 79.99890960531436690 ) ) ;
#80150=CARTESIAN_POINT ( 'NONE',  ( -12.06949235617756955, 12.14591786802309770, 90.62390960531436690 ) ) ;
#80151=CARTESIAN_POINT ( 'NONE',  ( -8.224510206698948167, 14.34966873604960824, 60.41557627198102409 ) ) ;
#80152=CARTESIAN_POINT ( 'NONE',  ( 18.62759615963271287, -10.81492255796078972, 73.33224293864769550 ) ) ;
#80153=CARTESIAN_POINT ( 'NONE',  ( -16.46253265017160317, 9.564922557960807481, 75.83224293864769550 ) ) ;
#80154=CARTESIAN_POINT ( 'NONE',  ( -0.05219959533907301413, -21.53943276465977519, 82.49890960531436690 ) ) ;
#80155=CARTESIAN_POINT ( 'NONE',  ( -16.51473224551082808, 9.474510206698731452, 83.33442372801899012 ) ) ;
#80156=CARTESIAN_POINT ( 'NONE',  ( -16.46253265017146816, -9.564922557961047289, 34.16775706135233293 ) ) ;
#80157=CARTESIAN_POINT ( 'NONE',  ( -12.14591786802309592, -12.06949235617757132, 71.87390960531438111 ) ) ;
#80158=CARTESIAN_POINT ( 'NONE',  ( 18.67979575497178502, 10.72451020669898547, 59.16557627198103120 ) ) ;
#80160=CARTESIAN_POINT ( 'NONE',  ( -12.06949235617739369, -12.14591786802326823, 104.3760903946856899 ) ) ;
#80162=CARTESIAN_POINT ( 'NONE',  ( -9.474510206698720793, -16.51473224551083518, 99.58442372801900433 ) ) ;
#80163=CARTESIAN_POINT ( 'NONE',  ( -12.06949235617756955, 12.14591786802309770, 65.62390960531436690 ) ) ;
#80164=CARTESIAN_POINT ( 'NONE',  ( -17.50000000000001421, 3.189878218039099878, 34.87051437428754497 ) ) ;
#80165=CARTESIAN_POINT ( 'NONE',  ( -19.03943276465977164, 0.05219959533909376836, 61.24890960531436690 ) ) ;
#80166=CARTESIAN_POINT ( 'NONE',  ( -13.97604488694527625, -13.89961937509977652, 26.87390960531434558 ) ) ;
#80167=CARTESIAN_POINT ( 'NONE',  ( 12.14591786802309770, 12.06949235617756955, 59.37390960531436690 ) ) ;
#80168=CARTESIAN_POINT ( 'NONE',  ( 19.03943276465977164, -0.05219959533909143690, 103.7489096053143669 ) ) ;
#80169=CARTESIAN_POINT ( 'NONE',  ( -19.03943276465977164, -0.05219959533935918106, 83.75109039468567573 ) ) ;
#80170=CARTESIAN_POINT ( 'NONE',  ( 16.51473224551069308, 9.474510206698969483, 64.16557627198102409 ) ) ;
#80171=CARTESIAN_POINT ( 'NONE',  ( -0.05219959533909027116, -19.03943276465977164, 87.49890960531436690 ) ) ;
#80172=CARTESIAN_POINT ( 'NONE',  ( -9.564922557960796823, -16.46253265017161027, 87.08224293864769550 ) ) ;
#80173=CARTESIAN_POINT ( 'NONE',  ( 21.52544592524344225, -5.823673210054117533, 63.54057627198103830 ) ) ;
#80174=CARTESIAN_POINT ( 'NONE',  ( 12.06949235617739724, 12.14591786802326823, 56.87609039468568994 ) ) ;
#80175=CARTESIAN_POINT ( 'NONE',  ( 0.05219959533936267826, -19.03943276465977164, 110.0010903946856757 ) ) ;
#80176=CARTESIAN_POINT ( 'NONE',  ( -16.51473224551069308, -9.474510206698971260, 61.66557627198103120 ) ) ;
#80177=CARTESIAN_POINT ( 'NONE',  ( -18.62759615963270932, 10.81492255796079327, 70.83224293864770971 ) ) ;
#80178=CARTESIAN_POINT ( 'NONE',  ( -19.03943276465977164, -0.05219959533935918106, 98.75109039468567573 ) ) ;
#80179=CARTESIAN_POINT ( 'NONE',  ( -12.14591786802309592, -12.06949235617757132, 26.87390960531435979 ) ) ;
#80180=CARTESIAN_POINT ( 'NONE',  ( -5.823673210054431948, 21.52544592524334988, 47.70942372801902565 ) ) ;
#80182=CARTESIAN_POINT ( 'NONE',  ( 4.379528057220092307, 16.55341960407617563, 67.29275706135234714 ) ) ;
#80183=CARTESIAN_POINT ( 'NONE',  ( -14.34966873604972548, 8.224510206698743886, 98.33442372801901854 ) ) ;
#80185=CARTESIAN_POINT ( 'NONE',  ( -4.483927247898782831, 16.52544592524335698, 77.70942372801900433 ) ) ;
#80186=CARTESIAN_POINT ( 'NONE',  ( 8.314922557961029526, -14.29746914071037800, 30.41775706135234358 ) ) ;
#80187=CARTESIAN_POINT ( 'NONE',  ( -5.049401038298153566, 19.05341960407611168, 45.20724293864769550 ) ) ;
#80188=CARTESIAN_POINT ( 'NONE',  ( 13.97604488694527802, 13.89961937509977652, 44.37390960531435269 ) ) ;
#80189=CARTESIAN_POINT ( 'NONE',  ( 19.05341960407611168, 5.049401038298154454, 53.95724293864770260 ) ) ;
#80190=CARTESIAN_POINT ( 'NONE',  ( -5.823673210054431948, 21.52544592524334988, 52.70942372801902565 ) ) ;
#80191=CARTESIAN_POINT ( 'NONE',  ( 14.29746914071037800, 8.314922557961029526, 51.66775706135234714 ) ) ;
#80192=CARTESIAN_POINT ( 'NONE',  ( -16.53943276465976808, 0.05219959533911058130, 36.24890960531435979 ) ) ;
#80193=CARTESIAN_POINT ( 'NONE',  ( -9.474510206698964154, 16.51473224551069663, 30.41557627198102054 ) ) ;
#80194=CARTESIAN_POINT ( 'NONE',  ( -16.46253265017160317, 9.564922557960807481, 40.83224293864769550 ) ) ;
#80195=CARTESIAN_POINT ( 'NONE',  ( 16.52544592524335698, 4.483927247898782831, 26.45942372801901854 ) ) ;
#80196=EDGE_CURVE ( 'NONE', #26208, #112608, #78704, .T. ) ;
#80197=CARTESIAN_POINT ( 'NONE',  ( 19.03943276465977164, 0.05219959533936151252, 86.25109039468567573 ) ) ;
#80198=CARTESIAN_POINT ( 'NONE',  ( 4.379528057220339221, -16.55341960407611168, 77.70724293864770971 ) ) ;
#80199=CARTESIAN_POINT ( 'NONE',  ( 5.153800228976335163, 19.02544592524342804, 54.79057627198103120 ) ) ;
#80200=CARTESIAN_POINT ( 'NONE',  ( 19.03943276465977164, 0.05219959533936151252, 91.25109039468566152 ) ) ;
#80201=CARTESIAN_POINT ( 'NONE',  ( 17.26058549869091507, -6.457015423128539489, 91.12254162523935008 ) ) ;
#80202=CARTESIAN_POINT ( 'NONE',  ( -0.05219959533937732626, 21.53943276465977519, 82.50109039468568994 ) ) ;
#80203=CARTESIAN_POINT ( 'NONE',  ( 8.314922557961029526, -14.29746914071037800, 55.41775706135234714 ) ) ;
#80205=CARTESIAN_POINT ( 'NONE',  ( 21.52544592524344225, -5.823673210054117533, 38.54057627198103120 ) ) ;
#80206=CARTESIAN_POINT ( 'NONE',  ( 14.29746914071037800, 8.314922557961029526, 36.66775706135234714 ) ) ;
#80207=CARTESIAN_POINT ( 'NONE',  ( -5.153800228976328057, -19.02544592524343514, 27.29057627198103120 ) ) ;
#80208=CARTESIAN_POINT ( 'NONE',  ( 16.51473224551083163, -9.474510206698727899, 30.83442372801900433 ) ) ;
#80210=CARTESIAN_POINT ( 'NONE',  ( 19.02544592524343514, -5.153800228976328945, 33.54057627198102409 ) ) ;
#80212=CARTESIAN_POINT ( 'NONE',  ( 19.02544592524343514, -5.153800228976328945, 68.54057627198103830 ) ) ;
#80213=CARTESIAN_POINT ( 'NONE',  ( 17.50000000000147438, -3.254303733634560825, 112.5239589307140449 ) ) ;
#80214=CARTESIAN_POINT ( 'NONE',  ( 19.02544592524334988, 5.153800228976608722, 21.45942372801899012 ) ) ;
#80215=CARTESIAN_POINT ( 'NONE',  ( 12.06949235617757843, -12.14591786802309237, 43.12390960531435269 ) ) ;
#80216=CARTESIAN_POINT ( 'NONE',  ( -9.474510206698964154, 16.51473224551069663, 45.41557627198103120 ) ) ;
#80217=CARTESIAN_POINT ( 'NONE',  ( 9.564922557960805705, 16.46253265017160317, 99.58224293864770971 ) ) ;
#80218=CARTESIAN_POINT ( 'NONE',  ( 5.719274019375673035, 21.55341960407619339, 72.29275706135236135 ) ) ;
#80219=CARTESIAN_POINT ( 'NONE',  ( -5.153800228976328057, -19.02544592524343514, 57.29057627198103120 ) ) ;
#80220=CARTESIAN_POINT ( 'NONE',  ( -10.81492255796105439, 18.62759615963255655, 67.91775706135234714 ) ) ;
#80221=CARTESIAN_POINT ( 'NONE',  ( -5.049401038298153566, 19.05341960407611168, 115.2072429386477097 ) ) ;
#80222=CARTESIAN_POINT ( 'NONE',  ( -9.474510206698964154, 16.51473224551069663, 30.41557627198102054 ) ) ;
#80223=CARTESIAN_POINT ( 'NONE',  ( -10.81492255796105439, 18.62759615963255655, 27.91775706135234358 ) ) ;
#80224=CARTESIAN_POINT ( 'NONE',  ( -5.153800228976607833, 19.02544592524334988, 42.70942372801901143 ) ) ;
#80225=CARTESIAN_POINT ( 'NONE',  ( 0.05219959533909260263, 19.03943276465977164, 24.99890960531435269 ) ) ;
#80226=CARTESIAN_POINT ( 'NONE',  ( -5.153800228976328057, -19.02544592524343514, 57.29057627198103120 ) ) ;
#80227=CARTESIAN_POINT ( 'NONE',  ( -19.02544592524334988, -5.153800228976617603, 108.9594237280189759 ) ) ;
#80228=CARTESIAN_POINT ( 'NONE',  ( 16.55341960407611168, 4.379528057220329451, 78.95724293864769550 ) ) ;
#80229=CARTESIAN_POINT ( 'NONE',  ( -18.62759615963270932, 10.81492255796079327, 30.83224293864770260 ) ) ;
#80230=CARTESIAN_POINT ( 'NONE',  ( 9.474510206698729675, 16.51473224551082808, 97.08442372801900433 ) ) ;
#80231=CARTESIAN_POINT ( 'NONE',  ( 0.05219959533907565091, 21.53943276465977519, 99.99890960531436690 ) ) ;
#80232=CARTESIAN_POINT ( 'NONE',  ( -15.80617190586768217, 15.72974639402176855, 63.12609039468568994 ) ) ;
#80233=CARTESIAN_POINT ( 'NONE',  ( -14.29746914071037622, -8.314922557961029526, 59.16775706135234714 ) ) ;
#80234=CARTESIAN_POINT ( 'NONE',  ( -8.314922557961024197, 14.29746914071037800, 57.91775706135234714 ) ) ;
#80235=CARTESIAN_POINT ( 'NONE',  ( -5.823673210054116645, -21.52544592524344225, 57.29057627198103120 ) ) ;
#80236=CARTESIAN_POINT ( 'NONE',  ( 16.51473224551069308, 9.474510206698969483, 54.16557627198103120 ) ) ;
#80237=CARTESIAN_POINT ( 'NONE',  ( -12.06949235617739369, -12.14591786802326823, 69.37609039468567573 ) ) ;
#80239=CARTESIAN_POINT ( 'NONE',  ( 0.05219959533907565091, 21.53943276465977519, 99.99890960531436690 ) ) ;
#80240=CARTESIAN_POINT ( 'NONE',  ( 12.14591786802309770, 12.06949235617756955, 49.37390960531436690 ) ) ;
#80241=CARTESIAN_POINT ( 'NONE',  ( 19.05341960407611168, 5.049401038298154454, 73.95724293864768129 ) ) ;
#80242=CARTESIAN_POINT ( 'NONE',  ( -4.379528057220086978, -16.55341960407618274, 79.79275706135236135 ) ) ;
#80243=CARTESIAN_POINT ( 'NONE',  ( -19.05341960407617563, 5.049401038297882671, 108.5427570613523187 ) ) ;
#80244=CARTESIAN_POINT ( 'NONE',  ( 10.72451020669898902, -18.67979575497178502, 102.9155762719810383 ) ) ;
#80245=CARTESIAN_POINT ( 'NONE',  ( 4.483927247898545687, 16.52544592524342804, 49.79057627198102409 ) ) ;
#80246=ORIENTED_EDGE ( 'NONE', *, *, #7150, .T. ) ;
#80247=CARTESIAN_POINT ( 'NONE',  ( -16.19135201231366494, 7.376712067591930655, 69.81319145947971094 ) ) ;
#80248=CARTESIAN_POINT ( 'NONE',  ( -18.67979575497178146, -10.72451020669898902, 86.66557627198102409 ) ) ;
#80249=CARTESIAN_POINT ( 'NONE',  ( 4.483927247898545687, 16.52544592524342804, 24.79057627198103120 ) ) ;
#80251=CARTESIAN_POINT ( 'NONE',  ( -17.12812012977024168, -6.668231424566069876, 56.35948759323144941 ) ) ;
#80252=CARTESIAN_POINT ( 'NONE',  ( -15.80617190586745835, -15.72974639402198527, 96.87390960531436690 ) ) ;
#80253=CARTESIAN_POINT ( 'NONE',  ( 5.049401038298161559, -19.05341960407611168, 102.7072429386476955 ) ) ;
#80254=CARTESIAN_POINT ( 'NONE',  ( 21.53943276465977519, 0.05219959533937863772, 26.25109039468567573 ) ) ;
#80255=CARTESIAN_POINT ( 'NONE',  ( -12.14591786802309592, -12.06949235617757132, 46.87390960531435979 ) ) ;
#80256=CARTESIAN_POINT ( 'NONE',  ( 12.06949235617739724, 12.14591786802326823, 46.87609039468568994 ) ) ;
#80257=CARTESIAN_POINT ( 'NONE',  ( -16.51473224551069308, -9.474510206698971260, 46.66557627198102409 ) ) ;
#80258=CARTESIAN_POINT ( 'NONE',  ( -0.05219959533936034679, 19.03943276465977164, 47.50109039468566863 ) ) ;
#80259=CARTESIAN_POINT ( 'NONE',  ( 19.05341960407611168, 5.049401038298154454, 78.95724293864769550 ) ) ;
#80260=CARTESIAN_POINT ( 'NONE',  ( -15.72974639402197994, 15.80617190586746368, 35.62390960531437401 ) ) ;
#80261=CARTESIAN_POINT ( 'NONE',  ( 17.59860650958989936, 7.585241751807028088, 64.07662985737508166 ) ) ;
#80262=CARTESIAN_POINT ( 'NONE',  ( -5.153800228976607833, 19.02544592524334988, 112.7094237280190043 ) ) ;
#80263=CARTESIAN_POINT ( 'NONE',  ( -16.46253265017146816, -9.564922557961047289, 54.16775706135234003 ) ) ;
#80264=CARTESIAN_POINT ( 'NONE',  ( 15.72974639402199770, -15.80617190586745480, 108.1239096053143811 ) ) ;
#80265=CARTESIAN_POINT ( 'NONE',  ( 14.29746914071049879, -8.314922557960816363, 38.33224293864768839 ) ) ;
#80266=CARTESIAN_POINT ( 'NONE',  ( 9.474510206698971260, -16.51473224551069308, 77.91557627198103830 ) ) ;
#80267=CARTESIAN_POINT ( 'NONE',  ( 15.80617190586746368, 15.72974639402197994, 64.37390960531435269 ) ) ;
#80268=CARTESIAN_POINT ( 'NONE',  ( -18.62759615963270932, 10.81492255796079327, 95.83224293864770971 ) ) ;
#80269=CARTESIAN_POINT ( 'NONE',  ( -8.224510206698735004, -14.34966873604973081, 19.58442372801901143 ) ) ;
#80270=CARTESIAN_POINT ( 'NONE',  ( -9.564922557960796823, -16.46253265017161027, 112.0822429386476955 ) ) ;
#80271=CARTESIAN_POINT ( 'NONE',  ( -15.80617190586768217, 15.72974639402176855, 93.12609039468568994 ) ) ;
#80272=CARTESIAN_POINT ( 'NONE',  ( 19.03943276465977164, -0.05219959533909143690, 88.74890960531436690 ) ) ;
#80273=CARTESIAN_POINT ( 'NONE',  ( -9.474510206698964154, 16.51473224551069663, 30.41557627198102054 ) ) ;
#80274=CARTESIAN_POINT ( 'NONE',  ( 0.05219959533909260263, 19.03943276465977164, 84.99890960531436690 ) ) ;
#80275=CARTESIAN_POINT ( 'NONE',  ( 8.314922557960818139, 14.29746914071049879, 104.5822429386477097 ) ) ;
#80276=CARTESIAN_POINT ( 'NONE',  ( -5.049401038298153566, 19.05341960407611168, 65.20724293864765286 ) ) ;
#80277=CARTESIAN_POINT ( 'NONE',  ( 8.314922557961029526, -14.29746914071037800, 20.41775706135234714 ) ) ;
#80279=CARTESIAN_POINT ( 'NONE',  ( 9.474510206698971260, -16.51473224551069308, 72.91557627198102409 ) ) ;
#80280=CARTESIAN_POINT ( 'NONE',  ( -5.823673210054431948, 21.52544592524334988, 102.7094237280190185 ) ) ;
#80281=CARTESIAN_POINT ( 'NONE',  ( -16.46253265017160317, 9.564922557960807481, 115.8322429386477097 ) ) ;
#80282=CARTESIAN_POINT ( 'NONE',  ( -14.34966873604972548, 8.224510206698743886, 93.33442372801901854 ) ) ;
#80284=CARTESIAN_POINT ( 'NONE',  ( 9.474510206698729675, 16.51473224551082808, 72.08442372801900433 ) ) ;
#80285=CARTESIAN_POINT ( 'NONE',  ( 9.564922557961047289, -16.46253265017146816, 20.41775706135233293 ) ) ;
#80287=CARTESIAN_POINT ( 'NONE',  ( -19.02544592524342804, 5.153800228976336051, 26.04057627198103120 ) ) ;
#80288=CARTESIAN_POINT ( 'NONE',  ( -8.224510206698948167, 14.34966873604960824, 35.41557627198102409 ) ) ;
#80290=CARTESIAN_POINT ( 'NONE',  ( 16.52544592524335698, 4.483927247898782831, 101.4594237280190185 ) ) ;
#80292=CARTESIAN_POINT ( 'NONE',  ( 16.52544592524335698, 4.483927247898782831, 76.45942372801901854 ) ) ;
#80293=CARTESIAN_POINT ( 'NONE',  ( -19.02544592524342804, 5.153800228976336051, 31.04057627198102409 ) ) ;
#80294=CARTESIAN_POINT ( 'NONE',  ( -21.55341960407619339, 5.719274019375674811, 93.54275706135234714 ) ) ;
#80295=CARTESIAN_POINT ( 'NONE',  ( 16.51473224551083163, -9.474510206698727899, 95.83442372801900433 ) ) ;
#80296=CARTESIAN_POINT ( 'NONE',  ( 5.823673210054444382, -21.52544592524334988, 75.20942372801901854 ) ) ;
#80297=CARTESIAN_POINT ( 'NONE',  ( -19.03943276465977164, -0.05219959533935918106, 58.75109039468566863 ) ) ;
#80298=CARTESIAN_POINT ( 'NONE',  ( 19.05341960407611168, 5.049401038298154454, 73.95724293864768129 ) ) ;
#80299=CARTESIAN_POINT ( 'NONE',  ( 16.46253265017160672, -9.564922557960803928, 73.33224293864769550 ) ) ;
#80300=CARTESIAN_POINT ( 'NONE',  ( 16.21995358207305671, 7.366697692864125457, 72.56448998487839219 ) ) ;
#80301=CARTESIAN_POINT ( 'NONE',  ( 8.314922557960818139, 14.29746914071049879, 64.58224293864769550 ) ) ;
#80302=CARTESIAN_POINT ( 'NONE',  ( -15.72974639402197994, 15.80617190586746368, 60.62390960531437401 ) ) ;
#80303=CARTESIAN_POINT ( 'NONE',  ( 5.153800228976335163, 19.02544592524342804, 49.79057627198100988 ) ) ;
#80304=CARTESIAN_POINT ( 'NONE',  ( 21.53943276465977519, -0.05219959533907433946, 88.74890960531436690 ) ) ;
#80305=CARTESIAN_POINT ( 'NONE',  ( -16.55341960407617563, 4.379528057220093196, 83.54275706135234714 ) ) ;
#80307=CARTESIAN_POINT ( 'NONE',  ( 14.29746914071049879, -8.314922557960816363, 78.33224293864770971 ) ) ;
#80309=CARTESIAN_POINT ( 'NONE',  ( -16.52544592524335698, -4.483927247898792601, 33.95942372801901143 ) ) ;
#80310=CARTESIAN_POINT ( 'NONE',  ( -16.46253265017160317, 9.564922557960807481, 25.83224293864769194 ) ) ;
#80311=CARTESIAN_POINT ( 'NONE',  ( 5.153800228976615827, -19.02544592524334988, 65.20942372801900433 ) ) ;
#80312=CARTESIAN_POINT ( 'NONE',  ( -14.29746914071049879, 8.314922557960819915, 65.83224293864769550 ) ) ;
#80313=CARTESIAN_POINT ( 'NONE',  ( 15.80617190586769283, -15.72974639402175789, 45.62609039468567573 ) ) ;
#80314=CARTESIAN_POINT ( 'NONE',  ( 9.474510206698971260, -16.51473224551069308, 22.91557627198102765 ) ) ;
#80315=CARTESIAN_POINT ( 'NONE',  ( -21.53943276465977519, 0.05219959533907696930, 96.24890960531435269 ) ) ;
#80317=CARTESIAN_POINT ( 'NONE',  ( 16.53943276465976808, -0.05219959533910856209, 93.74890960531436690 ) ) ;
#80319=CARTESIAN_POINT ( 'NONE',  ( -5.049401038298153566, 19.05341960407611168, 50.20724293864770260 ) ) ;
#80321=CARTESIAN_POINT ( 'NONE',  ( 5.049401038297881783, 19.05341960407617563, 82.29275706135229029 ) ) ;
#80322=CARTESIAN_POINT ( 'NONE',  ( -18.67979575497193778, 10.72451020669871902, 33.33442372801900433 ) ) ;
#80323=CARTESIAN_POINT ( 'NONE',  ( -19.05341960407611168, -5.049401038298163336, 71.45724293864766707 ) ) ;
#80324=CARTESIAN_POINT ( 'NONE',  ( 13.97604488694548053, -13.89961937509957401, 55.62609039468566863 ) ) ;
#80325=CARTESIAN_POINT ( 'NONE',  ( -13.89961937509977652, 13.97604488694528158, 45.62390960531433848 ) ) ;
#80326=EDGE_CURVE ( 'NONE', #139245, #123348, #21013, .T. ) ;
#80327=CARTESIAN_POINT ( 'NONE',  ( 8.224510206698953496, -14.34966873604960469, 67.91557627198102409 ) ) ;
#80328=CARTESIAN_POINT ( 'NONE',  ( -14.29746914071049879, 8.314922557960819915, 50.83224293864770971 ) ) ;
#80329=CARTESIAN_POINT ( 'NONE',  ( -9.564922557960796823, -16.46253265017161027, 72.08224293864770971 ) ) ;
#80330=CARTESIAN_POINT ( 'NONE',  ( -5.823673210054116645, -21.52544592524344225, 97.29057627198105251 ) ) ;
#80331=CARTESIAN_POINT ( 'NONE',  ( 19.02544592524343514, -5.153800228976328945, 68.54057627198103830 ) ) ;
#80332=CARTESIAN_POINT ( 'NONE',  ( -5.823673210054116645, -21.52544592524344225, 82.29057627198103830 ) ) ;
#80333=CARTESIAN_POINT ( 'NONE',  ( -5.153800228976607833, 19.02544592524334988, 22.70942372801899012 ) ) ;
#80334=CARTESIAN_POINT ( 'NONE',  ( 19.05341960407611168, 5.049401038298154454, 38.95724293864767418 ) ) ;
#80335=CARTESIAN_POINT ( 'NONE',  ( -4.379528057220086978, -16.55341960407618274, 104.7927570613523898 ) ) ;
#80336=CARTESIAN_POINT ( 'NONE',  ( -16.55341960407611168, -4.379528057220339221, 91.45724293864769550 ) ) ;
#80337=CARTESIAN_POINT ( 'NONE',  ( 19.05341960407617918, -5.049401038297876454, 111.0427570613523329 ) ) ;
#80339=CARTESIAN_POINT ( 'NONE',  ( 15.80617190586769283, -15.72974639402175789, 35.62609039468568994 ) ) ;
#80340=CARTESIAN_POINT ( 'NONE',  ( -16.51473224551082808, 9.474510206698731452, 48.33442372801900433 ) ) ;
#80341=CARTESIAN_POINT ( 'NONE',  ( 12.06949235617757843, -12.14591786802309237, 28.12390960531435979 ) ) ;
#80342=CARTESIAN_POINT ( 'NONE',  ( 15.72974639402199770, -15.80617190586745480, 73.12390960531436690 ) ) ;
#80343=CARTESIAN_POINT ( 'NONE',  ( -19.03943276465977164, 0.05219959533909376836, 96.24890960531436690 ) ) ;
#80344=CARTESIAN_POINT ( 'NONE',  ( 0.05219959533910956823, 16.53943276465976808, 59.99890960531436690 ) ) ;
#80345=CARTESIAN_POINT ( 'NONE',  ( 5.153800228976335163, 19.02544592524342804, 29.79057627198102409 ) ) ;
#80346=CARTESIAN_POINT ( 'NONE',  ( -0.05219959533909027116, -19.03943276465977164, 32.49890960531435979 ) ) ;
#80347=CARTESIAN_POINT ( 'NONE',  ( 0.05219959533936267826, -19.03943276465977164, 30.00109039468566863 ) ) ;
#80348=CARTESIAN_POINT ( 'NONE',  ( 0.05219959533934541429, -16.53943276465976808, 95.00109039468568994 ) ) ;
#80349=CARTESIAN_POINT ( 'NONE',  ( -10.81492255796105439, 18.62759615963255655, 37.91775706135235424 ) ) ;
#80350=CARTESIAN_POINT ( 'NONE',  ( -14.29746914071037622, -8.314922557961029526, 44.16775706135234714 ) ) ;
#80351=CARTESIAN_POINT ( 'NONE',  ( -21.55341960407610458, -5.719274019375992779, 26.45724293864768839 ) ) ;
#80352=CARTESIAN_POINT ( 'NONE',  ( 9.564922557960805705, 16.46253265017160317, 49.58224293864770260 ) ) ;
#80353=CARTESIAN_POINT ( 'NONE',  ( 21.55341960407619695, -5.719274019375665929, 96.04275706135236135 ) ) ;
#80354=CARTESIAN_POINT ( 'NONE',  ( -19.03943276465977164, 0.05219959533909376836, 81.24890960531436690 ) ) ;
#80355=CARTESIAN_POINT ( 'NONE',  ( -12.06949235617739369, -12.14591786802326823, 59.37609039468568284 ) ) ;
#80356=CARTESIAN_POINT ( 'NONE',  ( -4.379528057220328563, 16.55341960407611168, 110.2072429386477239 ) ) ;
#80357=CARTESIAN_POINT ( 'NONE',  ( 14.34966873604972726, -8.224510206698740333, 110.8344237280190043 ) ) ;
#80359=CARTESIAN_POINT ( 'NONE',  ( -21.55341960407619339, 5.719274019375674811, 58.54275706135235424 ) ) ;
#80360=CARTESIAN_POINT ( 'NONE',  ( 13.97604488694527802, 13.89961937509977652, 94.37390960531436690 ) ) ;
#80361=CARTESIAN_POINT ( 'NONE',  ( -19.05341960407611168, -5.049401038298163336, 71.45724293864766707 ) ) ;
#80362=CARTESIAN_POINT ( 'NONE',  ( -9.474510206698964154, 16.51473224551069663, 115.4155762719810241 ) ) ;
#80363=CARTESIAN_POINT ( 'NONE',  ( 16.55341960407611168, 4.379528057220329451, 38.95724293864768839 ) ) ;
#80364=CARTESIAN_POINT ( 'NONE',  ( 8.224510206698742110, 14.34966873604972548, 112.0844237280190185 ) ) ;
#80365=CARTESIAN_POINT ( 'NONE',  ( 8.314922557960818139, 14.29746914071049879, 34.58224293864770260 ) ) ;
#80367=CARTESIAN_POINT ( 'NONE',  ( -13.97604488694547697, 13.89961937509957934, 33.12609039468566863 ) ) ;
#80368=CARTESIAN_POINT ( 'NONE',  ( 9.564922557960805705, 16.46253265017160317, 79.58224293864769550 ) ) ;
#80369=CARTESIAN_POINT ( 'NONE',  ( 9.474510206698729675, 16.51473224551082808, 52.08442372801900433 ) ) ;
#80372=CARTESIAN_POINT ( 'NONE',  ( -19.05341960407617563, 5.049401038297882671, 88.54275706135230450 ) ) ;
#80373=CARTESIAN_POINT ( 'NONE',  ( -12.14591786802326823, 12.06949235617739902, 78.12609039468570415 ) ) ;
#80375=( BOUNDED_SURFACE ( )  B_SPLINE_SURFACE ( 3, 2, ( 
 ( #25379, #59657, #106163, #181051, #44507, #165871, #132530, #12203, #26371, #194219, #121331, #11197, #183024, #14152, #150705, #90007, #149699, #167846, #72873, #196230, #119368, #120337, #166868, #104189, #73867, #103196, #88011, #135537, #151691, #13181, #118370, #29346, #90975, #74844, #55684, #136507, #117358, #198187, #179054, #102194, #163882, #87021, #10195, #71855, #133524, #195216, #56697, #180064, #164876, #187013, #32315, #139474, #199178, #15153, #109143, #17143, #111127, #60644, #30322, #168817, #172816, #93968, #125317, #184010, #140474, #954, #62631, #122318, #49464, #187994, #95958, #170822, #1962, #126297, #63642, #45492, #155648, #94966, #78796, #137497, #91964, #110139, #46481, #48484, #124307, #153657, #34296, #156650, #157642, #79800, #75819, #169825, #171818, #18146, #107147, #76814, #33306, #64635, #138485, #141472, #2956, #200167, #61636, #123304, #184997, #108141, #31317, #92969, #186005, #154655, #16151, #77805, #47487, #175796, #80782, #50466, #19131, #131274, #100926, #82762, #188990, #38277, #112126, #99931, #177801, #142459, #160618, #161617, #130255, #23110, #7924, #114094, #37269, #116112, #69609, #5928, #53436, #22109, #83759, #127277, #84756, #3937, #173817, #98927, #192962, #65617, #115111, #35282, #52436, #146434, #96938, #97917, #129265, #158619, #20109, #4927, #145439, #128274, #6921, #67604, #39270, #36263, #190959, #81753, #68599, #143441, #21107, #54441, #66609, #189971, #51446, #191951, #159609, #113107, #176805, #174797, #144443, #58430, #8945, #71606, #132280, #10943, #135290, #87762, #11955, #88767, #166621, #101943, #104935, #182780, #181785, #43266, #42283, #120097, #180804, #73620, #150460, #151448, #103941, #44263, #165621, #118121, #27120, #72617, #28123, #134291, #196962, #55434, #89763, #12935, #119123, #74600, #136267, #197942, #26119, #85769, #163624, #195978, #59411, #121086, #147456, #117105, #178800, #162611, #24116, #70613, #193972, #40270, #149447, #57451, #25127, #86769, #148452, #9947, #133272, #194963, #56441, #179809, #41279, #102941, #164625, #31080, #168583, #184756, #106910, #16901, #13911, #47245, #78552, #32073, #1720, #92727, #48240, #715, #154416, #105921, #61398, #63396, #198939, #183770, #62387, #91722, #75577, #140227, #109895, #123070, #139240, #185757, #30081, #125073, #15910, #14915, #90740, #77568, #46241, #137254, #107895, #93729, #45256, #60406, #108903, #122079, #169582, #124057, #199935, #170582, #155411, #186770, #153417, #171579, #138252, #76576, #167606, #29101, #152423, #198598, #119770, #86430, #166283, #180471, #148116, #75240, #165285, #13573, #168244, #181454, #43919, #103609, #136911, #26778, #88420, #73283, #12603, #120740, #150114, #11615, #57109, #41943, #134953, #196631, #27780, #72269, #60066, #121734, #106567, #182439, #132937, #195636, #56095, #58100, #59073, #42932, #135937, #74267, #90403, #25786, #28766, #9607, #105581, #167267, #89422, #152088, #104596, #197607, #183426, #44910, #71272, #151111, #194624, #117776, #179470, #40935, #102607, #164293, #87432, #149117, #10608, #133946, #118783, #32717, #78202, #45896, #80194, #48882, #111535, #33702, #3357, #123704, #94369, #110537, #188392, #65032, #140875, #18547, #29740, #172218, #187414, #153064, #17545, #156048, #138889, #2364, #199585, #64045, #93373, #184415, #137903, #141866, #62040, #186416, #91373, #61053, #14566, #126688, #76224, #155060, #122725, #95365, #107549, #157050, #49869, #169225, #171228, #30734, #125715, #92381, #154067, #124718, #47893, #15562, #77220, #16555, #369, #79206, #185402, #46893, #108553, #170232, #31725, #109546, #139872, #1361, #63040, #111655, #32838, #16672, #171349, #94488, #156170, #154191, #49990, #125831, #173341, #2485, #80310, #142973, #158156, #62161, #48999, #139994, #140997, #93495, #17669, #155182, #34813, #77342, #141983, #96468, #126805, #19648, #64166, #66140, #107669, #187534, #1483, #169346, #81289 ),
 ( #15681, #4450, #63161, #110655, #30855, #139008, #92502, #127803, #189506, #79327, #488, #188513, #123825, #185523, #47015, #108674, #172335, #170352, #18664, #31844, #78321, #33824, #95484, #124840, #186540, #157170, #3471, #65148, #48013, #109669, #72910, #112641, #20632, #145968, #42563, #174333, #149735, #119405, #143976, #150740, #5456, #129782, #161145, #97449, #67139, #36789, #7450, #160148, #84289, #37802, #73902, #68131, #22642, #12240, #69134, #128797, #52957, #134579, #165907, #35803, #190496, #133562, #191479, #144969, #195252, #26408, #135572, #11236, #159135, #21639, #82284, #99465, #88047, #176332, #103232, #180101, #57735, #51969, #196266, #50981, #181088, #104226, #56737, #27405, #118407, #164914, #89050, #113628, #175323, #41569, #98455, #83293, #6450, #114633, #30359, #16188, #15191, #58705, #13218, #31356, #167883, #4849, #45529, #74881, #47525, #77843, #78834, #993, #170860, #91013, #46522, #90043, #76850, #124347, #153695, #186042, #108181, #138521, #60682, #120375, #136543, #92001, #61673, #32351, #182068, #151725, #198224, #94004, #62667, #122357, #106199, #184046, #107183, #168854, #43551, #139510, #123342, #109181, #185035, #169862, #155685, #17180, #59696, #93007, #29382, #154693, #183060, #197244, #44544, #105217, #166904, #28404, #121367, #152699, #14188, #75857, #137533, #199215, #35322, #140512, #80820, #129304, #33343, #79840, #4964, #49502, #171855, #82801, #37309, #142498, #81793, #190012, #188032, #52476, #173856, #172854, #63680, #20148, #3976, #95002, #65656, #97958, #141510, #156689, #51486, #18183, #50503, #96976, #19171, #158657, #143480, #66650, #2995, #128312, #157681, #64673, #67645, #114135, #189029, #175836, #113148, #2001, #174838, #34335, #125355, #191000, #127318, #98968, #22150, #36303, #159650, #112167, #160658, #21146, #144483, #5967, #187052, #48522, #110176, #126335, #111165, #95996, #85815, #132326, #25173, #69652, #10989, #196021, #71652, #72662, #101990, #165666, #163671, #39314, #86815, #194018, #179854, #55481, #24164, #134337, #176848, #23154, #148501, #193008, #115155, #26166, #180849, #147501, #9992, #133319, #131318, #57497, #117151, #116155, #6961, #195008, #8992, #38319, #70660, #41325, #84798, #99974, #56486, #161658, #178846, #40313, #162658, #118164, #102985, #164670, #146477, #87807, #100973, #7969, #119166, #42326, #149493, #103987, #83800, #145480, #68641, #177846, #130297, #191991, #53478, #54485, #108948, #122124, #184800, #44308, #154463, #167652, #105967, #13955, #153462, #61443, #29148, #90785, #197988, #182826, #152469, #75621, #168626, #12983, #15955, #139285, #14959, #77614, #45301, #27164, #106953, #137301, #30126, #198982, #123115, #60449, #76619, #120142, #91767, #762, #183812, #62433, #138297, #199978, #46286, #150504, #166667, #107942, #169629, #124105, #12001, #181833, #43312, #185805, #31125, #92773, #136313, #47292, #88812, #73664, #135336, #197009, #58475, #104980, #28168, #89810, #151492, #74647, #59458, #121132, #2762, #3745, #156450, #95762, #17950, #174609, #140273, #143246, #36075, #189783, #20909, #65422, #129067, #96741, #127083, #170629, #63443, #109942, #35088, #79603, #1766, #112915, #67412, #172617, #111932, #19918, #141272, #82568, #188791, #64438, #93775, #50274, #110931, #125119, #34105, #128080, #171624, #186817, #81560, #48287, #80587, #173618, #49273, #158430, #4729, #66419, #33112, #51255, #187804, #94768, #97724, #144249, #18942, #5733, #159414, #32118, #190768, #126108, #155456, #52243, #157447, #16946, #78600, #142261, #71419, #131079, #41090, #54251, #192768, #100737, #40070, #148262, #115923, #177613, #84563, #69413, #39081, #162418, #55246, #99741, #102753, #25935, #101747, #164441, #132088, #195789, #193777, #23920, #116914, #85574, #9755, #147261, #163436, #6728, #178607, #87578, #70421, #149265, #24933, #86578, #8751, #37074, #53241, #133083, #194773, #10757, #98734 ),
 ( #56247, #117928, #72421, #134098, #68406, #179618, #146241, #113900, #161425, #175598, #22917, #160427, #83568, #21916, #145247, #130058, #191758, #114918, #176611, #38085, #7727, #57261, #197756, #46048, #42093, #11767, #150272, #92537, #61207, #182592, #166437, #120892, #44076, #105735, #103758, #199741, #75391, #122879, #152240, #29893, #154226, #107703, #73433, #198753, #89575, #90558, #43079, #167422, #104746, #184567, #26932, #91531, #169382, #76383, #30890, #13725, #15716, #183581, #137063, #118935, #59223, #77376, #135104, #196780, #121888, #27932, #88574, #139044, #180620, #28918, #60218, #106724, #151261, #165437, #45066, #12751, #58248, #168398, #153218, #119916, #14723, #138060, #181602, #74416, #136082, #16707, #110691, #157207, #79364, #18701, #80348, #126844, #63198, #142020, #17707, #93533, #127840, #174371, #49036, #112679, #33861, #524, #3509, #94525, #62196, #189546, #141035, #51018, #82322, #95521, #158195, #2522, #35841, #64202, #125869, #187569, #188550, #34850, #172371, #65185, #171388, #156207, #50028, #111693, #173380, #186577, #97487, #159173, #96505, #20668, #19685, #123860, #81327, #143010, #4488, #66178, #185558, #47052, #108709, #155218, #170388, #31879, #78357, #140031, #1520, #124878, #48050, #109706, #32875, #177376, #85330, #179381, #132847, #38848, #100505, #40843, #194535, #130840, #178369, #147022, #8506, #52006, #163188, #5493, #113665, #162184, #56006, #67176, #39833, #9517, #36827, #102517, #98493, #22680, #54014, #190532, #160186, #129820, #23682, #52996, #70184, #192531, #164200, #161184, #115688, #25698, #131852, #21676, #146006, #24692, #117684, #128833, #83330, #193535, #84327, #37843, #55009, #116679, #144012, #101499, #175359, #114674, #145007, #86341, #148028, #69174, #71183, #6488, #68168, #191519, #176370, #99503, #7489, #106478, #167182, #44823, #105496, #136824, #60966, #199500, #107463, #120656, #152002, #137816, #13488, #57018, #182354, #168157, #28681, #149029, #103519, #121646, #58014, #90316, #135851, #165195, #122640, #29654, #169139, #91286, #184330, #181367, #75153, #152977, #45812, #87343, #198508, #76138, #10517, #14476, #72180, #133854, #59979, #183341, #196544, #195544, #118691, #180383, #151026, #41853, #26690, #88330, #119684, #43832, #150021, #11526, #73196, #134866, #42846, #12517, #104511, #166192, #27693, #89334, #74181, #197521, #58989, #111450, #141781, #173137, #48798, #34612, #125629, #3275, #65934, #81096, #185316, #172133, #62951, #63960, #16468, #155962, #78117, #96271, #285, #64947, #157957, #49785, #142774, #187327, #189305, #156965, #110452, #30644, #171141, #19448, #123621, #170143, #95282, #139786, #61954, #4255, #127606, #32630, #33619, #80113, #1274, #50782, #18462, #124631, #153981, #126606, #94284, #46807, #17459, #188308, #31638, #108466, #112442, #93287, #140788, #92297, #109458, #15478, #77135, #138804, #154972, #186326, #47808, #79115, #2277, #147790, #22437, #86099, #7247, #174131, #53770, #67929, #35602, #162943, #52754, #101254, #55765, #68932, #131606, #191279, #24450, #114423, #176124, #160944, #100262, #8262, #37595, #99257, #144765, #129583, #84086, #145765, #115444, #159942, #9276, #70942, #161943, #132610, #192290, #97248, #177135, #130594, #38606, #23438, #69942, #85085, #146769, #66930, #193291, #194299, #54765, #158936, #116439, #178128, #39595, #20425, #113424, #82075, #143768, #5249, #128593, #190287, #51763, #175116, #36584, #98239, #83089, #21429, #6250, #104270, #163964, #59741, #14232, #119447, #58748, #166945, #164957, #29424, #150785, #149778, #40605, #197285, #57777, #148787, #181132, #74922, #56779, #10276, #28448, #133605, #27452, #73945, #196307, #135614, #120417, #43593, #180143, #182108, #134623, #71935, #44585, #91055, #165952, #152742, #12280, #117439, #105259, #11280, #179137, #106242, #42606, #167924, #199261, #90084, #136585, #89093, #75903, #151766, #13259, #198265, #121410 ),
 ( #183104, #195298, #137577, #102276, #25462, #87102, #118452, #41612, #103277, #26450, #88092, #72953, #160460, #113934, #50309, #97760, #66452, #128113, #168899, #82600, #122402, #30405, #158465, #52276, #184092, #159447, #129103, #153740, #21951, #15236, #139556, #173657, #107228, #76895, #46568, #19953, #169909, #96776, #111965, #83601, #77888, #35124, #145280, #81595, #138566, #62713, #144281, #175633, #45575, #44, #143279, #1040, #154740, #4765, #36108, #60728, #20943, #92051, #31402, #61719, #189817, #5770, #186090, #112950, #51289, #67445, #123387, #190802, #185079, #108229, #174643, #37107, #93053, #98766, #16236, #124395, #103789, #99776, #85609, #116949, #53274, #22951, #192803, #101782, #25967, #133117, #42128, #57292, #161461, #148296, #39114, #40104, #54286, #132120, #115958, #10790, #176646, #179653, #72458, #87610, #118969, #163470, #165469, #194806, #24967, #6763, #147296, #195821, #84599, #146278, #71452, #177646, #38122, #149296, #26965, #8785, #9790, #56280, #100770, #180652, #86613, #162453, #130096, #117962, #70455, #7765, #193813, #164473, #69448, #131115, #41123, #23954, #178641, #102787, #55278, #134132, #88608, #68442, #191793, #114953, #167456, #43113, #77411, #123898, #198787, #62230, #183618, #150304, #29929, #44111, #11801, #139081, #28952, #559, #31915, #45101, #107739, #90593, #185597, #152275, #13759, #137101, #76419, #184603, #75427, #60253, #120927, #105769, #121924, #106758, #91568, #136116, #47086, #108747, #138095, #170423, #168433, #73465, #153256, #14758, #199776, #61243, #46084, #122915, #169420, #104781, #30925, #135138, #92573, #196812, #154261, #15752, #58279, #119948, #181633, #166469, #27967, #89607, #151296, #12785, #74450, #197792, #59258, #182626, #124914, #35876, #190567, #95557, #34886, #143045, #141073, #5529, #126881, #125906, #16743, #173415, #33900, #186612, #157244, #51052, #32910, #48084, #4523, #109740, #3543, #50068, #172411, #111729, #96541, #19719, #156243, #158229, #110730, #171424, #20703, #67209, #142057, #128867, #188587, #93568, #81361, #187605, #155254, #82359, #18738, #144047, #175394, #66216, #112714, #80385, #52042, #65221, #127876, #189580, #174407, #97522, #159209, #113698, #64240, #49074, #78392, #140068, #1559, #79402, #63235, #94564, #17745, #2558, #55043, #118727, #116713, #192566, #178403, #147058, #132880, #8541, #86375, #129856, #39867, #164235, #193571, #25731, #148060, #101533, #100539, #160222, #176405, #70219, #163226, #72214, #21712, #191554, #53031, #133888, #40878, #162218, #146040, #23717, #85365, #131886, #83366, #179413, #24726, #9551, #56039, #71217, #195580, #87377, #114712, #194569, #69208, #117717, #22715, #102551, #84362, #149062, #6524, #10550, #57052, #36862, #98529, #145042, #68203, #54049, #37880, #99538, #161220, #7524, #130876, #115723, #177411, #38882, #74214, #41887, #169172, #59021, #107495, #61985, #75185, #137851, #197553, #30676, #120688, #182387, #167216, #106513, #14509, #43865, #105530, #151057, #135882, #28713, #90350, #121680, #166224, #92329, #154015, #168191, #15510, #198542, #180415, #60013, #152035, #183376, #13520, #76171, #136857, #29687, #73228, #44857, #77167, #91319, #138837, #153010, #199531, #61001, #103554, #119716, #122673, #184362, #317, #165229, #134899, #196576, #26724, #45843, #88363, #89368, #150056, #11562, #58046, #181400, #42878, #104543, #27725, #12548, #49815, #158966, #174163, #78151, #64976, #155995, #156995, #109493, #48828, #171176, #127635, #93322, #96300, #189335, #142803, #35633, #18493, #82107, #111480, #80141, #123651, #63990, #112470, #16503, #62986, #188337, #32663, #155006, #65964, #20457, #125661, #126635, #173165, #94317, #97278, #141811, #17491, #46839, #3304, #187358, #139819, #110481, #81123, #124665, #1308, #34641, #186361, #33649, #157986, #2309, #19477, #4284, #50813, #47841, #143799, #79149, #5282, #140820, #172164, #185349, #108499 ),
 ( #95310, #170179, #31672, #84117, #53801, #193323, #101286, #7279, #145796, #37626, #22469, #68963, #115477, #8295, #52785, #194330, #179168, #54797, #55798, #85118, #148818, #146802, #130625, #69973, #177165, #162976, #38638, #116472, #159973, #131640, #117470, #23469, #40636, #178161, #39626, #192321, #190318, #6281, #100295, #24481, #102305, #51795, #21460, #83122, #163994, #70974, #161973, #176155, #86131, #147823, #9308, #113454, #132642, #25491, #87133, #66965, #128625, #175147, #36615, #144798, #98271, #99289, #67959, #114454, #129614, #160975, #191309, #180175, #183134, #14266, #29455, #60761, #105288, #168931, #136615, #166976, #10308, #150814, #199294, #103308, #149808, #74952, #119478, #41643, #152774, #107260, #12311, #151797, #59773, #57807, #122433, #43625, #42637, #133639, #90113, #73976, #164987, #135645, #167956, #11314, #26482, #121442, #88124, #120447, #28479, #89126, #13288, #198296, #118484, #91087, #71965, #72984, #44618, #184125, #195330, #106271, #75935, #134653, #30437, #196339, #197315, #182141, #56810, #181161, #104300, #137610, #45607, #92084, #58779, #165983, #27483, #63755, #50582, #48597, #31431, #155758, #172934, #65732, #76928, #93085, #171930, #94079, #47600, #125429, #126411, #173933, #49580, #79, #62744, #123417, #2076, #188108, #78909, #3073, #79913, #157761, #154769, #96071, #35401, #34413, #19251, #33419, #111243, #95078, #64749, #127400, #189109, #153773, #187125, #18260, #4054, #141585, #185110, #110249, #80898, #156766, #15268, #169940, #142575, #124424, #112242, #138597, #16266, #61749, #46600, #108260, #77917, #139584, #109254, #1069, #186120, #170933, #32425, #17256, #140586, #97052, #116235, #54563, #20224, #84879, #161740, #6049, #8052, #66732, #131399, #160738, #51564, #5046, #9070, #129385, #53558, #158734, #128392, #81872, #70740, #178929, #22230, #190089, #177926, #113228, #39394, #55562, #143564, #38398, #101054, #69731, #162739, #85896, #192076, #115236, #194100, #147584, #83879, #193087, #100054, #23235, #67727, #174918, #24247, #117236, #99049, #146556, #132408, #144563, #36382, #130378, #191081, #98036, #176928, #37391, #159733, #145561, #21230, #82885, #52554, #114215, #175920, #7039, #68721, #119245, #58555, #197088, #166746, #103070, #181911, #57575, #133401, #167728, #14032, #88891, #152544, #73745, #40399, #120221, #134419, #102070, #29226, #180929, #90859, #122200, #135417, #198068, #42404, #75697, #104067, #165749, #27242, #28249, #74727, #150583, #12082, #11070, #196105, #43391, #105062, #89889, #26247, #137377, #199056, #151572, #60525, #13061, #163755, #136391, #59534, #121213, #182903, #44387, #106042, #25255, #195090, #86897, #148581, #10072, #71731, #56573, #118247, #179938, #41405, #164752, #87887, #149574, #72748, #168702, #138373, #76697, #19019, #187880, #109026, #92851, #47371, #170705, #32195, #30204, #126184, #93852, #48365, #2839, #110021, #80665, #34180, #200053, #125198, #16033, #17024, #169706, #155529, #31200, #49347, #153539, #156529, #111009, #64517, #95841, #78677, #142341, #171700, #140353, #183892, #124185, #172695, #61522, #123191, #33189, #1841, #185886, #77691, #63523, #18028, #3821, #79682, #91845, #154537, #15036, #186894, #141352, #94848, #157525, #65500, #45377, #184880, #107030, #46362, #108020, #139359, #840, #62513, #175677, #145324, #146320, #84643, #131158, #52322, #160504, #22995, #21994, #35168, #113979, #53318, #37151, #188869, #19995, #130140, #112994, #83647, #67490, #81639, #7809, #114996, #192847, #176691, #69493, #36152, #6807, #38165, #127161, #50352, #191837, #112011, #173700, #96823, #158508, #4809, #99820, #161505, #129148, #143322, #174688, #66497, #68485, #159493, #97804, #128160, #98811, #189860, #20988, #82643, #51334, #144326, #5815, #190845, #180914, #148567, #42389, #87871, #25241, #149559, #179923, #165732, #41390, #119230, #162726, #11055, #197074, #26232, #58541, #104052 ),
 ( #178915, #133385, #195076, #56555, #116222, #12068, #118232, #134403, #88876, #196090, #105047, #120207, #24231, #72730, #102056, #103055, #55548, #164737, #117221, #73730, #39381, #27228, #181897, #43375, #57560, #166731, #150569, #69718, #135403, #163741, #131385, #28235, #10057, #89875, #151558, #193074, #54549, #86882, #177913, #71717, #101040, #85882, #147570, #9055, #70726, #132393, #40382, #194086, #15022, #61509, #154523, #199042, #140341, #125186, #171687, #124171, #91832, #185872, #31186, #168689, #92838, #123178, #109013, #184867, #62500, #106029, #16020, #1829, #169692, #63511, #47358, #77677, #76683, #136377, #152531, #46349, #139346, #48352, #198054, #167715, #29213, #110006, #17012, #138359, #122187, #200040, #108007, #825, #59520, #155517, #170692, #32181, #93837, #78664, #33176, #186882, #90846, #94835, #45364, #13047, #60512, #74714, #183879, #121197, #182890, #44373, #14018, #75684, #137363, #107017, #30190, #153525, #51320, #156514, #96809, #145312, #49334, #95828, #20974, #65486, #187866, #98799, #53307, #158495, #97791, #5803, #3808, #68474, #189846, #188856, #79668, #36139, #19982, #110996, #81625, #113966, #157512, #172682, #67476, #34166, #66484, #112981, #35153, #174674, #159480, #82631, #19006, #144313, #173687, #80652, #129136, #114985, #6796, #143308, #190833, #52309, #175665, #64504, #37140, #18015, #126171, #160493, #130129, #141339, #21983, #83635, #142328, #176678, #127148, #4795, #128146, #2826, #50339, #111996, #191826, #38154, #164503, #86643, #119976, #116980, #9821, #196841, #194838, #177677, #101813, #118999, #11830, #22982, #39145, #117994, #40136, #193844, #71482, #72489, #181662, #195851, #146309, #8815, #69482, #148326, #134162, #24999, #149325, #25996, #103818, #100800, #42158, #99808, #180682, #165498, #179683, #57323, #41155, #10819, #73496, #135168, #161494, #133147, #87639, #150335, #26994, #131147, #56311, #88639, #102818, #84632, #115988, #58308, #70485, #7798, #192835, #162484, #54316, #23985, #85642, #147328, #132151, #55308, #178672, #163501, #1586, #78419, #154289, #31941, #43141, #62257, #585, #166499, #30952, #107765, #152303, #15779, #12813, #77438, #106787, #197821, #151325, #155281, #75454, #199805, #104810, #74480, #27997, #16771, #124941, #108772, #137128, #59287, #139110, #123925, #63261, #89636, #184631, #185623, #47113, #170450, #93595, #138124, #136145, #169450, #61272, #120956, #183646, #140095, #182655, #44139, #92599, #13787, #105798, #167484, #28980, #45128, #46112, #90621, #198815, #60280, #76447, #121953, #168461, #122942, #29959, #91596, #153286, #14787, #125931, #79427, #97549, #2585, #96568, #143073, #65248, #4551, #66244, #112740, #49100, #127904, #3570, #141098, #113727, #160251, #34912, #98557, #19746, #186638, #189606, #80412, #48109, #175424, #126908, #36892, #68230, #81387, #144076, #188614, #21741, #50095, #111755, #173444, #174433, #20731, #158256, #51080, #157269, #142084, #35903, #159237, #82388, #172439, #83393, #145070, #6552, #5557, #67236, #128895, #190594, #52070, #109765, #171449, #32937, #94592, #156270, #64265, #17772, #187630, #110758, #33927, #95585, #18765, #193600, #53061, #69238, #163256, #71247, #165259, #114740, #84391, #22742, #26753, #133920, #55072, #38909, #116742, #178432, #39899, #176434, #72243, #101565, #194598, #149092, #56070, #88393, #180446, #146067, #132911, #162248, #24758, #115751, #86405, #177439, #195611, #99567, #102582, #57083, #10582, #41918, #148090, #37908, #103584, #23747, #9581, #191583, #161248, #129883, #150086, #11590, #118757, #85396, #7552, #40909, #130904, #192594, #54077, #117750, #100566, #164266, #147089, #8573, #179443, #25761, #70248, #131916, #87407, #107524, #76200, #137879, #181428, #92357, #134927, #42906, #168219, #62014, #196604, #169201, #138865, #166254, #170207, #27754, #152064, #183403, #119745, #89397, #73258, #345, #199560, #61029, #60042, #93349 ),
 ( #123678, #29716, #31700, #122701, #91348, #58075, #13549, #185377, #151086, #12577, #184391, #182415, #104572, #15538, #155035, #75215, #14539, #45871, #120716, #46867, #106543, #105558, #74242, #153040, #136887, #135911, #198572, #30707, #197582, #59049, #154043, #43895, #44886, #77196, #121710, #108528, #167244, #28743, #90379, #158014, #33676, #109521, #143829, #190347, #65005, #128652, #49843, #16530, #96327, #110510, #78177, #5309, #95338, #66993, #98301, #111507, #174191, #157023, #51823, #18521, #80168, #3331, #142832, #50840, #113483, #35659, #139846, #20486, #175177, #172191, #81150, #97307, #36643, #1335, #127663, #63015, #124694, #158993, #82135, #186391, #4311, #65994, #125688, #189363, #47868, #112497, #141840, #171203, #32693, #94344, #48855, #173193, #156023, #17520, #79178, #140849, #2338, #64019, #126662, #187387, #188366, #34669, #19505, #41672, #101316, #40665, #71004, #102334, #148847, #54828, #116502, #56838, #10338, #146832, #194360, #163005, #24512, #67987, #179197, #21490, #129641, #178190, #71994, #83151, #55827, #25520, #52815, #118513, #114482, #38668, #70001, #6309, #176186, #160002, #87166, #86162, #147852, #8326, #180203, #177195, #131671, #144825, #39655, #37655, #162002, #164024, #133668, #191337, #99320, #9339, #100323, #53833, #193352, #132672, #161004, #117500, #22498, #68992, #84145, #195358, #145824, #85146, #7307, #130656, #192350, #115507, #23498, #123442, #122459, #184152, #183162, #60788, #121470, #152803, #76953, #15293, #185135, #136641, #167984, #153799, #29482, #73013, #198324, #45633, #44646, #165016, #119509, #137636, #74003, #106298, #151824, #181190, #182168, #91113, #59800, #14295, #166013, #75963, #120477, #196368, #30462, #138623, #13313, #104, #199323, #103336, #107285, #197345, #26509, #92110, #43653, #61774, #88153, #168956, #149838, #105316, #11342, #167003, #28505, #90139, #134682, #57836, #74979, #42668, #135673, #58808, #104329, #27513, #89154, #150843, #12339, #158759, #5072, #157787, #125456, #19277, #64777, #2103, #126438, #156794, #142601, #18287, #96098, #139609, #188136, #173958, #3099, #35425, #80924, #49607, #110277, #169964, #186148, #79942, #111270, #81896, #31457, #1095, #62771, #143589, #50607, #171958, #155786, #33446, #95105, #141612, #93109, #189135, #172961, #34439, #65758, #4080, #66755, #97078, #124452, #127427, #78937, #112266, #32454, #20249, #94107, #128416, #16292, #46626, #108286, #154794, #77942, #47627, #109282, #170960, #17283, #140613, #187153, #63784, #48625, #129409, #54583, #99076, #21254, #132428, #86920, #192103, #131423, #39414, #37416, #102091, #23260, #22256, #113252, #69753, #130405, #82909, #53586, #147605, #191106, #144587, #101074, #6073, #100080, #146583, #36405, #194120, #176955, #116256, #9093, #177947, #25277, #40420, #67751, #193109, #83905, #84903, #175947, #115262, #160766, #55583, #159759, #162759, #117257, #70760, #163776, #8077, #148602, #24268, #85917, #190112, #38424, #178950, #52580, #114240, #10094, #145588, #7066, #71754, #51587, #161765, #174943, #98060, #68747, #48146, #166768, #165769, #56595, #13081, #73764, #164774, #135437, #90880, #72770, #26268, #44408, #149596, #43412, #89907, #12101, #151590, #74746, #59554, #196125, #136409, #150605, #87910, #63299, #109803, #181930, #171486, #28269, #133423, #198088, #27264, #195112, #124979, #197107, #186676, #17809, #121232, #152563, #58574, #32975, #120240, #105082, #182925, #106062, #167748, #29246, #14052, #104087, #88913, #75720, #137396, #199077, #119265, #94629, #156308, #118269, #179959, #41426, #103092, #11094, #134440, #57596, #180948, #42425, #189643, #128931, #172477, #97585, #6589, #35939, #68268, #190632, #159273, #143110, #2625, #18804, #112777, #20769, #114776, #64302, #33964, #95622, #176470, #83429, #4589, #188653, #66282, #127941, #51118, #79466, #129919, #144113, #5593, #174470, #99604, #96605, #82424, #37944 ) ),
 .UNSPECIFIED., .T., .F., .F. ) 
 B_SPLINE_SURFACE_WITH_KNOTS ( ( 4, 3, 4 ),
 ( 3, 2, 2, 2, 2, 2, 2, 2, 2, 2, 2, 2, 2, 2, 2, 2, 2, 2, 2, 2, 2, 2, 2, 2, 2, 2, 2, 2, 2, 2, 2, 2, 2, 2, 2, 2, 2, 2, 2, 2, 2, 2, 2, 2, 2, 2, 2, 2, 2, 2, 2, 2, 2, 2, 2, 2, 2, 2, 2, 2, 2, 2, 2, 2, 2, 2, 2, 2, 2, 2, 2, 2, 2, 2, 2, 2, 2, 2, 2, 2, 2, 2, 2, 2, 2, 2, 2, 2, 2, 2, 2, 2, 2, 2, 2, 2, 2, 2, 2, 2, 2, 2, 2, 2, 2, 2, 2, 2, 2, 2, 2, 2, 2, 2, 2, 2, 2, 2, 2, 2, 2, 2, 2, 2, 2, 2, 2, 2, 2, 2, 2, 2, 2, 2, 2, 2, 2, 2, 2, 2, 2, 2, 2, 2, 2, 2, 2, 2, 2, 2, 2, 2, 2, 2, 2, 2, 2, 2, 2, 2, 2, 2, 2, 2, 2, 2, 2, 2, 2, 2, 2, 2, 2, 2, 2, 2, 2, 2, 2, 2, 2, 2, 2, 2, 2, 2, 2, 2, 2, 2, 2, 2, 2, 2, 2, 2, 2, 2, 2, 2, 2, 2, 2, 2, 2, 2, 2, 2, 2, 2, 2, 2, 2, 2, 2, 2, 2, 2, 2, 2, 2, 2, 2, 2, 2, 2, 2, 2, 3 ),
 ( 0.000000000000000000, 0.5000000000000000000, 1.000000000000000000 ),
 ( 0.000000000000000000, 0.004385964912280701511, 0.008771929824561403022, 0.01315789473684210453, 0.01754385964912280604, 0.02192982456140350755, 0.02631578947368420907, 0.03070175438596491058, 0.03508771929824561209, 0.03947368421052631360, 0.04385964912280701511, 0.04824561403508771662, 0.05263157894736841813, 0.05701754385964911964, 0.06140350877192982115, 0.06578947368421052266, 0.07017543859649122417, 0.07456140350877192569, 0.07894736842105262720, 0.08333333333333332871, 0.08771929824561403022, 0.09210526315789473173, 0.09649122807017543324, 0.1008771929824561348, 0.1052631578947368363, 0.1096491228070175378, 0.1140350877192982393, 0.1184210526315789408, 0.1228070175438596423, 0.1271929824561403577, 0.1315789473684210453, 0.1359649122807017607, 0.1403508771929824483, 0.1447368421052631637, 0.1491228070175438514, 0.1535087719298245668, 0.1578947368421052544, 0.1622807017543859698, 0.1666666666666666574, 0.1710526315789473728, 0.1754385964912280604, 0.1798245614035087758, 0.1842105263157894635, 0.1885964912280701788, 0.1929824561403508665, 0.1973684210526315819, 0.2017543859649122695, 0.2061403508771929849, 0.2105263157894736725, 0.2149122807017543879, 0.2192982456140350755, 0.2236842105263157909, 0.2280701754385964786, 0.2324561403508771940, 0.2368421052631578816, 0.2412280701754385970, 0.2456140350877192846, 0.2500000000000000000, 0.2543859649122807154, 0.2587719298245614308, 0.2631578947368420907, 0.2675438596491228060, 0.2719298245614035214, 0.2763157894736842368, 0.2807017543859648967, 0.2850877192982456121, 0.2894736842105263275, 0.2938596491228070429, 0.2982456140350877027, 0.3026315789473684181, 0.3070175438596491335, 0.3114035087719298489, 0.3157894736842105088, 0.3201754385964912242, 0.3245614035087719396, 0.3289473684210526550, 0.3333333333333333148, 0.3377192982456140302, 0.3421052631578947456, 0.3464912280701754610, 0.3508771929824561209, 0.3552631578947368363, 0.3596491228070175517, 0.3640350877192982670, 0.3684210526315789269, 0.3728070175438596423, 0.3771929824561403577, 0.3815789473684210731, 0.3859649122807017330, 0.3903508771929824483, 0.3947368421052631637, 0.3991228070175438791, 0.4035087719298245390, 0.4078947368421052544, 0.4122807017543859698, 0.4166666666666666852, 0.4210526315789473450, 0.4254385964912280604, 0.4298245614035087758, 0.4342105263157894912, 0.4385964912280701511, 0.4429824561403508665, 0.4473684210526315819, 0.4517543859649122973, 0.4561403508771929571, 0.4605263157894736725, 0.4649122807017543879, 0.4692982456140351033, 0.4736842105263157632, 0.4780701754385964786, 0.4824561403508771940, 0.4868421052631579093, 0.4912280701754385692, 0.4956140350877192846, 0.5000000000000000000, 0.5043859649122807154, 0.5087719298245614308, 0.5131578947368421462, 0.5175438596491228616, 0.5219298245614034659, 0.5263157894736841813, 0.5307017543859648967, 0.5350877192982456121, 0.5394736842105263275, 0.5438596491228070429, 0.5482456140350877583, 0.5526315789473684736, 0.5570175438596490780, 0.5614035087719297934, 0.5657894736842105088, 0.5701754385964912242, 0.5745614035087719396, 0.5789473684210526550, 0.5833333333333333703, 0.5877192982456140857, 0.5921052631578946901, 0.5964912280701754055, 0.6008771929824561209, 0.6052631578947368363, 0.6096491228070175517, 0.6140350877192982670, 0.6184210526315789824, 0.6228070175438596978, 0.6271929824561403022, 0.6315789473684210176, 0.6359649122807017330, 0.6403508771929824483, 0.6447368421052631637, 0.6491228070175438791, 0.6535087719298245945, 0.6578947368421053099, 0.6622807017543859143, 0.6666666666666666297, 0.6710526315789473450, 0.6754385964912280604, 0.6798245614035087758, 0.6842105263157894912, 0.6885964912280702066, 0.6929824561403509220, 0.6973684210526315264, 0.7017543859649122417, 0.7061403508771929571, 0.7105263157894736725, 0.7149122807017543879, 0.7192982456140351033, 0.7236842105263158187, 0.7280701754385965341, 0.7324561403508771384, 0.7368421052631578538, 0.7412280701754385692, 0.7456140350877192846, 0.7500000000000000000, 0.7543859649122807154, 0.7587719298245614308, 0.7631578947368421462, 0.7675438596491228616, 0.7719298245614034659, 0.7763157894736841813, 0.7807017543859648967, 0.7850877192982456121, 0.7894736842105263275, 0.7938596491228070429, 0.7982456140350877583, 0.8026315789473684736, 0.8070175438596490780, 0.8114035087719297934, 0.8157894736842105088, 0.8201754385964912242, 0.8245614035087719396, 0.8289473684210526550, 0.8333333333333333703, 0.8377192982456140857, 0.8421052631578946901, 0.8464912280701754055, 0.8508771929824561209, 0.8552631578947368363, 0.8596491228070175517, 0.8640350877192982670, 0.8684210526315789824, 0.8728070175438596978, 0.8771929824561403022, 0.8815789473684210176, 0.8859649122807017330, 0.8903508771929824483, 0.8947368421052631637, 0.8991228070175438791, 0.9035087719298245945, 0.9078947368421053099, 0.9122807017543859143, 0.9166666666666666297, 0.9210526315789473450, 0.9254385964912280604, 0.9298245614035087758, 0.9342105263157894912, 0.9385964912280702066, 0.9429824561403509220, 0.9473684210526315264, 0.9517543859649122417, 0.9561403508771929571, 0.9605263157894736725, 0.9649122807017543879, 0.9692982456140351033, 0.9736842105263158187, 0.9780701754385965341, 0.9824561403508771384, 0.9868421052631578538, 0.9912280701754385692, 0.9956140350877192846, 1.000000000000000000 ),
 .UNSPECIFIED. ) 
 GEOMETRIC_REPRESENTATION_ITEM ( )  RATIONAL_B_SPLINE_SURFACE ( (
 ( 1.000000000000000000, 0.9659258262890683122, 1.000000000000000000, 0.9659258262890683122, 1.000000000000000000, 0.9659258262890683122, 1.000000000000000000, 0.9659258262890683122, 1.000000000000000000, 0.9659258262890683122, 1.000000000000000000, 0.9659258262890683122, 1.000000000000000000, 0.9659258262890683122, 1.000000000000000000, 0.9659258262890683122, 1.000000000000000000, 0.9659258262890683122, 1.000000000000000000, 0.9659258262890683122, 1.000000000000000000, 0.9659258262890683122, 1.000000000000000000, 0.9659258262890683122, 1.000000000000000000, 0.9659258262890683122, 1.000000000000000000, 0.9659258262890683122, 1.000000000000000000, 0.9659258262890683122, 1.000000000000000000, 0.9659258262890683122, 1.000000000000000000, 0.9659258262890683122, 1.000000000000000000, 0.9659258262890683122, 1.000000000000000000, 0.9659258262890683122, 1.000000000000000000, 0.9659258262890683122, 1.000000000000000000, 0.9659258262890683122, 1.000000000000000000, 0.9659258262890683122, 1.000000000000000000, 0.9659258262890683122, 1.000000000000000000, 0.9659258262890683122, 1.000000000000000000, 0.9659258262890683122, 1.000000000000000000, 0.9659258262890683122, 1.000000000000000000, 0.9659258262890683122, 1.000000000000000000, 0.9659258262890683122, 1.000000000000000000, 0.9659258262890683122, 1.000000000000000000, 0.9659258262890683122, 1.000000000000000000, 0.9659258262890683122, 1.000000000000000000, 0.9659258262890683122, 1.000000000000000000, 0.9659258262890683122, 1.000000000000000000, 0.9659258262890683122, 1.000000000000000000, 0.9659258262890683122, 1.000000000000000000, 0.9659258262890683122, 1.000000000000000000, 0.9659258262890683122, 1.000000000000000000, 0.9659258262890683122, 1.000000000000000000, 0.9659258262890683122, 1.000000000000000000, 0.9659258262890683122, 1.000000000000000000, 0.9659258262890683122, 1.000000000000000000, 0.9659258262890683122, 1.000000000000000000, 0.9659258262890683122, 1.000000000000000000, 0.9659258262890683122, 1.000000000000000000, 0.9659258262890683122, 1.000000000000000000, 0.9659258262890683122, 1.000000000000000000, 0.9659258262890683122, 1.000000000000000000, 0.9659258262890683122, 1.000000000000000000, 0.9659258262890683122, 1.000000000000000000, 0.9659258262890683122, 1.000000000000000000, 0.9659258262890683122, 1.000000000000000000, 0.9659258262890683122, 1.000000000000000000, 0.9659258262890683122, 1.000000000000000000, 0.9659258262890683122, 1.000000000000000000, 0.9659258262890683122, 1.000000000000000000, 0.9659258262890683122, 1.000000000000000000, 0.9659258262890683122, 1.000000000000000000, 0.9659258262890683122, 1.000000000000000000, 0.9659258262890683122, 1.000000000000000000, 0.9659258262890683122, 1.000000000000000000, 0.9659258262890683122, 1.000000000000000000, 0.9659258262890683122, 1.000000000000000000, 0.9659258262890683122, 1.000000000000000000, 0.9659258262890683122, 1.000000000000000000, 0.9659258262890683122, 1.000000000000000000, 0.9659258262890683122, 1.000000000000000000, 0.9659258262890683122, 1.000000000000000000, 0.9659258262890683122, 1.000000000000000000, 0.9659258262890683122, 1.000000000000000000, 0.9659258262890683122, 1.000000000000000000, 0.9659258262890683122, 1.000000000000000000, 0.9659258262890683122, 1.000000000000000000, 0.9659258262890683122, 1.000000000000000000, 0.9659258262890683122, 1.000000000000000000, 0.9659258262890683122, 1.000000000000000000, 0.9659258262890683122, 1.000000000000000000, 0.9659258262890683122, 1.000000000000000000, 0.9659258262890683122, 1.000000000000000000, 0.9659258262890683122, 1.000000000000000000, 0.9659258262890683122, 1.000000000000000000, 0.9659258262890683122, 1.000000000000000000, 0.9659258262890683122, 1.000000000000000000, 0.9659258262890683122, 1.000000000000000000, 0.9659258262890683122, 1.000000000000000000, 0.9659258262890683122, 1.000000000000000000, 0.9659258262890683122, 1.000000000000000000, 0.9659258262890683122, 1.000000000000000000, 0.9659258262890683122, 1.000000000000000000, 0.9659258262890683122, 1.000000000000000000, 0.9659258262890683122, 1.000000000000000000, 0.9659258262890683122, 1.000000000000000000, 0.9659258262890683122, 1.000000000000000000, 0.9659258262890683122, 1.000000000000000000, 0.9659258262890683122, 1.000000000000000000, 0.9659258262890683122, 1.000000000000000000, 0.9659258262890683122, 1.000000000000000000, 0.9659258262890683122, 1.000000000000000000, 0.9659258262890683122, 1.000000000000000000, 0.9659258262890683122, 1.000000000000000000, 0.9659258262890683122, 1.000000000000000000, 0.9659258262890683122, 1.000000000000000000, 0.9659258262890683122, 1.000000000000000000, 0.9659258262890683122, 1.000000000000000000, 0.9659258262890683122, 1.000000000000000000, 0.9659258262890683122, 1.000000000000000000, 0.9659258262890683122, 1.000000000000000000, 0.9659258262890683122, 1.000000000000000000, 0.9659258262890683122, 1.000000000000000000, 0.9659258262890683122, 1.000000000000000000, 0.9659258262890683122, 1.000000000000000000, 0.9659258262890683122, 1.000000000000000000, 0.9659258262890683122, 1.000000000000000000, 0.9659258262890683122, 1.000000000000000000, 0.9659258262890683122, 1.000000000000000000, 0.9659258262890683122, 1.000000000000000000, 0.9659258262890683122, 1.000000000000000000, 0.9659258262890683122, 1.000000000000000000, 0.9659258262890683122, 1.000000000000000000, 0.9659258262890683122, 1.000000000000000000, 0.9659258262890683122, 1.000000000000000000, 0.9659258262890683122, 1.000000000000000000, 0.9659258262890683122, 1.000000000000000000, 0.9659258262890683122, 1.000000000000000000, 0.9659258262890683122, 1.000000000000000000, 0.9659258262890683122, 1.000000000000000000, 0.9659258262890683122, 1.000000000000000000, 0.9659258262890683122, 1.000000000000000000, 0.9659258262890683122, 1.000000000000000000, 0.9659258262890683122, 1.000000000000000000, 0.9659258262890683122, 1.000000000000000000, 0.9659258262890683122, 1.000000000000000000, 0.9659258262890683122, 1.000000000000000000, 0.9659258262890683122, 1.000000000000000000, 0.9659258262890683122, 1.000000000000000000, 0.9659258262890683122, 1.000000000000000000, 0.9659258262890683122, 1.000000000000000000, 0.9659258262890683122, 1.000000000000000000, 0.9659258262890683122, 1.000000000000000000, 0.9659258262890683122, 1.000000000000000000, 0.9659258262890683122, 1.000000000000000000, 0.9659258262890683122, 1.000000000000000000, 0.9659258262890683122, 1.000000000000000000, 0.9659258262890683122, 1.000000000000000000, 0.9659258262890683122, 1.000000000000000000, 0.9659258262890683122, 1.000000000000000000, 0.9659258262890683122, 1.000000000000000000, 0.9659258262890683122, 1.000000000000000000, 0.9659258262890683122, 1.000000000000000000, 0.9659258262890683122, 1.000000000000000000, 0.9659258262890683122, 1.000000000000000000, 0.9659258262890683122, 1.000000000000000000, 0.9659258262890683122, 1.000000000000000000, 0.9659258262890683122, 1.000000000000000000, 0.9659258262890683122, 1.000000000000000000, 0.9659258262890683122, 1.000000000000000000, 0.9659258262890683122, 1.000000000000000000, 0.9659258262890683122, 1.000000000000000000, 0.9659258262890683122, 1.000000000000000000, 0.9659258262890683122, 1.000000000000000000, 0.9659258262890683122, 1.000000000000000000, 0.9659258262890683122, 1.000000000000000000, 0.9659258262890683122, 1.000000000000000000, 0.9659258262890683122, 1.000000000000000000, 0.9659258262890683122, 1.000000000000000000, 0.9659258262890683122, 1.000000000000000000, 0.9659258262890683122, 1.000000000000000000, 0.9659258262890683122, 1.000000000000000000, 0.9659258262890683122, 1.000000000000000000, 0.9659258262890683122, 1.000000000000000000, 0.9659258262890683122, 1.000000000000000000, 0.9659258262890683122, 1.000000000000000000, 0.9659258262890683122, 1.000000000000000000, 0.9659258262890683122, 1.000000000000000000, 0.9659258262890683122, 1.000000000000000000, 0.9659258262890683122, 1.000000000000000000, 0.9659258262890683122, 1.000000000000000000, 0.9659258262890683122, 1.000000000000000000, 0.9659258262890683122, 1.000000000000000000, 0.9659258262890683122, 1.000000000000000000, 0.9659258262890683122, 1.000000000000000000, 0.9659258262890683122, 1.000000000000000000, 0.9659258262890683122, 1.000000000000000000, 0.9659258262890683122, 1.000000000000000000, 0.9659258262890683122, 1.000000000000000000, 0.9659258262890683122, 1.000000000000000000, 0.9659258262890683122, 1.000000000000000000, 0.9659258262890683122, 1.000000000000000000, 0.9659258262890683122, 1.000000000000000000, 0.9659258262890683122, 1.000000000000000000, 0.9659258262890683122, 1.000000000000000000, 0.9659258262890683122, 1.000000000000000000, 0.9659258262890683122, 1.000000000000000000, 0.9659258262890683122, 1.000000000000000000, 0.9659258262890683122, 1.000000000000000000, 0.9659258262890683122, 1.000000000000000000, 0.9659258262890683122, 1.000000000000000000, 0.9659258262890683122, 1.000000000000000000, 0.9659258262890683122, 1.000000000000000000, 0.9659258262890683122, 1.000000000000000000, 0.9659258262890683122, 1.000000000000000000, 0.9659258262890683122, 1.000000000000000000, 0.9659258262890683122, 1.000000000000000000, 0.9659258262890683122, 1.000000000000000000, 0.9659258262890683122, 1.000000000000000000, 0.9659258262890683122, 1.000000000000000000, 0.9659258262890683122, 1.000000000000000000, 0.9659258262890683122, 1.000000000000000000, 0.9659258262890683122, 1.000000000000000000, 0.9659258262890683122, 1.000000000000000000, 0.9659258262890683122, 1.000000000000000000, 0.9659258262890683122, 1.000000000000000000, 0.9659258262890683122, 1.000000000000000000, 0.9659258262890683122, 1.000000000000000000, 0.9659258262890683122, 1.000000000000000000, 0.9659258262890683122, 1.000000000000000000, 0.9659258262890683122, 1.000000000000000000, 0.9659258262890683122, 1.000000000000000000, 0.9659258262890683122, 1.000000000000000000, 0.9659258262890683122, 1.000000000000000000, 0.9659258262890683122, 1.000000000000000000, 0.9659258262890683122, 1.000000000000000000, 0.9659258262890683122, 1.000000000000000000, 0.9659258262890683122, 1.000000000000000000, 0.9659258262890683122, 1.000000000000000000, 0.9659258262890683122, 1.000000000000000000, 0.9659258262890683122, 1.000000000000000000, 0.9659258262890683122, 1.000000000000000000, 0.9659258262890683122, 1.000000000000000000),
 ( 0.3333333333333333703, 0.3219752754296894559, 0.3333333333333333703, 0.3219752754296894559, 0.3333333333333333703, 0.3219752754296894559, 0.3333333333333333703, 0.3219752754296894559, 0.3333333333333333703, 0.3219752754296894559, 0.3333333333333333703, 0.3219752754296894559, 0.3333333333333333703, 0.3219752754296894559, 0.3333333333333333703, 0.3219752754296894559, 0.3333333333333333703, 0.3219752754296894559, 0.3333333333333333703, 0.3219752754296894559, 0.3333333333333333703, 0.3219752754296894559, 0.3333333333333333703, 0.3219752754296894559, 0.3333333333333333703, 0.3219752754296894559, 0.3333333333333333703, 0.3219752754296894559, 0.3333333333333333703, 0.3219752754296894559, 0.3333333333333333703, 0.3219752754296894559, 0.3333333333333333703, 0.3219752754296894559, 0.3333333333333333703, 0.3219752754296894559, 0.3333333333333333703, 0.3219752754296894559, 0.3333333333333333703, 0.3219752754296894559, 0.3333333333333333703, 0.3219752754296894559, 0.3333333333333333703, 0.3219752754296894559, 0.3333333333333333703, 0.3219752754296894559, 0.3333333333333333703, 0.3219752754296894559, 0.3333333333333333703, 0.3219752754296894559, 0.3333333333333333703, 0.3219752754296894559, 0.3333333333333333703, 0.3219752754296894559, 0.3333333333333333703, 0.3219752754296894559, 0.3333333333333333703, 0.3219752754296894559, 0.3333333333333333703, 0.3219752754296894559, 0.3333333333333333703, 0.3219752754296894559, 0.3333333333333333703, 0.3219752754296894559, 0.3333333333333333703, 0.3219752754296894559, 0.3333333333333333703, 0.3219752754296894559, 0.3333333333333333703, 0.3219752754296894559, 0.3333333333333333703, 0.3219752754296894559, 0.3333333333333333703, 0.3219752754296894559, 0.3333333333333333703, 0.3219752754296894559, 0.3333333333333333703, 0.3219752754296894559, 0.3333333333333333703, 0.3219752754296894559, 0.3333333333333333703, 0.3219752754296894559, 0.3333333333333333703, 0.3219752754296894559, 0.3333333333333333703, 0.3219752754296894559, 0.3333333333333333703, 0.3219752754296894559, 0.3333333333333333703, 0.3219752754296894559, 0.3333333333333333703, 0.3219752754296894559, 0.3333333333333333703, 0.3219752754296894559, 0.3333333333333333703, 0.3219752754296894559, 0.3333333333333333703, 0.3219752754296894559, 0.3333333333333333703, 0.3219752754296894559, 0.3333333333333333703, 0.3219752754296894559, 0.3333333333333333703, 0.3219752754296894559, 0.3333333333333333703, 0.3219752754296894559, 0.3333333333333333703, 0.3219752754296894559, 0.3333333333333333703, 0.3219752754296894559, 0.3333333333333333703, 0.3219752754296894559, 0.3333333333333333703, 0.3219752754296894559, 0.3333333333333333703, 0.3219752754296894559, 0.3333333333333333703, 0.3219752754296894559, 0.3333333333333333703, 0.3219752754296894559, 0.3333333333333333703, 0.3219752754296894559, 0.3333333333333333703, 0.3219752754296894559, 0.3333333333333333703, 0.3219752754296894559, 0.3333333333333333703, 0.3219752754296894559, 0.3333333333333333703, 0.3219752754296894559, 0.3333333333333333703, 0.3219752754296894559, 0.3333333333333333703, 0.3219752754296894559, 0.3333333333333333703, 0.3219752754296894559, 0.3333333333333333703, 0.3219752754296894559, 0.3333333333333333703, 0.3219752754296894559, 0.3333333333333333703, 0.3219752754296894559, 0.3333333333333333703, 0.3219752754296894559, 0.3333333333333333703, 0.3219752754296894559, 0.3333333333333333703, 0.3219752754296894559, 0.3333333333333333703, 0.3219752754296894559, 0.3333333333333333703, 0.3219752754296894559, 0.3333333333333333703, 0.3219752754296894559, 0.3333333333333333703, 0.3219752754296894559, 0.3333333333333333703, 0.3219752754296894559, 0.3333333333333333703, 0.3219752754296894559, 0.3333333333333333703, 0.3219752754296894559, 0.3333333333333333703, 0.3219752754296894559, 0.3333333333333333703, 0.3219752754296894559, 0.3333333333333333703, 0.3219752754296894559, 0.3333333333333333703, 0.3219752754296894559, 0.3333333333333333703, 0.3219752754296894559, 0.3333333333333333703, 0.3219752754296894559, 0.3333333333333333703, 0.3219752754296894559, 0.3333333333333333703, 0.3219752754296894559, 0.3333333333333333703, 0.3219752754296894559, 0.3333333333333333703, 0.3219752754296894559, 0.3333333333333333703, 0.3219752754296894559, 0.3333333333333333703, 0.3219752754296894559, 0.3333333333333333703, 0.3219752754296894559, 0.3333333333333333703, 0.3219752754296894559, 0.3333333333333333703, 0.3219752754296894559, 0.3333333333333333703, 0.3219752754296894559, 0.3333333333333333703, 0.3219752754296894559, 0.3333333333333333703, 0.3219752754296894559, 0.3333333333333333703, 0.3219752754296894559, 0.3333333333333333703, 0.3219752754296894559, 0.3333333333333333703, 0.3219752754296894559, 0.3333333333333333703, 0.3219752754296894559, 0.3333333333333333703, 0.3219752754296894559, 0.3333333333333333703, 0.3219752754296894559, 0.3333333333333333703, 0.3219752754296894559, 0.3333333333333333703, 0.3219752754296894559, 0.3333333333333333703, 0.3219752754296894559, 0.3333333333333333703, 0.3219752754296894559, 0.3333333333333333703, 0.3219752754296894559, 0.3333333333333333703, 0.3219752754296894559, 0.3333333333333333703, 0.3219752754296894559, 0.3333333333333333703, 0.3219752754296894559, 0.3333333333333333703, 0.3219752754296894559, 0.3333333333333333703, 0.3219752754296894559, 0.3333333333333333703, 0.3219752754296894559, 0.3333333333333333703, 0.3219752754296894559, 0.3333333333333333703, 0.3219752754296894559, 0.3333333333333333703, 0.3219752754296894559, 0.3333333333333333703, 0.3219752754296894559, 0.3333333333333333703, 0.3219752754296894559, 0.3333333333333333703, 0.3219752754296894559, 0.3333333333333333703, 0.3219752754296894559, 0.3333333333333333703, 0.3219752754296894559, 0.3333333333333333703, 0.3219752754296894559, 0.3333333333333333703, 0.3219752754296894559, 0.3333333333333333703, 0.3219752754296894559, 0.3333333333333333703, 0.3219752754296894559, 0.3333333333333333703, 0.3219752754296894559, 0.3333333333333333703, 0.3219752754296894559, 0.3333333333333333703, 0.3219752754296894559, 0.3333333333333333703, 0.3219752754296894559, 0.3333333333333333703, 0.3219752754296894559, 0.3333333333333333703, 0.3219752754296894559, 0.3333333333333333703, 0.3219752754296894559, 0.3333333333333333703, 0.3219752754296894559, 0.3333333333333333703, 0.3219752754296894559, 0.3333333333333333703, 0.3219752754296894559, 0.3333333333333333703, 0.3219752754296894559, 0.3333333333333333703, 0.3219752754296894559, 0.3333333333333333703, 0.3219752754296894559, 0.3333333333333333703, 0.3219752754296894559, 0.3333333333333333703, 0.3219752754296894559, 0.3333333333333333703, 0.3219752754296894559, 0.3333333333333333703, 0.3219752754296894559, 0.3333333333333333703, 0.3219752754296894559, 0.3333333333333333703, 0.3219752754296894559, 0.3333333333333333703, 0.3219752754296894559, 0.3333333333333333703, 0.3219752754296894559, 0.3333333333333333703, 0.3219752754296894559, 0.3333333333333333703, 0.3219752754296894559, 0.3333333333333333703, 0.3219752754296894559, 0.3333333333333333703, 0.3219752754296894559, 0.3333333333333333703, 0.3219752754296894559, 0.3333333333333333703, 0.3219752754296894559, 0.3333333333333333703, 0.3219752754296894559, 0.3333333333333333703, 0.3219752754296894559, 0.3333333333333333703, 0.3219752754296894559, 0.3333333333333333703, 0.3219752754296894559, 0.3333333333333333703, 0.3219752754296894559, 0.3333333333333333703, 0.3219752754296894559, 0.3333333333333333703, 0.3219752754296894559, 0.3333333333333333703, 0.3219752754296894559, 0.3333333333333333703, 0.3219752754296894559, 0.3333333333333333703, 0.3219752754296894559, 0.3333333333333333703, 0.3219752754296894559, 0.3333333333333333703, 0.3219752754296894559, 0.3333333333333333703, 0.3219752754296894559, 0.3333333333333333703, 0.3219752754296894559, 0.3333333333333333703, 0.3219752754296894559, 0.3333333333333333703, 0.3219752754296894559, 0.3333333333333333703, 0.3219752754296894559, 0.3333333333333333703, 0.3219752754296894559, 0.3333333333333333703, 0.3219752754296894559, 0.3333333333333333703, 0.3219752754296894559, 0.3333333333333333703, 0.3219752754296894559, 0.3333333333333333703, 0.3219752754296894559, 0.3333333333333333703, 0.3219752754296894559, 0.3333333333333333703, 0.3219752754296894559, 0.3333333333333333703, 0.3219752754296894559, 0.3333333333333333703, 0.3219752754296894559, 0.3333333333333333703, 0.3219752754296894559, 0.3333333333333333703, 0.3219752754296894559, 0.3333333333333333703, 0.3219752754296894559, 0.3333333333333333703, 0.3219752754296894559, 0.3333333333333333703, 0.3219752754296894559, 0.3333333333333333703, 0.3219752754296894559, 0.3333333333333333703, 0.3219752754296894559, 0.3333333333333333703, 0.3219752754296894559, 0.3333333333333333703, 0.3219752754296894559, 0.3333333333333333703, 0.3219752754296894559, 0.3333333333333333703, 0.3219752754296894559, 0.3333333333333333703, 0.3219752754296894559, 0.3333333333333333703, 0.3219752754296894559, 0.3333333333333333703, 0.3219752754296894559, 0.3333333333333333703, 0.3219752754296894559, 0.3333333333333333703, 0.3219752754296894559, 0.3333333333333333703, 0.3219752754296894559, 0.3333333333333333703, 0.3219752754296894559, 0.3333333333333333703, 0.3219752754296894559, 0.3333333333333333703, 0.3219752754296894559, 0.3333333333333333703, 0.3219752754296894559, 0.3333333333333333703, 0.3219752754296894559, 0.3333333333333333703, 0.3219752754296894559, 0.3333333333333333703, 0.3219752754296894559, 0.3333333333333333703, 0.3219752754296894559, 0.3333333333333333703, 0.3219752754296894559, 0.3333333333333333703, 0.3219752754296894559, 0.3333333333333333703, 0.3219752754296894559, 0.3333333333333333703, 0.3219752754296894559, 0.3333333333333333703, 0.3219752754296894559, 0.3333333333333333703, 0.3219752754296894559, 0.3333333333333333703, 0.3219752754296894559, 0.3333333333333333703, 0.3219752754296894559, 0.3333333333333333703, 0.3219752754296894559, 0.3333333333333333703, 0.3219752754296894559, 0.3333333333333333703, 0.3219752754296894559, 0.3333333333333333703, 0.3219752754296894559, 0.3333333333333333703, 0.3219752754296894559, 0.3333333333333333703, 0.3219752754296894559, 0.3333333333333333703, 0.3219752754296894559, 0.3333333333333333703, 0.3219752754296894559, 0.3333333333333333703, 0.3219752754296894559, 0.3333333333333333703, 0.3219752754296894559, 0.3333333333333333703, 0.3219752754296894559, 0.3333333333333333703, 0.3219752754296894559, 0.3333333333333333703, 0.3219752754296894559, 0.3333333333333333703, 0.3219752754296894559, 0.3333333333333333703),
 ( 0.3333333333333333703, 0.3219752754296894559, 0.3333333333333333703, 0.3219752754296894559, 0.3333333333333333703, 0.3219752754296894559, 0.3333333333333333703, 0.3219752754296894559, 0.3333333333333333703, 0.3219752754296894559, 0.3333333333333333703, 0.3219752754296894559, 0.3333333333333333703, 0.3219752754296894559, 0.3333333333333333703, 0.3219752754296894559, 0.3333333333333333703, 0.3219752754296894559, 0.3333333333333333703, 0.3219752754296894559, 0.3333333333333333703, 0.3219752754296894559, 0.3333333333333333703, 0.3219752754296894559, 0.3333333333333333703, 0.3219752754296894559, 0.3333333333333333703, 0.3219752754296894559, 0.3333333333333333703, 0.3219752754296894559, 0.3333333333333333703, 0.3219752754296894559, 0.3333333333333333703, 0.3219752754296894559, 0.3333333333333333703, 0.3219752754296894559, 0.3333333333333333703, 0.3219752754296894559, 0.3333333333333333703, 0.3219752754296894559, 0.3333333333333333703, 0.3219752754296894559, 0.3333333333333333703, 0.3219752754296894559, 0.3333333333333333703, 0.3219752754296894559, 0.3333333333333333703, 0.3219752754296894559, 0.3333333333333333703, 0.3219752754296894559, 0.3333333333333333703, 0.3219752754296894559, 0.3333333333333333703, 0.3219752754296894559, 0.3333333333333333703, 0.3219752754296894559, 0.3333333333333333703, 0.3219752754296894559, 0.3333333333333333703, 0.3219752754296894559, 0.3333333333333333703, 0.3219752754296894559, 0.3333333333333333703, 0.3219752754296894559, 0.3333333333333333703, 0.3219752754296894559, 0.3333333333333333703, 0.3219752754296894559, 0.3333333333333333703, 0.3219752754296894559, 0.3333333333333333703, 0.3219752754296894559, 0.3333333333333333703, 0.3219752754296894559, 0.3333333333333333703, 0.3219752754296894559, 0.3333333333333333703, 0.3219752754296894559, 0.3333333333333333703, 0.3219752754296894559, 0.3333333333333333703, 0.3219752754296894559, 0.3333333333333333703, 0.3219752754296894559, 0.3333333333333333703, 0.3219752754296894559, 0.3333333333333333703, 0.3219752754296894559, 0.3333333333333333703, 0.3219752754296894559, 0.3333333333333333703, 0.3219752754296894559, 0.3333333333333333703, 0.3219752754296894559, 0.3333333333333333703, 0.3219752754296894559, 0.3333333333333333703, 0.3219752754296894559, 0.3333333333333333703, 0.3219752754296894559, 0.3333333333333333703, 0.3219752754296894559, 0.3333333333333333703, 0.3219752754296894559, 0.3333333333333333703, 0.3219752754296894559, 0.3333333333333333703, 0.3219752754296894559, 0.3333333333333333703, 0.3219752754296894559, 0.3333333333333333703, 0.3219752754296894559, 0.3333333333333333703, 0.3219752754296894559, 0.3333333333333333703, 0.3219752754296894559, 0.3333333333333333703, 0.3219752754296894559, 0.3333333333333333703, 0.3219752754296894559, 0.3333333333333333703, 0.3219752754296894559, 0.3333333333333333703, 0.3219752754296894559, 0.3333333333333333703, 0.3219752754296894559, 0.3333333333333333703, 0.3219752754296894559, 0.3333333333333333703, 0.3219752754296894559, 0.3333333333333333703, 0.3219752754296894559, 0.3333333333333333703, 0.3219752754296894559, 0.3333333333333333703, 0.3219752754296894559, 0.3333333333333333703, 0.3219752754296894559, 0.3333333333333333703, 0.3219752754296894559, 0.3333333333333333703, 0.3219752754296894559, 0.3333333333333333703, 0.3219752754296894559, 0.3333333333333333703, 0.3219752754296894559, 0.3333333333333333703, 0.3219752754296894559, 0.3333333333333333703, 0.3219752754296894559, 0.3333333333333333703, 0.3219752754296894559, 0.3333333333333333703, 0.3219752754296894559, 0.3333333333333333703, 0.3219752754296894559, 0.3333333333333333703, 0.3219752754296894559, 0.3333333333333333703, 0.3219752754296894559, 0.3333333333333333703, 0.3219752754296894559, 0.3333333333333333703, 0.3219752754296894559, 0.3333333333333333703, 0.3219752754296894559, 0.3333333333333333703, 0.3219752754296894559, 0.3333333333333333703, 0.3219752754296894559, 0.3333333333333333703, 0.3219752754296894559, 0.3333333333333333703, 0.3219752754296894559, 0.3333333333333333703, 0.3219752754296894559, 0.3333333333333333703, 0.3219752754296894559, 0.3333333333333333703, 0.3219752754296894559, 0.3333333333333333703, 0.3219752754296894559, 0.3333333333333333703, 0.3219752754296894559, 0.3333333333333333703, 0.3219752754296894559, 0.3333333333333333703, 0.3219752754296894559, 0.3333333333333333703, 0.3219752754296894559, 0.3333333333333333703, 0.3219752754296894559, 0.3333333333333333703, 0.3219752754296894559, 0.3333333333333333703, 0.3219752754296894559, 0.3333333333333333703, 0.3219752754296894559, 0.3333333333333333703, 0.3219752754296894559, 0.3333333333333333703, 0.3219752754296894559, 0.3333333333333333703, 0.3219752754296894559, 0.3333333333333333703, 0.3219752754296894559, 0.3333333333333333703, 0.3219752754296894559, 0.3333333333333333703, 0.3219752754296894559, 0.3333333333333333703, 0.3219752754296894559, 0.3333333333333333703, 0.3219752754296894559, 0.3333333333333333703, 0.3219752754296894559, 0.3333333333333333703, 0.3219752754296894559, 0.3333333333333333703, 0.3219752754296894559, 0.3333333333333333703, 0.3219752754296894559, 0.3333333333333333703, 0.3219752754296894559, 0.3333333333333333703, 0.3219752754296894559, 0.3333333333333333703, 0.3219752754296894559, 0.3333333333333333703, 0.3219752754296894559, 0.3333333333333333703, 0.3219752754296894559, 0.3333333333333333703, 0.3219752754296894559, 0.3333333333333333703, 0.3219752754296894559, 0.3333333333333333703, 0.3219752754296894559, 0.3333333333333333703, 0.3219752754296894559, 0.3333333333333333703, 0.3219752754296894559, 0.3333333333333333703, 0.3219752754296894559, 0.3333333333333333703, 0.3219752754296894559, 0.3333333333333333703, 0.3219752754296894559, 0.3333333333333333703, 0.3219752754296894559, 0.3333333333333333703, 0.3219752754296894559, 0.3333333333333333703, 0.3219752754296894559, 0.3333333333333333703, 0.3219752754296894559, 0.3333333333333333703, 0.3219752754296894559, 0.3333333333333333703, 0.3219752754296894559, 0.3333333333333333703, 0.3219752754296894559, 0.3333333333333333703, 0.3219752754296894559, 0.3333333333333333703, 0.3219752754296894559, 0.3333333333333333703, 0.3219752754296894559, 0.3333333333333333703, 0.3219752754296894559, 0.3333333333333333703, 0.3219752754296894559, 0.3333333333333333703, 0.3219752754296894559, 0.3333333333333333703, 0.3219752754296894559, 0.3333333333333333703, 0.3219752754296894559, 0.3333333333333333703, 0.3219752754296894559, 0.3333333333333333703, 0.3219752754296894559, 0.3333333333333333703, 0.3219752754296894559, 0.3333333333333333703, 0.3219752754296894559, 0.3333333333333333703, 0.3219752754296894559, 0.3333333333333333703, 0.3219752754296894559, 0.3333333333333333703, 0.3219752754296894559, 0.3333333333333333703, 0.3219752754296894559, 0.3333333333333333703, 0.3219752754296894559, 0.3333333333333333703, 0.3219752754296894559, 0.3333333333333333703, 0.3219752754296894559, 0.3333333333333333703, 0.3219752754296894559, 0.3333333333333333703, 0.3219752754296894559, 0.3333333333333333703, 0.3219752754296894559, 0.3333333333333333703, 0.3219752754296894559, 0.3333333333333333703, 0.3219752754296894559, 0.3333333333333333703, 0.3219752754296894559, 0.3333333333333333703, 0.3219752754296894559, 0.3333333333333333703, 0.3219752754296894559, 0.3333333333333333703, 0.3219752754296894559, 0.3333333333333333703, 0.3219752754296894559, 0.3333333333333333703, 0.3219752754296894559, 0.3333333333333333703, 0.3219752754296894559, 0.3333333333333333703, 0.3219752754296894559, 0.3333333333333333703, 0.3219752754296894559, 0.3333333333333333703, 0.3219752754296894559, 0.3333333333333333703, 0.3219752754296894559, 0.3333333333333333703, 0.3219752754296894559, 0.3333333333333333703, 0.3219752754296894559, 0.3333333333333333703, 0.3219752754296894559, 0.3333333333333333703, 0.3219752754296894559, 0.3333333333333333703, 0.3219752754296894559, 0.3333333333333333703, 0.3219752754296894559, 0.3333333333333333703, 0.3219752754296894559, 0.3333333333333333703, 0.3219752754296894559, 0.3333333333333333703, 0.3219752754296894559, 0.3333333333333333703, 0.3219752754296894559, 0.3333333333333333703, 0.3219752754296894559, 0.3333333333333333703, 0.3219752754296894559, 0.3333333333333333703, 0.3219752754296894559, 0.3333333333333333703, 0.3219752754296894559, 0.3333333333333333703, 0.3219752754296894559, 0.3333333333333333703, 0.3219752754296894559, 0.3333333333333333703, 0.3219752754296894559, 0.3333333333333333703, 0.3219752754296894559, 0.3333333333333333703, 0.3219752754296894559, 0.3333333333333333703, 0.3219752754296894559, 0.3333333333333333703, 0.3219752754296894559, 0.3333333333333333703, 0.3219752754296894559, 0.3333333333333333703, 0.3219752754296894559, 0.3333333333333333703, 0.3219752754296894559, 0.3333333333333333703, 0.3219752754296894559, 0.3333333333333333703, 0.3219752754296894559, 0.3333333333333333703, 0.3219752754296894559, 0.3333333333333333703, 0.3219752754296894559, 0.3333333333333333703, 0.3219752754296894559, 0.3333333333333333703, 0.3219752754296894559, 0.3333333333333333703, 0.3219752754296894559, 0.3333333333333333703, 0.3219752754296894559, 0.3333333333333333703, 0.3219752754296894559, 0.3333333333333333703, 0.3219752754296894559, 0.3333333333333333703, 0.3219752754296894559, 0.3333333333333333703, 0.3219752754296894559, 0.3333333333333333703, 0.3219752754296894559, 0.3333333333333333703, 0.3219752754296894559, 0.3333333333333333703, 0.3219752754296894559, 0.3333333333333333703, 0.3219752754296894559, 0.3333333333333333703, 0.3219752754296894559, 0.3333333333333333703, 0.3219752754296894559, 0.3333333333333333703, 0.3219752754296894559, 0.3333333333333333703, 0.3219752754296894559, 0.3333333333333333703, 0.3219752754296894559, 0.3333333333333333703, 0.3219752754296894559, 0.3333333333333333703, 0.3219752754296894559, 0.3333333333333333703, 0.3219752754296894559, 0.3333333333333333703, 0.3219752754296894559, 0.3333333333333333703, 0.3219752754296894559, 0.3333333333333333703, 0.3219752754296894559, 0.3333333333333333703, 0.3219752754296894559, 0.3333333333333333703, 0.3219752754296894559, 0.3333333333333333703, 0.3219752754296894559, 0.3333333333333333703, 0.3219752754296894559, 0.3333333333333333703, 0.3219752754296894559, 0.3333333333333333703, 0.3219752754296894559, 0.3333333333333333703, 0.3219752754296894559, 0.3333333333333333703, 0.3219752754296894559, 0.3333333333333333703, 0.3219752754296894559, 0.3333333333333333703, 0.3219752754296894559, 0.3333333333333333703, 0.3219752754296894559, 0.3333333333333333703),
 ( 1.000000000000000000, 0.9659258262890683122, 1.000000000000000000, 0.9659258262890683122, 1.000000000000000000, 0.9659258262890683122, 1.000000000000000000, 0.9659258262890683122, 1.000000000000000000, 0.9659258262890683122, 1.000000000000000000, 0.9659258262890683122, 1.000000000000000000, 0.9659258262890683122, 1.000000000000000000, 0.9659258262890683122, 1.000000000000000000, 0.9659258262890683122, 1.000000000000000000, 0.9659258262890683122, 1.000000000000000000, 0.9659258262890683122, 1.000000000000000000, 0.9659258262890683122, 1.000000000000000000, 0.9659258262890683122, 1.000000000000000000, 0.9659258262890683122, 1.000000000000000000, 0.9659258262890683122, 1.000000000000000000, 0.9659258262890683122, 1.000000000000000000, 0.9659258262890683122, 1.000000000000000000, 0.9659258262890683122, 1.000000000000000000, 0.9659258262890683122, 1.000000000000000000, 0.9659258262890683122, 1.000000000000000000, 0.9659258262890683122, 1.000000000000000000, 0.9659258262890683122, 1.000000000000000000, 0.9659258262890683122, 1.000000000000000000, 0.9659258262890683122, 1.000000000000000000, 0.9659258262890683122, 1.000000000000000000, 0.9659258262890683122, 1.000000000000000000, 0.9659258262890683122, 1.000000000000000000, 0.9659258262890683122, 1.000000000000000000, 0.9659258262890683122, 1.000000000000000000, 0.9659258262890683122, 1.000000000000000000, 0.9659258262890683122, 1.000000000000000000, 0.9659258262890683122, 1.000000000000000000, 0.9659258262890683122, 1.000000000000000000, 0.9659258262890683122, 1.000000000000000000, 0.9659258262890683122, 1.000000000000000000, 0.9659258262890683122, 1.000000000000000000, 0.9659258262890683122, 1.000000000000000000, 0.9659258262890683122, 1.000000000000000000, 0.9659258262890683122, 1.000000000000000000, 0.9659258262890683122, 1.000000000000000000, 0.9659258262890683122, 1.000000000000000000, 0.9659258262890683122, 1.000000000000000000, 0.9659258262890683122, 1.000000000000000000, 0.9659258262890683122, 1.000000000000000000, 0.9659258262890683122, 1.000000000000000000, 0.9659258262890683122, 1.000000000000000000, 0.9659258262890683122, 1.000000000000000000, 0.9659258262890683122, 1.000000000000000000, 0.9659258262890683122, 1.000000000000000000, 0.9659258262890683122, 1.000000000000000000, 0.9659258262890683122, 1.000000000000000000, 0.9659258262890683122, 1.000000000000000000, 0.9659258262890683122, 1.000000000000000000, 0.9659258262890683122, 1.000000000000000000, 0.9659258262890683122, 1.000000000000000000, 0.9659258262890683122, 1.000000000000000000, 0.9659258262890683122, 1.000000000000000000, 0.9659258262890683122, 1.000000000000000000, 0.9659258262890683122, 1.000000000000000000, 0.9659258262890683122, 1.000000000000000000, 0.9659258262890683122, 1.000000000000000000, 0.9659258262890683122, 1.000000000000000000, 0.9659258262890683122, 1.000000000000000000, 0.9659258262890683122, 1.000000000000000000, 0.9659258262890683122, 1.000000000000000000, 0.9659258262890683122, 1.000000000000000000, 0.9659258262890683122, 1.000000000000000000, 0.9659258262890683122, 1.000000000000000000, 0.9659258262890683122, 1.000000000000000000, 0.9659258262890683122, 1.000000000000000000, 0.9659258262890683122, 1.000000000000000000, 0.9659258262890683122, 1.000000000000000000, 0.9659258262890683122, 1.000000000000000000, 0.9659258262890683122, 1.000000000000000000, 0.9659258262890683122, 1.000000000000000000, 0.9659258262890683122, 1.000000000000000000, 0.9659258262890683122, 1.000000000000000000, 0.9659258262890683122, 1.000000000000000000, 0.9659258262890683122, 1.000000000000000000, 0.9659258262890683122, 1.000000000000000000, 0.9659258262890683122, 1.000000000000000000, 0.9659258262890683122, 1.000000000000000000, 0.9659258262890683122, 1.000000000000000000, 0.9659258262890683122, 1.000000000000000000, 0.9659258262890683122, 1.000000000000000000, 0.9659258262890683122, 1.000000000000000000, 0.9659258262890683122, 1.000000000000000000, 0.9659258262890683122, 1.000000000000000000, 0.9659258262890683122, 1.000000000000000000, 0.9659258262890683122, 1.000000000000000000, 0.9659258262890683122, 1.000000000000000000, 0.9659258262890683122, 1.000000000000000000, 0.9659258262890683122, 1.000000000000000000, 0.9659258262890683122, 1.000000000000000000, 0.9659258262890683122, 1.000000000000000000, 0.9659258262890683122, 1.000000000000000000, 0.9659258262890683122, 1.000000000000000000, 0.9659258262890683122, 1.000000000000000000, 0.9659258262890683122, 1.000000000000000000, 0.9659258262890683122, 1.000000000000000000, 0.9659258262890683122, 1.000000000000000000, 0.9659258262890683122, 1.000000000000000000, 0.9659258262890683122, 1.000000000000000000, 0.9659258262890683122, 1.000000000000000000, 0.9659258262890683122, 1.000000000000000000, 0.9659258262890683122, 1.000000000000000000, 0.9659258262890683122, 1.000000000000000000, 0.9659258262890683122, 1.000000000000000000, 0.9659258262890683122, 1.000000000000000000, 0.9659258262890683122, 1.000000000000000000, 0.9659258262890683122, 1.000000000000000000, 0.9659258262890683122, 1.000000000000000000, 0.9659258262890683122, 1.000000000000000000, 0.9659258262890683122, 1.000000000000000000, 0.9659258262890683122, 1.000000000000000000, 0.9659258262890683122, 1.000000000000000000, 0.9659258262890683122, 1.000000000000000000, 0.9659258262890683122, 1.000000000000000000, 0.9659258262890683122, 1.000000000000000000, 0.9659258262890683122, 1.000000000000000000, 0.9659258262890683122, 1.000000000000000000, 0.9659258262890683122, 1.000000000000000000, 0.9659258262890683122, 1.000000000000000000, 0.9659258262890683122, 1.000000000000000000, 0.9659258262890683122, 1.000000000000000000, 0.9659258262890683122, 1.000000000000000000, 0.9659258262890683122, 1.000000000000000000, 0.9659258262890683122, 1.000000000000000000, 0.9659258262890683122, 1.000000000000000000, 0.9659258262890683122, 1.000000000000000000, 0.9659258262890683122, 1.000000000000000000, 0.9659258262890683122, 1.000000000000000000, 0.9659258262890683122, 1.000000000000000000, 0.9659258262890683122, 1.000000000000000000, 0.9659258262890683122, 1.000000000000000000, 0.9659258262890683122, 1.000000000000000000, 0.9659258262890683122, 1.000000000000000000, 0.9659258262890683122, 1.000000000000000000, 0.9659258262890683122, 1.000000000000000000, 0.9659258262890683122, 1.000000000000000000, 0.9659258262890683122, 1.000000000000000000, 0.9659258262890683122, 1.000000000000000000, 0.9659258262890683122, 1.000000000000000000, 0.9659258262890683122, 1.000000000000000000, 0.9659258262890683122, 1.000000000000000000, 0.9659258262890683122, 1.000000000000000000, 0.9659258262890683122, 1.000000000000000000, 0.9659258262890683122, 1.000000000000000000, 0.9659258262890683122, 1.000000000000000000, 0.9659258262890683122, 1.000000000000000000, 0.9659258262890683122, 1.000000000000000000, 0.9659258262890683122, 1.000000000000000000, 0.9659258262890683122, 1.000000000000000000, 0.9659258262890683122, 1.000000000000000000, 0.9659258262890683122, 1.000000000000000000, 0.9659258262890683122, 1.000000000000000000, 0.9659258262890683122, 1.000000000000000000, 0.9659258262890683122, 1.000000000000000000, 0.9659258262890683122, 1.000000000000000000, 0.9659258262890683122, 1.000000000000000000, 0.9659258262890683122, 1.000000000000000000, 0.9659258262890683122, 1.000000000000000000, 0.9659258262890683122, 1.000000000000000000, 0.9659258262890683122, 1.000000000000000000, 0.9659258262890683122, 1.000000000000000000, 0.9659258262890683122, 1.000000000000000000, 0.9659258262890683122, 1.000000000000000000, 0.9659258262890683122, 1.000000000000000000, 0.9659258262890683122, 1.000000000000000000, 0.9659258262890683122, 1.000000000000000000, 0.9659258262890683122, 1.000000000000000000, 0.9659258262890683122, 1.000000000000000000, 0.9659258262890683122, 1.000000000000000000, 0.9659258262890683122, 1.000000000000000000, 0.9659258262890683122, 1.000000000000000000, 0.9659258262890683122, 1.000000000000000000, 0.9659258262890683122, 1.000000000000000000, 0.9659258262890683122, 1.000000000000000000, 0.9659258262890683122, 1.000000000000000000, 0.9659258262890683122, 1.000000000000000000, 0.9659258262890683122, 1.000000000000000000, 0.9659258262890683122, 1.000000000000000000, 0.9659258262890683122, 1.000000000000000000, 0.9659258262890683122, 1.000000000000000000, 0.9659258262890683122, 1.000000000000000000, 0.9659258262890683122, 1.000000000000000000, 0.9659258262890683122, 1.000000000000000000, 0.9659258262890683122, 1.000000000000000000, 0.9659258262890683122, 1.000000000000000000, 0.9659258262890683122, 1.000000000000000000, 0.9659258262890683122, 1.000000000000000000, 0.9659258262890683122, 1.000000000000000000, 0.9659258262890683122, 1.000000000000000000, 0.9659258262890683122, 1.000000000000000000, 0.9659258262890683122, 1.000000000000000000, 0.9659258262890683122, 1.000000000000000000, 0.9659258262890683122, 1.000000000000000000, 0.9659258262890683122, 1.000000000000000000, 0.9659258262890683122, 1.000000000000000000, 0.9659258262890683122, 1.000000000000000000, 0.9659258262890683122, 1.000000000000000000, 0.9659258262890683122, 1.000000000000000000, 0.9659258262890683122, 1.000000000000000000, 0.9659258262890683122, 1.000000000000000000, 0.9659258262890683122, 1.000000000000000000, 0.9659258262890683122, 1.000000000000000000, 0.9659258262890683122, 1.000000000000000000, 0.9659258262890683122, 1.000000000000000000, 0.9659258262890683122, 1.000000000000000000, 0.9659258262890683122, 1.000000000000000000, 0.9659258262890683122, 1.000000000000000000, 0.9659258262890683122, 1.000000000000000000, 0.9659258262890683122, 1.000000000000000000, 0.9659258262890683122, 1.000000000000000000, 0.9659258262890683122, 1.000000000000000000, 0.9659258262890683122, 1.000000000000000000, 0.9659258262890683122, 1.000000000000000000, 0.9659258262890683122, 1.000000000000000000, 0.9659258262890683122, 1.000000000000000000, 0.9659258262890683122, 1.000000000000000000, 0.9659258262890683122, 1.000000000000000000, 0.9659258262890683122, 1.000000000000000000, 0.9659258262890683122, 1.000000000000000000, 0.9659258262890683122, 1.000000000000000000, 0.9659258262890683122, 1.000000000000000000, 0.9659258262890683122, 1.000000000000000000, 0.9659258262890683122, 1.000000000000000000, 0.9659258262890683122, 1.000000000000000000),
 ( 0.3333333333333333703, 0.3219752754296894559, 0.3333333333333333703, 0.3219752754296894559, 0.3333333333333333703, 0.3219752754296894559, 0.3333333333333333703, 0.3219752754296894559, 0.3333333333333333703, 0.3219752754296894559, 0.3333333333333333703, 0.3219752754296894559, 0.3333333333333333703, 0.3219752754296894559, 0.3333333333333333703, 0.3219752754296894559, 0.3333333333333333703, 0.3219752754296894559, 0.3333333333333333703, 0.3219752754296894559, 0.3333333333333333703, 0.3219752754296894559, 0.3333333333333333703, 0.3219752754296894559, 0.3333333333333333703, 0.3219752754296894559, 0.3333333333333333703, 0.3219752754296894559, 0.3333333333333333703, 0.3219752754296894559, 0.3333333333333333703, 0.3219752754296894559, 0.3333333333333333703, 0.3219752754296894559, 0.3333333333333333703, 0.3219752754296894559, 0.3333333333333333703, 0.3219752754296894559, 0.3333333333333333703, 0.3219752754296894559, 0.3333333333333333703, 0.3219752754296894559, 0.3333333333333333703, 0.3219752754296894559, 0.3333333333333333703, 0.3219752754296894559, 0.3333333333333333703, 0.3219752754296894559, 0.3333333333333333703, 0.3219752754296894559, 0.3333333333333333703, 0.3219752754296894559, 0.3333333333333333703, 0.3219752754296894559, 0.3333333333333333703, 0.3219752754296894559, 0.3333333333333333703, 0.3219752754296894559, 0.3333333333333333703, 0.3219752754296894559, 0.3333333333333333703, 0.3219752754296894559, 0.3333333333333333703, 0.3219752754296894559, 0.3333333333333333703, 0.3219752754296894559, 0.3333333333333333703, 0.3219752754296894559, 0.3333333333333333703, 0.3219752754296894559, 0.3333333333333333703, 0.3219752754296894559, 0.3333333333333333703, 0.3219752754296894559, 0.3333333333333333703, 0.3219752754296894559, 0.3333333333333333703, 0.3219752754296894559, 0.3333333333333333703, 0.3219752754296894559, 0.3333333333333333703, 0.3219752754296894559, 0.3333333333333333703, 0.3219752754296894559, 0.3333333333333333703, 0.3219752754296894559, 0.3333333333333333703, 0.3219752754296894559, 0.3333333333333333703, 0.3219752754296894559, 0.3333333333333333703, 0.3219752754296894559, 0.3333333333333333703, 0.3219752754296894559, 0.3333333333333333703, 0.3219752754296894559, 0.3333333333333333703, 0.3219752754296894559, 0.3333333333333333703, 0.3219752754296894559, 0.3333333333333333703, 0.3219752754296894559, 0.3333333333333333703, 0.3219752754296894559, 0.3333333333333333703, 0.3219752754296894559, 0.3333333333333333703, 0.3219752754296894559, 0.3333333333333333703, 0.3219752754296894559, 0.3333333333333333703, 0.3219752754296894559, 0.3333333333333333703, 0.3219752754296894559, 0.3333333333333333703, 0.3219752754296894559, 0.3333333333333333703, 0.3219752754296894559, 0.3333333333333333703, 0.3219752754296894559, 0.3333333333333333703, 0.3219752754296894559, 0.3333333333333333703, 0.3219752754296894559, 0.3333333333333333703, 0.3219752754296894559, 0.3333333333333333703, 0.3219752754296894559, 0.3333333333333333703, 0.3219752754296894559, 0.3333333333333333703, 0.3219752754296894559, 0.3333333333333333703, 0.3219752754296894559, 0.3333333333333333703, 0.3219752754296894559, 0.3333333333333333703, 0.3219752754296894559, 0.3333333333333333703, 0.3219752754296894559, 0.3333333333333333703, 0.3219752754296894559, 0.3333333333333333703, 0.3219752754296894559, 0.3333333333333333703, 0.3219752754296894559, 0.3333333333333333703, 0.3219752754296894559, 0.3333333333333333703, 0.3219752754296894559, 0.3333333333333333703, 0.3219752754296894559, 0.3333333333333333703, 0.3219752754296894559, 0.3333333333333333703, 0.3219752754296894559, 0.3333333333333333703, 0.3219752754296894559, 0.3333333333333333703, 0.3219752754296894559, 0.3333333333333333703, 0.3219752754296894559, 0.3333333333333333703, 0.3219752754296894559, 0.3333333333333333703, 0.3219752754296894559, 0.3333333333333333703, 0.3219752754296894559, 0.3333333333333333703, 0.3219752754296894559, 0.3333333333333333703, 0.3219752754296894559, 0.3333333333333333703, 0.3219752754296894559, 0.3333333333333333703, 0.3219752754296894559, 0.3333333333333333703, 0.3219752754296894559, 0.3333333333333333703, 0.3219752754296894559, 0.3333333333333333703, 0.3219752754296894559, 0.3333333333333333703, 0.3219752754296894559, 0.3333333333333333703, 0.3219752754296894559, 0.3333333333333333703, 0.3219752754296894559, 0.3333333333333333703, 0.3219752754296894559, 0.3333333333333333703, 0.3219752754296894559, 0.3333333333333333703, 0.3219752754296894559, 0.3333333333333333703, 0.3219752754296894559, 0.3333333333333333703, 0.3219752754296894559, 0.3333333333333333703, 0.3219752754296894559, 0.3333333333333333703, 0.3219752754296894559, 0.3333333333333333703, 0.3219752754296894559, 0.3333333333333333703, 0.3219752754296894559, 0.3333333333333333703, 0.3219752754296894559, 0.3333333333333333703, 0.3219752754296894559, 0.3333333333333333703, 0.3219752754296894559, 0.3333333333333333703, 0.3219752754296894559, 0.3333333333333333703, 0.3219752754296894559, 0.3333333333333333703, 0.3219752754296894559, 0.3333333333333333703, 0.3219752754296894559, 0.3333333333333333703, 0.3219752754296894559, 0.3333333333333333703, 0.3219752754296894559, 0.3333333333333333703, 0.3219752754296894559, 0.3333333333333333703, 0.3219752754296894559, 0.3333333333333333703, 0.3219752754296894559, 0.3333333333333333703, 0.3219752754296894559, 0.3333333333333333703, 0.3219752754296894559, 0.3333333333333333703, 0.3219752754296894559, 0.3333333333333333703, 0.3219752754296894559, 0.3333333333333333703, 0.3219752754296894559, 0.3333333333333333703, 0.3219752754296894559, 0.3333333333333333703, 0.3219752754296894559, 0.3333333333333333703, 0.3219752754296894559, 0.3333333333333333703, 0.3219752754296894559, 0.3333333333333333703, 0.3219752754296894559, 0.3333333333333333703, 0.3219752754296894559, 0.3333333333333333703, 0.3219752754296894559, 0.3333333333333333703, 0.3219752754296894559, 0.3333333333333333703, 0.3219752754296894559, 0.3333333333333333703, 0.3219752754296894559, 0.3333333333333333703, 0.3219752754296894559, 0.3333333333333333703, 0.3219752754296894559, 0.3333333333333333703, 0.3219752754296894559, 0.3333333333333333703, 0.3219752754296894559, 0.3333333333333333703, 0.3219752754296894559, 0.3333333333333333703, 0.3219752754296894559, 0.3333333333333333703, 0.3219752754296894559, 0.3333333333333333703, 0.3219752754296894559, 0.3333333333333333703, 0.3219752754296894559, 0.3333333333333333703, 0.3219752754296894559, 0.3333333333333333703, 0.3219752754296894559, 0.3333333333333333703, 0.3219752754296894559, 0.3333333333333333703, 0.3219752754296894559, 0.3333333333333333703, 0.3219752754296894559, 0.3333333333333333703, 0.3219752754296894559, 0.3333333333333333703, 0.3219752754296894559, 0.3333333333333333703, 0.3219752754296894559, 0.3333333333333333703, 0.3219752754296894559, 0.3333333333333333703, 0.3219752754296894559, 0.3333333333333333703, 0.3219752754296894559, 0.3333333333333333703, 0.3219752754296894559, 0.3333333333333333703, 0.3219752754296894559, 0.3333333333333333703, 0.3219752754296894559, 0.3333333333333333703, 0.3219752754296894559, 0.3333333333333333703, 0.3219752754296894559, 0.3333333333333333703, 0.3219752754296894559, 0.3333333333333333703, 0.3219752754296894559, 0.3333333333333333703, 0.3219752754296894559, 0.3333333333333333703, 0.3219752754296894559, 0.3333333333333333703, 0.3219752754296894559, 0.3333333333333333703, 0.3219752754296894559, 0.3333333333333333703, 0.3219752754296894559, 0.3333333333333333703, 0.3219752754296894559, 0.3333333333333333703, 0.3219752754296894559, 0.3333333333333333703, 0.3219752754296894559, 0.3333333333333333703, 0.3219752754296894559, 0.3333333333333333703, 0.3219752754296894559, 0.3333333333333333703, 0.3219752754296894559, 0.3333333333333333703, 0.3219752754296894559, 0.3333333333333333703, 0.3219752754296894559, 0.3333333333333333703, 0.3219752754296894559, 0.3333333333333333703, 0.3219752754296894559, 0.3333333333333333703, 0.3219752754296894559, 0.3333333333333333703, 0.3219752754296894559, 0.3333333333333333703, 0.3219752754296894559, 0.3333333333333333703, 0.3219752754296894559, 0.3333333333333333703, 0.3219752754296894559, 0.3333333333333333703, 0.3219752754296894559, 0.3333333333333333703, 0.3219752754296894559, 0.3333333333333333703, 0.3219752754296894559, 0.3333333333333333703, 0.3219752754296894559, 0.3333333333333333703, 0.3219752754296894559, 0.3333333333333333703, 0.3219752754296894559, 0.3333333333333333703, 0.3219752754296894559, 0.3333333333333333703, 0.3219752754296894559, 0.3333333333333333703, 0.3219752754296894559, 0.3333333333333333703, 0.3219752754296894559, 0.3333333333333333703, 0.3219752754296894559, 0.3333333333333333703, 0.3219752754296894559, 0.3333333333333333703, 0.3219752754296894559, 0.3333333333333333703, 0.3219752754296894559, 0.3333333333333333703, 0.3219752754296894559, 0.3333333333333333703, 0.3219752754296894559, 0.3333333333333333703, 0.3219752754296894559, 0.3333333333333333703, 0.3219752754296894559, 0.3333333333333333703, 0.3219752754296894559, 0.3333333333333333703, 0.3219752754296894559, 0.3333333333333333703, 0.3219752754296894559, 0.3333333333333333703, 0.3219752754296894559, 0.3333333333333333703, 0.3219752754296894559, 0.3333333333333333703, 0.3219752754296894559, 0.3333333333333333703, 0.3219752754296894559, 0.3333333333333333703, 0.3219752754296894559, 0.3333333333333333703, 0.3219752754296894559, 0.3333333333333333703, 0.3219752754296894559, 0.3333333333333333703, 0.3219752754296894559, 0.3333333333333333703, 0.3219752754296894559, 0.3333333333333333703, 0.3219752754296894559, 0.3333333333333333703, 0.3219752754296894559, 0.3333333333333333703, 0.3219752754296894559, 0.3333333333333333703, 0.3219752754296894559, 0.3333333333333333703, 0.3219752754296894559, 0.3333333333333333703, 0.3219752754296894559, 0.3333333333333333703, 0.3219752754296894559, 0.3333333333333333703, 0.3219752754296894559, 0.3333333333333333703, 0.3219752754296894559, 0.3333333333333333703, 0.3219752754296894559, 0.3333333333333333703, 0.3219752754296894559, 0.3333333333333333703, 0.3219752754296894559, 0.3333333333333333703, 0.3219752754296894559, 0.3333333333333333703, 0.3219752754296894559, 0.3333333333333333703, 0.3219752754296894559, 0.3333333333333333703, 0.3219752754296894559, 0.3333333333333333703, 0.3219752754296894559, 0.3333333333333333703, 0.3219752754296894559, 0.3333333333333333703, 0.3219752754296894559, 0.3333333333333333703, 0.3219752754296894559, 0.3333333333333333703, 0.3219752754296894559, 0.3333333333333333703),
 ( 0.3333333333333333703, 0.3219752754296894559, 0.3333333333333333703, 0.3219752754296894559, 0.3333333333333333703, 0.3219752754296894559, 0.3333333333333333703, 0.3219752754296894559, 0.3333333333333333703, 0.3219752754296894559, 0.3333333333333333703, 0.3219752754296894559, 0.3333333333333333703, 0.3219752754296894559, 0.3333333333333333703, 0.3219752754296894559, 0.3333333333333333703, 0.3219752754296894559, 0.3333333333333333703, 0.3219752754296894559, 0.3333333333333333703, 0.3219752754296894559, 0.3333333333333333703, 0.3219752754296894559, 0.3333333333333333703, 0.3219752754296894559, 0.3333333333333333703, 0.3219752754296894559, 0.3333333333333333703, 0.3219752754296894559, 0.3333333333333333703, 0.3219752754296894559, 0.3333333333333333703, 0.3219752754296894559, 0.3333333333333333703, 0.3219752754296894559, 0.3333333333333333703, 0.3219752754296894559, 0.3333333333333333703, 0.3219752754296894559, 0.3333333333333333703, 0.3219752754296894559, 0.3333333333333333703, 0.3219752754296894559, 0.3333333333333333703, 0.3219752754296894559, 0.3333333333333333703, 0.3219752754296894559, 0.3333333333333333703, 0.3219752754296894559, 0.3333333333333333703, 0.3219752754296894559, 0.3333333333333333703, 0.3219752754296894559, 0.3333333333333333703, 0.3219752754296894559, 0.3333333333333333703, 0.3219752754296894559, 0.3333333333333333703, 0.3219752754296894559, 0.3333333333333333703, 0.3219752754296894559, 0.3333333333333333703, 0.3219752754296894559, 0.3333333333333333703, 0.3219752754296894559, 0.3333333333333333703, 0.3219752754296894559, 0.3333333333333333703, 0.3219752754296894559, 0.3333333333333333703, 0.3219752754296894559, 0.3333333333333333703, 0.3219752754296894559, 0.3333333333333333703, 0.3219752754296894559, 0.3333333333333333703, 0.3219752754296894559, 0.3333333333333333703, 0.3219752754296894559, 0.3333333333333333703, 0.3219752754296894559, 0.3333333333333333703, 0.3219752754296894559, 0.3333333333333333703, 0.3219752754296894559, 0.3333333333333333703, 0.3219752754296894559, 0.3333333333333333703, 0.3219752754296894559, 0.3333333333333333703, 0.3219752754296894559, 0.3333333333333333703, 0.3219752754296894559, 0.3333333333333333703, 0.3219752754296894559, 0.3333333333333333703, 0.3219752754296894559, 0.3333333333333333703, 0.3219752754296894559, 0.3333333333333333703, 0.3219752754296894559, 0.3333333333333333703, 0.3219752754296894559, 0.3333333333333333703, 0.3219752754296894559, 0.3333333333333333703, 0.3219752754296894559, 0.3333333333333333703, 0.3219752754296894559, 0.3333333333333333703, 0.3219752754296894559, 0.3333333333333333703, 0.3219752754296894559, 0.3333333333333333703, 0.3219752754296894559, 0.3333333333333333703, 0.3219752754296894559, 0.3333333333333333703, 0.3219752754296894559, 0.3333333333333333703, 0.3219752754296894559, 0.3333333333333333703, 0.3219752754296894559, 0.3333333333333333703, 0.3219752754296894559, 0.3333333333333333703, 0.3219752754296894559, 0.3333333333333333703, 0.3219752754296894559, 0.3333333333333333703, 0.3219752754296894559, 0.3333333333333333703, 0.3219752754296894559, 0.3333333333333333703, 0.3219752754296894559, 0.3333333333333333703, 0.3219752754296894559, 0.3333333333333333703, 0.3219752754296894559, 0.3333333333333333703, 0.3219752754296894559, 0.3333333333333333703, 0.3219752754296894559, 0.3333333333333333703, 0.3219752754296894559, 0.3333333333333333703, 0.3219752754296894559, 0.3333333333333333703, 0.3219752754296894559, 0.3333333333333333703, 0.3219752754296894559, 0.3333333333333333703, 0.3219752754296894559, 0.3333333333333333703, 0.3219752754296894559, 0.3333333333333333703, 0.3219752754296894559, 0.3333333333333333703, 0.3219752754296894559, 0.3333333333333333703, 0.3219752754296894559, 0.3333333333333333703, 0.3219752754296894559, 0.3333333333333333703, 0.3219752754296894559, 0.3333333333333333703, 0.3219752754296894559, 0.3333333333333333703, 0.3219752754296894559, 0.3333333333333333703, 0.3219752754296894559, 0.3333333333333333703, 0.3219752754296894559, 0.3333333333333333703, 0.3219752754296894559, 0.3333333333333333703, 0.3219752754296894559, 0.3333333333333333703, 0.3219752754296894559, 0.3333333333333333703, 0.3219752754296894559, 0.3333333333333333703, 0.3219752754296894559, 0.3333333333333333703, 0.3219752754296894559, 0.3333333333333333703, 0.3219752754296894559, 0.3333333333333333703, 0.3219752754296894559, 0.3333333333333333703, 0.3219752754296894559, 0.3333333333333333703, 0.3219752754296894559, 0.3333333333333333703, 0.3219752754296894559, 0.3333333333333333703, 0.3219752754296894559, 0.3333333333333333703, 0.3219752754296894559, 0.3333333333333333703, 0.3219752754296894559, 0.3333333333333333703, 0.3219752754296894559, 0.3333333333333333703, 0.3219752754296894559, 0.3333333333333333703, 0.3219752754296894559, 0.3333333333333333703, 0.3219752754296894559, 0.3333333333333333703, 0.3219752754296894559, 0.3333333333333333703, 0.3219752754296894559, 0.3333333333333333703, 0.3219752754296894559, 0.3333333333333333703, 0.3219752754296894559, 0.3333333333333333703, 0.3219752754296894559, 0.3333333333333333703, 0.3219752754296894559, 0.3333333333333333703, 0.3219752754296894559, 0.3333333333333333703, 0.3219752754296894559, 0.3333333333333333703, 0.3219752754296894559, 0.3333333333333333703, 0.3219752754296894559, 0.3333333333333333703, 0.3219752754296894559, 0.3333333333333333703, 0.3219752754296894559, 0.3333333333333333703, 0.3219752754296894559, 0.3333333333333333703, 0.3219752754296894559, 0.3333333333333333703, 0.3219752754296894559, 0.3333333333333333703, 0.3219752754296894559, 0.3333333333333333703, 0.3219752754296894559, 0.3333333333333333703, 0.3219752754296894559, 0.3333333333333333703, 0.3219752754296894559, 0.3333333333333333703, 0.3219752754296894559, 0.3333333333333333703, 0.3219752754296894559, 0.3333333333333333703, 0.3219752754296894559, 0.3333333333333333703, 0.3219752754296894559, 0.3333333333333333703, 0.3219752754296894559, 0.3333333333333333703, 0.3219752754296894559, 0.3333333333333333703, 0.3219752754296894559, 0.3333333333333333703, 0.3219752754296894559, 0.3333333333333333703, 0.3219752754296894559, 0.3333333333333333703, 0.3219752754296894559, 0.3333333333333333703, 0.3219752754296894559, 0.3333333333333333703, 0.3219752754296894559, 0.3333333333333333703, 0.3219752754296894559, 0.3333333333333333703, 0.3219752754296894559, 0.3333333333333333703, 0.3219752754296894559, 0.3333333333333333703, 0.3219752754296894559, 0.3333333333333333703, 0.3219752754296894559, 0.3333333333333333703, 0.3219752754296894559, 0.3333333333333333703, 0.3219752754296894559, 0.3333333333333333703, 0.3219752754296894559, 0.3333333333333333703, 0.3219752754296894559, 0.3333333333333333703, 0.3219752754296894559, 0.3333333333333333703, 0.3219752754296894559, 0.3333333333333333703, 0.3219752754296894559, 0.3333333333333333703, 0.3219752754296894559, 0.3333333333333333703, 0.3219752754296894559, 0.3333333333333333703, 0.3219752754296894559, 0.3333333333333333703, 0.3219752754296894559, 0.3333333333333333703, 0.3219752754296894559, 0.3333333333333333703, 0.3219752754296894559, 0.3333333333333333703, 0.3219752754296894559, 0.3333333333333333703, 0.3219752754296894559, 0.3333333333333333703, 0.3219752754296894559, 0.3333333333333333703, 0.3219752754296894559, 0.3333333333333333703, 0.3219752754296894559, 0.3333333333333333703, 0.3219752754296894559, 0.3333333333333333703, 0.3219752754296894559, 0.3333333333333333703, 0.3219752754296894559, 0.3333333333333333703, 0.3219752754296894559, 0.3333333333333333703, 0.3219752754296894559, 0.3333333333333333703, 0.3219752754296894559, 0.3333333333333333703, 0.3219752754296894559, 0.3333333333333333703, 0.3219752754296894559, 0.3333333333333333703, 0.3219752754296894559, 0.3333333333333333703, 0.3219752754296894559, 0.3333333333333333703, 0.3219752754296894559, 0.3333333333333333703, 0.3219752754296894559, 0.3333333333333333703, 0.3219752754296894559, 0.3333333333333333703, 0.3219752754296894559, 0.3333333333333333703, 0.3219752754296894559, 0.3333333333333333703, 0.3219752754296894559, 0.3333333333333333703, 0.3219752754296894559, 0.3333333333333333703, 0.3219752754296894559, 0.3333333333333333703, 0.3219752754296894559, 0.3333333333333333703, 0.3219752754296894559, 0.3333333333333333703, 0.3219752754296894559, 0.3333333333333333703, 0.3219752754296894559, 0.3333333333333333703, 0.3219752754296894559, 0.3333333333333333703, 0.3219752754296894559, 0.3333333333333333703, 0.3219752754296894559, 0.3333333333333333703, 0.3219752754296894559, 0.3333333333333333703, 0.3219752754296894559, 0.3333333333333333703, 0.3219752754296894559, 0.3333333333333333703, 0.3219752754296894559, 0.3333333333333333703, 0.3219752754296894559, 0.3333333333333333703, 0.3219752754296894559, 0.3333333333333333703, 0.3219752754296894559, 0.3333333333333333703, 0.3219752754296894559, 0.3333333333333333703, 0.3219752754296894559, 0.3333333333333333703, 0.3219752754296894559, 0.3333333333333333703, 0.3219752754296894559, 0.3333333333333333703, 0.3219752754296894559, 0.3333333333333333703, 0.3219752754296894559, 0.3333333333333333703, 0.3219752754296894559, 0.3333333333333333703, 0.3219752754296894559, 0.3333333333333333703, 0.3219752754296894559, 0.3333333333333333703, 0.3219752754296894559, 0.3333333333333333703, 0.3219752754296894559, 0.3333333333333333703, 0.3219752754296894559, 0.3333333333333333703, 0.3219752754296894559, 0.3333333333333333703, 0.3219752754296894559, 0.3333333333333333703, 0.3219752754296894559, 0.3333333333333333703, 0.3219752754296894559, 0.3333333333333333703, 0.3219752754296894559, 0.3333333333333333703, 0.3219752754296894559, 0.3333333333333333703, 0.3219752754296894559, 0.3333333333333333703, 0.3219752754296894559, 0.3333333333333333703, 0.3219752754296894559, 0.3333333333333333703, 0.3219752754296894559, 0.3333333333333333703, 0.3219752754296894559, 0.3333333333333333703, 0.3219752754296894559, 0.3333333333333333703, 0.3219752754296894559, 0.3333333333333333703, 0.3219752754296894559, 0.3333333333333333703, 0.3219752754296894559, 0.3333333333333333703, 0.3219752754296894559, 0.3333333333333333703, 0.3219752754296894559, 0.3333333333333333703, 0.3219752754296894559, 0.3333333333333333703, 0.3219752754296894559, 0.3333333333333333703, 0.3219752754296894559, 0.3333333333333333703, 0.3219752754296894559, 0.3333333333333333703, 0.3219752754296894559, 0.3333333333333333703, 0.3219752754296894559, 0.3333333333333333703, 0.3219752754296894559, 0.3333333333333333703, 0.3219752754296894559, 0.3333333333333333703),
 ( 1.000000000000000000, 0.9659258262890683122, 1.000000000000000000, 0.9659258262890683122, 1.000000000000000000, 0.9659258262890683122, 1.000000000000000000, 0.9659258262890683122, 1.000000000000000000, 0.9659258262890683122, 1.000000000000000000, 0.9659258262890683122, 1.000000000000000000, 0.9659258262890683122, 1.000000000000000000, 0.9659258262890683122, 1.000000000000000000, 0.9659258262890683122, 1.000000000000000000, 0.9659258262890683122, 1.000000000000000000, 0.9659258262890683122, 1.000000000000000000, 0.9659258262890683122, 1.000000000000000000, 0.9659258262890683122, 1.000000000000000000, 0.9659258262890683122, 1.000000000000000000, 0.9659258262890683122, 1.000000000000000000, 0.9659258262890683122, 1.000000000000000000, 0.9659258262890683122, 1.000000000000000000, 0.9659258262890683122, 1.000000000000000000, 0.9659258262890683122, 1.000000000000000000, 0.9659258262890683122, 1.000000000000000000, 0.9659258262890683122, 1.000000000000000000, 0.9659258262890683122, 1.000000000000000000, 0.9659258262890683122, 1.000000000000000000, 0.9659258262890683122, 1.000000000000000000, 0.9659258262890683122, 1.000000000000000000, 0.9659258262890683122, 1.000000000000000000, 0.9659258262890683122, 1.000000000000000000, 0.9659258262890683122, 1.000000000000000000, 0.9659258262890683122, 1.000000000000000000, 0.9659258262890683122, 1.000000000000000000, 0.9659258262890683122, 1.000000000000000000, 0.9659258262890683122, 1.000000000000000000, 0.9659258262890683122, 1.000000000000000000, 0.9659258262890683122, 1.000000000000000000, 0.9659258262890683122, 1.000000000000000000, 0.9659258262890683122, 1.000000000000000000, 0.9659258262890683122, 1.000000000000000000, 0.9659258262890683122, 1.000000000000000000, 0.9659258262890683122, 1.000000000000000000, 0.9659258262890683122, 1.000000000000000000, 0.9659258262890683122, 1.000000000000000000, 0.9659258262890683122, 1.000000000000000000, 0.9659258262890683122, 1.000000000000000000, 0.9659258262890683122, 1.000000000000000000, 0.9659258262890683122, 1.000000000000000000, 0.9659258262890683122, 1.000000000000000000, 0.9659258262890683122, 1.000000000000000000, 0.9659258262890683122, 1.000000000000000000, 0.9659258262890683122, 1.000000000000000000, 0.9659258262890683122, 1.000000000000000000, 0.9659258262890683122, 1.000000000000000000, 0.9659258262890683122, 1.000000000000000000, 0.9659258262890683122, 1.000000000000000000, 0.9659258262890683122, 1.000000000000000000, 0.9659258262890683122, 1.000000000000000000, 0.9659258262890683122, 1.000000000000000000, 0.9659258262890683122, 1.000000000000000000, 0.9659258262890683122, 1.000000000000000000, 0.9659258262890683122, 1.000000000000000000, 0.9659258262890683122, 1.000000000000000000, 0.9659258262890683122, 1.000000000000000000, 0.9659258262890683122, 1.000000000000000000, 0.9659258262890683122, 1.000000000000000000, 0.9659258262890683122, 1.000000000000000000, 0.9659258262890683122, 1.000000000000000000, 0.9659258262890683122, 1.000000000000000000, 0.9659258262890683122, 1.000000000000000000, 0.9659258262890683122, 1.000000000000000000, 0.9659258262890683122, 1.000000000000000000, 0.9659258262890683122, 1.000000000000000000, 0.9659258262890683122, 1.000000000000000000, 0.9659258262890683122, 1.000000000000000000, 0.9659258262890683122, 1.000000000000000000, 0.9659258262890683122, 1.000000000000000000, 0.9659258262890683122, 1.000000000000000000, 0.9659258262890683122, 1.000000000000000000, 0.9659258262890683122, 1.000000000000000000, 0.9659258262890683122, 1.000000000000000000, 0.9659258262890683122, 1.000000000000000000, 0.9659258262890683122, 1.000000000000000000, 0.9659258262890683122, 1.000000000000000000, 0.9659258262890683122, 1.000000000000000000, 0.9659258262890683122, 1.000000000000000000, 0.9659258262890683122, 1.000000000000000000, 0.9659258262890683122, 1.000000000000000000, 0.9659258262890683122, 1.000000000000000000, 0.9659258262890683122, 1.000000000000000000, 0.9659258262890683122, 1.000000000000000000, 0.9659258262890683122, 1.000000000000000000, 0.9659258262890683122, 1.000000000000000000, 0.9659258262890683122, 1.000000000000000000, 0.9659258262890683122, 1.000000000000000000, 0.9659258262890683122, 1.000000000000000000, 0.9659258262890683122, 1.000000000000000000, 0.9659258262890683122, 1.000000000000000000, 0.9659258262890683122, 1.000000000000000000, 0.9659258262890683122, 1.000000000000000000, 0.9659258262890683122, 1.000000000000000000, 0.9659258262890683122, 1.000000000000000000, 0.9659258262890683122, 1.000000000000000000, 0.9659258262890683122, 1.000000000000000000, 0.9659258262890683122, 1.000000000000000000, 0.9659258262890683122, 1.000000000000000000, 0.9659258262890683122, 1.000000000000000000, 0.9659258262890683122, 1.000000000000000000, 0.9659258262890683122, 1.000000000000000000, 0.9659258262890683122, 1.000000000000000000, 0.9659258262890683122, 1.000000000000000000, 0.9659258262890683122, 1.000000000000000000, 0.9659258262890683122, 1.000000000000000000, 0.9659258262890683122, 1.000000000000000000, 0.9659258262890683122, 1.000000000000000000, 0.9659258262890683122, 1.000000000000000000, 0.9659258262890683122, 1.000000000000000000, 0.9659258262890683122, 1.000000000000000000, 0.9659258262890683122, 1.000000000000000000, 0.9659258262890683122, 1.000000000000000000, 0.9659258262890683122, 1.000000000000000000, 0.9659258262890683122, 1.000000000000000000, 0.9659258262890683122, 1.000000000000000000, 0.9659258262890683122, 1.000000000000000000, 0.9659258262890683122, 1.000000000000000000, 0.9659258262890683122, 1.000000000000000000, 0.9659258262890683122, 1.000000000000000000, 0.9659258262890683122, 1.000000000000000000, 0.9659258262890683122, 1.000000000000000000, 0.9659258262890683122, 1.000000000000000000, 0.9659258262890683122, 1.000000000000000000, 0.9659258262890683122, 1.000000000000000000, 0.9659258262890683122, 1.000000000000000000, 0.9659258262890683122, 1.000000000000000000, 0.9659258262890683122, 1.000000000000000000, 0.9659258262890683122, 1.000000000000000000, 0.9659258262890683122, 1.000000000000000000, 0.9659258262890683122, 1.000000000000000000, 0.9659258262890683122, 1.000000000000000000, 0.9659258262890683122, 1.000000000000000000, 0.9659258262890683122, 1.000000000000000000, 0.9659258262890683122, 1.000000000000000000, 0.9659258262890683122, 1.000000000000000000, 0.9659258262890683122, 1.000000000000000000, 0.9659258262890683122, 1.000000000000000000, 0.9659258262890683122, 1.000000000000000000, 0.9659258262890683122, 1.000000000000000000, 0.9659258262890683122, 1.000000000000000000, 0.9659258262890683122, 1.000000000000000000, 0.9659258262890683122, 1.000000000000000000, 0.9659258262890683122, 1.000000000000000000, 0.9659258262890683122, 1.000000000000000000, 0.9659258262890683122, 1.000000000000000000, 0.9659258262890683122, 1.000000000000000000, 0.9659258262890683122, 1.000000000000000000, 0.9659258262890683122, 1.000000000000000000, 0.9659258262890683122, 1.000000000000000000, 0.9659258262890683122, 1.000000000000000000, 0.9659258262890683122, 1.000000000000000000, 0.9659258262890683122, 1.000000000000000000, 0.9659258262890683122, 1.000000000000000000, 0.9659258262890683122, 1.000000000000000000, 0.9659258262890683122, 1.000000000000000000, 0.9659258262890683122, 1.000000000000000000, 0.9659258262890683122, 1.000000000000000000, 0.9659258262890683122, 1.000000000000000000, 0.9659258262890683122, 1.000000000000000000, 0.9659258262890683122, 1.000000000000000000, 0.9659258262890683122, 1.000000000000000000, 0.9659258262890683122, 1.000000000000000000, 0.9659258262890683122, 1.000000000000000000, 0.9659258262890683122, 1.000000000000000000, 0.9659258262890683122, 1.000000000000000000, 0.9659258262890683122, 1.000000000000000000, 0.9659258262890683122, 1.000000000000000000, 0.9659258262890683122, 1.000000000000000000, 0.9659258262890683122, 1.000000000000000000, 0.9659258262890683122, 1.000000000000000000, 0.9659258262890683122, 1.000000000000000000, 0.9659258262890683122, 1.000000000000000000, 0.9659258262890683122, 1.000000000000000000, 0.9659258262890683122, 1.000000000000000000, 0.9659258262890683122, 1.000000000000000000, 0.9659258262890683122, 1.000000000000000000, 0.9659258262890683122, 1.000000000000000000, 0.9659258262890683122, 1.000000000000000000, 0.9659258262890683122, 1.000000000000000000, 0.9659258262890683122, 1.000000000000000000, 0.9659258262890683122, 1.000000000000000000, 0.9659258262890683122, 1.000000000000000000, 0.9659258262890683122, 1.000000000000000000, 0.9659258262890683122, 1.000000000000000000, 0.9659258262890683122, 1.000000000000000000, 0.9659258262890683122, 1.000000000000000000, 0.9659258262890683122, 1.000000000000000000, 0.9659258262890683122, 1.000000000000000000, 0.9659258262890683122, 1.000000000000000000, 0.9659258262890683122, 1.000000000000000000, 0.9659258262890683122, 1.000000000000000000, 0.9659258262890683122, 1.000000000000000000, 0.9659258262890683122, 1.000000000000000000, 0.9659258262890683122, 1.000000000000000000, 0.9659258262890683122, 1.000000000000000000, 0.9659258262890683122, 1.000000000000000000, 0.9659258262890683122, 1.000000000000000000, 0.9659258262890683122, 1.000000000000000000, 0.9659258262890683122, 1.000000000000000000, 0.9659258262890683122, 1.000000000000000000, 0.9659258262890683122, 1.000000000000000000, 0.9659258262890683122, 1.000000000000000000, 0.9659258262890683122, 1.000000000000000000, 0.9659258262890683122, 1.000000000000000000, 0.9659258262890683122, 1.000000000000000000, 0.9659258262890683122, 1.000000000000000000, 0.9659258262890683122, 1.000000000000000000, 0.9659258262890683122, 1.000000000000000000, 0.9659258262890683122, 1.000000000000000000, 0.9659258262890683122, 1.000000000000000000, 0.9659258262890683122, 1.000000000000000000, 0.9659258262890683122, 1.000000000000000000, 0.9659258262890683122, 1.000000000000000000, 0.9659258262890683122, 1.000000000000000000, 0.9659258262890683122, 1.000000000000000000, 0.9659258262890683122, 1.000000000000000000, 0.9659258262890683122, 1.000000000000000000, 0.9659258262890683122, 1.000000000000000000, 0.9659258262890683122, 1.000000000000000000, 0.9659258262890683122, 1.000000000000000000, 0.9659258262890683122, 1.000000000000000000, 0.9659258262890683122, 1.000000000000000000, 0.9659258262890683122, 1.000000000000000000) ) ) 
 REPRESENTATION_ITEM ( '' )  SURFACE ( )  );
#80376=CARTESIAN_POINT ( 'NONE',  ( 16.46253265017160672, -9.564922557960803928, 108.3322429386476955 ) ) ;
#80377=CARTESIAN_POINT ( 'NONE',  ( 5.823673210054444382, -21.52544592524334988, 25.20942372801901854 ) ) ;
#80378=CARTESIAN_POINT ( 'NONE',  ( -13.97604488694547697, 13.89961937509957934, 88.12609039468563310 ) ) ;
#80380=CARTESIAN_POINT ( 'NONE',  ( -19.02544592524342804, 5.153800228976336051, 46.04057627198101699 ) ) ;
#80381=CARTESIAN_POINT ( 'NONE',  ( 16.51473224551069308, 9.474510206698969483, 89.16557627198103830 ) ) ;
#80382=CARTESIAN_POINT ( 'NONE',  ( 0.05219959533910956823, 16.53943276465976808, 64.99890960531435269 ) ) ;
#80383=CARTESIAN_POINT ( 'NONE',  ( -19.03943276465977164, 0.05219959533909376836, 46.24890960531435979 ) ) ;
#80384=CARTESIAN_POINT ( 'NONE',  ( -13.89961937509977652, 13.97604488694528158, 60.62390960531436690 ) ) ;
#80385=CARTESIAN_POINT ( 'NONE',  ( 13.89961937509957401, 13.97604488694547697, 61.87609039468566863 ) ) ;
#80386=CARTESIAN_POINT ( 'NONE',  ( 19.05341960407617918, -5.049401038297876454, 26.04275706135233293 ) ) ;
#80387=CARTESIAN_POINT ( 'NONE',  ( 16.51473224551069308, 9.474510206698969483, 69.16557627198102409 ) ) ;
#80388=CARTESIAN_POINT ( 'NONE',  ( 18.67979575497178502, 10.72451020669898547, 64.16557627198102409 ) ) ;
#80389=CARTESIAN_POINT ( 'NONE',  ( 12.14591786802309770, 12.06949235617756955, 64.37390960531435269 ) ) ;
#80390=CARTESIAN_POINT ( 'NONE',  ( -19.05341960407617563, 5.049401038297882671, 33.54275706135231871 ) ) ;
#80392=CARTESIAN_POINT ( 'NONE',  ( -10.72451020669898014, 18.67979575497178502, 45.41557627198103830 ) ) ;
#80393=CARTESIAN_POINT ( 'NONE',  ( 21.52544592524344225, -5.823673210054117533, 23.54057627198102765 ) ) ;
#80394=CARTESIAN_POINT ( 'NONE',  ( 19.03943276465977164, -0.05219959533909143690, 48.74890960531435979 ) ) ;
#80395=CARTESIAN_POINT ( 'NONE',  ( 5.153800228976335163, 19.02544592524342804, 39.79057627198100988 ) ) ;
#80396=CARTESIAN_POINT ( 'NONE',  ( 12.06949235617757843, -12.14591786802309237, 103.1239096053143811 ) ) ;
#80397=CARTESIAN_POINT ( 'NONE',  ( 15.80617190586746368, 15.72974639402197994, 114.3739096053143527 ) ) ;
#80398=CARTESIAN_POINT ( 'NONE',  ( 16.51473224551069308, 9.474510206698969483, 109.1655762719810383 ) ) ;
#80399=CARTESIAN_POINT ( 'NONE',  ( 21.53943276465977519, 0.05219959533937863772, 21.25109039468567218 ) ) ;
#80400=CARTESIAN_POINT ( 'NONE',  ( 12.14591786802309770, 12.06949235617756955, 114.3739096053143527 ) ) ;
#80401=CARTESIAN_POINT ( 'NONE',  ( -10.72451020669898014, 18.67979575497178502, 95.41557627198102409 ) ) ;
#80403=CARTESIAN_POINT ( 'NONE',  ( -19.03943276465977164, -0.05219959533935918106, 53.75109039468566863 ) ) ;
#80404=CARTESIAN_POINT ( 'NONE',  ( 13.97604488694527802, 13.89961937509977652, 24.37390960531435624 ) ) ;
#80405=CARTESIAN_POINT ( 'NONE',  ( 9.564922557960805705, 16.46253265017160317, 29.58224293864769550 ) ) ;
#80407=CARTESIAN_POINT ( 'NONE',  ( 8.224510206698742110, 14.34966873604972548, 42.08442372801901854 ) ) ;
#80408=CARTESIAN_POINT ( 'NONE',  ( 0.05219959533910956823, 16.53943276465976808, 114.9989096053143669 ) ) ;
#80410=CARTESIAN_POINT ( 'NONE',  ( -16.46253265017160317, 9.564922557960807481, 75.83224293864769550 ) ) ;
#80411=CARTESIAN_POINT ( 'NONE',  ( 0.05219959533910956823, 16.53943276465976808, 94.99890960531436690 ) ) ;
#80412=CARTESIAN_POINT ( 'NONE',  ( 21.52544592524344225, -5.823673210054117533, 48.54057627198103120 ) ) ;
#80413=CARTESIAN_POINT ( 'NONE',  ( -12.14591786802309592, -12.06949235617757132, 81.87390960531435269 ) ) ;
#80414=CARTESIAN_POINT ( 'NONE',  ( 4.379528057220092307, 16.55341960407617563, 32.29275706135235424 ) ) ;
#80415=CARTESIAN_POINT ( 'NONE',  ( -18.67979575497193778, 10.72451020669871902, 88.33442372801901854 ) ) ;
#80416=CARTESIAN_POINT ( 'NONE',  ( 5.153800228976335163, 19.02544592524342804, 29.79057627198102409 ) ) ;
#80417=CARTESIAN_POINT ( 'NONE',  ( -8.224510206698735004, -14.34966873604973081, 94.58442372801901854 ) ) ;
#80418=CARTESIAN_POINT ( 'NONE',  ( 4.379528057220339221, -16.55341960407611168, 47.70724293864770260 ) ) ;
#80419=CARTESIAN_POINT ( 'NONE',  ( -9.564922557960796823, -16.46253265017161027, 52.08224293864768839 ) ) ;
#80420=CARTESIAN_POINT ( 'NONE',  ( -15.72974639402176322, -15.80617190586768395, 99.37609039468568994 ) ) ;
#80421=CARTESIAN_POINT ( 'NONE',  ( 18.67979575497178502, 10.72451020669898547, 114.1655762719810383 ) ) ;
#80422=CARTESIAN_POINT ( 'NONE',  ( 21.52544592524334988, 5.823673210054432836, 66.45942372801903275 ) ) ;
#80423=CARTESIAN_POINT ( 'NONE',  ( 4.483927247898790824, -16.52544592524335698, 40.20942372801901854 ) ) ;
#80424=CARTESIAN_POINT ( 'NONE',  ( 14.29746914071049879, -8.314922557960816363, 63.33224293864770260 ) ) ;
#80425=CARTESIAN_POINT ( 'NONE',  ( -15.72974639402176322, -15.80617190586768395, 89.37609039468568994 ) ) ;
#80426=CARTESIAN_POINT ( 'NONE',  ( 14.34966873604960469, 8.224510206698951720, 24.16557627198103120 ) ) ;
#80427=CARTESIAN_POINT ( 'NONE',  ( 17.05587630539707433, -6.762274262136759084, 48.24180309037284076 ) ) ;
#80429=CARTESIAN_POINT ( 'NONE',  ( -12.06949235617756955, 12.14591786802309770, 45.62390960531436690 ) ) ;
#80430=CARTESIAN_POINT ( 'NONE',  ( 4.379528057220092307, 16.55341960407617563, 67.29275706135234714 ) ) ;
#80431=CARTESIAN_POINT ( 'NONE',  ( -9.474510206698964154, 16.51473224551069663, 85.41557627198102409 ) ) ;
#80432=CARTESIAN_POINT ( 'NONE',  ( -0.05219959533909027116, -19.03943276465977164, 97.49890960531436690 ) ) ;
#80433=CARTESIAN_POINT ( 'NONE',  ( 18.62759615963255655, 10.81492255796105972, 86.66775706135234714 ) ) ;
#80434=CARTESIAN_POINT ( 'NONE',  ( 8.224510206698742110, 14.34966873604972548, 107.0844237280190043 ) ) ;
#80435=CARTESIAN_POINT ( 'NONE',  ( 14.29746914071049879, -8.314922557960816363, 78.33224293864770971 ) ) ;
#80436=CARTESIAN_POINT ( 'NONE',  ( -16.46253265017160317, 9.564922557960807481, 80.83224293864769550 ) ) ;
#80438=CARTESIAN_POINT ( 'NONE',  ( 16.52544592524335698, 4.483927247898782831, 26.45942372801901854 ) ) ;
#80439=CARTESIAN_POINT ( 'NONE',  ( 5.153800228976335163, 19.02544592524342804, 29.79057627198102409 ) ) ;
#80440=CARTESIAN_POINT ( 'NONE',  ( -16.51473224551069308, -9.474510206698971260, 96.66557627198102409 ) ) ;
#80441=CARTESIAN_POINT ( 'NONE',  ( 14.29746914071037800, 8.314922557961029526, 26.66775706135235424 ) ) ;
#80443=CARTESIAN_POINT ( 'NONE',  ( -5.153800228976607833, 19.02544592524334988, 22.70942372801899012 ) ) ;
#80444=CARTESIAN_POINT ( 'NONE',  ( 0.05219959533934541429, -16.53943276465976808, 90.00109039468567573 ) ) ;
#80445=CARTESIAN_POINT ( 'NONE',  ( 5.049401038297881783, 19.05341960407617563, 112.2927570613523471 ) ) ;
#80446=CARTESIAN_POINT ( 'NONE',  ( -19.05341960407611168, -5.049401038298163336, 26.45724293864769550 ) ) ;
#80447=CARTESIAN_POINT ( 'NONE',  ( -12.14591786802326823, 12.06949235617739902, 83.12609039468568994 ) ) ;
#80448=CARTESIAN_POINT ( 'NONE',  ( 12.06949235617739724, 12.14591786802326823, 71.87609039468568994 ) ) ;
#80450=CARTESIAN_POINT ( 'NONE',  ( 19.05341960407617918, -5.049401038297876454, 71.04275706135234714 ) ) ;
#80451=CARTESIAN_POINT ( 'NONE',  ( -18.62759615963255300, -10.81492255796106328, 109.1677570613523613 ) ) ;
#80452=CARTESIAN_POINT ( 'NONE',  ( -0.05219959533909027116, -19.03943276465977164, 52.49890960531436690 ) ) ;
#80453=CARTESIAN_POINT ( 'NONE',  ( -19.05341960407611168, -5.049401038298163336, 91.45724293864766707 ) ) ;
#80454=CARTESIAN_POINT ( 'NONE',  ( 16.55341960407611168, 4.379528057220329451, 83.95724293864770971 ) ) ;
#80455=CARTESIAN_POINT ( 'NONE',  ( -13.97604488694547697, 13.89961937509957934, 53.12609039468565442 ) ) ;
#80456=CARTESIAN_POINT ( 'NONE',  ( -0.05219959533907301413, -21.53943276465977519, 52.49890960531435979 ) ) ;
#80457=CARTESIAN_POINT ( 'NONE',  ( -21.55341960407619339, 5.719274019375674811, 108.5427570613523756 ) ) ;
#80458=CARTESIAN_POINT ( 'NONE',  ( 0.05219959533909260263, 19.03943276465977164, 89.99890960531436690 ) ) ;
#80459=CARTESIAN_POINT ( 'NONE',  ( 18.67979575497194134, -10.72451020669871369, 110.8344237280190043 ) ) ;
#80460=CARTESIAN_POINT ( 'NONE',  ( -5.719274019375978568, 21.55341960407610458, 65.20724293864768129 ) ) ;
#80461=CARTESIAN_POINT ( 'NONE',  ( 5.049401038298161559, -19.05341960407611168, 92.70724293864769550 ) ) ;
#80462=CARTESIAN_POINT ( 'NONE',  ( -5.049401038297874678, -19.05341960407617918, 89.79275706135230450 ) ) ;
#80463=CARTESIAN_POINT ( 'NONE',  ( -9.564922557960796823, -16.46253265017161027, 97.08224293864769550 ) ) ;
#80464=CARTESIAN_POINT ( 'NONE',  ( -13.89961937509957401, -13.97604488694547875, 104.3760903946856757 ) ) ;
#80465=CARTESIAN_POINT ( 'NONE',  ( -13.97604488694527625, -13.89961937509977652, 21.87390960531435979 ) ) ;
#80466=CARTESIAN_POINT ( 'NONE',  ( -13.89961937509977652, 13.97604488694528158, 80.62390960531436690 ) ) ;
#80467=CARTESIAN_POINT ( 'NONE',  ( 5.719274019375991003, -21.55341960407610458, 82.70724293864770971 ) ) ;
#80468=AXIS2_PLACEMENT_3D ( 'NONE', #27384, #69874, #89030 ) ;
#80469=CARTESIAN_POINT ( 'NONE',  ( -16.52544592524335698, -4.483927247898792601, 48.95942372801902565 ) ) ;
#80470=CARTESIAN_POINT ( 'NONE',  ( 21.53943276465977519, 0.05219959533937863772, 46.25109039468567573 ) ) ;
#80471=CARTESIAN_POINT ( 'NONE',  ( -10.81492255796105439, 18.62759615963255655, 92.91775706135236135 ) ) ;
#80472=CARTESIAN_POINT ( 'NONE',  ( 16.55341960407618274, -4.379528057220086978, 91.04275706135236135 ) ) ;
#80473=CARTESIAN_POINT ( 'NONE',  ( -13.89961937509977652, 13.97604488694528158, 85.62390960531433848 ) ) ;
#80474=CARTESIAN_POINT ( 'NONE',  ( 14.29746914071049879, -8.314922557960816363, 88.33224293864769550 ) ) ;
#80475=CARTESIAN_POINT ( 'NONE',  ( -16.55341960407611168, -4.379528057220339221, 26.45724293864768839 ) ) ;
#80476=CARTESIAN_POINT ( 'NONE',  ( -5.049401038297874678, -19.05341960407617918, 64.79275706135233293 ) ) ;
#80477=CARTESIAN_POINT ( 'NONE',  ( -21.55341960407619339, 5.719274019375674811, 48.54275706135234714 ) ) ;
#80478=CARTESIAN_POINT ( 'NONE',  ( 19.03943276465977164, 0.05219959533936151252, 26.25109039468566507 ) ) ;
#80479=CARTESIAN_POINT ( 'NONE',  ( 12.06949235617757843, -12.14591786802309237, 98.12390960531436690 ) ) ;
#80480=CARTESIAN_POINT ( 'NONE',  ( -21.53943276465977519, 0.05219959533907696930, 21.24890960531436690 ) ) ;
#80481=CARTESIAN_POINT ( 'NONE',  ( -16.55341960407611168, -4.379528057220339221, 26.45724293864768839 ) ) ;
#80482=CARTESIAN_POINT ( 'NONE',  ( -21.53943276465977519, -0.05219959533937600094, 83.75109039468568994 ) ) ;
#80483=CARTESIAN_POINT ( 'NONE',  ( -12.14591786802326823, 12.06949235617739902, 53.12609039468568284 ) ) ;
#80484=CARTESIAN_POINT ( 'NONE',  ( 16.52544592524335698, 4.483927247898782831, 101.4594237280190185 ) ) ;
#80485=CARTESIAN_POINT ( 'NONE',  ( -15.72974639402176322, -15.80617190586768395, 59.37609039468568284 ) ) ;
#80487=CARTESIAN_POINT ( 'NONE',  ( 21.53943276465977519, 0.05219959533937863772, 26.25109039468567573 ) ) ;
#80488=CARTESIAN_POINT ( 'NONE',  ( -16.52544592524342804, 4.483927247898546575, 106.0405762719810525 ) ) ;
#80489=CARTESIAN_POINT ( 'NONE',  ( -5.153800228976328057, -19.02544592524343514, 32.29057627198102409 ) ) ;
#80490=CARTESIAN_POINT ( 'NONE',  ( -12.06949235617756955, 12.14591786802309770, 70.62390960531436690 ) ) ;
#80491=CARTESIAN_POINT ( 'NONE',  ( -0.05219959533909027116, -19.03943276465977164, 72.49890960531435269 ) ) ;
#80492=CARTESIAN_POINT ( 'NONE',  ( 8.314922557961029526, -14.29746914071037800, 110.4177570613523756 ) ) ;
#80493=CARTESIAN_POINT ( 'NONE',  ( 9.474510206698971260, -16.51473224551069308, 32.91557627198102409 ) ) ;
#80494=CARTESIAN_POINT ( 'NONE',  ( -15.72974639402197994, 15.80617190586746368, 50.62390960531435979 ) ) ;
#80495=CARTESIAN_POINT ( 'NONE',  ( -12.14591786802309592, -12.06949235617757132, 91.87390960531436690 ) ) ;
#80497=CARTESIAN_POINT ( 'NONE',  ( 5.719274019375991003, -21.55341960407610458, 92.70724293864770971 ) ) ;
#80498=CARTESIAN_POINT ( 'NONE',  ( -5.049401038298153566, 19.05341960407611168, 100.2072429386476955 ) ) ;
#80499=CARTESIAN_POINT ( 'NONE',  ( 19.02544592524343514, -5.153800228976328945, 53.54057627198102409 ) ) ;
#80500=CARTESIAN_POINT ( 'NONE',  ( 0.05219959533936267826, -19.03943276465977164, 90.00109039468567573 ) ) ;
#80501=CARTESIAN_POINT ( 'NONE',  ( 21.52544592524344225, -5.823673210054117533, 43.54057627198103830 ) ) ;
#80502=CARTESIAN_POINT ( 'NONE',  ( -5.719274019375665041, -21.55341960407619695, 64.79275706135234714 ) ) ;
#80503=CARTESIAN_POINT ( 'NONE',  ( 5.153800228976335163, 19.02544592524342804, 54.79057627198103120 ) ) ;
#80504=CARTESIAN_POINT ( 'NONE',  ( -19.02544592524342804, 5.153800228976336051, 91.04057627198100988 ) ) ;
#80505=CARTESIAN_POINT ( 'NONE',  ( -4.379528057220086978, -16.55341960407618274, 64.79275706135234714 ) ) ;
#80506=CARTESIAN_POINT ( 'NONE',  ( -18.67979575497193778, 10.72451020669871902, 38.33442372801900433 ) ) ;
#80507=CARTESIAN_POINT ( 'NONE',  ( -18.62759615963255300, -10.81492255796106328, 74.16775706135231871 ) ) ;
#80508=CARTESIAN_POINT ( 'NONE',  ( -21.55341960407610458, -5.719274019375992779, 26.45724293864768839 ) ) ;
#80509=CARTESIAN_POINT ( 'NONE',  ( -15.80617190586745835, -15.72974639402198527, 101.8739096053143811 ) ) ;
#80510=CARTESIAN_POINT ( 'NONE',  ( -15.80617190586768217, 15.72974639402176855, 38.12609039468567573 ) ) ;
#80511=CARTESIAN_POINT ( 'NONE',  ( -16.55341960407617563, 4.379528057220093196, 58.54275706135235424 ) ) ;
#80512=CARTESIAN_POINT ( 'NONE',  ( 15.72974639402199770, -15.80617190586745480, 68.12390960531436690 ) ) ;
#80513=CARTESIAN_POINT ( 'NONE',  ( 9.564922557961047289, -16.46253265017146816, 30.41775706135232937 ) ) ;
#80514=CARTESIAN_POINT ( 'NONE',  ( 5.153800228976335163, 19.02544592524342804, 74.79057627198103830 ) ) ;
#80515=CARTESIAN_POINT ( 'NONE',  ( -8.224510206698735004, -14.34966873604973081, 109.5844237280190328 ) ) ;
#80517=CARTESIAN_POINT ( 'NONE',  ( 0.05219959533909260263, 19.03943276465977164, 104.9989096053143669 ) ) ;
#80518=CARTESIAN_POINT ( 'NONE',  ( -17.49999999999999645, 5.499999999999997335, 120.0000000000000142 ) ) ;
#80519=CARTESIAN_POINT ( 'NONE',  ( 19.03943276465977164, 0.05219959533936151252, 81.25109039468567573 ) ) ;
#80520=CARTESIAN_POINT ( 'NONE',  ( -5.823673210054116645, -21.52544592524344225, 52.29057627198102409 ) ) ;
#80521=CARTESIAN_POINT ( 'NONE',  ( -14.29746914071049879, 8.314922557960819915, 35.83224293864768839 ) ) ;
#80522=CARTESIAN_POINT ( 'NONE',  ( -14.34966873604972548, 8.224510206698743886, 23.33442372801901499 ) ) ;
#80523=CARTESIAN_POINT ( 'NONE',  ( 5.153800228976335163, 19.02544592524342804, 34.79057627198102409 ) ) ;
#80524=CARTESIAN_POINT ( 'NONE',  ( -19.03943276465977164, -0.05219959533935918106, 113.7510903946856757 ) ) ;
#80525=CARTESIAN_POINT ( 'NONE',  ( 0.05219959533907565091, 21.53943276465977519, 84.99890960531436690 ) ) ;
#80526=CARTESIAN_POINT ( 'NONE',  ( -19.02544592524334988, -5.153800228976617603, 63.95942372801899012 ) ) ;
#80527=CARTESIAN_POINT ( 'NONE',  ( 0.05219959533934541429, -16.53943276465976808, 80.00109039468568994 ) ) ;
#80528=CARTESIAN_POINT ( 'NONE',  ( 19.02544592524343514, -5.153800228976328945, 68.54057627198103830 ) ) ;
#80529=CARTESIAN_POINT ( 'NONE',  ( -4.379528057220328563, 16.55341960407611168, 75.20724293864769550 ) ) ;
#80530=CARTESIAN_POINT ( 'NONE',  ( -19.03943276465977164, 0.05219959533909376836, 41.24890960531435269 ) ) ;
#80531=CARTESIAN_POINT ( 'NONE',  ( -0.05219959533910754901, -16.53943276465976808, 52.49890960531435979 ) ) ;
#80532=CARTESIAN_POINT ( 'NONE',  ( -16.51473224551069308, -9.474510206698971260, 21.66557627198102765 ) ) ;
#80534=CARTESIAN_POINT ( 'NONE',  ( -14.34966873604960291, -8.224510206698953496, 26.66557627198103475 ) ) ;
#80535=CARTESIAN_POINT ( 'NONE',  ( 13.97604488694527802, 13.89961937509977652, 74.37390960531436690 ) ) ;
#80537=CARTESIAN_POINT ( 'NONE',  ( 5.049401038297881783, 19.05341960407617563, 37.29275706135232582 ) ) ;
#80538=CARTESIAN_POINT ( 'NONE',  ( -0.05219959533934338120, 16.53943276465976808, 52.50109039468567573 ) ) ;
#80539=CARTESIAN_POINT ( 'NONE',  ( 15.80617190586746368, 15.72974639402197994, 69.37390960531436690 ) ) ;
#80540=CARTESIAN_POINT ( 'NONE',  ( 9.474510206698729675, 16.51473224551082808, 27.08442372801900433 ) ) ;
#80541=CARTESIAN_POINT ( 'NONE',  ( 9.474510206698971260, -16.51473224551069308, 72.91557627198102409 ) ) ;
#80543=CARTESIAN_POINT ( 'NONE',  ( 13.97604488694527802, 13.89961937509977652, 114.3739096053143669 ) ) ;
#80544=CARTESIAN_POINT ( 'NONE',  ( 18.67979575497194134, -10.72451020669871369, 40.83442372801901854 ) ) ;
#80545=CARTESIAN_POINT ( 'NONE',  ( -4.483927247898539470, -16.52544592524342804, 102.2905762719810383 ) ) ;
#80546=CARTESIAN_POINT ( 'NONE',  ( -15.80617190586745835, -15.72974639402198527, 106.8739096053143811 ) ) ;
#80547=CARTESIAN_POINT ( 'NONE',  ( 16.46253265017160672, -9.564922557960803928, 78.33224293864769550 ) ) ;
#80549=CARTESIAN_POINT ( 'NONE',  ( -21.52544592524334988, -5.823673210054445271, 23.95942372801901143 ) ) ;
#80551=CARTESIAN_POINT ( 'NONE',  ( 13.89961937509977652, -13.97604488694527269, 93.12390960531436690 ) ) ;
#80553=CARTESIAN_POINT ( 'NONE',  ( 19.03943276465977164, -0.05219959533909143690, 33.74890960531435979 ) ) ;
#80554=CARTESIAN_POINT ( 'NONE',  ( 16.51473224551083163, -9.474510206698727899, 110.8344237280190043 ) ) ;
#80556=CARTESIAN_POINT ( 'NONE',  ( 16.55341960407611168, 4.379528057220329451, 108.9572429386476955 ) ) ;
#80557=CARTESIAN_POINT ( 'NONE',  ( 10.72451020669871369, 18.67979575497193778, 92.08442372801901854 ) ) ;
#80558=CARTESIAN_POINT ( 'NONE',  ( 19.03943276465977164, -0.05219959533909143690, 78.74890960531436690 ) ) ;
#80559=CARTESIAN_POINT ( 'NONE',  ( 18.67979575497194134, -10.72451020669871369, 40.83442372801901854 ) ) ;
#80560=CARTESIAN_POINT ( 'NONE',  ( 21.52544592524334988, 5.823673210054432836, 21.45942372801901499 ) ) ;
#80562=CARTESIAN_POINT ( 'NONE',  ( -19.02544592524342804, 5.153800228976336051, 81.04057627198103830 ) ) ;
#80564=CARTESIAN_POINT ( 'NONE',  ( 16.55341960407618274, -4.379528057220086978, 31.04275706135234714 ) ) ;
#80565=CARTESIAN_POINT ( 'NONE',  ( 15.80617190586746368, 15.72974639402197994, 44.37390960531435979 ) ) ;
#80566=CARTESIAN_POINT ( 'NONE',  ( -0.05219959533937732626, 21.53943276465977519, 82.50109039468568994 ) ) ;
#80567=CARTESIAN_POINT ( 'NONE',  ( -13.97604488694527625, -13.89961937509977652, 111.8739096053143243 ) ) ;
#80568=CARTESIAN_POINT ( 'NONE',  ( 5.049401038297881783, 19.05341960407617563, 92.29275706135234714 ) ) ;
#80569=CARTESIAN_POINT ( 'NONE',  ( 5.153800228976335163, 19.02544592524342804, 64.79057627198100988 ) ) ;
#80570=CARTESIAN_POINT ( 'NONE',  ( -5.049401038298153566, 19.05341960407611168, 80.20724293864769550 ) ) ;
#80571=EDGE_CURVE ( 'NONE', #35831, #11669, #161688, .T. ) ;
#80572=CARTESIAN_POINT ( 'NONE',  ( 14.29746914071049879, -8.314922557960816363, 103.3322429386476955 ) ) ;
#80573=CARTESIAN_POINT ( 'NONE',  ( -16.53943276465976808, 0.05219959533911058130, 106.2489096053143811 ) ) ;
#80574=CARTESIAN_POINT ( 'NONE',  ( -19.02544592524342804, 5.153800228976336051, 106.0405762719810241 ) ) ;
#80575=CARTESIAN_POINT ( 'NONE',  ( -8.314922557961024197, 14.29746914071037800, 77.91775706135231871 ) ) ;
#80576=CARTESIAN_POINT ( 'NONE',  ( 8.224510206698953496, -14.34966873604960469, 52.91557627198103830 ) ) ;
#80577=CARTESIAN_POINT ( 'NONE',  ( 19.03943276465977164, -0.05219959533909143690, 38.74890960531436690 ) ) ;
#80578=CARTESIAN_POINT ( 'NONE',  ( 21.52544592524334988, 5.823673210054432836, 81.45942372801900433 ) ) ;
#80579=CARTESIAN_POINT ( 'NONE',  ( 21.53943276465977519, 0.05219959533937863772, 76.25109039468568994 ) ) ;
#80580=CARTESIAN_POINT ( 'NONE',  ( -19.05341960407617563, 5.049401038297882671, 88.54275706135230450 ) ) ;
#80581=CARTESIAN_POINT ( 'NONE',  ( 12.06949235617757843, -12.14591786802309237, 58.12390960531435979 ) ) ;
#80582=CARTESIAN_POINT ( 'NONE',  ( -10.81492255796078084, -18.62759615963271287, 107.0822429386476955 ) ) ;
#80583=CARTESIAN_POINT ( 'NONE',  ( -15.80617190586745835, -15.72974639402198527, 51.87390960531437401 ) ) ;
#80584=CARTESIAN_POINT ( 'NONE',  ( -16.81555441253553340, -7.025013491695471401, 104.3631455466574494 ) ) ;
#80586=CARTESIAN_POINT ( 'NONE',  ( 16.46253265017160672, -9.564922557960803928, 68.33224293864770971 ) ) ;
#80587=CARTESIAN_POINT ( 'NONE',  ( 0.05219959533910956823, 16.53943276465976808, 34.99890960531435979 ) ) ;
#80588=CARTESIAN_POINT ( 'NONE',  ( 4.379528057220339221, -16.55341960407611168, 27.70724293864769905 ) ) ;
#80589=CARTESIAN_POINT ( 'NONE',  ( -4.483927247898782831, 16.52544592524335698, 82.70942372801900433 ) ) ;
#80590=CARTESIAN_POINT ( 'NONE',  ( 13.89961937509957401, 13.97604488694547697, 36.87609039468565442 ) ) ;
#80592=CARTESIAN_POINT ( 'NONE',  ( -9.474510206698964154, 16.51473224551069663, 85.41557627198102409 ) ) ;
#80594=CARTESIAN_POINT ( 'NONE',  ( -8.314922557960811034, -14.29746914071050412, 57.08224293864769550 ) ) ;
#80595=CARTESIAN_POINT ( 'NONE',  ( -19.05341960407611168, -5.049401038298163336, 21.45724293864768839 ) ) ;
#80596=CARTESIAN_POINT ( 'NONE',  ( 5.823673210054125526, 21.52544592524343514, 24.79057627198103120 ) ) ;
#80597=CARTESIAN_POINT ( 'NONE',  ( -10.72451020669898014, 18.67979575497178502, 55.41557627198102409 ) ) ;
#80598=CARTESIAN_POINT ( 'NONE',  ( -8.314922557960811034, -14.29746914071050412, 92.08224293864769550 ) ) ;
#80599=CARTESIAN_POINT ( 'NONE',  ( -14.29746914071037622, -8.314922557961029526, 34.16775706135234714 ) ) ;
#80600=CARTESIAN_POINT ( 'NONE',  ( -16.52544592524342804, 4.483927247898546575, 76.04057627198102409 ) ) ;
#80602=CARTESIAN_POINT ( 'NONE',  ( 13.97604488694548053, -13.89961937509957401, 80.62609039468567573 ) ) ;
#80603=CARTESIAN_POINT ( 'NONE',  ( 19.05341960407611168, 5.049401038298154454, 113.9572429386477097 ) ) ;
#80605=CARTESIAN_POINT ( 'NONE',  ( 5.049401038298163336, -19.05341960407611168, 42.70724293864768839 ) ) ;
#80607=CARTESIAN_POINT ( 'NONE',  ( -4.379528057220086978, -16.55341960407618274, 34.79275706135235424 ) ) ;
#80608=CARTESIAN_POINT ( 'NONE',  ( 14.29746914071049879, -8.314922557960816363, 33.33224293864769550 ) ) ;
#80609=CARTESIAN_POINT ( 'NONE',  ( 18.62759615963271287, -10.81492255796078972, 58.33224293864768839 ) ) ;
#80610=CARTESIAN_POINT ( 'NONE',  ( 13.97604488694548053, -13.89961937509957401, 85.62609039468568994 ) ) ;
#80611=CARTESIAN_POINT ( 'NONE',  ( 18.67979575497178502, 10.72451020669898547, 54.16557627198103120 ) ) ;
#80612=CARTESIAN_POINT ( 'NONE',  ( 21.55341960407619695, -5.719274019375665929, 86.04275706135236135 ) ) ;
#80614=CARTESIAN_POINT ( 'NONE',  ( -14.29746914071037622, -8.314922557961029526, 29.16775706135234003 ) ) ;
#80615=CARTESIAN_POINT ( 'NONE',  ( 17.59860650958994555, -7.585241751806880650, 55.92337014262493966 ) ) ;
#80616=CARTESIAN_POINT ( 'NONE',  ( 19.02544592524343514, -5.153800228976328945, 88.54057627198102409 ) ) ;
#80617=CARTESIAN_POINT ( 'NONE',  ( -0.05219959533909027116, -19.03943276465977164, 32.49890960531435979 ) ) ;
#80618=CARTESIAN_POINT ( 'NONE',  ( 8.314922557960818139, 14.29746914071049879, 104.5822429386477097 ) ) ;
#80620=CARTESIAN_POINT ( 'NONE',  ( -0.05219959533909027116, -19.03943276465977164, 102.4989096053143669 ) ) ;
#80621=ORIENTED_EDGE ( 'NONE', *, *, #125103, .F. ) ;
#80622=CARTESIAN_POINT ( 'NONE',  ( 4.483927247898790824, -16.52544592524335698, 60.20942372801902565 ) ) ;
#80623=CARTESIAN_POINT ( 'NONE',  ( -10.81492255796078084, -18.62759615963271287, 97.08224293864770971 ) ) ;
#80624=CARTESIAN_POINT ( 'NONE',  ( 5.049401038298161559, -19.05341960407611168, 47.70724293864770260 ) ) ;
#80625=CARTESIAN_POINT ( 'NONE',  ( 19.03943276465977164, 0.05219959533936151252, 71.25109039468566152 ) ) ;
#80626=CARTESIAN_POINT ( 'NONE',  ( 21.52544592524334988, 5.823673210054432836, 31.45942372801901854 ) ) ;
#80627=CARTESIAN_POINT ( 'NONE',  ( 19.02544592524343514, -5.153800228976328945, 68.54057627198103830 ) ) ;
#80628=CARTESIAN_POINT ( 'NONE',  ( -16.46253265017160317, 9.564922557960807481, 100.8322429386477097 ) ) ;
#80630=CARTESIAN_POINT ( 'NONE',  ( -12.06949235617739369, -12.14591786802326823, 34.37609039468568284 ) ) ;
#80631=CARTESIAN_POINT ( 'NONE',  ( -21.53943276465977519, -0.05219959533937600094, 23.75109039468567929 ) ) ;
#80632=CARTESIAN_POINT ( 'NONE',  ( -14.29746914071049879, 8.314922557960819915, 100.8322429386477097 ) ) ;
#80633=CARTESIAN_POINT ( 'NONE',  ( 9.564922557960805705, 16.46253265017160317, 89.58224293864769550 ) ) ;
#80634=CARTESIAN_POINT ( 'NONE',  ( 5.049401038297881783, 19.05341960407617563, 77.29275706135231871 ) ) ;
#80635=CARTESIAN_POINT ( 'NONE',  ( -21.55341960407610458, -5.719274019375992779, 91.45724293864769550 ) ) ;
#80636=CARTESIAN_POINT ( 'NONE',  ( 4.483927247898545687, 16.52544592524342804, 49.79057627198102409 ) ) ;
#80637=CARTESIAN_POINT ( 'NONE',  ( -19.02544592524334988, -5.153800228976617603, 18.95942372801899722 ) ) ;
#80638=CARTESIAN_POINT ( 'NONE',  ( -4.379528057220086978, -16.55341960407618274, 74.79275706135234714 ) ) ;
#80639=CARTESIAN_POINT ( 'NONE',  ( -19.02544592524342804, 5.153800228976336051, 106.0405762719810241 ) ) ;
#80640=CARTESIAN_POINT ( 'NONE',  ( -19.02544592524342804, 5.153800228976336051, 46.04057627198101699 ) ) ;
#80641=CARTESIAN_POINT ( 'NONE',  ( -5.823673210054431948, 21.52544592524334988, 52.70942372801902565 ) ) ;
#80642=CARTESIAN_POINT ( 'NONE',  ( -21.53943276465977519, -0.05219959533937600094, 73.75109039468567573 ) ) ;
#80643=CARTESIAN_POINT ( 'NONE',  ( -16.46253265017160317, 9.564922557960807481, 55.83224293864769550 ) ) ;
#80644=CARTESIAN_POINT ( 'NONE',  ( -21.52544592524334988, -5.823673210054445271, 48.95942372801902565 ) ) ;
#80645=ADVANCED_FACE ( 'NONE', ( #163536, #162521, #8854, #25036, #86679, #84667, #193881, #9858, #71517, #147365 ), #43447, .T. ) ;
#80646=CARTESIAN_POINT ( 'NONE',  ( 9.474510206698729675, 16.51473224551082808, 87.08442372801900433 ) ) ;
#80647=CARTESIAN_POINT ( 'NONE',  ( 13.89961937509977652, -13.97604488694527269, 38.12390960531436690 ) ) ;
#80648=CARTESIAN_POINT ( 'NONE',  ( 16.52544592524335698, 4.483927247898782831, 86.45942372801901854 ) ) ;
#80649=CARTESIAN_POINT ( 'NONE',  ( 0.05219959533909260263, 19.03943276465977164, 59.99890960531436690 ) ) ;
#80650=CARTESIAN_POINT ( 'NONE',  ( 5.049401038298161559, -19.05341960407611168, 112.7072429386476813 ) ) ;
#80651=CARTESIAN_POINT ( 'NONE',  ( -13.89961937509977652, 13.97604488694528158, 45.62390960531433848 ) ) ;
#80652=CARTESIAN_POINT ( 'NONE',  ( -5.719274019375978568, 21.55341960407610458, 85.20724293864770971 ) ) ;
#80653=CARTESIAN_POINT ( 'NONE',  ( -0.05219959533934338120, 16.53943276465976808, 67.50109039468568994 ) ) ;
#80655=CARTESIAN_POINT ( 'NONE',  ( 0.05219959533936267826, -19.03943276465977164, 25.00109039468566152 ) ) ;
#80656=CARTESIAN_POINT ( 'NONE',  ( -5.049401038298153566, 19.05341960407611168, 65.20724293864765286 ) ) ;
#80657=CARTESIAN_POINT ( 'NONE',  ( 16.52544592524342804, -4.483927247898539470, 53.54057627198103120 ) ) ;
#80658=CARTESIAN_POINT ( 'NONE',  ( -16.52544592524342804, 4.483927247898546575, 96.04057627198102409 ) ) ;
#80659=CARTESIAN_POINT ( 'NONE',  ( 16.51473224551069308, 9.474510206698969483, 104.1655762719810241 ) ) ;
#80660=CARTESIAN_POINT ( 'NONE',  ( -5.153800228976328057, -19.02544592524343514, 87.29057627198103830 ) ) ;
#80661=CARTESIAN_POINT ( 'NONE',  ( -21.55341960407619339, 5.719274019375674811, 53.54275706135234714 ) ) ;
#80662=CARTESIAN_POINT ( 'NONE',  ( 9.474510206698971260, -16.51473224551069308, 102.9155762719810241 ) ) ;
#80663=CARTESIAN_POINT ( 'NONE',  ( 15.80617190586769283, -15.72974639402175789, 110.6260903946857042 ) ) ;
#80664=CARTESIAN_POINT ( 'NONE',  ( 0.05219959533934541429, -16.53943276465976808, 85.00109039468568994 ) ) ;
#80665=CARTESIAN_POINT ( 'NONE',  ( -15.80617190586768217, 15.72974639402176855, 43.12609039468568284 ) ) ;
#80666=CARTESIAN_POINT ( 'NONE',  ( 19.05341960407611168, 5.049401038298154454, 108.9572429386477097 ) ) ;
#80667=CARTESIAN_POINT ( 'NONE',  ( 10.72451020669898902, -18.67979575497178502, 107.9155762719810241 ) ) ;
#80668=CARTESIAN_POINT ( 'NONE',  ( -0.05219959533910754901, -16.53943276465976808, 57.49890960531435979 ) ) ;
#80669=CARTESIAN_POINT ( 'NONE',  ( 13.89961937509977652, -13.97604488694527269, 53.12390960531434558 ) ) ;
#80670=CARTESIAN_POINT ( 'NONE',  ( -14.29746914071049879, 8.314922557960819915, 85.83224293864768129 ) ) ;
#80671=CARTESIAN_POINT ( 'NONE',  ( 18.62759615963271287, -10.81492255796078972, 28.33224293864769550 ) ) ;
#80672=CARTESIAN_POINT ( 'NONE',  ( 16.51473224551083163, -9.474510206698727899, 40.83442372801900433 ) ) ;
#80673=CARTESIAN_POINT ( 'NONE',  ( -16.53943276465976808, 0.05219959533911058130, 116.2489096053143669 ) ) ;
#80675=CARTESIAN_POINT ( 'NONE',  ( 14.29746914071037800, 8.314922557961029526, 61.66775706135235424 ) ) ;
#80676=CARTESIAN_POINT ( 'NONE',  ( -16.51473224551069308, -9.474510206698971260, 71.66557627198102409 ) ) ;
#80678=CARTESIAN_POINT ( 'NONE',  ( -12.14591786802309592, -12.06949235617757132, 91.87390960531436690 ) ) ;
#80679=CARTESIAN_POINT ( 'NONE',  ( -5.823673210054116645, -21.52544592524344225, 32.29057627198102409 ) ) ;
#80681=CARTESIAN_POINT ( 'NONE',  ( 12.06949235617739724, 12.14591786802326823, 101.8760903946857042 ) ) ;
#80682=CARTESIAN_POINT ( 'NONE',  ( -16.51473224551082808, 9.474510206698731452, 113.3344237280190043 ) ) ;
#80683=CARTESIAN_POINT ( 'NONE',  ( -0.05219959533937732626, 21.53943276465977519, 82.50109039468568994 ) ) ;
#80684=CARTESIAN_POINT ( 'NONE',  ( -5.153800228976328057, -19.02544592524343514, 92.29057627198099567 ) ) ;
#80685=CARTESIAN_POINT ( 'NONE',  ( -5.823673210054116645, -21.52544592524344225, 107.2905762719810525 ) ) ;
#80686=CARTESIAN_POINT ( 'NONE',  ( 16.52544592524335698, 4.483927247898782831, 61.45942372801901854 ) ) ;
#80687=CARTESIAN_POINT ( 'NONE',  ( 13.97604488694527802, 13.89961937509977652, 24.37390960531435624 ) ) ;
#80688=CARTESIAN_POINT ( 'NONE',  ( 12.06949235617739724, 12.14591786802326823, 36.87609039468568994 ) ) ;
#80689=CARTESIAN_POINT ( 'NONE',  ( -16.51473224551082808, 9.474510206698731452, 98.33442372801900433 ) ) ;
#80690=CARTESIAN_POINT ( 'NONE',  ( -15.72974639402197994, 15.80617190586746368, 85.62390960531436690 ) ) ;
#80691=CARTESIAN_POINT ( 'NONE',  ( 19.03943276465977164, 0.05219959533936151252, 61.25109039468566863 ) ) ;
#80693=CARTESIAN_POINT ( 'NONE',  ( 5.719274019375991003, -21.55341960407610458, 97.70724293864772392 ) ) ;
#80695=CARTESIAN_POINT ( 'NONE',  ( -9.564922557960796823, -16.46253265017161027, 82.08224293864768129 ) ) ;
#80696=CARTESIAN_POINT ( 'NONE',  ( -8.314922557961024197, 14.29746914071037800, 32.91775706135234714 ) ) ;
#80698=CARTESIAN_POINT ( 'NONE',  ( 16.46253265017146816, 9.564922557961045513, 56.66775706135233293 ) ) ;
#80699=CARTESIAN_POINT ( 'NONE',  ( -15.80617190586745835, -15.72974639402198527, 111.8739096053143669 ) ) ;
#80700=CARTESIAN_POINT ( 'NONE',  ( 12.06949235617757843, -12.14591786802309237, 58.12390960531435979 ) ) ;
#80701=CARTESIAN_POINT ( 'NONE',  ( -16.46253265017160317, 9.564922557960807481, 65.83224293864769550 ) ) ;
#80702=CARTESIAN_POINT ( 'NONE',  ( 16.53943276465976808, 0.05219959533934440121, 31.25109039468568639 ) ) ;
#80703=CARTESIAN_POINT ( 'NONE',  ( -16.51473224551082808, 9.474510206698731452, 48.33442372801900433 ) ) ;
#80704=CARTESIAN_POINT ( 'NONE',  ( 0.05219959533937995610, -21.53943276465977519, 50.00109039468568994 ) ) ;
#80705=CARTESIAN_POINT ( 'NONE',  ( 9.564922557961047289, -16.46253265017146816, 105.4177570613523471 ) ) ;
#80706=CARTESIAN_POINT ( 'NONE',  ( -16.51473224551069308, -9.474510206698971260, 56.66557627198103120 ) ) ;
#80707=CARTESIAN_POINT ( 'NONE',  ( -16.51473224551082808, 9.474510206698731452, 78.33442372801900433 ) ) ;
#80708=CARTESIAN_POINT ( 'NONE',  ( -5.823673210054431948, 21.52544592524334988, 87.70942372801901854 ) ) ;
#80709=CARTESIAN_POINT ( 'NONE',  ( -5.153800228976607833, 19.02544592524334988, 67.70942372801900433 ) ) ;
#80710=CARTESIAN_POINT ( 'NONE',  ( 16.46253265017160672, -9.564922557960803928, 43.33224293864769550 ) ) ;
#80711=CARTESIAN_POINT ( 'NONE',  ( 18.62759615963271287, -10.81492255796078972, 58.33224293864768839 ) ) ;
#80712=CARTESIAN_POINT ( 'NONE',  ( -12.14591786802309592, -12.06949235617757132, 61.87390960531436690 ) ) ;
#80713=CARTESIAN_POINT ( 'NONE',  ( 13.97604488694548053, -13.89961937509957401, 65.62609039468567573 ) ) ;
#80715=CARTESIAN_POINT ( 'NONE',  ( -0.05219959533936034679, 19.03943276465977164, 27.50109039468566507 ) ) ;
#80716=CARTESIAN_POINT ( 'NONE',  ( -16.53943276465976808, -0.05219959533934237506, 103.7510903946857042 ) ) ;
#80717=CARTESIAN_POINT ( 'NONE',  ( -4.483927247898539470, -16.52544592524342804, 52.29057627198102409 ) ) ;
#80718=CARTESIAN_POINT ( 'NONE',  ( 21.55341960407619695, -5.719274019375665929, 86.04275706135236135 ) ) ;
#80720=CARTESIAN_POINT ( 'NONE',  ( -18.67979575497193778, 10.72451020669871902, 88.33442372801901854 ) ) ;
#80721=CARTESIAN_POINT ( 'NONE',  ( -5.719274019375978568, 21.55341960407610458, 95.20724293864769550 ) ) ;
#80722=CARTESIAN_POINT ( 'NONE',  ( 0.05219959533909260263, 19.03943276465977164, 44.99890960531435979 ) ) ;
#80723=CARTESIAN_POINT ( 'NONE',  ( -21.52544592524334988, -5.823673210054445271, 68.95942372801901854 ) ) ;
#80724=CARTESIAN_POINT ( 'NONE',  ( -5.049401038298153566, 19.05341960407611168, 55.20724293864769550 ) ) ;
#80725=CARTESIAN_POINT ( 'NONE',  ( 19.03943276465977164, -0.05219959533909143690, 63.74890960531435979 ) ) ;
#80726=CARTESIAN_POINT ( 'NONE',  ( -4.483927247898539470, -16.52544592524342804, 107.2905762719810525 ) ) ;
#80727=CARTESIAN_POINT ( 'NONE',  ( -16.46253265017160317, 9.564922557960807481, 110.8322429386476955 ) ) ;
#80728=CARTESIAN_POINT ( 'NONE',  ( 0.05219959533910956823, 16.53943276465976808, 49.99890960531437401 ) ) ;
#80729=CARTESIAN_POINT ( 'NONE',  ( -0.05219959533909027116, -19.03943276465977164, 27.49890960531435624 ) ) ;
#80730=CARTESIAN_POINT ( 'NONE',  ( -12.14591786802309592, -12.06949235617757132, 81.87390960531435269 ) ) ;
#80731=CARTESIAN_POINT ( 'NONE',  ( 18.62759615963271287, -10.81492255796078972, 93.33224293864769550 ) ) ;
#80732=CARTESIAN_POINT ( 'NONE',  ( -0.05219959533937732626, 21.53943276465977519, 37.50109039468568284 ) ) ;
#80734=CARTESIAN_POINT ( 'NONE',  ( -14.34966873604972548, 8.224510206698743886, 33.33442372801900433 ) ) ;
#80735=CARTESIAN_POINT ( 'NONE',  ( 21.55341960407610458, 5.719274019375980345, 83.95724293864770971 ) ) ;
#80736=CARTESIAN_POINT ( 'NONE',  ( -16.46253265017146816, -9.564922557961047289, 19.16775706135233293 ) ) ;
#80737=CARTESIAN_POINT ( 'NONE',  ( 13.89961937509977652, -13.97604488694527269, 88.12390960531438111 ) ) ;
#80738=CARTESIAN_POINT ( 'NONE',  ( -15.72974639402176322, -15.80617190586768395, 39.37609039468567573 ) ) ;
#80740=CARTESIAN_POINT ( 'NONE',  ( -15.80617190586745835, -15.72974639402198527, 31.87390960531435979 ) ) ;
#80741=CARTESIAN_POINT ( 'NONE',  ( -8.224510206698735004, -14.34966873604973081, 104.5844237280190185 ) ) ;
#80742=CARTESIAN_POINT ( 'NONE',  ( 21.52544592524334988, 5.823673210054432836, 51.45942372801901854 ) ) ;
#80743=CARTESIAN_POINT ( 'NONE',  ( -10.72451020669870658, -18.67979575497194134, 84.58442372801903275 ) ) ;
#80744=CARTESIAN_POINT ( 'NONE',  ( 19.05341960407617918, -5.049401038297876454, 26.04275706135233293 ) ) ;
#80745=CARTESIAN_POINT ( 'NONE',  ( 16.53943276465976808, 0.05219959533934440121, 86.25109039468568994 ) ) ;
#80746=CARTESIAN_POINT ( 'NONE',  ( 18.62759615963255655, 10.81492255796105972, 41.66775706135235424 ) ) ;
#80747=CARTESIAN_POINT ( 'NONE',  ( -9.564922557960796823, -16.46253265017161027, 47.08224293864769550 ) ) ;
#80748=CARTESIAN_POINT ( 'NONE',  ( 10.81492255796106328, -18.62759615963255655, 100.4177570613523471 ) ) ;
#80749=CARTESIAN_POINT ( 'NONE',  ( 16.46253265017160672, -9.564922557960803928, 113.3322429386476955 ) ) ;
#80750=CARTESIAN_POINT ( 'NONE',  ( -18.62759615963270932, 10.81492255796079327, 100.8322429386477097 ) ) ;
#80751=AXIS2_PLACEMENT_3D ( 'NONE', #34102, #125116, #48284 ) ;
#80752=CARTESIAN_POINT ( 'NONE',  ( -21.55341960407610458, -5.719274019375992779, 66.45724293864768129 ) ) ;
#80754=CARTESIAN_POINT ( 'NONE',  ( 21.52544592524344225, -5.823673210054117533, 63.54057627198103830 ) ) ;
#80755=CARTESIAN_POINT ( 'NONE',  ( -12.14591786802326823, 12.06949235617739902, 48.12609039468568284 ) ) ;
#80756=CARTESIAN_POINT ( 'NONE',  ( -0.05219959533910754901, -16.53943276465976808, 62.49890960531436690 ) ) ;
#80758=CARTESIAN_POINT ( 'NONE',  ( 19.03943276465977164, 0.05219959533936151252, 96.25109039468567573 ) ) ;
#80760=CARTESIAN_POINT ( 'NONE',  ( 8.314922557961029526, -14.29746914071037800, 20.41775706135234714 ) ) ;
#80761=CARTESIAN_POINT ( 'NONE',  ( 10.81492255796078972, 18.62759615963270932, 94.58224293864769550 ) ) ;
#80762=CARTESIAN_POINT ( 'NONE',  ( 21.53943276465977519, -0.05219959533907433946, 73.74890960531433848 ) ) ;
#80763=CARTESIAN_POINT ( 'NONE',  ( 21.52544592524344225, -5.823673210054117533, 23.54057627198102765 ) ) ;
#80764=CARTESIAN_POINT ( 'NONE',  ( -4.379528057220086978, -16.55341960407618274, 54.79275706135235424 ) ) ;
#80765=CARTESIAN_POINT ( 'NONE',  ( 13.97604488694527802, 13.89961937509977652, 69.37390960531436690 ) ) ;
#80766=CARTESIAN_POINT ( 'NONE',  ( -0.05219959533937732626, 21.53943276465977519, 32.50109039468568284 ) ) ;
#80767=CARTESIAN_POINT ( 'NONE',  ( 5.153800228976615827, -19.02544592524334988, 105.2094237280190185 ) ) ;
#80768=CARTESIAN_POINT ( 'NONE',  ( -19.05341960407611168, -5.049401038298163336, 111.4572429386476671 ) ) ;
#80769=CARTESIAN_POINT ( 'NONE',  ( 13.89961937509977652, -13.97604488694527269, 83.12390960531436690 ) ) ;
#80770=CARTESIAN_POINT ( 'NONE',  ( 18.62759615963271287, -10.81492255796078972, 88.33224293864769550 ) ) ;
#80771=CARTESIAN_POINT ( 'NONE',  ( -19.02544592524342804, 5.153800228976336051, 56.04057627198100988 ) ) ;
#80772=CARTESIAN_POINT ( 'NONE',  ( -16.62475595723695676, -7.163666690055258357, 59.47286648189533054 ) ) ;
#80773=CARTESIAN_POINT ( 'NONE',  ( 0.05219959533910956823, 16.53943276465976808, 64.99890960531435269 ) ) ;
#80774=CARTESIAN_POINT ( 'NONE',  ( -19.02544592524342804, 5.153800228976336051, 116.0405762719810383 ) ) ;
#80776=CARTESIAN_POINT ( 'NONE',  ( 21.53943276465977519, -0.05219959533907433946, 108.7489096053143669 ) ) ;
#80777=CARTESIAN_POINT ( 'NONE',  ( 16.46253265017146816, 9.564922557961045513, 61.66775706135234003 ) ) ;
#80778=CARTESIAN_POINT ( 'NONE',  ( 19.02544592524343514, -5.153800228976328945, 113.5405762719810241 ) ) ;
#80779=CARTESIAN_POINT ( 'NONE',  ( -9.564922557960796823, -16.46253265017161027, 27.08224293864769550 ) ) ;
#80780=CARTESIAN_POINT ( 'NONE',  ( -18.67979575497178146, -10.72451020669898902, 51.66557627198102409 ) ) ;
#80781=AXIS2_PLACEMENT_3D ( 'NONE', #143089, #50111, #36909 ) ;
#80782=CARTESIAN_POINT ( 'NONE',  ( -0.05219959533909027116, -19.03943276465977164, 92.49890960531436690 ) ) ;
#80783=CARTESIAN_POINT ( 'NONE',  ( -21.52544592524334988, -5.823673210054445271, 78.95942372801901854 ) ) ;
#80784=CARTESIAN_POINT ( 'NONE',  ( -19.05341960407611168, -5.049401038298163336, 56.45724293864768129 ) ) ;
#80785=CARTESIAN_POINT ( 'NONE',  ( 4.379528057220339221, -16.55341960407611168, 82.70724293864770971 ) ) ;
#80786=CARTESIAN_POINT ( 'NONE',  ( 0.05219959533934541429, -16.53943276465976808, 40.00109039468567573 ) ) ;
#80787=CARTESIAN_POINT ( 'NONE',  ( -10.72451020669870658, -18.67979575497194134, 59.58442372801901854 ) ) ;
#80789=CARTESIAN_POINT ( 'NONE',  ( -19.03943276465977164, -0.05219959533935918106, 28.75109039468566507 ) ) ;
#80790=CARTESIAN_POINT ( 'NONE',  ( -0.05219959533936034679, 19.03943276465977164, 77.50109039468566152 ) ) ;
#80791=CARTESIAN_POINT ( 'NONE',  ( -0.05219959533936034679, 19.03943276465977164, 42.50109039468566152 ) ) ;
#80792=CARTESIAN_POINT ( 'NONE',  ( 15.50000000000000178, -5.500000000000000888, 118.0000000000000142 ) ) ;
#80793=CARTESIAN_POINT ( 'NONE',  ( 15.80617190586769283, -15.72974639402175789, 35.62609039468568994 ) ) ;
#80795=CARTESIAN_POINT ( 'NONE',  ( 19.05341960407617918, -5.049401038297876454, 31.04275706135232227 ) ) ;
#80796=CARTESIAN_POINT ( 'NONE',  ( -16.46253265017160317, 9.564922557960807481, 50.83224293864770260 ) ) ;
#80797=CARTESIAN_POINT ( 'NONE',  ( 9.474510206698729675, 16.51473224551082808, 27.08442372801900433 ) ) ;
#80798=CARTESIAN_POINT ( 'NONE',  ( 14.29746914071037800, 8.314922557961029526, 101.6677570613523613 ) ) ;
#80799=CARTESIAN_POINT ( 'NONE',  ( 5.153800228976335163, 19.02544592524342804, 109.7905762719810099 ) ) ;
#80800=CARTESIAN_POINT ( 'NONE',  ( 0.05219959533937995610, -21.53943276465977519, 85.00109039468568994 ) ) ;
#80803=CARTESIAN_POINT ( 'NONE',  ( -10.81492255796105439, 18.62759615963255655, 87.91775706135234714 ) ) ;
#80805=CARTESIAN_POINT ( 'NONE',  ( 0.05219959533909260263, 19.03943276465977164, 99.99890960531436690 ) ) ;
#80806=CARTESIAN_POINT ( 'NONE',  ( 5.049401038298161559, -19.05341960407611168, 52.70724293864767418 ) ) ;
#80807=CARTESIAN_POINT ( 'NONE',  ( -15.80617190586745835, -15.72974639402198527, 56.87390960531436690 ) ) ;
#80808=CARTESIAN_POINT ( 'NONE',  ( -4.379528057220328563, 16.55341960407611168, 25.20724293864769550 ) ) ;
#80809=CARTESIAN_POINT ( 'NONE',  ( -0.05219959533910754901, -16.53943276465976808, 102.4989096053143811 ) ) ;
#80810=CARTESIAN_POINT ( 'NONE',  ( 19.02544592524343514, -5.153800228976328945, 93.54057627198102409 ) ) ;
#80811=CARTESIAN_POINT ( 'NONE',  ( -21.55341960407619339, 5.719274019375674811, 113.5427570613523756 ) ) ;
#80812=ADVANCED_FACE ( 'NONE', ( #99958 ), #13896, .T. ) ;
#80813=CARTESIAN_POINT ( 'NONE',  ( -16.46253265017160317, 9.564922557960807481, 30.83224293864769550 ) ) ;
#80814=CARTESIAN_POINT ( 'NONE',  ( -14.34966873604960291, -8.224510206698953496, 101.6655762719810383 ) ) ;
#80815=CARTESIAN_POINT ( 'NONE',  ( -5.719274019375665041, -21.55341960407619695, 59.79275706135234714 ) ) ;
#80816=CARTESIAN_POINT ( 'NONE',  ( 16.52544592524335698, 4.483927247898782831, 111.4594237280190328 ) ) ;
#80817=CARTESIAN_POINT ( 'NONE',  ( 5.049401038297881783, 19.05341960407617563, 67.29275706135234714 ) ) ;
#80819=CARTESIAN_POINT ( 'NONE',  ( 19.05341960407611168, 5.049401038298154454, 108.9572429386477097 ) ) ;
#80820=CARTESIAN_POINT ( 'NONE',  ( 8.224510206698953496, -14.34966873604960469, 82.91557627198103830 ) ) ;
#80821=CARTESIAN_POINT ( 'NONE',  ( -19.03943276465977164, -0.05219959533935918106, 53.75109039468566863 ) ) ;
#80822=CARTESIAN_POINT ( 'NONE',  ( -5.153800228976328057, -19.02544592524343514, 67.29057627198102409 ) ) ;
#80823=CARTESIAN_POINT ( 'NONE',  ( 14.34966873604960469, 8.224510206698951720, 59.16557627198103120 ) ) ;
#80824=CARTESIAN_POINT ( 'NONE',  ( -19.03943276465977164, -0.05219959533935918106, 93.75109039468566152 ) ) ;
#80825=CARTESIAN_POINT ( 'NONE',  ( 21.53943276465977519, -0.05219959533907433946, 38.74890960531435979 ) ) ;
#80828=CARTESIAN_POINT ( 'NONE',  ( -8.314922557960811034, -14.29746914071050412, 102.0822429386476955 ) ) ;
#80829=CARTESIAN_POINT ( 'NONE',  ( -18.22780087662123805, -5.499999999999968026, 98.98236817873106475 ) ) ;
#80830=CARTESIAN_POINT ( 'NONE',  ( 9.564922557960805705, 16.46253265017160317, 59.58224293864769550 ) ) ;
#80831=CARTESIAN_POINT ( 'NONE',  ( -21.53943276465977519, 0.05219959533907696930, 61.24890960531435979 ) ) ;
#80832=CARTESIAN_POINT ( 'NONE',  ( 19.05341960407611168, 5.049401038298154454, 38.95724293864767418 ) ) ;
#80833=CARTESIAN_POINT ( 'NONE',  ( -16.52544592524335698, -4.483927247898792601, 93.95942372801903275 ) ) ;
#80834=CARTESIAN_POINT ( 'NONE',  ( -9.474510206698964154, 16.51473224551069663, 75.41557627198103830 ) ) ;
#80835=CARTESIAN_POINT ( 'NONE',  ( 5.049401038297881783, 19.05341960407617563, 57.29275706135231871 ) ) ;
#80836=CARTESIAN_POINT ( 'NONE',  ( -21.55341960407619339, 5.719274019375674811, 73.54275706135234714 ) ) ;
#80837=CARTESIAN_POINT ( 'NONE',  ( -15.72974639402197994, 15.80617190586746368, 45.62390960531436690 ) ) ;
#80838=CARTESIAN_POINT ( 'NONE',  ( 19.03943276465977164, -0.05219959533909143690, 108.7489096053143527 ) ) ;
#80839=CARTESIAN_POINT ( 'NONE',  ( 19.05341960407611168, 5.049401038298154454, 23.95724293864769194 ) ) ;
#80840=CARTESIAN_POINT ( 'NONE',  ( 16.52544592524335698, 4.483927247898782831, 81.45942372801900433 ) ) ;
#80841=CARTESIAN_POINT ( 'NONE',  ( -5.153800228976607833, 19.02544592524334988, 102.7094237280189759 ) ) ;
#80843=CARTESIAN_POINT ( 'NONE',  ( 19.53091890409951858, 5.500000000000028422, 77.56097431831419442 ) ) ;
#80844=CARTESIAN_POINT ( 'NONE',  ( -18.62759615963255300, -10.81492255796106328, 99.16775706135234714 ) ) ;
#80846=CARTESIAN_POINT ( 'NONE',  ( -14.29746914071049879, 8.314922557960819915, 65.83224293864769550 ) ) ;
#80847=CARTESIAN_POINT ( 'NONE',  ( -4.483927247898539470, -16.52544592524342804, 72.29057627198102409 ) ) ;
#80848=CARTESIAN_POINT ( 'NONE',  ( 10.72451020669898902, -18.67979575497178502, 97.91557627198103830 ) ) ;
#80849=CARTESIAN_POINT ( 'NONE',  ( 15.72974639402199770, -15.80617190586745480, 83.12390960531436690 ) ) ;
#80851=CARTESIAN_POINT ( 'NONE',  ( 10.72451020669898902, -18.67979575497178502, 32.91557627198102409 ) ) ;
#80852=CARTESIAN_POINT ( 'NONE',  ( -0.05219959533934338120, 16.53943276465976808, 67.50109039468568994 ) ) ;
#80853=CARTESIAN_POINT ( 'NONE',  ( -16.55341960407611168, -4.379528057220339221, 91.45724293864769550 ) ) ;
#80854=CARTESIAN_POINT ( 'NONE',  ( 19.02544592524343514, -5.153800228976328945, 43.54057627198103120 ) ) ;
#80857=CARTESIAN_POINT ( 'NONE',  ( -12.14591786802326823, 12.06949235617739902, 98.12609039468570415 ) ) ;
#80858=CARTESIAN_POINT ( 'NONE',  ( -21.53943276465977519, -0.05219959533937600094, 33.75109039468568284 ) ) ;
#80859=CARTESIAN_POINT ( 'NONE',  ( 16.51473224551069308, 9.474510206698969483, 79.16557627198103830 ) ) ;
#80860=CARTESIAN_POINT ( 'NONE',  ( 15.72974639402176855, 15.80617190586768217, 71.87609039468568994 ) ) ;
#80863=ORIENTED_EDGE ( 'NONE', *, *, #127587, .F. ) ;
#80864=CARTESIAN_POINT ( 'NONE',  ( -18.67979575497193778, 10.72451020669871902, 53.33442372801901854 ) ) ;
#80865=CARTESIAN_POINT ( 'NONE',  ( 19.05341960407611168, 5.049401038298154454, 33.95724293864769550 ) ) ;
#80867=CARTESIAN_POINT ( 'NONE',  ( 19.05341960407611168, 5.049401038298154454, 88.95724293864769550 ) ) ;
#80868=CARTESIAN_POINT ( 'NONE',  ( 9.474510206698729675, 16.51473224551082808, 67.08442372801900433 ) ) ;
#80869=CARTESIAN_POINT ( 'NONE',  ( -10.81492255796105439, 18.62759615963255655, 22.91775706135235069 ) ) ;
#80870=CARTESIAN_POINT ( 'NONE',  ( -19.05341960407617563, 5.049401038297882671, 63.54275706135234003 ) ) ;
#80871=CARTESIAN_POINT ( 'NONE',  ( 5.049401038298161559, -19.05341960407611168, 22.70724293864769194 ) ) ;
#80872=CARTESIAN_POINT ( 'NONE',  ( -0.05219959533934338120, 16.53943276465976808, 102.5010903946856899 ) ) ;
#80873=CARTESIAN_POINT ( 'NONE',  ( 0.05219959533936267826, -19.03943276465977164, 65.00109039468567573 ) ) ;
#80874=CARTESIAN_POINT ( 'NONE',  ( 16.52544592524342804, -4.483927247898539470, 23.54057627198102765 ) ) ;
#80875=CARTESIAN_POINT ( 'NONE',  ( 16.51473224551083163, -9.474510206698727899, 50.83442372801899722 ) ) ;
#80876=CARTESIAN_POINT ( 'NONE',  ( 13.89961937509977652, -13.97604488694527269, 83.12390960531436690 ) ) ;
#80877=CARTESIAN_POINT ( 'NONE',  ( -21.52544592524334988, -5.823673210054445271, 93.95942372801903275 ) ) ;
#80878=CARTESIAN_POINT ( 'NONE',  ( 5.719274019375673035, 21.55341960407619339, 107.2927570613523471 ) ) ;
#80880=CARTESIAN_POINT ( 'NONE',  ( 18.62759615963255655, 10.81492255796105972, 91.66775706135234714 ) ) ;
#80881=CARTESIAN_POINT ( 'NONE',  ( -8.314922557961024197, 14.29746914071037800, 37.91775706135235424 ) ) ;
#80882=CARTESIAN_POINT ( 'NONE',  ( 16.46253265017160672, -9.564922557960803928, 93.33224293864769550 ) ) ;
#80883=CARTESIAN_POINT ( 'NONE',  ( 15.80617190586746368, 15.72974639402197994, 24.37390960531435979 ) ) ;
#80885=CARTESIAN_POINT ( 'NONE',  ( 5.153800228976335163, 19.02544592524342804, 84.79057627198099567 ) ) ;
#80886=CARTESIAN_POINT ( 'NONE',  ( -18.87255363501902394, -5.499999999999949374, 41.32513748171826506 ) ) ;
#80887=CARTESIAN_POINT ( 'NONE',  ( 16.46253265017146816, 9.564922557961045513, 71.66775706135233293 ) ) ;
#80888=CARTESIAN_POINT ( 'NONE',  ( 16.46253265017160672, -9.564922557960803928, 108.3322429386476955 ) ) ;
#80889=CARTESIAN_POINT ( 'NONE',  ( -5.719274019375665041, -21.55341960407619695, 104.7927570613523898 ) ) ;
#80890=CARTESIAN_POINT ( 'NONE',  ( -12.14591786802309592, -12.06949235617757132, 101.8739096053143811 ) ) ;
#80891=CARTESIAN_POINT ( 'NONE',  ( -5.823673210054116645, -21.52544592524344225, 52.29057627198102409 ) ) ;
#80892=CARTESIAN_POINT ( 'NONE',  ( -21.53943276465977519, 0.05219959533907696930, 41.24890960531435269 ) ) ;
#80893=CARTESIAN_POINT ( 'NONE',  ( 8.224510206698953496, -14.34966873604960469, 107.9155762719810241 ) ) ;
#80894=DIRECTION ( 'NONE',  ( 0.000000000000000000, 0.000000000000000000, -1.000000000000000000 ) ) ;
#80895=CARTESIAN_POINT ( 'NONE',  ( -13.97604488694547697, 13.89961937509957934, 63.12609039468566152 ) ) ;
#80896=CARTESIAN_POINT ( 'NONE',  ( 16.53943276465976808, -0.05219959533910856209, 23.74890960531435269 ) ) ;
#80897=CARTESIAN_POINT ( 'NONE',  ( 0.05219959533909260263, 19.03943276465977164, 99.99890960531436690 ) ) ;
#80898=CARTESIAN_POINT ( 'NONE',  ( -0.05219959533937732626, 21.53943276465977519, 77.50109039468567573 ) ) ;
#80899=CARTESIAN_POINT ( 'NONE',  ( -18.67979575497178146, -10.72451020669898902, 66.66557627198102409 ) ) ;
#80900=CARTESIAN_POINT ( 'NONE',  ( -21.52544592524334988, -5.823673210054445271, 38.95942372801901854 ) ) ;
#80901=CARTESIAN_POINT ( 'NONE',  ( -15.72974639402197994, 15.80617190586746368, 90.62390960531436690 ) ) ;
#80902=CARTESIAN_POINT ( 'NONE',  ( 21.53943276465977519, 0.05219959533937863772, 56.25109039468568284 ) ) ;
#80903=CARTESIAN_POINT ( 'NONE',  ( -13.89961937509977652, 13.97604488694528158, 25.62390960531434558 ) ) ;
#80904=CARTESIAN_POINT ( 'NONE',  ( -19.03943276465977164, 0.05219959533909376836, 86.24890960531436690 ) ) ;
#80905=CARTESIAN_POINT ( 'NONE',  ( 4.483927247898790824, -16.52544592524335698, 80.20942372801901854 ) ) ;
#80906=CARTESIAN_POINT ( 'NONE',  ( -14.29746914071049879, 8.314922557960819915, 105.8322429386476955 ) ) ;
#80907=CARTESIAN_POINT ( 'NONE',  ( -13.97604488694527625, -13.89961937509977652, 101.8739096053143811 ) ) ;
#80908=CARTESIAN_POINT ( 'NONE',  ( 16.55341960407611168, 4.379528057220329451, 58.95724293864770971 ) ) ;
#80909=CARTESIAN_POINT ( 'NONE',  ( -14.34966873604960291, -8.224510206698953496, 26.66557627198103475 ) ) ;
#80910=CARTESIAN_POINT ( 'NONE',  ( -16.51473224551069308, -9.474510206698971260, 51.66557627198102409 ) ) ;
#80911=CARTESIAN_POINT ( 'NONE',  ( 5.153800228976335163, 19.02544592524342804, 34.79057627198102409 ) ) ;
#80912=CARTESIAN_POINT ( 'NONE',  ( 5.823673210054125526, 21.52544592524343514, 44.79057627198103120 ) ) ;
#80913=CARTESIAN_POINT ( 'NONE',  ( -19.03943276465977164, -0.05219959533935918106, 23.75109039468566152 ) ) ;
#80915=CARTESIAN_POINT ( 'NONE',  ( 14.34966873604960469, 8.224510206698951720, 34.16557627198102409 ) ) ;
#80917=CARTESIAN_POINT ( 'NONE',  ( 15.80617190586769283, -15.72974639402175789, 45.62609039468567573 ) ) ;
#80919=CARTESIAN_POINT ( 'NONE',  ( 16.52544592524335698, 4.483927247898782831, 56.45942372801902565 ) ) ;
#80920=CARTESIAN_POINT ( 'NONE',  ( 5.153800228976615827, -19.02544592524334988, 60.20942372801899012 ) ) ;
#80921=CARTESIAN_POINT ( 'NONE',  ( -16.52544592524342804, 4.483927247898546575, 31.04057627198102409 ) ) ;
#80922=CARTESIAN_POINT ( 'NONE',  ( -12.14591786802326823, 12.06949235617739902, 108.1260903946856757 ) ) ;
#80923=CARTESIAN_POINT ( 'NONE',  ( 13.89961937509977652, -13.97604488694527269, 33.12390960531434558 ) ) ;
#80924=CARTESIAN_POINT ( 'NONE',  ( 9.564922557960805705, 16.46253265017160317, 64.58224293864769550 ) ) ;
#80925=CARTESIAN_POINT ( 'NONE',  ( -0.05219959533909027116, -19.03943276465977164, 32.49890960531435979 ) ) ;
#80926=CARTESIAN_POINT ( 'NONE',  ( -21.52544592524334988, -5.823673210054445271, 28.95942372801902209 ) ) ;
#80927=CARTESIAN_POINT ( 'NONE',  ( -19.05341960407611168, -5.049401038298163336, 46.45724293864768129 ) ) ;
#80929=CARTESIAN_POINT ( 'NONE',  ( -9.474510206698964154, 16.51473224551069663, 40.41557627198103120 ) ) ;
#80930=EDGE_CURVE ( 'NONE', #127622, #56210, #85071, .T. ) ;
#80931=CARTESIAN_POINT ( 'NONE',  ( 5.719274019375991003, -21.55341960407610458, 27.70724293864769905 ) ) ;
#80932=CARTESIAN_POINT ( 'NONE',  ( -15.72974639402176322, -15.80617190586768395, 64.37609039468568994 ) ) ;
#80933=CARTESIAN_POINT ( 'NONE',  ( 8.314922557960818139, 14.29746914071049879, 104.5822429386477097 ) ) ;
#80934=CARTESIAN_POINT ( 'NONE',  ( -13.89961937509977652, 13.97604488694528158, 115.6239096053143669 ) ) ;
#80935=CARTESIAN_POINT ( 'NONE',  ( 16.52544592524335698, 4.483927247898782831, 81.45942372801900433 ) ) ;
#80936=CARTESIAN_POINT ( 'NONE',  ( -15.72974639402176322, -15.80617190586768395, 89.37609039468568994 ) ) ;
#80937=CARTESIAN_POINT ( 'NONE',  ( 4.379528057220092307, 16.55341960407617563, 52.29275706135236135 ) ) ;
#80938=CARTESIAN_POINT ( 'NONE',  ( 9.564922557960805705, 16.46253265017160317, 89.58224293864769550 ) ) ;
#80940=CARTESIAN_POINT ( 'NONE',  ( 0.05219959533934541429, -16.53943276465976808, 35.00109039468568284 ) ) ;
#80941=CARTESIAN_POINT ( 'NONE',  ( 0.05219959533934541429, -16.53943276465976808, 30.00109039468568284 ) ) ;
#80942=CARTESIAN_POINT ( 'NONE',  ( 0.05219959533934541429, -16.53943276465976808, 95.00109039468568994 ) ) ;
#80943=CARTESIAN_POINT ( 'NONE',  ( -9.474510206698720793, -16.51473224551083518, 104.5844237280190043 ) ) ;
#80944=CARTESIAN_POINT ( 'NONE',  ( 15.80617190586746368, 15.72974639402197994, 99.37390960531436690 ) ) ;
#80945=CARTESIAN_POINT ( 'NONE',  ( -16.55341960407611168, -4.379528057220339221, 101.4572429386476955 ) ) ;
#80946=CARTESIAN_POINT ( 'NONE',  ( 5.153800228976615827, -19.02544592524334988, 100.2094237280190043 ) ) ;
#80947=CARTESIAN_POINT ( 'NONE',  ( -16.55341960407617563, 4.379528057220093196, 73.54275706135234714 ) ) ;
#80949=CARTESIAN_POINT ( 'NONE',  ( 16.51473224551083163, -9.474510206698727899, 75.83442372801900433 ) ) ;
#80950=CARTESIAN_POINT ( 'NONE',  ( -16.55341960407611168, -4.379528057220339221, 51.45724293864770260 ) ) ;
#80951=CARTESIAN_POINT ( 'NONE',  ( 14.34966873604960469, 8.224510206698951720, 29.16557627198103120 ) ) ;
#80952=CARTESIAN_POINT ( 'NONE',  ( -16.55341960407611168, -4.379528057220339221, 91.45724293864769550 ) ) ;
#80953=CARTESIAN_POINT ( 'NONE',  ( -5.049401038297874678, -19.05341960407617918, 39.79275706135232582 ) ) ;
#80954=CARTESIAN_POINT ( 'NONE',  ( -16.88567814943162659, 6.947325034625692730, 88.70998877347416567 ) ) ;
#80955=CARTESIAN_POINT ( 'NONE',  ( 21.55341960407619695, -5.719274019375665929, 36.04275706135234714 ) ) ;
#80956=CARTESIAN_POINT ( 'NONE',  ( -19.05341960407617563, 5.049401038297882671, 93.54275706135234714 ) ) ;
#80958=CARTESIAN_POINT ( 'NONE',  ( 16.46253265017160672, -9.564922557960803928, 88.33224293864769550 ) ) ;
#80959=CARTESIAN_POINT ( 'NONE',  ( 9.564922557960805705, 16.46253265017160317, 94.58224293864769550 ) ) ;
#80960=CARTESIAN_POINT ( 'NONE',  ( -15.72974639402197994, 15.80617190586746368, 55.62390960531436690 ) ) ;
#80961=CARTESIAN_POINT ( 'NONE',  ( 8.314922557960818139, 14.29746914071049879, 89.58224293864768129 ) ) ;
#80962=CARTESIAN_POINT ( 'NONE',  ( 0.05219959533909260263, 19.03943276465977164, 74.99890960531435269 ) ) ;
#80963=CARTESIAN_POINT ( 'NONE',  ( -13.89961937509977652, 13.97604488694528158, 30.62390960531435269 ) ) ;
#80964=CARTESIAN_POINT ( 'NONE',  ( 18.62759615963255655, 10.81492255796105972, 36.66775706135234714 ) ) ;
#80965=CARTESIAN_POINT ( 'NONE',  ( -10.72451020669870658, -18.67979575497194134, 74.58442372801901854 ) ) ;
#80966=CARTESIAN_POINT ( 'NONE',  ( -13.97604488694527625, -13.89961937509977652, 61.87390960531435979 ) ) ;
#80967=CARTESIAN_POINT ( 'NONE',  ( 16.53943276465976808, 0.05219959533934440121, 76.25109039468568994 ) ) ;
#80968=CARTESIAN_POINT ( 'NONE',  ( -10.81492255796105439, 18.62759615963255655, 32.91775706135234714 ) ) ;
#80969=CARTESIAN_POINT ( 'NONE',  ( 10.81492255796106328, -18.62759615963255655, 20.41775706135234714 ) ) ;
#80970=CARTESIAN_POINT ( 'NONE',  ( -16.51473224551082808, 9.474510206698731452, 48.33442372801900433 ) ) ;
#80971=CARTESIAN_POINT ( 'NONE',  ( 9.474510206698971260, -16.51473224551069308, 77.91557627198103830 ) ) ;
#80972=CARTESIAN_POINT ( 'NONE',  ( 13.89961937509957401, 13.97604488694547697, 36.87609039468565442 ) ) ;
#80973=CARTESIAN_POINT ( 'NONE',  ( -5.823673210054431948, 21.52544592524334988, 87.70942372801901854 ) ) ;
#80975=CARTESIAN_POINT ( 'NONE',  ( 0.05219959533907565091, 21.53943276465977519, 69.99890960531435269 ) ) ;
#80976=CARTESIAN_POINT ( 'NONE',  ( -14.34966873604960291, -8.224510206698953496, 51.66557627198102409 ) ) ;
#80977=CARTESIAN_POINT ( 'NONE',  ( 18.62759615963255655, 10.81492255796105972, 96.66775706135234714 ) ) ;
#80978=CARTESIAN_POINT ( 'NONE',  ( 16.46253265017146816, 9.564922557961045513, 26.66775706135234003 ) ) ;
#80979=CARTESIAN_POINT ( 'NONE',  ( 12.06949235617757843, -12.14591786802309237, 68.12390960531436690 ) ) ;
#80980=CARTESIAN_POINT ( 'NONE',  ( -16.51473224551069308, -9.474510206698971260, 26.66557627198103120 ) ) ;
#80981=CARTESIAN_POINT ( 'NONE',  ( -5.049401038297874678, -19.05341960407617918, 74.79275706135231871 ) ) ;
#80982=CARTESIAN_POINT ( 'NONE',  ( -0.05219959533910754901, -16.53943276465976808, 32.49890960531435979 ) ) ;
#80983=CARTESIAN_POINT ( 'NONE',  ( -0.05219959533937732626, 21.53943276465977519, 82.50109039468568994 ) ) ;
#80984=CARTESIAN_POINT ( 'NONE',  ( 19.05341960407611168, 5.049401038298154454, 73.95724293864768129 ) ) ;
#80985=CARTESIAN_POINT ( 'NONE',  ( -13.97604488694547697, 13.89961937509957934, 53.12609039468565442 ) ) ;
#80986=CARTESIAN_POINT ( 'NONE',  ( 18.62759615963271287, -10.81492255796078972, 53.33224293864769550 ) ) ;
#80987=CARTESIAN_POINT ( 'NONE',  ( 10.81492255796078972, 18.62759615963270932, 109.5822429386476955 ) ) ;
#80988=CARTESIAN_POINT ( 'NONE',  ( -13.97604488694547697, 13.89961937509957934, 108.1260903946856331 ) ) ;
#80989=CARTESIAN_POINT ( 'NONE',  ( -16.53943276465976808, -0.05219959533934237506, 68.75109039468568994 ) ) ;
#80991=CARTESIAN_POINT ( 'NONE',  ( -15.72974639402197994, 15.80617190586746368, 105.6239096053143669 ) ) ;
#80992=CARTESIAN_POINT ( 'NONE',  ( -0.05219959533910754901, -16.53943276465976808, 102.4989096053143811 ) ) ;
#80993=CARTESIAN_POINT ( 'NONE',  ( -17.49999999999999645, -3.189878218039150504, 30.12948562571235556 ) ) ;
#80994=CARTESIAN_POINT ( 'NONE',  ( 12.06949235617739724, 12.14591786802326823, 31.87609039468567929 ) ) ;
#80995=CARTESIAN_POINT ( 'NONE',  ( -0.05219959533907301413, -21.53943276465977519, 67.49890960531436690 ) ) ;
#80996=CARTESIAN_POINT ( 'NONE',  ( 12.14591786802327356, -12.06949235617739191, 100.6260903946857184 ) ) ;
#80997=CARTESIAN_POINT ( 'NONE',  ( -16.46253265017160317, 9.564922557960807481, 35.83224293864768839 ) ) ;
#80999=CARTESIAN_POINT ( 'NONE',  ( 4.483927247898790824, -16.52544592524335698, 65.20942372801901854 ) ) ;
#81000=CARTESIAN_POINT ( 'NONE',  ( 0.05219959533936267826, -19.03943276465977164, 65.00109039468567573 ) ) ;
#81001=CARTESIAN_POINT ( 'NONE',  ( 21.52544592524334988, 5.823673210054432836, 46.45942372801901854 ) ) ;
#81002=CARTESIAN_POINT ( 'NONE',  ( 21.53943276465977519, -0.05219959533907433946, 53.74890960531437401 ) ) ;
#81003=CARTESIAN_POINT ( 'NONE',  ( -14.29746914071037622, -8.314922557961029526, 99.16775706135234714 ) ) ;
#81004=CARTESIAN_POINT ( 'NONE',  ( 21.52544592524334988, 5.823673210054432836, 81.45942372801900433 ) ) ;
#81005=CARTESIAN_POINT ( 'NONE',  ( 5.823673210054125526, 21.52544592524343514, 49.79057627198102409 ) ) ;
#81006=CARTESIAN_POINT ( 'NONE',  ( 15.80617190586746368, 15.72974639402197994, 29.37390960531435269 ) ) ;
#81007=CARTESIAN_POINT ( 'NONE',  ( -16.52544592524335698, -4.483927247898792601, 73.95942372801901854 ) ) ;
#81008=CARTESIAN_POINT ( 'NONE',  ( -0.05219959533907301413, -21.53943276465977519, 42.49890960531435979 ) ) ;
#81010=CARTESIAN_POINT ( 'NONE',  ( -19.05341960407611168, -5.049401038298163336, 101.4572429386476955 ) ) ;
#81012=CARTESIAN_POINT ( 'NONE',  ( -9.474510206698964154, 16.51473224551069663, 25.41557627198103120 ) ) ;
#81013=CARTESIAN_POINT ( 'NONE',  ( 15.80617190586746368, 15.72974639402197994, 64.37390960531435269 ) ) ;
#81014=CARTESIAN_POINT ( 'NONE',  ( 16.53943276465976808, 0.05219959533934440121, 86.25109039468568994 ) ) ;
#81015=CARTESIAN_POINT ( 'NONE',  ( -0.05219959533937732626, 21.53943276465977519, 42.50109039468567573 ) ) ;
#81016=CARTESIAN_POINT ( 'NONE',  ( 0.05219959533936267826, -19.03943276465977164, 110.0010903946856757 ) ) ;
#81017=CARTESIAN_POINT ( 'NONE',  ( 14.34966873604960469, 8.224510206698951720, 99.16557627198100988 ) ) ;
#81018=CARTESIAN_POINT ( 'NONE',  ( 19.05341960407617918, -5.049401038297876454, 111.0427570613523329 ) ) ;
#81019=CARTESIAN_POINT ( 'NONE',  ( -19.02544592524342804, 5.153800228976336051, 41.04057627198103120 ) ) ;
#81021=CARTESIAN_POINT ( 'NONE',  ( -13.89961937509977652, 13.97604488694528158, 90.62390960531432427 ) ) ;
#81022=CARTESIAN_POINT ( 'NONE',  ( 4.379528057220092307, 16.55341960407617563, 72.29275706135236135 ) ) ;
#81023=CARTESIAN_POINT ( 'NONE',  ( -15.72974639402176322, -15.80617190586768395, 104.3760903946856899 ) ) ;
#81024=CARTESIAN_POINT ( 'NONE',  ( 21.52544592524344225, -5.823673210054117533, 68.54057627198103830 ) ) ;
#81025=CARTESIAN_POINT ( 'NONE',  ( 12.14591786802327356, -12.06949235617739191, 85.62609039468568994 ) ) ;
#81026=CARTESIAN_POINT ( 'NONE',  ( 0.05219959533936267826, -19.03943276465977164, 85.00109039468567573 ) ) ;
#81027=CARTESIAN_POINT ( 'NONE',  ( -19.02544592524342804, 5.153800228976336051, 36.04057627198100988 ) ) ;
#81028=CARTESIAN_POINT ( 'NONE',  ( -16.46253265017160317, 9.564922557960807481, 75.83224293864769550 ) ) ;
#81029=CARTESIAN_POINT ( 'NONE',  ( -19.05341960407611168, -5.049401038298163336, 36.45724293864766707 ) ) ;
#81030=CARTESIAN_POINT ( 'NONE',  ( -0.05219959533936034679, 19.03943276465977164, 77.50109039468566152 ) ) ;
#81032=CARTESIAN_POINT ( 'NONE',  ( -9.474510206698964154, 16.51473224551069663, 95.41557627198102409 ) ) ;
#81033=CARTESIAN_POINT ( 'NONE',  ( -4.379528057220328563, 16.55341960407611168, 55.20724293864770260 ) ) ;
#81034=CARTESIAN_POINT ( 'NONE',  ( -10.81492255796078084, -18.62759615963271287, 67.08224293864770971 ) ) ;
#81035=CARTESIAN_POINT ( 'NONE',  ( -17.49999999999998579, 3.512728167236896848, 105.2280999518112168 ) ) ;
#81036=CARTESIAN_POINT ( 'NONE',  ( 13.97604488694548053, -13.89961937509957401, 25.62609039468566507 ) ) ;
#81038=CARTESIAN_POINT ( 'NONE',  ( 19.05341960407611168, 5.049401038298154454, 68.95724293864769550 ) ) ;
#81039=CARTESIAN_POINT ( 'NONE',  ( 16.46253265017160672, -9.564922557960803928, 73.33224293864769550 ) ) ;
#81040=CARTESIAN_POINT ( 'NONE',  ( -16.53943276465976808, -0.05219959533934237506, 38.75109039468567573 ) ) ;
#81043=CARTESIAN_POINT ( 'NONE',  ( 16.55341960407618274, -4.379528057220086978, 81.04275706135236135 ) ) ;
#81044=CARTESIAN_POINT ( 'NONE',  ( 16.55341960407618274, -4.379528057220086978, 71.04275706135234714 ) ) ;
#81045=CARTESIAN_POINT ( 'NONE',  ( -15.72974639402197994, 15.80617190586746368, 90.62390960531436690 ) ) ;
#81046=CARTESIAN_POINT ( 'NONE',  ( 14.34966873604972726, -8.224510206698740333, 40.83442372801901854 ) ) ;
#81047=CARTESIAN_POINT ( 'NONE',  ( 19.05341960407611168, 5.049401038298154454, 43.95724293864769550 ) ) ;
#81049=CARTESIAN_POINT ( 'NONE',  ( -21.53943276465977519, -0.05219959533937600094, 48.75109039468568284 ) ) ;
#81050=CARTESIAN_POINT ( 'NONE',  ( 5.049401038297881783, 19.05341960407617563, 57.29275706135231871 ) ) ;
#81051=CARTESIAN_POINT ( 'NONE',  ( 21.55341960407619695, -5.719274019375665929, 91.04275706135236135 ) ) ;
#81052=CARTESIAN_POINT ( 'NONE',  ( -19.05341960407611168, -5.049401038298163336, 31.45724293864769550 ) ) ;
#81054=CARTESIAN_POINT ( 'NONE',  ( 10.81492255796078972, 18.62759615963270932, 54.58224293864769550 ) ) ;
#81055=CARTESIAN_POINT ( 'NONE',  ( -9.474510206698964154, 16.51473224551069663, 100.4155762719810241 ) ) ;
#81056=CARTESIAN_POINT ( 'NONE',  ( 4.379528057220339221, -16.55341960407611168, 107.7072429386476955 ) ) ;
#81057=CARTESIAN_POINT ( 'NONE',  ( -14.29746914071037622, -8.314922557961029526, 34.16775706135234714 ) ) ;
#81058=CARTESIAN_POINT ( 'NONE',  ( -4.483927247898782831, 16.52544592524335698, 107.7094237280190328 ) ) ;
#81060=CARTESIAN_POINT ( 'NONE',  ( -5.719274019375978568, 21.55341960407610458, 105.2072429386477097 ) ) ;
#81061=CARTESIAN_POINT ( 'NONE',  ( 4.483927247898545687, 16.52544592524342804, 44.79057627198103120 ) ) ;
#81062=CARTESIAN_POINT ( 'NONE',  ( 13.89961937509957401, 13.97604488694547697, 96.87609039468566152 ) ) ;
#81063=CARTESIAN_POINT ( 'NONE',  ( -19.02544592524334988, -5.153800228976617603, 28.95942372801900433 ) ) ;
#81064=CARTESIAN_POINT ( 'NONE',  ( 4.483927247898545687, 16.52544592524342804, 24.79057627198103120 ) ) ;
#81065=CARTESIAN_POINT ( 'NONE',  ( -0.05219959533907301413, -21.53943276465977519, 92.49890960531436690 ) ) ;
#81066=CARTESIAN_POINT ( 'NONE',  ( -18.62759615963270932, 10.81492255796079327, 50.83224293864770971 ) ) ;
#81067=CARTESIAN_POINT ( 'NONE',  ( 0.05219959533909260263, 19.03943276465977164, 59.99890960531436690 ) ) ;
#81068=CARTESIAN_POINT ( 'NONE',  ( -16.53943276465976808, 0.05219959533911058130, 41.24890960531435269 ) ) ;
#81069=CARTESIAN_POINT ( 'NONE',  ( -13.89961937509977652, 13.97604488694528158, 95.62390960531436690 ) ) ;
#81071=CARTESIAN_POINT ( 'NONE',  ( 19.05341960407617918, -5.049401038297876454, 41.04275706135233293 ) ) ;
#81072=CARTESIAN_POINT ( 'NONE',  ( -15.72974639402197994, 15.80617190586746368, 75.62390960531439532 ) ) ;
#81073=CARTESIAN_POINT ( 'NONE',  ( -4.379528057220328563, 16.55341960407611168, 100.2072429386476955 ) ) ;
#81074=CARTESIAN_POINT ( 'NONE',  ( -21.55341960407619339, 5.719274019375674811, 43.54275706135235424 ) ) ;
#81076=CARTESIAN_POINT ( 'NONE',  ( 14.34966873604972726, -8.224510206698740333, 110.8344237280190043 ) ) ;
#81077=CARTESIAN_POINT ( 'NONE',  ( 5.153800228976335163, 19.02544592524342804, 34.79057627198102409 ) ) ;
#81078=CARTESIAN_POINT ( 'NONE',  ( 19.02544592524343514, -5.153800228976328945, 88.54057627198102409 ) ) ;
#81080=CARTESIAN_POINT ( 'NONE',  ( -16.46253265017160317, 9.564922557960807481, 30.83224293864769550 ) ) ;
#81081=CARTESIAN_POINT ( 'NONE',  ( 8.314922557960818139, 14.29746914071049879, 39.58224293864769550 ) ) ;
#81083=CARTESIAN_POINT ( 'NONE',  ( 0.05219959533937995610, -21.53943276465977519, 80.00109039468568994 ) ) ;
#81085=CARTESIAN_POINT ( 'NONE',  ( -16.55341960407617563, 4.379528057220093196, 73.54275706135234714 ) ) ;
#81086=CARTESIAN_POINT ( 'NONE',  ( -5.049401038298153566, 19.05341960407611168, 60.20724293864768129 ) ) ;
#81087=CARTESIAN_POINT ( 'NONE',  ( 19.02544592524343514, -5.153800228976328945, 68.54057627198103830 ) ) ;
#81089=CARTESIAN_POINT ( 'NONE',  ( -10.81492255796105439, 18.62759615963255655, 112.9177570613523329 ) ) ;
#81090=CARTESIAN_POINT ( 'NONE',  ( 4.379528057220092307, 16.55341960407617563, 72.29275706135236135 ) ) ;
#81091=CARTESIAN_POINT ( 'NONE',  ( 5.823673210054444382, -21.52544592524334988, 105.2094237280190328 ) ) ;
#81092=CARTESIAN_POINT ( 'NONE',  ( 13.97604488694527802, 13.89961937509977652, 64.37390960531436690 ) ) ;
#81093=CARTESIAN_POINT ( 'NONE',  ( 5.823673210054125526, 21.52544592524343514, 39.79057627198103830 ) ) ;
#81094=CARTESIAN_POINT ( 'NONE',  ( -16.46253265017146816, -9.564922557961047289, 109.1677570613523471 ) ) ;
#81095=CARTESIAN_POINT ( 'NONE',  ( -15.80617190586768217, 15.72974639402176855, 63.12609039468568994 ) ) ;
#81096=CARTESIAN_POINT ( 'NONE',  ( -12.06949235617739369, -12.14591786802326823, 54.37609039468568994 ) ) ;
#81097=CARTESIAN_POINT ( 'NONE',  ( -18.62759615963270932, 10.81492255796079327, 95.83224293864770971 ) ) ;
#81098=CARTESIAN_POINT ( 'NONE',  ( -13.97604488694547697, 13.89961937509957934, 93.12609039468566152 ) ) ;
#81099=CARTESIAN_POINT ( 'NONE',  ( -9.474510206698964154, 16.51473224551069663, 80.41557627198103830 ) ) ;
#81100=CARTESIAN_POINT ( 'NONE',  ( 9.474510206698729675, 16.51473224551082808, 107.0844237280190043 ) ) ;
#81101=CARTESIAN_POINT ( 'NONE',  ( 19.05341960407617918, -5.049401038297876454, 96.04275706135231871 ) ) ;
#81102=CARTESIAN_POINT ( 'NONE',  ( 0.05219959533910956823, 16.53943276465976808, 59.99890960531436690 ) ) ;
#81103=CARTESIAN_POINT ( 'NONE',  ( -8.314922557961024197, 14.29746914071037800, 77.91775706135231871 ) ) ;
#81104=CARTESIAN_POINT ( 'NONE',  ( -10.72451020669898014, 18.67979575497178502, 110.4155762719810383 ) ) ;
#81105=CARTESIAN_POINT ( 'NONE',  ( 9.474510206698971260, -16.51473224551069308, 52.91557627198102409 ) ) ;
#81106=CARTESIAN_POINT ( 'NONE',  ( -5.049401038298153566, 19.05341960407611168, 60.20724293864768129 ) ) ;
#81107=CARTESIAN_POINT ( 'NONE',  ( -16.53943276465976808, -0.05219959533934237506, 68.75109039468568994 ) ) ;
#81109=CARTESIAN_POINT ( 'NONE',  ( 13.89961937509957401, 13.97604488694547697, 21.87609039468566152 ) ) ;
#81110=CARTESIAN_POINT ( 'NONE',  ( -16.46253265017160317, 9.564922557960807481, 30.83224293864769550 ) ) ;
#81112=CARTESIAN_POINT ( 'NONE',  ( -0.05219959533936034679, 19.03943276465977164, 107.5010903946856615 ) ) ;
#81113=CARTESIAN_POINT ( 'NONE',  ( 19.02544592524334988, 5.153800228976608722, 46.45942372801899012 ) ) ;
#81114=CARTESIAN_POINT ( 'NONE',  ( -4.379528057220086978, -16.55341960407618274, 29.79275706135234358 ) ) ;
#81115=CARTESIAN_POINT ( 'NONE',  ( 13.89961937509977652, -13.97604488694527269, 38.12390960531436690 ) ) ;
#81116=CARTESIAN_POINT ( 'NONE',  ( 9.564922557960805705, 16.46253265017160317, 64.58224293864769550 ) ) ;
#81117=CARTESIAN_POINT ( 'NONE',  ( -15.72974639402197994, 15.80617190586746368, 90.62390960531436690 ) ) ;
#81118=CARTESIAN_POINT ( 'NONE',  ( 19.03943276465977164, -0.05219959533909143690, 113.7489096053143669 ) ) ;
#81119=CARTESIAN_POINT ( 'NONE',  ( 16.46253265017160672, -9.564922557960803928, 48.33224293864769550 ) ) ;
#81121=CARTESIAN_POINT ( 'NONE',  ( -9.564922557961040184, 16.46253265017147172, 102.9177570613523329 ) ) ;
#81122=CARTESIAN_POINT ( 'NONE',  ( 8.224510206698953496, -14.34966873604960469, 67.91557627198102409 ) ) ;
#81123=CARTESIAN_POINT ( 'NONE',  ( -0.05219959533936034679, 19.03943276465977164, 22.50109039468566152 ) ) ;
#81124=CARTESIAN_POINT ( 'NONE',  ( -8.314922557960811034, -14.29746914071050412, 67.08224293864770971 ) ) ;
#81125=CARTESIAN_POINT ( 'NONE',  ( 15.72974639402176855, 15.80617190586768217, 81.87609039468568994 ) ) ;
#81126=CARTESIAN_POINT ( 'NONE',  ( -9.474510206698964154, 16.51473224551069663, 25.41557627198103120 ) ) ;
#81127=CARTESIAN_POINT ( 'NONE',  ( -10.72451020669870658, -18.67979575497194134, 84.58442372801903275 ) ) ;
#81128=CARTESIAN_POINT ( 'NONE',  ( 14.29746914071049879, -8.314922557960816363, 28.33224293864769550 ) ) ;
#81129=CARTESIAN_POINT ( 'NONE',  ( 10.81492255796106328, -18.62759615963255655, 75.41775706135233293 ) ) ;
#81130=CARTESIAN_POINT ( 'NONE',  ( 19.02544592524343514, -5.153800228976328945, 78.54057627198099567 ) ) ;
#81131=CARTESIAN_POINT ( 'NONE',  ( -15.80617190586768217, 15.72974639402176855, 38.12609039468567573 ) ) ;
#81132=CARTESIAN_POINT ( 'NONE',  ( -5.153800228976328057, -19.02544592524343514, 87.29057627198103830 ) ) ;
#81133=CARTESIAN_POINT ( 'NONE',  ( 4.483927247898545687, 16.52544592524342804, 99.79057627198103830 ) ) ;
#81134=CARTESIAN_POINT ( 'NONE',  ( -12.14591786802309592, -12.06949235617757132, 56.87390960531436690 ) ) ;
#81135=CARTESIAN_POINT ( 'NONE',  ( -18.67979575497178146, -10.72451020669898902, 66.66557627198102409 ) ) ;
#81136=CARTESIAN_POINT ( 'NONE',  ( 19.05341960407611168, 5.049401038298154454, 78.95724293864769550 ) ) ;
#81137=CARTESIAN_POINT ( 'NONE',  ( 15.80617190586746368, 15.72974639402197994, 84.37390960531438111 ) ) ;
#81138=CARTESIAN_POINT ( 'NONE',  ( 9.564922557961047289, -16.46253265017146816, 70.41775706135233293 ) ) ;
#81139=CARTESIAN_POINT ( 'NONE',  ( -13.97604488694547520, 13.89961937509957934, 33.12609039468566152 ) ) ;
#81140=CARTESIAN_POINT ( 'NONE',  ( -16.52544592524342804, 4.483927247898546575, 76.04057627198102409 ) ) ;
#81141=CARTESIAN_POINT ( 'NONE',  ( 21.52544592524344225, -5.823673210054117533, 48.54057627198103120 ) ) ;
#81143=CARTESIAN_POINT ( 'NONE',  ( -14.34966873604972548, 8.224510206698743886, 103.3344237280190043 ) ) ;
#81145=CARTESIAN_POINT ( 'NONE',  ( -0.05219959533936034679, 19.03943276465977164, 97.50109039468567573 ) ) ;
#81146=CARTESIAN_POINT ( 'NONE',  ( 12.06949235617757843, -12.14591786802309237, 63.12390960531435979 ) ) ;
#81147=CARTESIAN_POINT ( 'NONE',  ( -17.50000000000002132, 3.237210098469563313, 34.71236987379540295 ) ) ;
#81148=CARTESIAN_POINT ( 'NONE',  ( -9.474510206698964154, 16.51473224551069663, 60.41557627198102409 ) ) ;
#81149=CARTESIAN_POINT ( 'NONE',  ( 16.53943276465976808, -0.05219959533910856209, 53.74890960531437401 ) ) ;
#81150=CARTESIAN_POINT ( 'NONE',  ( -16.51473224551069308, -9.474510206698971260, 101.6655762719810241 ) ) ;
#81151=CARTESIAN_POINT ( 'NONE',  ( -19.02544592524334988, -5.153800228976617603, 78.95942372801900433 ) ) ;
#81152=CARTESIAN_POINT ( 'NONE',  ( -19.02544592524342804, 5.153800228976336051, 71.04057627198099567 ) ) ;
#81153=CARTESIAN_POINT ( 'NONE',  ( 16.51473224551069308, 9.474510206698969483, 79.16557627198103830 ) ) ;
#81154=CARTESIAN_POINT ( 'NONE',  ( -19.02544592524342804, 5.153800228976336051, 86.04057627198103830 ) ) ;
#81155=CARTESIAN_POINT ( 'NONE',  ( -5.719274019375978568, 21.55341960407610458, 65.20724293864768129 ) ) ;
#81156=CARTESIAN_POINT ( 'NONE',  ( 8.224510206698742110, 14.34966873604972548, 52.08442372801901854 ) ) ;
#81157=CARTESIAN_POINT ( 'NONE',  ( -5.153800228976607833, 19.02544592524335343, 102.7094237280189901 ) ) ;
#81158=CARTESIAN_POINT ( 'NONE',  ( 16.46253265017160672, -9.564922557960803928, 48.33224293864769550 ) ) ;
#81159=CARTESIAN_POINT ( 'NONE',  ( -15.80617190586745835, -15.72974639402198527, 56.87390960531436690 ) ) ;
#81160=CARTESIAN_POINT ( 'NONE',  ( 9.564922557961047289, -16.46253265017146816, 100.4177570613523329 ) ) ;
#81161=CARTESIAN_POINT ( 'NONE',  ( -8.224510206698948167, 14.34966873604960824, 25.41557627198103120 ) ) ;
#81162=CARTESIAN_POINT ( 'NONE',  ( 18.62759615963255655, 10.81492255796105972, 41.66775706135235424 ) ) ;
#81163=CARTESIAN_POINT ( 'NONE',  ( 13.89961937509957401, 13.97604488694547697, 41.87609039468566152 ) ) ;
#81164=CARTESIAN_POINT ( 'NONE',  ( 16.55341960407618274, -4.379528057220086978, 61.04275706135234714 ) ) ;
#81165=CARTESIAN_POINT ( 'NONE',  ( 8.314922557961029526, -14.29746914071037800, 100.4177570613523471 ) ) ;
#81167=CARTESIAN_POINT ( 'NONE',  ( 8.314922557961029526, -14.29746914071037800, 85.41775706135236135 ) ) ;
#81168=CARTESIAN_POINT ( 'NONE',  ( -14.29746914071037622, -8.314922557961029526, 34.16775706135234714 ) ) ;
#81169=CARTESIAN_POINT ( 'NONE',  ( 9.474510206698971260, -16.51473224551069308, 47.91557627198102409 ) ) ;
#81170=CARTESIAN_POINT ( 'NONE',  ( -5.049401038298153566, 19.05341960407611168, 45.20724293864769550 ) ) ;
#81171=CARTESIAN_POINT ( 'NONE',  ( -9.474510206698964154, 16.51473224551069663, 65.41557627198102409 ) ) ;
#81172=CARTESIAN_POINT ( 'NONE',  ( -10.81492255796105439, 18.62759615963255655, 57.91775706135234714 ) ) ;
#81173=CARTESIAN_POINT ( 'NONE',  ( -16.55341960407617563, 4.379528057220093196, 53.54275706135234714 ) ) ;
#81174=CARTESIAN_POINT ( 'NONE',  ( 4.483927247898790824, -16.52544592524335698, 110.2094237280190185 ) ) ;
#81175=CARTESIAN_POINT ( 'NONE',  ( -16.51473224551069308, -9.474510206698971260, 26.66557627198103120 ) ) ;
#81176=CARTESIAN_POINT ( 'NONE',  ( 10.81492255796106328, -18.62759615963255655, 110.4177570613523756 ) ) ;
#81177=CARTESIAN_POINT ( 'NONE',  ( 5.153800228976615827, -19.02544592524334988, 105.2094237280190185 ) ) ;
#81178=CARTESIAN_POINT ( 'NONE',  ( -13.89961937509957401, -13.97604488694547875, 79.37609039468567573 ) ) ;
#81179=CARTESIAN_POINT ( 'NONE',  ( -12.14591786802309592, -12.06949235617757132, 86.87390960531438111 ) ) ;
#81180=CARTESIAN_POINT ( 'NONE',  ( -9.564922557960796823, -16.46253265017161027, 42.08224293864769550 ) ) ;
#81181=CARTESIAN_POINT ( 'NONE',  ( -19.02544592524334988, -5.153800228976617603, 68.95942372801896170 ) ) ;
#81183=CARTESIAN_POINT ( 'NONE',  ( 15.72974639402176855, 15.80617190586768217, 81.87609039468568994 ) ) ;
#81184=CARTESIAN_POINT ( 'NONE',  ( -8.224510206698735004, -14.34966873604973081, 44.58442372801901854 ) ) ;
#81185=CARTESIAN_POINT ( 'NONE',  ( -17.49999999999999645, 3.189878218039151392, 24.87051437428774747 ) ) ;
#81186=CARTESIAN_POINT ( 'NONE',  ( 15.80617190586746368, 15.72974639402197994, 39.37390960531436690 ) ) ;
#81187=CARTESIAN_POINT ( 'NONE',  ( -16.52544592524335698, -4.483927247898792601, 28.95942372801902209 ) ) ;
#81188=CARTESIAN_POINT ( 'NONE',  ( 9.564922557960805705, 16.46253265017160317, 24.58224293864769194 ) ) ;
#81189=CARTESIAN_POINT ( 'NONE',  ( 9.564922557961047289, -16.46253265017146816, 25.41775706135234003 ) ) ;
#81191=CARTESIAN_POINT ( 'NONE',  ( 9.474510206698971260, -16.51473224551069308, 42.91557627198103120 ) ) ;
#81192=CARTESIAN_POINT ( 'NONE',  ( 17.58332526062528345, 7.635886036038587399, 56.57665040441533932 ) ) ;
#81193=CARTESIAN_POINT ( 'NONE',  ( -19.03943276465977164, 0.05219959533909376836, 76.24890960531435269 ) ) ;
#81194=CARTESIAN_POINT ( 'NONE',  ( 17.49999999999999645, -4.013004640162573189, 112.9460572099440725 ) ) ;
#81195=CARTESIAN_POINT ( 'NONE',  ( 5.823673210054444382, -21.52544592524334988, 110.2094237280190185 ) ) ;
#81196=CARTESIAN_POINT ( 'NONE',  ( -16.52544592524342804, 4.483927247898546575, 36.04057627198102409 ) ) ;
#81197=CARTESIAN_POINT ( 'NONE',  ( 16.51473224551069308, 9.474510206698969483, 39.16557627198103120 ) ) ;
#81198=CARTESIAN_POINT ( 'NONE',  ( -13.89961937509977652, 13.97604488694528158, 95.62390960531436690 ) ) ;
#81199=CARTESIAN_POINT ( 'NONE',  ( -21.52544592524334988, -5.823673210054445271, 63.95942372801901854 ) ) ;
#81200=CARTESIAN_POINT ( 'NONE',  ( -0.05219959533909027116, -19.03943276465977164, 52.49890960531436690 ) ) ;
#81201=CARTESIAN_POINT ( 'NONE',  ( 5.823673210054444382, -21.52544592524334988, 60.20942372801902565 ) ) ;
#81202=CARTESIAN_POINT ( 'NONE',  ( 18.67979575497178502, 10.72451020669898547, 29.16557627198103120 ) ) ;
#81203=CARTESIAN_POINT ( 'NONE',  ( 9.564922557960805705, 16.46253265017160317, 29.58224293864769550 ) ) ;
#81204=CARTESIAN_POINT ( 'NONE',  ( 21.53943276465977519, -0.05219959533907433946, 108.7489096053143669 ) ) ;
#81205=CARTESIAN_POINT ( 'NONE',  ( 13.97604488694548053, -13.89961937509957401, 45.62609039468566863 ) ) ;
#81206=CARTESIAN_POINT ( 'NONE',  ( 4.483927247898545687, 16.52544592524342804, 109.7905762719810383 ) ) ;
#81207=CARTESIAN_POINT ( 'NONE',  ( -19.05341960407611168, -5.049401038298163336, 56.45724293864768129 ) ) ;
#81208=CARTESIAN_POINT ( 'NONE',  ( 16.52544592524335698, 4.483927247898782831, 21.45942372801901499 ) ) ;
#81209=CARTESIAN_POINT ( 'NONE',  ( -4.483927247898539470, -16.52544592524342804, 77.29057627198102409 ) ) ;
#81210=CARTESIAN_POINT ( 'NONE',  ( -9.564922557960796823, -16.46253265017161027, 112.0822429386476955 ) ) ;
#81211=CARTESIAN_POINT ( 'NONE',  ( -9.564922557961040184, 16.46253265017147172, 87.91775706135233293 ) ) ;
#81212=CARTESIAN_POINT ( 'NONE',  ( -10.72451020669898014, 18.67979575497178502, 110.4155762719810383 ) ) ;
#81213=CARTESIAN_POINT ( 'NONE',  ( -21.53943276465977519, -0.05219959533937600094, 53.75109039468568994 ) ) ;
#81214=CARTESIAN_POINT ( 'NONE',  ( 0.05219959533934541429, -16.53943276465976808, 55.00109039468568284 ) ) ;
#81215=CARTESIAN_POINT ( 'NONE',  ( 14.34966873604972726, -8.224510206698740333, 60.83442372801901854 ) ) ;
#81216=CARTESIAN_POINT ( 'NONE',  ( 21.52544592524344225, -5.823673210054117533, 48.54057627198103120 ) ) ;
#81217=CARTESIAN_POINT ( 'NONE',  ( -13.97604488694527625, -13.89961937509977652, 51.87390960531436690 ) ) ;
#81219=CARTESIAN_POINT ( 'NONE',  ( -16.52544592524335698, -4.483927247898792601, 78.95942372801901854 ) ) ;
#81220=CARTESIAN_POINT ( 'NONE',  ( 18.62759615963271287, -10.81492255796078972, 98.33224293864769550 ) ) ;
#81221=CARTESIAN_POINT ( 'NONE',  ( -16.53943276465976808, 0.05219959533911058130, 56.24890960531436690 ) ) ;
#81222=CARTESIAN_POINT ( 'NONE',  ( -19.03943276465977164, 0.05219959533909376836, 66.24890960531436690 ) ) ;
#81223=CARTESIAN_POINT ( 'NONE',  ( 12.06949235617739724, 12.14591786802326823, 76.87609039468567573 ) ) ;
#81224=CARTESIAN_POINT ( 'NONE',  ( 9.474510206698729675, 16.51473224551082808, 102.0844237280190043 ) ) ;
#81225=CARTESIAN_POINT ( 'NONE',  ( -18.67979575497178146, -10.72451020669898902, 96.66557627198102409 ) ) ;
#81226=CARTESIAN_POINT ( 'NONE',  ( 4.379528057220339221, -16.55341960407611168, 42.70724293864770260 ) ) ;
#81228=CARTESIAN_POINT ( 'NONE',  ( -16.61371651742602396, 7.165104196376146817, 68.85415069992998838 ) ) ;
#81229=CARTESIAN_POINT ( 'NONE',  ( 5.719274019375991003, -21.55341960407610458, 77.70724293864770971 ) ) ;
#81230=CARTESIAN_POINT ( 'NONE',  ( -14.34966873604960291, -8.224510206698953496, 21.66557627198102409 ) ) ;
#81232=CARTESIAN_POINT ( 'NONE',  ( -16.38665767535054485, -7.295008042176057472, 54.73599135785457293 ) ) ;
#81233=CARTESIAN_POINT ( 'NONE',  ( 10.72451020669898902, -18.67979575497178502, 107.9155762719810241 ) ) ;
#81234=CARTESIAN_POINT ( 'NONE',  ( 5.823673210054444382, -21.52544592524334988, 25.20942372801901854 ) ) ;
#81235=CARTESIAN_POINT ( 'NONE',  ( 16.53943276465976808, -0.05219959533910856209, 43.74890960531435979 ) ) ;
#81236=CARTESIAN_POINT ( 'NONE',  ( -8.314922557961024197, 14.29746914071037800, 52.91775706135235424 ) ) ;
#81237=CARTESIAN_POINT ( 'NONE',  ( -19.05341960407611168, -5.049401038298163336, 51.45724293864770260 ) ) ;
#81238=CARTESIAN_POINT ( 'NONE',  ( -19.02544592524342804, 5.153800228976336051, 76.04057627198102409 ) ) ;
#81239=ORIENTED_EDGE ( 'NONE', *, *, #76155, .F. ) ;
#81240=CARTESIAN_POINT ( 'NONE',  ( -21.55341960407610458, -5.719274019375992779, 31.45724293864769550 ) ) ;
#81242=CARTESIAN_POINT ( 'NONE',  ( 12.06949235617739724, 12.14591786802326823, 26.87609039468567218 ) ) ;
#81243=CARTESIAN_POINT ( 'NONE',  ( -19.05341960407617563, 5.049401038297882671, 48.54275706135233293 ) ) ;
#81244=CARTESIAN_POINT ( 'NONE',  ( 15.72974639402199770, -15.80617190586745480, 103.1239096053143811 ) ) ;
#81245=CARTESIAN_POINT ( 'NONE',  ( 0.05219959533910956823, 16.53943276465976808, 39.99890960531436690 ) ) ;
#81246=CARTESIAN_POINT ( 'NONE',  ( 9.474510206698971260, -16.51473224551069308, 72.91557627198102409 ) ) ;
#81247=CARTESIAN_POINT ( 'NONE',  ( 5.823673210054125526, 21.52544592524343514, 64.79057627198103830 ) ) ;
#81248=CARTESIAN_POINT ( 'NONE',  ( 18.67979575497178502, 10.72451020669898547, 99.16557627198100988 ) ) ;
#81249=CARTESIAN_POINT ( 'NONE',  ( 14.34966873604972726, -8.224510206698740333, 30.83442372801902209 ) ) ;
#81250=CARTESIAN_POINT ( 'NONE',  ( 5.153800228976335163, 19.02544592524342804, 114.7905762719810241 ) ) ;
#81251=CARTESIAN_POINT ( 'NONE',  ( -21.52544592524334988, -5.823673210054445271, 83.95942372801900433 ) ) ;
#81252=CARTESIAN_POINT ( 'NONE',  ( -9.474510206698964154, 16.51473224551069663, 80.41557627198103830 ) ) ;
#81253=CARTESIAN_POINT ( 'NONE',  ( 13.97604488694527802, 13.89961937509977652, 24.37390960531435624 ) ) ;
#81254=CARTESIAN_POINT ( 'NONE',  ( -0.05219959533909027116, -19.03943276465977164, 87.49890960531436690 ) ) ;
#81255=CARTESIAN_POINT ( 'NONE',  ( -16.52544592524342804, 4.483927247898546575, 106.0405762719810525 ) ) ;
#81256=B_SPLINE_CURVE_WITH_KNOTS ( 'NONE', 3,
 ( #51259, #174614, #20914, #190772, #52247, #175602, #191762, #130063, #113904, #114922, #38090, #99745, #171284, #65083, #80247, #142909, #77272, #4391, #19585, #63095, #81228, #127741, #172269, #97387, #47949, #2418, #93427, #17601, #66075, #170284, #16607, #46947 ),
 .UNSPECIFIED., .F., .F.,
 ( 4, 2, 2, 2, 2, 2, 2, 2, 2, 2, 2, 2, 2, 2, 2, 4 ),
 ( 2.367436813247751133E-17, 0.0003712461730036969152, 0.0007424923460073700864, 0.001113738519011043312, 0.001484984692014716537, 0.002227477038022056266, 0.002598723211025725805, 0.002969969384029395344, 0.003341215557033064450, 0.003712461730036733989, 0.004083707903040402661, 0.004454954076044071766, 0.004826200249047740871, 0.005197446422051409977, 0.005568692595055079950, 0.005939938768058749055 ),
 .UNSPECIFIED. ) ;
#81257=CARTESIAN_POINT ( 'NONE',  ( -5.049401038297874678, -19.05341960407617918, 99.79275706135234714 ) ) ;
#81258=CARTESIAN_POINT ( 'NONE',  ( 17.50000000000000000, 5.500000000000001776, 33.78230962303567253 ) ) ;
#81259=CARTESIAN_POINT ( 'NONE',  ( 5.049401038298161559, -19.05341960407611168, 77.70724293864765286 ) ) ;
#81260=CARTESIAN_POINT ( 'NONE',  ( 0.05219959533937995610, -21.53943276465977519, 95.00109039468568994 ) ) ;
#81261=CARTESIAN_POINT ( 'NONE',  ( 5.823673210054125526, 21.52544592524343514, 24.79057627198103120 ) ) ;
#81262=CARTESIAN_POINT ( 'NONE',  ( 16.55341960407618274, -4.379528057220086978, 96.04275706135236135 ) ) ;
#81264=CARTESIAN_POINT ( 'NONE',  ( -19.02544592524334988, -5.153800228976617603, 58.95942372801900433 ) ) ;
#81265=CARTESIAN_POINT ( 'NONE',  ( -13.89961937509957401, -13.97604488694547875, 19.37609039468566507 ) ) ;
#81267=CARTESIAN_POINT ( 'NONE',  ( -0.05219959533909027116, -19.03943276465977164, 22.49890960531436690 ) ) ;
#81268=CARTESIAN_POINT ( 'NONE',  ( -12.06949235617756955, 12.14591786802309770, 25.62390960531435624 ) ) ;
#81270=CARTESIAN_POINT ( 'NONE',  ( 4.379528057220092307, 16.55341960407617563, 107.2927570613523471 ) ) ;
#81272=CARTESIAN_POINT ( 'NONE',  ( -8.314922557961024197, 14.29746914071037800, 82.91775706135234714 ) ) ;
#81273=CARTESIAN_POINT ( 'NONE',  ( -19.05341960407611168, -5.049401038298163336, 26.45724293864769550 ) ) ;
#81274=CARTESIAN_POINT ( 'NONE',  ( -10.72451020669870658, -18.67979575497194134, 99.58442372801900433 ) ) ;
#81275=CARTESIAN_POINT ( 'NONE',  ( -13.97604488694547697, 13.89961937509957934, 103.1260903946856473 ) ) ;
#81276=CARTESIAN_POINT ( 'NONE',  ( 5.823673210054444382, -21.52544592524334988, 65.20942372801901854 ) ) ;
#81277=CARTESIAN_POINT ( 'NONE',  ( 5.153800228976615827, -19.02544592524334988, 35.20942372801899722 ) ) ;
#81278=CARTESIAN_POINT ( 'NONE',  ( 19.03943276465977164, -0.05219959533909143690, 83.74890960531436690 ) ) ;
#81279=CARTESIAN_POINT ( 'NONE',  ( -0.05219959533909027116, -19.03943276465977164, 72.49890960531435269 ) ) ;
#81280=CARTESIAN_POINT ( 'NONE',  ( 17.44270441346519362, 5.991230190322990978, 73.86335079264227943 ) ) ;
#81281=CARTESIAN_POINT ( 'NONE',  ( 15.80617190586746368, 15.72974639402197994, 49.37390960531436690 ) ) ;
#81282=CARTESIAN_POINT ( 'NONE',  ( -9.474510206698964154, 16.51473224551069663, 45.41557627198103120 ) ) ;
#81283=CARTESIAN_POINT ( 'NONE',  ( 18.67979575497178502, 10.72451020669898547, 84.16557627198103830 ) ) ;
#81284=CARTESIAN_POINT ( 'NONE',  ( 12.06949235617739724, 12.14591786802326823, 81.87609039468568994 ) ) ;
#81286=CARTESIAN_POINT ( 'NONE',  ( -14.29746914071049879, 8.314922557960819915, 85.83224293864768129 ) ) ;
#81288=CARTESIAN_POINT ( 'NONE',  ( -8.314922557961024197, 14.29746914071037800, 42.91775706135235424 ) ) ;
#81289=CARTESIAN_POINT ( 'NONE',  ( -19.03943276465977164, 0.05219959533909376836, 21.24890960531436335 ) ) ;
#81290=CARTESIAN_POINT ( 'NONE',  ( 9.564922557961047289, -16.46253265017146816, 70.41775706135233293 ) ) ;
#81291=CARTESIAN_POINT ( 'NONE',  ( 14.29746914071049879, -8.314922557960816363, 73.33224293864769550 ) ) ;
#81292=CARTESIAN_POINT ( 'NONE',  ( -0.05219959533937732626, 21.53943276465977519, 42.50109039468567573 ) ) ;
#81294=CARTESIAN_POINT ( 'NONE',  ( -18.62759615963270932, 10.81492255796079327, 85.83224293864768129 ) ) ;
#81295=CARTESIAN_POINT ( 'NONE',  ( -19.03943276465977164, 0.05219959533909376836, 116.2489096053143669 ) ) ;
#81296=CARTESIAN_POINT ( 'NONE',  ( 12.14591786802309770, 12.06949235617756955, 69.37390960531436690 ) ) ;
#81298=CARTESIAN_POINT ( 'NONE',  ( 19.05341960407611168, 5.049401038298154454, 48.95724293864768129 ) ) ;
#81300=CARTESIAN_POINT ( 'NONE',  ( 13.97604488694548053, -13.89961937509957401, 75.62609039468564731 ) ) ;
#81301=CARTESIAN_POINT ( 'NONE',  ( 18.62759615963255655, 10.81492255796105972, 26.66775706135235424 ) ) ;
#81302=CARTESIAN_POINT ( 'NONE',  ( -19.03943276465977164, 0.05219959533909376836, 76.24890960531435269 ) ) ;
#81303=CARTESIAN_POINT ( 'NONE',  ( 13.97604488694548053, -13.89961937509957401, 50.62609039468566152 ) ) ;
#81304=CARTESIAN_POINT ( 'NONE',  ( 5.153800228976335163, 19.02544592524342804, 49.79057627198100988 ) ) ;
#81305=CARTESIAN_POINT ( 'NONE',  ( -16.55341960407611168, -4.379528057220339221, 61.45724293864770260 ) ) ;
#81306=CARTESIAN_POINT ( 'NONE',  ( 16.55341960407611168, 4.379528057220329451, 48.95724293864770971 ) ) ;
#81307=CARTESIAN_POINT ( 'NONE',  ( 16.46253265017160672, -9.564922557960803928, 78.33224293864769550 ) ) ;
#81308=CARTESIAN_POINT ( 'NONE',  ( -15.72974639402197994, 15.80617190586746368, 85.62390960531436690 ) ) ;
#81309=CARTESIAN_POINT ( 'NONE',  ( 5.049401038298161559, -19.05341960407611168, 67.70724293864769550 ) ) ;
#81310=CARTESIAN_POINT ( 'NONE',  ( 21.55341960407610458, 5.719274019375980345, 73.95724293864769550 ) ) ;
#81312=CARTESIAN_POINT ( 'NONE',  ( 19.03943276465977164, 0.05219959533936151252, 21.25109039468565797 ) ) ;
#81313=CARTESIAN_POINT ( 'NONE',  ( 16.51473224551069308, 9.474510206698969483, 29.16557627198103475 ) ) ;
#81314=CARTESIAN_POINT ( 'NONE',  ( -4.483927247898782831, 16.52544592524335698, 107.7094237280190328 ) ) ;
#81315=CARTESIAN_POINT ( 'NONE',  ( 16.55341960407611168, 4.379528057220329451, 98.95724293864770971 ) ) ;
#81316=CARTESIAN_POINT ( 'NONE',  ( 13.89961937509957401, 13.97604488694547697, 101.8760903946856331 ) ) ;
#81318=CARTESIAN_POINT ( 'NONE',  ( -10.81492255796105439, 18.62759615963255655, 27.91775706135234358 ) ) ;
#81319=CARTESIAN_POINT ( 'NONE',  ( -0.05219959533936034679, 19.03943276465977164, 52.50109039468566863 ) ) ;
#81320=CARTESIAN_POINT ( 'NONE',  ( 12.14591786802309770, 12.06949235617756955, 24.37390960531435979 ) ) ;
#81321=CARTESIAN_POINT ( 'NONE',  ( 21.53943276465977519, -0.05219959533907433946, 73.74890960531433848 ) ) ;
#81322=CARTESIAN_POINT ( 'NONE',  ( -13.97604488694527625, -13.89961937509977652, 96.87390960531433848 ) ) ;
#81323=CARTESIAN_POINT ( 'NONE',  ( -0.05219959533910754901, -16.53943276465976808, 62.49890960531436690 ) ) ;
#81325=CARTESIAN_POINT ( 'NONE',  ( 16.46253265017160672, -9.564922557960803928, 38.33224293864768839 ) ) ;
#81326=CARTESIAN_POINT ( 'NONE',  ( -21.53943276465977519, -0.05219959533937600094, 113.7510903946856757 ) ) ;
#81327=CARTESIAN_POINT ( 'NONE',  ( 16.53943276465976808, 0.05219959533934440121, 86.25109039468568994 ) ) ;
#81328=CARTESIAN_POINT ( 'NONE',  ( 21.53943276465977519, 0.05219959533937863772, 46.25109039468567573 ) ) ;
#81329=CARTESIAN_POINT ( 'NONE',  ( -8.224510206698735004, -14.34966873604973081, 39.58442372801901143 ) ) ;
#81330=CARTESIAN_POINT ( 'NONE',  ( -13.89961937509977652, 13.97604488694528158, 115.6239096053143669 ) ) ;
#81331=CARTESIAN_POINT ( 'NONE',  ( -5.049401038298153566, 19.05341960407611168, 60.20724293864768129 ) ) ;
#81332=CARTESIAN_POINT ( 'NONE',  ( -5.153800228976328057, -19.02544592524343514, 67.29057627198102409 ) ) ;
#81333=CARTESIAN_POINT ( 'NONE',  ( -16.53943276465976808, -0.05219959533934237506, 63.75109039468568284 ) ) ;
#81334=CARTESIAN_POINT ( 'NONE',  ( -14.29746914071049879, 8.314922557960819915, 110.8322429386476955 ) ) ;
#81335=CARTESIAN_POINT ( 'NONE',  ( -16.55341960407611168, -4.379528057220339221, 21.45724293864769550 ) ) ;
#81337=CARTESIAN_POINT ( 'NONE',  ( 18.67979575497194134, -10.72451020669871369, 60.83442372801901854 ) ) ;
#81338=CARTESIAN_POINT ( 'NONE',  ( -13.97604488694527625, -13.89961937509977652, 96.87390960531433848 ) ) ;
#81339=CARTESIAN_POINT ( 'NONE',  ( 19.03943276465977164, -0.05219959533909143690, 78.74890960531436690 ) ) ;
#81340=CARTESIAN_POINT ( 'NONE',  ( 13.97604488694527802, 13.89961937509977652, 114.3739096053143669 ) ) ;
#81341=CARTESIAN_POINT ( 'NONE',  ( -4.483927247898539470, -16.52544592524342804, 42.29057627198103120 ) ) ;
#81342=CARTESIAN_POINT ( 'NONE',  ( -4.483927247898782831, 16.52544592524335698, 112.7094237280190328 ) ) ;
#81343=CARTESIAN_POINT ( 'NONE',  ( 0.05219959533910956823, 16.53943276465976808, 39.99890960531436690 ) ) ;
#81345=CARTESIAN_POINT ( 'NONE',  ( -19.03943276465977164, -0.05219959533935918106, 43.75109039468566863 ) ) ;
#81346=CARTESIAN_POINT ( 'NONE',  ( 0.05219959533909260263, 19.03943276465977164, 79.99890960531436690 ) ) ;
#81347=CARTESIAN_POINT ( 'NONE',  ( 9.474510206698729675, 16.51473224551082808, 47.08442372801900433 ) ) ;
#81349=CARTESIAN_POINT ( 'NONE',  ( 17.58332526062526568, -7.635886036038552760, 68.42334959558466778 ) ) ;
#81350=CARTESIAN_POINT ( 'NONE',  ( -16.46253265017146816, -9.564922557961047289, 89.16775706135234714 ) ) ;
#81351=CARTESIAN_POINT ( 'NONE',  ( -4.483927247898782831, 16.52544592524335698, 67.70942372801901854 ) ) ;
#81353=CARTESIAN_POINT ( 'NONE',  ( 16.46253265017160672, -9.564922557960803928, 98.33224293864769550 ) ) ;
#81354=CARTESIAN_POINT ( 'NONE',  ( -5.719274019375665041, -21.55341960407619695, 34.79275706135235424 ) ) ;
#81355=CARTESIAN_POINT ( 'NONE',  ( -19.05341960407617563, 5.049401038297882671, 93.54275706135234714 ) ) ;
#81356=CARTESIAN_POINT ( 'NONE',  ( 17.13100169013300089, 6.664070546373171311, 86.73210164300154190 ) ) ;
#81357=CARTESIAN_POINT ( 'NONE',  ( -9.474510206698964154, 16.51473224551069663, 50.41557627198102409 ) ) ;
#81358=CARTESIAN_POINT ( 'NONE',  ( -9.474510206698964154, 16.51473224551069663, 95.41557627198102409 ) ) ;
#81359=CARTESIAN_POINT ( 'NONE',  ( -8.314922557960811034, -14.29746914071050412, 52.08224293864768839 ) ) ;
#81360=CARTESIAN_POINT ( 'NONE',  ( 19.03943276465977164, -0.05219959533909143690, 43.74890960531435979 ) ) ;
#81361=CARTESIAN_POINT ( 'NONE',  ( -19.03943276465977164, -0.05219959533935918106, 63.75109039468566863 ) ) ;
#81362=CARTESIAN_POINT ( 'NONE',  ( 16.51473224551083163, -9.474510206698727899, 30.83442372801900433 ) ) ;
#81363=CARTESIAN_POINT ( 'NONE',  ( -5.153800228976328057, -19.02544592524343514, 67.29057627198102409 ) ) ;
#81364=CARTESIAN_POINT ( 'NONE',  ( -21.52544592524343514, 5.823673210054127303, 61.04057627198103120 ) ) ;
#81365=CARTESIAN_POINT ( 'NONE',  ( 4.379528057220339221, -16.55341960407611168, 67.70724293864769550 ) ) ;
#81366=CARTESIAN_POINT ( 'NONE',  ( -5.823673210054431948, 21.52544592524334988, 112.7094237280190328 ) ) ;
#81368=CARTESIAN_POINT ( 'NONE',  ( -19.03943276465977164, 0.05219959533909376836, 116.2489096053143669 ) ) ;
#81369=CARTESIAN_POINT ( 'NONE',  ( 9.564922557960805705, 16.46253265017160317, 59.58224293864769550 ) ) ;
#81370=CARTESIAN_POINT ( 'NONE',  ( 0.05219959533909260263, 19.03943276465977164, 39.99890960531436690 ) ) ;
#81371=CARTESIAN_POINT ( 'NONE',  ( -8.314922557960811034, -14.29746914071050412, 97.08224293864770971 ) ) ;
#81372=CARTESIAN_POINT ( 'NONE',  ( -18.62759615963270932, 10.81492255796079327, 110.8322429386476955 ) ) ;
#81373=CARTESIAN_POINT ( 'NONE',  ( -5.049401038298153566, 19.05341960407611168, 115.2072429386477097 ) ) ;
#81374=CARTESIAN_POINT ( 'NONE',  ( -10.72451020669870658, -18.67979575497194134, 29.58442372801901854 ) ) ;
#81375=CARTESIAN_POINT ( 'NONE',  ( -0.05219959533910754901, -16.53943276465976808, 112.4989096053143669 ) ) ;
#81376=CARTESIAN_POINT ( 'NONE',  ( 10.72451020669871369, 18.67979575497193778, 77.08442372801901854 ) ) ;
#81377=CARTESIAN_POINT ( 'NONE',  ( -18.67979575497178146, -10.72451020669898902, 86.66557627198102409 ) ) ;
#81378=CARTESIAN_POINT ( 'NONE',  ( -16.51473224551082808, 9.474510206698731452, 33.33442372801899722 ) ) ;
#81379=CARTESIAN_POINT ( 'NONE',  ( 19.05341960407611168, 5.049401038298154454, 23.95724293864769194 ) ) ;
#81380=CARTESIAN_POINT ( 'NONE',  ( 19.52837319214027900, -5.499999999999890754, 77.10471352585537375 ) ) ;
#81382=CARTESIAN_POINT ( 'NONE',  ( -0.05219959533934338120, 16.53943276465976808, 52.50109039468567573 ) ) ;
#81383=CARTESIAN_POINT ( 'NONE',  ( 16.52544592524342804, -4.483927247898539470, 103.5405762719810383 ) ) ;
#81385=CARTESIAN_POINT ( 'NONE',  ( 19.02544592524343514, -5.153800228976328945, 78.54057627198099567 ) ) ;
#81386=CARTESIAN_POINT ( 'NONE',  ( 0.05219959533910956823, 16.53943276465976808, 99.99890960531436690 ) ) ;
#81387=CARTESIAN_POINT ( 'NONE',  ( -5.823673210054116645, -21.52544592524344225, 47.29057627198103120 ) ) ;
#81388=CARTESIAN_POINT ( 'NONE',  ( -8.224510206698948167, 14.34966873604960824, 60.41557627198102409 ) ) ;
#81389=CARTESIAN_POINT ( 'NONE',  ( -14.34966873604972548, 8.224510206698743886, 38.33442372801900433 ) ) ;
#81390=CARTESIAN_POINT ( 'NONE',  ( 0.05219959533937995610, -21.53943276465977519, 85.00109039468568994 ) ) ;
#81391=CARTESIAN_POINT ( 'NONE',  ( 16.62475595723696031, -7.163666690055368491, 78.02713351810469078 ) ) ;
#81392=CARTESIAN_POINT ( 'NONE',  ( 16.53943276465976808, 0.05219959533934440121, 101.2510903946856757 ) ) ;
#81393=CARTESIAN_POINT ( 'NONE',  ( -14.29746914071049879, 8.314922557960819915, 40.83224293864769550 ) ) ;
#81394=CARTESIAN_POINT ( 'NONE',  ( -16.46253265017160317, 9.564922557960807481, 35.83224293864768839 ) ) ;
#81395=CARTESIAN_POINT ( 'NONE',  ( 5.823673210054444382, -21.52544592524334988, 100.2094237280190043 ) ) ;
#81396=CARTESIAN_POINT ( 'NONE',  ( 18.67979575497178502, 10.72451020669898547, 104.1655762719810241 ) ) ;
#81397=CARTESIAN_POINT ( 'NONE',  ( -21.53943276465977519, -0.05219959533937600094, 63.75109039468568284 ) ) ;
#81398=CARTESIAN_POINT ( 'NONE',  ( 0.05219959533934541429, -16.53943276465976808, 45.00109039468568284 ) ) ;
#81399=CARTESIAN_POINT ( 'NONE',  ( 16.55341960407611168, 4.379528057220329451, 63.95724293864770260 ) ) ;
#81400=CARTESIAN_POINT ( 'NONE',  ( -5.719274019375665041, -21.55341960407619695, 84.79275706135234714 ) ) ;
#81401=CARTESIAN_POINT ( 'NONE',  ( -8.314922557961024197, 14.29746914071037800, 97.91775706135236135 ) ) ;
#81402=CARTESIAN_POINT ( 'NONE',  ( 16.36317988757058473, 7.306389748694950725, 28.40210391636777487 ) ) ;
#81404=CARTESIAN_POINT ( 'NONE',  ( 8.314922557960818139, 14.29746914071049879, 34.58224293864770260 ) ) ;
#81405=CARTESIAN_POINT ( 'NONE',  ( 12.14591786802327356, -12.06949235617739191, 70.62609039468567573 ) ) ;
#81406=CARTESIAN_POINT ( 'NONE',  ( -16.46253265017160317, 9.564922557960807481, 90.83224293864769550 ) ) ;
#81407=CARTESIAN_POINT ( 'NONE',  ( 19.02544592524343514, -5.153800228976328945, 98.54057627198100988 ) ) ;
#81408=CARTESIAN_POINT ( 'NONE',  ( 15.72974639402176855, 15.80617190586768217, 86.87609039468568994 ) ) ;
#81409=CARTESIAN_POINT ( 'NONE',  ( -4.483927247898782831, 16.52544592524335698, 82.70942372801900433 ) ) ;
#81410=CARTESIAN_POINT ( 'NONE',  ( 0.05219959533910956823, 16.53943276465976808, 59.99890960531436690 ) ) ;
#81411=CARTESIAN_POINT ( 'NONE',  ( -9.474510206698964154, 16.51473224551069663, 70.41557627198102409 ) ) ;
#81413=CARTESIAN_POINT ( 'NONE',  ( 8.314922557961029526, -14.29746914071037800, 30.41775706135234358 ) ) ;
#81414=CARTESIAN_POINT ( 'NONE',  ( 0.05219959533909260263, 19.03943276465977164, 34.99890960531435979 ) ) ;
#81415=CARTESIAN_POINT ( 'NONE',  ( -19.02544592524342804, 5.153800228976336051, 76.04057627198102409 ) ) ;
#81416=CARTESIAN_POINT ( 'NONE',  ( -12.06949235617739369, -12.14591786802326823, 19.37609039468568639 ) ) ;
#81418=CARTESIAN_POINT ( 'NONE',  ( 16.46253265017146816, 9.564922557961045513, 26.66775706135234003 ) ) ;
#81419=CARTESIAN_POINT ( 'NONE',  ( -16.55341960407617563, 4.379528057220093196, 78.54275706135236135 ) ) ;
#81420=CARTESIAN_POINT ( 'NONE',  ( 9.564922557961047289, -16.46253265017146816, 100.4177570613523329 ) ) ;
#81421=CARTESIAN_POINT ( 'NONE',  ( -13.97604488694527625, -13.89961937509977652, 21.87390960531435979 ) ) ;
#81422=CARTESIAN_POINT ( 'NONE',  ( -14.29746914071037622, -8.314922557961029526, 64.16775706135234714 ) ) ;
#81423=CARTESIAN_POINT ( 'NONE',  ( 4.483927247898790824, -16.52544592524335698, 50.20942372801901854 ) ) ;
#81425=CARTESIAN_POINT ( 'NONE',  ( 16.51473224551083163, -9.474510206698727899, 70.83442372801900433 ) ) ;
#81426=CARTESIAN_POINT ( 'NONE',  ( 9.564922557961047289, -16.46253265017146816, 20.41775706135233293 ) ) ;
#81427=CARTESIAN_POINT ( 'NONE',  ( -19.02544592524342804, 5.153800228976336051, 46.04057627198101699 ) ) ;
#81428=CARTESIAN_POINT ( 'NONE',  ( -9.474510206698964154, 16.51473224551069663, 80.41557627198103830 ) ) ;
#81429=CARTESIAN_POINT ( 'NONE',  ( -14.34966873604960291, -8.224510206698953496, 76.66557627198103830 ) ) ;
#81430=CARTESIAN_POINT ( 'NONE',  ( 16.51473224551083163, -9.474510206698727899, 40.83442372801900433 ) ) ;
#81431=CARTESIAN_POINT ( 'NONE',  ( 5.823673210054125526, 21.52544592524343514, 34.79057627198103120 ) ) ;
#81432=CARTESIAN_POINT ( 'NONE',  ( 21.55341960407619695, -5.719274019375665929, 111.0427570613523613 ) ) ;
#81433=CARTESIAN_POINT ( 'NONE',  ( 19.05341960407611168, 5.049401038298154454, 88.95724293864769550 ) ) ;
#81434=CARTESIAN_POINT ( 'NONE',  ( 5.719274019375673035, 21.55341960407619339, 107.2927570613523471 ) ) ;
#81435=CARTESIAN_POINT ( 'NONE',  ( 21.53943276465977519, -0.05219959533907433946, 63.74890960531435979 ) ) ;
#81436=CARTESIAN_POINT ( 'NONE',  ( -9.474510206698964154, 16.51473224551069663, 90.41557627198103830 ) ) ;
#81437=CARTESIAN_POINT ( 'NONE',  ( -16.46253265017146816, -9.564922557961047289, 84.16775706135233293 ) ) ;
#81438=CARTESIAN_POINT ( 'NONE',  ( 9.474510206698971260, -16.51473224551069308, 102.9155762719810241 ) ) ;
#81439=CARTESIAN_POINT ( 'NONE',  ( 13.89961937509957401, 13.97604488694547697, 101.8760903946856331 ) ) ;
#81440=CARTESIAN_POINT ( 'NONE',  ( -19.03943276465977164, 0.05219959533909376836, 26.24890960531435624 ) ) ;
#81441=CARTESIAN_POINT ( 'NONE',  ( -9.474510206698964154, 16.51473224551069663, 90.41557627198103830 ) ) ;
#81442=CARTESIAN_POINT ( 'NONE',  ( -10.81492255796078084, -18.62759615963271287, 57.08224293864769550 ) ) ;
#81443=CARTESIAN_POINT ( 'NONE',  ( -4.379528057220086978, -16.55341960407618274, 39.79275706135235424 ) ) ;
#81444=CARTESIAN_POINT ( 'NONE',  ( -0.05219959533937732626, 21.53943276465977519, 52.50109039468567573 ) ) ;
#81445=CARTESIAN_POINT ( 'NONE',  ( 21.52544592524334988, 5.823673210054432836, 91.45942372801901854 ) ) ;
#81446=CARTESIAN_POINT ( 'NONE',  ( -12.06949235617739369, -12.14591786802326823, 94.37609039468568994 ) ) ;
#81447=CARTESIAN_POINT ( 'NONE',  ( 19.03943276465977164, -0.05219959533909143690, 83.74890960531436690 ) ) ;
#81448=CARTESIAN_POINT ( 'NONE',  ( -4.379528057220328563, 16.55341960407611168, 95.20724293864769550 ) ) ;
#81449=CARTESIAN_POINT ( 'NONE',  ( -0.05219959533910754901, -16.53943276465976808, 22.49890960531436335 ) ) ;
#81450=CARTESIAN_POINT ( 'NONE',  ( 9.564922557961047289, -16.46253265017146816, 65.41775706135233293 ) ) ;
#81452=CARTESIAN_POINT ( 'NONE',  ( -5.719274019375665041, -21.55341960407619695, 39.79275706135235424 ) ) ;
#81453=CARTESIAN_POINT ( 'NONE',  ( 8.224510206698953496, -14.34966873604960469, 97.91557627198103830 ) ) ;
#81454=CARTESIAN_POINT ( 'NONE',  ( 13.97604488694527802, 13.89961937509977652, 114.3739096053143669 ) ) ;
#81455=CARTESIAN_POINT ( 'NONE',  ( -14.34966873604972548, 8.224510206698743886, 113.3344237280190328 ) ) ;
#81456=CARTESIAN_POINT ( 'NONE',  ( 18.62759615963255655, 10.81492255796105972, 91.66775706135234714 ) ) ;
#81457=CARTESIAN_POINT ( 'NONE',  ( -12.14591786802326823, 12.06949235617739902, 63.12609039468568994 ) ) ;
#81458=CARTESIAN_POINT ( 'NONE',  ( 15.72974639402176855, 15.80617190586768217, 46.87609039468568994 ) ) ;
#81460=CARTESIAN_POINT ( 'NONE',  ( -15.72974639402176322, -15.80617190586768395, 29.37609039468568284 ) ) ;
#81461=CARTESIAN_POINT ( 'NONE',  ( -8.314922557960811034, -14.29746914071050412, 107.0822429386476955 ) ) ;
#81462=CARTESIAN_POINT ( 'NONE',  ( 19.50973618000806198, 5.499999999999992895, 37.50000000000000000 ) ) ;
#81463=CARTESIAN_POINT ( 'NONE',  ( -8.314922557960811034, -14.29746914071050412, 67.08224293864770971 ) ) ;
#81464=CARTESIAN_POINT ( 'NONE',  ( 16.46253265017160672, -9.564922557960803928, 53.33224293864768839 ) ) ;
#81465=CARTESIAN_POINT ( 'NONE',  ( -14.29746914071037622, -8.314922557961029526, 104.1677570613523471 ) ) ;
#81466=CARTESIAN_POINT ( 'NONE',  ( 13.97604488694527802, 13.89961937509977652, 34.37390960531436690 ) ) ;
#81467=CARTESIAN_POINT ( 'NONE',  ( -18.62759615963270932, 10.81492255796079327, 40.83224293864769550 ) ) ;
#81468=CARTESIAN_POINT ( 'NONE',  ( 12.06949235617757843, -12.14591786802309237, 78.12390960531436690 ) ) ;
#81469=CARTESIAN_POINT ( 'NONE',  ( -15.72974639402197994, 15.80617190586746368, 95.62390960531436690 ) ) ;
#81470=CARTESIAN_POINT ( 'NONE',  ( 19.05341960407611168, 5.049401038298154454, 88.95724293864769550 ) ) ;
#81471=CARTESIAN_POINT ( 'NONE',  ( 9.474510206698971260, -16.51473224551069308, 57.91557627198103120 ) ) ;
#81472=CARTESIAN_POINT ( 'NONE',  ( -9.564922557961040184, 16.46253265017147172, 97.91775706135233293 ) ) ;
#81473=CARTESIAN_POINT ( 'NONE',  ( -18.67979575497178146, -10.72451020669898902, 41.66557627198103120 ) ) ;
#81474=CARTESIAN_POINT ( 'NONE',  ( -15.72974639402176322, -15.80617190586768395, 64.37609039468568994 ) ) ;
#81475=CARTESIAN_POINT ( 'NONE',  ( 13.97604488694527802, 13.89961937509977652, 49.37390960531434558 ) ) ;
#81476=CARTESIAN_POINT ( 'NONE',  ( 16.46253265017160672, -9.564922557960803928, 88.33224293864769550 ) ) ;
#81478=CARTESIAN_POINT ( 'NONE',  ( 16.53943276465976808, 0.05219959533934440121, 66.25109039468567573 ) ) ;
#81479=CARTESIAN_POINT ( 'NONE',  ( -5.823673210054431948, 21.52544592524334988, 37.70942372801900433 ) ) ;
#81480=CARTESIAN_POINT ( 'NONE',  ( -21.53943276465977519, -0.05219959533937600094, 68.75109039468568994 ) ) ;
#81481=CARTESIAN_POINT ( 'NONE',  ( 18.62759615963271287, -10.81492255796078972, 28.33224293864769550 ) ) ;
#81482=CARTESIAN_POINT ( 'NONE',  ( 10.72451020669898902, -18.67979575497178502, 102.9155762719810383 ) ) ;
#81483=CARTESIAN_POINT ( 'NONE',  ( -21.52544592524334988, -5.823673210054445271, 33.95942372801901143 ) ) ;
#81484=CARTESIAN_POINT ( 'NONE',  ( -0.05219959533934338120, 16.53943276465976808, 67.50109039468568994 ) ) ;
#81485=CARTESIAN_POINT ( 'NONE',  ( -21.55341960407610458, -5.719274019375992779, 66.45724293864768129 ) ) ;
#81486=CARTESIAN_POINT ( 'NONE',  ( -9.564922557961040184, 16.46253265017147172, 32.91775706135233293 ) ) ;
#81487=CARTESIAN_POINT ( 'NONE',  ( 13.89961937509977652, -13.97604488694527269, 73.12390960531436690 ) ) ;
#81488=CARTESIAN_POINT ( 'NONE',  ( 16.55341960407618274, -4.379528057220086978, 106.0427570613523471 ) ) ;
#81489=CARTESIAN_POINT ( 'NONE',  ( -17.50000000000014566, -3.292511757969676101, 104.9347972978947183 ) ) ;
#81490=CARTESIAN_POINT ( 'NONE',  ( -19.05341960407611168, -5.049401038298163336, 101.4572429386476955 ) ) ;
#81491=CARTESIAN_POINT ( 'NONE',  ( 17.50000000000000000, 5.499999999999992895, 81.70309617465829888 ) ) ;
#81492=CARTESIAN_POINT ( 'NONE',  ( 19.03943276465977164, 0.05219959533936151252, 76.25109039468566152 ) ) ;
#81493=CARTESIAN_POINT ( 'NONE',  ( -15.72974639402197994, 15.80617190586746368, 60.62390960531437401 ) ) ;
#81494=CARTESIAN_POINT ( 'NONE',  ( 8.224510206698953496, -14.34966873604960469, 32.91557627198102409 ) ) ;
#81495=CARTESIAN_POINT ( 'NONE',  ( -13.89961937509957401, -13.97604488694547875, 94.37609039468566152 ) ) ;
#81496=CARTESIAN_POINT ( 'NONE',  ( -5.153800228976328057, -19.02544592524343514, 22.29057627198102765 ) ) ;
#81497=CARTESIAN_POINT ( 'NONE',  ( -0.05219959533936034679, 19.03943276465977164, 112.5010903946856757 ) ) ;
#81498=CARTESIAN_POINT ( 'NONE',  ( -21.53943276465977519, 0.05219959533907696930, 86.24890960531436690 ) ) ;
#81499=CARTESIAN_POINT ( 'NONE',  ( -5.049401038297874678, -19.05341960407617918, 59.79275706135231871 ) ) ;
#81500=CARTESIAN_POINT ( 'NONE',  ( -16.52544592524335698, -4.483927247898792601, 83.95942372801900433 ) ) ;
#81501=CARTESIAN_POINT ( 'NONE',  ( 16.51473224551069308, 9.474510206698969483, 64.16557627198102409 ) ) ;
#81502=CARTESIAN_POINT ( 'NONE',  ( 14.29746914071049879, -8.314922557960816363, 63.33224293864770260 ) ) ;
#81503=CARTESIAN_POINT ( 'NONE',  ( -5.153800228976328057, -19.02544592524343514, 52.29057627198100988 ) ) ;
#81504=CARTESIAN_POINT ( 'NONE',  ( 16.53943276465976808, -0.05219959533910856209, 48.74890960531435979 ) ) ;
#81505=CARTESIAN_POINT ( 'NONE',  ( 13.89961937509977652, -13.97604488694527269, 23.12390960531436335 ) ) ;
#81507=CARTESIAN_POINT ( 'NONE',  ( 16.53943276465976808, -0.05219959533910856209, 33.74890960531436690 ) ) ;
#81508=CARTESIAN_POINT ( 'NONE',  ( 16.51473224551069308, 9.474510206698969483, 79.16557627198103830 ) ) ;
#81510=CARTESIAN_POINT ( 'NONE',  ( 13.89961937509957401, 13.97604488694547697, 36.87609039468565442 ) ) ;
#81511=CARTESIAN_POINT ( 'NONE',  ( -4.379528057220086978, -16.55341960407618274, 44.79275706135234714 ) ) ;
#81512=CARTESIAN_POINT ( 'NONE',  ( 18.67979575497178502, 10.72451020669898547, 49.16557627198102409 ) ) ;
#81513=CARTESIAN_POINT ( 'NONE',  ( 21.52544592524334988, 5.823673210054432836, 101.4594237280190185 ) ) ;
#81514=CARTESIAN_POINT ( 'NONE',  ( 16.51473224551069308, 9.474510206698969483, 74.16557627198103830 ) ) ;
#81515=CARTESIAN_POINT ( 'NONE',  ( 19.03943276465977164, -0.05219959533909143690, 113.7489096053143669 ) ) ;
#81516=CARTESIAN_POINT ( 'NONE',  ( 19.03943276465977164, -0.05219959533909143690, 108.7489096053143527 ) ) ;
#81517=CARTESIAN_POINT ( 'NONE',  ( -5.823673210054431948, 21.52544592524334988, 42.70942372801901854 ) ) ;
#81518=CARTESIAN_POINT ( 'NONE',  ( 16.53943276465976808, -0.05219959533910856209, 98.74890960531438111 ) ) ;
#81519=EDGE_CURVE ( 'NONE', #53380, #128521, #4249, .T. ) ;
#81520=CARTESIAN_POINT ( 'NONE',  ( 18.62759615963271287, -10.81492255796078972, 88.33224293864769550 ) ) ;
#81521=CARTESIAN_POINT ( 'NONE',  ( -13.97604488694527625, -13.89961937509977652, 86.87390960531436690 ) ) ;
#81523=CARTESIAN_POINT ( 'NONE',  ( 21.52544592524334988, 5.823673210054432836, 21.45942372801901499 ) ) ;
#81525=CARTESIAN_POINT ( 'NONE',  ( -16.46253265017160317, 9.564922557960807481, 90.83224293864769550 ) ) ;
#81526=CARTESIAN_POINT ( 'NONE',  ( 18.22780087662122384, -5.500000000000022204, 81.01540105326105845 ) ) ;
#81527=CARTESIAN_POINT ( 'NONE',  ( 19.05341960407611168, 5.049401038298154454, 28.95724293864769550 ) ) ;
#81528=CARTESIAN_POINT ( 'NONE',  ( -0.05219959533909027116, -19.03943276465977164, 32.49890960531435979 ) ) ;
#81529=CARTESIAN_POINT ( 'NONE',  ( 9.474510206698729675, 16.51473224551082808, 112.0844237280190043 ) ) ;
#81531=CARTESIAN_POINT ( 'NONE',  ( -14.34966873604960291, -8.224510206698953496, 106.6655762719810383 ) ) ;
#81532=CARTESIAN_POINT ( 'NONE',  ( -10.72451020669870658, -18.67979575497194134, 84.58442372801903275 ) ) ;
#81533=CARTESIAN_POINT ( 'NONE',  ( 16.46253265017160672, -9.564922557960803928, 63.33224293864769550 ) ) ;
#81534=CARTESIAN_POINT ( 'NONE',  ( -18.62759615963255300, -10.81492255796106328, 34.16775706135234714 ) ) ;
#81535=CARTESIAN_POINT ( 'NONE',  ( 21.53943276465977519, 0.05219959533937863772, 31.25109039468568639 ) ) ;
#81537=CARTESIAN_POINT ( 'NONE',  ( 5.153800228976335163, 19.02544592524342804, 79.79057627198102409 ) ) ;
#81539=CARTESIAN_POINT ( 'NONE',  ( 14.34966873604972726, -8.224510206698740333, 20.83442372801901143 ) ) ;
#81540=CARTESIAN_POINT ( 'NONE',  ( 10.81492255796078972, 18.62759615963270932, 44.58224293864769550 ) ) ;
#81541=CARTESIAN_POINT ( 'NONE',  ( -18.62759615963255300, -10.81492255796106328, 64.16775706135234714 ) ) ;
#81542=CARTESIAN_POINT ( 'NONE',  ( 19.02544592524343514, -5.153800228976328945, 103.5405762719809957 ) ) ;
#81544=CARTESIAN_POINT ( 'NONE',  ( -9.564922557961040184, 16.46253265017147172, 92.91775706135233293 ) ) ;
#81545=CARTESIAN_POINT ( 'NONE',  ( -19.05341960407611168, -5.049401038298163336, 56.45724293864768129 ) ) ;
#81546=CARTESIAN_POINT ( 'NONE',  ( 0.05219959533909260263, 19.03943276465977164, 89.99890960531436690 ) ) ;
#81547=CARTESIAN_POINT ( 'NONE',  ( 16.53943276465976808, -0.05219959533910856209, 93.74890960531436690 ) ) ;
#81548=CARTESIAN_POINT ( 'NONE',  ( 0.05219959533910956823, 16.53943276465976808, 109.9989096053143527 ) ) ;
#81549=CARTESIAN_POINT ( 'NONE',  ( -5.823673210054116645, -21.52544592524344225, 22.29057627198102765 ) ) ;
#81550=CARTESIAN_POINT ( 'NONE',  ( -0.05219959533910754901, -16.53943276465976808, 52.49890960531435979 ) ) ;
#81551=CARTESIAN_POINT ( 'NONE',  ( -19.02544592524342804, 5.153800228976336051, 46.04057627198101699 ) ) ;
#81552=CARTESIAN_POINT ( 'NONE',  ( -18.62759615963255300, -10.81492255796106328, 74.16775706135231871 ) ) ;
#81553=CARTESIAN_POINT ( 'NONE',  ( 19.03943276465977164, 0.05219959533936151252, 96.25109039468567573 ) ) ;
#81554=CARTESIAN_POINT ( 'NONE',  ( 14.29746914071049879, -8.314922557960816363, 58.33224293864768839 ) ) ;
#81555=CARTESIAN_POINT ( 'NONE',  ( -5.719274019375978568, 21.55341960407610458, 115.2072429386476955 ) ) ;
#81556=CARTESIAN_POINT ( 'NONE',  ( -10.81492255796078084, -18.62759615963271287, 42.08224293864769550 ) ) ;
#81557=CARTESIAN_POINT ( 'NONE',  ( 13.97604488694527802, 13.89961937509977652, 114.3739096053143669 ) ) ;
#81559=CARTESIAN_POINT ( 'NONE',  ( -16.46253265017160317, 9.564922557960807481, 65.83224293864769550 ) ) ;
#81560=CARTESIAN_POINT ( 'NONE',  ( -8.224510206698948167, 14.34966873604960824, 35.41557627198102409 ) ) ;
#81561=CARTESIAN_POINT ( 'NONE',  ( -16.55341960407617563, 4.379528057220093196, 108.5427570613523756 ) ) ;
#81562=CARTESIAN_POINT ( 'NONE',  ( -4.379528057220086978, -16.55341960407618274, 79.79275706135236135 ) ) ;
#81563=CARTESIAN_POINT ( 'NONE',  ( 19.02544592524334988, 5.153800228976608722, 41.45942372801900433 ) ) ;
#81565=CARTESIAN_POINT ( 'NONE',  ( 9.564922557960805705, 16.46253265017160317, 89.58224293864769550 ) ) ;
#81566=CARTESIAN_POINT ( 'NONE',  ( -13.89961937509977652, 13.97604488694528158, 50.62390960531435979 ) ) ;
#81567=CARTESIAN_POINT ( 'NONE',  ( 0.05219959533910956823, 16.53943276465976808, 54.99890960531435269 ) ) ;
#81568=CARTESIAN_POINT ( 'NONE',  ( -15.49999999999999822, 7.499999999999998224, 118.0000000000000142 ) ) ;
#81569=CARTESIAN_POINT ( 'NONE',  ( 15.80617190586746368, 15.72974639402197994, 24.37390960531435979 ) ) ;
#81570=CARTESIAN_POINT ( 'NONE',  ( -15.80617190586745835, -15.72974639402198527, 56.87390960531436690 ) ) ;
#81571=CARTESIAN_POINT ( 'NONE',  ( 14.34966873604960469, 8.224510206698951720, 84.16557627198103830 ) ) ;
#81572=CARTESIAN_POINT ( 'NONE',  ( 12.06949235617739724, 12.14591786802326823, 36.87609039468568994 ) ) ;
#81574=CARTESIAN_POINT ( 'NONE',  ( 16.52544592524342804, -4.483927247898539470, 73.54057627198102409 ) ) ;
#81576=CARTESIAN_POINT ( 'NONE',  ( 16.51473224551083163, -9.474510206698727899, 80.83442372801899012 ) ) ;
#81577=CARTESIAN_POINT ( 'NONE',  ( -13.97604488694527625, -13.89961937509977652, 111.8739096053143243 ) ) ;
#81580=CARTESIAN_POINT ( 'NONE',  ( 0.05219959533934541429, -16.53943276465976808, 25.00109039468567218 ) ) ;
#81581=CARTESIAN_POINT ( 'NONE',  ( 16.55341960407618274, -4.379528057220086978, 106.0427570613523471 ) ) ;
#81582=CARTESIAN_POINT ( 'NONE',  ( -9.564922557961040184, 16.46253265017147172, 77.91775706135234714 ) ) ;
#81583=CARTESIAN_POINT ( 'NONE',  ( -21.52544592524343514, 5.823673210054127303, 46.04057627198103830 ) ) ;
#81584=CARTESIAN_POINT ( 'NONE',  ( 10.72451020669871369, 18.67979575497193778, 72.08442372801899012 ) ) ;
#81585=FACE_OUTER_BOUND ( 'NONE', #106624, .T. ) ;
#81586=CARTESIAN_POINT ( 'NONE',  ( -0.05219959533934338120, 16.53943276465976808, 37.50109039468568284 ) ) ;
#81587=CARTESIAN_POINT ( 'NONE',  ( -9.564922557960796823, -16.46253265017161027, 22.08224293864768839 ) ) ;
#81588=CARTESIAN_POINT ( 'NONE',  ( -9.474510206698964154, 16.51473224551069663, 85.41557627198102409 ) ) ;
#81589=CARTESIAN_POINT ( 'NONE',  ( -0.05219959533909027116, -19.03943276465977164, 22.49890960531436690 ) ) ;
#81590=CARTESIAN_POINT ( 'NONE',  ( 16.53943276465976808, -0.05219959533910856209, 98.74890960531438111 ) ) ;
#81592=CARTESIAN_POINT ( 'NONE',  ( -0.05219959533909027116, -19.03943276465977164, 107.4989096053143527 ) ) ;
#81593=EDGE_LOOP ( 'NONE', ( #76799, #13396, #147113, #43043, #43588, #154879, #115421, #47823 ) ) ;
#81594=CARTESIAN_POINT ( 'NONE',  ( 14.29746914071037800, 8.314922557961029526, 61.66775706135235424 ) ) ;
#81595=CARTESIAN_POINT ( 'NONE',  ( -5.049401038297874678, -19.05341960407617918, 104.7927570613523471 ) ) ;
#81596=CARTESIAN_POINT ( 'NONE',  ( 10.72451020669898902, -18.67979575497178502, 72.91557627198103830 ) ) ;
#81597=CARTESIAN_POINT ( 'NONE',  ( 5.153800228976335163, 19.02544592524342804, 39.79057627198100988 ) ) ;
#81598=CARTESIAN_POINT ( 'NONE',  ( 19.03943276465977164, 0.05219959533936151252, 66.25109039468567573 ) ) ;
#81599=CARTESIAN_POINT ( 'NONE',  ( 18.67979575497194134, -10.72451020669871369, 20.83442372801901143 ) ) ;
#81600=CARTESIAN_POINT ( 'NONE',  ( -9.474510206698964154, 16.51473224551069663, 65.41557627198102409 ) ) ;
#81601=CARTESIAN_POINT ( 'NONE',  ( -5.153800228976328057, -19.02544592524343514, 112.2905762719810099 ) ) ;
#81603=CARTESIAN_POINT ( 'NONE',  ( 14.34966873604972726, -8.224510206698740333, 30.83442372801902209 ) ) ;
#81604=CARTESIAN_POINT ( 'NONE',  ( 5.823673210054125526, 21.52544592524343514, 99.79057627198103830 ) ) ;
#81605=CARTESIAN_POINT ( 'NONE',  ( 14.29746914071049879, -8.314922557960816363, 103.3322429386476955 ) ) ;
#81606=CARTESIAN_POINT ( 'NONE',  ( 9.474510206698971260, -16.51473224551069308, 92.91557627198103830 ) ) ;
#81607=CARTESIAN_POINT ( 'NONE',  ( 9.564922557961047289, -16.46253265017146816, 80.41775706135234714 ) ) ;
#81608=CARTESIAN_POINT ( 'NONE',  ( 5.823673210054125526, 21.52544592524343514, 84.79057627198102409 ) ) ;
#81609=CARTESIAN_POINT ( 'NONE',  ( 14.34966873604960469, 8.224510206698951720, 44.16557627198103120 ) ) ;
#81610=CARTESIAN_POINT ( 'NONE',  ( -15.80617190586768217, 15.72974639402176855, 113.1260903946856899 ) ) ;
#81611=CARTESIAN_POINT ( 'NONE',  ( 16.55341960407618274, -4.379528057220086978, 71.04275706135234714 ) ) ;
#81612=CARTESIAN_POINT ( 'NONE',  ( 13.97604488694527802, 13.89961937509977652, 99.37390960531436690 ) ) ;
#81613=ORIENTED_EDGE ( 'NONE', *, *, #164879, .T. ) ;
#81614=CARTESIAN_POINT ( 'NONE',  ( -9.474510206698964154, 16.51473224551069663, 45.41557627198103120 ) ) ;
#81615=CARTESIAN_POINT ( 'NONE',  ( -21.55341960407619339, 5.719274019375674811, 58.54275706135235424 ) ) ;
#81616=CARTESIAN_POINT ( 'NONE',  ( -18.67979575497193778, 10.72451020669871902, 73.33442372801901854 ) ) ;
#81617=CARTESIAN_POINT ( 'NONE',  ( 9.474510206698971260, -16.51473224551069308, 67.91557627198102409 ) ) ;
#81618=CARTESIAN_POINT ( 'NONE',  ( -10.81492255796105439, 18.62759615963255655, 37.91775706135235424 ) ) ;
#81619=CARTESIAN_POINT ( 'NONE',  ( -19.05341960407617563, 5.049401038297882671, 73.54275706135233293 ) ) ;
#81620=CARTESIAN_POINT ( 'NONE',  ( -5.049401038298153566, 19.05341960407611168, 35.20724293864768839 ) ) ;
#81621=CARTESIAN_POINT ( 'NONE',  ( 8.314922557961029526, -14.29746914071037800, 85.41775706135236135 ) ) ;
#81622=CARTESIAN_POINT ( 'NONE',  ( 19.02544592524343514, -5.153800228976328945, 58.54057627198102409 ) ) ;
#81623=CARTESIAN_POINT ( 'NONE',  ( -13.89961937509977652, 13.97604488694528158, 110.6239096053143243 ) ) ;
#81624=CARTESIAN_POINT ( 'NONE',  ( 9.564922557960805705, 16.46253265017160317, 34.58224293864770260 ) ) ;
#81625=CARTESIAN_POINT ( 'NONE',  ( 18.62759615963271287, -10.81492255796078972, 88.33224293864769550 ) ) ;
#81626=CARTESIAN_POINT ( 'NONE',  ( 16.53943276465976808, 0.05219959533934440121, 71.25109039468568994 ) ) ;
#81627=FACE_OUTER_BOUND ( 'NONE', #13644, .T. ) ;
#81628=CARTESIAN_POINT ( 'NONE',  ( -9.474510206698720793, -16.51473224551083518, 34.58442372801899722 ) ) ;
#81629=CARTESIAN_POINT ( 'NONE',  ( 19.05341960407611168, 5.049401038298154454, 58.95724293864768129 ) ) ;
#81630=CARTESIAN_POINT ( 'NONE',  ( 14.34966873604960469, 8.224510206698951720, 44.16557627198103120 ) ) ;
#81631=CARTESIAN_POINT ( 'NONE',  ( -4.379528057220328563, 16.55341960407611168, 85.20724293864770971 ) ) ;
#81632=CARTESIAN_POINT ( 'NONE',  ( 9.564922557960805705, 16.46253265017160317, 99.58224293864770971 ) ) ;
#81633=CARTESIAN_POINT ( 'NONE',  ( 16.46253265017160672, -9.564922557960803928, 83.33224293864768129 ) ) ;
#81634=CARTESIAN_POINT ( 'NONE',  ( 5.823673210054444382, -21.52544592524334988, 50.20942372801901854 ) ) ;
#81635=CARTESIAN_POINT ( 'NONE',  ( 5.049401038298161559, -19.05341960407611168, 92.70724293864769550 ) ) ;
#81637=CARTESIAN_POINT ( 'NONE',  ( 5.823673210054444382, -21.52544592524334988, 105.2094237280190328 ) ) ;
#81638=CARTESIAN_POINT ( 'NONE',  ( -16.55341960407617563, 4.379528057220093196, 83.54275706135234714 ) ) ;
#81639=CARTESIAN_POINT ( 'NONE',  ( -18.62759615963255300, -10.81492255796106328, 29.16775706135234003 ) ) ;
#81640=CARTESIAN_POINT ( 'NONE',  ( -15.80617190586745835, -15.72974639402198527, 101.8739096053143811 ) ) ;
#81641=CARTESIAN_POINT ( 'NONE',  ( -8.224510206698948167, 14.34966873604960824, 55.41557627198102409 ) ) ;
#81642=CARTESIAN_POINT ( 'NONE',  ( 9.564922557960805705, 16.46253265017160317, 39.58224293864768839 ) ) ;
#81643=CARTESIAN_POINT ( 'NONE',  ( 4.379528057220339221, -16.55341960407611168, 72.70724293864769550 ) ) ;
#81644=CARTESIAN_POINT ( 'NONE',  ( 0.05219959533907565091, 21.53943276465977519, 24.99890960531435624 ) ) ;
#81645=CARTESIAN_POINT ( 'NONE',  ( 5.049401038297881783, 19.05341960407617563, 27.29275706135232937 ) ) ;
#81646=CARTESIAN_POINT ( 'NONE',  ( -16.51473224551069308, -9.474510206698971260, 21.66557627198102765 ) ) ;
#81647=VERTEX_POINT ( 'NONE', #47312 ) ;
#81648=CARTESIAN_POINT ( 'NONE',  ( -14.34966873604972548, 8.224510206698743886, 73.33442372801901854 ) ) ;
#81649=CARTESIAN_POINT ( 'NONE',  ( 0.05219959533909260263, 19.03943276465977164, 69.99890960531435269 ) ) ;
#81651=CARTESIAN_POINT ( 'NONE',  ( 4.379528057220339221, -16.55341960407611168, 87.70724293864769550 ) ) ;
#81652=CARTESIAN_POINT ( 'NONE',  ( -10.81492255796078084, -18.62759615963271287, 32.08224293864769550 ) ) ;
#81654=CARTESIAN_POINT ( 'NONE',  ( 4.379528057220092307, 16.55341960407617563, 92.29275706135236135 ) ) ;
#81655=CARTESIAN_POINT ( 'NONE',  ( 9.474510206698729675, 16.51473224551082808, 112.0844237280190043 ) ) ;
#81656=CARTESIAN_POINT ( 'NONE',  ( -15.80617190586768217, 15.72974639402176855, 83.12609039468568994 ) ) ;
#81657=CARTESIAN_POINT ( 'NONE',  ( 19.02544592524343514, -5.153800228976328945, 93.54057627198102409 ) ) ;
#81658=CARTESIAN_POINT ( 'NONE',  ( -21.55341960407610458, -5.719274019375992779, 106.4572429386477097 ) ) ;
#81659=CARTESIAN_POINT ( 'NONE',  ( 16.53943276465976808, 0.05219959533934440121, 51.25109039468568994 ) ) ;
#81660=CARTESIAN_POINT ( 'NONE',  ( -5.153800228976328057, -19.02544592524343514, 32.29057627198102409 ) ) ;
#81661=CARTESIAN_POINT ( 'NONE',  ( -4.483927247898782831, 16.52544592524335698, 22.70942372801901499 ) ) ;
#81662=CARTESIAN_POINT ( 'NONE',  ( 5.049401038297881783, 19.05341960407617563, 92.29275706135234714 ) ) ;
#81663=CARTESIAN_POINT ( 'NONE',  ( -15.80617190586745835, -15.72974639402198527, 86.87390960531438111 ) ) ;
#81664=CARTESIAN_POINT ( 'NONE',  ( 16.46253265017146816, 9.564922557961045513, 51.66775706135233293 ) ) ;
#81665=CARTESIAN_POINT ( 'NONE',  ( 19.52217212775660826, -5.499999999999907629, 87.43993709005259518 ) ) ;
#81666=CARTESIAN_POINT ( 'NONE',  ( 21.52544592524344225, -5.823673210054117533, 98.54057627198105251 ) ) ;
#81668=CARTESIAN_POINT ( 'NONE',  ( 19.05341960407611168, 5.049401038298154454, 83.95724293864766707 ) ) ;
#81669=LINE ( 'NONE', #68515, #114286 ) ;
#81670=CARTESIAN_POINT ( 'NONE',  ( -16.52544592524335698, -4.483927247898792601, 38.95942372801901854 ) ) ;
#81672=CARTESIAN_POINT ( 'NONE',  ( -5.719274019375978568, 21.55341960407610458, 110.2072429386477239 ) ) ;
#81673=CARTESIAN_POINT ( 'NONE',  ( 4.483927247898545687, 16.52544592524342804, 59.79057627198103120 ) ) ;
#81674=CARTESIAN_POINT ( 'NONE',  ( -19.05341960407611168, -5.049401038298163336, 76.45724293864769550 ) ) ;
#81675=CARTESIAN_POINT ( 'NONE',  ( -4.379528057220086978, -16.55341960407618274, 34.79275706135235424 ) ) ;
#81676=CARTESIAN_POINT ( 'NONE',  ( 0.05219959533936267826, -19.03943276465977164, 45.00109039468566863 ) ) ;
#81677=CARTESIAN_POINT ( 'NONE',  ( -15.72974639402176322, -15.80617190586768395, 49.37609039468569705 ) ) ;
#81678=CARTESIAN_POINT ( 'NONE',  ( -0.05219959533936034679, 19.03943276465977164, 112.5010903946856757 ) ) ;
#81679=CARTESIAN_POINT ( 'NONE',  ( 19.02544592524343514, -5.153800228976328945, 53.54057627198102409 ) ) ;
#81680=EDGE_CURVE ( 'NONE', #151905, #29984, #41443, .T. ) ;
#81681=CARTESIAN_POINT ( 'NONE',  ( -9.564922557961040184, 16.46253265017147172, 87.91775706135233293 ) ) ;
#81682=CARTESIAN_POINT ( 'NONE',  ( -21.53943276465977519, -0.05219959533937600094, 83.75109039468568994 ) ) ;
#81683=CARTESIAN_POINT ( 'NONE',  ( 5.153800228976615827, -19.02544592524334988, 60.20942372801899012 ) ) ;
#81684=CARTESIAN_POINT ( 'NONE',  ( -5.049401038298153566, 19.05341960407611168, 40.20724293864768839 ) ) ;
#81685=CARTESIAN_POINT ( 'NONE',  ( -18.67979575497178146, -10.72451020669898902, 61.66557627198103120 ) ) ;
#81686=CARTESIAN_POINT ( 'NONE',  ( 4.379528057220339221, -16.55341960407611168, 57.70724293864770260 ) ) ;
#81688=CARTESIAN_POINT ( 'NONE',  ( 5.049401038297881783, 19.05341960407617563, 32.29275706135233293 ) ) ;
#81689=CARTESIAN_POINT ( 'NONE',  ( 16.53943276465976808, 0.05219959533934440121, 101.2510903946856757 ) ) ;
#81690=CARTESIAN_POINT ( 'NONE',  ( 8.314922557960818139, 14.29746914071049879, 54.58224293864769550 ) ) ;
#81691=CARTESIAN_POINT ( 'NONE',  ( 5.719274019375673035, 21.55341960407619339, 92.29275706135236135 ) ) ;
#81692=CARTESIAN_POINT ( 'NONE',  ( 5.823673210054444382, -21.52544592524334988, 85.20942372801901854 ) ) ;
#81693=CARTESIAN_POINT ( 'NONE',  ( -21.55341960407610458, -5.719274019375992779, 91.45724293864769550 ) ) ;
#81694=CARTESIAN_POINT ( 'NONE',  ( -5.153800228976328057, -19.02544592524343514, 52.29057627198100988 ) ) ;
#81695=CARTESIAN_POINT ( 'NONE',  ( 21.53943276465977519, 0.05219959533937863772, 76.25109039468568994 ) ) ;
#81696=CARTESIAN_POINT ( 'NONE',  ( 19.05341960407611168, 5.049401038298154454, 53.95724293864770260 ) ) ;
#81697=EDGE_LOOP ( 'NONE', ( #145815, #193197, #171709 ) ) ;
#81698=CARTESIAN_POINT ( 'NONE',  ( -19.05341960407611168, -5.049401038298163336, 61.45724293864769550 ) ) ;
#81699=CARTESIAN_POINT ( 'NONE',  ( 8.224510206698953496, -14.34966873604960469, 107.9155762719810241 ) ) ;
#81700=CARTESIAN_POINT ( 'NONE',  ( 5.153800228976335163, 19.02544592524342804, 114.7905762719810241 ) ) ;
#81701=CARTESIAN_POINT ( 'NONE',  ( 8.224510206698953496, -14.34966873604960469, 52.91557627198103830 ) ) ;
#81702=CARTESIAN_POINT ( 'NONE',  ( -0.05219959533909027116, -19.03943276465977164, 22.49890960531436690 ) ) ;
#81703=CARTESIAN_POINT ( 'NONE',  ( 14.29746914071049879, -8.314922557960816363, 68.33224293864769550 ) ) ;
#81704=CARTESIAN_POINT ( 'NONE',  ( 21.53943276465977519, -0.05219959533907433946, 83.74890960531435269 ) ) ;
#81705=CARTESIAN_POINT ( 'NONE',  ( 5.823673210054444382, -21.52544592524334988, 35.20942372801901854 ) ) ;
#81706=DIRECTION ( 'NONE',  ( -1.000000000000000000, 0.000000000000000000, -0.000000000000000000 ) ) ;
#81707=CARTESIAN_POINT ( 'NONE',  ( -4.483927247898782831, 16.52544592524335698, 37.70942372801900433 ) ) ;
#81708=CARTESIAN_POINT ( 'NONE',  ( 18.62759615963271287, -10.81492255796078972, 88.33224293864769550 ) ) ;
#81709=CARTESIAN_POINT ( 'NONE',  ( -5.823673210054431948, 21.52544592524334988, 107.7094237280190328 ) ) ;
#81710=CARTESIAN_POINT ( 'NONE',  ( 19.05341960407611168, 5.049401038298154454, 98.95724293864766707 ) ) ;
#81711=CARTESIAN_POINT ( 'NONE',  ( 5.719274019375673035, 21.55341960407619339, 47.29275706135234003 ) ) ;
#81713=CARTESIAN_POINT ( 'NONE',  ( 21.53943276465977519, -0.05219959533907433946, 23.74890960531435269 ) ) ;
#81714=CARTESIAN_POINT ( 'NONE',  ( 14.29746914071037800, 8.314922557961029526, 101.6677570613523613 ) ) ;
#81715=CARTESIAN_POINT ( 'NONE',  ( -5.719274019375665041, -21.55341960407619695, 49.79275706135234714 ) ) ;
#81716=CARTESIAN_POINT ( 'NONE',  ( -5.823673210054431948, 21.52544592524334988, 82.70942372801900433 ) ) ;
#81717=CARTESIAN_POINT ( 'NONE',  ( -9.564922557961040184, 16.46253265017147172, 22.91775706135233648 ) ) ;
#81718=CARTESIAN_POINT ( 'NONE',  ( 16.55341960407618274, -4.379528057220086978, 71.04275706135234714 ) ) ;
#81719=CARTESIAN_POINT ( 'NONE',  ( -5.719274019375665041, -21.55341960407619695, 44.79275706135234714 ) ) ;
#81720=CARTESIAN_POINT ( 'NONE',  ( 19.02544592524343514, -5.153800228976328945, 33.54057627198102409 ) ) ;
#81721=CARTESIAN_POINT ( 'NONE',  ( -10.81492255796105439, 18.62759615963255655, 102.9177570613523756 ) ) ;
#81722=CARTESIAN_POINT ( 'NONE',  ( -13.89961937509977652, 13.97604488694528158, 100.6239096053143669 ) ) ;
#81723=B_SPLINE_CURVE_WITH_KNOTS ( 'NONE', 3,
 ( #146172, #176540, #5665, #114846, #129002, #86510, #55177, #37002, #193708, #190700, #100669, #22847, #163365, #175527 ),
 .UNSPECIFIED., .F., .F.,
 ( 4, 2, 2, 2, 2, 2, 4 ),
 ( 0.002427643230453600375, 0.002603325520439084273, 0.002779007810424568171, 0.003130372390395535533, 0.003833101550337468522, 0.004535830710279402378, 0.005238559870221335367 ),
 .UNSPECIFIED. ) ;
#81724=CARTESIAN_POINT ( 'NONE',  ( 18.62759615963271287, -10.81492255796078972, 103.3322429386476955 ) ) ;
#81725=CARTESIAN_POINT ( 'NONE',  ( 17.60728821187776205, -5.500000000000032863, 88.36690927743606494 ) ) ;
#81726=CARTESIAN_POINT ( 'NONE',  ( 18.62759615963271287, -10.81492255796078972, 68.33224293864769550 ) ) ;
#81727=CARTESIAN_POINT ( 'NONE',  ( -0.05219959533934338120, 16.53943276465976808, 52.50109039468567573 ) ) ;
#81728=CARTESIAN_POINT ( 'NONE',  ( 14.34966873604960469, 8.224510206698951720, 44.16557627198103120 ) ) ;
#81730=CARTESIAN_POINT ( 'NONE',  ( 19.02544592524334988, 5.153800228976608722, 86.45942372801900433 ) ) ;
#81732=CARTESIAN_POINT ( 'NONE',  ( -16.55341960407617563, 4.379528057220093196, 28.54275706135234358 ) ) ;
#81733=CARTESIAN_POINT ( 'NONE',  ( -21.52544592524343514, 5.823673210054127303, 101.0405762719810383 ) ) ;
#81734=CARTESIAN_POINT ( 'NONE',  ( 18.67979575497178502, 10.72451020669898547, 79.16557627198103830 ) ) ;
#81735=CARTESIAN_POINT ( 'NONE',  ( 16.46253265017160672, -9.564922557960803928, 113.3322429386476955 ) ) ;
#81736=CARTESIAN_POINT ( 'NONE',  ( -16.55341960407617563, 4.379528057220093196, 48.54275706135234714 ) ) ;
#81737=CARTESIAN_POINT ( 'NONE',  ( -5.049401038298153566, 19.05341960407611168, 75.20724293864769550 ) ) ;
#81738=CARTESIAN_POINT ( 'NONE',  ( -15.72974639402176322, -15.80617190586768395, 24.37609039468567573 ) ) ;
#81739=CARTESIAN_POINT ( 'NONE',  ( -16.46253265017146816, -9.564922557961047289, 94.16775706135233293 ) ) ;
#81740=CARTESIAN_POINT ( 'NONE',  ( -16.46253265017160317, 9.564922557960807481, 110.8322429386476955 ) ) ;
#81741=CARTESIAN_POINT ( 'NONE',  ( 0.05219959533909260263, 19.03943276465977164, 89.99890960531436690 ) ) ;
#81742=CARTESIAN_POINT ( 'NONE',  ( -21.55341960407610458, -5.719274019375992779, 86.45724293864770971 ) ) ;
#81743=CARTESIAN_POINT ( 'NONE',  ( 9.474510206698971260, -16.51473224551069308, 57.91557627198103120 ) ) ;
#81745=CARTESIAN_POINT ( 'NONE',  ( 14.29746914071049879, -8.314922557960816363, 68.33224293864769550 ) ) ;
#81746=CARTESIAN_POINT ( 'NONE',  ( -10.81492255796078084, -18.62759615963271287, 22.08224293864769194 ) ) ;
#81748=CARTESIAN_POINT ( 'NONE',  ( -5.823673210054116645, -21.52544592524344225, 97.29057627198105251 ) ) ;
#81749=CARTESIAN_POINT ( 'NONE',  ( -16.46253265017146816, -9.564922557961047289, 64.16775706135233293 ) ) ;
#81750=CARTESIAN_POINT ( 'NONE',  ( 0.05219959533909260263, 19.03943276465977164, 114.9989096053143669 ) ) ;
#81751=FILL_AREA_STYLE_COLOUR ( '', #56542 ) ;
#81752=CARTESIAN_POINT ( 'NONE',  ( -21.55341960407610458, -5.719274019375992779, 56.45724293864768839 ) ) ;
#81753=CARTESIAN_POINT ( 'NONE',  ( -5.153800228976328057, -19.02544592524343514, 82.29057627198103830 ) ) ;
#81754=CARTESIAN_POINT ( 'NONE',  ( -18.67979575497193778, 10.72451020669871902, 83.33442372801903275 ) ) ;
#81755=CARTESIAN_POINT ( 'NONE',  ( 0.05219959533909260263, 19.03943276465977164, 44.99890960531435979 ) ) ;
#81757=CARTESIAN_POINT ( 'NONE',  ( 16.52544592524342804, -4.483927247898539470, 93.54057627198103830 ) ) ;
#81758=CARTESIAN_POINT ( 'NONE',  ( -8.314922557961024197, 14.29746914071037800, 32.91775706135234714 ) ) ;
#81759=CARTESIAN_POINT ( 'NONE',  ( 0.05219959533937995610, -21.53943276465977519, 65.00109039468568994 ) ) ;
#81761=CARTESIAN_POINT ( 'NONE',  ( -9.474510206698720793, -16.51473224551083518, 19.58442372801899722 ) ) ;
#81762=CARTESIAN_POINT ( 'NONE',  ( 13.89961937509957401, 13.97604488694547697, 76.87609039468566152 ) ) ;
#81764=CARTESIAN_POINT ( 'NONE',  ( 21.52544592524334988, 5.823673210054432836, 41.45942372801901143 ) ) ;
#81766=CARTESIAN_POINT ( 'NONE',  ( -19.02544592524334988, -5.153800228976617603, 28.95942372801900433 ) ) ;
#81767=CARTESIAN_POINT ( 'NONE',  ( 16.46253265017160672, -9.564922557960803928, 53.33224293864768839 ) ) ;
#81768=CARTESIAN_POINT ( 'NONE',  ( -16.51473224551082808, 9.474510206698731452, 33.33442372801899722 ) ) ;
#81769=CARTESIAN_POINT ( 'NONE',  ( -8.314922557961024197, 14.29746914071037800, 97.91775706135236135 ) ) ;
#81770=CARTESIAN_POINT ( 'NONE',  ( 16.46253265017160672, -9.564922557960803928, 103.3322429386476955 ) ) ;
#81771=CARTESIAN_POINT ( 'NONE',  ( -18.62759615963255300, -10.81492255796106328, 74.16775706135231871 ) ) ;
#81773=DIRECTION ( 'NONE',  ( 0.000000000000000000, 0.000000000000000000, -1.000000000000000000 ) ) ;
#81774=CARTESIAN_POINT ( 'NONE',  ( -21.55341960407619339, 5.719274019375674811, 83.54275706135234714 ) ) ;
#81777=CARTESIAN_POINT ( 'NONE',  ( -19.03943276465977164, 0.05219959533909376836, 101.2489096053143669 ) ) ;
#81778=CARTESIAN_POINT ( 'NONE',  ( -13.89961937509957401, -13.97604488694547875, 19.37609039468566507 ) ) ;
#81780=CARTESIAN_POINT ( 'NONE',  ( -0.05219959533909027116, -19.03943276465977164, 32.49890960531435979 ) ) ;
#81781=CARTESIAN_POINT ( 'NONE',  ( 18.67979575497178502, 10.72451020669898547, 59.16557627198103120 ) ) ;
#81782=CARTESIAN_POINT ( 'NONE',  ( 4.483927247898545687, 16.52544592524342804, 24.79057627198103120 ) ) ;
#81783=CARTESIAN_POINT ( 'NONE',  ( -4.379528057220328563, 16.55341960407611168, 100.2072429386476955 ) ) ;
#81784=CARTESIAN_POINT ( 'NONE',  ( -16.46253265017160317, 9.564922557960807481, 75.83224293864769550 ) ) ;
#81785=CARTESIAN_POINT ( 'NONE',  ( 16.46253265017146816, 9.564922557961045513, 26.66775706135234003 ) ) ;
#81786=CARTESIAN_POINT ( 'NONE',  ( -19.05341960407611168, -5.049401038298163336, 41.45724293864769550 ) ) ;
#81787=CARTESIAN_POINT ( 'NONE',  ( 16.52544592524342804, -4.483927247898539470, 108.5405762719810241 ) ) ;
#81788=CARTESIAN_POINT ( 'NONE',  ( -10.72451020669870658, -18.67979575497194134, 59.58442372801901854 ) ) ;
#81789=CARTESIAN_POINT ( 'NONE',  ( -18.62759615963270932, 10.81492255796079327, 90.83224293864769550 ) ) ;
#81790=CARTESIAN_POINT ( 'NONE',  ( 0.05219959533936267826, -19.03943276465977164, 60.00109039468566863 ) ) ;
#81792=CARTESIAN_POINT ( 'NONE',  ( -13.89961937509977652, 13.97604488694528158, 110.6239096053143243 ) ) ;
#81793=CARTESIAN_POINT ( 'NONE',  ( -14.29746914071049879, 8.314922557960819915, 80.83224293864769550 ) ) ;
#81794=CARTESIAN_POINT ( 'NONE',  ( -5.153800228976607833, 19.02544592524334988, 42.70942372801901143 ) ) ;
#81795=CARTESIAN_POINT ( 'NONE',  ( -5.049401038298153566, 19.05341960407611168, 65.20724293864765286 ) ) ;
#81796=CARTESIAN_POINT ( 'NONE',  ( 4.379528057220339221, -16.55341960407611168, 57.70724293864770260 ) ) ;
#81797=CARTESIAN_POINT ( 'NONE',  ( 16.51473224551083163, -9.474510206698727899, 75.83442372801900433 ) ) ;
#81799=CARTESIAN_POINT ( 'NONE',  ( -15.80617190586745835, -15.72974639402198527, 36.87390960531435979 ) ) ;
#81801=CARTESIAN_POINT ( 'NONE',  ( -14.34966873604960291, -8.224510206698953496, 106.6655762719810383 ) ) ;
#81803=CARTESIAN_POINT ( 'NONE',  ( -0.05219959533909027116, -19.03943276465977164, 52.49890960531436690 ) ) ;
#81804=CARTESIAN_POINT ( 'NONE',  ( -21.52544592524343514, 5.823673210054127303, 56.04057627198102409 ) ) ;
#81805=CARTESIAN_POINT ( 'NONE',  ( -9.474510206698964154, 16.51473224551069663, 35.41557627198102409 ) ) ;
#81806=CARTESIAN_POINT ( 'NONE',  ( -14.29746914071037622, -8.314922557961029526, 84.16775706135234714 ) ) ;
#81807=CARTESIAN_POINT ( 'NONE',  ( -5.153800228976328057, -19.02544592524343514, 77.29057627198099567 ) ) ;
#81808=CARTESIAN_POINT ( 'NONE',  ( -0.05219959533936034679, 19.03943276465977164, 57.50109039468566863 ) ) ;
#81809=CARTESIAN_POINT ( 'NONE',  ( -10.81492255796105439, 18.62759615963255655, 62.91775706135236135 ) ) ;
#81810=CARTESIAN_POINT ( 'NONE',  ( 10.81492255796078972, 18.62759615963270932, 54.58224293864769550 ) ) ;
#81811=CARTESIAN_POINT ( 'NONE',  ( -4.379528057220328563, 16.55341960407611168, 115.2072429386476955 ) ) ;
#81812=CARTESIAN_POINT ( 'NONE',  ( 16.52544592524335698, 4.483927247898782831, 86.45942372801901854 ) ) ;
#81813=CARTESIAN_POINT ( 'NONE',  ( 9.564922557961047289, -16.46253265017146816, 110.4177570613523471 ) ) ;
#81815=CARTESIAN_POINT ( 'NONE',  ( 19.49671883438228548, 5.499999999999968914, 77.39279849105680853 ) ) ;
#81816=CARTESIAN_POINT ( 'NONE',  ( -10.81492255796105439, 18.62759615963255655, 92.91775706135236135 ) ) ;
#81818=CARTESIAN_POINT ( 'NONE',  ( -14.29746914071049879, 8.314922557960819915, 40.83224293864769550 ) ) ;
#81819=CARTESIAN_POINT ( 'NONE',  ( -0.05219959533910754901, -16.53943276465976808, 57.49890960531435979 ) ) ;
#81820=CARTESIAN_POINT ( 'NONE',  ( -18.62759615963270932, 10.81492255796079327, 95.83224293864770971 ) ) ;
#81821=CARTESIAN_POINT ( 'NONE',  ( 15.80617190586746368, 15.72974639402197994, 94.37390960531436690 ) ) ;
#81823=CARTESIAN_POINT ( 'NONE',  ( -21.53943276465977519, 0.05219959533907696930, 26.24890960531435624 ) ) ;
#81824=CARTESIAN_POINT ( 'NONE',  ( 8.224510206698742110, 14.34966873604972548, 62.08442372801901143 ) ) ;
#81825=CARTESIAN_POINT ( 'NONE',  ( -8.224510206698948167, 14.34966873604960824, 80.41557627198103830 ) ) ;
#81826=CARTESIAN_POINT ( 'NONE',  ( 16.46253265017160672, -9.564922557960803928, 43.33224293864769550 ) ) ;
#81828=CARTESIAN_POINT ( 'NONE',  ( -12.06949235617739369, -12.14591786802326823, 94.37609039468568994 ) ) ;
#81829=CARTESIAN_POINT ( 'NONE',  ( 21.55341960407619695, -5.719274019375665929, 21.04275706135234714 ) ) ;
#81830=CARTESIAN_POINT ( 'NONE',  ( -16.51473224551069308, -9.474510206698971260, 86.66557627198102409 ) ) ;
#81831=CARTESIAN_POINT ( 'NONE',  ( -15.72974639402176322, -15.80617190586768395, 54.37609039468568994 ) ) ;
#81832=CARTESIAN_POINT ( 'NONE',  ( 19.05341960407611168, 5.049401038298154454, 103.9572429386476671 ) ) ;
#81835=CARTESIAN_POINT ( 'NONE',  ( -18.62759615963255300, -10.81492255796106328, 49.16775706135234003 ) ) ;
#81836=CARTESIAN_POINT ( 'NONE',  ( 19.02544592524343514, -5.153800228976328945, 43.54057627198103120 ) ) ;
#81838=CARTESIAN_POINT ( 'NONE',  ( 19.05341960407617918, -5.049401038297876454, 56.04275706135234714 ) ) ;
#81839=CARTESIAN_POINT ( 'NONE',  ( -15.80617190586768217, 15.72974639402176855, 33.12609039468569705 ) ) ;
#81840=CARTESIAN_POINT ( 'NONE',  ( 5.049401038297881783, 19.05341960407617563, 57.29275706135231871 ) ) ;
#81841=CARTESIAN_POINT ( 'NONE',  ( 0.05219959533909260263, 19.03943276465977164, 29.99890960531435979 ) ) ;
#81842=CARTESIAN_POINT ( 'NONE',  ( -4.483927247898782831, 16.52544592524335698, 87.70942372801901854 ) ) ;
#81843=CARTESIAN_POINT ( 'NONE',  ( -16.51473224551082808, 9.474510206698731452, 58.33442372801900433 ) ) ;
#81844=CARTESIAN_POINT ( 'NONE',  ( -12.06949235617739369, -12.14591786802326823, 99.37609039468568994 ) ) ;
#81846=ORIENTED_EDGE ( 'NONE', *, *, #64444, .F. ) ;
#81847=CARTESIAN_POINT ( 'NONE',  ( 16.46253265017160672, -9.564922557960803928, 88.33224293864769550 ) ) ;
#81848=CARTESIAN_POINT ( 'NONE',  ( 10.81492255796106328, -18.62759615963255655, 90.41775706135236135 ) ) ;
#81849=CARTESIAN_POINT ( 'NONE',  ( -21.53943276465977519, -0.05219959533937600094, 108.7510903946857042 ) ) ;
#81850=CARTESIAN_POINT ( 'NONE',  ( -18.22780087662124160, -5.499999999999927169, 88.98236817873107896 ) ) ;
#81851=CARTESIAN_POINT ( 'NONE',  ( 10.72451020669871369, 18.67979575497193778, 72.08442372801899012 ) ) ;
#81852=CARTESIAN_POINT ( 'NONE',  ( 16.55341960407618274, -4.379528057220086978, 36.04275706135234714 ) ) ;
#81853=CARTESIAN_POINT ( 'NONE',  ( 19.03943276465977164, -0.05219959533909143690, 78.74890960531436690 ) ) ;
#81854=CARTESIAN_POINT ( 'NONE',  ( 10.72451020669898902, -18.67979575497178502, 27.91557627198103830 ) ) ;
#81858=CARTESIAN_POINT ( 'NONE',  ( -5.049401038298153566, 19.05341960407611168, 60.20724293864768129 ) ) ;
#81859=CARTESIAN_POINT ( 'NONE',  ( -14.34966873604972548, 8.224510206698743886, 113.3344237280190328 ) ) ;
#81860=CARTESIAN_POINT ( 'NONE',  ( -17.44270441346520784, 5.991230190322873739, 98.63664920735773478 ) ) ;
#81861=CARTESIAN_POINT ( 'NONE',  ( -5.153800228976607833, 19.02544592524334988, 72.70942372801900433 ) ) ;
#81862=CARTESIAN_POINT ( 'NONE',  ( -9.564922557960796823, -16.46253265017161027, 102.0822429386477097 ) ) ;
#81863=CARTESIAN_POINT ( 'NONE',  ( -21.53943276465977519, -0.05219959533937600094, 98.75109039468568994 ) ) ;
#81864=CARTESIAN_POINT ( 'NONE',  ( -14.34966873604960291, -8.224510206698953496, 91.66557627198103830 ) ) ;
#81865=CARTESIAN_POINT ( 'NONE',  ( -21.55341960407610458, -5.719274019375992779, 51.45724293864770260 ) ) ;
#81866=CARTESIAN_POINT ( 'NONE',  ( -10.81492255796078084, -18.62759615963271287, 37.08224293864768129 ) ) ;
#81867=CARTESIAN_POINT ( 'NONE',  ( 16.52544592524342804, -4.483927247898539470, 103.5405762719810383 ) ) ;
#81869=CARTESIAN_POINT ( 'NONE',  ( -19.02544592524334988, -5.153800228976617603, 58.95942372801900433 ) ) ;
#81870=CARTESIAN_POINT ( 'NONE',  ( 12.14591786802309770, 12.06949235617756955, 24.37390960531435979 ) ) ;
#81871=CARTESIAN_POINT ( 'NONE',  ( 19.05341960407611168, 5.049401038298154454, 103.9572429386476671 ) ) ;
#81872=CARTESIAN_POINT ( 'NONE',  ( -15.72974639402176322, -15.80617190586768395, 69.37609039468567573 ) ) ;
#81873=CARTESIAN_POINT ( 'NONE',  ( -5.823673210054116645, -21.52544592524344225, 62.29057627198102409 ) ) ;
#81874=CARTESIAN_POINT ( 'NONE',  ( 21.55341960407619695, -5.719274019375665929, 46.04275706135234714 ) ) ;
#81875=CARTESIAN_POINT ( 'NONE',  ( 10.72451020669898902, -18.67979575497178502, 102.9155762719810383 ) ) ;
#81876=CARTESIAN_POINT ( 'NONE',  ( 21.53943276465977519, 0.05219959533937863772, 36.25109039468567573 ) ) ;
#81877=CARTESIAN_POINT ( 'NONE',  ( -5.049401038298153566, 19.05341960407611168, 30.20724293864768839 ) ) ;
#81878=CARTESIAN_POINT ( 'NONE',  ( 5.049401038297881783, 19.05341960407617563, 67.29275706135234714 ) ) ;
#81879=CARTESIAN_POINT ( 'NONE',  ( 16.53943276465976808, -0.05219959533910856209, 98.74890960531438111 ) ) ;
#81880=CARTESIAN_POINT ( 'NONE',  ( 19.02544592524343514, -5.153800228976328945, 108.5405762719810383 ) ) ;
#81881=CARTESIAN_POINT ( 'NONE',  ( -12.06949235617756955, 12.14591786802309770, 55.62390960531436690 ) ) ;
#81882=CARTESIAN_POINT ( 'NONE',  ( 8.314922557961029526, -14.29746914071037800, 110.4177570613523756 ) ) ;
#81883=CARTESIAN_POINT ( 'NONE',  ( -5.153800228976328057, -19.02544592524343514, 52.29057627198100988 ) ) ;
#81884=CARTESIAN_POINT ( 'NONE',  ( 0.05219959533910956823, 16.53943276465976808, 114.9989096053143669 ) ) ;
#81885=CARTESIAN_POINT ( 'NONE',  ( 18.67979575497178502, 10.72451020669898547, 29.16557627198103120 ) ) ;
#81886=CARTESIAN_POINT ( 'NONE',  ( -13.89961937509957401, -13.97604488694547875, 19.37609039468566507 ) ) ;
#81887=CARTESIAN_POINT ( 'NONE',  ( 18.09867054820434262, 5.499999999999818812, 51.48393025253587751 ) ) ;
#81888=CARTESIAN_POINT ( 'NONE',  ( 12.14591786802309770, 12.06949235617756955, 34.37390960531435979 ) ) ;
#81889=CARTESIAN_POINT ( 'NONE',  ( -15.80617190586768217, 15.72974639402176855, 53.12609039468568284 ) ) ;
#81891=CARTESIAN_POINT ( 'NONE',  ( -16.53943276465976808, -0.05219959533934237506, 63.75109039468568284 ) ) ;
#81892=CARTESIAN_POINT ( 'NONE',  ( -5.153800228976607833, 19.02544592524334988, 62.70942372801899722 ) ) ;
#81893=CARTESIAN_POINT ( 'NONE',  ( -16.55341960407611168, -4.379528057220339221, 31.45724293864769550 ) ) ;
#81894=CARTESIAN_POINT ( 'NONE',  ( -0.05219959533934338120, 16.53943276465976808, 112.5010903946857042 ) ) ;
#81895=CARTESIAN_POINT ( 'NONE',  ( 19.05341960407611168, 5.049401038298154454, 43.95724293864769550 ) ) ;
#81896=CARTESIAN_POINT ( 'NONE',  ( 13.89961937509977652, -13.97604488694527269, 63.12390960531435979 ) ) ;
#81897=CARTESIAN_POINT ( 'NONE',  ( 16.46253265017160672, -9.564922557960803928, 28.33224293864769550 ) ) ;
#81898=CARTESIAN_POINT ( 'NONE',  ( -15.80617190586768217, 15.72974639402176855, 33.12609039468569705 ) ) ;
#81899=CARTESIAN_POINT ( 'NONE',  ( 16.51473224551069308, 9.474510206698969483, 39.16557627198103120 ) ) ;
#81901=CARTESIAN_POINT ( 'NONE',  ( -19.05341960407611168, -5.049401038298163336, 36.45724293864766707 ) ) ;
#81902=CARTESIAN_POINT ( 'NONE',  ( -5.719274019375978568, 21.55341960407610458, 25.20724293864769550 ) ) ;
#81903=CARTESIAN_POINT ( 'NONE',  ( 0.05219959533937995610, -21.53943276465977519, 60.00109039468568284 ) ) ;
#81904=CARTESIAN_POINT ( 'NONE',  ( -16.55341960407611168, -4.379528057220339221, 106.4572429386477097 ) ) ;
#81905=CARTESIAN_POINT ( 'NONE',  ( 13.97604488694527802, 13.89961937509977652, 109.3739096053143669 ) ) ;
#81906=CARTESIAN_POINT ( 'NONE',  ( -12.14591786802326823, 12.06949235617739902, 78.12609039468570415 ) ) ;
#81907=CARTESIAN_POINT ( 'NONE',  ( -10.72451020669870658, -18.67979575497194134, 89.58442372801901854 ) ) ;
#81908=CARTESIAN_POINT ( 'NONE',  ( 12.06949235617739724, 12.14591786802326823, 51.87609039468568284 ) ) ;
#81909=CARTESIAN_POINT ( 'NONE',  ( -16.51473224551069308, -9.474510206698971260, 96.66557627198102409 ) ) ;
#81910=CARTESIAN_POINT ( 'NONE',  ( -16.55341960407617563, 4.379528057220093196, 38.54275706135234714 ) ) ;
#81911=CARTESIAN_POINT ( 'NONE',  ( -14.34966873604972548, 8.224510206698743886, 33.33442372801900433 ) ) ;
#81912=CARTESIAN_POINT ( 'NONE',  ( 8.224510206698742110, 14.34966873604972548, 82.08442372801901854 ) ) ;
#81913=CARTESIAN_POINT ( 'NONE',  ( 16.46253265017146816, 9.564922557961045513, 111.6677570613523329 ) ) ;
#81914=CARTESIAN_POINT ( 'NONE',  ( 15.72974639402199770, -15.80617190586745480, 103.1239096053143811 ) ) ;
#81915=CARTESIAN_POINT ( 'NONE',  ( 16.53943276465976808, -0.05219959533910856209, 98.74890960531438111 ) ) ;
#81916=CARTESIAN_POINT ( 'NONE',  ( -13.89961937509957401, -13.97604488694547875, 104.3760903946856757 ) ) ;
#81917=CARTESIAN_POINT ( 'NONE',  ( 16.53943276465976808, 0.05219959533934440121, 76.25109039468568994 ) ) ;
#81919=CARTESIAN_POINT ( 'NONE',  ( 5.049401038297881783, 19.05341960407617563, 67.29275706135234714 ) ) ;
#81920=CARTESIAN_POINT ( 'NONE',  ( 16.53943276465976808, -0.05219959533910856209, 48.74890960531435979 ) ) ;
#81921=CARTESIAN_POINT ( 'NONE',  ( -4.379528057220328563, 16.55341960407611168, 35.20724293864768839 ) ) ;
#81922=CARTESIAN_POINT ( 'NONE',  ( 14.34966873604960469, 8.224510206698951720, 99.16557627198100988 ) ) ;
#81923=CARTESIAN_POINT ( 'NONE',  ( -13.97604488694547697, 13.89961937509957934, 33.12609039468566863 ) ) ;
#81925=CARTESIAN_POINT ( 'NONE',  ( -18.62759615963255300, -10.81492255796106328, 39.16775706135235424 ) ) ;
#81926=CARTESIAN_POINT ( 'NONE',  ( 9.474510206698729675, 16.51473224551082808, 92.08442372801900433 ) ) ;
#81927=CARTESIAN_POINT ( 'NONE',  ( 0.05219959533909260263, 19.03943276465977164, 109.9989096053143669 ) ) ;
#81928=CARTESIAN_POINT ( 'NONE',  ( 9.474510206698971260, -16.51473224551069308, 97.91557627198102409 ) ) ;
#81929=CARTESIAN_POINT ( 'NONE',  ( -19.02544592524342804, 5.153800228976336051, 86.04057627198103830 ) ) ;
#81930=CARTESIAN_POINT ( 'NONE',  ( -0.05219959533907301413, -21.53943276465977519, 57.49890960531435979 ) ) ;
#81931=CARTESIAN_POINT ( 'NONE',  ( -16.53943276465976808, 0.05219959533911058130, 91.24890960531436690 ) ) ;
#81932=CARTESIAN_POINT ( 'NONE',  ( -9.564922557960796823, -16.46253265017161027, 72.08224293864770971 ) ) ;
#81933=CARTESIAN_POINT ( 'NONE',  ( -0.05219959533910754901, -16.53943276465976808, 112.4989096053143669 ) ) ;
#81935=CARTESIAN_POINT ( 'NONE',  ( -5.719274019375665041, -21.55341960407619695, 39.79275706135235424 ) ) ;
#81936=CARTESIAN_POINT ( 'NONE',  ( -15.80617190586768217, 15.72974639402176855, 78.12609039468570415 ) ) ;
#81937=CARTESIAN_POINT ( 'NONE',  ( 16.46253265017160672, -9.564922557960803928, 58.33224293864769550 ) ) ;
#81938=CARTESIAN_POINT ( 'NONE',  ( 4.483927247898790824, -16.52544592524335698, 80.20942372801901854 ) ) ;
#81940=CARTESIAN_POINT ( 'NONE',  ( -18.67979575497193778, 10.72451020669871902, 28.33442372801902209 ) ) ;
#81941=CARTESIAN_POINT ( 'NONE',  ( 21.52544592524334988, 5.823673210054432836, 26.45942372801901854 ) ) ;
#81942=CARTESIAN_POINT ( 'NONE',  ( 13.89961937509957401, 13.97604488694547697, 51.87609039468566863 ) ) ;
#81943=CARTESIAN_POINT ( 'NONE',  ( 5.153800228976335163, 19.02544592524342804, 84.79057627198099567 ) ) ;
#81944=CARTESIAN_POINT ( 'NONE',  ( 9.474510206698729675, 16.51473224551082808, 27.08442372801900433 ) ) ;
#81945=CARTESIAN_POINT ( 'NONE',  ( 5.823673210054444382, -21.52544592524334988, 90.20942372801903275 ) ) ;
#81946=CARTESIAN_POINT ( 'NONE',  ( -10.72451020669898014, 18.67979575497178502, 65.41557627198102409 ) ) ;
#81947=CARTESIAN_POINT ( 'NONE',  ( 16.53943276465976808, -0.05219959533910856209, 53.74890960531437401 ) ) ;
#81948=CARTESIAN_POINT ( 'NONE',  ( 10.72451020669871369, 18.67979575497193778, 87.08442372801901854 ) ) ;
#81949=CARTESIAN_POINT ( 'NONE',  ( 16.51473224551083163, -9.474510206698727899, 30.83442372801900433 ) ) ;
#81950=CARTESIAN_POINT ( 'NONE',  ( -14.34966873604960291, -8.224510206698953496, 71.66557627198100988 ) ) ;
#81951=CARTESIAN_POINT ( 'NONE',  ( 19.03943276465977164, -0.05219959533909143690, 28.74890960531435624 ) ) ;
#81952=CARTESIAN_POINT ( 'NONE',  ( -13.97604488694547697, 13.89961937509957934, 63.12609039468566152 ) ) ;
#81953=CARTESIAN_POINT ( 'NONE',  ( -4.483927247898539470, -16.52544592524342804, 32.29057627198102409 ) ) ;
#81954=CARTESIAN_POINT ( 'NONE',  ( -21.53943276465977519, -0.05219959533937600094, 78.75109039468568994 ) ) ;
#81955=CARTESIAN_POINT ( 'NONE',  ( -19.02544592524342804, 5.153800228976336051, 81.04057627198103830 ) ) ;
#81956=CARTESIAN_POINT ( 'NONE',  ( 16.46253265017146816, 9.564922557961045513, 51.66775706135233293 ) ) ;
#81957=CARTESIAN_POINT ( 'NONE',  ( 18.62759615963271287, -10.81492255796078972, 48.33224293864770260 ) ) ;
#81958=CARTESIAN_POINT ( 'NONE',  ( 18.62759615963255655, 10.81492255796105972, 41.66775706135235424 ) ) ;
#81959=CARTESIAN_POINT ( 'NONE',  ( 10.72451020669898902, -18.67979575497178502, 97.91557627198103830 ) ) ;
#81960=CARTESIAN_POINT ( 'NONE',  ( 13.97604488694548053, -13.89961937509957401, 95.62609039468563310 ) ) ;
#81961=CARTESIAN_POINT ( 'NONE',  ( -4.483927247898782831, 16.52544592524335698, 62.70942372801902565 ) ) ;
#81963=CARTESIAN_POINT ( 'NONE',  ( -21.55341960407610458, -5.719274019375992779, 101.4572429386476955 ) ) ;
#81964=CARTESIAN_POINT ( 'NONE',  ( 4.379528057220339221, -16.55341960407611168, 107.7072429386476955 ) ) ;
#81965=CARTESIAN_POINT ( 'NONE',  ( -17.50000000000011724, -3.292511757969963870, 29.93479729789457977 ) ) ;
#81966=CARTESIAN_POINT ( 'NONE',  ( -12.14591786802326823, 12.06949235617739902, 33.12609039468569705 ) ) ;
#81968=CARTESIAN_POINT ( 'NONE',  ( -10.81492255796078084, -18.62759615963271287, 62.08224293864769550 ) ) ;
#81969=CARTESIAN_POINT ( 'NONE',  ( 16.55341960407618274, -4.379528057220086978, 106.0427570613523471 ) ) ;
#81970=CARTESIAN_POINT ( 'NONE',  ( 19.05341960407611168, 5.049401038298154454, 28.95724293864769550 ) ) ;
#81971=CARTESIAN_POINT ( 'NONE',  ( 16.52544592524335698, 4.483927247898782831, 61.45942372801901854 ) ) ;
#81972=CARTESIAN_POINT ( 'NONE',  ( -5.049401038297874678, -19.05341960407617918, 59.79275706135231871 ) ) ;
#81973=CARTESIAN_POINT ( 'NONE',  ( 18.67979575497194134, -10.72451020669871369, 35.83442372801901143 ) ) ;
#81974=CARTESIAN_POINT ( 'NONE',  ( 5.719274019375991003, -21.55341960407610458, 52.70724293864769550 ) ) ;
#81975=CARTESIAN_POINT ( 'NONE',  ( -0.05219959533934338120, 16.53943276465976808, 92.50109039468567573 ) ) ;
#81976=CARTESIAN_POINT ( 'NONE',  ( -15.72974639402176322, -15.80617190586768395, 74.37609039468568994 ) ) ;
#81977=CARTESIAN_POINT ( 'NONE',  ( 0.05219959533907565091, 21.53943276465977519, 49.99890960531437401 ) ) ;
#81978=CARTESIAN_POINT ( 'NONE',  ( 15.80617190586746368, 15.72974639402197994, 39.37390960531436690 ) ) ;
#81979=EDGE_LOOP ( 'NONE', ( #3982, #157724, #70324, #80863 ) ) ;
#81980=CARTESIAN_POINT ( 'NONE',  ( -4.483927247898782831, 16.52544592524335698, 72.70942372801901854 ) ) ;
#81981=CARTESIAN_POINT ( 'NONE',  ( 5.719274019375991003, -21.55341960407610458, 27.70724293864769905 ) ) ;
#81983=CARTESIAN_POINT ( 'NONE',  ( 16.46253265017160672, -9.564922557960803928, 103.3322429386476955 ) ) ;
#81984=CARTESIAN_POINT ( 'NONE',  ( -8.314922557961024197, 14.29746914071037800, 107.9177570613523471 ) ) ;
#81986=CARTESIAN_POINT ( 'NONE',  ( 16.52544592524342804, -4.483927247898539470, 103.5405762719810383 ) ) ;
#81987=CARTESIAN_POINT ( 'NONE',  ( 21.55341960407610458, 5.719274019375980345, 58.95724293864770971 ) ) ;
#81988=CARTESIAN_POINT ( 'NONE',  ( 4.483927247898790824, -16.52544592524335698, 90.20942372801903275 ) ) ;
#81989=CARTESIAN_POINT ( 'NONE',  ( 0.05219959533937995610, -21.53943276465977519, 50.00109039468568994 ) ) ;
#81990=CARTESIAN_POINT ( 'NONE',  ( 13.89961937509957401, 13.97604488694547697, 106.8760903946856757 ) ) ;
#81991=CARTESIAN_POINT ( 'NONE',  ( -12.06949235617756955, 12.14591786802309770, 100.6239096053143811 ) ) ;
#81992=CARTESIAN_POINT ( 'NONE',  ( 13.89961937509977652, -13.97604488694527269, 48.12390960531435979 ) ) ;
#81993=CARTESIAN_POINT ( 'NONE',  ( 5.049401038298161559, -19.05341960407611168, 32.70724293864768129 ) ) ;
#81994=CARTESIAN_POINT ( 'NONE',  ( 17.50000000000000355, -5.624438216177593652, 38.31670344914644488 ) ) ;
#81995=CARTESIAN_POINT ( 'NONE',  ( -19.05341960407611168, -5.049401038298163336, 86.45724293864769550 ) ) ;
#81996=CARTESIAN_POINT ( 'NONE',  ( -16.52544592524335698, -4.483927247898792601, 73.95942372801901854 ) ) ;
#81997=CARTESIAN_POINT ( 'NONE',  ( 10.72451020669871369, 18.67979575497193778, 112.0844237280190185 ) ) ;
#81998=CARTESIAN_POINT ( 'NONE',  ( 15.80617190586746368, 15.72974639402197994, 49.37390960531436690 ) ) ;
#81999=CARTESIAN_POINT ( 'NONE',  ( 8.224510206698742110, 14.34966873604972548, 67.08442372801901854 ) ) ;
#82000=CARTESIAN_POINT ( 'NONE',  ( -13.97604488694547697, 13.89961937509957934, 83.12609039468564731 ) ) ;
#82002=CARTESIAN_POINT ( 'NONE',  ( -5.153800228976328057, -19.02544592524343514, 37.29057627198102409 ) ) ;
#82003=CARTESIAN_POINT ( 'NONE',  ( -16.51473224551069308, -9.474510206698971260, 81.66557627198103830 ) ) ;
#82004=CARTESIAN_POINT ( 'NONE',  ( -9.564922557960796823, -16.46253265017161027, 37.08224293864768839 ) ) ;
#82005=CARTESIAN_POINT ( 'NONE',  ( 5.049401038297881783, 19.05341960407617563, 72.29275706135234714 ) ) ;
#82007=CARTESIAN_POINT ( 'NONE',  ( 16.51473224551069308, 9.474510206698969483, 99.16557627198102409 ) ) ;
#82008=CARTESIAN_POINT ( 'NONE',  ( 16.55341960407611168, 4.379528057220329451, 53.95724293864770260 ) ) ;
#82009=CARTESIAN_POINT ( 'NONE',  ( -5.823673210054116645, -21.52544592524344225, 62.29057627198102409 ) ) ;
#82010=CARTESIAN_POINT ( 'NONE',  ( -17.50000000000000000, 3.345213924137368622, 104.5876862309435182 ) ) ;
#82011=CARTESIAN_POINT ( 'NONE',  ( -0.05219959533936034679, 19.03943276465977164, 32.50109039468566863 ) ) ;
#82013=CARTESIAN_POINT ( 'NONE',  ( 13.89961937509977652, -13.97604488694527269, 48.12390960531435979 ) ) ;
#82014=CARTESIAN_POINT ( 'NONE',  ( 5.049401038298161559, -19.05341960407611168, 57.70724293864769550 ) ) ;
#82015=CARTESIAN_POINT ( 'NONE',  ( -4.379528057220086978, -16.55341960407618274, 39.79275706135235424 ) ) ;
#82017=CARTESIAN_POINT ( 'NONE',  ( -16.52216118717207038, 7.221426719304506747, 108.9240097895301318 ) ) ;
#82018=CARTESIAN_POINT ( 'NONE',  ( -4.379528057220086978, -16.55341960407618274, 74.79275706135234714 ) ) ;
#82019=CARTESIAN_POINT ( 'NONE',  ( -5.823673210054116645, -21.52544592524344225, 97.29057627198105251 ) ) ;
#82021=CARTESIAN_POINT ( 'NONE',  ( 12.14591786802327356, -12.06949235617739191, 40.62609039468567573 ) ) ;
#82022=CARTESIAN_POINT ( 'NONE',  ( 16.51473224551069308, 9.474510206698969483, 39.16557627198103120 ) ) ;
#82023=CARTESIAN_POINT ( 'NONE',  ( 15.72974639402176855, 15.80617190586768217, 51.87609039468568284 ) ) ;
#82024=CARTESIAN_POINT ( 'NONE',  ( -5.049401038297874678, -19.05341960407617918, 64.79275706135233293 ) ) ;
#82025=CARTESIAN_POINT ( 'NONE',  ( -15.72974639402176322, -15.80617190586768395, 99.37609039468568994 ) ) ;
#82026=CARTESIAN_POINT ( 'NONE',  ( 5.049401038298161559, -19.05341960407611168, 22.70724293864769194 ) ) ;
#82027=CARTESIAN_POINT ( 'NONE',  ( -12.14591786802309592, -12.06949235617757132, 41.87390960531435979 ) ) ;
#82028=CARTESIAN_POINT ( 'NONE',  ( 19.39720447994797325, 5.499999999999973355, 42.16317477297180005 ) ) ;
#82029=CARTESIAN_POINT ( 'NONE',  ( 18.67979575497178502, 10.72451020669898547, 59.16557627198103120 ) ) ;
#82031=CARTESIAN_POINT ( 'NONE',  ( -9.564922557960796823, -16.46253265017161027, 97.08224293864769550 ) ) ;
#82032=CARTESIAN_POINT ( 'NONE',  ( 16.55341960407611168, 4.379528057220329451, 98.95724293864770971 ) ) ;
#82033=CARTESIAN_POINT ( 'NONE',  ( 12.14591786802327356, -12.06949235617739191, 20.62609039468568639 ) ) ;
#82034=CARTESIAN_POINT ( 'NONE',  ( 8.314922557961029526, -14.29746914071037800, 105.4177570613523613 ) ) ;
#82037=CARTESIAN_POINT ( 'NONE',  ( 10.81492255796078972, 18.62759615963270932, 104.5822429386477097 ) ) ;
#82038=CARTESIAN_POINT ( 'NONE',  ( 4.483927247898545687, 16.52544592524342804, 24.79057627198103120 ) ) ;
#82039=CARTESIAN_POINT ( 'NONE',  ( 13.97604488694527802, 13.89961937509977652, 114.3739096053143669 ) ) ;
#82040=CARTESIAN_POINT ( 'NONE',  ( 5.049401038297881783, 19.05341960407617563, 87.29275706135234714 ) ) ;
#82041=CARTESIAN_POINT ( 'NONE',  ( -5.719274019375665041, -21.55341960407619695, 104.7927570613523898 ) ) ;
#82042=CARTESIAN_POINT ( 'NONE',  ( 8.314922557960818139, 14.29746914071049879, 24.58224293864768839 ) ) ;
#82043=CARTESIAN_POINT ( 'NONE',  ( -0.05219959533907301413, -21.53943276465977519, 87.49890960531436690 ) ) ;
#82045=CARTESIAN_POINT ( 'NONE',  ( -5.719274019375978568, 21.55341960407610458, 55.20724293864770260 ) ) ;
#82047=CARTESIAN_POINT ( 'NONE',  ( 19.03943276465977164, -0.05219959533909143690, 58.74890960531435979 ) ) ;
#82048=CARTESIAN_POINT ( 'NONE',  ( 16.55341960407611168, 4.379528057220329451, 28.95724293864769905 ) ) ;
#82049=CARTESIAN_POINT ( 'NONE',  ( 5.153800228976335163, 19.02544592524342804, 79.79057627198102409 ) ) ;
#82050=CARTESIAN_POINT ( 'NONE',  ( 19.48894818550245844, -5.499999999999921840, 62.60307310435241135 ) ) ;
#82051=CARTESIAN_POINT ( 'NONE',  ( 9.564922557961047289, -16.46253265017146816, 40.41775706135234003 ) ) ;
#82052=CARTESIAN_POINT ( 'NONE',  ( -21.55341960407610458, -5.719274019375992779, 81.45724293864769550 ) ) ;
#82053=CARTESIAN_POINT ( 'NONE',  ( 12.14591786802309770, 12.06949235617756955, 89.37390960531435269 ) ) ;
#82054=AXIS2_PLACEMENT_3D ( 'NONE', #82060, #99242, #83075 ) ;
#82055=CARTESIAN_POINT ( 'NONE',  ( -18.67979575497193778, 10.72451020669871902, 38.33442372801900433 ) ) ;
#82057=CARTESIAN_POINT ( 'NONE',  ( 12.06949235617739724, 12.14591786802326823, 106.8760903946856899 ) ) ;
#82058=CARTESIAN_POINT ( 'NONE',  ( 19.02544592524343514, -5.153800228976328945, 38.54057627198103120 ) ) ;
#82059=CARTESIAN_POINT ( 'NONE',  ( -9.564922557960796823, -16.46253265017161027, 87.08224293864769550 ) ) ;
#82060=CARTESIAN_POINT ( 'NONE',  ( 0.000000000000000000, 0.000000000000000000, 0.000000000000000000 ) ) ;
#82061=CARTESIAN_POINT ( 'NONE',  ( -9.474510206698964154, 16.51473224551069663, 35.41557627198102409 ) ) ;
#82062=CARTESIAN_POINT ( 'NONE',  ( 4.379528057220339221, -16.55341960407611168, 47.70724293864770260 ) ) ;
#82063=CARTESIAN_POINT ( 'NONE',  ( -18.67979575497193778, 10.72451020669871902, 73.33442372801901854 ) ) ;
#82065=CARTESIAN_POINT ( 'NONE',  ( 0.05219959533934541429, -16.53943276465976808, 65.00109039468568994 ) ) ;
#82066=CARTESIAN_POINT ( 'NONE',  ( -19.05341960407611168, -5.049401038298163336, 41.45724293864769550 ) ) ;
#82067=CARTESIAN_POINT ( 'NONE',  ( -19.02544592524342804, 5.153800228976336051, 56.04057627198100988 ) ) ;
#82069=CARTESIAN_POINT ( 'NONE',  ( -5.823673210054431948, 21.52544592524334988, 112.7094237280190328 ) ) ;
#82070=CARTESIAN_POINT ( 'NONE',  ( 14.34966873604972726, -8.224510206698740333, 55.83442372801901854 ) ) ;
#82071=CARTESIAN_POINT ( 'NONE',  ( 0.05219959533937995610, -21.53943276465977519, 100.0010903946857042 ) ) ;
#82072=CARTESIAN_POINT ( 'NONE',  ( -21.53943276465977519, 0.05219959533907696930, 41.24890960531435269 ) ) ;
#82073=CARTESIAN_POINT ( 'NONE',  ( 16.51473224551083163, -9.474510206698727899, 105.8344237280190043 ) ) ;
#82074=CARTESIAN_POINT ( 'NONE',  ( 18.62759615963255655, 10.81492255796105972, 66.66775706135234714 ) ) ;
#82075=CARTESIAN_POINT ( 'NONE',  ( 12.06949235617739724, 12.14591786802326823, 31.87609039468567929 ) ) ;
#82076=CARTESIAN_POINT ( 'NONE',  ( 5.823673210054125526, 21.52544592524343514, 104.7905762719810241 ) ) ;
#82077=CARTESIAN_POINT ( 'NONE',  ( 9.564922557961047289, -16.46253265017146816, 95.41775706135233293 ) ) ;
#82078=CARTESIAN_POINT ( 'NONE',  ( -16.51473224551069308, -9.474510206698971260, 71.66557627198102409 ) ) ;
#82079=CARTESIAN_POINT ( 'NONE',  ( 16.51473224551083163, -9.474510206698727899, 110.8344237280190043 ) ) ;
#82081=CARTESIAN_POINT ( 'NONE',  ( 9.474510206698729675, 16.51473224551082808, 102.0844237280190043 ) ) ;
#82082=CARTESIAN_POINT ( 'NONE',  ( 12.06949235617757843, -12.14591786802309237, 63.12390960531435979 ) ) ;
#82083=CARTESIAN_POINT ( 'NONE',  ( -12.14591786802326823, 12.06949235617739902, 73.12609039468567573 ) ) ;
#82084=CARTESIAN_POINT ( 'NONE',  ( 21.55341960407619695, -5.719274019375665929, 21.04275706135234714 ) ) ;
#82085=CARTESIAN_POINT ( 'NONE',  ( 9.474510206698971260, -16.51473224551069308, 57.91557627198103120 ) ) ;
#82086=CARTESIAN_POINT ( 'NONE',  ( -0.05219959533909027116, -19.03943276465977164, 52.49890960531436690 ) ) ;
#82087=CARTESIAN_POINT ( 'NONE',  ( 4.379528057220092307, 16.55341960407617563, 67.29275706135234714 ) ) ;
#82092=CARTESIAN_POINT ( 'NONE',  ( 10.72451020669871369, 18.67979575497193778, 112.0844237280190185 ) ) ;
#82093=CARTESIAN_POINT ( 'NONE',  ( -19.03943276465977164, 0.05219959533909376836, 21.24890960531436335 ) ) ;
#82095=CARTESIAN_POINT ( 'NONE',  ( -19.03943276465977164, -0.05219959533935918106, 113.7510903946856757 ) ) ;
#82096=CARTESIAN_POINT ( 'NONE',  ( -21.52544592524343514, 5.823673210054127303, 46.04057627198103830 ) ) ;
#82097=CARTESIAN_POINT ( 'NONE',  ( -19.02544592524334988, -5.153800228976617603, 48.95942372801900433 ) ) ;
#82098=CARTESIAN_POINT ( 'NONE',  ( -12.06949235617739369, -12.14591786802326823, 34.37609039468568284 ) ) ;
#82099=CARTESIAN_POINT ( 'NONE',  ( -13.89961937509977652, 13.97604488694528158, 40.62390960531435979 ) ) ;
#82100=CARTESIAN_POINT ( 'NONE',  ( -19.05341960407611168, -5.049401038298163336, 46.45724293864768129 ) ) ;
#82101=CARTESIAN_POINT ( 'NONE',  ( -21.52544592524343514, 5.823673210054127303, 81.04057627198102409 ) ) ;
#82103=CARTESIAN_POINT ( 'NONE',  ( -0.05219959533909027116, -19.03943276465977164, 52.49890960531436690 ) ) ;
#82105=CARTESIAN_POINT ( 'NONE',  ( 16.46253265017146816, 9.564922557961045513, 91.66775706135234714 ) ) ;
#82106=CARTESIAN_POINT ( 'NONE',  ( -14.29746914071049879, 8.314922557960819915, 60.83224293864769550 ) ) ;
#82107=CARTESIAN_POINT ( 'NONE',  ( -5.153800228976607833, 19.02544592524334988, 27.70942372801899722 ) ) ;
#82109=CARTESIAN_POINT ( 'NONE',  ( 5.719274019375991003, -21.55341960407610458, 92.70724293864770971 ) ) ;
#82110=CARTESIAN_POINT ( 'NONE',  ( -21.55341960407619339, 5.719274019375674811, 83.54275706135234714 ) ) ;
#82111=CARTESIAN_POINT ( 'NONE',  ( 19.02544592524343514, -5.153800228976328945, 23.54057627198102054 ) ) ;
#82112=CARTESIAN_POINT ( 'NONE',  ( -21.52544592524334988, -5.823673210054445271, 83.95942372801900433 ) ) ;
#82113=CARTESIAN_POINT ( 'NONE',  ( -16.55341960407611168, -4.379528057220339221, 21.45724293864769550 ) ) ;
#82114=CARTESIAN_POINT ( 'NONE',  ( -10.72451020669870658, -18.67979575497194134, 74.58442372801901854 ) ) ;
#82115=CARTESIAN_POINT ( 'NONE',  ( -0.05219959533909027116, -19.03943276465977164, 67.49890960531436690 ) ) ;
#82116=CARTESIAN_POINT ( 'NONE',  ( 21.55341960407619695, -5.719274019375665929, 41.04275706135236135 ) ) ;
#82117=CARTESIAN_POINT ( 'NONE',  ( -19.05341960407611168, -5.049401038298163336, 81.45724293864769550 ) ) ;
#82118=CARTESIAN_POINT ( 'NONE',  ( 4.379528057220339221, -16.55341960407611168, 92.70724293864770971 ) ) ;
#82119=CARTESIAN_POINT ( 'NONE',  ( -16.55341960407611168, -4.379528057220339221, 56.45724293864768839 ) ) ;
#82120=CARTESIAN_POINT ( 'NONE',  ( 15.72974639402199770, -15.80617190586745480, 68.12390960531436690 ) ) ;
#82121=CARTESIAN_POINT ( 'NONE',  ( 5.153800228976335163, 19.02544592524342804, 54.79057627198103120 ) ) ;
#82122=CARTESIAN_POINT ( 'NONE',  ( -18.62759615963270932, 10.81492255796079327, 90.83224293864769550 ) ) ;
#82123=CARTESIAN_POINT ( 'NONE',  ( 19.05341960407617918, -5.049401038297876454, 61.04275706135232582 ) ) ;
#82124=CARTESIAN_POINT ( 'NONE',  ( 13.97604488694548053, -13.89961937509957401, 30.62609039468566863 ) ) ;
#82125=CARTESIAN_POINT ( 'NONE',  ( -16.55341960407611168, -4.379528057220339221, 81.45724293864769550 ) ) ;
#82126=CARTESIAN_POINT ( 'NONE',  ( -21.53943276465977519, 0.05219959533907696930, 56.24890960531436690 ) ) ;
#82127=CARTESIAN_POINT ( 'NONE',  ( 17.40805194822031510, 6.112264579159339739, 101.6662872748938895 ) ) ;
#82128=CARTESIAN_POINT ( 'NONE',  ( 8.314922557961029526, -14.29746914071037800, 95.41775706135234714 ) ) ;
#82130=CARTESIAN_POINT ( 'NONE',  ( 19.05341960407617918, -5.049401038297876454, 96.04275706135231871 ) ) ;
#82131=CARTESIAN_POINT ( 'NONE',  ( -0.05219959533910754901, -16.53943276465976808, 67.49890960531436690 ) ) ;
#82133=CARTESIAN_POINT ( 'NONE',  ( -13.97604488694527625, -13.89961937509977652, 56.87390960531434558 ) ) ;
#82134=CARTESIAN_POINT ( 'NONE',  ( -12.06949235617756955, 12.14591786802309770, 55.62390960531436690 ) ) ;
#82135=CARTESIAN_POINT ( 'NONE',  ( 0.05219959533909260263, 19.03943276465977164, 99.99890960531436690 ) ) ;
#82136=CARTESIAN_POINT ( 'NONE',  ( -9.564922557961040184, 16.46253265017147172, 72.91775706135233293 ) ) ;
#82137=CARTESIAN_POINT ( 'NONE',  ( 9.474510206698971260, -16.51473224551069308, 67.91557627198102409 ) ) ;
#82138=CARTESIAN_POINT ( 'NONE',  ( -16.46253265017160317, 9.564922557960807481, 85.83224293864769550 ) ) ;
#82139=CARTESIAN_POINT ( 'NONE',  ( 19.02544592524343514, -5.153800228976328945, 83.54057627198100988 ) ) ;
#82140=CARTESIAN_POINT ( 'NONE',  ( -21.55341960407610458, -5.719274019375992779, 56.45724293864768839 ) ) ;
#82141=CARTESIAN_POINT ( 'NONE',  ( -16.53943276465976808, -0.05219959533934237506, 53.75109039468568994 ) ) ;
#82142=CARTESIAN_POINT ( 'NONE',  ( -5.049401038298153566, 19.05341960407611168, 45.20724293864769550 ) ) ;
#82143=CARTESIAN_POINT ( 'NONE',  ( -15.72974639402197994, 15.80617190586746368, 50.62390960531435979 ) ) ;
#82144=CARTESIAN_POINT ( 'NONE',  ( 9.564922557961047289, -16.46253265017146816, 95.41775706135233293 ) ) ;
#82145=CARTESIAN_POINT ( 'NONE',  ( -8.314922557960811034, -14.29746914071050412, 22.08224293864769194 ) ) ;
#82146=CARTESIAN_POINT ( 'NONE',  ( -10.72451020669870658, -18.67979575497194134, 34.58442372801900433 ) ) ;
#82147=CARTESIAN_POINT ( 'NONE',  ( -9.564922557961040184, 16.46253265017147172, 32.91775706135233293 ) ) ;
#82148=CARTESIAN_POINT ( 'NONE',  ( 12.06949235617739724, 12.14591786802326823, 56.87609039468568994 ) ) ;
#82149=CARTESIAN_POINT ( 'NONE',  ( -14.29746914071037622, -8.314922557961029526, 89.16775706135236135 ) ) ;
#82150=CARTESIAN_POINT ( 'NONE',  ( 19.36337904590693881, -5.499999999999945821, 42.91494137495619299 ) ) ;
#82151=CARTESIAN_POINT ( 'NONE',  ( -14.34966873604972548, 8.224510206698743886, 83.33442372801903275 ) ) ;
#82152=CARTESIAN_POINT ( 'NONE',  ( -10.81492255796078084, -18.62759615963271287, 22.08224293864769194 ) ) ;
#82153=CARTESIAN_POINT ( 'NONE',  ( 8.224510206698742110, 14.34966873604972548, 37.08442372801901143 ) ) ;
#82154=CARTESIAN_POINT ( 'NONE',  ( -5.049401038298153566, 19.05341960407611168, 50.20724293864770260 ) ) ;
#82155=CARTESIAN_POINT ( 'NONE',  ( 9.564922557960805705, 16.46253265017160317, 44.58224293864769550 ) ) ;
#82156=CARTESIAN_POINT ( 'NONE',  ( 9.474510206698971260, -16.51473224551069308, 62.91557627198102409 ) ) ;
#82157=CARTESIAN_POINT ( 'NONE',  ( 10.81492255796106328, -18.62759615963255655, 45.41775706135234003 ) ) ;
#82158=CARTESIAN_POINT ( 'NONE',  ( -12.14591786802326823, 12.06949235617739902, 48.12609039468568284 ) ) ;
#82159=CARTESIAN_POINT ( 'NONE',  ( 14.29746914071037800, 8.314922557961029526, 106.6677570613523756 ) ) ;
#82160=CARTESIAN_POINT ( 'NONE',  ( -0.05219959533909027116, -19.03943276465977164, 27.49890960531435624 ) ) ;
#82161=CARTESIAN_POINT ( 'NONE',  ( -9.474510206698720793, -16.51473224551083518, 24.58442372801900078 ) ) ;
#82162=CARTESIAN_POINT ( 'NONE',  ( -9.474510206698720793, -16.51473224551083518, 109.5844237280190043 ) ) ;
#82163=CARTESIAN_POINT ( 'NONE',  ( 9.564922557961047289, -16.46253265017146816, 65.41775706135233293 ) ) ;
#82164=CARTESIAN_POINT ( 'NONE',  ( -12.14591786802309592, -12.06949235617757132, 71.87390960531438111 ) ) ;
#82165=CARTESIAN_POINT ( 'NONE',  ( 0.05219959533909260263, 19.03943276465977164, 34.99890960531435979 ) ) ;
#82166=CARTESIAN_POINT ( 'NONE',  ( -19.02544592524334988, -5.153800228976617603, 78.95942372801900433 ) ) ;
#82167=CARTESIAN_POINT ( 'NONE',  ( 16.38665767535053064, 7.295008042176054808, 77.23599135785458714 ) ) ;
#82168=CARTESIAN_POINT ( 'NONE',  ( -21.52544592524334988, -5.823673210054445271, 73.95942372801901854 ) ) ;
#82169=CARTESIAN_POINT ( 'NONE',  ( -4.379528057220086978, -16.55341960407618274, 39.79275706135235424 ) ) ;
#82170=CARTESIAN_POINT ( 'NONE',  ( -17.50000000000012434, 3.417042746627156014, 25.17380396232484685 ) ) ;
#82171=CARTESIAN_POINT ( 'NONE',  ( 10.72451020669898902, -18.67979575497178502, 37.91557627198102409 ) ) ;
#82172=CARTESIAN_POINT ( 'NONE',  ( 4.483927247898790824, -16.52544592524335698, 30.20942372801902565 ) ) ;
#82173=CARTESIAN_POINT ( 'NONE',  ( -5.049401038298153566, 19.05341960407611168, 25.20724293864768839 ) ) ;
#82174=CARTESIAN_POINT ( 'NONE',  ( -19.03943276465977164, -0.05219959533935918106, 23.75109039468566152 ) ) ;
#82176=CARTESIAN_POINT ( 'NONE',  ( 13.97604488694527802, 13.89961937509977652, 39.37390960531435269 ) ) ;
#82178=CARTESIAN_POINT ( 'NONE',  ( 13.97604488694527802, 13.89961937509977652, 59.37390960531434558 ) ) ;
#82179=CARTESIAN_POINT ( 'NONE',  ( 17.49999999999999289, -4.640572885337564735, 113.1378816454884344 ) ) ;
#82180=CARTESIAN_POINT ( 'NONE',  ( 16.46253265017146816, 9.564922557961045513, 26.66775706135234003 ) ) ;
#82181=CARTESIAN_POINT ( 'NONE',  ( 8.314922557960818139, 14.29746914071049879, 24.58224293864768839 ) ) ;
#82182=CARTESIAN_POINT ( 'NONE',  ( 9.474510206698971260, -16.51473224551069308, 27.91557627198103120 ) ) ;
#82183=EDGE_CURVE ( 'NONE', #114473, #119772, #146425, .T. ) ;
#82185=CARTESIAN_POINT ( 'NONE',  ( -16.46253265017160317, 9.564922557960807481, 90.83224293864769550 ) ) ;
#82186=CARTESIAN_POINT ( 'NONE',  ( -21.55341960407619339, 5.719274019375674811, 63.54275706135234003 ) ) ;
#82187=CARTESIAN_POINT ( 'NONE',  ( 19.02544592524343514, -5.153800228976328945, 33.54057627198102409 ) ) ;
#82188=CARTESIAN_POINT ( 'NONE',  ( -0.05219959533937732626, 21.53943276465977519, 67.50109039468568994 ) ) ;
#82189=CARTESIAN_POINT ( 'NONE',  ( -19.02544592524334988, -5.153800228976617603, 98.95942372801900433 ) ) ;
#82190=CARTESIAN_POINT ( 'NONE',  ( 10.72451020669898902, -18.67979575497178502, 27.91557627198103830 ) ) ;
#82191=CARTESIAN_POINT ( 'NONE',  ( -9.564922557960796823, -16.46253265017161027, 32.08224293864769550 ) ) ;
#82192=CARTESIAN_POINT ( 'NONE',  ( -10.72451020669898014, 18.67979575497178502, 115.4155762719810241 ) ) ;
#82193=CARTESIAN_POINT ( 'NONE',  ( -19.03943276465977164, -0.05219959533935918106, 33.75109039468566863 ) ) ;
#82194=CARTESIAN_POINT ( 'NONE',  ( -16.53943276465976808, 0.05219959533911058130, 116.2489096053143669 ) ) ;
#82195=CARTESIAN_POINT ( 'NONE',  ( 19.03943276465977164, -0.05219959533909143690, 68.74890960531436690 ) ) ;
#82196=CARTESIAN_POINT ( 'NONE',  ( -16.51473224551082808, 9.474510206698731452, 113.3344237280190043 ) ) ;
#82198=CARTESIAN_POINT ( 'NONE',  ( -14.34966873604960291, -8.224510206698953496, 81.66557627198103830 ) ) ;
#82199=CARTESIAN_POINT ( 'NONE',  ( -0.05219959533907301413, -21.53943276465977519, 22.49890960531436335 ) ) ;
#82200=CARTESIAN_POINT ( 'NONE',  ( -16.51473224551082808, 9.474510206698731452, 83.33442372801899012 ) ) ;
#82201=CARTESIAN_POINT ( 'NONE',  ( 10.81492255796078972, 18.62759615963270932, 89.58224293864768129 ) ) ;
#82202=CARTESIAN_POINT ( 'NONE',  ( 21.53943276465977519, 0.05219959533937863772, 46.25109039468567573 ) ) ;
#82203=CARTESIAN_POINT ( 'NONE',  ( 16.52544592524335698, 4.483927247898782831, 56.45942372801902565 ) ) ;
#82204=CARTESIAN_POINT ( 'NONE',  ( 12.06949235617739724, 12.14591786802326823, 51.87609039468568284 ) ) ;
#82205=CARTESIAN_POINT ( 'NONE',  ( -10.72451020669870658, -18.67979575497194134, 44.58442372801901854 ) ) ;
#82206=CARTESIAN_POINT ( 'NONE',  ( 21.55341960407610458, 5.719274019375980345, 48.95724293864770971 ) ) ;
#82208=CARTESIAN_POINT ( 'NONE',  ( 9.474510206698971260, -16.51473224551069308, 47.91557627198102409 ) ) ;
#82210=CARTESIAN_POINT ( 'NONE',  ( 0.05219959533934541429, -16.53943276465976808, 80.00109039468568994 ) ) ;
#82211=CARTESIAN_POINT ( 'NONE',  ( 15.80617190586746368, 15.72974639402197994, 104.3739096053143669 ) ) ;
#82212=CARTESIAN_POINT ( 'NONE',  ( 12.06949235617757843, -12.14591786802309237, 48.12390960531436690 ) ) ;
#82213=CARTESIAN_POINT ( 'NONE',  ( -14.34966873604972548, 8.224510206698743886, 68.33442372801900433 ) ) ;
#82214=CARTESIAN_POINT ( 'NONE',  ( 5.153800228976615827, -19.02544592524334988, 105.2094237280190185 ) ) ;
#82215=CARTESIAN_POINT ( 'NONE',  ( -18.62759615963270932, 10.81492255796079327, 100.8322429386477097 ) ) ;
#82216=CARTESIAN_POINT ( 'NONE',  ( 4.379528057220339221, -16.55341960407611168, 47.70724293864770260 ) ) ;
#82217=EDGE_CURVE ( 'NONE', #2480, #69839, #35108, .T. ) ;
#82218=ORIENTED_EDGE ( 'NONE', *, *, #3863, .F. ) ;
#82220=CARTESIAN_POINT ( 'NONE',  ( 21.52544592524344225, -5.823673210054117533, 78.54057627198103830 ) ) ;
#82221=CARTESIAN_POINT ( 'NONE',  ( 16.55341960407611168, 4.379528057220329451, 28.95724293864769905 ) ) ;
#82223=CARTESIAN_POINT ( 'NONE',  ( -16.52216118717207038, -7.221426719304521846, 56.07599021046991083 ) ) ;
#82224=CARTESIAN_POINT ( 'NONE',  ( -18.62759615963270932, 10.81492255796079327, 105.8322429386476955 ) ) ;
#82225=CARTESIAN_POINT ( 'NONE',  ( -21.53943276465977519, 0.05219959533907696930, 111.2489096053143669 ) ) ;
#82226=CARTESIAN_POINT ( 'NONE',  ( -16.53943276465976808, 0.05219959533911058130, 41.24890960531435269 ) ) ;
#82227=AXIS2_PLACEMENT_3D ( 'NONE', #101966, #59434, #150480 ) ;
#82228=CARTESIAN_POINT ( 'NONE',  ( 16.53943276465976808, 0.05219959533934440121, 51.25109039468568994 ) ) ;
#82229=CARTESIAN_POINT ( 'NONE',  ( 13.97604488694527802, 13.89961937509977652, 44.37390960531435269 ) ) ;
#82230=CARTESIAN_POINT ( 'NONE',  ( 13.89961937509977652, -13.97604488694527269, 73.12390960531436690 ) ) ;
#82232=CARTESIAN_POINT ( 'NONE',  ( 10.81492255796078972, 18.62759615963270932, 39.58224293864769550 ) ) ;
#82234=CARTESIAN_POINT ( 'NONE',  ( -19.02544592524334988, -5.153800228976617603, 108.9594237280189759 ) ) ;
#82235=CARTESIAN_POINT ( 'NONE',  ( 13.97604488694548053, -13.89961937509957401, 45.62609039468566863 ) ) ;
#82236=CARTESIAN_POINT ( 'NONE',  ( -21.52544592524343514, 5.823673210054127303, 106.0405762719810525 ) ) ;
#82237=CARTESIAN_POINT ( 'NONE',  ( -16.55341960407611168, -4.379528057220339221, 31.45724293864769550 ) ) ;
#82238=CARTESIAN_POINT ( 'NONE',  ( -5.049401038298153566, 19.05341960407611168, 80.20724293864769550 ) ) ;
#82239=CARTESIAN_POINT ( 'NONE',  ( 10.81492255796078972, 18.62759615963270932, 49.58224293864769550 ) ) ;
#82240=CARTESIAN_POINT ( 'NONE',  ( 15.80617190586746368, 15.72974639402197994, 84.37390960531438111 ) ) ;
#82241=CARTESIAN_POINT ( 'NONE',  ( 4.379528057220092307, 16.55341960407617563, 22.29275706135235069 ) ) ;
#82242=CARTESIAN_POINT ( 'NONE',  ( -21.55341960407610458, -5.719274019375992779, 21.45724293864769550 ) ) ;
#82243=CARTESIAN_POINT ( 'NONE',  ( -18.67979575497193778, 10.72451020669871902, 78.33442372801901854 ) ) ;
#82244=CARTESIAN_POINT ( 'NONE',  ( 19.03943276465977164, -0.05219959533909143690, 68.74890960531436690 ) ) ;
#82245=CARTESIAN_POINT ( 'NONE',  ( -0.05219959533909027116, -19.03943276465977164, 32.49890960531435979 ) ) ;
#82246=CARTESIAN_POINT ( 'NONE',  ( -5.049401038298153566, 19.05341960407611168, 80.20724293864769550 ) ) ;
#82247=CARTESIAN_POINT ( 'NONE',  ( -8.314922557960811034, -14.29746914071050412, 97.08224293864770971 ) ) ;
#82249=CARTESIAN_POINT ( 'NONE',  ( 13.89961937509957401, 13.97604488694547697, 106.8760903946856757 ) ) ;
#82250=CARTESIAN_POINT ( 'NONE',  ( 17.49999999999999645, -5.500000000000031086, 83.29690382534172954 ) ) ;
#82251=CARTESIAN_POINT ( 'NONE',  ( -19.05341960407611168, -5.049401038298163336, 71.45724293864766707 ) ) ;
#82252=CARTESIAN_POINT ( 'NONE',  ( 0.05219959533937995610, -21.53943276465977519, 85.00109039468568994 ) ) ;
#82253=CARTESIAN_POINT ( 'NONE',  ( -9.564922557960796823, -16.46253265017161027, 112.0822429386476955 ) ) ;
#82254=CARTESIAN_POINT ( 'NONE',  ( -0.05219959533934338120, 16.53943276465976808, 77.50109039468567573 ) ) ;
#82255=CARTESIAN_POINT ( 'NONE',  ( -17.05116617787826527, -6.768360034955819948, 76.34324446740801307 ) ) ;
#82256=CARTESIAN_POINT ( 'NONE',  ( -16.46253265017146816, -9.564922557961047289, 54.16775706135234003 ) ) ;
#82257=CARTESIAN_POINT ( 'NONE',  ( 15.80617190586769283, -15.72974639402175789, 110.6260903946857042 ) ) ;
#82261=CARTESIAN_POINT ( 'NONE',  ( -0.05219959533910754901, -16.53943276465976808, 27.49890960531435269 ) ) ;
#82262=FACE_OUTER_BOUND ( 'NONE', #76152, .T. ) ;
#82263=CARTESIAN_POINT ( 'NONE',  ( 12.06949235617739724, 12.14591786802326823, 101.8760903946857042 ) ) ;
#82265=CARTESIAN_POINT ( 'NONE',  ( 8.224510206698742110, 14.34966873604972548, 82.08442372801901854 ) ) ;
#82266=CARTESIAN_POINT ( 'NONE',  ( 5.823673210054444382, -21.52544592524334988, 95.20942372801903275 ) ) ;
#82267=CARTESIAN_POINT ( 'NONE',  ( -16.46253265017146816, -9.564922557961047289, 104.1677570613523329 ) ) ;
#82268=CARTESIAN_POINT ( 'NONE',  ( 18.62759615963255655, 10.81492255796105972, 61.66775706135235424 ) ) ;
#82269=CARTESIAN_POINT ( 'NONE',  ( 19.05341960407617918, -5.049401038297876454, 41.04275706135233293 ) ) ;
#82270=CARTESIAN_POINT ( 'NONE',  ( 9.564922557960805705, 16.46253265017160317, 79.58224293864769550 ) ) ;
#82271=CARTESIAN_POINT ( 'NONE',  ( 5.153800228976335163, 19.02544592524342804, 59.79057627198100988 ) ) ;
#82272=CARTESIAN_POINT ( 'NONE',  ( -13.97604488694527625, -13.89961937509977830, 86.87390960531436690 ) ) ;
#82273=CARTESIAN_POINT ( 'NONE',  ( 15.72974639402199770, -15.80617190586745480, 93.12390960531436690 ) ) ;
#82274=CARTESIAN_POINT ( 'NONE',  ( 5.719274019375991003, -21.55341960407610458, 47.70724293864770260 ) ) ;
#82275=CARTESIAN_POINT ( 'NONE',  ( -16.46253265017160317, 9.564922557960807481, 45.83224293864769550 ) ) ;
#82276=CARTESIAN_POINT ( 'NONE',  ( -16.55341960407617563, 4.379528057220093196, 63.54275706135234003 ) ) ;
#82279=CARTESIAN_POINT ( 'NONE',  ( 18.62759615963255655, 10.81492255796105972, 46.66775706135234714 ) ) ;
#82281=CARTESIAN_POINT ( 'NONE',  ( 0.05219959533910956823, 16.53943276465976808, 79.99890960531435269 ) ) ;
#82283=CARTESIAN_POINT ( 'NONE',  ( -14.29746914071037622, -8.314922557961029526, 44.16775706135234714 ) ) ;
#82284=CARTESIAN_POINT ( 'NONE',  ( -14.34966873604960291, -8.224510206698953496, 101.6655762719810383 ) ) ;
#82285=CARTESIAN_POINT ( 'NONE',  ( -16.51473224551082808, 9.474510206698731452, 53.33442372801900433 ) ) ;
#82286=CARTESIAN_POINT ( 'NONE',  ( -16.53943276465976808, 0.05219959533911058130, 66.24890960531436690 ) ) ;
#82287=CARTESIAN_POINT ( 'NONE',  ( 15.72974639402176855, 15.80617190586768217, 36.87609039468568994 ) ) ;
#82289=CARTESIAN_POINT ( 'NONE',  ( -9.474510206698964154, 16.51473224551069663, 25.41557627198103120 ) ) ;
#82290=CARTESIAN_POINT ( 'NONE',  ( -15.72974639402197994, 15.80617190586746368, 85.62390960531436690 ) ) ;
#82291=CARTESIAN_POINT ( 'NONE',  ( 5.049401038298161559, -19.05341960407611168, 102.7072429386476955 ) ) ;
#82292=CARTESIAN_POINT ( 'NONE',  ( 16.53943276465976808, -0.05219959533910856209, 68.74890960531435269 ) ) ;
#82295=CARTESIAN_POINT ( 'NONE',  ( 5.153800228976615827, -19.02544592524334988, 80.20942372801901854 ) ) ;
#82296=CARTESIAN_POINT ( 'NONE',  ( 10.81492255796078972, 18.62759615963270932, 114.5822429386477097 ) ) ;
#82297=CARTESIAN_POINT ( 'NONE',  ( 16.51473224551069308, 9.474510206698969483, 69.16557627198102409 ) ) ;
#82298=CARTESIAN_POINT ( 'NONE',  ( 16.46253265017146816, 9.564922557961045513, 61.66775706135234003 ) ) ;
#82299=CARTESIAN_POINT ( 'NONE',  ( -9.474510206698964154, 16.51473224551069663, 45.41557627198103120 ) ) ;
#82300=CARTESIAN_POINT ( 'NONE',  ( -4.483927247898539470, -16.52544592524342804, 62.29057627198102409 ) ) ;
#82301=EDGE_CURVE ( 'NONE', #68796, #138021, #21572, .T. ) ;
#82302=CARTESIAN_POINT ( 'NONE',  ( 14.34966873604960469, 8.224510206698951720, 49.16557627198102409 ) ) ;
#82303=CARTESIAN_POINT ( 'NONE',  ( 19.03943276465977164, -0.05219959533909143690, 73.74890960531435269 ) ) ;
#82304=CARTESIAN_POINT ( 'NONE',  ( 21.55341960407610458, 5.719274019375980345, 88.95724293864769550 ) ) ;
#82305=CARTESIAN_POINT ( 'NONE',  ( -5.153800228976328057, -19.02544592524343514, 67.29057627198102409 ) ) ;
#82306=CARTESIAN_POINT ( 'NONE',  ( 18.67979575497178502, 10.72451020669898547, 79.16557627198103830 ) ) ;
#82307=CARTESIAN_POINT ( 'NONE',  ( 21.52544592524334988, 5.823673210054432836, 111.4594237280190328 ) ) ;
#82308=PLANE ( 'NONE',  #96088 ) ;
#82309=CARTESIAN_POINT ( 'NONE',  ( -8.224510206698735004, -14.34966873604973081, 109.5844237280190328 ) ) ;
#82310=CARTESIAN_POINT ( 'NONE',  ( 12.06949235617757843, -12.14591786802309237, 98.12390960531436690 ) ) ;
#82311=CARTESIAN_POINT ( 'NONE',  ( -19.05341960407617563, 5.049401038297882671, 103.5427570613523329 ) ) ;
#82313=CARTESIAN_POINT ( 'NONE',  ( -15.80617190586768217, 15.72974639402176855, 23.12609039468567573 ) ) ;
#82314=CARTESIAN_POINT ( 'NONE',  ( -13.97604488694547697, 13.89961937509957934, 58.12609039468566863 ) ) ;
#82315=CARTESIAN_POINT ( 'NONE',  ( 4.379528057220092307, 16.55341960407617563, 102.2927570613523613 ) ) ;
#82316=CARTESIAN_POINT ( 'NONE',  ( 16.46253265017146816, 9.564922557961045513, 41.66775706135234003 ) ) ;
#82317=CARTESIAN_POINT ( 'NONE',  ( -19.05341960407611168, -5.049401038298163336, 101.4572429386476955 ) ) ;
#82318=CARTESIAN_POINT ( 'NONE',  ( 8.224510206698953496, -14.34966873604960469, 52.91557627198103830 ) ) ;
#82319=CARTESIAN_POINT ( 'NONE',  ( -19.49149378614655959, 5.499999999999766409, 49.43757513605356024 ) ) ;
#82320=CARTESIAN_POINT ( 'NONE',  ( 0.05219959533909260263, 19.03943276465977164, 34.99890960531435979 ) ) ;
#82321=CARTESIAN_POINT ( 'NONE',  ( -21.52544592524334988, -5.823673210054445271, 108.9594237280190185 ) ) ;
#82322=CARTESIAN_POINT ( 'NONE',  ( 16.53943276465976808, 0.05219959533934440121, 91.25109039468568994 ) ) ;
#82323=CARTESIAN_POINT ( 'NONE',  ( 0.05219959533937995610, -21.53943276465977519, 40.00109039468567573 ) ) ;
#82324=CARTESIAN_POINT ( 'NONE',  ( -14.34966873604972548, 8.224510206698743886, 38.33442372801900433 ) ) ;
#82325=CARTESIAN_POINT ( 'NONE',  ( -9.564922557960796823, -16.46253265017161027, 107.0822429386476955 ) ) ;
#82326=CARTESIAN_POINT ( 'NONE',  ( -0.05219959533909027116, -19.03943276465977164, 47.49890960531435979 ) ) ;
#82327=CARTESIAN_POINT ( 'NONE',  ( -19.03943276465977164, 0.05219959533909376836, 66.24890960531436690 ) ) ;
#82329=CARTESIAN_POINT ( 'NONE',  ( -0.05219959533934338120, 16.53943276465976808, 47.50109039468568994 ) ) ;
#82330=CARTESIAN_POINT ( 'NONE',  ( -16.55341960407611168, -4.379528057220339221, 111.4572429386476813 ) ) ;
#82331=CARTESIAN_POINT ( 'NONE',  ( -16.55341960407611168, -4.379528057220339221, 26.45724293864768839 ) ) ;
#82333=CARTESIAN_POINT ( 'NONE',  ( 21.53943276465977519, 0.05219959533937863772, 61.25109039468567573 ) ) ;
#82334=CARTESIAN_POINT ( 'NONE',  ( 19.05341960407611168, 5.049401038298154454, 88.95724293864769550 ) ) ;
#82335=CARTESIAN_POINT ( 'NONE',  ( 5.049401038298161559, -19.05341960407611168, 77.70724293864765286 ) ) ;
#82336=CARTESIAN_POINT ( 'NONE',  ( 9.564922557960805705, 16.46253265017160317, 94.58224293864769550 ) ) ;
#82337=CARTESIAN_POINT ( 'NONE',  ( 4.483927247898545687, 16.52544592524342804, 39.79057627198103830 ) ) ;
#82338=CARTESIAN_POINT ( 'NONE',  ( -12.14591786802309592, -12.06949235617757132, 21.87390960531436690 ) ) ;
#82339=CARTESIAN_POINT ( 'NONE',  ( 16.55341960407611168, 4.379528057220329451, 38.95724293864768839 ) ) ;
#82340=ORIENTED_EDGE ( 'NONE', *, *, #195934, .F. ) ;
#82341=CARTESIAN_POINT ( 'NONE',  ( 18.22780087662126647, 5.499999999999818812, 56.48236817873107185 ) ) ;
#82343=CARTESIAN_POINT ( 'NONE',  ( 9.474510206698971260, -16.51473224551069308, 67.91557627198102409 ) ) ;
#82344=CARTESIAN_POINT ( 'NONE',  ( 5.049401038297881783, 19.05341960407617563, 57.29275706135231871 ) ) ;
#82347=CARTESIAN_POINT ( 'NONE',  ( -5.049401038297874678, -19.05341960407617918, 84.79275706135233293 ) ) ;
#82348=CARTESIAN_POINT ( 'NONE',  ( 8.314922557961029526, -14.29746914071037800, 65.41775706135234714 ) ) ;
#82349=PRODUCT_DEFINITION_FORMATION_WITH_SPECIFIED_SOURCE ( 'ANY', '', #184101, .NOT_KNOWN. ) ;
#82350=CARTESIAN_POINT ( 'NONE',  ( 17.26172910966779384, 6.454744622555852018, 91.69353091350777163 ) ) ;
#82351=CARTESIAN_POINT ( 'NONE',  ( -5.049401038298153566, 19.05341960407611168, 85.20724293864766707 ) ) ;
#82352=CARTESIAN_POINT ( 'NONE',  ( 10.81492255796106328, -18.62759615963255655, 25.41775706135235779 ) ) ;
#82353=CARTESIAN_POINT ( 'NONE',  ( 0.05219959533936267826, -19.03943276465977164, 90.00109039468567573 ) ) ;
#82354=CARTESIAN_POINT ( 'NONE',  ( 16.21995358207305316, 7.366697692864115687, 87.56448998487846325 ) ) ;
#82355=CARTESIAN_POINT ( 'NONE',  ( -0.05219959533909027116, -19.03943276465977164, 42.49890960531435269 ) ) ;
#82356=CARTESIAN_POINT ( 'NONE',  ( -16.46253265017160317, 9.564922557960807481, 85.83224293864769550 ) ) ;
#82357=CARTESIAN_POINT ( 'NONE',  ( -14.34966873604960291, -8.224510206698953496, 51.66557627198102409 ) ) ;
#82358=CARTESIAN_POINT ( 'NONE',  ( -0.05219959533909027116, -19.03943276465977164, 47.49890960531435979 ) ) ;
#82359=CARTESIAN_POINT ( 'NONE',  ( -13.97604488694547697, 13.89961937509957934, 63.12609039468566152 ) ) ;
#82360=CARTESIAN_POINT ( 'NONE',  ( 4.483927247898545687, 16.52544592524342804, 84.79057627198102409 ) ) ;
#82361=CARTESIAN_POINT ( 'NONE',  ( 13.97604488694548053, -13.89961937509957401, 35.62609039468567573 ) ) ;
#82362=CARTESIAN_POINT ( 'NONE',  ( 13.89961937509977652, -13.97604488694527269, 63.12390960531435979 ) ) ;
#82364=CARTESIAN_POINT ( 'NONE',  ( 10.72451020669898902, -18.67979575497178502, 62.91557627198102409 ) ) ;
#82365=CARTESIAN_POINT ( 'NONE',  ( 4.379528057220339221, -16.55341960407611168, 62.70724293864769550 ) ) ;
#82366=CARTESIAN_POINT ( 'NONE',  ( -19.02544592524334988, -5.153800228976617603, 18.95942372801899722 ) ) ;
#82367=CARTESIAN_POINT ( 'NONE',  ( -19.03943276465977164, 0.05219959533909376836, 106.2489096053143669 ) ) ;
#82368=CARTESIAN_POINT ( 'NONE',  ( 21.55341960407610458, 5.719274019375980345, 28.95724293864769905 ) ) ;
#82369=CARTESIAN_POINT ( 'NONE',  ( -5.153800228976328057, -19.02544592524343514, 52.29057627198100988 ) ) ;
#82370=CARTESIAN_POINT ( 'NONE',  ( 9.474510206698971260, -16.51473224551069308, 32.91557627198102409 ) ) ;
#82371=CARTESIAN_POINT ( 'NONE',  ( -16.52544592524342804, 4.483927247898546575, 96.04057627198102409 ) ) ;
#82373=CARTESIAN_POINT ( 'NONE',  ( 5.719274019375991003, -21.55341960407610458, 112.7072429386476955 ) ) ;
#82374=CARTESIAN_POINT ( 'NONE',  ( 16.46253265017160672, -9.564922557960803928, 113.3322429386476955 ) ) ;
#82375=CARTESIAN_POINT ( 'NONE',  ( -21.53943276465977519, -0.05219959533937600094, 23.75109039468567929 ) ) ;
#82376=CARTESIAN_POINT ( 'NONE',  ( -9.564922557960796823, -16.46253265017161027, 107.0822429386476955 ) ) ;
#82377=CARTESIAN_POINT ( 'NONE',  ( -14.34966873604960291, -8.224510206698953496, 111.6655762719810525 ) ) ;
#82378=CARTESIAN_POINT ( 'NONE',  ( 15.72974639402176855, 15.80617190586768217, 81.87609039468568994 ) ) ;
#82379=CARTESIAN_POINT ( 'NONE',  ( 18.62759615963271287, -10.81492255796078972, 93.33224293864769550 ) ) ;
#82381=CARTESIAN_POINT ( 'NONE',  ( -9.564922557960796823, -16.46253265017161027, 52.08224293864768839 ) ) ;
#82383=CARTESIAN_POINT ( 'NONE',  ( 4.379528057220092307, 16.55341960407617563, 42.29275706135235424 ) ) ;
#82384=CARTESIAN_POINT ( 'NONE',  ( -8.314922557960811034, -14.29746914071050412, 102.0822429386476955 ) ) ;
#82386=CARTESIAN_POINT ( 'NONE',  ( -16.46253265017160317, 9.564922557960807481, 55.83224293864769550 ) ) ;
#82387=CARTESIAN_POINT ( 'NONE',  ( 4.483927247898545687, 16.52544592524342804, 89.79057627198103830 ) ) ;
#82388=CARTESIAN_POINT ( 'NONE',  ( 18.67979575497178502, 10.72451020669898547, 44.16557627198103120 ) ) ;
#82389=CARTESIAN_POINT ( 'NONE',  ( 16.55341960407611168, 4.379528057220329451, 58.95724293864770971 ) ) ;
#82390=CARTESIAN_POINT ( 'NONE',  ( -16.52544592524335698, -4.483927247898792601, 23.95942372801901143 ) ) ;
#82391=CARTESIAN_POINT ( 'NONE',  ( 0.05219959533937995610, -21.53943276465977519, 90.00109039468567573 ) ) ;
#82392=CARTESIAN_POINT ( 'NONE',  ( 17.31747979337950838, -6.344076630960993946, 76.12055131934818064 ) ) ;
#82393=CARTESIAN_POINT ( 'NONE',  ( -14.34966873604972548, 8.224510206698743886, 103.3344237280190043 ) ) ;
#82394=CARTESIAN_POINT ( 'NONE',  ( -0.05219959533910754901, -16.53943276465976808, 37.49890960531436690 ) ) ;
#82395=CARTESIAN_POINT ( 'NONE',  ( -5.153800228976328057, -19.02544592524343514, 32.29057627198102409 ) ) ;
#82396=CARTESIAN_POINT ( 'NONE',  ( 16.51473224551069308, 9.474510206698969483, 94.16557627198103830 ) ) ;
#82397=CARTESIAN_POINT ( 'NONE',  ( 0.05219959533907565091, 21.53943276465977519, 89.99890960531438111 ) ) ;
#82398=CARTESIAN_POINT ( 'NONE',  ( -14.34966873604972548, 8.224510206698743886, 43.33442372801901143 ) ) ;
#82399=CARTESIAN_POINT ( 'NONE',  ( 0.05219959533910956823, 16.53943276465976808, 64.99890960531435269 ) ) ;
#82400=CARTESIAN_POINT ( 'NONE',  ( -5.719274019375665041, -21.55341960407619695, 79.79275706135236135 ) ) ;
#82401=CARTESIAN_POINT ( 'NONE',  ( 12.06949235617739724, 12.14591786802326823, 96.87609039468568994 ) ) ;
#82402=CARTESIAN_POINT ( 'NONE',  ( 16.62475595723696387, 7.163666690055258357, 26.97286648189535185 ) ) ;
#82403=CARTESIAN_POINT ( 'NONE',  ( -18.22780087662121673, -5.500000000000063061, 66.48459894673892734 ) ) ;
#82404=CARTESIAN_POINT ( 'NONE',  ( 4.483927247898545687, 16.52544592524342804, 24.79057627198103120 ) ) ;
#82405=CARTESIAN_POINT ( 'NONE',  ( -12.06949235617739369, -12.14591786802326823, 69.37609039468567573 ) ) ;
#82406=CARTESIAN_POINT ( 'NONE',  ( 19.05341960407611168, 5.049401038298154454, 83.95724293864766707 ) ) ;
#82407=CARTESIAN_POINT ( 'NONE',  ( 13.97604488694527802, 13.89961937509977652, 99.37390960531436690 ) ) ;
#82408=CARTESIAN_POINT ( 'NONE',  ( -15.72974639402176322, -15.80617190586768395, 89.37609039468568994 ) ) ;
#82409=CARTESIAN_POINT ( 'NONE',  ( -0.05219959533934338120, 16.53943276465976808, 92.50109039468567573 ) ) ;
#82410=CARTESIAN_POINT ( 'NONE',  ( -14.29746914071049879, 8.314922557960819915, 55.83224293864770260 ) ) ;
#82411=CARTESIAN_POINT ( 'NONE',  ( 19.02544592524343514, -5.153800228976328945, 63.54057627198103830 ) ) ;
#82413=CARTESIAN_POINT ( 'NONE',  ( 5.153800228976615827, -19.02544592524334988, 105.2094237280190185 ) ) ;
#82414=CARTESIAN_POINT ( 'NONE',  ( -4.379528057220328563, 16.55341960407611168, 115.2072429386476955 ) ) ;
#82415=CARTESIAN_POINT ( 'NONE',  ( 5.049401038298161559, -19.05341960407611168, 77.70724293864765286 ) ) ;
#82416=CARTESIAN_POINT ( 'NONE',  ( 4.379528057220092307, 16.55341960407617563, 22.29275706135235069 ) ) ;
#82418=CARTESIAN_POINT ( 'NONE',  ( -9.474510206698720793, -16.51473224551083518, 24.58442372801900078 ) ) ;
#82419=CARTESIAN_POINT ( 'NONE',  ( -12.06949235617739369, -12.14591786802326823, 84.37609039468570415 ) ) ;
#82420=CARTESIAN_POINT ( 'NONE',  ( -5.153800228976607833, 19.02544592524334988, 112.7094237280190043 ) ) ;
#82421=CARTESIAN_POINT ( 'NONE',  ( -16.53943276465976808, 0.05219959533911058130, 111.2489096053143669 ) ) ;
#82422=CARTESIAN_POINT ( 'NONE',  ( 16.55341960407618274, -4.379528057220086978, 71.04275706135234714 ) ) ;
#82423=CARTESIAN_POINT ( 'NONE',  ( -8.224510206698735004, -14.34966873604973081, 49.58442372801901143 ) ) ;
#82424=CARTESIAN_POINT ( 'NONE',  ( -19.05341960407611168, -5.049401038298163336, 21.45724293864768839 ) ) ;
#82425=CARTESIAN_POINT ( 'NONE',  ( 0.05219959533936267826, -19.03943276465977164, 65.00109039468567573 ) ) ;
#82427=CARTESIAN_POINT ( 'NONE',  ( -21.52544592524334988, -5.823673210054445271, 108.9594237280190185 ) ) ;
#82428=CARTESIAN_POINT ( 'NONE',  ( 16.51473224551069308, 9.474510206698969483, 39.16557627198103120 ) ) ;
#82429=CARTESIAN_POINT ( 'NONE',  ( 5.049401038298161559, -19.05341960407611168, 77.70724293864765286 ) ) ;
#82430=CARTESIAN_POINT ( 'NONE',  ( -14.29746914071049879, 8.314922557960819915, 65.83224293864769550 ) ) ;
#82431=CARTESIAN_POINT ( 'NONE',  ( 9.564922557961047289, -16.46253265017146816, 35.41775706135233293 ) ) ;
#82432=CARTESIAN_POINT ( 'NONE',  ( 15.80617190586746368, 15.72974639402197994, 34.37390960531435979 ) ) ;
#82433=CARTESIAN_POINT ( 'NONE',  ( -0.05219959533937732626, 21.53943276465977519, 107.5010903946856899 ) ) ;
#82434=CARTESIAN_POINT ( 'NONE',  ( -16.51473224551069308, -9.474510206698971260, 86.66557627198102409 ) ) ;
#82435=CARTESIAN_POINT ( 'NONE',  ( -18.62759615963255300, -10.81492255796106328, 104.1677570613523471 ) ) ;
#82436=CARTESIAN_POINT ( 'NONE',  ( -18.67979575497178146, -10.72451020669898902, 66.66557627198102409 ) ) ;
#82437=CARTESIAN_POINT ( 'NONE',  ( -16.51473224551069308, -9.474510206698971260, 96.66557627198102409 ) ) ;
#82438=CARTESIAN_POINT ( 'NONE',  ( 5.153800228976615827, -19.02544592524334988, 75.20942372801896170 ) ) ;
#82439=CARTESIAN_POINT ( 'NONE',  ( 16.46253265017160672, -9.564922557960803928, 108.3322429386476955 ) ) ;
#82440=CARTESIAN_POINT ( 'NONE',  ( 9.474510206698729675, 16.51473224551082808, 92.08442372801900433 ) ) ;
#82441=CARTESIAN_POINT ( 'NONE',  ( 8.224510206698742110, 14.34966873604972548, 62.08442372801901143 ) ) ;
#82442=CARTESIAN_POINT ( 'NONE',  ( 12.06949235617757843, -12.14591786802309237, 113.1239096053143953 ) ) ;
#82443=CARTESIAN_POINT ( 'NONE',  ( -5.049401038298153566, 19.05341960407611168, 85.20724293864766707 ) ) ;
#82444=CARTESIAN_POINT ( 'NONE',  ( 18.67979575497178502, 10.72451020669898547, 64.16557627198102409 ) ) ;
#82445=CARTESIAN_POINT ( 'NONE',  ( -16.53943276465976808, -0.05219959533934237506, 28.75109039468567929 ) ) ;
#82446=CARTESIAN_POINT ( 'NONE',  ( 21.52544592524334988, 5.823673210054432836, 31.45942372801901854 ) ) ;
#82447=CARTESIAN_POINT ( 'NONE',  ( 21.53943276465977519, 0.05219959533937863772, 101.2510903946856757 ) ) ;
#82448=CARTESIAN_POINT ( 'NONE',  ( -16.52544592524335698, -4.483927247898792601, 98.95942372801903275 ) ) ;
#82449=CARTESIAN_POINT ( 'NONE',  ( -13.97604488694527625, -13.89961937509977652, 81.87390960531436690 ) ) ;
#82450=CARTESIAN_POINT ( 'NONE',  ( 14.29746914071049879, -8.314922557960816363, 83.33224293864769550 ) ) ;
#82451=CARTESIAN_POINT ( 'NONE',  ( 8.224510206698953496, -14.34966873604960469, 22.91557627198102765 ) ) ;
#82452=CARTESIAN_POINT ( 'NONE',  ( 5.049401038297881783, 19.05341960407617563, 67.29275706135234714 ) ) ;
#82453=CARTESIAN_POINT ( 'NONE',  ( 5.719274019375673035, 21.55341960407619339, 47.29275706135234003 ) ) ;
#82454=CARTESIAN_POINT ( 'NONE',  ( -16.55341960407611168, -4.379528057220339221, 96.45724293864770971 ) ) ;
#82455=CARTESIAN_POINT ( 'NONE',  ( 9.564922557960805705, 16.46253265017160317, 109.5822429386476955 ) ) ;
#82456=CARTESIAN_POINT ( 'NONE',  ( 8.314922557961029526, -14.29746914071037800, 105.4177570613523613 ) ) ;
#82457=CARTESIAN_POINT ( 'NONE',  ( -5.719274019375665041, -21.55341960407619695, 89.79275706135236135 ) ) ;
#82458=CARTESIAN_POINT ( 'NONE',  ( 14.34966873604972726, -8.224510206698740333, 50.83442372801901143 ) ) ;
#82459=CARTESIAN_POINT ( 'NONE',  ( 0.05219959533937995610, -21.53943276465977519, 45.00109039468568284 ) ) ;
#82460=EDGE_CURVE ( 'NONE', #107482, #188641, #158449, .T. ) ;
#82462=CARTESIAN_POINT ( 'NONE',  ( -18.67979575497178146, -10.72451020669898902, 111.6655762719810525 ) ) ;
#82463=CARTESIAN_POINT ( 'NONE',  ( -16.53943276465976808, 0.05219959533911058130, 96.24890960531435269 ) ) ;
#82465=CARTESIAN_POINT ( 'NONE',  ( 8.314922557960818139, 14.29746914071049879, 64.58224293864769550 ) ) ;
#82466=CARTESIAN_POINT ( 'NONE',  ( -16.55341960407617563, 4.379528057220093196, 108.5427570613523756 ) ) ;
#82467=CARTESIAN_POINT ( 'NONE',  ( 0.05219959533909260263, 19.03943276465977164, 34.99890960531435979 ) ) ;
#82468=CARTESIAN_POINT ( 'NONE',  ( -15.80617190586745835, -15.72974639402198527, 46.87390960531435979 ) ) ;
#82469=CARTESIAN_POINT ( 'NONE',  ( -14.34966873604960291, -8.224510206698953496, 76.66557627198103830 ) ) ;
#82471=CARTESIAN_POINT ( 'NONE',  ( 5.823673210054125526, 21.52544592524343514, 84.79057627198102409 ) ) ;
#82472=CARTESIAN_POINT ( 'NONE',  ( -13.97604488694527625, -13.89961937509977652, 86.87390960531436690 ) ) ;
#82473=CARTESIAN_POINT ( 'NONE',  ( -0.05219959533909027116, -19.03943276465977164, 42.49890960531435269 ) ) ;
#82474=CARTESIAN_POINT ( 'NONE',  ( -16.51473224551082808, 9.474510206698731452, 88.33442372801900433 ) ) ;
#82475=CARTESIAN_POINT ( 'NONE',  ( -18.62759615963270932, 10.81492255796079327, 30.83224293864770260 ) ) ;
#82476=CARTESIAN_POINT ( 'NONE',  ( -15.80617190586768217, 15.72974639402176855, 63.12609039468568994 ) ) ;
#82477=B_SPLINE_CURVE_WITH_KNOTS ( 'NONE', 3,
 ( #170203, #49840, #94340, #185372, #111504, #18517, #19502, #186387, #20482, #138861, #173190, #95334, #62009, #125684, #1331, #47864, #341, #46863, #141836, #123674 ),
 .UNSPECIFIED., .F., .F.,
 ( 4, 2, 2, 2, 2, 2, 2, 2, 2, 4 ),
 ( 0.000000000000000000, 0.0004987090165372711848, 0.0009974180330745423696, 0.001246772541343177908, 0.001496127049611813446, 0.001994836066149084739, 0.002493545082686355815, 0.002742899590954988968, 0.002992254099223622121, 0.003989672132298143457 ),
 .UNSPECIFIED. ) ;
#82478=CARTESIAN_POINT ( 'NONE',  ( 19.02544592524343514, -5.153800228976328945, 48.54057627198103120 ) ) ;
#82479=CARTESIAN_POINT ( 'NONE',  ( -13.89961937509977652, 13.97604488694528158, 85.62390960531433848 ) ) ;
#82480=ORIENTED_EDGE ( 'NONE', *, *, #98256, .T. ) ;
#82481=CARTESIAN_POINT ( 'NONE',  ( -14.29746914071037622, -8.314922557961029526, 69.16775706135234714 ) ) ;
#82482=CARTESIAN_POINT ( 'NONE',  ( -5.719274019375665041, -21.55341960407619695, 44.79275706135234714 ) ) ;
#82483=CARTESIAN_POINT ( 'NONE',  ( 21.53943276465977519, 0.05219959533937863772, 71.25109039468568994 ) ) ;
#82484=CARTESIAN_POINT ( 'NONE',  ( 21.53943276465977519, -0.05219959533907433946, 23.74890960531435269 ) ) ;
#82485=CARTESIAN_POINT ( 'NONE',  ( -0.05219959533907301413, -21.53943276465977519, 97.49890960531436690 ) ) ;
#82486=CARTESIAN_POINT ( 'NONE',  ( -18.62759615963255300, -10.81492255796106328, 19.16775706135234714 ) ) ;
#82487=CARTESIAN_POINT ( 'NONE',  ( -4.379528057220086978, -16.55341960407618274, 59.79275706135234714 ) ) ;
#82488=CARTESIAN_POINT ( 'NONE',  ( -21.53943276465977519, 0.05219959533907696930, 66.24890960531436690 ) ) ;
#82489=CARTESIAN_POINT ( 'NONE',  ( 5.049401038297881783, 19.05341960407617563, 22.29275706135233648 ) ) ;
#82490=VECTOR ( 'NONE', #87793, 1000.000000000000000 ) ;
#82491=CARTESIAN_POINT ( 'NONE',  ( 9.564922557960805705, 16.46253265017160317, 69.58224293864770971 ) ) ;
#82492=CARTESIAN_POINT ( 'NONE',  ( 14.29746914071037800, 8.314922557961029526, 106.6677570613523756 ) ) ;
#82493=CARTESIAN_POINT ( 'NONE',  ( -17.50000000000147793, -3.254303733634544837, 104.9760410692860688 ) ) ;
#82494=CARTESIAN_POINT ( 'NONE',  ( 5.153800228976335163, 19.02544592524342804, 89.79057627198102409 ) ) ;
#82495=CARTESIAN_POINT ( 'NONE',  ( -8.314922557961024197, 14.29746914071037800, 37.91775706135235424 ) ) ;
#82497=CARTESIAN_POINT ( 'NONE',  ( -5.153800228976607833, 19.02544592524334988, 87.70942372801897591 ) ) ;
#82499=CARTESIAN_POINT ( 'NONE',  ( -5.823673210054116645, -21.52544592524344225, 62.29057627198102409 ) ) ;
#82500=CARTESIAN_POINT ( 'NONE',  ( 14.29746914071049879, -8.314922557960816363, 23.33224293864769194 ) ) ;
#82501=CARTESIAN_POINT ( 'NONE',  ( 5.153800228976615827, -19.02544592524334988, 95.20942372801897591 ) ) ;
#82502=DIRECTION ( 'NONE',  ( 0.000000000000000000, 0.000000000000000000, -1.000000000000000000 ) ) ;
#82503=CARTESIAN_POINT ( 'NONE',  ( -19.05341960407617563, 5.049401038297882671, 93.54275706135234714 ) ) ;
#82504=CARTESIAN_POINT ( 'NONE',  ( 21.55341960407610458, 5.719274019375980345, 83.95724293864770971 ) ) ;
#82505=CARTESIAN_POINT ( 'NONE',  ( -9.474510206698720793, -16.51473224551083518, 54.58442372801899722 ) ) ;
#82507=CARTESIAN_POINT ( 'NONE',  ( -5.049401038298153566, 19.05341960407611168, 70.20724293864769550 ) ) ;
#82508=CARTESIAN_POINT ( 'NONE',  ( -4.483927247898539470, -16.52544592524342804, 62.29057627198102409 ) ) ;
#82509=CARTESIAN_POINT ( 'NONE',  ( 13.89961937509977652, -13.97604488694527269, 53.12390960531434558 ) ) ;
#82510=CARTESIAN_POINT ( 'NONE',  ( -4.379528057220328563, 16.55341960407611168, 50.20724293864769550 ) ) ;
#82513=CARTESIAN_POINT ( 'NONE',  ( 12.14591786802309770, 12.06949235617756955, 24.37390960531435979 ) ) ;
#82514=CARTESIAN_POINT ( 'NONE',  ( 19.03943276465977164, -0.05219959533909143690, 63.74890960531435979 ) ) ;
#82515=CARTESIAN_POINT ( 'NONE',  ( -17.59860650958993844, 7.585241751806885979, 73.42337014262493256 ) ) ;
#82516=CARTESIAN_POINT ( 'NONE',  ( -0.05219959533936034679, 19.03943276465977164, 32.50109039468566863 ) ) ;
#82517=CARTESIAN_POINT ( 'NONE',  ( -14.34966873604972548, 8.224510206698743886, 53.33442372801901854 ) ) ;
#82518=CARTESIAN_POINT ( 'NONE',  ( 21.53943276465977519, -0.05219959533907433946, 53.74890960531437401 ) ) ;
#82519=CARTESIAN_POINT ( 'NONE',  ( -18.67979575497193778, 10.72451020669871902, 103.3344237280190043 ) ) ;
#82520=CARTESIAN_POINT ( 'NONE',  ( -13.97604488694527625, -13.89961937509977652, 71.87390960531433848 ) ) ;
#82521=CARTESIAN_POINT ( 'NONE',  ( 9.474510206698971260, -16.51473224551069308, 112.9155762719810383 ) ) ;
#82522=CARTESIAN_POINT ( 'NONE',  ( 16.46253265017160672, -9.564922557960803928, 108.3322429386476955 ) ) ;
#82524=CARTESIAN_POINT ( 'NONE',  ( -15.72974639402176322, -15.80617190586768395, 34.37609039468568284 ) ) ;
#82526=CARTESIAN_POINT ( 'NONE',  ( 14.29746914071049879, -8.314922557960816363, 88.33224293864769550 ) ) ;
#82527=CARTESIAN_POINT ( 'NONE',  ( -18.67979575497178146, -10.72451020669898902, 86.66557627198102409 ) ) ;
#82528=CARTESIAN_POINT ( 'NONE',  ( -19.05341960407611168, -5.049401038298163336, 76.45724293864769550 ) ) ;
#82530=CARTESIAN_POINT ( 'NONE',  ( -13.89961937509977652, 13.97604488694528158, 80.62390960531436690 ) ) ;
#82531=CARTESIAN_POINT ( 'NONE',  ( -10.72451020669870658, -18.67979575497194134, 19.58442372801901143 ) ) ;
#82532=ORIENTED_EDGE ( 'NONE', *, *, #78822, .F. ) ;
#82533=CARTESIAN_POINT ( 'NONE',  ( -9.474510206698964154, 16.51473224551069663, 75.41557627198103830 ) ) ;
#82534=CARTESIAN_POINT ( 'NONE',  ( 19.52217212775660116, -5.499999999999906741, 97.43993709005258097 ) ) ;
#82535=CARTESIAN_POINT ( 'NONE',  ( -19.05341960407611168, -5.049401038298163336, 26.45724293864769550 ) ) ;
#82536=CARTESIAN_POINT ( 'NONE',  ( 9.564922557960805705, 16.46253265017160317, 34.58224293864770260 ) ) ;
#82537=CARTESIAN_POINT ( 'NONE',  ( 13.89961937509957401, 13.97604488694547697, 111.8760903946856757 ) ) ;
#82539=CARTESIAN_POINT ( 'NONE',  ( -4.379528057220328563, 16.55341960407611168, 110.2072429386477239 ) ) ;
#82540=CARTESIAN_POINT ( 'NONE',  ( -10.81492255796105439, 18.62759615963255655, 77.91775706135231871 ) ) ;
#82541=CARTESIAN_POINT ( 'NONE',  ( 0.05219959533909260263, 19.03943276465977164, 59.99890960531436690 ) ) ;
#82542=CARTESIAN_POINT ( 'NONE',  ( -10.81492255796105439, 18.62759615963255655, 37.91775706135235424 ) ) ;
#82543=CARTESIAN_POINT ( 'NONE',  ( -18.67979575497178146, -10.72451020669898902, 111.6655762719810525 ) ) ;
#82545=CARTESIAN_POINT ( 'NONE',  ( -13.89961937509977652, 13.97604488694528158, 80.62390960531436690 ) ) ;
#82547=CARTESIAN_POINT ( 'NONE',  ( -8.314922557961024197, 14.29746914071037800, 32.91775706135234714 ) ) ;
#82548=CARTESIAN_POINT ( 'NONE',  ( 0.05219959533907565091, 21.53943276465977519, 39.99890960531436690 ) ) ;
#82549=CARTESIAN_POINT ( 'NONE',  ( -10.81492255796105439, 18.62759615963255655, 67.91775706135234714 ) ) ;
#82550=CARTESIAN_POINT ( 'NONE',  ( -0.05219959533909027116, -19.03943276465977164, 112.4989096053143669 ) ) ;
#82551=CARTESIAN_POINT ( 'NONE',  ( 16.51473224551083163, -9.474510206698727899, 90.83442372801900433 ) ) ;
#82552=CARTESIAN_POINT ( 'NONE',  ( -19.02544592524342804, 5.153800228976336051, 46.04057627198101699 ) ) ;
#82553=CARTESIAN_POINT ( 'NONE',  ( -19.05341960407611168, -5.049401038298163336, 86.45724293864769550 ) ) ;
#82554=CARTESIAN_POINT ( 'NONE',  ( 16.55341960407611168, 4.379528057220329451, 93.95724293864770971 ) ) ;
#82555=CARTESIAN_POINT ( 'NONE',  ( -16.52544592524342804, 4.483927247898546575, 96.04057627198102409 ) ) ;
#82556=CARTESIAN_POINT ( 'NONE',  ( 9.474510206698971260, -16.51473224551069308, 112.9155762719810383 ) ) ;
#82557=CARTESIAN_POINT ( 'NONE',  ( 12.06949235617757843, -12.14591786802309237, 58.12390960531435979 ) ) ;
#82558=CARTESIAN_POINT ( 'NONE',  ( -16.51473224551069308, -9.474510206698971260, 41.66557627198103120 ) ) ;
#82559=CARTESIAN_POINT ( 'NONE',  ( -21.53943276465977519, -0.05219959533937600094, 63.75109039468568284 ) ) ;
#82560=CARTESIAN_POINT ( 'NONE',  ( 16.46253265017146816, 9.564922557961045513, 91.66775706135234714 ) ) ;
#82561=CARTESIAN_POINT ( 'NONE',  ( 16.55341960407611168, 4.379528057220329451, 63.95724293864770260 ) ) ;
#82562=CARTESIAN_POINT ( 'NONE',  ( -21.52544592524343514, 5.823673210054127303, 111.0405762719810525 ) ) ;
#82563=CARTESIAN_POINT ( 'NONE',  ( -15.72974639402197994, 15.80617190586746368, 40.62390960531435269 ) ) ;
#82565=CARTESIAN_POINT ( 'NONE',  ( -13.97604488694527625, -13.89961937509977652, 106.8739096053143669 ) ) ;
#82567=CARTESIAN_POINT ( 'NONE',  ( -19.02544592524342804, 5.153800228976336051, 61.04057627198103120 ) ) ;
#82568=CARTESIAN_POINT ( 'NONE',  ( 4.379528057220339221, -16.55341960407611168, 37.70724293864769550 ) ) ;
#82569=CARTESIAN_POINT ( 'NONE',  ( -16.52544592524335698, -4.483927247898792601, 98.95942372801903275 ) ) ;
#82570=CARTESIAN_POINT ( 'NONE',  ( 8.314922557961029526, -14.29746914071037800, 90.41775706135236135 ) ) ;
#82571=CARTESIAN_POINT ( 'NONE',  ( 9.564922557961047289, -16.46253265017146816, 35.41775706135233293 ) ) ;
#82573=CARTESIAN_POINT ( 'NONE',  ( 16.51473224551069308, 9.474510206698969483, 94.16557627198103830 ) ) ;
#82574=CARTESIAN_POINT ( 'NONE',  ( -13.97604488694527625, -13.89961937509977652, 51.87390960531436690 ) ) ;
#82575=CARTESIAN_POINT ( 'NONE',  ( -16.55341960407611168, -4.379528057220339221, 56.45724293864768839 ) ) ;
#82576=CARTESIAN_POINT ( 'NONE',  ( 17.26172910966780094, -6.454744622555852018, 103.3064690864922426 ) ) ;
#82577=CARTESIAN_POINT ( 'NONE',  ( 10.81492255796078972, 18.62759615963270932, 24.58224293864768839 ) ) ;
#82578=CARTESIAN_POINT ( 'NONE',  ( -10.81492255796078084, -18.62759615963271287, 42.08224293864769550 ) ) ;
#82579=CARTESIAN_POINT ( 'NONE',  ( 4.379528057220339221, -16.55341960407611168, 87.70724293864769550 ) ) ;
#82580=CARTESIAN_POINT ( 'NONE',  ( -14.34966873604972548, 8.224510206698743886, 33.33442372801900433 ) ) ;
#82581=CARTESIAN_POINT ( 'NONE',  ( 14.29746914071049879, -8.314922557960816363, 73.33224293864769550 ) ) ;
#82582=CARTESIAN_POINT ( 'NONE',  ( -18.39443945427638738, 5.500000000000031086, 63.51745347608650150 ) ) ;
#82583=CARTESIAN_POINT ( 'NONE',  ( -5.153800228976607833, 19.02544592524334988, 72.70942372801900433 ) ) ;
#82584=CARTESIAN_POINT ( 'NONE',  ( -19.03943276465977164, 0.05219959533909376836, 111.2489096053143669 ) ) ;
#82587=CARTESIAN_POINT ( 'NONE',  ( -12.14591786802326823, 12.06949235617739902, 23.12609039468567573 ) ) ;
#82588=CARTESIAN_POINT ( 'NONE',  ( -4.483927247898539470, -16.52544592524342804, 22.29057627198102765 ) ) ;
#82589=CARTESIAN_POINT ( 'NONE',  ( -16.51473224551082808, 9.474510206698731452, 73.33442372801900433 ) ) ;
#82590=CARTESIAN_POINT ( 'NONE',  ( 5.823673210054125526, 21.52544592524343514, 49.79057627198102409 ) ) ;
#82591=CARTESIAN_POINT ( 'NONE',  ( -5.823673210054431948, 21.52544592524334988, 67.70942372801901854 ) ) ;
#82592=CARTESIAN_POINT ( 'NONE',  ( 16.53943276465976808, 0.05219959533934440121, 36.25109039468567573 ) ) ;
#82593=CARTESIAN_POINT ( 'NONE',  ( 16.46253265017160672, -9.564922557960803928, 28.33224293864769550 ) ) ;
#82594=CARTESIAN_POINT ( 'NONE',  ( 9.474510206698971260, -16.51473224551069308, 82.91557627198103830 ) ) ;
#82596=CARTESIAN_POINT ( 'NONE',  ( -8.224510206698948167, 14.34966873604960824, 85.41557627198102409 ) ) ;
#82598=CARTESIAN_POINT ( 'NONE',  ( -19.03943276465977164, 0.05219959533909376836, 96.24890960531436690 ) ) ;
#82599=VERTEX_POINT ( 'NONE', #173639 ) ;
#82600=CARTESIAN_POINT ( 'NONE',  ( -5.049401038297874678, -19.05341960407617918, 109.7927570613523187 ) ) ;
#82601=CARTESIAN_POINT ( 'NONE',  ( 21.52544592524344225, -5.823673210054117533, 78.54057627198103830 ) ) ;
#82602=CARTESIAN_POINT ( 'NONE',  ( 0.05219959533909260263, 19.03943276465977164, 39.99890960531436690 ) ) ;
#82603=CARTESIAN_POINT ( 'NONE',  ( -19.02544592524334988, -5.153800228976617603, 73.95942372801900433 ) ) ;
#82604=CARTESIAN_POINT ( 'NONE',  ( 15.72974639402199770, -15.80617190586745480, 113.1239096053143953 ) ) ;
#82605=CARTESIAN_POINT ( 'NONE',  ( -19.03943276465977164, 0.05219959533909376836, 66.24890960531436690 ) ) ;
#82606=CARTESIAN_POINT ( 'NONE',  ( -0.05219959533909027116, -19.03943276465977164, 112.4989096053143669 ) ) ;
#82608=CARTESIAN_POINT ( 'NONE',  ( 8.314922557961029526, -14.29746914071037800, 30.41775706135234358 ) ) ;
#82609=CARTESIAN_POINT ( 'NONE',  ( -5.823673210054116645, -21.52544592524344225, 102.2905762719810383 ) ) ;
#82610=CARTESIAN_POINT ( 'NONE',  ( 12.14591786802309770, 12.06949235617756955, 104.3739096053143669 ) ) ;
#82611=CARTESIAN_POINT ( 'NONE',  ( -16.46253265017160317, 9.564922557960807481, 95.83224293864769550 ) ) ;
#82612=CARTESIAN_POINT ( 'NONE',  ( 13.97604488694548053, -13.89961937509957401, 55.62609039468566863 ) ) ;
#82613=CARTESIAN_POINT ( 'NONE',  ( -5.823673210054116645, -21.52544592524344225, 87.29057627198103830 ) ) ;
#82614=CARTESIAN_POINT ( 'NONE',  ( 14.29746914071049879, -8.314922557960816363, 48.33224293864770260 ) ) ;
#82615=CARTESIAN_POINT ( 'NONE',  ( 5.049401038297881783, 19.05341960407617563, 27.29275706135232937 ) ) ;
#82616=CARTESIAN_POINT ( 'NONE',  ( -16.52544592524335698, -4.483927247898792601, 58.95942372801902565 ) ) ;
#82617=CARTESIAN_POINT ( 'NONE',  ( 13.89961937509977652, -13.97604488694527269, 88.12390960531438111 ) ) ;
#82618=CARTESIAN_POINT ( 'NONE',  ( -19.05341960407611168, -5.049401038298163336, 41.45724293864769550 ) ) ;
#82619=CARTESIAN_POINT ( 'NONE',  ( 5.719274019375673035, 21.55341960407619339, 47.29275706135234003 ) ) ;
#82620=CARTESIAN_POINT ( 'NONE',  ( -5.823673210054431948, 21.52544592524334988, 62.70942372801902565 ) ) ;
#82621=CARTESIAN_POINT ( 'NONE',  ( 19.02544592524343514, -5.153800228976328945, 63.54057627198103830 ) ) ;
#82622=CARTESIAN_POINT ( 'NONE',  ( 21.55341960407619695, -5.719274019375665929, 31.04275706135234714 ) ) ;
#82623=CARTESIAN_POINT ( 'NONE',  ( -16.51473224551082808, 9.474510206698731452, 68.33442372801900433 ) ) ;
#82624=CARTESIAN_POINT ( 'NONE',  ( -9.564922557961040184, 16.46253265017147172, 72.91775706135233293 ) ) ;
#82625=CARTESIAN_POINT ( 'NONE',  ( 5.049401038298161559, -19.05341960407611168, 42.70724293864767418 ) ) ;
#82626=CARTESIAN_POINT ( 'NONE',  ( -12.14591786802326823, 12.06949235617739902, 88.12609039468570415 ) ) ;
#82627=CARTESIAN_POINT ( 'NONE',  ( 13.89961937509977652, -13.97604488694527269, 48.12390960531435979 ) ) ;
#82628=CARTESIAN_POINT ( 'NONE',  ( -13.97604488694527625, -13.89961937509977652, 26.87390960531434558 ) ) ;
#82629=CARTESIAN_POINT ( 'NONE',  ( 16.51473224551069308, 9.474510206698969483, 104.1655762719810241 ) ) ;
#82630=CARTESIAN_POINT ( 'NONE',  ( -5.153800228976328057, -19.02544592524343514, 37.29057627198102409 ) ) ;
#82631=CARTESIAN_POINT ( 'NONE',  ( -21.52544592524343514, 5.823673210054127303, 86.04057627198102409 ) ) ;
#82632=CARTESIAN_POINT ( 'NONE',  ( -8.314922557961024197, 14.29746914071037800, 57.91775706135234714 ) ) ;
#82633=CARTESIAN_POINT ( 'NONE',  ( -0.05219959533936034679, 19.03943276465977164, 37.50109039468567573 ) ) ;
#82634=CARTESIAN_POINT ( 'NONE',  ( -19.02544592524342804, 5.153800228976336051, 51.04057627198103120 ) ) ;
#82635=CARTESIAN_POINT ( 'NONE',  ( -14.29746914071049879, 8.314922557960819915, 45.83224293864769550 ) ) ;
#82636=CARTESIAN_POINT ( 'NONE',  ( 4.483927247898545687, 16.52544592524342804, 84.79057627198102409 ) ) ;
#82637=CARTESIAN_POINT ( 'NONE',  ( 19.03943276465977164, -0.05219959533909143690, 98.74890960531436690 ) ) ;
#82638=CARTESIAN_POINT ( 'NONE',  ( -5.049401038298153566, 19.05341960407611168, 85.20724293864766707 ) ) ;
#82639=CARTESIAN_POINT ( 'NONE',  ( -18.62759615963255300, -10.81492255796106328, 39.16775706135235424 ) ) ;
#82640=CARTESIAN_POINT ( 'NONE',  ( 16.46253265017160672, -9.564922557960803928, 88.33224293864769550 ) ) ;
#82641=CARTESIAN_POINT ( 'NONE',  ( -15.80617190586768217, 15.72974639402176855, 93.12609039468568994 ) ) ;
#82642=CARTESIAN_POINT ( 'NONE',  ( -8.314922557961024197, 14.29746914071037800, 82.91775706135234714 ) ) ;
#82643=CARTESIAN_POINT ( 'NONE',  ( -10.81492255796105439, 18.62759615963255655, 22.91775706135235069 ) ) ;
#82644=CARTESIAN_POINT ( 'NONE',  ( -15.80617190586745835, -15.72974639402198527, 91.87390960531436690 ) ) ;
#82645=CARTESIAN_POINT ( 'NONE',  ( 12.06949235617757843, -12.14591786802309237, 53.12390960531436690 ) ) ;
#82646=CARTESIAN_POINT ( 'NONE',  ( 13.89961937509977652, -13.97604488694527269, 43.12390960531434558 ) ) ;
#82647=CARTESIAN_POINT ( 'NONE',  ( -16.55341960407611168, -4.379528057220339221, 71.45724293864769550 ) ) ;
#82648=B_SPLINE_CURVE_WITH_KNOTS ( 'NONE', 3,
 ( #130502, #38517, #117349, #83999, #23349, #56688 ),
 .UNSPECIFIED., .F., .F.,
 ( 4, 2, 4 ),
 ( 0.000000000000000000, 0.0003837532665635236652, 0.0007675065331270473305 ),
 .UNSPECIFIED. ) ;
#82649=CARTESIAN_POINT ( 'NONE',  ( -10.81492255796078084, -18.62759615963271287, 27.08224293864769550 ) ) ;
#82650=CARTESIAN_POINT ( 'NONE',  ( 16.46253265017146816, 9.564922557961045513, 36.66775706135233293 ) ) ;
#82651=CARTESIAN_POINT ( 'NONE',  ( 12.06949235617757843, -12.14591786802309237, 103.1239096053143811 ) ) ;
#82653=CARTESIAN_POINT ( 'NONE',  ( 4.379528057220092307, 16.55341960407617563, 57.29275706135234714 ) ) ;
#82654=CARTESIAN_POINT ( 'NONE',  ( 0.05219959533909260263, 19.03943276465977164, 74.99890960531435269 ) ) ;
#82655=CARTESIAN_POINT ( 'NONE',  ( -17.15575107149451028, -6.384131856062659871, 21.29645598401388895 ) ) ;
#82656=CARTESIAN_POINT ( 'NONE',  ( 21.53943276465977519, -0.05219959533907433946, 43.74890960531435979 ) ) ;
#82657=CARTESIAN_POINT ( 'NONE',  ( -12.06949235617739369, -12.14591786802326823, 94.37609039468568994 ) ) ;
#82658=CARTESIAN_POINT ( 'NONE',  ( -5.153800228976607833, 19.02544592524334988, 107.7094237280189759 ) ) ;
#82659=CARTESIAN_POINT ( 'NONE',  ( 21.53943276465977519, 0.05219959533937863772, 81.25109039468568994 ) ) ;
#82660=CARTESIAN_POINT ( 'NONE',  ( -13.89961937509977652, 13.97604488694528158, 80.62390960531436690 ) ) ;
#82661=CARTESIAN_POINT ( 'NONE',  ( -18.67979575497178146, -10.72451020669898902, 106.6655762719810383 ) ) ;
#82662=CARTESIAN_POINT ( 'NONE',  ( -16.55341960407617563, 4.379528057220093196, 53.54275706135234714 ) ) ;
#82663=CARTESIAN_POINT ( 'NONE',  ( -16.53943276465976808, 0.05219959533911058130, 111.2489096053143669 ) ) ;
#82665=CARTESIAN_POINT ( 'NONE',  ( -16.55341960407617563, 4.379528057220093196, 23.54275706135235424 ) ) ;
#82666=CARTESIAN_POINT ( 'NONE',  ( -9.474510206698720793, -16.51473224551083518, 79.58442372801899012 ) ) ;
#82667=CARTESIAN_POINT ( 'NONE',  ( 10.72451020669898902, -18.67979575497178502, 82.91557627198103830 ) ) ;
#82668=CARTESIAN_POINT ( 'NONE',  ( -16.46253265017146816, -9.564922557961047289, 59.16775706135233293 ) ) ;
#82669=CARTESIAN_POINT ( 'NONE',  ( 30.00000000000000000, -5.499999999999992895, 102.5000000000000142 ) ) ;
#82670=CARTESIAN_POINT ( 'NONE',  ( -21.52544592524343514, 5.823673210054127303, 106.0405762719810525 ) ) ;
#82672=CARTESIAN_POINT ( 'NONE',  ( 13.89961937509977652, -13.97604488694527269, 78.12390960531433848 ) ) ;
#82674=CARTESIAN_POINT ( 'NONE',  ( -4.483927247898782831, 16.52544592524335698, 27.70942372801901854 ) ) ;
#82676=CARTESIAN_POINT ( 'NONE',  ( 21.53943276465977519, -0.05219959533907433946, 108.7489096053143669 ) ) ;
#82677=CARTESIAN_POINT ( 'NONE',  ( -0.05219959533910754901, -16.53943276465976808, 62.49890960531436690 ) ) ;
#82678=CARTESIAN_POINT ( 'NONE',  ( 16.46253265017160672, -9.564922557960803928, 63.33224293864769550 ) ) ;
#82679=CARTESIAN_POINT ( 'NONE',  ( 18.62759615963255655, 10.81492255796105972, 86.66775706135234714 ) ) ;
#82680=CARTESIAN_POINT ( 'NONE',  ( -0.05219959533934338120, 16.53943276465976808, 42.50109039468567573 ) ) ;
#82681=CARTESIAN_POINT ( 'NONE',  ( 19.03943276465977164, 0.05219959533936151252, 46.25109039468566863 ) ) ;
#82682=CARTESIAN_POINT ( 'NONE',  ( 10.81492255796106328, -18.62759615963255655, 50.41775706135235424 ) ) ;
#82683=CARTESIAN_POINT ( 'NONE',  ( 18.62759615963271287, -10.81492255796078972, 63.33224293864770260 ) ) ;
#82684=CARTESIAN_POINT ( 'NONE',  ( 19.02544592524334988, 5.153800228976608722, 106.4594237280190185 ) ) ;
#82685=CARTESIAN_POINT ( 'NONE',  ( -9.474510206698964154, 16.51473224551069663, 50.41557627198102409 ) ) ;
#82686=CARTESIAN_POINT ( 'NONE',  ( -5.049401038297874678, -19.05341960407617918, 64.79275706135233293 ) ) ;
#82687=CARTESIAN_POINT ( 'NONE',  ( -15.72974639402176322, -15.80617190586768395, 79.37609039468567573 ) ) ;
#82688=CARTESIAN_POINT ( 'NONE',  ( -19.03943276465977164, -0.05219959533935918106, 53.75109039468566863 ) ) ;
#82689=CARTESIAN_POINT ( 'NONE',  ( -19.03943276465977164, 0.05219959533909376836, 31.24890960531435979 ) ) ;
#82690=CARTESIAN_POINT ( 'NONE',  ( 10.72451020669898902, -18.67979575497178502, 52.91557627198103830 ) ) ;
#82691=CARTESIAN_POINT ( 'NONE',  ( -14.34966873604960291, -8.224510206698953496, 56.66557627198103830 ) ) ;
#82693=CARTESIAN_POINT ( 'NONE',  ( 19.02544592524334988, 5.153800228976608722, 26.45942372801899722 ) ) ;
#82694=CARTESIAN_POINT ( 'NONE',  ( 8.314922557961029526, -14.29746914071037800, 85.41775706135236135 ) ) ;
#82695=CARTESIAN_POINT ( 'NONE',  ( 12.14591786802309770, 12.06949235617756955, 59.37390960531436690 ) ) ;
#82696=CARTESIAN_POINT ( 'NONE',  ( -10.72451020669870658, -18.67979575497194134, 84.58442372801903275 ) ) ;
#82697=CARTESIAN_POINT ( 'NONE',  ( 21.52544592524334988, 5.823673210054432836, 76.45942372801901854 ) ) ;
#82698=CARTESIAN_POINT ( 'NONE',  ( 15.72974639402199770, -15.80617190586745480, 93.12390960531436690 ) ) ;
#82700=CARTESIAN_POINT ( 'NONE',  ( -9.564922557960796823, -16.46253265017161027, 47.08224293864769550 ) ) ;
#82701=CARTESIAN_POINT ( 'NONE',  ( 5.719274019375673035, 21.55341960407619339, 62.29275706135236845 ) ) ;
#82702=CARTESIAN_POINT ( 'NONE',  ( -13.97604488694527625, -13.89961937509977652, 36.87390960531436690 ) ) ;
#82704=CARTESIAN_POINT ( 'NONE',  ( -13.97604488694527625, -13.89961937509977652, 46.87390960531435979 ) ) ;
#82705=CARTESIAN_POINT ( 'NONE',  ( -12.06949235617756955, 12.14591786802309770, 100.6239096053143811 ) ) ;
#82706=CARTESIAN_POINT ( 'NONE',  ( 9.474510206698971260, -16.51473224551069308, 102.9155762719810241 ) ) ;
#82707=AXIS2_PLACEMENT_3D ( 'NONE', #97453, #3475, #65152 ) ;
#82708=CARTESIAN_POINT ( 'NONE',  ( 14.34966873604960469, 8.224510206698951720, 59.16557627198103120 ) ) ;
#82709=CARTESIAN_POINT ( 'NONE',  ( 12.06949235617757843, -12.14591786802309237, 113.1239096053143953 ) ) ;
#82710=CARTESIAN_POINT ( 'NONE',  ( 21.53943276465977519, -0.05219959533907433946, 78.74890960531436690 ) ) ;
#82711=CARTESIAN_POINT ( 'NONE',  ( 21.52544592524344225, -5.823673210054117533, 113.5405762719810383 ) ) ;
#82713=CARTESIAN_POINT ( 'NONE',  ( -8.314922557961024197, 14.29746914071037800, 32.91775706135234714 ) ) ;
#82715=CARTESIAN_POINT ( 'NONE',  ( 10.72451020669898902, -18.67979575497178502, 82.91557627198103830 ) ) ;
#82717=CARTESIAN_POINT ( 'NONE',  ( 0.05219959533937995610, -21.53943276465977519, 110.0010903946856757 ) ) ;
#82718=CARTESIAN_POINT ( 'NONE',  ( 19.02544592524343514, -5.153800228976328945, 98.54057627198100988 ) ) ;
#82719=CARTESIAN_POINT ( 'NONE',  ( -18.62759615963255300, -10.81492255796106328, 29.16775706135234003 ) ) ;
#82721=CARTESIAN_POINT ( 'NONE',  ( -0.05219959533907301413, -21.53943276465977519, 32.49890960531435979 ) ) ;
#82722=CARTESIAN_POINT ( 'NONE',  ( -12.14591786802326823, 12.06949235617739902, 98.12609039468570415 ) ) ;
#82723=CARTESIAN_POINT ( 'NONE',  ( -5.823673210054431948, 21.52544592524334988, 47.70942372801902565 ) ) ;
#82724=CARTESIAN_POINT ( 'NONE',  ( 21.53943276465977519, 0.05219959533937863772, 86.25109039468568994 ) ) ;
#82725=CARTESIAN_POINT ( 'NONE',  ( -10.81492255796105439, 18.62759615963255655, 107.9177570613523471 ) ) ;
#82726=CARTESIAN_POINT ( 'NONE',  ( -0.05219959533934338120, 16.53943276465976808, 72.50109039468568994 ) ) ;
#82727=CARTESIAN_POINT ( 'NONE',  ( -5.823673210054431948, 21.52544592524334988, 37.70942372801900433 ) ) ;
#82728=CARTESIAN_POINT ( 'NONE',  ( -13.97604488694527625, -13.89961937509977652, 31.87390960531435979 ) ) ;
#82729=CARTESIAN_POINT ( 'NONE',  ( -18.62759615963255300, -10.81492255796106328, 104.1677570613523471 ) ) ;
#82730=CARTESIAN_POINT ( 'NONE',  ( 0.05219959533909260263, 19.03943276465977164, 109.9989096053143669 ) ) ;
#82731=CARTESIAN_POINT ( 'NONE',  ( -15.72974639402197994, 15.80617190586746368, 105.6239096053143669 ) ) ;
#82733=CARTESIAN_POINT ( 'NONE',  ( 0.05219959533907565091, 21.53943276465977519, 64.99890960531435269 ) ) ;
#82734=CARTESIAN_POINT ( 'NONE',  ( 14.34966873604972726, -8.224510206698740333, 55.83442372801901854 ) ) ;
#82735=CARTESIAN_POINT ( 'NONE',  ( -12.06949235617756955, 12.14591786802309770, 45.62390960531436690 ) ) ;
#82737=CARTESIAN_POINT ( 'NONE',  ( -13.97604488694547697, 13.89961937509957934, 88.12609039468563310 ) ) ;
#82738=( BOUNDED_SURFACE ( )  B_SPLINE_SURFACE ( 3, 2, ( 
 ( #197980, #59450, #154903, #80048, #126542, #141717, #138733, #15404, #79048, #17392, #173069, #63893, #139717, #45741, #95215, #107393, #140722, #60893, #1205, #184259, #33553, #77061, #62882, #64881, #169066, #125564, #16402, #213, #47738, #108399, #2212, #122569, #188241, #124563, #187261, #123552, #171071, #49716, #196720, #172066, #30572, #109391, #3207, #157894, #111381, #92223, #153909, #94215, #34546, #78048, #31567, #96205, #110384, #61882, #73372, #185247, #186260, #155894, #32561, #93218, #46738, #156901, #48730, #135044, #170076, #18397, #5183, #114358, #52694, #127538, #190221, #38541, #130526, #193224, #54698, #176063, #65866, #66864, #174068, #116371, #178059, #6185, #82007, #39527, #99193, #128527, #101187, #112376, #84023, #83025, #19383, #37530, #50718, #192223, #175055, #189240, #53705, #160881, #100197, #22372, #81032, #35537, #115382, #51700, #4187, #97184, #177070, #158870, #8196, #20359, #68867, #159876, #143701, #191220, #113363, #145701, #36519, #69871, #67865, #7183, #98174, #161879, #131540, #142708, #23373, #21367, #85018, #146699, #144699, #129520, #117371, #132543, #181064, #121343, #103208, #118382, #198201, #197221, #163897, #59671, #70876, #88023, #42539, #149711, #180076, #194232, #120350, #57711, #183036, #148720, #40537, #10208, #119381, #196242, #55698, #133536, #182045, #73879, #136520, #44519, #104202, #9209, #71868, #179068, #162876, #24384, #11210, #25393, #86035, #165883, #195228, #147722, #102208, #27380, #26384, #87035, #89026, #56709, #135549, #41545, #164890, #58683, #150717, #43528, #12216, #72885, #134554, #105193, #166880, #28381, #90019, #151702, #13195, #74858, #186020, #75832, #139487, #141487, #93982, #969, #188008, #152675, #200180, #155662, #17158, #64650, #90988, #153671, #184023, #62645, #45505, #2970, #138498, #106175, #169838, #185010, #110153, #156665, #171831, #168831, #107160, #109158, #47502, #126312, #78811, #31332, #137510, #125331, #199191, #170837, #14164, #92983, #60658, #63658, #30336, #154668, #122331, #140490, #76827, #29358, #1978, #167858, #18160, #79816, #91977, #16164, #108156, #15168, #61649, #123317, #77818, #46495, #187028, #124322, #32329, #48499, #33319, #94980, #52450, #50479, #34310, #82775, #53450, #144456, #65631, #38290, #157657, #160631, #173831, #114107, #189985, #127291, #189004, #112139, #35296, #37283, #96952, #176818, #98940, #99944, #83772, #128287, #67617, #5941, #175810, #66623, #161630, #69623, #23124, #4939, #174811, #111141, #97931, #131289, #49478, #22122, #129278, #172831, #36276, #158632, #20123, #21119, #81767, #143454, #84769, #51459, #113121, #19146, #115125, #142474, #145452, #191964, #159624, #95973, #80796, #146447, #3952, #6934, #7940, #190973, #68613, #130269, #181802, #10958, #74616, #134307, #54456, #150474, #116126, #103957, #85785, #196977, #27134, #193988, #147471, #165636, #163640, #177815, #39285, #55450, #12951, #56457, #180818, #26135, #135305, #100942, #8961, #70629, #28138, #72632, #42297, #162626, #57466, #24133, #118136, #192977, #120112, #132296, #119138, #88781, #178815, #117121, #40285, #58444, #11969, #179825, #89778, #149463, #101959, #73634, #148469, #25142, #43281, #195993, #104950, #166636, #86784, #9962, #151463, #71622, #133288, #194978, #41295, #102956, #164640, #87778, #105936, #169596, #171593, #124072, #31094, #17918, #182795, #30097, #185773, #47260, #94737, #121101, #183784, #13925, #92742, #75592, #33081, #168597, #136282, #199949, #14930, #140242, #186785, #1734, #198953, #137271, #139254, #77582, #156417, #108917, #61413, #167621, #155425, #29117, #730, #44278, #123084, #90756, #93744, #60420, #184770, #125087, #152439, #170597, #76590, #122093, #107911, #91737, #62402, #45270, #48255, #46256, #32087, #106924, #154430, #109909, #59427, #16915, #153432, #15924, #63412, #197958, #138266, #78568, #49243, #97695, #38055, #19890, #35058, #114887, #113871 ),
 ( #65393, #174581, #112887, #187773, #50245, #98704, #190740, #53209, #176581, #36046, #126077, #127054, #34073, #99711, #161395, #66390, #142231, #79573, #159386, #188761, #141242, #172587, #67382, #20881, #21887, #64408, #95731, #157417, #2731, #82539, #129039, #110901, #144221, #18911, #4700, #80556, #6698, #3716, #5705, #52214, #111901, #173589, #96713, #145216, #158401, #175568, #81531, #143218, #37045, #128052, #191727, #189754, #51226, #160398, #83537, #68376, #130028, #40042, #148233, #54222, #103727, #147230, #115893, #133055, #193748, #104715, #25904, #23891, #7698, #56217, #26900, #117899, #39050, #11736, #131050, #134067, #8722, #87549, #163406, #100708, #162388, #85544, #70391, #10727, #132059, #150241, #72391, #73403, #57231, #101716, #41060, #179588, #149236, #24902, #135074, #43049, #196750, #178577, #9727, #84533, #71391, #22887, #146210, #195757, #102723, #69381, #194745, #55216, #116885, #164412, #86549, #118905, #58217, #180589, #42063, #192740, #88543, #177583, #165407, #119886, #181571, #12719, #74385, #31846, #136050, #139010, #93497, #16674, #46015, #154193, #155184, #184535, #48015, #107671, #27901, #123827, #89544, #77344, #59191, #170354, #490, #167390, #120860, #62163, #137029, #151230, #197725, #28886, #186542, #29861, #185525, #45034, #169348, #122847, #92504, #183548, #78323, #166406, #139996, #121856, #91498, #182560, #14688, #30857, #1485, #106692, #44043, #60186, #15683, #47017, #124842, #105703, #13692, #90526, #108676, #152208, #63163, #198719, #75359, #153185, #168365, #76350, #138027, #199710, #61175, #49001, #112643, #50983, #6452, #97451, #173344, #79329, #128799, #140999, #174335, #94490, #34815, #17671, #67141, #110657, #96470, #98457, #2487, #159137, #49992, #33826, #81291, #141985, #35805, #156172, #160150, #158158, #20634, #157172, #4452, #21642, #32840, #5459, #64168, #142975, #175325, #191481, #36791, #125833, #187536, #127805, #68133, #111657, #65150, #144971, #143978, #172337, #129784, #95486, #19650, #189509, #66142, #126807, #18666, #190498, #82286, #109671, #80312, #3473, #188515, #51971, #113630, #83295, #171351, #72141, #164165, #26652, #88295, #86304, #99467, #38811, #7452, #149983, #11489, #39797, #115650, #73160, #132812, #100469, #134830, #145970, #117648, #116644, #52959, #9482, #84291, #25663, #8471, #161147, #87308, #194498, #133817, #114635, #180346, #70146, #178334, #176334, #101461, #37805, #163152, #195508, #55971, #22644, #24655, #177340, #162148, #147993, #85292, #23644, #41814, #131816, #146984, #69136, #56981, #130803, #40808, #118655, #193495, #192494, #53978, #103482, #54974, #148991, #165160, #71146, #179345, #102478, #10481, #14440, #78084, #137778, #57979, #153945, #119651, #107429, #89300, #249, #30608, #197487, #150992, #169101, #167147, #181333, #42812, #58954, #16435, #59943, #184295, #29618, #138768, #104474, #12484, #74145, #31603, #76103, #45777, #166159, #60931, #27660, #121611, #196509, #123588, #135817, #122605, #92261, #182318, #120622, #43798, #61918, #105461, #15440, #28646, #90282, #77099, #93252, #108433, #170109, #151966, #183306, #198472, #13454, #154938, #75118, #44788, #136786, #185282, #106441, #168122, #91250, #152941, #199464, #46774, #140756, #124598, #173104, #143739, #34581, #155931, #128562, #47773, #50751, #63927, #142742, #80081, #17426, #79083, #2244, #125596, #127574, #187293, #66899, #189275, #190257, #174101, #18431, #157926, #96238, #65900, #156934, #51734, #162660, #116158, #109426, #112409, #35570, #48764, #1239, #110419, #5218, #172100, #97218, #33586, #62918, #158904, #39316, #177848, #100976, #24166, #64914, #141750, #171105, #139752, #3240, #126575, #32598, #20395, #95249, #94251, #49749, #188276, #186293, #4222, #111418, #19416, #81064, #82042, #119168, #101992, #74649, #194020, #197012, #9994, #88814, #26168, #163673, #25175, #148504, #86817, #73666, #71654, #12986, #135338 ),
 ( #180852, #165668, #150507, #136315, #41327, #132329, #179857, #58477, #120144, #44310, #70662, #133321, #195011, #42328, #56488, #121134, #118166, #85817, #149495, #164673, #89813, #197990, #151494, #102987, #87809, #12005, #27167, #182828, #181835, #10992, #55483, #104982, #117153, #43315, #178849, #72664, #40315, #166669, #134340, #196024, #59461, #57499, #28171, #103989, #105969, #167654, #147504, #8994, #13957, #17952, #77617, #93777, #76621, #124108, #79605, #152471, #125122, #122126, #62435, #94770, #110933, #156453, #183814, #198984, #60452, #186819, #185808, #64440, #14961, #106955, #138299, #47294, #108951, #137303, #199980, #48289, #140276, #2764, #126111, #170631, #75624, #61446, #45304, #187806, #49275, #15957, #91770, #29150, #32120, #123117, #90787, #168628, #155458, #92776, #30128, #16948, #153464, #1768, #184802, #46288, #63446, #78602, #109945, #171626, #107945, #169631, #33114, #31127, #154465, #139287, #141275, #764, #82570, #52245, #142264, #5737, #113902, #175600, #22919, #128082, #18944, #66421, #21919, #160429, #131081, #157450, #19920, #50276, #129069, #111934, #7729, #4732, #172620, #36077, #51257, #176613, #84565, #38088, #35090, #173621, #37077, #98736, #69415, #83570, #97726, #3747, #191760, #65424, #145249, #80589, #159416, #127085, #130061, #96743, #20912, #161427, #188794, #6730, #112917, #158433, #144251, #189786, #68408, #81562, #146243, #67414, #53243, #143248, #190770, #192770, #95764, #114920, #174612, #99743, #54254, #34107, #43080, #70424, #85577, #134101, #74417, #56249, #71421, #151262, #150273, #116916, #12752, #23922, #41092, #195791, #102756, #133085, #177615, #162420, #178609, #136083, #179620, #103759, #149267, #58249, #100739, #132090, #8753, #197757, #57263, #165438, #147263, #180622, #193779, #164443, #115925, #104747, #55248, #42094, #88575, #101750, #39083, #40072, #181603, #163438, #26933, #86581, #24935, #11769, #148264, #27933, #89576, #9757, #25937, #117931, #194775, #87580, #10759, #72423, #118937, #196781, #73434, #135105, #119917, #166438, #141036, #62197, #60219, #44077, #92538, #63199, #154227, #75392, #48051, #167423, #170389, #183582, #123861, #199742, #137064, #198754, #121889, #45067, #47053, #106725, #186578, #108710, #109707, #93534, #138061, #77377, #15717, #185559, #76384, #171389, #79365, #32876, #14724, #184568, #120893, #107704, #17708, #122880, #78358, #31880, #182593, #46049, #168399, #29894, #30891, #91532, #153219, #94526, #61208, #169383, #28919, #124879, #152241, #155219, #1521, #139045, #105736, #90559, #156208, #13726, #16708, #59224, #525, #140032, #190534, #191521, #20670, #84329, #144014, #64203, #160188, #125870, #113667, #95523, #6490, #36829, #3511, #157209, #175361, #173382, #52008, #99505, #114676, #176372, #2523, #127842, #4490, #33863, #37845, #19687, #189548, #18703, #83332, #126846, #80350, #112681, #34852, #187570, #5495, #65187, #49038, #35843, #68170, #97489, #142022, #52998, #110693, #98495, #188552, #67178, #143012, #50030, #111695, #96507, #158197, #21678, #81329, #129822, #145009, #161186, #22682, #66180, #82324, #159175, #128835, #51020, #172373, #174373, #73198, #101501, #71185, #7491, #194537, #104513, #9519, #165197, #149031, #69176, #132849, #8508, #55011, #117686, #178371, #70186, #134868, #24694, #39835, #115690, #150023, #38850, #133856, #88332, #131854, #192533, #54016, #11528, #177378, #118693, #196546, #58016, #25700, #195546, #119686, #164202, #27695, #87345, #130842, #103521, #100507, #57020, #162186, #181369, #180385, #147024, #23684, #41855, #116681, #85332, #193537, #163190, #166194, #56008, #26692, #179383, #42848, #86343, #148030, #40845, #146008, #10519, #102519, #72182, #153983, #58991, #14478, #109460, #16470, #197523, #15480, #61956, #75155, #151028, #90318, #154974, #105498, #138806, #59981, #12519, #152979, #168159, #93289, #139788, #78119, #152004, #28683, #92299, #30646 ),
 ( #1276, #182356, #287, #29656, #13490, #60968, #121648, #77137, #74183, #62953, #137818, #123623, #136826, #184332, #124633, #135853, #185318, #43834, #122642, #186328, #171143, #47810, #167184, #120658, #107465, #89336, #91288, #44825, #198510, #46809, #183343, #106480, #76140, #199502, #169141, #45814, #108468, #170145, #31640, #127608, #67931, #18464, #110454, #80115, #189307, #65936, #140790, #3277, #51765, #143770, #6252, #129585, #50784, #79118, #141783, #187329, #191281, #52756, #19450, #95284, #114425, #112444, #64949, #32632, #125631, #97250, #96273, #94286, #174133, #63962, #5251, #188310, #2279, #66932, #35604, #113426, #158938, #155964, #48800, #128595, #126608, #17461, #172135, #190289, #33621, #142776, #20427, #156967, #82077, #175118, #36586, #83091, #49787, #111453, #173139, #98241, #159944, #34614, #157959, #81098, #4257, #21431, #144767, #11281, #8265, #176127, #9278, #192293, #164958, #84088, #87103, #100264, #179138, #116441, #53772, #115446, #38608, #177137, #163965, #161945, #103278, #25463, #26451, #10277, #54767, #194300, #132611, #102277, #193293, #88093, #196308, #149779, #131608, #101256, #37597, #24452, #134624, #39597, #195299, #40607, #99259, #162945, #23440, #85087, #147792, #69944, #146771, #72955, #178130, #86101, #145767, #180144, #68934, #148788, #118453, #70943, #22439, #7249, #41613, #130596, #71936, #57778, #160946, #55766, #133606, #117440, #56781, #1041, #60729, #181133, #76896, #42607, #30406, #12281, #123388, #153742, #120418, #73946, #92052, #90085, #104271, #165953, #182109, #139557, #183105, #107229, #152743, #61720, #27453, #135615, #197286, #154741, #137579, #168900, #89095, #184093, #150786, #44586, #119448, #46569, #58749, #45576, #15237, #105260, #43594, #166946, #185080, #28449, #138567, #151767, #13260, #45, #16237, #31403, #93054, #74923, #106243, #121412, #136586, #77889, #198266, #167925, #59742, #108230, #29425, #91056, #14233, #75904, #199262, #122403, #169911, #47573, #96044, #66698, #50553, #157731, #5016, #109225, #17227, #155729, #98005, #80870, #112213, #170904, #127368, #32396, #188080, #82852, #190058, #94051, #189080, #35372, #48568, #124396, #63726, #128362, #78879, #173903, #33390, #186091, #97024, #159699, #174886, #36352, #144531, #49551, #62714, #158705, #19220, #140558, #95049, #81840, #20194, #21196, #2047, #142546, #125401, #110221, #187098, #171902, #156738, #111214, #18232, #79886, #4024, #141556, #3045, #64721, #143528, #126383, #172906, #65702, #34384, #51534, #113197, #52522, #178895, #85861, #86865, #24212, #67696, #22198, #40363, #176895, #191049, #114183, #163721, #83847, #116205, #147550, #175887, #39364, #9038, #70707, #56536, #161708, #37358, #100021, #55529, #194068, #164719, #99016, #53525, #145529, #162707, #7008, #41371, #38366, #6017, #69699, #84847, #10040, #118214, #71700, #68690, #130345, #132375, #117203, #103037, #102038, #131366, #160707, #25223, #192044, #148549, #115203, #193055, #23204, #133367, #146525, #54532, #195058, #8016, #179905, #177894, #101022, #26214, #87853, #129354, #72712, #183861, #28217, #57543, #137346, #150550, #180897, #151540, #135385, #17746, #182873, #27211, #134384, #74695, #60495, #136360, #42372, #45348, #196070, #29196, #88857, #44354, #43358, #104035, #165714, #12049, #73713, #106013, #197055, #122171, #167699, #107000, #152514, #181879, #59504, #198036, #90830, #120189, #168673, #156244, #32911, #58523, #166713, #11036, #89857, #149541, #121179, #94565, #14002, #105029, #75669, #13029, #199026, #119212, #162357, #192705, #118874, #8688, #23858, #99678, #134033, #22853, #117866, #72359, #54188, #176546, #38022, #195726, #161362, #102692, #57199, #180558, #9694, #179556, #42032, #148201, #11705, #71359, #191693, #87517, #53176, #41026, #84500, #103696, #164380, #131015, #146178, #25873, #100675, #114852, #7663, #115861, #150208, #193714, #149205, #163371, #165375, #69347 ),
 ( #85509, #26869, #10696, #177551, #88512, #39020, #55183, #133023, #116852, #147197, #70358, #129993, #24868, #132025, #178543, #40009, #101682, #86517, #194713, #56182, #189993, #176828, #116136, #115136, #69633, #38300, #6943, #159632, #147481, #84779, #25152, #68622, #163650, #71632, #24143, #23134, #97939, #160640, #8971, #100952, #86794, #148481, #146457, #36284, #175818, #144464, #9972, #51468, #99954, #52458, #113129, #131299, #37291, #174819, #82783, #54466, #53460, #21128, #7950, #5949, #162636, #145461, #67626, #85795, #192988, #70640, #177825, #129286, #190981, #132306, #22131, #114115, #98950, #193998, #83782, #161640, #39295, #130278, #55460, #117131, #178824, #40295, #191973, #101969, #27144, #182805, #121111, #91747, #118144, #180828, #10967, #89788, #72641, #168607, #165646, #133298, #196988, #11979, #137281, #183794, #198963, #196002, #134316, #136292, #74626, #30107, #44288, #58454, #102965, #152449, #164650, #197968, #179834, #120122, #41304, #90766, #57475, #181813, #122104, #26145, #105946, #73644, #119147, #104960, #88791, #59438, #87787, #45281, #43291, #167631, #42306, #28148, #106934, #56466, #29128, #149472, #166646, #60430, #14940, #153442, #103967, #150484, #151473, #194988, #135315, #12962, #13935, #75602, #187783, #169607, #80566, #110911, #77594, #31105, #49253, #47271, #138276, #123095, #139265, #96723, #140253, #64418, #109921, #18921, #61424, #92753, #154441, #111911, #94748, #126087, #184781, #141252, #46267, #1745, #158411, #3726, #107922, #2741, #172597, #62413, #65403, #35068, #199959, #156428, #34083, #108928, #15935, #95741, #173599, #188771, #50255, #76600, #155436, #142241, #741, #63423, #93755, #125098, #124083, #157427, #185784, #170608, #186796, #32098, #16926, #79583, #78579, #48267, #171604, #127064, #33092, #17929, #8732, #128062, #131060, #144231, #22897, #160408, #97705, #36056, #82549, #159396, #7708, #5715, #147240, #69391, #70401, #54232, #98714, #38065, #176591, #146220, #37055, #132069, #40051, #193758, #175578, #145226, #81541, #68386, #178587, #83547, #39060, #84543, #143228, #6708, #67392, #129049, #191737, #52224, #190750, #55226, #21897, #113881, #189764, #23901, #112897, #192749, #162398, #130038, #66400, #51236, #85554, #174591, #115903, #116895, #101727, #99721, #177593, #19900, #161405, #4710, #100718, #20891, #53219, #114897, #121866, #43059, #10737, #45044, #56227, #27911, #26910, #198730, #119896, #194755, #74395, #118915, #9737, #136060, #104725, #44053, #181581, #24912, #179598, #197735, #134077, #148243, #71401, #120870, #41070, #73413, #166417, #133065, #196760, #89554, #151240, #13702, #180599, #117909, #57241, #12729, #59201, #183558, #102733, #72401, #164422, #182570, #25915, #60196, #195767, #163416, #88553, #42073, #167400, #75369, #28896, #87559, #149246, #105713, #90536, #86559, #152218, #150252, #103737, #137039, #165417, #11746, #135084, #58227, #14699, #64178, #46025, #31856, #95496, #199719, #156183, #47028, #30868, #78334, #139021, #109682, #91508, #157182, #155195, #171363, #154203, #1496, #18676, #29871, #2497, #61185, #140007, #172347, #188525, #33836, #122857, #76361, #124853, #65160, #108686, #62173, #141995, #17682, #106702, #93509, #32851, #16684, #186553, #63174, #123837, #138038, #125843, #48025, #3483, #185535, #80322, #168375, #141010, #94501, #184545, #77354, #187545, #79340, #126819, #153195, #49012, #107681, #92514, #169358, #15693, #501, #110667, #170364, #19660, #68142, #8480, #190507, #5468, #85301, #99476, #50002, #36801, #176343, #175334, #129793, #98466, #67150, #81301, #7461, #144981, #146993, #128808, #23653, #131825, #84300, #83304, #158168, #20643, #69145, #161157, #70155, #111667, #6461, #96480, #35815, #4463, #173354, #34825, #160160, #112654, #142985, #191490, #97461, #66152, #127815, #114645, #113639, #189520, #52968, #50993, #22653, #51981, #174345, #145979, #37815, #130812 ),
 ( #192503, #53987, #100478, #21651, #159147, #143987, #115660, #177350, #82296, #38820, #162157, #71155, #149992, #132821, #28656, #25672, #193506, #56990, #72150, #197496, #43807, #58963, #55980, #194507, #196518, #134839, #90291, #181342, #118664, #163161, #12493, #24664, #57989, #178343, #180355, #101471, #151002, #117657, #41824, #182328, #86313, #42821, #133826, #179354, #165169, #87317, #119660, #39805, #105470, #103491, #104484, #40817, #88304, #167156, #116652, #89309, #148002, #26662, #120631, #75127, #151975, #74155, #166168, #13463, #54983, #11498, #9492, #102487, #164174, #149001, #10490, #73169, #195517, #27669, #135826, #184305, #18439, #29627, #1248, #259, #172109, #93262, #168131, #47782, #92270, #183315, #109434, #16444, #17435, #154948, #198481, #152950, #171116, #107438, #121620, #44797, #94259, #14449, #46783, #78093, #106452, #170118, #139762, #62927, #187302, #153954, #91259, #30617, #186302, #124607, #95259, #76112, #45786, #137789, #32606, #199473, #33595, #169110, #136795, #61928, #15450, #140764, #48773, #2253, #60940, #122615, #155939, #79091, #156942, #63935, #123597, #77108, #125604, #138778, #110428, #185291, #108442, #31612, #59953, #19425, #5226, #71662, #173113, #129561, #20404, #4231, #51743, #112418, #83067, #64923, #133329, #128571, #144742, #127583, #175094, #195020, #3250, #178857, #34589, #113404, #148512, #164682, #10002, #96246, #49759, #98218, #41335, #82052, #35580, #118174, #194028, #80090, #66908, #6229, #190266, #159921, #36563, #97226, #111427, #40323, #21410, #179865, #158913, #56496, #141758, #117161, #67908, #188285, #50761, #55491, #102996, #126583, #101999, #157934, #163681, #81072, #142751, #65910, #189283, #174110, #25184, #143747, #86826, #181843, #61455, #75633, #26176, #12994, #152479, #151502, #105977, #74657, #43323, #196031, #183822, #121142, #123125, #104990, #199988, #107953, #60460, #59469, #134349, #197020, #45312, #137311, #184810, #46296, #182836, #72672, #12013, #180861, #87817, #149503, #136324, #88822, #11000, #167662, #73674, #57507, #119176, #90795, #89821, #42337, #44318, #103998, #198992, #166678, #165676, #122135, #29158, #106962, #13966, #27175, #150515, #168636, #58486, #135346, #120153, #30136, #28179, #197999, #91779, #153473, #14969, #76629, #138307, #19929, #125131, #15965, #63454, #18951, #157457, #128090, #154473, #16956, #47303, #126118, #108960, #4740, #1776, #169640, #33121, #48297, #173629, #81570, #35099, #32128, #170639, #172626, #110940, #66429, #80597, #94778, #139295, #188801, #772, #34114, #77625, #156460, #62442, #127092, #93785, #17959, #158441, #124116, #142272, #109953, #155466, #141282, #186828, #95771, #185816, #143256, #79613, #3754, #78610, #50284, #65431, #189794, #51265, #2772, #140284, #171633, #64448, #31136, #92784, #187813, #49282, #111942, #96751, #160437, #194784, #5746, #177624, #176622, #148274, #69424, #144259, #23930, #68416, #159424, #85585, #192779, #193787, #131091, #174620, #129077, #147271, #83578, #97735, #20920, #70431, #190778, #22928, #54262, #82578, #146252, #115934, #39092, #163446, #130069, #67422, #6738, #162429, #100748, #71430, #52253, #21927, #8762, #191768, #53251, #113910, #116924, #175609, #132097, #55256, #37085, #98744, #145257, #178617, #114929, #40080, #101758, #24943, #86591, #9766, #133094, #112925, #36085, #38097, #99752, #161436, #84574, #7738, #149275, #60229, #90568, #57271, #10768, #28928, #26942, #117940, #102765, #118946, #76394, #119927, #44087, #89585, #198763, #41100, #72432, #134110, #91541, #74426, #105745, #164452, #120902, #25946, #181612, #138070, #183591, #87589, #182602, #152250, #42104, #45076, #14733, #179629, #136092, #167432, #88584, #195799, #13735, #153229, #168408, #29903, #56257, #135114, #121898, #180631, #43090, #73443, #104757, #103768, #165447, #106734, #150282, #11779, #197767, #196790, #58258, #166447, #27943, #75402, #151271, #12761 ),
 ( #59233, #137073, #124891, #30901, #80362, #123871, #92548, #109718, #170400, #81340, #2535, #535, #184577, #32888, #3523, #94538, #15727, #188564, #107713, #110705, #185569, #64216, #140043, #77387, #139055, #62207, #47063, #187582, #108723, #126858, #49050, #50043, #33876, #78369, #17720, #156220, #125882, #16719, #111707, #19698, #173393, #155230, #186590, #61217, #48062, #158208, #63211, #18715, #172385, #122889, #171401, #31891, #93545, #1532, #79378, #141049, #95535, #157222, #142035, #169392, #65199, #154237, #34863, #96518, #199751, #46058, #51031, #8519, #112692, #115700, #70197, #193548, #22693, #130852, #131864, #161197, #24705, #84340, #4501, #100517, #66192, #54027, #35854, #147035, #177389, #144026, #97500, #38860, #113678, #127854, #189559, #5507, #163201, #6501, #192544, #176383, #85342, #174384, #159186, #20681, #178381, #146019, #162196, #55021, #82336, #23694, #67189, #37857, #116691, #143023, #39845, #128846, #190545, #7502, #101511, #83343, #98505, #52019, #175372, #36840, #129833, #69186, #68181, #160200, #191532, #21690, #145020, #53009, #99516, #114688, #165207, #59990, #168168, #120667, #119696, #194547, #57031, #105508, #197533, #121658, #183352, #181379, #132859, #72192, #40856, #44835, #106490, #73208, #149041, #86354, #166203, #133866, #148040, #179393, #151038, #150033, #9529, #42857, #117696, #59001, #41866, #56018, #182365, #27704, #167195, #104522, #71195, #102530, #43843, #118704, #164213, #25710, #28692, #87355, #196555, #89347, #10529, #12528, #74193, #135862, #136836, #103532, #195557, #180395, #90328, #152013, #13499, #26702, #88342, #75164, #198519, #11540, #134879, #58026, #29665, #93298, #108478, #33630, #80123, #95292, #92309, #169151, #32641, #171153, #126616, #17471, #154984, #199511, #48808, #60977, #94295, #14487, #16479, #137828, #187338, #30655, #78129, #18473, #122653, #79127, #170156, #153992, #1286, #61965, #155974, #76149, #141792, #139797, #140800, #77146, #124643, #15489, #156976, #2289, #3286, #63971, #31649, #47820, #186338, #125641, #46818, #64957, #49796, #188318, #185328, #62962, #91297, #109469, #111462, #110462, #172143, #152988, #184341, #45823, #138816, #297, #123632, #107474, #66943, #7257, #51775, #128605, #142784, #177145, #65945, #160954, #115455, #97258, #19459, #81106, #38616, #4265, #145776, #100274, #23449, #52766, #22448, #161953, #191290, #54777, #114435, #34622, #130606, #96281, #84097, #127616, #85096, #68942, #174141, #189316, #192301, #143779, #157967, #50793, #35613, #193302, #36595, #53780, #6261, #146782, #112452, #158946, #20435, #8275, #176136, #69953, #82086, #37605, #5260, #98251, #173147, #131618, #190298, #99268, #113435, #175128, #159953, #21441, #83101, #144777, #67941, #129594, #39606, #165962, #13269, #28458, #90094, #198275, #195310, #182118, #101265, #41624, #133617, #103288, #147802, #197295, #40616, #9287, #26461, #87112, #116451, #119458, #117449, #162955, #149789, #120427, #11293, #132622, #105269, #24461, #27463, #102286, #181142, #56791, #194309, #55776, #179148, #163975, #104280, #25472, #89105, #148798, #43604, #150795, #166956, #12291, #118463, #134634, #72965, #42616, #180155, #151776, #136595, #74932, #71946, #164968, #178140, #88104, #86111, #196319, #135624, #73956, #70952, #57788, #10288, #58758, #184103, #15246, #153751, #94060, #138576, #76905, #29434, #63735, #152752, #47581, #2057, #45585, #106252, #167935, #125410, #91065, #32405, #187107, #110230, #139565, #109233, #48577, #77898, #141565, #1049, #121422, #17236, #183114, #170912, #14242, #171911, #155739, #60739, #75914, #78888, #30415, #44597, #137588, #122413, #79895, #123397, #140567, #93062, #33400, #199271, #107238, #168909, #95058, #62722, #156748, #92063, #124406, #56, #185089, #59752, #18242, #61729, #186099, #46578, #108239, #169919, #31411, #154749, #16246, #52531, #173913, #126392, #114192, #100032, #115212, #176905 ) ),
 .UNSPECIFIED., .T., .F., .T. ) 
 B_SPLINE_SURFACE_WITH_KNOTS ( ( 4, 3, 4 ),
 ( 3, 2, 2, 2, 2, 2, 2, 2, 2, 2, 2, 2, 2, 2, 2, 2, 2, 2, 2, 2, 2, 2, 2, 2, 2, 2, 2, 2, 2, 2, 2, 2, 2, 2, 2, 2, 2, 2, 2, 2, 2, 2, 2, 2, 2, 2, 2, 2, 2, 2, 2, 2, 2, 2, 2, 2, 2, 2, 2, 2, 2, 2, 2, 2, 2, 2, 2, 2, 2, 2, 2, 2, 2, 2, 2, 2, 2, 2, 2, 2, 2, 2, 2, 2, 2, 2, 2, 2, 2, 2, 2, 2, 2, 2, 2, 2, 2, 2, 2, 2, 2, 2, 2, 2, 2, 2, 2, 2, 2, 2, 2, 2, 2, 2, 2, 2, 2, 2, 2, 2, 2, 2, 2, 2, 2, 2, 2, 2, 2, 2, 2, 2, 2, 2, 2, 2, 2, 2, 2, 2, 2, 2, 2, 2, 2, 2, 2, 2, 2, 2, 2, 2, 2, 2, 2, 2, 2, 2, 2, 2, 2, 2, 2, 2, 2, 2, 2, 2, 2, 2, 2, 2, 2, 2, 2, 2, 2, 2, 2, 2, 2, 2, 2, 2, 2, 2, 2, 2, 2, 2, 2, 2, 2, 2, 2, 2, 2, 2, 2, 2, 2, 2, 2, 2, 2, 2, 2, 2, 2, 2, 2, 2, 2, 2, 2, 2, 2, 2, 2, 2, 2, 2, 2, 2, 2, 2, 2, 2, 3 ),
 ( 0.000000000000000000, 0.5000000000000000000, 1.000000000000000000 ),
 ( 0.000000000000000000, 0.004385964912280701511, 0.008771929824561403022, 0.01315789473684210453, 0.01754385964912280604, 0.02192982456140350755, 0.02631578947368420907, 0.03070175438596491058, 0.03508771929824561209, 0.03947368421052631360, 0.04385964912280701511, 0.04824561403508771662, 0.05263157894736841813, 0.05701754385964911964, 0.06140350877192982115, 0.06578947368421052266, 0.07017543859649122417, 0.07456140350877192569, 0.07894736842105262720, 0.08333333333333332871, 0.08771929824561403022, 0.09210526315789473173, 0.09649122807017543324, 0.1008771929824561348, 0.1052631578947368363, 0.1096491228070175378, 0.1140350877192982393, 0.1184210526315789408, 0.1228070175438596423, 0.1271929824561403577, 0.1315789473684210453, 0.1359649122807017607, 0.1403508771929824483, 0.1447368421052631637, 0.1491228070175438514, 0.1535087719298245668, 0.1578947368421052544, 0.1622807017543859698, 0.1666666666666666574, 0.1710526315789473728, 0.1754385964912280604, 0.1798245614035087758, 0.1842105263157894635, 0.1885964912280701788, 0.1929824561403508665, 0.1973684210526315819, 0.2017543859649122695, 0.2061403508771929849, 0.2105263157894736725, 0.2149122807017543879, 0.2192982456140350755, 0.2236842105263157909, 0.2280701754385964786, 0.2324561403508771940, 0.2368421052631578816, 0.2412280701754385970, 0.2456140350877192846, 0.2500000000000000000, 0.2543859649122807154, 0.2587719298245614308, 0.2631578947368420907, 0.2675438596491228060, 0.2719298245614035214, 0.2763157894736842368, 0.2807017543859648967, 0.2850877192982456121, 0.2894736842105263275, 0.2938596491228070429, 0.2982456140350877027, 0.3026315789473684181, 0.3070175438596491335, 0.3114035087719298489, 0.3157894736842105088, 0.3201754385964912242, 0.3245614035087719396, 0.3289473684210526550, 0.3333333333333333148, 0.3377192982456140302, 0.3421052631578947456, 0.3464912280701754610, 0.3508771929824561209, 0.3552631578947368363, 0.3596491228070175517, 0.3640350877192982670, 0.3684210526315789269, 0.3728070175438596423, 0.3771929824561403577, 0.3815789473684210731, 0.3859649122807017330, 0.3903508771929824483, 0.3947368421052631637, 0.3991228070175438791, 0.4035087719298245390, 0.4078947368421052544, 0.4122807017543859698, 0.4166666666666666852, 0.4210526315789473450, 0.4254385964912280604, 0.4298245614035087758, 0.4342105263157894912, 0.4385964912280701511, 0.4429824561403508665, 0.4473684210526315819, 0.4517543859649122973, 0.4561403508771929571, 0.4605263157894736725, 0.4649122807017543879, 0.4692982456140351033, 0.4736842105263157632, 0.4780701754385964786, 0.4824561403508771940, 0.4868421052631579093, 0.4912280701754385692, 0.4956140350877192846, 0.5000000000000000000, 0.5043859649122807154, 0.5087719298245614308, 0.5131578947368421462, 0.5175438596491228616, 0.5219298245614034659, 0.5263157894736841813, 0.5307017543859648967, 0.5350877192982456121, 0.5394736842105263275, 0.5438596491228070429, 0.5482456140350877583, 0.5526315789473684736, 0.5570175438596490780, 0.5614035087719297934, 0.5657894736842105088, 0.5701754385964912242, 0.5745614035087719396, 0.5789473684210526550, 0.5833333333333333703, 0.5877192982456140857, 0.5921052631578946901, 0.5964912280701754055, 0.6008771929824561209, 0.6052631578947368363, 0.6096491228070175517, 0.6140350877192982670, 0.6184210526315789824, 0.6228070175438596978, 0.6271929824561403022, 0.6315789473684210176, 0.6359649122807017330, 0.6403508771929824483, 0.6447368421052631637, 0.6491228070175438791, 0.6535087719298245945, 0.6578947368421053099, 0.6622807017543859143, 0.6666666666666666297, 0.6710526315789473450, 0.6754385964912280604, 0.6798245614035087758, 0.6842105263157894912, 0.6885964912280702066, 0.6929824561403509220, 0.6973684210526315264, 0.7017543859649122417, 0.7061403508771929571, 0.7105263157894736725, 0.7149122807017543879, 0.7192982456140351033, 0.7236842105263158187, 0.7280701754385965341, 0.7324561403508771384, 0.7368421052631578538, 0.7412280701754385692, 0.7456140350877192846, 0.7500000000000000000, 0.7543859649122807154, 0.7587719298245614308, 0.7631578947368421462, 0.7675438596491228616, 0.7719298245614034659, 0.7763157894736841813, 0.7807017543859648967, 0.7850877192982456121, 0.7894736842105263275, 0.7938596491228070429, 0.7982456140350877583, 0.8026315789473684736, 0.8070175438596490780, 0.8114035087719297934, 0.8157894736842105088, 0.8201754385964912242, 0.8245614035087719396, 0.8289473684210526550, 0.8333333333333333703, 0.8377192982456140857, 0.8421052631578946901, 0.8464912280701754055, 0.8508771929824561209, 0.8552631578947368363, 0.8596491228070175517, 0.8640350877192982670, 0.8684210526315789824, 0.8728070175438596978, 0.8771929824561403022, 0.8815789473684210176, 0.8859649122807017330, 0.8903508771929824483, 0.8947368421052631637, 0.8991228070175438791, 0.9035087719298245945, 0.9078947368421053099, 0.9122807017543859143, 0.9166666666666666297, 0.9210526315789473450, 0.9254385964912280604, 0.9298245614035087758, 0.9342105263157894912, 0.9385964912280702066, 0.9429824561403509220, 0.9473684210526315264, 0.9517543859649122417, 0.9561403508771929571, 0.9605263157894736725, 0.9649122807017543879, 0.9692982456140351033, 0.9736842105263158187, 0.9780701754385965341, 0.9824561403508771384, 0.9868421052631578538, 0.9912280701754385692, 0.9956140350877192846, 1.000000000000000000 ),
 .UNSPECIFIED. ) 
 GEOMETRIC_REPRESENTATION_ITEM ( )  RATIONAL_B_SPLINE_SURFACE ( (
 ( 1.000000000000000000, 0.9659258262890683122, 1.000000000000000000, 0.9659258262890683122, 1.000000000000000000, 0.9659258262890683122, 1.000000000000000000, 0.9659258262890683122, 1.000000000000000000, 0.9659258262890683122, 1.000000000000000000, 0.9659258262890683122, 1.000000000000000000, 0.9659258262890683122, 1.000000000000000000, 0.9659258262890683122, 1.000000000000000000, 0.9659258262890683122, 1.000000000000000000, 0.9659258262890683122, 1.000000000000000000, 0.9659258262890683122, 1.000000000000000000, 0.9659258262890683122, 1.000000000000000000, 0.9659258262890683122, 1.000000000000000000, 0.9659258262890683122, 1.000000000000000000, 0.9659258262890683122, 1.000000000000000000, 0.9659258262890683122, 1.000000000000000000, 0.9659258262890683122, 1.000000000000000000, 0.9659258262890683122, 1.000000000000000000, 0.9659258262890683122, 1.000000000000000000, 0.9659258262890683122, 1.000000000000000000, 0.9659258262890683122, 1.000000000000000000, 0.9659258262890683122, 1.000000000000000000, 0.9659258262890683122, 1.000000000000000000, 0.9659258262890683122, 1.000000000000000000, 0.9659258262890683122, 1.000000000000000000, 0.9659258262890683122, 1.000000000000000000, 0.9659258262890683122, 1.000000000000000000, 0.9659258262890683122, 1.000000000000000000, 0.9659258262890683122, 1.000000000000000000, 0.9659258262890683122, 1.000000000000000000, 0.9659258262890683122, 1.000000000000000000, 0.9659258262890683122, 1.000000000000000000, 0.9659258262890683122, 1.000000000000000000, 0.9659258262890683122, 1.000000000000000000, 0.9659258262890683122, 1.000000000000000000, 0.9659258262890683122, 1.000000000000000000, 0.9659258262890683122, 1.000000000000000000, 0.9659258262890683122, 1.000000000000000000, 0.9659258262890683122, 1.000000000000000000, 0.9659258262890683122, 1.000000000000000000, 0.9659258262890683122, 1.000000000000000000, 0.9659258262890683122, 1.000000000000000000, 0.9659258262890683122, 1.000000000000000000, 0.9659258262890683122, 1.000000000000000000, 0.9659258262890683122, 1.000000000000000000, 0.9659258262890683122, 1.000000000000000000, 0.9659258262890683122, 1.000000000000000000, 0.9659258262890683122, 1.000000000000000000, 0.9659258262890683122, 1.000000000000000000, 0.9659258262890683122, 1.000000000000000000, 0.9659258262890683122, 1.000000000000000000, 0.9659258262890683122, 1.000000000000000000, 0.9659258262890683122, 1.000000000000000000, 0.9659258262890683122, 1.000000000000000000, 0.9659258262890683122, 1.000000000000000000, 0.9659258262890683122, 1.000000000000000000, 0.9659258262890683122, 1.000000000000000000, 0.9659258262890683122, 1.000000000000000000, 0.9659258262890683122, 1.000000000000000000, 0.9659258262890683122, 1.000000000000000000, 0.9659258262890683122, 1.000000000000000000, 0.9659258262890683122, 1.000000000000000000, 0.9659258262890683122, 1.000000000000000000, 0.9659258262890683122, 1.000000000000000000, 0.9659258262890683122, 1.000000000000000000, 0.9659258262890683122, 1.000000000000000000, 0.9659258262890683122, 1.000000000000000000, 0.9659258262890683122, 1.000000000000000000, 0.9659258262890683122, 1.000000000000000000, 0.9659258262890683122, 1.000000000000000000, 0.9659258262890683122, 1.000000000000000000, 0.9659258262890683122, 1.000000000000000000, 0.9659258262890683122, 1.000000000000000000, 0.9659258262890683122, 1.000000000000000000, 0.9659258262890683122, 1.000000000000000000, 0.9659258262890683122, 1.000000000000000000, 0.9659258262890683122, 1.000000000000000000, 0.9659258262890683122, 1.000000000000000000, 0.9659258262890683122, 1.000000000000000000, 0.9659258262890683122, 1.000000000000000000, 0.9659258262890683122, 1.000000000000000000, 0.9659258262890683122, 1.000000000000000000, 0.9659258262890683122, 1.000000000000000000, 0.9659258262890683122, 1.000000000000000000, 0.9659258262890683122, 1.000000000000000000, 0.9659258262890683122, 1.000000000000000000, 0.9659258262890683122, 1.000000000000000000, 0.9659258262890683122, 1.000000000000000000, 0.9659258262890683122, 1.000000000000000000, 0.9659258262890683122, 1.000000000000000000, 0.9659258262890683122, 1.000000000000000000, 0.9659258262890683122, 1.000000000000000000, 0.9659258262890683122, 1.000000000000000000, 0.9659258262890683122, 1.000000000000000000, 0.9659258262890683122, 1.000000000000000000, 0.9659258262890683122, 1.000000000000000000, 0.9659258262890683122, 1.000000000000000000, 0.9659258262890683122, 1.000000000000000000, 0.9659258262890683122, 1.000000000000000000, 0.9659258262890683122, 1.000000000000000000, 0.9659258262890683122, 1.000000000000000000, 0.9659258262890683122, 1.000000000000000000, 0.9659258262890683122, 1.000000000000000000, 0.9659258262890683122, 1.000000000000000000, 0.9659258262890683122, 1.000000000000000000, 0.9659258262890683122, 1.000000000000000000, 0.9659258262890683122, 1.000000000000000000, 0.9659258262890683122, 1.000000000000000000, 0.9659258262890683122, 1.000000000000000000, 0.9659258262890683122, 1.000000000000000000, 0.9659258262890683122, 1.000000000000000000, 0.9659258262890683122, 1.000000000000000000, 0.9659258262890683122, 1.000000000000000000, 0.9659258262890683122, 1.000000000000000000, 0.9659258262890683122, 1.000000000000000000, 0.9659258262890683122, 1.000000000000000000, 0.9659258262890683122, 1.000000000000000000, 0.9659258262890683122, 1.000000000000000000, 0.9659258262890683122, 1.000000000000000000, 0.9659258262890683122, 1.000000000000000000, 0.9659258262890683122, 1.000000000000000000, 0.9659258262890683122, 1.000000000000000000, 0.9659258262890683122, 1.000000000000000000, 0.9659258262890683122, 1.000000000000000000, 0.9659258262890683122, 1.000000000000000000, 0.9659258262890683122, 1.000000000000000000, 0.9659258262890683122, 1.000000000000000000, 0.9659258262890683122, 1.000000000000000000, 0.9659258262890683122, 1.000000000000000000, 0.9659258262890683122, 1.000000000000000000, 0.9659258262890683122, 1.000000000000000000, 0.9659258262890683122, 1.000000000000000000, 0.9659258262890683122, 1.000000000000000000, 0.9659258262890683122, 1.000000000000000000, 0.9659258262890683122, 1.000000000000000000, 0.9659258262890683122, 1.000000000000000000, 0.9659258262890683122, 1.000000000000000000, 0.9659258262890683122, 1.000000000000000000, 0.9659258262890683122, 1.000000000000000000, 0.9659258262890683122, 1.000000000000000000, 0.9659258262890683122, 1.000000000000000000, 0.9659258262890683122, 1.000000000000000000, 0.9659258262890683122, 1.000000000000000000, 0.9659258262890683122, 1.000000000000000000, 0.9659258262890683122, 1.000000000000000000, 0.9659258262890683122, 1.000000000000000000, 0.9659258262890683122, 1.000000000000000000, 0.9659258262890683122, 1.000000000000000000, 0.9659258262890683122, 1.000000000000000000, 0.9659258262890683122, 1.000000000000000000, 0.9659258262890683122, 1.000000000000000000, 0.9659258262890683122, 1.000000000000000000, 0.9659258262890683122, 1.000000000000000000, 0.9659258262890683122, 1.000000000000000000, 0.9659258262890683122, 1.000000000000000000, 0.9659258262890683122, 1.000000000000000000, 0.9659258262890683122, 1.000000000000000000, 0.9659258262890683122, 1.000000000000000000, 0.9659258262890683122, 1.000000000000000000, 0.9659258262890683122, 1.000000000000000000, 0.9659258262890683122, 1.000000000000000000, 0.9659258262890683122, 1.000000000000000000, 0.9659258262890683122, 1.000000000000000000, 0.9659258262890683122, 1.000000000000000000, 0.9659258262890683122, 1.000000000000000000, 0.9659258262890683122, 1.000000000000000000, 0.9659258262890683122, 1.000000000000000000, 0.9659258262890683122, 1.000000000000000000, 0.9659258262890683122, 1.000000000000000000, 0.9659258262890683122, 1.000000000000000000, 0.9659258262890683122, 1.000000000000000000, 0.9659258262890683122, 1.000000000000000000, 0.9659258262890683122, 1.000000000000000000, 0.9659258262890683122, 1.000000000000000000, 0.9659258262890683122, 1.000000000000000000, 0.9659258262890683122, 1.000000000000000000, 0.9659258262890683122, 1.000000000000000000, 0.9659258262890683122, 1.000000000000000000, 0.9659258262890683122, 1.000000000000000000, 0.9659258262890683122, 1.000000000000000000, 0.9659258262890683122, 1.000000000000000000, 0.9659258262890683122, 1.000000000000000000, 0.9659258262890683122, 1.000000000000000000, 0.9659258262890683122, 1.000000000000000000, 0.9659258262890683122, 1.000000000000000000, 0.9659258262890683122, 1.000000000000000000, 0.9659258262890683122, 1.000000000000000000, 0.9659258262890683122, 1.000000000000000000, 0.9659258262890683122, 1.000000000000000000, 0.9659258262890683122, 1.000000000000000000, 0.9659258262890683122, 1.000000000000000000, 0.9659258262890683122, 1.000000000000000000, 0.9659258262890683122, 1.000000000000000000, 0.9659258262890683122, 1.000000000000000000, 0.9659258262890683122, 1.000000000000000000, 0.9659258262890683122, 1.000000000000000000, 0.9659258262890683122, 1.000000000000000000, 0.9659258262890683122, 1.000000000000000000, 0.9659258262890683122, 1.000000000000000000, 0.9659258262890683122, 1.000000000000000000, 0.9659258262890683122, 1.000000000000000000, 0.9659258262890683122, 1.000000000000000000, 0.9659258262890683122, 1.000000000000000000, 0.9659258262890683122, 1.000000000000000000, 0.9659258262890683122, 1.000000000000000000, 0.9659258262890683122, 1.000000000000000000, 0.9659258262890683122, 1.000000000000000000, 0.9659258262890683122, 1.000000000000000000, 0.9659258262890683122, 1.000000000000000000, 0.9659258262890683122, 1.000000000000000000, 0.9659258262890683122, 1.000000000000000000, 0.9659258262890683122, 1.000000000000000000, 0.9659258262890683122, 1.000000000000000000, 0.9659258262890683122, 1.000000000000000000, 0.9659258262890683122, 1.000000000000000000, 0.9659258262890683122, 1.000000000000000000, 0.9659258262890683122, 1.000000000000000000, 0.9659258262890683122, 1.000000000000000000, 0.9659258262890683122, 1.000000000000000000, 0.9659258262890683122, 1.000000000000000000, 0.9659258262890683122, 1.000000000000000000, 0.9659258262890683122, 1.000000000000000000, 0.9659258262890683122, 1.000000000000000000, 0.9659258262890683122, 1.000000000000000000, 0.9659258262890683122, 1.000000000000000000, 0.9659258262890683122, 1.000000000000000000, 0.9659258262890683122, 1.000000000000000000, 0.9659258262890683122, 1.000000000000000000),
 ( 0.3333333333333333703, 0.3219752754296894559, 0.3333333333333333703, 0.3219752754296894559, 0.3333333333333333703, 0.3219752754296894559, 0.3333333333333333703, 0.3219752754296894559, 0.3333333333333333703, 0.3219752754296894559, 0.3333333333333333703, 0.3219752754296894559, 0.3333333333333333703, 0.3219752754296894559, 0.3333333333333333703, 0.3219752754296894559, 0.3333333333333333703, 0.3219752754296894559, 0.3333333333333333703, 0.3219752754296894559, 0.3333333333333333703, 0.3219752754296894559, 0.3333333333333333703, 0.3219752754296894559, 0.3333333333333333703, 0.3219752754296894559, 0.3333333333333333703, 0.3219752754296894559, 0.3333333333333333703, 0.3219752754296894559, 0.3333333333333333703, 0.3219752754296894559, 0.3333333333333333703, 0.3219752754296894559, 0.3333333333333333703, 0.3219752754296894559, 0.3333333333333333703, 0.3219752754296894559, 0.3333333333333333703, 0.3219752754296894559, 0.3333333333333333703, 0.3219752754296894559, 0.3333333333333333703, 0.3219752754296894559, 0.3333333333333333703, 0.3219752754296894559, 0.3333333333333333703, 0.3219752754296894559, 0.3333333333333333703, 0.3219752754296894559, 0.3333333333333333703, 0.3219752754296894559, 0.3333333333333333703, 0.3219752754296894559, 0.3333333333333333703, 0.3219752754296894559, 0.3333333333333333703, 0.3219752754296894559, 0.3333333333333333703, 0.3219752754296894559, 0.3333333333333333703, 0.3219752754296894559, 0.3333333333333333703, 0.3219752754296894559, 0.3333333333333333703, 0.3219752754296894559, 0.3333333333333333703, 0.3219752754296894559, 0.3333333333333333703, 0.3219752754296894559, 0.3333333333333333703, 0.3219752754296894559, 0.3333333333333333703, 0.3219752754296894559, 0.3333333333333333703, 0.3219752754296894559, 0.3333333333333333703, 0.3219752754296894559, 0.3333333333333333703, 0.3219752754296894559, 0.3333333333333333703, 0.3219752754296894559, 0.3333333333333333703, 0.3219752754296894559, 0.3333333333333333703, 0.3219752754296894559, 0.3333333333333333703, 0.3219752754296894559, 0.3333333333333333703, 0.3219752754296894559, 0.3333333333333333703, 0.3219752754296894559, 0.3333333333333333703, 0.3219752754296894559, 0.3333333333333333703, 0.3219752754296894559, 0.3333333333333333703, 0.3219752754296894559, 0.3333333333333333703, 0.3219752754296894559, 0.3333333333333333703, 0.3219752754296894559, 0.3333333333333333703, 0.3219752754296894559, 0.3333333333333333703, 0.3219752754296894559, 0.3333333333333333703, 0.3219752754296894559, 0.3333333333333333703, 0.3219752754296894559, 0.3333333333333333703, 0.3219752754296894559, 0.3333333333333333703, 0.3219752754296894559, 0.3333333333333333703, 0.3219752754296894559, 0.3333333333333333703, 0.3219752754296894559, 0.3333333333333333703, 0.3219752754296894559, 0.3333333333333333703, 0.3219752754296894559, 0.3333333333333333703, 0.3219752754296894559, 0.3333333333333333703, 0.3219752754296894559, 0.3333333333333333703, 0.3219752754296894559, 0.3333333333333333703, 0.3219752754296894559, 0.3333333333333333703, 0.3219752754296894559, 0.3333333333333333703, 0.3219752754296894559, 0.3333333333333333703, 0.3219752754296894559, 0.3333333333333333703, 0.3219752754296894559, 0.3333333333333333703, 0.3219752754296894559, 0.3333333333333333703, 0.3219752754296894559, 0.3333333333333333703, 0.3219752754296894559, 0.3333333333333333703, 0.3219752754296894559, 0.3333333333333333703, 0.3219752754296894559, 0.3333333333333333703, 0.3219752754296894559, 0.3333333333333333703, 0.3219752754296894559, 0.3333333333333333703, 0.3219752754296894559, 0.3333333333333333703, 0.3219752754296894559, 0.3333333333333333703, 0.3219752754296894559, 0.3333333333333333703, 0.3219752754296894559, 0.3333333333333333703, 0.3219752754296894559, 0.3333333333333333703, 0.3219752754296894559, 0.3333333333333333703, 0.3219752754296894559, 0.3333333333333333703, 0.3219752754296894559, 0.3333333333333333703, 0.3219752754296894559, 0.3333333333333333703, 0.3219752754296894559, 0.3333333333333333703, 0.3219752754296894559, 0.3333333333333333703, 0.3219752754296894559, 0.3333333333333333703, 0.3219752754296894559, 0.3333333333333333703, 0.3219752754296894559, 0.3333333333333333703, 0.3219752754296894559, 0.3333333333333333703, 0.3219752754296894559, 0.3333333333333333703, 0.3219752754296894559, 0.3333333333333333703, 0.3219752754296894559, 0.3333333333333333703, 0.3219752754296894559, 0.3333333333333333703, 0.3219752754296894559, 0.3333333333333333703, 0.3219752754296894559, 0.3333333333333333703, 0.3219752754296894559, 0.3333333333333333703, 0.3219752754296894559, 0.3333333333333333703, 0.3219752754296894559, 0.3333333333333333703, 0.3219752754296894559, 0.3333333333333333703, 0.3219752754296894559, 0.3333333333333333703, 0.3219752754296894559, 0.3333333333333333703, 0.3219752754296894559, 0.3333333333333333703, 0.3219752754296894559, 0.3333333333333333703, 0.3219752754296894559, 0.3333333333333333703, 0.3219752754296894559, 0.3333333333333333703, 0.3219752754296894559, 0.3333333333333333703, 0.3219752754296894559, 0.3333333333333333703, 0.3219752754296894559, 0.3333333333333333703, 0.3219752754296894559, 0.3333333333333333703, 0.3219752754296894559, 0.3333333333333333703, 0.3219752754296894559, 0.3333333333333333703, 0.3219752754296894559, 0.3333333333333333703, 0.3219752754296894559, 0.3333333333333333703, 0.3219752754296894559, 0.3333333333333333703, 0.3219752754296894559, 0.3333333333333333703, 0.3219752754296894559, 0.3333333333333333703, 0.3219752754296894559, 0.3333333333333333703, 0.3219752754296894559, 0.3333333333333333703, 0.3219752754296894559, 0.3333333333333333703, 0.3219752754296894559, 0.3333333333333333703, 0.3219752754296894559, 0.3333333333333333703, 0.3219752754296894559, 0.3333333333333333703, 0.3219752754296894559, 0.3333333333333333703, 0.3219752754296894559, 0.3333333333333333703, 0.3219752754296894559, 0.3333333333333333703, 0.3219752754296894559, 0.3333333333333333703, 0.3219752754296894559, 0.3333333333333333703, 0.3219752754296894559, 0.3333333333333333703, 0.3219752754296894559, 0.3333333333333333703, 0.3219752754296894559, 0.3333333333333333703, 0.3219752754296894559, 0.3333333333333333703, 0.3219752754296894559, 0.3333333333333333703, 0.3219752754296894559, 0.3333333333333333703, 0.3219752754296894559, 0.3333333333333333703, 0.3219752754296894559, 0.3333333333333333703, 0.3219752754296894559, 0.3333333333333333703, 0.3219752754296894559, 0.3333333333333333703, 0.3219752754296894559, 0.3333333333333333703, 0.3219752754296894559, 0.3333333333333333703, 0.3219752754296894559, 0.3333333333333333703, 0.3219752754296894559, 0.3333333333333333703, 0.3219752754296894559, 0.3333333333333333703, 0.3219752754296894559, 0.3333333333333333703, 0.3219752754296894559, 0.3333333333333333703, 0.3219752754296894559, 0.3333333333333333703, 0.3219752754296894559, 0.3333333333333333703, 0.3219752754296894559, 0.3333333333333333703, 0.3219752754296894559, 0.3333333333333333703, 0.3219752754296894559, 0.3333333333333333703, 0.3219752754296894559, 0.3333333333333333703, 0.3219752754296894559, 0.3333333333333333703, 0.3219752754296894559, 0.3333333333333333703, 0.3219752754296894559, 0.3333333333333333703, 0.3219752754296894559, 0.3333333333333333703, 0.3219752754296894559, 0.3333333333333333703, 0.3219752754296894559, 0.3333333333333333703, 0.3219752754296894559, 0.3333333333333333703, 0.3219752754296894559, 0.3333333333333333703, 0.3219752754296894559, 0.3333333333333333703, 0.3219752754296894559, 0.3333333333333333703, 0.3219752754296894559, 0.3333333333333333703, 0.3219752754296894559, 0.3333333333333333703, 0.3219752754296894559, 0.3333333333333333703, 0.3219752754296894559, 0.3333333333333333703, 0.3219752754296894559, 0.3333333333333333703, 0.3219752754296894559, 0.3333333333333333703, 0.3219752754296894559, 0.3333333333333333703, 0.3219752754296894559, 0.3333333333333333703, 0.3219752754296894559, 0.3333333333333333703, 0.3219752754296894559, 0.3333333333333333703, 0.3219752754296894559, 0.3333333333333333703, 0.3219752754296894559, 0.3333333333333333703, 0.3219752754296894559, 0.3333333333333333703, 0.3219752754296894559, 0.3333333333333333703, 0.3219752754296894559, 0.3333333333333333703, 0.3219752754296894559, 0.3333333333333333703, 0.3219752754296894559, 0.3333333333333333703, 0.3219752754296894559, 0.3333333333333333703, 0.3219752754296894559, 0.3333333333333333703, 0.3219752754296894559, 0.3333333333333333703, 0.3219752754296894559, 0.3333333333333333703, 0.3219752754296894559, 0.3333333333333333703, 0.3219752754296894559, 0.3333333333333333703, 0.3219752754296894559, 0.3333333333333333703, 0.3219752754296894559, 0.3333333333333333703, 0.3219752754296894559, 0.3333333333333333703, 0.3219752754296894559, 0.3333333333333333703, 0.3219752754296894559, 0.3333333333333333703, 0.3219752754296894559, 0.3333333333333333703, 0.3219752754296894559, 0.3333333333333333703, 0.3219752754296894559, 0.3333333333333333703, 0.3219752754296894559, 0.3333333333333333703, 0.3219752754296894559, 0.3333333333333333703, 0.3219752754296894559, 0.3333333333333333703, 0.3219752754296894559, 0.3333333333333333703, 0.3219752754296894559, 0.3333333333333333703, 0.3219752754296894559, 0.3333333333333333703, 0.3219752754296894559, 0.3333333333333333703, 0.3219752754296894559, 0.3333333333333333703, 0.3219752754296894559, 0.3333333333333333703, 0.3219752754296894559, 0.3333333333333333703, 0.3219752754296894559, 0.3333333333333333703, 0.3219752754296894559, 0.3333333333333333703, 0.3219752754296894559, 0.3333333333333333703, 0.3219752754296894559, 0.3333333333333333703, 0.3219752754296894559, 0.3333333333333333703, 0.3219752754296894559, 0.3333333333333333703, 0.3219752754296894559, 0.3333333333333333703, 0.3219752754296894559, 0.3333333333333333703, 0.3219752754296894559, 0.3333333333333333703, 0.3219752754296894559, 0.3333333333333333703, 0.3219752754296894559, 0.3333333333333333703, 0.3219752754296894559, 0.3333333333333333703, 0.3219752754296894559, 0.3333333333333333703, 0.3219752754296894559, 0.3333333333333333703, 0.3219752754296894559, 0.3333333333333333703, 0.3219752754296894559, 0.3333333333333333703, 0.3219752754296894559, 0.3333333333333333703, 0.3219752754296894559, 0.3333333333333333703, 0.3219752754296894559, 0.3333333333333333703, 0.3219752754296894559, 0.3333333333333333703, 0.3219752754296894559, 0.3333333333333333703, 0.3219752754296894559, 0.3333333333333333703, 0.3219752754296894559, 0.3333333333333333703, 0.3219752754296894559, 0.3333333333333333703, 0.3219752754296894559, 0.3333333333333333703),
 ( 0.3333333333333333703, 0.3219752754296894559, 0.3333333333333333703, 0.3219752754296894559, 0.3333333333333333703, 0.3219752754296894559, 0.3333333333333333703, 0.3219752754296894559, 0.3333333333333333703, 0.3219752754296894559, 0.3333333333333333703, 0.3219752754296894559, 0.3333333333333333703, 0.3219752754296894559, 0.3333333333333333703, 0.3219752754296894559, 0.3333333333333333703, 0.3219752754296894559, 0.3333333333333333703, 0.3219752754296894559, 0.3333333333333333703, 0.3219752754296894559, 0.3333333333333333703, 0.3219752754296894559, 0.3333333333333333703, 0.3219752754296894559, 0.3333333333333333703, 0.3219752754296894559, 0.3333333333333333703, 0.3219752754296894559, 0.3333333333333333703, 0.3219752754296894559, 0.3333333333333333703, 0.3219752754296894559, 0.3333333333333333703, 0.3219752754296894559, 0.3333333333333333703, 0.3219752754296894559, 0.3333333333333333703, 0.3219752754296894559, 0.3333333333333333703, 0.3219752754296894559, 0.3333333333333333703, 0.3219752754296894559, 0.3333333333333333703, 0.3219752754296894559, 0.3333333333333333703, 0.3219752754296894559, 0.3333333333333333703, 0.3219752754296894559, 0.3333333333333333703, 0.3219752754296894559, 0.3333333333333333703, 0.3219752754296894559, 0.3333333333333333703, 0.3219752754296894559, 0.3333333333333333703, 0.3219752754296894559, 0.3333333333333333703, 0.3219752754296894559, 0.3333333333333333703, 0.3219752754296894559, 0.3333333333333333703, 0.3219752754296894559, 0.3333333333333333703, 0.3219752754296894559, 0.3333333333333333703, 0.3219752754296894559, 0.3333333333333333703, 0.3219752754296894559, 0.3333333333333333703, 0.3219752754296894559, 0.3333333333333333703, 0.3219752754296894559, 0.3333333333333333703, 0.3219752754296894559, 0.3333333333333333703, 0.3219752754296894559, 0.3333333333333333703, 0.3219752754296894559, 0.3333333333333333703, 0.3219752754296894559, 0.3333333333333333703, 0.3219752754296894559, 0.3333333333333333703, 0.3219752754296894559, 0.3333333333333333703, 0.3219752754296894559, 0.3333333333333333703, 0.3219752754296894559, 0.3333333333333333703, 0.3219752754296894559, 0.3333333333333333703, 0.3219752754296894559, 0.3333333333333333703, 0.3219752754296894559, 0.3333333333333333703, 0.3219752754296894559, 0.3333333333333333703, 0.3219752754296894559, 0.3333333333333333703, 0.3219752754296894559, 0.3333333333333333703, 0.3219752754296894559, 0.3333333333333333703, 0.3219752754296894559, 0.3333333333333333703, 0.3219752754296894559, 0.3333333333333333703, 0.3219752754296894559, 0.3333333333333333703, 0.3219752754296894559, 0.3333333333333333703, 0.3219752754296894559, 0.3333333333333333703, 0.3219752754296894559, 0.3333333333333333703, 0.3219752754296894559, 0.3333333333333333703, 0.3219752754296894559, 0.3333333333333333703, 0.3219752754296894559, 0.3333333333333333703, 0.3219752754296894559, 0.3333333333333333703, 0.3219752754296894559, 0.3333333333333333703, 0.3219752754296894559, 0.3333333333333333703, 0.3219752754296894559, 0.3333333333333333703, 0.3219752754296894559, 0.3333333333333333703, 0.3219752754296894559, 0.3333333333333333703, 0.3219752754296894559, 0.3333333333333333703, 0.3219752754296894559, 0.3333333333333333703, 0.3219752754296894559, 0.3333333333333333703, 0.3219752754296894559, 0.3333333333333333703, 0.3219752754296894559, 0.3333333333333333703, 0.3219752754296894559, 0.3333333333333333703, 0.3219752754296894559, 0.3333333333333333703, 0.3219752754296894559, 0.3333333333333333703, 0.3219752754296894559, 0.3333333333333333703, 0.3219752754296894559, 0.3333333333333333703, 0.3219752754296894559, 0.3333333333333333703, 0.3219752754296894559, 0.3333333333333333703, 0.3219752754296894559, 0.3333333333333333703, 0.3219752754296894559, 0.3333333333333333703, 0.3219752754296894559, 0.3333333333333333703, 0.3219752754296894559, 0.3333333333333333703, 0.3219752754296894559, 0.3333333333333333703, 0.3219752754296894559, 0.3333333333333333703, 0.3219752754296894559, 0.3333333333333333703, 0.3219752754296894559, 0.3333333333333333703, 0.3219752754296894559, 0.3333333333333333703, 0.3219752754296894559, 0.3333333333333333703, 0.3219752754296894559, 0.3333333333333333703, 0.3219752754296894559, 0.3333333333333333703, 0.3219752754296894559, 0.3333333333333333703, 0.3219752754296894559, 0.3333333333333333703, 0.3219752754296894559, 0.3333333333333333703, 0.3219752754296894559, 0.3333333333333333703, 0.3219752754296894559, 0.3333333333333333703, 0.3219752754296894559, 0.3333333333333333703, 0.3219752754296894559, 0.3333333333333333703, 0.3219752754296894559, 0.3333333333333333703, 0.3219752754296894559, 0.3333333333333333703, 0.3219752754296894559, 0.3333333333333333703, 0.3219752754296894559, 0.3333333333333333703, 0.3219752754296894559, 0.3333333333333333703, 0.3219752754296894559, 0.3333333333333333703, 0.3219752754296894559, 0.3333333333333333703, 0.3219752754296894559, 0.3333333333333333703, 0.3219752754296894559, 0.3333333333333333703, 0.3219752754296894559, 0.3333333333333333703, 0.3219752754296894559, 0.3333333333333333703, 0.3219752754296894559, 0.3333333333333333703, 0.3219752754296894559, 0.3333333333333333703, 0.3219752754296894559, 0.3333333333333333703, 0.3219752754296894559, 0.3333333333333333703, 0.3219752754296894559, 0.3333333333333333703, 0.3219752754296894559, 0.3333333333333333703, 0.3219752754296894559, 0.3333333333333333703, 0.3219752754296894559, 0.3333333333333333703, 0.3219752754296894559, 0.3333333333333333703, 0.3219752754296894559, 0.3333333333333333703, 0.3219752754296894559, 0.3333333333333333703, 0.3219752754296894559, 0.3333333333333333703, 0.3219752754296894559, 0.3333333333333333703, 0.3219752754296894559, 0.3333333333333333703, 0.3219752754296894559, 0.3333333333333333703, 0.3219752754296894559, 0.3333333333333333703, 0.3219752754296894559, 0.3333333333333333703, 0.3219752754296894559, 0.3333333333333333703, 0.3219752754296894559, 0.3333333333333333703, 0.3219752754296894559, 0.3333333333333333703, 0.3219752754296894559, 0.3333333333333333703, 0.3219752754296894559, 0.3333333333333333703, 0.3219752754296894559, 0.3333333333333333703, 0.3219752754296894559, 0.3333333333333333703, 0.3219752754296894559, 0.3333333333333333703, 0.3219752754296894559, 0.3333333333333333703, 0.3219752754296894559, 0.3333333333333333703, 0.3219752754296894559, 0.3333333333333333703, 0.3219752754296894559, 0.3333333333333333703, 0.3219752754296894559, 0.3333333333333333703, 0.3219752754296894559, 0.3333333333333333703, 0.3219752754296894559, 0.3333333333333333703, 0.3219752754296894559, 0.3333333333333333703, 0.3219752754296894559, 0.3333333333333333703, 0.3219752754296894559, 0.3333333333333333703, 0.3219752754296894559, 0.3333333333333333703, 0.3219752754296894559, 0.3333333333333333703, 0.3219752754296894559, 0.3333333333333333703, 0.3219752754296894559, 0.3333333333333333703, 0.3219752754296894559, 0.3333333333333333703, 0.3219752754296894559, 0.3333333333333333703, 0.3219752754296894559, 0.3333333333333333703, 0.3219752754296894559, 0.3333333333333333703, 0.3219752754296894559, 0.3333333333333333703, 0.3219752754296894559, 0.3333333333333333703, 0.3219752754296894559, 0.3333333333333333703, 0.3219752754296894559, 0.3333333333333333703, 0.3219752754296894559, 0.3333333333333333703, 0.3219752754296894559, 0.3333333333333333703, 0.3219752754296894559, 0.3333333333333333703, 0.3219752754296894559, 0.3333333333333333703, 0.3219752754296894559, 0.3333333333333333703, 0.3219752754296894559, 0.3333333333333333703, 0.3219752754296894559, 0.3333333333333333703, 0.3219752754296894559, 0.3333333333333333703, 0.3219752754296894559, 0.3333333333333333703, 0.3219752754296894559, 0.3333333333333333703, 0.3219752754296894559, 0.3333333333333333703, 0.3219752754296894559, 0.3333333333333333703, 0.3219752754296894559, 0.3333333333333333703, 0.3219752754296894559, 0.3333333333333333703, 0.3219752754296894559, 0.3333333333333333703, 0.3219752754296894559, 0.3333333333333333703, 0.3219752754296894559, 0.3333333333333333703, 0.3219752754296894559, 0.3333333333333333703, 0.3219752754296894559, 0.3333333333333333703, 0.3219752754296894559, 0.3333333333333333703, 0.3219752754296894559, 0.3333333333333333703, 0.3219752754296894559, 0.3333333333333333703, 0.3219752754296894559, 0.3333333333333333703, 0.3219752754296894559, 0.3333333333333333703, 0.3219752754296894559, 0.3333333333333333703, 0.3219752754296894559, 0.3333333333333333703, 0.3219752754296894559, 0.3333333333333333703, 0.3219752754296894559, 0.3333333333333333703, 0.3219752754296894559, 0.3333333333333333703, 0.3219752754296894559, 0.3333333333333333703, 0.3219752754296894559, 0.3333333333333333703, 0.3219752754296894559, 0.3333333333333333703, 0.3219752754296894559, 0.3333333333333333703, 0.3219752754296894559, 0.3333333333333333703, 0.3219752754296894559, 0.3333333333333333703, 0.3219752754296894559, 0.3333333333333333703, 0.3219752754296894559, 0.3333333333333333703, 0.3219752754296894559, 0.3333333333333333703, 0.3219752754296894559, 0.3333333333333333703, 0.3219752754296894559, 0.3333333333333333703, 0.3219752754296894559, 0.3333333333333333703, 0.3219752754296894559, 0.3333333333333333703, 0.3219752754296894559, 0.3333333333333333703, 0.3219752754296894559, 0.3333333333333333703, 0.3219752754296894559, 0.3333333333333333703, 0.3219752754296894559, 0.3333333333333333703, 0.3219752754296894559, 0.3333333333333333703, 0.3219752754296894559, 0.3333333333333333703, 0.3219752754296894559, 0.3333333333333333703, 0.3219752754296894559, 0.3333333333333333703, 0.3219752754296894559, 0.3333333333333333703, 0.3219752754296894559, 0.3333333333333333703, 0.3219752754296894559, 0.3333333333333333703, 0.3219752754296894559, 0.3333333333333333703, 0.3219752754296894559, 0.3333333333333333703, 0.3219752754296894559, 0.3333333333333333703, 0.3219752754296894559, 0.3333333333333333703, 0.3219752754296894559, 0.3333333333333333703, 0.3219752754296894559, 0.3333333333333333703, 0.3219752754296894559, 0.3333333333333333703, 0.3219752754296894559, 0.3333333333333333703, 0.3219752754296894559, 0.3333333333333333703, 0.3219752754296894559, 0.3333333333333333703, 0.3219752754296894559, 0.3333333333333333703, 0.3219752754296894559, 0.3333333333333333703, 0.3219752754296894559, 0.3333333333333333703, 0.3219752754296894559, 0.3333333333333333703, 0.3219752754296894559, 0.3333333333333333703, 0.3219752754296894559, 0.3333333333333333703, 0.3219752754296894559, 0.3333333333333333703, 0.3219752754296894559, 0.3333333333333333703, 0.3219752754296894559, 0.3333333333333333703),
 ( 1.000000000000000000, 0.9659258262890683122, 1.000000000000000000, 0.9659258262890683122, 1.000000000000000000, 0.9659258262890683122, 1.000000000000000000, 0.9659258262890683122, 1.000000000000000000, 0.9659258262890683122, 1.000000000000000000, 0.9659258262890683122, 1.000000000000000000, 0.9659258262890683122, 1.000000000000000000, 0.9659258262890683122, 1.000000000000000000, 0.9659258262890683122, 1.000000000000000000, 0.9659258262890683122, 1.000000000000000000, 0.9659258262890683122, 1.000000000000000000, 0.9659258262890683122, 1.000000000000000000, 0.9659258262890683122, 1.000000000000000000, 0.9659258262890683122, 1.000000000000000000, 0.9659258262890683122, 1.000000000000000000, 0.9659258262890683122, 1.000000000000000000, 0.9659258262890683122, 1.000000000000000000, 0.9659258262890683122, 1.000000000000000000, 0.9659258262890683122, 1.000000000000000000, 0.9659258262890683122, 1.000000000000000000, 0.9659258262890683122, 1.000000000000000000, 0.9659258262890683122, 1.000000000000000000, 0.9659258262890683122, 1.000000000000000000, 0.9659258262890683122, 1.000000000000000000, 0.9659258262890683122, 1.000000000000000000, 0.9659258262890683122, 1.000000000000000000, 0.9659258262890683122, 1.000000000000000000, 0.9659258262890683122, 1.000000000000000000, 0.9659258262890683122, 1.000000000000000000, 0.9659258262890683122, 1.000000000000000000, 0.9659258262890683122, 1.000000000000000000, 0.9659258262890683122, 1.000000000000000000, 0.9659258262890683122, 1.000000000000000000, 0.9659258262890683122, 1.000000000000000000, 0.9659258262890683122, 1.000000000000000000, 0.9659258262890683122, 1.000000000000000000, 0.9659258262890683122, 1.000000000000000000, 0.9659258262890683122, 1.000000000000000000, 0.9659258262890683122, 1.000000000000000000, 0.9659258262890683122, 1.000000000000000000, 0.9659258262890683122, 1.000000000000000000, 0.9659258262890683122, 1.000000000000000000, 0.9659258262890683122, 1.000000000000000000, 0.9659258262890683122, 1.000000000000000000, 0.9659258262890683122, 1.000000000000000000, 0.9659258262890683122, 1.000000000000000000, 0.9659258262890683122, 1.000000000000000000, 0.9659258262890683122, 1.000000000000000000, 0.9659258262890683122, 1.000000000000000000, 0.9659258262890683122, 1.000000000000000000, 0.9659258262890683122, 1.000000000000000000, 0.9659258262890683122, 1.000000000000000000, 0.9659258262890683122, 1.000000000000000000, 0.9659258262890683122, 1.000000000000000000, 0.9659258262890683122, 1.000000000000000000, 0.9659258262890683122, 1.000000000000000000, 0.9659258262890683122, 1.000000000000000000, 0.9659258262890683122, 1.000000000000000000, 0.9659258262890683122, 1.000000000000000000, 0.9659258262890683122, 1.000000000000000000, 0.9659258262890683122, 1.000000000000000000, 0.9659258262890683122, 1.000000000000000000, 0.9659258262890683122, 1.000000000000000000, 0.9659258262890683122, 1.000000000000000000, 0.9659258262890683122, 1.000000000000000000, 0.9659258262890683122, 1.000000000000000000, 0.9659258262890683122, 1.000000000000000000, 0.9659258262890683122, 1.000000000000000000, 0.9659258262890683122, 1.000000000000000000, 0.9659258262890683122, 1.000000000000000000, 0.9659258262890683122, 1.000000000000000000, 0.9659258262890683122, 1.000000000000000000, 0.9659258262890683122, 1.000000000000000000, 0.9659258262890683122, 1.000000000000000000, 0.9659258262890683122, 1.000000000000000000, 0.9659258262890683122, 1.000000000000000000, 0.9659258262890683122, 1.000000000000000000, 0.9659258262890683122, 1.000000000000000000, 0.9659258262890683122, 1.000000000000000000, 0.9659258262890683122, 1.000000000000000000, 0.9659258262890683122, 1.000000000000000000, 0.9659258262890683122, 1.000000000000000000, 0.9659258262890683122, 1.000000000000000000, 0.9659258262890683122, 1.000000000000000000, 0.9659258262890683122, 1.000000000000000000, 0.9659258262890683122, 1.000000000000000000, 0.9659258262890683122, 1.000000000000000000, 0.9659258262890683122, 1.000000000000000000, 0.9659258262890683122, 1.000000000000000000, 0.9659258262890683122, 1.000000000000000000, 0.9659258262890683122, 1.000000000000000000, 0.9659258262890683122, 1.000000000000000000, 0.9659258262890683122, 1.000000000000000000, 0.9659258262890683122, 1.000000000000000000, 0.9659258262890683122, 1.000000000000000000, 0.9659258262890683122, 1.000000000000000000, 0.9659258262890683122, 1.000000000000000000, 0.9659258262890683122, 1.000000000000000000, 0.9659258262890683122, 1.000000000000000000, 0.9659258262890683122, 1.000000000000000000, 0.9659258262890683122, 1.000000000000000000, 0.9659258262890683122, 1.000000000000000000, 0.9659258262890683122, 1.000000000000000000, 0.9659258262890683122, 1.000000000000000000, 0.9659258262890683122, 1.000000000000000000, 0.9659258262890683122, 1.000000000000000000, 0.9659258262890683122, 1.000000000000000000, 0.9659258262890683122, 1.000000000000000000, 0.9659258262890683122, 1.000000000000000000, 0.9659258262890683122, 1.000000000000000000, 0.9659258262890683122, 1.000000000000000000, 0.9659258262890683122, 1.000000000000000000, 0.9659258262890683122, 1.000000000000000000, 0.9659258262890683122, 1.000000000000000000, 0.9659258262890683122, 1.000000000000000000, 0.9659258262890683122, 1.000000000000000000, 0.9659258262890683122, 1.000000000000000000, 0.9659258262890683122, 1.000000000000000000, 0.9659258262890683122, 1.000000000000000000, 0.9659258262890683122, 1.000000000000000000, 0.9659258262890683122, 1.000000000000000000, 0.9659258262890683122, 1.000000000000000000, 0.9659258262890683122, 1.000000000000000000, 0.9659258262890683122, 1.000000000000000000, 0.9659258262890683122, 1.000000000000000000, 0.9659258262890683122, 1.000000000000000000, 0.9659258262890683122, 1.000000000000000000, 0.9659258262890683122, 1.000000000000000000, 0.9659258262890683122, 1.000000000000000000, 0.9659258262890683122, 1.000000000000000000, 0.9659258262890683122, 1.000000000000000000, 0.9659258262890683122, 1.000000000000000000, 0.9659258262890683122, 1.000000000000000000, 0.9659258262890683122, 1.000000000000000000, 0.9659258262890683122, 1.000000000000000000, 0.9659258262890683122, 1.000000000000000000, 0.9659258262890683122, 1.000000000000000000, 0.9659258262890683122, 1.000000000000000000, 0.9659258262890683122, 1.000000000000000000, 0.9659258262890683122, 1.000000000000000000, 0.9659258262890683122, 1.000000000000000000, 0.9659258262890683122, 1.000000000000000000, 0.9659258262890683122, 1.000000000000000000, 0.9659258262890683122, 1.000000000000000000, 0.9659258262890683122, 1.000000000000000000, 0.9659258262890683122, 1.000000000000000000, 0.9659258262890683122, 1.000000000000000000, 0.9659258262890683122, 1.000000000000000000, 0.9659258262890683122, 1.000000000000000000, 0.9659258262890683122, 1.000000000000000000, 0.9659258262890683122, 1.000000000000000000, 0.9659258262890683122, 1.000000000000000000, 0.9659258262890683122, 1.000000000000000000, 0.9659258262890683122, 1.000000000000000000, 0.9659258262890683122, 1.000000000000000000, 0.9659258262890683122, 1.000000000000000000, 0.9659258262890683122, 1.000000000000000000, 0.9659258262890683122, 1.000000000000000000, 0.9659258262890683122, 1.000000000000000000, 0.9659258262890683122, 1.000000000000000000, 0.9659258262890683122, 1.000000000000000000, 0.9659258262890683122, 1.000000000000000000, 0.9659258262890683122, 1.000000000000000000, 0.9659258262890683122, 1.000000000000000000, 0.9659258262890683122, 1.000000000000000000, 0.9659258262890683122, 1.000000000000000000, 0.9659258262890683122, 1.000000000000000000, 0.9659258262890683122, 1.000000000000000000, 0.9659258262890683122, 1.000000000000000000, 0.9659258262890683122, 1.000000000000000000, 0.9659258262890683122, 1.000000000000000000, 0.9659258262890683122, 1.000000000000000000, 0.9659258262890683122, 1.000000000000000000, 0.9659258262890683122, 1.000000000000000000, 0.9659258262890683122, 1.000000000000000000, 0.9659258262890683122, 1.000000000000000000, 0.9659258262890683122, 1.000000000000000000, 0.9659258262890683122, 1.000000000000000000, 0.9659258262890683122, 1.000000000000000000, 0.9659258262890683122, 1.000000000000000000, 0.9659258262890683122, 1.000000000000000000, 0.9659258262890683122, 1.000000000000000000, 0.9659258262890683122, 1.000000000000000000, 0.9659258262890683122, 1.000000000000000000, 0.9659258262890683122, 1.000000000000000000, 0.9659258262890683122, 1.000000000000000000, 0.9659258262890683122, 1.000000000000000000, 0.9659258262890683122, 1.000000000000000000, 0.9659258262890683122, 1.000000000000000000, 0.9659258262890683122, 1.000000000000000000, 0.9659258262890683122, 1.000000000000000000, 0.9659258262890683122, 1.000000000000000000, 0.9659258262890683122, 1.000000000000000000, 0.9659258262890683122, 1.000000000000000000, 0.9659258262890683122, 1.000000000000000000, 0.9659258262890683122, 1.000000000000000000, 0.9659258262890683122, 1.000000000000000000, 0.9659258262890683122, 1.000000000000000000, 0.9659258262890683122, 1.000000000000000000, 0.9659258262890683122, 1.000000000000000000, 0.9659258262890683122, 1.000000000000000000, 0.9659258262890683122, 1.000000000000000000, 0.9659258262890683122, 1.000000000000000000, 0.9659258262890683122, 1.000000000000000000, 0.9659258262890683122, 1.000000000000000000, 0.9659258262890683122, 1.000000000000000000, 0.9659258262890683122, 1.000000000000000000, 0.9659258262890683122, 1.000000000000000000, 0.9659258262890683122, 1.000000000000000000, 0.9659258262890683122, 1.000000000000000000, 0.9659258262890683122, 1.000000000000000000, 0.9659258262890683122, 1.000000000000000000, 0.9659258262890683122, 1.000000000000000000, 0.9659258262890683122, 1.000000000000000000, 0.9659258262890683122, 1.000000000000000000, 0.9659258262890683122, 1.000000000000000000, 0.9659258262890683122, 1.000000000000000000, 0.9659258262890683122, 1.000000000000000000, 0.9659258262890683122, 1.000000000000000000, 0.9659258262890683122, 1.000000000000000000, 0.9659258262890683122, 1.000000000000000000, 0.9659258262890683122, 1.000000000000000000, 0.9659258262890683122, 1.000000000000000000, 0.9659258262890683122, 1.000000000000000000, 0.9659258262890683122, 1.000000000000000000, 0.9659258262890683122, 1.000000000000000000, 0.9659258262890683122, 1.000000000000000000, 0.9659258262890683122, 1.000000000000000000),
 ( 0.3333333333333333703, 0.3219752754296894559, 0.3333333333333333703, 0.3219752754296894559, 0.3333333333333333703, 0.3219752754296894559, 0.3333333333333333703, 0.3219752754296894559, 0.3333333333333333703, 0.3219752754296894559, 0.3333333333333333703, 0.3219752754296894559, 0.3333333333333333703, 0.3219752754296894559, 0.3333333333333333703, 0.3219752754296894559, 0.3333333333333333703, 0.3219752754296894559, 0.3333333333333333703, 0.3219752754296894559, 0.3333333333333333703, 0.3219752754296894559, 0.3333333333333333703, 0.3219752754296894559, 0.3333333333333333703, 0.3219752754296894559, 0.3333333333333333703, 0.3219752754296894559, 0.3333333333333333703, 0.3219752754296894559, 0.3333333333333333703, 0.3219752754296894559, 0.3333333333333333703, 0.3219752754296894559, 0.3333333333333333703, 0.3219752754296894559, 0.3333333333333333703, 0.3219752754296894559, 0.3333333333333333703, 0.3219752754296894559, 0.3333333333333333703, 0.3219752754296894559, 0.3333333333333333703, 0.3219752754296894559, 0.3333333333333333703, 0.3219752754296894559, 0.3333333333333333703, 0.3219752754296894559, 0.3333333333333333703, 0.3219752754296894559, 0.3333333333333333703, 0.3219752754296894559, 0.3333333333333333703, 0.3219752754296894559, 0.3333333333333333703, 0.3219752754296894559, 0.3333333333333333703, 0.3219752754296894559, 0.3333333333333333703, 0.3219752754296894559, 0.3333333333333333703, 0.3219752754296894559, 0.3333333333333333703, 0.3219752754296894559, 0.3333333333333333703, 0.3219752754296894559, 0.3333333333333333703, 0.3219752754296894559, 0.3333333333333333703, 0.3219752754296894559, 0.3333333333333333703, 0.3219752754296894559, 0.3333333333333333703, 0.3219752754296894559, 0.3333333333333333703, 0.3219752754296894559, 0.3333333333333333703, 0.3219752754296894559, 0.3333333333333333703, 0.3219752754296894559, 0.3333333333333333703, 0.3219752754296894559, 0.3333333333333333703, 0.3219752754296894559, 0.3333333333333333703, 0.3219752754296894559, 0.3333333333333333703, 0.3219752754296894559, 0.3333333333333333703, 0.3219752754296894559, 0.3333333333333333703, 0.3219752754296894559, 0.3333333333333333703, 0.3219752754296894559, 0.3333333333333333703, 0.3219752754296894559, 0.3333333333333333703, 0.3219752754296894559, 0.3333333333333333703, 0.3219752754296894559, 0.3333333333333333703, 0.3219752754296894559, 0.3333333333333333703, 0.3219752754296894559, 0.3333333333333333703, 0.3219752754296894559, 0.3333333333333333703, 0.3219752754296894559, 0.3333333333333333703, 0.3219752754296894559, 0.3333333333333333703, 0.3219752754296894559, 0.3333333333333333703, 0.3219752754296894559, 0.3333333333333333703, 0.3219752754296894559, 0.3333333333333333703, 0.3219752754296894559, 0.3333333333333333703, 0.3219752754296894559, 0.3333333333333333703, 0.3219752754296894559, 0.3333333333333333703, 0.3219752754296894559, 0.3333333333333333703, 0.3219752754296894559, 0.3333333333333333703, 0.3219752754296894559, 0.3333333333333333703, 0.3219752754296894559, 0.3333333333333333703, 0.3219752754296894559, 0.3333333333333333703, 0.3219752754296894559, 0.3333333333333333703, 0.3219752754296894559, 0.3333333333333333703, 0.3219752754296894559, 0.3333333333333333703, 0.3219752754296894559, 0.3333333333333333703, 0.3219752754296894559, 0.3333333333333333703, 0.3219752754296894559, 0.3333333333333333703, 0.3219752754296894559, 0.3333333333333333703, 0.3219752754296894559, 0.3333333333333333703, 0.3219752754296894559, 0.3333333333333333703, 0.3219752754296894559, 0.3333333333333333703, 0.3219752754296894559, 0.3333333333333333703, 0.3219752754296894559, 0.3333333333333333703, 0.3219752754296894559, 0.3333333333333333703, 0.3219752754296894559, 0.3333333333333333703, 0.3219752754296894559, 0.3333333333333333703, 0.3219752754296894559, 0.3333333333333333703, 0.3219752754296894559, 0.3333333333333333703, 0.3219752754296894559, 0.3333333333333333703, 0.3219752754296894559, 0.3333333333333333703, 0.3219752754296894559, 0.3333333333333333703, 0.3219752754296894559, 0.3333333333333333703, 0.3219752754296894559, 0.3333333333333333703, 0.3219752754296894559, 0.3333333333333333703, 0.3219752754296894559, 0.3333333333333333703, 0.3219752754296894559, 0.3333333333333333703, 0.3219752754296894559, 0.3333333333333333703, 0.3219752754296894559, 0.3333333333333333703, 0.3219752754296894559, 0.3333333333333333703, 0.3219752754296894559, 0.3333333333333333703, 0.3219752754296894559, 0.3333333333333333703, 0.3219752754296894559, 0.3333333333333333703, 0.3219752754296894559, 0.3333333333333333703, 0.3219752754296894559, 0.3333333333333333703, 0.3219752754296894559, 0.3333333333333333703, 0.3219752754296894559, 0.3333333333333333703, 0.3219752754296894559, 0.3333333333333333703, 0.3219752754296894559, 0.3333333333333333703, 0.3219752754296894559, 0.3333333333333333703, 0.3219752754296894559, 0.3333333333333333703, 0.3219752754296894559, 0.3333333333333333703, 0.3219752754296894559, 0.3333333333333333703, 0.3219752754296894559, 0.3333333333333333703, 0.3219752754296894559, 0.3333333333333333703, 0.3219752754296894559, 0.3333333333333333703, 0.3219752754296894559, 0.3333333333333333703, 0.3219752754296894559, 0.3333333333333333703, 0.3219752754296894559, 0.3333333333333333703, 0.3219752754296894559, 0.3333333333333333703, 0.3219752754296894559, 0.3333333333333333703, 0.3219752754296894559, 0.3333333333333333703, 0.3219752754296894559, 0.3333333333333333703, 0.3219752754296894559, 0.3333333333333333703, 0.3219752754296894559, 0.3333333333333333703, 0.3219752754296894559, 0.3333333333333333703, 0.3219752754296894559, 0.3333333333333333703, 0.3219752754296894559, 0.3333333333333333703, 0.3219752754296894559, 0.3333333333333333703, 0.3219752754296894559, 0.3333333333333333703, 0.3219752754296894559, 0.3333333333333333703, 0.3219752754296894559, 0.3333333333333333703, 0.3219752754296894559, 0.3333333333333333703, 0.3219752754296894559, 0.3333333333333333703, 0.3219752754296894559, 0.3333333333333333703, 0.3219752754296894559, 0.3333333333333333703, 0.3219752754296894559, 0.3333333333333333703, 0.3219752754296894559, 0.3333333333333333703, 0.3219752754296894559, 0.3333333333333333703, 0.3219752754296894559, 0.3333333333333333703, 0.3219752754296894559, 0.3333333333333333703, 0.3219752754296894559, 0.3333333333333333703, 0.3219752754296894559, 0.3333333333333333703, 0.3219752754296894559, 0.3333333333333333703, 0.3219752754296894559, 0.3333333333333333703, 0.3219752754296894559, 0.3333333333333333703, 0.3219752754296894559, 0.3333333333333333703, 0.3219752754296894559, 0.3333333333333333703, 0.3219752754296894559, 0.3333333333333333703, 0.3219752754296894559, 0.3333333333333333703, 0.3219752754296894559, 0.3333333333333333703, 0.3219752754296894559, 0.3333333333333333703, 0.3219752754296894559, 0.3333333333333333703, 0.3219752754296894559, 0.3333333333333333703, 0.3219752754296894559, 0.3333333333333333703, 0.3219752754296894559, 0.3333333333333333703, 0.3219752754296894559, 0.3333333333333333703, 0.3219752754296894559, 0.3333333333333333703, 0.3219752754296894559, 0.3333333333333333703, 0.3219752754296894559, 0.3333333333333333703, 0.3219752754296894559, 0.3333333333333333703, 0.3219752754296894559, 0.3333333333333333703, 0.3219752754296894559, 0.3333333333333333703, 0.3219752754296894559, 0.3333333333333333703, 0.3219752754296894559, 0.3333333333333333703, 0.3219752754296894559, 0.3333333333333333703, 0.3219752754296894559, 0.3333333333333333703, 0.3219752754296894559, 0.3333333333333333703, 0.3219752754296894559, 0.3333333333333333703, 0.3219752754296894559, 0.3333333333333333703, 0.3219752754296894559, 0.3333333333333333703, 0.3219752754296894559, 0.3333333333333333703, 0.3219752754296894559, 0.3333333333333333703, 0.3219752754296894559, 0.3333333333333333703, 0.3219752754296894559, 0.3333333333333333703, 0.3219752754296894559, 0.3333333333333333703, 0.3219752754296894559, 0.3333333333333333703, 0.3219752754296894559, 0.3333333333333333703, 0.3219752754296894559, 0.3333333333333333703, 0.3219752754296894559, 0.3333333333333333703, 0.3219752754296894559, 0.3333333333333333703, 0.3219752754296894559, 0.3333333333333333703, 0.3219752754296894559, 0.3333333333333333703, 0.3219752754296894559, 0.3333333333333333703, 0.3219752754296894559, 0.3333333333333333703, 0.3219752754296894559, 0.3333333333333333703, 0.3219752754296894559, 0.3333333333333333703, 0.3219752754296894559, 0.3333333333333333703, 0.3219752754296894559, 0.3333333333333333703, 0.3219752754296894559, 0.3333333333333333703, 0.3219752754296894559, 0.3333333333333333703, 0.3219752754296894559, 0.3333333333333333703, 0.3219752754296894559, 0.3333333333333333703, 0.3219752754296894559, 0.3333333333333333703, 0.3219752754296894559, 0.3333333333333333703, 0.3219752754296894559, 0.3333333333333333703, 0.3219752754296894559, 0.3333333333333333703, 0.3219752754296894559, 0.3333333333333333703, 0.3219752754296894559, 0.3333333333333333703, 0.3219752754296894559, 0.3333333333333333703, 0.3219752754296894559, 0.3333333333333333703, 0.3219752754296894559, 0.3333333333333333703, 0.3219752754296894559, 0.3333333333333333703, 0.3219752754296894559, 0.3333333333333333703, 0.3219752754296894559, 0.3333333333333333703, 0.3219752754296894559, 0.3333333333333333703, 0.3219752754296894559, 0.3333333333333333703, 0.3219752754296894559, 0.3333333333333333703, 0.3219752754296894559, 0.3333333333333333703, 0.3219752754296894559, 0.3333333333333333703, 0.3219752754296894559, 0.3333333333333333703, 0.3219752754296894559, 0.3333333333333333703, 0.3219752754296894559, 0.3333333333333333703, 0.3219752754296894559, 0.3333333333333333703, 0.3219752754296894559, 0.3333333333333333703, 0.3219752754296894559, 0.3333333333333333703, 0.3219752754296894559, 0.3333333333333333703, 0.3219752754296894559, 0.3333333333333333703, 0.3219752754296894559, 0.3333333333333333703, 0.3219752754296894559, 0.3333333333333333703, 0.3219752754296894559, 0.3333333333333333703, 0.3219752754296894559, 0.3333333333333333703, 0.3219752754296894559, 0.3333333333333333703, 0.3219752754296894559, 0.3333333333333333703, 0.3219752754296894559, 0.3333333333333333703, 0.3219752754296894559, 0.3333333333333333703, 0.3219752754296894559, 0.3333333333333333703, 0.3219752754296894559, 0.3333333333333333703, 0.3219752754296894559, 0.3333333333333333703, 0.3219752754296894559, 0.3333333333333333703, 0.3219752754296894559, 0.3333333333333333703, 0.3219752754296894559, 0.3333333333333333703, 0.3219752754296894559, 0.3333333333333333703, 0.3219752754296894559, 0.3333333333333333703),
 ( 0.3333333333333333703, 0.3219752754296894559, 0.3333333333333333703, 0.3219752754296894559, 0.3333333333333333703, 0.3219752754296894559, 0.3333333333333333703, 0.3219752754296894559, 0.3333333333333333703, 0.3219752754296894559, 0.3333333333333333703, 0.3219752754296894559, 0.3333333333333333703, 0.3219752754296894559, 0.3333333333333333703, 0.3219752754296894559, 0.3333333333333333703, 0.3219752754296894559, 0.3333333333333333703, 0.3219752754296894559, 0.3333333333333333703, 0.3219752754296894559, 0.3333333333333333703, 0.3219752754296894559, 0.3333333333333333703, 0.3219752754296894559, 0.3333333333333333703, 0.3219752754296894559, 0.3333333333333333703, 0.3219752754296894559, 0.3333333333333333703, 0.3219752754296894559, 0.3333333333333333703, 0.3219752754296894559, 0.3333333333333333703, 0.3219752754296894559, 0.3333333333333333703, 0.3219752754296894559, 0.3333333333333333703, 0.3219752754296894559, 0.3333333333333333703, 0.3219752754296894559, 0.3333333333333333703, 0.3219752754296894559, 0.3333333333333333703, 0.3219752754296894559, 0.3333333333333333703, 0.3219752754296894559, 0.3333333333333333703, 0.3219752754296894559, 0.3333333333333333703, 0.3219752754296894559, 0.3333333333333333703, 0.3219752754296894559, 0.3333333333333333703, 0.3219752754296894559, 0.3333333333333333703, 0.3219752754296894559, 0.3333333333333333703, 0.3219752754296894559, 0.3333333333333333703, 0.3219752754296894559, 0.3333333333333333703, 0.3219752754296894559, 0.3333333333333333703, 0.3219752754296894559, 0.3333333333333333703, 0.3219752754296894559, 0.3333333333333333703, 0.3219752754296894559, 0.3333333333333333703, 0.3219752754296894559, 0.3333333333333333703, 0.3219752754296894559, 0.3333333333333333703, 0.3219752754296894559, 0.3333333333333333703, 0.3219752754296894559, 0.3333333333333333703, 0.3219752754296894559, 0.3333333333333333703, 0.3219752754296894559, 0.3333333333333333703, 0.3219752754296894559, 0.3333333333333333703, 0.3219752754296894559, 0.3333333333333333703, 0.3219752754296894559, 0.3333333333333333703, 0.3219752754296894559, 0.3333333333333333703, 0.3219752754296894559, 0.3333333333333333703, 0.3219752754296894559, 0.3333333333333333703, 0.3219752754296894559, 0.3333333333333333703, 0.3219752754296894559, 0.3333333333333333703, 0.3219752754296894559, 0.3333333333333333703, 0.3219752754296894559, 0.3333333333333333703, 0.3219752754296894559, 0.3333333333333333703, 0.3219752754296894559, 0.3333333333333333703, 0.3219752754296894559, 0.3333333333333333703, 0.3219752754296894559, 0.3333333333333333703, 0.3219752754296894559, 0.3333333333333333703, 0.3219752754296894559, 0.3333333333333333703, 0.3219752754296894559, 0.3333333333333333703, 0.3219752754296894559, 0.3333333333333333703, 0.3219752754296894559, 0.3333333333333333703, 0.3219752754296894559, 0.3333333333333333703, 0.3219752754296894559, 0.3333333333333333703, 0.3219752754296894559, 0.3333333333333333703, 0.3219752754296894559, 0.3333333333333333703, 0.3219752754296894559, 0.3333333333333333703, 0.3219752754296894559, 0.3333333333333333703, 0.3219752754296894559, 0.3333333333333333703, 0.3219752754296894559, 0.3333333333333333703, 0.3219752754296894559, 0.3333333333333333703, 0.3219752754296894559, 0.3333333333333333703, 0.3219752754296894559, 0.3333333333333333703, 0.3219752754296894559, 0.3333333333333333703, 0.3219752754296894559, 0.3333333333333333703, 0.3219752754296894559, 0.3333333333333333703, 0.3219752754296894559, 0.3333333333333333703, 0.3219752754296894559, 0.3333333333333333703, 0.3219752754296894559, 0.3333333333333333703, 0.3219752754296894559, 0.3333333333333333703, 0.3219752754296894559, 0.3333333333333333703, 0.3219752754296894559, 0.3333333333333333703, 0.3219752754296894559, 0.3333333333333333703, 0.3219752754296894559, 0.3333333333333333703, 0.3219752754296894559, 0.3333333333333333703, 0.3219752754296894559, 0.3333333333333333703, 0.3219752754296894559, 0.3333333333333333703, 0.3219752754296894559, 0.3333333333333333703, 0.3219752754296894559, 0.3333333333333333703, 0.3219752754296894559, 0.3333333333333333703, 0.3219752754296894559, 0.3333333333333333703, 0.3219752754296894559, 0.3333333333333333703, 0.3219752754296894559, 0.3333333333333333703, 0.3219752754296894559, 0.3333333333333333703, 0.3219752754296894559, 0.3333333333333333703, 0.3219752754296894559, 0.3333333333333333703, 0.3219752754296894559, 0.3333333333333333703, 0.3219752754296894559, 0.3333333333333333703, 0.3219752754296894559, 0.3333333333333333703, 0.3219752754296894559, 0.3333333333333333703, 0.3219752754296894559, 0.3333333333333333703, 0.3219752754296894559, 0.3333333333333333703, 0.3219752754296894559, 0.3333333333333333703, 0.3219752754296894559, 0.3333333333333333703, 0.3219752754296894559, 0.3333333333333333703, 0.3219752754296894559, 0.3333333333333333703, 0.3219752754296894559, 0.3333333333333333703, 0.3219752754296894559, 0.3333333333333333703, 0.3219752754296894559, 0.3333333333333333703, 0.3219752754296894559, 0.3333333333333333703, 0.3219752754296894559, 0.3333333333333333703, 0.3219752754296894559, 0.3333333333333333703, 0.3219752754296894559, 0.3333333333333333703, 0.3219752754296894559, 0.3333333333333333703, 0.3219752754296894559, 0.3333333333333333703, 0.3219752754296894559, 0.3333333333333333703, 0.3219752754296894559, 0.3333333333333333703, 0.3219752754296894559, 0.3333333333333333703, 0.3219752754296894559, 0.3333333333333333703, 0.3219752754296894559, 0.3333333333333333703, 0.3219752754296894559, 0.3333333333333333703, 0.3219752754296894559, 0.3333333333333333703, 0.3219752754296894559, 0.3333333333333333703, 0.3219752754296894559, 0.3333333333333333703, 0.3219752754296894559, 0.3333333333333333703, 0.3219752754296894559, 0.3333333333333333703, 0.3219752754296894559, 0.3333333333333333703, 0.3219752754296894559, 0.3333333333333333703, 0.3219752754296894559, 0.3333333333333333703, 0.3219752754296894559, 0.3333333333333333703, 0.3219752754296894559, 0.3333333333333333703, 0.3219752754296894559, 0.3333333333333333703, 0.3219752754296894559, 0.3333333333333333703, 0.3219752754296894559, 0.3333333333333333703, 0.3219752754296894559, 0.3333333333333333703, 0.3219752754296894559, 0.3333333333333333703, 0.3219752754296894559, 0.3333333333333333703, 0.3219752754296894559, 0.3333333333333333703, 0.3219752754296894559, 0.3333333333333333703, 0.3219752754296894559, 0.3333333333333333703, 0.3219752754296894559, 0.3333333333333333703, 0.3219752754296894559, 0.3333333333333333703, 0.3219752754296894559, 0.3333333333333333703, 0.3219752754296894559, 0.3333333333333333703, 0.3219752754296894559, 0.3333333333333333703, 0.3219752754296894559, 0.3333333333333333703, 0.3219752754296894559, 0.3333333333333333703, 0.3219752754296894559, 0.3333333333333333703, 0.3219752754296894559, 0.3333333333333333703, 0.3219752754296894559, 0.3333333333333333703, 0.3219752754296894559, 0.3333333333333333703, 0.3219752754296894559, 0.3333333333333333703, 0.3219752754296894559, 0.3333333333333333703, 0.3219752754296894559, 0.3333333333333333703, 0.3219752754296894559, 0.3333333333333333703, 0.3219752754296894559, 0.3333333333333333703, 0.3219752754296894559, 0.3333333333333333703, 0.3219752754296894559, 0.3333333333333333703, 0.3219752754296894559, 0.3333333333333333703, 0.3219752754296894559, 0.3333333333333333703, 0.3219752754296894559, 0.3333333333333333703, 0.3219752754296894559, 0.3333333333333333703, 0.3219752754296894559, 0.3333333333333333703, 0.3219752754296894559, 0.3333333333333333703, 0.3219752754296894559, 0.3333333333333333703, 0.3219752754296894559, 0.3333333333333333703, 0.3219752754296894559, 0.3333333333333333703, 0.3219752754296894559, 0.3333333333333333703, 0.3219752754296894559, 0.3333333333333333703, 0.3219752754296894559, 0.3333333333333333703, 0.3219752754296894559, 0.3333333333333333703, 0.3219752754296894559, 0.3333333333333333703, 0.3219752754296894559, 0.3333333333333333703, 0.3219752754296894559, 0.3333333333333333703, 0.3219752754296894559, 0.3333333333333333703, 0.3219752754296894559, 0.3333333333333333703, 0.3219752754296894559, 0.3333333333333333703, 0.3219752754296894559, 0.3333333333333333703, 0.3219752754296894559, 0.3333333333333333703, 0.3219752754296894559, 0.3333333333333333703, 0.3219752754296894559, 0.3333333333333333703, 0.3219752754296894559, 0.3333333333333333703, 0.3219752754296894559, 0.3333333333333333703, 0.3219752754296894559, 0.3333333333333333703, 0.3219752754296894559, 0.3333333333333333703, 0.3219752754296894559, 0.3333333333333333703, 0.3219752754296894559, 0.3333333333333333703, 0.3219752754296894559, 0.3333333333333333703, 0.3219752754296894559, 0.3333333333333333703, 0.3219752754296894559, 0.3333333333333333703, 0.3219752754296894559, 0.3333333333333333703, 0.3219752754296894559, 0.3333333333333333703, 0.3219752754296894559, 0.3333333333333333703, 0.3219752754296894559, 0.3333333333333333703, 0.3219752754296894559, 0.3333333333333333703, 0.3219752754296894559, 0.3333333333333333703, 0.3219752754296894559, 0.3333333333333333703, 0.3219752754296894559, 0.3333333333333333703, 0.3219752754296894559, 0.3333333333333333703, 0.3219752754296894559, 0.3333333333333333703, 0.3219752754296894559, 0.3333333333333333703, 0.3219752754296894559, 0.3333333333333333703, 0.3219752754296894559, 0.3333333333333333703, 0.3219752754296894559, 0.3333333333333333703, 0.3219752754296894559, 0.3333333333333333703, 0.3219752754296894559, 0.3333333333333333703, 0.3219752754296894559, 0.3333333333333333703, 0.3219752754296894559, 0.3333333333333333703, 0.3219752754296894559, 0.3333333333333333703, 0.3219752754296894559, 0.3333333333333333703, 0.3219752754296894559, 0.3333333333333333703, 0.3219752754296894559, 0.3333333333333333703, 0.3219752754296894559, 0.3333333333333333703, 0.3219752754296894559, 0.3333333333333333703, 0.3219752754296894559, 0.3333333333333333703, 0.3219752754296894559, 0.3333333333333333703, 0.3219752754296894559, 0.3333333333333333703, 0.3219752754296894559, 0.3333333333333333703, 0.3219752754296894559, 0.3333333333333333703, 0.3219752754296894559, 0.3333333333333333703, 0.3219752754296894559, 0.3333333333333333703, 0.3219752754296894559, 0.3333333333333333703, 0.3219752754296894559, 0.3333333333333333703, 0.3219752754296894559, 0.3333333333333333703, 0.3219752754296894559, 0.3333333333333333703, 0.3219752754296894559, 0.3333333333333333703, 0.3219752754296894559, 0.3333333333333333703, 0.3219752754296894559, 0.3333333333333333703, 0.3219752754296894559, 0.3333333333333333703, 0.3219752754296894559, 0.3333333333333333703),
 ( 1.000000000000000000, 0.9659258262890683122, 1.000000000000000000, 0.9659258262890683122, 1.000000000000000000, 0.9659258262890683122, 1.000000000000000000, 0.9659258262890683122, 1.000000000000000000, 0.9659258262890683122, 1.000000000000000000, 0.9659258262890683122, 1.000000000000000000, 0.9659258262890683122, 1.000000000000000000, 0.9659258262890683122, 1.000000000000000000, 0.9659258262890683122, 1.000000000000000000, 0.9659258262890683122, 1.000000000000000000, 0.9659258262890683122, 1.000000000000000000, 0.9659258262890683122, 1.000000000000000000, 0.9659258262890683122, 1.000000000000000000, 0.9659258262890683122, 1.000000000000000000, 0.9659258262890683122, 1.000000000000000000, 0.9659258262890683122, 1.000000000000000000, 0.9659258262890683122, 1.000000000000000000, 0.9659258262890683122, 1.000000000000000000, 0.9659258262890683122, 1.000000000000000000, 0.9659258262890683122, 1.000000000000000000, 0.9659258262890683122, 1.000000000000000000, 0.9659258262890683122, 1.000000000000000000, 0.9659258262890683122, 1.000000000000000000, 0.9659258262890683122, 1.000000000000000000, 0.9659258262890683122, 1.000000000000000000, 0.9659258262890683122, 1.000000000000000000, 0.9659258262890683122, 1.000000000000000000, 0.9659258262890683122, 1.000000000000000000, 0.9659258262890683122, 1.000000000000000000, 0.9659258262890683122, 1.000000000000000000, 0.9659258262890683122, 1.000000000000000000, 0.9659258262890683122, 1.000000000000000000, 0.9659258262890683122, 1.000000000000000000, 0.9659258262890683122, 1.000000000000000000, 0.9659258262890683122, 1.000000000000000000, 0.9659258262890683122, 1.000000000000000000, 0.9659258262890683122, 1.000000000000000000, 0.9659258262890683122, 1.000000000000000000, 0.9659258262890683122, 1.000000000000000000, 0.9659258262890683122, 1.000000000000000000, 0.9659258262890683122, 1.000000000000000000, 0.9659258262890683122, 1.000000000000000000, 0.9659258262890683122, 1.000000000000000000, 0.9659258262890683122, 1.000000000000000000, 0.9659258262890683122, 1.000000000000000000, 0.9659258262890683122, 1.000000000000000000, 0.9659258262890683122, 1.000000000000000000, 0.9659258262890683122, 1.000000000000000000, 0.9659258262890683122, 1.000000000000000000, 0.9659258262890683122, 1.000000000000000000, 0.9659258262890683122, 1.000000000000000000, 0.9659258262890683122, 1.000000000000000000, 0.9659258262890683122, 1.000000000000000000, 0.9659258262890683122, 1.000000000000000000, 0.9659258262890683122, 1.000000000000000000, 0.9659258262890683122, 1.000000000000000000, 0.9659258262890683122, 1.000000000000000000, 0.9659258262890683122, 1.000000000000000000, 0.9659258262890683122, 1.000000000000000000, 0.9659258262890683122, 1.000000000000000000, 0.9659258262890683122, 1.000000000000000000, 0.9659258262890683122, 1.000000000000000000, 0.9659258262890683122, 1.000000000000000000, 0.9659258262890683122, 1.000000000000000000, 0.9659258262890683122, 1.000000000000000000, 0.9659258262890683122, 1.000000000000000000, 0.9659258262890683122, 1.000000000000000000, 0.9659258262890683122, 1.000000000000000000, 0.9659258262890683122, 1.000000000000000000, 0.9659258262890683122, 1.000000000000000000, 0.9659258262890683122, 1.000000000000000000, 0.9659258262890683122, 1.000000000000000000, 0.9659258262890683122, 1.000000000000000000, 0.9659258262890683122, 1.000000000000000000, 0.9659258262890683122, 1.000000000000000000, 0.9659258262890683122, 1.000000000000000000, 0.9659258262890683122, 1.000000000000000000, 0.9659258262890683122, 1.000000000000000000, 0.9659258262890683122, 1.000000000000000000, 0.9659258262890683122, 1.000000000000000000, 0.9659258262890683122, 1.000000000000000000, 0.9659258262890683122, 1.000000000000000000, 0.9659258262890683122, 1.000000000000000000, 0.9659258262890683122, 1.000000000000000000, 0.9659258262890683122, 1.000000000000000000, 0.9659258262890683122, 1.000000000000000000, 0.9659258262890683122, 1.000000000000000000, 0.9659258262890683122, 1.000000000000000000, 0.9659258262890683122, 1.000000000000000000, 0.9659258262890683122, 1.000000000000000000, 0.9659258262890683122, 1.000000000000000000, 0.9659258262890683122, 1.000000000000000000, 0.9659258262890683122, 1.000000000000000000, 0.9659258262890683122, 1.000000000000000000, 0.9659258262890683122, 1.000000000000000000, 0.9659258262890683122, 1.000000000000000000, 0.9659258262890683122, 1.000000000000000000, 0.9659258262890683122, 1.000000000000000000, 0.9659258262890683122, 1.000000000000000000, 0.9659258262890683122, 1.000000000000000000, 0.9659258262890683122, 1.000000000000000000, 0.9659258262890683122, 1.000000000000000000, 0.9659258262890683122, 1.000000000000000000, 0.9659258262890683122, 1.000000000000000000, 0.9659258262890683122, 1.000000000000000000, 0.9659258262890683122, 1.000000000000000000, 0.9659258262890683122, 1.000000000000000000, 0.9659258262890683122, 1.000000000000000000, 0.9659258262890683122, 1.000000000000000000, 0.9659258262890683122, 1.000000000000000000, 0.9659258262890683122, 1.000000000000000000, 0.9659258262890683122, 1.000000000000000000, 0.9659258262890683122, 1.000000000000000000, 0.9659258262890683122, 1.000000000000000000, 0.9659258262890683122, 1.000000000000000000, 0.9659258262890683122, 1.000000000000000000, 0.9659258262890683122, 1.000000000000000000, 0.9659258262890683122, 1.000000000000000000, 0.9659258262890683122, 1.000000000000000000, 0.9659258262890683122, 1.000000000000000000, 0.9659258262890683122, 1.000000000000000000, 0.9659258262890683122, 1.000000000000000000, 0.9659258262890683122, 1.000000000000000000, 0.9659258262890683122, 1.000000000000000000, 0.9659258262890683122, 1.000000000000000000, 0.9659258262890683122, 1.000000000000000000, 0.9659258262890683122, 1.000000000000000000, 0.9659258262890683122, 1.000000000000000000, 0.9659258262890683122, 1.000000000000000000, 0.9659258262890683122, 1.000000000000000000, 0.9659258262890683122, 1.000000000000000000, 0.9659258262890683122, 1.000000000000000000, 0.9659258262890683122, 1.000000000000000000, 0.9659258262890683122, 1.000000000000000000, 0.9659258262890683122, 1.000000000000000000, 0.9659258262890683122, 1.000000000000000000, 0.9659258262890683122, 1.000000000000000000, 0.9659258262890683122, 1.000000000000000000, 0.9659258262890683122, 1.000000000000000000, 0.9659258262890683122, 1.000000000000000000, 0.9659258262890683122, 1.000000000000000000, 0.9659258262890683122, 1.000000000000000000, 0.9659258262890683122, 1.000000000000000000, 0.9659258262890683122, 1.000000000000000000, 0.9659258262890683122, 1.000000000000000000, 0.9659258262890683122, 1.000000000000000000, 0.9659258262890683122, 1.000000000000000000, 0.9659258262890683122, 1.000000000000000000, 0.9659258262890683122, 1.000000000000000000, 0.9659258262890683122, 1.000000000000000000, 0.9659258262890683122, 1.000000000000000000, 0.9659258262890683122, 1.000000000000000000, 0.9659258262890683122, 1.000000000000000000, 0.9659258262890683122, 1.000000000000000000, 0.9659258262890683122, 1.000000000000000000, 0.9659258262890683122, 1.000000000000000000, 0.9659258262890683122, 1.000000000000000000, 0.9659258262890683122, 1.000000000000000000, 0.9659258262890683122, 1.000000000000000000, 0.9659258262890683122, 1.000000000000000000, 0.9659258262890683122, 1.000000000000000000, 0.9659258262890683122, 1.000000000000000000, 0.9659258262890683122, 1.000000000000000000, 0.9659258262890683122, 1.000000000000000000, 0.9659258262890683122, 1.000000000000000000, 0.9659258262890683122, 1.000000000000000000, 0.9659258262890683122, 1.000000000000000000, 0.9659258262890683122, 1.000000000000000000, 0.9659258262890683122, 1.000000000000000000, 0.9659258262890683122, 1.000000000000000000, 0.9659258262890683122, 1.000000000000000000, 0.9659258262890683122, 1.000000000000000000, 0.9659258262890683122, 1.000000000000000000, 0.9659258262890683122, 1.000000000000000000, 0.9659258262890683122, 1.000000000000000000, 0.9659258262890683122, 1.000000000000000000, 0.9659258262890683122, 1.000000000000000000, 0.9659258262890683122, 1.000000000000000000, 0.9659258262890683122, 1.000000000000000000, 0.9659258262890683122, 1.000000000000000000, 0.9659258262890683122, 1.000000000000000000, 0.9659258262890683122, 1.000000000000000000, 0.9659258262890683122, 1.000000000000000000, 0.9659258262890683122, 1.000000000000000000, 0.9659258262890683122, 1.000000000000000000, 0.9659258262890683122, 1.000000000000000000, 0.9659258262890683122, 1.000000000000000000, 0.9659258262890683122, 1.000000000000000000, 0.9659258262890683122, 1.000000000000000000, 0.9659258262890683122, 1.000000000000000000, 0.9659258262890683122, 1.000000000000000000, 0.9659258262890683122, 1.000000000000000000, 0.9659258262890683122, 1.000000000000000000, 0.9659258262890683122, 1.000000000000000000, 0.9659258262890683122, 1.000000000000000000, 0.9659258262890683122, 1.000000000000000000, 0.9659258262890683122, 1.000000000000000000, 0.9659258262890683122, 1.000000000000000000, 0.9659258262890683122, 1.000000000000000000, 0.9659258262890683122, 1.000000000000000000, 0.9659258262890683122, 1.000000000000000000, 0.9659258262890683122, 1.000000000000000000, 0.9659258262890683122, 1.000000000000000000, 0.9659258262890683122, 1.000000000000000000, 0.9659258262890683122, 1.000000000000000000, 0.9659258262890683122, 1.000000000000000000, 0.9659258262890683122, 1.000000000000000000, 0.9659258262890683122, 1.000000000000000000, 0.9659258262890683122, 1.000000000000000000, 0.9659258262890683122, 1.000000000000000000, 0.9659258262890683122, 1.000000000000000000, 0.9659258262890683122, 1.000000000000000000, 0.9659258262890683122, 1.000000000000000000, 0.9659258262890683122, 1.000000000000000000, 0.9659258262890683122, 1.000000000000000000, 0.9659258262890683122, 1.000000000000000000, 0.9659258262890683122, 1.000000000000000000, 0.9659258262890683122, 1.000000000000000000, 0.9659258262890683122, 1.000000000000000000, 0.9659258262890683122, 1.000000000000000000, 0.9659258262890683122, 1.000000000000000000, 0.9659258262890683122, 1.000000000000000000, 0.9659258262890683122, 1.000000000000000000, 0.9659258262890683122, 1.000000000000000000, 0.9659258262890683122, 1.000000000000000000, 0.9659258262890683122, 1.000000000000000000, 0.9659258262890683122, 1.000000000000000000, 0.9659258262890683122, 1.000000000000000000) ) ) 
 REPRESENTATION_ITEM ( '' )  SURFACE ( )  );
#82740=CARTESIAN_POINT ( 'NONE',  ( -12.06949235617739369, -12.14591786802326823, 24.37609039468567573 ) ) ;
#82741=CARTESIAN_POINT ( 'NONE',  ( 15.80617190586746368, 15.72974639402197994, 94.37390960531436690 ) ) ;
#82742=CARTESIAN_POINT ( 'NONE',  ( 5.823673210054125526, 21.52544592524343514, 69.79057627198102409 ) ) ;
#82743=CARTESIAN_POINT ( 'NONE',  ( 10.72451020669898902, -18.67979575497178502, 22.91557627198102765 ) ) ;
#82744=CARTESIAN_POINT ( 'NONE',  ( -12.06949235617739369, -12.14591786802326823, 39.37609039468567573 ) ) ;
#82745=CARTESIAN_POINT ( 'NONE',  ( 0.05219959533909260263, 19.03943276465977164, 54.99890960531435979 ) ) ;
#82746=CARTESIAN_POINT ( 'NONE',  ( -5.823673210054431948, 21.52544592524334988, 32.70942372801900433 ) ) ;
#82747=CARTESIAN_POINT ( 'NONE',  ( -9.564922557961040184, 16.46253265017147172, 97.91775706135233293 ) ) ;
#82748=CARTESIAN_POINT ( 'NONE',  ( 5.049401038298161559, -19.05341960407611168, 112.7072429386476813 ) ) ;
#82749=CARTESIAN_POINT ( 'NONE',  ( -0.05219959533909027116, -19.03943276465977164, 92.49890960531436690 ) ) ;
#82750=CARTESIAN_POINT ( 'NONE',  ( -21.53943276465977519, 0.05219959533907696930, 96.24890960531435269 ) ) ;
#82751=CARTESIAN_POINT ( 'NONE',  ( 13.97604488694527802, 13.89961937509977652, 59.37390960531434558 ) ) ;
#82752=CARTESIAN_POINT ( 'NONE',  ( -17.48847506799967277, -5.747544572773808369, 59.17302562156722701 ) ) ;
#82753=CARTESIAN_POINT ( 'NONE',  ( -8.224510206698948167, 14.34966873604960824, 70.41557627198102409 ) ) ;
#82754=CARTESIAN_POINT ( 'NONE',  ( 19.03943276465977164, -0.05219959533909143690, 103.7489096053143669 ) ) ;
#82756=CARTESIAN_POINT ( 'NONE',  ( -5.153800228976607833, 19.02544592524334988, 77.70942372801900433 ) ) ;
#82757=CARTESIAN_POINT ( 'NONE',  ( -5.823673210054116645, -21.52544592524344225, 87.29057627198103830 ) ) ;
#82758=CARTESIAN_POINT ( 'NONE',  ( 9.474510206698729675, 16.51473224551082808, 47.08442372801900433 ) ) ;
#82759=CARTESIAN_POINT ( 'NONE',  ( -10.81492255796078084, -18.62759615963271287, 22.08224293864769194 ) ) ;
#82761=CARTESIAN_POINT ( 'NONE',  ( -15.72974639402197994, 15.80617190586746368, 55.62390960531436690 ) ) ;
#82762=CARTESIAN_POINT ( 'NONE',  ( -19.05341960407611168, -5.049401038298163336, 91.45724293864766707 ) ) ;
#82763=CARTESIAN_POINT ( 'NONE',  ( -5.719274019375665041, -21.55341960407619695, 79.79275706135236135 ) ) ;
#82764=CARTESIAN_POINT ( 'NONE',  ( 19.05341960407611168, 5.049401038298154454, 43.95724293864769550 ) ) ;
#82765=CARTESIAN_POINT ( 'NONE',  ( 16.52544592524342804, -4.483927247898539470, 78.54057627198103830 ) ) ;
#82766=CARTESIAN_POINT ( 'NONE',  ( -8.224510206698735004, -14.34966873604973081, 19.58442372801901143 ) ) ;
#82767=CARTESIAN_POINT ( 'NONE',  ( -0.05219959533937732626, 21.53943276465977519, 62.50109039468568284 ) ) ;
#82768=ORIENTED_EDGE ( 'NONE', *, *, #52659, .F. ) ;
#82769=CARTESIAN_POINT ( 'NONE',  ( 0.05219959533936267826, -19.03943276465977164, 20.00109039468567218 ) ) ;
#82770=CARTESIAN_POINT ( 'NONE',  ( 9.474510206698729675, 16.51473224551082808, 82.08442372801899012 ) ) ;
#82772=CARTESIAN_POINT ( 'NONE',  ( 10.72451020669871369, 18.67979575497193778, 27.08442372801901854 ) ) ;
#82774=CARTESIAN_POINT ( 'NONE',  ( 0.05219959533936267826, -19.03943276465977164, 20.00109039468567218 ) ) ;
#82775=CARTESIAN_POINT ( 'NONE',  ( -13.97604488694527625, -13.89961937509977652, 61.87390960531435979 ) ) ;
#82776=CARTESIAN_POINT ( 'NONE',  ( -5.153800228976607833, 19.02544592524334988, 27.70942372801899722 ) ) ;
#82777=CARTESIAN_POINT ( 'NONE',  ( -0.05219959533934338120, 16.53943276465976808, 102.5010903946856899 ) ) ;
#82778=CARTESIAN_POINT ( 'NONE',  ( -5.153800228976328057, -19.02544592524343514, 97.29057627198099567 ) ) ;
#82779=CARTESIAN_POINT ( 'NONE',  ( -5.823673210054431948, 21.52544592524334988, 72.70942372801901854 ) ) ;
#82781=CARTESIAN_POINT ( 'NONE',  ( -17.49999999999995737, -3.565345528328239588, 35.57505513193538604 ) ) ;
#82782=CARTESIAN_POINT ( 'NONE',  ( -15.80617190586768217, 15.72974639402176855, 88.12609039468570415 ) ) ;
#82783=CARTESIAN_POINT ( 'NONE',  ( -0.05219959533937732626, 21.53943276465977519, 102.5010903946856899 ) ) ;
#82785=CARTESIAN_POINT ( 'NONE',  ( 13.97604488694527802, 13.89961937509977652, 99.37390960531436690 ) ) ;
#82786=CARTESIAN_POINT ( 'NONE',  ( 13.97604488694548053, -13.89961937509957401, 20.62609039468567573 ) ) ;
#82788=CARTESIAN_POINT ( 'NONE',  ( 19.03943276465977164, -0.05219959533909143690, 43.74890960531435979 ) ) ;
#82789=CARTESIAN_POINT ( 'NONE',  ( 21.55341960407610458, 5.719274019375980345, 58.95724293864770971 ) ) ;
#82790=CARTESIAN_POINT ( 'NONE',  ( 12.06949235617739724, 12.14591786802326823, 106.8760903946856899 ) ) ;
#82791=CARTESIAN_POINT ( 'NONE',  ( -16.53943276465976808, 0.05219959533911058130, 96.24890960531435269 ) ) ;
#82792=CARTESIAN_POINT ( 'NONE',  ( 5.153800228976335163, 19.02544592524342804, 74.79057627198103830 ) ) ;
#82793=CARTESIAN_POINT ( 'NONE',  ( -15.80617190586768217, 15.72974639402176855, 108.1260903946856757 ) ) ;
#82794=CARTESIAN_POINT ( 'NONE',  ( -13.97604488694527625, -13.89961937509977652, 36.87390960531436690 ) ) ;
#82795=CARTESIAN_POINT ( 'NONE',  ( 4.483927247898545687, 16.52544592524342804, 99.79057627198103830 ) ) ;
#82796=CARTESIAN_POINT ( 'NONE',  ( -5.823673210054431948, 21.52544592524334988, 57.70942372801901143 ) ) ;
#82797=CARTESIAN_POINT ( 'NONE',  ( 21.53943276465977519, -0.05219959533907433946, 83.74890960531435269 ) ) ;
#82798=CARTESIAN_POINT ( 'NONE',  ( 19.03943276465977164, 0.05219959533936151252, 51.25109039468567573 ) ) ;
#82800=CARTESIAN_POINT ( 'NONE',  ( 19.02544592524343514, -5.153800228976328945, 98.54057627198100988 ) ) ;
#82801=CARTESIAN_POINT ( 'NONE',  ( -16.55341960407611168, -4.379528057220339221, 81.45724293864769550 ) ) ;
#82803=CARTESIAN_POINT ( 'NONE',  ( -5.049401038297874678, -19.05341960407617918, 39.79275706135232582 ) ) ;
#82804=CARTESIAN_POINT ( 'NONE',  ( -19.02544592524342804, 5.153800228976336051, 61.04057627198103120 ) ) ;
#82805=CARTESIAN_POINT ( 'NONE',  ( -8.314922557960811034, -14.29746914071050412, 52.08224293864768839 ) ) ;
#82806=CARTESIAN_POINT ( 'NONE',  ( 0.05219959533936267826, -19.03943276465977164, 80.00109039468567573 ) ) ;
#82808=CARTESIAN_POINT ( 'NONE',  ( 10.72451020669898902, -18.67979575497178502, 37.91557627198102409 ) ) ;
#82809=CARTESIAN_POINT ( 'NONE',  ( 16.53943276465976808, -0.05219959533910856209, 103.7489096053143669 ) ) ;
#82811=CARTESIAN_POINT ( 'NONE',  ( -9.474510206698964154, 16.51473224551069663, 60.41557627198102409 ) ) ;
#82812=CARTESIAN_POINT ( 'NONE',  ( -15.72974639402197994, 15.80617190586746368, 60.62390960531437401 ) ) ;
#82813=CARTESIAN_POINT ( 'NONE',  ( 13.97604488694527802, 13.89961937509977652, 24.37390960531435624 ) ) ;
#82814=CARTESIAN_POINT ( 'NONE',  ( -12.14591786802326823, 12.06949235617739902, 83.12609039468568994 ) ) ;
#82815=CARTESIAN_POINT ( 'NONE',  ( -13.97604488694527625, -13.89961937509977652, 56.87390960531434558 ) ) ;
#82816=CARTESIAN_POINT ( 'NONE',  ( -19.05341960407617563, 5.049401038297882671, 48.54275706135233293 ) ) ;
#82817=CARTESIAN_POINT ( 'NONE',  ( -21.55341960407619339, 5.719274019375674811, 68.54275706135234714 ) ) ;
#82819=CARTESIAN_POINT ( 'NONE',  ( -21.52544592524343514, 5.823673210054127303, 56.04057627198102409 ) ) ;
#82820=CARTESIAN_POINT ( 'NONE',  ( 19.03943276465977164, -0.05219959533909143690, 23.74890960531435269 ) ) ;
#82821=CARTESIAN_POINT ( 'NONE',  ( -4.379528057220086978, -16.55341960407618274, 84.79275706135234714 ) ) ;
#82822=CARTESIAN_POINT ( 'NONE',  ( -5.049401038297874678, -19.05341960407617918, 109.7927570613523187 ) ) ;
#82824=CARTESIAN_POINT ( 'NONE',  ( 19.20446147854521968, 5.500000000000081712, 76.88999695167670723 ) ) ;
#82825=CARTESIAN_POINT ( 'NONE',  ( -21.55341960407610458, -5.719274019375992779, 56.45724293864768839 ) ) ;
#82826=CARTESIAN_POINT ( 'NONE',  ( -10.81492255796105439, 18.62759615963255655, 102.9177570613523756 ) ) ;
#82827=CARTESIAN_POINT ( 'NONE',  ( 16.53943276465976808, -0.05219959533910856209, 48.74890960531435979 ) ) ;
#82828=CARTESIAN_POINT ( 'NONE',  ( 4.379528057220339221, -16.55341960407611168, 52.70724293864769550 ) ) ;
#82829=CARTESIAN_POINT ( 'NONE',  ( -10.81492255796078084, -18.62759615963271287, 82.08224293864768129 ) ) ;
#82830=CARTESIAN_POINT ( 'NONE',  ( 21.52544592524344225, -5.823673210054117533, 93.54057627198103830 ) ) ;
#82832=CARTESIAN_POINT ( 'NONE',  ( -0.05219959533907301413, -21.53943276465977519, 27.49890960531435269 ) ) ;
#82834=CARTESIAN_POINT ( 'NONE',  ( -4.379528057220086978, -16.55341960407618274, 69.79275706135234714 ) ) ;
#82835=CARTESIAN_POINT ( 'NONE',  ( 16.52544592524342804, -4.483927247898539470, 73.54057627198102409 ) ) ;
#82836=CARTESIAN_POINT ( 'NONE',  ( -5.153800228976328057, -19.02544592524343514, 37.29057627198102409 ) ) ;
#82839=EDGE_CURVE ( 'NONE', #169831, #84227, #8600, .T. ) ;
#82840=CARTESIAN_POINT ( 'NONE',  ( 8.224510206698742110, 14.34966873604972548, 97.08442372801904696 ) ) ;
#82841=CARTESIAN_POINT ( 'NONE',  ( -0.05219959533907301413, -21.53943276465977519, 112.4989096053143669 ) ) ;
#82842=CARTESIAN_POINT ( 'NONE',  ( -19.03943276465977164, 0.05219959533909376836, 81.24890960531436690 ) ) ;
#82843=CARTESIAN_POINT ( 'NONE',  ( 10.81492255796106328, -18.62759615963255655, 60.41775706135235424 ) ) ;
#82844=CARTESIAN_POINT ( 'NONE',  ( 19.05341960407611168, 5.049401038298154454, 108.9572429386477097 ) ) ;
#82847=CARTESIAN_POINT ( 'NONE',  ( -21.55341960407619339, 5.719274019375674811, 43.54275706135235424 ) ) ;
#82848=CARTESIAN_POINT ( 'NONE',  ( 9.564922557960805705, 16.46253265017160317, 34.58224293864770260 ) ) ;
#82849=CARTESIAN_POINT ( 'NONE',  ( 16.46253265017160672, -9.564922557960803928, 98.33224293864769550 ) ) ;
#82850=CARTESIAN_POINT ( 'NONE',  ( -9.564922557961040184, 16.46253265017147172, 52.91775706135233293 ) ) ;
#82851=CARTESIAN_POINT ( 'NONE',  ( 10.81492255796106328, -18.62759615963255655, 25.41775706135235779 ) ) ;
#82852=CARTESIAN_POINT ( 'NONE',  ( 5.049401038297881783, 19.05341960407617563, 62.29275706135234003 ) ) ;
#82854=CARTESIAN_POINT ( 'NONE',  ( 16.52544592524335698, 4.483927247898782831, 91.45942372801901854 ) ) ;
#82855=CARTESIAN_POINT ( 'NONE',  ( -19.03943276465977164, -0.05219959533935918106, 63.75109039468566863 ) ) ;
#82856=CARTESIAN_POINT ( 'NONE',  ( 16.55341960407618274, -4.379528057220086978, 101.0427570613523756 ) ) ;
#82859=CARTESIAN_POINT ( 'NONE',  ( 9.564922557960805705, 16.46253265017160317, 84.58224293864769550 ) ) ;
#82861=CARTESIAN_POINT ( 'NONE',  ( 15.80617190586769283, -15.72974639402175789, 95.62609039468568994 ) ) ;
#82862=CARTESIAN_POINT ( 'NONE',  ( 5.719274019375673035, 21.55341960407619339, 112.2927570613523471 ) ) ;
#82864=CARTESIAN_POINT ( 'NONE',  ( 5.153800228976335163, 19.02544592524342804, 94.79057627198103830 ) ) ;
#82865=CARTESIAN_POINT ( 'NONE',  ( 0.05219959533937995610, -21.53943276465977519, 80.00109039468568994 ) ) ;
#82866=CARTESIAN_POINT ( 'NONE',  ( 12.14591786802327356, -12.06949235617739191, 25.62609039468567929 ) ) ;
#82867=CARTESIAN_POINT ( 'NONE',  ( 13.97604488694527802, 13.89961937509977652, 79.37390960531435269 ) ) ;
#82868=CARTESIAN_POINT ( 'NONE',  ( -15.72974639402197994, 15.80617190586746368, 35.62390960531437401 ) ) ;
#82869=CARTESIAN_POINT ( 'NONE',  ( -5.049401038298153566, 19.05341960407611168, 95.20724293864770971 ) ) ;
#82871=CARTESIAN_POINT ( 'NONE',  ( 5.153800228976335163, 19.02544592524342804, 74.79057627198103830 ) ) ;
#82872=CARTESIAN_POINT ( 'NONE',  ( -9.474510206698964154, 16.51473224551069663, 65.41557627198102409 ) ) ;
#82873=CARTESIAN_POINT ( 'NONE',  ( 0.05219959533910956823, 16.53943276465976808, 24.99890960531435624 ) ) ;
#82875=CARTESIAN_POINT ( 'NONE',  ( 19.03943276465977164, 0.05219959533936151252, 71.25109039468566152 ) ) ;
#82876=CARTESIAN_POINT ( 'NONE',  ( -5.153800228976328057, -19.02544592524343514, 97.29057627198099567 ) ) ;
#82877=CARTESIAN_POINT ( 'NONE',  ( 16.52544592524342804, -4.483927247898539470, 83.54057627198102409 ) ) ;
#82878=CARTESIAN_POINT ( 'NONE',  ( -18.67979575497178146, -10.72451020669898902, 41.66557627198103120 ) ) ;
#82879=CARTESIAN_POINT ( 'NONE',  ( -18.67979575497178146, -10.72451020669898902, 26.66557627198103475 ) ) ;
#82880=CARTESIAN_POINT ( 'NONE',  ( 0.05219959533910956823, 16.53943276465976808, 99.99890960531436690 ) ) ;
#82882=CARTESIAN_POINT ( 'NONE',  ( -19.03943276465977164, -0.05219959533935918106, 43.75109039468566863 ) ) ;
#82883=CARTESIAN_POINT ( 'NONE',  ( 4.483927247898545687, 16.52544592524342804, 24.79057627198103120 ) ) ;
#82884=CARTESIAN_POINT ( 'NONE',  ( -9.474510206698964154, 16.51473224551069663, 105.4155762719810383 ) ) ;
#82885=CARTESIAN_POINT ( 'NONE',  ( 21.55341960407619695, -5.719274019375665929, 61.04275706135234714 ) ) ;
#82886=CARTESIAN_POINT ( 'NONE',  ( 18.62759615963271287, -10.81492255796078972, 63.33224293864770260 ) ) ;
#82887=CARTESIAN_POINT ( 'NONE',  ( 15.72974639402176855, 15.80617190586768217, 51.87609039468568284 ) ) ;
#82888=CARTESIAN_POINT ( 'NONE',  ( 5.719274019375991003, -21.55341960407610458, 77.70724293864770971 ) ) ;
#82889=CARTESIAN_POINT ( 'NONE',  ( 5.719274019375673035, 21.55341960407619339, 42.29275706135235424 ) ) ;
#82890=CARTESIAN_POINT ( 'NONE',  ( 16.55341960407611168, 4.379528057220329451, 108.9572429386476955 ) ) ;
#82891=CARTESIAN_POINT ( 'NONE',  ( -5.049401038297874678, -19.05341960407617918, 64.79275706135233293 ) ) ;
#82892=CARTESIAN_POINT ( 'NONE',  ( -19.02544592524342804, 5.153800228976336051, 46.04057627198101699 ) ) ;
#82893=CARTESIAN_POINT ( 'NONE',  ( 0.05219959533910956823, 16.53943276465976808, 104.9989096053143669 ) ) ;
#82894=CARTESIAN_POINT ( 'NONE',  ( 0.05219959533909260263, 19.03943276465977164, 104.9989096053143669 ) ) ;
#82895=CARTESIAN_POINT ( 'NONE',  ( 16.53943276465976808, -0.05219959533910856209, 43.74890960531435979 ) ) ;
#82896=CARTESIAN_POINT ( 'NONE',  ( -14.29746914071037622, -8.314922557961029526, 104.1677570613523471 ) ) ;
#82897=CARTESIAN_POINT ( 'NONE',  ( -13.89961937509977652, 13.97604488694528158, 55.62390960531434558 ) ) ;
#82898=CARTESIAN_POINT ( 'NONE',  ( -0.05219959533910754901, -16.53943276465976808, 112.4989096053143669 ) ) ;
#82899=CARTESIAN_POINT ( 'NONE',  ( -16.46253265017146816, -9.564922557961047289, 24.16775706135233648 ) ) ;
#82900=CARTESIAN_POINT ( 'NONE',  ( -9.564922557960796823, -16.46253265017161027, 112.0822429386476955 ) ) ;
#82901=CARTESIAN_POINT ( 'NONE',  ( -8.224510206698948167, 14.34966873604960824, 40.41557627198103120 ) ) ;
#82902=CARTESIAN_POINT ( 'NONE',  ( 21.52544592524334988, 5.823673210054432836, 46.45942372801901854 ) ) ;
#82903=CARTESIAN_POINT ( 'NONE',  ( -19.02544592524342804, 5.153800228976336051, 116.0405762719810383 ) ) ;
#82904=CARTESIAN_POINT ( 'NONE',  ( -8.314922557961024197, 14.29746914071037800, 57.91775706135234714 ) ) ;
#82905=EDGE_CURVE ( 'NONE', #47253, #60866, #34561, .T. ) ;
#82906=CARTESIAN_POINT ( 'NONE',  ( 8.224510206698953496, -14.34966873604960469, 27.91557627198103830 ) ) ;
#82907=CARTESIAN_POINT ( 'NONE',  ( 14.29746914071037800, 8.314922557961029526, 106.6677570613523756 ) ) ;
#82908=CARTESIAN_POINT ( 'NONE',  ( -14.29746914071037622, -8.314922557961029526, 24.16775706135235424 ) ) ;
#82909=CARTESIAN_POINT ( 'NONE',  ( -19.05341960407611168, -5.049401038298163336, 51.45724293864770260 ) ) ;
#82910=CARTESIAN_POINT ( 'NONE',  ( 16.55341960407611168, 4.379528057220329451, 108.9572429386476955 ) ) ;
#82911=CARTESIAN_POINT ( 'NONE',  ( -21.52544592524334988, -5.823673210054445271, 23.95942372801901143 ) ) ;
#82912=CARTESIAN_POINT ( 'NONE',  ( -5.049401038298153566, 19.05341960407611168, 40.20724293864768839 ) ) ;
#82913=CARTESIAN_POINT ( 'NONE',  ( 9.474510206698971260, -16.51473224551069308, 112.9155762719810383 ) ) ;
#82914=CARTESIAN_POINT ( 'NONE',  ( 16.46253265017160672, -9.564922557960803928, 28.33224293864769550 ) ) ;
#82915=CARTESIAN_POINT ( 'NONE',  ( 19.05341960407611168, 5.049401038298154454, 113.9572429386477097 ) ) ;
#82916=CARTESIAN_POINT ( 'NONE',  ( -17.26058549869092573, -6.457015423128558140, 36.37745837476068544 ) ) ;
#82918=CARTESIAN_POINT ( 'NONE',  ( -9.564922557960796823, -16.46253265017161027, 102.0822429386477097 ) ) ;
#82919=CARTESIAN_POINT ( 'NONE',  ( -21.55341960407619339, 5.719274019375674811, 48.54275706135234714 ) ) ;
#82920=CARTESIAN_POINT ( 'NONE',  ( -12.14591786802309592, -12.06949235617757132, 106.8739096053143811 ) ) ;
#82921=CARTESIAN_POINT ( 'NONE',  ( 19.05341960407611168, 5.049401038298154454, 108.9572429386477097 ) ) ;
#82922=CARTESIAN_POINT ( 'NONE',  ( 0.05219959533936267826, -19.03943276465977164, 70.00109039468566152 ) ) ;
#82923=CARTESIAN_POINT ( 'NONE',  ( 8.314922557961029526, -14.29746914071037800, 75.41775706135233293 ) ) ;
#82924=CARTESIAN_POINT ( 'NONE',  ( -15.80617190586768217, 15.72974639402176855, 93.12609039468568994 ) ) ;
#82925=CARTESIAN_POINT ( 'NONE',  ( 4.379528057220092307, 16.55341960407617563, 57.29275706135234714 ) ) ;
#82926=CARTESIAN_POINT ( 'NONE',  ( -9.564922557960796823, -16.46253265017161027, 97.08224293864769550 ) ) ;
#82927=CARTESIAN_POINT ( 'NONE',  ( 14.29746914071037800, 8.314922557961029526, 41.66775706135235424 ) ) ;
#82928=CARTESIAN_POINT ( 'NONE',  ( -0.05219959533934338120, 16.53943276465976808, 32.50109039468568284 ) ) ;
#82929=CARTESIAN_POINT ( 'NONE',  ( -4.483927247898782831, 16.52544592524335698, 77.70942372801900433 ) ) ;
#82930=CARTESIAN_POINT ( 'NONE',  ( -0.05219959533936034679, 19.03943276465977164, 107.5010903946856615 ) ) ;
#82931=CARTESIAN_POINT ( 'NONE',  ( 9.474510206698971260, -16.51473224551069308, 77.91557627198103830 ) ) ;
#82932=CARTESIAN_POINT ( 'NONE',  ( -5.823673210054116645, -21.52544592524344225, 92.29057627198103830 ) ) ;
#82933=CARTESIAN_POINT ( 'NONE',  ( -8.224510206698948167, 14.34966873604960824, 105.4155762719810383 ) ) ;
#82934=CARTESIAN_POINT ( 'NONE',  ( -13.89961937509957401, -13.97604488694547875, 109.3760903946856331 ) ) ;
#82935=CARTESIAN_POINT ( 'NONE',  ( -4.379528057220086978, -16.55341960407618274, 69.79275706135234714 ) ) ;
#82936=CARTESIAN_POINT ( 'NONE',  ( -16.52216118717247895, 7.221426719304377073, 43.92400978952973389 ) ) ;
#82937=CARTESIAN_POINT ( 'NONE',  ( -16.46253265017146816, -9.564922557961047289, 69.16775706135233293 ) ) ;
#82938=CARTESIAN_POINT ( 'NONE',  ( -8.224510206698948167, 14.34966873604960824, 50.41557627198103120 ) ) ;
#82939=CARTESIAN_POINT ( 'NONE',  ( 14.29746914071049879, -8.314922557960816363, 93.33224293864769550 ) ) ;
#82940=CARTESIAN_POINT ( 'NONE',  ( -13.89961937509957401, -13.97604488694547875, 39.37609039468566152 ) ) ;
#82941=CARTESIAN_POINT ( 'NONE',  ( -16.52216118717206683, 7.221426719304492536, 88.92400978953007495 ) ) ;
#82942=CARTESIAN_POINT ( 'NONE',  ( -10.72451020669870658, -18.67979575497194134, 34.58442372801900433 ) ) ;
#82943=CARTESIAN_POINT ( 'NONE',  ( 5.153800228976615827, -19.02544592524334988, 95.20942372801897591 ) ) ;
#82944=CARTESIAN_POINT ( 'NONE',  ( -9.564922557960796823, -16.46253265017161027, 112.0822429386476955 ) ) ;
#82945=CARTESIAN_POINT ( 'NONE',  ( -16.46253265017160317, 9.564922557960807481, 95.83224293864769550 ) ) ;
#82946=CARTESIAN_POINT ( 'NONE',  ( 10.72451020669871369, 18.67979575497193778, 107.0844237280190043 ) ) ;
#82947=CARTESIAN_POINT ( 'NONE',  ( 5.049401038298161559, -19.05341960407611168, 77.70724293864765286 ) ) ;
#82948=CARTESIAN_POINT ( 'NONE',  ( 0.05219959533907565091, 21.53943276465977519, 44.99890960531435979 ) ) ;
#82949=CARTESIAN_POINT ( 'NONE',  ( -4.483927247898539470, -16.52544592524342804, 97.29057627198105251 ) ) ;
#82950=CARTESIAN_POINT ( 'NONE',  ( 5.049401038298161559, -19.05341960407611168, 57.70724293864769550 ) ) ;
#82951=CARTESIAN_POINT ( 'NONE',  ( -14.29746914071049879, 8.314922557960819915, 110.8322429386476955 ) ) ;
#82953=CARTESIAN_POINT ( 'NONE',  ( 15.80617190586769283, -15.72974639402175789, 20.62609039468568639 ) ) ;
#82954=CARTESIAN_POINT ( 'NONE',  ( 10.72451020669871369, 18.67979575497193778, 82.08442372801901854 ) ) ;
#82955=CARTESIAN_POINT ( 'NONE',  ( 19.02544592524343514, -5.153800228976328945, 48.54057627198103120 ) ) ;
#82956=CARTESIAN_POINT ( 'NONE',  ( -16.52544592524335698, -4.483927247898792601, 78.95942372801901854 ) ) ;
#82957=CARTESIAN_POINT ( 'NONE',  ( -21.52544592524343514, 5.823673210054127303, 116.0405762719810383 ) ) ;
#82959=CARTESIAN_POINT ( 'NONE',  ( 21.52544592524334988, 5.823673210054432836, 31.45942372801901854 ) ) ;
#82960=CARTESIAN_POINT ( 'NONE',  ( -16.51473224551082808, 9.474510206698731452, 58.33442372801900433 ) ) ;
#82961=CARTESIAN_POINT ( 'NONE',  ( 16.46253265017160672, -9.564922557960803928, 63.33224293864769550 ) ) ;
#82962=CARTESIAN_POINT ( 'NONE',  ( 9.564922557961047289, -16.46253265017146816, 35.41775706135233293 ) ) ;
#82963=CARTESIAN_POINT ( 'NONE',  ( 10.81492255796106328, -18.62759615963255655, 65.41775706135234714 ) ) ;
#82964=CARTESIAN_POINT ( 'NONE',  ( -10.72451020669898014, 18.67979575497178502, 75.41557627198102409 ) ) ;
#82965=CARTESIAN_POINT ( 'NONE',  ( -4.379528057220328563, 16.55341960407611168, 55.20724293864770260 ) ) ;
#82966=CARTESIAN_POINT ( 'NONE',  ( 15.72974639402176855, 15.80617190586768217, 86.87609039468568994 ) ) ;
#82967=CARTESIAN_POINT ( 'NONE',  ( -5.153800228976607833, 19.02544592524334988, 32.70942372801899722 ) ) ;
#82968=CARTESIAN_POINT ( 'NONE',  ( -8.314922557960811034, -14.29746914071050412, 77.08224293864769550 ) ) ;
#82969=CARTESIAN_POINT ( 'NONE',  ( -12.06949235617756955, 12.14591786802309770, 115.6239096053143669 ) ) ;
#82970=CARTESIAN_POINT ( 'NONE',  ( 16.51473224551083163, -9.474510206698727899, 60.83442372801900433 ) ) ;
#82971=CARTESIAN_POINT ( 'NONE',  ( 8.224510206698953496, -14.34966873604960469, 27.91557627198103830 ) ) ;
#82973=CARTESIAN_POINT ( 'NONE',  ( 5.719274019375673035, 21.55341960407619339, 77.29275706135234714 ) ) ;
#82974=CARTESIAN_POINT ( 'NONE',  ( -0.05219959533909027116, -19.03943276465977164, 77.49890960531435269 ) ) ;
#82975=CARTESIAN_POINT ( 'NONE',  ( -16.51473224551082808, 9.474510206698731452, 48.33442372801900433 ) ) ;
#82976=CARTESIAN_POINT ( 'NONE',  ( -21.55341960407610458, -5.719274019375992779, 51.45724293864770260 ) ) ;
#82977=CARTESIAN_POINT ( 'NONE',  ( -10.72451020669870658, -18.67979575497194134, 44.58442372801901854 ) ) ;
#82978=CARTESIAN_POINT ( 'NONE',  ( 10.72451020669898902, -18.67979575497178502, 102.9155762719810383 ) ) ;
#82979=CARTESIAN_POINT ( 'NONE',  ( -5.153800228976607833, 19.02544592524334988, 92.70942372801901854 ) ) ;
#82980=CARTESIAN_POINT ( 'NONE',  ( 0.05219959533934541429, -16.53943276465976808, 60.00109039468568284 ) ) ;
#82981=DIRECTION ( 'NONE',  ( 0.000000000000000000, 0.000000000000000000, 1.000000000000000000 ) ) ;
#82982=CARTESIAN_POINT ( 'NONE',  ( 10.72451020669898902, -18.67979575497178502, 107.9155762719810241 ) ) ;
#82983=CARTESIAN_POINT ( 'NONE',  ( 16.55341960407611168, 4.379528057220329451, 88.95724293864769550 ) ) ;
#82984=CARTESIAN_POINT ( 'NONE',  ( -17.49999999999999289, -3.471454075611644541, 30.51667418855634395 ) ) ;
#82985=CARTESIAN_POINT ( 'NONE',  ( 8.224510206698742110, 14.34966873604972548, 37.08442372801901143 ) ) ;
#82986=CARTESIAN_POINT ( 'NONE',  ( 21.55341960407610458, 5.719274019375980345, 43.95724293864769550 ) ) ;
#82987=CARTESIAN_POINT ( 'NONE',  ( -16.53943276465976808, -0.05219959533934237506, 93.75109039468567573 ) ) ;
#82988=CARTESIAN_POINT ( 'NONE',  ( -19.03943276465977164, 0.05219959533909376836, 26.24890960531435624 ) ) ;
#82989=CARTESIAN_POINT ( 'NONE',  ( 0.05219959533934541429, -16.53943276465976808, 60.00109039468568284 ) ) ;
#82990=CARTESIAN_POINT ( 'NONE',  ( -21.55341960407619339, 5.719274019375674811, 38.54275706135234714 ) ) ;
#82991=CARTESIAN_POINT ( 'NONE',  ( -10.81492255796078084, -18.62759615963271287, 52.08224293864768839 ) ) ;
#82992=CARTESIAN_POINT ( 'NONE',  ( -8.224510206698735004, -14.34966873604973081, 84.58442372801903275 ) ) ;
#82993=CARTESIAN_POINT ( 'NONE',  ( 10.72451020669871369, 18.67979575497193778, 67.08442372801901854 ) ) ;
#82994=CARTESIAN_POINT ( 'NONE',  ( -5.719274019375978568, 21.55341960407610458, 50.20724293864769550 ) ) ;
#82995=CARTESIAN_POINT ( 'NONE',  ( -0.05219959533907301413, -21.53943276465977519, 37.49890960531436690 ) ) ;
#82997=CARTESIAN_POINT ( 'NONE',  ( 16.55341960407618274, -4.379528057220086978, 61.04275706135234714 ) ) ;
#82998=CARTESIAN_POINT ( 'NONE',  ( 10.72451020669898902, -18.67979575497178502, 37.91557627198102409 ) ) ;
#82999=VERTEX_POINT ( 'NONE', #161444 ) ;
#83000=CARTESIAN_POINT ( 'NONE',  ( 13.97604488694527802, 13.89961937509977652, 94.37390960531436690 ) ) ;
#83001=CARTESIAN_POINT ( 'NONE',  ( 16.55341960407611168, 4.379528057220329451, 23.95724293864769550 ) ) ;
#83003=CARTESIAN_POINT ( 'NONE',  ( 4.483927247898545687, 16.52544592524342804, 114.7905762719810383 ) ) ;
#83004=CARTESIAN_POINT ( 'NONE',  ( -15.72974639402197994, 15.80617190586746368, 60.62390960531437401 ) ) ;
#83005=CARTESIAN_POINT ( 'NONE',  ( 16.51473224551069308, 9.474510206698969483, 39.16557627198103120 ) ) ;
#83006=CARTESIAN_POINT ( 'NONE',  ( -12.06949235617739369, -12.14591786802326823, 89.37609039468568994 ) ) ;
#83007=CARTESIAN_POINT ( 'NONE',  ( -5.719274019375665041, -21.55341960407619695, 29.79275706135234358 ) ) ;
#83008=CARTESIAN_POINT ( 'NONE',  ( 5.049401038297881783, 19.05341960407617563, 87.29275706135234714 ) ) ;
#83009=CARTESIAN_POINT ( 'NONE',  ( 12.06949235617757843, -12.14591786802309237, 98.12390960531436690 ) ) ;
#83010=CARTESIAN_POINT ( 'NONE',  ( -0.05219959533909027116, -19.03943276465977164, 47.49890960531435979 ) ) ;
#83011=CARTESIAN_POINT ( 'NONE',  ( -19.03943276465977164, 0.05219959533909376836, 21.24890960531436335 ) ) ;
#83013=CARTESIAN_POINT ( 'NONE',  ( -19.05341960407611168, -5.049401038298163336, 76.45724293864769550 ) ) ;
#83014=CARTESIAN_POINT ( 'NONE',  ( 4.379528057220092307, 16.55341960407617563, 62.29275706135236845 ) ) ;
#83015=CARTESIAN_POINT ( 'NONE',  ( 15.80617190586769283, -15.72974639402175789, 105.6260903946856899 ) ) ;
#83016=CARTESIAN_POINT ( 'NONE',  ( -5.719274019375978568, 21.55341960407610458, 45.20724293864769550 ) ) ;
#83018=CARTESIAN_POINT ( 'NONE',  ( -8.314922557961024197, 14.29746914071037800, 72.91775706135234714 ) ) ;
#83019=CARTESIAN_POINT ( 'NONE',  ( 16.51473224551083163, -9.474510206698727899, 65.83442372801900433 ) ) ;
#83020=CARTESIAN_POINT ( 'NONE',  ( -18.62759615963255300, -10.81492255796106328, 59.16775706135234714 ) ) ;
#83021=CARTESIAN_POINT ( 'NONE',  ( 5.049401038298161559, -19.05341960407611168, 72.70724293864768129 ) ) ;
#83022=CARTESIAN_POINT ( 'NONE',  ( 13.89961937509977652, -13.97604488694527269, 33.12390960531434558 ) ) ;
#83023=CARTESIAN_POINT ( 'NONE',  ( 19.05341960407617918, -5.049401038297876454, 56.04275706135234714 ) ) ;
#83024=CARTESIAN_POINT ( 'NONE',  ( -5.049401038298153566, 19.05341960407611168, 110.2072429386476671 ) ) ;
#83025=CARTESIAN_POINT ( 'NONE',  ( 5.049401038298161559, -19.05341960407611168, 97.70724293864766707 ) ) ;
#83026=CARTESIAN_POINT ( 'NONE',  ( 8.314922557960818139, 14.29746914071049879, 49.58224293864769550 ) ) ;
#83027=CARTESIAN_POINT ( 'NONE',  ( 18.62759615963271287, -10.81492255796078972, 53.33224293864769550 ) ) ;
#83029=CARTESIAN_POINT ( 'NONE',  ( 19.03943276465977164, 0.05219959533936151252, 26.25109039468566507 ) ) ;
#83030=CARTESIAN_POINT ( 'NONE',  ( -17.05116617787825462, -6.768360034955808402, 81.34324446740802728 ) ) ;
#83031=CARTESIAN_POINT ( 'NONE',  ( 9.564922557960805705, 16.46253265017160317, 54.58224293864769550 ) ) ;
#83032=CARTESIAN_POINT ( 'NONE',  ( 16.52544592524335698, 4.483927247898782831, 41.45942372801901143 ) ) ;
#83035=CARTESIAN_POINT ( 'NONE',  ( 12.14591786802327356, -12.06949235617739191, 75.62609039468567573 ) ) ;
#83036=CARTESIAN_POINT ( 'NONE',  ( -15.80617190586745835, -15.72974639402198527, 101.8739096053143811 ) ) ;
#83037=CARTESIAN_POINT ( 'NONE',  ( -19.02544592524342804, 5.153800228976336051, 36.04057627198100988 ) ) ;
#83039=CARTESIAN_POINT ( 'NONE',  ( 10.81492255796106328, -18.62759615963255655, 40.41775706135234714 ) ) ;
#83040=CARTESIAN_POINT ( 'NONE',  ( -5.049401038297874678, -19.05341960407617918, 44.79275706135232582 ) ) ;
#83041=CARTESIAN_POINT ( 'NONE',  ( 19.02544592524343514, -5.153800228976328945, 48.54057627198103120 ) ) ;
#83042=CARTESIAN_POINT ( 'NONE',  ( 5.719274019375673035, 21.55341960407619339, 92.29275706135236135 ) ) ;
#83043=CARTESIAN_POINT ( 'NONE',  ( 17.31728774477274868, 6.344390552232392899, 96.68093348310684121 ) ) ;
#83044=CARTESIAN_POINT ( 'NONE',  ( 0.05219959533910956823, 16.53943276465976808, 34.99890960531435979 ) ) ;
#83046=CARTESIAN_POINT ( 'NONE',  ( -15.72974639402197994, 15.80617190586746368, 50.62390960531435979 ) ) ;
#83049=CARTESIAN_POINT ( 'NONE',  ( 16.51473224551069308, 9.474510206698969483, 99.16557627198102409 ) ) ;
#83050=CARTESIAN_POINT ( 'NONE',  ( -16.55341960407611168, -4.379528057220339221, 106.4572429386477097 ) ) ;
#83051=CARTESIAN_POINT ( 'NONE',  ( 4.483927247898790824, -16.52544592524335698, 20.20942372801900788 ) ) ;
#83052=CARTESIAN_POINT ( 'NONE',  ( -12.06949235617739369, -12.14591786802326823, 104.3760903946856899 ) ) ;
#83054=CARTESIAN_POINT ( 'NONE',  ( -9.564922557960796823, -16.46253265017161027, 102.0822429386477097 ) ) ;
#83055=CARTESIAN_POINT ( 'NONE',  ( -18.67979575497178146, -10.72451020669898902, 101.6655762719810383 ) ) ;
#83056=CARTESIAN_POINT ( 'NONE',  ( -14.34966873604960291, -8.224510206698953496, 26.66557627198103475 ) ) ;
#83057=CARTESIAN_POINT ( 'NONE',  ( 13.89961937509977652, -13.97604488694527269, 103.1239096053143527 ) ) ;
#83058=CARTESIAN_POINT ( 'NONE',  ( -13.97604488694547697, 13.89961937509957934, 98.12609039468566152 ) ) ;
#83059=CARTESIAN_POINT ( 'NONE',  ( -5.719274019375665041, -21.55341960407619695, 109.7927570613523613 ) ) ;
#83060=CARTESIAN_POINT ( 'NONE',  ( -15.80617190586745835, -15.72974639402198527, 91.87390960531436690 ) ) ;
#83061=CARTESIAN_POINT ( 'NONE',  ( -10.72451020669898014, 18.67979575497178502, 55.41557627198102409 ) ) ;
#83062=CARTESIAN_POINT ( 'NONE',  ( -19.05341960407611168, -5.049401038298163336, 66.45724293864769550 ) ) ;
#83063=CARTESIAN_POINT ( 'NONE',  ( -16.52544592524342804, 4.483927247898546575, 36.04057627198102409 ) ) ;
#83064=CARTESIAN_POINT ( 'NONE',  ( -9.474510206698964154, 16.51473224551069663, 80.41557627198103830 ) ) ;
#83065=CARTESIAN_POINT ( 'NONE',  ( 19.20446147854530139, 5.499999999999904965, 56.88999695167677828 ) ) ;
#83066=CARTESIAN_POINT ( 'NONE',  ( 19.03943276465977164, 0.05219959533936151252, 36.25109039468567573 ) ) ;
#83067=CARTESIAN_POINT ( 'NONE',  ( -10.72451020669898014, 18.67979575497178502, 85.41557627198102409 ) ) ;
#83068=CARTESIAN_POINT ( 'NONE',  ( -12.06949235617756955, 12.14591786802309770, 80.62390960531438111 ) ) ;
#83069=CARTESIAN_POINT ( 'NONE',  ( -0.05219959533937732626, 21.53943276465977519, 37.50109039468568284 ) ) ;
#83072=CARTESIAN_POINT ( 'NONE',  ( 0.05219959533934541429, -16.53943276465976808, 105.0010903946856757 ) ) ;
#83073=CARTESIAN_POINT ( 'NONE',  ( -19.03943276465977164, 0.05219959533909376836, 26.24890960531435624 ) ) ;
#83074=CARTESIAN_POINT ( 'NONE',  ( 19.03943276465977164, -0.05219959533909143690, 83.74890960531436690 ) ) ;
#83075=DIRECTION ( 'NONE',  ( 1.000000000000000000, 0.000000000000000000, 0.000000000000000000 ) ) ;
#83077=CARTESIAN_POINT ( 'NONE',  ( 14.34966873604960469, 8.224510206698951720, 39.16557627198102409 ) ) ;
#83078=CARTESIAN_POINT ( 'NONE',  ( -21.55341960407619339, 5.719274019375674811, 63.54275706135234003 ) ) ;
#83080=CARTESIAN_POINT ( 'NONE',  ( 5.153800228976335163, 19.02544592524342804, 39.79057627198100988 ) ) ;
#83081=CARTESIAN_POINT ( 'NONE',  ( -9.564922557960796823, -16.46253265017161027, 57.08224293864769550 ) ) ;
#83083=CARTESIAN_POINT ( 'NONE',  ( 18.62759615963255655, 10.81492255796105972, 111.6677570613523613 ) ) ;
#83084=CARTESIAN_POINT ( 'NONE',  ( -12.06949235617739369, -12.14591786802326823, 59.37609039468568284 ) ) ;
#83085=CARTESIAN_POINT ( 'NONE',  ( -18.67979575497193778, 10.72451020669871902, 88.33442372801901854 ) ) ;
#83086=CARTESIAN_POINT ( 'NONE',  ( 5.823673210054125526, 21.52544592524343514, 24.79057627198103120 ) ) ;
#83087=CARTESIAN_POINT ( 'NONE',  ( -19.03943276465977164, -0.05219959533935918106, 98.75109039468567573 ) ) ;
#83088=CARTESIAN_POINT ( 'NONE',  ( 5.719274019375673035, 21.55341960407619339, 72.29275706135236135 ) ) ;
#83089=CARTESIAN_POINT ( 'NONE',  ( 0.05219959533934541429, -16.53943276465976808, 30.00109039468568284 ) ) ;
#83090=CARTESIAN_POINT ( 'NONE',  ( 10.72451020669898902, -18.67979575497178502, 82.91557627198103830 ) ) ;
#83091=CARTESIAN_POINT ( 'NONE',  ( -5.049401038297874678, -19.05341960407617918, 94.79275706135230450 ) ) ;
#83092=CARTESIAN_POINT ( 'NONE',  ( -5.049401038298153566, 19.05341960407611168, 60.20724293864768129 ) ) ;
#83093=CARTESIAN_POINT ( 'NONE',  ( -16.53943276465976808, -0.05219959533934237506, 18.75109039468568639 ) ) ;
#83095=CARTESIAN_POINT ( 'NONE',  ( 16.46253265017146816, 9.564922557961045513, 101.6677570613523329 ) ) ;
#83096=CARTESIAN_POINT ( 'NONE',  ( 4.483927247898545687, 16.52544592524342804, 49.79057627198102409 ) ) ;
#83097=CARTESIAN_POINT ( 'NONE',  ( -16.46253265017146816, -9.564922557961047289, 74.16775706135234714 ) ) ;
#83098=CARTESIAN_POINT ( 'NONE',  ( 4.379528057220092307, 16.55341960407617563, 62.29275706135236845 ) ) ;
#83099=CARTESIAN_POINT ( 'NONE',  ( -0.05219959533937732626, 21.53943276465977519, 22.50109039468567573 ) ) ;
#83100=CARTESIAN_POINT ( 'NONE',  ( 9.474510206698971260, -16.51473224551069308, 42.91557627198103120 ) ) ;
#83101=CARTESIAN_POINT ( 'NONE',  ( 0.05219959533909260263, 19.03943276465977164, 49.99890960531435979 ) ) ;
#83103=CARTESIAN_POINT ( 'NONE',  ( -14.34966873604972548, 8.224510206698743886, 53.33442372801901854 ) ) ;
#83106=CARTESIAN_POINT ( 'NONE',  ( -16.46253265017160317, 9.564922557960807481, 110.8322429386476955 ) ) ;
#83107=DIRECTION ( 'NONE',  ( 0.000000000000000000, 0.04175967627138096189, 0.9991276842514722478 ) ) ;
#83109=CARTESIAN_POINT ( 'NONE',  ( -12.06949235617739369, -12.14591786802326823, 19.37609039468568639 ) ) ;
#83110=CARTESIAN_POINT ( 'NONE',  ( 5.719274019375991003, -21.55341960407610458, 42.70724293864770260 ) ) ;
#83111=CARTESIAN_POINT ( 'NONE',  ( -0.05219959533936034679, 19.03943276465977164, 47.50109039468566863 ) ) ;
#83112=CARTESIAN_POINT ( 'NONE',  ( -8.224510206698735004, -14.34966873604973081, 29.58442372801901854 ) ) ;
#83113=CARTESIAN_POINT ( 'NONE',  ( 13.97604488694527802, 13.89961937509977652, 24.37390960531435624 ) ) ;
#83114=CARTESIAN_POINT ( 'NONE',  ( 9.564922557960805705, 16.46253265017160317, 49.58224293864770260 ) ) ;
#83115=CARTESIAN_POINT ( 'NONE',  ( -10.81492255796078084, -18.62759615963271287, 87.08224293864769550 ) ) ;
#83116=CARTESIAN_POINT ( 'NONE',  ( -9.474510206698964154, 16.51473224551069663, 105.4155762719810383 ) ) ;
#83117=CARTESIAN_POINT ( 'NONE',  ( 13.97604488694527802, 13.89961937509977652, 49.37390960531434558 ) ) ;
#83119=CARTESIAN_POINT ( 'NONE',  ( 0.05219959533936267826, -19.03943276465977164, 85.00109039468567573 ) ) ;
#83120=CARTESIAN_POINT ( 'NONE',  ( 16.55341960407611168, 4.379528057220329451, 63.95724293864770260 ) ) ;
#83122=CARTESIAN_POINT ( 'NONE',  ( -5.719274019375665041, -21.55341960407619695, 104.7927570613523898 ) ) ;
#83123=CARTESIAN_POINT ( 'NONE',  ( -21.55341960407610458, -5.719274019375992779, 96.45724293864770971 ) ) ;
#83124=CARTESIAN_POINT ( 'NONE',  ( -15.72974639402176322, -15.80617190586768395, 89.37609039468568994 ) ) ;
#83125=CARTESIAN_POINT ( 'NONE',  ( 10.72451020669871369, 18.67979575497193778, 82.08442372801901854 ) ) ;
#83126=CARTESIAN_POINT ( 'NONE',  ( 19.03943276465977164, -0.05219959533909143690, 103.7489096053143669 ) ) ;
#83127=CARTESIAN_POINT ( 'NONE',  ( 16.52544592524335698, 4.483927247898782831, 106.4594237280190328 ) ) ;
#83128=CARTESIAN_POINT ( 'NONE',  ( 21.52544592524334988, 5.823673210054432836, 76.45942372801901854 ) ) ;
#83129=CARTESIAN_POINT ( 'NONE',  ( -16.51473224551069308, -9.474510206698971260, 61.66557627198103120 ) ) ;
#83130=CARTESIAN_POINT ( 'NONE',  ( -18.67979575497193778, 10.72451020669871902, 48.33442372801902565 ) ) ;
#83131=CARTESIAN_POINT ( 'NONE',  ( -9.474510206698964154, 16.51473224551069663, 85.41557627198102409 ) ) ;
#83132=CARTESIAN_POINT ( 'NONE',  ( -16.55341960407611168, -4.379528057220339221, 81.45724293864769550 ) ) ;
#83133=CARTESIAN_POINT ( 'NONE',  ( 4.483927247898545687, 16.52544592524342804, 54.79057627198104541 ) ) ;
#83134=CARTESIAN_POINT ( 'NONE',  ( 10.81492255796078972, 18.62759615963270932, 64.58224293864769550 ) ) ;
#83135=CARTESIAN_POINT ( 'NONE',  ( 16.51473224551069308, 9.474510206698969483, 59.16557627198102409 ) ) ;
#83136=CARTESIAN_POINT ( 'NONE',  ( 18.67979575497178502, 10.72451020669898547, 74.16557627198102409 ) ) ;
#83137=CARTESIAN_POINT ( 'NONE',  ( -16.46253265017146816, -9.564922557961047289, 59.16775706135233293 ) ) ;
#83138=CARTESIAN_POINT ( 'NONE',  ( -9.474510206698720793, -16.51473224551083518, 34.58442372801899722 ) ) ;
#83139=CARTESIAN_POINT ( 'NONE',  ( 16.52544592524342804, -4.483927247898539470, 73.54057627198102409 ) ) ;
#83141=CARTESIAN_POINT ( 'NONE',  ( -18.67979575497178146, -10.72451020669898902, 51.66557627198102409 ) ) ;
#83143=CARTESIAN_POINT ( 'NONE',  ( 4.483927247898790824, -16.52544592524335698, 105.2094237280190328 ) ) ;
#83145=EDGE_CURVE ( 'NONE', #91305, #50923, #187665, .T. ) ;
#83146=CARTESIAN_POINT ( 'NONE',  ( -5.049401038297874678, -19.05341960407617918, 99.79275706135234714 ) ) ;
#83147=CARTESIAN_POINT ( 'NONE',  ( -16.52544592524342804, 4.483927247898546575, 66.04057627198103830 ) ) ;
#83149=CARTESIAN_POINT ( 'NONE',  ( -16.51473224551069308, -9.474510206698971260, 66.66557627198102409 ) ) ;
#83150=CARTESIAN_POINT ( 'NONE',  ( 14.34966873604960469, 8.224510206698951720, 59.16557627198103120 ) ) ;
#83151=CARTESIAN_POINT ( 'NONE',  ( -13.89961937509977652, 13.97604488694528158, 90.62390960531432427 ) ) ;
#83152=CARTESIAN_POINT ( 'NONE',  ( 19.05341960407617918, -5.049401038297876454, 81.04275706135231871 ) ) ;
#83153=CARTESIAN_POINT ( 'NONE',  ( 16.51473224551069308, 9.474510206698969483, 69.16557627198102409 ) ) ;
#83154=CARTESIAN_POINT ( 'NONE',  ( -19.05341960407611168, -5.049401038298163336, 86.45724293864769550 ) ) ;
#83155=CARTESIAN_POINT ( 'NONE',  ( 5.049401038298161559, -19.05341960407611168, 72.70724293864768129 ) ) ;
#83156=CARTESIAN_POINT ( 'NONE',  ( 15.72974639402199770, -15.80617190586745480, 63.12390960531435979 ) ) ;
#83157=CARTESIAN_POINT ( 'NONE',  ( 8.314922557961029526, -14.29746914071037800, 55.41775706135234714 ) ) ;
#83158=CARTESIAN_POINT ( 'NONE',  ( -19.02544592524335343, -5.153800228976618492, 103.9594237280190043 ) ) ;
#83159=CARTESIAN_POINT ( 'NONE',  ( -19.03943276465977164, 0.05219959533909376836, 51.24890960531436690 ) ) ;
#83160=CARTESIAN_POINT ( 'NONE',  ( 5.823673210054125526, 21.52544592524343514, 54.79057627198104541 ) ) ;
#83161=CARTESIAN_POINT ( 'NONE',  ( 5.049401038297881783, 19.05341960407617563, 87.29275706135234714 ) ) ;
#83162=CARTESIAN_POINT ( 'NONE',  ( 12.14591786802309770, 12.06949235617756955, 29.37390960531435269 ) ) ;
#83163=CARTESIAN_POINT ( 'NONE',  ( 16.46253265017146816, 9.564922557961045513, 41.66775706135234003 ) ) ;
#83164=CARTESIAN_POINT ( 'NONE',  ( 4.379528057220092307, 16.55341960407617563, 62.29275706135236845 ) ) ;
#83165=CARTESIAN_POINT ( 'NONE',  ( -4.483927247898782831, 16.52544592524335698, 92.70942372801901854 ) ) ;
#83167=CARTESIAN_POINT ( 'NONE',  ( 16.53943276465976808, 0.05219959533934440121, 86.25109039468568994 ) ) ;
#83168=CARTESIAN_POINT ( 'NONE',  ( -21.52544592524343514, 5.823673210054127303, 31.04057627198102409 ) ) ;
#83169=CARTESIAN_POINT ( 'NONE',  ( 4.379528057220092307, 16.55341960407617563, 37.29275706135235424 ) ) ;
#83170=CARTESIAN_POINT ( 'NONE',  ( -19.03943276465977164, 0.05219959533909376836, 41.24890960531435269 ) ) ;
#83171=CARTESIAN_POINT ( 'NONE',  ( -16.51473224551069308, -9.474510206698971260, 51.66557627198102409 ) ) ;
#83172=CARTESIAN_POINT ( 'NONE',  ( -13.97604488694527625, -13.89961937509977652, 41.87390960531435979 ) ) ;
#83173=CARTESIAN_POINT ( 'NONE',  ( -18.62759615963255300, -10.81492255796106328, 39.16775706135235424 ) ) ;
#83174=CARTESIAN_POINT ( 'NONE',  ( -4.379528057220086978, -16.55341960407618274, 49.79275706135234714 ) ) ;
#83175=CARTESIAN_POINT ( 'NONE',  ( -16.52544592524335698, -4.483927247898792601, 108.9594237280190185 ) ) ;
#83176=CARTESIAN_POINT ( 'NONE',  ( -9.564922557960796823, -16.46253265017161027, 27.08224293864769550 ) ) ;
#83177=CARTESIAN_POINT ( 'NONE',  ( 0.05219959533937995610, -21.53943276465977519, 110.0010903946856757 ) ) ;
#83178=CARTESIAN_POINT ( 'NONE',  ( -16.52544592524335698, -4.483927247898792601, 18.95942372801901143 ) ) ;
#83179=CARTESIAN_POINT ( 'NONE',  ( -0.05219959533936034679, 19.03943276465977164, 62.50109039468566863 ) ) ;
#83180=CARTESIAN_POINT ( 'NONE',  ( -8.314922557960811034, -14.29746914071050412, 72.08224293864769550 ) ) ;
#83181=CARTESIAN_POINT ( 'NONE',  ( -13.89961937509977652, 13.97604488694528158, 40.62390960531435979 ) ) ;
#83182=CARTESIAN_POINT ( 'NONE',  ( 9.474510206698729675, 16.51473224551082808, 72.08442372801900433 ) ) ;
#83183=CARTESIAN_POINT ( 'NONE',  ( 17.05116617787825106, -6.768360034955811955, 91.15675553259201536 ) ) ;
#83184=CARTESIAN_POINT ( 'NONE',  ( 0.05219959533937995610, -21.53943276465977519, 80.00109039468568994 ) ) ;
#83185=CARTESIAN_POINT ( 'NONE',  ( 8.224510206698742110, 14.34966873604972548, 42.08442372801901854 ) ) ;
#83187=CARTESIAN_POINT ( 'NONE',  ( 15.72974639402199770, -15.80617190586745480, 38.12390960531436690 ) ) ;
#83188=CARTESIAN_POINT ( 'NONE',  ( -4.379528057220086978, -16.55341960407618274, 29.79275706135234358 ) ) ;
#83189=CARTESIAN_POINT ( 'NONE',  ( 17.49999999999999645, 5.500000000000010658, 88.78230962303567253 ) ) ;
#83190=CARTESIAN_POINT ( 'NONE',  ( 21.52544592524334988, 5.823673210054432836, 106.4594237280190328 ) ) ;
#83192=CARTESIAN_POINT ( 'NONE',  ( 9.564922557960805705, 16.46253265017160317, 44.58224293864769550 ) ) ;
#83194=CARTESIAN_POINT ( 'NONE',  ( 13.97604488694527802, 13.89961937509977652, 54.37390960531435979 ) ) ;
#83195=CARTESIAN_POINT ( 'NONE',  ( 21.52544592524334988, 5.823673210054432836, 71.45942372801901854 ) ) ;
#83196=CARTESIAN_POINT ( 'NONE',  ( 15.72974639402176855, 15.80617190586768217, 111.8760903946856615 ) ) ;
#83197=CARTESIAN_POINT ( 'NONE',  ( -16.55341960407611168, -4.379528057220339221, 21.45724293864769550 ) ) ;
#83198=CARTESIAN_POINT ( 'NONE',  ( -16.46253265017160317, 9.564922557960807481, 25.83224293864769194 ) ) ;
#83199=CARTESIAN_POINT ( 'NONE',  ( 19.03943276465977164, -0.05219959533909143690, 88.74890960531436690 ) ) ;
#83200=CARTESIAN_POINT ( 'NONE',  ( 5.823673210054444382, -21.52544592524334988, 55.20942372801902565 ) ) ;
#83201=CARTESIAN_POINT ( 'NONE',  ( 9.564922557960805705, 16.46253265017160317, 39.58224293864768839 ) ) ;
#83202=CARTESIAN_POINT ( 'NONE',  ( 5.719274019375673035, 21.55341960407619339, 67.29275706135234714 ) ) ;
#83203=CARTESIAN_POINT ( 'NONE',  ( 13.89961937509957401, 13.97604488694547697, 91.87609039468567573 ) ) ;
#83204=CARTESIAN_POINT ( 'NONE',  ( -9.564922557960796823, -16.46253265017161027, 112.0822429386476955 ) ) ;
#83205=CARTESIAN_POINT ( 'NONE',  ( -13.89961937509977652, 13.97604488694528158, 35.62390960531435269 ) ) ;
#83206=CARTESIAN_POINT ( 'NONE',  ( 21.53943276465977519, -0.05219959533907433946, 103.7489096053143669 ) ) ;
#83207=CARTESIAN_POINT ( 'NONE',  ( -16.46253265017146816, -9.564922557961047289, 34.16775706135233293 ) ) ;
#83208=CARTESIAN_POINT ( 'NONE',  ( -14.29746914071049879, 8.314922557960819915, 115.8322429386477097 ) ) ;
#83209=CARTESIAN_POINT ( 'NONE',  ( 0.05219959533909260263, 19.03943276465977164, 59.99890960531436690 ) ) ;
#83210=CARTESIAN_POINT ( 'NONE',  ( 19.05341960407617918, -5.049401038297876454, 96.04275706135231871 ) ) ;
#83211=CARTESIAN_POINT ( 'NONE',  ( -16.52544592524342804, 4.483927247898546575, 61.04057627198103120 ) ) ;
#83212=CARTESIAN_POINT ( 'NONE',  ( 18.67979575497178502, 10.72451020669898547, 29.16557627198103120 ) ) ;
#83213=CARTESIAN_POINT ( 'NONE',  ( -19.03943276465977164, -0.05219959533935918106, 88.75109039468567573 ) ) ;
#83214=CARTESIAN_POINT ( 'NONE',  ( -21.52544592524343514, 5.823673210054127303, 86.04057627198102409 ) ) ;
#83215=CARTESIAN_POINT ( 'NONE',  ( -15.72974639402176322, -15.80617190586768395, 49.37609039468569705 ) ) ;
#83216=CARTESIAN_POINT ( 'NONE',  ( -16.53943276465976808, -0.05219959533934237506, 38.75109039468567573 ) ) ;
#83217=CARTESIAN_POINT ( 'NONE',  ( -4.483927247898782831, 16.52544592524335698, 42.70942372801901854 ) ) ;
#83218=CARTESIAN_POINT ( 'NONE',  ( 21.55341960407619695, -5.719274019375665929, 46.04275706135234714 ) ) ;
#83219=CARTESIAN_POINT ( 'NONE',  ( 18.67979575497178502, 10.72451020669898547, 54.16557627198103120 ) ) ;
#83220=CARTESIAN_POINT ( 'NONE',  ( -19.02544592524342804, 5.153800228976336051, 41.04057627198103120 ) ) ;
#83222=CARTESIAN_POINT ( 'NONE',  ( 14.34966873604972726, -8.224510206698740333, 70.83442372801901854 ) ) ;
#83223=CARTESIAN_POINT ( 'NONE',  ( -5.823673210054116645, -21.52544592524344225, 107.2905762719810525 ) ) ;
#83224=CARTESIAN_POINT ( 'NONE',  ( 8.224510206698953496, -14.34966873604960469, 42.91557627198103120 ) ) ;
#83225=CARTESIAN_POINT ( 'NONE',  ( 16.52544592524335698, 4.483927247898782831, 56.45942372801902565 ) ) ;
#83226=CARTESIAN_POINT ( 'NONE',  ( 13.89961937509957401, 13.97604488694547697, 101.8760903946856331 ) ) ;
#83227=CARTESIAN_POINT ( 'NONE',  ( -5.823673210054116645, -21.52544592524344225, 102.2905762719810383 ) ) ;
#83228=CARTESIAN_POINT ( 'NONE',  ( 12.06949235617757843, -12.14591786802309237, 28.12390960531435979 ) ) ;
#83229=ORIENTED_EDGE ( 'NONE', *, *, #87285, .T. ) ;
#83230=CARTESIAN_POINT ( 'NONE',  ( -14.34966873604972548, 8.224510206698743886, 83.33442372801903275 ) ) ;
#83232=CARTESIAN_POINT ( 'NONE',  ( 10.81492255796078972, 18.62759615963270932, 79.58224293864769550 ) ) ;
#83233=CARTESIAN_POINT ( 'NONE',  ( -14.29746914071037622, -8.314922557961029526, 104.1677570613523471 ) ) ;
#83234=CARTESIAN_POINT ( 'NONE',  ( -17.05116617787826527, -6.768360034955705373, 56.34324446740804149 ) ) ;
#83235=CARTESIAN_POINT ( 'NONE',  ( 0.05219959533907565091, 21.53943276465977519, 104.9989096053143669 ) ) ;
#83236=CARTESIAN_POINT ( 'NONE',  ( -10.81492255796078084, -18.62759615963271287, 107.0822429386476955 ) ) ;
#83237=CARTESIAN_POINT ( 'NONE',  ( 16.55341960407611168, 4.379528057220329451, 38.95724293864768839 ) ) ;
#83238=CARTESIAN_POINT ( 'NONE',  ( 8.314922557961029526, -14.29746914071037800, 50.41775706135235424 ) ) ;
#83240=CARTESIAN_POINT ( 'NONE',  ( -5.153800228976328057, -19.02544592524343514, 42.29057627198101699 ) ) ;
#83241=CARTESIAN_POINT ( 'NONE',  ( -5.153800228976328057, -19.02544592524343514, 62.29057627198100988 ) ) ;
#83242=CARTESIAN_POINT ( 'NONE',  ( -19.03943276465977164, 0.05219959533909376836, 116.2489096053143669 ) ) ;
#83243=CARTESIAN_POINT ( 'NONE',  ( -16.46253265017160317, 9.564922557960807481, 65.83224293864769550 ) ) ;
#83244=CARTESIAN_POINT ( 'NONE',  ( 16.46253265017146816, 9.564922557961045513, 106.6677570613523471 ) ) ;
#83245=CARTESIAN_POINT ( 'NONE',  ( 9.474510206698729675, 16.51473224551082808, 47.08442372801900433 ) ) ;
#83246=CARTESIAN_POINT ( 'NONE',  ( -21.55341960407610458, -5.719274019375992779, 86.45724293864770971 ) ) ;
#83247=ADVANCED_FACE ( 'NONE', ( #129507 ), #154446, .F. ) ;
#83248=CARTESIAN_POINT ( 'NONE',  ( 16.53943276465976808, -0.05219959533910856209, 23.74890960531435269 ) ) ;
#83249=CARTESIAN_POINT ( 'NONE',  ( -9.564922557960796823, -16.46253265017161027, 82.08224293864768129 ) ) ;
#83250=CARTESIAN_POINT ( 'NONE',  ( 10.72451020669898902, -18.67979575497178502, 47.91557627198102409 ) ) ;
#83251=CARTESIAN_POINT ( 'NONE',  ( -10.72451020669898014, 18.67979575497178502, 85.41557627198102409 ) ) ;
#83252=CARTESIAN_POINT ( 'NONE',  ( 0.05219959533934541429, -16.53943276465976808, 30.00109039468568284 ) ) ;
#83253=CARTESIAN_POINT ( 'NONE',  ( -15.80617190586745835, -15.72974639402198527, 26.87390960531435979 ) ) ;
#83254=CARTESIAN_POINT ( 'NONE',  ( 0.05219959533937995610, -21.53943276465977519, 80.00109039468568994 ) ) ;
#83255=CARTESIAN_POINT ( 'NONE',  ( 13.97604488694527802, 13.89961937509977652, 74.37390960531436690 ) ) ;
#83257=CARTESIAN_POINT ( 'NONE',  ( 13.97604488694527802, 13.89961937509977652, 74.37390960531436690 ) ) ;
#83258=CARTESIAN_POINT ( 'NONE',  ( -16.52544592524342804, 4.483927247898546575, 91.04057627198103830 ) ) ;
#83260=CARTESIAN_POINT ( 'NONE',  ( -19.05341960407617563, 5.049401038297882671, 108.5427570613523187 ) ) ;
#83262=CARTESIAN_POINT ( 'NONE',  ( -5.049401038298153566, 19.05341960407611168, 75.20724293864769550 ) ) ;
#83264=CARTESIAN_POINT ( 'NONE',  ( -5.719274019375665041, -21.55341960407619695, 79.79275706135236135 ) ) ;
#83265=CARTESIAN_POINT ( 'NONE',  ( -5.153800228976328057, -19.02544592524343514, 97.29057627198099567 ) ) ;
#83266=CARTESIAN_POINT ( 'NONE',  ( -4.379528057220086978, -16.55341960407618274, 74.79275706135234714 ) ) ;
#83268=CARTESIAN_POINT ( 'NONE',  ( -19.05341960407617563, 5.049401038297882671, 53.54275706135231871 ) ) ;
#83269=CARTESIAN_POINT ( 'NONE',  ( -18.67979575497193778, 10.72451020669871902, 113.3344237280190328 ) ) ;
#83273=CARTESIAN_POINT ( 'NONE',  ( -0.05219959533934338120, 16.53943276465976808, 112.5010903946857042 ) ) ;
#83275=CARTESIAN_POINT ( 'NONE',  ( -0.05219959533934338120, 16.53943276465976808, 112.5010903946857042 ) ) ;
#83276=CARTESIAN_POINT ( 'NONE',  ( 12.06949235617739724, 12.14591786802326823, 86.87609039468568994 ) ) ;
#83277=CARTESIAN_POINT ( 'NONE',  ( 18.67979575497194134, -10.72451020669871369, 75.83442372801900433 ) ) ;
#83278=CARTESIAN_POINT ( 'NONE',  ( -5.153800228976607833, 19.02544592524334988, 82.70942372801897591 ) ) ;
#83279=CARTESIAN_POINT ( 'NONE',  ( -15.72974639402176322, -15.80617190586768395, 69.37609039468567573 ) ) ;
#83280=CARTESIAN_POINT ( 'NONE',  ( 16.46253265017146816, 9.564922557961045513, 41.66775706135234003 ) ) ;
#83281=CARTESIAN_POINT ( 'NONE',  ( 19.05341960407611168, 5.049401038298154454, 78.95724293864769550 ) ) ;
#83282=CARTESIAN_POINT ( 'NONE',  ( -9.474510206698964154, 16.51473224551069663, 55.41557627198103120 ) ) ;
#83283=CARTESIAN_POINT ( 'NONE',  ( -5.153800228976328057, -19.02544592524343514, 87.29057627198102409 ) ) ;
#83284=CARTESIAN_POINT ( 'NONE',  ( -5.719274019375978568, 21.55341960407610458, 90.20724293864770971 ) ) ;
#83285=CARTESIAN_POINT ( 'NONE',  ( -21.52544592524343514, 5.823673210054127303, 46.04057627198103830 ) ) ;
#83286=CARTESIAN_POINT ( 'NONE',  ( 13.89961937509977652, -13.97604488694527269, 48.12390960531435979 ) ) ;
#83287=CARTESIAN_POINT ( 'NONE',  ( -16.55341960407617563, 4.379528057220093196, 58.54275706135235424 ) ) ;
#83288=ORIENTED_EDGE ( 'NONE', *, *, #63230, .T. ) ;
#83289=CARTESIAN_POINT ( 'NONE',  ( -18.67979575497193778, 10.72451020669871902, 48.33442372801902565 ) ) ;
#83290=CARTESIAN_POINT ( 'NONE',  ( 16.55341960407611168, 4.379528057220329451, 68.95724293864769550 ) ) ;
#83292=CARTESIAN_POINT ( 'NONE',  ( -14.34966873604972548, 8.224510206698743886, 38.33442372801900433 ) ) ;
#83293=CARTESIAN_POINT ( 'NONE',  ( -4.483927247898539470, -16.52544592524342804, 97.29057627198105251 ) ) ;
#83294=CARTESIAN_POINT ( 'NONE',  ( 9.474510206698729675, 16.51473224551082808, 47.08442372801900433 ) ) ;
#83295=CARTESIAN_POINT ( 'NONE',  ( 4.483927247898545687, 16.52544592524342804, 64.79057627198103830 ) ) ;
#83296=CARTESIAN_POINT ( 'NONE',  ( 15.80617190586769283, -15.72974639402175789, 25.62609039468567929 ) ) ;
#83297=CARTESIAN_POINT ( 'NONE',  ( 9.474510206698971260, -16.51473224551069308, 27.91557627198103120 ) ) ;
#83298=CARTESIAN_POINT ( 'NONE',  ( 0.05219959533907565091, 21.53943276465977519, 94.99890960531436690 ) ) ;
#83299=CARTESIAN_POINT ( 'NONE',  ( -19.02544592524342804, 5.153800228976336051, 101.0405762719810241 ) ) ;
#83300=CARTESIAN_POINT ( 'NONE',  ( -14.34966873604960291, -8.224510206698953496, 76.66557627198103830 ) ) ;
#83303=CARTESIAN_POINT ( 'NONE',  ( -16.51473224551082808, 9.474510206698731452, 78.33442372801900433 ) ) ;
#83304=CARTESIAN_POINT ( 'NONE',  ( 0.05219959533937995610, -21.53943276465977519, 25.00109039468567218 ) ) ;
#83305=CARTESIAN_POINT ( 'NONE',  ( 19.05341960407611168, 5.049401038298154454, 68.95724293864769550 ) ) ;
#83306=CARTESIAN_POINT ( 'NONE',  ( -0.05219959533936034679, 19.03943276465977164, 52.50109039468566863 ) ) ;
#83307=CARTESIAN_POINT ( 'NONE',  ( 19.02544592524343514, -5.153800228976328945, 33.54057627198102409 ) ) ;
#83308=CARTESIAN_POINT ( 'NONE',  ( 14.34966873604960469, 8.224510206698951720, 69.16557627198102409 ) ) ;
#83309=CARTESIAN_POINT ( 'NONE',  ( -14.29746914071049879, 8.314922557960819915, 55.83224293864770260 ) ) ;
#83310=CARTESIAN_POINT ( 'NONE',  ( 5.049401038298161559, -19.05341960407611168, 67.70724293864769550 ) ) ;
#83311=CARTESIAN_POINT ( 'NONE',  ( 18.62759615963271287, -10.81492255796078972, 83.33224293864769550 ) ) ;
#83312=CARTESIAN_POINT ( 'NONE',  ( 5.153800228976335163, 19.02544592524342804, 54.79057627198103120 ) ) ;
#83314=CARTESIAN_POINT ( 'NONE',  ( -10.81492255796078084, -18.62759615963271287, 77.08224293864769550 ) ) ;
#83315=CARTESIAN_POINT ( 'NONE',  ( 21.52544592524334988, 5.823673210054432836, 101.4594237280190185 ) ) ;
#83316=CARTESIAN_POINT ( 'NONE',  ( -9.564922557960796823, -16.46253265017161027, 22.08224293864768839 ) ) ;
#83317=CARTESIAN_POINT ( 'NONE',  ( -14.34966873604960291, -8.224510206698953496, 21.66557627198102409 ) ) ;
#83318=CARTESIAN_POINT ( 'NONE',  ( 8.224510206698953496, -14.34966873604960469, 92.91557627198103830 ) ) ;
#83319=CARTESIAN_POINT ( 'NONE',  ( -19.03943276465977164, -0.05219959533935918106, 88.75109039468567573 ) ) ;
#83321=CARTESIAN_POINT ( 'NONE',  ( -21.53943276465977519, -0.05219959533937600094, 18.75109039468568639 ) ) ;
#83322=CARTESIAN_POINT ( 'NONE',  ( -9.564922557961040184, 16.46253265017147172, 52.91775706135233293 ) ) ;
#83323=CARTESIAN_POINT ( 'NONE',  ( -8.314922557961024197, 14.29746914071037800, 102.9177570613523756 ) ) ;
#83324=CARTESIAN_POINT ( 'NONE',  ( 9.564922557961047289, -16.46253265017146816, 25.41775706135234003 ) ) ;
#83325=CARTESIAN_POINT ( 'NONE',  ( 13.97604488694527802, 13.89961937509977652, 99.37390960531436690 ) ) ;
#83326=CARTESIAN_POINT ( 'NONE',  ( -5.719274019375978568, 21.55341960407610458, 65.20724293864768129 ) ) ;
#83328=CARTESIAN_POINT ( 'NONE',  ( 5.153800228976335163, 19.02544592524342804, 29.79057627198102409 ) ) ;
#83329=CARTESIAN_POINT ( 'NONE',  ( -5.049401038297874678, -19.05341960407617918, 19.79275706135233293 ) ) ;
#83330=CARTESIAN_POINT ( 'NONE',  ( -16.53943276465976808, -0.05219959533934237506, 73.75109039468567573 ) ) ;
#83331=CARTESIAN_POINT ( 'NONE',  ( 21.55341960407619695, -5.719274019375665929, 26.04275706135235779 ) ) ;
#83332=CARTESIAN_POINT ( 'NONE',  ( -8.224510206698735004, -14.34966873604973081, 44.58442372801901854 ) ) ;
#83333=CARTESIAN_POINT ( 'NONE',  ( -16.51473224551069308, -9.474510206698971260, 106.6655762719810383 ) ) ;
#83334=CARTESIAN_POINT ( 'NONE',  ( 9.564922557960805705, 16.46253265017160317, 54.58224293864769550 ) ) ;
#83335=CARTESIAN_POINT ( 'NONE',  ( -19.02544592524342804, 5.153800228976336051, 66.04057627198103830 ) ) ;
#83336=CARTESIAN_POINT ( 'NONE',  ( 16.53943276465976808, 0.05219959533934440121, 41.25109039468568284 ) ) ;
#83337=CARTESIAN_POINT ( 'NONE',  ( 16.55341960407611168, 4.379528057220329451, 93.95724293864770971 ) ) ;
#83338=CARTESIAN_POINT ( 'NONE',  ( -14.34966873604972548, 8.224510206698743886, 113.3344237280190328 ) ) ;
#83339=CARTESIAN_POINT ( 'NONE',  ( 0.05219959533909260263, 19.03943276465977164, 49.99890960531435979 ) ) ;
#83340=CARTESIAN_POINT ( 'NONE',  ( 18.62759615963255655, 10.81492255796105972, 56.66775706135235424 ) ) ;
#83341=CARTESIAN_POINT ( 'NONE',  ( 19.03943276465977164, -0.05219959533909143690, 83.74890960531436690 ) ) ;
#83342=CARTESIAN_POINT ( 'NONE',  ( 19.02544592524343514, -5.153800228976328945, 63.54057627198103830 ) ) ;
#83343=CARTESIAN_POINT ( 'NONE',  ( -5.153800228976328057, -19.02544592524343514, 92.29057627198099567 ) ) ;
#83345=CARTESIAN_POINT ( 'NONE',  ( 4.379528057220339221, -16.55341960407611168, 42.70724293864770260 ) ) ;
#83346=CARTESIAN_POINT ( 'NONE',  ( -12.06949235617739369, -12.14591786802326823, 94.37609039468568994 ) ) ;
#83347=CARTESIAN_POINT ( 'NONE',  ( -4.379528057220328563, 16.55341960407611168, 40.20724293864769550 ) ) ;
#83349=CARTESIAN_POINT ( 'NONE',  ( -16.46253265017146816, -9.564922557961047289, 44.16775706135232582 ) ) ;
#83351=CARTESIAN_POINT ( 'NONE',  ( -9.474510206698964154, 16.51473224551069663, 60.41557627198102409 ) ) ;
#83352=CARTESIAN_POINT ( 'NONE',  ( 16.51473224551083163, -9.474510206698727899, 35.83442372801899722 ) ) ;
#83355=CARTESIAN_POINT ( 'NONE',  ( -5.153800228976607833, 19.02544592524334988, 87.70942372801897591 ) ) ;
#83356=CARTESIAN_POINT ( 'NONE',  ( -14.29746914071037622, -8.314922557961029526, 74.16775706135231871 ) ) ;
#83357=CARTESIAN_POINT ( 'NONE',  ( 17.48847506799968698, 5.747544572773784388, 91.67302562156724832 ) ) ;
#83358=CARTESIAN_POINT ( 'NONE',  ( 19.05341960407611168, 5.049401038298154454, 88.95724293864769550 ) ) ;
#83359=CARTESIAN_POINT ( 'NONE',  ( -21.53943276465977519, -0.05219959533937600094, 33.75109039468568284 ) ) ;
#83360=CARTESIAN_POINT ( 'NONE',  ( 19.02544592524334988, 5.153800228976608722, 71.45942372801900433 ) ) ;
#83361=CARTESIAN_POINT ( 'NONE',  ( -9.474510206698964154, 16.51473224551069663, 115.4155762719810241 ) ) ;
#83362=CARTESIAN_POINT ( 'NONE',  ( -16.51473224551069308, -9.474510206698971260, 51.66557627198102409 ) ) ;
#83363=CARTESIAN_POINT ( 'NONE',  ( -19.02544592524342804, 5.153800228976336051, 96.04057627198103830 ) ) ;
#83364=CARTESIAN_POINT ( 'NONE',  ( 12.14591786802309770, 12.06949235617756955, 44.37390960531435979 ) ) ;
#83365=CARTESIAN_POINT ( 'NONE',  ( 0.05219959533909260263, 19.03943276465977164, 49.99890960531435979 ) ) ;
#83366=CARTESIAN_POINT ( 'NONE',  ( 19.03943276465977164, 0.05219959533936151252, 51.25109039468567573 ) ) ;
#83367=CARTESIAN_POINT ( 'NONE',  ( -16.52544592524342804, 4.483927247898546575, 91.04057627198103830 ) ) ;
#83368=CARTESIAN_POINT ( 'NONE',  ( 13.89961937509957401, 13.97604488694547697, 26.87609039468566507 ) ) ;
#83369=CARTESIAN_POINT ( 'NONE',  ( 13.97604488694527802, 13.89961937509977652, 69.37390960531436690 ) ) ;
#83370=CARTESIAN_POINT ( 'NONE',  ( 5.719274019375991003, -21.55341960407610458, 67.70724293864769550 ) ) ;
#83371=CARTESIAN_POINT ( 'NONE',  ( 8.314922557960818139, 14.29746914071049879, 69.58224293864769550 ) ) ;
#83372=CARTESIAN_POINT ( 'NONE',  ( 13.89961937509957401, 13.97604488694547697, 26.87609039468566507 ) ) ;
#83373=CARTESIAN_POINT ( 'NONE',  ( -9.474510206698964154, 16.51473224551069663, 105.4155762719810383 ) ) ;
#83374=CARTESIAN_POINT ( 'NONE',  ( -5.719274019375978568, 21.55341960407610458, 30.20724293864769550 ) ) ;
#83375=CARTESIAN_POINT ( 'NONE',  ( 13.89961937509977652, -13.97604488694527269, 53.12390960531434558 ) ) ;
#83376=CARTESIAN_POINT ( 'NONE',  ( 16.46253265017160672, -9.564922557960803928, 38.33224293864768839 ) ) ;
#83377=CARTESIAN_POINT ( 'NONE',  ( 16.55341960407611168, 4.379528057220329451, 98.95724293864770971 ) ) ;
#83378=CARTESIAN_POINT ( 'NONE',  ( 21.52544592524344225, -5.823673210054117533, 108.5405762719810241 ) ) ;
#83379=CARTESIAN_POINT ( 'NONE',  ( -5.049401038298153566, 19.05341960407611168, 105.2072429386476671 ) ) ;
#83380=CARTESIAN_POINT ( 'NONE',  ( -21.55341960407610458, -5.719274019375992779, 111.4572429386476813 ) ) ;
#83381=CARTESIAN_POINT ( 'NONE',  ( 13.97604488694527802, 13.89961937509977652, 109.3739096053143669 ) ) ;
#83382=CARTESIAN_POINT ( 'NONE',  ( 13.97604488694527802, 13.89961937509977652, 24.37390960531435624 ) ) ;
#83383=CARTESIAN_POINT ( 'NONE',  ( 21.52544592524334988, 5.823673210054432836, 81.45942372801900433 ) ) ;
#83384=CARTESIAN_POINT ( 'NONE',  ( -21.55341960407610458, -5.719274019375992779, 91.45724293864769550 ) ) ;
#83385=CARTESIAN_POINT ( 'NONE',  ( 16.29526858892874941, -7.335722546920139031, 106.7032940219979196 ) ) ;
#83388=CARTESIAN_POINT ( 'NONE',  ( -14.29746914071037622, -8.314922557961029526, 44.16775706135234714 ) ) ;
#83389=CARTESIAN_POINT ( 'NONE',  ( 0.05219959533910956823, 16.53943276465976808, 109.9989096053143527 ) ) ;
#83390=CARTESIAN_POINT ( 'NONE',  ( -17.50000000000000355, -3.512728167236954580, 109.7719000481887690 ) ) ;
#83391=CARTESIAN_POINT ( 'NONE',  ( 19.02544592524343514, -5.153800228976328945, 63.54057627198103830 ) ) ;
#83392=CARTESIAN_POINT ( 'NONE',  ( -0.05219959533910754901, -16.53943276465976808, 92.49890960531436690 ) ) ;
#83393=CARTESIAN_POINT ( 'NONE',  ( 21.53943276465977519, -0.05219959533907433946, 43.74890960531435979 ) ) ;
#83394=CARTESIAN_POINT ( 'NONE',  ( -0.05219959533910754901, -16.53943276465976808, 62.49890960531436690 ) ) ;
#83395=CARTESIAN_POINT ( 'NONE',  ( 4.483927247898790824, -16.52544592524335698, 20.20942372801900788 ) ) ;
#83396=CARTESIAN_POINT ( 'NONE',  ( -5.719274019375665041, -21.55341960407619695, 74.79275706135234714 ) ) ;
#83397=CARTESIAN_POINT ( 'NONE',  ( -12.14591786802326823, 12.06949235617739902, 103.1260903946856757 ) ) ;
#83398=CARTESIAN_POINT ( 'NONE',  ( 14.34966873604960469, 8.224510206698951720, 44.16557627198103120 ) ) ;
#83399=CARTESIAN_POINT ( 'NONE',  ( 13.89961937509977652, -13.97604488694527269, 33.12390960531434558 ) ) ;
#83400=CARTESIAN_POINT ( 'NONE',  ( 19.05341960407611168, 5.049401038298154454, 83.95724293864766707 ) ) ;
#83401=CARTESIAN_POINT ( 'NONE',  ( 15.80617190586746368, 15.72974639402197994, 99.37390960531436690 ) ) ;
#83402=CARTESIAN_POINT ( 'NONE',  ( 0.05219959533934541429, -16.53943276465976808, 20.00109039468568639 ) ) ;
#83403=CARTESIAN_POINT ( 'NONE',  ( -14.34966873604960291, -8.224510206698953496, 66.66557627198102409 ) ) ;
#83404=CARTESIAN_POINT ( 'NONE',  ( -0.05219959533937732626, 21.53943276465977519, 72.50109039468568994 ) ) ;
#83406=CARTESIAN_POINT ( 'NONE',  ( -0.05219959533934338120, 16.53943276465976808, 97.50109039468567573 ) ) ;
#83407=CARTESIAN_POINT ( 'NONE',  ( 17.49999999999999645, 5.624438216177604311, 26.68329655085357288 ) ) ;
#83408=CARTESIAN_POINT ( 'NONE',  ( -19.20446147854528007, -5.499999999999907629, 64.38999695167679249 ) ) ;
#83409=CARTESIAN_POINT ( 'NONE',  ( -4.483927247898539470, -16.52544592524342804, 32.29057627198102409 ) ) ;
#83410=CARTESIAN_POINT ( 'NONE',  ( 16.53943276465976808, 0.05219959533934440121, 76.25109039468568994 ) ) ;
#83411=CARTESIAN_POINT ( 'NONE',  ( 16.51473224551069308, 9.474510206698969483, 89.16557627198103830 ) ) ;
#83412=CARTESIAN_POINT ( 'NONE',  ( 0.05219959533909260263, 19.03943276465977164, 99.99890960531436690 ) ) ;
#83413=CARTESIAN_POINT ( 'NONE',  ( 21.53943276465977519, 0.05219959533937863772, 86.25109039468568994 ) ) ;
#83414=CARTESIAN_POINT ( 'NONE',  ( 12.14591786802327356, -12.06949235617739191, 85.62609039468568994 ) ) ;
#83415=CARTESIAN_POINT ( 'NONE',  ( 8.224510206698953496, -14.34966873604960469, 62.91557627198102409 ) ) ;
#83416=CARTESIAN_POINT ( 'NONE',  ( 9.564922557960805705, 16.46253265017160317, 69.58224293864770971 ) ) ;
#83418=CARTESIAN_POINT ( 'NONE',  ( -16.53943276465976808, -0.05219959533934237506, 18.75109039468568639 ) ) ;
#83419=CARTESIAN_POINT ( 'NONE',  ( -4.483927247898539470, -16.52544592524342804, 112.2905762719810241 ) ) ;
#83420=CARTESIAN_POINT ( 'NONE',  ( -9.474510206698964154, 16.51473224551069663, 75.41557627198103830 ) ) ;
#83421=CARTESIAN_POINT ( 'NONE',  ( -9.564922557961040184, 16.46253265017147172, 112.9177570613523329 ) ) ;
#83423=CARTESIAN_POINT ( 'NONE',  ( 18.62759615963255655, 10.81492255796105972, 111.6677570613523613 ) ) ;
#83424=CARTESIAN_POINT ( 'NONE',  ( -4.379528057220086978, -16.55341960407618274, 79.79275706135236135 ) ) ;
#83425=CARTESIAN_POINT ( 'NONE',  ( 5.049401038297881783, 19.05341960407617563, 92.29275706135234714 ) ) ;
#83426=CARTESIAN_POINT ( 'NONE',  ( 8.314922557960818139, 14.29746914071049879, 114.5822429386477097 ) ) ;
#83427=CARTESIAN_POINT ( 'NONE',  ( 8.224510206698742110, 14.34966873604972548, 72.08442372801899012 ) ) ;
#83428=CARTESIAN_POINT ( 'NONE',  ( -0.05219959533934338120, 16.53943276465976808, 47.50109039468568994 ) ) ;
#83429=CARTESIAN_POINT ( 'NONE',  ( 16.51473224551069308, 9.474510206698969483, 24.16557627198102765 ) ) ;
#83430=CARTESIAN_POINT ( 'NONE',  ( 13.97604488694548053, -13.89961937509957401, 65.62609039468567573 ) ) ;
#83431=CARTESIAN_POINT ( 'NONE',  ( 15.80617190586769283, -15.72974639402175789, 100.6260903946857184 ) ) ;
#83432=CARTESIAN_POINT ( 'NONE',  ( 19.02544592524343514, -5.153800228976328945, 33.54057627198102409 ) ) ;
#83433=CARTESIAN_POINT ( 'NONE',  ( 16.51473224551069308, 9.474510206698969483, 84.16557627198102409 ) ) ;
#83434=CARTESIAN_POINT ( 'NONE',  ( 14.34966873604960469, 8.224510206698951720, 69.16557627198102409 ) ) ;
#83435=CARTESIAN_POINT ( 'NONE',  ( -5.719274019375665041, -21.55341960407619695, 94.79275706135234714 ) ) ;
#83436=CARTESIAN_POINT ( 'NONE',  ( 9.564922557961047289, -16.46253265017146816, 40.41775706135234003 ) ) ;
#83437=CARTESIAN_POINT ( 'NONE',  ( 15.72974639402199770, -15.80617190586745480, 33.12390960531435979 ) ) ;
#83438=CARTESIAN_POINT ( 'NONE',  ( 21.53943276465977519, 0.05219959533937863772, 111.2510903946856899 ) ) ;
#83439=CARTESIAN_POINT ( 'NONE',  ( 9.564922557960805705, 16.46253265017160317, 74.58224293864769550 ) ) ;
#83440=CARTESIAN_POINT ( 'NONE',  ( 21.53943276465977519, 0.05219959533937863772, 106.2510903946856757 ) ) ;
#83441=CARTESIAN_POINT ( 'NONE',  ( 21.55341960407610458, 5.719274019375980345, 48.95724293864770971 ) ) ;
#83442=CARTESIAN_POINT ( 'NONE',  ( -19.03943276465977164, 0.05219959533909376836, 96.24890960531436690 ) ) ;
#83443=CARTESIAN_POINT ( 'NONE',  ( 5.153800228976615827, -19.02544592524334988, 70.20942372801899012 ) ) ;
#83444=CARTESIAN_POINT ( 'NONE',  ( -5.153800228976328057, -19.02544592524343514, 107.2905762719810383 ) ) ;
#83445=ADVANCED_FACE ( 'NONE', ( #6172, #7170, #189228 ), #191207, .F. ) ;
#83446=CARTESIAN_POINT ( 'NONE',  ( -9.474510206698720793, -16.51473224551083518, 89.58442372801900433 ) ) ;
#83447=CARTESIAN_POINT ( 'NONE',  ( 14.29746914071037800, 8.314922557961029526, 41.66775706135235424 ) ) ;
#83448=CARTESIAN_POINT ( 'NONE',  ( -12.06949235617756955, 12.14591786802309770, 115.6239096053143669 ) ) ;
#83449=CARTESIAN_POINT ( 'NONE',  ( 19.02544592524343514, -5.153800228976328945, 78.54057627198099567 ) ) ;
#83450=CARTESIAN_POINT ( 'NONE',  ( 5.823673210054125526, 21.52544592524343514, 59.79057627198103120 ) ) ;
#83451=CARTESIAN_POINT ( 'NONE',  ( 14.29746914071037800, 8.314922557961029526, 26.66775706135235424 ) ) ;
#83452=CARTESIAN_POINT ( 'NONE',  ( -15.72974639402176322, -15.80617190586768395, 29.37609039468568284 ) ) ;
#83453=CARTESIAN_POINT ( 'NONE',  ( -18.67979575497193778, 10.72451020669871902, 78.33442372801901854 ) ) ;
#83454=CARTESIAN_POINT ( 'NONE',  ( 4.483927247898790824, -16.52544592524335698, 85.20942372801901854 ) ) ;
#83455=CARTESIAN_POINT ( 'NONE',  ( -16.46253265017160317, 9.564922557960807481, 90.83224293864769550 ) ) ;
#83456=CARTESIAN_POINT ( 'NONE',  ( 4.379528057220339221, -16.55341960407611168, 72.70724293864769550 ) ) ;
#83457=CARTESIAN_POINT ( 'NONE',  ( 14.34966873604972726, -8.224510206698740333, 110.8344237280190043 ) ) ;
#83458=CARTESIAN_POINT ( 'NONE',  ( -9.474510206698720793, -16.51473224551083518, 54.58442372801899722 ) ) ;
#83459=CARTESIAN_POINT ( 'NONE',  ( -21.55341960407619339, 5.719274019375674811, 43.54275706135235424 ) ) ;
#83461=CARTESIAN_POINT ( 'NONE',  ( 0.05219959533910956823, 16.53943276465976808, 84.99890960531436690 ) ) ;
#83462=CARTESIAN_POINT ( 'NONE',  ( 5.153800228976335163, 19.02544592524342804, 109.7905762719810099 ) ) ;
#83463=CARTESIAN_POINT ( 'NONE',  ( 4.379528057220092307, 16.55341960407617563, 97.29275706135234714 ) ) ;
#83464=CARTESIAN_POINT ( 'NONE',  ( -10.72451020669870658, -18.67979575497194134, 89.58442372801901854 ) ) ;
#83465=CARTESIAN_POINT ( 'NONE',  ( 16.52544592524335698, 4.483927247898782831, 41.45942372801901143 ) ) ;
#83466=CARTESIAN_POINT ( 'NONE',  ( 0.05219959533937995610, -21.53943276465977519, 40.00109039468567573 ) ) ;
#83468=CARTESIAN_POINT ( 'NONE',  ( -21.53943276465977519, -0.05219959533937600094, 18.75109039468568639 ) ) ;
#83469=CARTESIAN_POINT ( 'NONE',  ( -12.14591786802309592, -12.06949235617757132, 86.87390960531438111 ) ) ;
#83470=CARTESIAN_POINT ( 'NONE',  ( 17.50000000000001066, -3.237210098469561093, 27.21236987379542782 ) ) ;
#83471=CARTESIAN_POINT ( 'NONE',  ( -14.34966873604960291, -8.224510206698953496, 66.66557627198102409 ) ) ;
#83472=CARTESIAN_POINT ( 'NONE',  ( 14.29746914071037800, 8.314922557961029526, 96.66775706135234714 ) ) ;
#83473=CARTESIAN_POINT ( 'NONE',  ( 16.51473224551069308, 9.474510206698969483, 44.16557627198103120 ) ) ;
#83474=CARTESIAN_POINT ( 'NONE',  ( 10.72451020669898902, -18.67979575497178502, 47.91557627198102409 ) ) ;
#83475=CARTESIAN_POINT ( 'NONE',  ( -12.06949235617756955, 12.14591786802309770, 80.62390960531438111 ) ) ;
#83476=CARTESIAN_POINT ( 'NONE',  ( -15.80617190586745835, -15.72974639402198527, 76.87390960531439532 ) ) ;
#83477=CARTESIAN_POINT ( 'NONE',  ( 16.46253265017160672, -9.564922557960803928, 83.33224293864768129 ) ) ;
#83478=CARTESIAN_POINT ( 'NONE',  ( -0.05219959533909027116, -19.03943276465977164, 37.49890960531436690 ) ) ;
#83479=CARTESIAN_POINT ( 'NONE',  ( -9.474510206698720793, -16.51473224551083518, 89.58442372801900433 ) ) ;
#83480=CARTESIAN_POINT ( 'NONE',  ( 10.81492255796078972, 18.62759615963270932, 34.58224293864770260 ) ) ;
#83481=CARTESIAN_POINT ( 'NONE',  ( 10.72451020669871369, 18.67979575497193778, 52.08442372801901854 ) ) ;
#83482=CARTESIAN_POINT ( 'NONE',  ( 19.02544592524343514, -5.153800228976328945, 58.54057627198102409 ) ) ;
#83483=CARTESIAN_POINT ( 'NONE',  ( 9.474510206698971260, -16.51473224551069308, 82.91557627198103830 ) ) ;
#83484=VERTEX_POINT ( 'NONE', #52682 ) ;
#83485=CARTESIAN_POINT ( 'NONE',  ( -12.06949235617739369, -12.14591786802326823, 44.37609039468567573 ) ) ;
#83486=CARTESIAN_POINT ( 'NONE',  ( 10.81492255796106328, -18.62759615963255655, 35.41775706135234003 ) ) ;
#83488=CARTESIAN_POINT ( 'NONE',  ( -5.823673210054431948, 21.52544592524334988, 77.70942372801900433 ) ) ;
#83489=CARTESIAN_POINT ( 'NONE',  ( 10.72451020669898902, -18.67979575497178502, 27.91557627198103830 ) ) ;
#83490=CARTESIAN_POINT ( 'NONE',  ( -21.52544592524343514, 5.823673210054127303, 91.04057627198103830 ) ) ;
#83491=CARTESIAN_POINT ( 'NONE',  ( 10.72451020669871369, 18.67979575497193778, 22.08442372801901143 ) ) ;
#83492=CARTESIAN_POINT ( 'NONE',  ( 8.314922557961029526, -14.29746914071037800, 70.41775706135236135 ) ) ;
#83493=CARTESIAN_POINT ( 'NONE',  ( 21.55341960407610458, 5.719274019375980345, 68.95724293864769550 ) ) ;
#83494=CARTESIAN_POINT ( 'NONE',  ( 19.02544592524334988, 5.153800228976608722, 21.45942372801899012 ) ) ;
#83495=CARTESIAN_POINT ( 'NONE',  ( 5.153800228976335163, 19.02544592524342804, 64.79057627198100988 ) ) ;
#83497=CARTESIAN_POINT ( 'NONE',  ( 16.46253265017160672, -9.564922557960803928, 83.33224293864768129 ) ) ;
#83498=CARTESIAN_POINT ( 'NONE',  ( 17.58332526062528345, 7.635886036038587399, 51.57665040441534643 ) ) ;
#83499=CARTESIAN_POINT ( 'NONE',  ( 9.474510206698729675, 16.51473224551082808, 77.08442372801900433 ) ) ;
#83500=CARTESIAN_POINT ( 'NONE',  ( 15.72974639402199770, -15.80617190586745480, 48.12390960531436690 ) ) ;
#83501=CARTESIAN_POINT ( 'NONE',  ( 12.06949235617739724, 12.14591786802326823, 111.8760903946856615 ) ) ;
#83502=CARTESIAN_POINT ( 'NONE',  ( 5.049401038297881783, 19.05341960407617563, 97.29275706135233293 ) ) ;
#83503=CARTESIAN_POINT ( 'NONE',  ( 5.153800228976335163, 19.02544592524342804, 39.79057627198102409 ) ) ;
#83504=CARTESIAN_POINT ( 'NONE',  ( -19.02544592524334988, -5.153800228976617603, 98.95942372801900433 ) ) ;
#83505=CARTESIAN_POINT ( 'NONE',  ( 10.81492255796078972, 18.62759615963270932, 84.58224293864769550 ) ) ;
#83506=CARTESIAN_POINT ( 'NONE',  ( 9.474510206698729675, 16.51473224551082808, 57.08442372801900433 ) ) ;
#83508=CARTESIAN_POINT ( 'NONE',  ( 19.05341960407611168, 5.049401038298154454, 53.95724293864770260 ) ) ;
#83509=CARTESIAN_POINT ( 'NONE',  ( 4.379528057220339221, -16.55341960407611168, 67.70724293864769550 ) ) ;
#83510=CARTESIAN_POINT ( 'NONE',  ( 19.05341960407611168, 5.049401038298154454, 43.95724293864769550 ) ) ;
#83511=CARTESIAN_POINT ( 'NONE',  ( 8.314922557960818139, 14.29746914071049879, 59.58224293864770260 ) ) ;
#83514=CARTESIAN_POINT ( 'NONE',  ( -0.05219959533910754901, -16.53943276465976808, 27.49890960531435269 ) ) ;
#83515=CARTESIAN_POINT ( 'NONE',  ( 9.474510206698971260, -16.51473224551069308, 62.91557627198102409 ) ) ;
#83517=CARTESIAN_POINT ( 'NONE',  ( -9.564922557961040184, 16.46253265017147172, 37.91775706135233293 ) ) ;
#83518=CARTESIAN_POINT ( 'NONE',  ( -12.14591786802326823, 12.06949235617739902, 53.12609039468568284 ) ) ;
#83519=CARTESIAN_POINT ( 'NONE',  ( 0.05219959533907565091, 21.53943276465977519, 54.99890960531435269 ) ) ;
#83520=CARTESIAN_POINT ( 'NONE',  ( 21.53943276465977519, 0.05219959533937863772, 101.2510903946856757 ) ) ;
#83521=CARTESIAN_POINT ( 'NONE',  ( 19.05341960407611168, 5.049401038298154454, 63.95724293864769550 ) ) ;
#83523=CARTESIAN_POINT ( 'NONE',  ( -9.474510206698964154, 16.51473224551069663, 100.4155762719810241 ) ) ;
#83525=CARTESIAN_POINT ( 'NONE',  ( -21.55341960407619339, 5.719274019375674811, 28.54275706135234358 ) ) ;
#83526=CARTESIAN_POINT ( 'NONE',  ( 4.483927247898545687, 16.52544592524342804, 94.79057627198105251 ) ) ;
#83527=CARTESIAN_POINT ( 'NONE',  ( 15.80617190586746368, 15.72974639402197994, 89.37390960531435269 ) ) ;
#83528=CARTESIAN_POINT ( 'NONE',  ( 9.474510206698971260, -16.51473224551069308, 77.91557627198103830 ) ) ;
#83529=CARTESIAN_POINT ( 'NONE',  ( 5.153800228976335163, 19.02544592524342804, 84.79057627198099567 ) ) ;
#83530=CARTESIAN_POINT ( 'NONE',  ( 10.81492255796078972, 18.62759615963270932, 109.5822429386476955 ) ) ;
#83532=CARTESIAN_POINT ( 'NONE',  ( 5.153800228976335163, 19.02544592524342804, 69.79057627198103830 ) ) ;
#83534=CARTESIAN_POINT ( 'NONE',  ( -16.52544592524342804, 4.483927247898546575, 101.0405762719810383 ) ) ;
#83535=CARTESIAN_POINT ( 'NONE',  ( 19.05341960407611168, 5.049401038298154454, 28.95724293864769550 ) ) ;
#83536=CARTESIAN_POINT ( 'NONE',  ( -13.97604488694547697, 13.89961937509957934, 98.12609039468566152 ) ) ;
#83537=CARTESIAN_POINT ( 'NONE',  ( 0.05219959533910956823, 16.53943276465976808, 104.9989096053143669 ) ) ;
#83538=CARTESIAN_POINT ( 'NONE',  ( 15.72974639402176855, 15.80617190586768217, 66.87609039468568994 ) ) ;
#83539=CARTESIAN_POINT ( 'NONE',  ( -13.89961937509977652, 13.97604488694528158, 60.62390960531436690 ) ) ;
#83540=CARTESIAN_POINT ( 'NONE',  ( -21.55341960407619339, 5.719274019375674811, 38.54275706135234714 ) ) ;
#83541=CARTESIAN_POINT ( 'NONE',  ( -15.72974639402197994, 15.80617190586746368, 105.6239096053143669 ) ) ;
#83543=CARTESIAN_POINT ( 'NONE',  ( 19.05341960407611168, 5.049401038298154454, 73.95724293864768129 ) ) ;
#83545=CARTESIAN_POINT ( 'NONE',  ( -0.05219959533934338120, 16.53943276465976808, 32.50109039468568284 ) ) ;
#83546=CARTESIAN_POINT ( 'NONE',  ( 15.72974639402199770, -15.80617190586745480, 28.12390960531435979 ) ) ;
#83547=CARTESIAN_POINT ( 'NONE',  ( -21.55341960407619339, 5.719274019375674811, 63.54275706135234003 ) ) ;
#83548=CARTESIAN_POINT ( 'NONE',  ( -5.153800228976328057, -19.02544592524343514, 112.2905762719810099 ) ) ;
#83549=CARTESIAN_POINT ( 'NONE',  ( 19.05341960407617918, -5.049401038297876454, 101.0427570613523045 ) ) ;
#83550=CARTESIAN_POINT ( 'NONE',  ( 19.02544592524343514, -5.153800228976328945, 43.54057627198103120 ) ) ;
#83551=CARTESIAN_POINT ( 'NONE',  ( 16.46253265017160672, -9.564922557960803928, 73.33224293864769550 ) ) ;
#83552=CARTESIAN_POINT ( 'NONE',  ( 16.53943276465976808, -0.05219959533910856209, 98.74890960531438111 ) ) ;
#83553=CARTESIAN_POINT ( 'NONE',  ( 13.89961937509977652, -13.97604488694527269, 113.1239096053143527 ) ) ;
#83554=CARTESIAN_POINT ( 'NONE',  ( -12.14591786802309592, -12.06949235617757132, 91.87390960531436690 ) ) ;
#83555=CARTESIAN_POINT ( 'NONE',  ( -19.03943276465977164, 0.05219959533909376836, 96.24890960531436690 ) ) ;
#83556=CARTESIAN_POINT ( 'NONE',  ( 14.34966873604960469, 8.224510206698951720, 59.16557627198103120 ) ) ;
#83558=CARTESIAN_POINT ( 'NONE',  ( -0.05219959533909027116, -19.03943276465977164, 47.49890960531435979 ) ) ;
#83559=CARTESIAN_POINT ( 'NONE',  ( 21.55341960407619695, -5.719274019375665929, 56.04275706135235424 ) ) ;
#83560=CARTESIAN_POINT ( 'NONE',  ( -9.474510206698720793, -16.51473224551083518, 99.58442372801900433 ) ) ;
#83561=CARTESIAN_POINT ( 'NONE',  ( 0.05219959533910956823, 16.53943276465976808, 49.99890960531437401 ) ) ;
#83562=CARTESIAN_POINT ( 'NONE',  ( 21.55341960407610458, 5.719274019375980345, 113.9572429386477239 ) ) ;
#83563=CARTESIAN_POINT ( 'NONE',  ( 18.62759615963271287, -10.81492255796078972, 43.33224293864769550 ) ) ;
#83564=CARTESIAN_POINT ( 'NONE',  ( -13.97604488694527625, -13.89961937509977652, 111.8739096053143243 ) ) ;
#83565=CARTESIAN_POINT ( 'NONE',  ( 0.05219959533910956823, 16.53943276465976808, 79.99890960531435269 ) ) ;
#83567=CARTESIAN_POINT ( 'NONE',  ( -5.049401038298153566, 19.05341960407611168, 50.20724293864770260 ) ) ;
#83568=CARTESIAN_POINT ( 'NONE',  ( 16.53943276465976808, 0.05219959533934440121, 111.2510903946856899 ) ) ;
#83569=CARTESIAN_POINT ( 'NONE',  ( 12.06949235617739724, 12.14591786802326823, 106.8760903946856899 ) ) ;
#83570=CARTESIAN_POINT ( 'NONE',  ( -16.52544592524335698, -4.483927247898792601, 83.95942372801900433 ) ) ;
#83571=CARTESIAN_POINT ( 'NONE',  ( -19.02544592524334988, -5.153800228976617603, 43.95942372801899012 ) ) ;
#83573=CARTESIAN_POINT ( 'NONE',  ( 13.89961937509977652, -13.97604488694527269, 93.12390960531436690 ) ) ;
#83574=CARTESIAN_POINT ( 'NONE',  ( 13.89961937509977652, -13.97604488694527269, 53.12390960531434558 ) ) ;
#83575=CARTESIAN_POINT ( 'NONE',  ( 14.34966873604960469, 8.224510206698951720, 64.16557627198102409 ) ) ;
#83576=CARTESIAN_POINT ( 'NONE',  ( -9.474510206698964154, 16.51473224551069663, 25.41557627198103120 ) ) ;
#83577=CARTESIAN_POINT ( 'NONE',  ( 5.049401038298161559, -19.05341960407611168, 107.7072429386476955 ) ) ;
#83578=CARTESIAN_POINT ( 'NONE',  ( 21.52544592524344225, -5.823673210054117533, 43.54057627198103830 ) ) ;
#83579=CARTESIAN_POINT ( 'NONE',  ( 16.53943276465976808, -0.05219959533910856209, 88.74890960531436690 ) ) ;
#83580=CARTESIAN_POINT ( 'NONE',  ( 4.483927247898790824, -16.52544592524335698, 35.20942372801901854 ) ) ;
#83581=CARTESIAN_POINT ( 'NONE',  ( -8.224510206698948167, 14.34966873604960824, 80.41557627198103830 ) ) ;
#83583=CARTESIAN_POINT ( 'NONE',  ( -9.474510206698720793, -16.51473224551083518, 74.58442372801900433 ) ) ;
#83584=CARTESIAN_POINT ( 'NONE',  ( 9.564922557960805705, 16.46253265017160317, 104.5822429386476955 ) ) ;
#83585=CARTESIAN_POINT ( 'NONE',  ( -16.46253265017146816, -9.564922557961047289, 74.16775706135234714 ) ) ;
#83586=CARTESIAN_POINT ( 'NONE',  ( -5.153800228976328057, -19.02544592524343514, 42.29057627198102409 ) ) ;
#83587=CARTESIAN_POINT ( 'NONE',  ( 4.483927247898790824, -16.52544592524335698, 30.20942372801902565 ) ) ;
#83588=CARTESIAN_POINT ( 'NONE',  ( 16.53943276465976808, 0.05219959533934440121, 106.2510903946856757 ) ) ;
#83589=CARTESIAN_POINT ( 'NONE',  ( 19.03943276465977164, 0.05219959533936151252, 76.25109039468566152 ) ) ;
#83590=CARTESIAN_POINT ( 'NONE',  ( 0.05219959533907565091, 21.53943276465977519, 39.99890960531436690 ) ) ;
#83591=CARTESIAN_POINT ( 'NONE',  ( 10.81492255796106328, -18.62759615963255655, 70.41775706135236135 ) ) ;
#83592=CARTESIAN_POINT ( 'NONE',  ( 18.85284094683695244, 5.500000000000118128, 38.82762727607044440 ) ) ;
#83593=CARTESIAN_POINT ( 'NONE',  ( 8.314922557961029526, -14.29746914071037800, 40.41775706135234714 ) ) ;
#83594=CARTESIAN_POINT ( 'NONE',  ( 9.474510206698971260, -16.51473224551069308, 27.91557627198103120 ) ) ;
#83595=CARTESIAN_POINT ( 'NONE',  ( 9.474510206698971260, -16.51473224551069308, 92.91557627198103830 ) ) ;
#83596=CARTESIAN_POINT ( 'NONE',  ( -13.89961937509977652, 13.97604488694528158, 25.62390960531434558 ) ) ;
#83597=CARTESIAN_POINT ( 'NONE',  ( 16.55341960407611168, 4.379528057220329451, 93.95724293864770971 ) ) ;
#83599=CARTESIAN_POINT ( 'NONE',  ( -16.51473224551069308, -9.474510206698971260, 86.66557627198102409 ) ) ;
#83600=ORIENTED_EDGE ( 'NONE', *, *, #163734, .T. ) ;
#83601=CARTESIAN_POINT ( 'NONE',  ( 13.97604488694548053, -13.89961937509957401, 105.6260903946856757 ) ) ;
#83602=CARTESIAN_POINT ( 'NONE',  ( 21.53943276465977519, -0.05219959533907433946, 83.74890960531435269 ) ) ;
#83603=CARTESIAN_POINT ( 'NONE',  ( -5.049401038298153566, 19.05341960407611168, 45.20724293864769550 ) ) ;
#83604=CARTESIAN_POINT ( 'NONE',  ( -9.474510206698720793, -16.51473224551083518, 69.58442372801901854 ) ) ;
#83605=CARTESIAN_POINT ( 'NONE',  ( -21.53943276465977519, -0.05219959533937600094, 18.75109039468568639 ) ) ;
#83606=CARTESIAN_POINT ( 'NONE',  ( -13.89961937509977652, 13.97604488694528158, 75.62390960531438111 ) ) ;
#83607=CARTESIAN_POINT ( 'NONE',  ( 19.02544592524343514, -5.153800228976328945, 103.5405762719809957 ) ) ;
#83608=EDGE_CURVE ( 'NONE', #160325, #179909, #66925, .T. ) ;
#83610=CARTESIAN_POINT ( 'NONE',  ( -8.224510206698735004, -14.34966873604973081, 39.58442372801901143 ) ) ;
#83611=CARTESIAN_POINT ( 'NONE',  ( 21.52544592524344225, -5.823673210054117533, 103.5405762719810383 ) ) ;
#83612=CARTESIAN_POINT ( 'NONE',  ( -8.314922557960811034, -14.29746914071050412, 112.0822429386477097 ) ) ;
#83613=CARTESIAN_POINT ( 'NONE',  ( 19.02544592524343514, -5.153800228976328945, 88.54057627198102409 ) ) ;
#83614=CARTESIAN_POINT ( 'NONE',  ( -19.05341960407617563, 5.049401038297882671, 63.54275706135234003 ) ) ;
#83615=CARTESIAN_POINT ( 'NONE',  ( -21.52544592524343514, 5.823673210054127303, 91.04057627198103830 ) ) ;
#83616=CARTESIAN_POINT ( 'NONE',  ( -5.823673210054116645, -21.52544592524344225, 77.29057627198102409 ) ) ;
#83617=CARTESIAN_POINT ( 'NONE',  ( 16.55341960407611168, 4.379528057220329451, 43.95724293864769550 ) ) ;
#83618=CARTESIAN_POINT ( 'NONE',  ( -5.049401038297874678, -19.05341960407617918, 24.79275706135233648 ) ) ;
#83619=CARTESIAN_POINT ( 'NONE',  ( 14.29746914071037800, 8.314922557961029526, 61.66775706135235424 ) ) ;
#83621=CARTESIAN_POINT ( 'NONE',  ( -19.02544592524342804, 5.153800228976336051, 91.04057627198100988 ) ) ;
#83622=CARTESIAN_POINT ( 'NONE',  ( -16.51473224551069308, -9.474510206698971260, 41.66557627198103120 ) ) ;
#83623=CARTESIAN_POINT ( 'NONE',  ( -10.72451020669870658, -18.67979575497194134, 54.58442372801901143 ) ) ;
#83624=CARTESIAN_POINT ( 'NONE',  ( -21.53943276465977519, -0.05219959533937600094, 68.75109039468568994 ) ) ;
#83625=CARTESIAN_POINT ( 'NONE',  ( -5.153800228976328057, -19.02544592524343514, 57.29057627198103120 ) ) ;
#83626=CARTESIAN_POINT ( 'NONE',  ( 10.81492255796106328, -18.62759615963255655, 40.41775706135234714 ) ) ;
#83627=CARTESIAN_POINT ( 'NONE',  ( -19.05341960407617563, 5.049401038297882671, 78.54275706135233293 ) ) ;
#83628=CARTESIAN_POINT ( 'NONE',  ( 5.153800228976615827, -19.02544592524334988, 70.20942372801899012 ) ) ;
#83629=CARTESIAN_POINT ( 'NONE',  ( -13.89961937509977652, 13.97604488694528158, 35.62390960531435269 ) ) ;
#83630=CARTESIAN_POINT ( 'NONE',  ( 12.06949235617739724, 12.14591786802326823, 81.87609039468568994 ) ) ;
#83631=CARTESIAN_POINT ( 'NONE',  ( 19.03943276465977164, -0.05219959533909143690, 58.74890960531435979 ) ) ;
#83633=CARTESIAN_POINT ( 'NONE',  ( 0.05219959533909260263, 19.03943276465977164, 94.99890960531436690 ) ) ;
#83634=CARTESIAN_POINT ( 'NONE',  ( 19.02544592524343514, -5.153800228976328945, 43.54057627198103120 ) ) ;
#83635=CARTESIAN_POINT ( 'NONE',  ( -15.80617190586745835, -15.72974639402198527, 81.87390960531435269 ) ) ;
#83636=CARTESIAN_POINT ( 'NONE',  ( -14.29746914071037622, -8.314922557961029526, 64.16775706135234714 ) ) ;
#83637=CARTESIAN_POINT ( 'NONE',  ( 10.72451020669871369, 18.67979575497193778, 112.0844237280190185 ) ) ;
#83638=CARTESIAN_POINT ( 'NONE',  ( 9.564922557960805705, 16.46253265017160317, 49.58224293864770260 ) ) ;
#83639=CARTESIAN_POINT ( 'NONE',  ( 16.52544592524342804, -4.483927247898539470, 48.54057627198103120 ) ) ;
#83640=CARTESIAN_POINT ( 'NONE',  ( -4.379528057220328563, 16.55341960407611168, 80.20724293864769550 ) ) ;
#83642=CARTESIAN_POINT ( 'NONE',  ( 9.474510206698971260, -16.51473224551069308, 72.91557627198102409 ) ) ;
#83643=CARTESIAN_POINT ( 'NONE',  ( -21.55341960407619339, 5.719274019375674811, 43.54275706135235424 ) ) ;
#83644=CARTESIAN_POINT ( 'NONE',  ( -19.03943276465977164, 0.05219959533909376836, 91.24890960531436690 ) ) ;
#83645=CARTESIAN_POINT ( 'NONE',  ( 10.81492255796106328, -18.62759615963255655, 95.41775706135234714 ) ) ;
#83646=CARTESIAN_POINT ( 'NONE',  ( -12.14591786802326823, 12.06949235617739902, 73.12609039468567573 ) ) ;
#83647=CARTESIAN_POINT ( 'NONE',  ( -10.72451020669870658, -18.67979575497194134, 29.58442372801901854 ) ) ;
#83648=CARTESIAN_POINT ( 'NONE',  ( 9.474510206698971260, -16.51473224551069308, 112.9155762719810383 ) ) ;
#83649=CARTESIAN_POINT ( 'NONE',  ( 18.67979575497178502, 10.72451020669898547, 94.16557627198103830 ) ) ;
#83650=CARTESIAN_POINT ( 'NONE',  ( -16.55341960407611168, -4.379528057220339221, 41.45724293864769550 ) ) ;
#83651=CARTESIAN_POINT ( 'NONE',  ( 19.05341960407611168, 5.049401038298154454, 43.95724293864769550 ) ) ;
#83652=CARTESIAN_POINT ( 'NONE',  ( 0.05219959533910956823, 16.53943276465976808, 69.99890960531435269 ) ) ;
#83653=CARTESIAN_POINT ( 'NONE',  ( 5.823673210054125526, 21.52544592524343514, 34.79057627198103120 ) ) ;
#83654=CARTESIAN_POINT ( 'NONE',  ( 19.02544592524334988, 5.153800228976608722, 36.45942372801900433 ) ) ;
#83655=CARTESIAN_POINT ( 'NONE',  ( 12.14591786802309770, 12.06949235617756955, 99.37390960531436690 ) ) ;
#83656=CARTESIAN_POINT ( 'NONE',  ( -19.02544592524342804, 5.153800228976336051, 106.0405762719810241 ) ) ;
#83657=ORIENTED_EDGE ( 'NONE', *, *, #179822, .T. ) ;
#83658=CARTESIAN_POINT ( 'NONE',  ( -4.483927247898782831, 16.52544592524335698, 52.70942372801902565 ) ) ;
#83659=CARTESIAN_POINT ( 'NONE',  ( 5.153800228976335163, 19.02544592524342804, 59.79057627198100988 ) ) ;
#83661=CARTESIAN_POINT ( 'NONE',  ( -16.53943276465976808, -0.05219959533934237506, 98.75109039468568994 ) ) ;
#83662=CARTESIAN_POINT ( 'NONE',  ( 19.03943276465977164, 0.05219959533936151252, 106.2510903946856615 ) ) ;
#83663=CARTESIAN_POINT ( 'NONE',  ( -0.05219959533937732626, 21.53943276465977519, 77.50109039468567573 ) ) ;
#83664=CARTESIAN_POINT ( 'NONE',  ( -19.03943276465977164, 0.05219959533909376836, 71.24890960531435269 ) ) ;
#83665=CARTESIAN_POINT ( 'NONE',  ( 21.52544592524344225, -5.823673210054117533, 103.5405762719810383 ) ) ;
#83666=CARTESIAN_POINT ( 'NONE',  ( 16.55341960407618274, -4.379528057220086978, 61.04275706135234714 ) ) ;
#83667=CARTESIAN_POINT ( 'NONE',  ( 8.224510206698953496, -14.34966873604960469, 112.9155762719810383 ) ) ;
#83668=CARTESIAN_POINT ( 'NONE',  ( -19.03943276465977164, -0.05219959533935918106, 113.7510903946856757 ) ) ;
#83669=CARTESIAN_POINT ( 'NONE',  ( -9.564922557961040184, 16.46253265017147172, 87.91775706135233293 ) ) ;
#83670=CARTESIAN_POINT ( 'NONE',  ( -0.05219959533907301413, -21.53943276465977519, 77.49890960531433848 ) ) ;
#83671=CARTESIAN_POINT ( 'NONE',  ( 13.97604488694548053, -13.89961937509957401, 60.62609039468564731 ) ) ;
#83673=CARTESIAN_POINT ( 'NONE',  ( 10.72451020669898902, -18.67979575497178502, 107.9155762719810241 ) ) ;
#83674=CARTESIAN_POINT ( 'NONE',  ( 17.50000000000002842, 3.805241302050184515, 27.12647527217411536 ) ) ;
#83675=CARTESIAN_POINT ( 'NONE',  ( 9.564922557960805705, 16.46253265017160317, 64.58224293864769550 ) ) ;
#83677=CARTESIAN_POINT ( 'NONE',  ( -12.06949235617739369, -12.14591786802326823, 19.37609039468568639 ) ) ;
#83679=CARTESIAN_POINT ( 'NONE',  ( -21.55341960407619339, 5.719274019375674811, 48.54275706135234714 ) ) ;
#83680=CARTESIAN_POINT ( 'NONE',  ( -10.72451020669898014, 18.67979575497178502, 100.4155762719810241 ) ) ;
#83681=CARTESIAN_POINT ( 'NONE',  ( 4.483927247898545687, 16.52544592524342804, 69.79057627198102409 ) ) ;
#83682=CARTESIAN_POINT ( 'NONE',  ( 9.474510206698971260, -16.51473224551069308, 67.91557627198102409 ) ) ;
#83683=CARTESIAN_POINT ( 'NONE',  ( -18.67979575497193778, 10.72451020669871902, 68.33442372801900433 ) ) ;
#83684=CARTESIAN_POINT ( 'NONE',  ( 14.34966873604972726, -8.224510206698740333, 25.83442372801901499 ) ) ;
#83685=CARTESIAN_POINT ( 'NONE',  ( 0.05219959533936267826, -19.03943276465977164, 30.00109039468566863 ) ) ;
#83686=CARTESIAN_POINT ( 'NONE',  ( -5.823673210054431948, 21.52544592524334988, 47.70942372801902565 ) ) ;
#83687=CARTESIAN_POINT ( 'NONE',  ( 15.72974639402199770, -15.80617190586745480, 113.1239096053143953 ) ) ;
#83688=CARTESIAN_POINT ( 'NONE',  ( 18.67979575497178502, 10.72451020669898547, 59.16557627198103120 ) ) ;
#83689=CARTESIAN_POINT ( 'NONE',  ( -9.474510206698720793, -16.51473224551083518, 99.58442372801900433 ) ) ;
#83690=CARTESIAN_POINT ( 'NONE',  ( -5.049401038297874678, -19.05341960407617918, 74.79275706135231871 ) ) ;
#83691=CARTESIAN_POINT ( 'NONE',  ( 21.53943276465977519, 0.05219959533937863772, 81.25109039468568994 ) ) ;
#83692=CARTESIAN_POINT ( 'NONE',  ( 5.049401038297881783, 19.05341960407617563, 47.29275706135231161 ) ) ;
#83693=CARTESIAN_POINT ( 'NONE',  ( 19.02544592524343514, -5.153800228976328945, 33.54057627198102409 ) ) ;
#83694=CARTESIAN_POINT ( 'NONE',  ( 15.80617190586746368, 15.72974639402197994, 54.37390960531435979 ) ) ;
#83695=CARTESIAN_POINT ( 'NONE',  ( 0.05219959533910956823, 16.53943276465976808, 49.99890960531437401 ) ) ;
#83696=CARTESIAN_POINT ( 'NONE',  ( -19.36337904590692105, 5.499999999999949374, 95.41494137495622851 ) ) ;
#83697=CARTESIAN_POINT ( 'NONE',  ( -13.89961937509957401, -13.97604488694547875, 29.37609039468565797 ) ) ;
#83698=CARTESIAN_POINT ( 'NONE',  ( -16.55341960407617563, 4.379528057220093196, 83.54275706135234714 ) ) ;
#83699=CARTESIAN_POINT ( 'NONE',  ( 16.55341960407611168, 4.379528057220329451, 58.95724293864770971 ) ) ;
#83700=CARTESIAN_POINT ( 'NONE',  ( -15.80617190586768217, 15.72974639402176855, 83.12609039468568994 ) ) ;
#83701=CARTESIAN_POINT ( 'NONE',  ( 21.55341960407619695, -5.719274019375665929, 86.04275706135236135 ) ) ;
#83702=CARTESIAN_POINT ( 'NONE',  ( -18.62759615963270932, 10.81492255796079327, 75.83224293864769550 ) ) ;
#83703=CARTESIAN_POINT ( 'NONE',  ( 9.564922557960805705, 16.46253265017160317, 39.58224293864768839 ) ) ;
#83704=CARTESIAN_POINT ( 'NONE',  ( 18.62759615963255655, 10.81492255796105972, 51.66775706135234714 ) ) ;
#83705=CARTESIAN_POINT ( 'NONE',  ( -13.97604488694527625, -13.89961937509977652, 41.87390960531435979 ) ) ;
#83706=CARTESIAN_POINT ( 'NONE',  ( 16.46253265017160672, -9.564922557960803928, 48.33224293864769550 ) ) ;
#83707=CARTESIAN_POINT ( 'NONE',  ( -0.05219959533910754901, -16.53943276465976808, 102.4989096053143811 ) ) ;
#83708=CARTESIAN_POINT ( 'NONE',  ( 19.02544592524343514, -5.153800228976328945, 103.5405762719809957 ) ) ;
#83709=CARTESIAN_POINT ( 'NONE',  ( 8.314922557960818139, 14.29746914071049879, 39.58224293864769550 ) ) ;
#83710=CARTESIAN_POINT ( 'NONE',  ( -14.29746914071049879, 8.314922557960819915, 105.8322429386476955 ) ) ;
#83711=CARTESIAN_POINT ( 'NONE',  ( -5.719274019375978568, 21.55341960407610458, 80.20724293864769550 ) ) ;
#83712=CARTESIAN_POINT ( 'NONE',  ( -10.72451020669870658, -18.67979575497194134, 24.58442372801901499 ) ) ;
#83714=CARTESIAN_POINT ( 'NONE',  ( -16.52544592524335698, -4.483927247898792601, 33.95942372801901143 ) ) ;
#83716=CARTESIAN_POINT ( 'NONE',  ( -21.55341960407610458, -5.719274019375992779, 66.45724293864768129 ) ) ;
#83717=CARTESIAN_POINT ( 'NONE',  ( -21.53943276465977519, -0.05219959533937600094, 88.75109039468567573 ) ) ;
#83718=CARTESIAN_POINT ( 'NONE',  ( -9.474510206698964154, 16.51473224551069663, 90.41557627198103830 ) ) ;
#83719=CARTESIAN_POINT ( 'NONE',  ( 18.67979575497194134, -10.72451020669871369, 25.83442372801901499 ) ) ;
#83720=CARTESIAN_POINT ( 'NONE',  ( 18.62759615963271287, -10.81492255796078972, 33.33224293864769550 ) ) ;
#83721=CARTESIAN_POINT ( 'NONE',  ( 16.55341960407618274, -4.379528057220086978, 96.04275706135236135 ) ) ;
#83722=CARTESIAN_POINT ( 'NONE',  ( 0.05219959533937995610, -21.53943276465977519, 80.00109039468568994 ) ) ;
#83723=CARTESIAN_POINT ( 'NONE',  ( -9.474510206698720793, -16.51473224551083518, 24.58442372801900078 ) ) ;
#83724=CARTESIAN_POINT ( 'NONE',  ( -14.34966873604972548, 8.224510206698743886, 68.33442372801900433 ) ) ;
#83725=CARTESIAN_POINT ( 'NONE',  ( 5.823673210054444382, -21.52544592524334988, 25.20942372801901854 ) ) ;
#83726=CARTESIAN_POINT ( 'NONE',  ( -19.02544592524342804, 5.153800228976336051, 31.04057627198102409 ) ) ;
#83727=CARTESIAN_POINT ( 'NONE',  ( -0.05219959533937732626, 21.53943276465977519, 107.5010903946856899 ) ) ;
#83728=CARTESIAN_POINT ( 'NONE',  ( -5.049401038298153566, 19.05341960407611168, 105.2072429386476671 ) ) ;
#83729=CARTESIAN_POINT ( 'NONE',  ( 5.823673210054125526, 21.52544592524343514, 99.79057627198103830 ) ) ;
#83731=CARTESIAN_POINT ( 'NONE',  ( -5.719274019375978568, 21.55341960407610458, 70.20724293864769550 ) ) ;
#83732=CARTESIAN_POINT ( 'NONE',  ( 4.483927247898790824, -16.52544592524335698, 50.20942372801901854 ) ) ;
#83733=CARTESIAN_POINT ( 'NONE',  ( 0.05219959533910956823, 16.53943276465976808, 54.99890960531435269 ) ) ;
#83735=CARTESIAN_POINT ( 'NONE',  ( 13.89961937509957401, 13.97604488694547697, 76.87609039468566152 ) ) ;
#83737=CARTESIAN_POINT ( 'NONE',  ( 4.379528057220092307, 16.55341960407617563, 32.29275706135235424 ) ) ;
#83738=CARTESIAN_POINT ( 'NONE',  ( -10.72451020669898014, 18.67979575497178502, 100.4155762719810241 ) ) ;
#83739=CARTESIAN_POINT ( 'NONE',  ( -4.379528057220328563, 16.55341960407611168, 60.20724293864768839 ) ) ;
#83740=CARTESIAN_POINT ( 'NONE',  ( -16.46253265017160317, 9.564922557960807481, 100.8322429386477097 ) ) ;
#83741=CARTESIAN_POINT ( 'NONE',  ( -4.483927247898782831, 16.52544592524335698, 37.70942372801900433 ) ) ;
#83742=CARTESIAN_POINT ( 'NONE',  ( 9.474510206698971260, -16.51473224551069308, 62.91557627198102409 ) ) ;
#83743=CARTESIAN_POINT ( 'NONE',  ( -15.80617190586768217, 15.72974639402176855, 28.12609039468568284 ) ) ;
#83744=CARTESIAN_POINT ( 'NONE',  ( -0.05219959533936034679, 19.03943276465977164, 102.5010903946856757 ) ) ;
#83745=CARTESIAN_POINT ( 'NONE',  ( 16.46253265017160672, -9.564922557960803928, 98.33224293864769550 ) ) ;
#83746=CARTESIAN_POINT ( 'NONE',  ( -0.05219959533909027116, -19.03943276465977164, 87.49890960531436690 ) ) ;
#83747=CARTESIAN_POINT ( 'NONE',  ( 5.719274019375991003, -21.55341960407610458, 87.70724293864769550 ) ) ;
#83748=CARTESIAN_POINT ( 'NONE',  ( -0.05219959533909027116, -19.03943276465977164, 42.49890960531435269 ) ) ;
#83750=CARTESIAN_POINT ( 'NONE',  ( 4.379528057220339221, -16.55341960407611168, 67.70724293864769550 ) ) ;
#83751=CARTESIAN_POINT ( 'NONE',  ( 9.474510206698971260, -16.51473224551069308, 97.91557627198102409 ) ) ;
#83753=CARTESIAN_POINT ( 'NONE',  ( -19.03943276465977164, -0.05219959533935918106, 78.75109039468567573 ) ) ;
#83754=CARTESIAN_POINT ( 'NONE',  ( -15.72974639402197994, 15.80617190586746368, 90.62390960531436690 ) ) ;
#83755=CARTESIAN_POINT ( 'NONE',  ( -13.89961937509957401, -13.97604488694547875, 44.37609039468566863 ) ) ;
#83756=CARTESIAN_POINT ( 'NONE',  ( -5.823673210054116645, -21.52544592524344225, 22.29057627198102765 ) ) ;
#83758=CARTESIAN_POINT ( 'NONE',  ( -10.72451020669898014, 18.67979575497178502, 35.41557627198102409 ) ) ;
#83759=CARTESIAN_POINT ( 'NONE',  ( -0.05219959533909027116, -19.03943276465977164, 87.49890960531436690 ) ) ;
#83760=CARTESIAN_POINT ( 'NONE',  ( 18.62759615963255655, 10.81492255796105972, 66.66775706135234714 ) ) ;
#83761=CARTESIAN_POINT ( 'NONE',  ( -19.02544592524342804, 5.153800228976336051, 36.04057627198100988 ) ) ;
#83762=CARTESIAN_POINT ( 'NONE',  ( -12.06949235617756955, 12.14591786802309770, 70.62390960531436690 ) ) ;
#83763=CARTESIAN_POINT ( 'NONE',  ( 12.14591786802327356, -12.06949235617739191, 25.62609039468567929 ) ) ;
#83764=CARTESIAN_POINT ( 'NONE',  ( 10.72451020669871369, 18.67979575497193778, 47.08442372801901854 ) ) ;
#83767=CARTESIAN_POINT ( 'NONE',  ( 19.02544592524334988, 5.153800228976608722, 86.45942372801900433 ) ) ;
#83768=CARTESIAN_POINT ( 'NONE',  ( 17.50000000000000000, 5.499999999999992895, 46.70309617465829888 ) ) ;
#83769=CARTESIAN_POINT ( 'NONE',  ( -18.62759615963255300, -10.81492255796106328, 19.16775706135234714 ) ) ;
#83770=CARTESIAN_POINT ( 'NONE',  ( -19.20446147854529784, -5.499999999999912070, 44.38999695167677118 ) ) ;
#83771=CARTESIAN_POINT ( 'NONE',  ( 16.51473224551083163, -9.474510206698727899, 20.83442372801899722 ) ) ;
#83772=CARTESIAN_POINT ( 'NONE',  ( 9.474510206698971260, -16.51473224551069308, 57.91557627198103120 ) ) ;
#83773=CARTESIAN_POINT ( 'NONE',  ( 16.46253265017146816, 9.564922557961045513, 21.66775706135233648 ) ) ;
#83774=CARTESIAN_POINT ( 'NONE',  ( -4.483927247898782831, 16.52544592524335698, 102.7094237280190185 ) ) ;
#83775=CARTESIAN_POINT ( 'NONE',  ( 5.049401038298161559, -19.05341960407611168, 107.7072429386476955 ) ) ;
#83776=CARTESIAN_POINT ( 'NONE',  ( -5.719274019375665041, -21.55341960407619695, 69.79275706135234714 ) ) ;
#83781=CARTESIAN_POINT ( 'NONE',  ( -15.72974639402176322, -15.80617190586768395, 74.37609039468568994 ) ) ;
#83782=CARTESIAN_POINT ( 'NONE',  ( -18.67979575497193778, 10.72451020669871902, 98.33442372801901854 ) ) ;
#83784=CARTESIAN_POINT ( 'NONE',  ( -13.89961937509977652, 13.97604488694528158, 85.62390960531433848 ) ) ;
#83785=CARTESIAN_POINT ( 'NONE',  ( -19.03943276465977164, -0.05219959533935918106, 28.75109039468566507 ) ) ;
#83787=CARTESIAN_POINT ( 'NONE',  ( -0.05219959533909027116, -19.03943276465977164, 37.49890960531436690 ) ) ;
#83788=CARTESIAN_POINT ( 'NONE',  ( 15.72974639402199770, -15.80617190586745480, 58.12390960531435979 ) ) ;
#83789=CARTESIAN_POINT ( 'NONE',  ( 16.55341960407618274, -4.379528057220086978, 101.0427570613523756 ) ) ;
#83790=CARTESIAN_POINT ( 'NONE',  ( 12.06949235617757843, -12.14591786802309237, 93.12390960531436690 ) ) ;
#83791=CARTESIAN_POINT ( 'NONE',  ( 19.05341960407611168, 5.049401038298154454, 83.95724293864766707 ) ) ;
#83792=CARTESIAN_POINT ( 'NONE',  ( -5.823673210054431948, 21.52544592524334988, 102.7094237280190185 ) ) ;
#83793=CARTESIAN_POINT ( 'NONE',  ( -19.03943276465977164, 0.05219959533909376836, 41.24890960531435269 ) ) ;
#83794=CARTESIAN_POINT ( 'NONE',  ( -16.55341960407611168, -4.379528057220339221, 91.45724293864769550 ) ) ;
#83795=CARTESIAN_POINT ( 'NONE',  ( -15.80617190586768217, 15.72974639402176855, 58.12609039468568994 ) ) ;
#83796=CARTESIAN_POINT ( 'NONE',  ( 10.72451020669898902, -18.67979575497178502, 92.91557627198103830 ) ) ;
#83797=CARTESIAN_POINT ( 'NONE',  ( 19.02544592524334988, 5.153800228976608722, 46.45942372801899012 ) ) ;
#83798=CARTESIAN_POINT ( 'NONE',  ( -15.49999999999999822, 5.499999999999997335, 120.0000000000000142 ) ) ;
#83799=CARTESIAN_POINT ( 'NONE',  ( 5.049401038298161559, -19.05341960407611168, 92.70724293864769550 ) ) ;
#83800=CARTESIAN_POINT ( 'NONE',  ( 14.29746914071049879, -8.314922557960816363, 58.33224293864768839 ) ) ;
#83801=CARTESIAN_POINT ( 'NONE',  ( 19.05341960407617918, -5.049401038297876454, 41.04275706135233293 ) ) ;
#83802=CARTESIAN_POINT ( 'NONE',  ( -0.05219959533909027116, -19.03943276465977164, 67.49890960531436690 ) ) ;
#83804=CARTESIAN_POINT ( 'NONE',  ( 14.29746914071049879, -8.314922557960816363, 43.33224293864769550 ) ) ;
#83805=CARTESIAN_POINT ( 'NONE',  ( 0.05219959533936267826, -19.03943276465977164, 85.00109039468567573 ) ) ;
#83807=CARTESIAN_POINT ( 'NONE',  ( 18.67979575497178502, 10.72451020669898547, 39.16557627198102409 ) ) ;
#83808=CARTESIAN_POINT ( 'NONE',  ( -14.34966873604960291, -8.224510206698953496, 96.66557627198102409 ) ) ;
#83810=CARTESIAN_POINT ( 'NONE',  ( 9.474510206698971260, -16.51473224551069308, 57.91557627198103120 ) ) ;
#83811=CARTESIAN_POINT ( 'NONE',  ( 10.72451020669898902, -18.67979575497178502, 57.91557627198103120 ) ) ;
#83812=CARTESIAN_POINT ( 'NONE',  ( -13.89961937509977652, 13.97604488694528158, 25.62390960531434558 ) ) ;
#83813=CARTESIAN_POINT ( 'NONE',  ( 12.14591786802327356, -12.06949235617739191, 80.62609039468567573 ) ) ;
#83814=CARTESIAN_POINT ( 'NONE',  ( 19.02544592524343514, -5.153800228976328945, 63.54057627198103830 ) ) ;
#83815=CARTESIAN_POINT ( 'NONE',  ( 5.049401038297881783, 19.05341960407617563, 37.29275706135232582 ) ) ;
#83816=CARTESIAN_POINT ( 'NONE',  ( 5.719274019375673035, 21.55341960407619339, 72.29275706135236135 ) ) ;
#83817=CARTESIAN_POINT ( 'NONE',  ( 21.55341960407610458, 5.719274019375980345, 53.95724293864770260 ) ) ;
#83818=CARTESIAN_POINT ( 'NONE',  ( -5.049401038298153566, 19.05341960407611168, 30.20724293864768839 ) ) ;
#83819=CARTESIAN_POINT ( 'NONE',  ( 13.97604488694548053, -13.89961937509957401, 110.6260903946856615 ) ) ;
#83820=CARTESIAN_POINT ( 'NONE',  ( -5.049401038298153566, 19.05341960407611168, 25.20724293864768484 ) ) ;
#83822=CARTESIAN_POINT ( 'NONE',  ( 10.81492255796078972, 18.62759615963270932, 44.58224293864769550 ) ) ;
#83823=CARTESIAN_POINT ( 'NONE',  ( 5.823673210054444382, -21.52544592524334988, 85.20942372801901854 ) ) ;
#83824=CARTESIAN_POINT ( 'NONE',  ( 8.224510206698953496, -14.34966873604960469, 42.91557627198103120 ) ) ;
#83825=CARTESIAN_POINT ( 'NONE',  ( 8.224510206698953496, -14.34966873604960469, 62.91557627198102409 ) ) ;
#83826=CARTESIAN_POINT ( 'NONE',  ( -18.62759615963270932, 10.81492255796079327, 80.83224293864769550 ) ) ;
#83827=CARTESIAN_POINT ( 'NONE',  ( 10.72451020669898902, -18.67979575497178502, 72.91557627198103830 ) ) ;
#83829=CARTESIAN_POINT ( 'NONE',  ( 21.52544592524344225, -5.823673210054117533, 38.54057627198103120 ) ) ;
#83830=CARTESIAN_POINT ( 'NONE',  ( -16.53943276465976808, -0.05219959533934237506, 48.75109039468568284 ) ) ;
#83831=CARTESIAN_POINT ( 'NONE',  ( -14.34966873604960291, -8.224510206698953496, 81.66557627198103830 ) ) ;
#83832=CARTESIAN_POINT ( 'NONE',  ( 5.049401038298161559, -19.05341960407611168, 27.70724293864769550 ) ) ;
#83834=CARTESIAN_POINT ( 'NONE',  ( -16.52544592524335698, -4.483927247898792601, 83.95942372801900433 ) ) ;
#83835=CARTESIAN_POINT ( 'NONE',  ( -10.72451020669870658, -18.67979575497194134, 24.58442372801901499 ) ) ;
#83836=CARTESIAN_POINT ( 'NONE',  ( 13.97604488694527802, 13.89961937509977652, 89.37390960531436690 ) ) ;
#83837=CARTESIAN_POINT ( 'NONE',  ( 21.53943276465977519, 0.05219959533937863772, 51.25109039468568994 ) ) ;
#83838=CARTESIAN_POINT ( 'NONE',  ( 16.51473224551069308, 9.474510206698969483, 104.1655762719810241 ) ) ;
#83842=CARTESIAN_POINT ( 'NONE',  ( -21.53943276465977519, -0.05219959533937600094, 43.75109039468568284 ) ) ;
#83843=CARTESIAN_POINT ( 'NONE',  ( 19.02544592524343514, -5.153800228976328945, 38.54057627198103120 ) ) ;
#83844=CARTESIAN_POINT ( 'NONE',  ( 13.89961937509977652, -13.97604488694527269, 108.1239096053143669 ) ) ;
#83845=CARTESIAN_POINT ( 'NONE',  ( 5.153800228976615827, -19.02544592524334988, 60.20942372801899012 ) ) ;
#83846=CARTESIAN_POINT ( 'NONE',  ( 15.72974639402176855, 15.80617190586768217, 26.87609039468567218 ) ) ;
#83847=CARTESIAN_POINT ( 'NONE',  ( -5.049401038297874678, -19.05341960407617918, 49.79275706135231871 ) ) ;
#83848=CARTESIAN_POINT ( 'NONE',  ( -19.02544592524342804, 5.153800228976336051, 31.04057627198102409 ) ) ;
#83849=CARTESIAN_POINT ( 'NONE',  ( -16.55341960407617563, 4.379528057220093196, 88.54275706135236135 ) ) ;
#83850=CARTESIAN_POINT ( 'NONE',  ( 13.97604488694548053, -13.89961937509957401, 65.62609039468567573 ) ) ;
#83851=CARTESIAN_POINT ( 'NONE',  ( -12.06949235617739369, -12.14591786802326823, 109.3760903946857042 ) ) ;
#83853=VERTEX_POINT ( 'NONE', #136331 ) ;
#83854=CARTESIAN_POINT ( 'NONE',  ( -19.02544592524342804, 5.153800228976336051, 86.04057627198103830 ) ) ;
#83855=CARTESIAN_POINT ( 'NONE',  ( 21.52544592524334988, 5.823673210054432836, 91.45942372801901854 ) ) ;
#83856=CARTESIAN_POINT ( 'NONE',  ( 21.55341960407619695, -5.719274019375665929, 101.0427570613523756 ) ) ;
#83858=CARTESIAN_POINT ( 'NONE',  ( -9.474510206698964154, 16.51473224551069663, 105.4155762719810383 ) ) ;
#83859=CARTESIAN_POINT ( 'NONE',  ( 10.81492255796106328, -18.62759615963255655, 75.41775706135233293 ) ) ;
#83860=CARTESIAN_POINT ( 'NONE',  ( 16.51473224551083163, -9.474510206698727899, 110.8344237280190043 ) ) ;
#83861=CARTESIAN_POINT ( 'NONE',  ( -0.05219959533909027116, -19.03943276465977164, 82.49890960531436690 ) ) ;
#83862=CARTESIAN_POINT ( 'NONE',  ( -15.80617190586745835, -15.72974639402198527, 36.87390960531435979 ) ) ;
#83863=CARTESIAN_POINT ( 'NONE',  ( 13.97604488694527802, 13.89961937509977652, 89.37390960531436690 ) ) ;
#83865=CARTESIAN_POINT ( 'NONE',  ( 19.05341960407611168, 5.049401038298154454, 73.95724293864768129 ) ) ;
#83866=CARTESIAN_POINT ( 'NONE',  ( -13.89961937509977652, 13.97604488694528158, 60.62390960531436690 ) ) ;
#83867=CARTESIAN_POINT ( 'NONE',  ( 8.224510206698742110, 14.34966873604972548, 102.0844237280190185 ) ) ;
#83868=CARTESIAN_POINT ( 'NONE',  ( -16.21995358207276539, 7.366697692864274671, 99.93551001512065568 ) ) ;
#83869=CARTESIAN_POINT ( 'NONE',  ( -5.153800228976607833, 19.02544592524334988, 77.70942372801900433 ) ) ;
#83870=CARTESIAN_POINT ( 'NONE',  ( 19.02544592524343514, -5.153800228976328945, 88.54057627198102409 ) ) ;
#83871=CARTESIAN_POINT ( 'NONE',  ( 0.05219959533910956823, 16.53943276465976808, 84.99890960531436690 ) ) ;
#83872=CARTESIAN_POINT ( 'NONE',  ( 15.80617190586746368, 15.72974639402197994, 29.37390960531435269 ) ) ;
#83873=CARTESIAN_POINT ( 'NONE',  ( 21.55341960407610458, 5.719274019375980345, 23.95724293864769550 ) ) ;
#83874=CARTESIAN_POINT ( 'NONE',  ( -8.314922557960811034, -14.29746914071050412, 97.08224293864770971 ) ) ;
#83876=CARTESIAN_POINT ( 'NONE',  ( -0.05219959533936034679, 19.03943276465977164, 47.50109039468566863 ) ) ;
#83877=CARTESIAN_POINT ( 'NONE',  ( -0.05219959533910754901, -16.53943276465976808, 27.49890960531435269 ) ) ;
#83878=CARTESIAN_POINT ( 'NONE',  ( -0.05219959533909027116, -19.03943276465977164, 107.4989096053143527 ) ) ;
#83879=CARTESIAN_POINT ( 'NONE',  ( 10.81492255796106328, -18.62759615963255655, 65.41775706135234714 ) ) ;
#83880=CARTESIAN_POINT ( 'NONE',  ( -21.55341960407610458, -5.719274019375992779, 61.45724293864770260 ) ) ;
#83881=CARTESIAN_POINT ( 'NONE',  ( -18.62759615963255300, -10.81492255796106328, 34.16775706135234714 ) ) ;
#83882=CARTESIAN_POINT ( 'NONE',  ( 10.72451020669898902, -18.67979575497178502, 82.91557627198103830 ) ) ;
#83883=CARTESIAN_POINT ( 'NONE',  ( -0.05219959533937732626, 21.53943276465977519, 42.50109039468567573 ) ) ;
#83884=CARTESIAN_POINT ( 'NONE',  ( 4.483927247898545687, 16.52544592524342804, 114.7905762719810383 ) ) ;
#83885=CARTESIAN_POINT ( 'NONE',  ( 19.05341960407617918, -5.049401038297876454, 71.04275706135234714 ) ) ;
#83886=CARTESIAN_POINT ( 'NONE',  ( 0.05219959533909260263, 19.03943276465977164, 39.99890960531436690 ) ) ;
#83887=CARTESIAN_POINT ( 'NONE',  ( -4.379528057220328563, 16.55341960407611168, 85.20724293864770971 ) ) ;
#83888=CARTESIAN_POINT ( 'NONE',  ( 19.05341960407611168, 5.049401038298154454, 93.95724293864769550 ) ) ;
#83889=CARTESIAN_POINT ( 'NONE',  ( -16.51473224551069308, -9.474510206698971260, 91.66557627198103830 ) ) ;
#83890=CARTESIAN_POINT ( 'NONE',  ( 14.29746914071049879, -8.314922557960816363, 108.3322429386477097 ) ) ;
#83891=CARTESIAN_POINT ( 'NONE',  ( -8.314922557960811034, -14.29746914071050412, 37.08224293864768129 ) ) ;
#83892=CARTESIAN_POINT ( 'NONE',  ( -8.314922557961024197, 14.29746914071037800, 97.91775706135236135 ) ) ;
#83893=CARTESIAN_POINT ( 'NONE',  ( 19.02544592524343514, -5.153800228976328945, 48.54057627198103120 ) ) ;
#83894=CARTESIAN_POINT ( 'NONE',  ( -9.564922557960796823, -16.46253265017161027, 27.08224293864769550 ) ) ;
#83895=CARTESIAN_POINT ( 'NONE',  ( -19.02544592524334988, -5.153800228976617603, 28.95942372801900433 ) ) ;
#83896=CARTESIAN_POINT ( 'NONE',  ( -16.46253265017160317, 9.564922557960807481, 115.8322429386477097 ) ) ;
#83897=CARTESIAN_POINT ( 'NONE',  ( 8.224510206698742110, 14.34966873604972548, 112.0844237280190185 ) ) ;
#83898=CARTESIAN_POINT ( 'NONE',  ( 18.62759615963255655, 10.81492255796105972, 51.66775706135234714 ) ) ;
#83900=CARTESIAN_POINT ( 'NONE',  ( 8.224510206698742110, 14.34966873604972548, 52.08442372801901854 ) ) ;
#83901=CARTESIAN_POINT ( 'NONE',  ( -12.06949235617756955, 12.14591786802309770, 30.62390960531436335 ) ) ;
#83902=CARTESIAN_POINT ( 'NONE',  ( 9.564922557960805705, 16.46253265017160317, 49.58224293864770260 ) ) ;
#83903=CARTESIAN_POINT ( 'NONE',  ( -8.224510206698735004, -14.34966873604973081, 99.58442372801900433 ) ) ;
#83904=CARTESIAN_POINT ( 'NONE',  ( 4.483927247898790824, -16.52544592524335698, 20.20942372801900788 ) ) ;
#83905=CARTESIAN_POINT ( 'NONE',  ( -0.05219959533909027116, -19.03943276465977164, 47.49890960531435979 ) ) ;
#83906=CARTESIAN_POINT ( 'NONE',  ( 4.379528057220339221, -16.55341960407611168, 112.7072429386476955 ) ) ;
#83907=CARTESIAN_POINT ( 'NONE',  ( -10.81492255796078084, -18.62759615963271287, 112.0822429386477097 ) ) ;
#83908=CARTESIAN_POINT ( 'NONE',  ( -19.05341960407611168, -5.049401038298163336, 41.45724293864769550 ) ) ;
#83909=CARTESIAN_POINT ( 'NONE',  ( 19.02544592524343514, -5.153800228976328945, 103.5405762719809957 ) ) ;
#83910=CARTESIAN_POINT ( 'NONE',  ( -9.474510206698964154, 16.51473224551069663, 35.41557627198102409 ) ) ;
#83911=CARTESIAN_POINT ( 'NONE',  ( 9.474510206698971260, -16.51473224551069308, 107.9155762719810383 ) ) ;
#83914=CARTESIAN_POINT ( 'NONE',  ( -0.05219959533909027116, -19.03943276465977164, 92.49890960531436690 ) ) ;
#83915=CARTESIAN_POINT ( 'NONE',  ( 21.55341960407619695, -5.719274019375665929, 51.04275706135234714 ) ) ;
#83916=CARTESIAN_POINT ( 'NONE',  ( 16.55341960407611168, 4.379528057220329451, 108.9572429386476955 ) ) ;
#83917=CARTESIAN_POINT ( 'NONE',  ( 5.153800228976335163, 19.02544592524342804, 109.7905762719810099 ) ) ;
#83918=CARTESIAN_POINT ( 'NONE',  ( -9.474510206698720793, -16.51473224551083518, 69.58442372801901854 ) ) ;
#83919=CARTESIAN_POINT ( 'NONE',  ( 12.06949235617739724, 12.14591786802326823, 61.87609039468568284 ) ) ;
#83921=CARTESIAN_POINT ( 'NONE',  ( -15.80617190586768217, 15.72974639402176855, 88.12609039468570415 ) ) ;
#83922=CARTESIAN_POINT ( 'NONE',  ( 8.314922557961029526, -14.29746914071037800, 60.41775706135235424 ) ) ;
#83923=CARTESIAN_POINT ( 'NONE',  ( -0.05219959533909027116, -19.03943276465977164, 82.49890960531436690 ) ) ;
#83924=CARTESIAN_POINT ( 'NONE',  ( -12.14591786802326823, 12.06949235617739902, 38.12609039468567573 ) ) ;
#83925=CARTESIAN_POINT ( 'NONE',  ( -9.474510206698720793, -16.51473224551083518, 104.5844237280190043 ) ) ;
#83926=CARTESIAN_POINT ( 'NONE',  ( -4.483927247898782831, 16.52544592524335698, 82.70942372801900433 ) ) ;
#83927=CARTESIAN_POINT ( 'NONE',  ( -16.46253265017146816, -9.564922557961047289, 99.16775706135233293 ) ) ;
#83928=CARTESIAN_POINT ( 'NONE',  ( -19.02544592524342804, 5.153800228976336051, 81.04057627198103830 ) ) ;
#83929=CARTESIAN_POINT ( 'NONE',  ( -21.52544592524343514, 5.823673210054127303, 101.0405762719810383 ) ) ;
#83930=CARTESIAN_POINT ( 'NONE',  ( -16.52544592524342804, 4.483927247898546575, 86.04057627198102409 ) ) ;
#83931=CARTESIAN_POINT ( 'NONE',  ( 13.97604488694548053, -13.89961937509957401, 110.6260903946856615 ) ) ;
#83932=CARTESIAN_POINT ( 'NONE',  ( -12.06949235617739369, -12.14591786802326823, 74.37609039468568994 ) ) ;
#83934=CARTESIAN_POINT ( 'NONE',  ( 0.05219959533936267826, -19.03943276465977164, 75.00109039468566152 ) ) ;
#83935=CARTESIAN_POINT ( 'NONE',  ( -12.06949235617756955, 12.14591786802309770, 30.62390960531436335 ) ) ;
#83936=CARTESIAN_POINT ( 'NONE',  ( 4.483927247898545687, 16.52544592524342804, 89.79057627198103830 ) ) ;
#83937=CARTESIAN_POINT ( 'NONE',  ( -9.564922557961040184, 16.46253265017147172, 32.91775706135233293 ) ) ;
#83938=CARTESIAN_POINT ( 'NONE',  ( -16.19135201231366139, 7.376712067591927990, 89.81319145947971094 ) ) ;
#83939=CARTESIAN_POINT ( 'NONE',  ( 18.62759615963255655, 10.81492255796105972, 21.66775706135235069 ) ) ;
#83940=CARTESIAN_POINT ( 'NONE',  ( 16.46253265017146816, 9.564922557961045513, 96.66775706135233293 ) ) ;
#83941=CARTESIAN_POINT ( 'NONE',  ( -5.049401038298153566, 19.05341960407611168, 110.2072429386476671 ) ) ;
#83942=CARTESIAN_POINT ( 'NONE',  ( 9.564922557960805705, 16.46253265017160317, 94.58224293864769550 ) ) ;
#83943=CARTESIAN_POINT ( 'NONE',  ( 18.62759615963255655, 10.81492255796105972, 96.66775706135234714 ) ) ;
#83944=CARTESIAN_POINT ( 'NONE',  ( -13.97604488694527625, -13.89961937509977652, 71.87390960531433848 ) ) ;
#83945=CARTESIAN_POINT ( 'NONE',  ( -18.62759615963270932, 10.81492255796079327, 40.83224293864769550 ) ) ;
#83946=CARTESIAN_POINT ( 'NONE',  ( -14.29746914071049879, 8.314922557960819915, 90.83224293864769550 ) ) ;
#83947=CARTESIAN_POINT ( 'NONE',  ( -13.89961937509977652, 13.97604488694528158, 50.62390960531435979 ) ) ;
#83948=CARTESIAN_POINT ( 'NONE',  ( 8.224510206698953496, -14.34966873604960469, 112.9155762719810383 ) ) ;
#83949=CARTESIAN_POINT ( 'NONE',  ( -5.719274019375665041, -21.55341960407619695, 24.79275706135235779 ) ) ;
#83950=CARTESIAN_POINT ( 'NONE',  ( -21.53943276465977519, -0.05219959533937600094, 58.75109039468568994 ) ) ;
#83951=CARTESIAN_POINT ( 'NONE',  ( 5.153800228976335163, 19.02544592524342804, 44.79057627198103830 ) ) ;
#83952=CARTESIAN_POINT ( 'NONE',  ( -16.53943276465976808, -0.05219959533934237506, 83.75109039468568994 ) ) ;
#83953=CARTESIAN_POINT ( 'NONE',  ( -10.81492255796105439, 18.62759615963255655, 22.91775706135235069 ) ) ;
#83955=CARTESIAN_POINT ( 'NONE',  ( 5.823673210054125526, 21.52544592524343514, 114.7905762719810383 ) ) ;
#83956=CARTESIAN_POINT ( 'NONE',  ( 13.97604488694548053, -13.89961937509957401, 50.62609039468566152 ) ) ;
#83957=CARTESIAN_POINT ( 'NONE',  ( 9.474510206698971260, -16.51473224551069308, 67.91557627198102409 ) ) ;
#83958=CARTESIAN_POINT ( 'NONE',  ( -19.05341960407617563, 5.049401038297882671, 33.54275706135231871 ) ) ;
#83959=CARTESIAN_POINT ( 'NONE',  ( -15.72974639402176322, -15.80617190586768395, 64.37609039468568994 ) ) ;
#83960=CARTESIAN_POINT ( 'NONE',  ( -15.72974639402197994, 15.80617190586746368, 70.62390960531436690 ) ) ;
#83961=CARTESIAN_POINT ( 'NONE',  ( -8.314922557960811034, -14.29746914071050412, 47.08224293864770260 ) ) ;
#83962=CARTESIAN_POINT ( 'NONE',  ( 5.823673210054444382, -21.52544592524334988, 95.20942372801903275 ) ) ;
#83963=CARTESIAN_POINT ( 'NONE',  ( -19.02544592524334988, -5.153800228976617603, 23.95942372801900078 ) ) ;
#83964=CARTESIAN_POINT ( 'NONE',  ( -12.06949235617756955, 12.14591786802309770, 65.62390960531436690 ) ) ;
#83965=CARTESIAN_POINT ( 'NONE',  ( -12.06949235617756955, 12.14591786802309770, 100.6239096053143811 ) ) ;
#83966=CARTESIAN_POINT ( 'NONE',  ( -9.474510206698720793, -16.51473224551083518, 54.58442372801899722 ) ) ;
#83967=CARTESIAN_POINT ( 'NONE',  ( -4.483927247898539470, -16.52544592524342804, 22.29057627198102765 ) ) ;
#83968=CARTESIAN_POINT ( 'NONE',  ( 5.823673210054444382, -21.52544592524334988, 75.20942372801901854 ) ) ;
#83969=CARTESIAN_POINT ( 'NONE',  ( -9.474510206698720793, -16.51473224551083518, 54.58442372801899722 ) ) ;
#83970=CARTESIAN_POINT ( 'NONE',  ( 18.62759615963271287, -10.81492255796078972, 58.33224293864768839 ) ) ;
#83971=CARTESIAN_POINT ( 'NONE',  ( -15.72974639402176322, -15.80617190586768395, 49.37609039468569705 ) ) ;
#83972=CARTESIAN_POINT ( 'NONE',  ( -21.53943276465977519, 0.05219959533907696930, 106.2489096053143811 ) ) ;
#83973=CARTESIAN_POINT ( 'NONE',  ( -16.46253265017146816, -9.564922557961047289, 104.1677570613523329 ) ) ;
#83974=CARTESIAN_POINT ( 'NONE',  ( 12.14591786802327356, -12.06949235617739191, 65.62609039468568994 ) ) ;
#83975=CARTESIAN_POINT ( 'NONE',  ( -17.60728821186567927, 5.500000000000037303, 55.86690927743004664 ) ) ;
#83976=CARTESIAN_POINT ( 'NONE',  ( 5.719274019375991003, -21.55341960407610458, 102.7072429386476955 ) ) ;
#83977=CARTESIAN_POINT ( 'NONE',  ( -12.06949235617756955, 12.14591786802309770, 85.62390960531436690 ) ) ;
#83978=CARTESIAN_POINT ( 'NONE',  ( -16.62475595723698873, -7.163666690055323194, 99.47286648189528080 ) ) ;
#83979=CARTESIAN_POINT ( 'NONE',  ( 4.483927247898790824, -16.52544592524335698, 25.20942372801901854 ) ) ;
#83981=CARTESIAN_POINT ( 'NONE',  ( 21.53943276465977519, -0.05219959533907433946, 48.74890960531435979 ) ) ;
#83982=CARTESIAN_POINT ( 'NONE',  ( 14.34966873604972726, -8.224510206698740333, 85.83442372801901854 ) ) ;
#83984=CARTESIAN_POINT ( 'NONE',  ( 14.29746914071037800, 8.314922557961029526, 66.66775706135234714 ) ) ;
#83985=CARTESIAN_POINT ( 'NONE',  ( 21.52544592524334988, 5.823673210054432836, 36.45942372801901143 ) ) ;
#83986=CARTESIAN_POINT ( 'NONE',  ( 21.52544592524344225, -5.823673210054117533, 53.54057627198103120 ) ) ;
#83987=CARTESIAN_POINT ( 'NONE',  ( 14.34966873604972726, -8.224510206698740333, 85.83442372801901854 ) ) ;
#83988=CARTESIAN_POINT ( 'NONE',  ( 19.02544592524343514, -5.153800228976328945, 93.54057627198102409 ) ) ;
#83989=CARTESIAN_POINT ( 'NONE',  ( -18.67979575497193778, 10.72451020669871902, 73.33442372801901854 ) ) ;
#83990=CARTESIAN_POINT ( 'NONE',  ( -0.05219959533907301413, -21.53943276465977519, 47.49890960531435979 ) ) ;
#83991=CARTESIAN_POINT ( 'NONE',  ( 5.719274019375991003, -21.55341960407610458, 32.70724293864770260 ) ) ;
#83993=CARTESIAN_POINT ( 'NONE',  ( -5.153800228976607833, 19.02544592524334988, 47.70942372801900433 ) ) ;
#83994=CARTESIAN_POINT ( 'NONE',  ( 12.06949235617739724, 12.14591786802326823, 66.87609039468568994 ) ) ;
#83995=CARTESIAN_POINT ( 'NONE',  ( -5.719274019375978568, 21.55341960407610458, 30.20724293864769550 ) ) ;
#83997=CARTESIAN_POINT ( 'NONE',  ( -9.474510206698964154, 16.51473224551069663, 100.4155762719810241 ) ) ;
#83998=CARTESIAN_POINT ( 'NONE',  ( 14.29746914071049879, -8.314922557960816363, 23.33224293864769194 ) ) ;
#83999=CARTESIAN_POINT ( 'NONE',  ( -17.72517630440434644, 5.499999999999979572, 85.92175719257211597 ) ) ;
#84000=CARTESIAN_POINT ( 'NONE',  ( -16.55341960407611168, -4.379528057220339221, 111.4572429386476813 ) ) ;
#84001=CARTESIAN_POINT ( 'NONE',  ( -21.52544592524343514, 5.823673210054127303, 51.04057627198103120 ) ) ;
#84002=CARTESIAN_POINT ( 'NONE',  ( 19.03943276465977164, -0.05219959533909143690, 38.74890960531436690 ) ) ;
#84004=CARTESIAN_POINT ( 'NONE',  ( 14.34966873604972726, -8.224510206698740333, 95.83442372801903275 ) ) ;
#84005=CARTESIAN_POINT ( 'NONE',  ( -5.719274019375665041, -21.55341960407619695, 34.79275706135235424 ) ) ;
#84006=CARTESIAN_POINT ( 'NONE',  ( -19.05341960407617563, 5.049401038297882671, 88.54275706135230450 ) ) ;
#84007=CARTESIAN_POINT ( 'NONE',  ( -16.53943276465976808, 0.05219959533911058130, 106.2489096053143811 ) ) ;
#84008=CARTESIAN_POINT ( 'NONE',  ( -13.97604488694527625, -13.89961937509977652, 51.87390960531436690 ) ) ;
#84009=CARTESIAN_POINT ( 'NONE',  ( -9.564922557960796823, -16.46253265017161027, 27.08224293864769550 ) ) ;
#84011=CARTESIAN_POINT ( 'NONE',  ( -13.89961937509977652, 13.97604488694528158, 75.62390960531438111 ) ) ;
#84012=CARTESIAN_POINT ( 'NONE',  ( -12.06949235617739369, -12.14591786802326823, 59.37609039468568284 ) ) ;
#84013=CARTESIAN_POINT ( 'NONE',  ( 0.05219959533937995610, -21.53943276465977519, 110.0010903946856757 ) ) ;
#84014=CARTESIAN_POINT ( 'NONE',  ( 5.823673210054125526, 21.52544592524343514, 44.79057627198103120 ) ) ;
#84015=CARTESIAN_POINT ( 'NONE',  ( -16.52544592524335698, -4.483927247898792601, 73.95942372801901854 ) ) ;
#84016=CARTESIAN_POINT ( 'NONE',  ( -16.51473224551082808, 9.474510206698731452, 48.33442372801900433 ) ) ;
#84017=CARTESIAN_POINT ( 'NONE',  ( 19.02544592524334988, 5.153800228976608722, 61.45942372801900433 ) ) ;
#84018=CARTESIAN_POINT ( 'NONE',  ( -10.72451020669870658, -18.67979575497194134, 64.58442372801900433 ) ) ;
#84019=CARTESIAN_POINT ( 'NONE',  ( -19.02544592524342804, 5.153800228976336051, 61.04057627198103120 ) ) ;
#84020=CARTESIAN_POINT ( 'NONE',  ( -19.03943276465977164, 0.05219959533909376836, 31.24890960531435979 ) ) ;
#84021=CARTESIAN_POINT ( 'NONE',  ( -9.564922557961040184, 16.46253265017147172, 62.91775706135233293 ) ) ;
#84022=CARTESIAN_POINT ( 'NONE',  ( 9.474510206698971260, -16.51473224551069308, 107.9155762719810383 ) ) ;
#84023=CARTESIAN_POINT ( 'NONE',  ( 9.474510206698971260, -16.51473224551069308, 97.91557627198102409 ) ) ;
#84024=CARTESIAN_POINT ( 'NONE',  ( 8.224510206698953496, -14.34966873604960469, 52.91557627198103830 ) ) ;
#84025=CARTESIAN_POINT ( 'NONE',  ( -5.719274019375978568, 21.55341960407610458, 45.20724293864769550 ) ) ;
#84026=CARTESIAN_POINT ( 'NONE',  ( -17.50000000000000000, 3.305555262949662954, 104.6251715215659459 ) ) ;
#84027=CARTESIAN_POINT ( 'NONE',  ( 5.823673210054444382, -21.52544592524334988, 105.2094237280190328 ) ) ;
#84029=CARTESIAN_POINT ( 'NONE',  ( -16.51473224551069308, -9.474510206698971260, 56.66557627198103120 ) ) ;
#84032=CARTESIAN_POINT ( 'NONE',  ( 8.224510206698742110, 14.34966873604972548, 72.08442372801899012 ) ) ;
#84033=CARTESIAN_POINT ( 'NONE',  ( 10.81492255796078972, 18.62759615963270932, 94.58224293864769550 ) ) ;
#84034=CARTESIAN_POINT ( 'NONE',  ( 8.314922557960818139, 14.29746914071049879, 49.58224293864769550 ) ) ;
#84035=CARTESIAN_POINT ( 'NONE',  ( -16.46253265017160317, 9.564922557960807481, 35.83224293864768839 ) ) ;
#84036=CARTESIAN_POINT ( 'NONE',  ( -9.474510206698964154, 16.51473224551069663, 115.4155762719810241 ) ) ;
#84037=CARTESIAN_POINT ( 'NONE',  ( -10.72451020669870658, -18.67979575497194134, 39.58442372801901143 ) ) ;
#84038=CARTESIAN_POINT ( 'NONE',  ( -19.02544592524334988, -5.153800228976617603, 48.95942372801900433 ) ) ;
#84039=CARTESIAN_POINT ( 'NONE',  ( 13.89961937509977652, -13.97604488694527269, 43.12390960531434558 ) ) ;
#84040=CARTESIAN_POINT ( 'NONE',  ( 15.80617190586769283, -15.72974639402175789, 90.62609039468567573 ) ) ;
#84041=CARTESIAN_POINT ( 'NONE',  ( 17.40861289039002457, 6.110651285853315073, 98.87232470827433417 ) ) ;
#84043=CARTESIAN_POINT ( 'NONE',  ( -14.34966873604960291, -8.224510206698953496, 46.66557627198102409 ) ) ;
#84045=CARTESIAN_POINT ( 'NONE',  ( 10.72451020669898902, -18.67979575497178502, 42.91557627198103120 ) ) ;
#84047=CARTESIAN_POINT ( 'NONE',  ( -19.05341960407611168, -5.049401038298163336, 106.4572429386476955 ) ) ;
#84048=CARTESIAN_POINT ( 'NONE',  ( -16.55341960407611168, -4.379528057220339221, 86.45724293864770971 ) ) ;
#84049=CARTESIAN_POINT ( 'NONE',  ( -8.314922557961024197, 14.29746914071037800, 27.91775706135234358 ) ) ;
#84051=CARTESIAN_POINT ( 'NONE',  ( -16.55341960407611168, -4.379528057220339221, 21.45724293864769550 ) ) ;
#84053=CARTESIAN_POINT ( 'NONE',  ( -0.05219959533909027116, -19.03943276465977164, 102.4989096053143669 ) ) ;
#84054=CARTESIAN_POINT ( 'NONE',  ( 21.53943276465977519, -0.05219959533907433946, 98.74890960531438111 ) ) ;
#84055=CARTESIAN_POINT ( 'NONE',  ( -14.29746914071049879, 8.314922557960819915, 25.83224293864769194 ) ) ;
#84056=CARTESIAN_POINT ( 'NONE',  ( -9.474510206698964154, 16.51473224551069663, 95.41557627198102409 ) ) ;
#84057=CARTESIAN_POINT ( 'NONE',  ( -13.89961937509957401, -13.97604488694547875, 99.37609039468567573 ) ) ;
#84058=CARTESIAN_POINT ( 'NONE',  ( -15.80617190586768217, 15.72974639402176855, 113.1260903946856899 ) ) ;
#84059=CARTESIAN_POINT ( 'NONE',  ( 5.823673210054125526, 21.52544592524343514, 94.79057627198105251 ) ) ;
#84060=CARTESIAN_POINT ( 'NONE',  ( 10.81492255796078972, 18.62759615963270932, 44.58224293864769550 ) ) ;
#84061=CARTESIAN_POINT ( 'NONE',  ( 9.474510206698971260, -16.51473224551069308, 57.91557627198103120 ) ) ;
#84062=CARTESIAN_POINT ( 'NONE',  ( 8.224510206698953496, -14.34966873604960469, 32.91557627198102409 ) ) ;
#84063=CARTESIAN_POINT ( 'NONE',  ( 5.049401038298161559, -19.05341960407611168, 82.70724293864770971 ) ) ;
#84065=CARTESIAN_POINT ( 'NONE',  ( -0.05219959533936034679, 19.03943276465977164, 32.50109039468566863 ) ) ;
#84066=CARTESIAN_POINT ( 'NONE',  ( 8.224510206698953496, -14.34966873604960469, 92.91557627198103830 ) ) ;
#84067=CARTESIAN_POINT ( 'NONE',  ( 21.53943276465977519, 0.05219959533937863772, 21.25109039468567218 ) ) ;
#84069=CARTESIAN_POINT ( 'NONE',  ( 0.05219959533934541429, -16.53943276465976808, 110.0010903946856757 ) ) ;
#84070=CARTESIAN_POINT ( 'NONE',  ( 16.51473224551069308, 9.474510206698969483, 24.16557627198102765 ) ) ;
#84071=CARTESIAN_POINT ( 'NONE',  ( 16.46253265017160672, -9.564922557960803928, 78.33224293864769550 ) ) ;
#84073=CARTESIAN_POINT ( 'NONE',  ( -14.34966873604960291, -8.224510206698953496, 46.66557627198102409 ) ) ;
#84074=CARTESIAN_POINT ( 'NONE',  ( -21.53943276465977519, -0.05219959533937600094, 53.75109039468568994 ) ) ;
#84076=CARTESIAN_POINT ( 'NONE',  ( -18.67979575497193778, 10.72451020669871902, 88.33442372801901854 ) ) ;
#84077=CARTESIAN_POINT ( 'NONE',  ( 19.02544592524343514, -5.153800228976328945, 48.54057627198103120 ) ) ;
#84078=CARTESIAN_POINT ( 'NONE',  ( -0.05219959533909027116, -19.03943276465977164, 52.49890960531436690 ) ) ;
#84080=CARTESIAN_POINT ( 'NONE',  ( -15.72974639402176322, -15.80617190586768395, 89.37609039468568994 ) ) ;
#84081=CARTESIAN_POINT ( 'NONE',  ( 16.55341960407618274, -4.379528057220086978, 56.04275706135235424 ) ) ;
#84082=CARTESIAN_POINT ( 'NONE',  ( 5.823673210054444382, -21.52544592524334988, 80.20942372801901854 ) ) ;
#84083=CARTESIAN_POINT ( 'NONE',  ( 5.153800228976335163, 19.02544592524342804, 114.7905762719810241 ) ) ;
#84084=CARTESIAN_POINT ( 'NONE',  ( -9.474510206698720793, -16.51473224551083518, 89.58442372801900433 ) ) ;
#84085=CARTESIAN_POINT ( 'NONE',  ( 15.80617190586769283, -15.72974639402175789, 70.62609039468567573 ) ) ;
#84086=CARTESIAN_POINT ( 'NONE',  ( -0.05219959533934338120, 16.53943276465976808, 37.50109039468568284 ) ) ;
#84087=CARTESIAN_POINT ( 'NONE',  ( -21.55341960407610458, -5.719274019375992779, 86.45724293864770971 ) ) ;
#84088=CARTESIAN_POINT ( 'NONE',  ( 19.05341960407617918, -5.049401038297876454, 91.04275706135234714 ) ) ;
#84089=CARTESIAN_POINT ( 'NONE',  ( -9.564922557960796823, -16.46253265017161027, 67.08224293864769550 ) ) ;
#84090=CARTESIAN_POINT ( 'NONE',  ( -19.02544592524334988, -5.153800228976617603, 98.95942372801900433 ) ) ;
#84092=CARTESIAN_POINT ( 'NONE',  ( -9.564922557961040184, 16.46253265017147172, 107.9177570613523471 ) ) ;
#84093=CARTESIAN_POINT ( 'NONE',  ( -4.483927247898539470, -16.52544592524342804, 52.29057627198102409 ) ) ;
#84094=CARTESIAN_POINT ( 'NONE',  ( 13.89961937509957401, 13.97604488694547697, 76.87609039468566152 ) ) ;
#84095=CARTESIAN_POINT ( 'NONE',  ( 4.483927247898790824, -16.52544592524335698, 55.20942372801902565 ) ) ;
#84096=CARTESIAN_POINT ( 'NONE',  ( -5.153800228976328057, -19.02544592524343514, 42.29057627198101699 ) ) ;
#84097=CARTESIAN_POINT ( 'NONE',  ( -9.564922557960796823, -16.46253265017161027, 57.08224293864769550 ) ) ;
#84098=CARTESIAN_POINT ( 'NONE',  ( 16.53943276465976808, 0.05219959533934440121, 61.25109039468567573 ) ) ;
#84101=CARTESIAN_POINT ( 'NONE',  ( -9.474510206698964154, 16.51473224551069663, 110.4155762719810383 ) ) ;
#84103=EDGE_LOOP ( 'NONE', ( #190428, #31418, #167975 ) ) ;
#84104=CARTESIAN_POINT ( 'NONE',  ( 13.89961937509957401, 13.97604488694547697, 111.8760903946856757 ) ) ;
#84105=CARTESIAN_POINT ( 'NONE',  ( -21.53943276465977519, 0.05219959533907696930, 36.24890960531435979 ) ) ;
#84106=CARTESIAN_POINT ( 'NONE',  ( 5.049401038297881783, 19.05341960407617563, 37.29275706135232582 ) ) ;
#84107=CARTESIAN_POINT ( 'NONE',  ( -4.379528057220086978, -16.55341960407618274, 24.79275706135235779 ) ) ;
#84108=CARTESIAN_POINT ( 'NONE',  ( 13.89961937509977652, -13.97604488694527269, 28.12390960531435624 ) ) ;
#84109=CARTESIAN_POINT ( 'NONE',  ( -13.89961937509977652, 13.97604488694528158, 55.62390960531434558 ) ) ;
#84110=CARTESIAN_POINT ( 'NONE',  ( -15.72974639402197994, 15.80617190586746368, 80.62390960531438111 ) ) ;
#84111=CARTESIAN_POINT ( 'NONE',  ( 9.474510206698971260, -16.51473224551069308, 97.91557627198102409 ) ) ;
#84112=CARTESIAN_POINT ( 'NONE',  ( -5.049401038298153566, 19.05341960407611168, 50.20724293864770260 ) ) ;
#84114=CARTESIAN_POINT ( 'NONE',  ( 19.03943276465977164, 0.05219959533936151252, 86.25109039468567573 ) ) ;
#84115=CARTESIAN_POINT ( 'NONE',  ( -12.14591786802309592, -12.06949235617757132, 71.87390960531438111 ) ) ;
#84116=CARTESIAN_POINT ( 'NONE',  ( 5.719274019375991003, -21.55341960407610458, 52.70724293864769550 ) ) ;
#84117=CARTESIAN_POINT ( 'NONE',  ( -15.80617190586768217, 15.72974639402176855, 113.1260903946856899 ) ) ;
#84118=CARTESIAN_POINT ( 'NONE',  ( -21.52544592524343514, 5.823673210054127303, 91.04057627198103830 ) ) ;
#84119=CARTESIAN_POINT ( 'NONE',  ( 5.823673210054444382, -21.52544592524334988, 75.20942372801901854 ) ) ;
#84120=CARTESIAN_POINT ( 'NONE',  ( 18.62759615963255655, 10.81492255796105972, 81.66775706135236135 ) ) ;
#84121=CARTESIAN_POINT ( 'NONE',  ( -13.97604488694527625, -13.89961937509977652, 111.8739096053143243 ) ) ;
#84122=CARTESIAN_POINT ( 'NONE',  ( -16.55341960407617563, 4.379528057220093196, 103.5427570613523613 ) ) ;
#84123=CARTESIAN_POINT ( 'NONE',  ( -21.55341960407619339, 5.719274019375674811, 78.54275706135236135 ) ) ;
#84124=CARTESIAN_POINT ( 'NONE',  ( -5.153800228976328057, -19.02544592524343514, 72.29057627198102409 ) ) ;
#84125=CARTESIAN_POINT ( 'NONE',  ( -5.823673210054431948, 21.52544592524334988, 32.70942372801900433 ) ) ;
#84126=CARTESIAN_POINT ( 'NONE',  ( -5.153800228976328057, -19.02544592524343514, 67.29057627198102409 ) ) ;
#84127=CARTESIAN_POINT ( 'NONE',  ( 4.483927247898545687, 16.52544592524342804, 74.79057627198105251 ) ) ;
#84128=CARTESIAN_POINT ( 'NONE',  ( 4.483927247898545687, 16.52544592524342804, 44.79057627198103120 ) ) ;
#84129=CARTESIAN_POINT ( 'NONE',  ( 18.67979575497178502, 10.72451020669898547, 54.16557627198103120 ) ) ;
#84130=CARTESIAN_POINT ( 'NONE',  ( -5.153800228976328057, -19.02544592524343514, 67.29057627198102409 ) ) ;
#84131=CARTESIAN_POINT ( 'NONE',  ( -18.62759615963270932, 10.81492255796079327, 65.83224293864769550 ) ) ;
#84132=CARTESIAN_POINT ( 'NONE',  ( -5.049401038297874678, -19.05341960407617918, 64.79275706135233293 ) ) ;
#84133=CARTESIAN_POINT ( 'NONE',  ( 0.05219959533936267826, -19.03943276465977164, 20.00109039468567218 ) ) ;
#84134=CARTESIAN_POINT ( 'NONE',  ( -8.224510206698948167, 14.34966873604960824, 60.41557627198102409 ) ) ;
#84135=CARTESIAN_POINT ( 'NONE',  ( 5.823673210054125526, 21.52544592524343514, 49.79057627198102409 ) ) ;
#84137=CARTESIAN_POINT ( 'NONE',  ( -22.00000000000000000, -1.163414459189985801E-14, 97.50000000000000000 ) ) ;
#84138=CARTESIAN_POINT ( 'NONE',  ( -16.55341960407617563, 4.379528057220093196, 103.5427570613523613 ) ) ;
#84140=CARTESIAN_POINT ( 'NONE',  ( 0.05219959533936267826, -19.03943276465977164, 85.00109039468567573 ) ) ;
#84141=CARTESIAN_POINT ( 'NONE',  ( -4.379528057220328563, 16.55341960407611168, 70.20724293864769550 ) ) ;
#84143=CARTESIAN_POINT ( 'NONE',  ( 0.05219959533909260263, 19.03943276465977164, 59.99890960531436690 ) ) ;
#84144=CARTESIAN_POINT ( 'NONE',  ( -0.05219959533910754901, -16.53943276465976808, 52.49890960531435979 ) ) ;
#84145=CARTESIAN_POINT ( 'NONE',  ( 16.46253265017160672, -9.564922557960803928, 83.33224293864768129 ) ) ;
#84146=CARTESIAN_POINT ( 'NONE',  ( -9.474510206698720793, -16.51473224551083518, 74.58442372801900433 ) ) ;
#84147=CARTESIAN_POINT ( 'NONE',  ( -19.02544592524342804, 5.153800228976336051, 56.04057627198100988 ) ) ;
#84148=CARTESIAN_POINT ( 'NONE',  ( -19.05341960407611168, -5.049401038298163336, 81.45724293864769550 ) ) ;
#84149=CARTESIAN_POINT ( 'NONE',  ( -13.97604488694527625, -13.89961937509977652, 66.87390960531436690 ) ) ;
#84150=CARTESIAN_POINT ( 'NONE',  ( 15.80617190586746368, 15.72974639402197994, 64.37390960531435269 ) ) ;
#84152=CARTESIAN_POINT ( 'NONE',  ( -13.97604488694527625, -13.89961937509977652, 46.87390960531435979 ) ) ;
#84153=CARTESIAN_POINT ( 'NONE',  ( -5.823673210054116645, -21.52544592524344225, 57.29057627198103120 ) ) ;
#84154=CARTESIAN_POINT ( 'NONE',  ( -9.474510206698720793, -16.51473224551083518, 84.58442372801900433 ) ) ;
#84155=CARTESIAN_POINT ( 'NONE',  ( -16.53943276465976808, -0.05219959533934237506, 113.7510903946856757 ) ) ;
#84156=CARTESIAN_POINT ( 'NONE',  ( -16.51473224551082808, 9.474510206698731452, 33.33442372801899722 ) ) ;
#84157=CARTESIAN_POINT ( 'NONE',  ( 12.14591786802327356, -12.06949235617739191, 60.62609039468567573 ) ) ;
#84158=CARTESIAN_POINT ( 'NONE',  ( -0.05219959533934338120, 16.53943276465976808, 87.50109039468568994 ) ) ;
#84160=CARTESIAN_POINT ( 'NONE',  ( 8.224510206698742110, 14.34966873604972548, 87.08442372801901854 ) ) ;
#84161=CARTESIAN_POINT ( 'NONE',  ( -9.474510206698964154, 16.51473224551069663, 115.4155762719810241 ) ) ;
#84162=CARTESIAN_POINT ( 'NONE',  ( 5.049401038298161559, -19.05341960407611168, 37.70724293864768839 ) ) ;
#84163=CARTESIAN_POINT ( 'NONE',  ( -4.379528057220086978, -16.55341960407618274, 34.79275706135235424 ) ) ;
#84164=CARTESIAN_POINT ( 'NONE',  ( 5.153800228976335163, 19.02544592524342804, 49.79057627198100988 ) ) ;
#84165=CARTESIAN_POINT ( 'NONE',  ( 18.67979575497194134, -10.72451020669871369, 40.83442372801901854 ) ) ;
#84166=CARTESIAN_POINT ( 'NONE',  ( 8.314922557961029526, -14.29746914071037800, 55.41775706135234714 ) ) ;
#84167=CARTESIAN_POINT ( 'NONE',  ( -16.53943276465976808, -0.05219959533934237506, 108.7510903946857042 ) ) ;
#84168=CARTESIAN_POINT ( 'NONE',  ( -13.97604488694527625, -13.89961937509977652, 26.87390960531434558 ) ) ;
#84169=CARTESIAN_POINT ( 'NONE',  ( 19.03943276465977164, 0.05219959533936151252, 21.25109039468565797 ) ) ;
#84170=CARTESIAN_POINT ( 'NONE',  ( -0.05219959533936034679, 19.03943276465977164, 112.5010903946856757 ) ) ;
#84171=CARTESIAN_POINT ( 'NONE',  ( 16.46253265017146816, 9.564922557961045513, 71.66775706135233293 ) ) ;
#84172=CARTESIAN_POINT ( 'NONE',  ( 4.483927247898545687, 16.52544592524342804, 69.79057627198102409 ) ) ;
#84173=CARTESIAN_POINT ( 'NONE',  ( -16.51473224551069308, -9.474510206698971260, 36.66557627198102409 ) ) ;
#84174=CARTESIAN_POINT ( 'NONE',  ( 16.51473224551083163, -9.474510206698727899, 70.83442372801900433 ) ) ;
#84175=CARTESIAN_POINT ( 'NONE',  ( 17.31747979337948706, -6.344076630961054342, 91.12055131934815222 ) ) ;
#84176=CARTESIAN_POINT ( 'NONE',  ( -21.53943276465977519, -0.05219959533937600094, 83.75109039468568994 ) ) ;
#84177=CARTESIAN_POINT ( 'NONE',  ( -12.06949235617739369, -12.14591786802326823, 39.37609039468567573 ) ) ;
#84179=CARTESIAN_POINT ( 'NONE',  ( 15.80617190586746368, 15.72974639402197994, 34.37390960531435979 ) ) ;
#84180=CARTESIAN_POINT ( 'NONE',  ( -12.14591786802326823, 12.06949235617739902, 23.12609039468567573 ) ) ;
#84181=CARTESIAN_POINT ( 'NONE',  ( -5.049401038298153566, 19.05341960407611168, 115.2072429386477097 ) ) ;
#84183=CARTESIAN_POINT ( 'NONE',  ( 13.97604488694527802, 13.89961937509977652, 34.37390960531436690 ) ) ;
#84185=CARTESIAN_POINT ( 'NONE',  ( -13.89961937509977652, 13.97604488694528158, 55.62390960531434558 ) ) ;
#84186=CARTESIAN_POINT ( 'NONE',  ( 15.80617190586769283, -15.72974639402175789, 60.62609039468567573 ) ) ;
#84187=CARTESIAN_POINT ( 'NONE',  ( 15.80617190586769283, -15.72974639402175789, 105.6260903946856899 ) ) ;
#84188=CARTESIAN_POINT ( 'NONE',  ( -0.05219959533910754901, -16.53943276465976808, 22.49890960531436335 ) ) ;
#84189=CARTESIAN_POINT ( 'NONE',  ( 19.05341960407611168, 5.049401038298154454, 33.95724293864769550 ) ) ;
#84190=CARTESIAN_POINT ( 'NONE',  ( -9.474510206698964154, 16.51473224551069663, 95.41557627198102409 ) ) ;
#84191=CARTESIAN_POINT ( 'NONE',  ( -5.719274019375665041, -21.55341960407619695, 54.79275706135235424 ) ) ;
#84192=CARTESIAN_POINT ( 'NONE',  ( -0.05219959533909027116, -19.03943276465977164, 42.49890960531435269 ) ) ;
#84193=CARTESIAN_POINT ( 'NONE',  ( 5.823673210054444382, -21.52544592524334988, 65.20942372801901854 ) ) ;
#84194=CARTESIAN_POINT ( 'NONE',  ( -9.474510206698720793, -16.51473224551083518, 94.58442372801900433 ) ) ;
#84195=CARTESIAN_POINT ( 'NONE',  ( -13.89961937509977652, 13.97604488694528158, 110.6239096053143243 ) ) ;
#84196=CARTESIAN_POINT ( 'NONE',  ( 19.05341960407611168, 5.049401038298154454, 28.95724293864769550 ) ) ;
#84197=CARTESIAN_POINT ( 'NONE',  ( 5.719274019375991003, -21.55341960407610458, 107.7072429386476955 ) ) ;
#84198=CARTESIAN_POINT ( 'NONE',  ( 9.564922557961047289, -16.46253265017146816, 30.41775706135232937 ) ) ;
#84199=CARTESIAN_POINT ( 'NONE',  ( -4.379528057220328563, 16.55341960407611168, 105.2072429386477097 ) ) ;
#84200=CARTESIAN_POINT ( 'NONE',  ( -13.89961937509977652, 13.97604488694528158, 60.62390960531436690 ) ) ;
#84201=CARTESIAN_POINT ( 'NONE',  ( -16.46253265017146816, -9.564922557961047289, 94.16775706135233293 ) ) ;
#84202=CARTESIAN_POINT ( 'NONE',  ( -16.53943276465976808, 0.05219959533911058130, 61.24890960531435979 ) ) ;
#84203=CARTESIAN_POINT ( 'NONE',  ( 19.05341960407617918, -5.049401038297876454, 21.04275706135232582 ) ) ;
#84204=CARTESIAN_POINT ( 'NONE',  ( 16.46253265017160672, -9.564922557960803928, 113.3322429386476955 ) ) ;
#84205=CARTESIAN_POINT ( 'NONE',  ( -5.153800228976607833, 19.02544592524334988, 87.70942372801897591 ) ) ;
#84206=CARTESIAN_POINT ( 'NONE',  ( -5.823673210054116645, -21.52544592524344225, 97.29057627198105251 ) ) ;
#84207=CARTESIAN_POINT ( 'NONE',  ( 5.823673210054444382, -21.52544592524334988, 40.20942372801901854 ) ) ;
#84208=CARTESIAN_POINT ( 'NONE',  ( -4.379528057220086978, -16.55341960407618274, 44.79275706135234714 ) ) ;
#84209=CARTESIAN_POINT ( 'NONE',  ( 16.55341960407618274, -4.379528057220086978, 111.0427570613523613 ) ) ;
#84210=CARTESIAN_POINT ( 'NONE',  ( 8.314922557961029526, -14.29746914071037800, 35.41775706135234003 ) ) ;
#84211=CARTESIAN_POINT ( 'NONE',  ( -15.80617190586768217, 15.72974639402176855, 48.12609039468568284 ) ) ;
#84212=CARTESIAN_POINT ( 'NONE',  ( -18.67979575497178146, -10.72451020669898902, 51.66557627198102409 ) ) ;
#84213=CARTESIAN_POINT ( 'NONE',  ( 19.05341960407611168, 5.049401038298154454, 28.95724293864769550 ) ) ;
#84215=CARTESIAN_POINT ( 'NONE',  ( 14.29746914071037800, 8.314922557961029526, 76.66775706135234714 ) ) ;
#84216=EDGE_CURVE ( 'NONE', #134048, #103535, #35073, .T. ) ;
#84217=CARTESIAN_POINT ( 'NONE',  ( 21.53943276465977519, -0.05219959533907433946, 93.74890960531436690 ) ) ;
#84218=CARTESIAN_POINT ( 'NONE',  ( 16.55341960407611168, 4.379528057220329451, 33.95724293864769550 ) ) ;
#84219=CARTESIAN_POINT ( 'NONE',  ( -16.52544592524335698, -4.483927247898792601, 68.95942372801901854 ) ) ;
#84220=CARTESIAN_POINT ( 'NONE',  ( -9.474510206698720793, -16.51473224551083518, 104.5844237280190043 ) ) ;
#84221=CARTESIAN_POINT ( 'NONE',  ( -21.55341960407610458, -5.719274019375992779, 101.4572429386476955 ) ) ;
#84222=CARTESIAN_POINT ( 'NONE',  ( -12.06949235617756955, 12.14591786802309770, 35.62390960531437401 ) ) ;
#84224=CARTESIAN_POINT ( 'NONE',  ( -14.29746914071037622, -8.314922557961029526, 84.16775706135234714 ) ) ;
#84226=CARTESIAN_POINT ( 'NONE',  ( 5.823673210054125526, 21.52544592524343514, 74.79057627198105251 ) ) ;
#84227=VERTEX_POINT ( 'NONE', #152485 ) ;
#84228=CARTESIAN_POINT ( 'NONE',  ( 12.06949235617739724, 12.14591786802326823, 101.8760903946857042 ) ) ;
#84229=VERTEX_POINT ( 'NONE', #198998 ) ;
#84231=CARTESIAN_POINT ( 'NONE',  ( 0.05219959533907565091, 21.53943276465977519, 89.99890960531438111 ) ) ;
#84232=CARTESIAN_POINT ( 'NONE',  ( -18.67979575497178146, -10.72451020669898902, 106.6655762719810383 ) ) ;
#84233=CARTESIAN_POINT ( 'NONE',  ( 16.52544592524342804, -4.483927247898539470, 38.54057627198103120 ) ) ;
#84234=CARTESIAN_POINT ( 'NONE',  ( 0.05219959533934541429, -16.53943276465976808, 30.00109039468568284 ) ) ;
#84235=CARTESIAN_POINT ( 'NONE',  ( -13.89961937509977652, 13.97604488694528158, 45.62390960531433848 ) ) ;
#84236=CARTESIAN_POINT ( 'NONE',  ( -9.474510206698964154, 16.51473224551069663, 70.41557627198102409 ) ) ;
#84238=CARTESIAN_POINT ( 'NONE',  ( -10.81492255796078084, -18.62759615963271287, 27.08224293864769550 ) ) ;
#84239=CARTESIAN_POINT ( 'NONE',  ( -0.05219959533909027116, -19.03943276465977164, 112.4989096053143669 ) ) ;
#84240=CARTESIAN_POINT ( 'NONE',  ( -13.89961937509957401, -13.97604488694547875, 99.37609039468567573 ) ) ;
#84241=CARTESIAN_POINT ( 'NONE',  ( 19.03943276465977164, 0.05219959533936151252, 51.25109039468567573 ) ) ;
#84242=CARTESIAN_POINT ( 'NONE',  ( -18.62759615963270932, 10.81492255796079327, 90.83224293864769550 ) ) ;
#84243=CARTESIAN_POINT ( 'NONE',  ( -8.314922557961024197, 14.29746914071037800, 107.9177570613523471 ) ) ;
#84244=CARTESIAN_POINT ( 'NONE',  ( -18.62759615963270932, 10.81492255796079327, 50.83224293864770971 ) ) ;
#84245=CARTESIAN_POINT ( 'NONE',  ( -18.62759615963270932, 10.81492255796079327, 75.83224293864769550 ) ) ;
#84246=CARTESIAN_POINT ( 'NONE',  ( 9.564922557961047289, -16.46253265017146816, 100.4177570613523329 ) ) ;
#84247=CARTESIAN_POINT ( 'NONE',  ( 16.51473224551069308, 9.474510206698969483, 104.1655762719810241 ) ) ;
#84248=CARTESIAN_POINT ( 'NONE',  ( 5.823673210054444382, -21.52544592524334988, 70.20942372801904696 ) ) ;
#84249=CARTESIAN_POINT ( 'NONE',  ( 13.97604488694527802, 13.89961937509977652, 69.37390960531436690 ) ) ;
#84251=CARTESIAN_POINT ( 'NONE',  ( -16.51473224551069308, -9.474510206698971260, 66.66557627198102409 ) ) ;
#84252=CARTESIAN_POINT ( 'NONE',  ( 16.52544592524342804, -4.483927247898539470, 93.54057627198103830 ) ) ;
#84254=CARTESIAN_POINT ( 'NONE',  ( -16.51473224551082808, 9.474510206698731452, 108.3344237280190043 ) ) ;
#84255=CARTESIAN_POINT ( 'NONE',  ( 16.62475595723694965, -7.163666690055372044, 83.02713351810466236 ) ) ;
#84256=CARTESIAN_POINT ( 'NONE',  ( 5.153800228976335163, 19.02544592524342804, 74.79057627198103830 ) ) ;
#84257=CARTESIAN_POINT ( 'NONE',  ( -21.55341960407619339, 5.719274019375674811, 78.54275706135236135 ) ) ;
#84258=CARTESIAN_POINT ( 'NONE',  ( 19.03943276465977164, -0.05219959533909143690, 93.74890960531435269 ) ) ;
#84259=CARTESIAN_POINT ( 'NONE',  ( 16.52544592524335698, 4.483927247898782831, 71.45942372801901854 ) ) ;
#84260=CARTESIAN_POINT ( 'NONE',  ( -16.20579543436678094, -7.371946100355095233, 75.56520834171877254 ) ) ;
#84262=CARTESIAN_POINT ( 'NONE',  ( 16.51473224551083163, -9.474510206698727899, 50.83442372801899722 ) ) ;
#84263=CARTESIAN_POINT ( 'NONE',  ( 5.153800228976615827, -19.02544592524334988, 20.20942372801899722 ) ) ;
#84267=CARTESIAN_POINT ( 'NONE',  ( 8.224510206698953496, -14.34966873604960469, 22.91557627198102765 ) ) ;
#84269=CARTESIAN_POINT ( 'NONE',  ( 12.14591786802327356, -12.06949235617739191, 90.62609039468567573 ) ) ;
#84271=CARTESIAN_POINT ( 'NONE',  ( -0.05219959533934338120, 16.53943276465976808, 62.50109039468568284 ) ) ;
#84272=CARTESIAN_POINT ( 'NONE',  ( -5.719274019375665041, -21.55341960407619695, 74.79275706135234714 ) ) ;
#84273=CARTESIAN_POINT ( 'NONE',  ( 16.46253265017146816, 9.564922557961045513, 86.66775706135233293 ) ) ;
#84274=CARTESIAN_POINT ( 'NONE',  ( 9.474510206698729675, 16.51473224551082808, 37.08442372801899722 ) ) ;
#84275=CARTESIAN_POINT ( 'NONE',  ( 16.51473224551069308, 9.474510206698969483, 84.16557627198102409 ) ) ;
#84276=CARTESIAN_POINT ( 'NONE',  ( 13.97604488694527802, 13.89961937509977652, 54.37390960531435979 ) ) ;
#84277=CARTESIAN_POINT ( 'NONE',  ( 5.049401038298163336, -19.05341960407611168, 87.70724293864769550 ) ) ;
#84278=CARTESIAN_POINT ( 'NONE',  ( -5.823673210054116645, -21.52544592524344225, 87.29057627198103830 ) ) ;
#84279=CARTESIAN_POINT ( 'NONE',  ( 21.53943276465977519, -0.05219959533907433946, 48.74890960531435979 ) ) ;
#84280=CARTESIAN_POINT ( 'NONE',  ( 16.46253265017160672, -9.564922557960803928, 33.33224293864770260 ) ) ;
#84281=CARTESIAN_POINT ( 'NONE',  ( -4.483927247898782831, 16.52544592524335698, 57.70942372801901143 ) ) ;
#84285=CARTESIAN_POINT ( 'NONE',  ( 18.67979575497194134, -10.72451020669871369, 50.83442372801901143 ) ) ;
#84286=CARTESIAN_POINT ( 'NONE',  ( 0.05219959533910956823, 16.53943276465976808, 59.99890960531436690 ) ) ;
#84288=CARTESIAN_POINT ( 'NONE',  ( -0.05219959533934338120, 16.53943276465976808, 42.50109039468567573 ) ) ;
#84289=CARTESIAN_POINT ( 'NONE',  ( -16.53943276465976808, 0.05219959533911058130, 106.2489096053143811 ) ) ;
#84290=CARTESIAN_POINT ( 'NONE',  ( -13.97604488694547697, 13.89961937509957934, 48.12609039468566863 ) ) ;
#84291=CARTESIAN_POINT ( 'NONE',  ( 0.05219959533910956823, 16.53943276465976808, 59.99890960531436690 ) ) ;
#84292=CARTESIAN_POINT ( 'NONE',  ( -5.823673210054431948, 21.52544592524334988, 27.70942372801901854 ) ) ;
#84293=CARTESIAN_POINT ( 'NONE',  ( -16.51473224551069308, -9.474510206698971260, 26.66557627198103120 ) ) ;
#84294=CARTESIAN_POINT ( 'NONE',  ( -18.62759615963270932, 10.81492255796079327, 90.83224293864769550 ) ) ;
#84295=CARTESIAN_POINT ( 'NONE',  ( -16.46253265017160317, 9.564922557960807481, 105.8322429386476955 ) ) ;
#84296=CARTESIAN_POINT ( 'NONE',  ( 0.05219959533910956823, 16.53943276465976808, 74.99890960531435269 ) ) ;
#84297=CARTESIAN_POINT ( 'NONE',  ( -19.05341960407611168, -5.049401038298163336, 111.4572429386476671 ) ) ;
#84299=CARTESIAN_POINT ( 'NONE',  ( 9.474510206698729675, 16.51473224551082808, 82.08442372801899012 ) ) ;
#84300=CARTESIAN_POINT ( 'NONE',  ( 5.823673210054444382, -21.52544592524334988, 25.20942372801901854 ) ) ;
#84301=CARTESIAN_POINT ( 'NONE',  ( -19.03943276465977164, 0.05219959533909376836, 71.24890960531435269 ) ) ;
#84302=CARTESIAN_POINT ( 'NONE',  ( -16.51473224551082808, 9.474510206698731452, 58.33442372801900433 ) ) ;
#84303=CARTESIAN_POINT ( 'NONE',  ( -0.05219959533909027116, -19.03943276465977164, 32.49890960531435979 ) ) ;
#84304=CARTESIAN_POINT ( 'NONE',  ( 10.72451020669871369, 18.67979575497193778, 62.08442372801901143 ) ) ;
#84306=CARTESIAN_POINT ( 'NONE',  ( 4.379528057220339221, -16.55341960407611168, 52.70724293864769550 ) ) ;
#84307=CARTESIAN_POINT ( 'NONE',  ( -13.89961937509977652, 13.97604488694528158, 60.62390960531436690 ) ) ;
#84308=CARTESIAN_POINT ( 'NONE',  ( 18.67979575497178502, 10.72451020669898547, 94.16557627198103830 ) ) ;
#84309=CARTESIAN_POINT ( 'NONE',  ( 5.049401038298161559, -19.05341960407611168, 52.70724293864767418 ) ) ;
#84311=CARTESIAN_POINT ( 'NONE',  ( -21.53943276465977519, 0.05219959533907696930, 86.24890960531436690 ) ) ;
#84312=CARTESIAN_POINT ( 'NONE',  ( 10.72451020669871369, 18.67979575497193778, 97.08442372801904696 ) ) ;
#84313=CARTESIAN_POINT ( 'NONE',  ( 19.05341960407611168, 5.049401038298154454, 23.95724293864769194 ) ) ;
#84314=CARTESIAN_POINT ( 'NONE',  ( -0.05219959533934338120, 16.53943276465976808, 102.5010903946856899 ) ) ;
#84315=CARTESIAN_POINT ( 'NONE',  ( -16.52544592524342804, 4.483927247898546575, 96.04057627198102409 ) ) ;
#84316=CARTESIAN_POINT ( 'NONE',  ( 5.049401038297881783, 19.05341960407617563, 92.29275706135234714 ) ) ;
#84318=CARTESIAN_POINT ( 'NONE',  ( -15.72974639402176322, -15.80617190586768395, 19.37609039468568639 ) ) ;
#84319=CARTESIAN_POINT ( 'NONE',  ( 5.153800228976615827, -19.02544592524334988, 35.20942372801899722 ) ) ;
#84320=CARTESIAN_POINT ( 'NONE',  ( 16.55341960407618274, -4.379528057220086978, 101.0427570613523756 ) ) ;
#84321=CARTESIAN_POINT ( 'NONE',  ( 0.05219959533936267826, -19.03943276465977164, 25.00109039468566152 ) ) ;
#84322=CARTESIAN_POINT ( 'NONE',  ( 19.02544592524343514, -5.153800228976328945, 103.5405762719809957 ) ) ;
#84323=CARTESIAN_POINT ( 'NONE',  ( -10.81492255796078084, -18.62759615963271287, 67.08224293864770971 ) ) ;
#84325=CARTESIAN_POINT ( 'NONE',  ( 16.55341960407611168, 4.379528057220329451, 113.9572429386477239 ) ) ;
#84326=CARTESIAN_POINT ( 'NONE',  ( -15.80617190586768217, 15.72974639402176855, 108.1260903946856757 ) ) ;
#84327=CARTESIAN_POINT ( 'NONE',  ( -14.34966873604972548, 8.224510206698743886, 73.33442372801901854 ) ) ;
#84328=CARTESIAN_POINT ( 'NONE',  ( -18.67979575497193778, 10.72451020669871902, 23.33442372801901499 ) ) ;
#84329=CARTESIAN_POINT ( 'NONE',  ( -4.379528057220086978, -16.55341960407618274, 49.79275706135234714 ) ) ;
#84330=CARTESIAN_POINT ( 'NONE',  ( 13.97604488694527802, 13.89961937509977652, 99.37390960531436690 ) ) ;
#84331=CARTESIAN_POINT ( 'NONE',  ( -19.05341960407611168, -5.049401038298163336, 46.45724293864768129 ) ) ;
#84332=CARTESIAN_POINT ( 'NONE',  ( -9.474510206698964154, 16.51473224551069663, 65.41557627198102409 ) ) ;
#84333=CARTESIAN_POINT ( 'NONE',  ( -14.34966873604972548, 8.224510206698743886, 48.33442372801902565 ) ) ;
#84334=CARTESIAN_POINT ( 'NONE',  ( 8.224510206698953496, -14.34966873604960469, 92.91557627198103830 ) ) ;
#84335=CARTESIAN_POINT ( 'NONE',  ( 8.224510206698742110, 14.34966873604972548, 97.08442372801904696 ) ) ;
#84336=CARTESIAN_POINT ( 'NONE',  ( 17.59860650958989936, 7.585241751807028088, 49.07662985737507455 ) ) ;
#84337=CARTESIAN_POINT ( 'NONE',  ( 5.719274019375673035, 21.55341960407619339, 52.29275706135236135 ) ) ;
#84338=CARTESIAN_POINT ( 'NONE',  ( 19.05341960407611168, 5.049401038298154454, 73.95724293864768129 ) ) ;
#84339=CARTESIAN_POINT ( 'NONE',  ( -5.049401038298153566, 19.05341960407611168, 65.20724293864765286 ) ) ;
#84340=CARTESIAN_POINT ( 'NONE',  ( -5.049401038298153566, 19.05341960407611168, 100.2072429386476955 ) ) ;
#84341=CARTESIAN_POINT ( 'NONE',  ( 8.314922557960818139, 14.29746914071049879, 44.58224293864769550 ) ) ;
#84342=CARTESIAN_POINT ( 'NONE',  ( -8.314922557961024197, 14.29746914071037800, 102.9177570613523756 ) ) ;
#84343=CARTESIAN_POINT ( 'NONE',  ( -0.05219959533910754901, -16.53943276465976808, 27.49890960531435269 ) ) ;
#84345=CARTESIAN_POINT ( 'NONE',  ( -13.97604488694547697, 13.89961937509957934, 48.12609039468566863 ) ) ;
#84346=CARTESIAN_POINT ( 'NONE',  ( -5.049401038298153566, 19.05341960407611168, 110.2072429386476671 ) ) ;
#84347=CARTESIAN_POINT ( 'NONE',  ( -13.89961937509977652, 13.97604488694528158, 60.62390960531436690 ) ) ;
#84348=CARTESIAN_POINT ( 'NONE',  ( -13.97604488694547697, 13.89961937509957934, 33.12609039468566863 ) ) ;
#84350=CARTESIAN_POINT ( 'NONE',  ( 18.22780087662122384, -5.500000000000022204, 71.01540105326107266 ) ) ;
#84351=CARTESIAN_POINT ( 'NONE',  ( -13.89961937509957401, -13.97604488694547875, 69.37609039468564731 ) ) ;
#84352=CARTESIAN_POINT ( 'NONE',  ( 4.483927247898790824, -16.52544592524335698, 70.20942372801904696 ) ) ;
#84354=CARTESIAN_POINT ( 'NONE',  ( -13.89961937509977652, 13.97604488694528158, 85.62390960531433848 ) ) ;
#84355=CARTESIAN_POINT ( 'NONE',  ( 21.52544592524334988, 5.823673210054432836, 31.45942372801901854 ) ) ;
#84356=CARTESIAN_POINT ( 'NONE',  ( 16.51473224551083163, -9.474510206698727899, 80.83442372801899012 ) ) ;
#84357=CARTESIAN_POINT ( 'NONE',  ( -5.049401038298153566, 19.05341960407611168, 115.2072429386477097 ) ) ;
#84358=CARTESIAN_POINT ( 'NONE',  ( 13.97604488694527802, 13.89961937509977652, 29.37390960531435979 ) ) ;
#84359=CARTESIAN_POINT ( 'NONE',  ( 5.153800228976335163, 19.02544592524342804, 89.79057627198102409 ) ) ;
#84360=CARTESIAN_POINT ( 'NONE',  ( 14.34966873604960469, 8.224510206698951720, 44.16557627198103120 ) ) ;
#84361=CARTESIAN_POINT ( 'NONE',  ( -0.05219959533909027116, -19.03943276465977164, 37.49890960531436690 ) ) ;
#84362=CARTESIAN_POINT ( 'NONE',  ( -16.51473224551082808, 9.474510206698731452, 48.33442372801900433 ) ) ;
#84364=CARTESIAN_POINT ( 'NONE',  ( -12.14591786802309592, -12.06949235617757132, 81.87390960531435269 ) ) ;
#84365=CARTESIAN_POINT ( 'NONE',  ( 13.89961937509957401, 13.97604488694547697, 31.87609039468566863 ) ) ;
#84366=CARTESIAN_POINT ( 'NONE',  ( -19.05341960407611168, -5.049401038298163336, 56.45724293864768129 ) ) ;
#84367=CARTESIAN_POINT ( 'NONE',  ( 0.05219959533907565091, 21.53943276465977519, 64.99890960531435269 ) ) ;
#84368=CARTESIAN_POINT ( 'NONE',  ( 8.314922557960818139, 14.29746914071049879, 59.58224293864770260 ) ) ;
#84369=CARTESIAN_POINT ( 'NONE',  ( 21.55341960407619695, -5.719274019375665929, 111.0427570613523613 ) ) ;
#84370=CARTESIAN_POINT ( 'NONE',  ( 13.89961937509977652, -13.97604488694527269, 108.1239096053143669 ) ) ;
#84371=CARTESIAN_POINT ( 'NONE',  ( 10.81492255796078972, 18.62759615963270932, 24.58224293864768839 ) ) ;
#84372=CARTESIAN_POINT ( 'NONE',  ( 9.474510206698971260, -16.51473224551069308, 52.91557627198102409 ) ) ;
#84373=CARTESIAN_POINT ( 'NONE',  ( -19.05341960407611168, -5.049401038298163336, 26.45724293864769550 ) ) ;
#84374=CARTESIAN_POINT ( 'NONE',  ( 0.05219959533910956823, 16.53943276465976808, 89.99890960531438111 ) ) ;
#84375=CARTESIAN_POINT ( 'NONE',  ( -18.62759615963270932, 10.81492255796079327, 95.83224293864770971 ) ) ;
#84376=CARTESIAN_POINT ( 'NONE',  ( -19.05341960407611168, -5.049401038298163336, 96.45724293864769550 ) ) ;
#84377=CARTESIAN_POINT ( 'NONE',  ( -10.72451020669898014, 18.67979575497178502, 105.4155762719810383 ) ) ;
#84378=CARTESIAN_POINT ( 'NONE',  ( 13.97604488694527802, 13.89961937509977652, 104.3739096053143385 ) ) ;
#84379=CARTESIAN_POINT ( 'NONE',  ( 0.05219959533909260263, 19.03943276465977164, 24.99890960531435269 ) ) ;
#84380=CARTESIAN_POINT ( 'NONE',  ( -10.81492255796105439, 18.62759615963255655, 82.91775706135234714 ) ) ;
#84381=CARTESIAN_POINT ( 'NONE',  ( 5.823673210054125526, 21.52544592524343514, 94.79057627198105251 ) ) ;
#84382=CARTESIAN_POINT ( 'NONE',  ( 16.79531203550646978, -7.028104445595627858, 106.2475501177955977 ) ) ;
#84383=CARTESIAN_POINT ( 'NONE',  ( -17.59860650958989936, -7.585241751807033417, 51.57662985737508876 ) ) ;
#84385=CARTESIAN_POINT ( 'NONE',  ( -4.483927247898782831, 16.52544592524335698, 37.70942372801900433 ) ) ;
#84386=CARTESIAN_POINT ( 'NONE',  ( -12.14591786802309592, -12.06949235617757132, 111.8739096053143669 ) ) ;
#84388=CARTESIAN_POINT ( 'NONE',  ( -19.02544592524342804, 5.153800228976336051, 61.04057627198103120 ) ) ;
#84389=CARTESIAN_POINT ( 'NONE',  ( -16.53943276465976808, 0.05219959533911058130, 91.24890960531436690 ) ) ;
#84391=CARTESIAN_POINT ( 'NONE',  ( 15.72974639402199770, -15.80617190586745480, 38.12390960531436690 ) ) ;
#84392=CARTESIAN_POINT ( 'NONE',  ( -16.52544592524342804, 4.483927247898546575, 61.04057627198103120 ) ) ;
#84393=CARTESIAN_POINT ( 'NONE',  ( -4.483927247898782831, 16.52544592524335698, 22.70942372801901499 ) ) ;
#84394=CARTESIAN_POINT ( 'NONE',  ( -5.823673210054431948, 21.52544592524334988, 67.70942372801901854 ) ) ;
#84396=CARTESIAN_POINT ( 'NONE',  ( -13.89961937509977652, 13.97604488694528158, 115.6239096053143669 ) ) ;
#84397=CARTESIAN_POINT ( 'NONE',  ( 16.52544592524335698, 4.483927247898782831, 91.45942372801901854 ) ) ;
#84398=CARTESIAN_POINT ( 'NONE',  ( -16.51473224551069308, -9.474510206698971260, 36.66557627198102409 ) ) ;
#84399=CARTESIAN_POINT ( 'NONE',  ( -5.049401038298153566, 19.05341960407611168, 95.20724293864770971 ) ) ;
#84400=CARTESIAN_POINT ( 'NONE',  ( 5.719274019375991003, -21.55341960407610458, 97.70724293864772392 ) ) ;
#84401=CARTESIAN_POINT ( 'NONE',  ( -0.05219959533934338120, 16.53943276465976808, 22.50109039468567573 ) ) ;
#84402=CARTESIAN_POINT ( 'NONE',  ( 12.06949235617757843, -12.14591786802309237, 68.12390960531436690 ) ) ;
#84403=CARTESIAN_POINT ( 'NONE',  ( -10.72451020669870658, -18.67979575497194134, 74.58442372801901854 ) ) ;
#84404=CARTESIAN_POINT ( 'NONE',  ( -8.224510206698735004, -14.34966873604973081, 104.5844237280190185 ) ) ;
#84405=CARTESIAN_POINT ( 'NONE',  ( 17.31728774477273092, 6.344390552232404445, 26.68093348310682345 ) ) ;
#84407=CARTESIAN_POINT ( 'NONE',  ( -0.05219959533910754901, -16.53943276465976808, 32.49890960531435979 ) ) ;
#84408=CARTESIAN_POINT ( 'NONE',  ( 14.34966873604972726, -8.224510206698740333, 70.83442372801901854 ) ) ;
#84409=CARTESIAN_POINT ( 'NONE',  ( 0.05219959533909260263, 19.03943276465977164, 89.99890960531436690 ) ) ;
#84410=CARTESIAN_POINT ( 'NONE',  ( -9.564922557960796823, -16.46253265017161027, 87.08224293864769550 ) ) ;
#84411=CARTESIAN_POINT ( 'NONE',  ( 5.823673210054444382, -21.52544592524334988, 85.20942372801901854 ) ) ;
#84412=CARTESIAN_POINT ( 'NONE',  ( 4.379528057220092307, 16.55341960407617563, 87.29275706135236135 ) ) ;
#84413=CARTESIAN_POINT ( 'NONE',  ( 4.483927247898545687, 16.52544592524342804, 59.79057627198103120 ) ) ;
#84414=CARTESIAN_POINT ( 'NONE',  ( -13.97604488694527625, -13.89961937509977652, 61.87390960531435979 ) ) ;
#84416=CARTESIAN_POINT ( 'NONE',  ( -16.46253265017146816, -9.564922557961047289, 104.1677570613523329 ) ) ;
#84417=CARTESIAN_POINT ( 'NONE',  ( 16.53943276465976808, -0.05219959533910856209, 103.7489096053143669 ) ) ;
#84418=CARTESIAN_POINT ( 'NONE',  ( 19.02544592524343514, -5.153800228976328945, 83.54057627198100988 ) ) ;
#84419=CARTESIAN_POINT ( 'NONE',  ( -16.51473224551082808, 9.474510206698731452, 108.3344237280190043 ) ) ;
#84421=CARTESIAN_POINT ( 'NONE',  ( -9.564922557961040184, 16.46253265017147172, 22.91775706135233648 ) ) ;
#84422=CARTESIAN_POINT ( 'NONE',  ( -14.29746914071037622, -8.314922557961029526, 84.16775706135234714 ) ) ;
#84423=CARTESIAN_POINT ( 'NONE',  ( -13.89961937509957401, -13.97604488694547875, 89.37609039468563310 ) ) ;
#84424=CARTESIAN_POINT ( 'NONE',  ( -0.05219959533909027116, -19.03943276465977164, 22.49890960531436690 ) ) ;
#84425=CARTESIAN_POINT ( 'NONE',  ( -8.314922557961024197, 14.29746914071037800, 62.91775706135236135 ) ) ;
#84427=CARTESIAN_POINT ( 'NONE',  ( -16.51473224551082808, 9.474510206698731452, 58.33442372801900433 ) ) ;
#84428=CARTESIAN_POINT ( 'NONE',  ( -18.62759615963255300, -10.81492255796106328, 99.16775706135234714 ) ) ;
#84429=CARTESIAN_POINT ( 'NONE',  ( -19.05341960407611168, -5.049401038298163336, 36.45724293864766707 ) ) ;
#84430=CARTESIAN_POINT ( 'NONE',  ( 19.03943276465977164, -0.05219959533909143690, 83.74890960531436690 ) ) ;
#84431=CARTESIAN_POINT ( 'NONE',  ( 16.52544592524342804, -4.483927247898539470, 73.54057627198102409 ) ) ;
#84432=CARTESIAN_POINT ( 'NONE',  ( -5.719274019375665041, -21.55341960407619695, 84.79275706135234714 ) ) ;
#84433=CARTESIAN_POINT ( 'NONE',  ( 5.153800228976615827, -19.02544592524334988, 55.20942372801899722 ) ) ;
#84434=CARTESIAN_POINT ( 'NONE',  ( -13.97604488694547697, 13.89961937509957934, 38.12609039468566152 ) ) ;
#84435=CARTESIAN_POINT ( 'NONE',  ( -10.81492255796078084, -18.62759615963271287, 32.08224293864769550 ) ) ;
#84436=CARTESIAN_POINT ( 'NONE',  ( -10.81492255796105439, 18.62759615963255655, 97.91775706135236135 ) ) ;
#84437=CARTESIAN_POINT ( 'NONE',  ( -0.05219959533909027116, -19.03943276465977164, 82.49890960531436690 ) ) ;
#84438=CARTESIAN_POINT ( 'NONE',  ( 15.72974639402176855, 15.80617190586768217, 106.8760903946856899 ) ) ;
#84439=CARTESIAN_POINT ( 'NONE',  ( -15.80617190586745835, -15.72974639402198527, 46.87390960531435979 ) ) ;
#84440=CARTESIAN_POINT ( 'NONE',  ( 19.05341960407611168, 5.049401038298154454, 93.95724293864769550 ) ) ;
#84441=CARTESIAN_POINT ( 'NONE',  ( -13.97604488694547697, 13.89961937509957934, 73.12609039468568994 ) ) ;
#84442=CARTESIAN_POINT ( 'NONE',  ( -19.02544592524342804, 5.153800228976336051, 101.0405762719810241 ) ) ;
#84443=CARTESIAN_POINT ( 'NONE',  ( 16.46253265017146816, 9.564922557961045513, 96.66775706135233293 ) ) ;
#84444=CARTESIAN_POINT ( 'NONE',  ( -4.483927247898782831, 16.52544592524335698, 37.70942372801900433 ) ) ;
#84445=CARTESIAN_POINT ( 'NONE',  ( 8.314922557960818139, 14.29746914071049879, 99.58224293864770971 ) ) ;
#84446=CARTESIAN_POINT ( 'NONE',  ( 13.97604488694527802, 13.89961937509977652, 79.37390960531435269 ) ) ;
#84447=CARTESIAN_POINT ( 'NONE',  ( -5.719274019375978568, 21.55341960407610458, 60.20724293864768839 ) ) ;
#84448=CARTESIAN_POINT ( 'NONE',  ( -14.34966873604972548, 8.224510206698743886, 33.33442372801900433 ) ) ;
#84449=CARTESIAN_POINT ( 'NONE',  ( -10.72451020669870658, -18.67979575497194134, 39.58442372801901143 ) ) ;
#84450=CARTESIAN_POINT ( 'NONE',  ( -18.62759615963255300, -10.81492255796106328, 84.16775706135234714 ) ) ;
#84451=CARTESIAN_POINT ( 'NONE',  ( 16.52544592524335698, 4.483927247898782831, 81.45942372801900433 ) ) ;
#84452=CARTESIAN_POINT ( 'NONE',  ( -16.46253265017160317, 9.564922557960807481, 80.83224293864769550 ) ) ;
#84453=CARTESIAN_POINT ( 'NONE',  ( 16.53943276465976808, -0.05219959533910856209, 73.74890960531433848 ) ) ;
#84454=CARTESIAN_POINT ( 'NONE',  ( 8.314922557961029526, -14.29746914071037800, 110.4177570613523756 ) ) ;
#84455=CARTESIAN_POINT ( 'NONE',  ( -16.46253265017146816, -9.564922557961047289, 59.16775706135233293 ) ) ;
#84456=CARTESIAN_POINT ( 'NONE',  ( 18.67979575497194134, -10.72451020669871369, 35.83442372801901143 ) ) ;
#84457=CARTESIAN_POINT ( 'NONE',  ( 4.379528057220339221, -16.55341960407611168, 82.70724293864770971 ) ) ;
#84458=CARTESIAN_POINT ( 'NONE',  ( 19.02544592524343514, -5.153800228976328945, 93.54057627198102409 ) ) ;
#84459=CARTESIAN_POINT ( 'NONE',  ( -8.224510206698735004, -14.34966873604973081, 104.5844237280190185 ) ) ;
#84460=CARTESIAN_POINT ( 'NONE',  ( 21.55341960407619695, -5.719274019375665929, 71.04275706135234714 ) ) ;
#84461=CARTESIAN_POINT ( 'NONE',  ( -16.52544592524335698, -4.483927247898792601, 38.95942372801901854 ) ) ;
#84462=CARTESIAN_POINT ( 'NONE',  ( 0.05219959533937995610, -21.53943276465977519, 35.00109039468568284 ) ) ;
#84464=CARTESIAN_POINT ( 'NONE',  ( -5.823673210054116645, -21.52544592524344225, 112.2905762719810241 ) ) ;
#84465=CARTESIAN_POINT ( 'NONE',  ( -14.34966873604960291, -8.224510206698953496, 86.66557627198102409 ) ) ;
#84467=CARTESIAN_POINT ( 'NONE',  ( -4.483927247898539470, -16.52544592524342804, 52.29057627198102409 ) ) ;
#84468=CARTESIAN_POINT ( 'NONE',  ( -5.153800228976328057, -19.02544592524343514, 22.29057627198102765 ) ) ;
#84469=CARTESIAN_POINT ( 'NONE',  ( 15.72974639402199770, -15.80617190586745480, 43.12390960531435269 ) ) ;
#84470=CARTESIAN_POINT ( 'NONE',  ( -8.314922557960811034, -14.29746914071050412, 77.08224293864769550 ) ) ;
#84471=CARTESIAN_POINT ( 'NONE',  ( 0.05219959533907565091, 21.53943276465977519, 79.99890960531435269 ) ) ;
#84472=CARTESIAN_POINT ( 'NONE',  ( -9.564922557960796823, -16.46253265017161027, 87.08224293864769550 ) ) ;
#84473=CARTESIAN_POINT ( 'NONE',  ( -16.51473224551069308, -9.474510206698971260, 41.66557627198103120 ) ) ;
#84474=CARTESIAN_POINT ( 'NONE',  ( 16.51473224551083163, -9.474510206698727899, 80.83442372801899012 ) ) ;
#84476=CARTESIAN_POINT ( 'NONE',  ( -18.62759615963270932, 10.81492255796079327, 25.83224293864769194 ) ) ;
#84477=CARTESIAN_POINT ( 'NONE',  ( -10.81492255796105439, 18.62759615963255655, 57.91775706135234714 ) ) ;
#84478=CARTESIAN_POINT ( 'NONE',  ( -10.81492255796078084, -18.62759615963271287, 62.08224293864769550 ) ) ;
#84479=CARTESIAN_POINT ( 'NONE',  ( -13.89961937509977652, 13.97604488694528158, 35.62390960531435269 ) ) ;
#84480=CARTESIAN_POINT ( 'NONE',  ( 9.474510206698971260, -16.51473224551069308, 77.91557627198103830 ) ) ;
#84482=CARTESIAN_POINT ( 'NONE',  ( -16.52544592524335698, -4.483927247898792601, 43.95942372801902565 ) ) ;
#84483=CARTESIAN_POINT ( 'NONE',  ( 21.55341960407619695, -5.719274019375665929, 36.04275706135234714 ) ) ;
#84484=CARTESIAN_POINT ( 'NONE',  ( 18.62759615963255655, 10.81492255796105972, 76.66775706135234714 ) ) ;
#84485=CARTESIAN_POINT ( 'NONE',  ( -19.03943276465977164, 0.05219959533909376836, 116.2489096053143669 ) ) ;
#84486=CARTESIAN_POINT ( 'NONE',  ( 5.719274019375991003, -21.55341960407610458, 92.70724293864770971 ) ) ;
#84487=CARTESIAN_POINT ( 'NONE',  ( 5.719274019375673035, 21.55341960407619339, 27.29275706135234358 ) ) ;
#84488=CARTESIAN_POINT ( 'NONE',  ( -4.379528057220086978, -16.55341960407618274, 49.79275706135234714 ) ) ;
#84489=CARTESIAN_POINT ( 'NONE',  ( 5.823673210054125526, 21.52544592524343514, 64.79057627198103830 ) ) ;
#84490=CARTESIAN_POINT ( 'NONE',  ( 21.55341960407619695, -5.719274019375665929, 111.0427570613523613 ) ) ;
#84491=CARTESIAN_POINT ( 'NONE',  ( 19.05341960407611168, 5.049401038298154454, 58.95724293864768129 ) ) ;
#84492=CARTESIAN_POINT ( 'NONE',  ( -19.02544592524342804, 5.153800228976336051, 111.0405762719810099 ) ) ;
#84493=CARTESIAN_POINT ( 'NONE',  ( -0.05219959533909027116, -19.03943276465977164, 92.49890960531436690 ) ) ;
#84495=CARTESIAN_POINT ( 'NONE',  ( 19.03943276465977164, 0.05219959533936151252, 71.25109039468566152 ) ) ;
#84496=CARTESIAN_POINT ( 'NONE',  ( -18.62759615963270932, 10.81492255796079327, 50.83224293864770971 ) ) ;
#84497=CARTESIAN_POINT ( 'NONE',  ( -16.55341960407611168, -4.379528057220339221, 31.45724293864769550 ) ) ;
#84498=CARTESIAN_POINT ( 'NONE',  ( -5.153800228976607833, 19.02544592524334988, 97.70942372801900433 ) ) ;
#84499=CARTESIAN_POINT ( 'NONE',  ( -19.03943276465977164, 0.05219959533909376836, 21.24890960531436335 ) ) ;
#84500=CARTESIAN_POINT ( 'NONE',  ( 13.89961937509957401, 13.97604488694547697, 21.87609039468566152 ) ) ;
#84501=CARTESIAN_POINT ( 'NONE',  ( -16.46253265017146816, -9.564922557961047289, 94.16775706135233293 ) ) ;
#84502=CARTESIAN_POINT ( 'NONE',  ( 5.719274019375991003, -21.55341960407610458, 82.70724293864770971 ) ) ;
#84503=CARTESIAN_POINT ( 'NONE',  ( -19.05341960407617563, 5.049401038297882671, 58.54275706135234003 ) ) ;
#84504=CARTESIAN_POINT ( 'NONE',  ( 16.62475595723699584, 7.163666690055298325, 106.9728664818953519 ) ) ;
#84505=CARTESIAN_POINT ( 'NONE',  ( 0.05219959533909260263, 19.03943276465977164, 54.99890960531435979 ) ) ;
#84506=CARTESIAN_POINT ( 'NONE',  ( 0.05219959533910956823, 16.53943276465976808, 59.99890960531436690 ) ) ;
#84507=CARTESIAN_POINT ( 'NONE',  ( -19.02544592524342804, 5.153800228976336051, 51.04057627198103120 ) ) ;
#84508=CARTESIAN_POINT ( 'NONE',  ( -12.14591786802309592, -12.06949235617757132, 51.87390960531437401 ) ) ;
#84510=CARTESIAN_POINT ( 'NONE',  ( -16.55341960407611168, -4.379528057220339221, 26.45724293864768839 ) ) ;
#84511=CARTESIAN_POINT ( 'NONE',  ( 16.51473224551069308, 9.474510206698969483, 59.16557627198102409 ) ) ;
#84512=CARTESIAN_POINT ( 'NONE',  ( 9.474510206698729675, 16.51473224551082808, 32.08442372801900433 ) ) ;
#84513=CARTESIAN_POINT ( 'NONE',  ( -16.53943276465976808, -0.05219959533934237506, 28.75109039468567929 ) ) ;
#84514=CARTESIAN_POINT ( 'NONE',  ( -5.823673210054116645, -21.52544592524344225, 52.29057627198102409 ) ) ;
#84515=CARTESIAN_POINT ( 'NONE',  ( 21.53943276465977519, 0.05219959533937863772, 106.2510903946856757 ) ) ;
#84517=CARTESIAN_POINT ( 'NONE',  ( 19.02544592524343514, -5.153800228976328945, 58.54057627198102409 ) ) ;
#84519=CARTESIAN_POINT ( 'NONE',  ( -16.51473224551069308, -9.474510206698971260, 91.66557627198103830 ) ) ;
#84521=CARTESIAN_POINT ( 'NONE',  ( -0.05219959533937732626, 21.53943276465977519, 27.50109039468567929 ) ) ;
#84522=CARTESIAN_POINT ( 'NONE',  ( -14.34966873604960291, -8.224510206698953496, 96.66557627198102409 ) ) ;
#84523=CARTESIAN_POINT ( 'NONE',  ( -15.72974639402197994, 15.80617190586746368, 85.62390960531436690 ) ) ;
#84524=CARTESIAN_POINT ( 'NONE',  ( -19.02544592524342804, 5.153800228976336051, 71.04057627198099567 ) ) ;
#84525=CARTESIAN_POINT ( 'NONE',  ( -19.03943276465977164, 0.05219959533909376836, 76.24890960531435269 ) ) ;
#84526=CARTESIAN_POINT ( 'NONE',  ( 10.81492255796078972, 18.62759615963270932, 104.5822429386477097 ) ) ;
#84528=CARTESIAN_POINT ( 'NONE',  ( -5.049401038298153566, 19.05341960407611168, 75.20724293864769550 ) ) ;
#84529=CARTESIAN_POINT ( 'NONE',  ( 19.53037848336980176, -5.499999999999991118, 97.35532783611445495 ) ) ;
#84530=CARTESIAN_POINT ( 'NONE',  ( -4.483927247898539470, -16.52544592524342804, 112.2905762719810241 ) ) ;
#84532=CARTESIAN_POINT ( 'NONE',  ( -9.474510206698720793, -16.51473224551083518, 89.58442372801900433 ) ) ;
#84533=CARTESIAN_POINT ( 'NONE',  ( -12.06949235617756955, 12.14591786802309770, 95.62390960531436690 ) ) ;
#84534=CARTESIAN_POINT ( 'NONE',  ( 15.72974639402176855, 15.80617190586768217, 71.87609039468568994 ) ) ;
#84535=CARTESIAN_POINT ( 'NONE',  ( -0.05219959533909027116, -19.03943276465977164, 62.49890960531435979 ) ) ;
#84536=CARTESIAN_POINT ( 'NONE',  ( -5.719274019375665041, -21.55341960407619695, 39.79275706135235424 ) ) ;
#84537=CARTESIAN_POINT ( 'NONE',  ( 10.81492255796078972, 18.62759615963270932, 114.5822429386477097 ) ) ;
#84539=CARTESIAN_POINT ( 'NONE',  ( 9.474510206698971260, -16.51473224551069308, 72.91557627198102409 ) ) ;
#84541=CARTESIAN_POINT ( 'NONE',  ( -14.29746914071037622, -8.314922557961029526, 29.16775706135234003 ) ) ;
#84542=CARTESIAN_POINT ( 'NONE',  ( -15.72974639402197994, 15.80617190586746368, 30.62390960531436335 ) ) ;
#84543=CARTESIAN_POINT ( 'NONE',  ( -15.80617190586768217, 15.72974639402176855, 63.12609039468568994 ) ) ;
#84544=CARTESIAN_POINT ( 'NONE',  ( 9.564922557960805705, 16.46253265017160317, 109.5822429386476955 ) ) ;
#84545=CARTESIAN_POINT ( 'NONE',  ( 5.049401038297881783, 19.05341960407617563, 97.29275706135233293 ) ) ;
#84546=CARTESIAN_POINT ( 'NONE',  ( 19.02544592524343514, -5.153800228976328945, 53.54057627198102409 ) ) ;
#84547=CARTESIAN_POINT ( 'NONE',  ( 16.51473224551069308, 9.474510206698969483, 74.16557627198103830 ) ) ;
#84548=CARTESIAN_POINT ( 'NONE',  ( 4.379528057220339221, -16.55341960407611168, 97.70724293864772392 ) ) ;
#84549=CARTESIAN_POINT ( 'NONE',  ( -5.049401038298153566, 19.05341960407611168, 105.2072429386476671 ) ) ;
#84550=CARTESIAN_POINT ( 'NONE',  ( -16.55341960407611168, -4.379528057220339221, 91.45724293864769550 ) ) ;
#84551=CARTESIAN_POINT ( 'NONE',  ( -0.05219959533909027116, -19.03943276465977164, 92.49890960531436690 ) ) ;
#84552=CARTESIAN_POINT ( 'NONE',  ( -8.314922557960811034, -14.29746914071050412, 47.08224293864770260 ) ) ;
#84553=CARTESIAN_POINT ( 'NONE',  ( -5.049401038298153566, 19.05341960407611168, 45.20724293864769550 ) ) ;
#84554=CARTESIAN_POINT ( 'NONE',  ( 18.62759615963255655, 10.81492255796105972, 56.66775706135235424 ) ) ;
#84555=CARTESIAN_POINT ( 'NONE',  ( -0.05219959533936034679, 19.03943276465977164, 97.50109039468567573 ) ) ;
#84556=CARTESIAN_POINT ( 'NONE',  ( 8.314922557960818139, 14.29746914071049879, 54.58224293864769550 ) ) ;
#84557=CARTESIAN_POINT ( 'NONE',  ( 21.53943276465977519, -0.05219959533907433946, 103.7489096053143669 ) ) ;
#84558=CARTESIAN_POINT ( 'NONE',  ( -21.53943276465977519, 0.05219959533907696930, 51.24890960531436690 ) ) ;
#84559=CARTESIAN_POINT ( 'NONE',  ( 19.03943276465977164, -0.05219959533909143690, 108.7489096053143527 ) ) ;
#84560=CARTESIAN_POINT ( 'NONE',  ( 14.29746914071049879, -8.314922557960816363, 83.33224293864769550 ) ) ;
#84562=CARTESIAN_POINT ( 'NONE',  ( 5.049401038298161559, -19.05341960407611168, 62.70724293864769550 ) ) ;
#84563=CARTESIAN_POINT ( 'NONE',  ( 8.224510206698953496, -14.34966873604960469, 27.91557627198103830 ) ) ;
#84564=CARTESIAN_POINT ( 'NONE',  ( 14.34966873604972726, -8.224510206698740333, 105.8344237280190328 ) ) ;
#84565=CARTESIAN_POINT ( 'NONE',  ( 8.314922557961029526, -14.29746914071037800, 85.41775706135236135 ) ) ;
#84566=CARTESIAN_POINT ( 'NONE',  ( -5.153800228976607833, 19.02544592524334988, 37.70942372801899722 ) ) ;
#84568=CARTESIAN_POINT ( 'NONE',  ( -16.51473224551069308, -9.474510206698971260, 106.6655762719810383 ) ) ;
#84569=CARTESIAN_POINT ( 'NONE',  ( -19.05341960407611168, -5.049401038298163336, 81.45724293864769550 ) ) ;
#84570=CARTESIAN_POINT ( 'NONE',  ( 9.564922557960805705, 16.46253265017160317, 39.58224293864768839 ) ) ;
#84571=CARTESIAN_POINT ( 'NONE',  ( -12.06949235617756955, 12.14591786802309770, 45.62390960531436690 ) ) ;
#84572=CARTESIAN_POINT ( 'NONE',  ( -19.03943276465977164, 0.05219959533909376836, 116.2489096053143669 ) ) ;
#84573=CARTESIAN_POINT ( 'NONE',  ( 16.46253265017160672, -9.564922557960803928, 108.3322429386476955 ) ) ;
#84574=CARTESIAN_POINT ( 'NONE',  ( 15.80617190586746368, 15.72974639402197994, 34.37390960531435979 ) ) ;
#84575=CARTESIAN_POINT ( 'NONE',  ( 16.55341960407611168, 4.379528057220329451, 88.95724293864769550 ) ) ;
#84576=CARTESIAN_POINT ( 'NONE',  ( 16.52544592524335698, 4.483927247898782831, 36.45942372801901143 ) ) ;
#84577=CARTESIAN_POINT ( 'NONE',  ( -16.52544592524342804, 4.483927247898546575, 71.04057627198103830 ) ) ;
#84578=CARTESIAN_POINT ( 'NONE',  ( 17.50000000000018119, -3.417042746626921534, 32.67380396232485396 ) ) ;
#84579=CARTESIAN_POINT ( 'NONE',  ( -5.049401038297874678, -19.05341960407617918, 64.79275706135233293 ) ) ;
#84580=CARTESIAN_POINT ( 'NONE',  ( -13.89961937509977652, 13.97604488694528158, 105.6239096053143527 ) ) ;
#84581=CARTESIAN_POINT ( 'NONE',  ( 16.46253265017146816, 9.564922557961045513, 76.66775706135234714 ) ) ;
#84582=CARTESIAN_POINT ( 'NONE',  ( 5.153800228976617603, -19.02544592524335343, 40.20942372801899012 ) ) ;
#84583=CARTESIAN_POINT ( 'NONE',  ( -0.05219959533934338120, 16.53943276465976808, 32.50109039468568284 ) ) ;
#84584=CARTESIAN_POINT ( 'NONE',  ( 8.314922557961029526, -14.29746914071037800, 105.4177570613523613 ) ) ;
#84585=CARTESIAN_POINT ( 'NONE',  ( 19.05341960407617918, -5.049401038297876454, 76.04275706135230450 ) ) ;
#84586=CARTESIAN_POINT ( 'NONE',  ( 21.55341960407610458, 5.719274019375980345, 38.95724293864768839 ) ) ;
#84587=CARTESIAN_POINT ( 'NONE',  ( 21.55341960407619695, -5.719274019375665929, 66.04275706135236135 ) ) ;
#84588=CARTESIAN_POINT ( 'NONE',  ( 19.43099193148526638, 5.500000000000092371, 38.23279185469454688 ) ) ;
#84589=CARTESIAN_POINT ( 'NONE',  ( -4.483927247898782831, 16.52544592524335698, 27.70942372801901854 ) ) ;
#84591=CARTESIAN_POINT ( 'NONE',  ( -9.564922557960796823, -16.46253265017161027, 92.08224293864769550 ) ) ;
#84593=CARTESIAN_POINT ( 'NONE',  ( 16.53943276465976808, -0.05219959533910856209, 88.74890960531436690 ) ) ;
#84594=CARTESIAN_POINT ( 'NONE',  ( 16.51473224551069308, 9.474510206698969483, 74.16557627198103830 ) ) ;
#84597=CARTESIAN_POINT ( 'NONE',  ( -5.153800228976328057, -19.02544592524343514, 87.29057627198103830 ) ) ;
#84599=CARTESIAN_POINT ( 'NONE',  ( 19.03943276465977164, 0.05219959533936151252, 91.25109039468566152 ) ) ;
#84600=CARTESIAN_POINT ( 'NONE',  ( 5.719274019375991003, -21.55341960407610458, 82.70724293864770971 ) ) ;
#84601=CARTESIAN_POINT ( 'NONE',  ( -13.89961937509977652, 13.97604488694528158, 30.62390960531435269 ) ) ;
#84602=CARTESIAN_POINT ( 'NONE',  ( 16.46253265017146816, 9.564922557961045513, 66.66775706135233293 ) ) ;
#84603=CARTESIAN_POINT ( 'NONE',  ( 10.81492255796078972, 18.62759615963270932, 109.5822429386476955 ) ) ;
#84604=CARTESIAN_POINT ( 'NONE',  ( -19.02544592524342804, 5.153800228976336051, 76.04057627198102409 ) ) ;
#84605=CARTESIAN_POINT ( 'NONE',  ( -5.153800228976328057, -19.02544592524343514, 107.2905762719810383 ) ) ;
#84607=CARTESIAN_POINT ( 'NONE',  ( -10.81492255796078084, -18.62759615963271287, 107.0822429386476955 ) ) ;
#84608=CARTESIAN_POINT ( 'NONE',  ( 16.55341960407611168, 4.379528057220329451, 88.95724293864769550 ) ) ;
#84609=CARTESIAN_POINT ( 'NONE',  ( -13.89961937509977652, 13.97604488694528158, 80.62390960531436690 ) ) ;
#84610=CARTESIAN_POINT ( 'NONE',  ( 16.51473224551083163, -9.474510206698727899, 60.83442372801900433 ) ) ;
#84611=CARTESIAN_POINT ( 'NONE',  ( 10.81492255796078972, 18.62759615963270932, 84.58224293864769550 ) ) ;
#84612=CARTESIAN_POINT ( 'NONE',  ( 10.72451020669898902, -18.67979575497178502, 67.91557627198102409 ) ) ;
#84613=CARTESIAN_POINT ( 'NONE',  ( -4.379528057220328563, 16.55341960407611168, 50.20724293864769550 ) ) ;
#84614=CARTESIAN_POINT ( 'NONE',  ( -21.52544592524334988, -5.823673210054445271, 98.95942372801903275 ) ) ;
#84615=CARTESIAN_POINT ( 'NONE',  ( -12.14591786802326823, 12.06949235617739902, 63.12609039468568994 ) ) ;
#84616=CARTESIAN_POINT ( 'NONE',  ( 13.89961937509977652, -13.97604488694527269, 98.12390960531433848 ) ) ;
#84617=CARTESIAN_POINT ( 'NONE',  ( -9.564922557960796823, -16.46253265017161027, 52.08224293864768839 ) ) ;
#84618=CARTESIAN_POINT ( 'NONE',  ( -15.80617190586768217, 15.72974639402176855, 48.12609039468568284 ) ) ;
#84619=CARTESIAN_POINT ( 'NONE',  ( -10.81492255796105439, 18.62759615963255655, 47.91775706135234714 ) ) ;
#84620=CARTESIAN_POINT ( 'NONE',  ( -5.153800228976328057, -19.02544592524343514, 67.29057627198102409 ) ) ;
#84621=CARTESIAN_POINT ( 'NONE',  ( 21.53943276465977519, 0.05219959533937863772, 36.25109039468567573 ) ) ;
#84622=CARTESIAN_POINT ( 'NONE',  ( 19.05341960407617918, -5.049401038297876454, 71.04275706135234714 ) ) ;
#84624=CARTESIAN_POINT ( 'NONE',  ( 9.474510206698729675, 16.51473224551082808, 77.08442372801900433 ) ) ;
#84625=CARTESIAN_POINT ( 'NONE',  ( 16.51473224551069308, 9.474510206698969483, 34.16557627198102409 ) ) ;
#84626=CARTESIAN_POINT ( 'NONE',  ( 8.224510206698742110, 14.34966873604972548, 87.08442372801901854 ) ) ;
#84627=CARTESIAN_POINT ( 'NONE',  ( -13.97604488694527625, -13.89961937509977652, 56.87390960531434558 ) ) ;
#84629=CARTESIAN_POINT ( 'NONE',  ( -9.564922557960796823, -16.46253265017161027, 102.0822429386477097 ) ) ;
#84630=CARTESIAN_POINT ( 'NONE',  ( 13.89961937509977652, -13.97604488694527269, 33.12390960531434558 ) ) ;
#84632=CARTESIAN_POINT ( 'NONE',  ( 15.80617190586746368, 15.72974639402197994, 69.37390960531436690 ) ) ;
#84633=CARTESIAN_POINT ( 'NONE',  ( 4.483927247898790824, -16.52544592524335698, 60.20942372801902565 ) ) ;
#84634=CARTESIAN_POINT ( 'NONE',  ( -0.05219959533936034679, 19.03943276465977164, 22.50109039468566152 ) ) ;
#84635=CARTESIAN_POINT ( 'NONE',  ( 9.564922557960805705, 16.46253265017160317, 59.58224293864769550 ) ) ;
#84636=CARTESIAN_POINT ( 'NONE',  ( -14.34966873604960291, -8.224510206698953496, 41.66557627198103120 ) ) ;
#84637=CARTESIAN_POINT ( 'NONE',  ( -8.314922557960811034, -14.29746914071050412, 77.08224293864769550 ) ) ;
#84638=CARTESIAN_POINT ( 'NONE',  ( -0.05219959533909027116, -19.03943276465977164, 82.49890960531436690 ) ) ;
#84639=CARTESIAN_POINT ( 'NONE',  ( 10.81492255796106328, -18.62759615963255655, 30.41775706135234358 ) ) ;
#84640=CARTESIAN_POINT ( 'NONE',  ( 19.02544592524343514, -5.153800228976328945, 88.54057627198102409 ) ) ;
#84641=CARTESIAN_POINT ( 'NONE',  ( 18.67979575497194134, -10.72451020669871369, 100.8344237280190185 ) ) ;
#84642=CARTESIAN_POINT ( 'NONE',  ( 14.34966873604972726, -8.224510206698740333, 65.83442372801900433 ) ) ;
#84643=CARTESIAN_POINT ( 'NONE',  ( -0.05219959533937732626, 21.53943276465977519, 32.50109039468568284 ) ) ;
#84644=CARTESIAN_POINT ( 'NONE',  ( 16.51473224551069308, 9.474510206698969483, 104.1655762719810241 ) ) ;
#84645=CARTESIAN_POINT ( 'NONE',  ( -15.72974639402197994, 15.80617190586746368, 90.62390960531436690 ) ) ;
#84646=CARTESIAN_POINT ( 'NONE',  ( -12.14591786802309592, -12.06949235617757132, 41.87390960531435979 ) ) ;
#84647=CARTESIAN_POINT ( 'NONE',  ( 19.05341960407611168, 5.049401038298154454, 38.95724293864767418 ) ) ;
#84648=CARTESIAN_POINT ( 'NONE',  ( 16.53943276465976808, -0.05219959533910856209, 73.74890960531433848 ) ) ;
#84649=CARTESIAN_POINT ( 'NONE',  ( -21.55341960407610458, -5.719274019375992779, 31.45724293864769550 ) ) ;
#84650=CARTESIAN_POINT ( 'NONE',  ( 9.474510206698729675, 16.51473224551082808, 27.08442372801900433 ) ) ;
#84651=CARTESIAN_POINT ( 'NONE',  ( 14.29746914071049879, -8.314922557960816363, 98.33224293864769550 ) ) ;
#84652=CARTESIAN_POINT ( 'NONE',  ( -13.89961937509977652, 13.97604488694528158, 110.6239096053143243 ) ) ;
#84654=CARTESIAN_POINT ( 'NONE',  ( -4.379528057220086978, -16.55341960407618274, 59.79275706135234714 ) ) ;
#84655=CARTESIAN_POINT ( 'NONE',  ( 13.97604488694527802, 13.89961937509977652, 49.37390960531434558 ) ) ;
#84657=CARTESIAN_POINT ( 'NONE',  ( 16.52544592524335698, 4.483927247898782831, 96.45942372801901854 ) ) ;
#84658=CARTESIAN_POINT ( 'NONE',  ( 16.51473224551083163, -9.474510206698727899, 95.83442372801900433 ) ) ;
#84659=CARTESIAN_POINT ( 'NONE',  ( 5.719274019375673035, 21.55341960407619339, 67.29275706135234714 ) ) ;
#84660=CARTESIAN_POINT ( 'NONE',  ( 13.89961937509977652, -13.97604488694527269, 78.12390960531433848 ) ) ;
#84661=CARTESIAN_POINT ( 'NONE',  ( -15.80617190586745835, -15.72974639402198527, 86.87390960531438111 ) ) ;
#84662=CARTESIAN_POINT ( 'NONE',  ( 4.379528057220092307, 16.55341960407617563, 47.29275706135234003 ) ) ;
#84663=CARTESIAN_POINT ( 'NONE',  ( 0.05219959533910956823, 16.53943276465976808, 109.9989096053143527 ) ) ;
#84664=CARTESIAN_POINT ( 'NONE',  ( 5.049401038297881783, 19.05341960407617563, 87.29275706135234714 ) ) ;
#84665=CARTESIAN_POINT ( 'NONE',  ( -15.80617190586745835, -15.72974639402198527, 76.87390960531439532 ) ) ;
#84666=CARTESIAN_POINT ( 'NONE',  ( 0.05219959533936267826, -19.03943276465977164, 45.00109039468566863 ) ) ;
#84667=FACE_BOUND ( 'NONE', #146672, .T. ) ;
#84668=CARTESIAN_POINT ( 'NONE',  ( 5.823673210054125526, 21.52544592524343514, 94.79057627198105251 ) ) ;
#84669=CARTESIAN_POINT ( 'NONE',  ( 17.50000000000000000, -5.500000000000000888, 120.0000000000000142 ) ) ;
#84670=CARTESIAN_POINT ( 'NONE',  ( -19.05341960407611168, -5.049401038298163336, 61.45724293864769550 ) ) ;
#84672=CARTESIAN_POINT ( 'NONE',  ( -13.97604488694547697, 13.89961937509957934, 113.1260903946856757 ) ) ;
#84674=CARTESIAN_POINT ( 'NONE',  ( 13.97604488694527802, 13.89961937509977652, 44.37390960531435269 ) ) ;
#84675=CARTESIAN_POINT ( 'NONE',  ( 18.62759615963271287, -10.81492255796078972, 108.3322429386477097 ) ) ;
#84676=CARTESIAN_POINT ( 'NONE',  ( -14.34966873604960291, -8.224510206698953496, 51.66557627198102409 ) ) ;
#84677=CARTESIAN_POINT ( 'NONE',  ( 19.05341960407611168, 5.049401038298154454, 58.95724293864768129 ) ) ;
#84678=CARTESIAN_POINT ( 'NONE',  ( -5.823673210054431948, 21.52544592524334988, 77.70942372801900433 ) ) ;
#84679=CARTESIAN_POINT ( 'NONE',  ( 0.05219959533934541429, -16.53943276465976808, 25.00109039468567218 ) ) ;
#84680=CARTESIAN_POINT ( 'NONE',  ( -16.51473224551082808, 9.474510206698731452, 33.33442372801899722 ) ) ;
#84681=CARTESIAN_POINT ( 'NONE',  ( 5.823673210054444382, -21.52544592524334988, 45.20942372801901854 ) ) ;
#84682=CARTESIAN_POINT ( 'NONE',  ( 21.55341960407619695, -5.719274019375665929, 21.04275706135234714 ) ) ;
#84683=CARTESIAN_POINT ( 'NONE',  ( 15.80617190586746368, 15.72974639402197994, 54.37390960531435979 ) ) ;
#84684=CARTESIAN_POINT ( 'NONE',  ( 16.46253265017146816, 9.564922557961045513, 101.6677570613523329 ) ) ;
#84685=CARTESIAN_POINT ( 'NONE',  ( -9.564922557961040184, 16.46253265017147172, 67.91775706135233293 ) ) ;
#84686=CARTESIAN_POINT ( 'NONE',  ( -21.52544592524334988, -5.823673210054445271, 78.95942372801901854 ) ) ;
#84687=CARTESIAN_POINT ( 'NONE',  ( 13.89961937509957401, 13.97604488694547697, 46.87609039468565442 ) ) ;
#84688=CARTESIAN_POINT ( 'NONE',  ( 19.02544592524343514, -5.153800228976328945, 28.54057627198102409 ) ) ;
#84689=CARTESIAN_POINT ( 'NONE',  ( -15.80617190586745835, -15.72974639402198527, 61.87390960531436690 ) ) ;
#84690=CARTESIAN_POINT ( 'NONE',  ( -16.55341960407611168, -4.379528057220339221, 51.45724293864770260 ) ) ;
#84691=CARTESIAN_POINT ( 'NONE',  ( -19.48894818550246200, 5.499999999999919176, 95.10307310435240424 ) ) ;
#84692=CARTESIAN_POINT ( 'NONE',  ( 16.46253265017146816, 9.564922557961045513, 21.66775706135233648 ) ) ;
#84693=CARTESIAN_POINT ( 'NONE',  ( -12.06949235617739369, -12.14591786802326823, 84.37609039468570415 ) ) ;
#84694=CARTESIAN_POINT ( 'NONE',  ( -4.379528057220328563, 16.55341960407611168, 40.20724293864769550 ) ) ;
#84695=CARTESIAN_POINT ( 'NONE',  ( -18.62759615963255300, -10.81492255796106328, 74.16775706135231871 ) ) ;
#84696=CARTESIAN_POINT ( 'NONE',  ( -21.52544592524334988, -5.823673210054445271, 78.95942372801901854 ) ) ;
#84697=CARTESIAN_POINT ( 'NONE',  ( -18.62759615963270932, 10.81492255796079327, 85.83224293864768129 ) ) ;
#84698=CARTESIAN_POINT ( 'NONE',  ( -16.46253265017160317, 9.564922557960807481, 35.83224293864768839 ) ) ;
#84699=CARTESIAN_POINT ( 'NONE',  ( -18.67979575497193778, 10.72451020669871902, 63.33442372801900433 ) ) ;
#84700=CARTESIAN_POINT ( 'NONE',  ( 0.05219959533909260263, 19.03943276465977164, 29.99890960531435979 ) ) ;
#84702=CARTESIAN_POINT ( 'NONE',  ( 19.03943276465977164, -0.05219959533909143690, 48.74890960531435979 ) ) ;
#84703=CARTESIAN_POINT ( 'NONE',  ( 4.483927247898545687, 16.52544592524342804, 89.79057627198103830 ) ) ;
#84704=CARTESIAN_POINT ( 'NONE',  ( 16.51473224551069308, 9.474510206698969483, 99.16557627198102409 ) ) ;
#84705=CARTESIAN_POINT ( 'NONE',  ( -16.52544592524342804, 4.483927247898546575, 36.04057627198102409 ) ) ;
#84706=CARTESIAN_POINT ( 'NONE',  ( -14.29746914071049879, 8.314922557960819915, 110.8322429386476955 ) ) ;
#84707=CARTESIAN_POINT ( 'NONE',  ( 5.719274019375991003, -21.55341960407610458, 82.70724293864770971 ) ) ;
#84708=CARTESIAN_POINT ( 'NONE',  ( -18.62759615963255300, -10.81492255796106328, 19.16775706135234714 ) ) ;
#84710=CARTESIAN_POINT ( 'NONE',  ( 0.05219959533934541429, -16.53943276465976808, 40.00109039468567573 ) ) ;
#84712=CARTESIAN_POINT ( 'NONE',  ( -18.62759615963270932, 10.81492255796079327, 65.83224293864769550 ) ) ;
#84713=CARTESIAN_POINT ( 'NONE',  ( -0.05219959533937732626, 21.53943276465977519, 97.50109039468567573 ) ) ;
#84714=CARTESIAN_POINT ( 'NONE',  ( 5.153800228976335163, 19.02544592524342804, 94.79057627198103830 ) ) ;
#84715=CARTESIAN_POINT ( 'NONE',  ( -5.719274019375665041, -21.55341960407619695, 24.79275706135235779 ) ) ;
#84716=CARTESIAN_POINT ( 'NONE',  ( -9.474510206698964154, 16.51473224551069663, 105.4155762719810383 ) ) ;
#84717=CARTESIAN_POINT ( 'NONE',  ( -4.379528057220086978, -16.55341960407618274, 94.79275706135234714 ) ) ;
#84718=CARTESIAN_POINT ( 'NONE',  ( -0.05219959533937732626, 21.53943276465977519, 67.50109039468568994 ) ) ;
#84719=CARTESIAN_POINT ( 'NONE',  ( -5.823673210054431948, 21.52544592524334988, 107.7094237280190328 ) ) ;
#84720=CARTESIAN_POINT ( 'NONE',  ( 8.314922557961029526, -14.29746914071037800, 75.41775706135233293 ) ) ;
#84721=CARTESIAN_POINT ( 'NONE',  ( -0.05219959533937732626, 21.53943276465977519, 27.50109039468567929 ) ) ;
#84722=CARTESIAN_POINT ( 'NONE',  ( -9.564922557960796823, -16.46253265017161027, 27.08224293864769550 ) ) ;
#84723=CARTESIAN_POINT ( 'NONE',  ( 5.719274019375673035, 21.55341960407619339, 92.29275706135236135 ) ) ;
#84724=CARTESIAN_POINT ( 'NONE',  ( -9.474510206698964154, 16.51473224551069663, 110.4155762719810383 ) ) ;
#84725=CARTESIAN_POINT ( 'NONE',  ( -15.80617190586745835, -15.72974639402198527, 96.87390960531436690 ) ) ;
#84726=CARTESIAN_POINT ( 'NONE',  ( 18.22780087662122739, 5.500000000000000888, 81.48236817873103632 ) ) ;
#84727=CARTESIAN_POINT ( 'NONE',  ( 18.67979575497178502, 10.72451020669898547, 54.16557627198103120 ) ) ;
#84728=CARTESIAN_POINT ( 'NONE',  ( 19.02544592524343514, -5.153800228976328945, 98.54057627198100988 ) ) ;
#84729=CARTESIAN_POINT ( 'NONE',  ( -16.52544592524342804, 4.483927247898546575, 46.04057627198103830 ) ) ;
#84731=CARTESIAN_POINT ( 'NONE',  ( 9.564922557961047289, -16.46253265017146816, 75.41775706135234714 ) ) ;
#84732=CARTESIAN_POINT ( 'NONE',  ( -16.61371651742600974, 7.165104196376165469, 103.8541506999300026 ) ) ;
#84733=CARTESIAN_POINT ( 'NONE',  ( -8.224510206698735004, -14.34966873604973081, 19.58442372801901143 ) ) ;
#84734=CARTESIAN_POINT ( 'NONE',  ( -18.67979575497178146, -10.72451020669898902, 91.66557627198103830 ) ) ;
#84735=CARTESIAN_POINT ( 'NONE',  ( -8.314922557960811034, -14.29746914071050412, 62.08224293864769550 ) ) ;
#84736=CARTESIAN_POINT ( 'NONE',  ( 5.049401038298161559, -19.05341960407611168, 97.70724293864766707 ) ) ;
#84737=CARTESIAN_POINT ( 'NONE',  ( -4.483927247898782831, 16.52544592524335698, 42.70942372801901854 ) ) ;
#84738=CARTESIAN_POINT ( 'NONE',  ( -9.564922557960796823, -16.46253265017161027, 52.08224293864768839 ) ) ;
#84739=CARTESIAN_POINT ( 'NONE',  ( -18.62759615963255300, -10.81492255796106328, 34.16775706135234714 ) ) ;
#84740=CARTESIAN_POINT ( 'NONE',  ( -19.05341960407617563, 5.049401038297882671, 103.5427570613523329 ) ) ;
#84742=CARTESIAN_POINT ( 'NONE',  ( 13.89961937509977652, -13.97604488694527269, 93.12390960531436690 ) ) ;
#84744=CARTESIAN_POINT ( 'NONE',  ( -5.049401038298153566, 19.05341960407611168, 85.20724293864766707 ) ) ;
#84745=CARTESIAN_POINT ( 'NONE',  ( 18.62759615963271287, -10.81492255796078972, 93.33224293864769550 ) ) ;
#84746=CARTESIAN_POINT ( 'NONE',  ( -19.02544592524342804, 5.153800228976336051, 46.04057627198101699 ) ) ;
#84747=CARTESIAN_POINT ( 'NONE',  ( -0.05219959533910754901, -16.53943276465976808, 72.49890960531435269 ) ) ;
#84748=CARTESIAN_POINT ( 'NONE',  ( 19.02544592524343514, -5.153800228976328945, 108.5405762719810383 ) ) ;
#84750=CARTESIAN_POINT ( 'NONE',  ( 5.153800228976615827, -19.02544592524334988, 60.20942372801899012 ) ) ;
#84751=CARTESIAN_POINT ( 'NONE',  ( 21.55341960407610458, 5.719274019375980345, 93.95724293864770971 ) ) ;
#84752=CARTESIAN_POINT ( 'NONE',  ( 16.51473224551083163, -9.474510206698727899, 50.83442372801899722 ) ) ;
#84753=CARTESIAN_POINT ( 'NONE',  ( 9.474510206698971260, -16.51473224551069308, 97.91557627198102409 ) ) ;
#84755=CARTESIAN_POINT ( 'NONE',  ( 10.72451020669898902, -18.67979575497178502, 47.91557627198102409 ) ) ;
#84756=CARTESIAN_POINT ( 'NONE',  ( -9.564922557960796823, -16.46253265017161027, 87.08224293864769550 ) ) ;
#84757=CARTESIAN_POINT ( 'NONE',  ( -0.05219959533937732626, 21.53943276465977519, 67.50109039468568994 ) ) ;
#84758=CARTESIAN_POINT ( 'NONE',  ( -13.97604488694527625, -13.89961937509977652, 31.87390960531435979 ) ) ;
#84759=CARTESIAN_POINT ( 'NONE',  ( -4.379528057220328563, 16.55341960407611168, 80.20724293864769550 ) ) ;
#84760=CARTESIAN_POINT ( 'NONE',  ( -14.29746914071037622, -8.314922557961029526, 29.16775706135234003 ) ) ;
#84761=CARTESIAN_POINT ( 'NONE',  ( -15.80617190586768217, 15.72974639402176855, 53.12609039468568284 ) ) ;
#84764=CARTESIAN_POINT ( 'NONE',  ( -16.51473224551082808, 9.474510206698731452, 68.33442372801900433 ) ) ;
#84766=CARTESIAN_POINT ( 'NONE',  ( 10.72451020669871369, 18.67979575497193778, 22.08442372801901143 ) ) ;
#84768=CARTESIAN_POINT ( 'NONE',  ( 16.46253265017146816, 9.564922557961045513, 21.66775706135233648 ) ) ;
#84769=CARTESIAN_POINT ( 'NONE',  ( 9.474510206698971260, -16.51473224551069308, 52.91557627198102409 ) ) ;
#84770=CARTESIAN_POINT ( 'NONE',  ( 0.05219959533937995610, -21.53943276465977519, 110.0010903946856757 ) ) ;
#84771=CARTESIAN_POINT ( 'NONE',  ( -14.29746914071037622, -8.314922557961029526, 104.1677570613523471 ) ) ;
#84772=CARTESIAN_POINT ( 'NONE',  ( 19.02544592524343514, -5.153800228976328945, 103.5405762719809957 ) ) ;
#84773=CARTESIAN_POINT ( 'NONE',  ( 10.81492255796106328, -18.62759615963255655, 75.41775706135233293 ) ) ;
#84775=CARTESIAN_POINT ( 'NONE',  ( 13.97604488694527802, 13.89961937509977652, 109.3739096053143669 ) ) ;
#84777=CARTESIAN_POINT ( 'NONE',  ( -14.29746914071037622, -8.314922557961029526, 64.16775706135234714 ) ) ;
#84778=CARTESIAN_POINT ( 'NONE',  ( -21.55341960407619339, 5.719274019375674811, 73.54275706135234714 ) ) ;
#84779=CARTESIAN_POINT ( 'NONE',  ( -5.823673210054431948, 21.52544592524334988, 107.7094237280190328 ) ) ;
#84781=CARTESIAN_POINT ( 'NONE',  ( -19.05341960407611168, -5.049401038298163336, 81.45724293864769550 ) ) ;
#84782=CARTESIAN_POINT ( 'NONE',  ( -9.474510206698964154, 16.51473224551069663, 105.4155762719810383 ) ) ;
#84785=CARTESIAN_POINT ( 'NONE',  ( 0.05219959533909260263, 19.03943276465977164, 39.99890960531436690 ) ) ;
#84786=CARTESIAN_POINT ( 'NONE',  ( 0.05219959533907565091, 21.53943276465977519, 44.99890960531435979 ) ) ;
#84787=CARTESIAN_POINT ( 'NONE',  ( 0.05219959533934541429, -16.53943276465976808, 100.0010903946857042 ) ) ;
#84788=CARTESIAN_POINT ( 'NONE',  ( 4.379528057220339221, -16.55341960407611168, 102.7072429386476955 ) ) ;
#84789=CARTESIAN_POINT ( 'NONE',  ( -13.89961937509977652, 13.97604488694528158, 85.62390960531433848 ) ) ;
#84790=CARTESIAN_POINT ( 'NONE',  ( -10.81492255796105439, 18.62759615963255655, 102.9177570613523756 ) ) ;
#84791=CARTESIAN_POINT ( 'NONE',  ( -16.46253265017160317, 9.564922557960807481, 40.83224293864769550 ) ) ;
#84792=CARTESIAN_POINT ( 'NONE',  ( -4.483927247898539470, -16.52544592524342804, 87.29057627198103830 ) ) ;
#84793=CARTESIAN_POINT ( 'NONE',  ( 21.55341960407619695, -5.719274019375665929, 36.04275706135234714 ) ) ;
#84794=CARTESIAN_POINT ( 'NONE',  ( 21.55341960407610458, 5.719274019375980345, 83.95724293864770971 ) ) ;
#84795=CARTESIAN_POINT ( 'NONE',  ( 0.05219959533936267826, -19.03943276465977164, 50.00109039468566863 ) ) ;
#84797=CARTESIAN_POINT ( 'NONE',  ( -5.049401038298153566, 19.05341960407611168, 100.2072429386476955 ) ) ;
#84798=CARTESIAN_POINT ( 'NONE',  ( -8.314922557960811034, -14.29746914071050412, 62.08224293864769550 ) ) ;
#84799=CARTESIAN_POINT ( 'NONE',  ( -9.564922557961040184, 16.46253265017147172, 42.91775706135234003 ) ) ;
#84800=CARTESIAN_POINT ( 'NONE',  ( -4.483927247898539470, -16.52544592524342804, 47.29057627198103120 ) ) ;
#84801=CARTESIAN_POINT ( 'NONE',  ( 13.97604488694548053, -13.89961937509957401, 80.62609039468567573 ) ) ;
#84803=CARTESIAN_POINT ( 'NONE',  ( 18.62759615963271287, -10.81492255796078972, 33.33224293864769550 ) ) ;
#84804=CARTESIAN_POINT ( 'NONE',  ( 14.34966873604960469, 8.224510206698951720, 94.16557627198103830 ) ) ;
#84806=CARTESIAN_POINT ( 'NONE',  ( -9.564922557960796823, -16.46253265017161027, 52.08224293864768839 ) ) ;
#84807=CARTESIAN_POINT ( 'NONE',  ( -21.53943276465977519, 0.05219959533907696930, 51.24890960531436690 ) ) ;
#84808=CARTESIAN_POINT ( 'NONE',  ( 13.97604488694527802, 13.89961937509977652, 34.37390960531436690 ) ) ;
#84809=CARTESIAN_POINT ( 'NONE',  ( 14.34966873604972726, -8.224510206698740333, 80.83442372801901854 ) ) ;
#84810=CARTESIAN_POINT ( 'NONE',  ( -19.03943276465977164, 0.05219959533909376836, 56.24890960531435979 ) ) ;
#84811=CARTESIAN_POINT ( 'NONE',  ( -13.89961937509957401, -13.97604488694547875, 44.37609039468566863 ) ) ;
#84812=CARTESIAN_POINT ( 'NONE',  ( 15.80617190586769283, -15.72974639402175789, 70.62609039468567573 ) ) ;
#84813=CARTESIAN_POINT ( 'NONE',  ( -21.53943276465977519, 0.05219959533907696930, 51.24890960531436690 ) ) ;
#84814=CARTESIAN_POINT ( 'NONE',  ( -14.29746914071049879, 8.314922557960819915, 115.8322429386477097 ) ) ;
#84815=EDGE_CURVE ( 'NONE', #114713, #20950, #188806, .T. ) ;
#84816=CARTESIAN_POINT ( 'NONE',  ( -9.564922557961040184, 16.46253265017147172, 97.91775706135233293 ) ) ;
#84819=CARTESIAN_POINT ( 'NONE',  ( -0.05219959533907301413, -21.53943276465977519, 47.49890960531435979 ) ) ;
#84820=CARTESIAN_POINT ( 'NONE',  ( -19.05341960407611168, -5.049401038298163336, 26.45724293864769550 ) ) ;
#84821=CARTESIAN_POINT ( 'NONE',  ( -0.05219959533937732626, 21.53943276465977519, 77.50109039468567573 ) ) ;
#84822=CARTESIAN_POINT ( 'NONE',  ( -4.483927247898539470, -16.52544592524342804, 42.29057627198103120 ) ) ;
#84823=CARTESIAN_POINT ( 'NONE',  ( -8.224510206698948167, 14.34966873604960824, 60.41557627198102409 ) ) ;
#84824=CARTESIAN_POINT ( 'NONE',  ( -21.55341960407610458, -5.719274019375992779, 76.45724293864769550 ) ) ;
#84825=CARTESIAN_POINT ( 'NONE',  ( 21.52544592524344225, -5.823673210054117533, 78.54057627198103830 ) ) ;
#84827=CARTESIAN_POINT ( 'NONE',  ( -15.80617190586745835, -15.72974639402198527, 36.87390960531435979 ) ) ;
#84828=CARTESIAN_POINT ( 'NONE',  ( -8.314922557961024197, 14.29746914071037800, 47.91775706135234714 ) ) ;
#84829=CARTESIAN_POINT ( 'NONE',  ( 4.483927247898545687, 16.52544592524342804, 79.79057627198102409 ) ) ;
#84830=CARTESIAN_POINT ( 'NONE',  ( -19.02544592524342804, 5.153800228976336051, 56.04057627198100988 ) ) ;
#84831=CARTESIAN_POINT ( 'NONE',  ( -0.05219959533909027116, -19.03943276465977164, 37.49890960531436690 ) ) ;
#84835=CARTESIAN_POINT ( 'NONE',  ( 8.224510206698742110, 14.34966873604972548, 77.08442372801901854 ) ) ;
#84836=CARTESIAN_POINT ( 'NONE',  ( -15.72974639402176322, -15.80617190586768395, 19.37609039468568639 ) ) ;
#84837=CARTESIAN_POINT ( 'NONE',  ( 5.153800228976335163, 19.02544592524342804, 69.79057627198103830 ) ) ;
#84838=CARTESIAN_POINT ( 'NONE',  ( 21.53943276465977519, 0.05219959533937863772, 56.25109039468568284 ) ) ;
#84839=CARTESIAN_POINT ( 'NONE',  ( 13.97604488694527802, 13.89961937509977652, 114.3739096053143669 ) ) ;
#84842=CARTESIAN_POINT ( 'NONE',  ( -10.72451020669870658, -18.67979575497194134, 49.58442372801901143 ) ) ;
#84843=FACE_OUTER_BOUND ( 'NONE', #168286, .T. ) ;
#84844=CARTESIAN_POINT ( 'NONE',  ( -16.51473224551069308, -9.474510206698971260, 106.6655762719810383 ) ) ;
#84845=CARTESIAN_POINT ( 'NONE',  ( -9.564922557961040184, 16.46253265017147172, 57.91775706135233293 ) ) ;
#84846=CARTESIAN_POINT ( 'NONE',  ( 10.81492255796078972, 18.62759615963270932, 114.5822429386477097 ) ) ;
#84847=CARTESIAN_POINT ( 'NONE',  ( 0.05219959533936267826, -19.03943276465977164, 45.00109039468566863 ) ) ;
#84848=CARTESIAN_POINT ( 'NONE',  ( 9.564922557960805705, 16.46253265017160317, 24.58224293864769194 ) ) ;
#84849=CARTESIAN_POINT ( 'NONE',  ( 0.05219959533934541429, -16.53943276465976808, 90.00109039468567573 ) ) ;
#84850=CARTESIAN_POINT ( 'NONE',  ( 19.02544592524334988, 5.153800228976608722, 56.45942372801898301 ) ) ;
#84851=CARTESIAN_POINT ( 'NONE',  ( 16.52544592524335698, 4.483927247898782831, 111.4594237280190328 ) ) ;
#84853=CARTESIAN_POINT ( 'NONE',  ( -19.02544592524342804, 5.153800228976336051, 81.04057627198103830 ) ) ;
#84854=CARTESIAN_POINT ( 'NONE',  ( -15.80617190586768217, 15.72974639402176855, 98.12609039468570415 ) ) ;
#84855=CARTESIAN_POINT ( 'NONE',  ( 21.52544592524334988, 5.823673210054432836, 96.45942372801901854 ) ) ;
#84856=CARTESIAN_POINT ( 'NONE',  ( 17.50000000000000000, 5.499999999999992895, 66.70309617465828467 ) ) ;
#84857=CARTESIAN_POINT ( 'NONE',  ( 19.05341960407611168, 5.049401038298154454, 98.95724293864766707 ) ) ;
#84858=CARTESIAN_POINT ( 'NONE',  ( 18.62759615963255655, 10.81492255796105972, 81.66775706135236135 ) ) ;
#84859=CARTESIAN_POINT ( 'NONE',  ( -19.05341960407617563, 5.049401038297882671, 113.5427570613523471 ) ) ;
#84860=CARTESIAN_POINT ( 'NONE',  ( -13.89961937509977652, 13.97604488694528158, 85.62390960531433848 ) ) ;
#84861=CARTESIAN_POINT ( 'NONE',  ( -15.80617190586745835, -15.72974639402198527, 26.87390960531435979 ) ) ;
#84862=CARTESIAN_POINT ( 'NONE',  ( -9.474510206698964154, 16.51473224551069663, 90.41557627198103830 ) ) ;
#84863=CARTESIAN_POINT ( 'NONE',  ( -16.29526858892876362, -7.335722546920120379, 90.79670597800210885 ) ) ;
#84864=CARTESIAN_POINT ( 'NONE',  ( -19.03943276465977164, 0.05219959533909376836, 81.24890960531436690 ) ) ;
#84865=CARTESIAN_POINT ( 'NONE',  ( -13.89961937509977652, 13.97604488694528158, 65.62390960531436690 ) ) ;
#84866=CARTESIAN_POINT ( 'NONE',  ( -0.05219959533934338120, 16.53943276465976808, 102.5010903946856899 ) ) ;
#84868=CARTESIAN_POINT ( 'NONE',  ( -13.97604488694547697, 13.89961937509957934, 53.12609039468565442 ) ) ;
#84869=CARTESIAN_POINT ( 'NONE',  ( -5.049401038298153566, 19.05341960407611168, 95.20724293864770971 ) ) ;
#84870=CARTESIAN_POINT ( 'NONE',  ( 14.34966873604960469, 8.224510206698951720, 89.16557627198102409 ) ) ;
#84871=CARTESIAN_POINT ( 'NONE',  ( -5.719274019375978568, 21.55341960407610458, 35.20724293864768839 ) ) ;
#84872=CARTESIAN_POINT ( 'NONE',  ( 5.049401038298161559, -19.05341960407611168, 112.7072429386476813 ) ) ;
#84874=CARTESIAN_POINT ( 'NONE',  ( 4.483927247898545687, 16.52544592524342804, 94.79057627198105251 ) ) ;
#84876=CARTESIAN_POINT ( 'NONE',  ( -5.153800228976607833, 19.02544592524334988, 42.70942372801901143 ) ) ;
#84877=CARTESIAN_POINT ( 'NONE',  ( -8.224510206698735004, -14.34966873604973081, 109.5844237280190328 ) ) ;
#84878=CARTESIAN_POINT ( 'NONE',  ( -16.46253265017160317, 9.564922557960807481, 90.83224293864769550 ) ) ;
#84879=CARTESIAN_POINT ( 'NONE',  ( 5.719274019375673035, 21.55341960407619339, 72.29275706135236135 ) ) ;
#84880=CARTESIAN_POINT ( 'NONE',  ( -15.72974639402197994, 15.80617190586746368, 60.62390960531437401 ) ) ;
#84881=CARTESIAN_POINT ( 'NONE',  ( -0.05219959533937732626, 21.53943276465977519, 27.50109039468567929 ) ) ;
#84882=CARTESIAN_POINT ( 'NONE',  ( -5.719274019375978568, 21.55341960407610458, 85.20724293864770971 ) ) ;
#84883=CARTESIAN_POINT ( 'NONE',  ( -0.05219959533937732626, 21.53943276465977519, 37.50109039468568284 ) ) ;
#84884=CARTESIAN_POINT ( 'NONE',  ( -8.224510206698948167, 14.34966873604960824, 105.4155762719810383 ) ) ;
#84885=CARTESIAN_POINT ( 'NONE',  ( 9.564922557961047289, -16.46253265017146816, 65.41775706135233293 ) ) ;
#84886=CARTESIAN_POINT ( 'NONE',  ( -5.049401038298153566, 19.05341960407611168, 50.20724293864770260 ) ) ;
#84887=CARTESIAN_POINT ( 'NONE',  ( 4.483927247898545687, 16.52544592524342804, 89.79057627198103830 ) ) ;
#84888=CARTESIAN_POINT ( 'NONE',  ( -9.564922557960796823, -16.46253265017161027, 97.08224293864769550 ) ) ;
#84889=CARTESIAN_POINT ( 'NONE',  ( 19.02544592524343514, -5.153800228976328945, 98.54057627198100988 ) ) ;
#84890=CARTESIAN_POINT ( 'NONE',  ( -0.05219959533910754901, -16.53943276465976808, 112.4989096053143669 ) ) ;
#84891=CARTESIAN_POINT ( 'NONE',  ( 8.224510206698953496, -14.34966873604960469, 42.91557627198103120 ) ) ;
#84892=CARTESIAN_POINT ( 'NONE',  ( -5.049401038298153566, 19.05341960407611168, 50.20724293864770260 ) ) ;
#84893=CARTESIAN_POINT ( 'NONE',  ( 16.46253265017160672, -9.564922557960803928, 23.33224293864769194 ) ) ;
#84894=CARTESIAN_POINT ( 'NONE',  ( 13.97604488694548053, -13.89961937509957401, 30.62609039468566863 ) ) ;
#84895=CARTESIAN_POINT ( 'NONE',  ( -19.03943276465977164, 0.05219959533909376836, 111.2489096053143669 ) ) ;
#84896=CARTESIAN_POINT ( 'NONE',  ( -16.53943276465976808, 0.05219959533911058130, 26.24890960531435624 ) ) ;
#84897=CARTESIAN_POINT ( 'NONE',  ( -0.05219959533937732626, 21.53943276465977519, 37.50109039468568284 ) ) ;
#84898=CARTESIAN_POINT ( 'NONE',  ( -16.46253265017160317, 9.564922557960807481, 110.8322429386476955 ) ) ;
#84899=CARTESIAN_POINT ( 'NONE',  ( 8.224510206698742110, 14.34966873604972548, 42.08442372801901854 ) ) ;
#84900=CARTESIAN_POINT ( 'NONE',  ( -16.53943276465976808, -0.05219959533934237506, 103.7510903946857042 ) ) ;
#84901=CARTESIAN_POINT ( 'NONE',  ( 12.14591786802327356, -12.06949235617739191, 90.62609039468567573 ) ) ;
#84902=CARTESIAN_POINT ( 'NONE',  ( -4.379528057220086978, -16.55341960407618274, 29.79275706135234358 ) ) ;
#84903=CARTESIAN_POINT ( 'NONE',  ( -5.153800228976328057, -19.02544592524343514, 47.29057627198102409 ) ) ;
#84905=CARTESIAN_POINT ( 'NONE',  ( 12.14591786802309770, 12.06949235617756955, 114.3739096053143527 ) ) ;
#84906=CARTESIAN_POINT ( 'NONE',  ( -21.53943276465977519, -0.05219959533937600094, 18.75109039468568639 ) ) ;
#84907=CARTESIAN_POINT ( 'NONE',  ( -9.564922557960796823, -16.46253265017161027, 37.08224293864768839 ) ) ;
#84908=CARTESIAN_POINT ( 'NONE',  ( 16.46253265017160672, -9.564922557960803928, 108.3322429386476955 ) ) ;
#84909=CARTESIAN_POINT ( 'NONE',  ( 9.474510206698971260, -16.51473224551069308, 37.91557627198102409 ) ) ;
#84910=CARTESIAN_POINT ( 'NONE',  ( 19.05341960407611168, 5.049401038298154454, 98.95724293864766707 ) ) ;
#84912=CARTESIAN_POINT ( 'NONE',  ( 5.049401038298161559, -19.05341960407611168, 92.70724293864769550 ) ) ;
#84913=CARTESIAN_POINT ( 'NONE',  ( 15.72974639402176855, 15.80617190586768217, 41.87609039468568284 ) ) ;
#84914=CARTESIAN_POINT ( 'NONE',  ( -4.379528057220328563, 16.55341960407611168, 105.2072429386477097 ) ) ;
#84915=CARTESIAN_POINT ( 'NONE',  ( 5.049401038298161559, -19.05341960407611168, 112.7072429386476813 ) ) ;
#84917=CARTESIAN_POINT ( 'NONE',  ( -12.14591786802326823, 12.06949235617739902, 58.12609039468568994 ) ) ;
#84918=CARTESIAN_POINT ( 'NONE',  ( -18.67979575497193778, 10.72451020669871902, 78.33442372801901854 ) ) ;
#84919=CARTESIAN_POINT ( 'NONE',  ( -8.224510206698735004, -14.34966873604973081, 39.58442372801901143 ) ) ;
#84920=CARTESIAN_POINT ( 'NONE',  ( -5.153800228976328057, -19.02544592524343514, 87.29057627198103830 ) ) ;
#84921=CARTESIAN_POINT ( 'NONE',  ( -19.03943276465977164, -0.05219959533935918106, 113.7510903946856757 ) ) ;
#84922=CARTESIAN_POINT ( 'NONE',  ( -8.314922557961024197, 14.29746914071037800, 82.91775706135234714 ) ) ;
#84923=CARTESIAN_POINT ( 'NONE',  ( -5.049401038297874678, -19.05341960407617918, 89.79275706135230450 ) ) ;
#84924=CARTESIAN_POINT ( 'NONE',  ( 16.46253265017160672, -9.564922557960803928, 68.33224293864770971 ) ) ;
#84925=CARTESIAN_POINT ( 'NONE',  ( -5.719274019375978568, 21.55341960407610458, 95.20724293864769550 ) ) ;
#84926=CARTESIAN_POINT ( 'NONE',  ( 16.53943276465976808, -0.05219959533910856209, 83.74890960531435269 ) ) ;
#84927=CARTESIAN_POINT ( 'NONE',  ( -9.474510206698720793, -16.51473224551083518, 84.58442372801900433 ) ) ;
#84928=CARTESIAN_POINT ( 'NONE',  ( 8.224510206698742110, 14.34966873604972548, 62.08442372801901143 ) ) ;
#84930=CARTESIAN_POINT ( 'NONE',  ( 16.46253265017146816, 9.564922557961045513, 76.66775706135234714 ) ) ;
#84931=CARTESIAN_POINT ( 'NONE',  ( -0.05219959533910754901, -16.53943276465976808, 32.49890960531435979 ) ) ;
#84932=CARTESIAN_POINT ( 'NONE',  ( 8.314922557960818139, 14.29746914071049879, 74.58224293864768129 ) ) ;
#84933=CARTESIAN_POINT ( 'NONE',  ( 19.02544592524334988, 5.153800228976608722, 26.45942372801899722 ) ) ;
#84934=CARTESIAN_POINT ( 'NONE',  ( -16.62475595723610411, 7.163666690055884523, 40.52713351810402287 ) ) ;
#84935=CARTESIAN_POINT ( 'NONE',  ( -10.72451020669870658, -18.67979575497194134, 29.58442372801901854 ) ) ;
#84936=CARTESIAN_POINT ( 'NONE',  ( 19.02544592524343514, -5.153800228976328945, 108.5405762719810383 ) ) ;
#84937=CARTESIAN_POINT ( 'NONE',  ( 13.97604488694527802, 13.89961937509977652, 84.37390960531433848 ) ) ;
#84938=CARTESIAN_POINT ( 'NONE',  ( 5.719274019375673035, 21.55341960407619339, 102.2927570613523613 ) ) ;
#84939=CARTESIAN_POINT ( 'NONE',  ( 0.05219959533909260263, 19.03943276465977164, 69.99890960531435269 ) ) ;
#84940=CARTESIAN_POINT ( 'NONE',  ( -21.53943276465977519, 0.05219959533907696930, 46.24890960531435979 ) ) ;
#84941=CARTESIAN_POINT ( 'NONE',  ( -4.379528057220328563, 16.55341960407611168, 80.20724293864769550 ) ) ;
#84942=CARTESIAN_POINT ( 'NONE',  ( 16.46253265017160672, -9.564922557960803928, 58.33224293864769550 ) ) ;
#84943=CARTESIAN_POINT ( 'NONE',  ( -16.55341960407611168, -4.379528057220339221, 106.4572429386477097 ) ) ;
#84944=CARTESIAN_POINT ( 'NONE',  ( -10.81492255796105439, 18.62759615963255655, 22.91775706135235069 ) ) ;
#84945=CARTESIAN_POINT ( 'NONE',  ( 18.62759615963255655, 10.81492255796105972, 56.66775706135235424 ) ) ;
#84946=CARTESIAN_POINT ( 'NONE',  ( 19.05341960407611168, 5.049401038298154454, 48.95724293864768129 ) ) ;
#84947=CARTESIAN_POINT ( 'NONE',  ( -14.34966873604972548, 8.224510206698743886, 73.33442372801901854 ) ) ;
#84948=CARTESIAN_POINT ( 'NONE',  ( 5.719274019375991003, -21.55341960407610458, 107.7072429386476955 ) ) ;
#84949=CARTESIAN_POINT ( 'NONE',  ( -10.72451020669870658, -18.67979575497194134, 19.58442372801901143 ) ) ;
#84950=CARTESIAN_POINT ( 'NONE',  ( 13.97604488694548053, -13.89961937509957401, 35.62609039468567573 ) ) ;
#84951=CARTESIAN_POINT ( 'NONE',  ( -9.564922557960796823, -16.46253265017161027, 62.08224293864769550 ) ) ;
#84952=CARTESIAN_POINT ( 'NONE',  ( -19.03943276465977164, -0.05219959533935918106, 33.75109039468566863 ) ) ;
#84953=CARTESIAN_POINT ( 'NONE',  ( -15.72974639402176322, -15.80617190586768395, 69.37609039468567573 ) ) ;
#84954=CARTESIAN_POINT ( 'NONE',  ( 21.52544592524344225, -5.823673210054117533, 63.54057627198103830 ) ) ;
#84955=CARTESIAN_POINT ( 'NONE',  ( -16.53943276465976808, 0.05219959533911058130, 41.24890960531435269 ) ) ;
#84956=CARTESIAN_POINT ( 'NONE',  ( 15.72974639402176855, 15.80617190586768217, 91.87609039468568994 ) ) ;
#84957=CARTESIAN_POINT ( 'NONE',  ( 0.05219959533936267826, -19.03943276465977164, 20.00109039468567218 ) ) ;
#84958=CARTESIAN_POINT ( 'NONE',  ( -14.34966873604960291, -8.224510206698953496, 56.66557627198103830 ) ) ;
#84959=CARTESIAN_POINT ( 'NONE',  ( -14.34966873604960291, -8.224510206698953496, 101.6655762719810383 ) ) ;
#84960=CARTESIAN_POINT ( 'NONE',  ( 16.51473224551083163, -9.474510206698727899, 55.83442372801899722 ) ) ;
#84961=CARTESIAN_POINT ( 'NONE',  ( 14.29746914071049879, -8.314922557960816363, 23.33224293864769194 ) ) ;
#84962=CARTESIAN_POINT ( 'NONE',  ( -18.67979575497193778, 10.72451020669871902, 63.33442372801900433 ) ) ;
#84963=CARTESIAN_POINT ( 'NONE',  ( -19.02544592524342804, 5.153800228976336051, 76.04057627198102409 ) ) ;
#84964=CARTESIAN_POINT ( 'NONE',  ( -9.564922557961040184, 16.46253265017147172, 42.91775706135234003 ) ) ;
#84965=CARTESIAN_POINT ( 'NONE',  ( 15.72974639402199770, -15.80617190586745480, 58.12390960531435979 ) ) ;
#84966=CARTESIAN_POINT ( 'NONE',  ( 10.81492255796106328, -18.62759615963255655, 45.41775706135234003 ) ) ;
#84967=CARTESIAN_POINT ( 'NONE',  ( 18.62759615963271287, -10.81492255796078972, 103.3322429386476955 ) ) ;
#84968=CARTESIAN_POINT ( 'NONE',  ( 19.02544592524334988, 5.153800228976608722, 96.45942372801897591 ) ) ;
#84969=CARTESIAN_POINT ( 'NONE',  ( -16.55341960407617563, 4.379528057220093196, 63.54275706135234003 ) ) ;
#84970=CARTESIAN_POINT ( 'NONE',  ( -18.62759615963270932, 10.81492255796079327, 110.8322429386476955 ) ) ;
#84971=CARTESIAN_POINT ( 'NONE',  ( -12.14591786802309592, -12.06949235617757132, 86.87390960531438111 ) ) ;
#84972=CARTESIAN_POINT ( 'NONE',  ( -17.40861289039002457, -6.110651285853315962, 101.3723247082743200 ) ) ;
#84973=CARTESIAN_POINT ( 'NONE',  ( 12.14591786802327356, -12.06949235617739191, 20.62609039468568639 ) ) ;
#84975=CARTESIAN_POINT ( 'NONE',  ( 21.55341960407610458, 5.719274019375980345, 48.95724293864770971 ) ) ;
#84976=CARTESIAN_POINT ( 'NONE',  ( -8.314922557961024197, 14.29746914071037800, 87.91775706135234714 ) ) ;
#84978=CARTESIAN_POINT ( 'NONE',  ( 12.06949235617739724, 12.14591786802326823, 71.87609039468568994 ) ) ;
#84979=CARTESIAN_POINT ( 'NONE',  ( -15.72974639402176322, -15.80617190586768395, 29.37609039468568284 ) ) ;
#84980=CARTESIAN_POINT ( 'NONE',  ( 5.823673210054125526, 21.52544592524343514, 39.79057627198103830 ) ) ;
#84981=CARTESIAN_POINT ( 'NONE',  ( -8.314922557961024197, 14.29746914071037800, 82.91775706135234714 ) ) ;
#84982=CARTESIAN_POINT ( 'NONE',  ( -19.05341960407611168, -5.049401038298163336, 96.45724293864769550 ) ) ;
#84983=CARTESIAN_POINT ( 'NONE',  ( -15.72974639402176322, -15.80617190586768395, 64.37609039468568994 ) ) ;
#84985=CARTESIAN_POINT ( 'NONE',  ( -21.53943276465977519, 0.05219959533907696930, 46.24890960531435979 ) ) ;
#84986=CARTESIAN_POINT ( 'NONE',  ( 21.55341960407610458, 5.719274019375980345, 38.95724293864768839 ) ) ;
#84988=CARTESIAN_POINT ( 'NONE',  ( 5.153800228976615827, -19.02544592524334988, 50.20942372801897591 ) ) ;
#84989=CARTESIAN_POINT ( 'NONE',  ( 12.06949235617739724, 12.14591786802326823, 71.87609039468568994 ) ) ;
#84990=CARTESIAN_POINT ( 'NONE',  ( 21.52544592524344225, -5.823673210054117533, 28.54057627198103120 ) ) ;
#84992=CARTESIAN_POINT ( 'NONE',  ( 16.46253265017160672, -9.564922557960803928, 83.33224293864768129 ) ) ;
#84993=CARTESIAN_POINT ( 'NONE',  ( -12.06949235617756955, 12.14591786802309770, 25.62390960531435624 ) ) ;
#84995=CARTESIAN_POINT ( 'NONE',  ( -16.52544592524342804, 4.483927247898546575, 106.0405762719810525 ) ) ;
#84996=CARTESIAN_POINT ( 'NONE',  ( -0.05219959533907301413, -21.53943276465977519, 47.49890960531435979 ) ) ;
#84997=CARTESIAN_POINT ( 'NONE',  ( 5.049401038298161559, -19.05341960407611168, 47.70724293864770260 ) ) ;
#84998=CARTESIAN_POINT ( 'NONE',  ( -4.379528057220086978, -16.55341960407618274, 74.79275706135234714 ) ) ;
#84999=CARTESIAN_POINT ( 'NONE',  ( -10.81492255796105439, 18.62759615963255655, 37.91775706135235424 ) ) ;
#85000=CARTESIAN_POINT ( 'NONE',  ( -19.02544592524334988, -5.153800228976617603, 88.95942372801897591 ) ) ;
#85001=CARTESIAN_POINT ( 'NONE',  ( 12.14591786802309770, 12.06949235617756955, 94.37390960531436690 ) ) ;
#85002=CARTESIAN_POINT ( 'NONE',  ( -9.474510206698964154, 16.51473224551069663, 50.41557627198102409 ) ) ;
#85003=CARTESIAN_POINT ( 'NONE',  ( 16.46253265017160672, -9.564922557960803928, 33.33224293864770260 ) ) ;
#85004=CARTESIAN_POINT ( 'NONE',  ( -5.823673210054431948, 21.52544592524334988, 102.7094237280190185 ) ) ;
#85005=CARTESIAN_POINT ( 'NONE',  ( -16.46253265017160317, 9.564922557960807481, 75.83224293864769550 ) ) ;
#85006=CARTESIAN_POINT ( 'NONE',  ( -4.483927247898782831, 16.52544592524335698, 62.70942372801902565 ) ) ;
#85007=B_SPLINE_CURVE_WITH_KNOTS ( 'NONE', 3,
 ( #174817, #34316, #65637, #173837, #79821, #190979, #95979, #2976, #158638, #127297, #128293, #189010, #21125, #50485, #189991, #52456, #82781, #112145, #22128, #156670, #144462, #35303 ),
 .UNSPECIFIED., .F., .F.,
 ( 4, 2, 2, 2, 2, 2, 2, 2, 2, 2, 4 ),
 ( 2.776912483567713316E-17, 0.001309639967555412338, 0.001964459951333103437, 0.002291869943221948227, 0.002455574939166377344, 0.002619279935110806028, 0.002782984931055234711, 0.002946689926999664262, 0.003274099918888506884, 0.003928919902666203404, 0.005238559870221597310 ),
 .UNSPECIFIED. ) ;
#85008=CARTESIAN_POINT ( 'NONE',  ( -21.53943276465977519, -0.05219959533937600094, 88.75109039468567573 ) ) ;
#85009=CARTESIAN_POINT ( 'NONE',  ( 10.81492255796078972, 18.62759615963270932, 49.58224293864769550 ) ) ;
#85010=CARTESIAN_POINT ( 'NONE',  ( 4.483927247898790824, -16.52544592524335698, 80.20942372801901854 ) ) ;
#85011=CARTESIAN_POINT ( 'NONE',  ( -9.564922557961040184, 16.46253265017147172, 47.91775706135233293 ) ) ;
#85012=CARTESIAN_POINT ( 'NONE',  ( 16.46253265017146816, 9.564922557961045513, 66.66775706135233293 ) ) ;
#85013=CARTESIAN_POINT ( 'NONE',  ( 10.72451020669871369, 18.67979575497193778, 62.08442372801901143 ) ) ;
#85014=CARTESIAN_POINT ( 'NONE',  ( -19.05341960407611168, -5.049401038298163336, 71.45724293864766707 ) ) ;
#85015=CARTESIAN_POINT ( 'NONE',  ( -19.05341960407611168, -5.049401038298163336, 21.45724293864768839 ) ) ;
#85016=CARTESIAN_POINT ( 'NONE',  ( -9.474510206698720793, -16.51473224551083518, 54.58442372801899722 ) ) ;
#85018=CARTESIAN_POINT ( 'NONE',  ( 0.05219959533909260263, 19.03943276465977164, 89.99890960531436690 ) ) ;
#85019=CARTESIAN_POINT ( 'NONE',  ( -12.06949235617756955, 12.14591786802309770, 50.62390960531435979 ) ) ;
#85020=CARTESIAN_POINT ( 'NONE',  ( -5.823673210054116645, -21.52544592524344225, 52.29057627198102409 ) ) ;
#85021=B_SPLINE_CURVE_WITH_KNOTS ( 'NONE', 3,
 ( #105134, #11147, #72821, #74797, #136459, #85967 ),
 .UNSPECIFIED., .F., .F.,
 ( 4, 2, 4 ),
 ( 0.003239945802372281181, 0.003620412082092138578, 0.004000878361811996409 ),
 .UNSPECIFIED. ) ;
#85023=CARTESIAN_POINT ( 'NONE',  ( -18.67979575497193778, 10.72451020669871902, 108.3344237280190185 ) ) ;
#85024=CARTESIAN_POINT ( 'NONE',  ( -17.31747979337951548, -6.344076630960987728, 81.37944868065184778 ) ) ;
#85025=CARTESIAN_POINT ( 'NONE',  ( -16.46253265017160317, 9.564922557960807481, 45.83224293864769550 ) ) ;
#85026=CARTESIAN_POINT ( 'NONE',  ( -5.049401038298153566, 19.05341960407611168, 85.20724293864769550 ) ) ;
#85027=CARTESIAN_POINT ( 'NONE',  ( -17.49999999999999289, 5.500000000000037303, 80.79690382534172954 ) ) ;
#85028=CARTESIAN_POINT ( 'NONE',  ( -17.31747979337947640, 6.344076630961060559, 108.6205513193481664 ) ) ;
#85029=CARTESIAN_POINT ( 'NONE',  ( 12.14591786802327356, -12.06949235617739191, 60.62609039468567573 ) ) ;
#85030=CARTESIAN_POINT ( 'NONE',  ( 21.55341960407610458, 5.719274019375980345, 78.95724293864769550 ) ) ;
#85031=CARTESIAN_POINT ( 'NONE',  ( -0.05219959533910754901, -16.53943276465976808, 57.49890960531435979 ) ) ;
#85032=CARTESIAN_POINT ( 'NONE',  ( -9.564922557960796823, -16.46253265017161027, 47.08224293864769550 ) ) ;
#85033=CARTESIAN_POINT ( 'NONE',  ( -19.03943276465977164, 0.05219959533909376836, 116.2489096053143669 ) ) ;
#85034=CARTESIAN_POINT ( 'NONE',  ( -0.05219959533937732626, 21.53943276465977519, 37.50109039468568284 ) ) ;
#85035=CARTESIAN_POINT ( 'NONE',  ( -0.05219959533936034679, 19.03943276465977164, 47.50109039468566863 ) ) ;
#85036=CARTESIAN_POINT ( 'NONE',  ( 16.46253265017160672, -9.564922557960803928, 33.33224293864770260 ) ) ;
#85037=CARTESIAN_POINT ( 'NONE',  ( -21.55341960407619339, 5.719274019375674811, 98.54275706135234714 ) ) ;
#85038=CARTESIAN_POINT ( 'NONE',  ( -18.22780087662114212, 5.499999999999995559, 48.51540105326107266 ) ) ;
#85039=CARTESIAN_POINT ( 'NONE',  ( -16.55341960407611168, -4.379528057220339221, 46.45724293864769550 ) ) ;
#85041=CARTESIAN_POINT ( 'NONE',  ( 5.719274019375991003, -21.55341960407610458, 37.70724293864769550 ) ) ;
#85043=CARTESIAN_POINT ( 'NONE',  ( 16.46253265017160672, -9.564922557960803928, 83.33224293864768129 ) ) ;
#85044=CARTESIAN_POINT ( 'NONE',  ( -12.14591786802309592, -12.06949235617757132, 86.87390960531438111 ) ) ;
#85045=CARTESIAN_POINT ( 'NONE',  ( 16.52544592524335698, 4.483927247898782831, 21.45942372801901499 ) ) ;
#85046=CARTESIAN_POINT ( 'NONE',  ( 16.53943276465976808, 0.05219959533934440121, 111.2510903946856899 ) ) ;
#85048=CARTESIAN_POINT ( 'NONE',  ( -19.03943276465977164, 0.05219959533909376836, 46.24890960531435979 ) ) ;
#85049=CARTESIAN_POINT ( 'NONE',  ( 16.51473224551069308, 9.474510206698969483, 84.16557627198102409 ) ) ;
#85050=CARTESIAN_POINT ( 'NONE',  ( -18.62759615963270932, 10.81492255796079327, 95.83224293864770971 ) ) ;
#85052=CARTESIAN_POINT ( 'NONE',  ( 16.53943276465976808, -0.05219959533910856209, 28.74890960531435624 ) ) ;
#85053=CARTESIAN_POINT ( 'NONE',  ( 9.564922557960805705, 16.46253265017160317, 104.5822429386476955 ) ) ;
#85054=CARTESIAN_POINT ( 'NONE',  ( 0.05219959533936267826, -19.03943276465977164, 75.00109039468566152 ) ) ;
#85055=CARTESIAN_POINT ( 'NONE',  ( -10.72451020669870658, -18.67979575497194134, 104.5844237280190185 ) ) ;
#85056=CARTESIAN_POINT ( 'NONE',  ( 18.62759615963271287, -10.81492255796078972, 83.33224293864769550 ) ) ;
#85057=CARTESIAN_POINT ( 'NONE',  ( 21.52544592524344225, -5.823673210054117533, 43.54057627198103830 ) ) ;
#85058=CARTESIAN_POINT ( 'NONE',  ( -0.05219959533909027116, -19.03943276465977164, 67.49890960531436690 ) ) ;
#85059=CARTESIAN_POINT ( 'NONE',  ( -8.224510206698948167, 14.34966873604960824, 30.41557627198101699 ) ) ;
#85060=CARTESIAN_POINT ( 'NONE',  ( -19.03943276465977164, 0.05219959533909376836, 81.24890960531436690 ) ) ;
#85061=VERTEX_POINT ( 'NONE', #6743 ) ;
#85063=CARTESIAN_POINT ( 'NONE',  ( -9.474510206698720793, -16.51473224551083518, 34.58442372801899722 ) ) ;
#85064=CARTESIAN_POINT ( 'NONE',  ( -0.05219959533910754901, -16.53943276465976808, 82.49890960531436690 ) ) ;
#85065=CARTESIAN_POINT ( 'NONE',  ( 21.55341960407619695, -5.719274019375665929, 26.04275706135235779 ) ) ;
#85067=CARTESIAN_POINT ( 'NONE',  ( -15.72974639402197994, 15.80617190586746368, 75.62390960531439532 ) ) ;
#85068=CARTESIAN_POINT ( 'NONE',  ( -12.14591786802326823, 12.06949235617739902, 98.12609039468570415 ) ) ;
#85069=CARTESIAN_POINT ( 'NONE',  ( -16.52544592524342804, 4.483927247898546575, 116.0405762719810383 ) ) ;
#85070=CARTESIAN_POINT ( 'NONE',  ( -16.46253265017160317, 9.564922557960807481, 75.83224293864769550 ) ) ;
#85071=LINE ( 'NONE', #193277, #164134 ) ;
#85072=CARTESIAN_POINT ( 'NONE',  ( 16.52544592524342804, -4.483927247898539470, 28.54057627198103120 ) ) ;
#85073=CARTESIAN_POINT ( 'NONE',  ( -10.81492255796105439, 18.62759615963255655, 57.91775706135234714 ) ) ;
#85075=CARTESIAN_POINT ( 'NONE',  ( 15.72974639402176855, 15.80617190586768217, 91.87609039468568994 ) ) ;
#85076=CARTESIAN_POINT ( 'NONE',  ( -9.474510206698964154, 16.51473224551069663, 40.41557627198103120 ) ) ;
#85077=CARTESIAN_POINT ( 'NONE',  ( -13.97604488694527625, -13.89961937509977652, 46.87390960531435979 ) ) ;
#85079=CARTESIAN_POINT ( 'NONE',  ( 15.80617190586769283, -15.72974639402175789, 95.62609039468568994 ) ) ;
#85080=CARTESIAN_POINT ( 'NONE',  ( 16.52544592524335698, 4.483927247898782831, 61.45942372801901854 ) ) ;
#85081=CARTESIAN_POINT ( 'NONE',  ( -10.72451020669870658, -18.67979575497194134, 79.58442372801903275 ) ) ;
#85082=CARTESIAN_POINT ( 'NONE',  ( -0.05219959533907301413, -21.53943276465977519, 22.49890960531436335 ) ) ;
#85083=CARTESIAN_POINT ( 'NONE',  ( 13.89961937509957401, 13.97604488694547697, 96.87609039468566152 ) ) ;
#85084=CARTESIAN_POINT ( 'NONE',  ( -18.62759615963255300, -10.81492255796106328, 54.16775706135235424 ) ) ;
#85085=CARTESIAN_POINT ( 'NONE',  ( -12.06949235617739369, -12.14591786802326823, 34.37609039468568284 ) ) ;
#85086=CARTESIAN_POINT ( 'NONE',  ( -21.53943276465977519, 0.05219959533907696930, 86.24890960531436690 ) ) ;
#85087=CARTESIAN_POINT ( 'NONE',  ( -19.02544592524334988, -5.153800228976617603, 83.95942372801901854 ) ) ;
#85088=CARTESIAN_POINT ( 'NONE',  ( 13.89961937509977652, -13.97604488694527269, 68.12390960531436690 ) ) ;
#85089=CARTESIAN_POINT ( 'NONE',  ( 5.153800228976615827, -19.02544592524334988, 95.20942372801897591 ) ) ;
#85090=CARTESIAN_POINT ( 'NONE',  ( -19.05341960407617563, 5.049401038297882671, 103.5427570613523329 ) ) ;
#85091=CARTESIAN_POINT ( 'NONE',  ( 16.55341960407611168, 4.379528057220329451, 53.95724293864770260 ) ) ;
#85092=CARTESIAN_POINT ( 'NONE',  ( 9.564922557961047289, -16.46253265017146816, 75.41775706135234714 ) ) ;
#85093=CARTESIAN_POINT ( 'NONE',  ( -4.379528057220086978, -16.55341960407618274, 54.79275706135235424 ) ) ;
#85094=CARTESIAN_POINT ( 'NONE',  ( -16.46253265017146816, -9.564922557961047289, 39.16775706135234003 ) ) ;
#85095=CARTESIAN_POINT ( 'NONE',  ( 5.153800228976335163, 19.02544592524342804, 39.79057627198100988 ) ) ;
#85096=CARTESIAN_POINT ( 'NONE',  ( -16.51473224551069308, -9.474510206698971260, 56.66557627198103120 ) ) ;
#85097=CARTESIAN_POINT ( 'NONE',  ( -16.55341960407617563, 4.379528057220093196, 58.54275706135235424 ) ) ;
#85100=CARTESIAN_POINT ( 'NONE',  ( -19.02544592524342804, 5.153800228976336051, 106.0405762719810241 ) ) ;
#85101=CARTESIAN_POINT ( 'NONE',  ( 5.153800228976335163, 19.02544592524342804, 24.79057627198102765 ) ) ;
#85103=CARTESIAN_POINT ( 'NONE',  ( -19.02544592524334988, -5.153800228976617603, 103.9594237280190043 ) ) ;
#85104=CARTESIAN_POINT ( 'NONE',  ( -21.53943276465977519, 0.05219959533907696930, 31.24890960531435979 ) ) ;
#85105=CARTESIAN_POINT ( 'NONE',  ( 16.51473224551083163, -9.474510206698727899, 35.83442372801899722 ) ) ;
#85106=CARTESIAN_POINT ( 'NONE',  ( -16.52544592524335698, -4.483927247898792601, 18.95942372801901143 ) ) ;
#85107=CARTESIAN_POINT ( 'NONE',  ( -5.049401038298153566, 19.05341960407611168, 35.20724293864768839 ) ) ;
#85108=CARTESIAN_POINT ( 'NONE',  ( 19.05341960407611168, 5.049401038298154454, 48.95724293864768129 ) ) ;
#85109=CARTESIAN_POINT ( 'NONE',  ( 5.719274019375991003, -21.55341960407610458, 67.70724293864769550 ) ) ;
#85110=CARTESIAN_POINT ( 'NONE',  ( -19.03943276465977164, 0.05219959533909376836, 101.2489096053143669 ) ) ;
#85112=EDGE_CURVE ( 'NONE', #190052, #93673, #182636, .T. ) ;
#85113=CARTESIAN_POINT ( 'NONE',  ( 19.05341960407611168, 5.049401038298154454, 38.95724293864767418 ) ) ;
#85115=CARTESIAN_POINT ( 'NONE',  ( 19.05341960407617918, -5.049401038297876454, 81.04275706135231871 ) ) ;
#85116=CARTESIAN_POINT ( 'NONE',  ( 14.29746914071049879, -8.314922557960816363, 63.33224293864770260 ) ) ;
#85117=CARTESIAN_POINT ( 'NONE',  ( -15.80617190586745835, -15.72974639402198527, 46.87390960531435979 ) ) ;
#85118=CARTESIAN_POINT ( 'NONE',  ( -5.719274019375665041, -21.55341960407619695, 109.7927570613523613 ) ) ;
#85119=CARTESIAN_POINT ( 'NONE',  ( -21.52544592524343514, 5.823673210054127303, 101.0405762719810383 ) ) ;
#85120=CARTESIAN_POINT ( 'NONE',  ( 5.719274019375673035, 21.55341960407619339, 67.29275706135234714 ) ) ;
#85121=CARTESIAN_POINT ( 'NONE',  ( -0.05219959533937732626, 21.53943276465977519, 82.50109039468568994 ) ) ;
#85122=CARTESIAN_POINT ( 'NONE',  ( -19.02544592524342804, 5.153800228976336051, 116.0405762719810383 ) ) ;
#85123=CARTESIAN_POINT ( 'NONE',  ( -4.379528057220086978, -16.55341960407618274, 104.7927570613523898 ) ) ;
#85124=CARTESIAN_POINT ( 'NONE',  ( -21.53943276465977519, -0.05219959533937600094, 73.75109039468567573 ) ) ;
#85125=CARTESIAN_POINT ( 'NONE',  ( 5.153800228976335163, 19.02544592524342804, 64.79057627198100988 ) ) ;
#85126=CARTESIAN_POINT ( 'NONE',  ( 13.97604488694548053, -13.89961937509957401, 30.62609039468566863 ) ) ;
#85127=CARTESIAN_POINT ( 'NONE',  ( 21.53943276465977519, 0.05219959533937863772, 36.25109039468567573 ) ) ;
#85128=CARTESIAN_POINT ( 'NONE',  ( 16.51473224551069308, 9.474510206698969483, 64.16557627198102409 ) ) ;
#85129=CARTESIAN_POINT ( 'NONE',  ( -4.379528057220328563, 16.55341960407611168, 80.20724293864769550 ) ) ;
#85130=CARTESIAN_POINT ( 'NONE',  ( -8.314922557960811034, -14.29746914071050412, 42.08224293864769550 ) ) ;
#85131=CARTESIAN_POINT ( 'NONE',  ( -15.80617190586745835, -15.72974639402198527, 61.87390960531436690 ) ) ;
#85132=CARTESIAN_POINT ( 'NONE',  ( 13.89961937509977652, -13.97604488694527269, 58.12390960531436690 ) ) ;
#85133=CARTESIAN_POINT ( 'NONE',  ( -21.53943276465977519, 0.05219959533907696930, 76.24890960531435269 ) ) ;
#85134=CARTESIAN_POINT ( 'NONE',  ( 5.153800228976615827, -19.02544592524334988, 70.20942372801899012 ) ) ;
#85136=CARTESIAN_POINT ( 'NONE',  ( 16.55341960407611168, 4.379528057220329451, 68.95724293864769550 ) ) ;
#85137=CARTESIAN_POINT ( 'NONE',  ( -21.55341960407610458, -5.719274019375992779, 41.45724293864769550 ) ) ;
#85140=CARTESIAN_POINT ( 'NONE',  ( -4.379528057220086978, -16.55341960407618274, 84.79275706135234714 ) ) ;
#85142=CARTESIAN_POINT ( 'NONE',  ( 19.03943276465977164, 0.05219959533936151252, 91.25109039468566152 ) ) ;
#85143=CARTESIAN_POINT ( 'NONE',  ( 16.52544592524342804, -4.483927247898539470, 58.54057627198103120 ) ) ;
#85144=CARTESIAN_POINT ( 'NONE',  ( -16.51473224551069308, -9.474510206698971260, 51.66557627198102409 ) ) ;
#85145=CARTESIAN_POINT ( 'NONE',  ( 4.379528057220339221, -16.55341960407611168, 37.70724293864769550 ) ) ;
#85146=CARTESIAN_POINT ( 'NONE',  ( 5.049401038298161559, -19.05341960407611168, 82.70724293864770971 ) ) ;
#85147=CARTESIAN_POINT ( 'NONE',  ( -19.03943276465977164, -0.05219959533935918106, 73.75109039468566152 ) ) ;
#85148=CARTESIAN_POINT ( 'NONE',  ( 5.049401038298161559, -19.05341960407611168, 47.70724293864770260 ) ) ;
#85149=CARTESIAN_POINT ( 'NONE',  ( 10.81492255796106328, -18.62759615963255655, 65.41775706135234714 ) ) ;
#85150=CARTESIAN_POINT ( 'NONE',  ( 0.05219959533909260263, 19.03943276465977164, 69.99890960531435269 ) ) ;
#85151=CARTESIAN_POINT ( 'NONE',  ( 9.564922557960805705, 16.46253265017160317, 29.58224293864769550 ) ) ;
#85152=CARTESIAN_POINT ( 'NONE',  ( -5.049401038298153566, 19.05341960407611168, 75.20724293864769550 ) ) ;
#85153=CARTESIAN_POINT ( 'NONE',  ( -21.55341960407610458, -5.719274019375992779, 51.45724293864770260 ) ) ;
#85154=CARTESIAN_POINT ( 'NONE',  ( 13.89961937509977652, -13.97604488694527269, 43.12390960531434558 ) ) ;
#85155=CARTESIAN_POINT ( 'NONE',  ( -15.72974639402197994, 15.80617190586746368, 60.62390960531437401 ) ) ;
#85156=CARTESIAN_POINT ( 'NONE',  ( -13.97604488694547697, 13.89961937509957934, 83.12609039468564731 ) ) ;
#85157=CARTESIAN_POINT ( 'NONE',  ( 8.314922557961029526, -14.29746914071037800, 105.4177570613523613 ) ) ;
#85158=CARTESIAN_POINT ( 'NONE',  ( -5.049401038297874678, -19.05341960407617918, 39.79275706135232582 ) ) ;
#85159=CARTESIAN_POINT ( 'NONE',  ( -8.224510206698735004, -14.34966873604973081, 54.58442372801901143 ) ) ;
#85160=CARTESIAN_POINT ( 'NONE',  ( 12.06949235617739724, 12.14591786802326823, 81.87609039468568994 ) ) ;
#85161=CARTESIAN_POINT ( 'NONE',  ( -12.06949235617739369, -12.14591786802326823, 69.37609039468567573 ) ) ;
#85162=CARTESIAN_POINT ( 'NONE',  ( -21.55341960407610458, -5.719274019375992779, 21.45724293864769550 ) ) ;
#85163=CARTESIAN_POINT ( 'NONE',  ( -5.049401038298153566, 19.05341960407611168, 35.20724293864768839 ) ) ;
#85164=CARTESIAN_POINT ( 'NONE',  ( 0.05219959533934541429, -16.53943276465976808, 40.00109039468567573 ) ) ;
#85165=CARTESIAN_POINT ( 'NONE',  ( 9.474510206698971260, -16.51473224551069308, 52.91557627198102409 ) ) ;
#85166=CARTESIAN_POINT ( 'NONE',  ( -21.52544592524334988, -5.823673210054445271, 43.95942372801902565 ) ) ;
#85167=CARTESIAN_POINT ( 'NONE',  ( -4.379528057220086978, -16.55341960407618274, 34.79275706135235424 ) ) ;
#85168=CARTESIAN_POINT ( 'NONE',  ( -4.483927247898782831, 16.52544592524335698, 112.7094237280190328 ) ) ;
#85170=CARTESIAN_POINT ( 'NONE',  ( 16.51473224551083163, -9.474510206698727899, 20.83442372801899722 ) ) ;
#85171=CARTESIAN_POINT ( 'NONE',  ( 13.89961937509957401, 13.97604488694547697, 106.8760903946856757 ) ) ;
#85172=CARTESIAN_POINT ( 'NONE',  ( 5.049401038297881783, 19.05341960407617563, 67.29275706135234714 ) ) ;
#85173=CARTESIAN_POINT ( 'NONE',  ( -14.34966873604960291, -8.224510206698953496, 71.66557627198100988 ) ) ;
#85174=CARTESIAN_POINT ( 'NONE',  ( 5.153800228976335163, 19.02544592524342804, 44.79057627198103830 ) ) ;
#85175=CARTESIAN_POINT ( 'NONE',  ( -13.89961937509957401, -13.97604488694547875, 54.37609039468565442 ) ) ;
#85176=DIRECTION ( 'NONE',  ( 0.000000000000000000, 4.336808689942013792E-16, 1.000000000000000000 ) ) ;
#85177=CARTESIAN_POINT ( 'NONE',  ( -10.72451020669870658, -18.67979575497194134, 59.58442372801901854 ) ) ;
#85178=CARTESIAN_POINT ( 'NONE',  ( -16.55341960407617563, 4.379528057220093196, 43.54275706135235424 ) ) ;
#85179=CARTESIAN_POINT ( 'NONE',  ( 18.56453257813361546, -5.500000000000034639, 58.49000423690687711 ) ) ;
#85180=CARTESIAN_POINT ( 'NONE',  ( -10.72451020669898014, 18.67979575497178502, 25.41557627198103120 ) ) ;
#85181=CARTESIAN_POINT ( 'NONE',  ( 16.55341960407618274, -4.379528057220086978, 26.04275706135235779 ) ) ;
#85182=CARTESIAN_POINT ( 'NONE',  ( -9.564922557960796823, -16.46253265017161027, 112.0822429386476955 ) ) ;
#85184=CARTESIAN_POINT ( 'NONE',  ( -16.51473224551069308, -9.474510206698971260, 31.66557627198102054 ) ) ;
#85185=CARTESIAN_POINT ( 'NONE',  ( -15.72974639402176322, -15.80617190586768395, 104.3760903946856899 ) ) ;
#85186=CARTESIAN_POINT ( 'NONE',  ( 5.153800228976335163, 19.02544592524342804, 54.79057627198103120 ) ) ;
#85187=CARTESIAN_POINT ( 'NONE',  ( -5.719274019375665041, -21.55341960407619695, 64.79275706135234714 ) ) ;
#85189=CARTESIAN_POINT ( 'NONE',  ( -5.823673210054431948, 21.52544592524334988, 97.70942372801904696 ) ) ;
#85190=CARTESIAN_POINT ( 'NONE',  ( -8.314922557961024197, 14.29746914071037800, 112.9177570613523329 ) ) ;
#85191=CARTESIAN_POINT ( 'NONE',  ( -19.05341960407611168, -5.049401038298163336, 26.45724293864769550 ) ) ;
#85192=CARTESIAN_POINT ( 'NONE',  ( 19.02544592524343514, -5.153800228976328945, 98.54057627198100988 ) ) ;
#85193=CARTESIAN_POINT ( 'NONE',  ( 21.52544592524334988, 5.823673210054432836, 61.45942372801901854 ) ) ;
#85194=CARTESIAN_POINT ( 'NONE',  ( -19.03943276465977164, 0.05219959533909376836, 41.24890960531435269 ) ) ;
#85195=AXIS2_PLACEMENT_3D ( 'NONE', #143036, #65211, #68194 ) ;
#85196=CARTESIAN_POINT ( 'NONE',  ( 18.62759615963255655, 10.81492255796105972, 51.66775706135234714 ) ) ;
#85197=CARTESIAN_POINT ( 'NONE',  ( 5.153800228976615827, -19.02544592524334988, 85.20942372801900433 ) ) ;
#85198=CARTESIAN_POINT ( 'NONE',  ( 0.05219959533909260263, 19.03943276465977164, 104.9989096053143669 ) ) ;
#85199=CARTESIAN_POINT ( 'NONE',  ( 16.52544592524342804, -4.483927247898539470, 113.5405762719810383 ) ) ;
#85200=CARTESIAN_POINT ( 'NONE',  ( 18.67979575497178502, 10.72451020669898547, 109.1655762719810383 ) ) ;
#85201=CARTESIAN_POINT ( 'NONE',  ( 19.03943276465977164, 0.05219959533936151252, 41.25109039468566152 ) ) ;
#85202=CARTESIAN_POINT ( 'NONE',  ( 4.483927247898545687, 16.52544592524342804, 94.79057627198105251 ) ) ;
#85203=CARTESIAN_POINT ( 'NONE',  ( -5.049401038298153566, 19.05341960407611168, 50.20724293864770260 ) ) ;
#85204=CARTESIAN_POINT ( 'NONE',  ( -9.564922557961040184, 16.46253265017147172, 97.91775706135233293 ) ) ;
#85205=CARTESIAN_POINT ( 'NONE',  ( -16.55341960407611168, -4.379528057220339221, 66.45724293864768129 ) ) ;
#85206=CARTESIAN_POINT ( 'NONE',  ( 0.05219959533937995610, -21.53943276465977519, 105.0010903946856757 ) ) ;
#85207=CARTESIAN_POINT ( 'NONE',  ( -0.05219959533909027116, -19.03943276465977164, 112.4989096053143669 ) ) ;
#85208=CARTESIAN_POINT ( 'NONE',  ( -13.89961937509957401, -13.97604488694547875, 94.37609039468566152 ) ) ;
#85209=CARTESIAN_POINT ( 'NONE',  ( 15.72974639402199770, -15.80617190586745480, 98.12390960531436690 ) ) ;
#85210=CARTESIAN_POINT ( 'NONE',  ( 18.62759615963255655, 10.81492255796105972, 46.66775706135234714 ) ) ;
#85211=CARTESIAN_POINT ( 'NONE',  ( -12.06949235617739369, -12.14591786802326823, 44.37609039468567573 ) ) ;
#85212=CARTESIAN_POINT ( 'NONE',  ( 14.29746914071037800, 8.314922557961029526, 111.6677570613523613 ) ) ;
#85213=CARTESIAN_POINT ( 'NONE',  ( -12.06949235617739369, -12.14591786802326823, 44.37609039468567573 ) ) ;
#85214=CARTESIAN_POINT ( 'NONE',  ( 0.05219959533937995610, -21.53943276465977519, 50.00109039468568994 ) ) ;
#85215=CARTESIAN_POINT ( 'NONE',  ( -5.719274019375978568, 21.55341960407610458, 40.20724293864769550 ) ) ;
#85216=CARTESIAN_POINT ( 'NONE',  ( 9.564922557960805705, 16.46253265017160317, 39.58224293864768839 ) ) ;
#85218=CARTESIAN_POINT ( 'NONE',  ( 12.06949235617739724, 12.14591786802326823, 61.87609039468568284 ) ) ;
#85219=CARTESIAN_POINT ( 'NONE',  ( -21.53943276465977519, 0.05219959533907696930, 86.24890960531436690 ) ) ;
#85220=CARTESIAN_POINT ( 'NONE',  ( 12.14591786802309770, 12.06949235617756955, 44.37390960531435979 ) ) ;
#85221=CARTESIAN_POINT ( 'NONE',  ( -8.314922557961024197, 14.29746914071037800, 62.91775706135236135 ) ) ;
#85222=CARTESIAN_POINT ( 'NONE',  ( 13.89961937509977652, -13.97604488694527269, 53.12390960531434558 ) ) ;
#85223=CARTESIAN_POINT ( 'NONE',  ( -9.564922557961040184, 16.46253265017147172, 102.9177570613523329 ) ) ;
#85224=CARTESIAN_POINT ( 'NONE',  ( -18.67979575497178146, -10.72451020669898902, 91.66557627198103830 ) ) ;
#85225=CARTESIAN_POINT ( 'NONE',  ( -14.34966873604960291, -8.224510206698953496, 36.66557627198103120 ) ) ;
#85227=CARTESIAN_POINT ( 'NONE',  ( 0.05219959533934541429, -16.53943276465976808, 85.00109039468568994 ) ) ;
#85229=CARTESIAN_POINT ( 'NONE',  ( 10.72451020669898902, -18.67979575497178502, 77.91557627198102409 ) ) ;
#85231=CARTESIAN_POINT ( 'NONE',  ( 16.55341960407618274, -4.379528057220086978, 111.0427570613523613 ) ) ;
#85232=ORIENTED_EDGE ( 'NONE', *, *, #53585, .F. ) ;
#85234=CARTESIAN_POINT ( 'NONE',  ( 5.719274019375991003, -21.55341960407610458, 82.70724293864770971 ) ) ;
#85235=CARTESIAN_POINT ( 'NONE',  ( 21.55341960407610458, 5.719274019375980345, 113.9572429386477239 ) ) ;
#85236=CARTESIAN_POINT ( 'NONE',  ( 16.53943276465976808, -0.05219959533910856209, 33.74890960531436690 ) ) ;
#85237=CARTESIAN_POINT ( 'NONE',  ( -16.52544592524335698, -4.483927247898792601, 28.95942372801902209 ) ) ;
#85238=CARTESIAN_POINT ( 'NONE',  ( -19.02544592524342804, 5.153800228976336051, 36.04057627198100988 ) ) ;
#85239=CARTESIAN_POINT ( 'NONE',  ( 0.05219959533909260263, 19.03943276465977164, 64.99890960531436690 ) ) ;
#85241=CARTESIAN_POINT ( 'NONE',  ( 5.049401038298161559, -19.05341960407611168, 112.7072429386476813 ) ) ;
#85243=CARTESIAN_POINT ( 'NONE',  ( 5.153800228976615827, -19.02544592524334988, 100.2094237280190043 ) ) ;
#85244=CARTESIAN_POINT ( 'NONE',  ( -16.51473224551082808, 9.474510206698731452, 43.33442372801900433 ) ) ;
#85245=CARTESIAN_POINT ( 'NONE',  ( 5.719274019375991003, -21.55341960407610458, 87.70724293864769550 ) ) ;
#85246=CARTESIAN_POINT ( 'NONE',  ( -4.379528057220328563, 16.55341960407611168, 25.20724293864769550 ) ) ;
#85247=CARTESIAN_POINT ( 'NONE',  ( -5.719274019375978568, 21.55341960407610458, 50.20724293864769550 ) ) ;
#85248=CARTESIAN_POINT ( 'NONE',  ( 5.823673210054125526, 21.52544592524343514, 79.79057627198102409 ) ) ;
#85249=CARTESIAN_POINT ( 'NONE',  ( 19.03943276465977164, 0.05219959533936151252, 106.2510903946856615 ) ) ;
#85250=CARTESIAN_POINT ( 'NONE',  ( 13.97604488694527802, 13.89961937509977652, 99.37390960531436690 ) ) ;
#85251=CARTESIAN_POINT ( 'NONE',  ( 18.67979575497194134, -10.72451020669871369, 70.83442372801901854 ) ) ;
#85252=CARTESIAN_POINT ( 'NONE',  ( -0.05219959533909027116, -19.03943276465977164, 67.49890960531436690 ) ) ;
#85253=CARTESIAN_POINT ( 'NONE',  ( -4.483927247898539470, -16.52544592524342804, 102.2905762719810383 ) ) ;
#85255=CARTESIAN_POINT ( 'NONE',  ( -16.51473224551069308, -9.474510206698971260, 76.66557627198103830 ) ) ;
#85256=CARTESIAN_POINT ( 'NONE',  ( -12.06949235617756955, 12.14591786802309770, 90.62390960531436690 ) ) ;
#85258=CARTESIAN_POINT ( 'NONE',  ( 0.05219959533936267826, -19.03943276465977164, 105.0010903946856615 ) ) ;
#85261=CARTESIAN_POINT ( 'NONE',  ( 9.564922557960805705, 16.46253265017160317, 54.58224293864769550 ) ) ;
#85262=CARTESIAN_POINT ( 'NONE',  ( 21.52544592524334988, 5.823673210054432836, 81.45942372801900433 ) ) ;
#85263=CARTESIAN_POINT ( 'NONE',  ( -13.89961937509977652, 13.97604488694528158, 100.6239096053143669 ) ) ;
#85264=CARTESIAN_POINT ( 'NONE',  ( -16.53943276465976808, -0.05219959533934237506, 83.75109039468568994 ) ) ;
#85265=CARTESIAN_POINT ( 'NONE',  ( -16.29526858892875651, -7.335722546920120379, 75.79670597800210885 ) ) ;
#85266=CARTESIAN_POINT ( 'NONE',  ( -19.03943276465977164, -0.05219959533935918106, 53.75109039468566863 ) ) ;
#85267=CARTESIAN_POINT ( 'NONE',  ( 15.72974639402176855, 15.80617190586768217, 101.8760903946857042 ) ) ;
#85270=CARTESIAN_POINT ( 'NONE',  ( -16.53943276465976808, 0.05219959533911058130, 26.24890960531435624 ) ) ;
#85272=CARTESIAN_POINT ( 'NONE',  ( -16.55341960407617563, 4.379528057220093196, 88.54275706135236135 ) ) ;
#85274=CARTESIAN_POINT ( 'NONE',  ( 8.224510206698742110, 14.34966873604972548, 67.08442372801901854 ) ) ;
#85275=CARTESIAN_POINT ( 'NONE',  ( 18.67979575497194134, -10.72451020669871369, 80.83442372801901854 ) ) ;
#85276=CARTESIAN_POINT ( 'NONE',  ( -13.97604488694547697, 13.89961937509957934, 88.12609039468563310 ) ) ;
#85277=CARTESIAN_POINT ( 'NONE',  ( 19.03943276465977164, 0.05219959533936151252, 46.25109039468566863 ) ) ;
#85278=CARTESIAN_POINT ( 'NONE',  ( -9.564922557960796823, -16.46253265017161027, 67.08224293864769550 ) ) ;
#85279=CARTESIAN_POINT ( 'NONE',  ( 9.474510206698971260, -16.51473224551069308, 62.91557627198102409 ) ) ;
#85280=CARTESIAN_POINT ( 'NONE',  ( 16.46253265017160672, -9.564922557960803928, 88.33224293864769550 ) ) ;
#85281=CARTESIAN_POINT ( 'NONE',  ( -10.81492255796078084, -18.62759615963271287, 77.08224293864769550 ) ) ;
#85283=CARTESIAN_POINT ( 'NONE',  ( -10.72451020669898014, 18.67979575497178502, 50.41557627198103120 ) ) ;
#85284=CARTESIAN_POINT ( 'NONE',  ( -9.474510206698964154, 16.51473224551069663, 30.41557627198102054 ) ) ;
#85285=CARTESIAN_POINT ( 'NONE',  ( 12.06949235617739724, 12.14591786802326823, 66.87609039468568994 ) ) ;
#85286=EDGE_LOOP ( 'NONE', ( #136633, #155954 ) ) ;
#85287=CARTESIAN_POINT ( 'NONE',  ( 10.81492255796106328, -18.62759615963255655, 35.41775706135234003 ) ) ;
#85288=CARTESIAN_POINT ( 'NONE',  ( 12.14591786802309770, 12.06949235617756955, 69.37390960531436690 ) ) ;
#85290=CARTESIAN_POINT ( 'NONE',  ( 8.314922557961029526, -14.29746914071037800, 25.41775706135235779 ) ) ;
#85291=CARTESIAN_POINT ( 'NONE',  ( 9.474510206698729675, 16.51473224551082808, 57.08442372801900433 ) ) ;
#85292=CARTESIAN_POINT ( 'NONE',  ( -8.224510206698948167, 14.34966873604960824, 55.41557627198102409 ) ) ;
#85293=CARTESIAN_POINT ( 'NONE',  ( -21.52544592524334988, -5.823673210054445271, 33.95942372801901143 ) ) ;
#85295=CARTESIAN_POINT ( 'NONE',  ( -18.67979575497178146, -10.72451020669898902, 76.66557627198103830 ) ) ;
#85296=CARTESIAN_POINT ( 'NONE',  ( -19.05341960407611168, -5.049401038298163336, 101.4572429386476955 ) ) ;
#85297=CARTESIAN_POINT ( 'NONE',  ( -0.05219959533910754901, -16.53943276465976808, 72.49890960531435269 ) ) ;
#85300=CARTESIAN_POINT ( 'NONE',  ( -19.03943276465977164, -0.05219959533935918106, 73.75109039468566152 ) ) ;
#85301=CARTESIAN_POINT ( 'NONE',  ( -21.55341960407619339, 5.719274019375674811, 28.54275706135234358 ) ) ;
#85302=CARTESIAN_POINT ( 'NONE',  ( -5.153800228976328057, -19.02544592524343514, 52.29057627198100988 ) ) ;
#85303=CARTESIAN_POINT ( 'NONE',  ( -16.46253265017146816, -9.564922557961047289, 49.16775706135233293 ) ) ;
#85304=CARTESIAN_POINT ( 'NONE',  ( -19.02544592524342804, 5.153800228976336051, 26.04057627198103120 ) ) ;
#85305=CARTESIAN_POINT ( 'NONE',  ( -10.81492255796105439, 18.62759615963255655, 62.91775706135236135 ) ) ;
#85306=EDGE_CURVE ( 'NONE', #65144, #133811, #57303, .T. ) ;
#85307=CARTESIAN_POINT ( 'NONE',  ( -17.31728774477272736, -6.344390552232369807, 69.18093348310679858 ) ) ;
#85308=CARTESIAN_POINT ( 'NONE',  ( 4.379528057220339221, -16.55341960407611168, 37.70724293864769550 ) ) ;
#85309=CARTESIAN_POINT ( 'NONE',  ( 5.049401038298161559, -19.05341960407611168, 57.70724293864769550 ) ) ;
#85311=CARTESIAN_POINT ( 'NONE',  ( -10.81492255796078084, -18.62759615963271287, 92.08224293864769550 ) ) ;
#85312=CARTESIAN_POINT ( 'NONE',  ( -9.474510206698964154, 16.51473224551069663, 60.41557627198102409 ) ) ;
#85314=CARTESIAN_POINT ( 'NONE',  ( 15.80617190586746368, 15.72974639402197994, 69.37390960531436690 ) ) ;
#85315=CARTESIAN_POINT ( 'NONE',  ( 21.53943276465977519, 0.05219959533937863772, 101.2510903946856757 ) ) ;
#85316=CARTESIAN_POINT ( 'NONE',  ( 0.05219959533909260263, 19.03943276465977164, 24.99890960531435269 ) ) ;
#85317=CARTESIAN_POINT ( 'NONE',  ( 16.55341960407618274, -4.379528057220086978, 96.04275706135236135 ) ) ;
#85318=CARTESIAN_POINT ( 'NONE',  ( 8.314922557960818139, 14.29746914071049879, 79.58224293864769550 ) ) ;
#85319=CARTESIAN_POINT ( 'NONE',  ( -16.46253265017146816, -9.564922557961047289, 94.16775706135233293 ) ) ;
#85320=ORIENTED_EDGE ( 'NONE', *, *, #178569, .T. ) ;
#85321=CARTESIAN_POINT ( 'NONE',  ( -21.53943276465977519, 0.05219959533907696930, 111.2489096053143669 ) ) ;
#85322=CARTESIAN_POINT ( 'NONE',  ( 19.02544592524334988, 5.153800228976608722, 41.45942372801900433 ) ) ;
#85323=CARTESIAN_POINT ( 'NONE',  ( -16.53943276465976808, -0.05219959533934237506, 103.7510903946857042 ) ) ;
#85324=CARTESIAN_POINT ( 'NONE',  ( -13.89961937509957401, -13.97604488694547875, 34.37609039468566863 ) ) ;
#85325=CARTESIAN_POINT ( 'NONE',  ( -5.049401038298153566, 19.05341960407611168, 95.20724293864770971 ) ) ;
#85326=CARTESIAN_POINT ( 'NONE',  ( 10.81492255796078972, 18.62759615963270932, 59.58224293864770260 ) ) ;
#85328=CARTESIAN_POINT ( 'NONE',  ( -9.564922557960796823, -16.46253265017161027, 22.08224293864768839 ) ) ;
#85329=CARTESIAN_POINT ( 'NONE',  ( 5.153800228976615827, -19.02544592524334988, 20.20942372801899722 ) ) ;
#85330=CARTESIAN_POINT ( 'NONE',  ( -0.05219959533934338120, 16.53943276465976808, 82.50109039468568994 ) ) ;
#85331=CARTESIAN_POINT ( 'NONE',  ( 18.62759615963255655, 10.81492255796105972, 26.66775706135235424 ) ) ;
#85332=CARTESIAN_POINT ( 'NONE',  ( 12.06949235617739724, 12.14591786802326823, 26.87609039468567218 ) ) ;
#85333=CARTESIAN_POINT ( 'NONE',  ( 5.153800228976335163, 19.02544592524342804, 99.79057627198102409 ) ) ;
#85334=CARTESIAN_POINT ( 'NONE',  ( 19.03943276465977164, -0.05219959533909143690, 43.74890960531435979 ) ) ;
#85335=CARTESIAN_POINT ( 'NONE',  ( 19.05341960407611168, 5.049401038298154454, 63.95724293864769550 ) ) ;
#85336=CARTESIAN_POINT ( 'NONE',  ( 14.34966873604972726, -8.224510206698740333, 45.83442372801901854 ) ) ;
#85337=CARTESIAN_POINT ( 'NONE',  ( 12.14591786802309770, 12.06949235617756955, 94.37390960531436690 ) ) ;
#85338=CARTESIAN_POINT ( 'NONE',  ( 8.314922557961029526, -14.29746914071037800, 95.41775706135234714 ) ) ;
#85339=CARTESIAN_POINT ( 'NONE',  ( 0.05219959533937995610, -21.53943276465977519, 40.00109039468567573 ) ) ;
#85340=CARTESIAN_POINT ( 'NONE',  ( 9.474510206698971260, -16.51473224551069308, 72.91557627198102409 ) ) ;
#85341=CARTESIAN_POINT ( 'NONE',  ( -5.049401038298153566, 19.05341960407611168, 70.20724293864769550 ) ) ;
#85342=CARTESIAN_POINT ( 'NONE',  ( -19.03943276465977164, 0.05219959533909376836, 96.24890960531436690 ) ) ;
#85343=CARTESIAN_POINT ( 'NONE',  ( 0.05219959533910956823, 16.53943276465976808, 34.99890960531435979 ) ) ;
#85344=CARTESIAN_POINT ( 'NONE',  ( -8.314922557961024197, 14.29746914071037800, 92.91775706135236135 ) ) ;
#85346=CARTESIAN_POINT ( 'NONE',  ( -9.474510206698720793, -16.51473224551083518, 39.58442372801899722 ) ) ;
#85347=CARTESIAN_POINT ( 'NONE',  ( 5.153800228976335163, 19.02544592524342804, 109.7905762719810099 ) ) ;
#85348=CARTESIAN_POINT ( 'NONE',  ( -19.02544592524342804, 5.153800228976336051, 66.04057627198103830 ) ) ;
#85349=CARTESIAN_POINT ( 'NONE',  ( 13.97604488694548053, -13.89961937509957401, 40.62609039468564731 ) ) ;
#85351=CARTESIAN_POINT ( 'NONE',  ( 19.49149378614663064, -5.499999999999580780, 71.93757513605363840 ) ) ;
#85352=CARTESIAN_POINT ( 'NONE',  ( -14.34966873604972548, 8.224510206698743886, 58.33442372801901143 ) ) ;
#85353=CARTESIAN_POINT ( 'NONE',  ( -0.05219959533936034679, 19.03943276465977164, 67.50109039468566152 ) ) ;
#85354=CARTESIAN_POINT ( 'NONE',  ( -14.29746914071037622, -8.314922557961029526, 54.16775706135235424 ) ) ;
#85356=CARTESIAN_POINT ( 'NONE',  ( -0.05219959533909027116, -19.03943276465977164, 87.49890960531436690 ) ) ;
#85357=CARTESIAN_POINT ( 'NONE',  ( -15.72974639402176322, -15.80617190586768395, 19.37609039468568639 ) ) ;
#85358=CARTESIAN_POINT ( 'NONE',  ( 13.89961937509957401, 13.97604488694547697, 81.87609039468564731 ) ) ;
#85359=CARTESIAN_POINT ( 'NONE',  ( -16.51473224551069308, -9.474510206698971260, 111.6655762719810383 ) ) ;
#85360=CARTESIAN_POINT ( 'NONE',  ( -5.049401038298153566, 19.05341960407611168, 30.20724293864768839 ) ) ;
#85362=CARTESIAN_POINT ( 'NONE',  ( -5.049401038298153566, 19.05341960407611168, 80.20724293864769550 ) ) ;
#85363=CARTESIAN_POINT ( 'NONE',  ( 8.314922557960818139, 14.29746914071049879, 54.58224293864769550 ) ) ;
#85364=CARTESIAN_POINT ( 'NONE',  ( 9.474510206698971260, -16.51473224551069308, 32.91557627198102409 ) ) ;
#85365=CARTESIAN_POINT ( 'NONE',  ( 16.46253265017146816, 9.564922557961045513, 51.66775706135233293 ) ) ;
#85366=CARTESIAN_POINT ( 'NONE',  ( -16.53943276465976808, 0.05219959533911058130, 91.24890960531436690 ) ) ;
#85367=CARTESIAN_POINT ( 'NONE',  ( -16.46253265017146816, -9.564922557961047289, 19.16775706135233293 ) ) ;
#85368=CARTESIAN_POINT ( 'NONE',  ( 0.05219959533909260263, 19.03943276465977164, 49.99890960531435979 ) ) ;
#85370=CARTESIAN_POINT ( 'NONE',  ( -10.81492255796078084, -18.62759615963271287, 47.08224293864770260 ) ) ;
#85371=CARTESIAN_POINT ( 'NONE',  ( 4.379528057220339221, -16.55341960407611168, 47.70724293864770260 ) ) ;
#85372=CARTESIAN_POINT ( 'NONE',  ( 13.89961937509957401, 13.97604488694547697, 21.87609039468566152 ) ) ;
#85373=CARTESIAN_POINT ( 'NONE',  ( -0.05219959533909027116, -19.03943276465977164, 107.4989096053143527 ) ) ;
#85374=CARTESIAN_POINT ( 'NONE',  ( 19.02544592524343514, -5.153800228976328945, 103.5405762719809957 ) ) ;
#85375=CARTESIAN_POINT ( 'NONE',  ( -19.02544592524342804, 5.153800228976336051, 36.04057627198100988 ) ) ;
#85376=CARTESIAN_POINT ( 'NONE',  ( -14.29746914071049879, 8.314922557960819915, 115.8322429386477097 ) ) ;
#85377=CARTESIAN_POINT ( 'NONE',  ( -14.29746914071049879, 8.314922557960819915, 90.83224293864769550 ) ) ;
#85378=CARTESIAN_POINT ( 'NONE',  ( 21.55341960407610458, 5.719274019375980345, 98.95724293864770971 ) ) ;
#85379=CARTESIAN_POINT ( 'NONE',  ( -19.02544592524342804, 5.153800228976336051, 101.0405762719810241 ) ) ;
#85380=CARTESIAN_POINT ( 'NONE',  ( -18.62759615963270932, 10.81492255796079327, 115.8322429386477097 ) ) ;
#85381=CARTESIAN_POINT ( 'NONE',  ( 5.153800228976335163, 19.02544592524342804, 99.79057627198102409 ) ) ;
#85383=CARTESIAN_POINT ( 'NONE',  ( -12.14591786802309592, -12.06949235617757132, 101.8739096053143811 ) ) ;
#85384=CARTESIAN_POINT ( 'NONE',  ( -5.049401038298153566, 19.05341960407611168, 65.20724293864765286 ) ) ;
#85385=CARTESIAN_POINT ( 'NONE',  ( -5.719274019375978568, 21.55341960407610458, 85.20724293864770971 ) ) ;
#85386=CARTESIAN_POINT ( 'NONE',  ( 17.48853670773245028, -5.747243402303111814, 106.1667129974999142 ) ) ;
#85388=CARTESIAN_POINT ( 'NONE',  ( -15.80617190586745835, -15.72974639402198527, 31.87390960531435979 ) ) ;
#85389=CARTESIAN_POINT ( 'NONE',  ( 18.87075004821571511, -5.499999999999891642, 66.17408112101047379 ) ) ;
#85390=CARTESIAN_POINT ( 'NONE',  ( 8.224510206698742110, 14.34966873604972548, 27.08442372801901854 ) ) ;
#85391=CARTESIAN_POINT ( 'NONE',  ( -16.52544592524342804, 4.483927247898546575, 106.0405762719810525 ) ) ;
#85393=CARTESIAN_POINT ( 'NONE',  ( -17.50000000000002132, -4.658240926743155264, 111.0552958218319901 ) ) ;
#85394=CARTESIAN_POINT ( 'NONE',  ( -0.05219959533909027116, -19.03943276465977164, 62.49890960531435979 ) ) ;
#85395=CARTESIAN_POINT ( 'NONE',  ( -4.483927247898539470, -16.52544592524342804, 82.29057627198103830 ) ) ;
#85396=CARTESIAN_POINT ( 'NONE',  ( 10.81492255796078972, 18.62759615963270932, 29.58224293864769905 ) ) ;
#85397=CARTESIAN_POINT ( 'NONE',  ( -8.224510206698948167, 14.34966873604960824, 65.41557627198102409 ) ) ;
#85398=CARTESIAN_POINT ( 'NONE',  ( -12.06949235617739369, -12.14591786802326823, 19.37609039468568639 ) ) ;
#85399=CARTESIAN_POINT ( 'NONE',  ( 21.52544592524334988, 5.823673210054432836, 76.45942372801901854 ) ) ;
#85401=CARTESIAN_POINT ( 'NONE',  ( 16.88567814943163015, -6.947325034625693618, 76.20998877347416567 ) ) ;
#85402=CARTESIAN_POINT ( 'NONE',  ( -19.05341960407611168, -5.049401038298163336, 106.4572429386476955 ) ) ;
#85403=CARTESIAN_POINT ( 'NONE',  ( -16.53943276465976808, -0.05219959533934237506, 88.75109039468567573 ) ) ;
#85404=CARTESIAN_POINT ( 'NONE',  ( 0.05219959533909260263, 19.03943276465977164, 44.99890960531435979 ) ) ;
#85405=CARTESIAN_POINT ( 'NONE',  ( 19.05341960407611168, 5.049401038298154454, 93.95724293864769550 ) ) ;
#85406=CARTESIAN_POINT ( 'NONE',  ( 5.719274019375991003, -21.55341960407610458, 92.70724293864770971 ) ) ;
#85407=CARTESIAN_POINT ( 'NONE',  ( -8.314922557961024197, 14.29746914071037800, 22.91775706135235069 ) ) ;
#85408=CARTESIAN_POINT ( 'NONE',  ( -8.224510206698948167, 14.34966873604960824, 45.41557627198103830 ) ) ;
#85409=CARTESIAN_POINT ( 'NONE',  ( 21.53943276465977519, 0.05219959533937863772, 66.25109039468567573 ) ) ;
#85410=CARTESIAN_POINT ( 'NONE',  ( -14.29746914071037622, -8.314922557961029526, 99.16775706135234714 ) ) ;
#85412=CARTESIAN_POINT ( 'NONE',  ( -17.40805194822031154, 6.112264579159342404, 80.83371272510612471 ) ) ;
#85413=CARTESIAN_POINT ( 'NONE',  ( 14.34966873604960469, 8.224510206698951720, 34.16557627198102409 ) ) ;
#85414=CARTESIAN_POINT ( 'NONE',  ( -14.29746914071037622, -8.314922557961029526, 59.16775706135234714 ) ) ;
#85415=CARTESIAN_POINT ( 'NONE',  ( 9.474510206698971260, -16.51473224551069308, 67.91557627198102409 ) ) ;
#85417=CARTESIAN_POINT ( 'NONE',  ( -9.474510206698964154, 16.51473224551069663, 85.41557627198102409 ) ) ;
#85418=CARTESIAN_POINT ( 'NONE',  ( -10.81492255796105439, 18.62759615963255655, 67.91775706135234714 ) ) ;
#85419=CARTESIAN_POINT ( 'NONE',  ( 14.29746914071037800, 8.314922557961029526, 71.66775706135234714 ) ) ;
#85420=CARTESIAN_POINT ( 'NONE',  ( 14.34966873604960469, 8.224510206698951720, 64.16557627198102409 ) ) ;
#85421=CARTESIAN_POINT ( 'NONE',  ( -5.153800228976328057, -19.02544592524343514, 67.29057627198102409 ) ) ;
#85423=CARTESIAN_POINT ( 'NONE',  ( -0.05219959533936034679, 19.03943276465977164, 107.5010903946856615 ) ) ;
#85424=CARTESIAN_POINT ( 'NONE',  ( 4.379528057220339221, -16.55341960407611168, 112.7072429386476955 ) ) ;
#85425=CARTESIAN_POINT ( 'NONE',  ( 16.46253265017160672, -9.564922557960803928, 83.33224293864768129 ) ) ;
#85426=CARTESIAN_POINT ( 'NONE',  ( -8.224510206698735004, -14.34966873604973081, 24.58442372801901499 ) ) ;
#85428=CARTESIAN_POINT ( 'NONE',  ( -21.52544592524334988, -5.823673210054445271, 103.9594237280190185 ) ) ;
#85429=CARTESIAN_POINT ( 'NONE',  ( -16.53943276465976808, -0.05219959533934237506, 83.75109039468568994 ) ) ;
#85430=CARTESIAN_POINT ( 'NONE',  ( 9.564922557961047289, -16.46253265017146816, 95.41775706135233293 ) ) ;
#85431=CARTESIAN_POINT ( 'NONE',  ( 16.53943276465976808, -0.05219959533910856209, 108.7489096053143669 ) ) ;
#85432=CARTESIAN_POINT ( 'NONE',  ( 16.53943276465976808, 0.05219959533934440121, 66.25109039468567573 ) ) ;
#85434=CARTESIAN_POINT ( 'NONE',  ( 19.02544592524334988, 5.153800228976608722, 56.45942372801898301 ) ) ;
#85435=CARTESIAN_POINT ( 'NONE',  ( -10.72451020669870658, -18.67979575497194134, 94.58442372801901854 ) ) ;
#85436=CARTESIAN_POINT ( 'NONE',  ( 19.03943276465977164, -0.05219959533909143690, 33.74890960531435979 ) ) ;
#85437=CARTESIAN_POINT ( 'NONE',  ( 9.564922557960805705, 16.46253265017160317, 79.58224293864769550 ) ) ;
#85438=CARTESIAN_POINT ( 'NONE',  ( 8.224510206698953496, -14.34966873604960469, 72.91557627198103830 ) ) ;
#85439=CARTESIAN_POINT ( 'NONE',  ( 0.05219959533937995610, -21.53943276465977519, 90.00109039468567573 ) ) ;
#85441=CARTESIAN_POINT ( 'NONE',  ( 19.03943276465977164, 0.05219959533936151252, 41.25109039468566152 ) ) ;
#85442=CARTESIAN_POINT ( 'NONE',  ( -9.564922557961040184, 16.46253265017147172, 42.91775706135234003 ) ) ;
#85443=CARTESIAN_POINT ( 'NONE',  ( 15.72974639402199770, -15.80617190586745480, 38.12390960531436690 ) ) ;
#85444=CARTESIAN_POINT ( 'NONE',  ( 18.62759615963255655, 10.81492255796105972, 91.66775706135234714 ) ) ;
#85445=CARTESIAN_POINT ( 'NONE',  ( 13.89961937509977652, -13.97604488694527269, 83.12390960531436690 ) ) ;
#85446=CARTESIAN_POINT ( 'NONE',  ( -18.67979575497193778, 10.72451020669871902, 93.33442372801901854 ) ) ;
#85447=CARTESIAN_POINT ( 'NONE',  ( 10.81492255796078972, 18.62759615963270932, 44.58224293864769550 ) ) ;
#85448=CARTESIAN_POINT ( 'NONE',  ( 5.049401038298161559, -19.05341960407611168, 87.70724293864769550 ) ) ;
#85449=CARTESIAN_POINT ( 'NONE',  ( 19.03943276465977164, 0.05219959533936151252, 76.25109039468566152 ) ) ;
#85450=CARTESIAN_POINT ( 'NONE',  ( -9.474510206698964154, 16.51473224551069663, 95.41557627198102409 ) ) ;
#85451=CARTESIAN_POINT ( 'NONE',  ( -13.97604488694547697, 13.89961937509957934, 93.12609039468566152 ) ) ;
#85452=CARTESIAN_POINT ( 'NONE',  ( 8.224510206698742110, 14.34966873604972548, 37.08442372801901143 ) ) ;
#85453=CARTESIAN_POINT ( 'NONE',  ( -4.483927247898539470, -16.52544592524342804, 107.2905762719810525 ) ) ;
#85454=CARTESIAN_POINT ( 'NONE',  ( -19.02544592524342804, 5.153800228976336051, 76.04057627198102409 ) ) ;
#85456=CARTESIAN_POINT ( 'NONE',  ( -21.55341960407610458, -5.719274019375992779, 66.45724293864768129 ) ) ;
#85457=CARTESIAN_POINT ( 'NONE',  ( 4.379528057220092307, 16.55341960407617563, 32.29275706135235424 ) ) ;
#85458=CARTESIAN_POINT ( 'NONE',  ( 21.52544592524334988, 5.823673210054432836, 36.45942372801901143 ) ) ;
#85459=CARTESIAN_POINT ( 'NONE',  ( -21.52544592524334988, -5.823673210054445271, 78.95942372801901854 ) ) ;
#85460=CARTESIAN_POINT ( 'NONE',  ( 14.29746914071037800, 8.314922557961029526, 86.66775706135234714 ) ) ;
#85461=CARTESIAN_POINT ( 'NONE',  ( 19.03943276465977164, -0.05219959533909143690, 68.74890960531436690 ) ) ;
#85462=CARTESIAN_POINT ( 'NONE',  ( -8.224510206698948167, 14.34966873604960824, 80.41557627198103830 ) ) ;
#85463=CARTESIAN_POINT ( 'NONE',  ( 14.34966873604972726, -8.224510206698740333, 100.8344237280190185 ) ) ;
#85464=CARTESIAN_POINT ( 'NONE',  ( -5.049401038297874678, -19.05341960407617918, 49.79275706135231871 ) ) ;
#85465=CARTESIAN_POINT ( 'NONE',  ( -5.823673210054431948, 21.52544592524334988, 27.70942372801901854 ) ) ;
#85466=CARTESIAN_POINT ( 'NONE',  ( 12.14591786802309770, 12.06949235617756955, 74.37390960531436690 ) ) ;
#85467=CARTESIAN_POINT ( 'NONE',  ( 13.89961937509977652, -13.97604488694527269, 103.1239096053143527 ) ) ;
#85468=CARTESIAN_POINT ( 'NONE',  ( -16.55341960407617563, 4.379528057220093196, 98.54275706135234714 ) ) ;
#85469=CARTESIAN_POINT ( 'NONE',  ( 0.05219959533937995610, -21.53943276465977519, 75.00109039468568994 ) ) ;
#85470=CARTESIAN_POINT ( 'NONE',  ( 12.14591786802327356, -12.06949235617739191, 50.62609039468568994 ) ) ;
#85471=CARTESIAN_POINT ( 'NONE',  ( 21.53943276465977519, 0.05219959533937863772, 46.25109039468567573 ) ) ;
#85472=CARTESIAN_POINT ( 'NONE',  ( 16.55341960407611168, 4.379528057220329451, 73.95724293864769550 ) ) ;
#85473=ORIENTED_EDGE ( 'NONE', *, *, #140308, .F. ) ;
#85474=CARTESIAN_POINT ( 'NONE',  ( 21.55341960407619695, -5.719274019375665929, 21.04275706135234714 ) ) ;
#85475=CARTESIAN_POINT ( 'NONE',  ( 17.49999999999996803, -3.805241302050390573, 27.87352472782592017 ) ) ;
#85476=CARTESIAN_POINT ( 'NONE',  ( -4.483927247898539470, -16.52544592524342804, 47.29057627198103120 ) ) ;
#85477=CARTESIAN_POINT ( 'NONE',  ( 5.153800228976335163, 19.02544592524342804, 24.79057627198102765 ) ) ;
#85478=CARTESIAN_POINT ( 'NONE',  ( 15.80617190586746368, 15.72974639402197994, 39.37390960531436690 ) ) ;
#85479=CARTESIAN_POINT ( 'NONE',  ( -4.379528057220328563, 16.55341960407611168, 75.20724293864769550 ) ) ;
#85480=CARTESIAN_POINT ( 'NONE',  ( 0.05219959533907565091, 21.53943276465977519, 84.99890960531436690 ) ) ;
#85481=CARTESIAN_POINT ( 'NONE',  ( -9.474510206698964154, 16.51473224551069663, 90.41557627198103830 ) ) ;
#85482=CARTESIAN_POINT ( 'NONE',  ( 9.564922557960805705, 16.46253265017160317, 34.58224293864770260 ) ) ;
#85483=CARTESIAN_POINT ( 'NONE',  ( -13.89961937509957401, -13.97604488694547875, 74.37609039468566152 ) ) ;
#85484=CARTESIAN_POINT ( 'NONE',  ( 5.823673210054444382, -21.52544592524334988, 55.20942372801902565 ) ) ;
#85485=CARTESIAN_POINT ( 'NONE',  ( -0.05219959533907301413, -21.53943276465977519, 67.49890960531436690 ) ) ;
#85486=CARTESIAN_POINT ( 'NONE',  ( 19.03943276465977164, -0.05219959533909143690, 33.74890960531435979 ) ) ;
#85487=CARTESIAN_POINT ( 'NONE',  ( 19.03943276465977164, -0.05219959533909143690, 68.74890960531436690 ) ) ;
#85489=CARTESIAN_POINT ( 'NONE',  ( -14.29746914071037622, -8.314922557961029526, 54.16775706135235424 ) ) ;
#85490=CARTESIAN_POINT ( 'NONE',  ( 18.62759615963255655, 10.81492255796105972, 26.66775706135235424 ) ) ;
#85492=CARTESIAN_POINT ( 'NONE',  ( 18.62759615963255655, 10.81492255796105972, 61.66775706135235424 ) ) ;
#85493=CARTESIAN_POINT ( 'NONE',  ( -5.049401038298153566, 19.05341960407611168, 110.2072429386476671 ) ) ;
#85494=CARTESIAN_POINT ( 'NONE',  ( -5.823673210054116645, -21.52544592524344225, 92.29057627198103830 ) ) ;
#85495=CARTESIAN_POINT ( 'NONE',  ( -15.72974639402176322, -15.80617190586768395, 24.37609039468567573 ) ) ;
#85496=CARTESIAN_POINT ( 'NONE',  ( 16.55341960407618274, -4.379528057220086978, 46.04275706135234714 ) ) ;
#85497=CARTESIAN_POINT ( 'NONE',  ( 21.53943276465977519, -0.05219959533907433946, 53.74890960531437401 ) ) ;
#85498=CARTESIAN_POINT ( 'NONE',  ( 0.05219959533936267826, -19.03943276465977164, 25.00109039468566152 ) ) ;
#85499=CARTESIAN_POINT ( 'NONE',  ( -13.89961937509977652, 13.97604488694528158, 55.62390960531434558 ) ) ;
#85500=CARTESIAN_POINT ( 'NONE',  ( 13.89961937509977652, -13.97604488694527269, 88.12390960531438111 ) ) ;
#85503=CARTESIAN_POINT ( 'NONE',  ( 9.564922557961047289, -16.46253265017146816, 65.41775706135233293 ) ) ;
#85504=CARTESIAN_POINT ( 'NONE',  ( 10.81492255796078972, 18.62759615963270932, 39.58224293864769550 ) ) ;
#85505=CARTESIAN_POINT ( 'NONE',  ( -16.53943276465976808, 0.05219959533911058130, 21.24890960531436690 ) ) ;
#85506=CARTESIAN_POINT ( 'NONE',  ( 9.474510206698729675, 16.51473224551082808, 97.08442372801900433 ) ) ;
#85509=CARTESIAN_POINT ( 'NONE',  ( -21.53943276465977519, -0.05219959533937600094, 113.7510903946856757 ) ) ;
#85510=CARTESIAN_POINT ( 'NONE',  ( -13.89961937509957401, -13.97604488694547875, 94.37609039468566152 ) ) ;
#85511=CARTESIAN_POINT ( 'NONE',  ( -13.97604488694547697, 13.89961937509957934, 43.12609039468566152 ) ) ;
#85512=CARTESIAN_POINT ( 'NONE',  ( 16.29526858892874941, 7.335722546920133702, 108.2967059780021231 ) ) ;
#85513=CARTESIAN_POINT ( 'NONE',  ( 0.05219959533909260263, 19.03943276465977164, 59.99890960531436690 ) ) ;
#85514=CARTESIAN_POINT ( 'NONE',  ( 16.55341960407611168, 4.379528057220329451, 58.95724293864770971 ) ) ;
#85515=CARTESIAN_POINT ( 'NONE',  ( -19.03943276465977164, 0.05219959533909376836, 31.24890960531435979 ) ) ;
#85516=CARTESIAN_POINT ( 'NONE',  ( 14.29746914071049879, -8.314922557960816363, 43.33224293864769550 ) ) ;
#85518=CARTESIAN_POINT ( 'NONE',  ( -16.55341960407611168, -4.379528057220339221, 21.45724293864769550 ) ) ;
#85519=CARTESIAN_POINT ( 'NONE',  ( 5.153800228976335163, 19.02544592524342804, 59.79057627198100988 ) ) ;
#85520=CARTESIAN_POINT ( 'NONE',  ( 0.05219959533936267826, -19.03943276465977164, 25.00109039468566152 ) ) ;
#85521=CARTESIAN_POINT ( 'NONE',  ( -4.379528057220086978, -16.55341960407618274, 34.79275706135235424 ) ) ;
#85522=CARTESIAN_POINT ( 'NONE',  ( -5.823673210054116645, -21.52544592524344225, 57.29057627198103120 ) ) ;
#85523=CARTESIAN_POINT ( 'NONE',  ( -18.62759615963255300, -10.81492255796106328, 104.1677570613523471 ) ) ;
#85525=CARTESIAN_POINT ( 'NONE',  ( 16.46253265017160672, -9.564922557960803928, 58.33224293864769550 ) ) ;
#85526=CARTESIAN_POINT ( 'NONE',  ( 19.03943276465977164, -0.05219959533909143690, 108.7489096053143527 ) ) ;
#85527=CARTESIAN_POINT ( 'NONE',  ( 16.46253265017160672, -9.564922557960803928, 103.3322429386476955 ) ) ;
#85529=CARTESIAN_POINT ( 'NONE',  ( 21.52544592524334988, 5.823673210054432836, 21.45942372801901499 ) ) ;
#85531=CARTESIAN_POINT ( 'NONE',  ( -4.379528057220328563, 16.55341960407611168, 90.20724293864770971 ) ) ;
#85532=CARTESIAN_POINT ( 'NONE',  ( -21.52544592524343514, 5.823673210054127303, 91.04057627198103830 ) ) ;
#85533=CARTESIAN_POINT ( 'NONE',  ( 13.89961937509977652, -13.97604488694527269, 63.12390960531435979 ) ) ;
#85534=CARTESIAN_POINT ( 'NONE',  ( -13.97604488694527625, -13.89961937509977652, 71.87390960531433848 ) ) ;
#85535=CARTESIAN_POINT ( 'NONE',  ( 15.80617190586746368, 15.72974639402197994, 109.3739096053143811 ) ) ;
#85537=CARTESIAN_POINT ( 'NONE',  ( 0.05219959533909260263, 19.03943276465977164, 69.99890960531435269 ) ) ;
#85540=CARTESIAN_POINT ( 'NONE',  ( 8.314922557960818139, 14.29746914071049879, 99.58224293864770971 ) ) ;
#85541=CARTESIAN_POINT ( 'NONE',  ( -9.564922557960796823, -16.46253265017161027, 22.08224293864768839 ) ) ;
#85542=CARTESIAN_POINT ( 'NONE',  ( -16.46253265017146816, -9.564922557961047289, 94.16775706135233293 ) ) ;
#85544=CARTESIAN_POINT ( 'NONE',  ( 12.14591786802309770, 12.06949235617756955, 99.37390960531436690 ) ) ;
#85545=CARTESIAN_POINT ( 'NONE',  ( 5.823673210054444382, -21.52544592524334988, 70.20942372801904696 ) ) ;
#85546=CARTESIAN_POINT ( 'NONE',  ( 19.05341960407611168, 5.049401038298154454, 68.95724293864769550 ) ) ;
#85547=CARTESIAN_POINT ( 'NONE',  ( 10.81492255796106328, -18.62759615963255655, 35.41775706135234003 ) ) ;
#85548=CARTESIAN_POINT ( 'NONE',  ( -18.62759615963255300, -10.81492255796106328, 19.16775706135234714 ) ) ;
#85549=CARTESIAN_POINT ( 'NONE',  ( -9.564922557960796823, -16.46253265017161027, 67.08224293864769550 ) ) ;
#85550=AXIS2_PLACEMENT_3D ( 'NONE', #46507, #136529, #124332 ) ;
#85552=CARTESIAN_POINT ( 'NONE',  ( 19.03943276465977164, 0.05219959533936151252, 111.2510903946856757 ) ) ;
#85553=CARTESIAN_POINT ( 'NONE',  ( 15.72974639402199770, -15.80617190586745480, 33.12390960531435979 ) ) ;
#85554=CARTESIAN_POINT ( 'NONE',  ( -18.62759615963255300, -10.81492255796106328, 59.16775706135234714 ) ) ;
#85556=CARTESIAN_POINT ( 'NONE',  ( -9.564922557960796823, -16.46253265017161027, 92.08224293864769550 ) ) ;
#85557=CARTESIAN_POINT ( 'NONE',  ( -9.564922557961040184, 16.46253265017147172, 87.91775706135233293 ) ) ;
#85558=CARTESIAN_POINT ( 'NONE',  ( 19.02544592524343514, -5.153800228976328945, 48.54057627198103120 ) ) ;
#85559=CARTESIAN_POINT ( 'NONE',  ( -5.049401038298153566, 19.05341960407611168, 75.20724293864769550 ) ) ;
#85560=CARTESIAN_POINT ( 'NONE',  ( -12.06949235617756955, 12.14591786802309770, 90.62390960531436690 ) ) ;
#85561=CARTESIAN_POINT ( 'NONE',  ( -19.03943276465977164, 0.05219959533909376836, 106.2489096053143669 ) ) ;
#85562=CARTESIAN_POINT ( 'NONE',  ( -0.05219959533910754901, -16.53943276465976808, 87.49890960531436690 ) ) ;
#85563=CARTESIAN_POINT ( 'NONE',  ( -5.153800228976328057, -19.02544592524343514, 97.29057627198099567 ) ) ;
#85564=CARTESIAN_POINT ( 'NONE',  ( 14.29746914071049879, -8.314922557960816363, 38.33224293864768839 ) ) ;
#85565=CARTESIAN_POINT ( 'NONE',  ( 9.564922557960805705, 16.46253265017160317, 29.58224293864769550 ) ) ;
#85567=CARTESIAN_POINT ( 'NONE',  ( 21.53943276465977519, 0.05219959533937863772, 61.25109039468567573 ) ) ;
#85568=CARTESIAN_POINT ( 'NONE',  ( -16.46253265017146816, -9.564922557961047289, 79.16775706135234714 ) ) ;
#85569=CARTESIAN_POINT ( 'NONE',  ( 12.14591786802309770, 12.06949235617756955, 54.37390960531435979 ) ) ;
#85570=CARTESIAN_POINT ( 'NONE',  ( 0.05219959533907565091, 21.53943276465977519, 104.9989096053143669 ) ) ;
#85571=CARTESIAN_POINT ( 'NONE',  ( 10.81492255796078972, 18.62759615963270932, 34.58224293864770260 ) ) ;
#85572=CARTESIAN_POINT ( 'NONE',  ( -8.314922557960811034, -14.29746914071050412, 77.08224293864769550 ) ) ;
#85573=CARTESIAN_POINT ( 'NONE',  ( -16.51473224551069308, -9.474510206698971260, 61.66557627198103120 ) ) ;
#85574=CARTESIAN_POINT ( 'NONE',  ( 4.483927247898545687, 16.52544592524342804, 24.79057627198103120 ) ) ;
#85576=CARTESIAN_POINT ( 'NONE',  ( -4.379528057220086978, -16.55341960407618274, 104.7927570613523898 ) ) ;
#85577=CARTESIAN_POINT ( 'NONE',  ( 14.29746914071037800, 8.314922557961029526, 76.66775706135234714 ) ) ;
#85578=CARTESIAN_POINT ( 'NONE',  ( 13.97604488694548053, -13.89961937509957401, 30.62609039468566863 ) ) ;
#85579=CARTESIAN_POINT ( 'NONE',  ( -16.46253265017160317, 9.564922557960807481, 105.8322429386476955 ) ) ;
#85580=CARTESIAN_POINT ( 'NONE',  ( 16.51473224551069308, 9.474510206698969483, 79.16557627198103830 ) ) ;
#85581=CARTESIAN_POINT ( 'NONE',  ( -19.05341960407611168, -5.049401038298163336, 36.45724293864766707 ) ) ;
#85582=CARTESIAN_POINT ( 'NONE',  ( 16.52544592524342804, -4.483927247898539470, 53.54057627198103120 ) ) ;
#85584=CARTESIAN_POINT ( 'NONE',  ( -5.153800228976328057, -19.02544592524343514, 102.2905762719810383 ) ) ;
#85585=CARTESIAN_POINT ( 'NONE',  ( 0.05219959533907565091, 21.53943276465977519, 44.99890960531435979 ) ) ;
#85586=CARTESIAN_POINT ( 'NONE',  ( -12.14591786802309592, -12.06949235617757132, 91.87390960531436690 ) ) ;
#85587=CARTESIAN_POINT ( 'NONE',  ( 12.14591786802327356, -12.06949235617739191, 30.62609039468567929 ) ) ;
#85588=CARTESIAN_POINT ( 'NONE',  ( -16.55341960407611168, -4.379528057220339221, 66.45724293864768129 ) ) ;
#85590=CARTESIAN_POINT ( 'NONE',  ( -5.153800228976607833, 19.02544592524334988, 67.70942372801900433 ) ) ;
#85591=CARTESIAN_POINT ( 'NONE',  ( -19.03943276465977164, 0.05219959533909376836, 106.2489096053143669 ) ) ;
#85592=CARTESIAN_POINT ( 'NONE',  ( -9.564922557961040184, 16.46253265017147172, 82.91775706135233293 ) ) ;
#85593=CARTESIAN_POINT ( 'NONE',  ( 17.59860650958994555, -7.585241751806880650, 40.92337014262493966 ) ) ;
#85594=CARTESIAN_POINT ( 'NONE',  ( 4.379528057220092307, 16.55341960407617563, 22.29275706135235069 ) ) ;
#85595=CARTESIAN_POINT ( 'NONE',  ( -0.05219959533934338120, 16.53943276465976808, 107.5010903946856899 ) ) ;
#85596=CARTESIAN_POINT ( 'NONE',  ( 5.153800228976615827, -19.02544592524334988, 70.20942372801899012 ) ) ;
#85597=CARTESIAN_POINT ( 'NONE',  ( 5.719274019375991003, -21.55341960407610458, 37.70724293864769550 ) ) ;
#85598=CARTESIAN_POINT ( 'NONE',  ( 10.81492255796106328, -18.62759615963255655, 50.41775706135235424 ) ) ;
#85600=CARTESIAN_POINT ( 'NONE',  ( -4.379528057220086978, -16.55341960407618274, 19.79275706135235069 ) ) ;
#85601=CARTESIAN_POINT ( 'NONE',  ( 17.49999999999998934, 3.258235366253115384, 22.47418410639502184 ) ) ;
#85602=CARTESIAN_POINT ( 'NONE',  ( -5.049401038298153566, 19.05341960407611168, 75.20724293864769550 ) ) ;
#85603=EDGE_CURVE ( 'NONE', #78316, #20950, #176626, .T. ) ;
#85605=CARTESIAN_POINT ( 'NONE',  ( -14.34966873604960291, -8.224510206698953496, 91.66557627198103830 ) ) ;
#85606=CARTESIAN_POINT ( 'NONE',  ( -5.049401038298153566, 19.05341960407611168, 80.20724293864769550 ) ) ;
#85607=CARTESIAN_POINT ( 'NONE',  ( 13.97604488694527802, 13.89961937509977652, 94.37390960531436690 ) ) ;
#85609=CARTESIAN_POINT ( 'NONE',  ( -0.05219959533936034679, 19.03943276465977164, 97.50109039468567573 ) ) ;
#85610=CARTESIAN_POINT ( 'NONE',  ( 15.72974639402199770, -15.80617190586745480, 73.12390960531436690 ) ) ;
#85611=CARTESIAN_POINT ( 'NONE',  ( -19.03943276465977164, 0.05219959533909376836, 31.24890960531435979 ) ) ;
#85612=CARTESIAN_POINT ( 'NONE',  ( 5.153800228976615827, -19.02544592524334988, 55.20942372801899722 ) ) ;
#85613=CARTESIAN_POINT ( 'NONE',  ( 13.89961937509977652, -13.97604488694527269, 53.12390960531434558 ) ) ;
#85614=CARTESIAN_POINT ( 'NONE',  ( -16.46253265017160317, 9.564922557960807481, 95.83224293864769550 ) ) ;
#85616=CARTESIAN_POINT ( 'NONE',  ( -15.80617190586745835, -15.72974639402198527, 101.8739096053143811 ) ) ;
#85617=CARTESIAN_POINT ( 'NONE',  ( -4.379528057220328563, 16.55341960407611168, 100.2072429386476955 ) ) ;
#85618=CARTESIAN_POINT ( 'NONE',  ( -16.51473224551069308, -9.474510206698971260, 86.66557627198102409 ) ) ;
#85619=CARTESIAN_POINT ( 'NONE',  ( -9.474510206698720793, -16.51473224551083518, 59.58442372801900433 ) ) ;
#85620=CARTESIAN_POINT ( 'NONE',  ( 15.80617190586746368, 15.72974639402197994, 94.37390960531436690 ) ) ;
#85621=CARTESIAN_POINT ( 'NONE',  ( -18.62759615963270932, 10.81492255796079327, 70.83224293864770971 ) ) ;
#85623=CARTESIAN_POINT ( 'NONE',  ( 14.34966873604960469, 8.224510206698951720, 34.16557627198102409 ) ) ;
#85624=CARTESIAN_POINT ( 'NONE',  ( -21.53943276465977519, -0.05219959533937600094, 98.75109039468568994 ) ) ;
#85625=CARTESIAN_POINT ( 'NONE',  ( -4.379528057220086978, -16.55341960407618274, 59.79275706135234714 ) ) ;
#85626=CARTESIAN_POINT ( 'NONE',  ( -16.51473224551069308, -9.474510206698971260, 91.66557627198103830 ) ) ;
#85627=CARTESIAN_POINT ( 'NONE',  ( 16.46253265017160672, -9.564922557960803928, 28.33224293864769550 ) ) ;
#85628=CARTESIAN_POINT ( 'NONE',  ( 18.62759615963255655, 10.81492255796105972, 36.66775706135234714 ) ) ;
#85629=CARTESIAN_POINT ( 'NONE',  ( 10.81492255796106328, -18.62759615963255655, 55.41775706135234714 ) ) ;
#85630=CARTESIAN_POINT ( 'NONE',  ( -0.05219959533909027116, -19.03943276465977164, 42.49890960531435269 ) ) ;
#85631=CARTESIAN_POINT ( 'NONE',  ( 15.72974639402176855, 15.80617190586768217, 36.87609039468568994 ) ) ;
#85632=CARTESIAN_POINT ( 'NONE',  ( 19.02544592524334988, 5.153800228976608722, 71.45942372801900433 ) ) ;
#85633=EDGE_CURVE ( 'NONE', #38745, #146788, #194818, .T. ) ;
#85634=CARTESIAN_POINT ( 'NONE',  ( -5.153800228976607833, 19.02544592524334988, 67.70942372801900433 ) ) ;
#85635=CARTESIAN_POINT ( 'NONE',  ( -13.97604488694527625, -13.89961937509977652, 26.87390960531434558 ) ) ;
#85636=CARTESIAN_POINT ( 'NONE',  ( 16.55341960407618274, -4.379528057220086978, 76.04275706135237556 ) ) ;
#85637=CARTESIAN_POINT ( 'NONE',  ( -5.049401038298153566, 19.05341960407611168, 55.20724293864769550 ) ) ;
#85639=CARTESIAN_POINT ( 'NONE',  ( -16.46253265017160317, 9.564922557960807481, 100.8322429386477097 ) ) ;
#85640=CARTESIAN_POINT ( 'NONE',  ( -16.51473224551069308, -9.474510206698971260, 36.66557627198102409 ) ) ;
#85642=CARTESIAN_POINT ( 'NONE',  ( -0.05219959533907301413, -21.53943276465977519, 67.49890960531436690 ) ) ;
#85643=CARTESIAN_POINT ( 'NONE',  ( -12.14591786802326823, 12.06949235617739902, 58.12609039468568994 ) ) ;
#85644=CARTESIAN_POINT ( 'NONE',  ( -16.46253265017146816, -9.564922557961047289, 24.16775706135233648 ) ) ;
#85645=CARTESIAN_POINT ( 'NONE',  ( -9.474510206698964154, 16.51473224551069663, 50.41557627198102409 ) ) ;
#85646=CARTESIAN_POINT ( 'NONE',  ( -4.483927247898539470, -16.52544592524342804, 42.29057627198103120 ) ) ;
#85647=CARTESIAN_POINT ( 'NONE',  ( 8.224510206698953496, -14.34966873604960469, 62.91557627198102409 ) ) ;
#85648=CARTESIAN_POINT ( 'NONE',  ( -5.153800228976328057, -19.02544592524343514, 77.29057627198099567 ) ) ;
#85649=CARTESIAN_POINT ( 'NONE',  ( 18.62759615963255655, 10.81492255796105972, 36.66775706135234714 ) ) ;
#85650=CARTESIAN_POINT ( 'NONE',  ( -16.51473224551069308, -9.474510206698971260, 96.66557627198102409 ) ) ;
#85651=CARTESIAN_POINT ( 'NONE',  ( 15.80617190586769283, -15.72974639402175789, 100.6260903946857184 ) ) ;
#85652=CARTESIAN_POINT ( 'NONE',  ( -8.314922557961024197, 14.29746914071037800, 67.91775706135234714 ) ) ;
#85653=CARTESIAN_POINT ( 'NONE',  ( 0.05219959533909260263, 19.03943276465977164, 104.9989096053143669 ) ) ;
#85654=CARTESIAN_POINT ( 'NONE',  ( -10.72451020669898014, 18.67979575497178502, 85.41557627198102409 ) ) ;
#85655=CARTESIAN_POINT ( 'NONE',  ( 14.29746914071049879, -8.314922557960816363, 48.33224293864770260 ) ) ;
#85656=CARTESIAN_POINT ( 'NONE',  ( -5.153800228976328057, -19.02544592524343514, 47.29057627198102409 ) ) ;
#85657=CARTESIAN_POINT ( 'NONE',  ( -4.483927247898782831, 16.52544592524335698, 57.70942372801901143 ) ) ;
#85658=CARTESIAN_POINT ( 'NONE',  ( -14.34966873604960291, -8.224510206698953496, 66.66557627198102409 ) ) ;
#85659=CARTESIAN_POINT ( 'NONE',  ( 9.474510206698971260, -16.51473224551069308, 107.9155762719810383 ) ) ;
#85660=CARTESIAN_POINT ( 'NONE',  ( 18.62759615963271287, -10.81492255796078972, 28.33224293864769550 ) ) ;
#85661=CARTESIAN_POINT ( 'NONE',  ( -9.564922557961040184, 16.46253265017147172, 32.91775706135233293 ) ) ;
#85662=CARTESIAN_POINT ( 'NONE',  ( -16.52544592524342804, 4.483927247898546575, 101.0405762719810383 ) ) ;
#85663=CARTESIAN_POINT ( 'NONE',  ( 9.474510206698971260, -16.51473224551069308, 112.9155762719810383 ) ) ;
#85664=ORIENTED_EDGE ( 'NONE', *, *, #177312, .F. ) ;
#85665=CARTESIAN_POINT ( 'NONE',  ( -12.06949235617739369, -12.14591786802326823, 59.37609039468568284 ) ) ;
#85666=CARTESIAN_POINT ( 'NONE',  ( 9.564922557960805705, 16.46253265017160317, 59.58224293864769550 ) ) ;
#85668=CARTESIAN_POINT ( 'NONE',  ( -16.51473224551082808, 9.474510206698731452, 43.33442372801900433 ) ) ;
#85669=CARTESIAN_POINT ( 'NONE',  ( 12.06949235617739724, 12.14591786802326823, 91.87609039468568994 ) ) ;
#85670=CARTESIAN_POINT ( 'NONE',  ( 5.153800228976615827, -19.02544592524334988, 90.20942372801900433 ) ) ;
#85671=CARTESIAN_POINT ( 'NONE',  ( -10.81492255796105439, 18.62759615963255655, 62.91775706135236135 ) ) ;
#85672=CARTESIAN_POINT ( 'NONE',  ( 16.46253265017160672, -9.564922557960803928, 73.33224293864769550 ) ) ;
#85673=CARTESIAN_POINT ( 'NONE',  ( -5.823673210054116645, -21.52544592524344225, 97.29057627198105251 ) ) ;
#85674=CARTESIAN_POINT ( 'NONE',  ( -12.14591786802309592, -12.06949235617757132, 111.8739096053143669 ) ) ;
#85675=CARTESIAN_POINT ( 'NONE',  ( -5.153800228976607833, 19.02544592524334988, 87.70942372801897591 ) ) ;
#85676=CARTESIAN_POINT ( 'NONE',  ( -15.80617190586745835, -15.72974639402198527, 81.87390960531435269 ) ) ;
#85677=CARTESIAN_POINT ( 'NONE',  ( 16.51473224551083163, -9.474510206698727899, 40.83442372801900433 ) ) ;
#85678=CARTESIAN_POINT ( 'NONE',  ( 19.39720447994795194, 5.500000000000020428, 97.16317477297175742 ) ) ;
#85679=CARTESIAN_POINT ( 'NONE',  ( 10.72451020669898902, -18.67979575497178502, 87.91557627198103830 ) ) ;
#85681=CARTESIAN_POINT ( 'NONE',  ( -19.02544592524342804, 5.153800228976336051, 66.04057627198103830 ) ) ;
#85683=CARTESIAN_POINT ( 'NONE',  ( 16.55341960407618274, -4.379528057220086978, 21.04275706135234714 ) ) ;
#85685=CARTESIAN_POINT ( 'NONE',  ( -19.05341960407611168, -5.049401038298163336, 51.45724293864770260 ) ) ;
#85686=CARTESIAN_POINT ( 'NONE',  ( -16.46253265017160317, 9.564922557960807481, 115.8322429386477097 ) ) ;
#85687=CARTESIAN_POINT ( 'NONE',  ( 21.55341960407610458, 5.719274019375980345, 98.95724293864770971 ) ) ;
#85688=CARTESIAN_POINT ( 'NONE',  ( -14.34966873604960291, -8.224510206698953496, 46.66557627198102409 ) ) ;
#85689=CARTESIAN_POINT ( 'NONE',  ( 0.05219959533937995610, -21.53943276465977519, 80.00109039468568994 ) ) ;
#85691=CARTESIAN_POINT ( 'NONE',  ( -4.379528057220086978, -16.55341960407618274, 29.79275706135234358 ) ) ;
#85692=CARTESIAN_POINT ( 'NONE',  ( -16.46253265017146816, -9.564922557961047289, 24.16775706135233648 ) ) ;
#85693=CARTESIAN_POINT ( 'NONE',  ( -16.52544592524342804, 4.483927247898546575, 26.04057627198103475 ) ) ;
#85694=CARTESIAN_POINT ( 'NONE',  ( -18.67979575497193778, 10.72451020669871902, 33.33442372801900433 ) ) ;
#85695=CARTESIAN_POINT ( 'NONE',  ( -5.719274019375665041, -21.55341960407619695, 19.79275706135235069 ) ) ;
#85696=CARTESIAN_POINT ( 'NONE',  ( 21.52544592524344225, -5.823673210054117533, 58.54057627198103120 ) ) ;
#85697=CARTESIAN_POINT ( 'NONE',  ( 19.02544592524334988, 5.153800228976608722, 96.45942372801897591 ) ) ;
#85698=CARTESIAN_POINT ( 'NONE',  ( 19.02544592524334988, 5.153800228976608722, 71.45942372801900433 ) ) ;
#85700=CARTESIAN_POINT ( 'NONE',  ( -15.72974639402176322, -15.80617190586768395, 74.37609039468568994 ) ) ;
#85701=CARTESIAN_POINT ( 'NONE',  ( 16.51473224551083163, -9.474510206698727899, 50.83442372801899722 ) ) ;
#85702=CARTESIAN_POINT ( 'NONE',  ( -5.153800228976328057, -19.02544592524343514, 22.29057627198102765 ) ) ;
#85703=CARTESIAN_POINT ( 'NONE',  ( 10.72451020669898902, -18.67979575497178502, 42.91557627198103120 ) ) ;
#85704=CARTESIAN_POINT ( 'NONE',  ( 16.55341960407611168, 4.379528057220329451, 53.95724293864770260 ) ) ;
#85705=CARTESIAN_POINT ( 'NONE',  ( -16.52216118717209881, -7.221426719304473885, 26.07599021046994281 ) ) ;
#85706=CARTESIAN_POINT ( 'NONE',  ( -15.80617190586768217, 15.72974639402176855, 108.1260903946856757 ) ) ;
#85707=CARTESIAN_POINT ( 'NONE',  ( 12.14591786802327356, -12.06949235617739191, 80.62609039468567573 ) ) ;
#85708=CARTESIAN_POINT ( 'NONE',  ( -12.14591786802309592, -12.06949235617757132, 46.87390960531435979 ) ) ;
#85709=CARTESIAN_POINT ( 'NONE',  ( 0.05219959533937995610, -21.53943276465977519, 70.00109039468568994 ) ) ;
#85710=CARTESIAN_POINT ( 'NONE',  ( -15.80617190586768217, 15.72974639402176855, 78.12609039468570415 ) ) ;
#85711=CARTESIAN_POINT ( 'NONE',  ( -5.823673210054116645, -21.52544592524344225, 82.29057627198103830 ) ) ;
#85712=CARTESIAN_POINT ( 'NONE',  ( 5.153800228976335163, 19.02544592524342804, 44.79057627198103830 ) ) ;
#85713=CARTESIAN_POINT ( 'NONE',  ( -5.823673210054431948, 21.52544592524334988, 57.70942372801901143 ) ) ;
#85714=CARTESIAN_POINT ( 'NONE',  ( -9.564922557960796823, -16.46253265017161027, 37.08224293864768839 ) ) ;
#85715=CARTESIAN_POINT ( 'NONE',  ( 19.05341960407611168, 5.049401038298154454, 48.95724293864768129 ) ) ;
#85716=CARTESIAN_POINT ( 'NONE',  ( -14.29746914071049879, 8.314922557960819915, 95.83224293864770971 ) ) ;
#85717=CARTESIAN_POINT ( 'NONE',  ( -9.474510206698964154, 16.51473224551069663, 95.41557627198102409 ) ) ;
#85718=CARTESIAN_POINT ( 'NONE',  ( 0.05219959533910956823, 16.53943276465976808, 34.99890960531435979 ) ) ;
#85719=CARTESIAN_POINT ( 'NONE',  ( -16.52544592524342804, 4.483927247898546575, 116.0405762719810383 ) ) ;
#85720=CARTESIAN_POINT ( 'NONE',  ( -10.81492255796078084, -18.62759615963271287, 77.08224293864769550 ) ) ;
#85721=CARTESIAN_POINT ( 'NONE',  ( 5.719274019375673035, 21.55341960407619339, 27.29275706135234358 ) ) ;
#85723=CARTESIAN_POINT ( 'NONE',  ( -16.53943276465976808, -0.05219959533934237506, 28.75109039468567929 ) ) ;
#85724=CARTESIAN_POINT ( 'NONE',  ( 15.72974639402199770, -15.80617190586745480, 68.12390960531436690 ) ) ;
#85725=CARTESIAN_POINT ( 'NONE',  ( 21.52544592524334988, 5.823673210054432836, 91.45942372801901854 ) ) ;
#85726=CARTESIAN_POINT ( 'NONE',  ( -19.03943276465977164, 0.05219959533909376836, 86.24890960531436690 ) ) ;
#85727=CARTESIAN_POINT ( 'NONE',  ( -5.719274019375665041, -21.55341960407619695, 29.79275706135234358 ) ) ;
#85728=CARTESIAN_POINT ( 'NONE',  ( -19.02544592524342804, 5.153800228976336051, 111.0405762719810099 ) ) ;
#85729=CARTESIAN_POINT ( 'NONE',  ( 8.314922557961029526, -14.29746914071037800, 90.41775706135236135 ) ) ;
#85730=CARTESIAN_POINT ( 'NONE',  ( 10.72451020669871369, 18.67979575497193778, 67.08442372801901854 ) ) ;
#85731=B_SPLINE_CURVE_WITH_KNOTS ( 'NONE', 3,
 ( #133382, #175904, #8034, #195073, #56552, #41387, #26229, #87868, #149556, #37376, #99033, #160723, #23220, #115220, #176912, #100039, #22215, #84863, #7024, #68706, #130363, #192060, #69715, #131382, #198051, #123176, #92836, #105044, #135400, #166728, #11052, #73727 ),
 .UNSPECIFIED., .F., .F.,
 ( 4, 2, 2, 2, 2, 2, 2, 2, 2, 2, 2, 2, 2, 2, 2, 4 ),
 ( 3.469446951953614189E-18, 0.0003712461730036830374, 0.0007424923460073626054, 0.001113738519011042011, 0.001484984692014721741, 0.002227477038022078817, 0.002598723211025754428, 0.002969969384029430039, 0.003341215557033105649, 0.003712461730036781260, 0.004083707903040456437, 0.004454954076044132481, 0.004826200249047807658, 0.005197446422051483703, 0.005568692595055158880, 0.005939938768058834057 ),
 .UNSPECIFIED. ) ;
#85732=CARTESIAN_POINT ( 'NONE',  ( 0.05219959533936267826, -19.03943276465977164, 20.00109039468567218 ) ) ;
#85733=CARTESIAN_POINT ( 'NONE',  ( -16.55341960407617563, 4.379528057220093196, 73.54275706135234714 ) ) ;
#85734=CARTESIAN_POINT ( 'NONE',  ( -21.55341960407619339, 5.719274019375674811, 28.54275706135234358 ) ) ;
#85735=CARTESIAN_POINT ( 'NONE',  ( -16.46253265017160317, 9.564922557960807481, 25.83224293864769194 ) ) ;
#85736=CARTESIAN_POINT ( 'NONE',  ( -21.55341960407619339, 5.719274019375674811, 93.54275706135234714 ) ) ;
#85737=CARTESIAN_POINT ( 'NONE',  ( 16.46253265017160672, -9.564922557960803928, 88.33224293864769550 ) ) ;
#85738=CARTESIAN_POINT ( 'NONE',  ( -21.52544592524343514, 5.823673210054127303, 86.04057627198102409 ) ) ;
#85739=CARTESIAN_POINT ( 'NONE',  ( -19.03943276465977164, -0.05219959533935918106, 53.75109039468566863 ) ) ;
#85740=CARTESIAN_POINT ( 'NONE',  ( 18.22780087662123805, -5.499999999999976019, 88.51763182126893525 ) ) ;
#85741=CARTESIAN_POINT ( 'NONE',  ( 18.62759615963271287, -10.81492255796078972, 48.33224293864770260 ) ) ;
#85742=CARTESIAN_POINT ( 'NONE',  ( -9.474510206698964154, 16.51473224551069663, 90.41557627198103830 ) ) ;
#85743=CARTESIAN_POINT ( 'NONE',  ( -8.224510206698948167, 14.34966873604960824, 55.41557627198102409 ) ) ;
#85745=CARTESIAN_POINT ( 'NONE',  ( 19.03943276465977164, 0.05219959533936151252, 81.25109039468567573 ) ) ;
#85747=CARTESIAN_POINT ( 'NONE',  ( -9.564922557961040184, 16.46253265017147172, 102.9177570613523329 ) ) ;
#85748=CARTESIAN_POINT ( 'NONE',  ( -21.52544592524343514, 5.823673210054127303, 86.04057627198102409 ) ) ;
#85749=CARTESIAN_POINT ( 'NONE',  ( 12.14591786802309770, 12.06949235617756955, 69.37390960531436690 ) ) ;
#85750=CARTESIAN_POINT ( 'NONE',  ( -13.89961937509977652, 13.97604488694528158, 105.6239096053143527 ) ) ;
#85751=CARTESIAN_POINT ( 'NONE',  ( -4.379528057220086978, -16.55341960407618274, 49.79275706135234714 ) ) ;
#85752=CARTESIAN_POINT ( 'NONE',  ( 16.51473224551069308, 9.474510206698969483, 59.16557627198102409 ) ) ;
#85753=CARTESIAN_POINT ( 'NONE',  ( -21.53943276465977519, 0.05219959533907696930, 111.2489096053143669 ) ) ;
#85754=CARTESIAN_POINT ( 'NONE',  ( 9.564922557961047289, -16.46253265017146816, 95.41775706135233293 ) ) ;
#85755=CARTESIAN_POINT ( 'NONE',  ( 19.02544592524343514, -5.153800228976328945, 93.54057627198102409 ) ) ;
#85756=CARTESIAN_POINT ( 'NONE',  ( -9.564922557960796823, -16.46253265017161027, 77.08224293864769550 ) ) ;
#85757=CARTESIAN_POINT ( 'NONE',  ( -21.55341960407610458, -5.719274019375992779, 71.45724293864769550 ) ) ;
#85758=CARTESIAN_POINT ( 'NONE',  ( -19.03943276465977164, 0.05219959533909376836, 46.24890960531435979 ) ) ;
#85760=CARTESIAN_POINT ( 'NONE',  ( -12.06949235617756955, 12.14591786802309770, 60.62390960531437401 ) ) ;
#85761=CARTESIAN_POINT ( 'NONE',  ( 5.153800228976335163, 19.02544592524342804, 99.79057627198102409 ) ) ;
#85763=CARTESIAN_POINT ( 'NONE',  ( 9.564922557961047289, -16.46253265017146816, 65.41775706135233293 ) ) ;
#85765=CARTESIAN_POINT ( 'NONE',  ( 18.62759615963271287, -10.81492255796078972, 88.33224293864769550 ) ) ;
#85766=CARTESIAN_POINT ( 'NONE',  ( -16.51473224551082808, 9.474510206698731452, 53.33442372801900433 ) ) ;
#85767=CARTESIAN_POINT ( 'NONE',  ( -9.474510206698964154, 16.51473224551069663, 95.41557627198102409 ) ) ;
#85768=CARTESIAN_POINT ( 'NONE',  ( -21.53943276465977519, 0.05219959533907696930, 36.24890960531435979 ) ) ;
#85769=CARTESIAN_POINT ( 'NONE',  ( -19.05341960407611168, -5.049401038298163336, 71.45724293864766707 ) ) ;
#85770=CARTESIAN_POINT ( 'NONE',  ( -21.55341960407619339, 5.719274019375674811, 68.54275706135234714 ) ) ;
#85771=CARTESIAN_POINT ( 'NONE',  ( 0.05219959533909260263, 19.03943276465977164, 39.99890960531436690 ) ) ;
#85772=CARTESIAN_POINT ( 'NONE',  ( 16.55341960407611168, 4.379528057220329451, 78.95724293864769550 ) ) ;
#85774=CARTESIAN_POINT ( 'NONE',  ( 14.34966873604972726, -8.224510206698740333, 20.83442372801901143 ) ) ;
#85775=CARTESIAN_POINT ( 'NONE',  ( -21.52544592524334988, -5.823673210054445271, 58.95942372801902565 ) ) ;
#85777=CARTESIAN_POINT ( 'NONE',  ( -9.474510206698964154, 16.51473224551069663, 110.4155762719810383 ) ) ;
#85778=CARTESIAN_POINT ( 'NONE',  ( 19.02544592524334988, 5.153800228976608722, 66.45942372801899012 ) ) ;
#85780=DIRECTION ( 'NONE',  ( 0.000000000000000000, 0.000000000000000000, -1.000000000000000000 ) ) ;
#85781=CARTESIAN_POINT ( 'NONE',  ( 15.80617190586769283, -15.72974639402175789, 25.62609039468567929 ) ) ;
#85782=CARTESIAN_POINT ( 'NONE',  ( 9.564922557960805705, 16.46253265017160317, 54.58224293864769550 ) ) ;
#85784=CARTESIAN_POINT ( 'NONE',  ( 9.474510206698729675, 16.51473224551082808, 22.08442372801899722 ) ) ;
#85785=CARTESIAN_POINT ( 'NONE',  ( -0.05219959533909027116, -19.03943276465977164, 47.49890960531435979 ) ) ;
#85786=CARTESIAN_POINT ( 'NONE',  ( 10.72451020669871369, 18.67979575497193778, 112.0844237280190185 ) ) ;
#85787=CARTESIAN_POINT ( 'NONE',  ( -0.05219959533934338120, 16.53943276465976808, 92.50109039468567573 ) ) ;
#85788=CARTESIAN_POINT ( 'NONE',  ( 9.564922557960805705, 16.46253265017160317, 99.58224293864770971 ) ) ;
#85789=CARTESIAN_POINT ( 'NONE',  ( -18.62759615963255300, -10.81492255796106328, 69.16775706135234714 ) ) ;
#85791=CARTESIAN_POINT ( 'NONE',  ( -19.02544592524342804, 5.153800228976336051, 111.0405762719810099 ) ) ;
#85793=CARTESIAN_POINT ( 'NONE',  ( -16.53943276465976808, -0.05219959533934237506, 68.75109039468568994 ) ) ;
#85794=CARTESIAN_POINT ( 'NONE',  ( -10.81492255796105439, 18.62759615963255655, 72.91775706135234714 ) ) ;
#85795=CARTESIAN_POINT ( 'NONE',  ( 15.80617190586769283, -15.72974639402175789, 100.6260903946857184 ) ) ;
#85797=CARTESIAN_POINT ( 'NONE',  ( -12.06949235617739369, -12.14591786802326823, 39.37609039468567573 ) ) ;
#85798=CARTESIAN_POINT ( 'NONE',  ( -16.46253265017160317, 9.564922557960807481, 85.83224293864769550 ) ) ;
#85799=CARTESIAN_POINT ( 'NONE',  ( 5.153800228976335163, 19.02544592524342804, 109.7905762719810099 ) ) ;
#85801=CARTESIAN_POINT ( 'NONE',  ( 17.12812012977024168, 6.668231424566063659, 43.85948759323144230 ) ) ;
#85802=CARTESIAN_POINT ( 'NONE',  ( 5.049401038298161559, -19.05341960407611168, 37.70724293864768839 ) ) ;
#85803=CARTESIAN_POINT ( 'NONE',  ( 21.53943276465977519, -0.05219959533907433946, 43.74890960531435979 ) ) ;
#85804=CARTESIAN_POINT ( 'NONE',  ( 14.29746914071037800, 8.314922557961029526, 106.6677570613523756 ) ) ;
#85805=CARTESIAN_POINT ( 'NONE',  ( 16.52544592524342804, -4.483927247898539470, 83.54057627198102409 ) ) ;
#85806=CARTESIAN_POINT ( 'NONE',  ( -19.03943276465977164, 0.05219959533909376836, 81.24890960531436690 ) ) ;
#85807=CARTESIAN_POINT ( 'NONE',  ( -21.52544592524334988, -5.823673210054445271, 103.9594237280190185 ) ) ;
#85808=CARTESIAN_POINT ( 'NONE',  ( 14.34966873604972726, -8.224510206698740333, 20.83442372801901143 ) ) ;
#85809=CARTESIAN_POINT ( 'NONE',  ( 12.14591786802309770, 12.06949235617756955, 94.37390960531436690 ) ) ;
#85810=CARTESIAN_POINT ( 'NONE',  ( 10.72451020669871369, 18.67979575497193778, 47.08442372801901854 ) ) ;
#85811=CARTESIAN_POINT ( 'NONE',  ( -21.55341960407610458, -5.719274019375992779, 81.45724293864769550 ) ) ;
#85812=CARTESIAN_POINT ( 'NONE',  ( -9.564922557961040184, 16.46253265017147172, 52.91775706135233293 ) ) ;
#85813=CARTESIAN_POINT ( 'NONE',  ( -16.46253265017160317, 9.564922557960807481, 45.83224293864769550 ) ) ;
#85814=CARTESIAN_POINT ( 'NONE',  ( 16.51473224551069308, 9.474510206698969483, 94.16557627198103830 ) ) ;
#85815=CARTESIAN_POINT ( 'NONE',  ( 0.05219959533910956823, 16.53943276465976808, 69.99890960531435269 ) ) ;
#85816=CARTESIAN_POINT ( 'NONE',  ( -16.53943276465976808, 0.05219959533911058130, 46.24890960531435979 ) ) ;
#85817=CARTESIAN_POINT ( 'NONE',  ( 4.483927247898790824, -16.52544592524335698, 110.2094237280190185 ) ) ;
#85818=CARTESIAN_POINT ( 'NONE',  ( 9.564922557961047289, -16.46253265017146816, 60.41775706135233293 ) ) ;
#85819=CARTESIAN_POINT ( 'NONE',  ( -19.52217212775661181, 5.499999999999920064, 84.93993709005259518 ) ) ;
#85820=CARTESIAN_POINT ( 'NONE',  ( 0.05219959533907565091, 21.53943276465977519, 24.99890960531435624 ) ) ;
#85821=CARTESIAN_POINT ( 'NONE',  ( 14.29746914071049879, -8.314922557960816363, 93.33224293864769550 ) ) ;
#85823=CARTESIAN_POINT ( 'NONE',  ( 9.474510206698971260, -16.51473224551069308, 42.91557627198103120 ) ) ;
#85824=CARTESIAN_POINT ( 'NONE',  ( 5.823673210054125526, 21.52544592524343514, 54.79057627198104541 ) ) ;
#85825=CARTESIAN_POINT ( 'NONE',  ( -13.97604488694527625, -13.89961937509977652, 26.87390960531434558 ) ) ;
#85826=CARTESIAN_POINT ( 'NONE',  ( -16.55341960407617563, 4.379528057220093196, 83.54275706135234714 ) ) ;
#85827=CARTESIAN_POINT ( 'NONE',  ( 16.51473224551069308, 9.474510206698969483, 64.16557627198102409 ) ) ;
#85828=CARTESIAN_POINT ( 'NONE',  ( -16.51473224551082808, 9.474510206698731452, 43.33442372801900433 ) ) ;
#85829=CARTESIAN_POINT ( 'NONE',  ( 10.81492255796106328, -18.62759615963255655, 50.41775706135235424 ) ) ;
#85830=CARTESIAN_POINT ( 'NONE',  ( 15.80617190586746368, 15.72974639402197994, 39.37390960531436690 ) ) ;
#85831=CARTESIAN_POINT ( 'NONE',  ( 4.483927247898545687, 16.52544592524342804, 104.7905762719810241 ) ) ;
#85832=CARTESIAN_POINT ( 'NONE',  ( -0.05219959533936034679, 19.03943276465977164, 97.50109039468567573 ) ) ;
#85834=CARTESIAN_POINT ( 'NONE',  ( 17.49999999999999645, 3.242565516156353134, 37.49999999998637179 ) ) ;
#85835=CARTESIAN_POINT ( 'NONE',  ( 15.80617190586746368, 15.72974639402197994, 49.37390960531436690 ) ) ;
#85836=CARTESIAN_POINT ( 'NONE',  ( -19.03943276465977164, 0.05219959533909376836, 21.24890960531436335 ) ) ;
#85837=CARTESIAN_POINT ( 'NONE',  ( -15.80617190586768217, 15.72974639402176855, 83.12609039468568994 ) ) ;
#85838=CARTESIAN_POINT ( 'NONE',  ( 12.06949235617757843, -12.14591786802309237, 43.12390960531435269 ) ) ;
#85839=CARTESIAN_POINT ( 'NONE',  ( -4.483927247898782831, 16.52544592524335698, 57.70942372801901143 ) ) ;
#85840=CARTESIAN_POINT ( 'NONE',  ( 12.14591786802309770, 12.06949235617756955, 59.37390960531436690 ) ) ;
#85841=CARTESIAN_POINT ( 'NONE',  ( 10.81492255796078972, 18.62759615963270932, 79.58224293864769550 ) ) ;
#85842=CARTESIAN_POINT ( 'NONE',  ( 21.52544592524344225, -5.823673210054117533, 73.54057627198102409 ) ) ;
#85844=CARTESIAN_POINT ( 'NONE',  ( -19.02544592524342804, 5.153800228976336051, 116.0405762719810383 ) ) ;
#85845=CARTESIAN_POINT ( 'NONE',  ( 13.89961937509977652, -13.97604488694527269, 68.12390960531436690 ) ) ;
#85846=CARTESIAN_POINT ( 'NONE',  ( -13.89961937509977652, 13.97604488694528158, 35.62390960531435269 ) ) ;
#85848=VERTEX_POINT ( 'NONE', #151277 ) ;
#85849=CARTESIAN_POINT ( 'NONE',  ( -12.06949235617739369, -12.14591786802326823, 79.37609039468567573 ) ) ;
#85850=CARTESIAN_POINT ( 'NONE',  ( -21.55341960407619339, 5.719274019375674811, 23.54275706135235424 ) ) ;
#85851=CARTESIAN_POINT ( 'NONE',  ( -9.474510206698964154, 16.51473224551069663, 70.41557627198102409 ) ) ;
#85852=CARTESIAN_POINT ( 'NONE',  ( -15.80617190586768217, 15.72974639402176855, 58.12609039468568994 ) ) ;
#85853=CARTESIAN_POINT ( 'NONE',  ( 19.02544592524343514, -5.153800228976328945, 113.5405762719810241 ) ) ;
#85856=CARTESIAN_POINT ( 'NONE',  ( -5.719274019375665041, -21.55341960407619695, 44.79275706135234714 ) ) ;
#85857=CARTESIAN_POINT ( 'NONE',  ( 9.474510206698971260, -16.51473224551069308, 22.91557627198102765 ) ) ;
#85858=CARTESIAN_POINT ( 'NONE',  ( 13.97604488694527802, 13.89961937509977652, 104.3739096053143385 ) ) ;
#85859=CARTESIAN_POINT ( 'NONE',  ( 13.97604488694548053, -13.89961937509957401, 55.62609039468566863 ) ) ;
#85860=CARTESIAN_POINT ( 'NONE',  ( 15.80617190586746368, 15.72974639402197994, 109.3739096053143811 ) ) ;
#85861=CARTESIAN_POINT ( 'NONE',  ( 13.89961937509957401, 13.97604488694547697, 51.87609039468566863 ) ) ;
#85862=CARTESIAN_POINT ( 'NONE',  ( -13.89961937509957401, -13.97604488694547875, 49.37609039468567573 ) ) ;
#85863=CARTESIAN_POINT ( 'NONE',  ( 12.14591786802327356, -12.06949235617739191, 110.6260903946857042 ) ) ;
#85864=ORIENTED_EDGE ( 'NONE', *, *, #29949, .T. ) ;
#85867=CARTESIAN_POINT ( 'NONE',  ( -9.564922557960796823, -16.46253265017161027, 77.08224293864769550 ) ) ;
#85869=CARTESIAN_POINT ( 'NONE',  ( -21.55341960407619339, 5.719274019375674811, 78.54275706135236135 ) ) ;
#85870=CARTESIAN_POINT ( 'NONE',  ( -21.55341960407619339, 5.719274019375674811, 98.54275706135234714 ) ) ;
#85872=CARTESIAN_POINT ( 'NONE',  ( -9.474510206698964154, 16.51473224551069663, 100.4155762719810241 ) ) ;
#85873=CARTESIAN_POINT ( 'NONE',  ( 10.72451020669871369, 18.67979575497193778, 77.08442372801901854 ) ) ;
#85874=CARTESIAN_POINT ( 'NONE',  ( 12.06949235617739724, 12.14591786802326823, 21.87609039468567573 ) ) ;
#85875=EDGE_CURVE ( 'NONE', #166568, #160624, #132132, .T. ) ;
#85876=CARTESIAN_POINT ( 'NONE',  ( -9.564922557960796823, -16.46253265017161027, 77.08224293864769550 ) ) ;
#85877=CARTESIAN_POINT ( 'NONE',  ( 10.72451020669898902, -18.67979575497178502, 22.91557627198102765 ) ) ;
#85878=CARTESIAN_POINT ( 'NONE',  ( 19.05341960407611168, 5.049401038298154454, 88.95724293864769550 ) ) ;
#85879=CARTESIAN_POINT ( 'NONE',  ( -16.51473224551082808, 9.474510206698731452, 88.33442372801900433 ) ) ;
#85880=CARTESIAN_POINT ( 'NONE',  ( 0.05219959533909260263, 19.03943276465977164, 79.99890960531436690 ) ) ;
#85881=CARTESIAN_POINT ( 'NONE',  ( -19.05341960407611168, -5.049401038298163336, 61.45724293864769550 ) ) ;
#85882=CARTESIAN_POINT ( 'NONE',  ( 5.719274019375991003, -21.55341960407610458, 107.7072429386476955 ) ) ;
#85883=CARTESIAN_POINT ( 'NONE',  ( -12.14591786802326823, 12.06949235617739902, 103.1260903946856757 ) ) ;
#85885=CARTESIAN_POINT ( 'NONE',  ( -19.02544592524334988, -5.153800228976617603, 63.95942372801899012 ) ) ;
#85886=CARTESIAN_POINT ( 'NONE',  ( -0.05219959533909027116, -19.03943276465977164, 87.49890960531436690 ) ) ;
#85887=CARTESIAN_POINT ( 'NONE',  ( 12.14591786802309770, 12.06949235617756955, 84.37390960531438111 ) ) ;
#85888=CARTESIAN_POINT ( 'NONE',  ( -13.89961937509977652, 13.97604488694528158, 30.62390960531435269 ) ) ;
#85889=CARTESIAN_POINT ( 'NONE',  ( -0.05219959533907301413, -21.53943276465977519, 32.49890960531435979 ) ) ;
#85890=CARTESIAN_POINT ( 'NONE',  ( 5.719274019375991003, -21.55341960407610458, 27.70724293864769905 ) ) ;
#85891=CARTESIAN_POINT ( 'NONE',  ( 8.224510206698953496, -14.34966873604960469, 87.91557627198103830 ) ) ;
#85892=CARTESIAN_POINT ( 'NONE',  ( -16.81555441253551564, 7.025013491695475842, 55.63685445334254354 ) ) ;
#85893=CARTESIAN_POINT ( 'NONE',  ( -19.02544592524334988, -5.153800228976617603, 48.95942372801900433 ) ) ;
#85894=CARTESIAN_POINT ( 'NONE',  ( -4.483927247898782831, 16.52544592524335698, 112.7094237280190328 ) ) ;
#85895=CARTESIAN_POINT ( 'NONE',  ( 13.97604488694527802, 13.89961937509977652, 94.37390960531436690 ) ) ;
#85896=CARTESIAN_POINT ( 'NONE',  ( 21.52544592524334988, 5.823673210054432836, 66.45942372801903275 ) ) ;
#85897=CARTESIAN_POINT ( 'NONE',  ( -15.72974639402197994, 15.80617190586746368, 45.62390960531436690 ) ) ;
#85898=CARTESIAN_POINT ( 'NONE',  ( 10.72451020669871369, 18.67979575497193778, 27.08442372801901854 ) ) ;
#85900=CARTESIAN_POINT ( 'NONE',  ( 0.05219959533907565091, 21.53943276465977519, 84.99890960531436690 ) ) ;
#85901=CARTESIAN_POINT ( 'NONE',  ( -16.55341960407611168, -4.379528057220339221, 106.4572429386477097 ) ) ;
#85902=CARTESIAN_POINT ( 'NONE',  ( 19.03943276465977164, 0.05219959533936151252, 76.25109039468566152 ) ) ;
#85903=CARTESIAN_POINT ( 'NONE',  ( -0.05219959533909027116, -19.03943276465977164, 47.49890960531435979 ) ) ;
#85904=CARTESIAN_POINT ( 'NONE',  ( -16.51473224551069308, -9.474510206698971260, 91.66557627198103830 ) ) ;
#85905=CARTESIAN_POINT ( 'NONE',  ( -5.049401038298153566, 19.05341960407611168, 100.2072429386476955 ) ) ;
#85906=CARTESIAN_POINT ( 'NONE',  ( -16.52544592524342804, 4.483927247898546575, 116.0405762719810383 ) ) ;
#85908=CARTESIAN_POINT ( 'NONE',  ( -12.14591786802309592, -12.06949235617757132, 41.87390960531435979 ) ) ;
#85909=CARTESIAN_POINT ( 'NONE',  ( -12.06949235617739369, -12.14591786802326823, 39.37609039468567573 ) ) ;
#85910=CARTESIAN_POINT ( 'NONE',  ( 5.823673210054444382, -21.52544592524334988, 110.2094237280190185 ) ) ;
#85911=CARTESIAN_POINT ( 'NONE',  ( -0.05219959533910754901, -16.53943276465976808, 27.49890960531435269 ) ) ;
#85912=CARTESIAN_POINT ( 'NONE',  ( 10.72451020669871369, 18.67979575497193778, 27.08442372801901854 ) ) ;
#85913=CARTESIAN_POINT ( 'NONE',  ( 5.049401038298161559, -19.05341960407611168, 107.7072429386476955 ) ) ;
#85914=CARTESIAN_POINT ( 'NONE',  ( 14.34966873604972726, -8.224510206698740333, 100.8344237280190185 ) ) ;
#85915=CARTESIAN_POINT ( 'NONE',  ( -12.06949235617739369, -12.14591786802326823, 94.37609039468568994 ) ) ;
#85916=CARTESIAN_POINT ( 'NONE',  ( 14.34966873604972726, -8.224510206698740333, 30.83442372801902209 ) ) ;
#85917=CARTESIAN_POINT ( 'NONE',  ( 9.564922557960805705, 16.46253265017160317, 44.58224293864769550 ) ) ;
#85918=CARTESIAN_POINT ( 'NONE',  ( -16.52544592524342804, 4.483927247898546575, 111.0405762719810525 ) ) ;
#85919=CARTESIAN_POINT ( 'NONE',  ( -18.67979575497193778, 10.72451020669871902, 23.33442372801901499 ) ) ;
#85920=CARTESIAN_POINT ( 'NONE',  ( -9.474510206698964154, 16.51473224551069663, 30.41557627198102054 ) ) ;
#85921=CARTESIAN_POINT ( 'NONE',  ( 19.03943276465977164, -0.05219959533909143690, 103.7489096053143669 ) ) ;
#85922=CARTESIAN_POINT ( 'NONE',  ( 10.72451020669871369, 18.67979575497193778, 27.08442372801901854 ) ) ;
#85923=CARTESIAN_POINT ( 'NONE',  ( 9.564922557960805705, 16.46253265017160317, 29.58224293864769550 ) ) ;
#85924=CARTESIAN_POINT ( 'NONE',  ( 13.89961937509977652, -13.97604488694527269, 108.1239096053143669 ) ) ;
#85925=CARTESIAN_POINT ( 'NONE',  ( -16.19135201231363652, -7.376712067592051447, 35.18680854052033169 ) ) ;
#85926=CARTESIAN_POINT ( 'NONE',  ( 19.03943276465977164, -0.05219959533909143690, 103.7489096053143669 ) ) ;
#85927=CARTESIAN_POINT ( 'NONE',  ( 18.62759615963255655, 10.81492255796105972, 41.66775706135235424 ) ) ;
#85928=CARTESIAN_POINT ( 'NONE',  ( 8.224510206698953496, -14.34966873604960469, 92.91557627198103830 ) ) ;
#85929=CARTESIAN_POINT ( 'NONE',  ( -5.049401038298153566, 19.05341960407611168, 95.20724293864770971 ) ) ;
#85930=CARTESIAN_POINT ( 'NONE',  ( 17.72696623605161292, -5.499999999999952038, 96.09811031808415294 ) ) ;
#85931=CARTESIAN_POINT ( 'NONE',  ( -14.29746914071037622, -8.314922557961029526, 69.16775706135234714 ) ) ;
#85932=CARTESIAN_POINT ( 'NONE',  ( 21.55341960407619695, -5.719274019375665929, 81.04275706135236135 ) ) ;
#85933=CARTESIAN_POINT ( 'NONE',  ( -16.55341960407617563, 4.379528057220093196, 43.54275706135235424 ) ) ;
#85934=CARTESIAN_POINT ( 'NONE',  ( 16.46253265017160672, -9.564922557960803928, 78.33224293864769550 ) ) ;
#85935=CARTESIAN_POINT ( 'NONE',  ( 4.483927247898790824, -16.52544592524335698, 20.20942372801900788 ) ) ;
#85936=CARTESIAN_POINT ( 'NONE',  ( 16.52544592524335698, 4.483927247898782831, 86.45942372801901854 ) ) ;
#85937=CARTESIAN_POINT ( 'NONE',  ( 5.153800228976615827, -19.02544592524334988, 90.20942372801900433 ) ) ;
#85938=CARTESIAN_POINT ( 'NONE',  ( 19.05341960407611168, 5.049401038298154454, 68.95724293864769550 ) ) ;
#85939=CARTESIAN_POINT ( 'NONE',  ( -15.72974639402197994, 15.80617190586746368, 85.62390960531436690 ) ) ;
#85940=CARTESIAN_POINT ( 'NONE',  ( -8.224510206698948167, 14.34966873604960824, 90.41557627198103830 ) ) ;
#85941=CARTESIAN_POINT ( 'NONE',  ( 0.05219959533936267826, -19.03943276465977164, 95.00109039468567573 ) ) ;
#85942=CARTESIAN_POINT ( 'NONE',  ( -12.06949235617739369, -12.14591786802326823, 54.37609039468568994 ) ) ;
#85943=CARTESIAN_POINT ( 'NONE',  ( -18.39443945427638738, 5.500000000000032863, 78.51745347608651571 ) ) ;
#85944=CARTESIAN_POINT ( 'NONE',  ( -19.05341960407617563, 5.049401038297882671, 53.54275706135231871 ) ) ;
#85945=CARTESIAN_POINT ( 'NONE',  ( 0.05219959533910956823, 16.53943276465976808, 34.99890960531435979 ) ) ;
#85946=CARTESIAN_POINT ( 'NONE',  ( -0.05219959533910754901, -16.53943276465976808, 77.49890960531433848 ) ) ;
#85947=CARTESIAN_POINT ( 'NONE',  ( 5.153800228976615827, -19.02544592524334988, 25.20942372801900433 ) ) ;
#85948=CARTESIAN_POINT ( 'NONE',  ( -19.52217212775660471, 5.499999999999917399, 89.93993709005258097 ) ) ;
#85949=CARTESIAN_POINT ( 'NONE',  ( -0.05219959533937732626, 21.53943276465977519, 27.50109039468567929 ) ) ;
#85950=( BOUNDED_SURFACE ( )  B_SPLINE_SURFACE ( 3, 2, ( 
 ( #120360, #168840, #90998, #31341, #105201, #139495, #14173, #182053, #108165, #977, #62653, #138507, #151710, #200189, #124330, #13203, #45514, #121352, #74866, #184032, #61658, #75842, #152684, #104210, #166888, #123326, #89034, #165891, #122341, #185020, #136528, #46505, #186028, #150725, #59680, #137519, #12224, #29367, #199200, #60668, #73887, #198209, #43536, #183045, #107169, #189013, #3961, #2979, #144466, #110161, #94988, #158641, #113131, #78819, #64658, #1986, #63666, #67628, #142483, #19156, #50488, #189995, #48507, #36286, #5951, #174821, #97942, #20132, #96961, #49488, #111150, #129288, #81777, #143463, #159634, #21130, #188017, #171840, #80805, #4948, #79824, #82785, #35306, #66632, #47510, #33327, #140498, #125339, #170846, #141495, #112148, #109166, #65641, #128296, #187037, #32337, #93990, #155670, #17166, #156673, #18168, #126320, #173840, #172840, #127300, #51470, #34319, #95982, #157666, #114118, #175820, #37293, #98952, #25155, #100955, #146459, #145463, #147484, #102968, #148484, #9975, #133301, #194992, #101972, #160642, #6945, #178828, #164653, #130281, #71635, #162640, #161642, #179837, #190983, #69635, #24146, #38302, #10971, #8974, #22133, #68624, #55463, #177828, #118147, #191975, #41307, #85798, #83784, #56469, #26148, #87790, #117134, #176830, #86797, #72644, #99956, #132309, #7952, #23136, #70643, #149475, #194001, #39298, #52460, #53462, #40298, #115138, #84781, #163653, #131301, #192990, #54468, #116138, #183797, #89791, #105949, #60433, #74629, #167634, #121114, #14943, #58457, #73647, #196005, #181816, #75605, #90769, #151475, #31108, #196991, #43295, #45284, #199962, #165649, #12965, #88794, #150487, #154444, #29131, #152453, #137284, #76603, #135318, #123098, #92756, #61427, #184784, #106937, #168610, #136295, #197971, #15938, #30110, #91750, #46270, #107925, #59441, #120125, #13938, #153445, #166650, #169610, #122107, #138280, #134319, #104963, #27147, #11982, #182808, #44291, #198966, #57478, #119150, #180832, #28151, #42309, #103970, #4714, #2744, #141255, #155439, #97708, #19903, #174594, #64421, #188775, #157430, #80569, #142244, #62416, #33095, #108931, #77597, #16929, #65406, #159399, #189767, #126090, #66403, #36059, #3729, #744, #156432, #78582, #127067, #50258, #124088, #128065, #94751, #139268, #49256, #51239, #170611, #186799, #185787, #111914, #47274, #140256, #173602, #35071, #112900, #109925, #32101, #96726, #93758, #158414, #48270, #81545, #171607, #1748, #143231, #63426, #17932, #172600, #125101, #187786, #79586, #110914, #34086, #95745, #18924, #84546, #21900, #54235, #101731, #114900, #116898, #176594, #6711, #144234, #53224, #52227, #24916, #130041, #99724, #115906, #70404, #23904, #68389, #7711, #161408, #86562, #98717, #146224, #178591, #85558, #132072, #147243, #129052, #190753, #5718, #37058, #193761, #191740, #38068, #22900, #160411, #82552, #177596, #55229, #69395, #40054, #131063, #192752, #20894, #163419, #39064, #67396, #100721, #83550, #113883, #162402, #8735, #175581, #145229, #51880, #32746, #18575, #156079, #17575, #21545, #96381, #173248, #142884, #143884, #2393, #190404, #160058, #67049, #113539, #112552, #50894, #3384, #65059, #98359, #174247, #97362, #128707, #175233, #141893, #125742, #34723, #159048, #33732, #36698, #189419, #35715, #83205, #187442, #94398, #79236, #124750, #95393, #4366, #1390, #158068, #20542, #140907, #63071, #186446, #47922, #109576, #171259, #64072, #82191, #111564, #157079, #48910, #19559, #110564, #5365, #172245, #80222, #126716, #188420, #49897, #81203, #66049, #127717, #84196, #102384, #54879, #115560, #133718, #144880, #23551, #178242, #192403, #165064, #101366, #68042, #99372, #9387, #131722, #72044, #145876, #195410, #116553, #37710, #148897, #56888, #118562, #71053, #130709, #40715, #26558, #53885, #86211, #162055, #177247, #24562, #179249, #39703, #193404, #6362, #7359, #132719 ),
 ( #163055, #161055, #52868, #87215, #180252, #38719, #147901, #100377, #194407, #41722, #146887, #103386, #8379, #85199, #10387, #55877, #114539, #22550, #117550, #129694, #69044, #164072, #25571, #70054, #191391, #176239, #167051, #121517, #135722, #108335, #44693, #11391, #42716, #152850, #75026, #15345, #89202, #77001, #198373, #181240, #92160, #138673, #153, #14344, #74051, #184199, #170015, #197393, #29528, #105364, #58858, #168031, #122509, #59850, #136691, #88201, #150895, #76010, #73061, #149885, #106347, #137685, #12389, #30509, #61822, #199370, #43702, #183212, #60834, #28552, #91161, #45681, #169005, #120525, #27562, #134733, #182218, #107332, #153847, #90189, #185185, #151872, #13362, #123492, #46675, #119557, #196415, #104378, #166061, #57885, #3631, #156334, #33000, #35963, #172503, #2650, #97610, #78484, #187692, #66306, #50158, #81448, #34978, #185683, #47173, #62315, #155344, #19807, #48171, #94654, #186700, #16833, #139168, #18829, #143135, #171511, #158319, #49162, #17834, #174496, #111817, #33990, #127966, #141161, #108832, #15839, #32002, #110821, #170512, #93659, #189669, #79492, #64327, #95646, #80474, #51142, #125994, #109828, #157334, #142147, #4614, #65310, #126970, #188678, #173505, #96631, #645, #112803, #140157, #77498, #1649, #123985, #63327, #125005, #22807, #150897, #58861, #162311, #82450, #37973, #160314, #8639, #23812, #144138, #12391, #176497, #120527, #130967, #74053, #190658, #68296, #182220, #85462, #5620, #21804, #147151, #70311, #135724, #191647, #197395, #131980, #52134, #193665, #129947, #55136, #53126, #20795, #166063, #43704, #99631, #54140, #116806, #146131, #113791, #67299, #104380, #159299, #114804, #192657, #145134, #178498, #128958, #161313, #175486, #84453, #7617, #36958, #69301, #98620, #83456, #115814, #177504, #42718, #38973, #100630, #6617, #27564, #89204, #187203, #168033, #77003, #155836, #139659, #171014, #124505, #75028, #136694, #151874, #44695, #109332, #137687, #122511, #76012, #106349, #28554, #108337, #32505, #60836, #47682, #138675, #107334, #63833, #1147, #123494, #17333, #30511, #198375, #125506, #121519, #155, #59852, #183214, #78989, #45683, #169007, #61824, #170018, #140663, #92163, #199372, #46678, #184201, #94157, #153849, #15347, #29530, #105366, #2155, #167053, #185187, #91163, #31508, #90191, #62822, #13364, #186200, #152852, #14347, #93161, #154846, #16343, #77992, #65809, #19328, #49657, #172007, #51639, #114300, #4130, #191162, #20299, #50656, #7121, #82965, #66804, #160822, #174007, #18337, #68803, #64825, #81947, #141660, #3152, #99132, #189183, #112317, #143639, #113303, #22310, #35478, #80976, #190163, #127478, #176002, #97127, #158811, #126487, #130462, #52635, #145641, #5122, #159813, #128467, #174994, #36459, #33495, #98116, #79992, #48674, #188185, #21308, #110326, #83961, #144642, #37471, #95154, #6125, #156842, #67808, #111321, #129463, #173011, #34490, #96148, #157837, #142651, #163830, #42480, #23311, #101126, #150659, #118322, #177009, #54634, #180015, #41482, #165825, #24321, #27322, #56649, #84955, #103147, #162812, #195168, #85970, #53640, #196180, #88969, #70814, #86973, #164828, #179005, #146637, #100135, #134493, #12157, #147660, #25332, #177998, #26324, #73822, #194172, #104143, #55636, #9147, #115317, #132483, #8130, #192160, #117309, #40473, #87964, #102145, #148660, #38478, #10148, #71808, #161816, #69808, #149652, #11150, #131475, #116309, #193162, #39465, #133476, #72824, #57652, #119318, #181005, #108095, #28324, #197162, #170779, #58628, #120294, #181987, #43469, #169780, #45449, #90931, #89963, #91921, #47444, #92924, #154610, #77763, #139429, #46436, #105137, #151643, #123260, #109100, #74800, #16105, #107103, #106117, #124264, #135492, #14108, #168773, #182979, #155604, #153613, #166823, #13138, #200123, #122274, #62586, #136463, #185959, #30275, #198143, #912, #32269, #93926, #61592 ),
 ( #184952, #59613, #121286, #15109, #31273, #44463, #17100, #167801, #29301, #152617, #76770, #75775, #137453, #138442, #183962, #199132, #60599, #18104, #140429, #126258, #20070, #35243, #34257, #175753, #141429, #187955, #189932, #144403, #110098, #95916, #33265, #94924, #98887, #173777, #156609, #96897, #52397, #50428, #67565, #37230, #5889, #129223, #51407, #128235, #80741, #142419, #160581, #113067, #174759, #190920, #114056, #19092, #2916, #112087, #36225, #111086, #78752, #64594, #81714, #157601, #49425, #158581, #97877, #143399, #127237, #1919, #172776, #4888, #63598, #125274, #66570, #159568, #3898, #21066, #186971, #82722, #65578, #48441, #171776, #188951, #79758, #8904, #102903, #146395, #161578, #83721, #69570, #163585, #178761, #177762, #119087, #84717, #131236, #133233, #87725, #53396, #39231, #176766, #38238, #42244, #117065, #99893, #40226, #195940, #193932, #10906, #180769, #149410, #72579, #194925, #71568, #24074, #85729, #103905, #56400, #118082, #134253, #57414, #162571, #7884, #55395, #179772, #54402, #22070, #9908, #41241, #145400, #192924, #115074, #23071, #6882, #116074, #25086, #68560, #101903, #164587, #100887, #130217, #191912, #147417, #70572, #132240, #86728, #26081, #148413, #121049, #120062, #122043, #77529, #123032, #184718, #107856, #169541, #76539, #135256, #181750, #153376, #139201, #104898, #46202, #75542, #136233, #154377, #165586, #44229, #198903, #12901, #185714, #183733, #88730, #43232, #30045, #152389, #92689, #166587, #15871, #137216, #58396, #31040, #676, #62347, #91686, #151413, #61361, #182744, #196928, #27084, #28087, #14878, #47205, #124017, #29067, #150425, #11920, #168547, #73584, #105886, #89727, #138215, #199897, #74565, #197907, #167573, #59377, #60371, #90706, #13875, #45219, #106874, #35006, #93691, #171541, #96661, #158348, #82481, #141191, #144165, #173537, #1680, #19837, #79521, #111847, #2680, #170543, #112833, #5650, #187722, #3662, #81478, #95679, #63358, #16863, #51173, #67327, #64357, #80505, #94684, #143165, #128989, #110851, #159328, #172535, #126026, #32034, #49193, #125035, #190687, #34021, #157365, #4645, #18859, #142178, #108864, #65340, #127000, #155374, #33029, #188708, #20824, #66336, #174525, #127997, #78514, #140188, #186731, #48202, #35992, #50190, #189700, #97639, #109856, #156363, #17866, #117845, #7645, #194694, #23840, #54170, #10675, #86498, #70340, #164359, #177532, #21833, #72339, #68325, #85489, #145163, #6647, #102674, #192687, #115843, #147178, #55163, #25854, #39001, #22835, #193694, #69329, #179538, #100657, #162339, #129975, #134014, #56164, #149186, #8667, #163353, #132007, #116833, #178524, #36988, #53155, #41007, #39991, #191675, #87498, #52162, #113819, #101662, #38004, #148182, #175514, #99659, #24849, #130995, #161343, #9676, #71341, #133004, #98650, #160344, #114834, #83485, #176528, #84482, #146159, #44980, #119837, #137973, #169296, #106640, #151182, #167338, #121803, #136003, #28835, #182508, #76295, #181522, #135025, #57178, #43001, #136979, #152158, #12670, #92451, #58170, #104668, #168313, #61121, #26849, #74337, #150185, #11686, #15631, #90476, #73352, #13641, #30802, #75308, #184485, #154139, #122795, #45964, #29809, #91445, #197674, #59139, #77288, #153133, #14636, #107618, #195706, #120809, #166353, #198668, #199655, #27851, #118855, #183496, #180538, #42012, #89492, #88490, #196700, #103676, #43988, #60135, #165355, #105649, #111606, #31794, #437, #174285, #62112, #123775, #185474, #46964, #173291, #48950, #94439, #93443, #95435, #50935, #96422, #158108, #81242, #142923, #49941, #108623, #155130, #126757, #112593, #78271, #19600, #110603, #109617, #127756, #138958, #17619, #172285, #186489, #159087, #157119, #170301, #16623, #3423, #125782, #66090, #34765, #4405, #189457, #139944, #1434, #63112, #124790, #35755, #171301, #156120, #32787, #47965, #79278, #141932, #97400, #140948, #20582 ),
 ( #2435, #64117, #187484, #33775, #18615, #80262, #65099, #188460, #194449, #39747, #101410, #24606, #86254, #193447, #51920, #36739, #70096, #55920, #21586, #163102, #192445, #52909, #71095, #82234, #161097, #115602, #129735, #102429, #38761, #5405, #98403, #146934, #69086, #9430, #83244, #132762, #53927, #175273, #147944, #117595, #179296, #8424, #68083, #178284, #164116, #191432, #23596, #99415, #114585, #162100, #116595, #177291, #130753, #143924, #144920, #131765, #67089, #128748, #100419, #54923, #6402, #40760, #190445, #113579, #37754, #85243, #160099, #22592, #176282, #84240, #145919, #7402, #165112, #87258, #73110, #167097, #182267, #181286, #122559, #88247, #134780, #136738, #91206, #56935, #42764, #180299, #41767, #45731, #120573, #103432, #43750, #199418, #197440, #14393, #184249, #152896, #76059, #198422, #151919, #166109, #58906, #12437, #106396, #149932, #26604, #148943, #196462, #28598, #105413, #104426, #107383, #11439, #57932, #59897, #137734, #118609, #27611, #119603, #89251, #25614, #90236, #150943, #13408, #60882, #75072, #10433, #72091, #133765, #195460, #121565, #183259, #74099, #135769, #44740, #168078, #29575, #37263, #98921, #109380, #93208, #2201, #67599, #1194, #22103, #159602, #21100, #6915, #154893, #203, #185235, #92213, #62871, #110372, #160613, #140711, #144436, #61872, #30562, #68593, #153899, #15394, #77051, #138722, #5922, #79036, #124552, #123542, #125553, #83753, #129258, #190953, #114088, #175789, #82756, #46727, #108389, #52430, #145432, #170066, #130249, #63882, #139707, #191944, #169055, #47727, #187250, #16391, #53429, #48719, #31557, #78038, #33541, #155883, #186249, #171060, #32550, #172054, #94203, #17380, #97911, #27114, #41272, #100920, #10937, #135284, #162605, #56434, #132274, #24109, #194957, #149441, #86763, #163618, #115106, #177794, #102934, #38271, #176798, #133266, #164619, #39264, #57444, #88760, #26113, #70607, #148446, #55428, #117099, #9941, #118114, #150453, #178794, #85763, #179803, #193965, #42277, #40263, #101936, #192957, #196956, #119117, #11949, #25119, #87756, #72610, #134284, #195972, #99925, #71600, #146428, #161610, #54436, #180798, #23104, #73613, #103935, #165615, #84750, #7918, #69602, #131269, #116106, #147450, #8938, #43260, #108896, #75570, #16894, #30074, #170575, #89755, #167599, #78545, #184749, #104928, #121078, #46234, #107888, #32066, #90733, #93722, #123063, #151441, #169575, #29094, #61391, #152416, #120091, #62380, #155404, #137246, #153409, #31072, #45249, #12928, #166614, #708, #140220, #13904, #91715, #44256, #92720, #58424, #60399, #181779, #122071, #198931, #28117, #183763, #74592, #136260, #106903, #168576, #154409, #14907, #76569, #197935, #138244, #199928, #59404, #182772, #15903, #105913, #77561, #124050, #139233, #185749, #47237, #48233, #141221, #5684, #34053, #18891, #172567, #2712, #125066, #4678, #67360, #157398, #144198, #173569, #3694, #160376, #36024, #19870, #113851, #127033, #171572, #21867, #17898, #35038, #94716, #156394, #52193, #64389, #190720, #111879, #79552, #129019, #175547, #37022, #128030, #187754, #97673, #83517, #49224, #143197, #80537, #110882, #81510, #159362, #96692, #50225, #1713, #126057, #189732, #186763, #63389, #66370, #51205, #95710, #98683, #109888, #112866, #142211, #158381, #174557, #65373, #20859, #188740, #82516, #33061, #84512, #6677, #192717, #86528, #101693, #100686, #42043, #7675, #54201, #56194, #10707, #176559, #162368, #99690, #161374, #165387, #40020, #22865, #163382, #118885, #116863, #134044, #103707, #72370, #195737, #117877, #194724, #147208, #8699, #26880, #179567, #41037, #57210, #180569, #85520, #69359, #178554, #102703, #177562, #145194, #133034, #164391, #68355, #131028, #38034, #146190, #130006, #39031, #148212, #191705, #24879, #25884, #115873, #53189, #114864, #23869, #70369, #132037, #193726, #87529, #55194, #9706, #71370, #149216, #469 ),
 ( #73383, #44022, #119867, #88523, #27881, #76328, #108655, #62143, #152189, #77322, #185505, #91478, #90507, #60166, #153166, #123807, #28867, #59172, #29841, #105683, #15663, #13673, #75340, #166385, #170333, #30835, #150219, #167370, #122827, #11716, #14667, #138005, #135055, #137010, #181552, #196731, #89523, #199689, #58199, #46996, #198700, #138990, #43031, #61154, #104697, #121835, #151212, #184516, #45996, #12700, #74366, #183529, #136032, #45013, #197706, #120841, #182540, #106672, #107651, #168345, #169328, #92483, #154172, #5438, #64149, #67122, #96453, #124822, #81274, #2467, #34798, #125813, #93476, #35788, #128780, #110637, #126789, #142956, #18648, #186522, #139976, #174318, #190480, #187516, #3455, #17650, #158140, #51952, #33807, #82266, #95467, #48982, #155163, #172318, #47996, #113612, #157153, #80294, #19632, #141966, #65132, #31826, #188495, #49974, #16655, #94471, #111638, #143958, #66124, #97435, #50967, #1465, #63143, #78303, #171332, #159120, #173323, #4436, #127789, #32820, #109650, #189489, #20616, #112626, #156152, #79310, #140979, #133799, #9466, #193479, #87291, #100451, #144952, #195490, #191463, #8455, #68115, #129767, #25646, #115634, #161129, #178317, #72125, #177323, #148975, #38794, #145953, #98437, #192476, #52941, #56965, #130784, #162131, #163135, #23627, #53959, #175306, #131800, #85275, #36772, #37785, #146966, #10464, #71129, #40792, #194482, #6433, #114615, #21620, #176315, #179328, #7434, #70128, #69118, #99449, #160132, #39780, #102461, #54956, #117630, #116628, #101444, #83277, #132795, #24638, #22625, #86287, #84272, #147977, #55954, #164149, #11472, #73143, #169085, #58937, #120606, #90266, #121594, #92243, #182300, #89283, #59926, #74129, #45760, #43780, #105445, #196493, #138751, #60913, #180330, #197471, #152924, #233, #183289, #44771, #103465, #135800, #149966, #118638, #57963, #106424, #41798, #30591, #167129, #107412, #15423, #168105, #165144, #28629, #119634, #29602, #91234, #26635, #153929, #151949, #77082, #13438, #88278, #134813, #27643, #181317, #14421, #42796, #104458, #76085, #137761, #166141, #150974, #12468, #199445, #75102, #122589, #136769, #184277, #198455, #123571, #65883, #158886, #140739, #156918, #173086, #48748, #16419, #170092, #4205, #35553, #32580, #33570, #80064, #111401, #186277, #127557, #97200, #34565, #17409, #95232, #188259, #2228, #18415, #110401, #142725, #47756, #1223, #185266, #109410, #3224, #141734, #79066, #20376, #124581, #171089, #96221, #189258, #93236, #63910, #78066, #139734, #82023, #64898, #62901, #126559, #143719, #49733, #50734, #61900, #112393, #174084, #157910, #19400, #125580, #187278, #46758, #81049, #108416, #31586, #154921, #172083, #94233, #155914, #101201, #37543, #55715, #193240, #54713, #40555, #129533, #36533, #21380, #128541, #99207, #146715, #132559, #177084, #178075, #98189, #66880, #102224, #190238, #51715, #113378, #175068, #39542, #115396, #160895, #159892, #161892, #117387, #162891, #24400, #147738, #9225, #116385, #83039, #144714, #86049, #114371, #84037, #70892, #23388, #176075, #194248, #5198, #145716, #38555, #52707, #25409, #85034, #6200, #67880, #69886, #192239, #179086, #191233, #163913, #100212, #22387, #87051, #7197, #68881, #131555, #130541, #53719, #8211, #149727, #120367, #119397, #11228, #58697, #151717, #12232, #89042, #148736, #72902, #105209, #133554, #71884, #28396, #43543, #195245, #106191, #181080, #152691, #73894, #167875, #180093, #134571, #14180, #166896, #56729, #196258, #90035, #13210, #29374, #57727, #91005, #74873, #41561, #136535, #42555, #182060, #104218, #10224, #118399, #103224, #197236, #198216, #44536, #59688, #165899, #27397, #164906, #26400, #135564, #121359, #150732, #183052, #88039, #131200, #179737, #192890, #99860, #52361, #146362, #22035, #149376, #84682, #116040, #117031, #69536, #7849, #10872, #85695, #177729, #129187, #191877, #100854, #41207 ),
 ( #132206, #194890, #54368, #71533, #162536, #39198, #87691, #163551, #147381, #102868, #24040, #98851, #190885, #145365, #8870, #83687, #6847, #164553, #70537, #193897, #55361, #178726, #26046, #40188, #161544, #101868, #25051, #56364, #86694, #148378, #68526, #114018, #133199, #175715, #9873, #118047, #37194, #160546, #130181, #53361, #115038, #176731, #38204, #23037, #60337, #92657, #184687, #136199, #61330, #169508, #75509, #195905, #151379, #73550, #12869, #89693, #154346, #29035, #59342, #72542, #135223, #44194, #123001, #106843, #138183, #91654, #42211, #103871, #119053, #11887, #76507, #104864, #74534, #43197, #196895, #57380, #137182, #199866, #28052, #14844, #105853, #197874, #31008, #168518, #90675, #46171, #121011, #165552, #134219, #88695, #167540, #27049, #150391, #107824, #182709, #152357, #13842, #198870, #180735, #122011, #166553, #183702, #45189, #58362, #30016, #153343, #120029, #181714, #176844, #36299, #5963, #99970, #83796, #97954, #116151, #127314, #67641, #160654, #174834, #147497, #145476, #50499, #81789, #191987, #114131, #54481, #128308, #177842, #37305, #20144, #131314, #39310, #100969, #53474, #113144, #23150, #8988, #159646, #68637, #144479, #21142, #6957, #161654, #98964, #175832, #189025, #190008, #115151, #112163, #173852, #130293, #38315, #51482, #69648, #162654, #84794, #82797, #22146, #146473, #129300, #7965, #193004, #24160, #190996, #66646, #35318, #52472, #85811, #96972, #158653, #143476, #4960, #118160, #181829, #136309, #101986, #87803, #25169, #86811, #90781, #165662, #89806, #40310, #163667, #117147, #9988, #74643, #102981, #149489, #41321, #71648, #194014, #73660, #197984, #26162, #12979, #42322, #72658, #29144, #104976, #88807, #182822, #196017, #148497, #152465, #133315, #103983, #195004, #56482, #121127, #10985, #134333, #27160, #135332, #44304, #57493, #164666, #11997, #119162, #59454, #180845, #105963, #120138, #70656, #167648, #132322, #150500, #166663, #55477, #197005, #58471, #178842, #43308, #179850, #28164, #151488, #1761, #34100, #126104, #77610, #2758, #110927, #16942, #137296, #92769, #14955, #63439, #78596, #198978, #64434, #31121, #172613, #185800, #187800, #45297, #123111, #95758, #140269, #60445, #76615, #125115, #186813, #49269, #46282, #13951, #48283, #106949, #109938, #184796, #171620, #107938, #75617, #17945, #122120, #154459, #108944, #33108, #758, #168622, #183809, #156446, #30122, #169624, #47288, #199974, #94764, #91763, #15951, #153457, #139281, #62429, #138293, #124101, #61439, #170625, #32114, #93771, #79599, #155452, #141268, #177609, #113896, #144245, #39077, #19914, #129063, #7723, #191753, #22912, #80583, #51251, #98729, #84558, #190764, #130053, #50270, #18938, #192764, #142257, #3741, #65418, #127079, #53236, #67408, #112911, #111928, #175594, #69409, #114912, #176606, #99736, #161420, #21912, #96737, #5729, #6723, #66414, #36071, #38080, #37070, #128076, #146236, #157443, #97720, #52239, #4725, #188787, #160423, #173614, #35084, #83563, #145242, #131075, #158426, #54247, #68401, #81556, #115919, #143242, #189779, #174605, #159410, #20905, #82563, #86575, #42090, #117925, #148259, #180617, #135101, #72418, #149262, #100734, #163432, #26929, #23917, #162415, #118932, #150269, #24930, #43076, #74413, #11763, #56244, #134095, #88571, #41087, #195785, #87575, #181599, #9752, #40067, #85571, #71416, #103755, #57258, #179614, #197753, #133080, #194770, #73430, #166434, #132085, #102750, #55243, #116911, #120889, #165434, #178604, #196777, #136079, #58245, #89572, #59220, #27929, #151258, #119913, #104743, #164438, #25932, #182588, #12748, #147257, #8748, #70418, #10754, #193774, #101744, #140027, #76379, #94520, #31875, #93529, #79359, #168394, #75387, #60214, #109701, #199737, #186572, #15712, #46044, #2517, #78353, #62192, #156202, #169378, #13721, #64197, #121884, #77372, #137059, #198749, #17702, #184563, #107699, #139040 ),
 ( #153214, #122875, #16703, #520, #14719, #32870, #44071, #30886, #123856, #91527, #125864, #185554, #167418, #183577, #108705, #92533, #171383, #45062, #141030, #154222, #106720, #48045, #105731, #28914, #170384, #29889, #1516, #90554, #138056, #47048, #61203, #155214, #63193, #124873, #152236, #35836, #187564, #50023, #113660, #110686, #49031, #5488, #36822, #111688, #129815, #161179, #98488, #143005, #159168, #175354, #127835, #20663, #174366, #68163, #173375, #126839, #172366, #34845, #128828, #144007, #4483, #84322, #96500, #158190, #160181, #52991, #18696, #66173, #142015, #3504, #7484, #82317, #65180, #67171, #22675, #190527, #176365, #146001, #114669, #37838, #21671, #83325, #189541, #51013, #69168, #145002, #6483, #99498, #33856, #112674, #19680, #52001, #191514, #81322, #95516, #157202, #80343, #188545, #97482, #164195, #23677, #85325, #181364, #71178, #132842, #102511, #133849, #104508, #194530, #101494, #72175, #86336, #58011, #56001, #119681, #180378, #130835, #42843, #192526, #9512, #165191, #12514, #195539, #57013, #115683, #148023, #162179, #54009, #70179, #118686, #151023, #166189, #117679, #27690, #89331, #41848, #177371, #179376, #131847, #103515, #26686, #38843, #100500, #40838, #147017, #25693, #8502, #193530, #39828, #55004, #88326, #116674, #178364, #150017, #11522, #163183, #24687, #87338, #73192, #149024, #134863, #10512, #196541, #168153, #135848, #78113, #171137, #152973, #169135, #185312, #60962, #28677, #182350, #16464, #47804, #44819, #45808, #59975, #77131, #32626, #76134, #124627, #137812, #106474, #197517, #91282, #167178, #94280, #29650, #122636, #61950, #14472, #199496, #155958, #30640, #184326, #74178, #136820, #107459, #186322, #108462, #139782, #93283, #43828, #105492, #120652, #13484, #1270, #92293, #153977, #15474, #75149, #58985, #138800, #62947, #281, #109454, #123617, #46803, #90312, #170139, #31634, #151998, #154968, #198504, #121642, #183337, #117185, #80109, #64943, #131351, #85845, #48794, #34608, #172129, #33615, #40346, #115187, #95278, #38350, #194051, #192026, #9023, #178879, #147535, #70692, #193039, #69684, #19444, #81092, #102021, #54517, #116189, #132359, #55514, #157953, #141777, #53510, #177878, #49781, #17455, #8000, #39346, #79111, #3271, #110448, #156961, #140784, #111446, #161692, #2273, #176880, #101005, #18458, #63956, #125625, #187323, #126602, #188304, #173133, #162689, #130329, #96267, #142770, #100005, #4251, #24195, #65930, #23187, #84830, #146510, #103019, #150533, #13013, #72693, #42356, #136344, #120172, #134368, #152497, #163704, #104018, #197039, #11020, #183842, #181863, #86848, #118196, #28199, #12033, #90814, #164702, #13985, #73696, #56518, #167682, #75651, #137329, #89841, #149524, #59488, #45331, #196052, #105012, #180881, #57527, #43342, #198019, #135368, #58506, #25206, #26198, #151522, #148533, #10024, #166696, #74677, #87837, #105995, #199010, #121163, #119196, #182856, #44338, #165697, #29178, #60478, #122153, #27195, #88841, #71684, #133350, #195041, #179888, #41355, #138327, #123145, #30155, #793, #48318, #34133, #78631, #79634, #200008, #168655, #142294, #91798, #153492, #14988, #76649, #141303, #16977, #62465, #61474, #63475, #18971, #64471, #126138, #49303, #110961, #171653, #46318, #93806, #156479, #15987, #185837, #2792, #125150, #77645, #95792, #106981, #47324, #140306, #154492, #127114, #186849, #184832, #107973, #33142, #155485, #157479, #169660, #80617, #1797, #31156, #172645, #3774, #65451, #94800, #92805, #187833, #188820, #139314, #109973, #124138, #108980, #17980, #170660, #32148, #98762, #50303, #112945, #176640, #173650, #111960, #68436, #99770, #174638, #192798, #23949, #161455, #5765, #21947, #38116, #190797, #83596, #37103, #131110, #36103, #189813, #35118, #97755, #191788, #6757, #67440, #147290, #159443, #20938, #22946, #115953, #81589, #129097, #4759, #66447, #70450, #145276, #128108 ) ),
 .UNSPECIFIED., .T., .F., .T. ) 
 B_SPLINE_SURFACE_WITH_KNOTS ( ( 4, 3, 4 ),
 ( 3, 2, 2, 2, 2, 2, 2, 2, 2, 2, 2, 2, 2, 2, 2, 2, 2, 2, 2, 2, 2, 2, 2, 2, 2, 2, 2, 2, 2, 2, 2, 2, 2, 2, 2, 2, 2, 2, 2, 2, 2, 2, 2, 2, 2, 2, 2, 2, 2, 2, 2, 2, 2, 2, 2, 2, 2, 2, 2, 2, 2, 2, 2, 2, 2, 2, 2, 2, 2, 2, 2, 2, 2, 2, 2, 2, 2, 2, 2, 2, 2, 2, 2, 2, 2, 2, 2, 2, 2, 2, 2, 2, 2, 2, 2, 2, 2, 2, 2, 2, 2, 2, 2, 2, 2, 2, 2, 2, 2, 2, 2, 2, 2, 2, 2, 2, 2, 2, 2, 2, 2, 2, 2, 2, 2, 2, 2, 2, 2, 2, 2, 2, 2, 2, 2, 2, 2, 2, 2, 2, 2, 2, 2, 2, 2, 2, 2, 2, 2, 2, 2, 2, 2, 2, 2, 2, 2, 2, 2, 2, 2, 2, 2, 2, 2, 2, 2, 2, 2, 2, 2, 2, 2, 2, 2, 2, 2, 2, 2, 2, 2, 2, 2, 2, 2, 2, 2, 2, 2, 2, 2, 2, 2, 2, 2, 2, 2, 2, 2, 2, 2, 2, 2, 2, 2, 2, 2, 2, 2, 2, 2, 2, 2, 2, 2, 2, 2, 2, 2, 2, 2, 2, 2, 2, 2, 2, 2, 2, 3 ),
 ( 0.000000000000000000, 0.5000000000000000000, 1.000000000000000000 ),
 ( 0.000000000000000000, 0.004385964912280701511, 0.008771929824561403022, 0.01315789473684210453, 0.01754385964912280604, 0.02192982456140350755, 0.02631578947368420907, 0.03070175438596491058, 0.03508771929824561209, 0.03947368421052631360, 0.04385964912280701511, 0.04824561403508771662, 0.05263157894736841813, 0.05701754385964911964, 0.06140350877192982115, 0.06578947368421052266, 0.07017543859649122417, 0.07456140350877192569, 0.07894736842105262720, 0.08333333333333332871, 0.08771929824561403022, 0.09210526315789473173, 0.09649122807017543324, 0.1008771929824561348, 0.1052631578947368363, 0.1096491228070175378, 0.1140350877192982393, 0.1184210526315789408, 0.1228070175438596423, 0.1271929824561403577, 0.1315789473684210453, 0.1359649122807017607, 0.1403508771929824483, 0.1447368421052631637, 0.1491228070175438514, 0.1535087719298245668, 0.1578947368421052544, 0.1622807017543859698, 0.1666666666666666574, 0.1710526315789473728, 0.1754385964912280604, 0.1798245614035087758, 0.1842105263157894635, 0.1885964912280701788, 0.1929824561403508665, 0.1973684210526315819, 0.2017543859649122695, 0.2061403508771929849, 0.2105263157894736725, 0.2149122807017543879, 0.2192982456140350755, 0.2236842105263157909, 0.2280701754385964786, 0.2324561403508771940, 0.2368421052631578816, 0.2412280701754385970, 0.2456140350877192846, 0.2500000000000000000, 0.2543859649122807154, 0.2587719298245614308, 0.2631578947368420907, 0.2675438596491228060, 0.2719298245614035214, 0.2763157894736842368, 0.2807017543859648967, 0.2850877192982456121, 0.2894736842105263275, 0.2938596491228070429, 0.2982456140350877027, 0.3026315789473684181, 0.3070175438596491335, 0.3114035087719298489, 0.3157894736842105088, 0.3201754385964912242, 0.3245614035087719396, 0.3289473684210526550, 0.3333333333333333148, 0.3377192982456140302, 0.3421052631578947456, 0.3464912280701754610, 0.3508771929824561209, 0.3552631578947368363, 0.3596491228070175517, 0.3640350877192982670, 0.3684210526315789269, 0.3728070175438596423, 0.3771929824561403577, 0.3815789473684210731, 0.3859649122807017330, 0.3903508771929824483, 0.3947368421052631637, 0.3991228070175438791, 0.4035087719298245390, 0.4078947368421052544, 0.4122807017543859698, 0.4166666666666666852, 0.4210526315789473450, 0.4254385964912280604, 0.4298245614035087758, 0.4342105263157894912, 0.4385964912280701511, 0.4429824561403508665, 0.4473684210526315819, 0.4517543859649122973, 0.4561403508771929571, 0.4605263157894736725, 0.4649122807017543879, 0.4692982456140351033, 0.4736842105263157632, 0.4780701754385964786, 0.4824561403508771940, 0.4868421052631579093, 0.4912280701754385692, 0.4956140350877192846, 0.5000000000000000000, 0.5043859649122807154, 0.5087719298245614308, 0.5131578947368421462, 0.5175438596491228616, 0.5219298245614034659, 0.5263157894736841813, 0.5307017543859648967, 0.5350877192982456121, 0.5394736842105263275, 0.5438596491228070429, 0.5482456140350877583, 0.5526315789473684736, 0.5570175438596490780, 0.5614035087719297934, 0.5657894736842105088, 0.5701754385964912242, 0.5745614035087719396, 0.5789473684210526550, 0.5833333333333333703, 0.5877192982456140857, 0.5921052631578946901, 0.5964912280701754055, 0.6008771929824561209, 0.6052631578947368363, 0.6096491228070175517, 0.6140350877192982670, 0.6184210526315789824, 0.6228070175438596978, 0.6271929824561403022, 0.6315789473684210176, 0.6359649122807017330, 0.6403508771929824483, 0.6447368421052631637, 0.6491228070175438791, 0.6535087719298245945, 0.6578947368421053099, 0.6622807017543859143, 0.6666666666666666297, 0.6710526315789473450, 0.6754385964912280604, 0.6798245614035087758, 0.6842105263157894912, 0.6885964912280702066, 0.6929824561403509220, 0.6973684210526315264, 0.7017543859649122417, 0.7061403508771929571, 0.7105263157894736725, 0.7149122807017543879, 0.7192982456140351033, 0.7236842105263158187, 0.7280701754385965341, 0.7324561403508771384, 0.7368421052631578538, 0.7412280701754385692, 0.7456140350877192846, 0.7500000000000000000, 0.7543859649122807154, 0.7587719298245614308, 0.7631578947368421462, 0.7675438596491228616, 0.7719298245614034659, 0.7763157894736841813, 0.7807017543859648967, 0.7850877192982456121, 0.7894736842105263275, 0.7938596491228070429, 0.7982456140350877583, 0.8026315789473684736, 0.8070175438596490780, 0.8114035087719297934, 0.8157894736842105088, 0.8201754385964912242, 0.8245614035087719396, 0.8289473684210526550, 0.8333333333333333703, 0.8377192982456140857, 0.8421052631578946901, 0.8464912280701754055, 0.8508771929824561209, 0.8552631578947368363, 0.8596491228070175517, 0.8640350877192982670, 0.8684210526315789824, 0.8728070175438596978, 0.8771929824561403022, 0.8815789473684210176, 0.8859649122807017330, 0.8903508771929824483, 0.8947368421052631637, 0.8991228070175438791, 0.9035087719298245945, 0.9078947368421053099, 0.9122807017543859143, 0.9166666666666666297, 0.9210526315789473450, 0.9254385964912280604, 0.9298245614035087758, 0.9342105263157894912, 0.9385964912280702066, 0.9429824561403509220, 0.9473684210526315264, 0.9517543859649122417, 0.9561403508771929571, 0.9605263157894736725, 0.9649122807017543879, 0.9692982456140351033, 0.9736842105263158187, 0.9780701754385965341, 0.9824561403508771384, 0.9868421052631578538, 0.9912280701754385692, 0.9956140350877192846, 1.000000000000000000 ),
 .UNSPECIFIED. ) 
 GEOMETRIC_REPRESENTATION_ITEM ( )  RATIONAL_B_SPLINE_SURFACE ( (
 ( 1.000000000000000000, 0.9659258262890683122, 1.000000000000000000, 0.9659258262890683122, 1.000000000000000000, 0.9659258262890683122, 1.000000000000000000, 0.9659258262890683122, 1.000000000000000000, 0.9659258262890683122, 1.000000000000000000, 0.9659258262890683122, 1.000000000000000000, 0.9659258262890683122, 1.000000000000000000, 0.9659258262890683122, 1.000000000000000000, 0.9659258262890683122, 1.000000000000000000, 0.9659258262890683122, 1.000000000000000000, 0.9659258262890683122, 1.000000000000000000, 0.9659258262890683122, 1.000000000000000000, 0.9659258262890683122, 1.000000000000000000, 0.9659258262890683122, 1.000000000000000000, 0.9659258262890683122, 1.000000000000000000, 0.9659258262890683122, 1.000000000000000000, 0.9659258262890683122, 1.000000000000000000, 0.9659258262890683122, 1.000000000000000000, 0.9659258262890683122, 1.000000000000000000, 0.9659258262890683122, 1.000000000000000000, 0.9659258262890683122, 1.000000000000000000, 0.9659258262890683122, 1.000000000000000000, 0.9659258262890683122, 1.000000000000000000, 0.9659258262890683122, 1.000000000000000000, 0.9659258262890683122, 1.000000000000000000, 0.9659258262890683122, 1.000000000000000000, 0.9659258262890683122, 1.000000000000000000, 0.9659258262890683122, 1.000000000000000000, 0.9659258262890683122, 1.000000000000000000, 0.9659258262890683122, 1.000000000000000000, 0.9659258262890683122, 1.000000000000000000, 0.9659258262890683122, 1.000000000000000000, 0.9659258262890683122, 1.000000000000000000, 0.9659258262890683122, 1.000000000000000000, 0.9659258262890683122, 1.000000000000000000, 0.9659258262890683122, 1.000000000000000000, 0.9659258262890683122, 1.000000000000000000, 0.9659258262890683122, 1.000000000000000000, 0.9659258262890683122, 1.000000000000000000, 0.9659258262890683122, 1.000000000000000000, 0.9659258262890683122, 1.000000000000000000, 0.9659258262890683122, 1.000000000000000000, 0.9659258262890683122, 1.000000000000000000, 0.9659258262890683122, 1.000000000000000000, 0.9659258262890683122, 1.000000000000000000, 0.9659258262890683122, 1.000000000000000000, 0.9659258262890683122, 1.000000000000000000, 0.9659258262890683122, 1.000000000000000000, 0.9659258262890683122, 1.000000000000000000, 0.9659258262890683122, 1.000000000000000000, 0.9659258262890683122, 1.000000000000000000, 0.9659258262890683122, 1.000000000000000000, 0.9659258262890683122, 1.000000000000000000, 0.9659258262890683122, 1.000000000000000000, 0.9659258262890683122, 1.000000000000000000, 0.9659258262890683122, 1.000000000000000000, 0.9659258262890683122, 1.000000000000000000, 0.9659258262890683122, 1.000000000000000000, 0.9659258262890683122, 1.000000000000000000, 0.9659258262890683122, 1.000000000000000000, 0.9659258262890683122, 1.000000000000000000, 0.9659258262890683122, 1.000000000000000000, 0.9659258262890683122, 1.000000000000000000, 0.9659258262890683122, 1.000000000000000000, 0.9659258262890683122, 1.000000000000000000, 0.9659258262890683122, 1.000000000000000000, 0.9659258262890683122, 1.000000000000000000, 0.9659258262890683122, 1.000000000000000000, 0.9659258262890683122, 1.000000000000000000, 0.9659258262890683122, 1.000000000000000000, 0.9659258262890683122, 1.000000000000000000, 0.9659258262890683122, 1.000000000000000000, 0.9659258262890683122, 1.000000000000000000, 0.9659258262890683122, 1.000000000000000000, 0.9659258262890683122, 1.000000000000000000, 0.9659258262890683122, 1.000000000000000000, 0.9659258262890683122, 1.000000000000000000, 0.9659258262890683122, 1.000000000000000000, 0.9659258262890683122, 1.000000000000000000, 0.9659258262890683122, 1.000000000000000000, 0.9659258262890683122, 1.000000000000000000, 0.9659258262890683122, 1.000000000000000000, 0.9659258262890683122, 1.000000000000000000, 0.9659258262890683122, 1.000000000000000000, 0.9659258262890683122, 1.000000000000000000, 0.9659258262890683122, 1.000000000000000000, 0.9659258262890683122, 1.000000000000000000, 0.9659258262890683122, 1.000000000000000000, 0.9659258262890683122, 1.000000000000000000, 0.9659258262890683122, 1.000000000000000000, 0.9659258262890683122, 1.000000000000000000, 0.9659258262890683122, 1.000000000000000000, 0.9659258262890683122, 1.000000000000000000, 0.9659258262890683122, 1.000000000000000000, 0.9659258262890683122, 1.000000000000000000, 0.9659258262890683122, 1.000000000000000000, 0.9659258262890683122, 1.000000000000000000, 0.9659258262890683122, 1.000000000000000000, 0.9659258262890683122, 1.000000000000000000, 0.9659258262890683122, 1.000000000000000000, 0.9659258262890683122, 1.000000000000000000, 0.9659258262890683122, 1.000000000000000000, 0.9659258262890683122, 1.000000000000000000, 0.9659258262890683122, 1.000000000000000000, 0.9659258262890683122, 1.000000000000000000, 0.9659258262890683122, 1.000000000000000000, 0.9659258262890683122, 1.000000000000000000, 0.9659258262890683122, 1.000000000000000000, 0.9659258262890683122, 1.000000000000000000, 0.9659258262890683122, 1.000000000000000000, 0.9659258262890683122, 1.000000000000000000, 0.9659258262890683122, 1.000000000000000000, 0.9659258262890683122, 1.000000000000000000, 0.9659258262890683122, 1.000000000000000000, 0.9659258262890683122, 1.000000000000000000, 0.9659258262890683122, 1.000000000000000000, 0.9659258262890683122, 1.000000000000000000, 0.9659258262890683122, 1.000000000000000000, 0.9659258262890683122, 1.000000000000000000, 0.9659258262890683122, 1.000000000000000000, 0.9659258262890683122, 1.000000000000000000, 0.9659258262890683122, 1.000000000000000000, 0.9659258262890683122, 1.000000000000000000, 0.9659258262890683122, 1.000000000000000000, 0.9659258262890683122, 1.000000000000000000, 0.9659258262890683122, 1.000000000000000000, 0.9659258262890683122, 1.000000000000000000, 0.9659258262890683122, 1.000000000000000000, 0.9659258262890683122, 1.000000000000000000, 0.9659258262890683122, 1.000000000000000000, 0.9659258262890683122, 1.000000000000000000, 0.9659258262890683122, 1.000000000000000000, 0.9659258262890683122, 1.000000000000000000, 0.9659258262890683122, 1.000000000000000000, 0.9659258262890683122, 1.000000000000000000, 0.9659258262890683122, 1.000000000000000000, 0.9659258262890683122, 1.000000000000000000, 0.9659258262890683122, 1.000000000000000000, 0.9659258262890683122, 1.000000000000000000, 0.9659258262890683122, 1.000000000000000000, 0.9659258262890683122, 1.000000000000000000, 0.9659258262890683122, 1.000000000000000000, 0.9659258262890683122, 1.000000000000000000, 0.9659258262890683122, 1.000000000000000000, 0.9659258262890683122, 1.000000000000000000, 0.9659258262890683122, 1.000000000000000000, 0.9659258262890683122, 1.000000000000000000, 0.9659258262890683122, 1.000000000000000000, 0.9659258262890683122, 1.000000000000000000, 0.9659258262890683122, 1.000000000000000000, 0.9659258262890683122, 1.000000000000000000, 0.9659258262890683122, 1.000000000000000000, 0.9659258262890683122, 1.000000000000000000, 0.9659258262890683122, 1.000000000000000000, 0.9659258262890683122, 1.000000000000000000, 0.9659258262890683122, 1.000000000000000000, 0.9659258262890683122, 1.000000000000000000, 0.9659258262890683122, 1.000000000000000000, 0.9659258262890683122, 1.000000000000000000, 0.9659258262890683122, 1.000000000000000000, 0.9659258262890683122, 1.000000000000000000, 0.9659258262890683122, 1.000000000000000000, 0.9659258262890683122, 1.000000000000000000, 0.9659258262890683122, 1.000000000000000000, 0.9659258262890683122, 1.000000000000000000, 0.9659258262890683122, 1.000000000000000000, 0.9659258262890683122, 1.000000000000000000, 0.9659258262890683122, 1.000000000000000000, 0.9659258262890683122, 1.000000000000000000, 0.9659258262890683122, 1.000000000000000000, 0.9659258262890683122, 1.000000000000000000, 0.9659258262890683122, 1.000000000000000000, 0.9659258262890683122, 1.000000000000000000, 0.9659258262890683122, 1.000000000000000000, 0.9659258262890683122, 1.000000000000000000, 0.9659258262890683122, 1.000000000000000000, 0.9659258262890683122, 1.000000000000000000, 0.9659258262890683122, 1.000000000000000000, 0.9659258262890683122, 1.000000000000000000, 0.9659258262890683122, 1.000000000000000000, 0.9659258262890683122, 1.000000000000000000, 0.9659258262890683122, 1.000000000000000000, 0.9659258262890683122, 1.000000000000000000, 0.9659258262890683122, 1.000000000000000000, 0.9659258262890683122, 1.000000000000000000, 0.9659258262890683122, 1.000000000000000000, 0.9659258262890683122, 1.000000000000000000, 0.9659258262890683122, 1.000000000000000000, 0.9659258262890683122, 1.000000000000000000, 0.9659258262890683122, 1.000000000000000000, 0.9659258262890683122, 1.000000000000000000, 0.9659258262890683122, 1.000000000000000000, 0.9659258262890683122, 1.000000000000000000, 0.9659258262890683122, 1.000000000000000000, 0.9659258262890683122, 1.000000000000000000, 0.9659258262890683122, 1.000000000000000000, 0.9659258262890683122, 1.000000000000000000, 0.9659258262890683122, 1.000000000000000000, 0.9659258262890683122, 1.000000000000000000, 0.9659258262890683122, 1.000000000000000000, 0.9659258262890683122, 1.000000000000000000, 0.9659258262890683122, 1.000000000000000000, 0.9659258262890683122, 1.000000000000000000, 0.9659258262890683122, 1.000000000000000000, 0.9659258262890683122, 1.000000000000000000, 0.9659258262890683122, 1.000000000000000000, 0.9659258262890683122, 1.000000000000000000, 0.9659258262890683122, 1.000000000000000000, 0.9659258262890683122, 1.000000000000000000, 0.9659258262890683122, 1.000000000000000000, 0.9659258262890683122, 1.000000000000000000, 0.9659258262890683122, 1.000000000000000000, 0.9659258262890683122, 1.000000000000000000, 0.9659258262890683122, 1.000000000000000000, 0.9659258262890683122, 1.000000000000000000, 0.9659258262890683122, 1.000000000000000000, 0.9659258262890683122, 1.000000000000000000, 0.9659258262890683122, 1.000000000000000000, 0.9659258262890683122, 1.000000000000000000, 0.9659258262890683122, 1.000000000000000000, 0.9659258262890683122, 1.000000000000000000, 0.9659258262890683122, 1.000000000000000000, 0.9659258262890683122, 1.000000000000000000, 0.9659258262890683122, 1.000000000000000000, 0.9659258262890683122, 1.000000000000000000, 0.9659258262890683122, 1.000000000000000000, 0.9659258262890683122, 1.000000000000000000, 0.9659258262890683122, 1.000000000000000000),
 ( 0.3333333333333333703, 0.3219752754296894559, 0.3333333333333333703, 0.3219752754296894559, 0.3333333333333333703, 0.3219752754296894559, 0.3333333333333333703, 0.3219752754296894559, 0.3333333333333333703, 0.3219752754296894559, 0.3333333333333333703, 0.3219752754296894559, 0.3333333333333333703, 0.3219752754296894559, 0.3333333333333333703, 0.3219752754296894559, 0.3333333333333333703, 0.3219752754296894559, 0.3333333333333333703, 0.3219752754296894559, 0.3333333333333333703, 0.3219752754296894559, 0.3333333333333333703, 0.3219752754296894559, 0.3333333333333333703, 0.3219752754296894559, 0.3333333333333333703, 0.3219752754296894559, 0.3333333333333333703, 0.3219752754296894559, 0.3333333333333333703, 0.3219752754296894559, 0.3333333333333333703, 0.3219752754296894559, 0.3333333333333333703, 0.3219752754296894559, 0.3333333333333333703, 0.3219752754296894559, 0.3333333333333333703, 0.3219752754296894559, 0.3333333333333333703, 0.3219752754296894559, 0.3333333333333333703, 0.3219752754296894559, 0.3333333333333333703, 0.3219752754296894559, 0.3333333333333333703, 0.3219752754296894559, 0.3333333333333333703, 0.3219752754296894559, 0.3333333333333333703, 0.3219752754296894559, 0.3333333333333333703, 0.3219752754296894559, 0.3333333333333333703, 0.3219752754296894559, 0.3333333333333333703, 0.3219752754296894559, 0.3333333333333333703, 0.3219752754296894559, 0.3333333333333333703, 0.3219752754296894559, 0.3333333333333333703, 0.3219752754296894559, 0.3333333333333333703, 0.3219752754296894559, 0.3333333333333333703, 0.3219752754296894559, 0.3333333333333333703, 0.3219752754296894559, 0.3333333333333333703, 0.3219752754296894559, 0.3333333333333333703, 0.3219752754296894559, 0.3333333333333333703, 0.3219752754296894559, 0.3333333333333333703, 0.3219752754296894559, 0.3333333333333333703, 0.3219752754296894559, 0.3333333333333333703, 0.3219752754296894559, 0.3333333333333333703, 0.3219752754296894559, 0.3333333333333333703, 0.3219752754296894559, 0.3333333333333333703, 0.3219752754296894559, 0.3333333333333333703, 0.3219752754296894559, 0.3333333333333333703, 0.3219752754296894559, 0.3333333333333333703, 0.3219752754296894559, 0.3333333333333333703, 0.3219752754296894559, 0.3333333333333333703, 0.3219752754296894559, 0.3333333333333333703, 0.3219752754296894559, 0.3333333333333333703, 0.3219752754296894559, 0.3333333333333333703, 0.3219752754296894559, 0.3333333333333333703, 0.3219752754296894559, 0.3333333333333333703, 0.3219752754296894559, 0.3333333333333333703, 0.3219752754296894559, 0.3333333333333333703, 0.3219752754296894559, 0.3333333333333333703, 0.3219752754296894559, 0.3333333333333333703, 0.3219752754296894559, 0.3333333333333333703, 0.3219752754296894559, 0.3333333333333333703, 0.3219752754296894559, 0.3333333333333333703, 0.3219752754296894559, 0.3333333333333333703, 0.3219752754296894559, 0.3333333333333333703, 0.3219752754296894559, 0.3333333333333333703, 0.3219752754296894559, 0.3333333333333333703, 0.3219752754296894559, 0.3333333333333333703, 0.3219752754296894559, 0.3333333333333333703, 0.3219752754296894559, 0.3333333333333333703, 0.3219752754296894559, 0.3333333333333333703, 0.3219752754296894559, 0.3333333333333333703, 0.3219752754296894559, 0.3333333333333333703, 0.3219752754296894559, 0.3333333333333333703, 0.3219752754296894559, 0.3333333333333333703, 0.3219752754296894559, 0.3333333333333333703, 0.3219752754296894559, 0.3333333333333333703, 0.3219752754296894559, 0.3333333333333333703, 0.3219752754296894559, 0.3333333333333333703, 0.3219752754296894559, 0.3333333333333333703, 0.3219752754296894559, 0.3333333333333333703, 0.3219752754296894559, 0.3333333333333333703, 0.3219752754296894559, 0.3333333333333333703, 0.3219752754296894559, 0.3333333333333333703, 0.3219752754296894559, 0.3333333333333333703, 0.3219752754296894559, 0.3333333333333333703, 0.3219752754296894559, 0.3333333333333333703, 0.3219752754296894559, 0.3333333333333333703, 0.3219752754296894559, 0.3333333333333333703, 0.3219752754296894559, 0.3333333333333333703, 0.3219752754296894559, 0.3333333333333333703, 0.3219752754296894559, 0.3333333333333333703, 0.3219752754296894559, 0.3333333333333333703, 0.3219752754296894559, 0.3333333333333333703, 0.3219752754296894559, 0.3333333333333333703, 0.3219752754296894559, 0.3333333333333333703, 0.3219752754296894559, 0.3333333333333333703, 0.3219752754296894559, 0.3333333333333333703, 0.3219752754296894559, 0.3333333333333333703, 0.3219752754296894559, 0.3333333333333333703, 0.3219752754296894559, 0.3333333333333333703, 0.3219752754296894559, 0.3333333333333333703, 0.3219752754296894559, 0.3333333333333333703, 0.3219752754296894559, 0.3333333333333333703, 0.3219752754296894559, 0.3333333333333333703, 0.3219752754296894559, 0.3333333333333333703, 0.3219752754296894559, 0.3333333333333333703, 0.3219752754296894559, 0.3333333333333333703, 0.3219752754296894559, 0.3333333333333333703, 0.3219752754296894559, 0.3333333333333333703, 0.3219752754296894559, 0.3333333333333333703, 0.3219752754296894559, 0.3333333333333333703, 0.3219752754296894559, 0.3333333333333333703, 0.3219752754296894559, 0.3333333333333333703, 0.3219752754296894559, 0.3333333333333333703, 0.3219752754296894559, 0.3333333333333333703, 0.3219752754296894559, 0.3333333333333333703, 0.3219752754296894559, 0.3333333333333333703, 0.3219752754296894559, 0.3333333333333333703, 0.3219752754296894559, 0.3333333333333333703, 0.3219752754296894559, 0.3333333333333333703, 0.3219752754296894559, 0.3333333333333333703, 0.3219752754296894559, 0.3333333333333333703, 0.3219752754296894559, 0.3333333333333333703, 0.3219752754296894559, 0.3333333333333333703, 0.3219752754296894559, 0.3333333333333333703, 0.3219752754296894559, 0.3333333333333333703, 0.3219752754296894559, 0.3333333333333333703, 0.3219752754296894559, 0.3333333333333333703, 0.3219752754296894559, 0.3333333333333333703, 0.3219752754296894559, 0.3333333333333333703, 0.3219752754296894559, 0.3333333333333333703, 0.3219752754296894559, 0.3333333333333333703, 0.3219752754296894559, 0.3333333333333333703, 0.3219752754296894559, 0.3333333333333333703, 0.3219752754296894559, 0.3333333333333333703, 0.3219752754296894559, 0.3333333333333333703, 0.3219752754296894559, 0.3333333333333333703, 0.3219752754296894559, 0.3333333333333333703, 0.3219752754296894559, 0.3333333333333333703, 0.3219752754296894559, 0.3333333333333333703, 0.3219752754296894559, 0.3333333333333333703, 0.3219752754296894559, 0.3333333333333333703, 0.3219752754296894559, 0.3333333333333333703, 0.3219752754296894559, 0.3333333333333333703, 0.3219752754296894559, 0.3333333333333333703, 0.3219752754296894559, 0.3333333333333333703, 0.3219752754296894559, 0.3333333333333333703, 0.3219752754296894559, 0.3333333333333333703, 0.3219752754296894559, 0.3333333333333333703, 0.3219752754296894559, 0.3333333333333333703, 0.3219752754296894559, 0.3333333333333333703, 0.3219752754296894559, 0.3333333333333333703, 0.3219752754296894559, 0.3333333333333333703, 0.3219752754296894559, 0.3333333333333333703, 0.3219752754296894559, 0.3333333333333333703, 0.3219752754296894559, 0.3333333333333333703, 0.3219752754296894559, 0.3333333333333333703, 0.3219752754296894559, 0.3333333333333333703, 0.3219752754296894559, 0.3333333333333333703, 0.3219752754296894559, 0.3333333333333333703, 0.3219752754296894559, 0.3333333333333333703, 0.3219752754296894559, 0.3333333333333333703, 0.3219752754296894559, 0.3333333333333333703, 0.3219752754296894559, 0.3333333333333333703, 0.3219752754296894559, 0.3333333333333333703, 0.3219752754296894559, 0.3333333333333333703, 0.3219752754296894559, 0.3333333333333333703, 0.3219752754296894559, 0.3333333333333333703, 0.3219752754296894559, 0.3333333333333333703, 0.3219752754296894559, 0.3333333333333333703, 0.3219752754296894559, 0.3333333333333333703, 0.3219752754296894559, 0.3333333333333333703, 0.3219752754296894559, 0.3333333333333333703, 0.3219752754296894559, 0.3333333333333333703, 0.3219752754296894559, 0.3333333333333333703, 0.3219752754296894559, 0.3333333333333333703, 0.3219752754296894559, 0.3333333333333333703, 0.3219752754296894559, 0.3333333333333333703, 0.3219752754296894559, 0.3333333333333333703, 0.3219752754296894559, 0.3333333333333333703, 0.3219752754296894559, 0.3333333333333333703, 0.3219752754296894559, 0.3333333333333333703, 0.3219752754296894559, 0.3333333333333333703, 0.3219752754296894559, 0.3333333333333333703, 0.3219752754296894559, 0.3333333333333333703, 0.3219752754296894559, 0.3333333333333333703, 0.3219752754296894559, 0.3333333333333333703, 0.3219752754296894559, 0.3333333333333333703, 0.3219752754296894559, 0.3333333333333333703, 0.3219752754296894559, 0.3333333333333333703, 0.3219752754296894559, 0.3333333333333333703, 0.3219752754296894559, 0.3333333333333333703, 0.3219752754296894559, 0.3333333333333333703, 0.3219752754296894559, 0.3333333333333333703, 0.3219752754296894559, 0.3333333333333333703, 0.3219752754296894559, 0.3333333333333333703, 0.3219752754296894559, 0.3333333333333333703, 0.3219752754296894559, 0.3333333333333333703, 0.3219752754296894559, 0.3333333333333333703, 0.3219752754296894559, 0.3333333333333333703, 0.3219752754296894559, 0.3333333333333333703, 0.3219752754296894559, 0.3333333333333333703, 0.3219752754296894559, 0.3333333333333333703, 0.3219752754296894559, 0.3333333333333333703, 0.3219752754296894559, 0.3333333333333333703, 0.3219752754296894559, 0.3333333333333333703, 0.3219752754296894559, 0.3333333333333333703, 0.3219752754296894559, 0.3333333333333333703, 0.3219752754296894559, 0.3333333333333333703, 0.3219752754296894559, 0.3333333333333333703, 0.3219752754296894559, 0.3333333333333333703, 0.3219752754296894559, 0.3333333333333333703, 0.3219752754296894559, 0.3333333333333333703, 0.3219752754296894559, 0.3333333333333333703, 0.3219752754296894559, 0.3333333333333333703, 0.3219752754296894559, 0.3333333333333333703, 0.3219752754296894559, 0.3333333333333333703, 0.3219752754296894559, 0.3333333333333333703, 0.3219752754296894559, 0.3333333333333333703, 0.3219752754296894559, 0.3333333333333333703, 0.3219752754296894559, 0.3333333333333333703, 0.3219752754296894559, 0.3333333333333333703, 0.3219752754296894559, 0.3333333333333333703, 0.3219752754296894559, 0.3333333333333333703, 0.3219752754296894559, 0.3333333333333333703, 0.3219752754296894559, 0.3333333333333333703, 0.3219752754296894559, 0.3333333333333333703, 0.3219752754296894559, 0.3333333333333333703, 0.3219752754296894559, 0.3333333333333333703, 0.3219752754296894559, 0.3333333333333333703),
 ( 0.3333333333333333703, 0.3219752754296894559, 0.3333333333333333703, 0.3219752754296894559, 0.3333333333333333703, 0.3219752754296894559, 0.3333333333333333703, 0.3219752754296894559, 0.3333333333333333703, 0.3219752754296894559, 0.3333333333333333703, 0.3219752754296894559, 0.3333333333333333703, 0.3219752754296894559, 0.3333333333333333703, 0.3219752754296894559, 0.3333333333333333703, 0.3219752754296894559, 0.3333333333333333703, 0.3219752754296894559, 0.3333333333333333703, 0.3219752754296894559, 0.3333333333333333703, 0.3219752754296894559, 0.3333333333333333703, 0.3219752754296894559, 0.3333333333333333703, 0.3219752754296894559, 0.3333333333333333703, 0.3219752754296894559, 0.3333333333333333703, 0.3219752754296894559, 0.3333333333333333703, 0.3219752754296894559, 0.3333333333333333703, 0.3219752754296894559, 0.3333333333333333703, 0.3219752754296894559, 0.3333333333333333703, 0.3219752754296894559, 0.3333333333333333703, 0.3219752754296894559, 0.3333333333333333703, 0.3219752754296894559, 0.3333333333333333703, 0.3219752754296894559, 0.3333333333333333703, 0.3219752754296894559, 0.3333333333333333703, 0.3219752754296894559, 0.3333333333333333703, 0.3219752754296894559, 0.3333333333333333703, 0.3219752754296894559, 0.3333333333333333703, 0.3219752754296894559, 0.3333333333333333703, 0.3219752754296894559, 0.3333333333333333703, 0.3219752754296894559, 0.3333333333333333703, 0.3219752754296894559, 0.3333333333333333703, 0.3219752754296894559, 0.3333333333333333703, 0.3219752754296894559, 0.3333333333333333703, 0.3219752754296894559, 0.3333333333333333703, 0.3219752754296894559, 0.3333333333333333703, 0.3219752754296894559, 0.3333333333333333703, 0.3219752754296894559, 0.3333333333333333703, 0.3219752754296894559, 0.3333333333333333703, 0.3219752754296894559, 0.3333333333333333703, 0.3219752754296894559, 0.3333333333333333703, 0.3219752754296894559, 0.3333333333333333703, 0.3219752754296894559, 0.3333333333333333703, 0.3219752754296894559, 0.3333333333333333703, 0.3219752754296894559, 0.3333333333333333703, 0.3219752754296894559, 0.3333333333333333703, 0.3219752754296894559, 0.3333333333333333703, 0.3219752754296894559, 0.3333333333333333703, 0.3219752754296894559, 0.3333333333333333703, 0.3219752754296894559, 0.3333333333333333703, 0.3219752754296894559, 0.3333333333333333703, 0.3219752754296894559, 0.3333333333333333703, 0.3219752754296894559, 0.3333333333333333703, 0.3219752754296894559, 0.3333333333333333703, 0.3219752754296894559, 0.3333333333333333703, 0.3219752754296894559, 0.3333333333333333703, 0.3219752754296894559, 0.3333333333333333703, 0.3219752754296894559, 0.3333333333333333703, 0.3219752754296894559, 0.3333333333333333703, 0.3219752754296894559, 0.3333333333333333703, 0.3219752754296894559, 0.3333333333333333703, 0.3219752754296894559, 0.3333333333333333703, 0.3219752754296894559, 0.3333333333333333703, 0.3219752754296894559, 0.3333333333333333703, 0.3219752754296894559, 0.3333333333333333703, 0.3219752754296894559, 0.3333333333333333703, 0.3219752754296894559, 0.3333333333333333703, 0.3219752754296894559, 0.3333333333333333703, 0.3219752754296894559, 0.3333333333333333703, 0.3219752754296894559, 0.3333333333333333703, 0.3219752754296894559, 0.3333333333333333703, 0.3219752754296894559, 0.3333333333333333703, 0.3219752754296894559, 0.3333333333333333703, 0.3219752754296894559, 0.3333333333333333703, 0.3219752754296894559, 0.3333333333333333703, 0.3219752754296894559, 0.3333333333333333703, 0.3219752754296894559, 0.3333333333333333703, 0.3219752754296894559, 0.3333333333333333703, 0.3219752754296894559, 0.3333333333333333703, 0.3219752754296894559, 0.3333333333333333703, 0.3219752754296894559, 0.3333333333333333703, 0.3219752754296894559, 0.3333333333333333703, 0.3219752754296894559, 0.3333333333333333703, 0.3219752754296894559, 0.3333333333333333703, 0.3219752754296894559, 0.3333333333333333703, 0.3219752754296894559, 0.3333333333333333703, 0.3219752754296894559, 0.3333333333333333703, 0.3219752754296894559, 0.3333333333333333703, 0.3219752754296894559, 0.3333333333333333703, 0.3219752754296894559, 0.3333333333333333703, 0.3219752754296894559, 0.3333333333333333703, 0.3219752754296894559, 0.3333333333333333703, 0.3219752754296894559, 0.3333333333333333703, 0.3219752754296894559, 0.3333333333333333703, 0.3219752754296894559, 0.3333333333333333703, 0.3219752754296894559, 0.3333333333333333703, 0.3219752754296894559, 0.3333333333333333703, 0.3219752754296894559, 0.3333333333333333703, 0.3219752754296894559, 0.3333333333333333703, 0.3219752754296894559, 0.3333333333333333703, 0.3219752754296894559, 0.3333333333333333703, 0.3219752754296894559, 0.3333333333333333703, 0.3219752754296894559, 0.3333333333333333703, 0.3219752754296894559, 0.3333333333333333703, 0.3219752754296894559, 0.3333333333333333703, 0.3219752754296894559, 0.3333333333333333703, 0.3219752754296894559, 0.3333333333333333703, 0.3219752754296894559, 0.3333333333333333703, 0.3219752754296894559, 0.3333333333333333703, 0.3219752754296894559, 0.3333333333333333703, 0.3219752754296894559, 0.3333333333333333703, 0.3219752754296894559, 0.3333333333333333703, 0.3219752754296894559, 0.3333333333333333703, 0.3219752754296894559, 0.3333333333333333703, 0.3219752754296894559, 0.3333333333333333703, 0.3219752754296894559, 0.3333333333333333703, 0.3219752754296894559, 0.3333333333333333703, 0.3219752754296894559, 0.3333333333333333703, 0.3219752754296894559, 0.3333333333333333703, 0.3219752754296894559, 0.3333333333333333703, 0.3219752754296894559, 0.3333333333333333703, 0.3219752754296894559, 0.3333333333333333703, 0.3219752754296894559, 0.3333333333333333703, 0.3219752754296894559, 0.3333333333333333703, 0.3219752754296894559, 0.3333333333333333703, 0.3219752754296894559, 0.3333333333333333703, 0.3219752754296894559, 0.3333333333333333703, 0.3219752754296894559, 0.3333333333333333703, 0.3219752754296894559, 0.3333333333333333703, 0.3219752754296894559, 0.3333333333333333703, 0.3219752754296894559, 0.3333333333333333703, 0.3219752754296894559, 0.3333333333333333703, 0.3219752754296894559, 0.3333333333333333703, 0.3219752754296894559, 0.3333333333333333703, 0.3219752754296894559, 0.3333333333333333703, 0.3219752754296894559, 0.3333333333333333703, 0.3219752754296894559, 0.3333333333333333703, 0.3219752754296894559, 0.3333333333333333703, 0.3219752754296894559, 0.3333333333333333703, 0.3219752754296894559, 0.3333333333333333703, 0.3219752754296894559, 0.3333333333333333703, 0.3219752754296894559, 0.3333333333333333703, 0.3219752754296894559, 0.3333333333333333703, 0.3219752754296894559, 0.3333333333333333703, 0.3219752754296894559, 0.3333333333333333703, 0.3219752754296894559, 0.3333333333333333703, 0.3219752754296894559, 0.3333333333333333703, 0.3219752754296894559, 0.3333333333333333703, 0.3219752754296894559, 0.3333333333333333703, 0.3219752754296894559, 0.3333333333333333703, 0.3219752754296894559, 0.3333333333333333703, 0.3219752754296894559, 0.3333333333333333703, 0.3219752754296894559, 0.3333333333333333703, 0.3219752754296894559, 0.3333333333333333703, 0.3219752754296894559, 0.3333333333333333703, 0.3219752754296894559, 0.3333333333333333703, 0.3219752754296894559, 0.3333333333333333703, 0.3219752754296894559, 0.3333333333333333703, 0.3219752754296894559, 0.3333333333333333703, 0.3219752754296894559, 0.3333333333333333703, 0.3219752754296894559, 0.3333333333333333703, 0.3219752754296894559, 0.3333333333333333703, 0.3219752754296894559, 0.3333333333333333703, 0.3219752754296894559, 0.3333333333333333703, 0.3219752754296894559, 0.3333333333333333703, 0.3219752754296894559, 0.3333333333333333703, 0.3219752754296894559, 0.3333333333333333703, 0.3219752754296894559, 0.3333333333333333703, 0.3219752754296894559, 0.3333333333333333703, 0.3219752754296894559, 0.3333333333333333703, 0.3219752754296894559, 0.3333333333333333703, 0.3219752754296894559, 0.3333333333333333703, 0.3219752754296894559, 0.3333333333333333703, 0.3219752754296894559, 0.3333333333333333703, 0.3219752754296894559, 0.3333333333333333703, 0.3219752754296894559, 0.3333333333333333703, 0.3219752754296894559, 0.3333333333333333703, 0.3219752754296894559, 0.3333333333333333703, 0.3219752754296894559, 0.3333333333333333703, 0.3219752754296894559, 0.3333333333333333703, 0.3219752754296894559, 0.3333333333333333703, 0.3219752754296894559, 0.3333333333333333703, 0.3219752754296894559, 0.3333333333333333703, 0.3219752754296894559, 0.3333333333333333703, 0.3219752754296894559, 0.3333333333333333703, 0.3219752754296894559, 0.3333333333333333703, 0.3219752754296894559, 0.3333333333333333703, 0.3219752754296894559, 0.3333333333333333703, 0.3219752754296894559, 0.3333333333333333703, 0.3219752754296894559, 0.3333333333333333703, 0.3219752754296894559, 0.3333333333333333703, 0.3219752754296894559, 0.3333333333333333703, 0.3219752754296894559, 0.3333333333333333703, 0.3219752754296894559, 0.3333333333333333703, 0.3219752754296894559, 0.3333333333333333703, 0.3219752754296894559, 0.3333333333333333703, 0.3219752754296894559, 0.3333333333333333703, 0.3219752754296894559, 0.3333333333333333703, 0.3219752754296894559, 0.3333333333333333703, 0.3219752754296894559, 0.3333333333333333703, 0.3219752754296894559, 0.3333333333333333703, 0.3219752754296894559, 0.3333333333333333703, 0.3219752754296894559, 0.3333333333333333703, 0.3219752754296894559, 0.3333333333333333703, 0.3219752754296894559, 0.3333333333333333703, 0.3219752754296894559, 0.3333333333333333703, 0.3219752754296894559, 0.3333333333333333703, 0.3219752754296894559, 0.3333333333333333703, 0.3219752754296894559, 0.3333333333333333703, 0.3219752754296894559, 0.3333333333333333703, 0.3219752754296894559, 0.3333333333333333703, 0.3219752754296894559, 0.3333333333333333703, 0.3219752754296894559, 0.3333333333333333703, 0.3219752754296894559, 0.3333333333333333703, 0.3219752754296894559, 0.3333333333333333703, 0.3219752754296894559, 0.3333333333333333703, 0.3219752754296894559, 0.3333333333333333703, 0.3219752754296894559, 0.3333333333333333703, 0.3219752754296894559, 0.3333333333333333703, 0.3219752754296894559, 0.3333333333333333703, 0.3219752754296894559, 0.3333333333333333703, 0.3219752754296894559, 0.3333333333333333703, 0.3219752754296894559, 0.3333333333333333703, 0.3219752754296894559, 0.3333333333333333703, 0.3219752754296894559, 0.3333333333333333703, 0.3219752754296894559, 0.3333333333333333703, 0.3219752754296894559, 0.3333333333333333703, 0.3219752754296894559, 0.3333333333333333703, 0.3219752754296894559, 0.3333333333333333703),
 ( 1.000000000000000000, 0.9659258262890683122, 1.000000000000000000, 0.9659258262890683122, 1.000000000000000000, 0.9659258262890683122, 1.000000000000000000, 0.9659258262890683122, 1.000000000000000000, 0.9659258262890683122, 1.000000000000000000, 0.9659258262890683122, 1.000000000000000000, 0.9659258262890683122, 1.000000000000000000, 0.9659258262890683122, 1.000000000000000000, 0.9659258262890683122, 1.000000000000000000, 0.9659258262890683122, 1.000000000000000000, 0.9659258262890683122, 1.000000000000000000, 0.9659258262890683122, 1.000000000000000000, 0.9659258262890683122, 1.000000000000000000, 0.9659258262890683122, 1.000000000000000000, 0.9659258262890683122, 1.000000000000000000, 0.9659258262890683122, 1.000000000000000000, 0.9659258262890683122, 1.000000000000000000, 0.9659258262890683122, 1.000000000000000000, 0.9659258262890683122, 1.000000000000000000, 0.9659258262890683122, 1.000000000000000000, 0.9659258262890683122, 1.000000000000000000, 0.9659258262890683122, 1.000000000000000000, 0.9659258262890683122, 1.000000000000000000, 0.9659258262890683122, 1.000000000000000000, 0.9659258262890683122, 1.000000000000000000, 0.9659258262890683122, 1.000000000000000000, 0.9659258262890683122, 1.000000000000000000, 0.9659258262890683122, 1.000000000000000000, 0.9659258262890683122, 1.000000000000000000, 0.9659258262890683122, 1.000000000000000000, 0.9659258262890683122, 1.000000000000000000, 0.9659258262890683122, 1.000000000000000000, 0.9659258262890683122, 1.000000000000000000, 0.9659258262890683122, 1.000000000000000000, 0.9659258262890683122, 1.000000000000000000, 0.9659258262890683122, 1.000000000000000000, 0.9659258262890683122, 1.000000000000000000, 0.9659258262890683122, 1.000000000000000000, 0.9659258262890683122, 1.000000000000000000, 0.9659258262890683122, 1.000000000000000000, 0.9659258262890683122, 1.000000000000000000, 0.9659258262890683122, 1.000000000000000000, 0.9659258262890683122, 1.000000000000000000, 0.9659258262890683122, 1.000000000000000000, 0.9659258262890683122, 1.000000000000000000, 0.9659258262890683122, 1.000000000000000000, 0.9659258262890683122, 1.000000000000000000, 0.9659258262890683122, 1.000000000000000000, 0.9659258262890683122, 1.000000000000000000, 0.9659258262890683122, 1.000000000000000000, 0.9659258262890683122, 1.000000000000000000, 0.9659258262890683122, 1.000000000000000000, 0.9659258262890683122, 1.000000000000000000, 0.9659258262890683122, 1.000000000000000000, 0.9659258262890683122, 1.000000000000000000, 0.9659258262890683122, 1.000000000000000000, 0.9659258262890683122, 1.000000000000000000, 0.9659258262890683122, 1.000000000000000000, 0.9659258262890683122, 1.000000000000000000, 0.9659258262890683122, 1.000000000000000000, 0.9659258262890683122, 1.000000000000000000, 0.9659258262890683122, 1.000000000000000000, 0.9659258262890683122, 1.000000000000000000, 0.9659258262890683122, 1.000000000000000000, 0.9659258262890683122, 1.000000000000000000, 0.9659258262890683122, 1.000000000000000000, 0.9659258262890683122, 1.000000000000000000, 0.9659258262890683122, 1.000000000000000000, 0.9659258262890683122, 1.000000000000000000, 0.9659258262890683122, 1.000000000000000000, 0.9659258262890683122, 1.000000000000000000, 0.9659258262890683122, 1.000000000000000000, 0.9659258262890683122, 1.000000000000000000, 0.9659258262890683122, 1.000000000000000000, 0.9659258262890683122, 1.000000000000000000, 0.9659258262890683122, 1.000000000000000000, 0.9659258262890683122, 1.000000000000000000, 0.9659258262890683122, 1.000000000000000000, 0.9659258262890683122, 1.000000000000000000, 0.9659258262890683122, 1.000000000000000000, 0.9659258262890683122, 1.000000000000000000, 0.9659258262890683122, 1.000000000000000000, 0.9659258262890683122, 1.000000000000000000, 0.9659258262890683122, 1.000000000000000000, 0.9659258262890683122, 1.000000000000000000, 0.9659258262890683122, 1.000000000000000000, 0.9659258262890683122, 1.000000000000000000, 0.9659258262890683122, 1.000000000000000000, 0.9659258262890683122, 1.000000000000000000, 0.9659258262890683122, 1.000000000000000000, 0.9659258262890683122, 1.000000000000000000, 0.9659258262890683122, 1.000000000000000000, 0.9659258262890683122, 1.000000000000000000, 0.9659258262890683122, 1.000000000000000000, 0.9659258262890683122, 1.000000000000000000, 0.9659258262890683122, 1.000000000000000000, 0.9659258262890683122, 1.000000000000000000, 0.9659258262890683122, 1.000000000000000000, 0.9659258262890683122, 1.000000000000000000, 0.9659258262890683122, 1.000000000000000000, 0.9659258262890683122, 1.000000000000000000, 0.9659258262890683122, 1.000000000000000000, 0.9659258262890683122, 1.000000000000000000, 0.9659258262890683122, 1.000000000000000000, 0.9659258262890683122, 1.000000000000000000, 0.9659258262890683122, 1.000000000000000000, 0.9659258262890683122, 1.000000000000000000, 0.9659258262890683122, 1.000000000000000000, 0.9659258262890683122, 1.000000000000000000, 0.9659258262890683122, 1.000000000000000000, 0.9659258262890683122, 1.000000000000000000, 0.9659258262890683122, 1.000000000000000000, 0.9659258262890683122, 1.000000000000000000, 0.9659258262890683122, 1.000000000000000000, 0.9659258262890683122, 1.000000000000000000, 0.9659258262890683122, 1.000000000000000000, 0.9659258262890683122, 1.000000000000000000, 0.9659258262890683122, 1.000000000000000000, 0.9659258262890683122, 1.000000000000000000, 0.9659258262890683122, 1.000000000000000000, 0.9659258262890683122, 1.000000000000000000, 0.9659258262890683122, 1.000000000000000000, 0.9659258262890683122, 1.000000000000000000, 0.9659258262890683122, 1.000000000000000000, 0.9659258262890683122, 1.000000000000000000, 0.9659258262890683122, 1.000000000000000000, 0.9659258262890683122, 1.000000000000000000, 0.9659258262890683122, 1.000000000000000000, 0.9659258262890683122, 1.000000000000000000, 0.9659258262890683122, 1.000000000000000000, 0.9659258262890683122, 1.000000000000000000, 0.9659258262890683122, 1.000000000000000000, 0.9659258262890683122, 1.000000000000000000, 0.9659258262890683122, 1.000000000000000000, 0.9659258262890683122, 1.000000000000000000, 0.9659258262890683122, 1.000000000000000000, 0.9659258262890683122, 1.000000000000000000, 0.9659258262890683122, 1.000000000000000000, 0.9659258262890683122, 1.000000000000000000, 0.9659258262890683122, 1.000000000000000000, 0.9659258262890683122, 1.000000000000000000, 0.9659258262890683122, 1.000000000000000000, 0.9659258262890683122, 1.000000000000000000, 0.9659258262890683122, 1.000000000000000000, 0.9659258262890683122, 1.000000000000000000, 0.9659258262890683122, 1.000000000000000000, 0.9659258262890683122, 1.000000000000000000, 0.9659258262890683122, 1.000000000000000000, 0.9659258262890683122, 1.000000000000000000, 0.9659258262890683122, 1.000000000000000000, 0.9659258262890683122, 1.000000000000000000, 0.9659258262890683122, 1.000000000000000000, 0.9659258262890683122, 1.000000000000000000, 0.9659258262890683122, 1.000000000000000000, 0.9659258262890683122, 1.000000000000000000, 0.9659258262890683122, 1.000000000000000000, 0.9659258262890683122, 1.000000000000000000, 0.9659258262890683122, 1.000000000000000000, 0.9659258262890683122, 1.000000000000000000, 0.9659258262890683122, 1.000000000000000000, 0.9659258262890683122, 1.000000000000000000, 0.9659258262890683122, 1.000000000000000000, 0.9659258262890683122, 1.000000000000000000, 0.9659258262890683122, 1.000000000000000000, 0.9659258262890683122, 1.000000000000000000, 0.9659258262890683122, 1.000000000000000000, 0.9659258262890683122, 1.000000000000000000, 0.9659258262890683122, 1.000000000000000000, 0.9659258262890683122, 1.000000000000000000, 0.9659258262890683122, 1.000000000000000000, 0.9659258262890683122, 1.000000000000000000, 0.9659258262890683122, 1.000000000000000000, 0.9659258262890683122, 1.000000000000000000, 0.9659258262890683122, 1.000000000000000000, 0.9659258262890683122, 1.000000000000000000, 0.9659258262890683122, 1.000000000000000000, 0.9659258262890683122, 1.000000000000000000, 0.9659258262890683122, 1.000000000000000000, 0.9659258262890683122, 1.000000000000000000, 0.9659258262890683122, 1.000000000000000000, 0.9659258262890683122, 1.000000000000000000, 0.9659258262890683122, 1.000000000000000000, 0.9659258262890683122, 1.000000000000000000, 0.9659258262890683122, 1.000000000000000000, 0.9659258262890683122, 1.000000000000000000, 0.9659258262890683122, 1.000000000000000000, 0.9659258262890683122, 1.000000000000000000, 0.9659258262890683122, 1.000000000000000000, 0.9659258262890683122, 1.000000000000000000, 0.9659258262890683122, 1.000000000000000000, 0.9659258262890683122, 1.000000000000000000, 0.9659258262890683122, 1.000000000000000000, 0.9659258262890683122, 1.000000000000000000, 0.9659258262890683122, 1.000000000000000000, 0.9659258262890683122, 1.000000000000000000, 0.9659258262890683122, 1.000000000000000000, 0.9659258262890683122, 1.000000000000000000, 0.9659258262890683122, 1.000000000000000000, 0.9659258262890683122, 1.000000000000000000, 0.9659258262890683122, 1.000000000000000000, 0.9659258262890683122, 1.000000000000000000, 0.9659258262890683122, 1.000000000000000000, 0.9659258262890683122, 1.000000000000000000, 0.9659258262890683122, 1.000000000000000000, 0.9659258262890683122, 1.000000000000000000, 0.9659258262890683122, 1.000000000000000000, 0.9659258262890683122, 1.000000000000000000, 0.9659258262890683122, 1.000000000000000000, 0.9659258262890683122, 1.000000000000000000, 0.9659258262890683122, 1.000000000000000000, 0.9659258262890683122, 1.000000000000000000, 0.9659258262890683122, 1.000000000000000000, 0.9659258262890683122, 1.000000000000000000, 0.9659258262890683122, 1.000000000000000000, 0.9659258262890683122, 1.000000000000000000, 0.9659258262890683122, 1.000000000000000000, 0.9659258262890683122, 1.000000000000000000, 0.9659258262890683122, 1.000000000000000000, 0.9659258262890683122, 1.000000000000000000, 0.9659258262890683122, 1.000000000000000000, 0.9659258262890683122, 1.000000000000000000, 0.9659258262890683122, 1.000000000000000000, 0.9659258262890683122, 1.000000000000000000, 0.9659258262890683122, 1.000000000000000000, 0.9659258262890683122, 1.000000000000000000, 0.9659258262890683122, 1.000000000000000000, 0.9659258262890683122, 1.000000000000000000, 0.9659258262890683122, 1.000000000000000000),
 ( 0.3333333333333333703, 0.3219752754296894559, 0.3333333333333333703, 0.3219752754296894559, 0.3333333333333333703, 0.3219752754296894559, 0.3333333333333333703, 0.3219752754296894559, 0.3333333333333333703, 0.3219752754296894559, 0.3333333333333333703, 0.3219752754296894559, 0.3333333333333333703, 0.3219752754296894559, 0.3333333333333333703, 0.3219752754296894559, 0.3333333333333333703, 0.3219752754296894559, 0.3333333333333333703, 0.3219752754296894559, 0.3333333333333333703, 0.3219752754296894559, 0.3333333333333333703, 0.3219752754296894559, 0.3333333333333333703, 0.3219752754296894559, 0.3333333333333333703, 0.3219752754296894559, 0.3333333333333333703, 0.3219752754296894559, 0.3333333333333333703, 0.3219752754296894559, 0.3333333333333333703, 0.3219752754296894559, 0.3333333333333333703, 0.3219752754296894559, 0.3333333333333333703, 0.3219752754296894559, 0.3333333333333333703, 0.3219752754296894559, 0.3333333333333333703, 0.3219752754296894559, 0.3333333333333333703, 0.3219752754296894559, 0.3333333333333333703, 0.3219752754296894559, 0.3333333333333333703, 0.3219752754296894559, 0.3333333333333333703, 0.3219752754296894559, 0.3333333333333333703, 0.3219752754296894559, 0.3333333333333333703, 0.3219752754296894559, 0.3333333333333333703, 0.3219752754296894559, 0.3333333333333333703, 0.3219752754296894559, 0.3333333333333333703, 0.3219752754296894559, 0.3333333333333333703, 0.3219752754296894559, 0.3333333333333333703, 0.3219752754296894559, 0.3333333333333333703, 0.3219752754296894559, 0.3333333333333333703, 0.3219752754296894559, 0.3333333333333333703, 0.3219752754296894559, 0.3333333333333333703, 0.3219752754296894559, 0.3333333333333333703, 0.3219752754296894559, 0.3333333333333333703, 0.3219752754296894559, 0.3333333333333333703, 0.3219752754296894559, 0.3333333333333333703, 0.3219752754296894559, 0.3333333333333333703, 0.3219752754296894559, 0.3333333333333333703, 0.3219752754296894559, 0.3333333333333333703, 0.3219752754296894559, 0.3333333333333333703, 0.3219752754296894559, 0.3333333333333333703, 0.3219752754296894559, 0.3333333333333333703, 0.3219752754296894559, 0.3333333333333333703, 0.3219752754296894559, 0.3333333333333333703, 0.3219752754296894559, 0.3333333333333333703, 0.3219752754296894559, 0.3333333333333333703, 0.3219752754296894559, 0.3333333333333333703, 0.3219752754296894559, 0.3333333333333333703, 0.3219752754296894559, 0.3333333333333333703, 0.3219752754296894559, 0.3333333333333333703, 0.3219752754296894559, 0.3333333333333333703, 0.3219752754296894559, 0.3333333333333333703, 0.3219752754296894559, 0.3333333333333333703, 0.3219752754296894559, 0.3333333333333333703, 0.3219752754296894559, 0.3333333333333333703, 0.3219752754296894559, 0.3333333333333333703, 0.3219752754296894559, 0.3333333333333333703, 0.3219752754296894559, 0.3333333333333333703, 0.3219752754296894559, 0.3333333333333333703, 0.3219752754296894559, 0.3333333333333333703, 0.3219752754296894559, 0.3333333333333333703, 0.3219752754296894559, 0.3333333333333333703, 0.3219752754296894559, 0.3333333333333333703, 0.3219752754296894559, 0.3333333333333333703, 0.3219752754296894559, 0.3333333333333333703, 0.3219752754296894559, 0.3333333333333333703, 0.3219752754296894559, 0.3333333333333333703, 0.3219752754296894559, 0.3333333333333333703, 0.3219752754296894559, 0.3333333333333333703, 0.3219752754296894559, 0.3333333333333333703, 0.3219752754296894559, 0.3333333333333333703, 0.3219752754296894559, 0.3333333333333333703, 0.3219752754296894559, 0.3333333333333333703, 0.3219752754296894559, 0.3333333333333333703, 0.3219752754296894559, 0.3333333333333333703, 0.3219752754296894559, 0.3333333333333333703, 0.3219752754296894559, 0.3333333333333333703, 0.3219752754296894559, 0.3333333333333333703, 0.3219752754296894559, 0.3333333333333333703, 0.3219752754296894559, 0.3333333333333333703, 0.3219752754296894559, 0.3333333333333333703, 0.3219752754296894559, 0.3333333333333333703, 0.3219752754296894559, 0.3333333333333333703, 0.3219752754296894559, 0.3333333333333333703, 0.3219752754296894559, 0.3333333333333333703, 0.3219752754296894559, 0.3333333333333333703, 0.3219752754296894559, 0.3333333333333333703, 0.3219752754296894559, 0.3333333333333333703, 0.3219752754296894559, 0.3333333333333333703, 0.3219752754296894559, 0.3333333333333333703, 0.3219752754296894559, 0.3333333333333333703, 0.3219752754296894559, 0.3333333333333333703, 0.3219752754296894559, 0.3333333333333333703, 0.3219752754296894559, 0.3333333333333333703, 0.3219752754296894559, 0.3333333333333333703, 0.3219752754296894559, 0.3333333333333333703, 0.3219752754296894559, 0.3333333333333333703, 0.3219752754296894559, 0.3333333333333333703, 0.3219752754296894559, 0.3333333333333333703, 0.3219752754296894559, 0.3333333333333333703, 0.3219752754296894559, 0.3333333333333333703, 0.3219752754296894559, 0.3333333333333333703, 0.3219752754296894559, 0.3333333333333333703, 0.3219752754296894559, 0.3333333333333333703, 0.3219752754296894559, 0.3333333333333333703, 0.3219752754296894559, 0.3333333333333333703, 0.3219752754296894559, 0.3333333333333333703, 0.3219752754296894559, 0.3333333333333333703, 0.3219752754296894559, 0.3333333333333333703, 0.3219752754296894559, 0.3333333333333333703, 0.3219752754296894559, 0.3333333333333333703, 0.3219752754296894559, 0.3333333333333333703, 0.3219752754296894559, 0.3333333333333333703, 0.3219752754296894559, 0.3333333333333333703, 0.3219752754296894559, 0.3333333333333333703, 0.3219752754296894559, 0.3333333333333333703, 0.3219752754296894559, 0.3333333333333333703, 0.3219752754296894559, 0.3333333333333333703, 0.3219752754296894559, 0.3333333333333333703, 0.3219752754296894559, 0.3333333333333333703, 0.3219752754296894559, 0.3333333333333333703, 0.3219752754296894559, 0.3333333333333333703, 0.3219752754296894559, 0.3333333333333333703, 0.3219752754296894559, 0.3333333333333333703, 0.3219752754296894559, 0.3333333333333333703, 0.3219752754296894559, 0.3333333333333333703, 0.3219752754296894559, 0.3333333333333333703, 0.3219752754296894559, 0.3333333333333333703, 0.3219752754296894559, 0.3333333333333333703, 0.3219752754296894559, 0.3333333333333333703, 0.3219752754296894559, 0.3333333333333333703, 0.3219752754296894559, 0.3333333333333333703, 0.3219752754296894559, 0.3333333333333333703, 0.3219752754296894559, 0.3333333333333333703, 0.3219752754296894559, 0.3333333333333333703, 0.3219752754296894559, 0.3333333333333333703, 0.3219752754296894559, 0.3333333333333333703, 0.3219752754296894559, 0.3333333333333333703, 0.3219752754296894559, 0.3333333333333333703, 0.3219752754296894559, 0.3333333333333333703, 0.3219752754296894559, 0.3333333333333333703, 0.3219752754296894559, 0.3333333333333333703, 0.3219752754296894559, 0.3333333333333333703, 0.3219752754296894559, 0.3333333333333333703, 0.3219752754296894559, 0.3333333333333333703, 0.3219752754296894559, 0.3333333333333333703, 0.3219752754296894559, 0.3333333333333333703, 0.3219752754296894559, 0.3333333333333333703, 0.3219752754296894559, 0.3333333333333333703, 0.3219752754296894559, 0.3333333333333333703, 0.3219752754296894559, 0.3333333333333333703, 0.3219752754296894559, 0.3333333333333333703, 0.3219752754296894559, 0.3333333333333333703, 0.3219752754296894559, 0.3333333333333333703, 0.3219752754296894559, 0.3333333333333333703, 0.3219752754296894559, 0.3333333333333333703, 0.3219752754296894559, 0.3333333333333333703, 0.3219752754296894559, 0.3333333333333333703, 0.3219752754296894559, 0.3333333333333333703, 0.3219752754296894559, 0.3333333333333333703, 0.3219752754296894559, 0.3333333333333333703, 0.3219752754296894559, 0.3333333333333333703, 0.3219752754296894559, 0.3333333333333333703, 0.3219752754296894559, 0.3333333333333333703, 0.3219752754296894559, 0.3333333333333333703, 0.3219752754296894559, 0.3333333333333333703, 0.3219752754296894559, 0.3333333333333333703, 0.3219752754296894559, 0.3333333333333333703, 0.3219752754296894559, 0.3333333333333333703, 0.3219752754296894559, 0.3333333333333333703, 0.3219752754296894559, 0.3333333333333333703, 0.3219752754296894559, 0.3333333333333333703, 0.3219752754296894559, 0.3333333333333333703, 0.3219752754296894559, 0.3333333333333333703, 0.3219752754296894559, 0.3333333333333333703, 0.3219752754296894559, 0.3333333333333333703, 0.3219752754296894559, 0.3333333333333333703, 0.3219752754296894559, 0.3333333333333333703, 0.3219752754296894559, 0.3333333333333333703, 0.3219752754296894559, 0.3333333333333333703, 0.3219752754296894559, 0.3333333333333333703, 0.3219752754296894559, 0.3333333333333333703, 0.3219752754296894559, 0.3333333333333333703, 0.3219752754296894559, 0.3333333333333333703, 0.3219752754296894559, 0.3333333333333333703, 0.3219752754296894559, 0.3333333333333333703, 0.3219752754296894559, 0.3333333333333333703, 0.3219752754296894559, 0.3333333333333333703, 0.3219752754296894559, 0.3333333333333333703, 0.3219752754296894559, 0.3333333333333333703, 0.3219752754296894559, 0.3333333333333333703, 0.3219752754296894559, 0.3333333333333333703, 0.3219752754296894559, 0.3333333333333333703, 0.3219752754296894559, 0.3333333333333333703, 0.3219752754296894559, 0.3333333333333333703, 0.3219752754296894559, 0.3333333333333333703, 0.3219752754296894559, 0.3333333333333333703, 0.3219752754296894559, 0.3333333333333333703, 0.3219752754296894559, 0.3333333333333333703, 0.3219752754296894559, 0.3333333333333333703, 0.3219752754296894559, 0.3333333333333333703, 0.3219752754296894559, 0.3333333333333333703, 0.3219752754296894559, 0.3333333333333333703, 0.3219752754296894559, 0.3333333333333333703, 0.3219752754296894559, 0.3333333333333333703, 0.3219752754296894559, 0.3333333333333333703, 0.3219752754296894559, 0.3333333333333333703, 0.3219752754296894559, 0.3333333333333333703, 0.3219752754296894559, 0.3333333333333333703, 0.3219752754296894559, 0.3333333333333333703, 0.3219752754296894559, 0.3333333333333333703, 0.3219752754296894559, 0.3333333333333333703, 0.3219752754296894559, 0.3333333333333333703, 0.3219752754296894559, 0.3333333333333333703, 0.3219752754296894559, 0.3333333333333333703, 0.3219752754296894559, 0.3333333333333333703, 0.3219752754296894559, 0.3333333333333333703, 0.3219752754296894559, 0.3333333333333333703, 0.3219752754296894559, 0.3333333333333333703, 0.3219752754296894559, 0.3333333333333333703, 0.3219752754296894559, 0.3333333333333333703, 0.3219752754296894559, 0.3333333333333333703, 0.3219752754296894559, 0.3333333333333333703, 0.3219752754296894559, 0.3333333333333333703, 0.3219752754296894559, 0.3333333333333333703),
 ( 0.3333333333333333703, 0.3219752754296894559, 0.3333333333333333703, 0.3219752754296894559, 0.3333333333333333703, 0.3219752754296894559, 0.3333333333333333703, 0.3219752754296894559, 0.3333333333333333703, 0.3219752754296894559, 0.3333333333333333703, 0.3219752754296894559, 0.3333333333333333703, 0.3219752754296894559, 0.3333333333333333703, 0.3219752754296894559, 0.3333333333333333703, 0.3219752754296894559, 0.3333333333333333703, 0.3219752754296894559, 0.3333333333333333703, 0.3219752754296894559, 0.3333333333333333703, 0.3219752754296894559, 0.3333333333333333703, 0.3219752754296894559, 0.3333333333333333703, 0.3219752754296894559, 0.3333333333333333703, 0.3219752754296894559, 0.3333333333333333703, 0.3219752754296894559, 0.3333333333333333703, 0.3219752754296894559, 0.3333333333333333703, 0.3219752754296894559, 0.3333333333333333703, 0.3219752754296894559, 0.3333333333333333703, 0.3219752754296894559, 0.3333333333333333703, 0.3219752754296894559, 0.3333333333333333703, 0.3219752754296894559, 0.3333333333333333703, 0.3219752754296894559, 0.3333333333333333703, 0.3219752754296894559, 0.3333333333333333703, 0.3219752754296894559, 0.3333333333333333703, 0.3219752754296894559, 0.3333333333333333703, 0.3219752754296894559, 0.3333333333333333703, 0.3219752754296894559, 0.3333333333333333703, 0.3219752754296894559, 0.3333333333333333703, 0.3219752754296894559, 0.3333333333333333703, 0.3219752754296894559, 0.3333333333333333703, 0.3219752754296894559, 0.3333333333333333703, 0.3219752754296894559, 0.3333333333333333703, 0.3219752754296894559, 0.3333333333333333703, 0.3219752754296894559, 0.3333333333333333703, 0.3219752754296894559, 0.3333333333333333703, 0.3219752754296894559, 0.3333333333333333703, 0.3219752754296894559, 0.3333333333333333703, 0.3219752754296894559, 0.3333333333333333703, 0.3219752754296894559, 0.3333333333333333703, 0.3219752754296894559, 0.3333333333333333703, 0.3219752754296894559, 0.3333333333333333703, 0.3219752754296894559, 0.3333333333333333703, 0.3219752754296894559, 0.3333333333333333703, 0.3219752754296894559, 0.3333333333333333703, 0.3219752754296894559, 0.3333333333333333703, 0.3219752754296894559, 0.3333333333333333703, 0.3219752754296894559, 0.3333333333333333703, 0.3219752754296894559, 0.3333333333333333703, 0.3219752754296894559, 0.3333333333333333703, 0.3219752754296894559, 0.3333333333333333703, 0.3219752754296894559, 0.3333333333333333703, 0.3219752754296894559, 0.3333333333333333703, 0.3219752754296894559, 0.3333333333333333703, 0.3219752754296894559, 0.3333333333333333703, 0.3219752754296894559, 0.3333333333333333703, 0.3219752754296894559, 0.3333333333333333703, 0.3219752754296894559, 0.3333333333333333703, 0.3219752754296894559, 0.3333333333333333703, 0.3219752754296894559, 0.3333333333333333703, 0.3219752754296894559, 0.3333333333333333703, 0.3219752754296894559, 0.3333333333333333703, 0.3219752754296894559, 0.3333333333333333703, 0.3219752754296894559, 0.3333333333333333703, 0.3219752754296894559, 0.3333333333333333703, 0.3219752754296894559, 0.3333333333333333703, 0.3219752754296894559, 0.3333333333333333703, 0.3219752754296894559, 0.3333333333333333703, 0.3219752754296894559, 0.3333333333333333703, 0.3219752754296894559, 0.3333333333333333703, 0.3219752754296894559, 0.3333333333333333703, 0.3219752754296894559, 0.3333333333333333703, 0.3219752754296894559, 0.3333333333333333703, 0.3219752754296894559, 0.3333333333333333703, 0.3219752754296894559, 0.3333333333333333703, 0.3219752754296894559, 0.3333333333333333703, 0.3219752754296894559, 0.3333333333333333703, 0.3219752754296894559, 0.3333333333333333703, 0.3219752754296894559, 0.3333333333333333703, 0.3219752754296894559, 0.3333333333333333703, 0.3219752754296894559, 0.3333333333333333703, 0.3219752754296894559, 0.3333333333333333703, 0.3219752754296894559, 0.3333333333333333703, 0.3219752754296894559, 0.3333333333333333703, 0.3219752754296894559, 0.3333333333333333703, 0.3219752754296894559, 0.3333333333333333703, 0.3219752754296894559, 0.3333333333333333703, 0.3219752754296894559, 0.3333333333333333703, 0.3219752754296894559, 0.3333333333333333703, 0.3219752754296894559, 0.3333333333333333703, 0.3219752754296894559, 0.3333333333333333703, 0.3219752754296894559, 0.3333333333333333703, 0.3219752754296894559, 0.3333333333333333703, 0.3219752754296894559, 0.3333333333333333703, 0.3219752754296894559, 0.3333333333333333703, 0.3219752754296894559, 0.3333333333333333703, 0.3219752754296894559, 0.3333333333333333703, 0.3219752754296894559, 0.3333333333333333703, 0.3219752754296894559, 0.3333333333333333703, 0.3219752754296894559, 0.3333333333333333703, 0.3219752754296894559, 0.3333333333333333703, 0.3219752754296894559, 0.3333333333333333703, 0.3219752754296894559, 0.3333333333333333703, 0.3219752754296894559, 0.3333333333333333703, 0.3219752754296894559, 0.3333333333333333703, 0.3219752754296894559, 0.3333333333333333703, 0.3219752754296894559, 0.3333333333333333703, 0.3219752754296894559, 0.3333333333333333703, 0.3219752754296894559, 0.3333333333333333703, 0.3219752754296894559, 0.3333333333333333703, 0.3219752754296894559, 0.3333333333333333703, 0.3219752754296894559, 0.3333333333333333703, 0.3219752754296894559, 0.3333333333333333703, 0.3219752754296894559, 0.3333333333333333703, 0.3219752754296894559, 0.3333333333333333703, 0.3219752754296894559, 0.3333333333333333703, 0.3219752754296894559, 0.3333333333333333703, 0.3219752754296894559, 0.3333333333333333703, 0.3219752754296894559, 0.3333333333333333703, 0.3219752754296894559, 0.3333333333333333703, 0.3219752754296894559, 0.3333333333333333703, 0.3219752754296894559, 0.3333333333333333703, 0.3219752754296894559, 0.3333333333333333703, 0.3219752754296894559, 0.3333333333333333703, 0.3219752754296894559, 0.3333333333333333703, 0.3219752754296894559, 0.3333333333333333703, 0.3219752754296894559, 0.3333333333333333703, 0.3219752754296894559, 0.3333333333333333703, 0.3219752754296894559, 0.3333333333333333703, 0.3219752754296894559, 0.3333333333333333703, 0.3219752754296894559, 0.3333333333333333703, 0.3219752754296894559, 0.3333333333333333703, 0.3219752754296894559, 0.3333333333333333703, 0.3219752754296894559, 0.3333333333333333703, 0.3219752754296894559, 0.3333333333333333703, 0.3219752754296894559, 0.3333333333333333703, 0.3219752754296894559, 0.3333333333333333703, 0.3219752754296894559, 0.3333333333333333703, 0.3219752754296894559, 0.3333333333333333703, 0.3219752754296894559, 0.3333333333333333703, 0.3219752754296894559, 0.3333333333333333703, 0.3219752754296894559, 0.3333333333333333703, 0.3219752754296894559, 0.3333333333333333703, 0.3219752754296894559, 0.3333333333333333703, 0.3219752754296894559, 0.3333333333333333703, 0.3219752754296894559, 0.3333333333333333703, 0.3219752754296894559, 0.3333333333333333703, 0.3219752754296894559, 0.3333333333333333703, 0.3219752754296894559, 0.3333333333333333703, 0.3219752754296894559, 0.3333333333333333703, 0.3219752754296894559, 0.3333333333333333703, 0.3219752754296894559, 0.3333333333333333703, 0.3219752754296894559, 0.3333333333333333703, 0.3219752754296894559, 0.3333333333333333703, 0.3219752754296894559, 0.3333333333333333703, 0.3219752754296894559, 0.3333333333333333703, 0.3219752754296894559, 0.3333333333333333703, 0.3219752754296894559, 0.3333333333333333703, 0.3219752754296894559, 0.3333333333333333703, 0.3219752754296894559, 0.3333333333333333703, 0.3219752754296894559, 0.3333333333333333703, 0.3219752754296894559, 0.3333333333333333703, 0.3219752754296894559, 0.3333333333333333703, 0.3219752754296894559, 0.3333333333333333703, 0.3219752754296894559, 0.3333333333333333703, 0.3219752754296894559, 0.3333333333333333703, 0.3219752754296894559, 0.3333333333333333703, 0.3219752754296894559, 0.3333333333333333703, 0.3219752754296894559, 0.3333333333333333703, 0.3219752754296894559, 0.3333333333333333703, 0.3219752754296894559, 0.3333333333333333703, 0.3219752754296894559, 0.3333333333333333703, 0.3219752754296894559, 0.3333333333333333703, 0.3219752754296894559, 0.3333333333333333703, 0.3219752754296894559, 0.3333333333333333703, 0.3219752754296894559, 0.3333333333333333703, 0.3219752754296894559, 0.3333333333333333703, 0.3219752754296894559, 0.3333333333333333703, 0.3219752754296894559, 0.3333333333333333703, 0.3219752754296894559, 0.3333333333333333703, 0.3219752754296894559, 0.3333333333333333703, 0.3219752754296894559, 0.3333333333333333703, 0.3219752754296894559, 0.3333333333333333703, 0.3219752754296894559, 0.3333333333333333703, 0.3219752754296894559, 0.3333333333333333703, 0.3219752754296894559, 0.3333333333333333703, 0.3219752754296894559, 0.3333333333333333703, 0.3219752754296894559, 0.3333333333333333703, 0.3219752754296894559, 0.3333333333333333703, 0.3219752754296894559, 0.3333333333333333703, 0.3219752754296894559, 0.3333333333333333703, 0.3219752754296894559, 0.3333333333333333703, 0.3219752754296894559, 0.3333333333333333703, 0.3219752754296894559, 0.3333333333333333703, 0.3219752754296894559, 0.3333333333333333703, 0.3219752754296894559, 0.3333333333333333703, 0.3219752754296894559, 0.3333333333333333703, 0.3219752754296894559, 0.3333333333333333703, 0.3219752754296894559, 0.3333333333333333703, 0.3219752754296894559, 0.3333333333333333703, 0.3219752754296894559, 0.3333333333333333703, 0.3219752754296894559, 0.3333333333333333703, 0.3219752754296894559, 0.3333333333333333703, 0.3219752754296894559, 0.3333333333333333703, 0.3219752754296894559, 0.3333333333333333703, 0.3219752754296894559, 0.3333333333333333703, 0.3219752754296894559, 0.3333333333333333703, 0.3219752754296894559, 0.3333333333333333703, 0.3219752754296894559, 0.3333333333333333703, 0.3219752754296894559, 0.3333333333333333703, 0.3219752754296894559, 0.3333333333333333703, 0.3219752754296894559, 0.3333333333333333703, 0.3219752754296894559, 0.3333333333333333703, 0.3219752754296894559, 0.3333333333333333703, 0.3219752754296894559, 0.3333333333333333703, 0.3219752754296894559, 0.3333333333333333703, 0.3219752754296894559, 0.3333333333333333703, 0.3219752754296894559, 0.3333333333333333703, 0.3219752754296894559, 0.3333333333333333703, 0.3219752754296894559, 0.3333333333333333703, 0.3219752754296894559, 0.3333333333333333703, 0.3219752754296894559, 0.3333333333333333703, 0.3219752754296894559, 0.3333333333333333703, 0.3219752754296894559, 0.3333333333333333703, 0.3219752754296894559, 0.3333333333333333703, 0.3219752754296894559, 0.3333333333333333703, 0.3219752754296894559, 0.3333333333333333703, 0.3219752754296894559, 0.3333333333333333703),
 ( 1.000000000000000000, 0.9659258262890683122, 1.000000000000000000, 0.9659258262890683122, 1.000000000000000000, 0.9659258262890683122, 1.000000000000000000, 0.9659258262890683122, 1.000000000000000000, 0.9659258262890683122, 1.000000000000000000, 0.9659258262890683122, 1.000000000000000000, 0.9659258262890683122, 1.000000000000000000, 0.9659258262890683122, 1.000000000000000000, 0.9659258262890683122, 1.000000000000000000, 0.9659258262890683122, 1.000000000000000000, 0.9659258262890683122, 1.000000000000000000, 0.9659258262890683122, 1.000000000000000000, 0.9659258262890683122, 1.000000000000000000, 0.9659258262890683122, 1.000000000000000000, 0.9659258262890683122, 1.000000000000000000, 0.9659258262890683122, 1.000000000000000000, 0.9659258262890683122, 1.000000000000000000, 0.9659258262890683122, 1.000000000000000000, 0.9659258262890683122, 1.000000000000000000, 0.9659258262890683122, 1.000000000000000000, 0.9659258262890683122, 1.000000000000000000, 0.9659258262890683122, 1.000000000000000000, 0.9659258262890683122, 1.000000000000000000, 0.9659258262890683122, 1.000000000000000000, 0.9659258262890683122, 1.000000000000000000, 0.9659258262890683122, 1.000000000000000000, 0.9659258262890683122, 1.000000000000000000, 0.9659258262890683122, 1.000000000000000000, 0.9659258262890683122, 1.000000000000000000, 0.9659258262890683122, 1.000000000000000000, 0.9659258262890683122, 1.000000000000000000, 0.9659258262890683122, 1.000000000000000000, 0.9659258262890683122, 1.000000000000000000, 0.9659258262890683122, 1.000000000000000000, 0.9659258262890683122, 1.000000000000000000, 0.9659258262890683122, 1.000000000000000000, 0.9659258262890683122, 1.000000000000000000, 0.9659258262890683122, 1.000000000000000000, 0.9659258262890683122, 1.000000000000000000, 0.9659258262890683122, 1.000000000000000000, 0.9659258262890683122, 1.000000000000000000, 0.9659258262890683122, 1.000000000000000000, 0.9659258262890683122, 1.000000000000000000, 0.9659258262890683122, 1.000000000000000000, 0.9659258262890683122, 1.000000000000000000, 0.9659258262890683122, 1.000000000000000000, 0.9659258262890683122, 1.000000000000000000, 0.9659258262890683122, 1.000000000000000000, 0.9659258262890683122, 1.000000000000000000, 0.9659258262890683122, 1.000000000000000000, 0.9659258262890683122, 1.000000000000000000, 0.9659258262890683122, 1.000000000000000000, 0.9659258262890683122, 1.000000000000000000, 0.9659258262890683122, 1.000000000000000000, 0.9659258262890683122, 1.000000000000000000, 0.9659258262890683122, 1.000000000000000000, 0.9659258262890683122, 1.000000000000000000, 0.9659258262890683122, 1.000000000000000000, 0.9659258262890683122, 1.000000000000000000, 0.9659258262890683122, 1.000000000000000000, 0.9659258262890683122, 1.000000000000000000, 0.9659258262890683122, 1.000000000000000000, 0.9659258262890683122, 1.000000000000000000, 0.9659258262890683122, 1.000000000000000000, 0.9659258262890683122, 1.000000000000000000, 0.9659258262890683122, 1.000000000000000000, 0.9659258262890683122, 1.000000000000000000, 0.9659258262890683122, 1.000000000000000000, 0.9659258262890683122, 1.000000000000000000, 0.9659258262890683122, 1.000000000000000000, 0.9659258262890683122, 1.000000000000000000, 0.9659258262890683122, 1.000000000000000000, 0.9659258262890683122, 1.000000000000000000, 0.9659258262890683122, 1.000000000000000000, 0.9659258262890683122, 1.000000000000000000, 0.9659258262890683122, 1.000000000000000000, 0.9659258262890683122, 1.000000000000000000, 0.9659258262890683122, 1.000000000000000000, 0.9659258262890683122, 1.000000000000000000, 0.9659258262890683122, 1.000000000000000000, 0.9659258262890683122, 1.000000000000000000, 0.9659258262890683122, 1.000000000000000000, 0.9659258262890683122, 1.000000000000000000, 0.9659258262890683122, 1.000000000000000000, 0.9659258262890683122, 1.000000000000000000, 0.9659258262890683122, 1.000000000000000000, 0.9659258262890683122, 1.000000000000000000, 0.9659258262890683122, 1.000000000000000000, 0.9659258262890683122, 1.000000000000000000, 0.9659258262890683122, 1.000000000000000000, 0.9659258262890683122, 1.000000000000000000, 0.9659258262890683122, 1.000000000000000000, 0.9659258262890683122, 1.000000000000000000, 0.9659258262890683122, 1.000000000000000000, 0.9659258262890683122, 1.000000000000000000, 0.9659258262890683122, 1.000000000000000000, 0.9659258262890683122, 1.000000000000000000, 0.9659258262890683122, 1.000000000000000000, 0.9659258262890683122, 1.000000000000000000, 0.9659258262890683122, 1.000000000000000000, 0.9659258262890683122, 1.000000000000000000, 0.9659258262890683122, 1.000000000000000000, 0.9659258262890683122, 1.000000000000000000, 0.9659258262890683122, 1.000000000000000000, 0.9659258262890683122, 1.000000000000000000, 0.9659258262890683122, 1.000000000000000000, 0.9659258262890683122, 1.000000000000000000, 0.9659258262890683122, 1.000000000000000000, 0.9659258262890683122, 1.000000000000000000, 0.9659258262890683122, 1.000000000000000000, 0.9659258262890683122, 1.000000000000000000, 0.9659258262890683122, 1.000000000000000000, 0.9659258262890683122, 1.000000000000000000, 0.9659258262890683122, 1.000000000000000000, 0.9659258262890683122, 1.000000000000000000, 0.9659258262890683122, 1.000000000000000000, 0.9659258262890683122, 1.000000000000000000, 0.9659258262890683122, 1.000000000000000000, 0.9659258262890683122, 1.000000000000000000, 0.9659258262890683122, 1.000000000000000000, 0.9659258262890683122, 1.000000000000000000, 0.9659258262890683122, 1.000000000000000000, 0.9659258262890683122, 1.000000000000000000, 0.9659258262890683122, 1.000000000000000000, 0.9659258262890683122, 1.000000000000000000, 0.9659258262890683122, 1.000000000000000000, 0.9659258262890683122, 1.000000000000000000, 0.9659258262890683122, 1.000000000000000000, 0.9659258262890683122, 1.000000000000000000, 0.9659258262890683122, 1.000000000000000000, 0.9659258262890683122, 1.000000000000000000, 0.9659258262890683122, 1.000000000000000000, 0.9659258262890683122, 1.000000000000000000, 0.9659258262890683122, 1.000000000000000000, 0.9659258262890683122, 1.000000000000000000, 0.9659258262890683122, 1.000000000000000000, 0.9659258262890683122, 1.000000000000000000, 0.9659258262890683122, 1.000000000000000000, 0.9659258262890683122, 1.000000000000000000, 0.9659258262890683122, 1.000000000000000000, 0.9659258262890683122, 1.000000000000000000, 0.9659258262890683122, 1.000000000000000000, 0.9659258262890683122, 1.000000000000000000, 0.9659258262890683122, 1.000000000000000000, 0.9659258262890683122, 1.000000000000000000, 0.9659258262890683122, 1.000000000000000000, 0.9659258262890683122, 1.000000000000000000, 0.9659258262890683122, 1.000000000000000000, 0.9659258262890683122, 1.000000000000000000, 0.9659258262890683122, 1.000000000000000000, 0.9659258262890683122, 1.000000000000000000, 0.9659258262890683122, 1.000000000000000000, 0.9659258262890683122, 1.000000000000000000, 0.9659258262890683122, 1.000000000000000000, 0.9659258262890683122, 1.000000000000000000, 0.9659258262890683122, 1.000000000000000000, 0.9659258262890683122, 1.000000000000000000, 0.9659258262890683122, 1.000000000000000000, 0.9659258262890683122, 1.000000000000000000, 0.9659258262890683122, 1.000000000000000000, 0.9659258262890683122, 1.000000000000000000, 0.9659258262890683122, 1.000000000000000000, 0.9659258262890683122, 1.000000000000000000, 0.9659258262890683122, 1.000000000000000000, 0.9659258262890683122, 1.000000000000000000, 0.9659258262890683122, 1.000000000000000000, 0.9659258262890683122, 1.000000000000000000, 0.9659258262890683122, 1.000000000000000000, 0.9659258262890683122, 1.000000000000000000, 0.9659258262890683122, 1.000000000000000000, 0.9659258262890683122, 1.000000000000000000, 0.9659258262890683122, 1.000000000000000000, 0.9659258262890683122, 1.000000000000000000, 0.9659258262890683122, 1.000000000000000000, 0.9659258262890683122, 1.000000000000000000, 0.9659258262890683122, 1.000000000000000000, 0.9659258262890683122, 1.000000000000000000, 0.9659258262890683122, 1.000000000000000000, 0.9659258262890683122, 1.000000000000000000, 0.9659258262890683122, 1.000000000000000000, 0.9659258262890683122, 1.000000000000000000, 0.9659258262890683122, 1.000000000000000000, 0.9659258262890683122, 1.000000000000000000, 0.9659258262890683122, 1.000000000000000000, 0.9659258262890683122, 1.000000000000000000, 0.9659258262890683122, 1.000000000000000000, 0.9659258262890683122, 1.000000000000000000, 0.9659258262890683122, 1.000000000000000000, 0.9659258262890683122, 1.000000000000000000, 0.9659258262890683122, 1.000000000000000000, 0.9659258262890683122, 1.000000000000000000, 0.9659258262890683122, 1.000000000000000000, 0.9659258262890683122, 1.000000000000000000, 0.9659258262890683122, 1.000000000000000000, 0.9659258262890683122, 1.000000000000000000, 0.9659258262890683122, 1.000000000000000000, 0.9659258262890683122, 1.000000000000000000, 0.9659258262890683122, 1.000000000000000000, 0.9659258262890683122, 1.000000000000000000, 0.9659258262890683122, 1.000000000000000000, 0.9659258262890683122, 1.000000000000000000, 0.9659258262890683122, 1.000000000000000000, 0.9659258262890683122, 1.000000000000000000, 0.9659258262890683122, 1.000000000000000000, 0.9659258262890683122, 1.000000000000000000, 0.9659258262890683122, 1.000000000000000000, 0.9659258262890683122, 1.000000000000000000, 0.9659258262890683122, 1.000000000000000000, 0.9659258262890683122, 1.000000000000000000, 0.9659258262890683122, 1.000000000000000000, 0.9659258262890683122, 1.000000000000000000, 0.9659258262890683122, 1.000000000000000000, 0.9659258262890683122, 1.000000000000000000, 0.9659258262890683122, 1.000000000000000000, 0.9659258262890683122, 1.000000000000000000, 0.9659258262890683122, 1.000000000000000000, 0.9659258262890683122, 1.000000000000000000, 0.9659258262890683122, 1.000000000000000000, 0.9659258262890683122, 1.000000000000000000, 0.9659258262890683122, 1.000000000000000000, 0.9659258262890683122, 1.000000000000000000, 0.9659258262890683122, 1.000000000000000000, 0.9659258262890683122, 1.000000000000000000, 0.9659258262890683122, 1.000000000000000000, 0.9659258262890683122, 1.000000000000000000, 0.9659258262890683122, 1.000000000000000000, 0.9659258262890683122, 1.000000000000000000, 0.9659258262890683122, 1.000000000000000000) ) ) 
 REPRESENTATION_ITEM ( '' )  SURFACE ( )  );
#85952=CARTESIAN_POINT ( 'NONE',  ( 9.474510206698971260, -16.51473224551069308, 82.91557627198103830 ) ) ;
#85953=CARTESIAN_POINT ( 'NONE',  ( -18.67979575497193778, 10.72451020669871902, 98.33442372801901854 ) ) ;
#85954=CARTESIAN_POINT ( 'NONE',  ( -5.049401038298153566, 19.05341960407611168, 75.20724293864769550 ) ) ;
#85955=CARTESIAN_POINT ( 'NONE',  ( -15.80617190586745835, -15.72974639402198527, 46.87390960531435979 ) ) ;
#85956=CARTESIAN_POINT ( 'NONE',  ( -8.314922557960811034, -14.29746914071050412, 77.08224293864769550 ) ) ;
#85957=CARTESIAN_POINT ( 'NONE',  ( -0.05219959533909027116, -19.03943276465977164, 62.49890960531435979 ) ) ;
#85958=CARTESIAN_POINT ( 'NONE',  ( 4.379528057220339221, -16.55341960407611168, 112.7072429386476955 ) ) ;
#85959=CARTESIAN_POINT ( 'NONE',  ( 21.53943276465977519, 0.05219959533937863772, 21.25109039468567218 ) ) ;
#85960=CARTESIAN_POINT ( 'NONE',  ( -21.52544592524334988, -5.823673210054445271, 63.95942372801901854 ) ) ;
#85961=CARTESIAN_POINT ( 'NONE',  ( 19.03943276465977164, -0.05219959533909143690, 38.74890960531436690 ) ) ;
#85962=CARTESIAN_POINT ( 'NONE',  ( -8.314922557961024197, 14.29746914071037800, 57.91775706135234714 ) ) ;
#85963=CARTESIAN_POINT ( 'NONE',  ( -5.823673210054116645, -21.52544592524344225, 112.2905762719810241 ) ) ;
#85964=CARTESIAN_POINT ( 'NONE',  ( -18.62759615963270932, 10.81492255796079327, 110.8322429386476955 ) ) ;
#85965=CARTESIAN_POINT ( 'NONE',  ( -9.474510206698720793, -16.51473224551083518, 44.58442372801900433 ) ) ;
#85966=CARTESIAN_POINT ( 'NONE',  ( 13.97604488694527802, 13.89961937509977652, 69.37390960531436690 ) ) ;
#85967=CARTESIAN_POINT ( 'NONE',  ( -18.22780087662122028, 5.500000000000031086, 83.51540105326107266 ) ) ;
#85968=CARTESIAN_POINT ( 'NONE',  ( -15.80617190586768217, 15.72974639402176855, 68.12609039468567573 ) ) ;
#85969=CARTESIAN_POINT ( 'NONE',  ( -18.62759615963270932, 10.81492255796079327, 55.83224293864770260 ) ) ;
#85970=CARTESIAN_POINT ( 'NONE',  ( -8.224510206698948167, 14.34966873604960824, 40.41557627198103120 ) ) ;
#85971=CARTESIAN_POINT ( 'NONE',  ( 5.719274019375673035, 21.55341960407619339, 77.29275706135234714 ) ) ;
#85972=CARTESIAN_POINT ( 'NONE',  ( -5.823673210054431948, 21.52544592524334988, 112.7094237280190328 ) ) ;
#85973=CARTESIAN_POINT ( 'NONE',  ( 14.34966873604960469, 8.224510206698951720, 54.16557627198103120 ) ) ;
#85974=CARTESIAN_POINT ( 'NONE',  ( 8.314922557960818139, 14.29746914071049879, 99.58224293864770971 ) ) ;
#85975=CARTESIAN_POINT ( 'NONE',  ( -16.46253265017146816, -9.564922557961047289, 64.16775706135233293 ) ) ;
#85976=CARTESIAN_POINT ( 'NONE',  ( -16.53943276465976808, 0.05219959533911058130, 26.24890960531435624 ) ) ;
#85977=CARTESIAN_POINT ( 'NONE',  ( 5.719274019375673035, 21.55341960407619339, 62.29275706135236845 ) ) ;
#85979=CARTESIAN_POINT ( 'NONE',  ( 9.474510206698971260, -16.51473224551069308, 67.91557627198102409 ) ) ;
#85980=CARTESIAN_POINT ( 'NONE',  ( -19.02544592524334988, -5.153800228976617603, 28.95942372801900433 ) ) ;
#85981=CARTESIAN_POINT ( 'NONE',  ( 5.719274019375991003, -21.55341960407610458, 32.70724293864770260 ) ) ;
#85982=CARTESIAN_POINT ( 'NONE',  ( 5.823673210054444382, -21.52544592524334988, 35.20942372801901854 ) ) ;
#85983=CARTESIAN_POINT ( 'NONE',  ( -18.62759615963270932, 10.81492255796079327, 105.8322429386476955 ) ) ;
#85984=CARTESIAN_POINT ( 'NONE',  ( -16.51473224551082808, 9.474510206698731452, 98.33442372801900433 ) ) ;
#85985=CARTESIAN_POINT ( 'NONE',  ( 4.379528057220092307, 16.55341960407617563, 52.29275706135236135 ) ) ;
#85986=CARTESIAN_POINT ( 'NONE',  ( -17.49999999999999289, 5.500000000000034639, 55.79690382534172954 ) ) ;
#85987=CARTESIAN_POINT ( 'NONE',  ( 10.81492255796078972, 18.62759615963270932, 99.58224293864770971 ) ) ;
#85988=CARTESIAN_POINT ( 'NONE',  ( -4.483927247898539470, -16.52544592524342804, 87.29057627198103830 ) ) ;
#85990=CARTESIAN_POINT ( 'NONE',  ( 16.52544592524335698, 4.483927247898782831, 26.45942372801901854 ) ) ;
#85991=CARTESIAN_POINT ( 'NONE',  ( -21.53943276465977519, 0.05219959533907696930, 51.24890960531436690 ) ) ;
#85992=CARTESIAN_POINT ( 'NONE',  ( 4.483927247898790824, -16.52544592524335698, 95.20942372801903275 ) ) ;
#85995=CARTESIAN_POINT ( 'NONE',  ( 0.05219959533934541429, -16.53943276465976808, 50.00109039468568994 ) ) ;
#85996=CARTESIAN_POINT ( 'NONE',  ( -21.52544592524334988, -5.823673210054445271, 28.95942372801902209 ) ) ;
#85997=CARTESIAN_POINT ( 'NONE',  ( 15.72974639402199770, -15.80617190586745480, 48.12390960531436690 ) ) ;
#85998=CARTESIAN_POINT ( 'NONE',  ( -14.34966873604972548, 8.224510206698743886, 78.33442372801901854 ) ) ;
#85999=CARTESIAN_POINT ( 'NONE',  ( 13.97604488694527802, 13.89961937509977652, 104.3739096053143385 ) ) ;
#86000=CARTESIAN_POINT ( 'NONE',  ( -15.72974639402176322, -15.80617190586768395, 69.37609039468567573 ) ) ;
#86001=CARTESIAN_POINT ( 'NONE',  ( 21.53943276465977519, -0.05219959533907433946, 33.74890960531436690 ) ) ;
#86002=CARTESIAN_POINT ( 'NONE',  ( 10.81492255796078972, 18.62759615963270932, 24.58224293864768839 ) ) ;
#86003=ORIENTED_EDGE ( 'NONE', *, *, #27064, .F. ) ;
#86004=CARTESIAN_POINT ( 'NONE',  ( -19.03943276465977164, -0.05219959533935918106, 58.75109039468566863 ) ) ;
#86005=CARTESIAN_POINT ( 'NONE',  ( -12.14591786802326823, 12.06949235617739902, 63.12609039468568994 ) ) ;
#86006=CARTESIAN_POINT ( 'NONE',  ( -15.72974639402197994, 15.80617190586746368, 35.62390960531437401 ) ) ;
#86008=CARTESIAN_POINT ( 'NONE',  ( -9.474510206698964154, 16.51473224551069663, 90.41557627198103830 ) ) ;
#86009=CARTESIAN_POINT ( 'NONE',  ( -14.29746914071037622, -8.314922557961029526, 109.1677570613523613 ) ) ;
#86011=CARTESIAN_POINT ( 'NONE',  ( -12.14591786802309592, -12.06949235617757132, 106.8739096053143811 ) ) ;
#86012=CARTESIAN_POINT ( 'NONE',  ( -5.719274019375978568, 21.55341960407610458, 45.20724293864769550 ) ) ;
#86013=CARTESIAN_POINT ( 'NONE',  ( -13.97604488694527625, -13.89961937509977652, 41.87390960531435979 ) ) ;
#86014=CARTESIAN_POINT ( 'NONE',  ( 0.05219959533934541429, -16.53943276465976808, 80.00109039468568994 ) ) ;
#86015=CARTESIAN_POINT ( 'NONE',  ( 21.52544592524334988, 5.823673210054432836, 31.45942372801901854 ) ) ;
#86016=CARTESIAN_POINT ( 'NONE',  ( 16.51473224551083163, -9.474510206698727899, 95.83442372801900433 ) ) ;
#86017=CARTESIAN_POINT ( 'NONE',  ( -16.52544592524342804, 4.483927247898546575, 96.04057627198102409 ) ) ;
#86018=CARTESIAN_POINT ( 'NONE',  ( -5.153800228976328057, -19.02544592524343514, 57.29057627198103120 ) ) ;
#86019=VECTOR ( 'NONE', #30250, 1000.000000000000000 ) ;
#86020=CARTESIAN_POINT ( 'NONE',  ( 13.97604488694527802, 13.89961937509977652, 29.37390960531435979 ) ) ;
#86021=CARTESIAN_POINT ( 'NONE',  ( -18.62759615963255300, -10.81492255796106328, 109.1677570613523613 ) ) ;
#86022=CARTESIAN_POINT ( 'NONE',  ( 19.03943276465977164, -0.05219959533909143690, 73.74890960531435269 ) ) ;
#86023=CARTESIAN_POINT ( 'NONE',  ( -14.29746914071037622, -8.314922557961029526, 64.16775706135234714 ) ) ;
#86024=CARTESIAN_POINT ( 'NONE',  ( 21.53943276465977519, 0.05219959533937863772, 96.25109039468568994 ) ) ;
#86025=CARTESIAN_POINT ( 'NONE',  ( 16.55341960407618274, -4.379528057220086978, 71.04275706135234714 ) ) ;
#86026=CARTESIAN_POINT ( 'NONE',  ( -16.51473224551082808, 9.474510206698731452, 58.33442372801900433 ) ) ;
#86027=EDGE_CURVE ( 'NONE', #83484, #113002, #64099, .T. ) ;
#86028=CARTESIAN_POINT ( 'NONE',  ( 19.05341960407617918, -5.049401038297876454, 66.04275706135233293 ) ) ;
#86030=CARTESIAN_POINT ( 'NONE',  ( -21.53943276465977519, -0.05219959533937600094, 63.75109039468568284 ) ) ;
#86031=CARTESIAN_POINT ( 'NONE',  ( 13.97604488694527802, 13.89961937509977652, 69.37390960531436690 ) ) ;
#86032=CARTESIAN_POINT ( 'NONE',  ( -5.153800228976328057, -19.02544592524343514, 57.29057627198103120 ) ) ;
#86033=CARTESIAN_POINT ( 'NONE',  ( 9.564922557961047289, -16.46253265017146816, 65.41775706135233293 ) ) ;
#86034=CARTESIAN_POINT ( 'NONE',  ( -13.89961937509977652, 13.97604488694528158, 115.6239096053143669 ) ) ;
#86035=CARTESIAN_POINT ( 'NONE',  ( -19.03943276465977164, 0.05219959533909376836, 81.24890960531436690 ) ) ;
#86036=CARTESIAN_POINT ( 'NONE',  ( -0.05219959533910754901, -16.53943276465976808, 42.49890960531435979 ) ) ;
#86037=CARTESIAN_POINT ( 'NONE',  ( -5.823673210054116645, -21.52544592524344225, 47.29057627198103120 ) ) ;
#86039=CARTESIAN_POINT ( 'NONE',  ( 21.55341960407619695, -5.719274019375665929, 106.0427570613523471 ) ) ;
#86040=CARTESIAN_POINT ( 'NONE',  ( -9.564922557960796823, -16.46253265017161027, 52.08224293864768839 ) ) ;
#86043=CARTESIAN_POINT ( 'NONE',  ( -17.50000000000001421, -5.499999999999956479, 26.28230962303566542 ) ) ;
#86044=CARTESIAN_POINT ( 'NONE',  ( -4.483927247898782831, 16.52544592524335698, 57.70942372801901143 ) ) ;
#86045=CARTESIAN_POINT ( 'NONE',  ( -21.55341960407610458, -5.719274019375992779, 76.45724293864769550 ) ) ;
#86046=CARTESIAN_POINT ( 'NONE',  ( 12.14591786802309770, 12.06949235617756955, 59.37390960531436690 ) ) ;
#86047=CARTESIAN_POINT ( 'NONE',  ( 5.153800228976335163, 19.02544592524342804, 24.79057627198102765 ) ) ;
#86048=CARTESIAN_POINT ( 'NONE',  ( -16.46253265017160317, 9.564922557960807481, 115.8322429386477097 ) ) ;
#86049=CARTESIAN_POINT ( 'NONE',  ( 0.05219959533937995610, -21.53943276465977519, 40.00109039468567573 ) ) ;
#86050=CARTESIAN_POINT ( 'NONE',  ( 16.46253265017146816, 9.564922557961045513, 46.66775706135233293 ) ) ;
#86051=CARTESIAN_POINT ( 'NONE',  ( -5.153800228976328057, -19.02544592524343514, 37.29057627198102409 ) ) ;
#86052=CARTESIAN_POINT ( 'NONE',  ( 18.62759615963255655, 10.81492255796105972, 86.66775706135234714 ) ) ;
#86054=CARTESIAN_POINT ( 'NONE',  ( -16.52544592524342804, 4.483927247898546575, 36.04057627198102409 ) ) ;
#86055=CARTESIAN_POINT ( 'NONE',  ( 17.49999999999999645, 5.076555817581245300, 113.6795149204977236 ) ) ;
#86056=CARTESIAN_POINT ( 'NONE',  ( -15.80617190586745835, -15.72974639402198527, 46.87390960531435979 ) ) ;
#86058=CARTESIAN_POINT ( 'NONE',  ( -13.89961937509977652, 13.97604488694528158, 85.62390960531433848 ) ) ;
#86059=CARTESIAN_POINT ( 'NONE',  ( 8.314922557960818139, 14.29746914071049879, 94.58224293864769550 ) ) ;
#86060=CARTESIAN_POINT ( 'NONE',  ( -4.483927247898782831, 16.52544592524335698, 22.70942372801901499 ) ) ;
#86061=CARTESIAN_POINT ( 'NONE',  ( -21.52544592524343514, 5.823673210054127303, 61.04057627198103120 ) ) ;
#86063=CARTESIAN_POINT ( 'NONE',  ( 19.03943276465977164, -0.05219959533909143690, 33.74890960531435979 ) ) ;
#86064=CARTESIAN_POINT ( 'NONE',  ( -16.51473224551069308, -9.474510206698971260, 86.66557627198102409 ) ) ;
#86065=CARTESIAN_POINT ( 'NONE',  ( -10.72451020669898014, 18.67979575497178502, 95.41557627198102409 ) ) ;
#86066=CARTESIAN_POINT ( 'NONE',  ( 4.379528057220092307, 16.55341960407617563, 112.2927570613523471 ) ) ;
#86067=CARTESIAN_POINT ( 'NONE',  ( 5.049401038298161559, -19.05341960407611168, 97.70724293864766707 ) ) ;
#86068=CARTESIAN_POINT ( 'NONE',  ( 9.564922557961047289, -16.46253265017146816, 85.41775706135233293 ) ) ;
#86069=CARTESIAN_POINT ( 'NONE',  ( -15.80617190586768217, 15.72974639402176855, 103.1260903946856757 ) ) ;
#86070=CARTESIAN_POINT ( 'NONE',  ( -10.72451020669898014, 18.67979575497178502, 70.41557627198102409 ) ) ;
#86071=CARTESIAN_POINT ( 'NONE',  ( -15.72974639402197994, 15.80617190586746368, 35.62390960531437401 ) ) ;
#86072=CARTESIAN_POINT ( 'NONE',  ( 9.564922557960805705, 16.46253265017160317, 54.58224293864769550 ) ) ;
#86073=CARTESIAN_POINT ( 'NONE',  ( 12.14591786802309770, 12.06949235617756955, 24.37390960531435979 ) ) ;
#86074=CARTESIAN_POINT ( 'NONE',  ( 19.05341960407611168, 5.049401038298154454, 73.95724293864768129 ) ) ;
#86076=CARTESIAN_POINT ( 'NONE',  ( 9.564922557961047289, -16.46253265017146816, 30.41775706135232937 ) ) ;
#86077=CARTESIAN_POINT ( 'NONE',  ( -16.52544592524342804, 4.483927247898546575, 91.04057627198103830 ) ) ;
#86078=CARTESIAN_POINT ( 'NONE',  ( 5.719274019375673035, 21.55341960407619339, 22.29275706135235069 ) ) ;
#86080=CARTESIAN_POINT ( 'NONE',  ( 21.52544592524344225, -5.823673210054117533, 68.54057627198103830 ) ) ;
#86081=CARTESIAN_POINT ( 'NONE',  ( -12.14591786802326823, 12.06949235617739902, 88.12609039468570415 ) ) ;
#86082=CARTESIAN_POINT ( 'NONE',  ( -8.314922557960811034, -14.29746914071050412, 112.0822429386477097 ) ) ;
#86083=CARTESIAN_POINT ( 'NONE',  ( 16.46253265017160672, -9.564922557960803928, 73.33224293864769550 ) ) ;
#86086=CARTESIAN_POINT ( 'NONE',  ( -0.05219959533910754901, -16.53943276465976808, 32.49890960531435979 ) ) ;
#86087=CARTESIAN_POINT ( 'NONE',  ( -15.72974639402176322, -15.80617190586768395, 59.37609039468568284 ) ) ;
#86088=CARTESIAN_POINT ( 'NONE',  ( -19.05341960407611168, -5.049401038298163336, 106.4572429386476955 ) ) ;
#86089=CARTESIAN_POINT ( 'NONE',  ( -21.52544592524334988, -5.823673210054445271, 88.95942372801901854 ) ) ;
#86090=CARTESIAN_POINT ( 'NONE',  ( 13.97604488694527802, 13.89961937509977652, 44.37390960531435269 ) ) ;
#86091=CARTESIAN_POINT ( 'NONE',  ( -19.02544592524342804, 5.153800228976336051, 51.04057627198103120 ) ) ;
#86092=EDGE_LOOP ( 'NONE', ( #137838, #150006 ) ) ;
#86093=CARTESIAN_POINT ( 'NONE',  ( -10.72451020669870658, -18.67979575497194134, 99.58442372801900433 ) ) ;
#86094=CARTESIAN_POINT ( 'NONE',  ( -12.06949235617739369, -12.14591786802326823, 64.37609039468568994 ) ) ;
#86095=CARTESIAN_POINT ( 'NONE',  ( -15.80617190586768217, 15.72974639402176855, 83.12609039468568994 ) ) ;
#86096=CARTESIAN_POINT ( 'NONE',  ( -10.72451020669898014, 18.67979575497178502, 25.41557627198103120 ) ) ;
#86097=CARTESIAN_POINT ( 'NONE',  ( -13.89961937509957401, -13.97604488694547875, 94.37609039468566152 ) ) ;
#86098=CARTESIAN_POINT ( 'NONE',  ( 15.72974639402176855, 15.80617190586768217, 56.87609039468568994 ) ) ;
#86099=CARTESIAN_POINT ( 'NONE',  ( 4.379528057220092307, 16.55341960407617563, 42.29275706135235424 ) ) ;
#86100=CARTESIAN_POINT ( 'NONE',  ( 0.05219959533907565091, 21.53943276465977519, 84.99890960531436690 ) ) ;
#86101=CARTESIAN_POINT ( 'NONE',  ( -5.153800228976607833, 19.02544592524334988, 82.70942372801897591 ) ) ;
#86102=CARTESIAN_POINT ( 'NONE',  ( -13.97604488694527625, -13.89961937509977652, 66.87390960531436690 ) ) ;
#86103=CARTESIAN_POINT ( 'NONE',  ( 19.05341960407617918, -5.049401038297876454, 101.0427570613523045 ) ) ;
#86104=CARTESIAN_POINT ( 'NONE',  ( -19.02544592524334988, -5.153800228976617603, 83.95942372801901854 ) ) ;
#86105=CARTESIAN_POINT ( 'NONE',  ( 16.52544592524342804, -4.483927247898539470, 53.54057627198103120 ) ) ;
#86107=CARTESIAN_POINT ( 'NONE',  ( -13.89961937509957401, -13.97604488694547875, 79.37609039468567573 ) ) ;
#86108=CARTESIAN_POINT ( 'NONE',  ( -14.29746914071037622, -8.314922557961029526, 59.16775706135234714 ) ) ;
#86109=CARTESIAN_POINT ( 'NONE',  ( 13.97604488694548053, -13.89961937509957401, 35.62609039468567573 ) ) ;
#86110=CARTESIAN_POINT ( 'NONE',  ( 5.049401038298161559, -19.05341960407611168, 42.70724293864767418 ) ) ;
#86111=CARTESIAN_POINT ( 'NONE',  ( -0.05219959533909027116, -19.03943276465977164, 37.49890960531436690 ) ) ;
#86112=CARTESIAN_POINT ( 'NONE',  ( -14.34966873604972548, 8.224510206698743886, 63.33442372801900433 ) ) ;
#86115=CARTESIAN_POINT ( 'NONE',  ( 13.89961937509977652, -13.97604488694527269, 108.1239096053143669 ) ) ;
#86116=CARTESIAN_POINT ( 'NONE',  ( -16.46253265017160317, 9.564922557960807481, 25.83224293864769194 ) ) ;
#86118=CARTESIAN_POINT ( 'NONE',  ( 16.51473224551083163, -9.474510206698727899, 100.8344237280190043 ) ) ;
#86119=CARTESIAN_POINT ( 'NONE',  ( -18.62759615963270932, 10.81492255796079327, 40.83224293864769550 ) ) ;
#86120=CARTESIAN_POINT ( 'NONE',  ( 5.153800228976615827, -19.02544592524334988, 25.20942372801900433 ) ) ;
#86121=CARTESIAN_POINT ( 'NONE',  ( 9.474510206698729675, 16.51473224551082808, 107.0844237280190043 ) ) ;
#86122=CARTESIAN_POINT ( 'NONE',  ( -16.46253265017160317, 9.564922557960807481, 25.83224293864769194 ) ) ;
#86123=CARTESIAN_POINT ( 'NONE',  ( 13.97604488694527802, 13.89961937509977652, 44.37390960531435269 ) ) ;
#86124=CARTESIAN_POINT ( 'NONE',  ( 21.52544592524344225, -5.823673210054117533, 68.54057627198103830 ) ) ;
#86125=CARTESIAN_POINT ( 'NONE',  ( 16.46253265017160672, -9.564922557960803928, 98.33224293864769550 ) ) ;
#86126=CARTESIAN_POINT ( 'NONE',  ( -5.049401038298153566, 19.05341960407611168, 40.20724293864768839 ) ) ;
#86128=CARTESIAN_POINT ( 'NONE',  ( 9.564922557961047289, -16.46253265017146816, 90.41775706135234714 ) ) ;
#86129=CARTESIAN_POINT ( 'NONE',  ( 14.34966873604960469, 8.224510206698951720, 49.16557627198102409 ) ) ;
#86130=CARTESIAN_POINT ( 'NONE',  ( 21.55341960407610458, 5.719274019375980345, 33.95724293864769550 ) ) ;
#86131=CARTESIAN_POINT ( 'NONE',  ( -21.53943276465977519, -0.05219959533937600094, 103.7510903946857042 ) ) ;
#86132=CARTESIAN_POINT ( 'NONE',  ( 5.719274019375991003, -21.55341960407610458, 102.7072429386476955 ) ) ;
#86133=CARTESIAN_POINT ( 'NONE',  ( -10.81492255796105439, 18.62759615963255655, 77.91775706135231871 ) ) ;
#86134=CARTESIAN_POINT ( 'NONE',  ( -21.52544592524334988, -5.823673210054445271, 73.95942372801901854 ) ) ;
#86136=CARTESIAN_POINT ( 'NONE',  ( 19.02544592524343514, -5.153800228976328945, 113.5405762719810241 ) ) ;
#86137=CARTESIAN_POINT ( 'NONE',  ( 4.379528057220092307, 16.55341960407617563, 112.2927570613523471 ) ) ;
#86138=CARTESIAN_POINT ( 'NONE',  ( -0.05219959533937732626, 21.53943276465977519, 57.50109039468568994 ) ) ;
#86139=CARTESIAN_POINT ( 'NONE',  ( 19.03943276465977164, -0.05219959533909143690, 68.74890960531436690 ) ) ;
#86140=CARTESIAN_POINT ( 'NONE',  ( 16.51473224551083163, -9.474510206698727899, 40.83442372801900433 ) ) ;
#86141=CARTESIAN_POINT ( 'NONE',  ( 18.67979575497194134, -10.72451020669871369, 35.83442372801901143 ) ) ;
#86142=CARTESIAN_POINT ( 'NONE',  ( -13.89961937509977652, 13.97604488694528158, 65.62390960531436690 ) ) ;
#86143=CARTESIAN_POINT ( 'NONE',  ( 8.224510206698953496, -14.34966873604960469, 77.91557627198102409 ) ) ;
#86144=CARTESIAN_POINT ( 'NONE',  ( -16.53943276465976808, 0.05219959533911058130, 41.24890960531435269 ) ) ;
#86145=CARTESIAN_POINT ( 'NONE',  ( -18.62759615963270932, 10.81492255796079327, 50.83224293864770971 ) ) ;
#86146=CARTESIAN_POINT ( 'NONE',  ( -9.564922557960796823, -16.46253265017161027, 57.08224293864769550 ) ) ;
#86147=CARTESIAN_POINT ( 'NONE',  ( 21.52544592524344225, -5.823673210054117533, 78.54057627198103830 ) ) ;
#86148=CARTESIAN_POINT ( 'NONE',  ( -5.049401038297874678, -19.05341960407617918, 44.79275706135232582 ) ) ;
#86150=CARTESIAN_POINT ( 'NONE',  ( -5.049401038297874678, -19.05341960407618274, 19.79275706135233293 ) ) ;
#86151=CARTESIAN_POINT ( 'NONE',  ( -12.14591786802309592, -12.06949235617757132, 56.87390960531436690 ) ) ;
#86152=CARTESIAN_POINT ( 'NONE',  ( -18.62759615963270932, 10.81492255796079327, 40.83224293864769550 ) ) ;
#86155=CARTESIAN_POINT ( 'NONE',  ( -0.05219959533934338120, 16.53943276465976808, 87.50109039468568994 ) ) ;
#86157=CARTESIAN_POINT ( 'NONE',  ( 19.02544592524334988, 5.153800228976608722, 91.45942372801900433 ) ) ;
#86158=CARTESIAN_POINT ( 'NONE',  ( 16.52544592524342804, -4.483927247898539470, 48.54057627198103120 ) ) ;
#86159=CARTESIAN_POINT ( 'NONE',  ( -18.22780087662121673, -5.500000000000063061, 61.48459894673894155 ) ) ;
#86160=CARTESIAN_POINT ( 'NONE',  ( 9.564922557960805705, 16.46253265017160317, 44.58224293864769550 ) ) ;
#86161=CARTESIAN_POINT ( 'NONE',  ( 14.34966873604960469, 8.224510206698951720, 44.16557627198103120 ) ) ;
#86162=CARTESIAN_POINT ( 'NONE',  ( 13.89961937509977652, -13.97604488694527269, 88.12390960531438111 ) ) ;
#86163=CARTESIAN_POINT ( 'NONE',  ( -5.153800228976328057, -19.02544592524343514, 52.29057627198100988 ) ) ;
#86164=CARTESIAN_POINT ( 'NONE',  ( -18.62759615963255300, -10.81492255796106328, 64.16775706135234714 ) ) ;
#86165=CARTESIAN_POINT ( 'NONE',  ( -13.97604488694527625, -13.89961937509977652, 71.87390960531433848 ) ) ;
#86166=CARTESIAN_POINT ( 'NONE',  ( 0.05219959533909260263, 19.03943276465977164, 29.99890960531435979 ) ) ;
#86168=CARTESIAN_POINT ( 'NONE',  ( 13.89961937509977652, -13.97604488694527269, 78.12390960531433848 ) ) ;
#86169=CARTESIAN_POINT ( 'NONE',  ( 5.823673210054125526, 21.52544592524343514, 44.79057627198103120 ) ) ;
#86170=CARTESIAN_POINT ( 'NONE',  ( 16.51473224551069308, 9.474510206698969483, 34.16557627198102409 ) ) ;
#86171=CARTESIAN_POINT ( 'NONE',  ( 10.81492255796078972, 18.62759615963270932, 44.58224293864769550 ) ) ;
#86172=CARTESIAN_POINT ( 'NONE',  ( -16.53943276465976808, -0.05219959533934237506, 103.7510903946857042 ) ) ;
#86173=CARTESIAN_POINT ( 'NONE',  ( 5.049401038297881783, 19.05341960407617563, 22.29275706135233648 ) ) ;
#86174=CARTESIAN_POINT ( 'NONE',  ( -8.314922557961024197, 14.29746914071037800, 47.91775706135234714 ) ) ;
#86175=CARTESIAN_POINT ( 'NONE',  ( -16.52544592524335698, -4.483927247898792601, 78.95942372801901854 ) ) ;
#86177=CARTESIAN_POINT ( 'NONE',  ( -16.53943276465976808, -0.05219959533934237506, 73.75109039468567573 ) ) ;
#86178=CARTESIAN_POINT ( 'NONE',  ( -21.52544592524343514, 5.823673210054127303, 26.04057627198103475 ) ) ;
#86179=CARTESIAN_POINT ( 'NONE',  ( 13.89961937509977652, -13.97604488694527269, 33.12390960531434558 ) ) ;
#86180=CARTESIAN_POINT ( 'NONE',  ( 12.14591786802327356, -12.06949235617739191, 35.62609039468568994 ) ) ;
#86181=CARTESIAN_POINT ( 'NONE',  ( -9.564922557960796823, -16.46253265017161027, 52.08224293864768839 ) ) ;
#86182=CARTESIAN_POINT ( 'NONE',  ( 5.719274019375673035, 21.55341960407619339, 37.29275706135235424 ) ) ;
#86183=CARTESIAN_POINT ( 'NONE',  ( 16.55341960407618274, -4.379528057220086978, 36.04275706135234714 ) ) ;
#86184=CARTESIAN_POINT ( 'NONE',  ( -14.29746914071037622, -8.314922557961029526, 104.1677570613523471 ) ) ;
#86186=CARTESIAN_POINT ( 'NONE',  ( 18.67979575497194134, -10.72451020669871369, 95.83442372801903275 ) ) ;
#86187=CARTESIAN_POINT ( 'NONE',  ( 9.564922557961047289, -16.46253265017146816, 90.41775706135234714 ) ) ;
#86188=CARTESIAN_POINT ( 'NONE',  ( -0.05219959533936034679, 19.03943276465977164, 52.50109039468566863 ) ) ;
#86189=CARTESIAN_POINT ( 'NONE',  ( -16.55341960407611168, -4.379528057220339221, 66.45724293864768129 ) ) ;
#86190=CARTESIAN_POINT ( 'NONE',  ( 4.483927247898545687, 16.52544592524342804, 114.7905762719810383 ) ) ;
#86191=CARTESIAN_POINT ( 'NONE',  ( -5.049401038297874678, -19.05341960407617918, 59.79275706135231871 ) ) ;
#86192=CARTESIAN_POINT ( 'NONE',  ( 17.48853670773247870, 5.747243402303063853, 78.83328700250008580 ) ) ;
#86193=CARTESIAN_POINT ( 'NONE',  ( -5.823673210054431948, 21.52544592524334988, 62.70942372801902565 ) ) ;
#86194=CARTESIAN_POINT ( 'NONE',  ( -16.52544592524335698, -4.483927247898792601, 33.95942372801901143 ) ) ;
#86195=CARTESIAN_POINT ( 'NONE',  ( -17.49999999999998579, 5.500000000000031974, 90.79690382534171533 ) ) ;
#86196=CARTESIAN_POINT ( 'NONE',  ( 0.05219959533907565091, 21.53943276465977519, 24.99890960531435624 ) ) ;
#86197=CARTESIAN_POINT ( 'NONE',  ( -9.564922557961040184, 16.46253265017147172, 112.9177570613523329 ) ) ;
#86198=CARTESIAN_POINT ( 'NONE',  ( -16.51473224551069308, -9.474510206698971260, 111.6655762719810383 ) ) ;
#86200=CARTESIAN_POINT ( 'NONE',  ( -16.52544592524342804, 4.483927247898546575, 116.0405762719810383 ) ) ;
#86201=CARTESIAN_POINT ( 'NONE',  ( -15.80617190586768217, 15.72974639402176855, 108.1260903946856757 ) ) ;
#86202=CARTESIAN_POINT ( 'NONE',  ( -16.46253265017160317, 9.564922557960807481, 60.83224293864769550 ) ) ;
#86203=CARTESIAN_POINT ( 'NONE',  ( -0.05219959533937732626, 21.53943276465977519, 67.50109039468568994 ) ) ;
#86204=CARTESIAN_POINT ( 'NONE',  ( 15.80617190586769283, -15.72974639402175789, 95.62609039468568994 ) ) ;
#86205=CARTESIAN_POINT ( 'NONE',  ( -4.483927247898539470, -16.52544592524342804, 22.29057627198102765 ) ) ;
#86206=CARTESIAN_POINT ( 'NONE',  ( 16.51473224551069308, 9.474510206698969483, 79.16557627198103830 ) ) ;
#86207=CARTESIAN_POINT ( 'NONE',  ( 15.72974639402176855, 15.80617190586768217, 61.87609039468568284 ) ) ;
#86208=CARTESIAN_POINT ( 'NONE',  ( -15.72974639402176322, -15.80617190586768395, 49.37609039468569705 ) ) ;
#86209=CARTESIAN_POINT ( 'NONE',  ( 16.46253265017146816, 9.564922557961045513, 76.66775706135234714 ) ) ;
#86210=CARTESIAN_POINT ( 'NONE',  ( -19.02544592524342804, 5.153800228976336051, 111.0405762719810099 ) ) ;
#86211=CARTESIAN_POINT ( 'NONE',  ( 13.89961937509977652, -13.97604488694527269, 23.12390960531436335 ) ) ;
#86212=CARTESIAN_POINT ( 'NONE',  ( 10.72451020669898902, -18.67979575497178502, 102.9155762719810383 ) ) ;
#86213=CARTESIAN_POINT ( 'NONE',  ( -9.564922557961040184, 16.46253265017147172, 37.91775706135233293 ) ) ;
#86214=CARTESIAN_POINT ( 'NONE',  ( -14.29746914071049879, 8.314922557960819915, 90.83224293864769550 ) ) ;
#86215=CARTESIAN_POINT ( 'NONE',  ( -9.474510206698964154, 16.51473224551069663, 45.41557627198103120 ) ) ;
#86216=CARTESIAN_POINT ( 'NONE',  ( 5.049401038297881783, 19.05341960407617563, 102.2927570613523045 ) ) ;
#86217=CARTESIAN_POINT ( 'NONE',  ( -16.52544592524342804, 4.483927247898546575, 56.04057627198102409 ) ) ;
#86218=CARTESIAN_POINT ( 'NONE',  ( 15.72974639402176855, 15.80617190586768217, 106.8760903946856899 ) ) ;
#86219=CARTESIAN_POINT ( 'NONE',  ( 13.97604488694527802, 13.89961937509977652, 99.37390960531436690 ) ) ;
#86220=CARTESIAN_POINT ( 'NONE',  ( -9.474510206698720793, -16.51473224551083518, 74.58442372801900433 ) ) ;
#86221=CARTESIAN_POINT ( 'NONE',  ( -21.53943276465977519, 0.05219959533907696930, 96.24890960531435269 ) ) ;
#86222=CARTESIAN_POINT ( 'NONE',  ( 5.823673210054444382, -21.52544592524334988, 45.20942372801901854 ) ) ;
#86223=CARTESIAN_POINT ( 'NONE',  ( 14.34966873604972726, -8.224510206698740333, 45.83442372801901854 ) ) ;
#86224=CARTESIAN_POINT ( 'NONE',  ( -4.483927247898782831, 16.52544592524335698, 87.70942372801901854 ) ) ;
#86225=CARTESIAN_POINT ( 'NONE',  ( 16.53943276465976808, 0.05219959533934440121, 41.25109039468568284 ) ) ;
#86226=CARTESIAN_POINT ( 'NONE',  ( -0.05219959533937732626, 21.53943276465977519, 32.50109039468568284 ) ) ;
#86227=CARTESIAN_POINT ( 'NONE',  ( 15.80617190586746368, 15.72974639402197994, 39.37390960531436690 ) ) ;
#86228=CARTESIAN_POINT ( 'NONE',  ( -19.05341960407611168, -5.049401038298163336, 36.45724293864766707 ) ) ;
#86230=CARTESIAN_POINT ( 'NONE',  ( -16.55341960407617563, 4.379528057220093196, 58.54275706135235424 ) ) ;
#86231=CARTESIAN_POINT ( 'NONE',  ( -10.72451020669898014, 18.67979575497178502, 95.41557627198102409 ) ) ;
#86232=CARTESIAN_POINT ( 'NONE',  ( -4.483927247898539470, -16.52544592524342804, 32.29057627198102409 ) ) ;
#86233=CARTESIAN_POINT ( 'NONE',  ( -8.314922557961024197, 14.29746914071037800, 67.91775706135234714 ) ) ;
#86234=CARTESIAN_POINT ( 'NONE',  ( 19.05341960407611168, 5.049401038298154454, 63.95724293864769550 ) ) ;
#86235=CARTESIAN_POINT ( 'NONE',  ( 13.97604488694548053, -13.89961937509957401, 85.62609039468568994 ) ) ;
#86236=CARTESIAN_POINT ( 'NONE',  ( 18.67979575497178502, 10.72451020669898547, 79.16557627198103830 ) ) ;
#86237=CARTESIAN_POINT ( 'NONE',  ( 12.14591786802309770, 12.06949235617756955, 29.37390960531435269 ) ) ;
#86238=ORIENTED_EDGE ( 'NONE', *, *, #46300, .F. ) ;
#86240=CARTESIAN_POINT ( 'NONE',  ( -21.55341960407610458, -5.719274019375992779, 66.45724293864768129 ) ) ;
#86242=CARTESIAN_POINT ( 'NONE',  ( -12.14591786802326823, 12.06949235617739902, 103.1260903946856757 ) ) ;
#86245=CARTESIAN_POINT ( 'NONE',  ( -10.81492255796078084, -18.62759615963271287, 92.08224293864769550 ) ) ;
#86246=CARTESIAN_POINT ( 'NONE',  ( -16.55341960407611168, -4.379528057220339221, 21.45724293864769550 ) ) ;
#86247=CARTESIAN_POINT ( 'NONE',  ( -14.29746914071037622, -8.314922557961029526, 34.16775706135234714 ) ) ;
#86248=CARTESIAN_POINT ( 'NONE',  ( 0.05219959533909260263, 19.03943276465977164, 29.99890960531435979 ) ) ;
#86249=CARTESIAN_POINT ( 'NONE',  ( -19.03943276465977164, 0.05219959533909376836, 66.24890960531436690 ) ) ;
#86251=CARTESIAN_POINT ( 'NONE',  ( -0.05219959533907301413, -21.53943276465977519, 22.49890960531436335 ) ) ;
#86253=CARTESIAN_POINT ( 'NONE',  ( 16.55341960407618274, -4.379528057220086978, 101.0427570613523756 ) ) ;
#86254=CARTESIAN_POINT ( 'NONE',  ( 19.03943276465977164, 0.05219959533936151252, 111.2510903946856757 ) ) ;
#86255=CARTESIAN_POINT ( 'NONE',  ( 13.97604488694548053, -13.89961937509957401, 35.62609039468567573 ) ) ;
#86256=CARTESIAN_POINT ( 'NONE',  ( -5.823673210054116645, -21.52544592524344225, 87.29057627198103830 ) ) ;
#86257=CARTESIAN_POINT ( 'NONE',  ( -8.314922557960811034, -14.29746914071050412, 22.08224293864769194 ) ) ;
#86258=CARTESIAN_POINT ( 'NONE',  ( -10.81492255796078084, -18.62759615963271287, 52.08224293864768839 ) ) ;
#86259=CARTESIAN_POINT ( 'NONE',  ( 10.81492255796078972, 18.62759615963270932, 84.58224293864769550 ) ) ;
#86260=CARTESIAN_POINT ( 'NONE',  ( 9.474510206698729675, 16.51473224551082808, 112.0844237280190043 ) ) ;
#86261=CARTESIAN_POINT ( 'NONE',  ( 5.049401038298161559, -19.05341960407611168, 107.7072429386476955 ) ) ;
#86262=CARTESIAN_POINT ( 'NONE',  ( -21.55341960407619339, 5.719274019375674811, 78.54275706135236135 ) ) ;
#86263=CARTESIAN_POINT ( 'NONE',  ( 5.153800228976335163, 19.02544592524342804, 64.79057627198100988 ) ) ;
#86264=CARTESIAN_POINT ( 'NONE',  ( -12.14591786802309592, -12.06949235617757132, 106.8739096053143811 ) ) ;
#86266=CARTESIAN_POINT ( 'NONE',  ( 16.51473224551069308, 9.474510206698969483, 74.16557627198103830 ) ) ;
#86267=CARTESIAN_POINT ( 'NONE',  ( 8.224510206698953496, -14.34966873604960469, 92.91557627198103830 ) ) ;
#86269=CARTESIAN_POINT ( 'NONE',  ( 5.153800228976615827, -19.02544592524334988, 95.20942372801897591 ) ) ;
#86270=CARTESIAN_POINT ( 'NONE',  ( 17.40861289039004944, -6.110651285853253789, 81.12767529172569425 ) ) ;
#86271=CARTESIAN_POINT ( 'NONE',  ( -9.564922557960796823, -16.46253265017161027, 57.08224293864769550 ) ) ;
#86272=CARTESIAN_POINT ( 'NONE',  ( -15.80617190586768217, 15.72974639402176855, 88.12609039468570415 ) ) ;
#86273=CARTESIAN_POINT ( 'NONE',  ( -13.89961937509977652, 13.97604488694528158, 95.62390960531436690 ) ) ;
#86274=CARTESIAN_POINT ( 'NONE',  ( -16.52544592524335698, -4.483927247898792601, 73.95942372801901854 ) ) ;
#86275=CARTESIAN_POINT ( 'NONE',  ( -17.50000000000000711, -5.500000000000025757, 51.28230962303570095 ) ) ;
#86276=CARTESIAN_POINT ( 'NONE',  ( -9.474510206698720793, -16.51473224551083518, 49.58442372801899722 ) ) ;
#86277=CARTESIAN_POINT ( 'NONE',  ( -5.719274019375665041, -21.55341960407619695, 104.7927570613523898 ) ) ;
#86280=CARTESIAN_POINT ( 'NONE',  ( -4.483927247898782831, 16.52544592524335698, 102.7094237280190185 ) ) ;
#86282=CARTESIAN_POINT ( 'NONE',  ( 4.379528057220092307, 16.55341960407617563, 87.29275706135236135 ) ) ;
#86284=CARTESIAN_POINT ( 'NONE',  ( 4.483927247898790824, -16.52544592524335698, 70.20942372801904696 ) ) ;
#86285=ORIENTED_EDGE ( 'NONE', *, *, #89035, .F. ) ;
#86287=CARTESIAN_POINT ( 'NONE',  ( 0.05219959533937995610, -21.53943276465977519, 75.00109039468568994 ) ) ;
#86288=CARTESIAN_POINT ( 'NONE',  ( 0.05219959533936267826, -19.03943276465977164, 90.00109039468567573 ) ) ;
#86289=CARTESIAN_POINT ( 'NONE',  ( 0.05219959533936267826, -19.03943276465977164, 30.00109039468566863 ) ) ;
#86290=CARTESIAN_POINT ( 'NONE',  ( 13.97604488694527802, 13.89961937509977652, 69.37390960531436690 ) ) ;
#86291=CARTESIAN_POINT ( 'NONE',  ( 16.51473224551069308, 9.474510206698969483, 59.16557627198102409 ) ) ;
#86292=DIRECTION ( 'NONE',  ( 0.000000000000000000, 0.000000000000000000, -1.000000000000000000 ) ) ;
#86293=CARTESIAN_POINT ( 'NONE',  ( 0.05219959533907565091, 21.53943276465977519, 74.99890960531435269 ) ) ;
#86294=AXIS2_PLACEMENT_3D ( 'NONE', #155248, #156237, #90587 ) ;
#86295=CARTESIAN_POINT ( 'NONE',  ( 15.72974639402199770, -15.80617190586745480, 33.12390960531435979 ) ) ;
#86296=CARTESIAN_POINT ( 'NONE',  ( 13.89961937509977652, -13.97604488694527269, 33.12390960531434558 ) ) ;
#86297=CARTESIAN_POINT ( 'NONE',  ( 14.34966873604972726, -8.224510206698740333, 65.83442372801900433 ) ) ;
#86299=CARTESIAN_POINT ( 'NONE',  ( 18.67979575497194134, -10.72451020669871369, 30.83442372801902209 ) ) ;
#86300=CARTESIAN_POINT ( 'NONE',  ( 8.224510206698953496, -14.34966873604960469, 67.91557627198102409 ) ) ;
#86302=CARTESIAN_POINT ( 'NONE',  ( 16.55341960407618274, -4.379528057220086978, 21.04275706135234714 ) ) ;
#86303=CARTESIAN_POINT ( 'NONE',  ( -16.46253265017146816, -9.564922557961047289, 59.16775706135233293 ) ) ;
#86304=CARTESIAN_POINT ( 'NONE',  ( 16.52544592524342804, -4.483927247898539470, 63.54057627198103830 ) ) ;
#86305=CARTESIAN_POINT ( 'NONE',  ( 5.823673210054444382, -21.52544592524334988, 30.20942372801902565 ) ) ;
#86307=CARTESIAN_POINT ( 'NONE',  ( 15.72974639402199770, -15.80617190586745480, 78.12390960531436690 ) ) ;
#86308=CARTESIAN_POINT ( 'NONE',  ( 19.02544592524343514, -5.153800228976328945, 98.54057627198100988 ) ) ;
#86309=CARTESIAN_POINT ( 'NONE',  ( -12.14591786802309592, -12.06949235617757132, 61.87390960531436690 ) ) ;
#86312=CARTESIAN_POINT ( 'NONE',  ( -16.51473224551082808, 9.474510206698731452, 63.33442372801900433 ) ) ;
#86313=CARTESIAN_POINT ( 'NONE',  ( 10.72451020669898902, -18.67979575497178502, 107.9155762719810241 ) ) ;
#86314=CARTESIAN_POINT ( 'NONE',  ( 5.049401038298161559, -19.05341960407611168, 57.70724293864769550 ) ) ;
#86316=CARTESIAN_POINT ( 'NONE',  ( 5.153800228976615827, -19.02544592524334988, 40.20942372801898301 ) ) ;
#86317=CARTESIAN_POINT ( 'NONE',  ( 19.02544592524343514, -5.153800228976328945, 28.54057627198102409 ) ) ;
#86318=CARTESIAN_POINT ( 'NONE',  ( 21.52544592524334988, 5.823673210054432836, 66.45942372801903275 ) ) ;
#86321=CARTESIAN_POINT ( 'NONE',  ( -8.314922557960811034, -14.29746914071050412, 47.08224293864770260 ) ) ;
#86322=CARTESIAN_POINT ( 'NONE',  ( -0.05219959533909027116, -19.03943276465977164, 67.49890960531436690 ) ) ;
#86323=CARTESIAN_POINT ( 'NONE',  ( 5.823673210054125526, 21.52544592524343514, 79.79057627198102409 ) ) ;
#86324=CARTESIAN_POINT ( 'NONE',  ( 13.97604488694527802, 13.89961937509977652, 64.37390960531436690 ) ) ;
#86326=CARTESIAN_POINT ( 'NONE',  ( 15.72974639402199770, -15.80617190586745480, 63.12390960531435979 ) ) ;
#86327=CARTESIAN_POINT ( 'NONE',  ( 15.80617190586769283, -15.72974639402175789, 95.62609039468568994 ) ) ;
#86329=CARTESIAN_POINT ( 'NONE',  ( -4.379528057220086978, -16.55341960407618274, 89.79275706135236135 ) ) ;
#86330=CARTESIAN_POINT ( 'NONE',  ( -14.34966873604960291, -8.224510206698953496, 76.66557627198103830 ) ) ;
#86331=CARTESIAN_POINT ( 'NONE',  ( 9.474510206698729675, 16.51473224551082808, 97.08442372801900433 ) ) ;
#86332=ORIENTED_EDGE ( 'NONE', *, *, #28653, .F. ) ;
#86333=CARTESIAN_POINT ( 'NONE',  ( 13.97604488694548053, -13.89961937509957401, 35.62609039468567573 ) ) ;
#86334=CARTESIAN_POINT ( 'NONE',  ( -12.14591786802326823, 12.06949235617739902, 108.1260903946856757 ) ) ;
#86335=CARTESIAN_POINT ( 'NONE',  ( -13.89961937509957401, -13.97604488694547875, 29.37609039468565797 ) ) ;
#86336=CARTESIAN_POINT ( 'NONE',  ( 13.89961937509977652, -13.97604488694527269, 93.12390960531436690 ) ) ;
#86337=CARTESIAN_POINT ( 'NONE',  ( 5.823673210054125526, 21.52544592524343514, 59.79057627198103120 ) ) ;
#86339=CARTESIAN_POINT ( 'NONE',  ( 16.53943276465976808, -0.05219959533910856209, 113.7489096053143527 ) ) ;
#86340=CARTESIAN_POINT ( 'NONE',  ( 10.81492255796106328, -18.62759615963255655, 95.41775706135234714 ) ) ;
#86341=CARTESIAN_POINT ( 'NONE',  ( 16.52544592524335698, 4.483927247898782831, 71.45942372801901854 ) ) ;
#86342=CARTESIAN_POINT ( 'NONE',  ( -18.62759615963255300, -10.81492255796106328, 29.16775706135234003 ) ) ;
#86343=CARTESIAN_POINT ( 'NONE',  ( 4.483927247898790824, -16.52544592524335698, 25.20942372801901854 ) ) ;
#86344=CARTESIAN_POINT ( 'NONE',  ( -19.03943276465977164, 0.05219959533909376836, 111.2489096053143669 ) ) ;
#86345=CARTESIAN_POINT ( 'NONE',  ( 9.564922557960805705, 16.46253265017160317, 39.58224293864768839 ) ) ;
#86346=CARTESIAN_POINT ( 'NONE',  ( -0.05219959533909027116, -19.03943276465977164, 57.49890960531435979 ) ) ;
#86348=CARTESIAN_POINT ( 'NONE',  ( 4.483927247898790824, -16.52544592524335698, 50.20942372801901854 ) ) ;
#86349=CARTESIAN_POINT ( 'NONE',  ( -8.314922557960811034, -14.29746914071050412, 92.08224293864769550 ) ) ;
#86350=CARTESIAN_POINT ( 'NONE',  ( 14.29746914071037800, 8.314922557961029526, 106.6677570613523756 ) ) ;
#86351=CARTESIAN_POINT ( 'NONE',  ( -10.81492255796105439, 18.62759615963255655, 37.91775706135235424 ) ) ;
#86352=CARTESIAN_POINT ( 'NONE',  ( 19.02544592524343514, -5.153800228976328945, 83.54057627198100988 ) ) ;
#86353=CARTESIAN_POINT ( 'NONE',  ( -19.02544592524342804, 5.153800228976336051, 61.04057627198103120 ) ) ;
#86354=CARTESIAN_POINT ( 'NONE',  ( -5.049401038298153566, 19.05341960407611168, 85.20724293864766707 ) ) ;
#86355=CARTESIAN_POINT ( 'NONE',  ( 14.34966873604960469, 8.224510206698951720, 29.16557627198103120 ) ) ;
#86356=CARTESIAN_POINT ( 'NONE',  ( -8.224510206698735004, -14.34966873604973081, 104.5844237280190185 ) ) ;
#86358=CARTESIAN_POINT ( 'NONE',  ( -13.89961937509957401, -13.97604488694547875, 49.37609039468567573 ) ) ;
#86359=CARTESIAN_POINT ( 'NONE',  ( 19.05341960407611168, 5.049401038298154454, 113.9572429386477097 ) ) ;
#86360=CARTESIAN_POINT ( 'NONE',  ( -16.51473224551069308, -9.474510206698971260, 56.66557627198103120 ) ) ;
#86361=CARTESIAN_POINT ( 'NONE',  ( 9.564922557961047289, -16.46253265017146816, 45.41775706135232582 ) ) ;
#86363=CARTESIAN_POINT ( 'NONE',  ( -16.53943276465976808, -0.05219959533934237506, 43.75109039468568284 ) ) ;
#86364=CARTESIAN_POINT ( 'NONE',  ( 19.03943276465977164, 0.05219959533936151252, 76.25109039468566152 ) ) ;
#86365=CARTESIAN_POINT ( 'NONE',  ( 4.483927247898790824, -16.52544592524335698, 60.20942372801902565 ) ) ;
#86367=CARTESIAN_POINT ( 'NONE',  ( -9.564922557960796823, -16.46253265017161027, 87.08224293864769550 ) ) ;
#86368=CARTESIAN_POINT ( 'NONE',  ( -18.67979575497178146, -10.72451020669898902, 111.6655762719810525 ) ) ;
#86369=CARTESIAN_POINT ( 'NONE',  ( -5.049401038297874678, -19.05341960407617918, 74.79275706135231871 ) ) ;
#86370=CARTESIAN_POINT ( 'NONE',  ( -13.97604488694527625, -13.89961937509977652, 106.8739096053143669 ) ) ;
#86371=CARTESIAN_POINT ( 'NONE',  ( -16.51473224551069308, -9.474510206698971260, 31.66557627198102054 ) ) ;
#86372=CARTESIAN_POINT ( 'NONE',  ( 5.049401038298161559, -19.05341960407611168, 82.70724293864770971 ) ) ;
#86373=CARTESIAN_POINT ( 'NONE',  ( -12.14591786802309592, -12.06949235617757132, 36.87390960531435979 ) ) ;
#86374=CARTESIAN_POINT ( 'NONE',  ( -16.51473224551069308, -9.474510206698971260, 31.66557627198102054 ) ) ;
#86375=CARTESIAN_POINT ( 'NONE',  ( 19.03943276465977164, 0.05219959533936151252, 56.25109039468566863 ) ) ;
#86376=CARTESIAN_POINT ( 'NONE',  ( 16.55341960407611168, 4.379528057220329451, 93.95724293864770971 ) ) ;
#86377=CARTESIAN_POINT ( 'NONE',  ( -10.72451020669870658, -18.67979575497194134, 109.5844237280190328 ) ) ;
#86378=CARTESIAN_POINT ( 'NONE',  ( 13.97604488694527802, 13.89961937509977652, 54.37390960531435979 ) ) ;
#86379=ADVANCED_FACE ( 'NONE', ( #90574 ), #46065, .F. ) ;
#86380=CARTESIAN_POINT ( 'NONE',  ( 21.53943276465977519, -0.05219959533907433946, 48.74890960531435979 ) ) ;
#86381=CARTESIAN_POINT ( 'NONE',  ( 0.05219959533910956823, 16.53943276465976808, 59.99890960531436690 ) ) ;
#86382=CARTESIAN_POINT ( 'NONE',  ( -0.05219959533937732626, 21.53943276465977519, 97.50109039468567573 ) ) ;
#86383=CARTESIAN_POINT ( 'NONE',  ( -13.97604488694527625, -13.89961937509977652, 111.8739096053143243 ) ) ;
#86384=CARTESIAN_POINT ( 'NONE',  ( -13.97604488694527625, -13.89961937509977652, 101.8739096053143811 ) ) ;
#86385=CARTESIAN_POINT ( 'NONE',  ( -16.46253265017160317, 9.564922557960807481, 45.83224293864769550 ) ) ;
#86386=CARTESIAN_POINT ( 'NONE',  ( -0.05219959533909027116, -19.03943276465977164, 22.49890960531436690 ) ) ;
#86387=CARTESIAN_POINT ( 'NONE',  ( 12.06949235617757843, -12.14591786802309237, 93.12390960531436690 ) ) ;
#86388=CARTESIAN_POINT ( 'NONE',  ( -10.72451020669898014, 18.67979575497178502, 95.41557627198102409 ) ) ;
#86389=CARTESIAN_POINT ( 'NONE',  ( -19.03943276465977164, 0.05219959533909376836, 96.24890960531436690 ) ) ;
#86390=CARTESIAN_POINT ( 'NONE',  ( -18.62759615963255300, -10.81492255796106328, 19.16775706135234714 ) ) ;
#86391=CARTESIAN_POINT ( 'NONE',  ( -19.05341960407611168, -5.049401038298163336, 101.4572429386476955 ) ) ;
#86393=CARTESIAN_POINT ( 'NONE',  ( 8.314922557960818139, 14.29746914071049879, 99.58224293864770971 ) ) ;
#86394=CARTESIAN_POINT ( 'NONE',  ( 5.153800228976335163, 19.02544592524342804, 74.79057627198103830 ) ) ;
#86395=CARTESIAN_POINT ( 'NONE',  ( -21.55341960407610458, -5.719274019375992779, 76.45724293864769550 ) ) ;
#86397=CARTESIAN_POINT ( 'NONE',  ( 15.72974639402199770, -15.80617190586745480, 28.12390960531435979 ) ) ;
#86399=CARTESIAN_POINT ( 'NONE',  ( -8.314922557961024197, 14.29746914071037800, 32.91775706135234714 ) ) ;
#86400=CARTESIAN_POINT ( 'NONE',  ( -16.53943276465976808, 0.05219959533911058130, 96.24890960531435269 ) ) ;
#86402=CARTESIAN_POINT ( 'NONE',  ( -19.02544592524342804, 5.153800228976336051, 86.04057627198103830 ) ) ;
#86403=CARTESIAN_POINT ( 'NONE',  ( 5.049401038298161559, -19.05341960407611168, 62.70724293864769550 ) ) ;
#86404=CARTESIAN_POINT ( 'NONE',  ( 16.53943276465976808, -0.05219959533910856209, 78.74890960531436690 ) ) ;
#86405=CARTESIAN_POINT ( 'NONE',  ( 21.52544592524344225, -5.823673210054117533, 33.54057627198102409 ) ) ;
#86406=CARTESIAN_POINT ( 'NONE',  ( 16.53943276465976808, -0.05219959533910856209, 58.74890960531436690 ) ) ;
#86407=CARTESIAN_POINT ( 'NONE',  ( 12.14591786802327356, -12.06949235617739191, 25.62609039468567929 ) ) ;
#86408=CARTESIAN_POINT ( 'NONE',  ( 21.52544592524334988, 5.823673210054432836, 71.45942372801901854 ) ) ;
#86410=CARTESIAN_POINT ( 'NONE',  ( -9.474510206698964154, 16.51473224551069663, 115.4155762719810241 ) ) ;
#86411=CARTESIAN_POINT ( 'NONE',  ( -4.379528057220086978, -16.55341960407618274, 89.79275706135236135 ) ) ;
#86412=CARTESIAN_POINT ( 'NONE',  ( -13.97604488694527625, -13.89961937509977652, 26.87390960531434558 ) ) ;
#86413=CARTESIAN_POINT ( 'NONE',  ( 16.51473224551069308, 9.474510206698969483, 84.16557627198102409 ) ) ;
#86414=CARTESIAN_POINT ( 'NONE',  ( 21.53943276465977519, -0.05219959533907433946, 98.74890960531438111 ) ) ;
#86415=CARTESIAN_POINT ( 'NONE',  ( 16.52544592524335698, 4.483927247898782831, 26.45942372801901854 ) ) ;
#86416=CARTESIAN_POINT ( 'NONE',  ( -0.05219959533910754901, -16.53943276465976808, 52.49890960531435979 ) ) ;
#86417=CARTESIAN_POINT ( 'NONE',  ( -15.80617190586768217, 15.72974639402176855, 78.12609039468570415 ) ) ;
#86418=CARTESIAN_POINT ( 'NONE',  ( -4.379528057220086978, -16.55341960407618274, 89.79275706135236135 ) ) ;
#86419=CARTESIAN_POINT ( 'NONE',  ( -5.049401038298153566, 19.05341960407611168, 115.2072429386477097 ) ) ;
#86420=CARTESIAN_POINT ( 'NONE',  ( 17.26058549869090797, 6.457015423128630971, 28.87745837476070321 ) ) ;
#86421=CARTESIAN_POINT ( 'NONE',  ( -16.19135201231366139, 7.376712067591925326, 79.81319145947969673 ) ) ;
#86422=CARTESIAN_POINT ( 'NONE',  ( -8.224510206698735004, -14.34966873604973081, 109.5844237280190328 ) ) ;
#86423=CARTESIAN_POINT ( 'NONE',  ( 4.379528057220092307, 16.55341960407617563, 62.29275706135236845 ) ) ;
#86424=CARTESIAN_POINT ( 'NONE',  ( -16.51473224551069308, -9.474510206698971260, 66.66557627198102409 ) ) ;
#86425=CARTESIAN_POINT ( 'NONE',  ( -13.89961937509977652, 13.97604488694528158, 80.62390960531436690 ) ) ;
#86426=CARTESIAN_POINT ( 'NONE',  ( -21.52544592524334988, -5.823673210054445271, 68.95942372801901854 ) ) ;
#86427=CARTESIAN_POINT ( 'NONE',  ( -16.55341960407617563, 4.379528057220093196, 73.54275706135234714 ) ) ;
#86428=CARTESIAN_POINT ( 'NONE',  ( 16.55341960407611168, 4.379528057220329451, 48.95724293864770971 ) ) ;
#86429=CARTESIAN_POINT ( 'NONE',  ( -19.02544592524342804, 5.153800228976336051, 61.04057627198103120 ) ) ;
#86430=CARTESIAN_POINT ( 'NONE',  ( 13.97604488694527802, 13.89961937509977652, 54.37390960531435979 ) ) ;
#86432=CARTESIAN_POINT ( 'NONE',  ( -14.29746914071037622, -8.314922557961029526, 19.16775706135234714 ) ) ;
#86433=CARTESIAN_POINT ( 'NONE',  ( 16.53943276465976808, -0.05219959533910856209, 108.7489096053143669 ) ) ;
#86434=CARTESIAN_POINT ( 'NONE',  ( 9.474510206698971260, -16.51473224551069308, 62.91557627198102409 ) ) ;
#86435=CARTESIAN_POINT ( 'NONE',  ( -13.89961937509957401, -13.97604488694547875, 99.37609039468567573 ) ) ;
#86437=CARTESIAN_POINT ( 'NONE',  ( -10.81492255796105439, 18.62759615963255655, 97.91775706135236135 ) ) ;
#86438=CARTESIAN_POINT ( 'NONE',  ( 16.55341960407618274, -4.379528057220086978, 66.04275706135236135 ) ) ;
#86439=CARTESIAN_POINT ( 'NONE',  ( 5.153800228976615827, -19.02544592524334988, 95.20942372801897591 ) ) ;
#86440=CARTESIAN_POINT ( 'NONE',  ( -18.67979575497178146, -10.72451020669898902, 61.66557627198103120 ) ) ;
#86441=CARTESIAN_POINT ( 'NONE',  ( -16.52544592524335698, -4.483927247898792601, 58.95942372801902565 ) ) ;
#86443=CARTESIAN_POINT ( 'NONE',  ( -13.89961937509957401, -13.97604488694547875, 59.37609039468566863 ) ) ;
#86444=CARTESIAN_POINT ( 'NONE',  ( -15.72974639402176322, -15.80617190586768395, 99.37609039468568994 ) ) ;
#86445=CARTESIAN_POINT ( 'NONE',  ( 14.34966873604960469, 8.224510206698951720, 114.1655762719810383 ) ) ;
#86446=CARTESIAN_POINT ( 'NONE',  ( 19.02544592524343514, -5.153800228976328945, 68.54057627198103830 ) ) ;
#86447=CARTESIAN_POINT ( 'NONE',  ( 16.53943276465976808, -0.05219959533910856209, 58.74890960531436690 ) ) ;
#86449=CARTESIAN_POINT ( 'NONE',  ( 21.52544592524334988, 5.823673210054432836, 96.45942372801901854 ) ) ;
#86450=CARTESIAN_POINT ( 'NONE',  ( -5.049401038297874678, -19.05341960407617918, 44.79275706135232582 ) ) ;
#86451=CARTESIAN_POINT ( 'NONE',  ( -9.474510206698720793, -16.51473224551083518, 34.58442372801899722 ) ) ;
#86452=CARTESIAN_POINT ( 'NONE',  ( 9.474510206698971260, -16.51473224551069308, 112.9155762719810383 ) ) ;
#86453=CARTESIAN_POINT ( 'NONE',  ( -21.52544592524334988, -5.823673210054445271, 93.95942372801903275 ) ) ;
#86454=CARTESIAN_POINT ( 'NONE',  ( 9.474510206698971260, -16.51473224551069308, 82.91557627198103830 ) ) ;
#86455=CARTESIAN_POINT ( 'NONE',  ( 5.719274019375673035, 21.55341960407619339, 97.29275706135234714 ) ) ;
#86456=CARTESIAN_POINT ( 'NONE',  ( -5.719274019375978568, 21.55341960407610458, 55.20724293864770260 ) ) ;
#86457=CARTESIAN_POINT ( 'NONE',  ( -13.89961937509977652, 13.97604488694528158, 80.62390960531436690 ) ) ;
#86458=CARTESIAN_POINT ( 'NONE',  ( 13.89961937509957401, 13.97604488694547697, 71.87609039468567573 ) ) ;
#86459=CARTESIAN_POINT ( 'NONE',  ( -16.51473224551069308, -9.474510206698971260, 46.66557627198102409 ) ) ;
#86460=CARTESIAN_POINT ( 'NONE',  ( 16.51473224551069308, 9.474510206698969483, 84.16557627198102409 ) ) ;
#86461=CARTESIAN_POINT ( 'NONE',  ( 13.97604488694548053, -13.89961937509957401, 85.62609039468568994 ) ) ;
#86462=CARTESIAN_POINT ( 'NONE',  ( 8.314922557961029526, -14.29746914071037800, 40.41775706135234714 ) ) ;
#86463=CARTESIAN_POINT ( 'NONE',  ( 4.483927247898545687, 16.52544592524342804, 104.7905762719810241 ) ) ;
#86464=CARTESIAN_POINT ( 'NONE',  ( -19.03943276465977164, 0.05219959533909376836, 76.24890960531435269 ) ) ;
#86465=CARTESIAN_POINT ( 'NONE',  ( 5.719274019375991003, -21.55341960407610458, 47.70724293864770260 ) ) ;
#86466=CARTESIAN_POINT ( 'NONE',  ( 8.224510206698742110, 14.34966873604972548, 32.08442372801901854 ) ) ;
#86467=CARTESIAN_POINT ( 'NONE',  ( 18.67979575497194134, -10.72451020669871369, 35.83442372801901143 ) ) ;
#86468=CARTESIAN_POINT ( 'NONE',  ( -18.62759615963255300, -10.81492255796106328, 89.16775706135236135 ) ) ;
#86469=CARTESIAN_POINT ( 'NONE',  ( -4.379528057220086978, -16.55341960407618274, 84.79275706135234714 ) ) ;
#86470=CARTESIAN_POINT ( 'NONE',  ( -19.03943276465977164, 0.05219959533909376836, 81.24890960531436690 ) ) ;
#86471=CARTESIAN_POINT ( 'NONE',  ( -0.05219959533934338120, 16.53943276465976808, 102.5010903946856899 ) ) ;
#86472=CARTESIAN_POINT ( 'NONE',  ( -19.02544592524334988, -5.153800228976617603, 53.95942372801898301 ) ) ;
#86474=CARTESIAN_POINT ( 'NONE',  ( 21.55341960407619695, -5.719274019375665929, 36.04275706135234714 ) ) ;
#86475=CARTESIAN_POINT ( 'NONE',  ( -12.06949235617756955, 12.14591786802309770, 75.62390960531439532 ) ) ;
#86476=CARTESIAN_POINT ( 'NONE',  ( -19.02544592524342804, 5.153800228976336051, 101.0405762719810241 ) ) ;
#86477=CARTESIAN_POINT ( 'NONE',  ( 12.06949235617739724, 12.14591786802326823, 106.8760903946856899 ) ) ;
#86478=CARTESIAN_POINT ( 'NONE',  ( -18.67979575497193778, 10.72451020669871902, 73.33442372801901854 ) ) ;
#86479=CARTESIAN_POINT ( 'NONE',  ( -14.34966873604972548, 8.224510206698743886, 43.33442372801901143 ) ) ;
#86480=CARTESIAN_POINT ( 'NONE',  ( 5.823673210054444382, -21.52544592524334988, 30.20942372801902565 ) ) ;
#86481=CARTESIAN_POINT ( 'NONE',  ( 14.34966873604960469, 8.224510206698951720, 69.16557627198102409 ) ) ;
#86483=CARTESIAN_POINT ( 'NONE',  ( -5.823673210054431948, 21.52544592524334988, 22.70942372801901499 ) ) ;
#86484=CARTESIAN_POINT ( 'NONE',  ( -16.53943276465976808, 0.05219959533911058130, 51.24890960531436690 ) ) ;
#86486=CARTESIAN_POINT ( 'NONE',  ( 15.72974639402199770, -15.80617190586745480, 28.12390960531435979 ) ) ;
#86487=CARTESIAN_POINT ( 'NONE',  ( -21.52544592524334988, -5.823673210054445271, 53.95942372801900433 ) ) ;
#86488=CARTESIAN_POINT ( 'NONE',  ( 8.224510206698953496, -14.34966873604960469, 62.91557627198102409 ) ) ;
#86489=CARTESIAN_POINT ( 'NONE',  ( 18.67979575497178502, 10.72451020669898547, 74.16557627198102409 ) ) ;
#86490=CARTESIAN_POINT ( 'NONE',  ( 9.564922557960805705, 16.46253265017160317, 79.58224293864769550 ) ) ;
#86491=CARTESIAN_POINT ( 'NONE',  ( -19.05341960407611168, -5.049401038298163336, 36.45724293864766707 ) ) ;
#86492=CARTESIAN_POINT ( 'NONE',  ( 5.153800228976615827, -19.02544592524334988, 75.20942372801896170 ) ) ;
#86493=CARTESIAN_POINT ( 'NONE',  ( -18.67979575497193778, 10.72451020669871902, 53.33442372801901854 ) ) ;
#86494=CARTESIAN_POINT ( 'NONE',  ( 10.81492255796078972, 18.62759615963270932, 64.58224293864769550 ) ) ;
#86495=CARTESIAN_POINT ( 'NONE',  ( -9.564922557960796823, -16.46253265017161027, 42.08224293864769550 ) ) ;
#86496=CARTESIAN_POINT ( 'NONE',  ( -9.564922557960796823, -16.46253265017161027, 67.08224293864769550 ) ) ;
#86497=ORIENTED_EDGE ( 'NONE', *, *, #126426, .F. ) ;
#86498=CARTESIAN_POINT ( 'NONE',  ( 12.14591786802327356, -12.06949235617739191, 55.62609039468568284 ) ) ;
#86499=CARTESIAN_POINT ( 'NONE',  ( -21.55341960407619339, 5.719274019375674811, 28.54275706135234358 ) ) ;
#86500=CARTESIAN_POINT ( 'NONE',  ( 18.67979575497194134, -10.72451020669871369, 55.83442372801901854 ) ) ;
#86501=CARTESIAN_POINT ( 'NONE',  ( -19.03943276465977164, 0.05219959533909376836, 101.2489096053143669 ) ) ;
#86502=CARTESIAN_POINT ( 'NONE',  ( 21.55341960407610458, 5.719274019375980345, 88.95724293864769550 ) ) ;
#86503=CARTESIAN_POINT ( 'NONE',  ( -5.823673210054431948, 21.52544592524334988, 22.70942372801901499 ) ) ;
#86504=CARTESIAN_POINT ( 'NONE',  ( -12.14591786802326823, 12.06949235617739902, 53.12609039468568284 ) ) ;
#86505=CARTESIAN_POINT ( 'NONE',  ( 21.55341960407610458, 5.719274019375980345, 43.95724293864769550 ) ) ;
#86506=CARTESIAN_POINT ( 'NONE',  ( 19.02544592524334988, 5.153800228976608722, 26.45942372801899722 ) ) ;
#86507=CARTESIAN_POINT ( 'NONE',  ( -9.474510206698964154, 16.51473224551069663, 60.41557627198102409 ) ) ;
#86508=CARTESIAN_POINT ( 'NONE',  ( -9.474510206698964154, 16.51473224551069663, 105.4155762719810383 ) ) ;
#86509=CARTESIAN_POINT ( 'NONE',  ( -5.049401038298153566, 19.05341960407611168, 95.20724293864770971 ) ) ;
#86510=CARTESIAN_POINT ( 'NONE',  ( 17.49999999999999645, 3.341627039121310982, 102.9223102399844976 ) ) ;
#86512=CARTESIAN_POINT ( 'NONE',  ( 19.05341960407617918, -5.049401038297876454, 66.04275706135233293 ) ) ;
#86513=CARTESIAN_POINT ( 'NONE',  ( -18.62759615963270932, 10.81492255796079327, 45.83224293864769550 ) ) ;
#86514=CARTESIAN_POINT ( 'NONE',  ( 0.05219959533910956823, 16.53943276465976808, 29.99890960531435979 ) ) ;
#86515=CARTESIAN_POINT ( 'NONE',  ( 13.97604488694548053, -13.89961937509957401, 80.62609039468567573 ) ) ;
#86516=CARTESIAN_POINT ( 'NONE',  ( -17.49999999999998579, 5.500000000000032863, 60.79690382534172244 ) ) ;
#86517=CARTESIAN_POINT ( 'NONE',  ( 5.823673210054444382, -21.52544592524334988, 110.2094237280190185 ) ) ;
#86518=CARTESIAN_POINT ( 'NONE',  ( -9.564922557961040184, 16.46253265017147172, 77.91775706135234714 ) ) ;
#86519=CARTESIAN_POINT ( 'NONE',  ( -19.03943276465977164, -0.05219959533935918106, 43.75109039468566863 ) ) ;
#86521=CARTESIAN_POINT ( 'NONE',  ( -16.46253265017160317, 9.564922557960807481, 60.83224293864769550 ) ) ;
#86522=CARTESIAN_POINT ( 'NONE',  ( 16.52544592524342804, -4.483927247898539470, 53.54057627198103120 ) ) ;
#86523=CARTESIAN_POINT ( 'NONE',  ( -19.05341960407611168, -5.049401038298163336, 31.45724293864769550 ) ) ;
#86524=CARTESIAN_POINT ( 'NONE',  ( -16.53943276465976808, 0.05219959533911058130, 46.24890960531435979 ) ) ;
#86525=CARTESIAN_POINT ( 'NONE',  ( -19.03943276465977164, -1.327063459122257427E-13, 20.00000000000001776 ) ) ;
#86526=CARTESIAN_POINT ( 'NONE',  ( -12.14591786802326823, 12.06949235617739902, 113.1260903946856899 ) ) ;
#86527=CARTESIAN_POINT ( 'NONE',  ( 13.97604488694527802, 13.89961937509977652, 69.37390960531436690 ) ) ;
#86528=CARTESIAN_POINT ( 'NONE',  ( 19.02544592524334988, 5.153800228976608722, 31.45942372801900433 ) ) ;
#86529=CARTESIAN_POINT ( 'NONE',  ( -8.314922557961024197, 14.29746914071037800, 37.91775706135235424 ) ) ;
#86530=CARTESIAN_POINT ( 'NONE',  ( -15.72974639402197994, 15.80617190586746368, 35.62390960531437401 ) ) ;
#86531=CARTESIAN_POINT ( 'NONE',  ( 21.53943276465977519, 0.05219959533937863772, 86.25109039468568994 ) ) ;
#86533=CARTESIAN_POINT ( 'NONE',  ( 19.02544592524343514, -5.153800228976328945, 63.54057627198103830 ) ) ;
#86534=CARTESIAN_POINT ( 'NONE',  ( 16.51473224551069308, 9.474510206698969483, 104.1655762719810241 ) ) ;
#86535=CARTESIAN_POINT ( 'NONE',  ( 19.05341960407611168, 5.049401038298154454, 98.95724293864766707 ) ) ;
#86537=CARTESIAN_POINT ( 'NONE',  ( -21.55341960407619339, 5.719274019375674811, 23.54275706135235424 ) ) ;
#86538=CARTESIAN_POINT ( 'NONE',  ( 12.14591786802309770, 12.06949235617756955, 79.37390960531436690 ) ) ;
#86539=CARTESIAN_POINT ( 'NONE',  ( 18.67979575497178502, 10.72451020669898547, 79.16557627198103830 ) ) ;
#86540=CARTESIAN_POINT ( 'NONE',  ( 19.05341960407611168, 5.049401038298154454, 73.95724293864768129 ) ) ;
#86541=CARTESIAN_POINT ( 'NONE',  ( -13.89961937509977652, 13.97604488694528158, 75.62390960531438111 ) ) ;
#86542=CARTESIAN_POINT ( 'NONE',  ( 15.72974639402199770, -15.80617190586745480, 108.1239096053143811 ) ) ;
#86544=CARTESIAN_POINT ( 'NONE',  ( 9.564922557960805705, 16.46253265017160317, 74.58224293864769550 ) ) ;
#86545=CARTESIAN_POINT ( 'NONE',  ( 12.14591786802309770, 12.06949235617756955, 104.3739096053143669 ) ) ;
#86546=CARTESIAN_POINT ( 'NONE',  ( 16.46253265017160672, -9.564922557960803928, 23.33224293864769194 ) ) ;
#86547=CARTESIAN_POINT ( 'NONE',  ( -16.51473224551069308, -9.474510206698971260, 61.66557627198103120 ) ) ;
#86548=CARTESIAN_POINT ( 'NONE',  ( 5.153800228976615827, -19.02544592524334988, 90.20942372801900433 ) ) ;
#86549=CARTESIAN_POINT ( 'NONE',  ( 14.29746914071049879, -8.314922557960816363, 93.33224293864769550 ) ) ;
#86550=CARTESIAN_POINT ( 'NONE',  ( 18.62759615963255655, 10.81492255796105972, 76.66775706135234714 ) ) ;
#86551=CARTESIAN_POINT ( 'NONE',  ( -16.46253265017160317, 9.564922557960807481, 50.83224293864770260 ) ) ;
#86552=CARTESIAN_POINT ( 'NONE',  ( -15.80617190586745835, -15.72974639402198527, 111.8739096053143669 ) ) ;
#86553=CARTESIAN_POINT ( 'NONE',  ( 15.72974639402199770, -15.80617190586745480, 108.1239096053143811 ) ) ;
#86555=CARTESIAN_POINT ( 'NONE',  ( 0.05219959533909260263, 19.03943276465977164, 69.99890960531435269 ) ) ;
#86557=CARTESIAN_POINT ( 'NONE',  ( 13.89961937509957401, 13.97604488694547697, 106.8760903946856757 ) ) ;
#86558=CARTESIAN_POINT ( 'NONE',  ( 21.52544592524344225, -5.823673210054117533, 28.54057627198103120 ) ) ;
#86559=CARTESIAN_POINT ( 'NONE',  ( -5.719274019375665041, -21.55341960407619695, 44.79275706135234714 ) ) ;
#86560=CARTESIAN_POINT ( 'NONE',  ( 19.02544592524343514, -5.153800228976328945, 93.54057627198102409 ) ) ;
#86561=CARTESIAN_POINT ( 'NONE',  ( -16.46253265017146816, -9.564922557961047289, 84.16775706135233293 ) ) ;
#86562=CARTESIAN_POINT ( 'NONE',  ( 13.97604488694527802, 13.89961937509977652, 49.37390960531434558 ) ) ;
#86563=CARTESIAN_POINT ( 'NONE',  ( 9.474510206698971260, -16.51473224551069308, 72.91557627198102409 ) ) ;
#86564=CARTESIAN_POINT ( 'NONE',  ( -8.224510206698948167, 14.34966873604960824, 85.41557627198102409 ) ) ;
#86565=CARTESIAN_POINT ( 'NONE',  ( 13.97604488694527802, 13.89961937509977652, 104.3739096053143385 ) ) ;
#86566=CARTESIAN_POINT ( 'NONE',  ( 16.53943276465976808, -0.05219959533910856209, 93.74890960531436690 ) ) ;
#86567=CARTESIAN_POINT ( 'NONE',  ( -0.05219959533909027116, -19.03943276465977164, 102.4989096053143669 ) ) ;
#86568=CARTESIAN_POINT ( 'NONE',  ( 14.34966873604960469, 8.224510206698951720, 39.16557627198102409 ) ) ;
#86569=CARTESIAN_POINT ( 'NONE',  ( -13.97604488694527625, -13.89961937509977652, 21.87390960531435979 ) ) ;
#86571=CARTESIAN_POINT ( 'NONE',  ( 5.719274019375673035, 21.55341960407619339, 52.29275706135236135 ) ) ;
#86572=CARTESIAN_POINT ( 'NONE',  ( 19.03943276465977164, 0.05219959533936151252, 86.25109039468567573 ) ) ;
#86573=CARTESIAN_POINT ( 'NONE',  ( -0.05219959533910754901, -16.53943276465976808, 42.49890960531435979 ) ) ;
#86574=CARTESIAN_POINT ( 'NONE',  ( 5.823673210054125526, 21.52544592524343514, 99.79057627198103830 ) ) ;
#86575=CARTESIAN_POINT ( 'NONE',  ( -10.72451020669898014, 18.67979575497178502, 40.41557627198103120 ) ) ;
#86576=CARTESIAN_POINT ( 'NONE',  ( -4.379528057220328563, 16.55341960407611168, 85.20724293864770971 ) ) ;
#86577=CARTESIAN_POINT ( 'NONE',  ( 19.03943276465977164, -0.05219959533909143690, 58.74890960531435979 ) ) ;
#86578=CARTESIAN_POINT ( 'NONE',  ( 4.379528057220339221, -16.55341960407611168, 22.70724293864769194 ) ) ;
#86580=CARTESIAN_POINT ( 'NONE',  ( -8.224510206698735004, -14.34966873604973081, 99.58442372801900433 ) ) ;
#86581=CARTESIAN_POINT ( 'NONE',  ( -4.483927247898782831, 16.52544592524335698, 67.70942372801901854 ) ) ;
#86582=CARTESIAN_POINT ( 'NONE',  ( 19.02544592524334988, 5.153800228976608722, 31.45942372801900433 ) ) ;
#86583=CARTESIAN_POINT ( 'NONE',  ( 19.02544592524343514, -5.153800228976328945, 93.54057627198102409 ) ) ;
#86584=CARTESIAN_POINT ( 'NONE',  ( 0.05219959533909260263, 19.03943276465977164, 79.99890960531436690 ) ) ;
#86585=CARTESIAN_POINT ( 'NONE',  ( -4.483927247898782831, 16.52544592524335698, 82.70942372801900433 ) ) ;
#86586=CARTESIAN_POINT ( 'NONE',  ( 9.474510206698971260, -16.51473224551069308, 32.91557627198102409 ) ) ;
#86588=CARTESIAN_POINT ( 'NONE',  ( -0.05219959533910754901, -16.53943276465976808, 42.49890960531435979 ) ) ;
#86590=CARTESIAN_POINT ( 'NONE',  ( -16.46253265017160317, 9.564922557960807481, 105.8322429386476955 ) ) ;
#86591=CARTESIAN_POINT ( 'NONE',  ( -21.52544592524343514, 5.823673210054127303, 36.04057627198102409 ) ) ;
#86592=CARTESIAN_POINT ( 'NONE',  ( -16.55341960407611168, -4.379528057220339221, 66.45724293864768129 ) ) ;
#86593=CARTESIAN_POINT ( 'NONE',  ( 0.05219959533934541429, -16.53943276465976808, 20.00109039468568639 ) ) ;
#86594=CARTESIAN_POINT ( 'NONE',  ( -4.483927247898539470, -16.52544592524342804, 62.29057627198102409 ) ) ;
#86596=CARTESIAN_POINT ( 'NONE',  ( -9.474510206698720793, -16.51473224551083518, 59.58442372801900433 ) ) ;
#86597=CARTESIAN_POINT ( 'NONE',  ( 13.97604488694527802, 13.89961937509977652, 99.37390960531436690 ) ) ;
#86598=CARTESIAN_POINT ( 'NONE',  ( 9.564922557961047289, -16.46253265017146816, 75.41775706135234714 ) ) ;
#86600=CARTESIAN_POINT ( 'NONE',  ( -19.05341960407617563, 5.049401038297882671, 108.5427570613523187 ) ) ;
#86601=CARTESIAN_POINT ( 'NONE',  ( 16.53943276465976808, 0.05219959533934440121, 91.25109039468568994 ) ) ;
#86602=CARTESIAN_POINT ( 'NONE',  ( -19.05341960407611168, -5.049401038298163336, 36.45724293864766707 ) ) ;
#86603=CARTESIAN_POINT ( 'NONE',  ( -18.67979575497178146, -10.72451020669898902, 36.66557627198103120 ) ) ;
#86604=CARTESIAN_POINT ( 'NONE',  ( -21.52544592524334988, -5.823673210054445271, 48.95942372801902565 ) ) ;
#86605=CARTESIAN_POINT ( 'NONE',  ( -12.06949235617739369, -12.14591786802326823, 19.37609039468568639 ) ) ;
#86606=CARTESIAN_POINT ( 'NONE',  ( 17.50000000000001421, 3.235083232844117251, 22.78281610344516039 ) ) ;
#86607=CARTESIAN_POINT ( 'NONE',  ( 16.46253265017160672, -9.564922557960803928, 68.33224293864770971 ) ) ;
#86609=CARTESIAN_POINT ( 'NONE',  ( 12.14591786802309770, 12.06949235617756955, 94.37390960531436690 ) ) ;
#86610=CARTESIAN_POINT ( 'NONE',  ( -19.03943276465977164, 0.05219959533909376836, 81.24890960531436690 ) ) ;
#86611=CARTESIAN_POINT ( 'NONE',  ( -16.46253265017160317, 9.564922557960807481, 85.83224293864769550 ) ) ;
#86613=CARTESIAN_POINT ( 'NONE',  ( -19.03943276465977164, -0.05219959533935918106, 88.75109039468567573 ) ) ;
#86614=CARTESIAN_POINT ( 'NONE',  ( 10.72451020669898902, -18.67979575497178502, 67.91557627198102409 ) ) ;
#86615=CARTESIAN_POINT ( 'NONE',  ( 16.46253265017160672, -9.564922557960803928, 23.33224293864769194 ) ) ;
#86616=CARTESIAN_POINT ( 'NONE',  ( 9.564922557961047289, -16.46253265017146816, 50.41775706135233293 ) ) ;
#86617=CARTESIAN_POINT ( 'NONE',  ( 13.97604488694527802, 13.89961937509977652, 54.37390960531435979 ) ) ;
#86618=CARTESIAN_POINT ( 'NONE',  ( 5.049401038298161559, -19.05341960407611168, 87.70724293864769550 ) ) ;
#86620=CARTESIAN_POINT ( 'NONE',  ( 18.62759615963271287, -10.81492255796078972, 88.33224293864769550 ) ) ;
#86621=CARTESIAN_POINT ( 'NONE',  ( -4.379528057220328563, 16.55341960407611168, 90.20724293864770971 ) ) ;
#86622=CARTESIAN_POINT ( 'NONE',  ( -5.153800228976607833, 19.02544592524334988, 67.70942372801900433 ) ) ;
#86623=CARTESIAN_POINT ( 'NONE',  ( 18.67979575497178502, 10.72451020669898547, 89.16557627198102409 ) ) ;
#86624=CARTESIAN_POINT ( 'NONE',  ( 15.72974639402199770, -15.80617190586745480, 78.12390960531436690 ) ) ;
#86625=CARTESIAN_POINT ( 'NONE',  ( -12.14591786802309592, -12.06949235617757132, 26.87390960531435979 ) ) ;
#86626=CARTESIAN_POINT ( 'NONE',  ( 15.80617190586769283, -15.72974639402175789, 105.6260903946856899 ) ) ;
#86627=CARTESIAN_POINT ( 'NONE',  ( 4.379528057220092307, 16.55341960407617563, 52.29275706135236135 ) ) ;
#86628=CARTESIAN_POINT ( 'NONE',  ( 19.02544592524343514, -5.153800228976328945, 83.54057627198100988 ) ) ;
#86629=CARTESIAN_POINT ( 'NONE',  ( -19.05341960407611168, -5.049401038298163336, 36.45724293864766707 ) ) ;
#86630=CARTESIAN_POINT ( 'NONE',  ( 18.62759615963255655, 10.81492255796105972, 41.66775706135235424 ) ) ;
#86631=CARTESIAN_POINT ( 'NONE',  ( -15.72974639402176322, -15.80617190586768395, 59.37609039468568284 ) ) ;
#86632=CARTESIAN_POINT ( 'NONE',  ( -13.97604488694527625, -13.89961937509977652, 46.87390960531435979 ) ) ;
#86633=CARTESIAN_POINT ( 'NONE',  ( 0.05219959533937995610, -21.53943276465977519, 25.00109039468567218 ) ) ;
#86634=CARTESIAN_POINT ( 'NONE',  ( 13.89961937509957401, 13.97604488694547697, 56.87609039468564731 ) ) ;
#86635=CARTESIAN_POINT ( 'NONE',  ( 19.02544592524334988, 5.153800228976608722, 76.45942372801897591 ) ) ;
#86636=CARTESIAN_POINT ( 'NONE',  ( 0.05219959533934541429, -16.53943276465976808, 30.00109039468568284 ) ) ;
#86637=CARTESIAN_POINT ( 'NONE',  ( 13.97604488694527802, 13.89961937509977652, 29.37390960531435979 ) ) ;
#86638=CARTESIAN_POINT ( 'NONE',  ( -12.06949235617739369, -12.14591786802326823, 69.37609039468567573 ) ) ;
#86639=CARTESIAN_POINT ( 'NONE',  ( -16.46253265017160317, 9.564922557960807481, 40.83224293864769550 ) ) ;
#86641=CARTESIAN_POINT ( 'NONE',  ( 19.02544592524343514, -5.153800228976328945, 93.54057627198102409 ) ) ;
#86642=CARTESIAN_POINT ( 'NONE',  ( 16.51473224551069308, 9.474510206698969483, 24.16557627198102765 ) ) ;
#86643=CARTESIAN_POINT ( 'NONE',  ( 15.80617190586746368, 15.72974639402197994, 79.37390960531436690 ) ) ;
#86644=CARTESIAN_POINT ( 'NONE',  ( -8.224510206698735004, -14.34966873604973081, 54.58442372801901143 ) ) ;
#86645=CARTESIAN_POINT ( 'NONE',  ( 16.51473224551083163, -9.474510206698727899, 20.83442372801899722 ) ) ;
#86646=CARTESIAN_POINT ( 'NONE',  ( -19.03943276465977164, 0.05219959533909376836, 46.24890960531435979 ) ) ;
#86647=CARTESIAN_POINT ( 'NONE',  ( -4.379528057220328563, 16.55341960407611168, 30.20724293864769550 ) ) ;
#86648=CARTESIAN_POINT ( 'NONE',  ( -12.14591786802309592, -12.06949235617757132, 66.87390960531436690 ) ) ;
#86649=CARTESIAN_POINT ( 'NONE',  ( -16.51473224551069308, -9.474510206698971260, 71.66557627198102409 ) ) ;
#86650=CARTESIAN_POINT ( 'NONE',  ( -18.67979575497193778, 10.72451020669871902, 38.33442372801900433 ) ) ;
#86651=CARTESIAN_POINT ( 'NONE',  ( 19.03943276465977164, -0.05219959533909143690, 78.74890960531436690 ) ) ;
#86652=CARTESIAN_POINT ( 'NONE',  ( 15.80617190586769283, -15.72974639402175789, 90.62609039468567573 ) ) ;
#86653=CARTESIAN_POINT ( 'NONE',  ( 12.06949235617739724, 12.14591786802326823, 71.87609039468568994 ) ) ;
#86654=CARTESIAN_POINT ( 'NONE',  ( -9.474510206698964154, 16.51473224551069663, 105.4155762719810383 ) ) ;
#86655=CARTESIAN_POINT ( 'NONE',  ( -14.29746914071049879, 8.314922557960819915, 50.83224293864770971 ) ) ;
#86656=CARTESIAN_POINT ( 'NONE',  ( 19.02544592524343514, -5.153800228976328945, 28.54057627198102409 ) ) ;
#86657=CARTESIAN_POINT ( 'NONE',  ( -0.05219959533934338120, 16.53943276465976808, 52.50109039468567573 ) ) ;
#86658=CARTESIAN_POINT ( 'NONE',  ( -14.29746914071049879, 8.314922557960819915, 50.83224293864770971 ) ) ;
#86659=CARTESIAN_POINT ( 'NONE',  ( -9.564922557960796823, -16.46253265017161027, 107.0822429386476955 ) ) ;
#86660=CARTESIAN_POINT ( 'NONE',  ( -21.55341960407610458, -5.719274019375992779, 36.45724293864768839 ) ) ;
#86661=CARTESIAN_POINT ( 'NONE',  ( 19.02544592524334988, 5.153800228976608722, 21.45942372801899012 ) ) ;
#86662=CARTESIAN_POINT ( 'NONE',  ( -12.14591786802309592, -12.06949235617757132, 96.87390960531436690 ) ) ;
#86663=CARTESIAN_POINT ( 'NONE',  ( -16.51473224551069308, -9.474510206698971260, 91.66557627198103830 ) ) ;
#86666=CARTESIAN_POINT ( 'NONE',  ( -16.55341960407617563, 4.379528057220093196, 53.54275706135234714 ) ) ;
#86667=CARTESIAN_POINT ( 'NONE',  ( -0.05219959533909027116, -19.03943276465977164, 52.49890960531436690 ) ) ;
#86668=CARTESIAN_POINT ( 'NONE',  ( 17.72566875460849189, 5.499999999999970690, 101.5781329180409642 ) ) ;
#86669=CARTESIAN_POINT ( 'NONE',  ( -13.97604488694547697, 13.89961937509957934, 43.12609039468566152 ) ) ;
#86670=CARTESIAN_POINT ( 'NONE',  ( -12.06949235617739369, -12.14591786802326823, 79.37609039468567573 ) ) ;
#86671=CARTESIAN_POINT ( 'NONE',  ( 19.02544592524334988, 5.153800228976608722, 91.45942372801900433 ) ) ;
#86672=CARTESIAN_POINT ( 'NONE',  ( -15.80617190586768217, 15.72974639402176855, 73.12609039468567573 ) ) ;
#86673=CARTESIAN_POINT ( 'NONE',  ( 9.474510206698971260, -16.51473224551069308, 77.91557627198103830 ) ) ;
#86674=CARTESIAN_POINT ( 'NONE',  ( -15.80617190586745835, -15.72974639402198527, 91.87390960531436690 ) ) ;
#86675=CARTESIAN_POINT ( 'NONE',  ( 4.483927247898545687, 16.52544592524342804, 94.79057627198105251 ) ) ;
#86676=CARTESIAN_POINT ( 'NONE',  ( 19.02544592524334988, 5.153800228976608722, 76.45942372801897591 ) ) ;
#86677=CARTESIAN_POINT ( 'NONE',  ( -5.719274019375978568, 21.55341960407610458, 75.20724293864769550 ) ) ;
#86678=CARTESIAN_POINT ( 'NONE',  ( -16.46253265017146816, -9.564922557961047289, 44.16775706135232582 ) ) ;
#86679=FACE_BOUND ( 'NONE', #119871, .T. ) ;
#86680=CARTESIAN_POINT ( 'NONE',  ( 5.823673210054125526, 21.52544592524343514, 89.79057627198103830 ) ) ;
#86681=CARTESIAN_POINT ( 'NONE',  ( -17.13100169013299379, 6.664070546373142889, 85.76789835699847231 ) ) ;
#86682=CARTESIAN_POINT ( 'NONE',  ( -9.474510206698964154, 16.51473224551069663, 70.41557627198102409 ) ) ;
#86684=CARTESIAN_POINT ( 'NONE',  ( -4.379528057220086978, -16.55341960407618274, 19.79275706135235069 ) ) ;
#86686=CARTESIAN_POINT ( 'NONE',  ( -13.89961937509977652, 13.97604488694528158, 40.62390960531435979 ) ) ;
#86687=CARTESIAN_POINT ( 'NONE',  ( 19.02544592524343514, -5.153800228976328945, 108.5405762719810383 ) ) ;
#86688=CARTESIAN_POINT ( 'NONE',  ( 0.05219959533907565091, 21.53943276465977519, 89.99890960531438111 ) ) ;
#86689=CARTESIAN_POINT ( 'NONE',  ( -8.314922557960811034, -14.29746914071050412, 52.08224293864768839 ) ) ;
#86690=CARTESIAN_POINT ( 'NONE',  ( 21.53943276465977519, 0.05219959533937863772, 71.25109039468568994 ) ) ;
#86691=CARTESIAN_POINT ( 'NONE',  ( -12.06949235617739369, -12.14591786802326823, 24.37609039468567573 ) ) ;
#86692=CARTESIAN_POINT ( 'NONE',  ( 5.049401038297881783, 19.05341960407617563, 32.29275706135233293 ) ) ;
#86693=CARTESIAN_POINT ( 'NONE',  ( -16.55341960407611168, -4.379528057220339221, 31.45724293864769550 ) ) ;
#86694=CARTESIAN_POINT ( 'NONE',  ( -10.72451020669898014, 18.67979575497178502, 110.4155762719810383 ) ) ;
#86695=CARTESIAN_POINT ( 'NONE',  ( -12.06949235617756955, 12.14591786802309770, 55.62390960531436690 ) ) ;
#86696=CARTESIAN_POINT ( 'NONE',  ( 19.05341960407617918, -5.049401038297876454, 91.04275706135234714 ) ) ;
#86697=CARTESIAN_POINT ( 'NONE',  ( 19.05341960407617918, -5.049401038297876454, 71.04275706135234714 ) ) ;
#86698=CARTESIAN_POINT ( 'NONE',  ( -5.719274019375665041, -21.55341960407619695, 69.79275706135234714 ) ) ;
#86699=CARTESIAN_POINT ( 'NONE',  ( -9.564922557961040184, 16.46253265017147172, 57.91775706135233293 ) ) ;
#86700=CARTESIAN_POINT ( 'NONE',  ( 12.06949235617757843, -12.14591786802309237, 113.1239096053143953 ) ) ;
#86701=CARTESIAN_POINT ( 'NONE',  ( 0.05219959533907565091, 21.53943276465977519, 44.99890960531435979 ) ) ;
#86702=CARTESIAN_POINT ( 'NONE',  ( 8.314922557960818139, 14.29746914071049879, 44.58224293864769550 ) ) ;
#86703=CARTESIAN_POINT ( 'NONE',  ( -18.87075004821569024, 5.499999999999995559, 93.67408112101048800 ) ) ;
#86704=CARTESIAN_POINT ( 'NONE',  ( 9.564922557961047289, -16.46253265017146816, 20.41775706135233293 ) ) ;
#86705=CARTESIAN_POINT ( 'NONE',  ( -16.53943276465976808, -0.05219959533934237506, 78.75109039468568994 ) ) ;
#86706=CARTESIAN_POINT ( 'NONE',  ( 16.53943276465976808, -0.05219959533910856209, 38.74890960531435979 ) ) ;
#86707=CARTESIAN_POINT ( 'NONE',  ( -21.55341960407619339, 5.719274019375674811, 78.54275706135236135 ) ) ;
#86708=CARTESIAN_POINT ( 'NONE',  ( 5.823673210054444382, -21.52544592524334988, 65.20942372801901854 ) ) ;
#86709=CARTESIAN_POINT ( 'NONE',  ( 21.55341960407610458, 5.719274019375980345, 78.95724293864769550 ) ) ;
#86710=CARTESIAN_POINT ( 'NONE',  ( 19.02544592524343514, -5.153800228976328945, 38.54057627198103120 ) ) ;
#86711=CARTESIAN_POINT ( 'NONE',  ( -21.52544592524334988, -5.823673210054445271, 53.95942372801900433 ) ) ;
#86712=CARTESIAN_POINT ( 'NONE',  ( -5.049401038298153566, 19.05341960407611168, 40.20724293864768839 ) ) ;
#86713=CARTESIAN_POINT ( 'NONE',  ( -9.564922557960796823, -16.46253265017161027, 52.08224293864768839 ) ) ;
#86714=CARTESIAN_POINT ( 'NONE',  ( 12.06949235617757843, -12.14591786802309237, 98.12390960531436690 ) ) ;
#86715=CARTESIAN_POINT ( 'NONE',  ( 9.564922557960805705, 16.46253265017160317, 79.58224293864769550 ) ) ;
#86716=CARTESIAN_POINT ( 'NONE',  ( -12.06949235617756955, 12.14591786802309770, 45.62390960531436690 ) ) ;
#86717=CARTESIAN_POINT ( 'NONE',  ( -14.29746914071049879, 8.314922557960819915, 95.83224293864770971 ) ) ;
#86718=CARTESIAN_POINT ( 'NONE',  ( 5.719274019375991003, -21.55341960407610458, 67.70724293864769550 ) ) ;
#86719=CARTESIAN_POINT ( 'NONE',  ( -15.80617190586768217, 15.72974639402176855, 23.12609039468567573 ) ) ;
#86721=CARTESIAN_POINT ( 'NONE',  ( 19.05341960407611168, 5.049401038298154454, 78.95724293864769550 ) ) ;
#86722=CARTESIAN_POINT ( 'NONE',  ( -9.564922557961040184, 16.46253265017147172, 112.9177570613523329 ) ) ;
#86723=CARTESIAN_POINT ( 'NONE',  ( -5.719274019375978568, 21.55341960407610458, 65.20724293864768129 ) ) ;
#86724=CARTESIAN_POINT ( 'NONE',  ( -0.05219959533937732626, 21.53943276465977519, 92.50109039468567573 ) ) ;
#86725=CARTESIAN_POINT ( 'NONE',  ( 9.474510206698971260, -16.51473224551069308, 77.91557627198103830 ) ) ;
#86726=CARTESIAN_POINT ( 'NONE',  ( -10.81492255796105439, 18.62759615963255655, 27.91775706135234358 ) ) ;
#86727=CARTESIAN_POINT ( 'NONE',  ( 19.05341960407611168, 5.049401038298154454, 108.9572429386477097 ) ) ;
#86728=CARTESIAN_POINT ( 'NONE',  ( -14.29746914071037622, -8.314922557961029526, 84.16775706135234714 ) ) ;
#86729=CARTESIAN_POINT ( 'NONE',  ( -18.67979575497193778, 10.72451020669871902, 73.33442372801901854 ) ) ;
#86730=CARTESIAN_POINT ( 'NONE',  ( -15.72974639402176322, -15.80617190586768395, 94.37609039468568994 ) ) ;
#86731=CARTESIAN_POINT ( 'NONE',  ( 8.224510206698742110, 14.34966873604972548, 57.08442372801901854 ) ) ;
#86732=CARTESIAN_POINT ( 'NONE',  ( 5.719274019375673035, 21.55341960407619339, 22.29275706135235069 ) ) ;
#86733=CARTESIAN_POINT ( 'NONE',  ( -13.89961937509977652, 13.97604488694528158, 115.6239096053143669 ) ) ;
#86734=CARTESIAN_POINT ( 'NONE',  ( -21.52544592524334988, -5.823673210054445271, 93.95942372801903275 ) ) ;
#86735=CARTESIAN_POINT ( 'NONE',  ( 19.05341960407611168, 5.049401038298154454, 98.95724293864766707 ) ) ;
#86736=CARTESIAN_POINT ( 'NONE',  ( 21.52544592524344225, -5.823673210054117533, 93.54057627198103830 ) ) ;
#86737=CARTESIAN_POINT ( 'NONE',  ( 16.51473224551083163, -9.474510206698727899, 55.83442372801899722 ) ) ;
#86739=CARTESIAN_POINT ( 'NONE',  ( 5.823673210054125526, 21.52544592524343514, 59.79057627198103120 ) ) ;
#86740=CARTESIAN_POINT ( 'NONE',  ( -16.46253265017160317, 9.564922557960807481, 100.8322429386477097 ) ) ;
#86741=CARTESIAN_POINT ( 'NONE',  ( 16.55341960407611168, 4.379528057220329451, 38.95724293864768839 ) ) ;
#86743=CARTESIAN_POINT ( 'NONE',  ( -0.05219959533936034679, 19.03943276465977164, 72.50109039468566152 ) ) ;
#86747=CARTESIAN_POINT ( 'NONE',  ( -16.51473224551082808, 9.474510206698731452, 113.3344237280190043 ) ) ;
#86748=CARTESIAN_POINT ( 'NONE',  ( 21.52544592524344225, -5.823673210054117533, 83.54057627198102409 ) ) ;
#86749=CARTESIAN_POINT ( 'NONE',  ( 4.483927247898545687, 16.52544592524342804, 59.79057627198103120 ) ) ;
#86750=CARTESIAN_POINT ( 'NONE',  ( -13.97604488694527625, -13.89961937509977652, 101.8739096053143811 ) ) ;
#86751=CARTESIAN_POINT ( 'NONE',  ( -0.05219959533934338120, 16.53943276465976808, 32.50109039468568284 ) ) ;
#86752=CARTESIAN_POINT ( 'NONE',  ( -9.564922557960796823, -16.46253265017161027, 62.08224293864769550 ) ) ;
#86753=CARTESIAN_POINT ( 'NONE',  ( -5.823673210054116645, -21.52544592524344225, 112.2905762719810241 ) ) ;
#86754=CARTESIAN_POINT ( 'NONE',  ( -9.474510206698720793, -16.51473224551083518, 84.58442372801900433 ) ) ;
#86755=CARTESIAN_POINT ( 'NONE',  ( 5.153800228976335163, 19.02544592524342804, 99.79057627198102409 ) ) ;
#86756=CARTESIAN_POINT ( 'NONE',  ( -0.05219959533909027116, -19.03943276465977164, 72.49890960531435269 ) ) ;
#86757=CARTESIAN_POINT ( 'NONE',  ( 10.81492255796078972, 18.62759615963270932, 79.58224293864769550 ) ) ;
#86758=CARTESIAN_POINT ( 'NONE',  ( -9.474510206698964154, 16.51473224551069663, 50.41557627198102409 ) ) ;
#86760=CARTESIAN_POINT ( 'NONE',  ( 16.52544592524342804, -4.483927247898539470, 58.54057627198103120 ) ) ;
#86761=CARTESIAN_POINT ( 'NONE',  ( 16.46253265017160672, -9.564922557960803928, 103.3322429386476955 ) ) ;
#86763=CARTESIAN_POINT ( 'NONE',  ( -5.049401038297874678, -19.05341960407617918, 69.79275706135233293 ) ) ;
#86764=CARTESIAN_POINT ( 'NONE',  ( 10.72451020669898902, -18.67979575497178502, 82.91557627198103830 ) ) ;
#86765=CARTESIAN_POINT ( 'NONE',  ( 9.564922557961047289, -16.46253265017146816, 50.41775706135233293 ) ) ;
#86766=CARTESIAN_POINT ( 'NONE',  ( 0.05219959533909260263, 19.03943276465977164, 104.9989096053143669 ) ) ;
#86768=CARTESIAN_POINT ( 'NONE',  ( -15.80617190586745835, -15.72974639402198527, 46.87390960531435979 ) ) ;
#86769=CARTESIAN_POINT ( 'NONE',  ( 13.89961937509977652, -13.97604488694527269, 68.12390960531436690 ) ) ;
#86770=CARTESIAN_POINT ( 'NONE',  ( 21.53943276465977519, 0.05219959533937863772, 66.25109039468567573 ) ) ;
#86771=CARTESIAN_POINT ( 'NONE',  ( 13.89961937509977652, -13.97604488694527269, 33.12390960531434558 ) ) ;
#86772=CARTESIAN_POINT ( 'NONE',  ( -10.72451020669870658, -18.67979575497194134, 19.58442372801901143 ) ) ;
#86773=VERTEX_POINT ( 'NONE', #21696 ) ;
#86774=CARTESIAN_POINT ( 'NONE',  ( -5.719274019375665041, -21.55341960407619695, 54.79275706135235424 ) ) ;
#86776=CARTESIAN_POINT ( 'NONE',  ( 17.50000000000000355, 5.499999999999998224, 20.00000000000000000 ) ) ;
#86777=CARTESIAN_POINT ( 'NONE',  ( 0.05219959533936267826, -19.03943276465977164, 70.00109039468566152 ) ) ;
#86779=CARTESIAN_POINT ( 'NONE',  ( 21.55341960407619695, -5.719274019375665929, 26.04275706135235779 ) ) ;
#86780=CARTESIAN_POINT ( 'NONE',  ( 19.03943276465977164, -0.05219959533909143690, 53.74890960531436690 ) ) ;
#86781=CARTESIAN_POINT ( 'NONE',  ( -12.14591786802326823, 12.06949235617739902, 38.12609039468567573 ) ) ;
#86783=CARTESIAN_POINT ( 'NONE',  ( 21.52544592524334988, 5.823673210054432836, 111.4594237280190328 ) ) ;
#86784=CARTESIAN_POINT ( 'NONE',  ( 9.474510206698971260, -16.51473224551069308, 37.91557627198102409 ) ) ;
#86785=CARTESIAN_POINT ( 'NONE',  ( 21.53943276465977519, 0.05219959533937863772, 111.2510903946856899 ) ) ;
#86786=CARTESIAN_POINT ( 'NONE',  ( 12.06949235617739724, 12.14591786802326823, 91.87609039468568994 ) ) ;
#86787=CARTESIAN_POINT ( 'NONE',  ( 13.97604488694527802, 13.89961937509977652, 84.37390960531433848 ) ) ;
#86788=CARTESIAN_POINT ( 'NONE',  ( -5.823673210054431948, 21.52544592524334988, 57.70942372801901143 ) ) ;
#86789=CARTESIAN_POINT ( 'NONE',  ( 30.00000000000000000, -5.510910596163089556E-15, 42.49999999999999289 ) ) ;
#86792=CARTESIAN_POINT ( 'NONE',  ( -12.06949235617739369, -12.14591786802326823, 54.37609039468568994 ) ) ;
#86793=CARTESIAN_POINT ( 'NONE',  ( -15.80617190586768217, 15.72974639402176855, 73.12609039468567573 ) ) ;
#86794=CARTESIAN_POINT ( 'NONE',  ( 10.81492255796106328, -18.62759615963255655, 105.4177570613523613 ) ) ;
#86796=CARTESIAN_POINT ( 'NONE',  ( -8.314922557961024197, 14.29746914071037800, 32.91775706135234714 ) ) ;
#86797=CARTESIAN_POINT ( 'NONE',  ( 13.97604488694527802, 13.89961937509977652, 84.37390960531433848 ) ) ;
#86798=CARTESIAN_POINT ( 'NONE',  ( -16.51473224551069308, -9.474510206698971260, 111.6655762719810383 ) ) ;
#86801=B_SPLINE_CURVE_WITH_KNOTS ( 'NONE', 3,
 ( #100441, #191453, #162121, #99438, #37774, #173312, #5427, #97423, #159109, #35776, #23618, #20603, #66113, #36761, #98424, #161118, #84260, #85265, #142944, #144941, #6423, #146956, #38784, #82255, #143947, #68104, #52930, #19621, #145942, #51941, #53948, #112615 ),
 .UNSPECIFIED., .F., .F.,
 ( 4, 2, 2, 2, 2, 2, 2, 2, 2, 2, 2, 2, 2, 2, 2, 4 ),
 ( 4.336808689942017736E-18, 0.0003712461730036848806, 0.0007424923460073654244, 0.001113738519011045914, 0.001484984692014726512, 0.002227477038022087491, 0.002598723211025768306, 0.002969969384029448687, 0.003341215557033129068, 0.003712461730036809883, 0.004083707903040490264, 0.004454954076044170645, 0.004826200249047851026, 0.005197446422051532275, 0.005568692595055212656, 0.005939938768058893037 ),
 .UNSPECIFIED. ) ;
#86802=CARTESIAN_POINT ( 'NONE',  ( -5.153800228976328057, -19.02544592524343514, 27.29057627198103120 ) ) ;
#86803=CARTESIAN_POINT ( 'NONE',  ( 10.81492255796078972, 18.62759615963270932, 44.58224293864769550 ) ) ;
#86804=CARTESIAN_POINT ( 'NONE',  ( -4.379528057220086978, -16.55341960407618274, 104.7927570613523898 ) ) ;
#86805=CARTESIAN_POINT ( 'NONE',  ( 14.34966873604960469, 8.224510206698951720, 84.16557627198103830 ) ) ;
#86806=CARTESIAN_POINT ( 'NONE',  ( 9.474510206698971260, -16.51473224551069308, 67.91557627198102409 ) ) ;
#86807=CARTESIAN_POINT ( 'NONE',  ( 10.72451020669871369, 18.67979575497193778, 92.08442372801901854 ) ) ;
#86808=CARTESIAN_POINT ( 'NONE',  ( -14.34966873604972548, 8.224510206698743886, 28.33442372801902209 ) ) ;
#86809=CARTESIAN_POINT ( 'NONE',  ( -12.14591786802309592, -12.06949235617757132, 91.87390960531436690 ) ) ;
#86810=CARTESIAN_POINT ( 'NONE',  ( 10.72451020669871369, 18.67979575497193778, 42.08442372801901854 ) ) ;
#86811=CARTESIAN_POINT ( 'NONE',  ( 18.67979575497178502, 10.72451020669898547, 79.16557627198103830 ) ) ;
#86812=CARTESIAN_POINT ( 'NONE',  ( 16.46253265017146816, 9.564922557961045513, 56.66775706135233293 ) ) ;
#86814=CARTESIAN_POINT ( 'NONE',  ( 13.97604488694527802, 13.89961937509977652, 99.37390960531436690 ) ) ;
#86815=CARTESIAN_POINT ( 'NONE',  ( -0.05219959533910754901, -16.53943276465976808, 67.49890960531436690 ) ) ;
#86816=CARTESIAN_POINT ( 'NONE',  ( 16.52544592524342804, -4.483927247898539470, 53.54057627198103120 ) ) ;
#86817=CARTESIAN_POINT ( 'NONE',  ( -8.314922557960811034, -14.29746914071050412, 22.08224293864769194 ) ) ;
#86818=CARTESIAN_POINT ( 'NONE',  ( -19.03943276465977164, -0.05219959533935918106, 63.75109039468566863 ) ) ;
#86819=CARTESIAN_POINT ( 'NONE',  ( 9.564922557961047289, -16.46253265017146816, 90.41775706135234714 ) ) ;
#86820=CARTESIAN_POINT ( 'NONE',  ( 19.02544592524343514, -5.153800228976328945, 113.5405762719810241 ) ) ;
#86822=CARTESIAN_POINT ( 'NONE',  ( 8.224510206698953496, -14.34966873604960469, 82.91557627198103830 ) ) ;
#86824=CARTESIAN_POINT ( 'NONE',  ( -5.049401038298153566, 19.05341960407611168, 50.20724293864770260 ) ) ;
#86825=CARTESIAN_POINT ( 'NONE',  ( -0.05219959533907301413, -21.53943276465977519, 52.49890960531435979 ) ) ;
#86826=CARTESIAN_POINT ( 'NONE',  ( 18.67979575497178502, 10.72451020669898547, 74.16557627198102409 ) ) ;
#86827=CARTESIAN_POINT ( 'NONE',  ( 8.224510206698953496, -14.34966873604960469, 112.9155762719810383 ) ) ;
#86828=CARTESIAN_POINT ( 'NONE',  ( 4.379528057220092307, 16.55341960407617563, 67.29275706135234714 ) ) ;
#86829=CARTESIAN_POINT ( 'NONE',  ( 13.89961937509977652, -13.97604488694527269, 43.12390960531434558 ) ) ;
#86830=CARTESIAN_POINT ( 'NONE',  ( -9.474510206698720793, -16.51473224551083518, 34.58442372801899722 ) ) ;
#86831=CARTESIAN_POINT ( 'NONE',  ( -0.05219959533937732626, 21.53943276465977519, 57.50109039468568994 ) ) ;
#86832=CARTESIAN_POINT ( 'NONE',  ( 12.06949235617757843, -12.14591786802309237, 103.1239096053143811 ) ) ;
#86833=CARTESIAN_POINT ( 'NONE',  ( 16.51473224551083163, -9.474510206698727899, 85.83442372801900433 ) ) ;
#86835=CARTESIAN_POINT ( 'NONE',  ( 17.50000000000004263, 3.647616755428117585, 37.20330205721256078 ) ) ;
#86836=CARTESIAN_POINT ( 'NONE',  ( -10.72451020669898014, 18.67979575497178502, 50.41557627198103120 ) ) ;
#86837=CARTESIAN_POINT ( 'NONE',  ( -9.564922557960796823, -16.46253265017161027, 27.08224293864769550 ) ) ;
#86838=CARTESIAN_POINT ( 'NONE',  ( 18.67979575497194134, -10.72451020669871369, 80.83442372801901854 ) ) ;
#86840=CARTESIAN_POINT ( 'NONE',  ( 16.52544592524342804, -4.483927247898539470, 38.54057627198103120 ) ) ;
#86841=CARTESIAN_POINT ( 'NONE',  ( -12.14591786802326823, 12.06949235617739902, 53.12609039468568284 ) ) ;
#86842=CARTESIAN_POINT ( 'NONE',  ( 16.55341960407611168, 4.379528057220329451, 38.95724293864768839 ) ) ;
#86843=CARTESIAN_POINT ( 'NONE',  ( 18.62759615963271287, -10.81492255796078972, 88.33224293864769550 ) ) ;
#86844=CARTESIAN_POINT ( 'NONE',  ( 18.62759615963271287, -10.81492255796078972, 78.33224293864770971 ) ) ;
#86846=CARTESIAN_POINT ( 'NONE',  ( -0.05219959533936034679, 19.03943276465977164, 77.50109039468566152 ) ) ;
#86847=CARTESIAN_POINT ( 'NONE',  ( 16.51473224551069308, 9.474510206698969483, 114.1655762719810241 ) ) ;
#86848=CARTESIAN_POINT ( 'NONE',  ( -0.05219959533909027116, -19.03943276465977164, 52.49890960531436690 ) ) ;
#86849=CARTESIAN_POINT ( 'NONE',  ( 19.03943276465977164, -0.05219959533909143690, 33.74890960531435979 ) ) ;
#86853=CARTESIAN_POINT ( 'NONE',  ( -12.14591786802326823, 12.06949235617739902, 83.12609039468568994 ) ) ;
#86854=CARTESIAN_POINT ( 'NONE',  ( 21.53943276465977519, -0.05219959533907433946, 103.7489096053143669 ) ) ;
#86855=CARTESIAN_POINT ( 'NONE',  ( -19.05341960407611168, -5.049401038298163336, 71.45724293864766707 ) ) ;
#86856=CARTESIAN_POINT ( 'NONE',  ( -15.72974639402176322, -15.80617190586768395, 44.37609039468567573 ) ) ;
#86857=CARTESIAN_POINT ( 'NONE',  ( 13.89961937509977652, -13.97604488694527269, 93.12390960531436690 ) ) ;
#86860=CARTESIAN_POINT ( 'NONE',  ( -21.53943276465977519, -0.05219959533937600094, 38.75109039468567573 ) ) ;
#86861=CARTESIAN_POINT ( 'NONE',  ( 5.049401038298161559, -19.05341960407611168, 27.70724293864769550 ) ) ;
#86862=CARTESIAN_POINT ( 'NONE',  ( 13.97604488694527802, 13.89961937509977652, 109.3739096053143669 ) ) ;
#86863=CARTESIAN_POINT ( 'NONE',  ( -5.153800228976607833, 19.02544592524334988, 42.70942372801901143 ) ) ;
#86864=CARTESIAN_POINT ( 'NONE',  ( -21.53943276465977519, 0.05219959533907696930, 111.2489096053143669 ) ) ;
#86865=CARTESIAN_POINT ( 'NONE',  ( 16.46253265017146816, 9.564922557961045513, 51.66775706135233293 ) ) ;
#86866=CARTESIAN_POINT ( 'NONE',  ( -5.049401038297874678, -19.05341960407617918, 44.79275706135232582 ) ) ;
#86867=CARTESIAN_POINT ( 'NONE',  ( 8.314922557961029526, -14.29746914071037800, 85.41775706135236135 ) ) ;
#86869=CARTESIAN_POINT ( 'NONE',  ( -19.03943276465977164, 0.05219959533909376836, 76.24890960531435269 ) ) ;
#86870=CARTESIAN_POINT ( 'NONE',  ( -10.81492255796105439, 18.62759615963255655, 77.91775706135231871 ) ) ;
#86871=CARTESIAN_POINT ( 'NONE',  ( -21.52544592524334988, -5.823673210054445271, 93.95942372801903275 ) ) ;
#86873=CARTESIAN_POINT ( 'NONE',  ( -13.89961937509977652, 13.97604488694528158, 90.62390960531432427 ) ) ;
#86874=CARTESIAN_POINT ( 'NONE',  ( 21.52544592524334988, 5.823673210054432836, 66.45942372801903275 ) ) ;
#86875=CARTESIAN_POINT ( 'NONE',  ( 13.97604488694548053, -13.89961937509957401, 95.62609039468563310 ) ) ;
#86876=CARTESIAN_POINT ( 'NONE',  ( -5.049401038298153566, 19.05341960407611168, 70.20724293864769550 ) ) ;
#86877=CARTESIAN_POINT ( 'NONE',  ( 19.03943276465977164, -0.05219959533909143690, 108.7489096053143527 ) ) ;
#86878=CARTESIAN_POINT ( 'NONE',  ( -19.03943276465977164, 0.05219959533909376836, 86.24890960531436690 ) ) ;
#86880=CARTESIAN_POINT ( 'NONE',  ( 19.03943276465977164, -0.05219959533909143690, 63.74890960531435979 ) ) ;
#86881=CARTESIAN_POINT ( 'NONE',  ( 13.89961937509977652, -13.97604488694527269, 53.12390960531434558 ) ) ;
#86882=CARTESIAN_POINT ( 'NONE',  ( 21.52544592524344225, -5.823673210054117533, 108.5405762719810241 ) ) ;
#86883=CARTESIAN_POINT ( 'NONE',  ( -8.314922557961024197, 14.29746914071037800, 102.9177570613523756 ) ) ;
#86885=CARTESIAN_POINT ( 'NONE',  ( 5.049401038297881783, 19.05341960407617563, 57.29275706135231871 ) ) ;
#86886=CARTESIAN_POINT ( 'NONE',  ( -13.89961937509977652, 13.97604488694528158, 90.62390960531432427 ) ) ;
#86887=CARTESIAN_POINT ( 'NONE',  ( 4.379528057220339221, -16.55341960407611168, 72.70724293864769550 ) ) ;
#86888=CARTESIAN_POINT ( 'NONE',  ( 14.29746914071049879, -8.314922557960816363, 108.3322429386477097 ) ) ;
#86889=CARTESIAN_POINT ( 'NONE',  ( 18.62759615963271287, -10.81492255796078972, 28.33224293864769550 ) ) ;
#86891=CARTESIAN_POINT ( 'NONE',  ( -18.62759615963270932, 10.81492255796079327, 25.83224293864769194 ) ) ;
#86892=CARTESIAN_POINT ( 'NONE',  ( 4.483927247898545687, 16.52544592524342804, 89.79057627198103830 ) ) ;
#86894=CARTESIAN_POINT ( 'NONE',  ( 16.46253265017146816, 9.564922557961045513, 31.66775706135232937 ) ) ;
#86895=CARTESIAN_POINT ( 'NONE',  ( -16.52544592524335698, -4.483927247898792601, 108.9594237280190185 ) ) ;
#86896=CARTESIAN_POINT ( 'NONE',  ( 19.02544592524343514, -5.153800228976328945, 93.54057627198102409 ) ) ;
#86897=CARTESIAN_POINT ( 'NONE',  ( -21.52544592524334988, -5.823673210054445271, 48.95942372801902565 ) ) ;
#86898=CARTESIAN_POINT ( 'NONE',  ( -5.719274019375978568, 21.55341960407610458, 50.20724293864769550 ) ) ;
#86899=CARTESIAN_POINT ( 'NONE',  ( 10.81492255796106328, -18.62759615963255655, 35.41775706135234003 ) ) ;
#86900=VERTEX_POINT ( 'NONE', #63216 ) ;
#86901=CARTESIAN_POINT ( 'NONE',  ( 10.81492255796078972, 18.62759615963270932, 79.58224293864769550 ) ) ;
#86902=CARTESIAN_POINT ( 'NONE',  ( -8.314922557960811034, -14.29746914071050412, 102.0822429386476955 ) ) ;
#86903=CARTESIAN_POINT ( 'NONE',  ( 5.153800228976615827, -19.02544592524334988, 60.20942372801899012 ) ) ;
#86904=CARTESIAN_POINT ( 'NONE',  ( -0.05219959533909027116, -19.03943276465977164, 42.49890960531435269 ) ) ;
#86905=CARTESIAN_POINT ( 'NONE',  ( -5.049401038298153566, 19.05341960407611168, 100.2072429386476955 ) ) ;
#86906=CARTESIAN_POINT ( 'NONE',  ( -13.97604488694527625, -13.89961937509977652, 96.87390960531433848 ) ) ;
#86907=CARTESIAN_POINT ( 'NONE',  ( 8.314922557960818139, 14.29746914071049879, 114.5822429386477097 ) ) ;
#86908=CARTESIAN_POINT ( 'NONE',  ( 16.55341960407611168, 4.379528057220329451, 38.95724293864768839 ) ) ;
#86909=CARTESIAN_POINT ( 'NONE',  ( 14.29746914071037800, 8.314922557961029526, 36.66775706135234714 ) ) ;
#86910=CARTESIAN_POINT ( 'NONE',  ( -5.823673210054431948, 21.52544592524334988, 112.7094237280190328 ) ) ;
#86912=CARTESIAN_POINT ( 'NONE',  ( 12.14591786802309770, 12.06949235617756955, 24.37390960531435979 ) ) ;
#86913=CARTESIAN_POINT ( 'NONE',  ( 5.719274019375673035, 21.55341960407619339, 27.29275706135234358 ) ) ;
#86914=CARTESIAN_POINT ( 'NONE',  ( -19.05341960407611168, -5.049401038298163336, 111.4572429386476671 ) ) ;
#86915=CARTESIAN_POINT ( 'NONE',  ( -0.05219959533934338120, 16.53943276465976808, 52.50109039468567573 ) ) ;
#86916=CARTESIAN_POINT ( 'NONE',  ( -12.14591786802326823, 12.06949235617739902, 113.1260903946856899 ) ) ;
#86917=CARTESIAN_POINT ( 'NONE',  ( 8.224510206698742110, 14.34966873604972548, 92.08442372801901854 ) ) ;
#86918=CARTESIAN_POINT ( 'NONE',  ( 8.224510206698742110, 14.34966873604972548, 22.08442372801901143 ) ) ;
#86920=CARTESIAN_POINT ( 'NONE',  ( 19.03943276465977164, -0.05219959533909143690, 53.74890960531436690 ) ) ;
#86921=CARTESIAN_POINT ( 'NONE',  ( -14.34966873604960291, -8.224510206698953496, 101.6655762719810383 ) ) ;
#86922=CARTESIAN_POINT ( 'NONE',  ( 21.55341960407610458, 5.719274019375980345, 113.9572429386477239 ) ) ;
#86923=CARTESIAN_POINT ( 'NONE',  ( -16.46253265017160317, 9.564922557960807481, 35.83224293864768839 ) ) ;
#86924=CARTESIAN_POINT ( 'NONE',  ( 13.89961937509977652, -13.97604488694527269, 108.1239096053143669 ) ) ;
#86925=CARTESIAN_POINT ( 'NONE',  ( -18.62759615963255300, -10.81492255796106328, 39.16775706135235424 ) ) ;
#86926=CARTESIAN_POINT ( 'NONE',  ( 5.153800228976335163, 19.02544592524342804, 24.79057627198102765 ) ) ;
#86927=CARTESIAN_POINT ( 'NONE',  ( 0.05219959533909260263, 19.03943276465977164, 109.9989096053143669 ) ) ;
#86928=CARTESIAN_POINT ( 'NONE',  ( -17.49999999999998579, -5.499999999999973355, 101.2823096230356583 ) ) ;
#86929=CARTESIAN_POINT ( 'NONE',  ( -16.51473224551069308, -9.474510206698971260, 96.66557627198102409 ) ) ;
#86930=CARTESIAN_POINT ( 'NONE',  ( 21.52544592524334988, 5.823673210054432836, 46.45942372801901854 ) ) ;
#86931=CARTESIAN_POINT ( 'NONE',  ( 8.224510206698953496, -14.34966873604960469, 87.91557627198103830 ) ) ;
#86932=CARTESIAN_POINT ( 'NONE',  ( 19.02544592524343514, -5.153800228976328945, 98.54057627198100988 ) ) ;
#86934=CARTESIAN_POINT ( 'NONE',  ( -12.14591786802326823, 12.06949235617739902, 63.12609039468568994 ) ) ;
#86935=CARTESIAN_POINT ( 'NONE',  ( -10.72451020669870658, -18.67979575497194134, 74.58442372801901854 ) ) ;
#86936=CARTESIAN_POINT ( 'NONE',  ( -8.224510206698735004, -14.34966873604973081, 34.58442372801900433 ) ) ;
#86937=CARTESIAN_POINT ( 'NONE',  ( 5.049401038298161559, -19.05341960407611168, 87.70724293864769550 ) ) ;
#86938=CARTESIAN_POINT ( 'NONE',  ( -19.02544592524334988, -5.153800228976617603, 103.9594237280190043 ) ) ;
#86939=CARTESIAN_POINT ( 'NONE',  ( 8.314922557961029526, -14.29746914071037800, 70.41775706135236135 ) ) ;
#86940=CARTESIAN_POINT ( 'NONE',  ( 9.474510206698729675, 16.51473224551082808, 22.08442372801899722 ) ) ;
#86941=CARTESIAN_POINT ( 'NONE',  ( 5.049401038297881783, 19.05341960407617563, 92.29275706135234714 ) ) ;
#86942=CARTESIAN_POINT ( 'NONE',  ( 13.97604488694527802, 13.89961937509977652, 59.37390960531434558 ) ) ;
#86943=CARTESIAN_POINT ( 'NONE',  ( 10.72451020669898902, -18.67979575497178502, 87.91557627198103830 ) ) ;
#86944=CARTESIAN_POINT ( 'NONE',  ( 14.34966873604960469, 8.224510206698951720, 89.16557627198102409 ) ) ;
#86945=CARTESIAN_POINT ( 'NONE',  ( 5.049401038297881783, 19.05341960407617563, 87.29275706135234714 ) ) ;
#86946=CARTESIAN_POINT ( 'NONE',  ( -12.06949235617739369, -12.14591786802326823, 59.37609039468568284 ) ) ;
#86948=CARTESIAN_POINT ( 'NONE',  ( 19.02544592524334988, 5.153800228976608722, 56.45942372801898301 ) ) ;
#86949=CARTESIAN_POINT ( 'NONE',  ( -16.52544592524342804, 4.483927247898546575, 31.04057627198102409 ) ) ;
#86950=CARTESIAN_POINT ( 'NONE',  ( 14.34966873604960469, 8.224510206698951720, 84.16557627198103830 ) ) ;
#86951=CARTESIAN_POINT ( 'NONE',  ( 16.46253265017146816, 9.564922557961045513, 26.66775706135234003 ) ) ;
#86952=CARTESIAN_POINT ( 'NONE',  ( -16.19135201231351218, 7.376712067592062994, 39.81319145947881566 ) ) ;
#86953=CARTESIAN_POINT ( 'NONE',  ( 15.72974639402176855, 15.80617190586768217, 21.87609039468567573 ) ) ;
#86954=CARTESIAN_POINT ( 'NONE',  ( -19.02544592524342804, 5.153800228976336051, 106.0405762719810241 ) ) ;
#86955=CARTESIAN_POINT ( 'NONE',  ( -19.03943276465977164, 0.05219959533909376836, 81.24890960531436690 ) ) ;
#86956=CARTESIAN_POINT ( 'NONE',  ( -21.52544592524334988, -5.823673210054445271, 98.95942372801903275 ) ) ;
#86957=CARTESIAN_POINT ( 'NONE',  ( 0.05219959533909260263, 19.03943276465977164, 79.99890960531436690 ) ) ;
#86958=CARTESIAN_POINT ( 'NONE',  ( 21.52544592524344225, -5.823673210054117533, 38.54057627198103120 ) ) ;
#86959=CARTESIAN_POINT ( 'NONE',  ( -8.224510206698948167, 14.34966873604960824, 85.41557627198102409 ) ) ;
#86960=CARTESIAN_POINT ( 'NONE',  ( -13.97604488694527625, -13.89961937509977652, 56.87390960531434558 ) ) ;
#86961=CARTESIAN_POINT ( 'NONE',  ( 14.34966873604960469, 8.224510206698951720, 104.1655762719810241 ) ) ;
#86962=CARTESIAN_POINT ( 'NONE',  ( -18.67979575497193778, 10.72451020669871902, 28.33442372801902209 ) ) ;
#86963=CARTESIAN_POINT ( 'NONE',  ( 15.80617190586769283, -15.72974639402175789, 65.62609039468568994 ) ) ;
#86964=CARTESIAN_POINT ( 'NONE',  ( -9.564922557960796823, -16.46253265017161027, 37.08224293864768839 ) ) ;
#86965=CARTESIAN_POINT ( 'NONE',  ( -0.05219959533934338120, 16.53943276465976808, 57.50109039468568994 ) ) ;
#86966=CARTESIAN_POINT ( 'NONE',  ( 5.719274019375673035, 21.55341960407619339, 22.29275706135235069 ) ) ;
#86967=CARTESIAN_POINT ( 'NONE',  ( 21.53943276465977519, -0.05219959533907433946, 108.7489096053143669 ) ) ;
#86968=CARTESIAN_POINT ( 'NONE',  ( 16.46253265017146816, 9.564922557961045513, 41.66775706135234003 ) ) ;
#86969=CARTESIAN_POINT ( 'NONE',  ( -16.51473224551069308, -9.474510206698971260, 51.66557627198102409 ) ) ;
#86971=CARTESIAN_POINT ( 'NONE',  ( -21.55341960407619339, 5.719274019375674811, 73.54275706135234714 ) ) ;
#86972=CARTESIAN_POINT ( 'NONE',  ( -0.05219959533907301413, -21.53943276465977519, 52.49890960531435979 ) ) ;
#86973=CARTESIAN_POINT ( 'NONE',  ( 12.14591786802309770, 12.06949235617756955, 39.37390960531436690 ) ) ;
#86974=CARTESIAN_POINT ( 'NONE',  ( 10.81492255796106328, -18.62759615963255655, 70.41775706135236135 ) ) ;
#86975=CARTESIAN_POINT ( 'NONE',  ( 5.719274019375673035, 21.55341960407619339, 107.2927570613523471 ) ) ;
#86976=CARTESIAN_POINT ( 'NONE',  ( 4.379528057220339221, -16.55341960407611168, 62.70724293864769550 ) ) ;
#86977=CARTESIAN_POINT ( 'NONE',  ( 14.29746914071049879, -8.314922557960816363, 98.33224293864769550 ) ) ;
#86978=CARTESIAN_POINT ( 'NONE',  ( 13.97604488694548053, -13.89961937509957401, 50.62609039468566152 ) ) ;
#86979=CARTESIAN_POINT ( 'NONE',  ( 12.14591786802327356, -12.06949235617739191, 110.6260903946857042 ) ) ;
#86980=CARTESIAN_POINT ( 'NONE',  ( -10.72451020669870658, -18.67979575497194134, 74.58442372801901854 ) ) ;
#86981=CARTESIAN_POINT ( 'NONE',  ( -13.97604488694527625, -13.89961937509977652, 61.87390960531435979 ) ) ;
#86982=CARTESIAN_POINT ( 'NONE',  ( -19.05341960407617563, 5.049401038297882671, 38.54275706135233293 ) ) ;
#86983=CARTESIAN_POINT ( 'NONE',  ( 10.81492255796078972, 18.62759615963270932, 39.58224293864769550 ) ) ;
#86984=CARTESIAN_POINT ( 'NONE',  ( -10.72451020669870658, -18.67979575497194134, 34.58442372801900433 ) ) ;
#86985=CARTESIAN_POINT ( 'NONE',  ( 21.55341960407610458, 5.719274019375980345, 83.95724293864770971 ) ) ;
#86986=CARTESIAN_POINT ( 'NONE',  ( 19.05341960407617918, -5.049401038297876454, 86.04275706135233293 ) ) ;
#86987=CARTESIAN_POINT ( 'NONE',  ( -14.34966873604972548, 8.224510206698743886, 53.33442372801901854 ) ) ;
#86989=CARTESIAN_POINT ( 'NONE',  ( 21.55341960407610458, 5.719274019375980345, 98.95724293864770971 ) ) ;
#86990=CARTESIAN_POINT ( 'NONE',  ( -0.05219959533910754901, -16.53943276465976808, 92.49890960531436690 ) ) ;
#86991=CARTESIAN_POINT ( 'NONE',  ( 17.72560187377285601, 5.500000000000050626, 41.57814504131319211 ) ) ;
#86992=CARTESIAN_POINT ( 'NONE',  ( 4.379528057220092307, 16.55341960407617563, 22.29275706135235069 ) ) ;
#86993=CARTESIAN_POINT ( 'NONE',  ( -15.80617190586745835, -15.72974639402198527, 46.87390960531435979 ) ) ;
#86994=CARTESIAN_POINT ( 'NONE',  ( 8.224510206698742110, 14.34966873604972548, 77.08442372801901854 ) ) ;
#86995=CARTESIAN_POINT ( 'NONE',  ( -30.00000000000000000, 5.499999999999992895, 37.50000000000000000 ) ) ;
#86996=CARTESIAN_POINT ( 'NONE',  ( -4.379528057220086978, -16.55341960407618274, 54.79275706135235424 ) ) ;
#86997=CARTESIAN_POINT ( 'NONE',  ( -0.05219959533937732626, 21.53943276465977519, 22.50109039468567573 ) ) ;
#86998=CARTESIAN_POINT ( 'NONE',  ( 0.05219959533907565091, 21.53943276465977519, 49.99890960531437401 ) ) ;
#86999=CARTESIAN_POINT ( 'NONE',  ( 14.29746914071037800, 8.314922557961029526, 81.66775706135236135 ) ) ;
#87000=CARTESIAN_POINT ( 'NONE',  ( -16.46253265017160317, 9.564922557960807481, 95.83224293864769550 ) ) ;
#87001=CARTESIAN_POINT ( 'NONE',  ( -21.52544592524334988, -5.823673210054445271, 58.95942372801902565 ) ) ;
#87002=CARTESIAN_POINT ( 'NONE',  ( 5.153800228976335163, 19.02544592524342804, 24.79057627198102765 ) ) ;
#87003=CARTESIAN_POINT ( 'NONE',  ( 0.05219959533907565091, 21.53943276465977519, 39.99890960531436690 ) ) ;
#87004=CARTESIAN_POINT ( 'NONE',  ( -5.719274019375978568, 21.55341960407610458, 25.20724293864769550 ) ) ;
#87006=CARTESIAN_POINT ( 'NONE',  ( 16.46253265017146816, 9.564922557961045513, 41.66775706135234003 ) ) ;
#87007=CARTESIAN_POINT ( 'NONE',  ( -8.314922557961024197, 14.29746914071037800, 62.91775706135236135 ) ) ;
#87008=CARTESIAN_POINT ( 'NONE',  ( -5.823673210054116645, -21.52544592524344225, 22.29057627198102765 ) ) ;
#87010=EDGE_CURVE ( 'NONE', #145773, #188324, #18719, .T. ) ;
#87011=CARTESIAN_POINT ( 'NONE',  ( 5.049401038298161559, -19.05341960407611168, 92.70724293864769550 ) ) ;
#87012=CARTESIAN_POINT ( 'NONE',  ( 8.314922557961029526, -14.29746914071037800, 95.41775706135234714 ) ) ;
#87013=CARTESIAN_POINT ( 'NONE',  ( -18.22780087662124160, -5.499999999999927169, 78.98236817873106475 ) ) ;
#87014=CARTESIAN_POINT ( 'NONE',  ( 16.53943276465976808, -0.05219959533910856209, 93.74890960531436690 ) ) ;
#87015=CARTESIAN_POINT ( 'NONE',  ( 18.67979575497178502, 10.72451020669898547, 44.16557627198103120 ) ) ;
#87016=CARTESIAN_POINT ( 'NONE',  ( -9.474510206698964154, 16.51473224551069663, 30.41557627198102054 ) ) ;
#87017=CARTESIAN_POINT ( 'NONE',  ( 4.379528057220092307, 16.55341960407617563, 77.29275706135234714 ) ) ;
#87018=CARTESIAN_POINT ( 'NONE',  ( 5.719274019375673035, 21.55341960407619339, 32.29275706135235424 ) ) ;
#87019=CARTESIAN_POINT ( 'NONE',  ( -5.153800228976607833, 19.02544592524334988, 92.70942372801901854 ) ) ;
#87020=CARTESIAN_POINT ( 'NONE',  ( -16.51473224551069308, -9.474510206698971260, 41.66557627198103120 ) ) ;
#87021=CARTESIAN_POINT ( 'NONE',  ( 5.049401038298161559, -19.05341960407611168, 107.7072429386476955 ) ) ;
#87022=CARTESIAN_POINT ( 'NONE',  ( 10.81492255796106328, -18.62759615963255655, 110.4177570613523756 ) ) ;
#87023=CARTESIAN_POINT ( 'NONE',  ( 19.02544592524343514, -5.153800228976328945, 83.54057627198100988 ) ) ;
#87025=CARTESIAN_POINT ( 'NONE',  ( 14.34966873604972726, -8.224510206698740333, 65.83442372801900433 ) ) ;
#87026=CARTESIAN_POINT ( 'NONE',  ( -21.52544592524334988, -5.823673210054445271, 98.95942372801903275 ) ) ;
#87027=CARTESIAN_POINT ( 'NONE',  ( 13.97604488694548053, -13.89961937509957401, 50.62609039468566152 ) ) ;
#87028=CARTESIAN_POINT ( 'NONE',  ( -9.474510206698720793, -16.51473224551083518, 64.58442372801900433 ) ) ;
#87030=CARTESIAN_POINT ( 'NONE',  ( -10.81492255796105439, 18.62759615963255655, 67.91775706135234714 ) ) ;
#87031=CARTESIAN_POINT ( 'NONE',  ( 19.05341960407611168, 5.049401038298154454, 63.95724293864769550 ) ) ;
#87032=CARTESIAN_POINT ( 'NONE',  ( 16.46253265017160672, -9.564922557960803928, 58.33224293864769550 ) ) ;
#87033=CARTESIAN_POINT ( 'NONE',  ( -5.049401038297874678, -19.05341960407617918, 59.79275706135231871 ) ) ;
#87034=CARTESIAN_POINT ( 'NONE',  ( 5.049401038298161559, -19.05341960407611168, 112.7072429386476813 ) ) ;
#87035=CARTESIAN_POINT ( 'NONE',  ( 5.153800228976335163, 19.02544592524342804, 79.79057627198102409 ) ) ;
#87036=CARTESIAN_POINT ( 'NONE',  ( 12.14591786802309770, 12.06949235617756955, 44.37390960531435979 ) ) ;
#87037=CARTESIAN_POINT ( 'NONE',  ( -18.62759615963270932, 10.81492255796079327, 35.83224293864768839 ) ) ;
#87038=CARTESIAN_POINT ( 'NONE',  ( -17.97214573761833378, -5.499999999999959144, 96.46970049038655759 ) ) ;
#87039=CARTESIAN_POINT ( 'NONE',  ( -21.55341960407619339, 5.719274019375674811, 113.5427570613523756 ) ) ;
#87041=CARTESIAN_POINT ( 'NONE',  ( -13.97604488694527625, -13.89961937509977652, 36.87390960531436690 ) ) ;
#87042=CARTESIAN_POINT ( 'NONE',  ( -18.22780087662123805, 5.499999999999981348, 86.01763182126894947 ) ) ;
#87044=CARTESIAN_POINT ( 'NONE',  ( -21.52544592524334988, -5.823673210054445271, 68.95942372801901854 ) ) ;
#87046=CARTESIAN_POINT ( 'NONE',  ( -4.379528057220086978, -16.55341960407618274, 64.79275706135234714 ) ) ;
#87047=CARTESIAN_POINT ( 'NONE',  ( 21.55341960407610458, 5.719274019375980345, 83.95724293864770971 ) ) ;
#87048=CARTESIAN_POINT ( 'NONE',  ( -16.52544592524342804, 4.483927247898546575, 51.04057627198103120 ) ) ;
#87049=CARTESIAN_POINT ( 'NONE',  ( 19.03943276465977164, -0.05219959533909143690, 23.74890960531435269 ) ) ;
#87050=CARTESIAN_POINT ( 'NONE',  ( -5.049401038298153566, 19.05341960407611168, 105.2072429386476671 ) ) ;
#87051=CARTESIAN_POINT ( 'NONE',  ( 10.81492255796106328, -18.62759615963255655, 35.41775706135234003 ) ) ;
#87052=CARTESIAN_POINT ( 'NONE',  ( 5.153800228976615827, -19.02544592524334988, 50.20942372801897591 ) ) ;
#87053=CARTESIAN_POINT ( 'NONE',  ( 19.02544592524343514, -5.153800228976328945, 38.54057627198103120 ) ) ;
#87054=CARTESIAN_POINT ( 'NONE',  ( -5.719274019375665041, -21.55341960407619695, 79.79275706135236135 ) ) ;
#87055=CARTESIAN_POINT ( 'NONE',  ( 17.05116617787827948, -6.768360034955673399, 31.15675553259201180 ) ) ;
#87056=CARTESIAN_POINT ( 'NONE',  ( 0.05219959533910956823, 16.53943276465976808, 29.99890960531435979 ) ) ;
#87057=CARTESIAN_POINT ( 'NONE',  ( 17.50000000000002487, 4.658240926743192567, 113.5552958218319901 ) ) ;
#87058=CARTESIAN_POINT ( 'NONE',  ( -10.81492255796078084, -18.62759615963271287, 47.08224293864770260 ) ) ;
#87060=CARTESIAN_POINT ( 'NONE',  ( -19.03943276465977164, 0.05219959533909376836, 96.24890960531436690 ) ) ;
#87061=CARTESIAN_POINT ( 'NONE',  ( -8.224510206698948167, 14.34966873604960824, 90.41557627198103830 ) ) ;
#87062=CARTESIAN_POINT ( 'NONE',  ( 16.51473224551083163, -9.474510206698727899, 100.8344237280190043 ) ) ;
#87063=CARTESIAN_POINT ( 'NONE',  ( -18.67979575497178146, -10.72451020669898902, 56.66557627198103830 ) ) ;
#87064=ORIENTED_EDGE ( 'NONE', *, *, #15340, .T. ) ;
#87065=CARTESIAN_POINT ( 'NONE',  ( -13.89961937509977652, 13.97604488694528158, 30.62390960531435269 ) ) ;
#87066=CARTESIAN_POINT ( 'NONE',  ( -9.564922557960796823, -16.46253265017161027, 87.08224293864769550 ) ) ;
#87067=CARTESIAN_POINT ( 'NONE',  ( 10.72451020669898902, -18.67979575497178502, 87.91557627198103830 ) ) ;
#87068=CARTESIAN_POINT ( 'NONE',  ( 4.379528057220092307, 16.55341960407617563, 107.2927570613523471 ) ) ;
#87069=CARTESIAN_POINT ( 'NONE',  ( -19.02544592524342804, 5.153800228976336051, 101.0405762719810241 ) ) ;
#87070=CARTESIAN_POINT ( 'NONE',  ( -16.51473224551082808, 9.474510206698731452, 83.33442372801899012 ) ) ;
#87071=CARTESIAN_POINT ( 'NONE',  ( 10.81492255796106328, -18.62759615963255655, 95.41775706135234714 ) ) ;
#87072=CARTESIAN_POINT ( 'NONE',  ( -18.62759615963270932, 10.81492255796079327, 75.83224293864769550 ) ) ;
#87073=CARTESIAN_POINT ( 'NONE',  ( 15.72974639402199770, -15.80617190586745480, 43.12390960531435269 ) ) ;
#87074=CARTESIAN_POINT ( 'NONE',  ( 5.153800228976335163, 19.02544592524342804, 54.79057627198103120 ) ) ;
#87075=CARTESIAN_POINT ( 'NONE',  ( -16.53943276465976808, -0.05219959533934237506, 108.7510903946857042 ) ) ;
#87076=CARTESIAN_POINT ( 'NONE',  ( 5.153800228976335163, 19.02544592524342804, 69.79057627198103830 ) ) ;
#87078=CARTESIAN_POINT ( 'NONE',  ( 18.22780087662121673, 5.500000000000056843, 38.98459894673893444 ) ) ;
#87079=CARTESIAN_POINT ( 'NONE',  ( -16.51473224551082808, 9.474510206698731452, 28.33442372801900433 ) ) ;
#87080=CARTESIAN_POINT ( 'NONE',  ( 8.224510206698953496, -14.34966873604960469, 77.91557627198102409 ) ) ;
#87081=CARTESIAN_POINT ( 'NONE',  ( 21.55341960407619695, -5.719274019375665929, 21.04275706135234714 ) ) ;
#87083=CARTESIAN_POINT ( 'NONE',  ( -10.72451020669898014, 18.67979575497178502, 65.41557627198102409 ) ) ;
#87084=CARTESIAN_POINT ( 'NONE',  ( 4.483927247898790824, -16.52544592524335698, 90.20942372801903275 ) ) ;
#87085=CARTESIAN_POINT ( 'NONE',  ( 16.51473224551069308, 9.474510206698969483, 29.16557627198103475 ) ) ;
#87086=CARTESIAN_POINT ( 'NONE',  ( -19.05341960407611168, -5.049401038298163336, 71.45724293864766707 ) ) ;
#87088=CARTESIAN_POINT ( 'NONE',  ( -12.06949235617756955, 12.14591786802309770, 35.62390960531437401 ) ) ;
#87090=CARTESIAN_POINT ( 'NONE',  ( -0.05219959533937732626, 21.53943276465977519, 57.50109039468568994 ) ) ;
#87091=CARTESIAN_POINT ( 'NONE',  ( 9.564922557960805705, 16.46253265017160317, 114.5822429386476955 ) ) ;
#87092=CARTESIAN_POINT ( 'NONE',  ( 0.05219959533937995610, -21.53943276465977519, 100.0010903946857042 ) ) ;
#87093=CARTESIAN_POINT ( 'NONE',  ( -5.049401038298153566, 19.05341960407611168, 30.20724293864768839 ) ) ;
#87094=CARTESIAN_POINT ( 'NONE',  ( 9.474510206698971260, -16.51473224551069308, 32.91557627198102409 ) ) ;
#87096=CARTESIAN_POINT ( 'NONE',  ( -18.62759615963255300, -10.81492255796106328, 99.16775706135234714 ) ) ;
#87097=CARTESIAN_POINT ( 'NONE',  ( 8.224510206698742110, 14.34966873604972548, 47.08442372801901854 ) ) ;
#87098=CARTESIAN_POINT ( 'NONE',  ( 18.67979575497194134, -10.72451020669871369, 80.83442372801901854 ) ) ;
#87099=CARTESIAN_POINT ( 'NONE',  ( 13.97604488694527802, 13.89961937509977652, 99.37390960531436690 ) ) ;
#87100=CARTESIAN_POINT ( 'NONE',  ( -19.03943276465977164, -0.05219959533935918106, 88.75109039468567573 ) ) ;
#87101=CARTESIAN_POINT ( 'NONE',  ( 10.72451020669871369, 18.67979575497193778, 57.08442372801901854 ) ) ;
#87102=CARTESIAN_POINT ( 'NONE',  ( -5.153800228976607833, 19.02544592524334988, 112.7094237280190043 ) ) ;
#87103=CARTESIAN_POINT ( 'NONE',  ( 16.51473224551083163, -9.474510206698727899, 90.83442372801900433 ) ) ;
#87104=CARTESIAN_POINT ( 'NONE',  ( -9.564922557960796823, -16.46253265017161027, 47.08224293864769550 ) ) ;
#87105=CARTESIAN_POINT ( 'NONE',  ( -19.05341960407617563, 5.049401038297882671, 93.54275706135234714 ) ) ;
#87106=CARTESIAN_POINT ( 'NONE',  ( 9.564922557961047289, -16.46253265017146816, 90.41775706135234714 ) ) ;
#87107=CARTESIAN_POINT ( 'NONE',  ( 8.314922557960818139, 14.29746914071049879, 49.58224293864769550 ) ) ;
#87108=CARTESIAN_POINT ( 'NONE',  ( -16.46253265017146816, -9.564922557961047289, 69.16775706135233293 ) ) ;
#87109=CARTESIAN_POINT ( 'NONE',  ( 4.379528057220092307, 16.55341960407617563, 67.29275706135234714 ) ) ;
#87110=CARTESIAN_POINT ( 'NONE',  ( -16.46253265017146816, -9.564922557961047289, 24.16775706135233648 ) ) ;
#87111=CARTESIAN_POINT ( 'NONE',  ( 13.97604488694527802, 13.89961937509977652, 39.37390960531435269 ) ) ;
#87112=CARTESIAN_POINT ( 'NONE',  ( -13.89961937509977652, 13.97604488694528158, 45.62390960531433848 ) ) ;
#87113=CARTESIAN_POINT ( 'NONE',  ( -8.314922557961024197, 14.29746914071037800, 57.91775706135234714 ) ) ;
#87116=CARTESIAN_POINT ( 'NONE',  ( -13.97604488694527625, -13.89961937509977652, 101.8739096053143811 ) ) ;
#87118=CARTESIAN_POINT ( 'NONE',  ( 17.50000000000000000, -5.500000000000000888, 120.0000000000000142 ) ) ;
#87120=CARTESIAN_POINT ( 'NONE',  ( 5.049401038297881783, 19.05341960407617563, 102.2927570613523045 ) ) ;
#87121=CIRCLE ( 'NONE', #106605, 2.000000000000001776 ) ;
#87122=CARTESIAN_POINT ( 'NONE',  ( -5.719274019375978568, 21.55341960407610458, 40.20724293864769550 ) ) ;
#87123=CARTESIAN_POINT ( 'NONE',  ( 9.474510206698729675, 16.51473224551082808, 37.08442372801899722 ) ) ;
#87124=CARTESIAN_POINT ( 'NONE',  ( 16.55341960407618274, -4.379528057220086978, 21.04275706135234714 ) ) ;
#87125=CARTESIAN_POINT ( 'NONE',  ( -9.564922557960796823, -16.46253265017161027, 32.08224293864769550 ) ) ;
#87126=CARTESIAN_POINT ( 'NONE',  ( -19.02544592524342804, 5.153800228976336051, 31.04057627198102409 ) ) ;
#87127=CARTESIAN_POINT ( 'NONE',  ( 15.72974639402199770, -15.80617190586745480, 78.12390960531436690 ) ) ;
#87128=CARTESIAN_POINT ( 'NONE',  ( -13.89961937509977652, 13.97604488694528158, 40.62390960531435979 ) ) ;
#87130=CARTESIAN_POINT ( 'NONE',  ( -5.153800228976607833, 19.02544592524334988, 82.70942372801897591 ) ) ;
#87131=CARTESIAN_POINT ( 'NONE',  ( -8.224510206698948167, 14.34966873604960824, 50.41557627198103120 ) ) ;
#87132=CARTESIAN_POINT ( 'NONE',  ( -10.72451020669898014, 18.67979575497178502, 30.41557627198101699 ) ) ;
#87133=CARTESIAN_POINT ( 'NONE',  ( -0.05219959533937732626, 21.53943276465977519, 102.5010903946856899 ) ) ;
#87135=CARTESIAN_POINT ( 'NONE',  ( 15.72974639402199770, -15.80617190586745480, 88.12390960531436690 ) ) ;
#87136=CARTESIAN_POINT ( 'NONE',  ( -18.62759615963255300, -10.81492255796106328, 69.16775706135234714 ) ) ;
#87137=CARTESIAN_POINT ( 'NONE',  ( 10.81492255796106328, -18.62759615963255655, 60.41775706135235424 ) ) ;
#87138=CARTESIAN_POINT ( 'NONE',  ( 9.564922557960805705, 16.46253265017160317, 104.5822429386476955 ) ) ;
#87139=CARTESIAN_POINT ( 'NONE',  ( 16.52544592524335698, 4.483927247898782831, 101.4594237280190185 ) ) ;
#87140=CARTESIAN_POINT ( 'NONE',  ( 15.80617190586769283, -15.72974639402175789, 65.62609039468568994 ) ) ;
#87141=CARTESIAN_POINT ( 'NONE',  ( 0.05219959533909260263, 19.03943276465977164, 54.99890960531435979 ) ) ;
#87142=( BOUNDED_SURFACE ( )  B_SPLINE_SURFACE ( 3, 2, ( 
 ( #8012, #101018, #69695, #148545, #131362, #162703, #10036, #54528, #116201, #39360, #71696, #24208, #133363, #200021, #106009, #167695, #154505, #105025, #152509, #182869, #166709, #184847, #47338, #137342, #124152, #153505, #89853, #61489, #185851, #123159, #151536, #807, #77659, #13998, #32162, #169673, #31169, #16992, #29192, #13025, #91813, #90826, #75665, #139328, #108993, #15002, #16001, #74690, #136356, #106996, #199022, #46331, #170674, #107986, #138341, #60491, #93819, #122167, #183857, #92819, #62480, #155499, #78646, #140321, #1811, #121175, #168669, #63489, #181875, #43354, #28213, #198032, #45344, #59500, #44350, #30169, #76662, #171668, #97771, #49317, #156494, #17996, #142310, #33157, #95808, #2807, #36119, #158476, #79649, #129114, #175644, #37118, #109988, #94816, #173668, #159458, #64485, #3790, #82611, #160471, #4776, #20954, #96787, #35135, #141318, #19964, #65467, #126152, #186864, #143290, #174654, #110977, #81606, #187848, #128126, #66464, #157494, #189828, #67456, #144292, #111976, #5782, #172662, #34149, #48333, #18987, #51300, #112961, #80633, #21962, #127130, #188836, #50321, #83613, #190813, #52288, #113945, #98777, #145291, #125165, #6774, #23963, #85618, #55287, #132129, #116959, #70464, #193822, #147305, #162462, #69458, #131125, #22961, #38133, #191803, #177655, #8794, #39124, #53284, #178650, #68453, #146288, #130107, #114963, #176656, #99786, #192813, #7775, #161472, #100779, #115967, #84609, #54295, #20599, #21604, #141951, #18632, #174303, #19617, #128765, #176298, #51937, #5423, #158125, #114601, #81259, #142940, #160117, #6419, #68100, #191449, #52926, #113597, #188479, #35772, #98420, #175291, #83262, #144937, #84256, #4422, #37770, #48967, #127774, #95452, #157137, #129752, #173308, #80279, #3440, #66108, #65116, #189474, #126774, #99432, #82251, #49959, #161114, #22610, #145938, #33792, #111623, #97419, #7419, #34782, #50952, #69103, #130769, #190464, #110621, #143942, #159105, #96438, #67106, #112611, #36757, #172303, #10448, #41783, #116613, #40776, #38780, #195474, #72108, #24623, #133781, #134797, #103450, #179312, #73128, #178301, #131783, #53944, #39765, #56950, #148959, #147961, #89268, #54941, #101429, #146952, #27628, #102445, #118624, #87274, #164132, #149951, #192461, #25630, #165128, #26620, #150959, #181302, #12453, #57948, #42780, #88263, #11456, #194466, #55937, #163120, #193464, #117614, #196478, #86271, #180315, #119619, #74115, #9448, #104442, #166126, #115619, #177308, #100436, #162117, #23614, #85261, #71113, #132779, #8440, #70113, #133191, #194882, #56356, #11880, #87684, #73543, #162528, #69526, #148370, #24031, #85685, #195898, #165545, #9865, #10865, #131191, #7840, #163543, #8861, #118038, #27042, #41199, #179729, #147372, #103864, #70528, #132197, #149369, #57373, #119046, #180728, #42204, #102861, #177720, #25043, #72535, #164546, #134211, #88688, #135216, #193888, #150384, #38196, #117023, #84674, #146353, #196888, #55353, #192881, #54359, #178718, #116031, #40180, #39188, #58355, #71524, #100846, #120022, #99852, #161536, #23029, #101859, #86686, #26039, #59334, #198863, #139159, #16824, #61322, #15829, #153335, #30008, #89686, #76499, #122004, #151371, #43188, #199856, #30999, #105846, #91646, #28045, #184679, #122993, #13835, #46162, #123976, #92648, #168510, #62306, #167533, #121004, #104857, #29028, #107816, #138175, #137175, #78475, #44187, #90668, #136192, #140148, #14836, #169500, #154337, #77489, #636, #181707, #197867, #12862, #185674, #155335, #152350, #47164, #75501, #108823, #1640, #183695, #31992, #60330, #170502, #93650, #74527, #63317, #166546, #45181, #182702, #106835, #126961, #128949, #187684, #81440, #111809, #6609, #49154, #96622, #175478, #159290, #190650, #34970, #127958, #98612, #143126, #110812, #172495, #97602, #48162, #158311, #174488, #52126, #109820, #113782, #80465, #67291, #19799, #20787 ),
 ( #33982, #36950, #160306, #83448, #4606, #186692, #66298, #142139, #21796, #50150, #145125, #35955, #124997, #171503, #32992, #82442, #144130, #94646, #189661, #51134, #156326, #3623, #95638, #112794, #5612, #17826, #79484, #141153, #2642, #157326, #65302, #64318, #125986, #18821, #188670, #173497, #132969, #54132, #53118, #114796, #116798, #102640, #146123, #85453, #25818, #103643, #148148, #164325, #39956, #178489, #176489, #163316, #8631, #37965, #129939, #86463, #117810, #192649, #101627, #99623, #71306, #9639, #100621, #194659, #10641, #179503, #55128, #56128, #161304, #40969, #38965, #22799, #24814, #150149, #26813, #7607, #72302, #165321, #87464, #149151, #84445, #69293, #133980, #41976, #162303, #195671, #115805, #57142, #88453, #70303, #118818, #23803, #180504, #68288, #130959, #191638, #177495, #147143, #131972, #193656, #13607, #15595, #74301, #168278, #198634, #93408, #135970, #183461, #62074, #45929, #77253, #121768, #14602, #185438, #29775, #197641, #59107, #184449, #134987, #44947, #61087, #138921, #196665, #402, #167304, #154101, #106602, #107584, #120772, #31759, #92415, #123739, #136945, #181488, #11650, #137936, #91410, #153098, #58134, #46928, #60100, #182473, #108588, #170265, #73316, #76258, #119803, #199620, #28800, #42966, #122759, #104629, #169262, #166318, #27815, #89456, #30768, #151145, #12636, #43954, #105616, #90439, #152125, #75275, #111570, #173254, #82198, #159054, #97368, #158074, #125748, #95399, #34729, #127723, #126722, #124756, #141899, #157085, #186452, #80228, #19565, #49904, #17582, #96387, #51886, #36704, #171265, #81209, #139907, #79242, #142890, #35721, #109582, #20548, #67055, #18581, #3390, #64078, #94404, #63077, #4372, #143890, #66056, #47928, #174253, #189425, #50900, #112558, #128713, #5371, #190410, #140913, #32753, #65065, #2399, #187448, #113545, #175239, #188426, #155094, #156085, #48916, #16588, #110570, #78236, #1397, #172251, #33739, #7365, #164078, #69050, #192409, #9393, #55883, #117556, #40721, #102390, #163062, #37716, #85205, #147907, #101372, #71059, #194413, #133724, #130716, #87221, #98366, #177253, #144886, #6368, #132725, #22556, #129700, #191397, #115566, #68048, #53891, #176245, #179256, #131728, #25577, #148903, #52874, #84202, #83211, #114546, #146894, #10393, #99378, #38725, #72050, #195416, #178248, #56894, #70060, #8385, #161061, #193410, #100383, #145882, #160064, #116559, #118568, #162061, #54885, #23557, #24568, #39709, #86217, #180258, #21551, #91168, #28559, #122516, #166068, #181246, #103392, #89209, #183219, #198380, #197400, #138680, #104385, #150902, #196421, #77008, #90196, #44700, #136699, #151879, #199377, #41728, #13369, #152857, #76017, #161, #30516, #61829, #107339, #92168, #14352, #137692, #121524, #184206, #60841, #75033, #45688, #27570, #42723, #165070, #12396, #106354, #59857, #58866, #123499, #74058, #135729, #57891, #26564, #168038, #29535, #169012, #153854, #15352, #88207, #149891, #11398, #73067, #134739, #119563, #120532, #182225, #43710, #105371, #167058, #187208, #48679, #94162, #124510, #93166, #64831, #127484, #126493, #154851, #4136, #79998, #141666, #3158, #158817, #34496, #20305, #109337, #16349, #95160, #171019, #32510, #142657, #112323, #156848, #157843, #77997, #139664, #110331, #155841, #188191, #174013, #49663, #111327, #17338, #50662, #78994, #140668, #96154, #65815, #189189, #35484, #97133, #173017, #186205, #172012, #19334, #80982, #81953, #143645, #5128, #2160, #66810, #185192, #63838, #31513, #1152, #46683, #125511, #62827, #47687, #33501, #18343, #108342, #170023, #39471, #161822, #132489, #70820, #82971, #114306, #113309, #175000, #177015, #162818, #6131, #145647, #85976, #163836, #8136, #24327, #100141, #38484, #36465, #23317, #68809, #98122, #190169, #146643, #178004, #52641, #84961, #159819, #131481, #69814, #160828, #83967, #193168, #147666, #21314, #54640, #25338 ),
 ( #130468, #192166, #37477, #67814, #144648, #116315, #194178, #101132, #129469, #9154, #55642, #117315, #179011, #102151, #40479, #86979, #176008, #191168, #148666, #99138, #22316, #10154, #128473, #51645, #7127, #53646, #115323, #197166, #42485, #151647, #199136, #74804, #28328, #181011, #137457, #104148, #165830, #182983, #29305, #90935, #14112, #75779, #136467, #11156, #58632, #121290, #198147, #44467, #167805, #107107, #27327, #60603, #71814, #150663, #118328, #180021, #106121, #196186, #103153, #164834, #88973, #41488, #12161, #149658, #152621, #105141, #122278, #183966, #26330, #57658, #56655, #87970, #120298, #45453, #72830, #73826, #168777, #30279, #13142, #91925, #43473, #181991, #134500, #166827, #135496, #119324, #133482, #89967, #153617, #59617, #195174, #61596, #18108, #33269, #47448, #94928, #157605, #64598, #1923, #95920, #139434, #154614, #76774, #62590, #156613, #171781, #170783, #112091, #77767, #186975, #138446, #79762, #32273, #142423, #140433, #3902, #126262, #15113, #127241, #200127, #172780, #187959, #173781, #141433, #2920, #123265, #93930, #124268, #49429, #111090, #65582, #19096, #80745, #34261, #185963, #155609, #188955, #50432, #48445, #184956, #63602, #17104, #46440, #125278, #35248, #110102, #916, #96901, #108099, #169784, #31277, #92928, #16109, #109104, #78756, #39234, #113071, #100890, #70575, #23075, #51411, #7887, #129227, #143403, #130220, #40229, #117068, #97881, #162574, #193935, #191915, #145403, #174763, #66574, #24077, #132243, #190924, #53399, #144407, #161581, #55398, #160584, #8907, #114060, #84720, #192927, #36229, #146398, #178764, #52401, #176769, #54405, #22073, #85733, #21070, #115077, #6885, #158585, #82726, #38241, #20074, #116077, #147420, #68563, #69573, #81718, #99896, #5893, #67569, #131239, #4892, #177765, #128239, #189936, #159572, #175757, #37234, #98890, #83724, #430, #149413, #124783, #185467, #16616, #27087, #71571, #186481, #28090, #11923, #43235, #25089, #31787, #88733, #10909, #46957, #155122, #63105, #196931, #58399, #120065, #78264, #154130, #139936, #26084, #133236, #73587, #87728, #72582, #62104, #93436, #135259, #77281, #194928, #56403, #150428, #134256, #181753, #1426, #104901, #166590, #195943, #170293, #57417, #119090, #15624, #123767, #108616, #101906, #163588, #92444, #41244, #138950, #86731, #148416, #9911, #118085, #179775, #180772, #102906, #164590, #42247, #103908, #165589, #20575, #172279, #79270, #140941, #65092, #94432, #18608, #125775, #159081, #81236, #51914, #190438, #2428, #33768, #32780, #156113, #96415, #82228, #187475, #126751, #5399, #83238, #127750, #143918, #19593, #158101, #17611, #142917, #188453, #64108, #109609, #66084, #97395, #95428, #4399, #48944, #50928, #189451, #80256, #112586, #113573, #67082, #34756, #128742, #157112, #110597, #171293, #141926, #174280, #35749, #3417, #144914, #49934, #111599, #173283, #6397, #175267, #36733, #98396, #160094, #21580, #47958, #68076, #129730, #25607, #26596, #180291, #149924, #56926, #41759, #102421, #40753, #193441, #54917, #100413, #130748, #99408, #71088, #133757, #132755, #161091, #10425, #164108, #178278, #72083, #115596, #192440, #52903, #38756, #194442, #147937, #146928, #88239, #53922, #162094, #145912, #11431, #39741, #55913, #86247, #101403, #148935, #191427, #163097, #87251, #195452, #73101, #103424, #114579, #118601, #165103, #176277, #37748, #116589, #24600, #23589, #177285, #22586, #117587, #84234, #179288, #7397, #69081, #9423, #85237, #8418, #70090, #131759, #170058, #58898, #166101, #44733, #120564, #182258, #92206, #61865, #106389, #107376, #27603, #104418, #59890, #105405, #14385, #123534, #137727, #91199, #43743, #196, #167090, #28591, #45723, #153890, #15387, #77044, #138715, #199411, #74091, #121556, #184242, #60875, #169048, #30554, #31549, #90228, #185228, #134771, #13401, #181278, #42755, #46719, #151912, #89242, #150935, #75065 ),
 ( #12428, #136731, #108382, #93201, #76051, #154886, #168070, #183252, #135761, #29568, #198413, #197432, #196454, #152889, #16384, #122552, #57924, #119595, #81016, #96189, #110365, #157878, #20341, #3191, #47720, #98157, #4171, #188225, #19367, #1186, #5164, #64864, #187242, #81990, #128510, #36503, #49698, #139700, #142691, #33534, #66847, #126526, #190205, #127519, #78031, #51684, #62863, #35520, #189223, #159857, #65849, #50701, #124545, #95196, #125546, #34529, #112360, #113346, #143683, #175038, #174051, #48712, #18379, #97168, #158853, #111363, #109371, #173052, #80031, #171053, #186242, #32543, #94196, #140703, #155876, #17373, #79028, #2193, #63875, #172047, #156882, #141700, #102190, #176044, #163878, #133522, #86016, #114341, #70858, #192204, #6168, #193206, #103193, #180061, #160864, #25377, #56694, #54679, #8176, #37512, #129503, #87019, #195214, #53686, #116353, #7166, #24365, #118368, #23355, #71853, #177053, #147705, #55681, #99174, #9193, #41530, #115363, #39510, #117355, #85000, #148705, #84006, #178042, #69852, #21350, #145684, #101170, #83008, #179051, #10193, #131520, #132527, #144683, #162858, #68849, #130508, #194216, #67848, #40519, #191203, #38523, #100179, #52678, #22354, #161861, #146681, #74841, #150702, #89011, #122315, #91961, #120334, #107144, #136504, #60641, #12200, #184993, #45489, #76811, #90004, #134539, #46477, #90972, #198184, #106160, #88009, #153654, #151686, #73865, #168814, #15149, #123301, #59654, #26369, #167842, #182029, #138482, #13178, #200163, #14149, #164874, #61633, #149697, #184006, #75816, #11195, #29343, #152659, #72870, #43512, #135534, #121328, #183020, #196227, #30318, #57697, #137494, #197205, #105178, #44504, #199174, #119365, #181049, #42524, #166864, #104187, #165869, #27365, #58668, #28366, #126293, #4923, #189967, #124303, #34292, #92965, #170818, #95953, #188987, #62625, #50462, #20105, #172812, #950, #157638, #78791, #154651, #79795, #108137, #66605, #47482, #112121, #143436, #141468, #94961, #186000, #16146, #173813, #81749, #140469, #2952, #93964, #111122, #128269, #110135, #158615, #63637, #19127, #142455, #109139, #80777, #169821, #1958, #187990, #3933, #171814, #35278, #32310, #64631, #156646, #31312, #155644, #49460, #77801, #65613, #96933, #18141, #127273, #139470, #17139, #125313, #187009, #48479, #33302, #148448, #117101, #99927, #97913, #178796, #69605, #147452, #53432, #55430, #114090, #7920, #38273, #133268, #175791, #23106, #101939, #85766, #40265, #161612, #54438, #25121, #131271, #37265, #98923, #24111, #174793, #9943, #163620, #84752, #159604, #86765, #6917, #193967, #146430, #8940, #160615, #71602, #132276, #51442, #176800, #21103, #113102, #177796, #192959, #116108, #36259, #82758, #39266, #22105, #144438, #5924, #67601, #100922, #129260, #162607, #68595, #190955, #70609, #52432, #83755, #145434, #130251, #191946, #115108, #105916, #153412, #197938, #59407, #179805, #150456, #42279, #151444, #12931, #122074, #198935, #137249, #121081, #165617, #135286, #74595, #167602, #166617, #164621, #181781, #196958, #26115, #120093, #182776, #89758, #57446, #136263, #91718, #76572, #10939, #44259, #41274, #119119, #29097, #75573, #149443, #60402, #106906, #90736, #87758, #152419, #27116, #102936, #28119, #194959, #14911, #134287, #183766, #30077, #13907, #43262, #72612, #195974, #45252, #168579, #88763, #56436, #180800, #118117, #103937, #58426, #11951, #73615, #104930, #172570, #31076, #2715, #35041, #32069, #169578, #92723, #155407, #184752, #108899, #15906, #49227, #171575, #142214, #80540, #154412, #124053, #123066, #46237, #186766, #34056, #77564, #16897, #95714, #173572, #17901, #157401, #109891, #48236, #107891, #33064, #78548, #139236, #199931, #156397, #187757, #62383, #94719, #711, #141224, #79556, #170578, #64392, #3697, #110885, #125069, #18894, #185752, #47241, #61394, #93725, #126060, #65376, #140223, #96695 ),
 ( #158384, #127036, #19873, #188743, #50228, #111882, #138247, #1716, #63392, #190723, #20862, #189735, #161377, #23872, #22868, #51208, #100689, #115876, #66373, #52196, #67363, #131031, #116866, #5687, #112869, #191708, #129022, #113854, #39034, #8702, #53192, #54204, #174560, #36027, #6680, #175550, #84515, #70372, #146193, #38037, #37025, #147211, #98686, #160379, #192720, #162371, #85523, #132040, #193729, #7678, #82519, #68358, #177565, #69362, #55197, #178557, #40023, #21870, #101696, #81513, #83520, #128033, #97676, #163385, #145197, #143200, #4681, #159365, #144201, #130009, #114867, #176562, #99693, #74369, #60168, #149219, #56197, #135058, #10710, #72373, #182542, #152191, #196734, #197709, #117880, #194727, #150222, #195740, #104700, #13675, #27884, #181555, #134047, #90509, #57213, #118888, #136035, #44024, #105685, #167372, #28869, #89526, #164394, #11719, #59175, #151215, #120843, #75342, #121837, #180572, #137012, #24882, #103710, #71373, #133037, #198702, #42046, #179570, #41040, #165390, #102706, #26883, #25887, #183531, #58202, #45015, #106674, #87532, #88526, #9709, #73386, #119870, #86531, #43034, #166388, #148215, #12703, #47998, #2469, #139978, #16657, #76330, #63145, #108657, #138007, #29843, #186524, #17652, #92485, #78305, #14669, #171334, #109652, #471, #32822, #110639, #79312, #155165, #48984, #154174, #107653, #91480, #15665, #94473, #124824, #123809, #65134, #30837, #77324, #122829, #3457, #1467, #156154, #140981, #64151, #125815, #168347, #187518, #172320, #33809, #126791, #157155, #188497, #95469, #18650, #80296, #141968, #170335, #31828, #138992, #169330, #199691, #49976, #153168, #61156, #184518, #45998, #62145, #185507, #46998, #93478, #163906, #175308, #179077, #174320, #118392, #102217, #71877, #128782, #19634, #180086, #70885, #113614, #83279, #34800, #87044, #190482, #35790, #25402, #10217, #56721, #36774, #173325, #147731, #20618, #148729, #51954, #133547, #132553, #111640, #96455, #158142, #195237, #81276, #142958, #40548, #4438, #189491, #98439, #160134, #55708, #117380, #66126, #127791, #50969, #112628, #9218, #194241, #97437, #159122, #82268, #21622, #143960, #5440, #67124, #17301, #156812, #187171, #154811, #110294, #191869, #176723, #108303, #18304, #76970, #16309, #79960, #172978, #46643, #37185, #6839, #141629, #185153, #3119, #62788, #138641, #63802, #92129, #53352, #31474, #98843, #130172, #125475, #78955, #169983, #122, #160538, #68518, #124469, #48642, #77959, #95122, #115030, #94124, #145357, #47648, #64794, #126455, #93126, #188153, #153816, #186166, #171976, #49626, #155803, #22027, #139626, #33464, #140630, #15311, #1114, #111288, #61791, #83679, #123461, #2120, #109299, #170978, #32471, #113328, #3176, #64849, #129487, #81001, #188209, #49681, #174032, #126511, #127502, #34514, #67831, #190189, #160845, #99156, #111345, #142675, #141685, #173036, #5148, #191185, #96172, #35503, #114323, #192184, #36484, #52661, #128494, #66830, #157862, #51664, #97153, #19352, #18363, #175021, #6151, #4154, #98140, #65833, #159838, #21332, #189207, #82990, #22334, #176025, #143666, #37494, #50684, #112342, #80016, #158836, #144666, #83985, #20324, #53665, #81973, #145664, #7145, #115343, #68829, #130488, #177033, #38503, #156867, #100159, #148684, #11174, #134519, #135515, #88991, #58650, #165849, #150682, #72849, #149676, #102169, #163857, #9172, #39490, #8156, #180040, #56673, #146661, #10172, #161841, #196205, #84979, #70839, #85996, #57677, #197186, #24345, #131499, #71832, #147685, #132507, #119345, #27345, #133501, #181029, #193186, #69832, #25356, #194196, #41509, #12180, #103172, #118346, #55661, #73844, #117335, #179030, #42503, #104167, #120316, #182010, #23335, #164852, #101150, #86997, #54659, #26348, #116333, #178022, #162837, #40497, #195193, #87988, #122295, #200144, #199154, #140449, #106140, #90952, #198165, #78773, #30299, #184973 ),
 ( #93946, #77782, #109121, #153635, #46458, #17121, #61614, #1939, #183985, #45470, #59635, #63619, #170799, #91942, #89985, #32291, #60621, #185981, #15130, #139451, #152639, #125295, #124284, #155625, #168795, #13160, #43492, #169801, #76792, #108118, #166845, #105159, #138463, #14129, #47464, #28347, #151666, #123282, #74824, #31294, #107124, #136485, #92946, #121309, #154632, #183001, #44485, #167823, #932, #16127, #29322, #62606, #75796, #137474, #142439, #34276, #143419, #4906, #114073, #190938, #129242, #189951, #157621, #127257, #66589, #159587, #158599, #156628, #173796, #188970, #18123, #112105, #51425, #81733, #49443, #128253, #83738, #68578, #2935, #113085, #171796, #111106, #174777, #67584, #141450, #52415, #98905, #36243, #79778, #97896, #19111, #33284, #20089, #186991, #145417, #126277, #175774, #22088, #21084, #35262, #64615, #94944, #37248, #160598, #80761, #82741, #172795, #144421, #95935, #5907, #6899, #48461, #187974, #110118, #3917, #65597, #50446, #96917, #84734, #72596, #42261, #194943, #23089, #179789, #100905, #115091, #101921, #11935, #88746, #69587, #134270, #165601, #163603, #117084, #146412, #38256, #195957, #103921, #162589, #25104, #116091, #133251, #27100, #132259, #180784, #85748, #56419, #164605, #7903, #118099, #150439, #24094, #148431, #26099, #193950, #57430, #192942, #86748, #178779, #130234, #54421, #9926, #191930, #87742, #119103, #40247, #41258, #53414, #71585, #176783, #8923, #55413, #131254, #99910, #161595, #102920, #177779, #39249, #147435, #70591, #149427, #10923, #121063, #93705, #154391, #185731, #198915, #43246, #155387, #199911, #183748, #14892, #196942, #691, #60384, #182757, #15886, #124032, #32048, #45234, #135270, #76553, #29079, #62363, #122056, #47220, #123046, #73598, #108879, #58410, #31055, #184732, #120077, #138229, #61375, #181765, #90718, #44241, #30059, #91700, #170558, #77544, #139216, #46217, #105898, #13888, #153394, #107870, #106888, #104914, #168561, #75555, #166601, #169558, #92703, #28101, #89740, #151426, #12913, #74577, #152401, #136245, #197921, #167584, #59389, #137231, #66352, #144181, #188723, #189715, #109870, #186746, #142194, #187736, #96676, #5667, #19853, #173552, #126040, #82499, #49207, #110865, #128013, #174540, #36007, #159345, #20841, #81493, #156376, #3677, #51188, #143180, #112849, #97656, #52176, #172550, #67343, #16877, #95693, #63372, #125049, #129004, #141205, #48216, #171554, #34036, #33044, #157381, #94699, #190703, #50208, #113834, #175530, #17881, #2695, #1696, #79535, #65355, #37004, #64372, #18874, #98665, #78528, #158364, #140202, #111862, #127016, #80520, #35021, #4660, #68339, #21849, #178539, #9690, #84496, #8683, #6661, #163367, #40005, #192701, #101677, #102688, #71355, #147193, #41022, #146174, #99674, #83500, #7659, #24863, #116848, #115857, #57195, #22849, #69343, #114848, #195722, #70354, #86513, #55179, #132021, #117861, #160359, #193710, #133019, #194709, #118870, #149201, #180554, #25869, #10691, #56178, #179552, #162353, #23854, #131010, #161358, #129989, #148197, #164376, #191689, #87513, #42028, #72355, #145177, #134029, #177547, #53171, #85504, #176542, #38018, #54184, #39016, #100671, #61141, #14654, #62130, #106659, #168332, #88507, #59157, #151198, #60152, #121821, #30822, #107638, #45983, #29828, #74352, #44007, #183516, #76314, #75326, #73368, #90493, #105669, #135040, #28853, #91465, #198685, #166370, #44999, #455, #185492, #119853, #153152, #150203, #27867, #137992, #184503, #58185, #169315, #15650, #199675, #196716, #122813, #136018, #11701, #136996, #103692, #123794, #43016, #92470, #138977, #154159, #152175, #181537, #104683, #77308, #165371, #197692, #26865, #89508, #12686, #120826, #167355, #182526, #13658, #49961, #81261, #139963, #111625, #143944, #140966, #65118, #142942, #48969, #50954, #109636, #3442, #33794, #128767, #171319, #18635, #97421, #4424, #112613 ),
 ( #2454, #189476, #80281, #157139, #188481, #173310, #186509, #159107, #172305, #16642, #67109, #34785, #141953, #96440, #170320, #174305, #95454, #156139, #35774, #20601, #82253, #64136, #158127, #66110, #1452, #19619, #5425, #125800, #126776, #127776, #110623, #46982, #32806, #108642, #31812, #93463, #94458, #155149, #78289, #63130, #124809, #47983, #17637, #79297, #187502, #148962, #69105, #192463, #6421, #87277, #55940, #38782, #36759, #117617, #145940, #132782, #162119, #100438, #131786, #54943, #129754, #102448, #115622, #160119, #10451, #116615, #23616, #193466, #113599, #179315, #177310, #99435, #194469, #40779, #72111, #85263, #51939, #178303, #7421, #164136, #146954, #25633, #39767, #190466, #175293, #98422, #147964, #101431, #21606, #163122, #24625, #83265, #130771, #37772, #8442, #70115, #144939, #68102, #191451, #86273, #161116, #53946, #9451, #71116, #52928, #114603, #176300, #22612, #84258, #58925, #198442, #28617, #196481, #151937, #30579, #15411, #149954, #59914, #118627, #57951, #121582, #14410, #88266, #76074, #45748, #183277, #26623, #44758, #104445, #180318, #105432, #133784, #92230, #73131, #137750, #169073, #167115, #120593, #11459, #41786, #199434, #107400, #166129, #90254, #119622, #136757, #153916, #135788, #195477, #75090, #89271, #60902, #182288, #122576, #106413, #56953, #103453, #165131, #91223, #168094, #134800, #29592, #152914, #181305, #150962, #42783, #13426, #184266, #27631, #12457, #74117, #197459, #43768, #17399, #33559, #49723, #48737, #46747, #63900, #79056, #108406, #2218, #141724, #172073, #139723, #95222, #174075, #158877, #93225, #3214, #61889, #1212, #64888, #157901, #31574, #19390, #189247, #126549, #170082, #188249, #47745, #123559, #110391, #77069, #35544, #16408, #81039, #112383, #156908, #125570, #154910, #185254, #142715, #50725, #109398, #18405, #62890, #80054, #97191, #140729, #127547, #32569, #111390, #173076, #78054, #34553, #138739, #171078, #96212, #4195, #187268, #65873, #124570, #220, #186266, #94222, #155902, #194974, #73630, #57461, #88777, #133284, #26131, #196973, #41291, #181798, #101954, #25138, #39282, #120108, #150470, #71618, #69620, #11965, #178811, #165632, #56453, #118132, #164636, #87774, #162623, #135300, #148465, #192974, #43277, #149459, #179820, #10954, #143710, #58440, #9958, #132292, #27130, #104946, #20366, #102952, #119134, #7937, #193984, #8958, #72628, #82014, #147468, #54453, #55446, #180814, #103953, #134303, #131286, #195989, #42293, #116123, #177812, #100939, #117117, #24129, #85782, #70626, #40281, #163636, #86780, #75588, #60417, #77579, #124068, #185770, #108914, #170594, #31091, #105932, #153429, #15921, #169593, #139251, #62399, #1731, #137267, #155422, #166632, #45267, #12947, #74612, #727, #90752, #197954, #59423, #183781, #136278, #198950, #44274, #47257, #199946, #32084, #93741, #121097, #152435, #151459, #182791, #14927, #16912, #167617, #106921, #78565, #63409, #46253, #140238, #138263, #76587, #29113, #61410, #168594, #13921, #28134, #184767, #125084, #122090, #123081, #30094, #92739, #107907, #91733, #154427, #186782, #48252, #89774, #190738, #34070, #49240, #171590, #157414, #51223, #66387, #65390, #6696, #172583, #18908, #64405, #145214, #96710, #112884, #4696, #158398, #67379, #109906, #19887, #20878, #144218, #68374, #98702, #130026, #175566, #160396, #82536, #159383, #111898, #173586, #80553, #110898, #17915, #189751, #128049, #156413, #81528, #33078, #174578, #36043, #37042, #113869, #52212, #97692, #142228, #50242, #5702, #129037, #143215, #79570, #21885, #35055, #141239, #83535, #191725, #94734, #95728, #2728, #126074, #187770, #3713, #127051, #188757, #115891, #179585, #134063, #7696, #195754, #165404, #117895, #146208, #102720, #23889, #38053, #24899, #135071, #11733, #192738, #57228, #88540, #86546, #40039, #69378, #161393, #118902, #26897, #85541, #148230, #39048, #56214, #150237 ) ),
 .UNSPECIFIED., .T., .F., .F. ) 
 B_SPLINE_SURFACE_WITH_KNOTS ( ( 4, 3, 4 ),
 ( 3, 2, 2, 2, 2, 2, 2, 2, 2, 2, 2, 2, 2, 2, 2, 2, 2, 2, 2, 2, 2, 2, 2, 2, 2, 2, 2, 2, 2, 2, 2, 2, 2, 2, 2, 2, 2, 2, 2, 2, 2, 2, 2, 2, 2, 2, 2, 2, 2, 2, 2, 2, 2, 2, 2, 2, 2, 2, 2, 2, 2, 2, 2, 2, 2, 2, 2, 2, 2, 2, 2, 2, 2, 2, 2, 2, 2, 2, 2, 2, 2, 2, 2, 2, 2, 2, 2, 2, 2, 2, 2, 2, 2, 2, 2, 2, 2, 2, 2, 2, 2, 2, 2, 2, 2, 2, 2, 2, 2, 2, 2, 2, 2, 2, 2, 2, 2, 2, 2, 2, 2, 2, 2, 2, 2, 2, 2, 2, 2, 2, 2, 2, 2, 2, 2, 2, 2, 2, 2, 2, 2, 2, 2, 2, 2, 2, 2, 2, 2, 2, 2, 2, 2, 2, 2, 2, 2, 2, 2, 2, 2, 2, 2, 2, 2, 2, 2, 2, 2, 2, 2, 2, 2, 2, 2, 2, 2, 2, 2, 2, 2, 2, 2, 2, 2, 2, 2, 2, 2, 2, 2, 2, 2, 2, 2, 2, 2, 2, 2, 2, 2, 2, 2, 2, 2, 2, 2, 2, 2, 2, 2, 2, 2, 2, 2, 2, 2, 2, 2, 2, 2, 2, 2, 2, 2, 2, 2, 2, 3 ),
 ( 0.000000000000000000, 0.5000000000000000000, 1.000000000000000000 ),
 ( 0.000000000000000000, 0.004385964912280701511, 0.008771929824561403022, 0.01315789473684210453, 0.01754385964912280604, 0.02192982456140350755, 0.02631578947368420907, 0.03070175438596491058, 0.03508771929824561209, 0.03947368421052631360, 0.04385964912280701511, 0.04824561403508771662, 0.05263157894736841813, 0.05701754385964911964, 0.06140350877192982115, 0.06578947368421052266, 0.07017543859649122417, 0.07456140350877192569, 0.07894736842105262720, 0.08333333333333332871, 0.08771929824561403022, 0.09210526315789473173, 0.09649122807017543324, 0.1008771929824561348, 0.1052631578947368363, 0.1096491228070175378, 0.1140350877192982393, 0.1184210526315789408, 0.1228070175438596423, 0.1271929824561403577, 0.1315789473684210453, 0.1359649122807017607, 0.1403508771929824483, 0.1447368421052631637, 0.1491228070175438514, 0.1535087719298245668, 0.1578947368421052544, 0.1622807017543859698, 0.1666666666666666574, 0.1710526315789473728, 0.1754385964912280604, 0.1798245614035087758, 0.1842105263157894635, 0.1885964912280701788, 0.1929824561403508665, 0.1973684210526315819, 0.2017543859649122695, 0.2061403508771929849, 0.2105263157894736725, 0.2149122807017543879, 0.2192982456140350755, 0.2236842105263157909, 0.2280701754385964786, 0.2324561403508771940, 0.2368421052631578816, 0.2412280701754385970, 0.2456140350877192846, 0.2500000000000000000, 0.2543859649122807154, 0.2587719298245614308, 0.2631578947368420907, 0.2675438596491228060, 0.2719298245614035214, 0.2763157894736842368, 0.2807017543859648967, 0.2850877192982456121, 0.2894736842105263275, 0.2938596491228070429, 0.2982456140350877027, 0.3026315789473684181, 0.3070175438596491335, 0.3114035087719298489, 0.3157894736842105088, 0.3201754385964912242, 0.3245614035087719396, 0.3289473684210526550, 0.3333333333333333148, 0.3377192982456140302, 0.3421052631578947456, 0.3464912280701754610, 0.3508771929824561209, 0.3552631578947368363, 0.3596491228070175517, 0.3640350877192982670, 0.3684210526315789269, 0.3728070175438596423, 0.3771929824561403577, 0.3815789473684210731, 0.3859649122807017330, 0.3903508771929824483, 0.3947368421052631637, 0.3991228070175438791, 0.4035087719298245390, 0.4078947368421052544, 0.4122807017543859698, 0.4166666666666666852, 0.4210526315789473450, 0.4254385964912280604, 0.4298245614035087758, 0.4342105263157894912, 0.4385964912280701511, 0.4429824561403508665, 0.4473684210526315819, 0.4517543859649122973, 0.4561403508771929571, 0.4605263157894736725, 0.4649122807017543879, 0.4692982456140351033, 0.4736842105263157632, 0.4780701754385964786, 0.4824561403508771940, 0.4868421052631579093, 0.4912280701754385692, 0.4956140350877192846, 0.5000000000000000000, 0.5043859649122807154, 0.5087719298245614308, 0.5131578947368421462, 0.5175438596491228616, 0.5219298245614034659, 0.5263157894736841813, 0.5307017543859648967, 0.5350877192982456121, 0.5394736842105263275, 0.5438596491228070429, 0.5482456140350877583, 0.5526315789473684736, 0.5570175438596490780, 0.5614035087719297934, 0.5657894736842105088, 0.5701754385964912242, 0.5745614035087719396, 0.5789473684210526550, 0.5833333333333333703, 0.5877192982456140857, 0.5921052631578946901, 0.5964912280701754055, 0.6008771929824561209, 0.6052631578947368363, 0.6096491228070175517, 0.6140350877192982670, 0.6184210526315789824, 0.6228070175438596978, 0.6271929824561403022, 0.6315789473684210176, 0.6359649122807017330, 0.6403508771929824483, 0.6447368421052631637, 0.6491228070175438791, 0.6535087719298245945, 0.6578947368421053099, 0.6622807017543859143, 0.6666666666666666297, 0.6710526315789473450, 0.6754385964912280604, 0.6798245614035087758, 0.6842105263157894912, 0.6885964912280702066, 0.6929824561403509220, 0.6973684210526315264, 0.7017543859649122417, 0.7061403508771929571, 0.7105263157894736725, 0.7149122807017543879, 0.7192982456140351033, 0.7236842105263158187, 0.7280701754385965341, 0.7324561403508771384, 0.7368421052631578538, 0.7412280701754385692, 0.7456140350877192846, 0.7500000000000000000, 0.7543859649122807154, 0.7587719298245614308, 0.7631578947368421462, 0.7675438596491228616, 0.7719298245614034659, 0.7763157894736841813, 0.7807017543859648967, 0.7850877192982456121, 0.7894736842105263275, 0.7938596491228070429, 0.7982456140350877583, 0.8026315789473684736, 0.8070175438596490780, 0.8114035087719297934, 0.8157894736842105088, 0.8201754385964912242, 0.8245614035087719396, 0.8289473684210526550, 0.8333333333333333703, 0.8377192982456140857, 0.8421052631578946901, 0.8464912280701754055, 0.8508771929824561209, 0.8552631578947368363, 0.8596491228070175517, 0.8640350877192982670, 0.8684210526315789824, 0.8728070175438596978, 0.8771929824561403022, 0.8815789473684210176, 0.8859649122807017330, 0.8903508771929824483, 0.8947368421052631637, 0.8991228070175438791, 0.9035087719298245945, 0.9078947368421053099, 0.9122807017543859143, 0.9166666666666666297, 0.9210526315789473450, 0.9254385964912280604, 0.9298245614035087758, 0.9342105263157894912, 0.9385964912280702066, 0.9429824561403509220, 0.9473684210526315264, 0.9517543859649122417, 0.9561403508771929571, 0.9605263157894736725, 0.9649122807017543879, 0.9692982456140351033, 0.9736842105263158187, 0.9780701754385965341, 0.9824561403508771384, 0.9868421052631578538, 0.9912280701754385692, 0.9956140350877192846, 1.000000000000000000 ),
 .UNSPECIFIED. ) 
 GEOMETRIC_REPRESENTATION_ITEM ( )  RATIONAL_B_SPLINE_SURFACE ( (
 ( 1.000000000000000000, 0.9659258262890683122, 1.000000000000000000, 0.9659258262890683122, 1.000000000000000000, 0.9659258262890683122, 1.000000000000000000, 0.9659258262890683122, 1.000000000000000000, 0.9659258262890683122, 1.000000000000000000, 0.9659258262890683122, 1.000000000000000000, 0.9659258262890683122, 1.000000000000000000, 0.9659258262890683122, 1.000000000000000000, 0.9659258262890683122, 1.000000000000000000, 0.9659258262890683122, 1.000000000000000000, 0.9659258262890683122, 1.000000000000000000, 0.9659258262890683122, 1.000000000000000000, 0.9659258262890683122, 1.000000000000000000, 0.9659258262890683122, 1.000000000000000000, 0.9659258262890683122, 1.000000000000000000, 0.9659258262890683122, 1.000000000000000000, 0.9659258262890683122, 1.000000000000000000, 0.9659258262890683122, 1.000000000000000000, 0.9659258262890683122, 1.000000000000000000, 0.9659258262890683122, 1.000000000000000000, 0.9659258262890683122, 1.000000000000000000, 0.9659258262890683122, 1.000000000000000000, 0.9659258262890683122, 1.000000000000000000, 0.9659258262890683122, 1.000000000000000000, 0.9659258262890683122, 1.000000000000000000, 0.9659258262890683122, 1.000000000000000000, 0.9659258262890683122, 1.000000000000000000, 0.9659258262890683122, 1.000000000000000000, 0.9659258262890683122, 1.000000000000000000, 0.9659258262890683122, 1.000000000000000000, 0.9659258262890683122, 1.000000000000000000, 0.9659258262890683122, 1.000000000000000000, 0.9659258262890683122, 1.000000000000000000, 0.9659258262890683122, 1.000000000000000000, 0.9659258262890683122, 1.000000000000000000, 0.9659258262890683122, 1.000000000000000000, 0.9659258262890683122, 1.000000000000000000, 0.9659258262890683122, 1.000000000000000000, 0.9659258262890683122, 1.000000000000000000, 0.9659258262890683122, 1.000000000000000000, 0.9659258262890683122, 1.000000000000000000, 0.9659258262890683122, 1.000000000000000000, 0.9659258262890683122, 1.000000000000000000, 0.9659258262890683122, 1.000000000000000000, 0.9659258262890683122, 1.000000000000000000, 0.9659258262890683122, 1.000000000000000000, 0.9659258262890683122, 1.000000000000000000, 0.9659258262890683122, 1.000000000000000000, 0.9659258262890683122, 1.000000000000000000, 0.9659258262890683122, 1.000000000000000000, 0.9659258262890683122, 1.000000000000000000, 0.9659258262890683122, 1.000000000000000000, 0.9659258262890683122, 1.000000000000000000, 0.9659258262890683122, 1.000000000000000000, 0.9659258262890683122, 1.000000000000000000, 0.9659258262890683122, 1.000000000000000000, 0.9659258262890683122, 1.000000000000000000, 0.9659258262890683122, 1.000000000000000000, 0.9659258262890683122, 1.000000000000000000, 0.9659258262890683122, 1.000000000000000000, 0.9659258262890683122, 1.000000000000000000, 0.9659258262890683122, 1.000000000000000000, 0.9659258262890683122, 1.000000000000000000, 0.9659258262890683122, 1.000000000000000000, 0.9659258262890683122, 1.000000000000000000, 0.9659258262890683122, 1.000000000000000000, 0.9659258262890683122, 1.000000000000000000, 0.9659258262890683122, 1.000000000000000000, 0.9659258262890683122, 1.000000000000000000, 0.9659258262890683122, 1.000000000000000000, 0.9659258262890683122, 1.000000000000000000, 0.9659258262890683122, 1.000000000000000000, 0.9659258262890683122, 1.000000000000000000, 0.9659258262890683122, 1.000000000000000000, 0.9659258262890683122, 1.000000000000000000, 0.9659258262890683122, 1.000000000000000000, 0.9659258262890683122, 1.000000000000000000, 0.9659258262890683122, 1.000000000000000000, 0.9659258262890683122, 1.000000000000000000, 0.9659258262890683122, 1.000000000000000000, 0.9659258262890683122, 1.000000000000000000, 0.9659258262890683122, 1.000000000000000000, 0.9659258262890683122, 1.000000000000000000, 0.9659258262890683122, 1.000000000000000000, 0.9659258262890683122, 1.000000000000000000, 0.9659258262890683122, 1.000000000000000000, 0.9659258262890683122, 1.000000000000000000, 0.9659258262890683122, 1.000000000000000000, 0.9659258262890683122, 1.000000000000000000, 0.9659258262890683122, 1.000000000000000000, 0.9659258262890683122, 1.000000000000000000, 0.9659258262890683122, 1.000000000000000000, 0.9659258262890683122, 1.000000000000000000, 0.9659258262890683122, 1.000000000000000000, 0.9659258262890683122, 1.000000000000000000, 0.9659258262890683122, 1.000000000000000000, 0.9659258262890683122, 1.000000000000000000, 0.9659258262890683122, 1.000000000000000000, 0.9659258262890683122, 1.000000000000000000, 0.9659258262890683122, 1.000000000000000000, 0.9659258262890683122, 1.000000000000000000, 0.9659258262890683122, 1.000000000000000000, 0.9659258262890683122, 1.000000000000000000, 0.9659258262890683122, 1.000000000000000000, 0.9659258262890683122, 1.000000000000000000, 0.9659258262890683122, 1.000000000000000000, 0.9659258262890683122, 1.000000000000000000, 0.9659258262890683122, 1.000000000000000000, 0.9659258262890683122, 1.000000000000000000, 0.9659258262890683122, 1.000000000000000000, 0.9659258262890683122, 1.000000000000000000, 0.9659258262890683122, 1.000000000000000000, 0.9659258262890683122, 1.000000000000000000, 0.9659258262890683122, 1.000000000000000000, 0.9659258262890683122, 1.000000000000000000, 0.9659258262890683122, 1.000000000000000000, 0.9659258262890683122, 1.000000000000000000, 0.9659258262890683122, 1.000000000000000000, 0.9659258262890683122, 1.000000000000000000, 0.9659258262890683122, 1.000000000000000000, 0.9659258262890683122, 1.000000000000000000, 0.9659258262890683122, 1.000000000000000000, 0.9659258262890683122, 1.000000000000000000, 0.9659258262890683122, 1.000000000000000000, 0.9659258262890683122, 1.000000000000000000, 0.9659258262890683122, 1.000000000000000000, 0.9659258262890683122, 1.000000000000000000, 0.9659258262890683122, 1.000000000000000000, 0.9659258262890683122, 1.000000000000000000, 0.9659258262890683122, 1.000000000000000000, 0.9659258262890683122, 1.000000000000000000, 0.9659258262890683122, 1.000000000000000000, 0.9659258262890683122, 1.000000000000000000, 0.9659258262890683122, 1.000000000000000000, 0.9659258262890683122, 1.000000000000000000, 0.9659258262890683122, 1.000000000000000000, 0.9659258262890683122, 1.000000000000000000, 0.9659258262890683122, 1.000000000000000000, 0.9659258262890683122, 1.000000000000000000, 0.9659258262890683122, 1.000000000000000000, 0.9659258262890683122, 1.000000000000000000, 0.9659258262890683122, 1.000000000000000000, 0.9659258262890683122, 1.000000000000000000, 0.9659258262890683122, 1.000000000000000000, 0.9659258262890683122, 1.000000000000000000, 0.9659258262890683122, 1.000000000000000000, 0.9659258262890683122, 1.000000000000000000, 0.9659258262890683122, 1.000000000000000000, 0.9659258262890683122, 1.000000000000000000, 0.9659258262890683122, 1.000000000000000000, 0.9659258262890683122, 1.000000000000000000, 0.9659258262890683122, 1.000000000000000000, 0.9659258262890683122, 1.000000000000000000, 0.9659258262890683122, 1.000000000000000000, 0.9659258262890683122, 1.000000000000000000, 0.9659258262890683122, 1.000000000000000000, 0.9659258262890683122, 1.000000000000000000, 0.9659258262890683122, 1.000000000000000000, 0.9659258262890683122, 1.000000000000000000, 0.9659258262890683122, 1.000000000000000000, 0.9659258262890683122, 1.000000000000000000, 0.9659258262890683122, 1.000000000000000000, 0.9659258262890683122, 1.000000000000000000, 0.9659258262890683122, 1.000000000000000000, 0.9659258262890683122, 1.000000000000000000, 0.9659258262890683122, 1.000000000000000000, 0.9659258262890683122, 1.000000000000000000, 0.9659258262890683122, 1.000000000000000000, 0.9659258262890683122, 1.000000000000000000, 0.9659258262890683122, 1.000000000000000000, 0.9659258262890683122, 1.000000000000000000, 0.9659258262890683122, 1.000000000000000000, 0.9659258262890683122, 1.000000000000000000, 0.9659258262890683122, 1.000000000000000000, 0.9659258262890683122, 1.000000000000000000, 0.9659258262890683122, 1.000000000000000000, 0.9659258262890683122, 1.000000000000000000, 0.9659258262890683122, 1.000000000000000000, 0.9659258262890683122, 1.000000000000000000, 0.9659258262890683122, 1.000000000000000000, 0.9659258262890683122, 1.000000000000000000, 0.9659258262890683122, 1.000000000000000000, 0.9659258262890683122, 1.000000000000000000, 0.9659258262890683122, 1.000000000000000000, 0.9659258262890683122, 1.000000000000000000, 0.9659258262890683122, 1.000000000000000000, 0.9659258262890683122, 1.000000000000000000, 0.9659258262890683122, 1.000000000000000000, 0.9659258262890683122, 1.000000000000000000, 0.9659258262890683122, 1.000000000000000000, 0.9659258262890683122, 1.000000000000000000, 0.9659258262890683122, 1.000000000000000000, 0.9659258262890683122, 1.000000000000000000, 0.9659258262890683122, 1.000000000000000000, 0.9659258262890683122, 1.000000000000000000, 0.9659258262890683122, 1.000000000000000000, 0.9659258262890683122, 1.000000000000000000, 0.9659258262890683122, 1.000000000000000000, 0.9659258262890683122, 1.000000000000000000, 0.9659258262890683122, 1.000000000000000000, 0.9659258262890683122, 1.000000000000000000, 0.9659258262890683122, 1.000000000000000000, 0.9659258262890683122, 1.000000000000000000, 0.9659258262890683122, 1.000000000000000000, 0.9659258262890683122, 1.000000000000000000, 0.9659258262890683122, 1.000000000000000000, 0.9659258262890683122, 1.000000000000000000, 0.9659258262890683122, 1.000000000000000000, 0.9659258262890683122, 1.000000000000000000, 0.9659258262890683122, 1.000000000000000000, 0.9659258262890683122, 1.000000000000000000, 0.9659258262890683122, 1.000000000000000000, 0.9659258262890683122, 1.000000000000000000, 0.9659258262890683122, 1.000000000000000000, 0.9659258262890683122, 1.000000000000000000, 0.9659258262890683122, 1.000000000000000000, 0.9659258262890683122, 1.000000000000000000, 0.9659258262890683122, 1.000000000000000000, 0.9659258262890683122, 1.000000000000000000, 0.9659258262890683122, 1.000000000000000000, 0.9659258262890683122, 1.000000000000000000, 0.9659258262890683122, 1.000000000000000000, 0.9659258262890683122, 1.000000000000000000, 0.9659258262890683122, 1.000000000000000000, 0.9659258262890683122, 1.000000000000000000, 0.9659258262890683122, 1.000000000000000000, 0.9659258262890683122, 1.000000000000000000, 0.9659258262890683122, 1.000000000000000000),
 ( 0.3333333333333333703, 0.3219752754296894559, 0.3333333333333333703, 0.3219752754296894559, 0.3333333333333333703, 0.3219752754296894559, 0.3333333333333333703, 0.3219752754296894559, 0.3333333333333333703, 0.3219752754296894559, 0.3333333333333333703, 0.3219752754296894559, 0.3333333333333333703, 0.3219752754296894559, 0.3333333333333333703, 0.3219752754296894559, 0.3333333333333333703, 0.3219752754296894559, 0.3333333333333333703, 0.3219752754296894559, 0.3333333333333333703, 0.3219752754296894559, 0.3333333333333333703, 0.3219752754296894559, 0.3333333333333333703, 0.3219752754296894559, 0.3333333333333333703, 0.3219752754296894559, 0.3333333333333333703, 0.3219752754296894559, 0.3333333333333333703, 0.3219752754296894559, 0.3333333333333333703, 0.3219752754296894559, 0.3333333333333333703, 0.3219752754296894559, 0.3333333333333333703, 0.3219752754296894559, 0.3333333333333333703, 0.3219752754296894559, 0.3333333333333333703, 0.3219752754296894559, 0.3333333333333333703, 0.3219752754296894559, 0.3333333333333333703, 0.3219752754296894559, 0.3333333333333333703, 0.3219752754296894559, 0.3333333333333333703, 0.3219752754296894559, 0.3333333333333333703, 0.3219752754296894559, 0.3333333333333333703, 0.3219752754296894559, 0.3333333333333333703, 0.3219752754296894559, 0.3333333333333333703, 0.3219752754296894559, 0.3333333333333333703, 0.3219752754296894559, 0.3333333333333333703, 0.3219752754296894559, 0.3333333333333333703, 0.3219752754296894559, 0.3333333333333333703, 0.3219752754296894559, 0.3333333333333333703, 0.3219752754296894559, 0.3333333333333333703, 0.3219752754296894559, 0.3333333333333333703, 0.3219752754296894559, 0.3333333333333333703, 0.3219752754296894559, 0.3333333333333333703, 0.3219752754296894559, 0.3333333333333333703, 0.3219752754296894559, 0.3333333333333333703, 0.3219752754296894559, 0.3333333333333333703, 0.3219752754296894559, 0.3333333333333333703, 0.3219752754296894559, 0.3333333333333333703, 0.3219752754296894559, 0.3333333333333333703, 0.3219752754296894559, 0.3333333333333333703, 0.3219752754296894559, 0.3333333333333333703, 0.3219752754296894559, 0.3333333333333333703, 0.3219752754296894559, 0.3333333333333333703, 0.3219752754296894559, 0.3333333333333333703, 0.3219752754296894559, 0.3333333333333333703, 0.3219752754296894559, 0.3333333333333333703, 0.3219752754296894559, 0.3333333333333333703, 0.3219752754296894559, 0.3333333333333333703, 0.3219752754296894559, 0.3333333333333333703, 0.3219752754296894559, 0.3333333333333333703, 0.3219752754296894559, 0.3333333333333333703, 0.3219752754296894559, 0.3333333333333333703, 0.3219752754296894559, 0.3333333333333333703, 0.3219752754296894559, 0.3333333333333333703, 0.3219752754296894559, 0.3333333333333333703, 0.3219752754296894559, 0.3333333333333333703, 0.3219752754296894559, 0.3333333333333333703, 0.3219752754296894559, 0.3333333333333333703, 0.3219752754296894559, 0.3333333333333333703, 0.3219752754296894559, 0.3333333333333333703, 0.3219752754296894559, 0.3333333333333333703, 0.3219752754296894559, 0.3333333333333333703, 0.3219752754296894559, 0.3333333333333333703, 0.3219752754296894559, 0.3333333333333333703, 0.3219752754296894559, 0.3333333333333333703, 0.3219752754296894559, 0.3333333333333333703, 0.3219752754296894559, 0.3333333333333333703, 0.3219752754296894559, 0.3333333333333333703, 0.3219752754296894559, 0.3333333333333333703, 0.3219752754296894559, 0.3333333333333333703, 0.3219752754296894559, 0.3333333333333333703, 0.3219752754296894559, 0.3333333333333333703, 0.3219752754296894559, 0.3333333333333333703, 0.3219752754296894559, 0.3333333333333333703, 0.3219752754296894559, 0.3333333333333333703, 0.3219752754296894559, 0.3333333333333333703, 0.3219752754296894559, 0.3333333333333333703, 0.3219752754296894559, 0.3333333333333333703, 0.3219752754296894559, 0.3333333333333333703, 0.3219752754296894559, 0.3333333333333333703, 0.3219752754296894559, 0.3333333333333333703, 0.3219752754296894559, 0.3333333333333333703, 0.3219752754296894559, 0.3333333333333333703, 0.3219752754296894559, 0.3333333333333333703, 0.3219752754296894559, 0.3333333333333333703, 0.3219752754296894559, 0.3333333333333333703, 0.3219752754296894559, 0.3333333333333333703, 0.3219752754296894559, 0.3333333333333333703, 0.3219752754296894559, 0.3333333333333333703, 0.3219752754296894559, 0.3333333333333333703, 0.3219752754296894559, 0.3333333333333333703, 0.3219752754296894559, 0.3333333333333333703, 0.3219752754296894559, 0.3333333333333333703, 0.3219752754296894559, 0.3333333333333333703, 0.3219752754296894559, 0.3333333333333333703, 0.3219752754296894559, 0.3333333333333333703, 0.3219752754296894559, 0.3333333333333333703, 0.3219752754296894559, 0.3333333333333333703, 0.3219752754296894559, 0.3333333333333333703, 0.3219752754296894559, 0.3333333333333333703, 0.3219752754296894559, 0.3333333333333333703, 0.3219752754296894559, 0.3333333333333333703, 0.3219752754296894559, 0.3333333333333333703, 0.3219752754296894559, 0.3333333333333333703, 0.3219752754296894559, 0.3333333333333333703, 0.3219752754296894559, 0.3333333333333333703, 0.3219752754296894559, 0.3333333333333333703, 0.3219752754296894559, 0.3333333333333333703, 0.3219752754296894559, 0.3333333333333333703, 0.3219752754296894559, 0.3333333333333333703, 0.3219752754296894559, 0.3333333333333333703, 0.3219752754296894559, 0.3333333333333333703, 0.3219752754296894559, 0.3333333333333333703, 0.3219752754296894559, 0.3333333333333333703, 0.3219752754296894559, 0.3333333333333333703, 0.3219752754296894559, 0.3333333333333333703, 0.3219752754296894559, 0.3333333333333333703, 0.3219752754296894559, 0.3333333333333333703, 0.3219752754296894559, 0.3333333333333333703, 0.3219752754296894559, 0.3333333333333333703, 0.3219752754296894559, 0.3333333333333333703, 0.3219752754296894559, 0.3333333333333333703, 0.3219752754296894559, 0.3333333333333333703, 0.3219752754296894559, 0.3333333333333333703, 0.3219752754296894559, 0.3333333333333333703, 0.3219752754296894559, 0.3333333333333333703, 0.3219752754296894559, 0.3333333333333333703, 0.3219752754296894559, 0.3333333333333333703, 0.3219752754296894559, 0.3333333333333333703, 0.3219752754296894559, 0.3333333333333333703, 0.3219752754296894559, 0.3333333333333333703, 0.3219752754296894559, 0.3333333333333333703, 0.3219752754296894559, 0.3333333333333333703, 0.3219752754296894559, 0.3333333333333333703, 0.3219752754296894559, 0.3333333333333333703, 0.3219752754296894559, 0.3333333333333333703, 0.3219752754296894559, 0.3333333333333333703, 0.3219752754296894559, 0.3333333333333333703, 0.3219752754296894559, 0.3333333333333333703, 0.3219752754296894559, 0.3333333333333333703, 0.3219752754296894559, 0.3333333333333333703, 0.3219752754296894559, 0.3333333333333333703, 0.3219752754296894559, 0.3333333333333333703, 0.3219752754296894559, 0.3333333333333333703, 0.3219752754296894559, 0.3333333333333333703, 0.3219752754296894559, 0.3333333333333333703, 0.3219752754296894559, 0.3333333333333333703, 0.3219752754296894559, 0.3333333333333333703, 0.3219752754296894559, 0.3333333333333333703, 0.3219752754296894559, 0.3333333333333333703, 0.3219752754296894559, 0.3333333333333333703, 0.3219752754296894559, 0.3333333333333333703, 0.3219752754296894559, 0.3333333333333333703, 0.3219752754296894559, 0.3333333333333333703, 0.3219752754296894559, 0.3333333333333333703, 0.3219752754296894559, 0.3333333333333333703, 0.3219752754296894559, 0.3333333333333333703, 0.3219752754296894559, 0.3333333333333333703, 0.3219752754296894559, 0.3333333333333333703, 0.3219752754296894559, 0.3333333333333333703, 0.3219752754296894559, 0.3333333333333333703, 0.3219752754296894559, 0.3333333333333333703, 0.3219752754296894559, 0.3333333333333333703, 0.3219752754296894559, 0.3333333333333333703, 0.3219752754296894559, 0.3333333333333333703, 0.3219752754296894559, 0.3333333333333333703, 0.3219752754296894559, 0.3333333333333333703, 0.3219752754296894559, 0.3333333333333333703, 0.3219752754296894559, 0.3333333333333333703, 0.3219752754296894559, 0.3333333333333333703, 0.3219752754296894559, 0.3333333333333333703, 0.3219752754296894559, 0.3333333333333333703, 0.3219752754296894559, 0.3333333333333333703, 0.3219752754296894559, 0.3333333333333333703, 0.3219752754296894559, 0.3333333333333333703, 0.3219752754296894559, 0.3333333333333333703, 0.3219752754296894559, 0.3333333333333333703, 0.3219752754296894559, 0.3333333333333333703, 0.3219752754296894559, 0.3333333333333333703, 0.3219752754296894559, 0.3333333333333333703, 0.3219752754296894559, 0.3333333333333333703, 0.3219752754296894559, 0.3333333333333333703, 0.3219752754296894559, 0.3333333333333333703, 0.3219752754296894559, 0.3333333333333333703, 0.3219752754296894559, 0.3333333333333333703, 0.3219752754296894559, 0.3333333333333333703, 0.3219752754296894559, 0.3333333333333333703, 0.3219752754296894559, 0.3333333333333333703, 0.3219752754296894559, 0.3333333333333333703, 0.3219752754296894559, 0.3333333333333333703, 0.3219752754296894559, 0.3333333333333333703, 0.3219752754296894559, 0.3333333333333333703, 0.3219752754296894559, 0.3333333333333333703, 0.3219752754296894559, 0.3333333333333333703, 0.3219752754296894559, 0.3333333333333333703, 0.3219752754296894559, 0.3333333333333333703, 0.3219752754296894559, 0.3333333333333333703, 0.3219752754296894559, 0.3333333333333333703, 0.3219752754296894559, 0.3333333333333333703, 0.3219752754296894559, 0.3333333333333333703, 0.3219752754296894559, 0.3333333333333333703, 0.3219752754296894559, 0.3333333333333333703, 0.3219752754296894559, 0.3333333333333333703, 0.3219752754296894559, 0.3333333333333333703, 0.3219752754296894559, 0.3333333333333333703, 0.3219752754296894559, 0.3333333333333333703, 0.3219752754296894559, 0.3333333333333333703, 0.3219752754296894559, 0.3333333333333333703, 0.3219752754296894559, 0.3333333333333333703, 0.3219752754296894559, 0.3333333333333333703, 0.3219752754296894559, 0.3333333333333333703, 0.3219752754296894559, 0.3333333333333333703, 0.3219752754296894559, 0.3333333333333333703, 0.3219752754296894559, 0.3333333333333333703, 0.3219752754296894559, 0.3333333333333333703, 0.3219752754296894559, 0.3333333333333333703, 0.3219752754296894559, 0.3333333333333333703, 0.3219752754296894559, 0.3333333333333333703, 0.3219752754296894559, 0.3333333333333333703, 0.3219752754296894559, 0.3333333333333333703, 0.3219752754296894559, 0.3333333333333333703, 0.3219752754296894559, 0.3333333333333333703, 0.3219752754296894559, 0.3333333333333333703, 0.3219752754296894559, 0.3333333333333333703),
 ( 0.3333333333333333703, 0.3219752754296894559, 0.3333333333333333703, 0.3219752754296894559, 0.3333333333333333703, 0.3219752754296894559, 0.3333333333333333703, 0.3219752754296894559, 0.3333333333333333703, 0.3219752754296894559, 0.3333333333333333703, 0.3219752754296894559, 0.3333333333333333703, 0.3219752754296894559, 0.3333333333333333703, 0.3219752754296894559, 0.3333333333333333703, 0.3219752754296894559, 0.3333333333333333703, 0.3219752754296894559, 0.3333333333333333703, 0.3219752754296894559, 0.3333333333333333703, 0.3219752754296894559, 0.3333333333333333703, 0.3219752754296894559, 0.3333333333333333703, 0.3219752754296894559, 0.3333333333333333703, 0.3219752754296894559, 0.3333333333333333703, 0.3219752754296894559, 0.3333333333333333703, 0.3219752754296894559, 0.3333333333333333703, 0.3219752754296894559, 0.3333333333333333703, 0.3219752754296894559, 0.3333333333333333703, 0.3219752754296894559, 0.3333333333333333703, 0.3219752754296894559, 0.3333333333333333703, 0.3219752754296894559, 0.3333333333333333703, 0.3219752754296894559, 0.3333333333333333703, 0.3219752754296894559, 0.3333333333333333703, 0.3219752754296894559, 0.3333333333333333703, 0.3219752754296894559, 0.3333333333333333703, 0.3219752754296894559, 0.3333333333333333703, 0.3219752754296894559, 0.3333333333333333703, 0.3219752754296894559, 0.3333333333333333703, 0.3219752754296894559, 0.3333333333333333703, 0.3219752754296894559, 0.3333333333333333703, 0.3219752754296894559, 0.3333333333333333703, 0.3219752754296894559, 0.3333333333333333703, 0.3219752754296894559, 0.3333333333333333703, 0.3219752754296894559, 0.3333333333333333703, 0.3219752754296894559, 0.3333333333333333703, 0.3219752754296894559, 0.3333333333333333703, 0.3219752754296894559, 0.3333333333333333703, 0.3219752754296894559, 0.3333333333333333703, 0.3219752754296894559, 0.3333333333333333703, 0.3219752754296894559, 0.3333333333333333703, 0.3219752754296894559, 0.3333333333333333703, 0.3219752754296894559, 0.3333333333333333703, 0.3219752754296894559, 0.3333333333333333703, 0.3219752754296894559, 0.3333333333333333703, 0.3219752754296894559, 0.3333333333333333703, 0.3219752754296894559, 0.3333333333333333703, 0.3219752754296894559, 0.3333333333333333703, 0.3219752754296894559, 0.3333333333333333703, 0.3219752754296894559, 0.3333333333333333703, 0.3219752754296894559, 0.3333333333333333703, 0.3219752754296894559, 0.3333333333333333703, 0.3219752754296894559, 0.3333333333333333703, 0.3219752754296894559, 0.3333333333333333703, 0.3219752754296894559, 0.3333333333333333703, 0.3219752754296894559, 0.3333333333333333703, 0.3219752754296894559, 0.3333333333333333703, 0.3219752754296894559, 0.3333333333333333703, 0.3219752754296894559, 0.3333333333333333703, 0.3219752754296894559, 0.3333333333333333703, 0.3219752754296894559, 0.3333333333333333703, 0.3219752754296894559, 0.3333333333333333703, 0.3219752754296894559, 0.3333333333333333703, 0.3219752754296894559, 0.3333333333333333703, 0.3219752754296894559, 0.3333333333333333703, 0.3219752754296894559, 0.3333333333333333703, 0.3219752754296894559, 0.3333333333333333703, 0.3219752754296894559, 0.3333333333333333703, 0.3219752754296894559, 0.3333333333333333703, 0.3219752754296894559, 0.3333333333333333703, 0.3219752754296894559, 0.3333333333333333703, 0.3219752754296894559, 0.3333333333333333703, 0.3219752754296894559, 0.3333333333333333703, 0.3219752754296894559, 0.3333333333333333703, 0.3219752754296894559, 0.3333333333333333703, 0.3219752754296894559, 0.3333333333333333703, 0.3219752754296894559, 0.3333333333333333703, 0.3219752754296894559, 0.3333333333333333703, 0.3219752754296894559, 0.3333333333333333703, 0.3219752754296894559, 0.3333333333333333703, 0.3219752754296894559, 0.3333333333333333703, 0.3219752754296894559, 0.3333333333333333703, 0.3219752754296894559, 0.3333333333333333703, 0.3219752754296894559, 0.3333333333333333703, 0.3219752754296894559, 0.3333333333333333703, 0.3219752754296894559, 0.3333333333333333703, 0.3219752754296894559, 0.3333333333333333703, 0.3219752754296894559, 0.3333333333333333703, 0.3219752754296894559, 0.3333333333333333703, 0.3219752754296894559, 0.3333333333333333703, 0.3219752754296894559, 0.3333333333333333703, 0.3219752754296894559, 0.3333333333333333703, 0.3219752754296894559, 0.3333333333333333703, 0.3219752754296894559, 0.3333333333333333703, 0.3219752754296894559, 0.3333333333333333703, 0.3219752754296894559, 0.3333333333333333703, 0.3219752754296894559, 0.3333333333333333703, 0.3219752754296894559, 0.3333333333333333703, 0.3219752754296894559, 0.3333333333333333703, 0.3219752754296894559, 0.3333333333333333703, 0.3219752754296894559, 0.3333333333333333703, 0.3219752754296894559, 0.3333333333333333703, 0.3219752754296894559, 0.3333333333333333703, 0.3219752754296894559, 0.3333333333333333703, 0.3219752754296894559, 0.3333333333333333703, 0.3219752754296894559, 0.3333333333333333703, 0.3219752754296894559, 0.3333333333333333703, 0.3219752754296894559, 0.3333333333333333703, 0.3219752754296894559, 0.3333333333333333703, 0.3219752754296894559, 0.3333333333333333703, 0.3219752754296894559, 0.3333333333333333703, 0.3219752754296894559, 0.3333333333333333703, 0.3219752754296894559, 0.3333333333333333703, 0.3219752754296894559, 0.3333333333333333703, 0.3219752754296894559, 0.3333333333333333703, 0.3219752754296894559, 0.3333333333333333703, 0.3219752754296894559, 0.3333333333333333703, 0.3219752754296894559, 0.3333333333333333703, 0.3219752754296894559, 0.3333333333333333703, 0.3219752754296894559, 0.3333333333333333703, 0.3219752754296894559, 0.3333333333333333703, 0.3219752754296894559, 0.3333333333333333703, 0.3219752754296894559, 0.3333333333333333703, 0.3219752754296894559, 0.3333333333333333703, 0.3219752754296894559, 0.3333333333333333703, 0.3219752754296894559, 0.3333333333333333703, 0.3219752754296894559, 0.3333333333333333703, 0.3219752754296894559, 0.3333333333333333703, 0.3219752754296894559, 0.3333333333333333703, 0.3219752754296894559, 0.3333333333333333703, 0.3219752754296894559, 0.3333333333333333703, 0.3219752754296894559, 0.3333333333333333703, 0.3219752754296894559, 0.3333333333333333703, 0.3219752754296894559, 0.3333333333333333703, 0.3219752754296894559, 0.3333333333333333703, 0.3219752754296894559, 0.3333333333333333703, 0.3219752754296894559, 0.3333333333333333703, 0.3219752754296894559, 0.3333333333333333703, 0.3219752754296894559, 0.3333333333333333703, 0.3219752754296894559, 0.3333333333333333703, 0.3219752754296894559, 0.3333333333333333703, 0.3219752754296894559, 0.3333333333333333703, 0.3219752754296894559, 0.3333333333333333703, 0.3219752754296894559, 0.3333333333333333703, 0.3219752754296894559, 0.3333333333333333703, 0.3219752754296894559, 0.3333333333333333703, 0.3219752754296894559, 0.3333333333333333703, 0.3219752754296894559, 0.3333333333333333703, 0.3219752754296894559, 0.3333333333333333703, 0.3219752754296894559, 0.3333333333333333703, 0.3219752754296894559, 0.3333333333333333703, 0.3219752754296894559, 0.3333333333333333703, 0.3219752754296894559, 0.3333333333333333703, 0.3219752754296894559, 0.3333333333333333703, 0.3219752754296894559, 0.3333333333333333703, 0.3219752754296894559, 0.3333333333333333703, 0.3219752754296894559, 0.3333333333333333703, 0.3219752754296894559, 0.3333333333333333703, 0.3219752754296894559, 0.3333333333333333703, 0.3219752754296894559, 0.3333333333333333703, 0.3219752754296894559, 0.3333333333333333703, 0.3219752754296894559, 0.3333333333333333703, 0.3219752754296894559, 0.3333333333333333703, 0.3219752754296894559, 0.3333333333333333703, 0.3219752754296894559, 0.3333333333333333703, 0.3219752754296894559, 0.3333333333333333703, 0.3219752754296894559, 0.3333333333333333703, 0.3219752754296894559, 0.3333333333333333703, 0.3219752754296894559, 0.3333333333333333703, 0.3219752754296894559, 0.3333333333333333703, 0.3219752754296894559, 0.3333333333333333703, 0.3219752754296894559, 0.3333333333333333703, 0.3219752754296894559, 0.3333333333333333703, 0.3219752754296894559, 0.3333333333333333703, 0.3219752754296894559, 0.3333333333333333703, 0.3219752754296894559, 0.3333333333333333703, 0.3219752754296894559, 0.3333333333333333703, 0.3219752754296894559, 0.3333333333333333703, 0.3219752754296894559, 0.3333333333333333703, 0.3219752754296894559, 0.3333333333333333703, 0.3219752754296894559, 0.3333333333333333703, 0.3219752754296894559, 0.3333333333333333703, 0.3219752754296894559, 0.3333333333333333703, 0.3219752754296894559, 0.3333333333333333703, 0.3219752754296894559, 0.3333333333333333703, 0.3219752754296894559, 0.3333333333333333703, 0.3219752754296894559, 0.3333333333333333703, 0.3219752754296894559, 0.3333333333333333703, 0.3219752754296894559, 0.3333333333333333703, 0.3219752754296894559, 0.3333333333333333703, 0.3219752754296894559, 0.3333333333333333703, 0.3219752754296894559, 0.3333333333333333703, 0.3219752754296894559, 0.3333333333333333703, 0.3219752754296894559, 0.3333333333333333703, 0.3219752754296894559, 0.3333333333333333703, 0.3219752754296894559, 0.3333333333333333703, 0.3219752754296894559, 0.3333333333333333703, 0.3219752754296894559, 0.3333333333333333703, 0.3219752754296894559, 0.3333333333333333703, 0.3219752754296894559, 0.3333333333333333703, 0.3219752754296894559, 0.3333333333333333703, 0.3219752754296894559, 0.3333333333333333703, 0.3219752754296894559, 0.3333333333333333703, 0.3219752754296894559, 0.3333333333333333703, 0.3219752754296894559, 0.3333333333333333703, 0.3219752754296894559, 0.3333333333333333703, 0.3219752754296894559, 0.3333333333333333703, 0.3219752754296894559, 0.3333333333333333703, 0.3219752754296894559, 0.3333333333333333703, 0.3219752754296894559, 0.3333333333333333703, 0.3219752754296894559, 0.3333333333333333703, 0.3219752754296894559, 0.3333333333333333703, 0.3219752754296894559, 0.3333333333333333703, 0.3219752754296894559, 0.3333333333333333703, 0.3219752754296894559, 0.3333333333333333703, 0.3219752754296894559, 0.3333333333333333703, 0.3219752754296894559, 0.3333333333333333703, 0.3219752754296894559, 0.3333333333333333703, 0.3219752754296894559, 0.3333333333333333703, 0.3219752754296894559, 0.3333333333333333703, 0.3219752754296894559, 0.3333333333333333703, 0.3219752754296894559, 0.3333333333333333703, 0.3219752754296894559, 0.3333333333333333703, 0.3219752754296894559, 0.3333333333333333703, 0.3219752754296894559, 0.3333333333333333703, 0.3219752754296894559, 0.3333333333333333703, 0.3219752754296894559, 0.3333333333333333703, 0.3219752754296894559, 0.3333333333333333703),
 ( 1.000000000000000000, 0.9659258262890683122, 1.000000000000000000, 0.9659258262890683122, 1.000000000000000000, 0.9659258262890683122, 1.000000000000000000, 0.9659258262890683122, 1.000000000000000000, 0.9659258262890683122, 1.000000000000000000, 0.9659258262890683122, 1.000000000000000000, 0.9659258262890683122, 1.000000000000000000, 0.9659258262890683122, 1.000000000000000000, 0.9659258262890683122, 1.000000000000000000, 0.9659258262890683122, 1.000000000000000000, 0.9659258262890683122, 1.000000000000000000, 0.9659258262890683122, 1.000000000000000000, 0.9659258262890683122, 1.000000000000000000, 0.9659258262890683122, 1.000000000000000000, 0.9659258262890683122, 1.000000000000000000, 0.9659258262890683122, 1.000000000000000000, 0.9659258262890683122, 1.000000000000000000, 0.9659258262890683122, 1.000000000000000000, 0.9659258262890683122, 1.000000000000000000, 0.9659258262890683122, 1.000000000000000000, 0.9659258262890683122, 1.000000000000000000, 0.9659258262890683122, 1.000000000000000000, 0.9659258262890683122, 1.000000000000000000, 0.9659258262890683122, 1.000000000000000000, 0.9659258262890683122, 1.000000000000000000, 0.9659258262890683122, 1.000000000000000000, 0.9659258262890683122, 1.000000000000000000, 0.9659258262890683122, 1.000000000000000000, 0.9659258262890683122, 1.000000000000000000, 0.9659258262890683122, 1.000000000000000000, 0.9659258262890683122, 1.000000000000000000, 0.9659258262890683122, 1.000000000000000000, 0.9659258262890683122, 1.000000000000000000, 0.9659258262890683122, 1.000000000000000000, 0.9659258262890683122, 1.000000000000000000, 0.9659258262890683122, 1.000000000000000000, 0.9659258262890683122, 1.000000000000000000, 0.9659258262890683122, 1.000000000000000000, 0.9659258262890683122, 1.000000000000000000, 0.9659258262890683122, 1.000000000000000000, 0.9659258262890683122, 1.000000000000000000, 0.9659258262890683122, 1.000000000000000000, 0.9659258262890683122, 1.000000000000000000, 0.9659258262890683122, 1.000000000000000000, 0.9659258262890683122, 1.000000000000000000, 0.9659258262890683122, 1.000000000000000000, 0.9659258262890683122, 1.000000000000000000, 0.9659258262890683122, 1.000000000000000000, 0.9659258262890683122, 1.000000000000000000, 0.9659258262890683122, 1.000000000000000000, 0.9659258262890683122, 1.000000000000000000, 0.9659258262890683122, 1.000000000000000000, 0.9659258262890683122, 1.000000000000000000, 0.9659258262890683122, 1.000000000000000000, 0.9659258262890683122, 1.000000000000000000, 0.9659258262890683122, 1.000000000000000000, 0.9659258262890683122, 1.000000000000000000, 0.9659258262890683122, 1.000000000000000000, 0.9659258262890683122, 1.000000000000000000, 0.9659258262890683122, 1.000000000000000000, 0.9659258262890683122, 1.000000000000000000, 0.9659258262890683122, 1.000000000000000000, 0.9659258262890683122, 1.000000000000000000, 0.9659258262890683122, 1.000000000000000000, 0.9659258262890683122, 1.000000000000000000, 0.9659258262890683122, 1.000000000000000000, 0.9659258262890683122, 1.000000000000000000, 0.9659258262890683122, 1.000000000000000000, 0.9659258262890683122, 1.000000000000000000, 0.9659258262890683122, 1.000000000000000000, 0.9659258262890683122, 1.000000000000000000, 0.9659258262890683122, 1.000000000000000000, 0.9659258262890683122, 1.000000000000000000, 0.9659258262890683122, 1.000000000000000000, 0.9659258262890683122, 1.000000000000000000, 0.9659258262890683122, 1.000000000000000000, 0.9659258262890683122, 1.000000000000000000, 0.9659258262890683122, 1.000000000000000000, 0.9659258262890683122, 1.000000000000000000, 0.9659258262890683122, 1.000000000000000000, 0.9659258262890683122, 1.000000000000000000, 0.9659258262890683122, 1.000000000000000000, 0.9659258262890683122, 1.000000000000000000, 0.9659258262890683122, 1.000000000000000000, 0.9659258262890683122, 1.000000000000000000, 0.9659258262890683122, 1.000000000000000000, 0.9659258262890683122, 1.000000000000000000, 0.9659258262890683122, 1.000000000000000000, 0.9659258262890683122, 1.000000000000000000, 0.9659258262890683122, 1.000000000000000000, 0.9659258262890683122, 1.000000000000000000, 0.9659258262890683122, 1.000000000000000000, 0.9659258262890683122, 1.000000000000000000, 0.9659258262890683122, 1.000000000000000000, 0.9659258262890683122, 1.000000000000000000, 0.9659258262890683122, 1.000000000000000000, 0.9659258262890683122, 1.000000000000000000, 0.9659258262890683122, 1.000000000000000000, 0.9659258262890683122, 1.000000000000000000, 0.9659258262890683122, 1.000000000000000000, 0.9659258262890683122, 1.000000000000000000, 0.9659258262890683122, 1.000000000000000000, 0.9659258262890683122, 1.000000000000000000, 0.9659258262890683122, 1.000000000000000000, 0.9659258262890683122, 1.000000000000000000, 0.9659258262890683122, 1.000000000000000000, 0.9659258262890683122, 1.000000000000000000, 0.9659258262890683122, 1.000000000000000000, 0.9659258262890683122, 1.000000000000000000, 0.9659258262890683122, 1.000000000000000000, 0.9659258262890683122, 1.000000000000000000, 0.9659258262890683122, 1.000000000000000000, 0.9659258262890683122, 1.000000000000000000, 0.9659258262890683122, 1.000000000000000000, 0.9659258262890683122, 1.000000000000000000, 0.9659258262890683122, 1.000000000000000000, 0.9659258262890683122, 1.000000000000000000, 0.9659258262890683122, 1.000000000000000000, 0.9659258262890683122, 1.000000000000000000, 0.9659258262890683122, 1.000000000000000000, 0.9659258262890683122, 1.000000000000000000, 0.9659258262890683122, 1.000000000000000000, 0.9659258262890683122, 1.000000000000000000, 0.9659258262890683122, 1.000000000000000000, 0.9659258262890683122, 1.000000000000000000, 0.9659258262890683122, 1.000000000000000000, 0.9659258262890683122, 1.000000000000000000, 0.9659258262890683122, 1.000000000000000000, 0.9659258262890683122, 1.000000000000000000, 0.9659258262890683122, 1.000000000000000000, 0.9659258262890683122, 1.000000000000000000, 0.9659258262890683122, 1.000000000000000000, 0.9659258262890683122, 1.000000000000000000, 0.9659258262890683122, 1.000000000000000000, 0.9659258262890683122, 1.000000000000000000, 0.9659258262890683122, 1.000000000000000000, 0.9659258262890683122, 1.000000000000000000, 0.9659258262890683122, 1.000000000000000000, 0.9659258262890683122, 1.000000000000000000, 0.9659258262890683122, 1.000000000000000000, 0.9659258262890683122, 1.000000000000000000, 0.9659258262890683122, 1.000000000000000000, 0.9659258262890683122, 1.000000000000000000, 0.9659258262890683122, 1.000000000000000000, 0.9659258262890683122, 1.000000000000000000, 0.9659258262890683122, 1.000000000000000000, 0.9659258262890683122, 1.000000000000000000, 0.9659258262890683122, 1.000000000000000000, 0.9659258262890683122, 1.000000000000000000, 0.9659258262890683122, 1.000000000000000000, 0.9659258262890683122, 1.000000000000000000, 0.9659258262890683122, 1.000000000000000000, 0.9659258262890683122, 1.000000000000000000, 0.9659258262890683122, 1.000000000000000000, 0.9659258262890683122, 1.000000000000000000, 0.9659258262890683122, 1.000000000000000000, 0.9659258262890683122, 1.000000000000000000, 0.9659258262890683122, 1.000000000000000000, 0.9659258262890683122, 1.000000000000000000, 0.9659258262890683122, 1.000000000000000000, 0.9659258262890683122, 1.000000000000000000, 0.9659258262890683122, 1.000000000000000000, 0.9659258262890683122, 1.000000000000000000, 0.9659258262890683122, 1.000000000000000000, 0.9659258262890683122, 1.000000000000000000, 0.9659258262890683122, 1.000000000000000000, 0.9659258262890683122, 1.000000000000000000, 0.9659258262890683122, 1.000000000000000000, 0.9659258262890683122, 1.000000000000000000, 0.9659258262890683122, 1.000000000000000000, 0.9659258262890683122, 1.000000000000000000, 0.9659258262890683122, 1.000000000000000000, 0.9659258262890683122, 1.000000000000000000, 0.9659258262890683122, 1.000000000000000000, 0.9659258262890683122, 1.000000000000000000, 0.9659258262890683122, 1.000000000000000000, 0.9659258262890683122, 1.000000000000000000, 0.9659258262890683122, 1.000000000000000000, 0.9659258262890683122, 1.000000000000000000, 0.9659258262890683122, 1.000000000000000000, 0.9659258262890683122, 1.000000000000000000, 0.9659258262890683122, 1.000000000000000000, 0.9659258262890683122, 1.000000000000000000, 0.9659258262890683122, 1.000000000000000000, 0.9659258262890683122, 1.000000000000000000, 0.9659258262890683122, 1.000000000000000000, 0.9659258262890683122, 1.000000000000000000, 0.9659258262890683122, 1.000000000000000000, 0.9659258262890683122, 1.000000000000000000, 0.9659258262890683122, 1.000000000000000000, 0.9659258262890683122, 1.000000000000000000, 0.9659258262890683122, 1.000000000000000000, 0.9659258262890683122, 1.000000000000000000, 0.9659258262890683122, 1.000000000000000000, 0.9659258262890683122, 1.000000000000000000, 0.9659258262890683122, 1.000000000000000000, 0.9659258262890683122, 1.000000000000000000, 0.9659258262890683122, 1.000000000000000000, 0.9659258262890683122, 1.000000000000000000, 0.9659258262890683122, 1.000000000000000000, 0.9659258262890683122, 1.000000000000000000, 0.9659258262890683122, 1.000000000000000000, 0.9659258262890683122, 1.000000000000000000, 0.9659258262890683122, 1.000000000000000000, 0.9659258262890683122, 1.000000000000000000, 0.9659258262890683122, 1.000000000000000000, 0.9659258262890683122, 1.000000000000000000, 0.9659258262890683122, 1.000000000000000000, 0.9659258262890683122, 1.000000000000000000, 0.9659258262890683122, 1.000000000000000000, 0.9659258262890683122, 1.000000000000000000, 0.9659258262890683122, 1.000000000000000000, 0.9659258262890683122, 1.000000000000000000, 0.9659258262890683122, 1.000000000000000000, 0.9659258262890683122, 1.000000000000000000, 0.9659258262890683122, 1.000000000000000000, 0.9659258262890683122, 1.000000000000000000, 0.9659258262890683122, 1.000000000000000000, 0.9659258262890683122, 1.000000000000000000, 0.9659258262890683122, 1.000000000000000000, 0.9659258262890683122, 1.000000000000000000, 0.9659258262890683122, 1.000000000000000000, 0.9659258262890683122, 1.000000000000000000, 0.9659258262890683122, 1.000000000000000000, 0.9659258262890683122, 1.000000000000000000, 0.9659258262890683122, 1.000000000000000000, 0.9659258262890683122, 1.000000000000000000, 0.9659258262890683122, 1.000000000000000000),
 ( 0.3333333333333333703, 0.3219752754296894559, 0.3333333333333333703, 0.3219752754296894559, 0.3333333333333333703, 0.3219752754296894559, 0.3333333333333333703, 0.3219752754296894559, 0.3333333333333333703, 0.3219752754296894559, 0.3333333333333333703, 0.3219752754296894559, 0.3333333333333333703, 0.3219752754296894559, 0.3333333333333333703, 0.3219752754296894559, 0.3333333333333333703, 0.3219752754296894559, 0.3333333333333333703, 0.3219752754296894559, 0.3333333333333333703, 0.3219752754296894559, 0.3333333333333333703, 0.3219752754296894559, 0.3333333333333333703, 0.3219752754296894559, 0.3333333333333333703, 0.3219752754296894559, 0.3333333333333333703, 0.3219752754296894559, 0.3333333333333333703, 0.3219752754296894559, 0.3333333333333333703, 0.3219752754296894559, 0.3333333333333333703, 0.3219752754296894559, 0.3333333333333333703, 0.3219752754296894559, 0.3333333333333333703, 0.3219752754296894559, 0.3333333333333333703, 0.3219752754296894559, 0.3333333333333333703, 0.3219752754296894559, 0.3333333333333333703, 0.3219752754296894559, 0.3333333333333333703, 0.3219752754296894559, 0.3333333333333333703, 0.3219752754296894559, 0.3333333333333333703, 0.3219752754296894559, 0.3333333333333333703, 0.3219752754296894559, 0.3333333333333333703, 0.3219752754296894559, 0.3333333333333333703, 0.3219752754296894559, 0.3333333333333333703, 0.3219752754296894559, 0.3333333333333333703, 0.3219752754296894559, 0.3333333333333333703, 0.3219752754296894559, 0.3333333333333333703, 0.3219752754296894559, 0.3333333333333333703, 0.3219752754296894559, 0.3333333333333333703, 0.3219752754296894559, 0.3333333333333333703, 0.3219752754296894559, 0.3333333333333333703, 0.3219752754296894559, 0.3333333333333333703, 0.3219752754296894559, 0.3333333333333333703, 0.3219752754296894559, 0.3333333333333333703, 0.3219752754296894559, 0.3333333333333333703, 0.3219752754296894559, 0.3333333333333333703, 0.3219752754296894559, 0.3333333333333333703, 0.3219752754296894559, 0.3333333333333333703, 0.3219752754296894559, 0.3333333333333333703, 0.3219752754296894559, 0.3333333333333333703, 0.3219752754296894559, 0.3333333333333333703, 0.3219752754296894559, 0.3333333333333333703, 0.3219752754296894559, 0.3333333333333333703, 0.3219752754296894559, 0.3333333333333333703, 0.3219752754296894559, 0.3333333333333333703, 0.3219752754296894559, 0.3333333333333333703, 0.3219752754296894559, 0.3333333333333333703, 0.3219752754296894559, 0.3333333333333333703, 0.3219752754296894559, 0.3333333333333333703, 0.3219752754296894559, 0.3333333333333333703, 0.3219752754296894559, 0.3333333333333333703, 0.3219752754296894559, 0.3333333333333333703, 0.3219752754296894559, 0.3333333333333333703, 0.3219752754296894559, 0.3333333333333333703, 0.3219752754296894559, 0.3333333333333333703, 0.3219752754296894559, 0.3333333333333333703, 0.3219752754296894559, 0.3333333333333333703, 0.3219752754296894559, 0.3333333333333333703, 0.3219752754296894559, 0.3333333333333333703, 0.3219752754296894559, 0.3333333333333333703, 0.3219752754296894559, 0.3333333333333333703, 0.3219752754296894559, 0.3333333333333333703, 0.3219752754296894559, 0.3333333333333333703, 0.3219752754296894559, 0.3333333333333333703, 0.3219752754296894559, 0.3333333333333333703, 0.3219752754296894559, 0.3333333333333333703, 0.3219752754296894559, 0.3333333333333333703, 0.3219752754296894559, 0.3333333333333333703, 0.3219752754296894559, 0.3333333333333333703, 0.3219752754296894559, 0.3333333333333333703, 0.3219752754296894559, 0.3333333333333333703, 0.3219752754296894559, 0.3333333333333333703, 0.3219752754296894559, 0.3333333333333333703, 0.3219752754296894559, 0.3333333333333333703, 0.3219752754296894559, 0.3333333333333333703, 0.3219752754296894559, 0.3333333333333333703, 0.3219752754296894559, 0.3333333333333333703, 0.3219752754296894559, 0.3333333333333333703, 0.3219752754296894559, 0.3333333333333333703, 0.3219752754296894559, 0.3333333333333333703, 0.3219752754296894559, 0.3333333333333333703, 0.3219752754296894559, 0.3333333333333333703, 0.3219752754296894559, 0.3333333333333333703, 0.3219752754296894559, 0.3333333333333333703, 0.3219752754296894559, 0.3333333333333333703, 0.3219752754296894559, 0.3333333333333333703, 0.3219752754296894559, 0.3333333333333333703, 0.3219752754296894559, 0.3333333333333333703, 0.3219752754296894559, 0.3333333333333333703, 0.3219752754296894559, 0.3333333333333333703, 0.3219752754296894559, 0.3333333333333333703, 0.3219752754296894559, 0.3333333333333333703, 0.3219752754296894559, 0.3333333333333333703, 0.3219752754296894559, 0.3333333333333333703, 0.3219752754296894559, 0.3333333333333333703, 0.3219752754296894559, 0.3333333333333333703, 0.3219752754296894559, 0.3333333333333333703, 0.3219752754296894559, 0.3333333333333333703, 0.3219752754296894559, 0.3333333333333333703, 0.3219752754296894559, 0.3333333333333333703, 0.3219752754296894559, 0.3333333333333333703, 0.3219752754296894559, 0.3333333333333333703, 0.3219752754296894559, 0.3333333333333333703, 0.3219752754296894559, 0.3333333333333333703, 0.3219752754296894559, 0.3333333333333333703, 0.3219752754296894559, 0.3333333333333333703, 0.3219752754296894559, 0.3333333333333333703, 0.3219752754296894559, 0.3333333333333333703, 0.3219752754296894559, 0.3333333333333333703, 0.3219752754296894559, 0.3333333333333333703, 0.3219752754296894559, 0.3333333333333333703, 0.3219752754296894559, 0.3333333333333333703, 0.3219752754296894559, 0.3333333333333333703, 0.3219752754296894559, 0.3333333333333333703, 0.3219752754296894559, 0.3333333333333333703, 0.3219752754296894559, 0.3333333333333333703, 0.3219752754296894559, 0.3333333333333333703, 0.3219752754296894559, 0.3333333333333333703, 0.3219752754296894559, 0.3333333333333333703, 0.3219752754296894559, 0.3333333333333333703, 0.3219752754296894559, 0.3333333333333333703, 0.3219752754296894559, 0.3333333333333333703, 0.3219752754296894559, 0.3333333333333333703, 0.3219752754296894559, 0.3333333333333333703, 0.3219752754296894559, 0.3333333333333333703, 0.3219752754296894559, 0.3333333333333333703, 0.3219752754296894559, 0.3333333333333333703, 0.3219752754296894559, 0.3333333333333333703, 0.3219752754296894559, 0.3333333333333333703, 0.3219752754296894559, 0.3333333333333333703, 0.3219752754296894559, 0.3333333333333333703, 0.3219752754296894559, 0.3333333333333333703, 0.3219752754296894559, 0.3333333333333333703, 0.3219752754296894559, 0.3333333333333333703, 0.3219752754296894559, 0.3333333333333333703, 0.3219752754296894559, 0.3333333333333333703, 0.3219752754296894559, 0.3333333333333333703, 0.3219752754296894559, 0.3333333333333333703, 0.3219752754296894559, 0.3333333333333333703, 0.3219752754296894559, 0.3333333333333333703, 0.3219752754296894559, 0.3333333333333333703, 0.3219752754296894559, 0.3333333333333333703, 0.3219752754296894559, 0.3333333333333333703, 0.3219752754296894559, 0.3333333333333333703, 0.3219752754296894559, 0.3333333333333333703, 0.3219752754296894559, 0.3333333333333333703, 0.3219752754296894559, 0.3333333333333333703, 0.3219752754296894559, 0.3333333333333333703, 0.3219752754296894559, 0.3333333333333333703, 0.3219752754296894559, 0.3333333333333333703, 0.3219752754296894559, 0.3333333333333333703, 0.3219752754296894559, 0.3333333333333333703, 0.3219752754296894559, 0.3333333333333333703, 0.3219752754296894559, 0.3333333333333333703, 0.3219752754296894559, 0.3333333333333333703, 0.3219752754296894559, 0.3333333333333333703, 0.3219752754296894559, 0.3333333333333333703, 0.3219752754296894559, 0.3333333333333333703, 0.3219752754296894559, 0.3333333333333333703, 0.3219752754296894559, 0.3333333333333333703, 0.3219752754296894559, 0.3333333333333333703, 0.3219752754296894559, 0.3333333333333333703, 0.3219752754296894559, 0.3333333333333333703, 0.3219752754296894559, 0.3333333333333333703, 0.3219752754296894559, 0.3333333333333333703, 0.3219752754296894559, 0.3333333333333333703, 0.3219752754296894559, 0.3333333333333333703, 0.3219752754296894559, 0.3333333333333333703, 0.3219752754296894559, 0.3333333333333333703, 0.3219752754296894559, 0.3333333333333333703, 0.3219752754296894559, 0.3333333333333333703, 0.3219752754296894559, 0.3333333333333333703, 0.3219752754296894559, 0.3333333333333333703, 0.3219752754296894559, 0.3333333333333333703, 0.3219752754296894559, 0.3333333333333333703, 0.3219752754296894559, 0.3333333333333333703, 0.3219752754296894559, 0.3333333333333333703, 0.3219752754296894559, 0.3333333333333333703, 0.3219752754296894559, 0.3333333333333333703, 0.3219752754296894559, 0.3333333333333333703, 0.3219752754296894559, 0.3333333333333333703, 0.3219752754296894559, 0.3333333333333333703, 0.3219752754296894559, 0.3333333333333333703, 0.3219752754296894559, 0.3333333333333333703, 0.3219752754296894559, 0.3333333333333333703, 0.3219752754296894559, 0.3333333333333333703, 0.3219752754296894559, 0.3333333333333333703, 0.3219752754296894559, 0.3333333333333333703, 0.3219752754296894559, 0.3333333333333333703, 0.3219752754296894559, 0.3333333333333333703, 0.3219752754296894559, 0.3333333333333333703, 0.3219752754296894559, 0.3333333333333333703, 0.3219752754296894559, 0.3333333333333333703, 0.3219752754296894559, 0.3333333333333333703, 0.3219752754296894559, 0.3333333333333333703, 0.3219752754296894559, 0.3333333333333333703, 0.3219752754296894559, 0.3333333333333333703, 0.3219752754296894559, 0.3333333333333333703, 0.3219752754296894559, 0.3333333333333333703, 0.3219752754296894559, 0.3333333333333333703, 0.3219752754296894559, 0.3333333333333333703, 0.3219752754296894559, 0.3333333333333333703, 0.3219752754296894559, 0.3333333333333333703, 0.3219752754296894559, 0.3333333333333333703, 0.3219752754296894559, 0.3333333333333333703, 0.3219752754296894559, 0.3333333333333333703, 0.3219752754296894559, 0.3333333333333333703, 0.3219752754296894559, 0.3333333333333333703, 0.3219752754296894559, 0.3333333333333333703, 0.3219752754296894559, 0.3333333333333333703, 0.3219752754296894559, 0.3333333333333333703, 0.3219752754296894559, 0.3333333333333333703, 0.3219752754296894559, 0.3333333333333333703, 0.3219752754296894559, 0.3333333333333333703, 0.3219752754296894559, 0.3333333333333333703, 0.3219752754296894559, 0.3333333333333333703, 0.3219752754296894559, 0.3333333333333333703, 0.3219752754296894559, 0.3333333333333333703, 0.3219752754296894559, 0.3333333333333333703, 0.3219752754296894559, 0.3333333333333333703, 0.3219752754296894559, 0.3333333333333333703, 0.3219752754296894559, 0.3333333333333333703, 0.3219752754296894559, 0.3333333333333333703),
 ( 0.3333333333333333703, 0.3219752754296894559, 0.3333333333333333703, 0.3219752754296894559, 0.3333333333333333703, 0.3219752754296894559, 0.3333333333333333703, 0.3219752754296894559, 0.3333333333333333703, 0.3219752754296894559, 0.3333333333333333703, 0.3219752754296894559, 0.3333333333333333703, 0.3219752754296894559, 0.3333333333333333703, 0.3219752754296894559, 0.3333333333333333703, 0.3219752754296894559, 0.3333333333333333703, 0.3219752754296894559, 0.3333333333333333703, 0.3219752754296894559, 0.3333333333333333703, 0.3219752754296894559, 0.3333333333333333703, 0.3219752754296894559, 0.3333333333333333703, 0.3219752754296894559, 0.3333333333333333703, 0.3219752754296894559, 0.3333333333333333703, 0.3219752754296894559, 0.3333333333333333703, 0.3219752754296894559, 0.3333333333333333703, 0.3219752754296894559, 0.3333333333333333703, 0.3219752754296894559, 0.3333333333333333703, 0.3219752754296894559, 0.3333333333333333703, 0.3219752754296894559, 0.3333333333333333703, 0.3219752754296894559, 0.3333333333333333703, 0.3219752754296894559, 0.3333333333333333703, 0.3219752754296894559, 0.3333333333333333703, 0.3219752754296894559, 0.3333333333333333703, 0.3219752754296894559, 0.3333333333333333703, 0.3219752754296894559, 0.3333333333333333703, 0.3219752754296894559, 0.3333333333333333703, 0.3219752754296894559, 0.3333333333333333703, 0.3219752754296894559, 0.3333333333333333703, 0.3219752754296894559, 0.3333333333333333703, 0.3219752754296894559, 0.3333333333333333703, 0.3219752754296894559, 0.3333333333333333703, 0.3219752754296894559, 0.3333333333333333703, 0.3219752754296894559, 0.3333333333333333703, 0.3219752754296894559, 0.3333333333333333703, 0.3219752754296894559, 0.3333333333333333703, 0.3219752754296894559, 0.3333333333333333703, 0.3219752754296894559, 0.3333333333333333703, 0.3219752754296894559, 0.3333333333333333703, 0.3219752754296894559, 0.3333333333333333703, 0.3219752754296894559, 0.3333333333333333703, 0.3219752754296894559, 0.3333333333333333703, 0.3219752754296894559, 0.3333333333333333703, 0.3219752754296894559, 0.3333333333333333703, 0.3219752754296894559, 0.3333333333333333703, 0.3219752754296894559, 0.3333333333333333703, 0.3219752754296894559, 0.3333333333333333703, 0.3219752754296894559, 0.3333333333333333703, 0.3219752754296894559, 0.3333333333333333703, 0.3219752754296894559, 0.3333333333333333703, 0.3219752754296894559, 0.3333333333333333703, 0.3219752754296894559, 0.3333333333333333703, 0.3219752754296894559, 0.3333333333333333703, 0.3219752754296894559, 0.3333333333333333703, 0.3219752754296894559, 0.3333333333333333703, 0.3219752754296894559, 0.3333333333333333703, 0.3219752754296894559, 0.3333333333333333703, 0.3219752754296894559, 0.3333333333333333703, 0.3219752754296894559, 0.3333333333333333703, 0.3219752754296894559, 0.3333333333333333703, 0.3219752754296894559, 0.3333333333333333703, 0.3219752754296894559, 0.3333333333333333703, 0.3219752754296894559, 0.3333333333333333703, 0.3219752754296894559, 0.3333333333333333703, 0.3219752754296894559, 0.3333333333333333703, 0.3219752754296894559, 0.3333333333333333703, 0.3219752754296894559, 0.3333333333333333703, 0.3219752754296894559, 0.3333333333333333703, 0.3219752754296894559, 0.3333333333333333703, 0.3219752754296894559, 0.3333333333333333703, 0.3219752754296894559, 0.3333333333333333703, 0.3219752754296894559, 0.3333333333333333703, 0.3219752754296894559, 0.3333333333333333703, 0.3219752754296894559, 0.3333333333333333703, 0.3219752754296894559, 0.3333333333333333703, 0.3219752754296894559, 0.3333333333333333703, 0.3219752754296894559, 0.3333333333333333703, 0.3219752754296894559, 0.3333333333333333703, 0.3219752754296894559, 0.3333333333333333703, 0.3219752754296894559, 0.3333333333333333703, 0.3219752754296894559, 0.3333333333333333703, 0.3219752754296894559, 0.3333333333333333703, 0.3219752754296894559, 0.3333333333333333703, 0.3219752754296894559, 0.3333333333333333703, 0.3219752754296894559, 0.3333333333333333703, 0.3219752754296894559, 0.3333333333333333703, 0.3219752754296894559, 0.3333333333333333703, 0.3219752754296894559, 0.3333333333333333703, 0.3219752754296894559, 0.3333333333333333703, 0.3219752754296894559, 0.3333333333333333703, 0.3219752754296894559, 0.3333333333333333703, 0.3219752754296894559, 0.3333333333333333703, 0.3219752754296894559, 0.3333333333333333703, 0.3219752754296894559, 0.3333333333333333703, 0.3219752754296894559, 0.3333333333333333703, 0.3219752754296894559, 0.3333333333333333703, 0.3219752754296894559, 0.3333333333333333703, 0.3219752754296894559, 0.3333333333333333703, 0.3219752754296894559, 0.3333333333333333703, 0.3219752754296894559, 0.3333333333333333703, 0.3219752754296894559, 0.3333333333333333703, 0.3219752754296894559, 0.3333333333333333703, 0.3219752754296894559, 0.3333333333333333703, 0.3219752754296894559, 0.3333333333333333703, 0.3219752754296894559, 0.3333333333333333703, 0.3219752754296894559, 0.3333333333333333703, 0.3219752754296894559, 0.3333333333333333703, 0.3219752754296894559, 0.3333333333333333703, 0.3219752754296894559, 0.3333333333333333703, 0.3219752754296894559, 0.3333333333333333703, 0.3219752754296894559, 0.3333333333333333703, 0.3219752754296894559, 0.3333333333333333703, 0.3219752754296894559, 0.3333333333333333703, 0.3219752754296894559, 0.3333333333333333703, 0.3219752754296894559, 0.3333333333333333703, 0.3219752754296894559, 0.3333333333333333703, 0.3219752754296894559, 0.3333333333333333703, 0.3219752754296894559, 0.3333333333333333703, 0.3219752754296894559, 0.3333333333333333703, 0.3219752754296894559, 0.3333333333333333703, 0.3219752754296894559, 0.3333333333333333703, 0.3219752754296894559, 0.3333333333333333703, 0.3219752754296894559, 0.3333333333333333703, 0.3219752754296894559, 0.3333333333333333703, 0.3219752754296894559, 0.3333333333333333703, 0.3219752754296894559, 0.3333333333333333703, 0.3219752754296894559, 0.3333333333333333703, 0.3219752754296894559, 0.3333333333333333703, 0.3219752754296894559, 0.3333333333333333703, 0.3219752754296894559, 0.3333333333333333703, 0.3219752754296894559, 0.3333333333333333703, 0.3219752754296894559, 0.3333333333333333703, 0.3219752754296894559, 0.3333333333333333703, 0.3219752754296894559, 0.3333333333333333703, 0.3219752754296894559, 0.3333333333333333703, 0.3219752754296894559, 0.3333333333333333703, 0.3219752754296894559, 0.3333333333333333703, 0.3219752754296894559, 0.3333333333333333703, 0.3219752754296894559, 0.3333333333333333703, 0.3219752754296894559, 0.3333333333333333703, 0.3219752754296894559, 0.3333333333333333703, 0.3219752754296894559, 0.3333333333333333703, 0.3219752754296894559, 0.3333333333333333703, 0.3219752754296894559, 0.3333333333333333703, 0.3219752754296894559, 0.3333333333333333703, 0.3219752754296894559, 0.3333333333333333703, 0.3219752754296894559, 0.3333333333333333703, 0.3219752754296894559, 0.3333333333333333703, 0.3219752754296894559, 0.3333333333333333703, 0.3219752754296894559, 0.3333333333333333703, 0.3219752754296894559, 0.3333333333333333703, 0.3219752754296894559, 0.3333333333333333703, 0.3219752754296894559, 0.3333333333333333703, 0.3219752754296894559, 0.3333333333333333703, 0.3219752754296894559, 0.3333333333333333703, 0.3219752754296894559, 0.3333333333333333703, 0.3219752754296894559, 0.3333333333333333703, 0.3219752754296894559, 0.3333333333333333703, 0.3219752754296894559, 0.3333333333333333703, 0.3219752754296894559, 0.3333333333333333703, 0.3219752754296894559, 0.3333333333333333703, 0.3219752754296894559, 0.3333333333333333703, 0.3219752754296894559, 0.3333333333333333703, 0.3219752754296894559, 0.3333333333333333703, 0.3219752754296894559, 0.3333333333333333703, 0.3219752754296894559, 0.3333333333333333703, 0.3219752754296894559, 0.3333333333333333703, 0.3219752754296894559, 0.3333333333333333703, 0.3219752754296894559, 0.3333333333333333703, 0.3219752754296894559, 0.3333333333333333703, 0.3219752754296894559, 0.3333333333333333703, 0.3219752754296894559, 0.3333333333333333703, 0.3219752754296894559, 0.3333333333333333703, 0.3219752754296894559, 0.3333333333333333703, 0.3219752754296894559, 0.3333333333333333703, 0.3219752754296894559, 0.3333333333333333703, 0.3219752754296894559, 0.3333333333333333703, 0.3219752754296894559, 0.3333333333333333703, 0.3219752754296894559, 0.3333333333333333703, 0.3219752754296894559, 0.3333333333333333703, 0.3219752754296894559, 0.3333333333333333703, 0.3219752754296894559, 0.3333333333333333703, 0.3219752754296894559, 0.3333333333333333703, 0.3219752754296894559, 0.3333333333333333703, 0.3219752754296894559, 0.3333333333333333703, 0.3219752754296894559, 0.3333333333333333703, 0.3219752754296894559, 0.3333333333333333703, 0.3219752754296894559, 0.3333333333333333703, 0.3219752754296894559, 0.3333333333333333703, 0.3219752754296894559, 0.3333333333333333703, 0.3219752754296894559, 0.3333333333333333703, 0.3219752754296894559, 0.3333333333333333703, 0.3219752754296894559, 0.3333333333333333703, 0.3219752754296894559, 0.3333333333333333703, 0.3219752754296894559, 0.3333333333333333703, 0.3219752754296894559, 0.3333333333333333703, 0.3219752754296894559, 0.3333333333333333703, 0.3219752754296894559, 0.3333333333333333703, 0.3219752754296894559, 0.3333333333333333703, 0.3219752754296894559, 0.3333333333333333703, 0.3219752754296894559, 0.3333333333333333703, 0.3219752754296894559, 0.3333333333333333703, 0.3219752754296894559, 0.3333333333333333703, 0.3219752754296894559, 0.3333333333333333703, 0.3219752754296894559, 0.3333333333333333703, 0.3219752754296894559, 0.3333333333333333703, 0.3219752754296894559, 0.3333333333333333703, 0.3219752754296894559, 0.3333333333333333703, 0.3219752754296894559, 0.3333333333333333703, 0.3219752754296894559, 0.3333333333333333703, 0.3219752754296894559, 0.3333333333333333703, 0.3219752754296894559, 0.3333333333333333703, 0.3219752754296894559, 0.3333333333333333703, 0.3219752754296894559, 0.3333333333333333703, 0.3219752754296894559, 0.3333333333333333703, 0.3219752754296894559, 0.3333333333333333703, 0.3219752754296894559, 0.3333333333333333703, 0.3219752754296894559, 0.3333333333333333703, 0.3219752754296894559, 0.3333333333333333703, 0.3219752754296894559, 0.3333333333333333703, 0.3219752754296894559, 0.3333333333333333703, 0.3219752754296894559, 0.3333333333333333703, 0.3219752754296894559, 0.3333333333333333703, 0.3219752754296894559, 0.3333333333333333703, 0.3219752754296894559, 0.3333333333333333703, 0.3219752754296894559, 0.3333333333333333703, 0.3219752754296894559, 0.3333333333333333703),
 ( 1.000000000000000000, 0.9659258262890683122, 1.000000000000000000, 0.9659258262890683122, 1.000000000000000000, 0.9659258262890683122, 1.000000000000000000, 0.9659258262890683122, 1.000000000000000000, 0.9659258262890683122, 1.000000000000000000, 0.9659258262890683122, 1.000000000000000000, 0.9659258262890683122, 1.000000000000000000, 0.9659258262890683122, 1.000000000000000000, 0.9659258262890683122, 1.000000000000000000, 0.9659258262890683122, 1.000000000000000000, 0.9659258262890683122, 1.000000000000000000, 0.9659258262890683122, 1.000000000000000000, 0.9659258262890683122, 1.000000000000000000, 0.9659258262890683122, 1.000000000000000000, 0.9659258262890683122, 1.000000000000000000, 0.9659258262890683122, 1.000000000000000000, 0.9659258262890683122, 1.000000000000000000, 0.9659258262890683122, 1.000000000000000000, 0.9659258262890683122, 1.000000000000000000, 0.9659258262890683122, 1.000000000000000000, 0.9659258262890683122, 1.000000000000000000, 0.9659258262890683122, 1.000000000000000000, 0.9659258262890683122, 1.000000000000000000, 0.9659258262890683122, 1.000000000000000000, 0.9659258262890683122, 1.000000000000000000, 0.9659258262890683122, 1.000000000000000000, 0.9659258262890683122, 1.000000000000000000, 0.9659258262890683122, 1.000000000000000000, 0.9659258262890683122, 1.000000000000000000, 0.9659258262890683122, 1.000000000000000000, 0.9659258262890683122, 1.000000000000000000, 0.9659258262890683122, 1.000000000000000000, 0.9659258262890683122, 1.000000000000000000, 0.9659258262890683122, 1.000000000000000000, 0.9659258262890683122, 1.000000000000000000, 0.9659258262890683122, 1.000000000000000000, 0.9659258262890683122, 1.000000000000000000, 0.9659258262890683122, 1.000000000000000000, 0.9659258262890683122, 1.000000000000000000, 0.9659258262890683122, 1.000000000000000000, 0.9659258262890683122, 1.000000000000000000, 0.9659258262890683122, 1.000000000000000000, 0.9659258262890683122, 1.000000000000000000, 0.9659258262890683122, 1.000000000000000000, 0.9659258262890683122, 1.000000000000000000, 0.9659258262890683122, 1.000000000000000000, 0.9659258262890683122, 1.000000000000000000, 0.9659258262890683122, 1.000000000000000000, 0.9659258262890683122, 1.000000000000000000, 0.9659258262890683122, 1.000000000000000000, 0.9659258262890683122, 1.000000000000000000, 0.9659258262890683122, 1.000000000000000000, 0.9659258262890683122, 1.000000000000000000, 0.9659258262890683122, 1.000000000000000000, 0.9659258262890683122, 1.000000000000000000, 0.9659258262890683122, 1.000000000000000000, 0.9659258262890683122, 1.000000000000000000, 0.9659258262890683122, 1.000000000000000000, 0.9659258262890683122, 1.000000000000000000, 0.9659258262890683122, 1.000000000000000000, 0.9659258262890683122, 1.000000000000000000, 0.9659258262890683122, 1.000000000000000000, 0.9659258262890683122, 1.000000000000000000, 0.9659258262890683122, 1.000000000000000000, 0.9659258262890683122, 1.000000000000000000, 0.9659258262890683122, 1.000000000000000000, 0.9659258262890683122, 1.000000000000000000, 0.9659258262890683122, 1.000000000000000000, 0.9659258262890683122, 1.000000000000000000, 0.9659258262890683122, 1.000000000000000000, 0.9659258262890683122, 1.000000000000000000, 0.9659258262890683122, 1.000000000000000000, 0.9659258262890683122, 1.000000000000000000, 0.9659258262890683122, 1.000000000000000000, 0.9659258262890683122, 1.000000000000000000, 0.9659258262890683122, 1.000000000000000000, 0.9659258262890683122, 1.000000000000000000, 0.9659258262890683122, 1.000000000000000000, 0.9659258262890683122, 1.000000000000000000, 0.9659258262890683122, 1.000000000000000000, 0.9659258262890683122, 1.000000000000000000, 0.9659258262890683122, 1.000000000000000000, 0.9659258262890683122, 1.000000000000000000, 0.9659258262890683122, 1.000000000000000000, 0.9659258262890683122, 1.000000000000000000, 0.9659258262890683122, 1.000000000000000000, 0.9659258262890683122, 1.000000000000000000, 0.9659258262890683122, 1.000000000000000000, 0.9659258262890683122, 1.000000000000000000, 0.9659258262890683122, 1.000000000000000000, 0.9659258262890683122, 1.000000000000000000, 0.9659258262890683122, 1.000000000000000000, 0.9659258262890683122, 1.000000000000000000, 0.9659258262890683122, 1.000000000000000000, 0.9659258262890683122, 1.000000000000000000, 0.9659258262890683122, 1.000000000000000000, 0.9659258262890683122, 1.000000000000000000, 0.9659258262890683122, 1.000000000000000000, 0.9659258262890683122, 1.000000000000000000, 0.9659258262890683122, 1.000000000000000000, 0.9659258262890683122, 1.000000000000000000, 0.9659258262890683122, 1.000000000000000000, 0.9659258262890683122, 1.000000000000000000, 0.9659258262890683122, 1.000000000000000000, 0.9659258262890683122, 1.000000000000000000, 0.9659258262890683122, 1.000000000000000000, 0.9659258262890683122, 1.000000000000000000, 0.9659258262890683122, 1.000000000000000000, 0.9659258262890683122, 1.000000000000000000, 0.9659258262890683122, 1.000000000000000000, 0.9659258262890683122, 1.000000000000000000, 0.9659258262890683122, 1.000000000000000000, 0.9659258262890683122, 1.000000000000000000, 0.9659258262890683122, 1.000000000000000000, 0.9659258262890683122, 1.000000000000000000, 0.9659258262890683122, 1.000000000000000000, 0.9659258262890683122, 1.000000000000000000, 0.9659258262890683122, 1.000000000000000000, 0.9659258262890683122, 1.000000000000000000, 0.9659258262890683122, 1.000000000000000000, 0.9659258262890683122, 1.000000000000000000, 0.9659258262890683122, 1.000000000000000000, 0.9659258262890683122, 1.000000000000000000, 0.9659258262890683122, 1.000000000000000000, 0.9659258262890683122, 1.000000000000000000, 0.9659258262890683122, 1.000000000000000000, 0.9659258262890683122, 1.000000000000000000, 0.9659258262890683122, 1.000000000000000000, 0.9659258262890683122, 1.000000000000000000, 0.9659258262890683122, 1.000000000000000000, 0.9659258262890683122, 1.000000000000000000, 0.9659258262890683122, 1.000000000000000000, 0.9659258262890683122, 1.000000000000000000, 0.9659258262890683122, 1.000000000000000000, 0.9659258262890683122, 1.000000000000000000, 0.9659258262890683122, 1.000000000000000000, 0.9659258262890683122, 1.000000000000000000, 0.9659258262890683122, 1.000000000000000000, 0.9659258262890683122, 1.000000000000000000, 0.9659258262890683122, 1.000000000000000000, 0.9659258262890683122, 1.000000000000000000, 0.9659258262890683122, 1.000000000000000000, 0.9659258262890683122, 1.000000000000000000, 0.9659258262890683122, 1.000000000000000000, 0.9659258262890683122, 1.000000000000000000, 0.9659258262890683122, 1.000000000000000000, 0.9659258262890683122, 1.000000000000000000, 0.9659258262890683122, 1.000000000000000000, 0.9659258262890683122, 1.000000000000000000, 0.9659258262890683122, 1.000000000000000000, 0.9659258262890683122, 1.000000000000000000, 0.9659258262890683122, 1.000000000000000000, 0.9659258262890683122, 1.000000000000000000, 0.9659258262890683122, 1.000000000000000000, 0.9659258262890683122, 1.000000000000000000, 0.9659258262890683122, 1.000000000000000000, 0.9659258262890683122, 1.000000000000000000, 0.9659258262890683122, 1.000000000000000000, 0.9659258262890683122, 1.000000000000000000, 0.9659258262890683122, 1.000000000000000000, 0.9659258262890683122, 1.000000000000000000, 0.9659258262890683122, 1.000000000000000000, 0.9659258262890683122, 1.000000000000000000, 0.9659258262890683122, 1.000000000000000000, 0.9659258262890683122, 1.000000000000000000, 0.9659258262890683122, 1.000000000000000000, 0.9659258262890683122, 1.000000000000000000, 0.9659258262890683122, 1.000000000000000000, 0.9659258262890683122, 1.000000000000000000, 0.9659258262890683122, 1.000000000000000000, 0.9659258262890683122, 1.000000000000000000, 0.9659258262890683122, 1.000000000000000000, 0.9659258262890683122, 1.000000000000000000, 0.9659258262890683122, 1.000000000000000000, 0.9659258262890683122, 1.000000000000000000, 0.9659258262890683122, 1.000000000000000000, 0.9659258262890683122, 1.000000000000000000, 0.9659258262890683122, 1.000000000000000000, 0.9659258262890683122, 1.000000000000000000, 0.9659258262890683122, 1.000000000000000000, 0.9659258262890683122, 1.000000000000000000, 0.9659258262890683122, 1.000000000000000000, 0.9659258262890683122, 1.000000000000000000, 0.9659258262890683122, 1.000000000000000000, 0.9659258262890683122, 1.000000000000000000, 0.9659258262890683122, 1.000000000000000000, 0.9659258262890683122, 1.000000000000000000, 0.9659258262890683122, 1.000000000000000000, 0.9659258262890683122, 1.000000000000000000, 0.9659258262890683122, 1.000000000000000000, 0.9659258262890683122, 1.000000000000000000, 0.9659258262890683122, 1.000000000000000000, 0.9659258262890683122, 1.000000000000000000, 0.9659258262890683122, 1.000000000000000000, 0.9659258262890683122, 1.000000000000000000, 0.9659258262890683122, 1.000000000000000000, 0.9659258262890683122, 1.000000000000000000, 0.9659258262890683122, 1.000000000000000000, 0.9659258262890683122, 1.000000000000000000, 0.9659258262890683122, 1.000000000000000000, 0.9659258262890683122, 1.000000000000000000, 0.9659258262890683122, 1.000000000000000000, 0.9659258262890683122, 1.000000000000000000, 0.9659258262890683122, 1.000000000000000000, 0.9659258262890683122, 1.000000000000000000, 0.9659258262890683122, 1.000000000000000000, 0.9659258262890683122, 1.000000000000000000, 0.9659258262890683122, 1.000000000000000000, 0.9659258262890683122, 1.000000000000000000, 0.9659258262890683122, 1.000000000000000000, 0.9659258262890683122, 1.000000000000000000, 0.9659258262890683122, 1.000000000000000000, 0.9659258262890683122, 1.000000000000000000, 0.9659258262890683122, 1.000000000000000000, 0.9659258262890683122, 1.000000000000000000, 0.9659258262890683122, 1.000000000000000000, 0.9659258262890683122, 1.000000000000000000, 0.9659258262890683122, 1.000000000000000000, 0.9659258262890683122, 1.000000000000000000, 0.9659258262890683122, 1.000000000000000000, 0.9659258262890683122, 1.000000000000000000, 0.9659258262890683122, 1.000000000000000000, 0.9659258262890683122, 1.000000000000000000, 0.9659258262890683122, 1.000000000000000000, 0.9659258262890683122, 1.000000000000000000, 0.9659258262890683122, 1.000000000000000000, 0.9659258262890683122, 1.000000000000000000, 0.9659258262890683122, 1.000000000000000000) ) ) 
 REPRESENTATION_ITEM ( '' )  SURFACE ( )  );
#87143=CARTESIAN_POINT ( 'NONE',  ( -9.474510206698720793, -16.51473224551083518, 34.58442372801899722 ) ) ;
#87144=CARTESIAN_POINT ( 'NONE',  ( 10.81492255796106328, -18.62759615963255655, 25.41775706135235779 ) ) ;
#87145=CARTESIAN_POINT ( 'NONE',  ( 13.97604488694527802, 13.89961937509977652, 74.37390960531436690 ) ) ;
#87146=CARTESIAN_POINT ( 'NONE',  ( -0.05219959533910754901, -16.53943276465976808, 82.49890960531436690 ) ) ;
#87147=CARTESIAN_POINT ( 'NONE',  ( -8.314922557960811034, -14.29746914071050412, 47.08224293864770260 ) ) ;
#87148=CARTESIAN_POINT ( 'NONE',  ( -18.67979575497178146, -10.72451020669898902, 61.66557627198103120 ) ) ;
#87149=CARTESIAN_POINT ( 'NONE',  ( -16.46253265017160317, 9.564922557960807481, 45.83224293864769550 ) ) ;
#87150=CARTESIAN_POINT ( 'NONE',  ( -18.67979575497178146, -10.72451020669898902, 66.66557627198102409 ) ) ;
#87151=CARTESIAN_POINT ( 'NONE',  ( 5.049401038297881783, 19.05341960407617563, 52.29275706135234003 ) ) ;
#87152=CARTESIAN_POINT ( 'NONE',  ( 9.474510206698729675, 16.51473224551082808, 27.08442372801900433 ) ) ;
#87153=CARTESIAN_POINT ( 'NONE',  ( 4.379528057220339221, -16.55341960407611168, 67.70724293864769550 ) ) ;
#87154=CARTESIAN_POINT ( 'NONE',  ( 15.72974639402199770, -15.80617190586745480, 43.12390960531435269 ) ) ;
#87157=CARTESIAN_POINT ( 'NONE',  ( 17.05587630539788080, 6.762274262135703928, 101.7581969096269177 ) ) ;
#87158=CARTESIAN_POINT ( 'NONE',  ( -14.34966873604972548, 8.224510206698743886, 88.33442372801901854 ) ) ;
#87160=CARTESIAN_POINT ( 'NONE',  ( -19.05341960407617563, 5.049401038297882671, 88.54275706135230450 ) ) ;
#87161=CARTESIAN_POINT ( 'NONE',  ( -12.06949235617756955, 12.14591786802309770, 55.62390960531436690 ) ) ;
#87162=CARTESIAN_POINT ( 'NONE',  ( 16.31925111598461342, -7.325300261831395154, 52.66424538967255842 ) ) ;
#87163=CARTESIAN_POINT ( 'NONE',  ( 16.46253265017160672, -9.564922557960803928, 53.33224293864768839 ) ) ;
#87164=CARTESIAN_POINT ( 'NONE',  ( -0.05219959533910754901, -16.53943276465976808, 42.49890960531435979 ) ) ;
#87166=CARTESIAN_POINT ( 'NONE',  ( 16.46253265017160672, -9.564922557960803928, 88.33224293864769550 ) ) ;
#87167=CARTESIAN_POINT ( 'NONE',  ( 19.02544592524343514, -5.153800228976328945, 53.54057627198102409 ) ) ;
#87168=CARTESIAN_POINT ( 'NONE',  ( 5.823673210054444382, -21.52544592524334988, 60.20942372801902565 ) ) ;
#87169=CARTESIAN_POINT ( 'NONE',  ( 19.03943276465977164, -0.05219959533909143690, 73.74890960531435269 ) ) ;
#87170=CARTESIAN_POINT ( 'NONE',  ( 19.05341960407611168, 5.049401038298154454, 28.95724293864769550 ) ) ;
#87171=CARTESIAN_POINT ( 'NONE',  ( 16.51473224551069308, 9.474510206698969483, 74.16557627198103830 ) ) ;
#87172=CARTESIAN_POINT ( 'NONE',  ( 15.80617190586746368, 15.72974639402197994, 44.37390960531435979 ) ) ;
#87173=CARTESIAN_POINT ( 'NONE',  ( -13.89961937509977652, 13.97604488694528158, 30.62390960531435269 ) ) ;
#87174=CARTESIAN_POINT ( 'NONE',  ( 0.05219959533907565091, 21.53943276465977519, 44.99890960531435979 ) ) ;
#87175=CARTESIAN_POINT ( 'NONE',  ( 8.314922557961029526, -14.29746914071037800, 110.4177570613523756 ) ) ;
#87176=CARTESIAN_POINT ( 'NONE',  ( 9.474510206698729675, 16.51473224551082808, 27.08442372801900433 ) ) ;
#87177=CARTESIAN_POINT ( 'NONE',  ( 14.29746914071037800, 8.314922557961029526, 41.66775706135235424 ) ) ;
#87178=CARTESIAN_POINT ( 'NONE',  ( -16.52544592524335698, -4.483927247898792601, 83.95942372801900433 ) ) ;
#87179=CARTESIAN_POINT ( 'NONE',  ( -17.97058386085787163, -5.500000000000017764, 94.00390968646219392 ) ) ;
#87180=CARTESIAN_POINT ( 'NONE',  ( 4.379528057220092307, 16.55341960407617563, 72.29275706135236135 ) ) ;
#87181=CARTESIAN_POINT ( 'NONE',  ( -0.05219959533934338120, 16.53943276465976808, 57.50109039468568994 ) ) ;
#87182=CARTESIAN_POINT ( 'NONE',  ( -16.46253265017160317, 9.564922557960807481, 110.8322429386476955 ) ) ;
#87183=CARTESIAN_POINT ( 'NONE',  ( 19.02544592524343514, -5.153800228976328945, 33.54057627198102409 ) ) ;
#87184=CARTESIAN_POINT ( 'NONE',  ( 16.52544592524335698, 4.483927247898782831, 41.45942372801901143 ) ) ;
#87185=CARTESIAN_POINT ( 'NONE',  ( 19.05341960407611168, 5.049401038298154454, 48.95724293864768129 ) ) ;
#87186=CARTESIAN_POINT ( 'NONE',  ( -21.55341960407619339, 5.719274019375674811, 23.54275706135235424 ) ) ;
#87187=CARTESIAN_POINT ( 'NONE',  ( -8.314922557961024197, 14.29746914071037800, 37.91775706135235424 ) ) ;
#87188=CARTESIAN_POINT ( 'NONE',  ( -14.29746914071037622, -8.314922557961029526, 94.16775706135237556 ) ) ;
#87190=CARTESIAN_POINT ( 'NONE',  ( 0.05219959533937995610, -21.53943276465977519, 100.0010903946857042 ) ) ;
#87191=CARTESIAN_POINT ( 'NONE',  ( -19.05341960407617563, 5.049401038297882671, 103.5427570613523329 ) ) ;
#87192=CARTESIAN_POINT ( 'NONE',  ( 9.564922557961047289, -16.46253265017146816, 50.41775706135233293 ) ) ;
#87193=CARTESIAN_POINT ( 'NONE',  ( 4.379528057220339221, -16.55341960407611168, 52.70724293864769550 ) ) ;
#87194=CARTESIAN_POINT ( 'NONE',  ( 16.51473224551069308, 9.474510206698969483, 24.16557627198102765 ) ) ;
#87195=CARTESIAN_POINT ( 'NONE',  ( 19.05341960407617918, -5.049401038297876454, 56.04275706135234714 ) ) ;
#87196=CARTESIAN_POINT ( 'NONE',  ( 17.40861289039003523, 6.110651285853276882, 78.87232470827434838 ) ) ;
#87197=CARTESIAN_POINT ( 'NONE',  ( -21.52544592524334988, -5.823673210054445271, 68.95942372801901854 ) ) ;
#87198=CARTESIAN_POINT ( 'NONE',  ( -4.379528057220086978, -16.55341960407618274, 29.79275706135234358 ) ) ;
#87199=CARTESIAN_POINT ( 'NONE',  ( 19.36337904590692105, -5.499999999999940492, 57.91494137495621430 ) ) ;
#87200=CARTESIAN_POINT ( 'NONE',  ( -19.03943276465977164, 0.05219959533909376836, 116.2489096053143669 ) ) ;
#87201=CARTESIAN_POINT ( 'NONE',  ( -9.474510206698720793, -16.51473224551083518, 104.5844237280190043 ) ) ;
#87202=CARTESIAN_POINT ( 'NONE',  ( 0.05219959533909260263, 19.03943276465977164, 109.9989096053143669 ) ) ;
#87204=CARTESIAN_POINT ( 'NONE',  ( -19.02544592524342804, 5.153800228976336051, 31.04057627198102409 ) ) ;
#87205=CARTESIAN_POINT ( 'NONE',  ( 18.62759615963255655, 10.81492255796105972, 106.6677570613523756 ) ) ;
#87206=CARTESIAN_POINT ( 'NONE',  ( -0.05219959533909027116, -19.03943276465977164, 37.49890960531436690 ) ) ;
#87207=CARTESIAN_POINT ( 'NONE',  ( 15.72974639402176855, 15.80617190586768217, 61.87609039468568284 ) ) ;
#87208=CARTESIAN_POINT ( 'NONE',  ( -21.55341960407619339, 5.719274019375674811, 108.5427570613523756 ) ) ;
#87209=CARTESIAN_POINT ( 'NONE',  ( 8.314922557961029526, -14.29746914071037800, 105.4177570613523613 ) ) ;
#87210=CARTESIAN_POINT ( 'NONE',  ( 19.03943276465977164, -0.05219959533909143690, 78.74890960531436690 ) ) ;
#87211=CARTESIAN_POINT ( 'NONE',  ( -18.62759615963255300, -10.81492255796106328, 54.16775706135235424 ) ) ;
#87212=CARTESIAN_POINT ( 'NONE',  ( 15.72974639402176855, 15.80617190586768217, 46.87609039468568994 ) ) ;
#87213=CARTESIAN_POINT ( 'NONE',  ( -5.153800228976607833, 19.02544592524334988, 82.70942372801897591 ) ) ;
#87214=CARTESIAN_POINT ( 'NONE',  ( 13.89961937509977652, -13.97604488694527269, 108.1239096053143669 ) ) ;
#87215=CARTESIAN_POINT ( 'NONE',  ( -12.06949235617756955, 12.14591786802309770, 115.6239096053143669 ) ) ;
#87216=CARTESIAN_POINT ( 'NONE',  ( -18.67979575497178146, -10.72451020669898902, 91.66557627198103830 ) ) ;
#87217=CARTESIAN_POINT ( 'NONE',  ( -9.474510206698720793, -16.51473224551083518, 19.58442372801899722 ) ) ;
#87218=CARTESIAN_POINT ( 'NONE',  ( 4.379528057220339221, -16.55341960407611168, 102.7072429386476955 ) ) ;
#87219=CARTESIAN_POINT ( 'NONE',  ( -9.474510206698964154, 16.51473224551069663, 55.41557627198103120 ) ) ;
#87220=CARTESIAN_POINT ( 'NONE',  ( -5.153800228976607833, 19.02544592524334988, 92.70942372801901854 ) ) ;
#87221=CARTESIAN_POINT ( 'NONE',  ( 0.05219959533910956823, 16.53943276465976808, 64.99890960531435269 ) ) ;
#87222=CARTESIAN_POINT ( 'NONE',  ( -15.72974639402176322, -15.80617190586768395, 109.3760903946857042 ) ) ;
#87223=CARTESIAN_POINT ( 'NONE',  ( -9.474510206698964154, 16.51473224551069663, 105.4155762719810383 ) ) ;
#87224=CARTESIAN_POINT ( 'NONE',  ( -19.03943276465977164, -0.05219959533935918106, 78.75109039468567573 ) ) ;
#87225=CARTESIAN_POINT ( 'NONE',  ( -5.823673210054116645, -21.52544592524344225, 77.29057627198102409 ) ) ;
#87226=CARTESIAN_POINT ( 'NONE',  ( 21.52544592524334988, 5.823673210054432836, 31.45942372801901854 ) ) ;
#87227=CARTESIAN_POINT ( 'NONE',  ( -8.224510206698735004, -14.34966873604973081, 24.58442372801901499 ) ) ;
#87228=CARTESIAN_POINT ( 'NONE',  ( 4.379528057220092307, 16.55341960407617563, 92.29275706135236135 ) ) ;
#87229=CARTESIAN_POINT ( 'NONE',  ( -12.14591786802326823, 12.06949235617739902, 48.12609039468568284 ) ) ;
#87230=CARTESIAN_POINT ( 'NONE',  ( -18.62759615963255300, -10.81492255796106328, 39.16775706135235424 ) ) ;
#87231=CARTESIAN_POINT ( 'NONE',  ( 21.52544592524344225, -5.823673210054117533, 38.54057627198103120 ) ) ;
#87232=CARTESIAN_POINT ( 'NONE',  ( -19.05341960407611168, -5.049401038298163336, 31.45724293864769550 ) ) ;
#87234=CARTESIAN_POINT ( 'NONE',  ( 8.314922557961029526, -14.29746914071037800, 65.41775706135234714 ) ) ;
#87235=CARTESIAN_POINT ( 'NONE',  ( 21.55341960407610458, 5.719274019375980345, 83.95724293864770971 ) ) ;
#87236=CARTESIAN_POINT ( 'NONE',  ( -16.52544592524342804, 4.483927247898546575, 36.04057627198102409 ) ) ;
#87237=CARTESIAN_POINT ( 'NONE',  ( -16.55341960407617563, 4.379528057220093196, 48.54275706135234714 ) ) ;
#87238=CARTESIAN_POINT ( 'NONE',  ( -5.049401038298153566, 19.05341960407611168, 55.20724293864769550 ) ) ;
#87239=CARTESIAN_POINT ( 'NONE',  ( -16.52544592524335698, -4.483927247898792601, 93.95942372801903275 ) ) ;
#87240=CARTESIAN_POINT ( 'NONE',  ( -13.89961937509957401, -13.97604488694547875, 84.37609039468567573 ) ) ;
#87241=CARTESIAN_POINT ( 'NONE',  ( 5.719274019375991003, -21.55341960407610458, 87.70724293864769550 ) ) ;
#87242=CARTESIAN_POINT ( 'NONE',  ( 8.224510206698953496, -14.34966873604960469, 27.91557627198103830 ) ) ;
#87245=CARTESIAN_POINT ( 'NONE',  ( 10.81492255796078972, 18.62759615963270932, 59.58224293864770260 ) ) ;
#87246=CARTESIAN_POINT ( 'NONE',  ( 8.314922557961029526, -14.29746914071037800, 100.4177570613523471 ) ) ;
#87248=CARTESIAN_POINT ( 'NONE',  ( 17.50000000000001421, -3.385507783985830521, 102.6446170133486930 ) ) ;
#87249=CARTESIAN_POINT ( 'NONE',  ( 21.52544592524344225, -5.823673210054117533, 83.54057627198102409 ) ) ;
#87250=CARTESIAN_POINT ( 'NONE',  ( -12.14591786802326823, 12.06949235617739902, 113.1260903946856899 ) ) ;
#87251=CARTESIAN_POINT ( 'NONE',  ( -12.14591786802326823, 12.06949235617739902, 33.12609039468569705 ) ) ;
#87252=CARTESIAN_POINT ( 'NONE',  ( -19.03943276465977164, 0.05219959533909376836, 31.24890960531435979 ) ) ;
#87253=CARTESIAN_POINT ( 'NONE',  ( 19.03943276465977164, -0.05219959533909143690, 48.74890960531435979 ) ) ;
#87255=CARTESIAN_POINT ( 'NONE',  ( 9.564922557960805705, 16.46253265017160317, 114.5822429386476955 ) ) ;
#87257=CARTESIAN_POINT ( 'NONE',  ( -4.483927247898782831, 16.52544592524335698, 97.70942372801904696 ) ) ;
#87258=CARTESIAN_POINT ( 'NONE',  ( -19.05341960407617563, 5.049401038297882671, 98.54275706135233293 ) ) ;
#87259=CARTESIAN_POINT ( 'NONE',  ( -19.05341960407617563, 5.049401038297882671, 38.54275706135233293 ) ) ;
#87260=CARTESIAN_POINT ( 'NONE',  ( 21.55341960407610458, 5.719274019375980345, 83.95724293864770971 ) ) ;
#87261=CARTESIAN_POINT ( 'NONE',  ( 4.483927247898790824, -16.52544592524335698, 110.2094237280190185 ) ) ;
#87262=CARTESIAN_POINT ( 'NONE',  ( -18.62759615963270932, 10.81492255796079327, 30.83224293864770260 ) ) ;
#87263=CARTESIAN_POINT ( 'NONE',  ( -5.153800228976607833, 19.02544592524334988, 107.7094237280189759 ) ) ;
#87264=CARTESIAN_POINT ( 'NONE',  ( 9.564922557960805705, 16.46253265017160317, 104.5822429386476955 ) ) ;
#87265=CARTESIAN_POINT ( 'NONE',  ( -5.823673210054431948, 21.52544592524334988, 67.70942372801901854 ) ) ;
#87266=CARTESIAN_POINT ( 'NONE',  ( 19.03943276465977164, -0.05219959533909143690, 58.74890960531435979 ) ) ;
#87268=CARTESIAN_POINT ( 'NONE',  ( -14.34966873604960291, -8.224510206698953496, 106.6655762719810383 ) ) ;
#87270=CARTESIAN_POINT ( 'NONE',  ( 19.02544592524343514, -5.153800228976328945, 68.54057627198103830 ) ) ;
#87271=CARTESIAN_POINT ( 'NONE',  ( -4.483927247898539470, -16.52544592524342804, 72.29057627198102409 ) ) ;
#87273=CARTESIAN_POINT ( 'NONE',  ( -16.46253265017146816, -9.564922557961047289, 94.16775706135233293 ) ) ;
#87274=CARTESIAN_POINT ( 'NONE',  ( -19.03943276465977164, 0.05219959533909376836, 61.24890960531436690 ) ) ;
#87276=CARTESIAN_POINT ( 'NONE',  ( -16.46253265017160317, 9.564922557960807481, 70.83224293864770971 ) ) ;
#87277=CARTESIAN_POINT ( 'NONE',  ( -19.02544592524342804, 5.153800228976336051, 106.0405762719810241 ) ) ;
#87278=CARTESIAN_POINT ( 'NONE',  ( -14.29746914071037622, -8.314922557961029526, 59.16775706135234714 ) ) ;
#87280=CARTESIAN_POINT ( 'NONE',  ( -13.97604488694547697, 13.89961937509957934, 43.12609039468566152 ) ) ;
#87281=CARTESIAN_POINT ( 'NONE',  ( 10.72451020669871369, 18.67979575497193778, 102.0844237280190185 ) ) ;
#87283=CARTESIAN_POINT ( 'NONE',  ( 9.474510206698971260, -16.51473224551069308, 107.9155762719810383 ) ) ;
#87284=CARTESIAN_POINT ( 'NONE',  ( 14.29746914071037800, 8.314922557961029526, 96.66775706135234714 ) ) ;
#87285=EDGE_CURVE ( 'NONE', #94244, #44638, #153592, .T. ) ;
#87286=CARTESIAN_POINT ( 'NONE',  ( 9.564922557961047289, -16.46253265017146816, 75.41775706135234714 ) ) ;
#87287=CARTESIAN_POINT ( 'NONE',  ( -0.05219959533934338120, 16.53943276465976808, 92.50109039468567573 ) ) ;
#87288=CARTESIAN_POINT ( 'NONE',  ( -17.05116617787826527, 6.768360034955678728, 28.65675553259198693 ) ) ;
#87289=CARTESIAN_POINT ( 'NONE',  ( 14.29746914071037800, 8.314922557961029526, 61.66775706135235424 ) ) ;
#87291=CARTESIAN_POINT ( 'NONE',  ( 18.62759615963255655, 10.81492255796105972, 86.66775706135234714 ) ) ;
#87292=CARTESIAN_POINT ( 'NONE',  ( 5.049401038297881783, 19.05341960407617563, 92.29275706135234714 ) ) ;
#87293=CARTESIAN_POINT ( 'NONE',  ( -13.89961937509957401, -13.97604488694547875, 24.37609039468565442 ) ) ;
#87294=CARTESIAN_POINT ( 'NONE',  ( -19.03943276465977164, 0.05219959533909376836, 61.24890960531436690 ) ) ;
#87295=CARTESIAN_POINT ( 'NONE',  ( -0.05219959533909027116, -19.03943276465977164, 47.49890960531435979 ) ) ;
#87297=CARTESIAN_POINT ( 'NONE',  ( -18.67979575497178146, -10.72451020669898902, 86.66557627198102409 ) ) ;
#87299=CARTESIAN_POINT ( 'NONE',  ( 0.05219959533907565091, 21.53943276465977519, 34.99890960531435979 ) ) ;
#87300=CARTESIAN_POINT ( 'NONE',  ( -19.02544592524342804, 5.153800228976336051, 36.04057627198100988 ) ) ;
#87301=CARTESIAN_POINT ( 'NONE',  ( -8.224510206698735004, -14.34966873604973081, 49.58442372801901143 ) ) ;
#87303=CARTESIAN_POINT ( 'NONE',  ( 18.62759615963255655, 10.81492255796105972, 31.66775706135234358 ) ) ;
#87304=CARTESIAN_POINT ( 'NONE',  ( -16.52544592524342804, 4.483927247898546575, 61.04057627198103120 ) ) ;
#87306=CARTESIAN_POINT ( 'NONE',  ( -12.06949235617739369, -12.14591786802326823, 19.37609039468568639 ) ) ;
#87307=CARTESIAN_POINT ( 'NONE',  ( -19.03943276465977164, -0.05219959533935918106, 43.75109039468566863 ) ) ;
#87308=CARTESIAN_POINT ( 'NONE',  ( 14.34966873604960469, 8.224510206698951720, 59.16557627198103120 ) ) ;
#87309=CARTESIAN_POINT ( 'NONE',  ( -15.72974639402197994, 15.80617190586746368, 115.6239096053143669 ) ) ;
#87311=CARTESIAN_POINT ( 'NONE',  ( 21.52544592524344225, -5.823673210054117533, 83.54057627198102409 ) ) ;
#87312=CARTESIAN_POINT ( 'NONE',  ( 16.51473224551069308, 9.474510206698969483, 84.16557627198102409 ) ) ;
#87313=CARTESIAN_POINT ( 'NONE',  ( -16.52544592524342804, 4.483927247898546575, 56.04057627198102409 ) ) ;
#87314=CARTESIAN_POINT ( 'NONE',  ( 19.05341960407611168, 5.049401038298154454, 113.9572429386477097 ) ) ;
#87316=CARTESIAN_POINT ( 'NONE',  ( -0.05219959533936034679, 19.03943276465977164, 67.50109039468566152 ) ) ;
#87317=CARTESIAN_POINT ( 'NONE',  ( -15.80617190586745835, -15.72974639402198527, 106.8739096053143811 ) ) ;
#87318=CARTESIAN_POINT ( 'NONE',  ( -5.049401038298153566, 19.05341960407611168, 55.20724293864769550 ) ) ;
#87319=CARTESIAN_POINT ( 'NONE',  ( 5.049401038297881783, 19.05341960407617563, 42.29275706135234003 ) ) ;
#87320=CARTESIAN_POINT ( 'NONE',  ( 16.46253265017160672, -9.564922557960803928, 33.33224293864770260 ) ) ;
#87321=CARTESIAN_POINT ( 'NONE',  ( 5.719274019375673035, 21.55341960407619339, 62.29275706135236845 ) ) ;
#87322=CARTESIAN_POINT ( 'NONE',  ( -17.13100169013299734, -6.664070546373136672, 69.23210164300149927 ) ) ;
#87323=CARTESIAN_POINT ( 'NONE',  ( 4.379528057220339221, -16.55341960407611168, 42.70724293864770260 ) ) ;
#87324=CARTESIAN_POINT ( 'NONE',  ( 19.02544592524343514, -5.153800228976328945, 63.54057627198103830 ) ) ;
#87325=CARTESIAN_POINT ( 'NONE',  ( 21.52544592524344225, -5.823673210054117533, 68.54057627198103830 ) ) ;
#87326=CARTESIAN_POINT ( 'NONE',  ( 16.46253265017160672, -9.564922557960803928, 53.33224293864768839 ) ) ;
#87328=CARTESIAN_POINT ( 'NONE',  ( -21.52544592524343514, 5.823673210054127303, 61.04057627198103120 ) ) ;
#87329=CARTESIAN_POINT ( 'NONE',  ( 21.53943276465977519, 0.05219959533937863772, 106.2510903946856757 ) ) ;
#87331=CARTESIAN_POINT ( 'NONE',  ( 14.29746914071037800, 8.314922557961029526, 96.66775706135234714 ) ) ;
#87332=CARTESIAN_POINT ( 'NONE',  ( 4.483927247898545687, 16.52544592524342804, 84.79057627198102409 ) ) ;
#87333=CARTESIAN_POINT ( 'NONE',  ( -19.05341960407611168, -5.049401038298163336, 66.45724293864769550 ) ) ;
#87335=CARTESIAN_POINT ( 'NONE',  ( 19.02544592524334988, 5.153800228976608722, 36.45942372801900433 ) ) ;
#87336=CARTESIAN_POINT ( 'NONE',  ( -14.34966873604972548, 8.224510206698743886, 83.33442372801903275 ) ) ;
#87337=CARTESIAN_POINT ( 'NONE',  ( 9.564922557961047289, -16.46253265017146816, 30.41775706135232937 ) ) ;
#87338=CARTESIAN_POINT ( 'NONE',  ( 19.02544592524343514, -5.153800228976328945, 83.54057627198100988 ) ) ;
#87339=CARTESIAN_POINT ( 'NONE',  ( -5.719274019375978568, 21.55341960407610458, 60.20724293864768839 ) ) ;
#87341=CARTESIAN_POINT ( 'NONE',  ( 19.05341960407611168, 5.049401038298154454, 23.95724293864769194 ) ) ;
#87342=CARTESIAN_POINT ( 'NONE',  ( 21.55341960407619695, -5.719274019375665929, 96.04275706135236135 ) ) ;
#87343=CARTESIAN_POINT ( 'NONE',  ( -4.483927247898782831, 16.52544592524335698, 62.70942372801902565 ) ) ;
#87344=CARTESIAN_POINT ( 'NONE',  ( -18.62759615963255300, -10.81492255796106328, 34.16775706135234714 ) ) ;
#87345=CARTESIAN_POINT ( 'NONE',  ( -12.06949235617739369, -12.14591786802326823, 29.37609039468568284 ) ) ;
#87346=CARTESIAN_POINT ( 'NONE',  ( -9.564922557960796823, -16.46253265017161027, 97.08224293864769550 ) ) ;
#87347=CARTESIAN_POINT ( 'NONE',  ( 0.05219959533909260263, 19.03943276465977164, 44.99890960531435979 ) ) ;
#87348=CARTESIAN_POINT ( 'NONE',  ( -9.474510206698964154, 16.51473224551069663, 55.41557627198103120 ) ) ;
#87349=CARTESIAN_POINT ( 'NONE',  ( 4.483927247898790824, -16.52544592524335698, 35.20942372801901854 ) ) ;
#87350=CARTESIAN_POINT ( 'NONE',  ( 0.05219959533910956823, 16.53943276465976808, 89.99890960531438111 ) ) ;
#87351=CARTESIAN_POINT ( 'NONE',  ( -4.483927247898782831, 16.52544592524335698, 102.7094237280190185 ) ) ;
#87352=CARTESIAN_POINT ( 'NONE',  ( -0.05219959533937732626, 21.53943276465977519, 47.50109039468568994 ) ) ;
#87353=CARTESIAN_POINT ( 'NONE',  ( 13.97604488694527802, 13.89961937509977652, 79.37390960531435269 ) ) ;
#87354=CARTESIAN_POINT ( 'NONE',  ( 13.89961937509977652, -13.97604488694527269, 58.12390960531436690 ) ) ;
#87355=CARTESIAN_POINT ( 'NONE',  ( -5.049401038298153566, 19.05341960407611168, 80.20724293864769550 ) ) ;
#87356=CARTESIAN_POINT ( 'NONE',  ( -4.483927247898539470, -16.52544592524342804, 37.29057627198102409 ) ) ;
#87357=CARTESIAN_POINT ( 'NONE',  ( -14.29746914071037622, -8.314922557961029526, 104.1677570613523471 ) ) ;
#87359=CARTESIAN_POINT ( 'NONE',  ( 19.05341960407617918, -5.049401038297876454, 46.04275706135233293 ) ) ;
#87362=CARTESIAN_POINT ( 'NONE',  ( 13.97604488694527802, 13.89961937509977652, 44.37390960531435269 ) ) ;
#87363=CARTESIAN_POINT ( 'NONE',  ( -9.474510206698720793, -16.51473224551083518, 44.58442372801900433 ) ) ;
#87365=CARTESIAN_POINT ( 'NONE',  ( -8.314922557961024197, 14.29746914071037800, 47.91775706135234714 ) ) ;
#87366=CARTESIAN_POINT ( 'NONE',  ( -19.03943276465977164, -0.05219959533935918106, 73.75109039468566152 ) ) ;
#87367=CARTESIAN_POINT ( 'NONE',  ( -16.53943276465976808, -0.05219959533934237506, 58.75109039468568994 ) ) ;
#87368=CARTESIAN_POINT ( 'NONE',  ( -18.22780087662123805, 5.499999999999981348, 71.01763182126894947 ) ) ;
#87369=CARTESIAN_POINT ( 'NONE',  ( 9.474510206698971260, -16.51473224551069308, 82.91557627198103830 ) ) ;
#87370=CARTESIAN_POINT ( 'NONE',  ( 15.72974639402199770, -15.80617190586745480, 113.1239096053143953 ) ) ;
#87371=CARTESIAN_POINT ( 'NONE',  ( -0.05219959533936034679, 19.03943276465977164, 72.50109039468566152 ) ) ;
#87372=CARTESIAN_POINT ( 'NONE',  ( 9.474510206698971260, -16.51473224551069308, 107.9155762719810383 ) ) ;
#87373=CARTESIAN_POINT ( 'NONE',  ( 16.46253265017160672, -9.564922557960803928, 38.33224293864768839 ) ) ;
#87374=CARTESIAN_POINT ( 'NONE',  ( -19.05341960407611168, -5.049401038298163336, 76.45724293864769550 ) ) ;
#87375=CARTESIAN_POINT ( 'NONE',  ( 14.34966873604960469, 8.224510206698951720, 29.16557627198103120 ) ) ;
#87376=CARTESIAN_POINT ( 'NONE',  ( -13.89961937509977652, 13.97604488694528158, 30.62390960531435269 ) ) ;
#87377=CARTESIAN_POINT ( 'NONE',  ( -5.049401038297874678, -19.05341960407617918, 49.79275706135231871 ) ) ;
#87378=CARTESIAN_POINT ( 'NONE',  ( 4.379528057220339221, -16.55341960407611168, 67.70724293864769550 ) ) ;
#87379=CARTESIAN_POINT ( 'NONE',  ( -5.049401038297874678, -19.05341960407617918, 19.79275706135233293 ) ) ;
#87380=CARTESIAN_POINT ( 'NONE',  ( 5.049401038298161559, -19.05341960407611168, 57.70724293864769550 ) ) ;
#87381=CARTESIAN_POINT ( 'NONE',  ( 10.81492255796078972, 18.62759615963270932, 44.58224293864769550 ) ) ;
#87382=CARTESIAN_POINT ( 'NONE',  ( 16.55341960407611168, 4.379528057220329451, 58.95724293864770971 ) ) ;
#87383=CARTESIAN_POINT ( 'NONE',  ( 10.72451020669871369, 18.67979575497193778, 107.0844237280190043 ) ) ;
#87384=CARTESIAN_POINT ( 'NONE',  ( 16.46253265017160672, -9.564922557960803928, 98.33224293864769550 ) ) ;
#87385=CARTESIAN_POINT ( 'NONE',  ( 5.153800228976335163, 19.02544592524342804, 104.7905762719809957 ) ) ;
#87386=CARTESIAN_POINT ( 'NONE',  ( 13.89961937509977652, -13.97604488694527269, 43.12390960531434558 ) ) ;
#87387=CARTESIAN_POINT ( 'NONE',  ( -9.564922557960796823, -16.46253265017161027, 27.08224293864769550 ) ) ;
#87388=CARTESIAN_POINT ( 'NONE',  ( 16.53943276465976808, -0.05219959533910856209, 88.74890960531436690 ) ) ;
#87389=CARTESIAN_POINT ( 'NONE',  ( 15.80617190586746368, 15.72974639402197994, 99.37390960531436690 ) ) ;
#87390=CARTESIAN_POINT ( 'NONE',  ( 9.564922557960805705, 16.46253265017160317, 104.5822429386476955 ) ) ;
#87391=CARTESIAN_POINT ( 'NONE',  ( 21.55341960407610458, 5.719274019375980345, 113.9572429386477239 ) ) ;
#87392=CARTESIAN_POINT ( 'NONE',  ( -19.03943276465977164, 0.05219959533909376836, 96.24890960531436690 ) ) ;
#87393=DIRECTION ( 'NONE',  ( -0.000000000000000000, -0.000000000000000000, 1.000000000000000000 ) ) ;
#87394=CARTESIAN_POINT ( 'NONE',  ( 14.29746914071049879, -8.314922557960816363, 108.3322429386477097 ) ) ;
#87395=CARTESIAN_POINT ( 'NONE',  ( -13.89961937509977652, 13.97604488694528158, 70.62390960531432427 ) ) ;
#87396=CARTESIAN_POINT ( 'NONE',  ( 15.80617190586746368, 15.72974639402197994, 79.37390960531436690 ) ) ;
#87399=CARTESIAN_POINT ( 'NONE',  ( 21.53943276465977519, -0.05219959533907433946, 23.74890960531435269 ) ) ;
#87401=CARTESIAN_POINT ( 'NONE',  ( -12.06949235617739369, -12.14591786802326823, 34.37609039468568284 ) ) ;
#87402=CARTESIAN_POINT ( 'NONE',  ( 14.29746914071049879, -8.314922557960816363, 88.33224293864769550 ) ) ;
#87403=CARTESIAN_POINT ( 'NONE',  ( -17.49999999999997868, -4.640572885337623354, 109.3621183545115798 ) ) ;
#87404=CARTESIAN_POINT ( 'NONE',  ( 19.05341960407611168, 5.049401038298154454, 83.95724293864766707 ) ) ;
#87405=CARTESIAN_POINT ( 'NONE',  ( -0.05219959533909027116, -19.03943276465977164, 42.49890960531435269 ) ) ;
#87406=CARTESIAN_POINT ( 'NONE',  ( -16.55341960407611168, -4.379528057220339221, 76.45724293864769550 ) ) ;
#87407=CARTESIAN_POINT ( 'NONE',  ( -21.55341960407610458, -5.719274019375992779, 26.45724293864768839 ) ) ;
#87408=CARTESIAN_POINT ( 'NONE',  ( -4.379528057220328563, 16.55341960407611168, 50.20724293864769550 ) ) ;
#87409=CARTESIAN_POINT ( 'NONE',  ( 19.03943276465977164, 0.05219959533936151252, 101.2510903946856757 ) ) ;
#87410=CARTESIAN_POINT ( 'NONE',  ( -10.81492255796105439, 18.62759615963255655, 77.91775706135231871 ) ) ;
#87412=CARTESIAN_POINT ( 'NONE',  ( 0.05219959533909260263, 19.03943276465977164, 109.9989096053143669 ) ) ;
#87413=CARTESIAN_POINT ( 'NONE',  ( -4.379528057220086978, -16.55341960407618274, 84.79275706135234714 ) ) ;
#87414=DIRECTION ( 'NONE',  ( -0.000000000000000000, 1.000000000000000000, -0.000000000000000000 ) ) ;
#87415=CARTESIAN_POINT ( 'NONE',  ( -13.97604488694527625, -13.89961937509977652, 81.87390960531436690 ) ) ;
#87416=CARTESIAN_POINT ( 'NONE',  ( 0.05219959533907565091, 21.53943276465977519, 84.99890960531436690 ) ) ;
#87417=CARTESIAN_POINT ( 'NONE',  ( -4.379528057220086978, -16.55341960407618274, 24.79275706135235779 ) ) ;
#87418=CARTESIAN_POINT ( 'NONE',  ( 16.53943276465976808, -0.05219959533910856209, 53.74890960531437401 ) ) ;
#87419=CARTESIAN_POINT ( 'NONE',  ( -5.823673210054431948, 21.52544592524334988, 72.70942372801901854 ) ) ;
#87420=CARTESIAN_POINT ( 'NONE',  ( 16.53943276465976808, 0.05219959533934440121, 86.25109039468568994 ) ) ;
#87421=CARTESIAN_POINT ( 'NONE',  ( 18.67979575497178502, 10.72451020669898547, 29.16557627198103120 ) ) ;
#87422=CARTESIAN_POINT ( 'NONE',  ( 9.564922557960805705, 16.46253265017160317, 109.5822429386476955 ) ) ;
#87424=CARTESIAN_POINT ( 'NONE',  ( -14.34966873604972548, 8.224510206698743886, 103.3344237280190043 ) ) ;
#87425=CARTESIAN_POINT ( 'NONE',  ( -4.483927247898782831, 16.52544592524335698, 57.70942372801901143 ) ) ;
#87426=CARTESIAN_POINT ( 'NONE',  ( 19.02544592524343514, -5.153800228976328945, 73.54057627198103830 ) ) ;
#87427=CARTESIAN_POINT ( 'NONE',  ( -5.049401038298153566, 19.05341960407611168, 90.20724293864766707 ) ) ;
#87428=CARTESIAN_POINT ( 'NONE',  ( 10.72451020669871369, 18.67979575497193778, 72.08442372801899012 ) ) ;
#87429=CARTESIAN_POINT ( 'NONE',  ( -0.05219959533934338120, 16.53943276465976808, 82.50109039468568994 ) ) ;
#87430=CARTESIAN_POINT ( 'NONE',  ( -12.06949235617756955, 12.14591786802309770, 45.62390960531436690 ) ) ;
#87431=CARTESIAN_POINT ( 'NONE',  ( 9.564922557960805705, 16.46253265017160317, 59.58224293864769550 ) ) ;
#87432=CARTESIAN_POINT ( 'NONE',  ( -0.05219959533909027116, -19.03943276465977164, 42.49890960531435269 ) ) ;
#87434=CARTESIAN_POINT ( 'NONE',  ( -5.153800228976607833, 19.02544592524334988, 92.70942372801901854 ) ) ;
#87435=CARTESIAN_POINT ( 'NONE',  ( 4.379528057220339221, -16.55341960407611168, 92.70724293864770971 ) ) ;
#87436=CARTESIAN_POINT ( 'NONE',  ( -5.049401038298153566, 19.05341960407611168, 60.20724293864768129 ) ) ;
#87437=CARTESIAN_POINT ( 'NONE',  ( 5.153800228976615827, -19.02544592524334988, 100.2094237280190043 ) ) ;
#87439=CARTESIAN_POINT ( 'NONE',  ( -5.719274019375665041, -21.55341960407619695, 104.7927570613523898 ) ) ;
#87440=CARTESIAN_POINT ( 'NONE',  ( 4.483927247898790824, -16.52544592524335698, 65.20942372801901854 ) ) ;
#87441=CARTESIAN_POINT ( 'NONE',  ( -13.97604488694547697, 13.89961937509957934, 88.12609039468563310 ) ) ;
#87442=CARTESIAN_POINT ( 'NONE',  ( 5.719274019375991003, -21.55341960407610458, 67.70724293864769550 ) ) ;
#87443=CARTESIAN_POINT ( 'NONE',  ( -8.224510206698735004, -14.34966873604973081, 59.58442372801901854 ) ) ;
#87445=CARTESIAN_POINT ( 'NONE',  ( -16.46253265017146816, -9.564922557961047289, 59.16775706135233293 ) ) ;
#87446=CARTESIAN_POINT ( 'NONE',  ( 10.72451020669871369, 18.67979575497193778, 102.0844237280190185 ) ) ;
#87447=CARTESIAN_POINT ( 'NONE',  ( 8.314922557960818139, 14.29746914071049879, 114.5822429386477097 ) ) ;
#87448=CARTESIAN_POINT ( 'NONE',  ( -19.03943276465977164, 0.05219959533909376836, 66.24890960531436690 ) ) ;
#87449=CARTESIAN_POINT ( 'NONE',  ( 14.34966873604960469, 8.224510206698951720, 59.16557627198103120 ) ) ;
#87450=CARTESIAN_POINT ( 'NONE',  ( -21.53943276465977519, -0.05219959533937600094, 88.75109039468567573 ) ) ;
#87451=CARTESIAN_POINT ( 'NONE',  ( 9.474510206698729675, 16.51473224551082808, 42.08442372801900433 ) ) ;
#87452=CARTESIAN_POINT ( 'NONE',  ( -9.564922557961040184, 16.46253265017147172, 22.91775706135233648 ) ) ;
#87453=CARTESIAN_POINT ( 'NONE',  ( -0.05219959533909027116, -19.03943276465977164, 112.4989096053143669 ) ) ;
#87454=CARTESIAN_POINT ( 'NONE',  ( -21.55341960407619339, 5.719274019375674811, 98.54275706135234714 ) ) ;
#87455=CARTESIAN_POINT ( 'NONE',  ( -19.03943276465977164, 0.05219959533909376836, 81.24890960531436690 ) ) ;
#87456=CARTESIAN_POINT ( 'NONE',  ( 21.55341960407619695, -5.719274019375665929, 96.04275706135236135 ) ) ;
#87457=CARTESIAN_POINT ( 'NONE',  ( -0.05219959533907301413, -21.53943276465977519, 47.49890960531435979 ) ) ;
#87458=CARTESIAN_POINT ( 'NONE',  ( 19.03943276465977164, -0.05219959533909143690, 78.74890960531436690 ) ) ;
#87459=CARTESIAN_POINT ( 'NONE',  ( 16.46253265017146816, 9.564922557961045513, 66.66775706135233293 ) ) ;
#87460=CARTESIAN_POINT ( 'NONE',  ( -13.89961937509977652, 13.97604488694528158, 45.62390960531433848 ) ) ;
#87461=CARTESIAN_POINT ( 'NONE',  ( -19.03943276465977164, 0.05219959533909376836, 86.24890960531436690 ) ) ;
#87462=CARTESIAN_POINT ( 'NONE',  ( 13.89961937509957401, 13.97604488694547697, 86.87609039468567573 ) ) ;
#87463=CARTESIAN_POINT ( 'NONE',  ( -12.06949235617739369, -12.14591786802326823, 39.37609039468567573 ) ) ;
#87464=CARTESIAN_POINT ( 'NONE',  ( 0.05219959533910956823, 16.53943276465976808, 99.99890960531436690 ) ) ;
#87465=CARTESIAN_POINT ( 'NONE',  ( 13.89961937509977652, -13.97604488694527269, 73.12390960531436690 ) ) ;
#87466=CARTESIAN_POINT ( 'NONE',  ( 21.55341960407610458, 5.719274019375980345, 43.95724293864769550 ) ) ;
#87467=CARTESIAN_POINT ( 'NONE',  ( -19.05341960407617563, 5.049401038297882671, 113.5427570613523471 ) ) ;
#87468=CARTESIAN_POINT ( 'NONE',  ( 0.05219959533907565091, 21.53943276465977519, 114.9989096053143669 ) ) ;
#87469=CARTESIAN_POINT ( 'NONE',  ( -18.67979575497193778, 10.72451020669871902, 88.33442372801901854 ) ) ;
#87470=CARTESIAN_POINT ( 'NONE',  ( -14.34966873604972548, 8.224510206698743886, 78.33442372801901854 ) ) ;
#87471=CARTESIAN_POINT ( 'NONE',  ( -5.049401038298153566, 19.05341960407611168, 80.20724293864769550 ) ) ;
#87472=CARTESIAN_POINT ( 'NONE',  ( 16.55341960407618274, -4.379528057220086978, 106.0427570613523471 ) ) ;
#87473=CARTESIAN_POINT ( 'NONE',  ( 5.049401038297881783, 19.05341960407617563, 57.29275706135231871 ) ) ;
#87474=CARTESIAN_POINT ( 'NONE',  ( -18.62759615963255300, -10.81492255796106328, 34.16775706135234714 ) ) ;
#87475=CARTESIAN_POINT ( 'NONE',  ( -12.14591786802309592, -12.06949235617757132, 81.87390960531435269 ) ) ;
#87476=CARTESIAN_POINT ( 'NONE',  ( -5.049401038298153566, 19.05341960407611168, 100.2072429386476955 ) ) ;
#87477=CARTESIAN_POINT ( 'NONE',  ( -14.29746914071037622, -8.314922557961029526, 84.16775706135234714 ) ) ;
#87478=CARTESIAN_POINT ( 'NONE',  ( 5.823673210054444382, -21.52544592524334988, 70.20942372801904696 ) ) ;
#87479=CARTESIAN_POINT ( 'NONE',  ( 8.224510206698742110, 14.34966873604972548, 32.08442372801901854 ) ) ;
#87480=CARTESIAN_POINT ( 'NONE',  ( -15.80617190586768217, 15.72974639402176855, 28.12609039468568284 ) ) ;
#87481=CARTESIAN_POINT ( 'NONE',  ( 8.224510206698953496, -14.34966873604960469, 77.91557627198102409 ) ) ;
#87483=CARTESIAN_POINT ( 'NONE',  ( -15.80617190586745835, -15.72974639402198527, 96.87390960531436690 ) ) ;
#87484=CARTESIAN_POINT ( 'NONE',  ( 12.06949235617757843, -12.14591786802309237, 58.12390960531435979 ) ) ;
#87485=ORIENTED_EDGE ( 'NONE', *, *, #174158, .T. ) ;
#87486=CARTESIAN_POINT ( 'NONE',  ( 16.51473224551069308, 9.474510206698969483, 24.16557627198102765 ) ) ;
#87487=CARTESIAN_POINT ( 'NONE',  ( 18.62759615963271287, -10.81492255796078972, 23.33224293864769194 ) ) ;
#87488=CARTESIAN_POINT ( 'NONE',  ( 21.55341960407619695, -5.719274019375665929, 51.04275706135234714 ) ) ;
#87489=CARTESIAN_POINT ( 'NONE',  ( -16.53943276465976808, 0.05219959533911058130, 71.24890960531435269 ) ) ;
#87490=CARTESIAN_POINT ( 'NONE',  ( -21.55341960407610458, -5.719274019375992779, 61.45724293864770260 ) ) ;
#87491=CARTESIAN_POINT ( 'NONE',  ( 13.89961937509977652, -13.97604488694527269, 68.12390960531436690 ) ) ;
#87492=CARTESIAN_POINT ( 'NONE',  ( 13.97604488694527802, 13.89961937509977652, 29.37390960531435979 ) ) ;
#87493=CARTESIAN_POINT ( 'NONE',  ( -5.153800228976607833, 19.02544592524334988, 77.70942372801900433 ) ) ;
#87494=CARTESIAN_POINT ( 'NONE',  ( 15.72974639402199770, -15.80617190586745480, 68.12390960531436690 ) ) ;
#87495=CARTESIAN_POINT ( 'NONE',  ( 19.02544592524343514, -5.153800228976328945, 38.54057627198103120 ) ) ;
#87496=CARTESIAN_POINT ( 'NONE',  ( -19.03943276465977164, 0.05219959533909376836, 66.24890960531436690 ) ) ;
#87498=CARTESIAN_POINT ( 'NONE',  ( -8.314922557961024197, 14.29746914071037800, 47.91775706135234714 ) ) ;
#87499=CARTESIAN_POINT ( 'NONE',  ( 5.823673210054444382, -21.52544592524334988, 30.20942372801902565 ) ) ;
#87500=CARTESIAN_POINT ( 'NONE',  ( -15.72974639402176322, -15.80617190586768395, 54.37609039468568994 ) ) ;
#87501=CARTESIAN_POINT ( 'NONE',  ( 13.97604488694527802, 13.89961937509977652, 99.37390960531436690 ) ) ;
#87502=CARTESIAN_POINT ( 'NONE',  ( -21.55341960407610458, -5.719274019375992779, 91.45724293864769550 ) ) ;
#87503=CARTESIAN_POINT ( 'NONE',  ( 5.823673210054125526, 21.52544592524343514, 109.7905762719810383 ) ) ;
#87504=CARTESIAN_POINT ( 'NONE',  ( 16.52544592524335698, 4.483927247898782831, 56.45942372801902565 ) ) ;
#87505=CARTESIAN_POINT ( 'NONE',  ( -21.52544592524343514, 5.823673210054127303, 51.04057627198103120 ) ) ;
#87506=CARTESIAN_POINT ( 'NONE',  ( -10.72451020669870658, -18.67979575497194134, 99.58442372801900433 ) ) ;
#87507=CARTESIAN_POINT ( 'NONE',  ( 16.51473224551069308, 9.474510206698969483, 49.16557627198102409 ) ) ;
#87508=CARTESIAN_POINT ( 'NONE',  ( -5.049401038298153566, 19.05341960407611168, 105.2072429386476671 ) ) ;
#87509=CARTESIAN_POINT ( 'NONE',  ( 9.564922557960805705, 16.46253265017160317, 79.58224293864769550 ) ) ;
#87511=CARTESIAN_POINT ( 'NONE',  ( -0.05219959533936034679, 19.03943276465977164, 72.50109039468566152 ) ) ;
#87512=CARTESIAN_POINT ( 'NONE',  ( 21.53943276465977519, 0.05219959533937863772, 111.2510903946856899 ) ) ;
#87513=CARTESIAN_POINT ( 'NONE',  ( -21.52544592524343514, 5.823673210054127303, 41.04057627198103120 ) ) ;
#87514=CARTESIAN_POINT ( 'NONE',  ( 16.55341960407618274, -4.379528057220086978, 111.0427570613523613 ) ) ;
#87515=CARTESIAN_POINT ( 'NONE',  ( 9.564922557961047289, -16.46253265017146816, 90.41775706135234714 ) ) ;
#87517=CARTESIAN_POINT ( 'NONE',  ( -0.05219959533936034679, 19.03943276465977164, 22.50109039468566152 ) ) ;
#87518=CARTESIAN_POINT ( 'NONE',  ( -5.153800228976607833, 19.02544592524334988, 87.70942372801897591 ) ) ;
#87519=CARTESIAN_POINT ( 'NONE',  ( -13.97604488694547697, 13.89961937509957934, 38.12609039468566152 ) ) ;
#87520=CARTESIAN_POINT ( 'NONE',  ( -17.49999999999999645, -5.499999999999992895, 44.20309617465829888 ) ) ;
#87521=CARTESIAN_POINT ( 'NONE',  ( -5.049401038298153566, 19.05341960407611168, 60.20724293864768129 ) ) ;
#87522=CARTESIAN_POINT ( 'NONE',  ( 14.34966873604960469, 8.224510206698951720, 44.16557627198103120 ) ) ;
#87524=CARTESIAN_POINT ( 'NONE',  ( 19.05341960407611168, 5.049401038298154454, 28.95724293864769550 ) ) ;
#87525=CARTESIAN_POINT ( 'NONE',  ( -4.379528057220328563, 16.55341960407611168, 40.20724293864769550 ) ) ;
#87527=CARTESIAN_POINT ( 'NONE',  ( -14.29746914071037622, -8.314922557961029526, 109.1677570613523613 ) ) ;
#87528=CARTESIAN_POINT ( 'NONE',  ( -5.153800228976328057, -19.02544592524343514, 52.29057627198100988 ) ) ;
#87529=CARTESIAN_POINT ( 'NONE',  ( -5.049401038297874678, -19.05341960407617918, 19.79275706135233293 ) ) ;
#87530=CARTESIAN_POINT ( 'NONE',  ( 16.55341960407618274, -4.379528057220086978, 31.04275706135234714 ) ) ;
#87531=CARTESIAN_POINT ( 'NONE',  ( 21.55341960407610458, 5.719274019375980345, 38.95724293864768839 ) ) ;
#87532=CARTESIAN_POINT ( 'NONE',  ( 5.719274019375673035, 21.55341960407619339, 87.29275706135236135 ) ) ;
#87533=ORIENTED_EDGE ( 'NONE', *, *, #97920, .F. ) ;
#87534=CARTESIAN_POINT ( 'NONE',  ( -19.05341960407611168, -5.049401038298163336, 101.4572429386476955 ) ) ;
#87535=CARTESIAN_POINT ( 'NONE',  ( -5.153800228976328057, -19.02544592524343514, 102.2905762719810383 ) ) ;
#87537=CARTESIAN_POINT ( 'NONE',  ( -18.67979575497193778, 10.72451020669871902, 28.33442372801902209 ) ) ;
#87538=CARTESIAN_POINT ( 'NONE',  ( 4.483927247898545687, 16.52544592524342804, 79.79057627198102409 ) ) ;
#87539=CARTESIAN_POINT ( 'NONE',  ( 0.05219959533907565091, 21.53943276465977519, 69.99890960531435269 ) ) ;
#87540=CARTESIAN_POINT ( 'NONE',  ( 9.564922557960805705, 16.46253265017160317, 74.58224293864769550 ) ) ;
#87541=CARTESIAN_POINT ( 'NONE',  ( 19.03943276465977164, -0.05219959533909143690, 78.74890960531436690 ) ) ;
#87542=CARTESIAN_POINT ( 'NONE',  ( -0.05219959533907301413, -21.53943276465977519, 107.4989096053143669 ) ) ;
#87543=ORIENTED_EDGE ( 'NONE', *, *, #117399, .T. ) ;
#87544=CARTESIAN_POINT ( 'NONE',  ( 19.02544592524343514, -5.153800228976328945, 63.54057627198103830 ) ) ;
#87545=CARTESIAN_POINT ( 'NONE',  ( 14.34966873604960469, 8.224510206698951720, 104.1655762719810241 ) ) ;
#87547=CARTESIAN_POINT ( 'NONE',  ( 19.02544592524343514, -5.153800228976328945, 58.54057627198102409 ) ) ;
#87548=CARTESIAN_POINT ( 'NONE',  ( -13.97604488694547697, 13.89961937509957934, 88.12609039468563310 ) ) ;
#87549=CARTESIAN_POINT ( 'NONE',  ( -4.379528057220328563, 16.55341960407611168, 100.2072429386476955 ) ) ;
#87550=CARTESIAN_POINT ( 'NONE',  ( 0.05219959533937995610, -21.53943276465977519, 60.00109039468568284 ) ) ;
#87551=CARTESIAN_POINT ( 'NONE',  ( 5.049401038298161559, -19.05341960407611168, 42.70724293864767418 ) ) ;
#87552=CARTESIAN_POINT ( 'NONE',  ( -21.55341960407610458, -5.719274019375992779, 111.4572429386476813 ) ) ;
#87553=CARTESIAN_POINT ( 'NONE',  ( 16.52544592524342804, -4.483927247898539470, 103.5405762719810383 ) ) ;
#87555=CARTESIAN_POINT ( 'NONE',  ( -19.02544592524342804, 5.153800228976336051, 71.04057627198099567 ) ) ;
#87557=CARTESIAN_POINT ( 'NONE',  ( -19.02544592524334988, -5.153800228976617603, 108.9594237280189759 ) ) ;
#87558=CARTESIAN_POINT ( 'NONE',  ( 10.72451020669898902, -18.67979575497178502, 27.91557627198103830 ) ) ;
#87559=CARTESIAN_POINT ( 'NONE',  ( 15.80617190586769283, -15.72974639402175789, 45.62609039468567573 ) ) ;
#87560=CARTESIAN_POINT ( 'NONE',  ( -19.05341960407611168, -5.049401038298163336, 96.45724293864769550 ) ) ;
#87561=CARTESIAN_POINT ( 'NONE',  ( 0.05219959533936267826, -19.03943276465977164, 85.00109039468567573 ) ) ;
#87562=CARTESIAN_POINT ( 'NONE',  ( 19.02544592524343514, -5.153800228976328945, 73.54057627198103830 ) ) ;
#87563=CARTESIAN_POINT ( 'NONE',  ( -0.05219959533910754901, -16.53943276465976808, 87.49890960531436690 ) ) ;
#87564=CARTESIAN_POINT ( 'NONE',  ( 19.02544592524343514, -5.153800228976328945, 103.5405762719809957 ) ) ;
#87565=CARTESIAN_POINT ( 'NONE',  ( -14.34966873604960291, -8.224510206698953496, 76.66557627198103830 ) ) ;
#87566=CARTESIAN_POINT ( 'NONE',  ( -5.153800228976328057, -19.02544592524343514, 92.29057627198099567 ) ) ;
#87567=CARTESIAN_POINT ( 'NONE',  ( 5.049401038298161559, -19.05341960407611168, 47.70724293864770260 ) ) ;
#87568=CARTESIAN_POINT ( 'NONE',  ( -16.52544592524342804, 4.483927247898546575, 41.04057627198103120 ) ) ;
#87569=CARTESIAN_POINT ( 'NONE',  ( 19.03943276465977164, -0.05219959533909143690, 28.74890960531435624 ) ) ;
#87571=CARTESIAN_POINT ( 'NONE',  ( -18.67979575497193778, 10.72451020669871902, 48.33442372801902565 ) ) ;
#87572=CARTESIAN_POINT ( 'NONE',  ( -16.51473224551082808, 9.474510206698731452, 78.33442372801900433 ) ) ;
#87573=CARTESIAN_POINT ( 'NONE',  ( -8.224510206698948167, 14.34966873604960824, 55.41557627198102409 ) ) ;
#87574=CARTESIAN_POINT ( 'NONE',  ( 18.62759615963271287, -10.81492255796078972, 103.3322429386476955 ) ) ;
#87575=CARTESIAN_POINT ( 'NONE',  ( -10.72451020669898014, 18.67979575497178502, 35.41557627198102409 ) ) ;
#87576=CARTESIAN_POINT ( 'NONE',  ( 16.55341960407611168, 4.379528057220329451, 88.95724293864769550 ) ) ;
#87577=CARTESIAN_POINT ( 'NONE',  ( 5.049401038298161559, -19.05341960407611168, 47.70724293864770260 ) ) ;
#87578=CARTESIAN_POINT ( 'NONE',  ( 16.52544592524342804, -4.483927247898539470, 23.54057627198102765 ) ) ;
#87579=CARTESIAN_POINT ( 'NONE',  ( -16.53943276465976808, -0.05219959533934237506, 88.75109039468567573 ) ) ;
#87580=CARTESIAN_POINT ( 'NONE',  ( 12.14591786802327356, -12.06949235617739191, 65.62609039468568994 ) ) ;
#87581=CARTESIAN_POINT ( 'NONE',  ( -9.474510206698720793, -16.51473224551083518, 24.58442372801900078 ) ) ;
#87582=CARTESIAN_POINT ( 'NONE',  ( 9.564922557960805705, 16.46253265017160317, 89.58224293864769550 ) ) ;
#87583=CARTESIAN_POINT ( 'NONE',  ( -5.049401038298153566, 19.05341960407611168, 75.20724293864769550 ) ) ;
#87584=CARTESIAN_POINT ( 'NONE',  ( 12.06949235617739724, 12.14591786802326823, 76.87609039468567573 ) ) ;
#87585=CARTESIAN_POINT ( 'NONE',  ( -9.474510206698964154, 16.51473224551069663, 40.41557627198103120 ) ) ;
#87586=CARTESIAN_POINT ( 'NONE',  ( -16.52544592524342804, 4.483927247898546575, 46.04057627198103830 ) ) ;
#87588=CARTESIAN_POINT ( 'NONE',  ( 5.153800228976335163, 19.02544592524342804, 104.7905762719809957 ) ) ;
#87589=CARTESIAN_POINT ( 'NONE',  ( 18.62759615963271287, -10.81492255796078972, 28.33224293864769550 ) ) ;
#87590=CARTESIAN_POINT ( 'NONE',  ( 16.53943276465976808, -0.05219959533910856209, 68.74890960531435269 ) ) ;
#87591=CARTESIAN_POINT ( 'NONE',  ( -4.483927247898539470, -16.52544592524342804, 67.29057627198103830 ) ) ;
#87592=CARTESIAN_POINT ( 'NONE',  ( 17.50000000000001421, -3.189878218039136293, 32.37051437428772260 ) ) ;
#87593=CARTESIAN_POINT ( 'NONE',  ( -5.049401038297874678, -19.05341960407617918, 69.79275706135233293 ) ) ;
#87594=CARTESIAN_POINT ( 'NONE',  ( 13.89961937509977652, -13.97604488694527269, 88.12390960531438111 ) ) ;
#87595=CARTESIAN_POINT ( 'NONE',  ( -19.03943276465977164, -0.05219959533935918106, 78.75109039468567573 ) ) ;
#87597=CARTESIAN_POINT ( 'NONE',  ( 5.153800228976615827, -19.02544592524334988, 105.2094237280190185 ) ) ;
#87598=CARTESIAN_POINT ( 'NONE',  ( 4.379528057220092307, 16.55341960407617563, 102.2927570613523613 ) ) ;
#87599=CARTESIAN_POINT ( 'NONE',  ( 13.89961937509977652, -13.97604488694527269, 33.12390960531434558 ) ) ;
#87600=CARTESIAN_POINT ( 'NONE',  ( 15.80617190586746368, 15.72974639402197994, 39.37390960531436690 ) ) ;
#87601=CARTESIAN_POINT ( 'NONE',  ( 21.53943276465977519, 0.05219959533937863772, 61.25109039468567573 ) ) ;
#87602=CARTESIAN_POINT ( 'NONE',  ( -12.14591786802326823, 12.06949235617739902, 28.12609039468568284 ) ) ;
#87604=CARTESIAN_POINT ( 'NONE',  ( 19.05341960407611168, 5.049401038298154454, 78.95724293864769550 ) ) ;
#87606=CARTESIAN_POINT ( 'NONE',  ( 16.52544592524342804, -4.483927247898539470, 68.54057627198103830 ) ) ;
#87607=CARTESIAN_POINT ( 'NONE',  ( -9.564922557960796823, -16.46253265017161027, 77.08224293864769550 ) ) ;
#87608=CARTESIAN_POINT ( 'NONE',  ( 19.03943276465977164, -0.05219959533909143690, 78.74890960531436690 ) ) ;
#87610=CARTESIAN_POINT ( 'NONE',  ( -13.97604488694547697, 13.89961937509957934, 93.12609039468566152 ) ) ;
#87611=CARTESIAN_POINT ( 'NONE',  ( 15.72974639402199770, -15.80617190586745480, 58.12390960531435979 ) ) ;
#87612=CARTESIAN_POINT ( 'NONE',  ( -0.05219959533909027116, -19.03943276465977164, 32.49890960531435979 ) ) ;
#87613=CARTESIAN_POINT ( 'NONE',  ( 5.153800228976615827, -19.02544592524334988, 60.20942372801899012 ) ) ;
#87614=CARTESIAN_POINT ( 'NONE',  ( 9.474510206698971260, -16.51473224551069308, 57.91557627198103120 ) ) ;
#87615=CARTESIAN_POINT ( 'NONE',  ( 16.46253265017160672, -9.564922557960803928, 93.33224293864769550 ) ) ;
#87617=CARTESIAN_POINT ( 'NONE',  ( 21.53943276465977519, -0.05219959533907433946, 88.74890960531436690 ) ) ;
#87618=CARTESIAN_POINT ( 'NONE',  ( -0.05219959533910754901, -16.53943276465976808, 92.49890960531436690 ) ) ;
#87619=CARTESIAN_POINT ( 'NONE',  ( -16.46253265017146816, -9.564922557961047289, 44.16775706135232582 ) ) ;
#87620=CARTESIAN_POINT ( 'NONE',  ( 0.05219959533907565091, 21.53943276465977519, 89.99890960531438111 ) ) ;
#87621=CARTESIAN_POINT ( 'NONE',  ( -21.52544592524343514, 5.823673210054127303, 76.04057627198102409 ) ) ;
#87622=CARTESIAN_POINT ( 'NONE',  ( -8.314922557960811034, -14.29746914071050412, 32.08224293864769550 ) ) ;
#87623=CARTESIAN_POINT ( 'NONE',  ( 15.80617190586769283, -15.72974639402175789, 100.6260903946857184 ) ) ;
#87624=CARTESIAN_POINT ( 'NONE',  ( 16.51473224551069308, 9.474510206698969483, 74.16557627198103830 ) ) ;
#87625=CARTESIAN_POINT ( 'NONE',  ( 5.049401038298161559, -19.05341960407611168, 32.70724293864768129 ) ) ;
#87626=CARTESIAN_POINT ( 'NONE',  ( -5.823673210054431948, 21.52544592524334988, 42.70942372801901854 ) ) ;
#87627=CARTESIAN_POINT ( 'NONE',  ( 18.62759615963255655, 10.81492255796105972, 51.66775706135234714 ) ) ;
#87628=CARTESIAN_POINT ( 'NONE',  ( 19.05341960407611168, 5.049401038298154454, 48.95724293864768129 ) ) ;
#87629=CARTESIAN_POINT ( 'NONE',  ( 21.55341960407610458, 5.719274019375980345, 113.9572429386477239 ) ) ;
#87630=CARTESIAN_POINT ( 'NONE',  ( -5.049401038297874678, -19.05341960407617918, 59.79275706135231871 ) ) ;
#87631=CARTESIAN_POINT ( 'NONE',  ( -5.153800228976328057, -19.02544592524343514, 37.29057627198102409 ) ) ;
#87632=CARTESIAN_POINT ( 'NONE',  ( -12.06949235617739369, -12.14591786802326823, 24.37609039468567573 ) ) ;
#87633=CARTESIAN_POINT ( 'NONE',  ( 13.89961937509977652, -13.97604488694527269, 23.12390960531436335 ) ) ;
#87634=CARTESIAN_POINT ( 'NONE',  ( 4.483927247898790824, -16.52544592524335698, 75.20942372801901854 ) ) ;
#87635=CARTESIAN_POINT ( 'NONE',  ( -13.89961937509977652, 13.97604488694528158, 35.62390960531435269 ) ) ;
#87637=CARTESIAN_POINT ( 'NONE',  ( 19.02544592524343514, -5.153800228976328945, 83.54057627198100988 ) ) ;
#87638=CARTESIAN_POINT ( 'NONE',  ( 9.564922557960805705, 16.46253265017160317, 29.58224293864769550 ) ) ;
#87639=CARTESIAN_POINT ( 'NONE',  ( -18.62759615963270932, 10.81492255796079327, 70.83224293864770971 ) ) ;
#87640=CARTESIAN_POINT ( 'NONE',  ( 4.483927247898790824, -16.52544592524335698, 45.20942372801901854 ) ) ;
#87641=CARTESIAN_POINT ( 'NONE',  ( 21.55341960407619695, -5.719274019375665929, 111.0427570613523613 ) ) ;
#87642=CARTESIAN_POINT ( 'NONE',  ( 13.97604488694527802, 13.89961937509977652, 34.37390960531436690 ) ) ;
#87643=CARTESIAN_POINT ( 'NONE',  ( 12.06949235617757843, -12.14591786802309237, 28.12390960531435979 ) ) ;
#87644=CARTESIAN_POINT ( 'NONE',  ( 8.224510206698953496, -14.34966873604960469, 72.91557627198103830 ) ) ;
#87645=CARTESIAN_POINT ( 'NONE',  ( -19.03943276465977164, 0.05219959533909376836, 61.24890960531436690 ) ) ;
#87646=CARTESIAN_POINT ( 'NONE',  ( -19.03943276465977164, -0.05219959533935918106, 18.75109039468567218 ) ) ;
#87647=CARTESIAN_POINT ( 'NONE',  ( -21.53943276465977519, -0.05219959533937600094, 18.75109039468568639 ) ) ;
#87648=CARTESIAN_POINT ( 'NONE',  ( -16.46253265017160317, 9.564922557960807481, 85.83224293864769550 ) ) ;
#87649=CARTESIAN_POINT ( 'NONE',  ( -5.719274019375665041, -21.55341960407619695, 79.79275706135236135 ) ) ;
#87650=CARTESIAN_POINT ( 'NONE',  ( 14.29746914071037800, 8.314922557961029526, 61.66775706135235424 ) ) ;
#87651=EDGE_CURVE ( 'NONE', #99459, #9532, #127859, .T. ) ;
#87652=CARTESIAN_POINT ( 'NONE',  ( 13.97604488694527802, 13.89961937509977652, 104.3739096053143385 ) ) ;
#87653=CARTESIAN_POINT ( 'NONE',  ( -14.34966873604960291, -8.224510206698953496, 31.66557627198102054 ) ) ;
#87654=CARTESIAN_POINT ( 'NONE',  ( 5.049401038298161559, -19.05341960407611168, 27.70724293864769550 ) ) ;
#87655=CARTESIAN_POINT ( 'NONE',  ( -4.379528057220086978, -16.55341960407618274, 49.79275706135234714 ) ) ;
#87656=CARTESIAN_POINT ( 'NONE',  ( -16.52544592524342804, 4.483927247898546575, 51.04057627198103120 ) ) ;
#87657=CARTESIAN_POINT ( 'NONE',  ( -12.06949235617739369, -12.14591786802326823, 99.37609039468568994 ) ) ;
#87658=CARTESIAN_POINT ( 'NONE',  ( -9.564922557960796823, -16.46253265017161027, 112.0822429386476955 ) ) ;
#87659=CARTESIAN_POINT ( 'NONE',  ( 15.80617190586746368, 15.72974639402197994, 34.37390960531435979 ) ) ;
#87660=CARTESIAN_POINT ( 'NONE',  ( 18.62759615963255655, 10.81492255796105972, 111.6677570613523613 ) ) ;
#87661=CARTESIAN_POINT ( 'NONE',  ( -16.53943276465976808, 0.05219959533911058130, 86.24890960531436690 ) ) ;
#87662=CARTESIAN_POINT ( 'NONE',  ( -9.474510206698964154, 16.51473224551069663, 90.41557627198103830 ) ) ;
#87664=CARTESIAN_POINT ( 'NONE',  ( -12.06949235617739369, -12.14591786802326823, 44.37609039468567573 ) ) ;
#87665=CARTESIAN_POINT ( 'NONE',  ( 5.049401038298161559, -19.05341960407611168, 57.70724293864769550 ) ) ;
#87667=CARTESIAN_POINT ( 'NONE',  ( 5.153800228976615827, -19.02544592524334988, 50.20942372801897591 ) ) ;
#87668=CARTESIAN_POINT ( 'NONE',  ( 16.51473224551069308, 9.474510206698969483, 44.16557627198103120 ) ) ;
#87669=CARTESIAN_POINT ( 'NONE',  ( 8.314922557961029526, -14.29746914071037800, 75.41775706135233293 ) ) ;
#87670=CARTESIAN_POINT ( 'NONE',  ( -13.89961937509957401, -13.97604488694547875, 99.37609039468567573 ) ) ;
#87671=CARTESIAN_POINT ( 'NONE',  ( -18.67979575497193778, 10.72451020669871902, 68.33442372801900433 ) ) ;
#87672=CARTESIAN_POINT ( 'NONE',  ( 16.46253265017160672, -9.564922557960803928, 63.33224293864769550 ) ) ;
#87673=CARTESIAN_POINT ( 'NONE',  ( -21.55341960407610458, -5.719274019375992779, 91.45724293864769550 ) ) ;
#87674=CARTESIAN_POINT ( 'NONE',  ( 12.14591786802309770, 12.06949235617756955, 99.37390960531436690 ) ) ;
#87675=CARTESIAN_POINT ( 'NONE',  ( -19.02544592524334988, -5.153800228976617603, 68.95942372801896170 ) ) ;
#87676=CARTESIAN_POINT ( 'NONE',  ( -21.52544592524343514, 5.823673210054127303, 61.04057627198103120 ) ) ;
#87677=CARTESIAN_POINT ( 'NONE',  ( 13.89961937509957401, 13.97604488694547697, 41.87609039468566152 ) ) ;
#87678=CARTESIAN_POINT ( 'NONE',  ( 9.474510206698971260, -16.51473224551069308, 112.9155762719810383 ) ) ;
#87679=CARTESIAN_POINT ( 'NONE',  ( -15.80617190586745835, -15.72974639402198527, 96.87390960531436690 ) ) ;
#87680=CARTESIAN_POINT ( 'NONE',  ( -16.31925111598455658, 7.325300261831604764, 85.16424538967253000 ) ) ;
#87681=CARTESIAN_POINT ( 'NONE',  ( 13.89961937509957401, 13.97604488694547697, 101.8760903946856331 ) ) ;
#87682=CARTESIAN_POINT ( 'NONE',  ( 13.89961937509957579, 13.97604488694547520, 96.87609039468567573 ) ) ;
#87683=CARTESIAN_POINT ( 'NONE',  ( -16.53943276465976808, -0.05219959533934237506, 23.75109039468567929 ) ) ;
#87684=CARTESIAN_POINT ( 'NONE',  ( 5.049401038298161559, -19.05341960407611168, 52.70724293864767418 ) ) ;
#87685=CARTESIAN_POINT ( 'NONE',  ( 13.97604488694527802, 13.89961937509977652, 104.3739096053143385 ) ) ;
#87686=CARTESIAN_POINT ( 'NONE',  ( -5.719274019375978568, 21.55341960407610458, 90.20724293864770971 ) ) ;
#87687=CARTESIAN_POINT ( 'NONE',  ( -21.55341960407619339, 5.719274019375674811, 73.54275706135234714 ) ) ;
#87688=CARTESIAN_POINT ( 'NONE',  ( 16.55341960407618274, -4.379528057220086978, 26.04275706135235779 ) ) ;
#87689=CARTESIAN_POINT ( 'NONE',  ( 19.02544592524334988, 5.153800228976608722, 26.45942372801899722 ) ) ;
#87690=CARTESIAN_POINT ( 'NONE',  ( -14.29746914071049879, 8.314922557960819915, 30.83224293864770260 ) ) ;
#87691=CARTESIAN_POINT ( 'NONE',  ( 0.05219959533907565091, 21.53943276465977519, 114.9989096053143669 ) ) ;
#87692=CARTESIAN_POINT ( 'NONE',  ( -12.14591786802309592, -12.06949235617757132, 51.87390960531437401 ) ) ;
#87693=CARTESIAN_POINT ( 'NONE',  ( 0.05219959533936267826, -19.03943276465977164, 95.00109039468567573 ) ) ;
#87694=CARTESIAN_POINT ( 'NONE',  ( 19.02544592524334988, 5.153800228976608722, 61.45942372801900433 ) ) ;
#87695=CARTESIAN_POINT ( 'NONE',  ( -10.72451020669870658, -18.67979575497194134, 64.58442372801900433 ) ) ;
#87696=CARTESIAN_POINT ( 'NONE',  ( 16.51473224551083163, -9.474510206698727899, 45.83442372801900433 ) ) ;
#87697=CARTESIAN_POINT ( 'NONE',  ( 19.02544592524343514, -5.153800228976328945, 23.54057627198102054 ) ) ;
#87698=CARTESIAN_POINT ( 'NONE',  ( 5.719274019375991003, -21.55341960407610458, 37.70724293864769550 ) ) ;
#87699=CARTESIAN_POINT ( 'NONE',  ( -4.379528057220328563, 16.55341960407611168, 55.20724293864770260 ) ) ;
#87700=CARTESIAN_POINT ( 'NONE',  ( -16.46253265017146816, -9.564922557961047289, 19.16775706135233293 ) ) ;
#87701=CARTESIAN_POINT ( 'NONE',  ( 12.14591786802327356, -12.06949235617739191, 70.62609039468567573 ) ) ;
#87702=CARTESIAN_POINT ( 'NONE',  ( -16.53943276465976808, 0.05219959533911058130, 36.24890960531435979 ) ) ;
#87703=CARTESIAN_POINT ( 'NONE',  ( -21.55341960407619339, 5.719274019375674811, 73.54275706135234714 ) ) ;
#87704=CARTESIAN_POINT ( 'NONE',  ( -15.72974639402176322, -15.80617190586768395, 64.37609039468568994 ) ) ;
#87705=CARTESIAN_POINT ( 'NONE',  ( -15.80617190586745835, -15.72974639402198527, 81.87390960531435269 ) ) ;
#87706=CARTESIAN_POINT ( 'NONE',  ( -5.049401038298153566, 19.05341960407611168, 35.20724293864768839 ) ) ;
#87707=CARTESIAN_POINT ( 'NONE',  ( 0.05219959533937995610, -21.53943276465977519, 45.00109039468568284 ) ) ;
#87708=CARTESIAN_POINT ( 'NONE',  ( 9.474510206698971260, -16.51473224551069308, 22.91557627198102765 ) ) ;
#87709=CARTESIAN_POINT ( 'NONE',  ( -13.89961937509977652, 13.97604488694528158, 35.62390960531435269 ) ) ;
#87710=CARTESIAN_POINT ( 'NONE',  ( 8.224510206698953496, -14.34966873604960469, 97.91557627198103830 ) ) ;
#87711=CARTESIAN_POINT ( 'NONE',  ( 16.51473224551069308, 9.474510206698969483, 79.16557627198103830 ) ) ;
#87712=CARTESIAN_POINT ( 'NONE',  ( -14.34966873604960291, -8.224510206698953496, 36.66557627198103120 ) ) ;
#87713=CARTESIAN_POINT ( 'NONE',  ( -12.06949235617756955, 12.14591786802309770, 95.62390960531436690 ) ) ;
#87714=CARTESIAN_POINT ( 'NONE',  ( 10.81492255796078972, 18.62759615963270932, 64.58224293864769550 ) ) ;
#87715=CARTESIAN_POINT ( 'NONE',  ( 18.67979575497178502, 10.72451020669898547, 109.1655762719810383 ) ) ;
#87716=CARTESIAN_POINT ( 'NONE',  ( 5.153800228976335163, 19.02544592524342804, 114.7905762719810241 ) ) ;
#87718=CARTESIAN_POINT ( 'NONE',  ( -5.049401038298153566, 19.05341960407611168, 60.20724293864768129 ) ) ;
#87719=CARTESIAN_POINT ( 'NONE',  ( -14.29746914071037622, -8.314922557961029526, 29.16775706135234003 ) ) ;
#87720=CARTESIAN_POINT ( 'NONE',  ( 21.55341960407610458, 5.719274019375980345, 68.95724293864769550 ) ) ;
#87721=CARTESIAN_POINT ( 'NONE',  ( -5.719274019375665041, -21.55341960407619695, 89.79275706135236135 ) ) ;
#87722=CARTESIAN_POINT ( 'NONE',  ( -16.46253265017160317, 9.564922557960807481, 85.83224293864769550 ) ) ;
#87723=CARTESIAN_POINT ( 'NONE',  ( -18.62759615963270932, 10.81492255796079327, 115.8322429386477097 ) ) ;
#87724=CARTESIAN_POINT ( 'NONE',  ( -5.153800228976328057, -19.02544592524343514, 107.2905762719810383 ) ) ;
#87725=CARTESIAN_POINT ( 'NONE',  ( -14.29746914071037622, -8.314922557961029526, 94.16775706135237556 ) ) ;
#87726=CARTESIAN_POINT ( 'NONE',  ( 5.823673210054444382, -21.52544592524334988, 70.20942372801904696 ) ) ;
#87727=CARTESIAN_POINT ( 'NONE',  ( 5.823673210054444382, -21.52544592524334988, 100.2094237280190043 ) ) ;
#87728=CARTESIAN_POINT ( 'NONE',  ( -0.05219959533934338120, 16.53943276465976808, 62.50109039468568284 ) ) ;
#87729=CARTESIAN_POINT ( 'NONE',  ( 15.80617190586769283, -15.72974639402175789, 30.62609039468567929 ) ) ;
#87730=CARTESIAN_POINT ( 'NONE',  ( -13.97604488694527625, -13.89961937509977652, 111.8739096053143243 ) ) ;
#87731=CARTESIAN_POINT ( 'NONE',  ( 10.72451020669871369, 18.67979575497193778, 87.08442372801901854 ) ) ;
#87732=CARTESIAN_POINT ( 'NONE',  ( 0.05219959533909260263, 19.03943276465977164, 94.99890960531436690 ) ) ;
#87733=CARTESIAN_POINT ( 'NONE',  ( 5.823673210054125526, 21.52544592524343514, 94.79057627198105251 ) ) ;
#87734=CARTESIAN_POINT ( 'NONE',  ( 16.46253265017146816, 9.564922557961045513, 61.66775706135234003 ) ) ;
#87735=CARTESIAN_POINT ( 'NONE',  ( 10.81492255796078972, 18.62759615963270932, 49.58224293864769550 ) ) ;
#87736=CARTESIAN_POINT ( 'NONE',  ( 9.474510206698971260, -16.51473224551069308, 97.91557627198102409 ) ) ;
#87737=CARTESIAN_POINT ( 'NONE',  ( 16.52544592524342804, -4.483927247898539470, 33.54057627198102409 ) ) ;
#87739=CARTESIAN_POINT ( 'NONE',  ( -5.153800228976607833, 19.02544592524334988, 77.70942372801900433 ) ) ;
#87741=CARTESIAN_POINT ( 'NONE',  ( -9.474510206698720793, -16.51473224551083518, 109.5844237280190043 ) ) ;
#87742=CARTESIAN_POINT ( 'NONE',  ( -5.823673210054116645, -21.52544592524344225, 82.29057627198103830 ) ) ;
#87743=CARTESIAN_POINT ( 'NONE',  ( -14.34966873604960291, -8.224510206698953496, 66.66557627198102409 ) ) ;
#87744=CARTESIAN_POINT ( 'NONE',  ( -16.53943276465976808, -0.05219959533934237506, 28.75109039468567929 ) ) ;
#87745=CARTESIAN_POINT ( 'NONE',  ( -9.564922557960796823, -16.46253265017161027, 42.08224293864769550 ) ) ;
#87746=CARTESIAN_POINT ( 'NONE',  ( -10.72451020669898014, 18.67979575497178502, 115.4155762719810241 ) ) ;
#87747=CARTESIAN_POINT ( 'NONE',  ( 19.05341960407617918, -5.049401038297876454, 86.04275706135233293 ) ) ;
#87748=CARTESIAN_POINT ( 'NONE',  ( 13.97604488694527802, 13.89961937509977652, 89.37390960531436690 ) ) ;
#87749=CARTESIAN_POINT ( 'NONE',  ( 16.46253265017160672, -9.564922557960803928, 78.33224293864769550 ) ) ;
#87750=CARTESIAN_POINT ( 'NONE',  ( -21.52544592524343514, 5.823673210054127303, 76.04057627198102409 ) ) ;
#87751=CARTESIAN_POINT ( 'NONE',  ( -19.03943276465977164, 0.05219959533909376836, 51.24890960531436690 ) ) ;
#87753=CARTESIAN_POINT ( 'NONE',  ( 12.06949235617757843, -12.14591786802309237, 58.12390960531435979 ) ) ;
#87754=CARTESIAN_POINT ( 'NONE',  ( -16.46253265017160317, 9.564922557960807481, 85.83224293864769550 ) ) ;
#87756=CARTESIAN_POINT ( 'NONE',  ( -13.97604488694547697, 13.89961937509957934, 63.12609039468566152 ) ) ;
#87757=CARTESIAN_POINT ( 'NONE',  ( -0.05219959533907301413, -21.53943276465977519, 72.49890960531435269 ) ) ;
#87758=CARTESIAN_POINT ( 'NONE',  ( 5.153800228976615827, -19.02544592524334988, 35.20942372801899722 ) ) ;
#87759=CARTESIAN_POINT ( 'NONE',  ( 19.02544592524343514, -5.153800228976328945, 103.5405762719809957 ) ) ;
#87761=CARTESIAN_POINT ( 'NONE',  ( 21.53943276465977519, -0.05219959533907433946, 43.74890960531435979 ) ) ;
#87762=CARTESIAN_POINT ( 'NONE',  ( 13.89961937509977652, -13.97604488694527269, 78.12390960531433848 ) ) ;
#87763=CARTESIAN_POINT ( 'NONE',  ( 15.72974639402176855, 15.80617190586768217, 66.87609039468568994 ) ) ;
#87764=CARTESIAN_POINT ( 'NONE',  ( 0.05219959533909260263, 19.03943276465977164, 24.99890960531435269 ) ) ;
#87765=CARTESIAN_POINT ( 'NONE',  ( 21.53943276465977519, -0.05219959533907433946, 113.7489096053143527 ) ) ;
#87767=CARTESIAN_POINT ( 'NONE',  ( 21.55341960407619695, -5.719274019375665929, 56.04275706135235424 ) ) ;
#87769=DIRECTION ( 'NONE',  ( 1.000000000000000000, -0.000000000000000000, -0.000000000000000000 ) ) ;
#87770=CARTESIAN_POINT ( 'NONE',  ( -9.474510206698720793, -16.51473224551083518, 69.58442372801901854 ) ) ;
#87773=CARTESIAN_POINT ( 'NONE',  ( 21.55341960407610458, 5.719274019375980345, 103.9572429386476813 ) ) ;
#87774=CARTESIAN_POINT ( 'NONE',  ( -5.153800228976328057, -19.02544592524343514, 62.29057627198100988 ) ) ;
#87775=CARTESIAN_POINT ( 'NONE',  ( 16.53943276465976808, 0.05219959533934440121, 36.25109039468567573 ) ) ;
#87777=CARTESIAN_POINT ( 'NONE',  ( -0.05219959533937732626, 21.53943276465977519, 97.50109039468567573 ) ) ;
#87778=CARTESIAN_POINT ( 'NONE',  ( -19.02544592524342804, 5.153800228976336051, 36.04057627198100988 ) ) ;
#87779=CARTESIAN_POINT ( 'NONE',  ( 10.72451020669871369, 18.67979575497193778, 107.0844237280190043 ) ) ;
#87780=CARTESIAN_POINT ( 'NONE',  ( 16.46253265017160672, -9.564922557960803928, 83.33224293864768129 ) ) ;
#87781=CARTESIAN_POINT ( 'NONE',  ( -15.80617190586768217, 15.72974639402176855, 63.12609039468568994 ) ) ;
#87783=CARTESIAN_POINT ( 'NONE',  ( 13.89961937509977652, -13.97604488694527269, 108.1239096053143669 ) ) ;
#87785=CARTESIAN_POINT ( 'NONE',  ( 4.379528057220092307, 16.55341960407617563, 47.29275706135234003 ) ) ;
#87786=CARTESIAN_POINT ( 'NONE',  ( 21.53943276465977519, 0.05219959533937863772, 76.25109039468568994 ) ) ;
#87787=CARTESIAN_POINT ( 'NONE',  ( -0.05219959533937732626, 21.53943276465977519, 87.50109039468568994 ) ) ;
#87789=CARTESIAN_POINT ( 'NONE',  ( 4.379528057220092307, 16.55341960407617563, 22.29275706135235069 ) ) ;
#87790=CARTESIAN_POINT ( 'NONE',  ( 0.05219959533909260263, 19.03943276465977164, 84.99890960531436690 ) ) ;
#87791=CARTESIAN_POINT ( 'NONE',  ( 5.049401038298161559, -19.05341960407611168, 112.7072429386476813 ) ) ;
#87793=DIRECTION ( 'NONE',  ( -0.000000000000000000, -0.000000000000000000, 1.000000000000000000 ) ) ;
#87794=CARTESIAN_POINT ( 'NONE',  ( 0.05219959533910956823, 16.53943276465976808, 114.9989096053143669 ) ) ;
#87795=CARTESIAN_POINT ( 'NONE',  ( -21.55341960407610458, -5.719274019375992779, 46.45724293864769550 ) ) ;
#87796=CARTESIAN_POINT ( 'NONE',  ( 16.52544592524335698, 4.483927247898782831, 96.45942372801901854 ) ) ;
#87797=CARTESIAN_POINT ( 'NONE',  ( -4.379528057220328563, 16.55341960407611168, 80.20724293864769550 ) ) ;
#87798=CARTESIAN_POINT ( 'NONE',  ( -9.474510206698964154, 16.51473224551069663, 70.41557627198102409 ) ) ;
#87799=CARTESIAN_POINT ( 'NONE',  ( -10.72451020669870658, -18.67979575497194134, 89.58442372801901854 ) ) ;
#87800=CARTESIAN_POINT ( 'NONE',  ( -16.52544592524335698, -4.483927247898792601, 18.95942372801901143 ) ) ;
#87801=CARTESIAN_POINT ( 'NONE',  ( 4.379528057220339221, -16.55341960407611168, 87.70724293864769550 ) ) ;
#87802=CARTESIAN_POINT ( 'NONE',  ( -0.05219959533937732626, 21.53943276465977519, 42.50109039468567573 ) ) ;
#87803=CARTESIAN_POINT ( 'NONE',  ( 10.81492255796078972, 18.62759615963270932, 79.58224293864769550 ) ) ;
#87804=CARTESIAN_POINT ( 'NONE',  ( 19.05341960407617918, -5.049401038297876454, 41.04275706135233293 ) ) ;
#87805=CARTESIAN_POINT ( 'NONE',  ( -5.049401038298153566, 19.05341960407611168, 45.20724293864769550 ) ) ;
#87806=CARTESIAN_POINT ( 'NONE',  ( 16.51473224551069308, 9.474510206698969483, 79.16557627198103830 ) ) ;
#87807=CARTESIAN_POINT ( 'NONE',  ( 4.483927247898545687, 16.52544592524342804, 59.79057627198103120 ) ) ;
#87808=CARTESIAN_POINT ( 'NONE',  ( 8.224510206698953496, -14.34966873604960469, 37.91557627198102409 ) ) ;
#87809=CARTESIAN_POINT ( 'NONE',  ( -16.53943276465976808, -0.05219959533934237506, 108.7510903946857042 ) ) ;
#87810=CARTESIAN_POINT ( 'NONE',  ( 13.89961937509957401, 13.97604488694547697, 61.87609039468566863 ) ) ;
#87811=CARTESIAN_POINT ( 'NONE',  ( 19.52851543214742946, 5.500000000000025757, 52.89357721762586095 ) ) ;
#87812=CARTESIAN_POINT ( 'NONE',  ( 10.72451020669898902, -18.67979575497178502, 27.91557627198103830 ) ) ;
#87813=CARTESIAN_POINT ( 'NONE',  ( -16.55341960407611168, -4.379528057220339221, 81.45724293864769550 ) ) ;
#87814=CARTESIAN_POINT ( 'NONE',  ( 18.22780087662119897, -5.500000000000146549, 38.51763182126893525 ) ) ;
#87815=CARTESIAN_POINT ( 'NONE',  ( -5.049401038298153566, 19.05341960407611168, 45.20724293864769550 ) ) ;
#87816=CARTESIAN_POINT ( 'NONE',  ( -5.823673210054116645, -21.52544592524344225, 52.29057627198102409 ) ) ;
#87817=CARTESIAN_POINT ( 'NONE',  ( 10.72451020669898902, -18.67979575497178502, 67.91557627198102409 ) ) ;
#87818=CARTESIAN_POINT ( 'NONE',  ( -4.483927247898539470, -16.52544592524342804, 107.2905762719810525 ) ) ;
#87819=CARTESIAN_POINT ( 'NONE',  ( 8.314922557961029526, -14.29746914071037800, 60.41775706135235424 ) ) ;
#87820=CARTESIAN_POINT ( 'NONE',  ( -19.03943276465977164, 0.05219959533909376836, 41.24890960531435269 ) ) ;
#87821=CARTESIAN_POINT ( 'NONE',  ( -18.62759615963255300, -10.81492255796106328, 59.16775706135234714 ) ) ;
#87822=CARTESIAN_POINT ( 'NONE',  ( 8.224510206698953496, -14.34966873604960469, 107.9155762719810241 ) ) ;
#87823=CARTESIAN_POINT ( 'NONE',  ( -13.89961937509957401, -13.97604488694547875, 84.37609039468567573 ) ) ;
#87826=CARTESIAN_POINT ( 'NONE',  ( 21.52544592524344225, -5.823673210054117533, 43.54057627198103830 ) ) ;
#87827=CARTESIAN_POINT ( 'NONE',  ( 19.02544592524343514, -5.153800228976328945, 28.54057627198102409 ) ) ;
#87828=CARTESIAN_POINT ( 'NONE',  ( 0.05219959533937995610, -21.53943276465977519, 85.00109039468568994 ) ) ;
#87829=CARTESIAN_POINT ( 'NONE',  ( 16.53943276465976808, -0.05219959533910856209, 33.74890960531436690 ) ) ;
#87830=CARTESIAN_POINT ( 'NONE',  ( 14.34966873604972726, -8.224510206698740333, 50.83442372801901143 ) ) ;
#87831=CARTESIAN_POINT ( 'NONE',  ( -16.53943276465976808, 0.05219959533911058130, 46.24890960531435979 ) ) ;
#87832=CARTESIAN_POINT ( 'NONE',  ( 18.62759615963271287, -10.81492255796078972, 73.33224293864769550 ) ) ;
#87833=CARTESIAN_POINT ( 'NONE',  ( -10.72451020669898014, 18.67979575497178502, 80.41557627198103830 ) ) ;
#87835=CARTESIAN_POINT ( 'NONE',  ( -5.049401038297874678, -19.05341960407617918, 89.79275706135230450 ) ) ;
#87836=CARTESIAN_POINT ( 'NONE',  ( -19.03943276465977164, 0.05219959533909376836, 116.2489096053143669 ) ) ;
#87837=CARTESIAN_POINT ( 'NONE',  ( -19.02544592524342804, 5.153800228976336051, 46.04057627198101699 ) ) ;
#87838=CARTESIAN_POINT ( 'NONE',  ( -4.379528057220328563, 16.55341960407611168, 115.2072429386476955 ) ) ;
#87840=ORIENTED_EDGE ( 'NONE', *, *, #134567, .T. ) ;
#87841=CARTESIAN_POINT ( 'NONE',  ( 0.05219959533934541429, -16.53943276465976808, 80.00109039468568994 ) ) ;
#87842=CARTESIAN_POINT ( 'NONE',  ( -5.719274019375978568, 21.55341960407610458, 110.2072429386477239 ) ) ;
#87843=CARTESIAN_POINT ( 'NONE',  ( -0.05219959533909027116, -19.03943276465977164, 72.49890960531435269 ) ) ;
#87844=CARTESIAN_POINT ( 'NONE',  ( -5.719274019375665041, -21.55341960407619695, 34.79275706135235424 ) ) ;
#87845=CARTESIAN_POINT ( 'NONE',  ( -19.03943276465977164, 0.05219959533909376836, 101.2489096053143669 ) ) ;
#87848=CARTESIAN_POINT ( 'NONE',  ( 18.62759615963255655, 10.81492255796105972, 26.66775706135235424 ) ) ;
#87849=CARTESIAN_POINT ( 'NONE',  ( -5.049401038298153566, 19.05341960407611168, 25.20724293864768484 ) ) ;
#87850=CARTESIAN_POINT ( 'NONE',  ( 5.049401038297881783, 19.05341960407617563, 87.29275706135234714 ) ) ;
#87851=CARTESIAN_POINT ( 'NONE',  ( -19.05341960407617563, 5.049401038297882671, 38.54275706135233293 ) ) ;
#87852=CARTESIAN_POINT ( 'NONE',  ( 21.52544592524344225, -5.823673210054117533, 108.5405762719810241 ) ) ;
#87853=CARTESIAN_POINT ( 'NONE',  ( -13.89961937509957401, -13.97604488694547875, 39.37609039468566152 ) ) ;
#87854=CARTESIAN_POINT ( 'NONE',  ( -5.049401038297874678, -19.05341960407617918, 49.79275706135231871 ) ) ;
#87855=CARTESIAN_POINT ( 'NONE',  ( 12.06949235617739724, 12.14591786802326823, 91.87609039468568994 ) ) ;
#87858=CARTESIAN_POINT ( 'NONE',  ( 19.05341960407611168, 5.049401038298154454, 68.95724293864769550 ) ) ;
#87859=CARTESIAN_POINT ( 'NONE',  ( 5.823673210054444382, -21.52544592524334988, 75.20942372801901854 ) ) ;
#87860=CARTESIAN_POINT ( 'NONE',  ( -21.55341960407619339, 5.719274019375674811, 93.54275706135234714 ) ) ;
#87861=CARTESIAN_POINT ( 'NONE',  ( 17.50000000000000000, -5.499999999999992895, 66.21769037696435589 ) ) ;
#87862=CARTESIAN_POINT ( 'NONE',  ( 19.05341960407611168, 5.049401038298154454, 88.95724293864769550 ) ) ;
#87863=CARTESIAN_POINT ( 'NONE',  ( 0.05219959533937995610, -21.53943276465977519, 65.00109039468568994 ) ) ;
#87864=CARTESIAN_POINT ( 'NONE',  ( 19.03943276465977164, 0.05219959533936151252, 96.25109039468567573 ) ) ;
#87865=CARTESIAN_POINT ( 'NONE',  ( -16.46253265017160317, 9.564922557960807481, 60.83224293864769550 ) ) ;
#87866=CARTESIAN_POINT ( 'NONE',  ( 5.049401038298161559, -19.05341960407611168, 112.7072429386476813 ) ) ;
#87867=CARTESIAN_POINT ( 'NONE',  ( -9.474510206698964154, 16.51473224551069663, 75.41557627198103830 ) ) ;
#87868=CARTESIAN_POINT ( 'NONE',  ( -17.13100169013300444, -6.664070546373141113, 89.23210164300155611 ) ) ;
#87869=CARTESIAN_POINT ( 'NONE',  ( -9.474510206698964154, 16.51473224551069663, 65.41557627198102409 ) ) ;
#87870=CARTESIAN_POINT ( 'NONE',  ( -0.05219959533909027116, -19.03943276465977164, 47.49890960531435979 ) ) ;
#87871=CARTESIAN_POINT ( 'NONE',  ( 21.53943276465977519, 0.05219959533937863772, 21.25109039468567218 ) ) ;
#87872=CARTESIAN_POINT ( 'NONE',  ( 8.224510206698742110, 14.34966873604972548, 97.08442372801904696 ) ) ;
#87875=CARTESIAN_POINT ( 'NONE',  ( -13.89961937509957401, -13.97604488694547875, 59.37609039468566863 ) ) ;
#87876=CARTESIAN_POINT ( 'NONE',  ( 13.97604488694527802, 13.89961937509977652, 79.37390960531435269 ) ) ;
#87877=CARTESIAN_POINT ( 'NONE',  ( 4.483927247898545687, 16.52544592524342804, 74.79057627198105251 ) ) ;
#87878=CARTESIAN_POINT ( 'NONE',  ( 8.224510206698953496, -14.34966873604960469, 112.9155762719810383 ) ) ;
#87879=CARTESIAN_POINT ( 'NONE',  ( -21.55341960407610458, -5.719274019375992779, 31.45724293864769550 ) ) ;
#87880=CARTESIAN_POINT ( 'NONE',  ( 16.51473224551069308, 9.474510206698969483, 104.1655762719810241 ) ) ;
#87881=CARTESIAN_POINT ( 'NONE',  ( 16.55341960407611168, 4.379528057220329451, 93.95724293864770971 ) ) ;
#87882=CARTESIAN_POINT ( 'NONE',  ( 5.049401038298163336, -19.05341960407611168, 82.70724293864769550 ) ) ;
#87883=CARTESIAN_POINT ( 'NONE',  ( 0.05219959533936267826, -19.03943276465977164, 30.00109039468566863 ) ) ;
#87884=CARTESIAN_POINT ( 'NONE',  ( 8.224510206698742110, 14.34966873604972548, 112.0844237280190185 ) ) ;
#87885=CARTESIAN_POINT ( 'NONE',  ( -13.97604488694527625, -13.89961937509977652, 86.87390960531436690 ) ) ;
#87887=CARTESIAN_POINT ( 'NONE',  ( 10.72451020669871369, 18.67979575497193778, 47.08442372801901854 ) ) ;
#87888=CARTESIAN_POINT ( 'NONE',  ( 15.72974639402199770, -15.80617190586745480, 38.12390960531436690 ) ) ;
#87889=CARTESIAN_POINT ( 'NONE',  ( 18.67979575497194134, -10.72451020669871369, 25.83442372801901499 ) ) ;
#87891=CARTESIAN_POINT ( 'NONE',  ( -10.72451020669898014, 18.67979575497178502, 65.41557627198102409 ) ) ;
#87892=CARTESIAN_POINT ( 'NONE',  ( -14.34966873604960291, -8.224510206698953496, 91.66557627198103830 ) ) ;
#87893=CARTESIAN_POINT ( 'NONE',  ( -5.049401038297874678, -19.05341960407617918, 54.79275706135234003 ) ) ;
#87894=CARTESIAN_POINT ( 'NONE',  ( 13.89961937509977652, -13.97604488694527269, 33.12390960531434558 ) ) ;
#87895=CARTESIAN_POINT ( 'NONE',  ( 9.474510206698971260, -16.51473224551069308, 97.91557627198102409 ) ) ;
#87896=CARTESIAN_POINT ( 'NONE',  ( 13.97604488694527802, 13.89961937509977652, 94.37390960531436690 ) ) ;
#87897=CARTESIAN_POINT ( 'NONE',  ( 5.153800228976335163, 19.02544592524342804, 24.79057627198102765 ) ) ;
#87898=CARTESIAN_POINT ( 'NONE',  ( 14.34966873604960469, 8.224510206698951720, 29.16557627198103120 ) ) ;
#87899=CARTESIAN_POINT ( 'NONE',  ( -8.224510206698735004, -14.34966873604973081, 39.58442372801901143 ) ) ;
#87900=CARTESIAN_POINT ( 'NONE',  ( -21.53943276465977519, -0.05219959533937600094, 108.7510903946857042 ) ) ;
#87901=CARTESIAN_POINT ( 'NONE',  ( -16.51473224551069308, -9.474510206698971260, 96.66557627198102409 ) ) ;
#87902=CARTESIAN_POINT ( 'NONE',  ( 4.379528057220339221, -16.55341960407611168, 27.70724293864769905 ) ) ;
#87903=CARTESIAN_POINT ( 'NONE',  ( 21.52544592524334988, 5.823673210054432836, 31.45942372801901854 ) ) ;
#87904=CARTESIAN_POINT ( 'NONE',  ( 16.46253265017160672, -9.564922557960803928, 48.33224293864769550 ) ) ;
#87905=CARTESIAN_POINT ( 'NONE',  ( -14.34966873604972548, 8.224510206698743886, 48.33442372801902565 ) ) ;
#87906=CARTESIAN_POINT ( 'NONE',  ( -4.379528057220086978, -16.55341960407618274, 104.7927570613523898 ) ) ;
#87907=CARTESIAN_POINT ( 'NONE',  ( 16.53943276465976808, 0.05219959533934440121, 96.25109039468568994 ) ) ;
#87909=CARTESIAN_POINT ( 'NONE',  ( -13.89961937509957401, -13.97604488694547875, 109.3760903946856331 ) ) ;
#87910=CARTESIAN_POINT ( 'NONE',  ( -13.97604488694527625, -13.89961937509977652, 36.87390960531436690 ) ) ;
#87911=CARTESIAN_POINT ( 'NONE',  ( -16.53943276465976808, 0.05219959533911058130, 96.24890960531435269 ) ) ;
#87912=CARTESIAN_POINT ( 'NONE',  ( 10.72451020669898902, -18.67979575497178502, 107.9155762719810241 ) ) ;
#87913=CARTESIAN_POINT ( 'NONE',  ( -9.474510206698964154, 16.51473224551069663, 35.41557627198102409 ) ) ;
#87914=CARTESIAN_POINT ( 'NONE',  ( 5.049401038298161559, -19.05341960407611168, 107.7072429386476955 ) ) ;
#87915=CARTESIAN_POINT ( 'NONE',  ( 21.53943276465977519, 0.05219959533937863772, 31.25109039468568639 ) ) ;
#87917=CARTESIAN_POINT ( 'NONE',  ( -9.564922557960796823, -16.46253265017161027, 102.0822429386477097 ) ) ;
#87919=CARTESIAN_POINT ( 'NONE',  ( -16.46253265017160317, 9.564922557960807481, 80.83224293864769550 ) ) ;
#87920=CARTESIAN_POINT ( 'NONE',  ( 15.72974639402176855, 15.80617190586768217, 36.87609039468568994 ) ) ;
#87921=CARTESIAN_POINT ( 'NONE',  ( -16.55341960407611168, -4.379528057220339221, 96.45724293864770971 ) ) ;
#87922=CARTESIAN_POINT ( 'NONE',  ( 9.564922557960805705, 16.46253265017160317, 94.58224293864769550 ) ) ;
#87923=CARTESIAN_POINT ( 'NONE',  ( 9.564922557961047289, -16.46253265017146816, 20.41775706135233293 ) ) ;
#87924=CARTESIAN_POINT ( 'NONE',  ( -4.379528057220086978, -16.55341960407618274, 59.79275706135234714 ) ) ;
#87925=CARTESIAN_POINT ( 'NONE',  ( -15.80617190586768217, 15.72974639402176855, 83.12609039468568994 ) ) ;
#87926=CARTESIAN_POINT ( 'NONE',  ( 12.14591786802327356, -12.06949235617739191, 35.62609039468568994 ) ) ;
#87927=CARTESIAN_POINT ( 'NONE',  ( 0.05219959533909260263, 19.03943276465977164, 79.99890960531436690 ) ) ;
#87928=CARTESIAN_POINT ( 'NONE',  ( -13.97604488694547697, 13.89961937509957934, 98.12609039468566152 ) ) ;
#87929=CARTESIAN_POINT ( 'NONE',  ( 4.483927247898790824, -16.52544592524335698, 75.20942372801901854 ) ) ;
#87930=CARTESIAN_POINT ( 'NONE',  ( -18.67979575497193778, 10.72451020669871902, 113.3344237280190328 ) ) ;
#87931=CARTESIAN_POINT ( 'NONE',  ( 13.89961937509957401, 13.97604488694547697, 91.87609039468567573 ) ) ;
#87932=CARTESIAN_POINT ( 'NONE',  ( -16.51473224551069308, -9.474510206698971260, 61.66557627198103120 ) ) ;
#87933=CARTESIAN_POINT ( 'NONE',  ( 18.62759615963271287, -10.81492255796078972, 83.33224293864769550 ) ) ;
#87934=CARTESIAN_POINT ( 'NONE',  ( 12.14591786802309770, 12.06949235617756955, 89.37390960531435269 ) ) ;
#87935=CARTESIAN_POINT ( 'NONE',  ( -5.049401038297874678, -19.05341960407617918, 89.79275706135230450 ) ) ;
#87936=CARTESIAN_POINT ( 'NONE',  ( -12.14591786802326823, 12.06949235617739902, 58.12609039468568994 ) ) ;
#87937=CARTESIAN_POINT ( 'NONE',  ( -18.56453257813363678, 5.500000000000053291, 80.99000423690688422 ) ) ;
#87938=CARTESIAN_POINT ( 'NONE',  ( 16.46253265017146816, 9.564922557961045513, 61.66775706135234003 ) ) ;
#87939=CARTESIAN_POINT ( 'NONE',  ( 0.05219959533910956823, 16.53943276465976808, 29.99890960531435979 ) ) ;
#87940=CARTESIAN_POINT ( 'NONE',  ( -12.06949235617756955, 12.14591786802309770, 80.62390960531438111 ) ) ;
#87941=CARTESIAN_POINT ( 'NONE',  ( 16.46253265017146816, 9.564922557961045513, 21.66775706135233648 ) ) ;
#87942=CARTESIAN_POINT ( 'NONE',  ( -10.81492255796105439, 18.62759615963255655, 22.91775706135235069 ) ) ;
#87943=CARTESIAN_POINT ( 'NONE',  ( -19.03943276465977164, 0.05219959533909376836, 96.24890960531436690 ) ) ;
#87944=CARTESIAN_POINT ( 'NONE',  ( -19.02544592524342804, 5.153800228976336051, 76.04057627198102409 ) ) ;
#87945=CARTESIAN_POINT ( 'NONE',  ( 15.80617190586769283, -15.72974639402175789, 90.62609039468567573 ) ) ;
#87946=CARTESIAN_POINT ( 'NONE',  ( -13.89961937509977652, 13.97604488694528158, 60.62390960531436690 ) ) ;
#87948=CARTESIAN_POINT ( 'NONE',  ( -15.80617190586745835, -15.72974639402198527, 31.87390960531435979 ) ) ;
#87949=CARTESIAN_POINT ( 'NONE',  ( -16.55341960407611168, -4.379528057220339221, 81.45724293864769550 ) ) ;
#87950=CARTESIAN_POINT ( 'NONE',  ( 19.03943276465977164, -0.05219959533909143690, 43.74890960531435979 ) ) ;
#87951=CARTESIAN_POINT ( 'NONE',  ( 16.55341960407611168, 4.379528057220329451, 93.95724293864770971 ) ) ;
#87952=CARTESIAN_POINT ( 'NONE',  ( -10.81492255796078084, -18.62759615963271287, 112.0822429386477097 ) ) ;
#87953=CARTESIAN_POINT ( 'NONE',  ( 10.81492255796106328, -18.62759615963255655, 65.41775706135234714 ) ) ;
#87954=CARTESIAN_POINT ( 'NONE',  ( -16.51473224551069308, -9.474510206698971260, 26.66557627198103120 ) ) ;
#87956=CARTESIAN_POINT ( 'NONE',  ( -14.34966873604972548, 8.224510206698743886, 63.33442372801900433 ) ) ;
#87957=CARTESIAN_POINT ( 'NONE',  ( 0.05219959533907565091, 21.53943276465977519, 99.99890960531436690 ) ) ;
#87958=CARTESIAN_POINT ( 'NONE',  ( -15.72974639402176322, -15.80617190586768395, 19.37609039468568639 ) ) ;
#87959=CARTESIAN_POINT ( 'NONE',  ( -19.03943276465977164, -0.05219959533935918106, 43.75109039468566863 ) ) ;
#87960=CARTESIAN_POINT ( 'NONE',  ( 13.89961937509977652, -13.97604488694527269, 48.12390960531435979 ) ) ;
#87961=CARTESIAN_POINT ( 'NONE',  ( -9.474510206698964154, 16.51473224551069663, 115.4155762719810241 ) ) ;
#87962=CARTESIAN_POINT ( 'NONE',  ( 18.67979575497194134, -10.72451020669871369, 55.83442372801901854 ) ) ;
#87963=CARTESIAN_POINT ( 'NONE',  ( -5.823673210054116645, -21.52544592524344225, 57.29057627198103120 ) ) ;
#87964=CARTESIAN_POINT ( 'NONE',  ( 4.483927247898545687, 16.52544592524342804, 34.79057627198103120 ) ) ;
#87965=CARTESIAN_POINT ( 'NONE',  ( 0.05219959533937995610, -21.53943276465977519, 80.00109039468568994 ) ) ;
#87966=CARTESIAN_POINT ( 'NONE',  ( -15.72974639402176322, -15.80617190586768395, 104.3760903946856899 ) ) ;
#87967=CARTESIAN_POINT ( 'NONE',  ( 14.34966873604960469, 8.224510206698951720, 59.16557627198103120 ) ) ;
#87968=CARTESIAN_POINT ( 'NONE',  ( -4.379528057220328563, 16.55341960407611168, 105.2072429386477097 ) ) ;
#87969=CARTESIAN_POINT ( 'NONE',  ( 0.05219959533936267826, -19.03943276465977164, 40.00109039468566152 ) ) ;
#87970=CARTESIAN_POINT ( 'NONE',  ( -16.52544592524335698, -4.483927247898792601, 98.95942372801903275 ) ) ;
#87971=CARTESIAN_POINT ( 'NONE',  ( 21.55341960407619695, -5.719274019375665929, 66.04275706135236135 ) ) ;
#87972=CARTESIAN_POINT ( 'NONE',  ( -5.049401038298153566, 19.05341960407611168, 65.20724293864765286 ) ) ;
#87973=CARTESIAN_POINT ( 'NONE',  ( 19.05341960407617918, -5.049401038297876454, 36.04275706135234003 ) ) ;
#87974=CARTESIAN_POINT ( 'NONE',  ( 18.67979575497178502, 10.72451020669898547, 34.16557627198102409 ) ) ;
#87975=CARTESIAN_POINT ( 'NONE',  ( 5.719274019375673035, 21.55341960407619339, 32.29275706135235424 ) ) ;
#87976=CARTESIAN_POINT ( 'NONE',  ( 18.67979575497178502, 10.72451020669898547, 94.16557627198103830 ) ) ;
#87977=CARTESIAN_POINT ( 'NONE',  ( 0.05219959533936267826, -19.03943276465977164, 85.00109039468567573 ) ) ;
#87978=CARTESIAN_POINT ( 'NONE',  ( 12.14591786802327356, -12.06949235617739191, 55.62609039468568284 ) ) ;
#87980=CARTESIAN_POINT ( 'NONE',  ( -10.81492255796078084, -18.62759615963271287, 97.08224293864770971 ) ) ;
#87981=CARTESIAN_POINT ( 'NONE',  ( 12.14591786802309770, 12.06949235617756955, 79.37390960531436690 ) ) ;
#87983=CARTESIAN_POINT ( 'NONE',  ( -4.483927247898782831, 16.52544592524335698, 27.70942372801901854 ) ) ;
#87984=CARTESIAN_POINT ( 'NONE',  ( -18.67979575497178146, -10.72451020669898902, 41.66557627198103120 ) ) ;
#87985=CARTESIAN_POINT ( 'NONE',  ( -12.06949235617739369, -12.14591786802326823, 79.37609039468567573 ) ) ;
#87986=DIRECTION ( 'NONE',  ( -0.000000000000000000, -0.000000000000000000, -1.000000000000000000 ) ) ;
#87987=CARTESIAN_POINT ( 'NONE',  ( -4.483927247898782831, 16.52544592524335698, 52.70942372801902565 ) ) ;
#87988=CARTESIAN_POINT ( 'NONE',  ( 18.67979575497194134, -10.72451020669871369, 20.83442372801901143 ) ) ;
#87989=CARTESIAN_POINT ( 'NONE',  ( -5.823673210054116645, -21.52544592524344225, 47.29057627198103120 ) ) ;
#87990=CARTESIAN_POINT ( 'NONE',  ( 8.224510206698742110, 14.34966873604972548, 77.08442372801901854 ) ) ;
#87991=CARTESIAN_POINT ( 'NONE',  ( 16.51473224551069308, 9.474510206698969483, 84.16557627198102409 ) ) ;
#87992=CARTESIAN_POINT ( 'NONE',  ( 21.53943276465977519, 0.05219959533937863772, 51.25109039468568994 ) ) ;
#87993=CARTESIAN_POINT ( 'NONE',  ( 9.564922557960805705, 16.46253265017160317, 24.58224293864769194 ) ) ;
#87994=CARTESIAN_POINT ( 'NONE',  ( 21.52544592524344225, -5.823673210054117533, 38.54057627198103120 ) ) ;
#87995=CARTESIAN_POINT ( 'NONE',  ( 5.719274019375991003, -21.55341960407610458, 22.70724293864769194 ) ) ;
#87996=EDGE_LOOP ( 'NONE', ( #62706, #169589, #103661, #38623, #199402, #155209, #69693, #49053 ) ) ;
#87997=CARTESIAN_POINT ( 'NONE',  ( -5.153800228976607833, 19.02544592524334988, 37.70942372801899722 ) ) ;
#87998=CARTESIAN_POINT ( 'NONE',  ( -8.224510206698735004, -14.34966873604973081, 49.58442372801901143 ) ) ;
#87999=CARTESIAN_POINT ( 'NONE',  ( 19.02544592524343514, -5.153800228976328945, 108.5405762719810383 ) ) ;
#88001=CARTESIAN_POINT ( 'NONE',  ( -16.46253265017160317, 9.564922557960807481, 90.83224293864769550 ) ) ;
#88002=CARTESIAN_POINT ( 'NONE',  ( 12.06949235617739724, 12.14591786802326823, 101.8760903946857042 ) ) ;
#88004=CARTESIAN_POINT ( 'NONE',  ( 16.55341960407611168, 4.379528057220329451, 88.95724293864769550 ) ) ;
#88005=CARTESIAN_POINT ( 'NONE',  ( -18.67979575497178146, -10.72451020669898902, 51.66557627198102409 ) ) ;
#88006=CARTESIAN_POINT ( 'NONE',  ( 13.89961937509977652, -13.97604488694527269, 28.12390960531435624 ) ) ;
#88007=CARTESIAN_POINT ( 'NONE',  ( -16.53943276465976808, -0.05219959533934237506, 73.75109039468567573 ) ) ;
#88008=CARTESIAN_POINT ( 'NONE',  ( -15.72974639402197994, 15.80617190586746368, 115.6239096053143669 ) ) ;
#88009=CARTESIAN_POINT ( 'NONE',  ( -13.89961937509957401, -13.97604488694547875, 79.37609039468567573 ) ) ;
#88010=CARTESIAN_POINT ( 'NONE',  ( 9.564922557960805705, 16.46253265017160317, 34.58224293864770260 ) ) ;
#88011=CARTESIAN_POINT ( 'NONE',  ( -16.46253265017160317, 9.564922557960807481, 110.8322429386476955 ) ) ;
#88012=CARTESIAN_POINT ( 'NONE',  ( -15.80617190586768217, 15.72974639402176855, 108.1260903946856757 ) ) ;
#88013=CARTESIAN_POINT ( 'NONE',  ( -13.89961937509977652, 13.97604488694528158, 70.62390960531432427 ) ) ;
#88014=CARTESIAN_POINT ( 'NONE',  ( 0.05219959533934541429, -16.53943276465976808, 50.00109039468568994 ) ) ;
#88015=CARTESIAN_POINT ( 'NONE',  ( -18.67979575497193778, 10.72451020669871902, 88.33442372801901854 ) ) ;
#88016=CARTESIAN_POINT ( 'NONE',  ( -5.153800228976607833, 19.02544592524334988, 47.70942372801900433 ) ) ;
#88017=CARTESIAN_POINT ( 'NONE',  ( -16.51473224551082808, 9.474510206698731452, 58.33442372801900433 ) ) ;
#88019=CARTESIAN_POINT ( 'NONE',  ( -5.719274019375665041, -21.55341960407619695, 54.79275706135235424 ) ) ;
#88020=CARTESIAN_POINT ( 'NONE',  ( -19.03943276465977164, 0.05219959533909376836, 21.24890960531436335 ) ) ;
#88021=CARTESIAN_POINT ( 'NONE',  ( -16.46253265017146816, -9.564922557961047289, 44.16775706135232582 ) ) ;
#88022=CARTESIAN_POINT ( 'NONE',  ( -16.46253265017160317, 9.564922557960807481, 95.83224293864769550 ) ) ;
#88023=CARTESIAN_POINT ( 'NONE',  ( -13.97604488694527625, -13.89961937509977652, 86.87390960531436690 ) ) ;
#88024=CARTESIAN_POINT ( 'NONE',  ( -8.314922557960811034, -14.29746914071050412, 42.08224293864769550 ) ) ;
#88025=CARTESIAN_POINT ( 'NONE',  ( -21.55341960407610458, -5.719274019375992779, 31.45724293864769550 ) ) ;
#88028=CARTESIAN_POINT ( 'NONE',  ( 5.719274019375673035, 21.55341960407619339, 107.2927570613523471 ) ) ;
#88030=CARTESIAN_POINT ( 'NONE',  ( 16.51473224551069308, 9.474510206698969483, 39.16557627198103120 ) ) ;
#88031=CARTESIAN_POINT ( 'NONE',  ( -9.474510206698964154, 16.51473224551069663, 85.41557627198102409 ) ) ;
#88032=CARTESIAN_POINT ( 'NONE',  ( -17.60728821186568283, 5.500000000000041744, 80.86690927743008217 ) ) ;
#88034=CARTESIAN_POINT ( 'NONE',  ( -8.224510206698735004, -14.34966873604973081, 59.58442372801901854 ) ) ;
#88035=CARTESIAN_POINT ( 'NONE',  ( 15.80617190586746368, 15.72974639402197994, 89.37390960531435269 ) ) ;
#88036=CARTESIAN_POINT ( 'NONE',  ( -14.34966873604960291, -8.224510206698953496, 56.66557627198103830 ) ) ;
#88037=CARTESIAN_POINT ( 'NONE',  ( -9.564922557960796823, -16.46253265017161027, 22.08224293864768839 ) ) ;
#88038=CARTESIAN_POINT ( 'NONE',  ( -0.05219959533909027116, -19.03943276465977164, 112.4989096053143669 ) ) ;
#88039=CARTESIAN_POINT ( 'NONE',  ( -10.81492255796105439, 18.62759615963255655, 22.91775706135235069 ) ) ;
#88040=CARTESIAN_POINT ( 'NONE',  ( 13.89961937509957401, 13.97604488694547697, 36.87609039468565442 ) ) ;
#88041=CARTESIAN_POINT ( 'NONE',  ( 19.03943276465977164, -0.05219959533909143690, 38.74890960531436690 ) ) ;
#88042=CARTESIAN_POINT ( 'NONE',  ( -21.53943276465977519, -0.05219959533937600094, 78.75109039468568994 ) ) ;
#88043=CARTESIAN_POINT ( 'NONE',  ( 16.29526858892873165, -7.335722546920260712, 31.70329402199793734 ) ) ;
#88044=CARTESIAN_POINT ( 'NONE',  ( 14.34966873604960469, 8.224510206698951720, 24.16557627198103120 ) ) ;
#88045=CARTESIAN_POINT ( 'NONE',  ( 17.50000000000000000, -5.499999999999992895, 101.2176903769643559 ) ) ;
#88046=CARTESIAN_POINT ( 'NONE',  ( -18.67979575497178146, -10.72451020669898902, 46.66557627198102409 ) ) ;
#88047=CARTESIAN_POINT ( 'NONE',  ( -16.53943276465976808, 0.05219959533911058130, 101.2489096053143669 ) ) ;
#88048=CARTESIAN_POINT ( 'NONE',  ( -18.09867054820433907, -5.499999999999827693, 38.98393025253586330 ) ) ;
#88049=CARTESIAN_POINT ( 'NONE',  ( -9.474510206698964154, 16.51473224551069663, 85.41557627198102409 ) ) ;
#88050=CARTESIAN_POINT ( 'NONE',  ( 16.53943276465976808, -0.05219959533910856209, 73.74890960531433848 ) ) ;
#88051=CARTESIAN_POINT ( 'NONE',  ( -9.564922557961040184, 16.46253265017147172, 107.9177570613523471 ) ) ;
#88052=CARTESIAN_POINT ( 'NONE',  ( 21.53943276465977519, -0.05219959533907433946, 58.74890960531436690 ) ) ;
#88054=CARTESIAN_POINT ( 'NONE',  ( -0.05219959533909027116, -19.03943276465977164, 32.49890960531435979 ) ) ;
#88055=ADVANCED_FACE ( 'NONE', ( #149046 ), #893, .T. ) ;
#88056=CARTESIAN_POINT ( 'NONE',  ( -13.97604488694527625, -13.89961937509977652, 91.87390960531432427 ) ) ;
#88057=CARTESIAN_POINT ( 'NONE',  ( 21.55341960407610458, 5.719274019375980345, 88.95724293864769550 ) ) ;
#88058=CARTESIAN_POINT ( 'NONE',  ( -0.05219959533934338120, 16.53943276465976808, 102.5010903946856899 ) ) ;
#88059=CARTESIAN_POINT ( 'NONE',  ( 19.03943276465977164, -0.05219959533909143690, 93.74890960531435269 ) ) ;
#88060=CARTESIAN_POINT ( 'NONE',  ( -16.46253265017146816, -9.564922557961047289, 84.16775706135233293 ) ) ;
#88061=CARTESIAN_POINT ( 'NONE',  ( 5.823673210054444382, -21.52544592524334988, 100.2094237280190043 ) ) ;
#88062=CARTESIAN_POINT ( 'NONE',  ( 21.53943276465977519, -0.05219959533907433946, 73.74890960531433848 ) ) ;
#88063=CARTESIAN_POINT ( 'NONE',  ( 5.719274019375991003, -21.55341960407610458, 42.70724293864770260 ) ) ;
#88064=CARTESIAN_POINT ( 'NONE',  ( 9.564922557960805705, 16.46253265017160317, 44.58224293864769550 ) ) ;
#88065=CARTESIAN_POINT ( 'NONE',  ( -4.483927247898539470, -16.52544592524342804, 22.29057627198102765 ) ) ;
#88066=CARTESIAN_POINT ( 'NONE',  ( 5.049401038298161559, -19.05341960407611168, 62.70724293864769550 ) ) ;
#88067=ORIENTED_EDGE ( 'NONE', *, *, #95479, .T. ) ;
#88069=CARTESIAN_POINT ( 'NONE',  ( -19.03943276465977164, -0.05219959533935918106, 33.75109039468566863 ) ) ;
#88070=CARTESIAN_POINT ( 'NONE',  ( 0.05219959533910956823, 16.53943276465976808, 74.99890960531435269 ) ) ;
#88071=( BOUNDED_CURVE ( )  B_SPLINE_CURVE ( 2, ( #8680, #113832, #98663, #70352, #189713, #160357, #21847, #101675, #131007, #54182, #132019, #83498, #115855 ),
 .UNSPECIFIED., .F., .F. ) 
 B_SPLINE_CURVE_WITH_KNOTS ( ( 3, 2, 2, 2, 2, 2, 3 ),
 ( 0.6340550636175563692, 0.6359649122807017330, 0.6403508771929824483, 0.6447368421052631637, 0.6491228070175438791, 0.6535087719298245945, 0.6554643004150603192 ),
 .UNSPECIFIED. ) 
 CURVE ( )  GEOMETRIC_REPRESENTATION_ITEM ( )  RATIONAL_B_SPLINE_CURVE ( ( 0.9832469066685285419, 0.9851625545550100060, 1.000000000000000000, 0.9659258262890683122, 1.000000000000000000, 0.9659258262890683122, 1.000000000000000000, 0.9659258262890683122, 1.000000000000000000, 0.9659258262890683122, 1.000000000000000000, 0.9848076720550078544, 0.9831626618144001517 ) ) 
 REPRESENTATION_ITEM ( '' )  );
#88072=CARTESIAN_POINT ( 'NONE',  ( -15.72974639402176322, -15.80617190586768395, 29.37609039468568284 ) ) ;
#88074=CARTESIAN_POINT ( 'NONE',  ( 18.62759615963271287, -10.81492255796078972, 53.33224293864769550 ) ) ;
#88075=CARTESIAN_POINT ( 'NONE',  ( -16.53943276465976808, -0.05219959533934237506, 98.75109039468568994 ) ) ;
#88076=CARTESIAN_POINT ( 'NONE',  ( -12.14591786802309592, -12.06949235617757132, 101.8739096053143811 ) ) ;
#88077=CARTESIAN_POINT ( 'NONE',  ( 9.474510206698971260, -16.51473224551069308, 67.91557627198102409 ) ) ;
#88079=CARTESIAN_POINT ( 'NONE',  ( 16.55341960407611168, 4.379528057220329451, 23.95724293864769550 ) ) ;
#88080=CARTESIAN_POINT ( 'NONE',  ( -0.05219959533937732626, 21.53943276465977519, 47.50109039468568994 ) ) ;
#88081=CARTESIAN_POINT ( 'NONE',  ( 13.97604488694527802, 13.89961937509977652, 114.3739096053143669 ) ) ;
#88082=CARTESIAN_POINT ( 'NONE',  ( -5.719274019375665041, -21.55341960407619695, 74.79275706135234714 ) ) ;
#88083=CARTESIAN_POINT ( 'NONE',  ( -0.05219959533909027116, -19.03943276465977164, 32.49890960531435979 ) ) ;
#88084=CARTESIAN_POINT ( 'NONE',  ( -9.564922557960796823, -16.46253265017161027, 37.08224293864768839 ) ) ;
#88086=CARTESIAN_POINT ( 'NONE',  ( 18.67979575497194134, -10.72451020669871369, 95.83442372801903275 ) ) ;
#88087=CARTESIAN_POINT ( 'NONE',  ( -8.224510206698735004, -14.34966873604973081, 49.58442372801901143 ) ) ;
#88088=CARTESIAN_POINT ( 'NONE',  ( 5.719274019375673035, 21.55341960407619339, 72.29275706135236135 ) ) ;
#88089=CARTESIAN_POINT ( 'NONE',  ( -0.05219959533909027116, -19.03943276465977164, 97.49890960531436690 ) ) ;
#88090=CARTESIAN_POINT ( 'NONE',  ( -19.02544592524334988, -5.153800228976617603, 78.95942372801900433 ) ) ;
#88091=CARTESIAN_POINT ( 'NONE',  ( -10.81492255796105439, 18.62759615963255655, 52.91775706135235424 ) ) ;
#88092=CARTESIAN_POINT ( 'NONE',  ( 16.46253265017146816, 9.564922557961045513, 111.6677570613523329 ) ) ;
#88093=CARTESIAN_POINT ( 'NONE',  ( 13.89961937509957401, 13.97604488694547697, 86.87609039468567573 ) ) ;
#88094=CARTESIAN_POINT ( 'NONE',  ( 19.03943276465977164, -0.05219959533909143690, 53.74890960531436690 ) ) ;
#88095=CARTESIAN_POINT ( 'NONE',  ( -9.564922557961040184, 16.46253265017147172, 77.91775706135234714 ) ) ;
#88096=CARTESIAN_POINT ( 'NONE',  ( 16.53943276465976808, -0.05219959533910856209, 28.74890960531435624 ) ) ;
#88097=CARTESIAN_POINT ( 'NONE',  ( 19.02544592524334988, 5.153800228976608722, 91.45942372801900433 ) ) ;
#88098=CARTESIAN_POINT ( 'NONE',  ( -16.55341960407611168, -4.379528057220339221, 41.45724293864769550 ) ) ;
#88099=CARTESIAN_POINT ( 'NONE',  ( -5.153800228976607833, 19.02544592524334988, 62.70942372801899722 ) ) ;
#88100=B_SPLINE_CURVE_WITH_KNOTS ( 'NONE', 3,
 ( #138542, #135591, #120394, #107205, #198244, #76872, #185056, #59717, #121389, #183081, #106219, #167903, #29403, #199237, #169885, #108204, #91033, #14210, #109201, #51509, #2022, #21168, #191022, #3019, #33363, #64696, #170880, #171874, #95022, #67669, #66673, #174859 ),
 .UNSPECIFIED., .F., .F.,
 ( 4, 2, 2, 2, 2, 2, 2, 2, 2, 2, 2, 2, 2, 2, 2, 4 ),
 ( 2.539163526713095107E-17, 0.0003712461730036967526, 0.0007424923460073681349, 0.001113738519011039626, 0.001484984692014710899, 0.002227477038022051929, 0.002598723211025729708, 0.002969969384029407054, 0.003341215557033084399, 0.003712461730036761744, 0.004083707903040438222, 0.004454954076044116001, 0.004826200249047792913, 0.005197446422051470692, 0.005568692595055147604, 0.005939938768058825383 ),
 .UNSPECIFIED. ) ;
#88101=CARTESIAN_POINT ( 'NONE',  ( -16.53943276465976808, -0.05219959533934237506, 53.75109039468568994 ) ) ;
#88102=CARTESIAN_POINT ( 'NONE',  ( -13.97604488694547697, 13.89961937509957934, 23.12609039468565442 ) ) ;
#88103=CARTESIAN_POINT ( 'NONE',  ( 16.46253265017160672, -9.564922557960803928, 23.33224293864769194 ) ) ;
#88104=CARTESIAN_POINT ( 'NONE',  ( 5.049401038298161559, -19.05341960407611168, 37.70724293864768839 ) ) ;
#88105=CARTESIAN_POINT ( 'NONE',  ( -12.06949235617739369, -12.14591786802326823, 49.37609039468569705 ) ) ;
#88106=CARTESIAN_POINT ( 'NONE',  ( 17.50000000000000000, 5.499999999999995559, 113.7823096230356583 ) ) ;
#88109=CARTESIAN_POINT ( 'NONE',  ( 13.97604488694527802, 13.89961937509977652, 89.37390960531436690 ) ) ;
#88110=CARTESIAN_POINT ( 'NONE',  ( 17.69326672847916271, 2.167987141922683492, 102.5000000000000284 ) ) ;
#88111=VERTEX_POINT ( 'NONE', #22170 ) ;
#88112=CARTESIAN_POINT ( 'NONE',  ( -5.049401038297874678, -19.05341960407617918, 94.79275706135230450 ) ) ;
#88113=CARTESIAN_POINT ( 'NONE',  ( 19.03943276465977164, -0.05219959533909143690, 113.7489096053143669 ) ) ;
#88114=CARTESIAN_POINT ( 'NONE',  ( 13.97604488694548053, -13.89961937509957401, 30.62609039468566863 ) ) ;
#88115=CARTESIAN_POINT ( 'NONE',  ( 14.34966873604972726, -8.224510206698740333, 20.83442372801901143 ) ) ;
#88116=CARTESIAN_POINT ( 'NONE',  ( -4.379528057220328563, 16.55341960407611168, 105.2072429386477097 ) ) ;
#88117=CARTESIAN_POINT ( 'NONE',  ( 16.51473224551069308, 9.474510206698969483, 34.16557627198102409 ) ) ;
#88118=CARTESIAN_POINT ( 'NONE',  ( 5.823673210054125526, 21.52544592524343514, 74.79057627198105251 ) ) ;
#88119=CARTESIAN_POINT ( 'NONE',  ( 9.564922557960805705, 16.46253265017160317, 39.58224293864768839 ) ) ;
#88121=CARTESIAN_POINT ( 'NONE',  ( 0.05219959533936267826, -19.03943276465977164, 75.00109039468566152 ) ) ;
#88122=CARTESIAN_POINT ( 'NONE',  ( -4.379528057220328563, 16.55341960407611168, 55.20724293864770260 ) ) ;
#88123=CARTESIAN_POINT ( 'NONE',  ( 21.53943276465977519, -0.05219959533907433946, 38.74890960531435979 ) ) ;
#88124=CARTESIAN_POINT ( 'NONE',  ( -0.05219959533937732626, 21.53943276465977519, 92.50109039468567573 ) ) ;
#88125=CARTESIAN_POINT ( 'NONE',  ( -18.62759615963270932, 10.81492255796079327, 85.83224293864768129 ) ) ;
#88126=CARTESIAN_POINT ( 'NONE',  ( -18.62759615963255300, -10.81492255796106328, 74.16775706135231871 ) ) ;
#88127=CARTESIAN_POINT ( 'NONE',  ( -21.55341960407619339, 5.719274019375674811, 58.54275706135235424 ) ) ;
#88128=CARTESIAN_POINT ( 'NONE',  ( 5.049401038298161559, -19.05341960407611168, 97.70724293864766707 ) ) ;
#88129=CARTESIAN_POINT ( 'NONE',  ( -8.224510206698735004, -14.34966873604973081, 94.58442372801901854 ) ) ;
#88130=CARTESIAN_POINT ( 'NONE',  ( -15.80617190586768217, 15.72974639402176855, 63.12609039468568994 ) ) ;
#88131=CARTESIAN_POINT ( 'NONE',  ( -19.02544592524342804, 5.153800228976336051, 51.04057627198103120 ) ) ;
#88132=CARTESIAN_POINT ( 'NONE',  ( 10.81492255796106328, -18.62759615963255655, 30.41775706135234358 ) ) ;
#88133=CARTESIAN_POINT ( 'NONE',  ( 5.153800228976335163, 19.02544592524342804, 74.79057627198103830 ) ) ;
#88134=CARTESIAN_POINT ( 'NONE',  ( -12.14591786802309592, -12.06949235617757132, 66.87390960531436690 ) ) ;
#88135=CARTESIAN_POINT ( 'NONE',  ( 8.224510206698953496, -14.34966873604960469, 47.91557627198102409 ) ) ;
#88136=CARTESIAN_POINT ( 'NONE',  ( -21.55341960407610458, -5.719274019375992779, 56.45724293864768839 ) ) ;
#88137=CARTESIAN_POINT ( 'NONE',  ( -13.97604488694527625, -13.89961937509977652, 41.87390960531435979 ) ) ;
#88138=CARTESIAN_POINT ( 'NONE',  ( 21.52544592524344225, -5.823673210054117533, 53.54057627198103120 ) ) ;
#88139=CARTESIAN_POINT ( 'NONE',  ( 19.02544592524334988, 5.153800228976608722, 46.45942372801899012 ) ) ;
#88140=CARTESIAN_POINT ( 'NONE',  ( -13.89961937509957401, -13.97604488694547697, 24.37609039468565797 ) ) ;
#88141=CARTESIAN_POINT ( 'NONE',  ( 8.314922557960818139, 14.29746914071049879, 64.58224293864769550 ) ) ;
#88142=CARTESIAN_POINT ( 'NONE',  ( 21.55341960407610458, 5.719274019375980345, 33.95724293864769550 ) ) ;
#88145=CARTESIAN_POINT ( 'NONE',  ( -14.34966873604972548, 8.224510206698743886, 83.33442372801903275 ) ) ;
#88146=CARTESIAN_POINT ( 'NONE',  ( -13.97604488694547697, 13.89961937509957934, 88.12609039468563310 ) ) ;
#88147=EDGE_CURVE ( 'NONE', #17083, #121093, #138951, .T. ) ;
#88148=CARTESIAN_POINT ( 'NONE',  ( 14.34966873604960469, 8.224510206698951720, 54.16557627198103120 ) ) ;
#88150=CARTESIAN_POINT ( 'NONE',  ( -16.46253265017160317, 9.564922557960807481, 45.83224293864769550 ) ) ;
#88151=CARTESIAN_POINT ( 'NONE',  ( 16.55341960407611168, 4.379528057220329451, 38.95724293864768839 ) ) ;
#88152=CARTESIAN_POINT ( 'NONE',  ( -19.02544592524342804, 5.153800228976336051, 51.04057627198103120 ) ) ;
#88153=CARTESIAN_POINT ( 'NONE',  ( -9.564922557960796823, -16.46253265017161027, 72.08224293864770971 ) ) ;
#88154=CARTESIAN_POINT ( 'NONE',  ( 19.05341960407611168, 5.049401038298154454, 48.95724293864768129 ) ) ;
#88155=CARTESIAN_POINT ( 'NONE',  ( -10.81492255796105439, 18.62759615963255655, 57.91775706135234714 ) ) ;
#88156=CARTESIAN_POINT ( 'NONE',  ( 5.153800228976335163, 19.02544592524342804, 69.79057627198103830 ) ) ;
#88157=CARTESIAN_POINT ( 'NONE',  ( -0.05219959533909027116, -19.03943276465977164, 32.49890960531435979 ) ) ;
#88158=CARTESIAN_POINT ( 'NONE',  ( -16.46253265017160317, 9.564922557960807481, 60.83224293864769550 ) ) ;
#88159=CARTESIAN_POINT ( 'NONE',  ( -18.67979575497178146, -10.72451020669898902, 51.66557627198102409 ) ) ;
#88160=CARTESIAN_POINT ( 'NONE',  ( -5.153800228976328057, -19.02544592524343514, 37.29057627198102409 ) ) ;
#88161=CARTESIAN_POINT ( 'NONE',  ( -10.72451020669898014, 18.67979575497178502, 35.41557627198102409 ) ) ;
#88163=CARTESIAN_POINT ( 'NONE',  ( 16.53943276465976808, 0.05219959533934440121, 106.2510903946856757 ) ) ;
#88164=CARTESIAN_POINT ( 'NONE',  ( -9.474510206698720793, -16.51473224551083518, 24.58442372801900078 ) ) ;
#88165=CARTESIAN_POINT ( 'NONE',  ( 8.314922557961029526, -14.29746914071037800, 40.41775706135234714 ) ) ;
#88166=CARTESIAN_POINT ( 'NONE',  ( 8.314922557961029526, -14.29746914071037800, 75.41775706135233293 ) ) ;
#88168=CARTESIAN_POINT ( 'NONE',  ( -4.483927247898782831, 16.52544592524335698, 72.70942372801901854 ) ) ;
#88169=CARTESIAN_POINT ( 'NONE',  ( -8.314922557961024197, 14.29746914071037800, 52.91775706135235424 ) ) ;
#88170=CARTESIAN_POINT ( 'NONE',  ( 5.049401038298161559, -19.05341960407611168, 107.7072429386476955 ) ) ;
#88171=CARTESIAN_POINT ( 'NONE',  ( 4.483927247898790824, -16.52544592524335698, 40.20942372801901854 ) ) ;
#88172=CARTESIAN_POINT ( 'NONE',  ( 0.05219959533909260263, 19.03943276465977164, 39.99890960531436690 ) ) ;
#88173=CARTESIAN_POINT ( 'NONE',  ( -21.52544592524334988, -5.823673210054445271, 28.95942372801902209 ) ) ;
#88174=CARTESIAN_POINT ( 'NONE',  ( 14.29746914071037800, 8.314922557961029526, 31.66775706135234358 ) ) ;
#88175=CARTESIAN_POINT ( 'NONE',  ( -16.52544592524335698, -4.483927247898792601, 103.9594237280190185 ) ) ;
#88177=CARTESIAN_POINT ( 'NONE',  ( 10.81492255796106328, -18.62759615963255655, 100.4177570613523471 ) ) ;
#88178=CARTESIAN_POINT ( 'NONE',  ( -5.153800228976607833, 19.02544592524334988, 97.70942372801900433 ) ) ;
#88179=CARTESIAN_POINT ( 'NONE',  ( 12.06949235617757843, -12.14591786802309237, 53.12390960531436690 ) ) ;
#88180=CARTESIAN_POINT ( 'NONE',  ( -0.05219959533909027116, -19.03943276465977164, 27.49890960531435624 ) ) ;
#88181=CARTESIAN_POINT ( 'NONE',  ( -13.97604488694547697, 13.89961937509957934, 58.12609039468566863 ) ) ;
#88182=CARTESIAN_POINT ( 'NONE',  ( 17.05116617787824040, 6.768360034955837712, 78.84324446740806991 ) ) ;
#88183=CARTESIAN_POINT ( 'NONE',  ( 15.80617190586769283, -15.72974639402175789, 65.62609039468568994 ) ) ;
#88184=CARTESIAN_POINT ( 'NONE',  ( 12.06949235617739724, 12.14591786802326823, 21.87609039468567573 ) ) ;
#88185=LINE ( 'NONE', #75993, #89094 ) ;
#88186=CARTESIAN_POINT ( 'NONE',  ( 5.719274019375991003, -21.55341960407610458, 22.70724293864769194 ) ) ;
#88187=CARTESIAN_POINT ( 'NONE',  ( -0.05219959533936034679, 19.03943276465977164, 112.5010903946856757 ) ) ;
#88189=CARTESIAN_POINT ( 'NONE',  ( 0.05219959533936267826, -19.03943276465977164, 50.00109039468566863 ) ) ;
#88190=CARTESIAN_POINT ( 'NONE',  ( 5.049401038298161559, -19.05341960407611168, 27.70724293864769550 ) ) ;
#88191=CARTESIAN_POINT ( 'NONE',  ( 0.05219959533937995610, -21.53943276465977519, 105.0010903946856757 ) ) ;
#88192=CARTESIAN_POINT ( 'NONE',  ( -16.51473224551069308, -9.474510206698971260, 46.66557627198102409 ) ) ;
#88193=CARTESIAN_POINT ( 'NONE',  ( -0.05219959533937732626, 21.53943276465977519, 52.50109039468567573 ) ) ;
#88194=CARTESIAN_POINT ( 'NONE',  ( -15.72974639402176322, -15.80617190586768395, 104.3760903946856899 ) ) ;
#88195=CARTESIAN_POINT ( 'NONE',  ( 0.05219959533934541429, -16.53943276465976808, 110.0010903946856757 ) ) ;
#88196=CARTESIAN_POINT ( 'NONE',  ( 19.02544592524343514, -5.153800228976328945, 83.54057627198100988 ) ) ;
#88197=CARTESIAN_POINT ( 'NONE',  ( -21.52544592524334988, -5.823673210054445271, 38.95942372801901854 ) ) ;
#88198=CARTESIAN_POINT ( 'NONE',  ( 10.72451020669871369, 18.67979575497193778, 47.08442372801901854 ) ) ;
#88199=CARTESIAN_POINT ( 'NONE',  ( -5.049401038297874678, -19.05341960407617918, 79.79275706135233293 ) ) ;
#88200=CARTESIAN_POINT ( 'NONE',  ( -9.564922557960796823, -16.46253265017161027, 92.08224293864769550 ) ) ;
#88201=CARTESIAN_POINT ( 'NONE',  ( 4.483927247898545687, 16.52544592524342804, 104.7905762719810241 ) ) ;
#88202=CARTESIAN_POINT ( 'NONE',  ( -18.62759615963270932, 10.81492255796079327, 90.83224293864769550 ) ) ;
#88203=CARTESIAN_POINT ( 'NONE',  ( 0.05219959533936267826, -19.03943276465977164, 25.00109039468566152 ) ) ;
#88204=CARTESIAN_POINT ( 'NONE',  ( 12.06949235617757843, -12.14591786802309237, 98.12390960531436690 ) ) ;
#88205=CARTESIAN_POINT ( 'NONE',  ( 0.05219959533909260263, 19.03943276465977164, 54.99890960531435979 ) ) ;
#88206=CARTESIAN_POINT ( 'NONE',  ( -13.97604488694547697, 13.89961937509957934, 78.12609039468567573 ) ) ;
#88207=CARTESIAN_POINT ( 'NONE',  ( 12.14591786802309770, 12.06949235617756955, 44.37390960531435979 ) ) ;
#88208=CARTESIAN_POINT ( 'NONE',  ( -5.823673210054431948, 21.52544592524334988, 102.7094237280190185 ) ) ;
#88209=CARTESIAN_POINT ( 'NONE',  ( -16.51473224551069308, -9.474510206698971260, 111.6655762719810383 ) ) ;
#88210=CARTESIAN_POINT ( 'NONE',  ( -13.97604488694547697, 13.89961937509957934, 73.12609039468568994 ) ) ;
#88211=CARTESIAN_POINT ( 'NONE',  ( 5.823673210054125526, 21.52544592524343514, 74.79057627198105251 ) ) ;
#88212=CARTESIAN_POINT ( 'NONE',  ( -21.52544592524334988, -5.823673210054445271, 28.95942372801902209 ) ) ;
#88213=CARTESIAN_POINT ( 'NONE',  ( 16.53943276465976808, 0.05219959533934440121, 31.25109039468568639 ) ) ;
#88214=CARTESIAN_POINT ( 'NONE',  ( -16.53943276465976808, -0.05219959533934237506, 98.75109039468568994 ) ) ;
#88215=CARTESIAN_POINT ( 'NONE',  ( -19.05341960407611168, -5.049401038298163336, 31.45724293864769550 ) ) ;
#88216=CARTESIAN_POINT ( 'NONE',  ( -18.62759615963255300, -10.81492255796106328, 34.16775706135234714 ) ) ;
#88217=CARTESIAN_POINT ( 'NONE',  ( -10.81492255796078084, -18.62759615963271287, 37.08224293864768129 ) ) ;
#88218=CARTESIAN_POINT ( 'NONE',  ( -16.51473224551069308, -9.474510206698971260, 26.66557627198103120 ) ) ;
#88220=CARTESIAN_POINT ( 'NONE',  ( -8.224510206698735004, -14.34966873604973081, 59.58442372801901854 ) ) ;
#88221=CARTESIAN_POINT ( 'NONE',  ( 16.52544592524342804, -4.483927247898539470, 93.54057627198103830 ) ) ;
#88222=CARTESIAN_POINT ( 'NONE',  ( 18.67979575497178502, 10.72451020669898547, 84.16557627198103830 ) ) ;
#88223=CARTESIAN_POINT ( 'NONE',  ( 4.379528057220092307, 16.55341960407617563, 112.2927570613523471 ) ) ;
#88224=CARTESIAN_POINT ( 'NONE',  ( 16.52544592524335698, 4.483927247898782831, 51.45942372801901854 ) ) ;
#88225=CARTESIAN_POINT ( 'NONE',  ( 19.02544592524343514, -5.153800228976328945, 63.54057627198103830 ) ) ;
#88226=CARTESIAN_POINT ( 'NONE',  ( 16.52544592524335698, 4.483927247898782831, 91.45942372801901854 ) ) ;
#88227=CARTESIAN_POINT ( 'NONE',  ( 19.03943276465977164, 0.05219959533936151252, 86.25109039468567573 ) ) ;
#88228=CARTESIAN_POINT ( 'NONE',  ( 21.55341960407610458, 5.719274019375980345, 83.95724293864770971 ) ) ;
#88229=CARTESIAN_POINT ( 'NONE',  ( -16.55341960407611168, -4.379528057220339221, 21.45724293864769550 ) ) ;
#88231=CARTESIAN_POINT ( 'NONE',  ( -5.049401038298153566, 19.05341960407611168, 115.2072429386477097 ) ) ;
#88232=CARTESIAN_POINT ( 'NONE',  ( -18.67979575497178146, -10.72451020669898902, 66.66557627198102409 ) ) ;
#88233=CARTESIAN_POINT ( 'NONE',  ( -14.29746914071037622, -8.314922557961029526, 94.16775706135237556 ) ) ;
#88235=CARTESIAN_POINT ( 'NONE',  ( -10.81492255796078084, -18.62759615963271287, 27.08224293864769550 ) ) ;
#88237=CARTESIAN_POINT ( 'NONE',  ( 0.05219959533907565091, 21.53943276465977519, 94.99890960531436690 ) ) ;
#88238=CARTESIAN_POINT ( 'NONE',  ( 12.06949235617757843, -12.14591786802309237, 23.12390960531436335 ) ) ;
#88239=CARTESIAN_POINT ( 'NONE',  ( 12.14591786802327356, -12.06949235617739191, 35.62609039468568994 ) ) ;
#88240=CARTESIAN_POINT ( 'NONE',  ( 16.46253265017160672, -9.564922557960803928, 28.33224293864769550 ) ) ;
#88241=CARTESIAN_POINT ( 'NONE',  ( -14.34966873604972548, 8.224510206698743886, 33.33442372801900433 ) ) ;
#88242=CARTESIAN_POINT ( 'NONE',  ( -0.05219959533909027116, -19.03943276465977164, 57.49890960531435979 ) ) ;
#88244=CARTESIAN_POINT ( 'NONE',  ( 19.03943276465977164, -0.05219959533909143690, 108.7489096053143527 ) ) ;
#88246=CARTESIAN_POINT ( 'NONE',  ( 16.53943276465976808, 0.05219959533934440121, 106.2510903946856757 ) ) ;
#88247=CARTESIAN_POINT ( 'NONE',  ( 5.049401038297881783, 19.05341960407617563, 97.29275706135233293 ) ) ;
#88248=CARTESIAN_POINT ( 'NONE',  ( -13.89961937509957401, -13.97604488694547875, 34.37609039468566863 ) ) ;
#88249=CARTESIAN_POINT ( 'NONE',  ( -21.55341960407610458, -5.719274019375992779, 81.45724293864769550 ) ) ;
#88250=CARTESIAN_POINT ( 'NONE',  ( 14.34966873604972726, -8.224510206698740333, 105.8344237280190328 ) ) ;
#88251=CARTESIAN_POINT ( 'NONE',  ( -21.55341960407610458, -5.719274019375992779, 36.45724293864768839 ) ) ;
#88252=CARTESIAN_POINT ( 'NONE',  ( -16.46253265017146816, -9.564922557961047289, 104.1677570613523329 ) ) ;
#88253=CARTESIAN_POINT ( 'NONE',  ( 13.97604488694527802, 13.89961937509977652, 104.3739096053143385 ) ) ;
#88254=CARTESIAN_POINT ( 'NONE',  ( 18.62759615963255655, 10.81492255796105972, 66.66775706135234714 ) ) ;
#88255=CARTESIAN_POINT ( 'NONE',  ( 19.02544592524343514, -5.153800228976328945, 63.54057627198103830 ) ) ;
#88256=CARTESIAN_POINT ( 'NONE',  ( 8.314922557960818139, 14.29746914071049879, 94.58224293864769550 ) ) ;
#88257=CARTESIAN_POINT ( 'NONE',  ( -16.38665767535050577, -7.295008042176168495, 84.73599135785454450 ) ) ;
#88258=CARTESIAN_POINT ( 'NONE',  ( -8.224510206698948167, 14.34966873604960824, 80.41557627198103830 ) ) ;
#88259=CARTESIAN_POINT ( 'NONE',  ( 15.80617190586746368, 15.72974639402197994, 69.37390960531436690 ) ) ;
#88260=VERTEX_POINT ( 'NONE', #113170 ) ;
#88261=CARTESIAN_POINT ( 'NONE',  ( 9.564922557961047289, -16.46253265017146816, 90.41775706135234714 ) ) ;
#88263=CARTESIAN_POINT ( 'NONE',  ( 19.03943276465977164, -0.05219959533909143690, 58.74890960531435979 ) ) ;
#88264=CARTESIAN_POINT ( 'NONE',  ( 17.48853670773243962, -5.747243402303062076, 71.16671299749988577 ) ) ;
#88265=CARTESIAN_POINT ( 'NONE',  ( 0.05219959533909260263, 19.03943276465977164, 79.99890960531436690 ) ) ;
#88266=CARTESIAN_POINT ( 'NONE',  ( -16.46253265017160317, 9.564922557960807481, 90.83224293864769550 ) ) ;
#88267=CARTESIAN_POINT ( 'NONE',  ( 14.34966873604972726, -8.224510206698740333, 65.83442372801900433 ) ) ;
#88269=CARTESIAN_POINT ( 'NONE',  ( 5.153800228976615827, -19.02544592524334988, 45.20942372801901143 ) ) ;
#88271=CARTESIAN_POINT ( 'NONE',  ( 13.89961937509977652, -13.97604488694527269, 108.1239096053143669 ) ) ;
#88272=CARTESIAN_POINT ( 'NONE',  ( 0.05219959533934541429, -16.53943276465976808, 105.0010903946856757 ) ) ;
#88274=CARTESIAN_POINT ( 'NONE',  ( -16.55341960407617563, 4.379528057220093196, 98.54275706135234714 ) ) ;
#88275=CARTESIAN_POINT ( 'NONE',  ( -17.12812012977024168, 6.668231424566044119, 28.64051240676857191 ) ) ;
#88276=CARTESIAN_POINT ( 'NONE',  ( -12.06949235617739369, -12.14591786802326823, 64.37609039468568994 ) ) ;
#88278=CARTESIAN_POINT ( 'NONE',  ( -15.72974639402176322, -15.80617190586768395, 64.37609039468568994 ) ) ;
#88279=CARTESIAN_POINT ( 'NONE',  ( 13.89961937509957401, 13.97604488694547697, 71.87609039468567573 ) ) ;
#88280=CARTESIAN_POINT ( 'NONE',  ( -19.03943276465977164, -0.05219959533935918106, 28.75109039468566507 ) ) ;
#88281=CARTESIAN_POINT ( 'NONE',  ( 0.05219959533909260263, 19.03943276465977164, 64.99890960531436690 ) ) ;
#88282=CARTESIAN_POINT ( 'NONE',  ( 5.049401038298161559, -19.05341960407611168, 42.70724293864767418 ) ) ;
#88284=CARTESIAN_POINT ( 'NONE',  ( 18.67979575497178502, 10.72451020669898547, 79.16557627198103830 ) ) ;
#88285=CARTESIAN_POINT ( 'NONE',  ( -18.62759615963270932, 10.81492255796079327, 30.83224293864770260 ) ) ;
#88286=CARTESIAN_POINT ( 'NONE',  ( -0.05219959533909027116, -19.03943276465977164, 27.49890960531435624 ) ) ;
#88287=CARTESIAN_POINT ( 'NONE',  ( -4.379528057220086978, -16.55341960407618274, 49.79275706135234714 ) ) ;
#88290=CARTESIAN_POINT ( 'NONE',  ( -0.05219959533937732626, 21.53943276465977519, 37.50109039468568284 ) ) ;
#88291=CARTESIAN_POINT ( 'NONE',  ( 16.55341960407611168, 4.379528057220329451, 53.95724293864770260 ) ) ;
#88293=CARTESIAN_POINT ( 'NONE',  ( 4.483927247898790824, -16.52544592524335698, 25.20942372801901854 ) ) ;
#88294=CARTESIAN_POINT ( 'NONE',  ( -5.049401038297874678, -19.05341960407617918, 44.79275706135232582 ) ) ;
#88295=CARTESIAN_POINT ( 'NONE',  ( 16.53943276465976808, -0.05219959533910856209, 63.74890960531435979 ) ) ;
#88296=CARTESIAN_POINT ( 'NONE',  ( -5.823673210054116645, -21.52544592524344225, 112.2905762719810241 ) ) ;
#88298=CARTESIAN_POINT ( 'NONE',  ( -5.823673210054116645, -21.52544592524344225, 72.29057627198102409 ) ) ;
#88299=CARTESIAN_POINT ( 'NONE',  ( -16.51473224551069308, -9.474510206698971260, 96.66557627198102409 ) ) ;
#88300=CARTESIAN_POINT ( 'NONE',  ( 8.224510206698953496, -14.34966873604960469, 67.91557627198102409 ) ) ;
#88301=CARTESIAN_POINT ( 'NONE',  ( 0.05219959533909260263, 19.03943276465977164, 99.99890960531436690 ) ) ;
#88302=CARTESIAN_POINT ( 'NONE',  ( -18.22780087662114212, 5.499999999999995559, 48.51540105326107266 ) ) ;
#88303=CARTESIAN_POINT ( 'NONE',  ( 9.474510206698729675, 16.51473224551082808, 62.08442372801899722 ) ) ;
#88304=CARTESIAN_POINT ( 'NONE',  ( -10.72451020669898014, 18.67979575497178502, 105.4155762719810383 ) ) ;
#88305=CARTESIAN_POINT ( 'NONE',  ( -16.51473224551069308, -9.474510206698971260, 56.66557627198103120 ) ) ;
#88306=CARTESIAN_POINT ( 'NONE',  ( 0.05219959533936267826, -19.03943276465977164, 45.00109039468566863 ) ) ;
#88307=CARTESIAN_POINT ( 'NONE',  ( -12.06949235617756955, 12.14591786802309770, 110.6239096053143669 ) ) ;
#88308=CARTESIAN_POINT ( 'NONE',  ( -21.52544592524334988, -5.823673210054445271, 58.95942372801902565 ) ) ;
#88309=CARTESIAN_POINT ( 'NONE',  ( -16.79531203550649820, -7.028104445595611871, 71.25244988220447340 ) ) ;
#88310=CARTESIAN_POINT ( 'NONE',  ( -4.379528057220328563, 16.55341960407611168, 45.20724293864769550 ) ) ;
#88311=CARTESIAN_POINT ( 'NONE',  ( -19.03943276465977164, 0.05219959533909376836, 51.24890960531436690 ) ) ;
#88312=CARTESIAN_POINT ( 'NONE',  ( 5.049401038298161559, -19.05341960407611168, 112.7072429386476813 ) ) ;
#88313=CARTESIAN_POINT ( 'NONE',  ( 21.52544592524344225, -5.823673210054117533, 78.54057627198103830 ) ) ;
#88315=CARTESIAN_POINT ( 'NONE',  ( 5.049401038298161559, -19.05341960407611168, 47.70724293864770260 ) ) ;
#88316=CARTESIAN_POINT ( 'NONE',  ( -10.81492255796078084, -18.62759615963271287, 62.08224293864769550 ) ) ;
#88317=CARTESIAN_POINT ( 'NONE',  ( -15.80617190586768217, 15.72974639402176855, 83.12609039468568994 ) ) ;
#88319=CARTESIAN_POINT ( 'NONE',  ( -14.29746914071037622, -8.314922557961029526, 94.16775706135237556 ) ) ;
#88320=CARTESIAN_POINT ( 'NONE',  ( -12.14591786802309592, -12.06949235617757132, 81.87390960531435269 ) ) ;
#88321=CARTESIAN_POINT ( 'NONE',  ( 16.51473224551069308, 9.474510206698969483, 64.16557627198102409 ) ) ;
#88323=CARTESIAN_POINT ( 'NONE',  ( 5.153800228976615827, -19.02544592524334988, 45.20942372801901143 ) ) ;
#88324=CARTESIAN_POINT ( 'NONE',  ( 8.314922557961029526, -14.29746914071037800, 85.41775706135236135 ) ) ;
#88325=CARTESIAN_POINT ( 'NONE',  ( 13.89961937509957401, 13.97604488694547697, 21.87609039468566152 ) ) ;
#88326=CARTESIAN_POINT ( 'NONE',  ( 0.05219959533909260263, 19.03943276465977164, 84.99890960531436690 ) ) ;
#88327=CARTESIAN_POINT ( 'NONE',  ( -10.72451020669898014, 18.67979575497178502, 50.41557627198103120 ) ) ;
#88329=CARTESIAN_POINT ( 'NONE',  ( 10.72451020669871369, 18.67979575497193778, 102.0844237280190185 ) ) ;
#88330=CARTESIAN_POINT ( 'NONE',  ( -12.06949235617739369, -12.14591786802326823, 59.37609039468568284 ) ) ;
#88331=CARTESIAN_POINT ( 'NONE',  ( 15.80617190586769283, -15.72974639402175789, 20.62609039468568639 ) ) ;
#88332=CARTESIAN_POINT ( 'NONE',  ( 4.379528057220092307, 16.55341960407617563, 32.29275706135235424 ) ) ;
#88333=CARTESIAN_POINT ( 'NONE',  ( 9.474510206698971260, -16.51473224551069308, 92.91557627198103830 ) ) ;
#88334=CARTESIAN_POINT ( 'NONE',  ( 19.03943276465977164, -0.05219959533909143690, 38.74890960531436690 ) ) ;
#88335=CARTESIAN_POINT ( 'NONE',  ( 16.46253265017160672, -9.564922557960803928, 58.33224293864769550 ) ) ;
#88336=CARTESIAN_POINT ( 'NONE',  ( 4.379528057220092307, 16.55341960407617563, 32.29275706135235424 ) ) ;
#88337=CARTESIAN_POINT ( 'NONE',  ( -4.379528057220328563, 16.55341960407611168, 75.20724293864769550 ) ) ;
#88338=CARTESIAN_POINT ( 'NONE',  ( 16.53943276465976808, 0.05219959533934440121, 81.25109039468568994 ) ) ;
#88339=CARTESIAN_POINT ( 'NONE',  ( -21.55341960407619339, 5.719274019375674811, 43.54275706135235424 ) ) ;
#88340=CARTESIAN_POINT ( 'NONE',  ( 5.049401038298161559, -19.05341960407611168, 62.70724293864769550 ) ) ;
#88341=CARTESIAN_POINT ( 'NONE',  ( -5.049401038298153566, 19.05341960407611168, 55.20724293864769550 ) ) ;
#88342=CARTESIAN_POINT ( 'NONE',  ( -9.564922557960796823, -16.46253265017161027, 77.08224293864769550 ) ) ;
#88343=CARTESIAN_POINT ( 'NONE',  ( -8.314922557960811034, -14.29746914071050412, 32.08224293864769550 ) ) ;
#88344=CARTESIAN_POINT ( 'NONE',  ( -16.52544592524335698, -4.483927247898792601, 83.95942372801900433 ) ) ;
#88346=CARTESIAN_POINT ( 'NONE',  ( 9.474510206698729675, 16.51473224551082808, 27.08442372801900433 ) ) ;
#88347=CARTESIAN_POINT ( 'NONE',  ( -19.02544592524342804, 5.153800228976336051, 106.0405762719810241 ) ) ;
#88348=CARTESIAN_POINT ( 'NONE',  ( -5.153800228976328057, -19.02544592524343514, 52.29057627198100988 ) ) ;
#88349=CARTESIAN_POINT ( 'NONE',  ( -5.049401038297874678, -19.05341960407617918, 24.79275706135233648 ) ) ;
#88351=CARTESIAN_POINT ( 'NONE',  ( 4.379528057220092307, 16.55341960407617563, 42.29275706135235424 ) ) ;
#88352=CARTESIAN_POINT ( 'NONE',  ( 16.46253265017146816, 9.564922557961045513, 66.66775706135233293 ) ) ;
#88353=CARTESIAN_POINT ( 'NONE',  ( -12.06949235617739369, -12.14591786802326823, 54.37609039468568994 ) ) ;
#88354=CARTESIAN_POINT ( 'NONE',  ( -19.03943276465977164, 0.05219959533909376836, 116.2489096053143669 ) ) ;
#88355=CARTESIAN_POINT ( 'NONE',  ( 16.46253265017160672, -9.564922557960803928, 73.33224293864769550 ) ) ;
#88356=CARTESIAN_POINT ( 'NONE',  ( -0.05219959533907301413, -21.53943276465977519, 112.4989096053143669 ) ) ;
#88357=CARTESIAN_POINT ( 'NONE',  ( -16.46253265017146816, -9.564922557961047289, 69.16775706135233293 ) ) ;
#88358=CARTESIAN_POINT ( 'NONE',  ( 13.89961937509977652, -13.97604488694527269, 103.1239096053143527 ) ) ;
#88359=CARTESIAN_POINT ( 'NONE',  ( -16.51473224551069308, -9.474510206698971260, 36.66557627198102409 ) ) ;
#88360=CARTESIAN_POINT ( 'NONE',  ( -19.05341960407611168, -5.049401038298163336, 81.45724293864769550 ) ) ;
#88361=CARTESIAN_POINT ( 'NONE',  ( -4.379528057220328563, 16.55341960407611168, 40.20724293864769550 ) ) ;
#88362=CARTESIAN_POINT ( 'NONE',  ( 13.89961937509977652, -13.97604488694527269, 38.12390960531436690 ) ) ;
#88363=CARTESIAN_POINT ( 'NONE',  ( -16.51473224551082808, 9.474510206698731452, 33.33442372801899722 ) ) ;
#88364=CARTESIAN_POINT ( 'NONE',  ( 8.224510206698953496, -14.34966873604960469, 72.91557627198103830 ) ) ;
#88365=CARTESIAN_POINT ( 'NONE',  ( 9.564922557961047289, -16.46253265017146816, 20.41775706135233293 ) ) ;
#88366=CARTESIAN_POINT ( 'NONE',  ( -9.564922557960796823, -16.46253265017161027, 52.08224293864768839 ) ) ;
#88367=CARTESIAN_POINT ( 'NONE',  ( 4.483927247898545687, 16.52544592524342804, 49.79057627198102409 ) ) ;
#88368=CARTESIAN_POINT ( 'NONE',  ( -5.823673210054431948, 21.52544592524334988, 102.7094237280190185 ) ) ;
#88369=CARTESIAN_POINT ( 'NONE',  ( 13.97604488694527802, 13.89961937509977652, 89.37390960531436690 ) ) ;
#88370=CARTESIAN_POINT ( 'NONE',  ( 19.03943276465977164, -0.05219959533909143690, 113.7489096053143669 ) ) ;
#88371=CARTESIAN_POINT ( 'NONE',  ( 19.02544592524343514, -5.153800228976328945, 38.54057627198103120 ) ) ;
#88372=CARTESIAN_POINT ( 'NONE',  ( -16.51473224551069308, -9.474510206698971260, 21.66557627198102765 ) ) ;
#88373=CARTESIAN_POINT ( 'NONE',  ( 8.314922557960818139, 14.29746914071049879, 84.58224293864769550 ) ) ;
#88374=CARTESIAN_POINT ( 'NONE',  ( -15.72974639402197994, 15.80617190586746368, 95.62390960531436690 ) ) ;
#88375=CARTESIAN_POINT ( 'NONE',  ( -19.05341960407611168, -5.049401038298163336, 81.45724293864769550 ) ) ;
#88376=CARTESIAN_POINT ( 'NONE',  ( -10.72451020669898014, 18.67979575497178502, 100.4155762719810241 ) ) ;
#88377=CARTESIAN_POINT ( 'NONE',  ( -5.049401038298153566, 19.05341960407611168, 85.20724293864766707 ) ) ;
#88379=CARTESIAN_POINT ( 'NONE',  ( 14.29746914071049879, -8.314922557960816363, 103.3322429386476955 ) ) ;
#88380=CARTESIAN_POINT ( 'NONE',  ( -0.05219959533909027116, -19.03943276465977164, 77.49890960531435269 ) ) ;
#88381=CARTESIAN_POINT ( 'NONE',  ( -15.80617190586745835, -15.72974639402198527, 76.87390960531439532 ) ) ;
#88383=CARTESIAN_POINT ( 'NONE',  ( -15.80617190586745835, -15.72974639402198527, 26.87390960531435979 ) ) ;
#88385=CARTESIAN_POINT ( 'NONE',  ( -16.52544592524335698, -4.483927247898792601, 28.95942372801902209 ) ) ;
#88387=CARTESIAN_POINT ( 'NONE',  ( -12.06949235617756955, 12.14591786802309770, 90.62390960531436690 ) ) ;
#88388=CARTESIAN_POINT ( 'NONE',  ( -16.81555441253550853, -7.025013491695485612, 94.36314554665744936 ) ) ;
#88389=CARTESIAN_POINT ( 'NONE',  ( 19.03943276465977164, -0.05219959533909143690, 88.74890960531436690 ) ) ;
#88390=CARTESIAN_POINT ( 'NONE',  ( 0.05219959533909260263, 19.03943276465977164, 39.99890960531436690 ) ) ;
#88391=CARTESIAN_POINT ( 'NONE',  ( 16.53943276465976808, -0.05219959533910856209, 83.74890960531435269 ) ) ;
#88393=CARTESIAN_POINT ( 'NONE',  ( 0.05219959533907565091, 21.53943276465977519, 34.99890960531435979 ) ) ;
#88394=CARTESIAN_POINT ( 'NONE',  ( 8.314922557960818139, 14.29746914071049879, 49.58224293864769550 ) ) ;
#88395=CARTESIAN_POINT ( 'NONE',  ( -19.03943276465977164, -0.05219959533935918106, 108.7510903946856615 ) ) ;
#88396=CARTESIAN_POINT ( 'NONE',  ( 10.81492255796106328, -18.62759615963255655, 65.41775706135234714 ) ) ;
#88398=CARTESIAN_POINT ( 'NONE',  ( 9.474510206698971260, -16.51473224551069308, 102.9155762719810241 ) ) ;
#88399=CARTESIAN_POINT ( 'NONE',  ( -14.29746914071037622, -8.314922557961029526, 84.16775706135234714 ) ) ;
#88400=CARTESIAN_POINT ( 'NONE',  ( -9.564922557960796823, -16.46253265017161027, 27.08224293864769550 ) ) ;
#88401=CARTESIAN_POINT ( 'NONE',  ( -16.51473224551069308, -9.474510206698971260, 81.66557627198103830 ) ) ;
#88402=CARTESIAN_POINT ( 'NONE',  ( 10.72451020669898902, -18.67979575497178502, 87.91557627198103830 ) ) ;
#88403=CARTESIAN_POINT ( 'NONE',  ( -19.05341960407617563, 5.049401038297882671, 108.5427570613523187 ) ) ;
#88404=CARTESIAN_POINT ( 'NONE',  ( -8.224510206698948167, 14.34966873604960824, 50.41557627198103120 ) ) ;
#88405=CARTESIAN_POINT ( 'NONE',  ( -21.53943276465977519, -0.05219959533937600094, 63.75109039468568284 ) ) ;
#88406=CARTESIAN_POINT ( 'NONE',  ( -4.483927247898782831, 16.52544592524335698, 92.70942372801901854 ) ) ;
#88407=CARTESIAN_POINT ( 'NONE',  ( -19.02544592524342804, 5.153800228976336051, 116.0405762719810383 ) ) ;
#88408=CARTESIAN_POINT ( 'NONE',  ( 13.97604488694527802, 13.89961937509977830, 114.3739096053143669 ) ) ;
#88410=CARTESIAN_POINT ( 'NONE',  ( 14.34966873604972726, -8.224510206698740333, 110.8344237280190043 ) ) ;
#88411=CARTESIAN_POINT ( 'NONE',  ( 16.52544592524335698, 4.483927247898782831, 61.45942372801901854 ) ) ;
#88412=CARTESIAN_POINT ( 'NONE',  ( 19.05341960407611168, 5.049401038298154454, 73.95724293864768129 ) ) ;
#88414=CARTESIAN_POINT ( 'NONE',  ( 9.564922557960805705, 16.46253265017160317, 84.58224293864769550 ) ) ;
#88415=CARTESIAN_POINT ( 'NONE',  ( -21.55341960407619339, 5.719274019375674811, 68.54275706135234714 ) ) ;
#88417=CARTESIAN_POINT ( 'NONE',  ( 16.52544592524335698, 4.483927247898782831, 76.45942372801901854 ) ) ;
#88418=CARTESIAN_POINT ( 'NONE',  ( -12.06949235617756955, 12.14591786802309770, 50.62390960531435979 ) ) ;
#88419=CARTESIAN_POINT ( 'NONE',  ( -0.05219959533909027116, -19.03943276465977164, 57.49890960531435979 ) ) ;
#88420=CARTESIAN_POINT ( 'NONE',  ( -16.51473224551069308, -9.474510206698971260, 51.66557627198102409 ) ) ;
#88421=CARTESIAN_POINT ( 'NONE',  ( -16.53943276465976808, -0.05219959533934237506, 38.75109039468567573 ) ) ;
#88423=CARTESIAN_POINT ( 'NONE',  ( 13.97604488694548053, -13.89961937509957401, 95.62609039468563310 ) ) ;
#88424=CARTESIAN_POINT ( 'NONE',  ( -12.06949235617756955, 12.14591786802309770, 100.6239096053143811 ) ) ;
#88425=CARTESIAN_POINT ( 'NONE',  ( -5.153800228976328057, -19.02544592524343514, 62.29057627198100988 ) ) ;
#88426=CARTESIAN_POINT ( 'NONE',  ( 13.89961937509957401, 13.97604488694547697, 106.8760903946856757 ) ) ;
#88428=CARTESIAN_POINT ( 'NONE',  ( -15.80617190586768217, 15.72974639402176855, 108.1260903946856757 ) ) ;
#88429=CARTESIAN_POINT ( 'NONE',  ( -8.224510206698735004, -14.34966873604973081, 69.58442372801900433 ) ) ;
#88431=CARTESIAN_POINT ( 'NONE',  ( 15.80617190586746368, 15.72974639402197994, 69.37390960531436690 ) ) ;
#88432=CARTESIAN_POINT ( 'NONE',  ( -8.224510206698735004, -14.34966873604973081, 49.58442372801901143 ) ) ;
#88434=CARTESIAN_POINT ( 'NONE',  ( -16.51473224551082808, 9.474510206698731452, 53.33442372801900433 ) ) ;
#88435=CARTESIAN_POINT ( 'NONE',  ( 13.97604488694527802, 13.89961937509977652, 94.37390960531436690 ) ) ;
#88436=CARTESIAN_POINT ( 'NONE',  ( -16.53943276465976808, 0.05219959533911058130, 116.2489096053143669 ) ) ;
#88437=CARTESIAN_POINT ( 'NONE',  ( 16.51473224551069308, 9.474510206698969483, 59.16557627198102409 ) ) ;
#88438=CARTESIAN_POINT ( 'NONE',  ( -0.05219959533910754901, -16.53943276465976808, 52.49890960531435979 ) ) ;
#88439=CARTESIAN_POINT ( 'NONE',  ( -21.53943276465977519, -0.05219959533937600094, 73.75109039468567573 ) ) ;
#88440=CARTESIAN_POINT ( 'NONE',  ( 0.05219959533936267826, -19.03943276465977164, 50.00109039468566863 ) ) ;
#88441=CARTESIAN_POINT ( 'NONE',  ( 13.97604488694548053, -13.89961937509957401, 30.62609039468566863 ) ) ;
#88442=CARTESIAN_POINT ( 'NONE',  ( -13.97604488694527625, -13.89961937509977652, 51.87390960531436690 ) ) ;
#88443=CARTESIAN_POINT ( 'NONE',  ( 18.67979575497178502, 10.72451020669898547, 29.16557627198103120 ) ) ;
#88444=CARTESIAN_POINT ( 'NONE',  ( 5.823673210054444382, -21.52544592524334988, 90.20942372801903275 ) ) ;
#88445=CARTESIAN_POINT ( 'NONE',  ( 13.89961937509977652, -13.97604488694527269, 68.12390960531436690 ) ) ;
#88446=CARTESIAN_POINT ( 'NONE',  ( -10.72451020669870658, -18.67979575497194134, 89.58442372801901854 ) ) ;
#88447=CARTESIAN_POINT ( 'NONE',  ( 5.823673210054125526, 21.52544592524343514, 39.79057627198103830 ) ) ;
#88448=CARTESIAN_POINT ( 'NONE',  ( 16.51473224551069308, 9.474510206698969483, 89.16557627198103830 ) ) ;
#88449=CARTESIAN_POINT ( 'NONE',  ( 0.05219959533936267826, -19.03943276465977164, 65.00109039468567573 ) ) ;
#88450=CARTESIAN_POINT ( 'NONE',  ( 5.049401038298161559, -19.05341960407611168, 37.70724293864768839 ) ) ;
#88451=CARTESIAN_POINT ( 'NONE',  ( 19.05341960407611168, 5.049401038298154454, 93.95724293864769550 ) ) ;
#88452=CARTESIAN_POINT ( 'NONE',  ( -4.483927247898782831, 16.52544592524335698, 32.70942372801900433 ) ) ;
#88453=CARTESIAN_POINT ( 'NONE',  ( 8.224510206698953496, -14.34966873604960469, 97.91557627198103830 ) ) ;
#88454=CARTESIAN_POINT ( 'NONE',  ( -16.46253265017160317, 9.564922557960807481, 75.83224293864769550 ) ) ;
#88455=CARTESIAN_POINT ( 'NONE',  ( -0.05219959533907301413, -21.53943276465977519, 47.49890960531435979 ) ) ;
#88456=CARTESIAN_POINT ( 'NONE',  ( -13.89961937509957401, -13.97604488694547875, 109.3760903946856331 ) ) ;
#88457=CARTESIAN_POINT ( 'NONE',  ( 5.823673210054444382, -21.52544592524334988, 25.20942372801901854 ) ) ;
#88458=CARTESIAN_POINT ( 'NONE',  ( -10.72451020669870658, -18.67979575497194134, 64.58442372801900433 ) ) ;
#88459=CARTESIAN_POINT ( 'NONE',  ( 0.05219959533934541429, -16.53943276465976808, 65.00109039468568994 ) ) ;
#88461=CARTESIAN_POINT ( 'NONE',  ( -13.89961937509977652, 13.97604488694528158, 70.62390960531432427 ) ) ;
#88462=CARTESIAN_POINT ( 'NONE',  ( -12.14591786802326823, 12.06949235617739902, 98.12609039468570415 ) ) ;
#88463=CARTESIAN_POINT ( 'NONE',  ( -13.97604488694547697, 13.89961937509957934, 38.12609039468566152 ) ) ;
#88464=CARTESIAN_POINT ( 'NONE',  ( -0.05219959533937732626, 21.53943276465977519, 32.50109039468568284 ) ) ;
#88465=CARTESIAN_POINT ( 'NONE',  ( 12.06949235617757843, -12.14591786802309237, 63.12390960531435979 ) ) ;
#88466=CARTESIAN_POINT ( 'NONE',  ( 5.049401038298161559, -19.05341960407611168, 102.7072429386476955 ) ) ;
#88467=CARTESIAN_POINT ( 'NONE',  ( -12.06949235617739369, -12.14591786802326823, 84.37609039468570415 ) ) ;
#88468=CARTESIAN_POINT ( 'NONE',  ( 21.52544592524334988, 5.823673210054432836, 66.45942372801903275 ) ) ;
#88469=CARTESIAN_POINT ( 'NONE',  ( 12.06949235617739724, 12.14591786802326823, 26.87609039468567218 ) ) ;
#88470=CARTESIAN_POINT ( 'NONE',  ( 18.67979575497194134, -10.72451020669871369, 25.83442372801901499 ) ) ;
#88471=CARTESIAN_POINT ( 'NONE',  ( 12.06949235617757843, -12.14591786802309237, 63.12390960531435979 ) ) ;
#88472=VERTEX_POINT ( 'NONE', #96997 ) ;
#88473=CARTESIAN_POINT ( 'NONE',  ( 21.52544592524344225, -5.823673210054117533, 103.5405762719810383 ) ) ;
#88474=CARTESIAN_POINT ( 'NONE',  ( 16.55341960407611168, 4.379528057220329451, 38.95724293864768839 ) ) ;
#88476=CARTESIAN_POINT ( 'NONE',  ( -19.02544592524342804, 5.153800228976336051, 31.04057627198102409 ) ) ;
#88477=CARTESIAN_POINT ( 'NONE',  ( 10.81492255796078972, 18.62759615963270932, 24.58224293864768839 ) ) ;
#88478=CARTESIAN_POINT ( 'NONE',  ( -21.52544592524334988, -5.823673210054445271, 33.95942372801901143 ) ) ;
#88479=CARTESIAN_POINT ( 'NONE',  ( -0.05219959533910754901, -16.53943276465976808, 67.49890960531436690 ) ) ;
#88481=CARTESIAN_POINT ( 'NONE',  ( -21.53943276465977519, 0.05219959533907696930, 61.24890960531435979 ) ) ;
#88482=CARTESIAN_POINT ( 'NONE',  ( -13.89961937509977652, 13.97604488694528158, 75.62390960531438111 ) ) ;
#88484=CARTESIAN_POINT ( 'NONE',  ( -16.46253265017160317, 9.564922557960807481, 25.83224293864769194 ) ) ;
#88485=CARTESIAN_POINT ( 'NONE',  ( -16.51473224551082808, 9.474510206698731452, 73.33442372801900433 ) ) ;
#88486=CARTESIAN_POINT ( 'NONE',  ( -21.52544592524343514, 5.823673210054127303, 51.04057627198103120 ) ) ;
#88487=CARTESIAN_POINT ( 'NONE',  ( 16.46253265017160672, -9.564922557960803928, 43.33224293864769550 ) ) ;
#88488=CARTESIAN_POINT ( 'NONE',  ( 19.05341960407611168, 5.049401038298154454, 68.95724293864769550 ) ) ;
#88490=CARTESIAN_POINT ( 'NONE',  ( 14.29746914071037800, 8.314922557961029526, 31.66775706135234358 ) ) ;
#88491=CARTESIAN_POINT ( 'NONE',  ( 10.81492255796106328, -18.62759615963255655, 20.41775706135234714 ) ) ;
#88492=CARTESIAN_POINT ( 'NONE',  ( -0.05219959533910754901, -16.53943276465976808, 42.49890960531435979 ) ) ;
#88493=CARTESIAN_POINT ( 'NONE',  ( 21.52544592524334988, 5.823673210054432836, 61.45942372801901854 ) ) ;
#88494=CARTESIAN_POINT ( 'NONE',  ( 19.02544592524343514, -5.153800228976328945, 103.5405762719809957 ) ) ;
#88495=CARTESIAN_POINT ( 'NONE',  ( 5.719274019375991003, -21.55341960407610458, 72.70724293864769550 ) ) ;
#88496=CARTESIAN_POINT ( 'NONE',  ( 10.72451020669898902, -18.67979575497178502, 112.9155762719810383 ) ) ;
#88497=CARTESIAN_POINT ( 'NONE',  ( -8.224510206698735004, -14.34966873604973081, 49.58442372801901143 ) ) ;
#88499=CARTESIAN_POINT ( 'NONE',  ( 10.81492255796078972, 18.62759615963270932, 49.58224293864769550 ) ) ;
#88500=CARTESIAN_POINT ( 'NONE',  ( 10.72451020669871369, 18.67979575497193778, 107.0844237280190043 ) ) ;
#88501=CARTESIAN_POINT ( 'NONE',  ( 0.05219959533909260263, 19.03943276465977164, 49.99890960531435979 ) ) ;
#88502=CARTESIAN_POINT ( 'NONE',  ( -19.03943276465977164, 0.05219959533909376836, 96.24890960531436690 ) ) ;
#88503=CARTESIAN_POINT ( 'NONE',  ( -19.03943276465977164, 0.05219959533909376836, 81.24890960531436690 ) ) ;
#88505=CARTESIAN_POINT ( 'NONE',  ( -13.97604488694547697, 13.89961937509957934, 73.12609039468568994 ) ) ;
#88506=CARTESIAN_POINT ( 'NONE',  ( 13.89961937509957401, 13.97604488694547697, 21.87609039468566152 ) ) ;
#88507=CARTESIAN_POINT ( 'NONE',  ( -5.823673210054116645, -21.52544592524344225, 37.29057627198102409 ) ) ;
#88508=CARTESIAN_POINT ( 'NONE',  ( 0.05219959533934541429, -16.53943276465976808, 105.0010903946856757 ) ) ;
#88510=CARTESIAN_POINT ( 'NONE',  ( -19.05341960407617563, 5.049401038297882671, 88.54275706135230450 ) ) ;
#88511=CARTESIAN_POINT ( 'NONE',  ( -17.05116617787826172, 6.768360034955673399, 58.65675553259200115 ) ) ;
#88512=CARTESIAN_POINT ( 'NONE',  ( -10.81492255796105439, 18.62759615963255655, 112.9177570613523329 ) ) ;
#88513=CARTESIAN_POINT ( 'NONE',  ( 9.564922557961047289, -16.46253265017146816, 85.41775706135233293 ) ) ;
#88514=CARTESIAN_POINT ( 'NONE',  ( 5.153800228976615827, -19.02544592524334988, 50.20942372801897591 ) ) ;
#88516=CARTESIAN_POINT ( 'NONE',  ( 13.97604488694527802, 13.89961937509977652, 44.37390960531435269 ) ) ;
#88517=CARTESIAN_POINT ( 'NONE',  ( 0.05219959533910956823, 16.53943276465976808, 49.99890960531437401 ) ) ;
#88518=CARTESIAN_POINT ( 'NONE',  ( 0.05219959533909260263, 19.03943276465977164, 29.99890960531435979 ) ) ;
#88519=CARTESIAN_POINT ( 'NONE',  ( 4.379528057220339221, -16.55341960407611168, 37.70724293864769550 ) ) ;
#88520=CARTESIAN_POINT ( 'NONE',  ( -17.49999999999999645, -5.500000000000000888, 120.0000000000000142 ) ) ;
#88521=CARTESIAN_POINT ( 'NONE',  ( 16.53943276465976808, 0.05219959533934440121, 106.2510903946856757 ) ) ;
#88522=CARTESIAN_POINT ( 'NONE',  ( -16.46253265017160317, 9.564922557960807481, 55.83224293864769550 ) ) ;
#88523=CARTESIAN_POINT ( 'NONE',  ( -15.80617190586768217, 15.72974639402176855, 113.1260903946856899 ) ) ;
#88524=CARTESIAN_POINT ( 'NONE',  ( -14.34966873604972548, 8.224510206698743886, 33.33442372801900433 ) ) ;
#88525=CARTESIAN_POINT ( 'NONE',  ( 21.55341960407610458, 5.719274019375980345, 43.95724293864769550 ) ) ;
#88526=CARTESIAN_POINT ( 'NONE',  ( 10.72451020669871369, 18.67979575497193778, 87.08442372801901854 ) ) ;
#88528=CARTESIAN_POINT ( 'NONE',  ( -9.474510206698964154, 16.51473224551069663, 100.4155762719810241 ) ) ;
#88529=CARTESIAN_POINT ( 'NONE',  ( -16.51473224551069308, -9.474510206698971260, 86.66557627198102409 ) ) ;
#88531=CARTESIAN_POINT ( 'NONE',  ( -15.72974639402197994, 15.80617190586746368, 110.6239096053143669 ) ) ;
#88532=CARTESIAN_POINT ( 'NONE',  ( 0.05219959533910956823, 16.53943276465976808, 79.99890960531435269 ) ) ;
#88533=CARTESIAN_POINT ( 'NONE',  ( 18.67979575497178502, 10.72451020669898547, 69.16557627198102409 ) ) ;
#88534=CARTESIAN_POINT ( 'NONE',  ( 13.89961937509977652, -13.97604488694527269, 73.12390960531436690 ) ) ;
#88535=CARTESIAN_POINT ( 'NONE',  ( 0.05219959533909260263, 19.03943276465977164, 74.99890960531435269 ) ) ;
#88536=CARTESIAN_POINT ( 'NONE',  ( 21.55341960407610458, 5.719274019375980345, 93.95724293864770971 ) ) ;
#88537=EDGE_LOOP ( 'NONE', ( #25645, #176271, #76669, #64102, #170590, #176458, #187765, #195446 ) ) ;
#88538=CARTESIAN_POINT ( 'NONE',  ( 16.51473224551069308, 9.474510206698969483, 54.16557627198103120 ) ) ;
#88539=CARTESIAN_POINT ( 'NONE',  ( 16.55341960407611168, 4.379528057220329451, 93.95724293864770971 ) ) ;
#88540=CARTESIAN_POINT ( 'NONE',  ( 19.02544592524343514, -5.153800228976328945, 23.54057627198102054 ) ) ;
#88541=CARTESIAN_POINT ( 'NONE',  ( -13.89961937509977652, 13.97604488694528158, 65.62390960531436690 ) ) ;
#88542=CARTESIAN_POINT ( 'NONE',  ( 19.05341960407617918, -5.049401038297876454, 76.04275706135230450 ) ) ;
#88543=CARTESIAN_POINT ( 'NONE',  ( -8.314922557960811034, -14.29746914071050412, 92.08224293864769550 ) ) ;
#88544=CARTESIAN_POINT ( 'NONE',  ( -21.53943276465977519, -0.05219959533937600094, 58.75109039468568994 ) ) ;
#88545=CARTESIAN_POINT ( 'NONE',  ( 19.03943276465977164, -0.05219959533909143690, 48.74890960531435979 ) ) ;
#88546=CARTESIAN_POINT ( 'NONE',  ( -18.62759615963270932, 10.81492255796079327, 115.8322429386477097 ) ) ;
#88547=CARTESIAN_POINT ( 'NONE',  ( -0.05219959533910754901, -16.53943276465976808, 97.49890960531436690 ) ) ;
#88549=CARTESIAN_POINT ( 'NONE',  ( -13.89961937509977652, 13.97604488694528158, 55.62390960531434558 ) ) ;
#88551=CARTESIAN_POINT ( 'NONE',  ( 16.51473224551083163, -9.474510206698727899, 105.8344237280190043 ) ) ;
#88552=CARTESIAN_POINT ( 'NONE',  ( 13.89961937509977652, -13.97604488694527269, 113.1239096053143527 ) ) ;
#88553=CARTESIAN_POINT ( 'NONE',  ( 18.62759615963255655, 10.81492255796105972, 46.66775706135234714 ) ) ;
#88554=CARTESIAN_POINT ( 'NONE',  ( 19.02544592524343514, -5.153800228976328945, 98.54057627198100988 ) ) ;
#88555=CARTESIAN_POINT ( 'NONE',  ( -9.474510206698720793, -16.51473224551083518, 84.58442372801900433 ) ) ;
#88556=CARTESIAN_POINT ( 'NONE',  ( -0.05219959533909027116, -19.03943276465977164, 57.49890960531435979 ) ) ;
#88557=CARTESIAN_POINT ( 'NONE',  ( 16.53943276465976808, -0.05219959533910856209, 78.74890960531436690 ) ) ;
#88558=CARTESIAN_POINT ( 'NONE',  ( 16.46253265017160672, -9.564922557960803928, 83.33224293864768129 ) ) ;
#88559=CARTESIAN_POINT ( 'NONE',  ( -14.29746914071049879, 8.314922557960819915, 75.83224293864769550 ) ) ;
#88560=CARTESIAN_POINT ( 'NONE',  ( -9.564922557960796823, -16.46253265017161027, 87.08224293864769550 ) ) ;
#88562=CARTESIAN_POINT ( 'NONE',  ( -13.89961937509957401, -13.97604488694547875, 44.37609039468566863 ) ) ;
#88563=CARTESIAN_POINT ( 'NONE',  ( 13.97604488694527802, 13.89961937509977652, 44.37390960531435269 ) ) ;
#88564=CARTESIAN_POINT ( 'NONE',  ( 16.52544592524342804, -4.483927247898539470, 38.54057627198103120 ) ) ;
#88565=CARTESIAN_POINT ( 'NONE',  ( 16.46253265017160672, -9.564922557960803928, 28.33224293864769550 ) ) ;
#88567=CARTESIAN_POINT ( 'NONE',  ( -15.80617190586768217, 15.72974639402176855, 43.12609039468568284 ) ) ;
#88568=CARTESIAN_POINT ( 'NONE',  ( 19.03943276465977164, 0.05219959533936151252, 76.25109039468566152 ) ) ;
#88569=CARTESIAN_POINT ( 'NONE',  ( 12.14591786802309770, 12.06949235617756955, 34.37390960531435979 ) ) ;
#88570=CARTESIAN_POINT ( 'NONE',  ( 10.81492255796078972, 18.62759615963270932, 99.58224293864770971 ) ) ;
#88571=CARTESIAN_POINT ( 'NONE',  ( -21.52544592524343514, 5.823673210054127303, 36.04057627198102409 ) ) ;
#88572=CARTESIAN_POINT ( 'NONE',  ( -16.55341960407611168, -4.379528057220339221, 76.45724293864769550 ) ) ;
#88573=CARTESIAN_POINT ( 'NONE',  ( -0.05219959533909027116, -19.03943276465977164, 42.49890960531435269 ) ) ;
#88574=CARTESIAN_POINT ( 'NONE',  ( 0.05219959533934541429, -16.53943276465976808, 100.0010903946857042 ) ) ;
#88575=CARTESIAN_POINT ( 'NONE',  ( -14.29746914071037622, -8.314922557961029526, 69.16775706135234714 ) ) ;
#88576=CARTESIAN_POINT ( 'NONE',  ( -19.02544592524334988, -5.153800228976617603, 23.95942372801900078 ) ) ;
#88577=CARTESIAN_POINT ( 'NONE',  ( 5.049401038298161559, -19.05341960407611168, 92.70724293864769550 ) ) ;
#88578=CARTESIAN_POINT ( 'NONE',  ( 16.46253265017160672, -9.564922557960803928, 83.33224293864768129 ) ) ;
#88579=CARTESIAN_POINT ( 'NONE',  ( -16.52544592524335698, -4.483927247898792601, 73.95942372801901854 ) ) ;
#88580=CARTESIAN_POINT ( 'NONE',  ( 19.03943276465977164, -0.05219959533909143690, 33.74890960531435979 ) ) ;
#88581=CARTESIAN_POINT ( 'NONE',  ( 16.52544592524342804, -4.483927247898539470, 43.54057627198103830 ) ) ;
#88582=CARTESIAN_POINT ( 'NONE',  ( -13.97604488694527625, -13.89961937509977652, 101.8739096053143811 ) ) ;
#88583=CARTESIAN_POINT ( 'NONE',  ( -16.46253265017160317, 9.564922557960807481, 90.83224293864769550 ) ) ;
#88584=CARTESIAN_POINT ( 'NONE',  ( -21.55341960407610458, -5.719274019375992779, 26.45724293864768839 ) ) ;
#88585=CARTESIAN_POINT ( 'NONE',  ( -12.06949235617756955, 12.14591786802309770, 70.62390960531436690 ) ) ;
#88586=VERTEX_POINT ( 'NONE', #45319 ) ;
#88587=CARTESIAN_POINT ( 'NONE',  ( -14.29746914071049879, 8.314922557960819915, 65.83224293864769550 ) ) ;
#88588=CARTESIAN_POINT ( 'NONE',  ( 4.379528057220092307, 16.55341960407617563, 52.29275706135236135 ) ) ;
#88589=CARTESIAN_POINT ( 'NONE',  ( 17.49999999999999645, -3.237210098469573971, 32.21236987379557348 ) ) ;
#88591=CARTESIAN_POINT ( 'NONE',  ( -19.02544592524334988, -5.153800228976617603, 68.95942372801896170 ) ) ;
#88592=CARTESIAN_POINT ( 'NONE',  ( 5.153800228976335163, 19.02544592524342804, 84.79057627198099567 ) ) ;
#88593=CARTESIAN_POINT ( 'NONE',  ( 9.474510206698729675, 16.51473224551082808, 62.08442372801899722 ) ) ;
#88595=CARTESIAN_POINT ( 'NONE',  ( -14.29746914071037622, -8.314922557961029526, 19.16775706135234714 ) ) ;
#88596=CARTESIAN_POINT ( 'NONE',  ( -12.14591786802326823, 12.06949235617739902, 98.12609039468570415 ) ) ;
#88597=MECHANICAL_DESIGN_GEOMETRIC_PRESENTATION_REPRESENTATION('',(#149949),#198437);
#88598=CARTESIAN_POINT ( 'NONE',  ( -5.153800228976328057, -19.02544592524343514, 42.29057627198101699 ) ) ;
#88599=CARTESIAN_POINT ( 'NONE',  ( 18.62759615963271287, -10.81492255796078972, 28.33224293864769550 ) ) ;
#88600=CARTESIAN_POINT ( 'NONE',  ( -10.81492255796105439, 18.62759615963255655, 57.91775706135234714 ) ) ;
#88601=CARTESIAN_POINT ( 'NONE',  ( -9.564922557961040184, 16.46253265017147172, 102.9177570613523329 ) ) ;
#88603=CARTESIAN_POINT ( 'NONE',  ( 19.05341960407611168, 5.049401038298154454, 73.95724293864768129 ) ) ;
#88605=CARTESIAN_POINT ( 'NONE',  ( 8.224510206698953496, -14.34966873604960469, 77.91557627198102409 ) ) ;
#88606=CARTESIAN_POINT ( 'NONE',  ( -16.51473224551069308, -9.474510206698971260, 76.66557627198103830 ) ) ;
#88607=CARTESIAN_POINT ( 'NONE',  ( -19.02544592524342804, 5.153800228976336051, 76.04057627198102409 ) ) ;
#88608=CARTESIAN_POINT ( 'NONE',  ( 9.564922557961047289, -16.46253265017146816, 85.41775706135233293 ) ) ;
#88609=CARTESIAN_POINT ( 'NONE',  ( 21.52544592524344225, -5.823673210054117533, 63.54057627198103830 ) ) ;
#88610=CARTESIAN_POINT ( 'NONE',  ( 19.03943276465977164, -0.05219959533909143690, 33.74890960531435979 ) ) ;
#88611=CARTESIAN_POINT ( 'NONE',  ( 19.03943276465977164, 0.05219959533936151252, 61.25109039468566863 ) ) ;
#88612=CARTESIAN_POINT ( 'NONE',  ( -13.97604488694527625, -13.89961937509977652, 51.87390960531436690 ) ) ;
#88613=CARTESIAN_POINT ( 'NONE',  ( 9.474510206698971260, -16.51473224551069308, 87.91557627198102409 ) ) ;
#88615=CARTESIAN_POINT ( 'NONE',  ( -5.823673210054116645, -21.52544592524344225, 92.29057627198103830 ) ) ;
#88616=CARTESIAN_POINT ( 'NONE',  ( 12.06949235617757843, -12.14591786802309237, 93.12390960531436690 ) ) ;
#88617=CARTESIAN_POINT ( 'NONE',  ( -16.51473224551082808, 9.474510206698731452, 48.33442372801900433 ) ) ;
#88618=CARTESIAN_POINT ( 'NONE',  ( 5.823673210054125526, 21.52544592524343514, 79.79057627198102409 ) ) ;
#88619=CARTESIAN_POINT ( 'NONE',  ( 10.81492255796078972, 18.62759615963270932, 54.58224293864769550 ) ) ;
#88620=CARTESIAN_POINT ( 'NONE',  ( 16.52544592524342804, -4.483927247898539470, 28.54057627198103120 ) ) ;
#88621=CARTESIAN_POINT ( 'NONE',  ( -21.55341960407619339, 5.719274019375674811, 103.5427570613523613 ) ) ;
#88622=CARTESIAN_POINT ( 'NONE',  ( 13.89961937509977652, -13.97604488694527269, 73.12390960531436690 ) ) ;
#88623=CARTESIAN_POINT ( 'NONE',  ( -19.03943276465977164, 0.05219959533909376836, 36.24890960531436690 ) ) ;
#88625=CARTESIAN_POINT ( 'NONE',  ( 10.81492255796106328, -18.62759615963255655, 35.41775706135234003 ) ) ;
#88626=EDGE_CURVE ( 'NONE', #45948, #135096, #71751, .T. ) ;
#88627=CARTESIAN_POINT ( 'NONE',  ( -21.52544592524334988, -5.823673210054445271, 58.95942372801902565 ) ) ;
#88628=CARTESIAN_POINT ( 'NONE',  ( 13.97604488694527802, 13.89961937509977652, 49.37390960531434558 ) ) ;
#88629=CARTESIAN_POINT ( 'NONE',  ( -10.81492255796105439, 18.62759615963255655, 27.91775706135234358 ) ) ;
#88630=CARTESIAN_POINT ( 'NONE',  ( 9.474510206698729675, 16.51473224551082808, 62.08442372801899722 ) ) ;
#88631=CARTESIAN_POINT ( 'NONE',  ( -16.51473224551069308, -9.474510206698971260, 31.66557627198102054 ) ) ;
#88632=CARTESIAN_POINT ( 'NONE',  ( -8.224510206698735004, -14.34966873604973081, 34.58442372801900433 ) ) ;
#88633=CARTESIAN_POINT ( 'NONE',  ( -13.97604488694527625, -13.89961937509977652, 31.87390960531435979 ) ) ;
#88634=CARTESIAN_POINT ( 'NONE',  ( -14.34966873604972548, 8.224510206698743886, 78.33442372801901854 ) ) ;
#88635=CARTESIAN_POINT ( 'NONE',  ( -19.02544592524342804, 5.153800228976336051, 36.04057627198100988 ) ) ;
#88637=CARTESIAN_POINT ( 'NONE',  ( -16.51473224551069308, -9.474510206698971260, 91.66557627198103830 ) ) ;
#88638=CARTESIAN_POINT ( 'NONE',  ( 5.153800228976335163, 19.02544592524342804, 24.79057627198102765 ) ) ;
#88639=CARTESIAN_POINT ( 'NONE',  ( 5.823673210054125526, 21.52544592524343514, 69.79057627198102409 ) ) ;
#88640=CARTESIAN_POINT ( 'NONE',  ( -4.379528057220086978, -16.55341960407618274, 49.79275706135234714 ) ) ;
#88641=CARTESIAN_POINT ( 'NONE',  ( -5.823673210054431948, 21.52544592524334988, 102.7094237280190185 ) ) ;
#88642=CARTESIAN_POINT ( 'NONE',  ( 19.02544592524343514, -5.153800228976328945, 43.54057627198103120 ) ) ;
#88643=CARTESIAN_POINT ( 'NONE',  ( -4.483927247898539470, -16.52544592524342804, 27.29057627198103120 ) ) ;
#88644=CARTESIAN_POINT ( 'NONE',  ( 0.05219959533910956823, 16.53943276465976808, 64.99890960531435269 ) ) ;
#88645=CARTESIAN_POINT ( 'NONE',  ( -13.97604488694527625, -13.89961937509977652, 66.87390960531436690 ) ) ;
#88646=CARTESIAN_POINT ( 'NONE',  ( -0.05219959533937732626, 21.53943276465977519, 107.5010903946856899 ) ) ;
#88647=CARTESIAN_POINT ( 'NONE',  ( -21.55341960407619339, 5.719274019375674811, 23.54275706135235424 ) ) ;
#88648=CARTESIAN_POINT ( 'NONE',  ( 5.049401038298161559, -19.05341960407611168, 82.70724293864770971 ) ) ;
#88649=CARTESIAN_POINT ( 'NONE',  ( -5.719274019375665041, -21.55341960407619695, 89.79275706135236135 ) ) ;
#88650=CARTESIAN_POINT ( 'NONE',  ( -4.379528057220086978, -16.55341960407618274, 69.79275706135234714 ) ) ;
#88651=CARTESIAN_POINT ( 'NONE',  ( 8.314922557961029526, -14.29746914071037800, 35.41775706135234003 ) ) ;
#88652=CARTESIAN_POINT ( 'NONE',  ( -16.55341960407611168, -4.379528057220339221, 96.45724293864770971 ) ) ;
#88653=CARTESIAN_POINT ( 'NONE',  ( 10.81492255796106328, -18.62759615963255655, 105.4177570613523613 ) ) ;
#88654=CARTESIAN_POINT ( 'NONE',  ( 8.314922557960818139, 14.29746914071049879, 34.58224293864770260 ) ) ;
#88655=CARTESIAN_POINT ( 'NONE',  ( -19.05341960407611168, -5.049401038298163336, 31.45724293864769550 ) ) ;
#88656=CARTESIAN_POINT ( 'NONE',  ( 14.34966873604972726, -8.224510206698740333, 50.83442372801901143 ) ) ;
#88657=CARTESIAN_POINT ( 'NONE',  ( 8.314922557960818139, 14.29746914071049879, 49.58224293864769550 ) ) ;
#88658=CARTESIAN_POINT ( 'NONE',  ( -16.53943276465976808, -0.05219959533934237506, 98.75109039468568994 ) ) ;
#88659=CARTESIAN_POINT ( 'NONE',  ( 15.72974639402199770, -15.80617190586745480, 23.12390960531436335 ) ) ;
#88660=CARTESIAN_POINT ( 'NONE',  ( -18.67979575497178146, -10.72451020669898902, 36.66557627198103120 ) ) ;
#88661=CARTESIAN_POINT ( 'NONE',  ( -21.53943276465977519, -0.05219959533937600094, 108.7510903946857042 ) ) ;
#88662=ADVANCED_FACE ( 'NONE', ( #127920 ), #191598, .F. ) ;
#88663=CARTESIAN_POINT ( 'NONE',  ( -8.224510206698948167, 14.34966873604960824, 80.41557627198103830 ) ) ;
#88664=CARTESIAN_POINT ( 'NONE',  ( 13.89961937509977652, -13.97604488694527269, 93.12390960531436690 ) ) ;
#88666=CARTESIAN_POINT ( 'NONE',  ( 8.314922557961029526, -14.29746914071037800, 45.41775706135234003 ) ) ;
#88667=CARTESIAN_POINT ( 'NONE',  ( -13.97604488694527625, -13.89961937509977652, 36.87390960531436690 ) ) ;
#88668=CARTESIAN_POINT ( 'NONE',  ( -16.52544592524335698, -4.483927247898792601, 38.95942372801901854 ) ) ;
#88670=CARTESIAN_POINT ( 'NONE',  ( 5.153800228976615827, -19.02544592524334988, 55.20942372801899722 ) ) ;
#88671=CARTESIAN_POINT ( 'NONE',  ( -13.97604488694527625, -13.89961937509977652, 51.87390960531436690 ) ) ;
#88672=CARTESIAN_POINT ( 'NONE',  ( -8.224510206698735004, -14.34966873604973081, 74.58442372801901854 ) ) ;
#88673=CARTESIAN_POINT ( 'NONE',  ( 13.97604488694548053, -13.89961937509957401, 100.6260903946856615 ) ) ;
#88674=CARTESIAN_POINT ( 'NONE',  ( -5.153800228976607833, 19.02544592524334988, 32.70942372801899722 ) ) ;
#88675=CARTESIAN_POINT ( 'NONE',  ( -19.03943276465977164, 0.05219959533909376836, 66.24890960531436690 ) ) ;
#88677=CARTESIAN_POINT ( 'NONE',  ( 16.53943276465976808, -0.05219959533910856209, 93.74890960531436690 ) ) ;
#88678=CARTESIAN_POINT ( 'NONE',  ( 5.153800228976615827, -19.02544592524334988, 65.20942372801900433 ) ) ;
#88679=CARTESIAN_POINT ( 'NONE',  ( 15.72974639402199770, -15.80617190586745480, 68.12390960531436690 ) ) ;
#88680=CARTESIAN_POINT ( 'NONE',  ( 9.564922557961047289, -16.46253265017146816, 35.41775706135233293 ) ) ;
#88681=CARTESIAN_POINT ( 'NONE',  ( -5.049401038298153566, 19.05341960407611168, 110.2072429386476671 ) ) ;
#88683=CARTESIAN_POINT ( 'NONE',  ( 0.05219959533907565091, 21.53943276465977519, 84.99890960531436690 ) ) ;
#88684=CARTESIAN_POINT ( 'NONE',  ( -16.61371651742600619, 7.165104196376140600, 83.85415069992994574 ) ) ;
#88685=CARTESIAN_POINT ( 'NONE',  ( -19.05341960407617563, 5.049401038297882671, 98.54275706135233293 ) ) ;
#88687=CARTESIAN_POINT ( 'NONE',  ( 4.379528057220092307, 16.55341960407617563, 27.29275706135234358 ) ) ;
#88688=CARTESIAN_POINT ( 'NONE',  ( -13.89961937509977652, 13.97604488694528158, 45.62390960531433848 ) ) ;
#88689=CARTESIAN_POINT ( 'NONE',  ( -15.80617190586745835, -15.72974639402198527, 21.87390960531436690 ) ) ;
#88690=CARTESIAN_POINT ( 'NONE',  ( 5.719274019375991003, -21.55341960407610458, 92.70724293864770971 ) ) ;
#88691=CARTESIAN_POINT ( 'NONE',  ( 5.823673210054444382, -21.52544592524334988, 65.20942372801901854 ) ) ;
#88692=CARTESIAN_POINT ( 'NONE',  ( -0.05219959533936034679, 19.03943276465977164, 112.5010903946856757 ) ) ;
#88693=CARTESIAN_POINT ( 'NONE',  ( 18.67979575497194134, -10.72451020669871369, 105.8344237280190328 ) ) ;
#88694=CARTESIAN_POINT ( 'NONE',  ( -16.55341960407611168, -4.379528057220339221, 21.45724293864769550 ) ) ;
#88695=CARTESIAN_POINT ( 'NONE',  ( 5.719274019375991003, -21.55341960407610458, 97.70724293864772392 ) ) ;
#88696=CARTESIAN_POINT ( 'NONE',  ( -16.53943276465976808, 0.05219959533911058130, 56.24890960531436690 ) ) ;
#88697=CARTESIAN_POINT ( 'NONE',  ( -9.564922557961040184, 16.46253265017147172, 82.91775706135233293 ) ) ;
#88698=CARTESIAN_POINT ( 'NONE',  ( 19.03943276465977164, 0.05219959533936151252, 56.25109039468566863 ) ) ;
#88699=CARTESIAN_POINT ( 'NONE',  ( 15.72974639402176855, 15.80617190586768217, 66.87609039468568994 ) ) ;
#88700=CARTESIAN_POINT ( 'NONE',  ( 9.564922557961047289, -16.46253265017146816, 35.41775706135233293 ) ) ;
#88701=CARTESIAN_POINT ( 'NONE',  ( -0.05219959533909027116, -19.03943276465977164, 22.49890960531436690 ) ) ;
#88702=CARTESIAN_POINT ( 'NONE',  ( -15.80617190586745835, -15.72974639402198527, 41.87390960531435979 ) ) ;
#88703=CARTESIAN_POINT ( 'NONE',  ( -16.52544592524342804, 4.483927247898546575, 36.04057627198102409 ) ) ;
#88704=CARTESIAN_POINT ( 'NONE',  ( 10.72451020669871369, 18.67979575497193778, 107.0844237280190043 ) ) ;
#88705=CARTESIAN_POINT ( 'NONE',  ( -0.05219959533934338120, 16.53943276465976808, 67.50109039468568994 ) ) ;
#88706=CARTESIAN_POINT ( 'NONE',  ( 8.224510206698953496, -14.34966873604960469, 42.91557627198103120 ) ) ;
#88707=CARTESIAN_POINT ( 'NONE',  ( 5.719274019375673035, 21.55341960407619339, 62.29275706135236845 ) ) ;
#88708=CARTESIAN_POINT ( 'NONE',  ( 10.72451020669871369, 18.67979575497193778, 72.08442372801899012 ) ) ;
#88709=CARTESIAN_POINT ( 'NONE',  ( 21.52544592524344225, -5.823673210054117533, 68.54057627198103830 ) ) ;
#88712=CARTESIAN_POINT ( 'NONE',  ( -19.03943276465977164, 0.05219959533909376836, 21.24890960531436335 ) ) ;
#88713=CARTESIAN_POINT ( 'NONE',  ( 5.719274019375673035, 21.55341960407619339, 37.29275706135235424 ) ) ;
#88714=CARTESIAN_POINT ( 'NONE',  ( -8.314922557960811034, -14.29746914071050412, 112.0822429386477097 ) ) ;
#88715=CARTESIAN_POINT ( 'NONE',  ( 13.89961937509977652, -13.97604488694527269, 33.12390960531434558 ) ) ;
#88716=CARTESIAN_POINT ( 'NONE',  ( -0.05219959533910754901, -16.53943276465976808, 87.49890960531436690 ) ) ;
#88717=CARTESIAN_POINT ( 'NONE',  ( 5.153800228976335163, 19.02544592524342804, 89.79057627198102409 ) ) ;
#88718=CARTESIAN_POINT ( 'NONE',  ( -4.483927247898539470, -16.52544592524342804, 22.29057627198102765 ) ) ;
#88719=CARTESIAN_POINT ( 'NONE',  ( 8.224510206698953496, -14.34966873604960469, 97.91557627198103830 ) ) ;
#88720=CARTESIAN_POINT ( 'NONE',  ( -15.80617190586745835, -15.72974639402198527, 71.87390960531438111 ) ) ;
#88721=CARTESIAN_POINT ( 'NONE',  ( 18.67979575497178502, 10.72451020669898547, 104.1655762719810241 ) ) ;
#88723=CARTESIAN_POINT ( 'NONE',  ( -13.97604488694527625, -13.89961937509977652, 66.87390960531436690 ) ) ;
#88724=CARTESIAN_POINT ( 'NONE',  ( 16.52544592524335698, 4.483927247898782831, 26.45942372801901854 ) ) ;
#88725=CARTESIAN_POINT ( 'NONE',  ( 10.81492255796078972, 18.62759615963270932, 54.58224293864769550 ) ) ;
#88727=CARTESIAN_POINT ( 'NONE',  ( 5.719274019375673035, 21.55341960407619339, 87.29275706135236135 ) ) ;
#88728=CARTESIAN_POINT ( 'NONE',  ( 13.89961937509977652, -13.97604488694527269, 83.12390960531436690 ) ) ;
#88729=CARTESIAN_POINT ( 'NONE',  ( -19.03943276465977164, 0.05219959533909376836, 106.2489096053143669 ) ) ;
#88730=CARTESIAN_POINT ( 'NONE',  ( -16.55341960407617563, 4.379528057220093196, 78.54275706135236135 ) ) ;
#88731=CARTESIAN_POINT ( 'NONE',  ( 10.81492255796106328, -18.62759615963255655, 75.41775706135233293 ) ) ;
#88732=CARTESIAN_POINT ( 'NONE',  ( 18.67979575497194134, -10.72451020669871369, 105.8344237280190328 ) ) ;
#88733=CARTESIAN_POINT ( 'NONE',  ( 8.314922557961029526, -14.29746914071037800, 65.41775706135234714 ) ) ;
#88734=CARTESIAN_POINT ( 'NONE',  ( -18.67979575497178146, -10.72451020669898902, 111.6655762719810525 ) ) ;
#88736=CARTESIAN_POINT ( 'NONE',  ( -0.05219959533909027116, -19.03943276465977164, 112.4989096053143669 ) ) ;
#88737=CARTESIAN_POINT ( 'NONE',  ( -0.05219959533907301413, -21.53943276465977519, 87.49890960531436690 ) ) ;
#88738=CARTESIAN_POINT ( 'NONE',  ( 13.97604488694548053, -13.89961937509957401, 50.62609039468566152 ) ) ;
#88739=CARTESIAN_POINT ( 'NONE',  ( 15.72974639402199770, -15.80617190586745480, 48.12390960531436690 ) ) ;
#88740=CARTESIAN_POINT ( 'NONE',  ( -19.05341960407611168, -5.049401038298163336, 91.45724293864766707 ) ) ;
#88741=CARTESIAN_POINT ( 'NONE',  ( -8.314922557960811034, -14.29746914071050412, 37.08224293864768129 ) ) ;
#88745=CARTESIAN_POINT ( 'NONE',  ( 19.05341960407617918, -5.049401038297876454, 111.0427570613523329 ) ) ;
#88746=CARTESIAN_POINT ( 'NONE',  ( 10.81492255796078972, 18.62759615963270932, 89.58224293864768129 ) ) ;
#88747=CARTESIAN_POINT ( 'NONE',  ( -12.06949235617756955, 12.14591786802309770, 45.62390960531436690 ) ) ;
#88748=CARTESIAN_POINT ( 'NONE',  ( -16.55341960407617563, 4.379528057220093196, 33.54275706135234714 ) ) ;
#88749=CARTESIAN_POINT ( 'NONE',  ( -16.46253265017160317, 9.564922557960807481, 45.83224293864769550 ) ) ;
#88750=CARTESIAN_POINT ( 'NONE',  ( 21.53943276465977519, -0.05219959533907433946, 108.7489096053143669 ) ) ;
#88751=CARTESIAN_POINT ( 'NONE',  ( 19.05341960407617918, -5.049401038297876454, 91.04275706135234714 ) ) ;
#88752=CARTESIAN_POINT ( 'NONE',  ( -9.564922557960796823, -16.46253265017161027, 82.08224293864768129 ) ) ;
#88753=CARTESIAN_POINT ( 'NONE',  ( -9.474510206698964154, 16.51473224551069663, 75.41557627198103830 ) ) ;
#88754=CARTESIAN_POINT ( 'NONE',  ( -0.05219959533907301413, -21.53943276465977519, 82.49890960531436690 ) ) ;
#88755=CARTESIAN_POINT ( 'NONE',  ( 9.474510206698971260, -16.51473224551069308, 37.91557627198102409 ) ) ;
#88757=CARTESIAN_POINT ( 'NONE',  ( -14.34966873604960291, -8.224510206698953496, 61.66557627198103120 ) ) ;
#88758=CARTESIAN_POINT ( 'NONE',  ( 16.51473224551069308, 9.474510206698969483, 84.16557627198102409 ) ) ;
#88760=CARTESIAN_POINT ( 'NONE',  ( -0.05219959533936034679, 19.03943276465977164, 67.50109039468566152 ) ) ;
#88761=CARTESIAN_POINT ( 'NONE',  ( -21.55341960407610458, -5.719274019375992779, 51.45724293864770260 ) ) ;
#88762=CARTESIAN_POINT ( 'NONE',  ( 0.05219959533907565091, 21.53943276465977519, 74.99890960531435269 ) ) ;
#88763=CARTESIAN_POINT ( 'NONE',  ( 13.89961937509957401, 13.97604488694547697, 31.87609039468566863 ) ) ;
#88764=CARTESIAN_POINT ( 'NONE',  ( -19.02544592524342804, 5.153800228976336051, 101.0405762719810241 ) ) ;
#88766=CARTESIAN_POINT ( 'NONE',  ( -18.67979575497178146, -10.72451020669898902, 31.66557627198102054 ) ) ;
#88767=CARTESIAN_POINT ( 'NONE',  ( 5.049401038298161559, -19.05341960407611168, 77.70724293864765286 ) ) ;
#88768=CARTESIAN_POINT ( 'NONE',  ( -21.52544592524334988, -5.823673210054445271, 48.95942372801902565 ) ) ;
#88769=CARTESIAN_POINT ( 'NONE',  ( 16.51473224551069308, 9.474510206698969483, 29.16557627198103475 ) ) ;
#88770=CARTESIAN_POINT ( 'NONE',  ( 5.823673210054125526, 21.52544592524343514, 114.7905762719810383 ) ) ;
#88772=CARTESIAN_POINT ( 'NONE',  ( -15.72974639402176322, -15.80617190586768395, 39.37609039468567573 ) ) ;
#88774=CARTESIAN_POINT ( 'NONE',  ( 19.03943276465977164, -0.05219959533909143690, 98.74890960531436690 ) ) ;
#88776=CARTESIAN_POINT ( 'NONE',  ( 21.52544592524344225, -5.823673210054117533, 113.5405762719810383 ) ) ;
#88777=CARTESIAN_POINT ( 'NONE',  ( -19.03943276465977164, 0.05219959533909376836, 66.24890960531436690 ) ) ;
#88778=CARTESIAN_POINT ( 'NONE',  ( 4.483927247898790824, -16.52544592524335698, 20.20942372801900788 ) ) ;
#88780=CARTESIAN_POINT ( 'NONE',  ( 5.719274019375673035, 21.55341960407619339, 107.2927570613523471 ) ) ;
#88781=CARTESIAN_POINT ( 'NONE',  ( -19.05341960407611168, -5.049401038298163336, 41.45724293864769550 ) ) ;
#88782=CARTESIAN_POINT ( 'NONE',  ( -21.53943276465977519, -0.05219959533937600094, 98.75109039468568994 ) ) ;
#88783=CARTESIAN_POINT ( 'NONE',  ( 9.564922557960805705, 16.46253265017160317, 89.58224293864769550 ) ) ;
#88784=CARTESIAN_POINT ( 'NONE',  ( -21.55341960407619339, 5.719274019375674811, 53.54275706135234714 ) ) ;
#88786=CARTESIAN_POINT ( 'NONE',  ( -5.049401038298153566, 19.05341960407611168, 115.2072429386477097 ) ) ;
#88788=CARTESIAN_POINT ( 'NONE',  ( -16.52544592524335698, -4.483927247898792601, 58.95942372801902565 ) ) ;
#88789=CARTESIAN_POINT ( 'NONE',  ( -12.06949235617739369, -12.14591786802326823, 64.37609039468568994 ) ) ;
#88790=CARTESIAN_POINT ( 'NONE',  ( -5.823673210054431948, 21.52544592524334988, 62.70942372801902565 ) ) ;
#88791=CARTESIAN_POINT ( 'NONE',  ( -10.81492255796105439, 18.62759615963255655, 87.91775706135234714 ) ) ;
#88793=CARTESIAN_POINT ( 'NONE',  ( 8.224510206698742110, 14.34966873604972548, 32.08442372801901854 ) ) ;
#88794=CARTESIAN_POINT ( 'NONE',  ( -13.89961937509977652, 13.97604488694528158, 75.62390960531438111 ) ) ;
#88795=CARTESIAN_POINT ( 'NONE',  ( 9.474510206698971260, -16.51473224551069308, 112.9155762719810383 ) ) ;
#88796=CARTESIAN_POINT ( 'NONE',  ( 16.38665767535054130, 7.295008042176048590, 42.23599135785459424 ) ) ;
#88797=CARTESIAN_POINT ( 'NONE',  ( 19.05341960407611168, 5.049401038298154454, 23.95724293864769194 ) ) ;
#88798=CARTESIAN_POINT ( 'NONE',  ( 21.52544592524344225, -5.823673210054117533, 38.54057627198103120 ) ) ;
#88799=CARTESIAN_POINT ( 'NONE',  ( 14.34966873604972726, -8.224510206698740333, 90.83442372801901854 ) ) ;
#88800=CARTESIAN_POINT ( 'NONE',  ( -8.314922557960811034, -14.29746914071050412, 77.08224293864769550 ) ) ;
#88801=CARTESIAN_POINT ( 'NONE',  ( 0.05219959533909260263, 19.03943276465977164, 64.99890960531436690 ) ) ;
#88802=CARTESIAN_POINT ( 'NONE',  ( -18.62759615963255300, -10.81492255796106328, 89.16775706135236135 ) ) ;
#88804=CARTESIAN_POINT ( 'NONE',  ( -4.379528057220086978, -16.55341960407618274, 24.79275706135235779 ) ) ;
#88805=CARTESIAN_POINT ( 'NONE',  ( -8.224510206698948167, 14.34966873604960824, 70.41557627198102409 ) ) ;
#88806=CARTESIAN_POINT ( 'NONE',  ( 5.719274019375673035, 21.55341960407619339, 37.29275706135235424 ) ) ;
#88807=CARTESIAN_POINT ( 'NONE',  ( 10.81492255796078972, 18.62759615963270932, 74.58224293864768129 ) ) ;
#88809=CARTESIAN_POINT ( 'NONE',  ( -19.02544592524334988, -5.153800228976617603, 33.95942372801897591 ) ) ;
#88811=CARTESIAN_POINT ( 'NONE',  ( -5.153800228976328057, -19.02544592524343514, 77.29057627198099567 ) ) ;
#88812=CARTESIAN_POINT ( 'NONE',  ( -14.29746914071049879, 8.314922557960819915, 45.83224293864769550 ) ) ;
#88813=CARTESIAN_POINT ( 'NONE',  ( -8.224510206698948167, 14.34966873604960824, 40.41557627198103120 ) ) ;
#88814=CARTESIAN_POINT ( 'NONE',  ( 12.06949235617757843, -12.14591786802309237, 23.12390960531436335 ) ) ;
#88815=CARTESIAN_POINT ( 'NONE',  ( 13.97604488694548053, -13.89961937509957401, 65.62609039468567573 ) ) ;
#88816=CARTESIAN_POINT ( 'NONE',  ( 17.05587630539784882, 6.762274262135711922, 46.75819690962689634 ) ) ;
#88817=CARTESIAN_POINT ( 'NONE',  ( 21.52544592524344225, -5.823673210054117533, 28.54057627198103120 ) ) ;
#88818=CARTESIAN_POINT ( 'NONE',  ( -12.06949235617756955, 12.14591786802309770, 85.62390960531436690 ) ) ;
#88819=LINE ( 'NONE', #90792, #146539 ) ;
#88820=CARTESIAN_POINT ( 'NONE',  ( 5.153800228976335163, 19.02544592524342804, 39.79057627198100988 ) ) ;
#88821=CARTESIAN_POINT ( 'NONE',  ( -10.72451020669898014, 18.67979575497178502, 35.41557627198102409 ) ) ;
#88822=CARTESIAN_POINT ( 'NONE',  ( -5.823673210054116645, -21.52544592524344225, 67.29057627198103830 ) ) ;
#88823=CARTESIAN_POINT ( 'NONE',  ( -8.224510206698948167, 14.34966873604960824, 105.4155762719810383 ) ) ;
#88824=CARTESIAN_POINT ( 'NONE',  ( -4.483927247898782831, 16.52544592524335698, 67.70942372801901854 ) ) ;
#88825=CARTESIAN_POINT ( 'NONE',  ( 19.05341960407611168, 5.049401038298154454, 53.95724293864770260 ) ) ;
#88826=CARTESIAN_POINT ( 'NONE',  ( -21.52544592524334988, -5.823673210054445271, 58.95942372801902565 ) ) ;
#88827=CARTESIAN_POINT ( 'NONE',  ( 16.52544592524342804, -4.483927247898539470, 103.5405762719810383 ) ) ;
#88828=CARTESIAN_POINT ( 'NONE',  ( 19.05341960407617918, -5.049401038297876454, 91.04275706135234714 ) ) ;
#88831=CARTESIAN_POINT ( 'NONE',  ( 10.72451020669898902, -18.67979575497178502, 37.91557627198102409 ) ) ;
#88833=CARTESIAN_POINT ( 'NONE',  ( 15.80617190586769283, -15.72974639402175789, 65.62609039468568994 ) ) ;
#88834=CARTESIAN_POINT ( 'NONE',  ( -16.52544592524335698, -4.483927247898792601, 58.95942372801902565 ) ) ;
#88835=CARTESIAN_POINT ( 'NONE',  ( 12.14591786802309770, 12.06949235617756955, 49.37390960531436690 ) ) ;
#88836=CARTESIAN_POINT ( 'NONE',  ( 5.719274019375991003, -21.55341960407610458, 62.70724293864769550 ) ) ;
#88837=CARTESIAN_POINT ( 'NONE',  ( -5.719274019375978568, 21.55341960407610458, 65.20724293864768129 ) ) ;
#88839=CARTESIAN_POINT ( 'NONE',  ( -9.474510206698720793, -16.51473224551083518, 89.58442372801900433 ) ) ;
#88840=CARTESIAN_POINT ( 'NONE',  ( -19.03943276465977164, 0.05219959533909376836, 111.2489096053143669 ) ) ;
#88841=CARTESIAN_POINT ( 'NONE',  ( 19.02544592524343514, -5.153800228976328945, 43.54057627198103120 ) ) ;
#88842=CARTESIAN_POINT ( 'NONE',  ( -19.02544592524342804, 5.153800228976336051, 26.04057627198103120 ) ) ;
#88843=CARTESIAN_POINT ( 'NONE',  ( 9.474510206698971260, -16.51473224551069308, 112.9155762719810383 ) ) ;
#88845=CARTESIAN_POINT ( 'NONE',  ( -12.14591786802326823, 12.06949235617739902, 73.12609039468567573 ) ) ;
#88846=CARTESIAN_POINT ( 'NONE',  ( 18.62759615963271287, -10.81492255796078972, 98.33224293864769550 ) ) ;
#88847=CARTESIAN_POINT ( 'NONE',  ( 9.564922557960805705, 16.46253265017160317, 74.58224293864769550 ) ) ;
#88848=CARTESIAN_POINT ( 'NONE',  ( 21.53943276465977519, 0.05219959533937863772, 36.25109039468567573 ) ) ;
#88849=CARTESIAN_POINT ( 'NONE',  ( -19.02544592524342804, 5.153800228976336051, 96.04057627198103830 ) ) ;
#88852=CARTESIAN_POINT ( 'NONE',  ( 21.55341960407619695, -5.719274019375665929, 36.04275706135234714 ) ) ;
#88853=CARTESIAN_POINT ( 'NONE',  ( -16.46253265017160317, 9.564922557960807481, 25.83224293864769194 ) ) ;
#88854=CARTESIAN_POINT ( 'NONE',  ( -19.03943276465977164, -0.05219959533935918106, 88.75109039468567573 ) ) ;
#88855=CARTESIAN_POINT ( 'NONE',  ( -16.46253265017146816, -9.564922557961047289, 39.16775706135234003 ) ) ;
#88856=CARTESIAN_POINT ( 'NONE',  ( 15.80617190586746368, 15.72974639402197994, 114.3739096053143527 ) ) ;
#88857=CARTESIAN_POINT ( 'NONE',  ( -5.049401038297874678, -19.05341960407617918, 34.79275706135233293 ) ) ;
#88858=CARTESIAN_POINT ( 'NONE',  ( 9.474510206698729675, 16.51473224551082808, 52.08442372801900433 ) ) ;
#88859=CARTESIAN_POINT ( 'NONE',  ( 16.52544592524335698, 4.483927247898782831, 96.45942372801901854 ) ) ;
#88861=CARTESIAN_POINT ( 'NONE',  ( -9.564922557960796823, -16.46253265017161027, 67.08224293864769550 ) ) ;
#88863=CARTESIAN_POINT ( 'NONE',  ( -15.80617190586768217, 15.72974639402176855, 83.12609039468568994 ) ) ;
#88865=CARTESIAN_POINT ( 'NONE',  ( -21.53943276465977519, -0.05219959533937600094, 93.75109039468567573 ) ) ;
#88867=CARTESIAN_POINT ( 'NONE',  ( 13.97604488694527802, 13.89961937509977652, 89.37390960531436690 ) ) ;
#88868=CARTESIAN_POINT ( 'NONE',  ( 15.72974639402176855, 15.80617190586768217, 56.87609039468568994 ) ) ;
#88869=CARTESIAN_POINT ( 'NONE',  ( -9.564922557961040184, 16.46253265017147172, 102.9177570613523329 ) ) ;
#88870=CARTESIAN_POINT ( 'NONE',  ( 16.51473224551069308, 9.474510206698969483, 64.16557627198102409 ) ) ;
#88871=CARTESIAN_POINT ( 'NONE',  ( -16.51473224551069308, -9.474510206698971260, 111.6655762719810383 ) ) ;
#88872=CARTESIAN_POINT ( 'NONE',  ( 19.02544592524343514, -5.153800228976328945, 78.54057627198099567 ) ) ;
#88873=CARTESIAN_POINT ( 'NONE',  ( 17.50000000000001776, -3.252092809005011187, 22.52397829382482897 ) ) ;
#88874=CARTESIAN_POINT ( 'NONE',  ( -16.51473224551069308, -9.474510206698971260, 71.66557627198102409 ) ) ;
#88875=CARTESIAN_POINT ( 'NONE',  ( 19.02544592524343514, -5.153800228976328945, 48.54057627198103120 ) ) ;
#88876=CARTESIAN_POINT ( 'NONE',  ( 10.81492255796078972, 18.62759615963270932, 114.5822429386477097 ) ) ;
#88877=CARTESIAN_POINT ( 'NONE',  ( -4.379528057220086978, -16.55341960407618274, 89.79275706135236135 ) ) ;
#88880=CARTESIAN_POINT ( 'NONE',  ( 13.89961937509957401, 13.97604488694547697, 61.87609039468566863 ) ) ;
#88881=CARTESIAN_POINT ( 'NONE',  ( 5.049401038298161559, -19.05341960407611168, 77.70724293864765286 ) ) ;
#88882=CARTESIAN_POINT ( 'NONE',  ( -4.379528057220328563, 16.55341960407611168, 70.20724293864769550 ) ) ;
#88883=CARTESIAN_POINT ( 'NONE',  ( 14.34966873604960469, 8.224510206698951720, 114.1655762719810383 ) ) ;
#88884=CARTESIAN_POINT ( 'NONE',  ( 13.97604488694527802, 13.89961937509977652, 114.3739096053143669 ) ) ;
#88885=CARTESIAN_POINT ( 'NONE',  ( -19.02544592524342804, 5.153800228976336051, 111.0405762719810099 ) ) ;
#88886=CARTESIAN_POINT ( 'NONE',  ( -0.05219959533910754901, -16.53943276465976808, 77.49890960531433848 ) ) ;
#88887=FACE_OUTER_BOUND ( 'NONE', #87996, .T. ) ;
#88888=CARTESIAN_POINT ( 'NONE',  ( 13.89961937509957401, 13.97604488694547697, 31.87609039468566863 ) ) ;
#88889=CARTESIAN_POINT ( 'NONE',  ( 8.314922557961029526, -14.29746914071037800, 110.4177570613523756 ) ) ;
#88890=CARTESIAN_POINT ( 'NONE',  ( 13.89961937509977652, -13.97604488694527269, 88.12390960531438111 ) ) ;
#88891=CARTESIAN_POINT ( 'NONE',  ( -5.823673210054431948, 21.52544592524334988, 57.70942372801901143 ) ) ;
#88892=CARTESIAN_POINT ( 'NONE',  ( -21.52544592524343514, 5.823673210054127303, 46.04057627198103830 ) ) ;
#88893=CARTESIAN_POINT ( 'NONE',  ( -5.719274019375665041, -21.55341960407619695, 24.79275706135235779 ) ) ;
#88894=CARTESIAN_POINT ( 'NONE',  ( 18.67979575497178502, 10.72451020669898547, 64.16557627198102409 ) ) ;
#88895=CARTESIAN_POINT ( 'NONE',  ( -14.29746914071049879, 8.314922557960819915, 100.8322429386477097 ) ) ;
#88896=CARTESIAN_POINT ( 'NONE',  ( -5.153800228976607833, 19.02544592524334988, 62.70942372801899722 ) ) ;
#88898=CARTESIAN_POINT ( 'NONE',  ( -19.03943276465977164, 0.05219959533909376836, 26.24890960531435624 ) ) ;
#88899=( BOUNDED_SURFACE ( )  B_SPLINE_SURFACE ( 3, 2, ( 
 ( #88354, #116704, #71208, #11553, #72205, #131877, #39858, #133879, #178394, #163215, #132871, #195570, #117708, #179404, #102542, #119707, #181390, #78142, #169164, #139810, #122665, #92321, #136848, #107486, #105521, #199523, #30668, #93313, #47832, #171167, #309, #32654, #108491, #13511, #184353, #61977, #182378, #1298, #43856, #154006, #109484, #183366, #44848, #75176, #60004, #185340, #170170, #120679, #62976, #168181, #167206, #124656, #90340, #186352, #94308, #155986, #15502, #152025, #154997, #138829, #31663, #28704, #46831, #198533, #91309, #45835, #140811, #16493, #121671, #2301, #153001, #123643, #29677, #77159, #106504, #17483, #79140, #14500, #76162, #137842, #60991, #36367, #148563, #177909, #38382, #131381, #129369, #39377, #51549, #9051, #23219, #191065, #159715, #176911, #37375, #100038, #98020, #193070, #21212, #53541, #128377, #82869, #66716, #190073, #175903, #68705, #99032, #147566, #101036, #113213, #160722, #144547, #54545, #161724, #6032, #194082, #116218, #117217, #162722, #8033, #67711, #52538, #69714, #22214, #84862, #146540, #55545, #114199, #24227, #83863, #132389, #85878, #70722, #174902, #7023, #178911, #145545, #130362, #40378, #102052, #163737, #192059, #115219, #25237, #86878, #107013, #198050, #14015, #12064, #73726, #133381, #74710, #195072, #135399, #118228, #10053, #119226, #56551, #168686, #121193, #179919, #27224, #166727, #197070, #167713, #182886, #181893, #26228, #41386, #103051, #45361, #60509, #183876, #58537, #122184, #164733, #43371, #75681, #91829, #105043, #44369, #88872, #150565, #28231, #151553, #104048, #137360, #30187, #120203, #106026, #89871, #13043, #42385, #71713, #136373, #59516, #87867, #149555, #11051, #29209, #72726, #134399, #90843, #196086, #152528, #57556, #199039, #180910, #165728, #127145, #186879, #93834, #18011, #138356, #154520, #822, #173683, #49332, #78661, #17009, #35150, #185869, #110003, #187863, #31184, #79665, #110993, #172678, #140336, #77674, #184863, #126168, #33173, #34163, #171684, #188852, #3805, #169689, #47355, #125183, #153522, #62496, #200038, #48349, #94832, #95824, #32178, #109010, #15019, #76680, #157509, #108003, #92835, #156510, #16017, #124167, #141336, #2823, #50336, #139343, #1826, #65483, #170689, #19003, #63508, #142325, #61506, #111993, #64501, #123175, #80649, #46346, #155514, #98795, #68470, #112977, #83631, #81622, #175661, #6791, #69477, #23981, #147324, #176674, #8812, #84627, #189843, #160489, #38150, #158492, #54312, #19979, #145308, #85637, #159476, #20970, #51316, #36135, #161490, #146305, #96806, #177673, #144309, #143305, #39141, #66481, #115984, #100796, #162479, #130125, #128143, #131143, #114981, #7794, #4791, #22978, #174670, #67472, #21979, #116976, #192831, #97787, #178668, #129131, #99804, #5799, #191822, #82627, #70481, #53302, #132147, #193840, #190829, #55304, #52305, #113962, #37135, #11826, #104806, #102814, #12809, #24995, #182651, #196837, #164499, #133143, #150331, #10815, #73491, #71478, #166495, #194834, #26990, #101809, #9817, #40131, #163497, #149321, #42154, #72485, #120952, #74476, #86639, #134158, #56307, #27993, #135164, #117989, #167480, #89632, #90617, #136141, #181658, #179679, #43137, #28975, #44135, #152299, #151320, #41151, #103814, #197817, #148322, #59282, #25992, #88635, #13783, #87635, #195846, #57319, #118995, #105794, #75450, #180678, #137124, #165494, #58305, #198811, #119972, #60276, #121949, #49096, #31937, #153282, #156266, #1582, #32932, #91592, #48105, #14783, #154285, #47109, #3566, #17767, #183642, #65244, #15775, #124937, #30948, #108768, #46107, #79423, #155277, #109761, #94587, #76443, #157265, #138120, #45124, #141094, #16766, #171445, #107761, #2581, #168457, #125927, #140090, #169446, #199801, #93591, #77434, #78414, #61268, #64261, #122938, #170446, #106782, #184625, #29954, #92595, #139106, #185619, #580, #187626, #110753, #62251, #123920 ),
 ( #63257, #172434, #186634, #33923, #95580, #18761, #80408, #142080, #98553, #100562, #189602, #113723, #177435, #51075, #192590, #175419, #115747, #50091, #162242, #37904, #23742, #84386, #36887, #146063, #128890, #160247, #143068, #21737, #111751, #5553, #83389, #99563, #54073, #38905, #6547, #147085, #161244, #126904, #8569, #159232, #68226, #174429, #190590, #112736, #22738, #145066, #191578, #176430, #19742, #85391, #96564, #188610, #7547, #129879, #53056, #35899, #69233, #173439, #130900, #114736, #97545, #81383, #34908, #20727, #158252, #4546, #66240, #127900, #82384, #144072, #67232, #52066, #131912, #179438, #72238, #40904, #151080, #104566, #55068, #102577, #101559, #134922, #180441, #163251, #197577, #58070, #120710, #166249, #11585, #39892, #73252, #59044, #12571, #193596, #74237, #24753, #86400, #196599, #9576, #117743, #150080, #41913, #43890, #132906, #57078, #182410, #194593, #135906, #118752, #105553, #116738, #167239, #181423, #28737, #27749, #103579, #89392, #133914, #165254, #148085, #26748, #178428, #149087, #88387, #42901, #90374, #152059, #119740, #70244, #71242, #56064, #195605, #164261, #25756, #87402, #10576, #62008, #2333, #76195, #137874, #106537, #153034, #78172, #63010, #13544, #94339, #61024, #60037, #156018, #183398, #32688, #171198, #79173, #123673, #44881, #186385, #31695, #124689, #121705, #139841, #168214, #184385, #77191, #1330, #30702, #140844, #17515, #64014, #95333, #154038, #125683, #14534, #199555, #187381, #170202, #47863, #107519, #91343, #16525, #155030, #110505, #109516, #48850, #15533, #138860, #136881, #172186, #198567, #340, #29711, #75210, #122696, #45866, #33671, #169195, #92352, #185371, #93344, #46862, #108523, #129637, #128648, #173189, #126658, #141835, #192346, #7303, #130652, #143825, #68988, #49839, #190343, #22494, #38664, #51819, #67983, #35655, #174187, #113479, #98296, #50836, #84141, #53828, #20481, #191333, #175173, #36639, #189359, #157018, #159998, #5305, #115503, #3327, #65000, #82131, #177191, #188362, #144821, #18516, #21486, #34665, #83147, #52811, #80163, #111503, #6305, #97303, #114478, #96323, #158010, #4307, #19501, #176181, #66989, #37651, #81146, #112493, #99316, #161000, #142827, #145820, #65990, #127659, #158989, #24507, #131666, #73008, #180199, #181185, #118509, #73999, #150839, #116498, #194356, #71990, #120472, #147848, #85143, #133664, #195354, #134677, #179193, #55823, #100319, #193348, #103332, #132668, #56834, #41668, #89150, #163001, #87161, #135669, #146828, #8322, #164020, #12335, #69998, #88148, #197341, #165011, #178186, #26505, #11337, #58804, #182164, #149833, #40661, #196363, #54824, #101312, #9334, #161998, #57831, #25516, #148843, #23494, #117496, #119504, #42662, #39651, #104324, #166009, #27509, #10334, #86158, #71000, #102330, #123437, #124448, #61769, #17279, #94103, #59796, #137632, #15289, #63780, #91109, #28501, #76949, #138618, #77938, #122455, #199318, #43649, #136637, #46621, #75958, #100, #185130, #32450, #106294, #108282, #60784, #109277, #62767, #186144, #125452, #184148, #47623, #183158, #44642, #170956, #169960, #31452, #45629, #121466, #93105, #154790, #140609, #16288, #155782, #107281, #168952, #166999, #139605, #90135, #30458, #151820, #105312, #152798, #13309, #2099, #1091, #74975, #92106, #78933, #153794, #198319, #167980, #29478, #14290, #156790, #171954, #22252, #37413, #160762, #173955, #99072, #79938, #20245, #52577, #68743, #158756, #98056, #65755, #4077, #81893, #128413, #80921, #114237, #83901, #50604, #21251, #143586, #5069, #19274, #187148, #66752, #48621, #159756, #190109, #51584, #49603, #82906, #33442, #129406, #113249, #111266, #141608, #97075, #157784, #174939, #18283, #36402, #3095, #35422, #110273, #64772, #95101, #126434, #96095, #189132, #142597, #67748, #144584, #188132, #127424, #172957, #6070, #191103, #34435, #175943, #145584, #7062, #112263, #71750 ),
 ( #23257, #133420, #162756, #86916, #10091, #119262, #193106, #195109, #147602, #196122, #149593, #72767, #14819, #70757, #11090, #69750, #131419, #134437, #148599, #56592, #24265, #8074, #118266, #179956, #29991, #41423, #57592, #132425, #194117, #53581, #103089, #115258, #55580, #38421, #130401, #39411, #176951, #91630, #164770, #100077, #9089, #26265, #117254, #87906, #183678, #102088, #146579, #161762, #84900, #168493, #45163, #106819, #178946, #153318, #54580, #163773, #192099, #116253, #25274, #177944, #40417, #101071, #85914, #17804, #170483, #142117, #173475, #140127, #110791, #32970, #94624, #108804, #158289, #156303, #63294, #111787, #122975, #139141, #49133, #48141, #184662, #124974, #34948, #46144, #107798, #1618, #126940, #169482, #64297, #96600, #79461, #92630, #141130, #187662, #50127, #76480, #109798, #16803, #2620, #61305, #77471, #123956, #138157, #172472, #186671, #171481, #199838, #31973, #125964, #33959, #154321, #95617, #157302, #18799, #80444, #618, #30982, #3602, #65281, #188648, #15810, #62288, #185654, #47146, #93629, #155314, #78453, #67268, #4584, #53093, #114771, #54108, #98588, #113759, #19778, #112772, #22774, #52102, #176465, #99599, #8607, #82419, #84422, #36926, #85429, #38940, #162279, #101601, #160282, #100597, #159268, #20764, #23779, #37938, #146099, #175455, #97580, #7583, #161279, #116774, #69269, #147120, #21773, #83424, #143105, #130935, #66277, #145101, #127936, #81419, #128926, #189638, #178465, #192626, #51113, #6584, #115782, #68263, #177471, #70280, #191614, #35934, #174465, #144108, #55104, #131948, #193632, #129914, #39932, #5588, #190627, #28774, #44919, #134962, #74276, #41952, #180481, #196640, #104605, #57118, #90412, #60074, #26787, #197616, #119779, #135946, #181463, #12612, #71280, #27789, #132945, #133954, #88429, #183434, #59081, #163289, #24790, #195645, #166293, #10616, #150123, #25794, #149125, #182447, #136919, #72277, #56103, #198606, #194633, #86438, #120748, #58109, #89431, #87440, #43927, #148124, #105589, #42941, #118792, #117784, #73292, #103618, #151120, #179478, #167275, #40943, #11624, #9615, #102615, #164301, #165294, #152097, #13581, #75248, #121742, #140883, #91383, #15570, #137912, #171236, #16563, #199594, #33711, #94377, #157058, #2373, #47901, #76232, #109555, #95373, #48890, #29748, #110545, #61061, #122733, #32725, #45904, #154076, #186425, #78210, #80203, #169235, #93382, #18555, #30741, #172226, #155068, #141874, #153072, #3365, #17554, #65040, #64053, #139880, #125723, #108562, #1369, #184424, #63048, #14574, #185411, #124727, #79214, #126696, #188400, #156057, #106575, #187422, #107557, #170240, #168252, #92389, #77228, #138897, #377, #62049, #123714, #46902, #31734, #189397, #114518, #99353, #49878, #130689, #97342, #96361, #192383, #19539, #69024, #7339, #115540, #98338, #81184, #113519, #100357, #158049, #37688, #85178, #191371, #66030, #52847, #161036, #23532, #146867, #83185, #190384, #176219, #34704, #50874, #159028, #70034, #145857, #175213, #36678, #131703, #82169, #6342, #84177, #127697, #22530, #53866, #177228, #160037, #174226, #142866, #38700, #129673, #162036, #68022, #8359, #111543, #112532, #143865, #21524, #173228, #20521, #4345, #144859, #35695, #5344, #128687, #67028, #51859, #86194, #196398, #25554, #149868, #73043, #182198, #55858, #57867, #10370, #58840, #12370, #135704, #75008, #133700, #74033, #132702, #194391, #197375, #11373, #119539, #87198, #71035, #181222, #134715, #90170, #42698, #120507, #195392, #56870, #116534, #104359, #178222, #118545, #101348, #193384, #102366, #39686, #151853, #166043, #163037, #72027, #27543, #180235, #150876, #89184, #165047, #9370, #24544, #147884, #28534, #43683, #167032, #41704, #105345, #117532, #26540, #13344, #54860, #88184, #179230, #103369, #40696, #164055, #148879, #30492, #2135, #33478, #136, #170992, #93140, #155817, #32485, #92143, #183193 ),
 ( #61805, #123475, #156825, #168988, #154825, #94138, #14327, #62802, #17315, #78970, #185167, #60817, #168014, #109313, #16323, #140645, #77973, #110308, #187185, #152833, #153830, #108317, #18318, #184182, #121499, #169997, #31488, #63815, #15325, #76984, #136673, #29510, #139640, #138655, #1128, #124484, #125488, #199352, #186180, #46658, #48656, #171990, #95136, #198355, #47662, #59829, #75992, #137665, #44675, #106328, #91144, #122491, #45664, #107315, #51618, #160801, #36438, #129442, #173988, #35457, #3133, #113283, #64808, #97108, #126469, #79975, #4110, #188167, #22289, #159791, #49640, #112298, #128446, #158791, #144621, #21286, #143618, #34470, #111303, #172992, #99109, #175980, #83940, #20280, #37448, #96129, #5102, #191141, #141643, #82943, #157818, #174974, #190142, #6104, #52614, #66784, #19308, #80956, #98093, #142631, #114276, #65789, #127458, #67785, #81926, #189164, #50636, #106976, #168650, #124131, #110954, #30150, #48311, #95785, #1790, #76642, #63468, #171645, #34126, #172638, #157471, #47317, #18964, #153486, #93798, #126131, #142287, #32141, #33135, #139307, #77638, #155478, #125143, #154485, #187826, #80610, #185830, #94793, #16970, #79627, #156472, #15979, #91792, #108972, #60472, #14982, #138320, #170653, #122148, #200002, #109966, #183837, #186842, #61468, #17973, #141295, #45326, #123139, #78624, #786, #2785, #184825, #46311, #107966, #169653, #64464, #140299, #49295, #31149, #92797, #62458, #38108, #81582, #130082, #99763, #161448, #67433, #128101, #35111, #176633, #83589, #84585, #21938, #177636, #54273, #19941, #97748, #175622, #23942, #51277, #188813, #37096, #98755, #22939, #82589, #159436, #3767, #96763, #6750, #36096, #160448, #145269, #192791, #66440, #68429, #20931, #69435, #146265, #7750, #85596, #144270, #131103, #143268, #4751, #115946, #191781, #53263, #5757, #189805, #114940, #39103, #100759, #162441, #65444, #129090, #190790, #127106, #50296, #111953, #52264, #173642, #158452, #112938, #174631, #113922, #155686, #124349, #17181, #109182, #60683, #141511, #108183, #107184, #2996, #30360, #79841, #77844, #126336, #64674, #188033, #142499, #994, #49503, #200192, #61674, #111166, #78835, #187053, #154694, #138522, #63681, #2003, #157682, #48523, #172856, #62668, #186044, #184047, #125356, #45530, #47526, #168855, #122358, #169864, #92003, #19172, #110177, #170861, #140513, #34337, #32352, #18185, #33344, #94005, #76851, #153697, #15192, #95997, #80821, #123343, #171856, #185036, #46523, #95003, #31357, #93008, #156691, #16189, #139511, #21148, #175837, #145482, #97959, #72409, #103746, #67647, #38320, #160659, #23156, #99975, #159651, #50505, #191001, #42081, #112168, #173857, #129305, #57249, #35323, #191992, #165425, #6962, #20149, #68642, #115157, #180608, #26919, #37311, #144484, #130298, #189031, #4966, #51487, #88562, #161659, #52477, #114136, #3977, #36304, #22151, #84799, #81794, #53479, #146478, #10745, #98969, #128313, #96977, #176849, #83801, #134086, #195776, #65657, #118923, #143481, #82803, #127319, #158658, #113149, #66652, #190014, #174839, #5968, #28905, #44062, #150260, #43067, #153205, #182579, #106711, #29880, #139031, #12738, #14710, #92524, #31865, #90545, #30877, #89563, #151249, #154213, #168385, #76370, #105722, #27920, #138047, #91518, #47038, #199728, #15703, #152227, #13712, #73421, #61194, #135092, #75378, #58236, #11754, #59211, #196768, #108695, #122866, #198740, #184554, #77363, #137050, #107690, #46035, #121875, #166425, #119904, #181590, #185544, #510, #123846, #60205, #62182, #104734, #183568, #170374, #74404, #45053, #169369, #136070, #167409, #197744, #120880, #187554, #159158, #190517, #157192, #127825, #50013, #112664, #189531, #49021, #140017, #80333, #128818, #1506, #63183, #18686, #143997, #124863, #81312, #51991, #34835, #109691, #96490, #4473, #67161, #113650, #126829, #33846, #158180, #78343, #94510 ),
 ( #186562, #19670, #3494, #48035, #20653, #142995, #5478, #51003, #66163, #171373, #174356, #82307, #35826, #16693, #97472, #32860, #156192, #175344, #17692, #141020, #173365, #65170, #93519, #79349, #142005, #155204, #2507, #64187, #188535, #125854, #110676, #172356, #95506, #111678, #21661, #72165, #87329, #10503, #23667, #149015, #129805, #70169, #102502, #118677, #8492, #148014, #115673, #53999, #131837, #178355, #130825, #164186, #133840, #100490, #71169, #193520, #55992, #132833, #192516, #83315, #85315, #195530, #144992, #6473, #162169, #57004, #68153, #24678, #36812, #39819, #52980, #101485, #9503, #98478, #160171, #54995, #177361, #163174, #191504, #37828, #84312, #114659, #194520, #147007, #116664, #176355, #69158, #86327, #117670, #99488, #179367, #40829, #25684, #161168, #22665, #145991, #7474, #38832, #60953, #198495, #153967, #30630, #196532, #74169, #151989, #271, #27681, #165182, #13476, #75140, #14462, #58976, #135839, #180369, #73183, #183328, #12505, #136811, #59966, #169125, #42834, #44809, #197508, #45798, #199486, #122627, #61940, #120643, #184317, #119672, #181355, #107450, #121633, #106464, #182341, #58002, #168143, #29640, #77121, #91272, #92283, #43819, #105483, #103506, #152963, #26677, #167169, #88317, #41838, #89322, #150007, #138790, #76124, #28668, #137802, #15464, #90303, #11513, #134854, #104499, #166180, #151014, #81083, #96258, #95269, #139773, #93274, #108453, #158924, #174119, #97236, #110439, #35590, #16455, #156952, #189293, #5237, #18449, #34599, #2264, #140775, #80100, #64934, #141768, #65921, #126593, #171128, #187314, #186313, #109445, #142761, #20413, #32617, #78104, #82063, #154959, #123608, #157944, #3261, #188295, #47795, #19435, #170130, #127594, #49772, #94271, #1261, #33606, #155949, #111437, #62938, #173124, #124618, #172120, #185303, #17446, #46794, #31624, #79102, #125616, #63947, #4241, #50770, #48785, #112430, #143756, #131594, #177123, #98228, #194287, #54753, #117427, #101242, #8250, #36573, #69930, #55753, #9264, #190276, #70930, #21418, #83078, #193279, #6239, #114411, #146756, #38594, #40593, #129571, #53758, #179125, #191268, #132597, #115432, #102264, #51752, #163952, #178115, #25450, #24438, #100250, #86087, #68920, #161931, #144754, #23426, #113413, #145753, #85073, #39583, #87090, #148775, #116427, #66918, #162931, #159931, #130582, #147778, #128582, #175104, #67918, #52743, #176112, #37583, #99245, #160933, #192277, #22424, #84074, #7235, #45564, #56766, #118438, #73934, #60717, #180131, #198255, #107217, #151756, #26438, #13249, #121400, #184080, #168888, #43583, #150774, #74912, #195285, #11268, #57765, #30393, #106231, #135603, #197274, #92040, #42594, #166935, #44575, #88080, #136575, #167914, #29414, #58737, #134611, #41600, #183094, #90073, #91045, #28438, #10264, #122391, #149766, #104257, #182099, #71923, #119435, #103265, #105249, #59731, #152732, #89082, #165940, #133593, #164945, #14222, #27440, #75892, #137567, #199250, #72941, #196295, #12269, #181120, #120406, #96032, #35361, #94039, #34372, #93041, #154728, #157719, #110209, #79875, #47560, #31391, #156726, #95035, #50541, #141544, #19208, #155717, #17214, #76884, #18219, #138555, #78866, #61706, #153729, #62700, #33, #112202, #3033, #2034, #171890, #80858, #140546, #111201, #126371, #125389, #169898, #123376, #185068, #189069, #4013, #127356, #63714, #65691, #46556, #187086, #142534, #15225, #48556, #64709, #32384, #170892, #173892, #188068, #108218, #49539, #16224, #33377, #172893, #77876, #139543, #1028, #109213, #124383, #186078, #39352, #51523, #113186, #100010, #36341, #144520, #176884, #68679, #70696, #159687, #83835, #147539, #21185, #162695, #145517, #85850, #20183, #132364, #8005, #194057, #54521, #6997, #116194, #99005, #130334, #174875, #192032, #81829, #175875, #53514, #69688, #24201, #9027, #38355, #55518, #84836, #190048, #160696, #161696 ),
 ( #6005, #143516, #101011, #66688, #177883, #117191, #178884, #115192, #128350, #131355, #23193, #146515, #5005, #193044, #97994, #67685, #22187, #97013, #82841, #158694, #129343, #191038, #52511, #114172, #37347, #103026, #26203, #59493, #13991, #87842, #133356, #75658, #10029, #122159, #151529, #12038, #105018, #164708, #13018, #25212, #182862, #197044, #149530, #195046, #150538, #11025, #73702, #71689, #166702, #56525, #27200, #102027, #118203, #40352, #163709, #72700, #42361, #134373, #121168, #74683, #86854, #196059, #179894, #28205, #135374, #41360, #167688, #89846, #90819, #136349, #181868, #57532, #43347, #29185, #198025, #119201, #180886, #44343, #106001, #137335, #152502, #199015, #104024, #165703, #148538, #60484, #88846, #58512, #120178, #183848, #92811, #168661, #80623, #48324, #32154, #1802, #187839, #108985, #141309, #156485, #155491, #200013, #153497, #30161, #18977, #34139, #157484, #170666, #95798, #76654, #16983, #49308, #65457, #78637, #94806, #62472, #799, #142300, #17987, #14994, #186855, #3780, #47330, #79640, #140312, #2798, #64476, #139319, #91805, #93811, #45336, #138333, #61480, #63480, #106988, #123151, #171659, #184839, #125156, #46324, #109979, #126143, #107978, #169666, #33148, #124144, #110967, #31161, #154498, #15993, #77651, #172651, #185843, #190803, #147297, #159448, #83602, #161462, #4766, #53275, #22952, #84600, #52277, #51290, #158466, #99777, #6764, #7766, #145281, #100771, #177647, #143280, #20944, #98767, #8786, #174644, #111966, #160461, #21952, #146279, #5771, #82601, #127120, #19954, #130097, #144282, #68443, #191794, #115959, #189818, #114954, #67446, #192805, #69449, #131116, #188826, #129104, #54287, #66453, #128115, #39115, #176647, #96777, #38123, #162454, #23955, #50310, #85610, #81596, #112951, #173658, #36109, #97761, #35125, #113935, #175634, #37108, #57293, #120928, #194807, #136117, #118970, #59259, #193814, #105770, #181634, #167457, #27968, #180653, #89608, #72459, #42129, #86614, #103790, #55279, #149297, #165470, #43114, #197793, #182627, #150305, #44112, #58280, #163471, #134133, #11802, #132121, #151297, #116950, #26966, #28953, #133118, #56281, #88609, #195822, #73466, #135139, #70456, #12786, #117963, #178642, #74451, #40105, #90594, #152276, #101783, #196813, #24968, #104782, #119949, #166470, #148297, #9791, #71453, #41124, #179654, #102788, #164474, #25968, #87611, #10791, #155255, #61244, #77412, #76420, #199777, #35622, #190307, #122916, #106759, #51783, #183619, #98260, #127624, #185598, #78393, #138096, #189324, #198788, #158955, #170424, #184604, #168434, #123899, #46085, #47087, #45102, #140069, #29930, #560, #75428, #91569, #13760, #137102, #107740, #15753, #169421, #97267, #50801, #60254, #30926, #153257, #1560, #108748, #14759, #143788, #65953, #66952, #112459, #16744, #113443, #92574, #121925, #174151, #31916, #20445, #154262, #82096, #139082, #5271, #93570, #62231, #128614, #175136, #36603, #193311, #191298, #24469, #52774, #146790, #21449, #129602, #159962, #83110, #68950, #161961, #130613, #40624, #194318, #144787, #192309, #114443, #86119, #69961, #176144, #87122, #147810, #10297, #55786, #101273, #37614, #162963, #148807, #102294, #6270, #163983, #99276, #160963, #9296, #22457, #7266, #39614, #131627, #133627, #84105, #8283, #71954, #145784, #25480, #54785, #195319, #67948, #56799, #70962, #118472, #117457, #116460, #179156, #23457, #178149, #53789, #132630, #115464, #38626, #180162, #41632, #177153, #100283, #85104, #153761, #91075, #196328, #166965, #44606, #164976, #60748, #26471, #151786, #92072, #165970, #27472, #198284, #28467, #59762, #13277, #103297, #184113, #150803, #149797, #45595, #72973, #122421, #107248, #168919, #74941, #134642, #75923, #121430, #152762, #11303, #167945, #57796, #73965, #90102, #123405, #119467, #136604, #183123, #30425, #106261, #12299, #29443, #89115, #135634, #15256, #76914, #197304 ),
 ( #138585, #14252, #58768, #137598, #120436, #182129, #66, #61737, #43613, #181150, #185098, #42625, #88113, #199281, #104289, #105277, #109242, #19241, #31420, #189099, #3062, #170922, #139573, #156756, #17245, #79903, #77906, #111233, #1058, #33409, #108248, #16255, #46587, #169928, #155747, #48586, #78897, #127389, #80888, #93072, #140575, #62732, #172924, #18250, #124414, #173922, #34403, #97042, #142565, #188097, #186108, #49570, #35391, #50572, #154757, #112232, #47589, #32413, #96061, #94068, #2065, #126401, #141574, #20214, #63744, #95068, #158724, #125418, #81862, #64739, #143551, #187114, #5036, #157749, #66722, #4044, #65721, #128383, #110238, #171919, #6039, #176918, #174909, #68712, #100045, #162730, #117225, #40387, #69722, #102060, #177917, #82876, #53548, #131389, #51555, #147574, #113219, #38389, #178919, #52545, #114206, #84869, #115226, #146547, #161731, #190079, #70730, #37382, #36373, #132397, #159723, #9060, #194090, #55552, #23226, #21220, #24236, #193078, #163745, #175911, #54553, #7030, #25245, #86886, #148571, #71721, #130369, #10061, #129375, #191072, #98027, #8041, #116226, #83870, #67718, #39385, #101044, #144554, #85886, #99039, #192066, #160729, #22221, #145552, #118237, #197078, #41395, #133390, #42394, #179928, #30194, #198058, #181901, #151562, #137367, #58545, #90850, #106033, #105051, #149564, #103060, #164742, #168693, #183883, #107021, #120211, #45368, #26237, #166735, #199046, #15026, #28239, #44377, #12072, #150573, #91836, #167719, #87876, #136381, #153529, #43379, #29217, #89879, #152535, #14022, #88881, #11060, #13051, #195081, #72736, #134409, #74718, #56561, #196095, #121201, #57565, #59524, #119235, #182893, #75688, #180919, #104057, #60516, #73734, #122191, #165737, #27232, #135407, #96813, #172686, #1833, #140345, #158499, #109017, #33180, #111000, #154527, #2830, #34171, #95832, #63515, #830, #108011, #49338, #156519, #157516, #94839, #50343, #127152, #92842, #170696, #48356, #76687, #124175, #61513, #110010, #171691, #19010, #155521, #32185, #138363, #169696, #79672, #93842, #18019, #80656, #141343, #185876, #125190, #139350, #62504, #142332, #112002, #47362, #31190, #173691, #46353, #200044, #187870, #64508, #126175, #17016, #3812, #123182, #65490, #188860, #78669, #16024, #186886, #35158, #184871, #77682, #84635, #51324, #6799, #81629, #189851, #19986, #143312, #129139, #21986, #190836, #100804, #54319, #4799, #52312, #131150, #8819, #97795, #192839, #99811, #162487, #38157, #193847, #70488, #36143, #113970, #191829, #40139, #67480, #66488, #53310, #114988, #115991, #98802, #175668, #128151, #112985, #22987, #37143, #176682, #161497, #132154, #82634, #146312, #160496, #85645, #39148, #23988, #101816, #83638, #147331, #159483, #20977, #55312, #7801, #69485, #145316, #144317, #177680, #116983, #178676, #174678, #5806, #68477, #130132, #86646, #28000, #148329, #26997, #71485, #163504, #72492, #9824, #60283, #89640, #11834, #181665, #167488, #88642, #120959, #136148, #135171, #179686, #133151, #194841, #198818, #13791, #137131, #150338, #75457, #56315, #196844, #28983, #45132, #58311, #74483, #42161, #180685, #121956, #197824, #117997, #103821, #90624, #182658, #105801, #25002, #165501, #44142, #102821, #164506, #152306, #119979, #151328, #57326, #41158, #166502, #104813, #183649, #12816, #26000, #73499, #43144, #87642, #59290, #149328, #10822, #134166, #195854, #119002, #91599, #3574, #171453, #155285, #124945, #110762, #31945, #64269, #79431, #78424, #122946, #76450, #153289, #142088, #157273, #80416, #93599, #18769, #199808, #140099, #172443, #188618, #1590, #17776, #185626, #123928, #65252, #141102, #138127, #109769, #126912, #170454, #2589, #63265, #125935, #187634, #62260, #14790, #16775, #106790, #61275, #184634, #186642, #168464, #46115, #94596, #29962, #48113, #107768, #32941, #49104, #169453, #30955, #156275, #47117, #33931, #92602 ) ),
 .UNSPECIFIED., .T., .F., .F. ) 
 B_SPLINE_SURFACE_WITH_KNOTS ( ( 4, 3, 4 ),
 ( 3, 2, 2, 2, 2, 2, 2, 2, 2, 2, 2, 2, 2, 2, 2, 2, 2, 2, 2, 2, 2, 2, 2, 2, 2, 2, 2, 2, 2, 2, 2, 2, 2, 2, 2, 2, 2, 2, 2, 2, 2, 2, 2, 2, 2, 2, 2, 2, 2, 2, 2, 2, 2, 2, 2, 2, 2, 2, 2, 2, 2, 2, 2, 2, 2, 2, 2, 2, 2, 2, 2, 2, 2, 2, 2, 2, 2, 2, 2, 2, 2, 2, 2, 2, 2, 2, 2, 2, 2, 2, 2, 2, 2, 2, 2, 2, 2, 2, 2, 2, 2, 2, 2, 2, 2, 2, 2, 2, 2, 2, 2, 2, 2, 2, 2, 2, 2, 2, 2, 2, 2, 2, 2, 2, 2, 2, 2, 2, 2, 2, 2, 2, 2, 2, 2, 2, 2, 2, 2, 2, 2, 2, 2, 2, 2, 2, 2, 2, 2, 2, 2, 2, 2, 2, 2, 2, 2, 2, 2, 2, 2, 2, 2, 2, 2, 2, 2, 2, 2, 2, 2, 2, 2, 2, 2, 2, 2, 2, 2, 2, 2, 2, 2, 2, 2, 2, 2, 2, 2, 2, 2, 2, 2, 2, 2, 2, 2, 2, 2, 2, 2, 2, 2, 2, 2, 2, 2, 2, 2, 2, 2, 2, 2, 2, 2, 2, 2, 2, 2, 2, 2, 2, 2, 2, 2, 2, 2, 2, 3 ),
 ( 0.000000000000000000, 0.5000000000000000000, 1.000000000000000000 ),
 ( 0.000000000000000000, 0.004385964912280701511, 0.008771929824561403022, 0.01315789473684210453, 0.01754385964912280604, 0.02192982456140350755, 0.02631578947368420907, 0.03070175438596491058, 0.03508771929824561209, 0.03947368421052631360, 0.04385964912280701511, 0.04824561403508771662, 0.05263157894736841813, 0.05701754385964911964, 0.06140350877192982115, 0.06578947368421052266, 0.07017543859649122417, 0.07456140350877192569, 0.07894736842105262720, 0.08333333333333332871, 0.08771929824561403022, 0.09210526315789473173, 0.09649122807017543324, 0.1008771929824561348, 0.1052631578947368363, 0.1096491228070175378, 0.1140350877192982393, 0.1184210526315789408, 0.1228070175438596423, 0.1271929824561403577, 0.1315789473684210453, 0.1359649122807017607, 0.1403508771929824483, 0.1447368421052631637, 0.1491228070175438514, 0.1535087719298245668, 0.1578947368421052544, 0.1622807017543859698, 0.1666666666666666574, 0.1710526315789473728, 0.1754385964912280604, 0.1798245614035087758, 0.1842105263157894635, 0.1885964912280701788, 0.1929824561403508665, 0.1973684210526315819, 0.2017543859649122695, 0.2061403508771929849, 0.2105263157894736725, 0.2149122807017543879, 0.2192982456140350755, 0.2236842105263157909, 0.2280701754385964786, 0.2324561403508771940, 0.2368421052631578816, 0.2412280701754385970, 0.2456140350877192846, 0.2500000000000000000, 0.2543859649122807154, 0.2587719298245614308, 0.2631578947368420907, 0.2675438596491228060, 0.2719298245614035214, 0.2763157894736842368, 0.2807017543859648967, 0.2850877192982456121, 0.2894736842105263275, 0.2938596491228070429, 0.2982456140350877027, 0.3026315789473684181, 0.3070175438596491335, 0.3114035087719298489, 0.3157894736842105088, 0.3201754385964912242, 0.3245614035087719396, 0.3289473684210526550, 0.3333333333333333148, 0.3377192982456140302, 0.3421052631578947456, 0.3464912280701754610, 0.3508771929824561209, 0.3552631578947368363, 0.3596491228070175517, 0.3640350877192982670, 0.3684210526315789269, 0.3728070175438596423, 0.3771929824561403577, 0.3815789473684210731, 0.3859649122807017330, 0.3903508771929824483, 0.3947368421052631637, 0.3991228070175438791, 0.4035087719298245390, 0.4078947368421052544, 0.4122807017543859698, 0.4166666666666666852, 0.4210526315789473450, 0.4254385964912280604, 0.4298245614035087758, 0.4342105263157894912, 0.4385964912280701511, 0.4429824561403508665, 0.4473684210526315819, 0.4517543859649122973, 0.4561403508771929571, 0.4605263157894736725, 0.4649122807017543879, 0.4692982456140351033, 0.4736842105263157632, 0.4780701754385964786, 0.4824561403508771940, 0.4868421052631579093, 0.4912280701754385692, 0.4956140350877192846, 0.5000000000000000000, 0.5043859649122807154, 0.5087719298245614308, 0.5131578947368421462, 0.5175438596491228616, 0.5219298245614034659, 0.5263157894736841813, 0.5307017543859648967, 0.5350877192982456121, 0.5394736842105263275, 0.5438596491228070429, 0.5482456140350877583, 0.5526315789473684736, 0.5570175438596490780, 0.5614035087719297934, 0.5657894736842105088, 0.5701754385964912242, 0.5745614035087719396, 0.5789473684210526550, 0.5833333333333333703, 0.5877192982456140857, 0.5921052631578946901, 0.5964912280701754055, 0.6008771929824561209, 0.6052631578947368363, 0.6096491228070175517, 0.6140350877192982670, 0.6184210526315789824, 0.6228070175438596978, 0.6271929824561403022, 0.6315789473684210176, 0.6359649122807017330, 0.6403508771929824483, 0.6447368421052631637, 0.6491228070175438791, 0.6535087719298245945, 0.6578947368421053099, 0.6622807017543859143, 0.6666666666666666297, 0.6710526315789473450, 0.6754385964912280604, 0.6798245614035087758, 0.6842105263157894912, 0.6885964912280702066, 0.6929824561403509220, 0.6973684210526315264, 0.7017543859649122417, 0.7061403508771929571, 0.7105263157894736725, 0.7149122807017543879, 0.7192982456140351033, 0.7236842105263158187, 0.7280701754385965341, 0.7324561403508771384, 0.7368421052631578538, 0.7412280701754385692, 0.7456140350877192846, 0.7500000000000000000, 0.7543859649122807154, 0.7587719298245614308, 0.7631578947368421462, 0.7675438596491228616, 0.7719298245614034659, 0.7763157894736841813, 0.7807017543859648967, 0.7850877192982456121, 0.7894736842105263275, 0.7938596491228070429, 0.7982456140350877583, 0.8026315789473684736, 0.8070175438596490780, 0.8114035087719297934, 0.8157894736842105088, 0.8201754385964912242, 0.8245614035087719396, 0.8289473684210526550, 0.8333333333333333703, 0.8377192982456140857, 0.8421052631578946901, 0.8464912280701754055, 0.8508771929824561209, 0.8552631578947368363, 0.8596491228070175517, 0.8640350877192982670, 0.8684210526315789824, 0.8728070175438596978, 0.8771929824561403022, 0.8815789473684210176, 0.8859649122807017330, 0.8903508771929824483, 0.8947368421052631637, 0.8991228070175438791, 0.9035087719298245945, 0.9078947368421053099, 0.9122807017543859143, 0.9166666666666666297, 0.9210526315789473450, 0.9254385964912280604, 0.9298245614035087758, 0.9342105263157894912, 0.9385964912280702066, 0.9429824561403509220, 0.9473684210526315264, 0.9517543859649122417, 0.9561403508771929571, 0.9605263157894736725, 0.9649122807017543879, 0.9692982456140351033, 0.9736842105263158187, 0.9780701754385965341, 0.9824561403508771384, 0.9868421052631578538, 0.9912280701754385692, 0.9956140350877192846, 1.000000000000000000 ),
 .UNSPECIFIED. ) 
 GEOMETRIC_REPRESENTATION_ITEM ( )  RATIONAL_B_SPLINE_SURFACE ( (
 ( 1.000000000000000000, 0.9659258262890683122, 1.000000000000000000, 0.9659258262890683122, 1.000000000000000000, 0.9659258262890683122, 1.000000000000000000, 0.9659258262890683122, 1.000000000000000000, 0.9659258262890683122, 1.000000000000000000, 0.9659258262890683122, 1.000000000000000000, 0.9659258262890683122, 1.000000000000000000, 0.9659258262890683122, 1.000000000000000000, 0.9659258262890683122, 1.000000000000000000, 0.9659258262890683122, 1.000000000000000000, 0.9659258262890683122, 1.000000000000000000, 0.9659258262890683122, 1.000000000000000000, 0.9659258262890683122, 1.000000000000000000, 0.9659258262890683122, 1.000000000000000000, 0.9659258262890683122, 1.000000000000000000, 0.9659258262890683122, 1.000000000000000000, 0.9659258262890683122, 1.000000000000000000, 0.9659258262890683122, 1.000000000000000000, 0.9659258262890683122, 1.000000000000000000, 0.9659258262890683122, 1.000000000000000000, 0.9659258262890683122, 1.000000000000000000, 0.9659258262890683122, 1.000000000000000000, 0.9659258262890683122, 1.000000000000000000, 0.9659258262890683122, 1.000000000000000000, 0.9659258262890683122, 1.000000000000000000, 0.9659258262890683122, 1.000000000000000000, 0.9659258262890683122, 1.000000000000000000, 0.9659258262890683122, 1.000000000000000000, 0.9659258262890683122, 1.000000000000000000, 0.9659258262890683122, 1.000000000000000000, 0.9659258262890683122, 1.000000000000000000, 0.9659258262890683122, 1.000000000000000000, 0.9659258262890683122, 1.000000000000000000, 0.9659258262890683122, 1.000000000000000000, 0.9659258262890683122, 1.000000000000000000, 0.9659258262890683122, 1.000000000000000000, 0.9659258262890683122, 1.000000000000000000, 0.9659258262890683122, 1.000000000000000000, 0.9659258262890683122, 1.000000000000000000, 0.9659258262890683122, 1.000000000000000000, 0.9659258262890683122, 1.000000000000000000, 0.9659258262890683122, 1.000000000000000000, 0.9659258262890683122, 1.000000000000000000, 0.9659258262890683122, 1.000000000000000000, 0.9659258262890683122, 1.000000000000000000, 0.9659258262890683122, 1.000000000000000000, 0.9659258262890683122, 1.000000000000000000, 0.9659258262890683122, 1.000000000000000000, 0.9659258262890683122, 1.000000000000000000, 0.9659258262890683122, 1.000000000000000000, 0.9659258262890683122, 1.000000000000000000, 0.9659258262890683122, 1.000000000000000000, 0.9659258262890683122, 1.000000000000000000, 0.9659258262890683122, 1.000000000000000000, 0.9659258262890683122, 1.000000000000000000, 0.9659258262890683122, 1.000000000000000000, 0.9659258262890683122, 1.000000000000000000, 0.9659258262890683122, 1.000000000000000000, 0.9659258262890683122, 1.000000000000000000, 0.9659258262890683122, 1.000000000000000000, 0.9659258262890683122, 1.000000000000000000, 0.9659258262890683122, 1.000000000000000000, 0.9659258262890683122, 1.000000000000000000, 0.9659258262890683122, 1.000000000000000000, 0.9659258262890683122, 1.000000000000000000, 0.9659258262890683122, 1.000000000000000000, 0.9659258262890683122, 1.000000000000000000, 0.9659258262890683122, 1.000000000000000000, 0.9659258262890683122, 1.000000000000000000, 0.9659258262890683122, 1.000000000000000000, 0.9659258262890683122, 1.000000000000000000, 0.9659258262890683122, 1.000000000000000000, 0.9659258262890683122, 1.000000000000000000, 0.9659258262890683122, 1.000000000000000000, 0.9659258262890683122, 1.000000000000000000, 0.9659258262890683122, 1.000000000000000000, 0.9659258262890683122, 1.000000000000000000, 0.9659258262890683122, 1.000000000000000000, 0.9659258262890683122, 1.000000000000000000, 0.9659258262890683122, 1.000000000000000000, 0.9659258262890683122, 1.000000000000000000, 0.9659258262890683122, 1.000000000000000000, 0.9659258262890683122, 1.000000000000000000, 0.9659258262890683122, 1.000000000000000000, 0.9659258262890683122, 1.000000000000000000, 0.9659258262890683122, 1.000000000000000000, 0.9659258262890683122, 1.000000000000000000, 0.9659258262890683122, 1.000000000000000000, 0.9659258262890683122, 1.000000000000000000, 0.9659258262890683122, 1.000000000000000000, 0.9659258262890683122, 1.000000000000000000, 0.9659258262890683122, 1.000000000000000000, 0.9659258262890683122, 1.000000000000000000, 0.9659258262890683122, 1.000000000000000000, 0.9659258262890683122, 1.000000000000000000, 0.9659258262890683122, 1.000000000000000000, 0.9659258262890683122, 1.000000000000000000, 0.9659258262890683122, 1.000000000000000000, 0.9659258262890683122, 1.000000000000000000, 0.9659258262890683122, 1.000000000000000000, 0.9659258262890683122, 1.000000000000000000, 0.9659258262890683122, 1.000000000000000000, 0.9659258262890683122, 1.000000000000000000, 0.9659258262890683122, 1.000000000000000000, 0.9659258262890683122, 1.000000000000000000, 0.9659258262890683122, 1.000000000000000000, 0.9659258262890683122, 1.000000000000000000, 0.9659258262890683122, 1.000000000000000000, 0.9659258262890683122, 1.000000000000000000, 0.9659258262890683122, 1.000000000000000000, 0.9659258262890683122, 1.000000000000000000, 0.9659258262890683122, 1.000000000000000000, 0.9659258262890683122, 1.000000000000000000, 0.9659258262890683122, 1.000000000000000000, 0.9659258262890683122, 1.000000000000000000, 0.9659258262890683122, 1.000000000000000000, 0.9659258262890683122, 1.000000000000000000, 0.9659258262890683122, 1.000000000000000000, 0.9659258262890683122, 1.000000000000000000, 0.9659258262890683122, 1.000000000000000000, 0.9659258262890683122, 1.000000000000000000, 0.9659258262890683122, 1.000000000000000000, 0.9659258262890683122, 1.000000000000000000, 0.9659258262890683122, 1.000000000000000000, 0.9659258262890683122, 1.000000000000000000, 0.9659258262890683122, 1.000000000000000000, 0.9659258262890683122, 1.000000000000000000, 0.9659258262890683122, 1.000000000000000000, 0.9659258262890683122, 1.000000000000000000, 0.9659258262890683122, 1.000000000000000000, 0.9659258262890683122, 1.000000000000000000, 0.9659258262890683122, 1.000000000000000000, 0.9659258262890683122, 1.000000000000000000, 0.9659258262890683122, 1.000000000000000000, 0.9659258262890683122, 1.000000000000000000, 0.9659258262890683122, 1.000000000000000000, 0.9659258262890683122, 1.000000000000000000, 0.9659258262890683122, 1.000000000000000000, 0.9659258262890683122, 1.000000000000000000, 0.9659258262890683122, 1.000000000000000000, 0.9659258262890683122, 1.000000000000000000, 0.9659258262890683122, 1.000000000000000000, 0.9659258262890683122, 1.000000000000000000, 0.9659258262890683122, 1.000000000000000000, 0.9659258262890683122, 1.000000000000000000, 0.9659258262890683122, 1.000000000000000000, 0.9659258262890683122, 1.000000000000000000, 0.9659258262890683122, 1.000000000000000000, 0.9659258262890683122, 1.000000000000000000, 0.9659258262890683122, 1.000000000000000000, 0.9659258262890683122, 1.000000000000000000, 0.9659258262890683122, 1.000000000000000000, 0.9659258262890683122, 1.000000000000000000, 0.9659258262890683122, 1.000000000000000000, 0.9659258262890683122, 1.000000000000000000, 0.9659258262890683122, 1.000000000000000000, 0.9659258262890683122, 1.000000000000000000, 0.9659258262890683122, 1.000000000000000000, 0.9659258262890683122, 1.000000000000000000, 0.9659258262890683122, 1.000000000000000000, 0.9659258262890683122, 1.000000000000000000, 0.9659258262890683122, 1.000000000000000000, 0.9659258262890683122, 1.000000000000000000, 0.9659258262890683122, 1.000000000000000000, 0.9659258262890683122, 1.000000000000000000, 0.9659258262890683122, 1.000000000000000000, 0.9659258262890683122, 1.000000000000000000, 0.9659258262890683122, 1.000000000000000000, 0.9659258262890683122, 1.000000000000000000, 0.9659258262890683122, 1.000000000000000000, 0.9659258262890683122, 1.000000000000000000, 0.9659258262890683122, 1.000000000000000000, 0.9659258262890683122, 1.000000000000000000, 0.9659258262890683122, 1.000000000000000000, 0.9659258262890683122, 1.000000000000000000, 0.9659258262890683122, 1.000000000000000000, 0.9659258262890683122, 1.000000000000000000, 0.9659258262890683122, 1.000000000000000000, 0.9659258262890683122, 1.000000000000000000, 0.9659258262890683122, 1.000000000000000000, 0.9659258262890683122, 1.000000000000000000, 0.9659258262890683122, 1.000000000000000000, 0.9659258262890683122, 1.000000000000000000, 0.9659258262890683122, 1.000000000000000000, 0.9659258262890683122, 1.000000000000000000, 0.9659258262890683122, 1.000000000000000000, 0.9659258262890683122, 1.000000000000000000, 0.9659258262890683122, 1.000000000000000000, 0.9659258262890683122, 1.000000000000000000, 0.9659258262890683122, 1.000000000000000000, 0.9659258262890683122, 1.000000000000000000, 0.9659258262890683122, 1.000000000000000000, 0.9659258262890683122, 1.000000000000000000, 0.9659258262890683122, 1.000000000000000000, 0.9659258262890683122, 1.000000000000000000, 0.9659258262890683122, 1.000000000000000000, 0.9659258262890683122, 1.000000000000000000, 0.9659258262890683122, 1.000000000000000000, 0.9659258262890683122, 1.000000000000000000, 0.9659258262890683122, 1.000000000000000000, 0.9659258262890683122, 1.000000000000000000, 0.9659258262890683122, 1.000000000000000000, 0.9659258262890683122, 1.000000000000000000, 0.9659258262890683122, 1.000000000000000000, 0.9659258262890683122, 1.000000000000000000, 0.9659258262890683122, 1.000000000000000000, 0.9659258262890683122, 1.000000000000000000, 0.9659258262890683122, 1.000000000000000000, 0.9659258262890683122, 1.000000000000000000, 0.9659258262890683122, 1.000000000000000000, 0.9659258262890683122, 1.000000000000000000, 0.9659258262890683122, 1.000000000000000000, 0.9659258262890683122, 1.000000000000000000, 0.9659258262890683122, 1.000000000000000000, 0.9659258262890683122, 1.000000000000000000, 0.9659258262890683122, 1.000000000000000000, 0.9659258262890683122, 1.000000000000000000, 0.9659258262890683122, 1.000000000000000000, 0.9659258262890683122, 1.000000000000000000, 0.9659258262890683122, 1.000000000000000000, 0.9659258262890683122, 1.000000000000000000, 0.9659258262890683122, 1.000000000000000000, 0.9659258262890683122, 1.000000000000000000, 0.9659258262890683122, 1.000000000000000000, 0.9659258262890683122, 1.000000000000000000, 0.9659258262890683122, 1.000000000000000000, 0.9659258262890683122, 1.000000000000000000, 0.9659258262890683122, 1.000000000000000000),
 ( 0.3333333333333333703, 0.3219752754296894559, 0.3333333333333333703, 0.3219752754296894559, 0.3333333333333333703, 0.3219752754296894559, 0.3333333333333333703, 0.3219752754296894559, 0.3333333333333333703, 0.3219752754296894559, 0.3333333333333333703, 0.3219752754296894559, 0.3333333333333333703, 0.3219752754296894559, 0.3333333333333333703, 0.3219752754296894559, 0.3333333333333333703, 0.3219752754296894559, 0.3333333333333333703, 0.3219752754296894559, 0.3333333333333333703, 0.3219752754296894559, 0.3333333333333333703, 0.3219752754296894559, 0.3333333333333333703, 0.3219752754296894559, 0.3333333333333333703, 0.3219752754296894559, 0.3333333333333333703, 0.3219752754296894559, 0.3333333333333333703, 0.3219752754296894559, 0.3333333333333333703, 0.3219752754296894559, 0.3333333333333333703, 0.3219752754296894559, 0.3333333333333333703, 0.3219752754296894559, 0.3333333333333333703, 0.3219752754296894559, 0.3333333333333333703, 0.3219752754296894559, 0.3333333333333333703, 0.3219752754296894559, 0.3333333333333333703, 0.3219752754296894559, 0.3333333333333333703, 0.3219752754296894559, 0.3333333333333333703, 0.3219752754296894559, 0.3333333333333333703, 0.3219752754296894559, 0.3333333333333333703, 0.3219752754296894559, 0.3333333333333333703, 0.3219752754296894559, 0.3333333333333333703, 0.3219752754296894559, 0.3333333333333333703, 0.3219752754296894559, 0.3333333333333333703, 0.3219752754296894559, 0.3333333333333333703, 0.3219752754296894559, 0.3333333333333333703, 0.3219752754296894559, 0.3333333333333333703, 0.3219752754296894559, 0.3333333333333333703, 0.3219752754296894559, 0.3333333333333333703, 0.3219752754296894559, 0.3333333333333333703, 0.3219752754296894559, 0.3333333333333333703, 0.3219752754296894559, 0.3333333333333333703, 0.3219752754296894559, 0.3333333333333333703, 0.3219752754296894559, 0.3333333333333333703, 0.3219752754296894559, 0.3333333333333333703, 0.3219752754296894559, 0.3333333333333333703, 0.3219752754296894559, 0.3333333333333333703, 0.3219752754296894559, 0.3333333333333333703, 0.3219752754296894559, 0.3333333333333333703, 0.3219752754296894559, 0.3333333333333333703, 0.3219752754296894559, 0.3333333333333333703, 0.3219752754296894559, 0.3333333333333333703, 0.3219752754296894559, 0.3333333333333333703, 0.3219752754296894559, 0.3333333333333333703, 0.3219752754296894559, 0.3333333333333333703, 0.3219752754296894559, 0.3333333333333333703, 0.3219752754296894559, 0.3333333333333333703, 0.3219752754296894559, 0.3333333333333333703, 0.3219752754296894559, 0.3333333333333333703, 0.3219752754296894559, 0.3333333333333333703, 0.3219752754296894559, 0.3333333333333333703, 0.3219752754296894559, 0.3333333333333333703, 0.3219752754296894559, 0.3333333333333333703, 0.3219752754296894559, 0.3333333333333333703, 0.3219752754296894559, 0.3333333333333333703, 0.3219752754296894559, 0.3333333333333333703, 0.3219752754296894559, 0.3333333333333333703, 0.3219752754296894559, 0.3333333333333333703, 0.3219752754296894559, 0.3333333333333333703, 0.3219752754296894559, 0.3333333333333333703, 0.3219752754296894559, 0.3333333333333333703, 0.3219752754296894559, 0.3333333333333333703, 0.3219752754296894559, 0.3333333333333333703, 0.3219752754296894559, 0.3333333333333333703, 0.3219752754296894559, 0.3333333333333333703, 0.3219752754296894559, 0.3333333333333333703, 0.3219752754296894559, 0.3333333333333333703, 0.3219752754296894559, 0.3333333333333333703, 0.3219752754296894559, 0.3333333333333333703, 0.3219752754296894559, 0.3333333333333333703, 0.3219752754296894559, 0.3333333333333333703, 0.3219752754296894559, 0.3333333333333333703, 0.3219752754296894559, 0.3333333333333333703, 0.3219752754296894559, 0.3333333333333333703, 0.3219752754296894559, 0.3333333333333333703, 0.3219752754296894559, 0.3333333333333333703, 0.3219752754296894559, 0.3333333333333333703, 0.3219752754296894559, 0.3333333333333333703, 0.3219752754296894559, 0.3333333333333333703, 0.3219752754296894559, 0.3333333333333333703, 0.3219752754296894559, 0.3333333333333333703, 0.3219752754296894559, 0.3333333333333333703, 0.3219752754296894559, 0.3333333333333333703, 0.3219752754296894559, 0.3333333333333333703, 0.3219752754296894559, 0.3333333333333333703, 0.3219752754296894559, 0.3333333333333333703, 0.3219752754296894559, 0.3333333333333333703, 0.3219752754296894559, 0.3333333333333333703, 0.3219752754296894559, 0.3333333333333333703, 0.3219752754296894559, 0.3333333333333333703, 0.3219752754296894559, 0.3333333333333333703, 0.3219752754296894559, 0.3333333333333333703, 0.3219752754296894559, 0.3333333333333333703, 0.3219752754296894559, 0.3333333333333333703, 0.3219752754296894559, 0.3333333333333333703, 0.3219752754296894559, 0.3333333333333333703, 0.3219752754296894559, 0.3333333333333333703, 0.3219752754296894559, 0.3333333333333333703, 0.3219752754296894559, 0.3333333333333333703, 0.3219752754296894559, 0.3333333333333333703, 0.3219752754296894559, 0.3333333333333333703, 0.3219752754296894559, 0.3333333333333333703, 0.3219752754296894559, 0.3333333333333333703, 0.3219752754296894559, 0.3333333333333333703, 0.3219752754296894559, 0.3333333333333333703, 0.3219752754296894559, 0.3333333333333333703, 0.3219752754296894559, 0.3333333333333333703, 0.3219752754296894559, 0.3333333333333333703, 0.3219752754296894559, 0.3333333333333333703, 0.3219752754296894559, 0.3333333333333333703, 0.3219752754296894559, 0.3333333333333333703, 0.3219752754296894559, 0.3333333333333333703, 0.3219752754296894559, 0.3333333333333333703, 0.3219752754296894559, 0.3333333333333333703, 0.3219752754296894559, 0.3333333333333333703, 0.3219752754296894559, 0.3333333333333333703, 0.3219752754296894559, 0.3333333333333333703, 0.3219752754296894559, 0.3333333333333333703, 0.3219752754296894559, 0.3333333333333333703, 0.3219752754296894559, 0.3333333333333333703, 0.3219752754296894559, 0.3333333333333333703, 0.3219752754296894559, 0.3333333333333333703, 0.3219752754296894559, 0.3333333333333333703, 0.3219752754296894559, 0.3333333333333333703, 0.3219752754296894559, 0.3333333333333333703, 0.3219752754296894559, 0.3333333333333333703, 0.3219752754296894559, 0.3333333333333333703, 0.3219752754296894559, 0.3333333333333333703, 0.3219752754296894559, 0.3333333333333333703, 0.3219752754296894559, 0.3333333333333333703, 0.3219752754296894559, 0.3333333333333333703, 0.3219752754296894559, 0.3333333333333333703, 0.3219752754296894559, 0.3333333333333333703, 0.3219752754296894559, 0.3333333333333333703, 0.3219752754296894559, 0.3333333333333333703, 0.3219752754296894559, 0.3333333333333333703, 0.3219752754296894559, 0.3333333333333333703, 0.3219752754296894559, 0.3333333333333333703, 0.3219752754296894559, 0.3333333333333333703, 0.3219752754296894559, 0.3333333333333333703, 0.3219752754296894559, 0.3333333333333333703, 0.3219752754296894559, 0.3333333333333333703, 0.3219752754296894559, 0.3333333333333333703, 0.3219752754296894559, 0.3333333333333333703, 0.3219752754296894559, 0.3333333333333333703, 0.3219752754296894559, 0.3333333333333333703, 0.3219752754296894559, 0.3333333333333333703, 0.3219752754296894559, 0.3333333333333333703, 0.3219752754296894559, 0.3333333333333333703, 0.3219752754296894559, 0.3333333333333333703, 0.3219752754296894559, 0.3333333333333333703, 0.3219752754296894559, 0.3333333333333333703, 0.3219752754296894559, 0.3333333333333333703, 0.3219752754296894559, 0.3333333333333333703, 0.3219752754296894559, 0.3333333333333333703, 0.3219752754296894559, 0.3333333333333333703, 0.3219752754296894559, 0.3333333333333333703, 0.3219752754296894559, 0.3333333333333333703, 0.3219752754296894559, 0.3333333333333333703, 0.3219752754296894559, 0.3333333333333333703, 0.3219752754296894559, 0.3333333333333333703, 0.3219752754296894559, 0.3333333333333333703, 0.3219752754296894559, 0.3333333333333333703, 0.3219752754296894559, 0.3333333333333333703, 0.3219752754296894559, 0.3333333333333333703, 0.3219752754296894559, 0.3333333333333333703, 0.3219752754296894559, 0.3333333333333333703, 0.3219752754296894559, 0.3333333333333333703, 0.3219752754296894559, 0.3333333333333333703, 0.3219752754296894559, 0.3333333333333333703, 0.3219752754296894559, 0.3333333333333333703, 0.3219752754296894559, 0.3333333333333333703, 0.3219752754296894559, 0.3333333333333333703, 0.3219752754296894559, 0.3333333333333333703, 0.3219752754296894559, 0.3333333333333333703, 0.3219752754296894559, 0.3333333333333333703, 0.3219752754296894559, 0.3333333333333333703, 0.3219752754296894559, 0.3333333333333333703, 0.3219752754296894559, 0.3333333333333333703, 0.3219752754296894559, 0.3333333333333333703, 0.3219752754296894559, 0.3333333333333333703, 0.3219752754296894559, 0.3333333333333333703, 0.3219752754296894559, 0.3333333333333333703, 0.3219752754296894559, 0.3333333333333333703, 0.3219752754296894559, 0.3333333333333333703, 0.3219752754296894559, 0.3333333333333333703, 0.3219752754296894559, 0.3333333333333333703, 0.3219752754296894559, 0.3333333333333333703, 0.3219752754296894559, 0.3333333333333333703, 0.3219752754296894559, 0.3333333333333333703, 0.3219752754296894559, 0.3333333333333333703, 0.3219752754296894559, 0.3333333333333333703, 0.3219752754296894559, 0.3333333333333333703, 0.3219752754296894559, 0.3333333333333333703, 0.3219752754296894559, 0.3333333333333333703, 0.3219752754296894559, 0.3333333333333333703, 0.3219752754296894559, 0.3333333333333333703, 0.3219752754296894559, 0.3333333333333333703, 0.3219752754296894559, 0.3333333333333333703, 0.3219752754296894559, 0.3333333333333333703, 0.3219752754296894559, 0.3333333333333333703, 0.3219752754296894559, 0.3333333333333333703, 0.3219752754296894559, 0.3333333333333333703, 0.3219752754296894559, 0.3333333333333333703, 0.3219752754296894559, 0.3333333333333333703, 0.3219752754296894559, 0.3333333333333333703, 0.3219752754296894559, 0.3333333333333333703, 0.3219752754296894559, 0.3333333333333333703, 0.3219752754296894559, 0.3333333333333333703, 0.3219752754296894559, 0.3333333333333333703, 0.3219752754296894559, 0.3333333333333333703, 0.3219752754296894559, 0.3333333333333333703, 0.3219752754296894559, 0.3333333333333333703, 0.3219752754296894559, 0.3333333333333333703, 0.3219752754296894559, 0.3333333333333333703, 0.3219752754296894559, 0.3333333333333333703, 0.3219752754296894559, 0.3333333333333333703, 0.3219752754296894559, 0.3333333333333333703, 0.3219752754296894559, 0.3333333333333333703, 0.3219752754296894559, 0.3333333333333333703, 0.3219752754296894559, 0.3333333333333333703, 0.3219752754296894559, 0.3333333333333333703),
 ( 0.3333333333333333703, 0.3219752754296894559, 0.3333333333333333703, 0.3219752754296894559, 0.3333333333333333703, 0.3219752754296894559, 0.3333333333333333703, 0.3219752754296894559, 0.3333333333333333703, 0.3219752754296894559, 0.3333333333333333703, 0.3219752754296894559, 0.3333333333333333703, 0.3219752754296894559, 0.3333333333333333703, 0.3219752754296894559, 0.3333333333333333703, 0.3219752754296894559, 0.3333333333333333703, 0.3219752754296894559, 0.3333333333333333703, 0.3219752754296894559, 0.3333333333333333703, 0.3219752754296894559, 0.3333333333333333703, 0.3219752754296894559, 0.3333333333333333703, 0.3219752754296894559, 0.3333333333333333703, 0.3219752754296894559, 0.3333333333333333703, 0.3219752754296894559, 0.3333333333333333703, 0.3219752754296894559, 0.3333333333333333703, 0.3219752754296894559, 0.3333333333333333703, 0.3219752754296894559, 0.3333333333333333703, 0.3219752754296894559, 0.3333333333333333703, 0.3219752754296894559, 0.3333333333333333703, 0.3219752754296894559, 0.3333333333333333703, 0.3219752754296894559, 0.3333333333333333703, 0.3219752754296894559, 0.3333333333333333703, 0.3219752754296894559, 0.3333333333333333703, 0.3219752754296894559, 0.3333333333333333703, 0.3219752754296894559, 0.3333333333333333703, 0.3219752754296894559, 0.3333333333333333703, 0.3219752754296894559, 0.3333333333333333703, 0.3219752754296894559, 0.3333333333333333703, 0.3219752754296894559, 0.3333333333333333703, 0.3219752754296894559, 0.3333333333333333703, 0.3219752754296894559, 0.3333333333333333703, 0.3219752754296894559, 0.3333333333333333703, 0.3219752754296894559, 0.3333333333333333703, 0.3219752754296894559, 0.3333333333333333703, 0.3219752754296894559, 0.3333333333333333703, 0.3219752754296894559, 0.3333333333333333703, 0.3219752754296894559, 0.3333333333333333703, 0.3219752754296894559, 0.3333333333333333703, 0.3219752754296894559, 0.3333333333333333703, 0.3219752754296894559, 0.3333333333333333703, 0.3219752754296894559, 0.3333333333333333703, 0.3219752754296894559, 0.3333333333333333703, 0.3219752754296894559, 0.3333333333333333703, 0.3219752754296894559, 0.3333333333333333703, 0.3219752754296894559, 0.3333333333333333703, 0.3219752754296894559, 0.3333333333333333703, 0.3219752754296894559, 0.3333333333333333703, 0.3219752754296894559, 0.3333333333333333703, 0.3219752754296894559, 0.3333333333333333703, 0.3219752754296894559, 0.3333333333333333703, 0.3219752754296894559, 0.3333333333333333703, 0.3219752754296894559, 0.3333333333333333703, 0.3219752754296894559, 0.3333333333333333703, 0.3219752754296894559, 0.3333333333333333703, 0.3219752754296894559, 0.3333333333333333703, 0.3219752754296894559, 0.3333333333333333703, 0.3219752754296894559, 0.3333333333333333703, 0.3219752754296894559, 0.3333333333333333703, 0.3219752754296894559, 0.3333333333333333703, 0.3219752754296894559, 0.3333333333333333703, 0.3219752754296894559, 0.3333333333333333703, 0.3219752754296894559, 0.3333333333333333703, 0.3219752754296894559, 0.3333333333333333703, 0.3219752754296894559, 0.3333333333333333703, 0.3219752754296894559, 0.3333333333333333703, 0.3219752754296894559, 0.3333333333333333703, 0.3219752754296894559, 0.3333333333333333703, 0.3219752754296894559, 0.3333333333333333703, 0.3219752754296894559, 0.3333333333333333703, 0.3219752754296894559, 0.3333333333333333703, 0.3219752754296894559, 0.3333333333333333703, 0.3219752754296894559, 0.3333333333333333703, 0.3219752754296894559, 0.3333333333333333703, 0.3219752754296894559, 0.3333333333333333703, 0.3219752754296894559, 0.3333333333333333703, 0.3219752754296894559, 0.3333333333333333703, 0.3219752754296894559, 0.3333333333333333703, 0.3219752754296894559, 0.3333333333333333703, 0.3219752754296894559, 0.3333333333333333703, 0.3219752754296894559, 0.3333333333333333703, 0.3219752754296894559, 0.3333333333333333703, 0.3219752754296894559, 0.3333333333333333703, 0.3219752754296894559, 0.3333333333333333703, 0.3219752754296894559, 0.3333333333333333703, 0.3219752754296894559, 0.3333333333333333703, 0.3219752754296894559, 0.3333333333333333703, 0.3219752754296894559, 0.3333333333333333703, 0.3219752754296894559, 0.3333333333333333703, 0.3219752754296894559, 0.3333333333333333703, 0.3219752754296894559, 0.3333333333333333703, 0.3219752754296894559, 0.3333333333333333703, 0.3219752754296894559, 0.3333333333333333703, 0.3219752754296894559, 0.3333333333333333703, 0.3219752754296894559, 0.3333333333333333703, 0.3219752754296894559, 0.3333333333333333703, 0.3219752754296894559, 0.3333333333333333703, 0.3219752754296894559, 0.3333333333333333703, 0.3219752754296894559, 0.3333333333333333703, 0.3219752754296894559, 0.3333333333333333703, 0.3219752754296894559, 0.3333333333333333703, 0.3219752754296894559, 0.3333333333333333703, 0.3219752754296894559, 0.3333333333333333703, 0.3219752754296894559, 0.3333333333333333703, 0.3219752754296894559, 0.3333333333333333703, 0.3219752754296894559, 0.3333333333333333703, 0.3219752754296894559, 0.3333333333333333703, 0.3219752754296894559, 0.3333333333333333703, 0.3219752754296894559, 0.3333333333333333703, 0.3219752754296894559, 0.3333333333333333703, 0.3219752754296894559, 0.3333333333333333703, 0.3219752754296894559, 0.3333333333333333703, 0.3219752754296894559, 0.3333333333333333703, 0.3219752754296894559, 0.3333333333333333703, 0.3219752754296894559, 0.3333333333333333703, 0.3219752754296894559, 0.3333333333333333703, 0.3219752754296894559, 0.3333333333333333703, 0.3219752754296894559, 0.3333333333333333703, 0.3219752754296894559, 0.3333333333333333703, 0.3219752754296894559, 0.3333333333333333703, 0.3219752754296894559, 0.3333333333333333703, 0.3219752754296894559, 0.3333333333333333703, 0.3219752754296894559, 0.3333333333333333703, 0.3219752754296894559, 0.3333333333333333703, 0.3219752754296894559, 0.3333333333333333703, 0.3219752754296894559, 0.3333333333333333703, 0.3219752754296894559, 0.3333333333333333703, 0.3219752754296894559, 0.3333333333333333703, 0.3219752754296894559, 0.3333333333333333703, 0.3219752754296894559, 0.3333333333333333703, 0.3219752754296894559, 0.3333333333333333703, 0.3219752754296894559, 0.3333333333333333703, 0.3219752754296894559, 0.3333333333333333703, 0.3219752754296894559, 0.3333333333333333703, 0.3219752754296894559, 0.3333333333333333703, 0.3219752754296894559, 0.3333333333333333703, 0.3219752754296894559, 0.3333333333333333703, 0.3219752754296894559, 0.3333333333333333703, 0.3219752754296894559, 0.3333333333333333703, 0.3219752754296894559, 0.3333333333333333703, 0.3219752754296894559, 0.3333333333333333703, 0.3219752754296894559, 0.3333333333333333703, 0.3219752754296894559, 0.3333333333333333703, 0.3219752754296894559, 0.3333333333333333703, 0.3219752754296894559, 0.3333333333333333703, 0.3219752754296894559, 0.3333333333333333703, 0.3219752754296894559, 0.3333333333333333703, 0.3219752754296894559, 0.3333333333333333703, 0.3219752754296894559, 0.3333333333333333703, 0.3219752754296894559, 0.3333333333333333703, 0.3219752754296894559, 0.3333333333333333703, 0.3219752754296894559, 0.3333333333333333703, 0.3219752754296894559, 0.3333333333333333703, 0.3219752754296894559, 0.3333333333333333703, 0.3219752754296894559, 0.3333333333333333703, 0.3219752754296894559, 0.3333333333333333703, 0.3219752754296894559, 0.3333333333333333703, 0.3219752754296894559, 0.3333333333333333703, 0.3219752754296894559, 0.3333333333333333703, 0.3219752754296894559, 0.3333333333333333703, 0.3219752754296894559, 0.3333333333333333703, 0.3219752754296894559, 0.3333333333333333703, 0.3219752754296894559, 0.3333333333333333703, 0.3219752754296894559, 0.3333333333333333703, 0.3219752754296894559, 0.3333333333333333703, 0.3219752754296894559, 0.3333333333333333703, 0.3219752754296894559, 0.3333333333333333703, 0.3219752754296894559, 0.3333333333333333703, 0.3219752754296894559, 0.3333333333333333703, 0.3219752754296894559, 0.3333333333333333703, 0.3219752754296894559, 0.3333333333333333703, 0.3219752754296894559, 0.3333333333333333703, 0.3219752754296894559, 0.3333333333333333703, 0.3219752754296894559, 0.3333333333333333703, 0.3219752754296894559, 0.3333333333333333703, 0.3219752754296894559, 0.3333333333333333703, 0.3219752754296894559, 0.3333333333333333703, 0.3219752754296894559, 0.3333333333333333703, 0.3219752754296894559, 0.3333333333333333703, 0.3219752754296894559, 0.3333333333333333703, 0.3219752754296894559, 0.3333333333333333703, 0.3219752754296894559, 0.3333333333333333703, 0.3219752754296894559, 0.3333333333333333703, 0.3219752754296894559, 0.3333333333333333703, 0.3219752754296894559, 0.3333333333333333703, 0.3219752754296894559, 0.3333333333333333703, 0.3219752754296894559, 0.3333333333333333703, 0.3219752754296894559, 0.3333333333333333703, 0.3219752754296894559, 0.3333333333333333703, 0.3219752754296894559, 0.3333333333333333703, 0.3219752754296894559, 0.3333333333333333703, 0.3219752754296894559, 0.3333333333333333703, 0.3219752754296894559, 0.3333333333333333703, 0.3219752754296894559, 0.3333333333333333703, 0.3219752754296894559, 0.3333333333333333703, 0.3219752754296894559, 0.3333333333333333703, 0.3219752754296894559, 0.3333333333333333703, 0.3219752754296894559, 0.3333333333333333703, 0.3219752754296894559, 0.3333333333333333703, 0.3219752754296894559, 0.3333333333333333703, 0.3219752754296894559, 0.3333333333333333703, 0.3219752754296894559, 0.3333333333333333703, 0.3219752754296894559, 0.3333333333333333703, 0.3219752754296894559, 0.3333333333333333703, 0.3219752754296894559, 0.3333333333333333703, 0.3219752754296894559, 0.3333333333333333703, 0.3219752754296894559, 0.3333333333333333703, 0.3219752754296894559, 0.3333333333333333703, 0.3219752754296894559, 0.3333333333333333703, 0.3219752754296894559, 0.3333333333333333703, 0.3219752754296894559, 0.3333333333333333703, 0.3219752754296894559, 0.3333333333333333703, 0.3219752754296894559, 0.3333333333333333703, 0.3219752754296894559, 0.3333333333333333703, 0.3219752754296894559, 0.3333333333333333703, 0.3219752754296894559, 0.3333333333333333703, 0.3219752754296894559, 0.3333333333333333703, 0.3219752754296894559, 0.3333333333333333703, 0.3219752754296894559, 0.3333333333333333703, 0.3219752754296894559, 0.3333333333333333703, 0.3219752754296894559, 0.3333333333333333703, 0.3219752754296894559, 0.3333333333333333703, 0.3219752754296894559, 0.3333333333333333703, 0.3219752754296894559, 0.3333333333333333703, 0.3219752754296894559, 0.3333333333333333703, 0.3219752754296894559, 0.3333333333333333703, 0.3219752754296894559, 0.3333333333333333703),
 ( 1.000000000000000000, 0.9659258262890683122, 1.000000000000000000, 0.9659258262890683122, 1.000000000000000000, 0.9659258262890683122, 1.000000000000000000, 0.9659258262890683122, 1.000000000000000000, 0.9659258262890683122, 1.000000000000000000, 0.9659258262890683122, 1.000000000000000000, 0.9659258262890683122, 1.000000000000000000, 0.9659258262890683122, 1.000000000000000000, 0.9659258262890683122, 1.000000000000000000, 0.9659258262890683122, 1.000000000000000000, 0.9659258262890683122, 1.000000000000000000, 0.9659258262890683122, 1.000000000000000000, 0.9659258262890683122, 1.000000000000000000, 0.9659258262890683122, 1.000000000000000000, 0.9659258262890683122, 1.000000000000000000, 0.9659258262890683122, 1.000000000000000000, 0.9659258262890683122, 1.000000000000000000, 0.9659258262890683122, 1.000000000000000000, 0.9659258262890683122, 1.000000000000000000, 0.9659258262890683122, 1.000000000000000000, 0.9659258262890683122, 1.000000000000000000, 0.9659258262890683122, 1.000000000000000000, 0.9659258262890683122, 1.000000000000000000, 0.9659258262890683122, 1.000000000000000000, 0.9659258262890683122, 1.000000000000000000, 0.9659258262890683122, 1.000000000000000000, 0.9659258262890683122, 1.000000000000000000, 0.9659258262890683122, 1.000000000000000000, 0.9659258262890683122, 1.000000000000000000, 0.9659258262890683122, 1.000000000000000000, 0.9659258262890683122, 1.000000000000000000, 0.9659258262890683122, 1.000000000000000000, 0.9659258262890683122, 1.000000000000000000, 0.9659258262890683122, 1.000000000000000000, 0.9659258262890683122, 1.000000000000000000, 0.9659258262890683122, 1.000000000000000000, 0.9659258262890683122, 1.000000000000000000, 0.9659258262890683122, 1.000000000000000000, 0.9659258262890683122, 1.000000000000000000, 0.9659258262890683122, 1.000000000000000000, 0.9659258262890683122, 1.000000000000000000, 0.9659258262890683122, 1.000000000000000000, 0.9659258262890683122, 1.000000000000000000, 0.9659258262890683122, 1.000000000000000000, 0.9659258262890683122, 1.000000000000000000, 0.9659258262890683122, 1.000000000000000000, 0.9659258262890683122, 1.000000000000000000, 0.9659258262890683122, 1.000000000000000000, 0.9659258262890683122, 1.000000000000000000, 0.9659258262890683122, 1.000000000000000000, 0.9659258262890683122, 1.000000000000000000, 0.9659258262890683122, 1.000000000000000000, 0.9659258262890683122, 1.000000000000000000, 0.9659258262890683122, 1.000000000000000000, 0.9659258262890683122, 1.000000000000000000, 0.9659258262890683122, 1.000000000000000000, 0.9659258262890683122, 1.000000000000000000, 0.9659258262890683122, 1.000000000000000000, 0.9659258262890683122, 1.000000000000000000, 0.9659258262890683122, 1.000000000000000000, 0.9659258262890683122, 1.000000000000000000, 0.9659258262890683122, 1.000000000000000000, 0.9659258262890683122, 1.000000000000000000, 0.9659258262890683122, 1.000000000000000000, 0.9659258262890683122, 1.000000000000000000, 0.9659258262890683122, 1.000000000000000000, 0.9659258262890683122, 1.000000000000000000, 0.9659258262890683122, 1.000000000000000000, 0.9659258262890683122, 1.000000000000000000, 0.9659258262890683122, 1.000000000000000000, 0.9659258262890683122, 1.000000000000000000, 0.9659258262890683122, 1.000000000000000000, 0.9659258262890683122, 1.000000000000000000, 0.9659258262890683122, 1.000000000000000000, 0.9659258262890683122, 1.000000000000000000, 0.9659258262890683122, 1.000000000000000000, 0.9659258262890683122, 1.000000000000000000, 0.9659258262890683122, 1.000000000000000000, 0.9659258262890683122, 1.000000000000000000, 0.9659258262890683122, 1.000000000000000000, 0.9659258262890683122, 1.000000000000000000, 0.9659258262890683122, 1.000000000000000000, 0.9659258262890683122, 1.000000000000000000, 0.9659258262890683122, 1.000000000000000000, 0.9659258262890683122, 1.000000000000000000, 0.9659258262890683122, 1.000000000000000000, 0.9659258262890683122, 1.000000000000000000, 0.9659258262890683122, 1.000000000000000000, 0.9659258262890683122, 1.000000000000000000, 0.9659258262890683122, 1.000000000000000000, 0.9659258262890683122, 1.000000000000000000, 0.9659258262890683122, 1.000000000000000000, 0.9659258262890683122, 1.000000000000000000, 0.9659258262890683122, 1.000000000000000000, 0.9659258262890683122, 1.000000000000000000, 0.9659258262890683122, 1.000000000000000000, 0.9659258262890683122, 1.000000000000000000, 0.9659258262890683122, 1.000000000000000000, 0.9659258262890683122, 1.000000000000000000, 0.9659258262890683122, 1.000000000000000000, 0.9659258262890683122, 1.000000000000000000, 0.9659258262890683122, 1.000000000000000000, 0.9659258262890683122, 1.000000000000000000, 0.9659258262890683122, 1.000000000000000000, 0.9659258262890683122, 1.000000000000000000, 0.9659258262890683122, 1.000000000000000000, 0.9659258262890683122, 1.000000000000000000, 0.9659258262890683122, 1.000000000000000000, 0.9659258262890683122, 1.000000000000000000, 0.9659258262890683122, 1.000000000000000000, 0.9659258262890683122, 1.000000000000000000, 0.9659258262890683122, 1.000000000000000000, 0.9659258262890683122, 1.000000000000000000, 0.9659258262890683122, 1.000000000000000000, 0.9659258262890683122, 1.000000000000000000, 0.9659258262890683122, 1.000000000000000000, 0.9659258262890683122, 1.000000000000000000, 0.9659258262890683122, 1.000000000000000000, 0.9659258262890683122, 1.000000000000000000, 0.9659258262890683122, 1.000000000000000000, 0.9659258262890683122, 1.000000000000000000, 0.9659258262890683122, 1.000000000000000000, 0.9659258262890683122, 1.000000000000000000, 0.9659258262890683122, 1.000000000000000000, 0.9659258262890683122, 1.000000000000000000, 0.9659258262890683122, 1.000000000000000000, 0.9659258262890683122, 1.000000000000000000, 0.9659258262890683122, 1.000000000000000000, 0.9659258262890683122, 1.000000000000000000, 0.9659258262890683122, 1.000000000000000000, 0.9659258262890683122, 1.000000000000000000, 0.9659258262890683122, 1.000000000000000000, 0.9659258262890683122, 1.000000000000000000, 0.9659258262890683122, 1.000000000000000000, 0.9659258262890683122, 1.000000000000000000, 0.9659258262890683122, 1.000000000000000000, 0.9659258262890683122, 1.000000000000000000, 0.9659258262890683122, 1.000000000000000000, 0.9659258262890683122, 1.000000000000000000, 0.9659258262890683122, 1.000000000000000000, 0.9659258262890683122, 1.000000000000000000, 0.9659258262890683122, 1.000000000000000000, 0.9659258262890683122, 1.000000000000000000, 0.9659258262890683122, 1.000000000000000000, 0.9659258262890683122, 1.000000000000000000, 0.9659258262890683122, 1.000000000000000000, 0.9659258262890683122, 1.000000000000000000, 0.9659258262890683122, 1.000000000000000000, 0.9659258262890683122, 1.000000000000000000, 0.9659258262890683122, 1.000000000000000000, 0.9659258262890683122, 1.000000000000000000, 0.9659258262890683122, 1.000000000000000000, 0.9659258262890683122, 1.000000000000000000, 0.9659258262890683122, 1.000000000000000000, 0.9659258262890683122, 1.000000000000000000, 0.9659258262890683122, 1.000000000000000000, 0.9659258262890683122, 1.000000000000000000, 0.9659258262890683122, 1.000000000000000000, 0.9659258262890683122, 1.000000000000000000, 0.9659258262890683122, 1.000000000000000000, 0.9659258262890683122, 1.000000000000000000, 0.9659258262890683122, 1.000000000000000000, 0.9659258262890683122, 1.000000000000000000, 0.9659258262890683122, 1.000000000000000000, 0.9659258262890683122, 1.000000000000000000, 0.9659258262890683122, 1.000000000000000000, 0.9659258262890683122, 1.000000000000000000, 0.9659258262890683122, 1.000000000000000000, 0.9659258262890683122, 1.000000000000000000, 0.9659258262890683122, 1.000000000000000000, 0.9659258262890683122, 1.000000000000000000, 0.9659258262890683122, 1.000000000000000000, 0.9659258262890683122, 1.000000000000000000, 0.9659258262890683122, 1.000000000000000000, 0.9659258262890683122, 1.000000000000000000, 0.9659258262890683122, 1.000000000000000000, 0.9659258262890683122, 1.000000000000000000, 0.9659258262890683122, 1.000000000000000000, 0.9659258262890683122, 1.000000000000000000, 0.9659258262890683122, 1.000000000000000000, 0.9659258262890683122, 1.000000000000000000, 0.9659258262890683122, 1.000000000000000000, 0.9659258262890683122, 1.000000000000000000, 0.9659258262890683122, 1.000000000000000000, 0.9659258262890683122, 1.000000000000000000, 0.9659258262890683122, 1.000000000000000000, 0.9659258262890683122, 1.000000000000000000, 0.9659258262890683122, 1.000000000000000000, 0.9659258262890683122, 1.000000000000000000, 0.9659258262890683122, 1.000000000000000000, 0.9659258262890683122, 1.000000000000000000, 0.9659258262890683122, 1.000000000000000000, 0.9659258262890683122, 1.000000000000000000, 0.9659258262890683122, 1.000000000000000000, 0.9659258262890683122, 1.000000000000000000, 0.9659258262890683122, 1.000000000000000000, 0.9659258262890683122, 1.000000000000000000, 0.9659258262890683122, 1.000000000000000000, 0.9659258262890683122, 1.000000000000000000, 0.9659258262890683122, 1.000000000000000000, 0.9659258262890683122, 1.000000000000000000, 0.9659258262890683122, 1.000000000000000000, 0.9659258262890683122, 1.000000000000000000, 0.9659258262890683122, 1.000000000000000000, 0.9659258262890683122, 1.000000000000000000, 0.9659258262890683122, 1.000000000000000000, 0.9659258262890683122, 1.000000000000000000, 0.9659258262890683122, 1.000000000000000000, 0.9659258262890683122, 1.000000000000000000, 0.9659258262890683122, 1.000000000000000000, 0.9659258262890683122, 1.000000000000000000, 0.9659258262890683122, 1.000000000000000000, 0.9659258262890683122, 1.000000000000000000, 0.9659258262890683122, 1.000000000000000000, 0.9659258262890683122, 1.000000000000000000, 0.9659258262890683122, 1.000000000000000000, 0.9659258262890683122, 1.000000000000000000, 0.9659258262890683122, 1.000000000000000000, 0.9659258262890683122, 1.000000000000000000, 0.9659258262890683122, 1.000000000000000000, 0.9659258262890683122, 1.000000000000000000, 0.9659258262890683122, 1.000000000000000000, 0.9659258262890683122, 1.000000000000000000, 0.9659258262890683122, 1.000000000000000000, 0.9659258262890683122, 1.000000000000000000, 0.9659258262890683122, 1.000000000000000000, 0.9659258262890683122, 1.000000000000000000, 0.9659258262890683122, 1.000000000000000000),
 ( 0.3333333333333333703, 0.3219752754296894559, 0.3333333333333333703, 0.3219752754296894559, 0.3333333333333333703, 0.3219752754296894559, 0.3333333333333333703, 0.3219752754296894559, 0.3333333333333333703, 0.3219752754296894559, 0.3333333333333333703, 0.3219752754296894559, 0.3333333333333333703, 0.3219752754296894559, 0.3333333333333333703, 0.3219752754296894559, 0.3333333333333333703, 0.3219752754296894559, 0.3333333333333333703, 0.3219752754296894559, 0.3333333333333333703, 0.3219752754296894559, 0.3333333333333333703, 0.3219752754296894559, 0.3333333333333333703, 0.3219752754296894559, 0.3333333333333333703, 0.3219752754296894559, 0.3333333333333333703, 0.3219752754296894559, 0.3333333333333333703, 0.3219752754296894559, 0.3333333333333333703, 0.3219752754296894559, 0.3333333333333333703, 0.3219752754296894559, 0.3333333333333333703, 0.3219752754296894559, 0.3333333333333333703, 0.3219752754296894559, 0.3333333333333333703, 0.3219752754296894559, 0.3333333333333333703, 0.3219752754296894559, 0.3333333333333333703, 0.3219752754296894559, 0.3333333333333333703, 0.3219752754296894559, 0.3333333333333333703, 0.3219752754296894559, 0.3333333333333333703, 0.3219752754296894559, 0.3333333333333333703, 0.3219752754296894559, 0.3333333333333333703, 0.3219752754296894559, 0.3333333333333333703, 0.3219752754296894559, 0.3333333333333333703, 0.3219752754296894559, 0.3333333333333333703, 0.3219752754296894559, 0.3333333333333333703, 0.3219752754296894559, 0.3333333333333333703, 0.3219752754296894559, 0.3333333333333333703, 0.3219752754296894559, 0.3333333333333333703, 0.3219752754296894559, 0.3333333333333333703, 0.3219752754296894559, 0.3333333333333333703, 0.3219752754296894559, 0.3333333333333333703, 0.3219752754296894559, 0.3333333333333333703, 0.3219752754296894559, 0.3333333333333333703, 0.3219752754296894559, 0.3333333333333333703, 0.3219752754296894559, 0.3333333333333333703, 0.3219752754296894559, 0.3333333333333333703, 0.3219752754296894559, 0.3333333333333333703, 0.3219752754296894559, 0.3333333333333333703, 0.3219752754296894559, 0.3333333333333333703, 0.3219752754296894559, 0.3333333333333333703, 0.3219752754296894559, 0.3333333333333333703, 0.3219752754296894559, 0.3333333333333333703, 0.3219752754296894559, 0.3333333333333333703, 0.3219752754296894559, 0.3333333333333333703, 0.3219752754296894559, 0.3333333333333333703, 0.3219752754296894559, 0.3333333333333333703, 0.3219752754296894559, 0.3333333333333333703, 0.3219752754296894559, 0.3333333333333333703, 0.3219752754296894559, 0.3333333333333333703, 0.3219752754296894559, 0.3333333333333333703, 0.3219752754296894559, 0.3333333333333333703, 0.3219752754296894559, 0.3333333333333333703, 0.3219752754296894559, 0.3333333333333333703, 0.3219752754296894559, 0.3333333333333333703, 0.3219752754296894559, 0.3333333333333333703, 0.3219752754296894559, 0.3333333333333333703, 0.3219752754296894559, 0.3333333333333333703, 0.3219752754296894559, 0.3333333333333333703, 0.3219752754296894559, 0.3333333333333333703, 0.3219752754296894559, 0.3333333333333333703, 0.3219752754296894559, 0.3333333333333333703, 0.3219752754296894559, 0.3333333333333333703, 0.3219752754296894559, 0.3333333333333333703, 0.3219752754296894559, 0.3333333333333333703, 0.3219752754296894559, 0.3333333333333333703, 0.3219752754296894559, 0.3333333333333333703, 0.3219752754296894559, 0.3333333333333333703, 0.3219752754296894559, 0.3333333333333333703, 0.3219752754296894559, 0.3333333333333333703, 0.3219752754296894559, 0.3333333333333333703, 0.3219752754296894559, 0.3333333333333333703, 0.3219752754296894559, 0.3333333333333333703, 0.3219752754296894559, 0.3333333333333333703, 0.3219752754296894559, 0.3333333333333333703, 0.3219752754296894559, 0.3333333333333333703, 0.3219752754296894559, 0.3333333333333333703, 0.3219752754296894559, 0.3333333333333333703, 0.3219752754296894559, 0.3333333333333333703, 0.3219752754296894559, 0.3333333333333333703, 0.3219752754296894559, 0.3333333333333333703, 0.3219752754296894559, 0.3333333333333333703, 0.3219752754296894559, 0.3333333333333333703, 0.3219752754296894559, 0.3333333333333333703, 0.3219752754296894559, 0.3333333333333333703, 0.3219752754296894559, 0.3333333333333333703, 0.3219752754296894559, 0.3333333333333333703, 0.3219752754296894559, 0.3333333333333333703, 0.3219752754296894559, 0.3333333333333333703, 0.3219752754296894559, 0.3333333333333333703, 0.3219752754296894559, 0.3333333333333333703, 0.3219752754296894559, 0.3333333333333333703, 0.3219752754296894559, 0.3333333333333333703, 0.3219752754296894559, 0.3333333333333333703, 0.3219752754296894559, 0.3333333333333333703, 0.3219752754296894559, 0.3333333333333333703, 0.3219752754296894559, 0.3333333333333333703, 0.3219752754296894559, 0.3333333333333333703, 0.3219752754296894559, 0.3333333333333333703, 0.3219752754296894559, 0.3333333333333333703, 0.3219752754296894559, 0.3333333333333333703, 0.3219752754296894559, 0.3333333333333333703, 0.3219752754296894559, 0.3333333333333333703, 0.3219752754296894559, 0.3333333333333333703, 0.3219752754296894559, 0.3333333333333333703, 0.3219752754296894559, 0.3333333333333333703, 0.3219752754296894559, 0.3333333333333333703, 0.3219752754296894559, 0.3333333333333333703, 0.3219752754296894559, 0.3333333333333333703, 0.3219752754296894559, 0.3333333333333333703, 0.3219752754296894559, 0.3333333333333333703, 0.3219752754296894559, 0.3333333333333333703, 0.3219752754296894559, 0.3333333333333333703, 0.3219752754296894559, 0.3333333333333333703, 0.3219752754296894559, 0.3333333333333333703, 0.3219752754296894559, 0.3333333333333333703, 0.3219752754296894559, 0.3333333333333333703, 0.3219752754296894559, 0.3333333333333333703, 0.3219752754296894559, 0.3333333333333333703, 0.3219752754296894559, 0.3333333333333333703, 0.3219752754296894559, 0.3333333333333333703, 0.3219752754296894559, 0.3333333333333333703, 0.3219752754296894559, 0.3333333333333333703, 0.3219752754296894559, 0.3333333333333333703, 0.3219752754296894559, 0.3333333333333333703, 0.3219752754296894559, 0.3333333333333333703, 0.3219752754296894559, 0.3333333333333333703, 0.3219752754296894559, 0.3333333333333333703, 0.3219752754296894559, 0.3333333333333333703, 0.3219752754296894559, 0.3333333333333333703, 0.3219752754296894559, 0.3333333333333333703, 0.3219752754296894559, 0.3333333333333333703, 0.3219752754296894559, 0.3333333333333333703, 0.3219752754296894559, 0.3333333333333333703, 0.3219752754296894559, 0.3333333333333333703, 0.3219752754296894559, 0.3333333333333333703, 0.3219752754296894559, 0.3333333333333333703, 0.3219752754296894559, 0.3333333333333333703, 0.3219752754296894559, 0.3333333333333333703, 0.3219752754296894559, 0.3333333333333333703, 0.3219752754296894559, 0.3333333333333333703, 0.3219752754296894559, 0.3333333333333333703, 0.3219752754296894559, 0.3333333333333333703, 0.3219752754296894559, 0.3333333333333333703, 0.3219752754296894559, 0.3333333333333333703, 0.3219752754296894559, 0.3333333333333333703, 0.3219752754296894559, 0.3333333333333333703, 0.3219752754296894559, 0.3333333333333333703, 0.3219752754296894559, 0.3333333333333333703, 0.3219752754296894559, 0.3333333333333333703, 0.3219752754296894559, 0.3333333333333333703, 0.3219752754296894559, 0.3333333333333333703, 0.3219752754296894559, 0.3333333333333333703, 0.3219752754296894559, 0.3333333333333333703, 0.3219752754296894559, 0.3333333333333333703, 0.3219752754296894559, 0.3333333333333333703, 0.3219752754296894559, 0.3333333333333333703, 0.3219752754296894559, 0.3333333333333333703, 0.3219752754296894559, 0.3333333333333333703, 0.3219752754296894559, 0.3333333333333333703, 0.3219752754296894559, 0.3333333333333333703, 0.3219752754296894559, 0.3333333333333333703, 0.3219752754296894559, 0.3333333333333333703, 0.3219752754296894559, 0.3333333333333333703, 0.3219752754296894559, 0.3333333333333333703, 0.3219752754296894559, 0.3333333333333333703, 0.3219752754296894559, 0.3333333333333333703, 0.3219752754296894559, 0.3333333333333333703, 0.3219752754296894559, 0.3333333333333333703, 0.3219752754296894559, 0.3333333333333333703, 0.3219752754296894559, 0.3333333333333333703, 0.3219752754296894559, 0.3333333333333333703, 0.3219752754296894559, 0.3333333333333333703, 0.3219752754296894559, 0.3333333333333333703, 0.3219752754296894559, 0.3333333333333333703, 0.3219752754296894559, 0.3333333333333333703, 0.3219752754296894559, 0.3333333333333333703, 0.3219752754296894559, 0.3333333333333333703, 0.3219752754296894559, 0.3333333333333333703, 0.3219752754296894559, 0.3333333333333333703, 0.3219752754296894559, 0.3333333333333333703, 0.3219752754296894559, 0.3333333333333333703, 0.3219752754296894559, 0.3333333333333333703, 0.3219752754296894559, 0.3333333333333333703, 0.3219752754296894559, 0.3333333333333333703, 0.3219752754296894559, 0.3333333333333333703, 0.3219752754296894559, 0.3333333333333333703, 0.3219752754296894559, 0.3333333333333333703, 0.3219752754296894559, 0.3333333333333333703, 0.3219752754296894559, 0.3333333333333333703, 0.3219752754296894559, 0.3333333333333333703, 0.3219752754296894559, 0.3333333333333333703, 0.3219752754296894559, 0.3333333333333333703, 0.3219752754296894559, 0.3333333333333333703, 0.3219752754296894559, 0.3333333333333333703, 0.3219752754296894559, 0.3333333333333333703, 0.3219752754296894559, 0.3333333333333333703, 0.3219752754296894559, 0.3333333333333333703, 0.3219752754296894559, 0.3333333333333333703, 0.3219752754296894559, 0.3333333333333333703, 0.3219752754296894559, 0.3333333333333333703, 0.3219752754296894559, 0.3333333333333333703, 0.3219752754296894559, 0.3333333333333333703, 0.3219752754296894559, 0.3333333333333333703, 0.3219752754296894559, 0.3333333333333333703, 0.3219752754296894559, 0.3333333333333333703, 0.3219752754296894559, 0.3333333333333333703, 0.3219752754296894559, 0.3333333333333333703, 0.3219752754296894559, 0.3333333333333333703, 0.3219752754296894559, 0.3333333333333333703, 0.3219752754296894559, 0.3333333333333333703, 0.3219752754296894559, 0.3333333333333333703, 0.3219752754296894559, 0.3333333333333333703, 0.3219752754296894559, 0.3333333333333333703, 0.3219752754296894559, 0.3333333333333333703, 0.3219752754296894559, 0.3333333333333333703, 0.3219752754296894559, 0.3333333333333333703, 0.3219752754296894559, 0.3333333333333333703, 0.3219752754296894559, 0.3333333333333333703, 0.3219752754296894559, 0.3333333333333333703, 0.3219752754296894559, 0.3333333333333333703, 0.3219752754296894559, 0.3333333333333333703, 0.3219752754296894559, 0.3333333333333333703),
 ( 0.3333333333333333703, 0.3219752754296894559, 0.3333333333333333703, 0.3219752754296894559, 0.3333333333333333703, 0.3219752754296894559, 0.3333333333333333703, 0.3219752754296894559, 0.3333333333333333703, 0.3219752754296894559, 0.3333333333333333703, 0.3219752754296894559, 0.3333333333333333703, 0.3219752754296894559, 0.3333333333333333703, 0.3219752754296894559, 0.3333333333333333703, 0.3219752754296894559, 0.3333333333333333703, 0.3219752754296894559, 0.3333333333333333703, 0.3219752754296894559, 0.3333333333333333703, 0.3219752754296894559, 0.3333333333333333703, 0.3219752754296894559, 0.3333333333333333703, 0.3219752754296894559, 0.3333333333333333703, 0.3219752754296894559, 0.3333333333333333703, 0.3219752754296894559, 0.3333333333333333703, 0.3219752754296894559, 0.3333333333333333703, 0.3219752754296894559, 0.3333333333333333703, 0.3219752754296894559, 0.3333333333333333703, 0.3219752754296894559, 0.3333333333333333703, 0.3219752754296894559, 0.3333333333333333703, 0.3219752754296894559, 0.3333333333333333703, 0.3219752754296894559, 0.3333333333333333703, 0.3219752754296894559, 0.3333333333333333703, 0.3219752754296894559, 0.3333333333333333703, 0.3219752754296894559, 0.3333333333333333703, 0.3219752754296894559, 0.3333333333333333703, 0.3219752754296894559, 0.3333333333333333703, 0.3219752754296894559, 0.3333333333333333703, 0.3219752754296894559, 0.3333333333333333703, 0.3219752754296894559, 0.3333333333333333703, 0.3219752754296894559, 0.3333333333333333703, 0.3219752754296894559, 0.3333333333333333703, 0.3219752754296894559, 0.3333333333333333703, 0.3219752754296894559, 0.3333333333333333703, 0.3219752754296894559, 0.3333333333333333703, 0.3219752754296894559, 0.3333333333333333703, 0.3219752754296894559, 0.3333333333333333703, 0.3219752754296894559, 0.3333333333333333703, 0.3219752754296894559, 0.3333333333333333703, 0.3219752754296894559, 0.3333333333333333703, 0.3219752754296894559, 0.3333333333333333703, 0.3219752754296894559, 0.3333333333333333703, 0.3219752754296894559, 0.3333333333333333703, 0.3219752754296894559, 0.3333333333333333703, 0.3219752754296894559, 0.3333333333333333703, 0.3219752754296894559, 0.3333333333333333703, 0.3219752754296894559, 0.3333333333333333703, 0.3219752754296894559, 0.3333333333333333703, 0.3219752754296894559, 0.3333333333333333703, 0.3219752754296894559, 0.3333333333333333703, 0.3219752754296894559, 0.3333333333333333703, 0.3219752754296894559, 0.3333333333333333703, 0.3219752754296894559, 0.3333333333333333703, 0.3219752754296894559, 0.3333333333333333703, 0.3219752754296894559, 0.3333333333333333703, 0.3219752754296894559, 0.3333333333333333703, 0.3219752754296894559, 0.3333333333333333703, 0.3219752754296894559, 0.3333333333333333703, 0.3219752754296894559, 0.3333333333333333703, 0.3219752754296894559, 0.3333333333333333703, 0.3219752754296894559, 0.3333333333333333703, 0.3219752754296894559, 0.3333333333333333703, 0.3219752754296894559, 0.3333333333333333703, 0.3219752754296894559, 0.3333333333333333703, 0.3219752754296894559, 0.3333333333333333703, 0.3219752754296894559, 0.3333333333333333703, 0.3219752754296894559, 0.3333333333333333703, 0.3219752754296894559, 0.3333333333333333703, 0.3219752754296894559, 0.3333333333333333703, 0.3219752754296894559, 0.3333333333333333703, 0.3219752754296894559, 0.3333333333333333703, 0.3219752754296894559, 0.3333333333333333703, 0.3219752754296894559, 0.3333333333333333703, 0.3219752754296894559, 0.3333333333333333703, 0.3219752754296894559, 0.3333333333333333703, 0.3219752754296894559, 0.3333333333333333703, 0.3219752754296894559, 0.3333333333333333703, 0.3219752754296894559, 0.3333333333333333703, 0.3219752754296894559, 0.3333333333333333703, 0.3219752754296894559, 0.3333333333333333703, 0.3219752754296894559, 0.3333333333333333703, 0.3219752754296894559, 0.3333333333333333703, 0.3219752754296894559, 0.3333333333333333703, 0.3219752754296894559, 0.3333333333333333703, 0.3219752754296894559, 0.3333333333333333703, 0.3219752754296894559, 0.3333333333333333703, 0.3219752754296894559, 0.3333333333333333703, 0.3219752754296894559, 0.3333333333333333703, 0.3219752754296894559, 0.3333333333333333703, 0.3219752754296894559, 0.3333333333333333703, 0.3219752754296894559, 0.3333333333333333703, 0.3219752754296894559, 0.3333333333333333703, 0.3219752754296894559, 0.3333333333333333703, 0.3219752754296894559, 0.3333333333333333703, 0.3219752754296894559, 0.3333333333333333703, 0.3219752754296894559, 0.3333333333333333703, 0.3219752754296894559, 0.3333333333333333703, 0.3219752754296894559, 0.3333333333333333703, 0.3219752754296894559, 0.3333333333333333703, 0.3219752754296894559, 0.3333333333333333703, 0.3219752754296894559, 0.3333333333333333703, 0.3219752754296894559, 0.3333333333333333703, 0.3219752754296894559, 0.3333333333333333703, 0.3219752754296894559, 0.3333333333333333703, 0.3219752754296894559, 0.3333333333333333703, 0.3219752754296894559, 0.3333333333333333703, 0.3219752754296894559, 0.3333333333333333703, 0.3219752754296894559, 0.3333333333333333703, 0.3219752754296894559, 0.3333333333333333703, 0.3219752754296894559, 0.3333333333333333703, 0.3219752754296894559, 0.3333333333333333703, 0.3219752754296894559, 0.3333333333333333703, 0.3219752754296894559, 0.3333333333333333703, 0.3219752754296894559, 0.3333333333333333703, 0.3219752754296894559, 0.3333333333333333703, 0.3219752754296894559, 0.3333333333333333703, 0.3219752754296894559, 0.3333333333333333703, 0.3219752754296894559, 0.3333333333333333703, 0.3219752754296894559, 0.3333333333333333703, 0.3219752754296894559, 0.3333333333333333703, 0.3219752754296894559, 0.3333333333333333703, 0.3219752754296894559, 0.3333333333333333703, 0.3219752754296894559, 0.3333333333333333703, 0.3219752754296894559, 0.3333333333333333703, 0.3219752754296894559, 0.3333333333333333703, 0.3219752754296894559, 0.3333333333333333703, 0.3219752754296894559, 0.3333333333333333703, 0.3219752754296894559, 0.3333333333333333703, 0.3219752754296894559, 0.3333333333333333703, 0.3219752754296894559, 0.3333333333333333703, 0.3219752754296894559, 0.3333333333333333703, 0.3219752754296894559, 0.3333333333333333703, 0.3219752754296894559, 0.3333333333333333703, 0.3219752754296894559, 0.3333333333333333703, 0.3219752754296894559, 0.3333333333333333703, 0.3219752754296894559, 0.3333333333333333703, 0.3219752754296894559, 0.3333333333333333703, 0.3219752754296894559, 0.3333333333333333703, 0.3219752754296894559, 0.3333333333333333703, 0.3219752754296894559, 0.3333333333333333703, 0.3219752754296894559, 0.3333333333333333703, 0.3219752754296894559, 0.3333333333333333703, 0.3219752754296894559, 0.3333333333333333703, 0.3219752754296894559, 0.3333333333333333703, 0.3219752754296894559, 0.3333333333333333703, 0.3219752754296894559, 0.3333333333333333703, 0.3219752754296894559, 0.3333333333333333703, 0.3219752754296894559, 0.3333333333333333703, 0.3219752754296894559, 0.3333333333333333703, 0.3219752754296894559, 0.3333333333333333703, 0.3219752754296894559, 0.3333333333333333703, 0.3219752754296894559, 0.3333333333333333703, 0.3219752754296894559, 0.3333333333333333703, 0.3219752754296894559, 0.3333333333333333703, 0.3219752754296894559, 0.3333333333333333703, 0.3219752754296894559, 0.3333333333333333703, 0.3219752754296894559, 0.3333333333333333703, 0.3219752754296894559, 0.3333333333333333703, 0.3219752754296894559, 0.3333333333333333703, 0.3219752754296894559, 0.3333333333333333703, 0.3219752754296894559, 0.3333333333333333703, 0.3219752754296894559, 0.3333333333333333703, 0.3219752754296894559, 0.3333333333333333703, 0.3219752754296894559, 0.3333333333333333703, 0.3219752754296894559, 0.3333333333333333703, 0.3219752754296894559, 0.3333333333333333703, 0.3219752754296894559, 0.3333333333333333703, 0.3219752754296894559, 0.3333333333333333703, 0.3219752754296894559, 0.3333333333333333703, 0.3219752754296894559, 0.3333333333333333703, 0.3219752754296894559, 0.3333333333333333703, 0.3219752754296894559, 0.3333333333333333703, 0.3219752754296894559, 0.3333333333333333703, 0.3219752754296894559, 0.3333333333333333703, 0.3219752754296894559, 0.3333333333333333703, 0.3219752754296894559, 0.3333333333333333703, 0.3219752754296894559, 0.3333333333333333703, 0.3219752754296894559, 0.3333333333333333703, 0.3219752754296894559, 0.3333333333333333703, 0.3219752754296894559, 0.3333333333333333703, 0.3219752754296894559, 0.3333333333333333703, 0.3219752754296894559, 0.3333333333333333703, 0.3219752754296894559, 0.3333333333333333703, 0.3219752754296894559, 0.3333333333333333703, 0.3219752754296894559, 0.3333333333333333703, 0.3219752754296894559, 0.3333333333333333703, 0.3219752754296894559, 0.3333333333333333703, 0.3219752754296894559, 0.3333333333333333703, 0.3219752754296894559, 0.3333333333333333703, 0.3219752754296894559, 0.3333333333333333703, 0.3219752754296894559, 0.3333333333333333703, 0.3219752754296894559, 0.3333333333333333703, 0.3219752754296894559, 0.3333333333333333703, 0.3219752754296894559, 0.3333333333333333703, 0.3219752754296894559, 0.3333333333333333703, 0.3219752754296894559, 0.3333333333333333703, 0.3219752754296894559, 0.3333333333333333703, 0.3219752754296894559, 0.3333333333333333703, 0.3219752754296894559, 0.3333333333333333703, 0.3219752754296894559, 0.3333333333333333703, 0.3219752754296894559, 0.3333333333333333703, 0.3219752754296894559, 0.3333333333333333703, 0.3219752754296894559, 0.3333333333333333703, 0.3219752754296894559, 0.3333333333333333703, 0.3219752754296894559, 0.3333333333333333703, 0.3219752754296894559, 0.3333333333333333703, 0.3219752754296894559, 0.3333333333333333703, 0.3219752754296894559, 0.3333333333333333703, 0.3219752754296894559, 0.3333333333333333703, 0.3219752754296894559, 0.3333333333333333703, 0.3219752754296894559, 0.3333333333333333703, 0.3219752754296894559, 0.3333333333333333703, 0.3219752754296894559, 0.3333333333333333703, 0.3219752754296894559, 0.3333333333333333703, 0.3219752754296894559, 0.3333333333333333703, 0.3219752754296894559, 0.3333333333333333703, 0.3219752754296894559, 0.3333333333333333703, 0.3219752754296894559, 0.3333333333333333703, 0.3219752754296894559, 0.3333333333333333703, 0.3219752754296894559, 0.3333333333333333703, 0.3219752754296894559, 0.3333333333333333703, 0.3219752754296894559, 0.3333333333333333703, 0.3219752754296894559, 0.3333333333333333703, 0.3219752754296894559, 0.3333333333333333703, 0.3219752754296894559, 0.3333333333333333703, 0.3219752754296894559, 0.3333333333333333703, 0.3219752754296894559, 0.3333333333333333703),
 ( 1.000000000000000000, 0.9659258262890683122, 1.000000000000000000, 0.9659258262890683122, 1.000000000000000000, 0.9659258262890683122, 1.000000000000000000, 0.9659258262890683122, 1.000000000000000000, 0.9659258262890683122, 1.000000000000000000, 0.9659258262890683122, 1.000000000000000000, 0.9659258262890683122, 1.000000000000000000, 0.9659258262890683122, 1.000000000000000000, 0.9659258262890683122, 1.000000000000000000, 0.9659258262890683122, 1.000000000000000000, 0.9659258262890683122, 1.000000000000000000, 0.9659258262890683122, 1.000000000000000000, 0.9659258262890683122, 1.000000000000000000, 0.9659258262890683122, 1.000000000000000000, 0.9659258262890683122, 1.000000000000000000, 0.9659258262890683122, 1.000000000000000000, 0.9659258262890683122, 1.000000000000000000, 0.9659258262890683122, 1.000000000000000000, 0.9659258262890683122, 1.000000000000000000, 0.9659258262890683122, 1.000000000000000000, 0.9659258262890683122, 1.000000000000000000, 0.9659258262890683122, 1.000000000000000000, 0.9659258262890683122, 1.000000000000000000, 0.9659258262890683122, 1.000000000000000000, 0.9659258262890683122, 1.000000000000000000, 0.9659258262890683122, 1.000000000000000000, 0.9659258262890683122, 1.000000000000000000, 0.9659258262890683122, 1.000000000000000000, 0.9659258262890683122, 1.000000000000000000, 0.9659258262890683122, 1.000000000000000000, 0.9659258262890683122, 1.000000000000000000, 0.9659258262890683122, 1.000000000000000000, 0.9659258262890683122, 1.000000000000000000, 0.9659258262890683122, 1.000000000000000000, 0.9659258262890683122, 1.000000000000000000, 0.9659258262890683122, 1.000000000000000000, 0.9659258262890683122, 1.000000000000000000, 0.9659258262890683122, 1.000000000000000000, 0.9659258262890683122, 1.000000000000000000, 0.9659258262890683122, 1.000000000000000000, 0.9659258262890683122, 1.000000000000000000, 0.9659258262890683122, 1.000000000000000000, 0.9659258262890683122, 1.000000000000000000, 0.9659258262890683122, 1.000000000000000000, 0.9659258262890683122, 1.000000000000000000, 0.9659258262890683122, 1.000000000000000000, 0.9659258262890683122, 1.000000000000000000, 0.9659258262890683122, 1.000000000000000000, 0.9659258262890683122, 1.000000000000000000, 0.9659258262890683122, 1.000000000000000000, 0.9659258262890683122, 1.000000000000000000, 0.9659258262890683122, 1.000000000000000000, 0.9659258262890683122, 1.000000000000000000, 0.9659258262890683122, 1.000000000000000000, 0.9659258262890683122, 1.000000000000000000, 0.9659258262890683122, 1.000000000000000000, 0.9659258262890683122, 1.000000000000000000, 0.9659258262890683122, 1.000000000000000000, 0.9659258262890683122, 1.000000000000000000, 0.9659258262890683122, 1.000000000000000000, 0.9659258262890683122, 1.000000000000000000, 0.9659258262890683122, 1.000000000000000000, 0.9659258262890683122, 1.000000000000000000, 0.9659258262890683122, 1.000000000000000000, 0.9659258262890683122, 1.000000000000000000, 0.9659258262890683122, 1.000000000000000000, 0.9659258262890683122, 1.000000000000000000, 0.9659258262890683122, 1.000000000000000000, 0.9659258262890683122, 1.000000000000000000, 0.9659258262890683122, 1.000000000000000000, 0.9659258262890683122, 1.000000000000000000, 0.9659258262890683122, 1.000000000000000000, 0.9659258262890683122, 1.000000000000000000, 0.9659258262890683122, 1.000000000000000000, 0.9659258262890683122, 1.000000000000000000, 0.9659258262890683122, 1.000000000000000000, 0.9659258262890683122, 1.000000000000000000, 0.9659258262890683122, 1.000000000000000000, 0.9659258262890683122, 1.000000000000000000, 0.9659258262890683122, 1.000000000000000000, 0.9659258262890683122, 1.000000000000000000, 0.9659258262890683122, 1.000000000000000000, 0.9659258262890683122, 1.000000000000000000, 0.9659258262890683122, 1.000000000000000000, 0.9659258262890683122, 1.000000000000000000, 0.9659258262890683122, 1.000000000000000000, 0.9659258262890683122, 1.000000000000000000, 0.9659258262890683122, 1.000000000000000000, 0.9659258262890683122, 1.000000000000000000, 0.9659258262890683122, 1.000000000000000000, 0.9659258262890683122, 1.000000000000000000, 0.9659258262890683122, 1.000000000000000000, 0.9659258262890683122, 1.000000000000000000, 0.9659258262890683122, 1.000000000000000000, 0.9659258262890683122, 1.000000000000000000, 0.9659258262890683122, 1.000000000000000000, 0.9659258262890683122, 1.000000000000000000, 0.9659258262890683122, 1.000000000000000000, 0.9659258262890683122, 1.000000000000000000, 0.9659258262890683122, 1.000000000000000000, 0.9659258262890683122, 1.000000000000000000, 0.9659258262890683122, 1.000000000000000000, 0.9659258262890683122, 1.000000000000000000, 0.9659258262890683122, 1.000000000000000000, 0.9659258262890683122, 1.000000000000000000, 0.9659258262890683122, 1.000000000000000000, 0.9659258262890683122, 1.000000000000000000, 0.9659258262890683122, 1.000000000000000000, 0.9659258262890683122, 1.000000000000000000, 0.9659258262890683122, 1.000000000000000000, 0.9659258262890683122, 1.000000000000000000, 0.9659258262890683122, 1.000000000000000000, 0.9659258262890683122, 1.000000000000000000, 0.9659258262890683122, 1.000000000000000000, 0.9659258262890683122, 1.000000000000000000, 0.9659258262890683122, 1.000000000000000000, 0.9659258262890683122, 1.000000000000000000, 0.9659258262890683122, 1.000000000000000000, 0.9659258262890683122, 1.000000000000000000, 0.9659258262890683122, 1.000000000000000000, 0.9659258262890683122, 1.000000000000000000, 0.9659258262890683122, 1.000000000000000000, 0.9659258262890683122, 1.000000000000000000, 0.9659258262890683122, 1.000000000000000000, 0.9659258262890683122, 1.000000000000000000, 0.9659258262890683122, 1.000000000000000000, 0.9659258262890683122, 1.000000000000000000, 0.9659258262890683122, 1.000000000000000000, 0.9659258262890683122, 1.000000000000000000, 0.9659258262890683122, 1.000000000000000000, 0.9659258262890683122, 1.000000000000000000, 0.9659258262890683122, 1.000000000000000000, 0.9659258262890683122, 1.000000000000000000, 0.9659258262890683122, 1.000000000000000000, 0.9659258262890683122, 1.000000000000000000, 0.9659258262890683122, 1.000000000000000000, 0.9659258262890683122, 1.000000000000000000, 0.9659258262890683122, 1.000000000000000000, 0.9659258262890683122, 1.000000000000000000, 0.9659258262890683122, 1.000000000000000000, 0.9659258262890683122, 1.000000000000000000, 0.9659258262890683122, 1.000000000000000000, 0.9659258262890683122, 1.000000000000000000, 0.9659258262890683122, 1.000000000000000000, 0.9659258262890683122, 1.000000000000000000, 0.9659258262890683122, 1.000000000000000000, 0.9659258262890683122, 1.000000000000000000, 0.9659258262890683122, 1.000000000000000000, 0.9659258262890683122, 1.000000000000000000, 0.9659258262890683122, 1.000000000000000000, 0.9659258262890683122, 1.000000000000000000, 0.9659258262890683122, 1.000000000000000000, 0.9659258262890683122, 1.000000000000000000, 0.9659258262890683122, 1.000000000000000000, 0.9659258262890683122, 1.000000000000000000, 0.9659258262890683122, 1.000000000000000000, 0.9659258262890683122, 1.000000000000000000, 0.9659258262890683122, 1.000000000000000000, 0.9659258262890683122, 1.000000000000000000, 0.9659258262890683122, 1.000000000000000000, 0.9659258262890683122, 1.000000000000000000, 0.9659258262890683122, 1.000000000000000000, 0.9659258262890683122, 1.000000000000000000, 0.9659258262890683122, 1.000000000000000000, 0.9659258262890683122, 1.000000000000000000, 0.9659258262890683122, 1.000000000000000000, 0.9659258262890683122, 1.000000000000000000, 0.9659258262890683122, 1.000000000000000000, 0.9659258262890683122, 1.000000000000000000, 0.9659258262890683122, 1.000000000000000000, 0.9659258262890683122, 1.000000000000000000, 0.9659258262890683122, 1.000000000000000000, 0.9659258262890683122, 1.000000000000000000, 0.9659258262890683122, 1.000000000000000000, 0.9659258262890683122, 1.000000000000000000, 0.9659258262890683122, 1.000000000000000000, 0.9659258262890683122, 1.000000000000000000, 0.9659258262890683122, 1.000000000000000000, 0.9659258262890683122, 1.000000000000000000, 0.9659258262890683122, 1.000000000000000000, 0.9659258262890683122, 1.000000000000000000, 0.9659258262890683122, 1.000000000000000000, 0.9659258262890683122, 1.000000000000000000, 0.9659258262890683122, 1.000000000000000000, 0.9659258262890683122, 1.000000000000000000, 0.9659258262890683122, 1.000000000000000000, 0.9659258262890683122, 1.000000000000000000, 0.9659258262890683122, 1.000000000000000000, 0.9659258262890683122, 1.000000000000000000, 0.9659258262890683122, 1.000000000000000000, 0.9659258262890683122, 1.000000000000000000, 0.9659258262890683122, 1.000000000000000000, 0.9659258262890683122, 1.000000000000000000, 0.9659258262890683122, 1.000000000000000000, 0.9659258262890683122, 1.000000000000000000, 0.9659258262890683122, 1.000000000000000000, 0.9659258262890683122, 1.000000000000000000, 0.9659258262890683122, 1.000000000000000000, 0.9659258262890683122, 1.000000000000000000, 0.9659258262890683122, 1.000000000000000000, 0.9659258262890683122, 1.000000000000000000, 0.9659258262890683122, 1.000000000000000000, 0.9659258262890683122, 1.000000000000000000, 0.9659258262890683122, 1.000000000000000000, 0.9659258262890683122, 1.000000000000000000, 0.9659258262890683122, 1.000000000000000000, 0.9659258262890683122, 1.000000000000000000, 0.9659258262890683122, 1.000000000000000000, 0.9659258262890683122, 1.000000000000000000, 0.9659258262890683122, 1.000000000000000000, 0.9659258262890683122, 1.000000000000000000, 0.9659258262890683122, 1.000000000000000000, 0.9659258262890683122, 1.000000000000000000, 0.9659258262890683122, 1.000000000000000000, 0.9659258262890683122, 1.000000000000000000, 0.9659258262890683122, 1.000000000000000000, 0.9659258262890683122, 1.000000000000000000, 0.9659258262890683122, 1.000000000000000000, 0.9659258262890683122, 1.000000000000000000, 0.9659258262890683122, 1.000000000000000000, 0.9659258262890683122, 1.000000000000000000, 0.9659258262890683122, 1.000000000000000000, 0.9659258262890683122, 1.000000000000000000, 0.9659258262890683122, 1.000000000000000000, 0.9659258262890683122, 1.000000000000000000, 0.9659258262890683122, 1.000000000000000000, 0.9659258262890683122, 1.000000000000000000, 0.9659258262890683122, 1.000000000000000000) ) ) 
 REPRESENTATION_ITEM ( '' )  SURFACE ( )  );
#88900=CARTESIAN_POINT ( 'NONE',  ( -19.02544592524342804, 5.153800228976336051, 86.04057627198103830 ) ) ;
#88901=CARTESIAN_POINT ( 'NONE',  ( 0.05219959533909260263, 19.03943276465977164, 79.99890960531436690 ) ) ;
#88902=CARTESIAN_POINT ( 'NONE',  ( -14.29746914071049879, 8.314922557960819915, 105.8322429386476955 ) ) ;
#88904=CARTESIAN_POINT ( 'NONE',  ( 8.224510206698953496, -14.34966873604960469, 32.91557627198102409 ) ) ;
#88905=CARTESIAN_POINT ( 'NONE',  ( 4.483927247898790824, -16.52544592524335698, 45.20942372801901854 ) ) ;
#88906=CARTESIAN_POINT ( 'NONE',  ( -0.05219959533937732626, 21.53943276465977519, 107.5010903946856899 ) ) ;
#88907=CARTESIAN_POINT ( 'NONE',  ( -5.153800228976328057, -19.02544592524343514, 97.29057627198099567 ) ) ;
#88908=CARTESIAN_POINT ( 'NONE',  ( 21.52544592524334988, 5.823673210054432836, 36.45942372801901143 ) ) ;
#88909=CARTESIAN_POINT ( 'NONE',  ( 19.02544592524343514, -5.153800228976328945, 43.54057627198103120 ) ) ;
#88910=CARTESIAN_POINT ( 'NONE',  ( 0.05219959533934541429, -16.53943276465976808, 50.00109039468568994 ) ) ;
#88911=CARTESIAN_POINT ( 'NONE',  ( 4.379528057220092307, 16.55341960407617563, 82.29275706135234714 ) ) ;
#88912=CARTESIAN_POINT ( 'NONE',  ( 19.02544592524334988, 5.153800228976608722, 106.4594237280190185 ) ) ;
#88913=CARTESIAN_POINT ( 'NONE',  ( -19.05341960407611168, -5.049401038298163336, 31.45724293864769550 ) ) ;
#88914=CARTESIAN_POINT ( 'NONE',  ( -12.06949235617756955, 12.14591786802309770, 95.62390960531436690 ) ) ;
#88915=CARTESIAN_POINT ( 'NONE',  ( -5.823673210054116645, -21.52544592524344225, 97.29057627198105251 ) ) ;
#88916=CARTESIAN_POINT ( 'NONE',  ( -0.05219959533936034679, 19.03943276465977164, 82.50109039468567573 ) ) ;
#88917=CARTESIAN_POINT ( 'NONE',  ( 9.564922557960805705, 16.46253265017160317, 29.58224293864769550 ) ) ;
#88918=CARTESIAN_POINT ( 'NONE',  ( 19.03943276465977164, -0.05219959533909143690, 88.74890960531436690 ) ) ;
#88919=CARTESIAN_POINT ( 'NONE',  ( -10.81492255796105439, 18.62759615963255655, 32.91775706135234714 ) ) ;
#88921=CARTESIAN_POINT ( 'NONE',  ( 9.564922557960805705, 16.46253265017160317, 94.58224293864769550 ) ) ;
#88923=CARTESIAN_POINT ( 'NONE',  ( 19.03943276465977164, -0.05219959533909143690, 88.74890960531436690 ) ) ;
#88924=CARTESIAN_POINT ( 'NONE',  ( -15.72974639402176322, -15.80617190586768395, 34.37609039468568284 ) ) ;
#88925=CARTESIAN_POINT ( 'NONE',  ( 4.379528057220339221, -16.55341960407611168, 92.70724293864770971 ) ) ;
#88926=CARTESIAN_POINT ( 'NONE',  ( -13.97604488694527625, -13.89961937509977652, 101.8739096053143811 ) ) ;
#88927=CARTESIAN_POINT ( 'NONE',  ( 19.02544592524334988, 5.153800228976608722, 21.45942372801899012 ) ) ;
#88928=CARTESIAN_POINT ( 'NONE',  ( -14.29746914071037622, -8.314922557961029526, 54.16775706135235424 ) ) ;
#88929=CARTESIAN_POINT ( 'NONE',  ( -15.72974639402176322, -15.80617190586768395, 84.37609039468570415 ) ) ;
#88930=CARTESIAN_POINT ( 'NONE',  ( -14.29746914071037622, -8.314922557961029526, 44.16775706135234714 ) ) ;
#88931=CARTESIAN_POINT ( 'NONE',  ( 5.153800228976335163, 19.02544592524342804, 69.79057627198103830 ) ) ;
#88932=CARTESIAN_POINT ( 'NONE',  ( -16.51473224551082808, 9.474510206698731452, 93.33442372801900433 ) ) ;
#88933=CARTESIAN_POINT ( 'NONE',  ( 12.14591786802327356, -12.06949235617739191, 70.62609039468567573 ) ) ;
#88934=CARTESIAN_POINT ( 'NONE',  ( -18.67979575497193778, 10.72451020669871902, 108.3344237280190185 ) ) ;
#88936=CARTESIAN_POINT ( 'NONE',  ( 9.564922557961047289, -16.46253265017146816, 85.41775706135233293 ) ) ;
#88937=CARTESIAN_POINT ( 'NONE',  ( 13.89961937509977652, -13.97604488694527269, 63.12390960531435979 ) ) ;
#88938=CARTESIAN_POINT ( 'NONE',  ( -21.55341960407610458, -5.719274019375992779, 86.45724293864770971 ) ) ;
#88939=CARTESIAN_POINT ( 'NONE',  ( 4.379528057220339221, -16.55341960407611168, 82.70724293864770971 ) ) ;
#88940=CARTESIAN_POINT ( 'NONE',  ( -19.02544592524334988, -5.153800228976617603, 83.95942372801901854 ) ) ;
#88942=CARTESIAN_POINT ( 'NONE',  ( 5.049401038297881783, 19.05341960407617563, 52.29275706135234003 ) ) ;
#88943=CARTESIAN_POINT ( 'NONE',  ( 14.29746914071037800, 8.314922557961029526, 111.6677570613523613 ) ) ;
#88944=CARTESIAN_POINT ( 'NONE',  ( -8.224510206698948167, 14.34966873604960824, 80.41557627198103830 ) ) ;
#88945=CARTESIAN_POINT ( 'NONE',  ( -0.05219959533936034679, 19.03943276465977164, 22.50109039468566152 ) ) ;
#88946=CARTESIAN_POINT ( 'NONE',  ( -16.29526858892907271, 7.335722546920045772, 39.20329402199734403 ) ) ;
#88947=CARTESIAN_POINT ( 'NONE',  ( 21.55341960407610458, 5.719274019375980345, 103.9572429386476813 ) ) ;
#88948=CARTESIAN_POINT ( 'NONE',  ( -16.51473224551069308, -9.474510206698971260, 106.6655762719810383 ) ) ;
#88949=CARTESIAN_POINT ( 'NONE',  ( 9.564922557960805705, 16.46253265017160317, 84.58224293864769550 ) ) ;
#88950=CARTESIAN_POINT ( 'NONE',  ( 21.55341960407619695, -5.719274019375665929, 86.04275706135236135 ) ) ;
#88951=CARTESIAN_POINT ( 'NONE',  ( 13.97604488694527802, 13.89961937509977652, 59.37390960531434558 ) ) ;
#88952=CARTESIAN_POINT ( 'NONE',  ( -16.46253265017160317, 9.564922557960807481, 40.83224293864769550 ) ) ;
#88953=CARTESIAN_POINT ( 'NONE',  ( -18.62759615963270932, 10.81492255796079327, 25.83224293864769194 ) ) ;
#88955=CARTESIAN_POINT ( 'NONE',  ( -0.05219959533910754901, -16.53943276465976808, 77.49890960531433848 ) ) ;
#88956=CARTESIAN_POINT ( 'NONE',  ( -9.564922557960796823, -16.46253265017161027, 47.08224293864769550 ) ) ;
#88957=CARTESIAN_POINT ( 'NONE',  ( 16.53943276465976808, -0.05219959533910856209, 98.74890960531438111 ) ) ;
#88958=CARTESIAN_POINT ( 'NONE',  ( -10.72451020669898014, 18.67979575497178502, 115.4155762719810241 ) ) ;
#88959=CARTESIAN_POINT ( 'NONE',  ( 5.823673210054444382, -21.52544592524334988, 50.20942372801901854 ) ) ;
#88960=CARTESIAN_POINT ( 'NONE',  ( 5.153800228976335163, 19.02544592524342804, 24.79057627198102765 ) ) ;
#88961=CARTESIAN_POINT ( 'NONE',  ( 16.53943276465976808, 0.05219959533934440121, 66.25109039468567573 ) ) ;
#88962=CARTESIAN_POINT ( 'NONE',  ( -18.62759615963270932, 10.81492255796079327, 100.8322429386477097 ) ) ;
#88963=CARTESIAN_POINT ( 'NONE',  ( 18.67979575497178502, 10.72451020669898547, 104.1655762719810241 ) ) ;
#88964=CARTESIAN_POINT ( 'NONE',  ( -19.05341960407617563, 5.049401038297882671, 43.54275706135232582 ) ) ;
#88965=CARTESIAN_POINT ( 'NONE',  ( -13.97604488694527625, -13.89961937509977652, 46.87390960531435979 ) ) ;
#88966=CARTESIAN_POINT ( 'NONE',  ( 13.97604488694527802, 13.89961937509977652, 114.3739096053143669 ) ) ;
#88967=CARTESIAN_POINT ( 'NONE',  ( 18.62759615963255655, 10.81492255796105972, 61.66775706135235424 ) ) ;
#88968=CARTESIAN_POINT ( 'NONE',  ( -21.55341960407610458, -5.719274019375992779, 56.45724293864768839 ) ) ;
#88969=CARTESIAN_POINT ( 'NONE',  ( 4.483927247898545687, 16.52544592524342804, 39.79057627198103830 ) ) ;
#88970=CARTESIAN_POINT ( 'NONE',  ( 18.67979575497194134, -10.72451020669871369, 75.83442372801900433 ) ) ;
#88971=CARTESIAN_POINT ( 'NONE',  ( -15.80617190586768217, 15.72974639402176855, 113.1260903946856899 ) ) ;
#88972=CARTESIAN_POINT ( 'NONE',  ( -5.049401038297874678, -19.05341960407617918, 44.79275706135232582 ) ) ;
#88973=CARTESIAN_POINT ( 'NONE',  ( 16.53943276465976808, 0.05219959533934440121, 101.2510903946856757 ) ) ;
#88974=CARTESIAN_POINT ( 'NONE',  ( 15.72974639402176855, 15.80617190586768217, 56.87609039468568994 ) ) ;
#88975=CARTESIAN_POINT ( 'NONE',  ( -19.05341960407611168, -5.049401038298163336, 56.45724293864768129 ) ) ;
#88976=CARTESIAN_POINT ( 'NONE',  ( -0.05219959533936034679, 19.03943276465977164, 37.50109039468567573 ) ) ;
#88977=CARTESIAN_POINT ( 'NONE',  ( 5.823673210054125526, 21.52544592524343514, 39.79057627198103830 ) ) ;
#88978=CARTESIAN_POINT ( 'NONE',  ( 0.05219959533937995610, -21.53943276465977519, 30.00109039468568284 ) ) ;
#88979=CARTESIAN_POINT ( 'NONE',  ( 21.55341960407610458, 5.719274019375980345, 88.95724293864769550 ) ) ;
#88980=CARTESIAN_POINT ( 'NONE',  ( -19.05341960407617563, 5.049401038297882671, 88.54275706135230450 ) ) ;
#88981=CARTESIAN_POINT ( 'NONE',  ( 16.53943276465976808, 0.05219959533934440121, 51.25109039468568994 ) ) ;
#88983=CARTESIAN_POINT ( 'NONE',  ( -10.81492255796078084, -18.62759615963271287, 92.08224293864769550 ) ) ;
#88984=CARTESIAN_POINT ( 'NONE',  ( -16.52544592524335698, -4.483927247898792601, 73.95942372801901854 ) ) ;
#88985=CARTESIAN_POINT ( 'NONE',  ( -8.314922557960811034, -14.29746914071050412, 82.08224293864768129 ) ) ;
#88987=CARTESIAN_POINT ( 'NONE',  ( 0.05219959533936267826, -19.03943276465977164, 100.0010903946856757 ) ) ;
#88988=CARTESIAN_POINT ( 'NONE',  ( -18.62759615963270932, 10.81492255796079327, 30.83224293864770260 ) ) ;
#88989=DIRECTION ( 'NONE',  ( 1.000000000000000000, -0.000000000000000000, -0.000000000000000000 ) ) ;
#88990=CARTESIAN_POINT ( 'NONE',  ( 4.483927247898790824, -16.52544592524335698, 55.20942372801902565 ) ) ;
#88991=CARTESIAN_POINT ( 'NONE',  ( -10.81492255796105439, 18.62759615963255655, 32.91775706135234714 ) ) ;
#88992=CARTESIAN_POINT ( 'NONE',  ( -5.719274019375978568, 21.55341960407610458, 50.20724293864769550 ) ) ;
#88993=CARTESIAN_POINT ( 'NONE',  ( 4.483927247898790824, -16.52544592524335698, 70.20942372801904696 ) ) ;
#88994=CARTESIAN_POINT ( 'NONE',  ( 5.153800228976335163, 19.02544592524342804, 79.79057627198102409 ) ) ;
#88995=CARTESIAN_POINT ( 'NONE',  ( 21.53943276465977519, 0.05219959533937863772, 61.25109039468567573 ) ) ;
#88996=CARTESIAN_POINT ( 'NONE',  ( -16.46253265017160317, 9.564922557960807481, 25.83224293864769194 ) ) ;
#88997=CARTESIAN_POINT ( 'NONE',  ( 18.62759615963271287, -10.81492255796078972, 23.33224293864769194 ) ) ;
#88999=CARTESIAN_POINT ( 'NONE',  ( -5.049401038297874678, -19.05341960407617918, 39.79275706135232582 ) ) ;
#89000=CARTESIAN_POINT ( 'NONE',  ( 4.379528057220092307, 16.55341960407617563, 57.29275706135234714 ) ) ;
#89001=CARTESIAN_POINT ( 'NONE',  ( -5.049401038298153566, 19.05341960407611168, 115.2072429386477097 ) ) ;
#89003=CARTESIAN_POINT ( 'NONE',  ( 13.97604488694527802, 13.89961937509977652, 89.37390960531436690 ) ) ;
#89004=CARTESIAN_POINT ( 'NONE',  ( 12.06949235617739724, 12.14591786802326823, 96.87609039468568994 ) ) ;
#89006=CARTESIAN_POINT ( 'NONE',  ( -16.53943276465976808, 0.05219959533911058130, 101.2489096053143669 ) ) ;
#89007=CARTESIAN_POINT ( 'NONE',  ( 10.72451020669898902, -18.67979575497178502, 32.91557627198102409 ) ) ;
#89008=CARTESIAN_POINT ( 'NONE',  ( -5.153800228976328057, -19.02544592524343514, 37.29057627198102409 ) ) ;
#89009=CARTESIAN_POINT ( 'NONE',  ( 14.29746914071037800, 8.314922557961029526, 76.66775706135234714 ) ) ;
#89010=CARTESIAN_POINT ( 'NONE',  ( 0.05219959533937995610, -21.53943276465977519, 20.00109039468568639 ) ) ;
#89011=CARTESIAN_POINT ( 'NONE',  ( -9.564922557961040184, 16.46253265017147172, 82.91775706135233293 ) ) ;
#89012=CARTESIAN_POINT ( 'NONE',  ( -19.02544592524342804, 5.153800228976336051, 46.04057627198101699 ) ) ;
#89015=CARTESIAN_POINT ( 'NONE',  ( 10.72451020669871369, 18.67979575497193778, 107.0844237280190043 ) ) ;
#89016=CARTESIAN_POINT ( 'NONE',  ( 13.97604488694527802, 13.89961937509977652, 59.37390960531434558 ) ) ;
#89017=CARTESIAN_POINT ( 'NONE',  ( 12.14591786802327356, -12.06949235617739191, 45.62609039468567573 ) ) ;
#89018=CARTESIAN_POINT ( 'NONE',  ( 0.05219959533937995610, -21.53943276465977519, 95.00109039468568994 ) ) ;
#89019=CARTESIAN_POINT ( 'NONE',  ( -19.05341960407617563, 5.049401038297882671, 43.54275706135232582 ) ) ;
#89020=CARTESIAN_POINT ( 'NONE',  ( 9.474510206698729675, 16.51473224551082808, 47.08442372801900433 ) ) ;
#89022=CARTESIAN_POINT ( 'NONE',  ( -10.72451020669870658, -18.67979575497194134, 44.58442372801901854 ) ) ;
#89023=CARTESIAN_POINT ( 'NONE',  ( -13.89961937509977652, 13.97604488694528158, 25.62390960531434558 ) ) ;
#89024=CARTESIAN_POINT ( 'NONE',  ( 9.564922557961047289, -16.46253265017146816, 45.41775706135232582 ) ) ;
#89025=CARTESIAN_POINT ( 'NONE',  ( 5.049401038298161559, -19.05341960407611168, 102.7072429386476955 ) ) ;
#89026=CARTESIAN_POINT ( 'NONE',  ( 9.564922557960805705, 16.46253265017160317, 79.58224293864769550 ) ) ;
#89027=CARTESIAN_POINT ( 'NONE',  ( 12.06949235617757843, -12.14591786802309237, 38.12390960531436690 ) ) ;
#89028=CARTESIAN_POINT ( 'NONE',  ( -0.05219959533907301413, -21.53943276465977519, 32.49890960531435979 ) ) ;
#89030=DIRECTION ( 'NONE',  ( 0.000000000000000000, 0.000000000000000000, 1.000000000000000000 ) ) ;
#89031=CARTESIAN_POINT ( 'NONE',  ( 5.823673210054444382, -21.52544592524334988, 95.20942372801903275 ) ) ;
#89033=CARTESIAN_POINT ( 'NONE',  ( 5.049401038298161559, -19.05341960407611168, 37.70724293864768839 ) ) ;
#89034=CARTESIAN_POINT ( 'NONE',  ( -16.46253265017160317, 9.564922557960807481, 110.8322429386476955 ) ) ;
#89035=EDGE_CURVE ( 'NONE', #86900, #128850, #146580, .T. ) ;
#89037=CARTESIAN_POINT ( 'NONE',  ( -14.29746914071037622, -8.314922557961029526, 64.16775706135234714 ) ) ;
#89038=CARTESIAN_POINT ( 'NONE',  ( 15.72974639402199770, -15.80617190586745480, 83.12390960531436690 ) ) ;
#89039=CARTESIAN_POINT ( 'NONE',  ( 8.224510206698953496, -14.34966873604960469, 37.91557627198102409 ) ) ;
#89040=CARTESIAN_POINT ( 'NONE',  ( 19.05341960407611168, 5.049401038298154454, 33.95724293864769550 ) ) ;
#89041=CARTESIAN_POINT ( 'NONE',  ( 19.05341960407611168, 5.049401038298154454, 113.9572429386477097 ) ) ;
#89042=CARTESIAN_POINT ( 'NONE',  ( -0.05219959533937732626, 21.53943276465977519, 32.50109039468568284 ) ) ;
#89043=CARTESIAN_POINT ( 'NONE',  ( 5.153800228976615827, -19.02544592524334988, 40.20942372801898301 ) ) ;
#89044=CARTESIAN_POINT ( 'NONE',  ( 16.46253265017160672, -9.564922557960803928, 38.33224293864768839 ) ) ;
#89045=CARTESIAN_POINT ( 'NONE',  ( 0.05219959533937995610, -21.53943276465977519, 85.00109039468568994 ) ) ;
#89046=CARTESIAN_POINT ( 'NONE',  ( 17.50000000000000000, -5.500000000000000888, 33.29690382534174375 ) ) ;
#89047=CARTESIAN_POINT ( 'NONE',  ( 8.224510206698953496, -14.34966873604960469, 22.91557627198102765 ) ) ;
#89049=CARTESIAN_POINT ( 'NONE',  ( 15.80617190586746368, 15.72974639402197994, 24.37390960531435979 ) ) ;
#89050=CARTESIAN_POINT ( 'NONE',  ( 14.29746914071049879, -8.314922557960816363, 98.33224293864769550 ) ) ;
#89052=CARTESIAN_POINT ( 'NONE',  ( 17.50000000000000000, 5.499999999999995559, 108.7823096230356867 ) ) ;
#89053=CARTESIAN_POINT ( 'NONE',  ( 0.05219959533909260263, 19.03943276465977164, 89.99890960531436690 ) ) ;
#89054=CARTESIAN_POINT ( 'NONE',  ( -4.483927247898539470, -16.52544592524342804, 77.29057627198102409 ) ) ;
#89055=CARTESIAN_POINT ( 'NONE',  ( -16.46253265017146816, -9.564922557961047289, 109.1677570613523471 ) ) ;
#89056=CARTESIAN_POINT ( 'NONE',  ( 10.72451020669898902, -18.67979575497178502, 62.91557627198102409 ) ) ;
#89058=CARTESIAN_POINT ( 'NONE',  ( -9.474510206698964154, 16.51473224551069663, 30.41557627198102054 ) ) ;
#89059=CARTESIAN_POINT ( 'NONE',  ( -19.02544592524342804, 5.153800228976336051, 81.04057627198103830 ) ) ;
#89060=CARTESIAN_POINT ( 'NONE',  ( 18.67979575497178502, 10.72451020669898547, 89.16557627198102409 ) ) ;
#89061=CARTESIAN_POINT ( 'NONE',  ( -8.224510206698735004, -14.34966873604973081, 99.58442372801900433 ) ) ;
#89062=CARTESIAN_POINT ( 'NONE',  ( -16.51473224551069308, -9.474510206698971260, 86.66557627198102409 ) ) ;
#89063=CARTESIAN_POINT ( 'NONE',  ( 13.97604488694548053, -13.89961937509957401, 85.62609039468568994 ) ) ;
#89064=CARTESIAN_POINT ( 'NONE',  ( 21.52544592524334988, 5.823673210054432836, 91.45942372801901854 ) ) ;
#89065=CARTESIAN_POINT ( 'NONE',  ( -15.72974639402197994, 15.80617190586746368, 75.62390960531439532 ) ) ;
#89066=CARTESIAN_POINT ( 'NONE',  ( -21.52544592524343514, 5.823673210054127303, 31.04057627198102409 ) ) ;
#89067=CARTESIAN_POINT ( 'NONE',  ( -0.05219959533909027116, -19.03943276465977164, 47.49890960531435979 ) ) ;
#89068=CARTESIAN_POINT ( 'NONE',  ( -16.53943276465976808, -0.05219959533934237506, 113.7510903946856757 ) ) ;
#89069=CARTESIAN_POINT ( 'NONE',  ( 19.03943276465977164, -0.05219959533909143690, 63.74890960531435979 ) ) ;
#89071=CARTESIAN_POINT ( 'NONE',  ( 21.52544592524334988, 5.823673210054432836, 106.4594237280190328 ) ) ;
#89072=CARTESIAN_POINT ( 'NONE',  ( 8.314922557960818139, 14.29746914071049879, 69.58224293864769550 ) ) ;
#89073=CARTESIAN_POINT ( 'NONE',  ( -18.62759615963270932, 10.81492255796079327, 105.8322429386476955 ) ) ;
#89074=CARTESIAN_POINT ( 'NONE',  ( 10.81492255796078972, 18.62759615963270932, 109.5822429386476955 ) ) ;
#89076=CARTESIAN_POINT ( 'NONE',  ( 5.719274019375991003, -21.55341960407610458, 57.70724293864770260 ) ) ;
#89077=CARTESIAN_POINT ( 'NONE',  ( 0.05219959533934541429, -16.53943276465976808, 90.00109039468567573 ) ) ;
#89078=CARTESIAN_POINT ( 'NONE',  ( 16.53943276465976808, -0.05219959533910856209, 103.7489096053143669 ) ) ;
#89079=CARTESIAN_POINT ( 'NONE',  ( -13.89961937509977652, 13.97604488694528158, 55.62390960531434558 ) ) ;
#89081=CARTESIAN_POINT ( 'NONE',  ( 16.55341960407611168, 4.379528057220329451, 28.95724293864769905 ) ) ;
#89082=CARTESIAN_POINT ( 'NONE',  ( -10.81492255796105439, 18.62759615963255655, 42.91775706135235424 ) ) ;
#89083=CARTESIAN_POINT ( 'NONE',  ( 16.51473224551069308, 9.474510206698969483, 104.1655762719810241 ) ) ;
#89084=CARTESIAN_POINT ( 'NONE',  ( 0.05219959533937995610, -21.53943276465977519, 75.00109039468568994 ) ) ;
#89085=CARTESIAN_POINT ( 'NONE',  ( -16.46253265017160317, 9.564922557960807481, 30.83224293864769550 ) ) ;
#89086=CARTESIAN_POINT ( 'NONE',  ( 16.51473224551069308, 9.474510206698969483, 44.16557627198103120 ) ) ;
#89088=CARTESIAN_POINT ( 'NONE',  ( -15.80617190586768217, 15.72974639402176855, 78.12609039468570415 ) ) ;
#89089=CARTESIAN_POINT ( 'NONE',  ( -18.67979575497193778, 10.72451020669871902, 78.33442372801901854 ) ) ;
#89090=CARTESIAN_POINT ( 'NONE',  ( -13.89961937509977652, 13.97604488694528158, 105.6239096053143527 ) ) ;
#89091=CARTESIAN_POINT ( 'NONE',  ( 13.89961937509957401, 13.97604488694547697, 76.87609039468566152 ) ) ;
#89092=CARTESIAN_POINT ( 'NONE',  ( -21.53943276465977519, -0.05219959533937600094, 53.75109039468568994 ) ) ;
#89093=CARTESIAN_POINT ( 'NONE',  ( -4.379528057220086978, -16.55341960407618274, 19.79275706135235069 ) ) ;
#89094=VECTOR ( 'NONE', #107316, 1000.000000000000000 ) ;
#89095=CARTESIAN_POINT ( 'NONE',  ( -16.51473224551082808, 9.474510206698731452, 73.33442372801900433 ) ) ;
#89096=CARTESIAN_POINT ( 'NONE',  ( 5.049401038298161559, -19.05341960407611168, 52.70724293864767418 ) ) ;
#89097=CARTESIAN_POINT ( 'NONE',  ( 19.05341960407617918, -5.049401038297876454, 81.04275706135231871 ) ) ;
#89098=CARTESIAN_POINT ( 'NONE',  ( 14.34966873604960469, 8.224510206698951720, 24.16557627198103120 ) ) ;
#89099=CARTESIAN_POINT ( 'NONE',  ( 5.153800228976615827, -19.02544592524334988, 95.20942372801897591 ) ) ;
#89100=CARTESIAN_POINT ( 'NONE',  ( 12.14591786802309770, 12.06949235617756955, 39.37390960531436690 ) ) ;
#89101=CARTESIAN_POINT ( 'NONE',  ( 16.51473224551083163, -9.474510206698727899, 65.83442372801900433 ) ) ;
#89102=CARTESIAN_POINT ( 'NONE',  ( 14.29746914071037800, 8.314922557961029526, 51.66775706135234714 ) ) ;
#89103=CARTESIAN_POINT ( 'NONE',  ( -9.474510206698720793, -16.51473224551083518, 19.58442372801899722 ) ) ;
#89105=CARTESIAN_POINT ( 'NONE',  ( -19.03943276465977164, 0.05219959533909376836, 41.24890960531435269 ) ) ;
#89106=CARTESIAN_POINT ( 'NONE',  ( 18.56453257813364033, -5.500000000000045297, 73.49000423690687001 ) ) ;
#89107=CARTESIAN_POINT ( 'NONE',  ( 16.52544592524335698, 4.483927247898782831, 51.45942372801901854 ) ) ;
#89110=CARTESIAN_POINT ( 'NONE',  ( -0.05219959533909027116, -19.03943276465977164, 97.49890960531436690 ) ) ;
#89111=DIRECTION ( 'NONE',  ( 0.000000000000000000, 0.000000000000000000, -1.000000000000000000 ) ) ;
#89113=CARTESIAN_POINT ( 'NONE',  ( 13.97604488694548053, -13.89961937509957401, 95.62609039468563310 ) ) ;
#89115=CARTESIAN_POINT ( 'NONE',  ( -10.81492255796078084, -18.62759615963271287, 22.08224293864769194 ) ) ;
#89116=CARTESIAN_POINT ( 'NONE',  ( -0.05219959533937732626, 21.53943276465977519, 107.5010903946856899 ) ) ;
#89117=CARTESIAN_POINT ( 'NONE',  ( -5.153800228976607833, 19.02544592524334988, 112.7094237280190043 ) ) ;
#89118=CARTESIAN_POINT ( 'NONE',  ( 5.049401038298161559, -19.05341960407611168, 22.70724293864769194 ) ) ;
#89119=CARTESIAN_POINT ( 'NONE',  ( -9.564922557960796823, -16.46253265017161027, 32.08224293864769550 ) ) ;
#89120=CARTESIAN_POINT ( 'NONE',  ( -18.62759615963270932, 10.81492255796079327, 55.83224293864770260 ) ) ;
#89121=CARTESIAN_POINT ( 'NONE',  ( 13.97604488694527802, 13.89961937509977652, 39.37390960531435269 ) ) ;
#89123=CARTESIAN_POINT ( 'NONE',  ( -0.05219959533936034679, 19.03943276465977164, 77.50109039468566152 ) ) ;
#89124=CARTESIAN_POINT ( 'NONE',  ( -4.379528057220328563, 16.55341960407611168, 50.20724293864769550 ) ) ;
#89125=CARTESIAN_POINT ( 'NONE',  ( 5.823673210054125526, 21.52544592524343514, 29.79057627198102409 ) ) ;
#89126=CARTESIAN_POINT ( 'NONE',  ( 15.72974639402176855, 15.80617190586768217, 91.87609039468568994 ) ) ;
#89127=CARTESIAN_POINT ( 'NONE',  ( -0.05219959533907301413, -21.53943276465977519, 87.49890960531436690 ) ) ;
#89128=CARTESIAN_POINT ( 'NONE',  ( 5.823673210054444382, -21.52544592524334988, 60.20942372801902565 ) ) ;
#89129=CARTESIAN_POINT ( 'NONE',  ( 5.823673210054444382, -21.52544592524334988, 70.20942372801904696 ) ) ;
#89130=CARTESIAN_POINT ( 'NONE',  ( 9.474510206698971260, -16.51473224551069308, 92.91557627198103830 ) ) ;
#89131=CARTESIAN_POINT ( 'NONE',  ( 4.379528057220092307, 16.55341960407617563, 87.29275706135236135 ) ) ;
#89132=CARTESIAN_POINT ( 'NONE',  ( 5.823673210054444382, -21.52544592524334988, 60.20942372801902565 ) ) ;
#89133=CARTESIAN_POINT ( 'NONE',  ( 13.89961937509977652, -13.97604488694527269, 58.12390960531436690 ) ) ;
#89134=CARTESIAN_POINT ( 'NONE',  ( 13.97604488694527802, 13.89961937509977652, 24.37390960531435624 ) ) ;
#89135=CARTESIAN_POINT ( 'NONE',  ( -16.51473224551069308, -9.474510206698971260, 56.66557627198103120 ) ) ;
#89136=CARTESIAN_POINT ( 'NONE',  ( 14.29746914071049879, -8.314922557960816363, 63.33224293864770260 ) ) ;
#89137=CARTESIAN_POINT ( 'NONE',  ( -12.06949235617756955, 12.14591786802309770, 35.62390960531437401 ) ) ;
#89138=CARTESIAN_POINT ( 'NONE',  ( -10.81492255796078084, -18.62759615963271287, 42.08224293864769550 ) ) ;
#89139=CARTESIAN_POINT ( 'NONE',  ( 13.89961937509977652, -13.97604488694527269, 53.12390960531434558 ) ) ;
#89140=CARTESIAN_POINT ( 'NONE',  ( 10.72451020669898902, -18.67979575497178502, 62.91557627198102409 ) ) ;
#89141=CARTESIAN_POINT ( 'NONE',  ( 5.153800228976615827, -19.02544592524334988, 50.20942372801897591 ) ) ;
#89143=CARTESIAN_POINT ( 'NONE',  ( -16.55341960407611168, -4.379528057220339221, 56.45724293864768839 ) ) ;
#89144=CARTESIAN_POINT ( 'NONE',  ( 5.823673210054125526, 21.52544592524343514, 44.79057627198103120 ) ) ;
#89146=ORIENTED_EDGE ( 'NONE', *, *, #25866, .T. ) ;
#89148=CARTESIAN_POINT ( 'NONE',  ( -8.224510206698735004, -14.34966873604973081, 89.58442372801901854 ) ) ;
#89149=CARTESIAN_POINT ( 'NONE',  ( 19.05341960407617918, -5.049401038297876454, 71.04275706135234714 ) ) ;
#89150=CARTESIAN_POINT ( 'NONE',  ( -16.52544592524342804, 4.483927247898546575, 56.04057627198102409 ) ) ;
#89151=CARTESIAN_POINT ( 'NONE',  ( -19.49190055781009789, -5.500000000000056843, 60.56116087098778422 ) ) ;
#89152=CARTESIAN_POINT ( 'NONE',  ( -4.379528057220328563, 16.55341960407611168, 35.20724293864768839 ) ) ;
#89153=CARTESIAN_POINT ( 'NONE',  ( 13.89961937509977652, -13.97604488694527269, 48.12390960531435979 ) ) ;
#89154=CARTESIAN_POINT ( 'NONE',  ( 19.03943276465977164, -0.05219959533909143690, 68.74890960531436690 ) ) ;
#89155=CARTESIAN_POINT ( 'NONE',  ( -16.46253265017160317, 9.564922557960807481, 40.83224293864769550 ) ) ;
#89156=CARTESIAN_POINT ( 'NONE',  ( 15.72974639402176855, 15.80617190586768217, 51.87609039468568284 ) ) ;
#89157=CARTESIAN_POINT ( 'NONE',  ( 9.474510206698971260, -16.51473224551069308, 77.91557627198103830 ) ) ;
#89158=CARTESIAN_POINT ( 'NONE',  ( -0.05219959533909027116, -19.03943276465977164, 27.49890960531435624 ) ) ;
#89159=CARTESIAN_POINT ( 'NONE',  ( -13.97604488694527625, -13.89961937509977652, 61.87390960531435979 ) ) ;
#89160=CARTESIAN_POINT ( 'NONE',  ( -15.80617190586745835, -15.72974639402198527, 46.87390960531435979 ) ) ;
#89161=CARTESIAN_POINT ( 'NONE',  ( 13.97604488694527802, 13.89961937509977652, 34.37390960531436690 ) ) ;
#89162=CARTESIAN_POINT ( 'NONE',  ( -5.823673210054116645, -21.52544592524344225, 47.29057627198103120 ) ) ;
#89163=CARTESIAN_POINT ( 'NONE',  ( -4.379528057220086978, -16.55341960407618274, 104.7927570613523898 ) ) ;
#89164=CARTESIAN_POINT ( 'NONE',  ( 19.05341960407617918, -5.049401038297876454, 26.04275706135233293 ) ) ;
#89165=CARTESIAN_POINT ( 'NONE',  ( -8.224510206698735004, -14.34966873604973081, 49.58442372801901143 ) ) ;
#89166=CARTESIAN_POINT ( 'NONE',  ( 12.06949235617739724, 12.14591786802326823, 86.87609039468568994 ) ) ;
#89168=CARTESIAN_POINT ( 'NONE',  ( -4.483927247898782831, 16.52544592524335698, 62.70942372801902565 ) ) ;
#89169=CARTESIAN_POINT ( 'NONE',  ( 14.29746914071037800, 8.314922557961029526, 46.66775706135234714 ) ) ;
#89170=CARTESIAN_POINT ( 'NONE',  ( -16.51473224551069308, -9.474510206698971260, 101.6655762719810241 ) ) ;
#89171=CARTESIAN_POINT ( 'NONE',  ( 0.05219959533934541429, -16.53943276465976808, 30.00109039468568284 ) ) ;
#89172=CARTESIAN_POINT ( 'NONE',  ( 13.97604488694527802, 13.89961937509977652, 39.37390960531435269 ) ) ;
#89173=CARTESIAN_POINT ( 'NONE',  ( -18.67979575497193778, 10.72451020669871902, 28.33442372801902209 ) ) ;
#89174=CARTESIAN_POINT ( 'NONE',  ( -12.14591786802326823, 12.06949235617739902, 38.12609039468567573 ) ) ;
#89175=CARTESIAN_POINT ( 'NONE',  ( -16.52544592524335698, -4.483927247898792601, 98.95942372801903275 ) ) ;
#89177=CARTESIAN_POINT ( 'NONE',  ( -18.62759615963255300, -10.81492255796106328, 99.16775706135234714 ) ) ;
#89178=CARTESIAN_POINT ( 'NONE',  ( 16.46253265017146816, 9.564922557961045513, 101.6677570613523329 ) ) ;
#89179=CARTESIAN_POINT ( 'NONE',  ( -4.379528057220328563, 16.55341960407611168, 55.20724293864770260 ) ) ;
#89180=CARTESIAN_POINT ( 'NONE',  ( -13.89961937509977652, 13.97604488694528158, 30.62390960531435269 ) ) ;
#89181=CARTESIAN_POINT ( 'NONE',  ( 5.153800228976615827, -19.02544592524334988, 65.20942372801900433 ) ) ;
#89183=CARTESIAN_POINT ( 'NONE',  ( 5.719274019375673035, 21.55341960407619339, 52.29275706135236135 ) ) ;
#89184=CARTESIAN_POINT ( 'NONE',  ( -4.379528057220086978, -16.55341960407618274, 24.79275706135235779 ) ) ;
#89185=CARTESIAN_POINT ( 'NONE',  ( 17.48853670773247515, 5.747243402303061188, 83.83328700250011423 ) ) ;
#89186=CARTESIAN_POINT ( 'NONE',  ( 18.67979575497178502, 10.72451020669898547, 29.16557627198103120 ) ) ;
#89187=CARTESIAN_POINT ( 'NONE',  ( 5.719274019375991003, -21.55341960407610458, 67.70724293864769550 ) ) ;
#89188=CARTESIAN_POINT ( 'NONE',  ( -14.29746914071037622, -8.314922557961029526, 19.16775706135234714 ) ) ;
#89189=CARTESIAN_POINT ( 'NONE',  ( 13.89961937509977652, -13.97604488694527269, 103.1239096053143527 ) ) ;
#89190=CARTESIAN_POINT ( 'NONE',  ( 5.049401038298161559, -19.05341960407611168, 22.70724293864769194 ) ) ;
#89191=CARTESIAN_POINT ( 'NONE',  ( -21.53943276465977519, -0.05219959533937600094, 113.7510903946856757 ) ) ;
#89192=CARTESIAN_POINT ( 'NONE',  ( 13.97604488694527802, 13.89961937509977652, 44.37390960531435269 ) ) ;
#89194=CARTESIAN_POINT ( 'NONE',  ( -18.62759615963255300, -10.81492255796106328, 49.16775706135234003 ) ) ;
#89195=CARTESIAN_POINT ( 'NONE',  ( 21.55341960407619695, -5.719274019375665929, 91.04275706135236135 ) ) ;
#89196=CARTESIAN_POINT ( 'NONE',  ( 12.06949235617739724, 12.14591786802326823, 101.8760903946857042 ) ) ;
#89197=CARTESIAN_POINT ( 'NONE',  ( -19.05341960407611168, -5.049401038298163336, 76.45724293864769550 ) ) ;
#89198=CARTESIAN_POINT ( 'NONE',  ( 21.52544592524334988, 5.823673210054432836, 46.45942372801901854 ) ) ;
#89199=CARTESIAN_POINT ( 'NONE',  ( 0.05219959533937995610, -21.53943276465977519, 40.00109039468567573 ) ) ;
#89200=CARTESIAN_POINT ( 'NONE',  ( -19.05341960407617563, 5.049401038297882671, 73.54275706135233293 ) ) ;
#89201=CARTESIAN_POINT ( 'NONE',  ( 19.02544592524343514, -5.153800228976328945, 93.54057627198102409 ) ) ;
#89202=CARTESIAN_POINT ( 'NONE',  ( 16.53943276465976808, -0.05219959533910856209, 108.7489096053143669 ) ) ;
#89203=CARTESIAN_POINT ( 'NONE',  ( -10.81492255796078084, -18.62759615963271287, 102.0822429386476955 ) ) ;
#89204=CARTESIAN_POINT ( 'NONE',  ( -16.52544592524342804, 4.483927247898546575, 71.04057627198103830 ) ) ;
#89205=CARTESIAN_POINT ( 'NONE',  ( 21.53943276465977519, 0.05219959533937863772, 111.2510903946856899 ) ) ;
#89206=CARTESIAN_POINT ( 'NONE',  ( -16.53943276465976808, 0.05219959533911058130, 101.2489096053143669 ) ) ;
#89207=CARTESIAN_POINT ( 'NONE',  ( 16.51473224551069308, 9.474510206698969483, 49.16557627198102409 ) ) ;
#89208=CARTESIAN_POINT ( 'NONE',  ( 19.03943276465977164, 0.05219959533936151252, 91.25109039468566152 ) ) ;
#89209=CARTESIAN_POINT ( 'NONE',  ( 14.34966873604960469, 8.224510206698951720, 54.16557627198103120 ) ) ;
#89210=CARTESIAN_POINT ( 'NONE',  ( -21.55341960407619339, 5.719274019375674811, 103.5427570613523613 ) ) ;
#89211=CARTESIAN_POINT ( 'NONE',  ( -19.05341960407611168, -5.049401038298163336, 101.4572429386476955 ) ) ;
#89212=CARTESIAN_POINT ( 'NONE',  ( -16.46253265017146816, -9.564922557961047289, 69.16775706135233293 ) ) ;
#89213=CARTESIAN_POINT ( 'NONE',  ( -21.55341960407610458, -5.719274019375992779, 76.45724293864769550 ) ) ;
#89214=CARTESIAN_POINT ( 'NONE',  ( 18.67979575497194134, -10.72451020669871369, 30.83442372801902209 ) ) ;
#89215=CARTESIAN_POINT ( 'NONE',  ( -12.06949235617739369, -12.14591786802326823, 24.37609039468567573 ) ) ;
#89216=CARTESIAN_POINT ( 'NONE',  ( 8.224510206698742110, 14.34966873604972548, 92.08442372801901854 ) ) ;
#89217=CARTESIAN_POINT ( 'NONE',  ( 17.05587630539785238, 6.762274262135715475, 61.75819690962688924 ) ) ;
#89218=CARTESIAN_POINT ( 'NONE',  ( -5.719274019375665041, -21.55341960407619695, 29.79275706135234358 ) ) ;
#89219=CARTESIAN_POINT ( 'NONE',  ( -4.379528057220328563, 16.55341960407611168, 110.2072429386477239 ) ) ;
#89221=CARTESIAN_POINT ( 'NONE',  ( -4.483927247898782831, 16.52544592524335698, 62.70942372801902565 ) ) ;
#89222=CARTESIAN_POINT ( 'NONE',  ( -12.06949235617756955, 12.14591786802309770, 80.62390960531438111 ) ) ;
#89223=CARTESIAN_POINT ( 'NONE',  ( 5.823673210054125526, 21.52544592524343514, 74.79057627198105251 ) ) ;
#89224=CARTESIAN_POINT ( 'NONE',  ( 8.224510206698953496, -14.34966873604960469, 22.91557627198102765 ) ) ;
#89225=CARTESIAN_POINT ( 'NONE',  ( 8.224510206698742110, 14.34966873604972548, 47.08442372801901854 ) ) ;
#89226=CARTESIAN_POINT ( 'NONE',  ( 16.51473224551069308, 9.474510206698969483, 49.16557627198102409 ) ) ;
#89227=CARTESIAN_POINT ( 'NONE',  ( -16.53943276465976808, -0.05219959533934237506, 98.75109039468568994 ) ) ;
#89228=CARTESIAN_POINT ( 'NONE',  ( -13.97604488694547697, 13.89961937509957934, 88.12609039468563310 ) ) ;
#89229=CARTESIAN_POINT ( 'NONE',  ( 10.81492255796078972, 18.62759615963270932, 89.58224293864768129 ) ) ;
#89230=CARTESIAN_POINT ( 'NONE',  ( 16.55341960407611168, 4.379528057220329451, 23.95724293864769550 ) ) ;
#89231=ORIENTED_EDGE ( 'NONE', *, *, #114658, .F. ) ;
#89233=CARTESIAN_POINT ( 'NONE',  ( -0.05219959533907301413, -21.53943276465977519, 62.49890960531436690 ) ) ;
#89234=ORIENTED_EDGE ( 'NONE', *, *, #94263, .T. ) ;
#89235=CARTESIAN_POINT ( 'NONE',  ( 4.379528057220092307, 16.55341960407617563, 87.29275706135236135 ) ) ;
#89237=CARTESIAN_POINT ( 'NONE',  ( 10.81492255796078972, 18.62759615963270932, 29.58224293864769905 ) ) ;
#89238=CARTESIAN_POINT ( 'NONE',  ( -19.01533133064924641, 5.499999999999450218, 73.76586590595742621 ) ) ;
#89239=CARTESIAN_POINT ( 'NONE',  ( 5.823673210054125526, 21.52544592524343514, 79.79057627198102409 ) ) ;
#89241=CARTESIAN_POINT ( 'NONE',  ( -12.14591786802309592, -12.06949235617757132, 26.87390960531435979 ) ) ;
#89242=CARTESIAN_POINT ( 'NONE',  ( -14.29746914071037622, -8.314922557961029526, 19.16775706135234714 ) ) ;
#89243=CARTESIAN_POINT ( 'NONE',  ( 16.46253265017160672, -9.564922557960803928, 33.33224293864770260 ) ) ;
#89244=CARTESIAN_POINT ( 'NONE',  ( -12.06949235617739369, -12.14591786802326823, 34.37609039468568284 ) ) ;
#89246=CARTESIAN_POINT ( 'NONE',  ( -16.46253265017160317, 9.564922557960807481, 50.83224293864770260 ) ) ;
#89248=CARTESIAN_POINT ( 'NONE',  ( -5.049401038298153566, 19.05341960407611168, 110.2072429386476671 ) ) ;
#89249=CARTESIAN_POINT ( 'NONE',  ( 9.474510206698971260, -16.51473224551069308, 102.9155762719810241 ) ) ;
#89250=CARTESIAN_POINT ( 'NONE',  ( -8.224510206698735004, -14.34966873604973081, 94.58442372801901854 ) ) ;
#89251=CARTESIAN_POINT ( 'NONE',  ( -16.46253265017146816, -9.564922557961047289, 89.16775706135234714 ) ) ;
#89252=CARTESIAN_POINT ( 'NONE',  ( -0.05219959533936034679, 19.03943276465977164, 32.50109039468566863 ) ) ;
#89253=CARTESIAN_POINT ( 'NONE',  ( 5.823673210054125526, 21.52544592524343514, 69.79057627198102409 ) ) ;
#89254=CARTESIAN_POINT ( 'NONE',  ( 4.379528057220092307, 16.55341960407617563, 97.29275706135234714 ) ) ;
#89255=CARTESIAN_POINT ( 'NONE',  ( -5.823673210054116645, -21.52544592524344225, 32.29057627198102409 ) ) ;
#89256=CARTESIAN_POINT ( 'NONE',  ( -16.51473224551082808, 9.474510206698731452, 93.33442372801900433 ) ) ;
#89257=CARTESIAN_POINT ( 'NONE',  ( 5.049401038298161559, -19.05341960407611168, 47.70724293864770260 ) ) ;
#89258=CARTESIAN_POINT ( 'NONE',  ( -9.564922557960796823, -16.46253265017161027, 87.08224293864769550 ) ) ;
#89259=CARTESIAN_POINT ( 'NONE',  ( -10.81492255796105439, 18.62759615963255655, 62.91775706135236135 ) ) ;
#89260=CARTESIAN_POINT ( 'NONE',  ( 9.564922557960805705, 16.46253265017160317, 64.58224293864769550 ) ) ;
#89261=CARTESIAN_POINT ( 'NONE',  ( 14.34966873604960469, 8.224510206698951720, 104.1655762719810241 ) ) ;
#89263=CARTESIAN_POINT ( 'NONE',  ( -8.314922557960811034, -14.29746914071050412, 77.08224293864769550 ) ) ;
#89264=CARTESIAN_POINT ( 'NONE',  ( -21.52544592524343514, 5.823673210054127303, 71.04057627198103830 ) ) ;
#89265=CARTESIAN_POINT ( 'NONE',  ( -5.153800228976607833, 19.02544592524334988, 92.70942372801901854 ) ) ;
#89267=CARTESIAN_POINT ( 'NONE',  ( 18.22780087662122384, 5.500000000000018652, 93.98459894673892734 ) ) ;
#89268=CARTESIAN_POINT ( 'NONE',  ( 5.049401038298161559, -19.05341960407611168, 62.70724293864769550 ) ) ;
#89270=CARTESIAN_POINT ( 'NONE',  ( -9.564922557960796823, -16.46253265017161027, 82.08224293864768129 ) ) ;
#89271=CARTESIAN_POINT ( 'NONE',  ( 0.05219959533909260263, 19.03943276465977164, 84.99890960531436690 ) ) ;
#89272=EDGE_CURVE ( 'NONE', #192686, #142224, #58294, .T. ) ;
#89273=CARTESIAN_POINT ( 'NONE',  ( -16.55341960407617563, 4.379528057220093196, 68.54275706135234714 ) ) ;
#89274=CARTESIAN_POINT ( 'NONE',  ( -17.26058549869088665, -6.457015423128631859, 51.37745837476068544 ) ) ;
#89275=CARTESIAN_POINT ( 'NONE',  ( -19.03943276465977164, -0.05219959533935918106, 48.75109039468566863 ) ) ;
#89277=CARTESIAN_POINT ( 'NONE',  ( -13.89961937509977652, 13.97604488694528158, 115.6239096053143669 ) ) ;
#89278=CARTESIAN_POINT ( 'NONE',  ( -4.483927247898782831, 16.52544592524335698, 97.70942372801904696 ) ) ;
#89280=CARTESIAN_POINT ( 'NONE',  ( 12.06949235617739724, 12.14591786802326823, 81.87609039468568994 ) ) ;
#89282=CARTESIAN_POINT ( 'NONE',  ( -4.379528057220086978, -16.55341960407618274, 49.79275706135234714 ) ) ;
#89283=CARTESIAN_POINT ( 'NONE',  ( 10.72451020669871369, 18.67979575497193778, 72.08442372801899012 ) ) ;
#89284=CARTESIAN_POINT ( 'NONE',  ( 19.05341960407617918, -5.049401038297876454, 71.04275706135234714 ) ) ;
#89285=CARTESIAN_POINT ( 'NONE',  ( 13.89961937509957401, 13.97604488694547697, 31.87609039468566863 ) ) ;
#89286=CARTESIAN_POINT ( 'NONE',  ( -13.97604488694527625, -13.89961937509977652, 61.87390960531435979 ) ) ;
#89287=CARTESIAN_POINT ( 'NONE',  ( 9.474510206698971260, -16.51473224551069308, 47.91557627198102409 ) ) ;
#89289=CARTESIAN_POINT ( 'NONE',  ( -10.72451020669898014, 18.67979575497178502, 65.41557627198102409 ) ) ;
#89290=CARTESIAN_POINT ( 'NONE',  ( 21.55341960407610458, 5.719274019375980345, 38.95724293864768839 ) ) ;
#89291=CARTESIAN_POINT ( 'NONE',  ( -4.379528057220328563, 16.55341960407611168, 115.2072429386476955 ) ) ;
#89292=CARTESIAN_POINT ( 'NONE',  ( 16.52544592524335698, 4.483927247898782831, 46.45942372801901854 ) ) ;
#89295=CARTESIAN_POINT ( 'NONE',  ( -0.05219959533937732626, 21.53943276465977519, 32.50109039468568284 ) ) ;
#89296=CARTESIAN_POINT ( 'NONE',  ( -8.224510206698948167, 14.34966873604960824, 55.41557627198102409 ) ) ;
#89298=CARTESIAN_POINT ( 'NONE',  ( -16.55341960407617563, 4.379528057220093196, 28.54275706135234358 ) ) ;
#89299=CARTESIAN_POINT ( 'NONE',  ( 19.02544592524334988, 5.153800228976608722, 46.45942372801899012 ) ) ;
#89300=CARTESIAN_POINT ( 'NONE',  ( 8.314922557960818139, 14.29746914071049879, 49.58224293864769550 ) ) ;
#89301=CARTESIAN_POINT ( 'NONE',  ( -5.719274019375978568, 21.55341960407610458, 115.2072429386476955 ) ) ;
#89303=CARTESIAN_POINT ( 'NONE',  ( -0.05219959533907301413, -21.53943276465977519, 77.49890960531433848 ) ) ;
#89304=CARTESIAN_POINT ( 'NONE',  ( -9.474510206698964154, 16.51473224551069663, 95.41557627198102409 ) ) ;
#89305=CARTESIAN_POINT ( 'NONE',  ( -4.379528057220328563, 16.55341960407611168, 60.20724293864768839 ) ) ;
#89306=CARTESIAN_POINT ( 'NONE',  ( -0.05219959533909027116, -19.03943276465977164, 107.4989096053143527 ) ) ;
#89308=CARTESIAN_POINT ( 'NONE',  ( 13.97604488694548053, -13.89961937509957401, 70.62609039468567573 ) ) ;
#89309=CARTESIAN_POINT ( 'NONE',  ( 5.823673210054125526, 21.52544592524343514, 104.7905762719810241 ) ) ;
#89310=CARTESIAN_POINT ( 'NONE',  ( -13.97604488694527625, -13.89961937509977652, 56.87390960531434558 ) ) ;
#89311=CARTESIAN_POINT ( 'NONE',  ( -14.34966873604960291, -8.224510206698953496, 111.6655762719810525 ) ) ;
#89312=CARTESIAN_POINT ( 'NONE',  ( 0.05219959533937995610, -21.53943276465977519, 50.00109039468568994 ) ) ;
#89314=CARTESIAN_POINT ( 'NONE',  ( 8.224510206698953496, -14.34966873604960469, 42.91557627198103120 ) ) ;
#89315=CARTESIAN_POINT ( 'NONE',  ( 16.51473224551069308, 9.474510206698969483, 44.16557627198103120 ) ) ;
#89316=CARTESIAN_POINT ( 'NONE',  ( 13.89961937509977652, -13.97604488694527269, 98.12390960531433848 ) ) ;
#89317=CARTESIAN_POINT ( 'NONE',  ( 10.81492255796078972, 18.62759615963270932, 74.58224293864768129 ) ) ;
#89319=CARTESIAN_POINT ( 'NONE',  ( -19.02544592524342804, 5.153800228976336051, 41.04057627198103120 ) ) ;
#89320=ORIENTED_EDGE ( 'NONE', *, *, #163734, .F. ) ;
#89321=CARTESIAN_POINT ( 'NONE',  ( 15.80617190586746368, 15.72974639402197994, 64.37390960531435269 ) ) ;
#89322=CARTESIAN_POINT ( 'NONE',  ( -5.823673210054431948, 21.52544592524334988, 82.70942372801900433 ) ) ;
#89323=CARTESIAN_POINT ( 'NONE',  ( 15.50000000000000178, 5.499999999999998224, 118.0000000000000142 ) ) ;
#89324=CARTESIAN_POINT ( 'NONE',  ( -12.06949235617739369, -12.14591786802326823, 84.37609039468570415 ) ) ;
#89325=CARTESIAN_POINT ( 'NONE',  ( -8.314922557960811034, -14.29746914071050412, 87.08224293864769550 ) ) ;
#89326=CARTESIAN_POINT ( 'NONE',  ( -16.46253265017160317, 9.564922557960807481, 65.83224293864769550 ) ) ;
#89328=CARTESIAN_POINT ( 'NONE',  ( 5.153800228976615827, -19.02544592524334988, 20.20942372801899722 ) ) ;
#89329=CARTESIAN_POINT ( 'NONE',  ( -4.379528057220086978, -16.55341960407618274, 89.79275706135236135 ) ) ;
#89330=CARTESIAN_POINT ( 'NONE',  ( 18.62759615963255655, 10.81492255796105972, 106.6677570613523756 ) ) ;
#89331=CARTESIAN_POINT ( 'NONE',  ( 16.46253265017160672, -9.564922557960803928, 88.33224293864769550 ) ) ;
#89332=CARTESIAN_POINT ( 'NONE',  ( 10.81492255796078972, 18.62759615963270932, 49.58224293864769550 ) ) ;
#89333=CARTESIAN_POINT ( 'NONE',  ( 5.719274019375673035, 21.55341960407619339, 97.29275706135234714 ) ) ;
#89334=CARTESIAN_POINT ( 'NONE',  ( 12.06949235617739724, 12.14591786802326823, 56.87609039468568994 ) ) ;
#89335=CARTESIAN_POINT ( 'NONE',  ( -5.719274019375665041, -21.55341960407619695, 19.79275706135235069 ) ) ;
#89336=CARTESIAN_POINT ( 'NONE',  ( -19.05341960407617563, 5.049401038297882671, 108.5427570613523187 ) ) ;
#89337=CARTESIAN_POINT ( 'NONE',  ( -5.049401038298153566, 19.05341960407611168, 90.20724293864766707 ) ) ;
#89338=CARTESIAN_POINT ( 'NONE',  ( -16.53943276465976808, -0.05219959533934237506, 33.75109039468568284 ) ) ;
#89339=CARTESIAN_POINT ( 'NONE',  ( 5.049401038298161559, -19.05341960407611168, 57.70724293864769550 ) ) ;
#89341=CARTESIAN_POINT ( 'NONE',  ( -4.379528057220086978, -16.55341960407618274, 39.79275706135235424 ) ) ;
#89342=CARTESIAN_POINT ( 'NONE',  ( -0.05219959533910754901, -16.53943276465976808, 82.49890960531436690 ) ) ;
#89343=CARTESIAN_POINT ( 'NONE',  ( 8.314922557961029526, -14.29746914071037800, 85.41775706135236135 ) ) ;
#89345=CARTESIAN_POINT ( 'NONE',  ( 21.55341960407619695, -5.719274019375665929, 41.04275706135236135 ) ) ;
#89346=CARTESIAN_POINT ( 'NONE',  ( -5.153800228976328057, -19.02544592524343514, 62.29057627198100988 ) ) ;
#89347=CARTESIAN_POINT ( 'NONE',  ( 5.153800228976335163, 19.02544592524342804, 79.79057627198102409 ) ) ;
#89348=CARTESIAN_POINT ( 'NONE',  ( 12.06949235617757843, -12.14591786802309237, 28.12390960531435979 ) ) ;
#89349=CARTESIAN_POINT ( 'NONE',  ( 14.29746914071037800, 8.314922557961029526, 86.66775706135234714 ) ) ;
#89351=ORIENTED_EDGE ( 'NONE', *, *, #6212, .F. ) ;
#89352=CARTESIAN_POINT ( 'NONE',  ( -9.474510206698720793, -16.51473224551083518, 24.58442372801900078 ) ) ;
#89353=CARTESIAN_POINT ( 'NONE',  ( 0.05219959533909260263, 19.03943276465977164, 104.9989096053143669 ) ) ;
#89354=CARTESIAN_POINT ( 'NONE',  ( -13.97604488694527625, -13.89961937509977652, 51.87390960531436690 ) ) ;
#89356=CARTESIAN_POINT ( 'NONE',  ( 0.05219959533934541429, -16.53943276465976808, 40.00109039468567573 ) ) ;
#89357=CARTESIAN_POINT ( 'NONE',  ( -5.049401038297874678, -19.05341960407617918, 64.79275706135233293 ) ) ;
#89358=CARTESIAN_POINT ( 'NONE',  ( 14.34966873604972726, -8.224510206698740333, 50.83442372801901143 ) ) ;
#89360=CARTESIAN_POINT ( 'NONE',  ( -0.05219959533909027116, -19.03943276465977164, 72.49890960531435269 ) ) ;
#89361=CARTESIAN_POINT ( 'NONE',  ( 10.81492255796078972, 18.62759615963270932, 114.5822429386477097 ) ) ;
#89362=CARTESIAN_POINT ( 'NONE',  ( -5.153800228976607833, 19.02544592524334988, 62.70942372801899722 ) ) ;
#89363=CARTESIAN_POINT ( 'NONE',  ( 13.97604488694527802, 13.89961937509977652, 109.3739096053143669 ) ) ;
#89365=CARTESIAN_POINT ( 'NONE',  ( -0.05219959533909027116, -19.03943276465977164, 72.49890960531435269 ) ) ;
#89366=CARTESIAN_POINT ( 'NONE',  ( -4.379528057220328563, 16.55341960407611168, 35.20724293864768839 ) ) ;
#89368=CARTESIAN_POINT ( 'NONE',  ( -13.97604488694547697, 13.89961937509957934, 33.12609039468566863 ) ) ;
#89369=CARTESIAN_POINT ( 'NONE',  ( -0.05219959533910754901, -16.53943276465976808, 72.49890960531435269 ) ) ;
#89370=CARTESIAN_POINT ( 'NONE',  ( -15.80617190586768217, 15.72974639402176855, 113.1260903946856899 ) ) ;
#89371=CARTESIAN_POINT ( 'NONE',  ( -16.51473224551069308, -9.474510206698971260, 41.66557627198103120 ) ) ;
#89372=CARTESIAN_POINT ( 'NONE',  ( 14.34966873604960469, 8.224510206698951720, 44.16557627198103120 ) ) ;
#89373=CARTESIAN_POINT ( 'NONE',  ( -21.52544592524334988, -5.823673210054445271, 103.9594237280190185 ) ) ;
#89374=CARTESIAN_POINT ( 'NONE',  ( 5.049401038298161559, -19.05341960407611168, 87.70724293864769550 ) ) ;
#89375=CARTESIAN_POINT ( 'NONE',  ( 19.02544592524343514, -5.153800228976328945, 108.5405762719810383 ) ) ;
#89376=CARTESIAN_POINT ( 'NONE',  ( 0.05219959533909260263, 19.03943276465977164, 44.99890960531435979 ) ) ;
#89377=CARTESIAN_POINT ( 'NONE',  ( 4.483927247898545687, 16.52544592524342804, 109.7905762719810383 ) ) ;
#89378=CARTESIAN_POINT ( 'NONE',  ( 12.14591786802309770, 12.06949235617756955, 79.37390960531436690 ) ) ;
#89379=CARTESIAN_POINT ( 'NONE',  ( 10.81492255796078972, 18.62759615963270932, 89.58224293864768129 ) ) ;
#89380=CARTESIAN_POINT ( 'NONE',  ( 5.049401038298161559, -19.05341960407611168, 82.70724293864770971 ) ) ;
#89381=CARTESIAN_POINT ( 'NONE',  ( 21.52544592524344225, -5.823673210054117533, 103.5405762719810383 ) ) ;
#89382=CARTESIAN_POINT ( 'NONE',  ( 9.564922557960805705, 16.46253265017160317, 84.58224293864769550 ) ) ;
#89383=CARTESIAN_POINT ( 'NONE',  ( -18.56101223717332260, -5.500000000000064837, 91.44978406935680937 ) ) ;
#89384=CARTESIAN_POINT ( 'NONE',  ( 4.483927247898545687, 16.52544592524342804, 109.7905762719810383 ) ) ;
#89386=CARTESIAN_POINT ( 'NONE',  ( 16.46253265017160672, -9.564922557960803928, 73.33224293864769550 ) ) ;
#89387=CARTESIAN_POINT ( 'NONE',  ( -10.81492255796078084, -18.62759615963271287, 82.08224293864768129 ) ) ;
#89389=CARTESIAN_POINT ( 'NONE',  ( -10.81492255796078084, -18.62759615963271287, 27.08224293864769550 ) ) ;
#89391=CARTESIAN_POINT ( 'NONE',  ( 16.53943276465976808, 0.05219959533934440121, 21.25109039468567218 ) ) ;
#89392=CARTESIAN_POINT ( 'NONE',  ( -8.314922557960811034, -14.29746914071050412, 92.08224293864769550 ) ) ;
#89393=CARTESIAN_POINT ( 'NONE',  ( -16.20579543436678449, -7.371946100355106779, 95.56520834171877254 ) ) ;
#89394=CARTESIAN_POINT ( 'NONE',  ( -5.049401038298153566, 19.05341960407611168, 90.20724293864766707 ) ) ;
#89395=CARTESIAN_POINT ( 'NONE',  ( 19.05341960407611168, 5.049401038298154454, 43.95724293864769550 ) ) ;
#89396=CARTESIAN_POINT ( 'NONE',  ( -16.53943276465976808, 0.05219959533911058130, 86.24890960531436690 ) ) ;
#89397=CARTESIAN_POINT ( 'NONE',  ( -0.05219959533907301413, -21.53943276465977519, 22.49890960531436335 ) ) ;
#89398=CARTESIAN_POINT ( 'NONE',  ( 12.14591786802309770, 12.06949235617756955, 49.37390960531436690 ) ) ;
#89399=CARTESIAN_POINT ( 'NONE',  ( -0.05219959533936034679, 19.03943276465977164, 102.5010903946856757 ) ) ;
#89400=CARTESIAN_POINT ( 'NONE',  ( -10.72451020669870658, -18.67979575497194134, 59.58442372801901854 ) ) ;
#89402=CARTESIAN_POINT ( 'NONE',  ( 19.05341960407611168, 5.049401038298154454, 103.9572429386476671 ) ) ;
#89403=CARTESIAN_POINT ( 'NONE',  ( 10.72451020669898902, -18.67979575497178502, 92.91557627198103830 ) ) ;
#89404=CARTESIAN_POINT ( 'NONE',  ( 0.05219959533934541429, -16.53943276465976808, 85.00109039468568994 ) ) ;
#89405=CARTESIAN_POINT ( 'NONE',  ( 13.97604488694527802, 13.89961937509977652, 24.37390960531435624 ) ) ;
#89406=CARTESIAN_POINT ( 'NONE',  ( 0.05219959533909260263, 19.03943276465977164, 79.99890960531436690 ) ) ;
#89407=CARTESIAN_POINT ( 'NONE',  ( 21.52544592524344225, -5.823673210054117533, 78.54057627198103830 ) ) ;
#89408=CARTESIAN_POINT ( 'NONE',  ( 13.97604488694548053, -13.89961937509957401, 105.6260903946856757 ) ) ;
#89409=CARTESIAN_POINT ( 'NONE',  ( 8.224510206698953496, -14.34966873604960469, 47.91557627198102409 ) ) ;
#89410=CARTESIAN_POINT ( 'NONE',  ( 0.05219959533937995610, -21.53943276465977519, 55.00109039468568284 ) ) ;
#89411=CARTESIAN_POINT ( 'NONE',  ( 4.379528057220092307, 16.55341960407617563, 87.29275706135236135 ) ) ;
#89412=CARTESIAN_POINT ( 'NONE',  ( 16.51473224551069308, 9.474510206698969483, 114.1655762719810241 ) ) ;
#89413=CARTESIAN_POINT ( 'NONE',  ( -13.89961937509977830, 13.97604488694528158, 110.6239096053143527 ) ) ;
#89415=CARTESIAN_POINT ( 'NONE',  ( -12.06949235617739369, -12.14591786802326823, 104.3760903946856899 ) ) ;
#89416=CARTESIAN_POINT ( 'NONE',  ( 14.29746914071037800, 8.314922557961029526, 56.66775706135235424 ) ) ;
#89417=CARTESIAN_POINT ( 'NONE',  ( 16.46253265017160672, -9.564922557960803928, 68.33224293864770971 ) ) ;
#89418=CARTESIAN_POINT ( 'NONE',  ( 0.05219959533909260263, 19.03943276465977164, 79.99890960531436690 ) ) ;
#89419=CARTESIAN_POINT ( 'NONE',  ( -12.06949235617739369, -12.14591786802326823, 74.37609039468568994 ) ) ;
#89420=CARTESIAN_POINT ( 'NONE',  ( -16.53943276465976808, 0.05219959533911058130, 46.24890960531435979 ) ) ;
#89421=CARTESIAN_POINT ( 'NONE',  ( 16.46253265017160672, -9.564922557960803928, 58.33224293864769550 ) ) ;
#89422=CARTESIAN_POINT ( 'NONE',  ( -9.474510206698964154, 16.51473224551069663, 45.41557627198103120 ) ) ;
#89423=CARTESIAN_POINT ( 'NONE',  ( -4.483927247898782831, 16.52544592524335698, 42.70942372801901854 ) ) ;
#89425=CARTESIAN_POINT ( 'NONE',  ( -16.46253265017146816, -9.564922557961047289, 94.16775706135233293 ) ) ;
#89426=CARTESIAN_POINT ( 'NONE',  ( 8.224510206698953496, -14.34966873604960469, 97.91557627198103830 ) ) ;
#89427=CARTESIAN_POINT ( 'NONE',  ( -5.049401038298153566, 19.05341960407611168, 65.20724293864765286 ) ) ;
#89428=CARTESIAN_POINT ( 'NONE',  ( -9.474510206698720793, -16.51473224551083518, 94.58442372801900433 ) ) ;
#89430=CARTESIAN_POINT ( 'NONE',  ( -21.55341960407619339, 5.719274019375674811, 98.54275706135234714 ) ) ;
#89431=CARTESIAN_POINT ( 'NONE',  ( 8.314922557961029526, -14.29746914071037800, 65.41775706135234714 ) ) ;
#89432=DIRECTION ( 'NONE',  ( -0.000000000000000000, -0.000000000000000000, 1.000000000000000000 ) ) ;
#89433=CARTESIAN_POINT ( 'NONE',  ( -18.62759615963270932, 10.81492255796079327, 60.83224293864769550 ) ) ;
#89434=CARTESIAN_POINT ( 'NONE',  ( 14.34966873604972726, -8.224510206698740333, 50.83442372801901143 ) ) ;
#89435=DIRECTION ( 'NONE',  ( -1.000000000000000000, 0.000000000000000000, 0.000000000000000000 ) ) ;
#89436=CARTESIAN_POINT ( 'NONE',  ( -13.89961937509957401, -13.97604488694547875, 39.37609039468566152 ) ) ;
#89437=CARTESIAN_POINT ( 'NONE',  ( -13.97604488694527625, -13.89961937509977652, 91.87390960531432427 ) ) ;
#89438=CARTESIAN_POINT ( 'NONE',  ( 16.53943276465976808, -0.05219959533910856209, 113.7489096053143527 ) ) ;
#89439=CARTESIAN_POINT ( 'NONE',  ( 19.02544592524343514, -5.153800228976328945, 63.54057627198103830 ) ) ;
#89440=CARTESIAN_POINT ( 'NONE',  ( -5.823673210054431948, 21.52544592524334988, 82.70942372801900433 ) ) ;
#89441=CARTESIAN_POINT ( 'NONE',  ( -16.46253265017146816, -9.564922557961047289, 44.16775706135232582 ) ) ;
#89442=CARTESIAN_POINT ( 'NONE',  ( -5.153800228976607833, 19.02544592524334988, 32.70942372801899722 ) ) ;
#89443=CARTESIAN_POINT ( 'NONE',  ( -13.97604488694527625, -13.89961937509977652, 56.87390960531434558 ) ) ;
#89444=CARTESIAN_POINT ( 'NONE',  ( 19.03943276465977164, -0.05219959533909143690, 113.7489096053143669 ) ) ;
#89445=CARTESIAN_POINT ( 'NONE',  ( -10.72451020669870658, -18.67979575497194134, 89.58442372801901854 ) ) ;
#89446=CARTESIAN_POINT ( 'NONE',  ( -9.564922557960796823, -16.46253265017161027, 67.08224293864769550 ) ) ;
#89448=CARTESIAN_POINT ( 'NONE',  ( 18.67979575497194134, -10.72451020669871369, 95.83442372801903275 ) ) ;
#89449=CARTESIAN_POINT ( 'NONE',  ( 5.719274019375991003, -21.55341960407610458, 32.70724293864770260 ) ) ;
#89450=CARTESIAN_POINT ( 'NONE',  ( 9.474510206698971260, -16.51473224551069308, 77.91557627198103830 ) ) ;
#89451=CARTESIAN_POINT ( 'NONE',  ( -21.52544592524334988, -5.823673210054445271, 38.95942372801901854 ) ) ;
#89452=CARTESIAN_POINT ( 'NONE',  ( -19.02544592524334988, -5.153800228976617603, 58.95942372801900433 ) ) ;
#89453=CARTESIAN_POINT ( 'NONE',  ( -0.05219959533909027116, -19.03943276465977164, 47.49890960531435979 ) ) ;
#89454=CARTESIAN_POINT ( 'NONE',  ( -16.51473224551069308, -9.474510206698971260, 86.66557627198102409 ) ) ;
#89455=CARTESIAN_POINT ( 'NONE',  ( -12.06949235617739369, -12.14591786802326823, 24.37609039468567573 ) ) ;
#89456=CARTESIAN_POINT ( 'NONE',  ( 16.55341960407611168, 4.379528057220329451, 83.95724293864770971 ) ) ;
#89457=CARTESIAN_POINT ( 'NONE',  ( 19.02544592524343514, -5.153800228976328945, 73.54057627198103830 ) ) ;
#89458=CARTESIAN_POINT ( 'NONE',  ( -21.55341960407610458, -5.719274019375992779, 46.45724293864769550 ) ) ;
#89459=B_SPLINE_CURVE_WITH_KNOTS ( 'NONE', 3,
 ( #4821, #20007, #113005, #161518, #55335, #8842, #37164, #143334, #66509, #129160, #69506, #175689, #174699, #131172, #192862, #51345, #21000, #190857, #82655, #54341, #98823, #58337, #134192, #102843 ),
 .UNSPECIFIED., .F., .F.,
 ( 4, 2, 2, 2, 2, 2, 2, 2, 2, 2, 2, 4 ),
 ( 3.849469143858236616E-15, 0.0003995125125255656411, 0.0007990250250472818224, 0.0009987812813081384765, 0.001198537537568994914, 0.001398293793829851351, 0.001598050050090707788, 0.001797806306351564225, 0.001997562562612420229, 0.002397075075134141777, 0.002796587587655863325, 0.003196100100177584440 ),
 .UNSPECIFIED. ) ;
#89460=CARTESIAN_POINT ( 'NONE',  ( 19.02544592524334988, 5.153800228976608722, 111.4594237280190043 ) ) ;
#89461=CARTESIAN_POINT ( 'NONE',  ( 21.53943276465977519, 0.05219959533937863772, 26.25109039468567573 ) ) ;
#89462=CARTESIAN_POINT ( 'NONE',  ( 0.05219959533937995610, -21.53943276465977519, 75.00109039468568994 ) ) ;
#89463=CARTESIAN_POINT ( 'NONE',  ( -14.29746914071037622, -8.314922557961029526, 64.16775706135234714 ) ) ;
#89464=CARTESIAN_POINT ( 'NONE',  ( -16.53943276465976808, -0.05219959533934237506, 63.75109039468568284 ) ) ;
#89465=CARTESIAN_POINT ( 'NONE',  ( 0.05219959533909260263, 19.03943276465977164, 64.99890960531436690 ) ) ;
#89466=CARTESIAN_POINT ( 'NONE',  ( -16.53943276465976808, -0.05219959533934237506, 103.7510903946857042 ) ) ;
#89467=CARTESIAN_POINT ( 'NONE',  ( 16.46253265017146816, 9.564922557961045513, 46.66775706135233293 ) ) ;
#89468=CARTESIAN_POINT ( 'NONE',  ( -5.719274019375978568, 21.55341960407610458, 115.2072429386476955 ) ) ;
#89469=CARTESIAN_POINT ( 'NONE',  ( -14.29746914071049879, 8.314922557960819915, 60.83224293864769550 ) ) ;
#89470=CARTESIAN_POINT ( 'NONE',  ( -0.05219959533909027116, -19.03943276465977164, 87.49890960531436690 ) ) ;
#89471=CARTESIAN_POINT ( 'NONE',  ( -8.314922557961024197, 14.29746914071037800, 82.91775706135234714 ) ) ;
#89472=CARTESIAN_POINT ( 'NONE',  ( 5.823673210054444382, -21.52544592524334988, 65.20942372801901854 ) ) ;
#89473=CARTESIAN_POINT ( 'NONE',  ( -4.483927247898782831, 16.52544592524335698, 37.70942372801900433 ) ) ;
#89474=CARTESIAN_POINT ( 'NONE',  ( 21.52544592524334988, 5.823673210054432836, 21.45942372801901499 ) ) ;
#89475=CARTESIAN_POINT ( 'NONE',  ( -16.52544592524342804, 4.483927247898546575, 61.04057627198103120 ) ) ;
#89477=CARTESIAN_POINT ( 'NONE',  ( -10.81492255796078084, -18.62759615963271287, 107.0822429386476955 ) ) ;
#89478=CARTESIAN_POINT ( 'NONE',  ( -0.05219959533910754901, -16.53943276465976808, 42.49890960531435979 ) ) ;
#89481=CARTESIAN_POINT ( 'NONE',  ( 10.81492255796078972, 18.62759615963270932, 29.58224293864769905 ) ) ;
#89482=CARTESIAN_POINT ( 'NONE',  ( -15.72974639402176322, -15.80617190586768395, 39.37609039468567573 ) ) ;
#89483=CARTESIAN_POINT ( 'NONE',  ( -4.483927247898539470, -16.52544592524342804, 67.29057627198103830 ) ) ;
#89485=CARTESIAN_POINT ( 'NONE',  ( 10.72451020669898902, -18.67979575497178502, 72.91557627198103830 ) ) ;
#89486=CARTESIAN_POINT ( 'NONE',  ( -16.51473224551069308, -9.474510206698971260, 71.66557627198102409 ) ) ;
#89487=CARTESIAN_POINT ( 'NONE',  ( 5.049401038298161559, -19.05341960407611168, 27.70724293864769550 ) ) ;
#89488=CARTESIAN_POINT ( 'NONE',  ( -0.05219959533936034679, 19.03943276465977164, 62.50109039468566863 ) ) ;
#89489=CARTESIAN_POINT ( 'NONE',  ( -15.72974639402197994, 15.80617190586746368, 50.62390960531435979 ) ) ;
#89490=CARTESIAN_POINT ( 'NONE',  ( 13.97604488694527802, 13.89961937509977652, 59.37390960531434558 ) ) ;
#89492=CARTESIAN_POINT ( 'NONE',  ( 12.06949235617739724, 12.14591786802326823, 31.87609039468567929 ) ) ;
#89493=CARTESIAN_POINT ( 'NONE',  ( -18.67979575497178146, -10.72451020669898902, 111.6655762719810525 ) ) ;
#89494=CARTESIAN_POINT ( 'NONE',  ( 16.52544592524342804, -4.483927247898539470, 53.54057627198103120 ) ) ;
#89495=CARTESIAN_POINT ( 'NONE',  ( 5.049401038298161559, -19.05341960407611168, 97.70724293864766707 ) ) ;
#89496=CARTESIAN_POINT ( 'NONE',  ( -5.719274019375978568, 21.55341960407610458, 70.20724293864769550 ) ) ;
#89497=CARTESIAN_POINT ( 'NONE',  ( 10.81492255796078972, 18.62759615963270932, 109.5822429386476955 ) ) ;
#89498=CARTESIAN_POINT ( 'NONE',  ( -8.224510206698735004, -14.34966873604973081, 34.58442372801900433 ) ) ;
#89499=VECTOR ( 'NONE', #77542, 1000.000000000000000 ) ;
#89500=CARTESIAN_POINT ( 'NONE',  ( -5.719274019375978568, 21.55341960407610458, 35.20724293864768839 ) ) ;
#89501=CARTESIAN_POINT ( 'NONE',  ( 18.62759615963255655, 10.81492255796105972, 96.66775706135234714 ) ) ;
#89502=CARTESIAN_POINT ( 'NONE',  ( 0.05219959533909260263, 19.03943276465977164, 39.99890960531436690 ) ) ;
#89503=CARTESIAN_POINT ( 'NONE',  ( 19.05341960407611168, 5.049401038298154454, 98.95724293864766707 ) ) ;
#89504=CARTESIAN_POINT ( 'NONE',  ( 19.02544592524343514, -5.153800228976328945, 73.54057627198103830 ) ) ;
#89506=CARTESIAN_POINT ( 'NONE',  ( 5.049401038297881783, 19.05341960407617563, 52.29275706135234003 ) ) ;
#89507=CARTESIAN_POINT ( 'NONE',  ( 21.52544592524334988, 5.823673210054432836, 106.4594237280190328 ) ) ;
#89508=CARTESIAN_POINT ( 'NONE',  ( -21.53943276465977519, 0.05219959533907696930, 26.24890960531435624 ) ) ;
#89509=CARTESIAN_POINT ( 'NONE',  ( 14.34966873604972726, -8.224510206698740333, 110.8344237280190043 ) ) ;
#89510=CARTESIAN_POINT ( 'NONE',  ( -5.049401038297874678, -19.05341960407617918, 79.79275706135233293 ) ) ;
#89511=PLANE ( 'NONE',  #160 ) ;
#89512=CARTESIAN_POINT ( 'NONE',  ( 19.02544592524334988, 5.153800228976608722, 86.45942372801900433 ) ) ;
#89513=CARTESIAN_POINT ( 'NONE',  ( 19.05341960407617918, -5.049401038297876454, 41.04275706135233293 ) ) ;
#89514=CARTESIAN_POINT ( 'NONE',  ( -17.49999999999999645, -5.624438216177608751, 44.18329655085357643 ) ) ;
#89515=CARTESIAN_POINT ( 'NONE',  ( -13.97604488694527625, -13.89961937509977652, 41.87390960531435979 ) ) ;
#89516=CARTESIAN_POINT ( 'NONE',  ( -4.379528057220328563, 16.55341960407611168, 55.20724293864770260 ) ) ;
#89517=CARTESIAN_POINT ( 'NONE',  ( -13.89961937509977652, 13.97604488694528158, 30.62390960531435269 ) ) ;
#89518=CARTESIAN_POINT ( 'NONE',  ( 14.34966873604960469, 8.224510206698951720, 39.16557627198102409 ) ) ;
#89519=CARTESIAN_POINT ( 'NONE',  ( 17.50000000000000000, -7.500000000000000888, 118.0000000000000142 ) ) ;
#89520=CARTESIAN_POINT ( 'NONE',  ( -16.52544592524335698, -4.483927247898792601, 103.9594237280190185 ) ) ;
#89521=CARTESIAN_POINT ( 'NONE',  ( 16.46253265017160672, -9.564922557960803928, 53.33224293864768839 ) ) ;
#89523=CARTESIAN_POINT ( 'NONE',  ( 21.53943276465977519, 0.05219959533937863772, 106.2510903946856757 ) ) ;
#89524=CARTESIAN_POINT ( 'NONE',  ( 12.06949235617739724, 12.14591786802326823, 21.87609039468567573 ) ) ;
#89525=CARTESIAN_POINT ( 'NONE',  ( -18.67979575497178146, -10.72451020669898902, 41.66557627198103120 ) ) ;
#89526=CARTESIAN_POINT ( 'NONE',  ( -5.823673210054431948, 21.52544592524334988, 92.70942372801901854 ) ) ;
#89528=CARTESIAN_POINT ( 'NONE',  ( 9.564922557960805705, 16.46253265017160317, 99.58224293864770971 ) ) ;
#89529=CARTESIAN_POINT ( 'NONE',  ( 5.049401038298161559, -19.05341960407611168, 87.70724293864769550 ) ) ;
#89531=CARTESIAN_POINT ( 'NONE',  ( 0.05219959533907565091, 21.53943276465977519, 104.9989096053143669 ) ) ;
#89533=CARTESIAN_POINT ( 'NONE',  ( 8.224510206698953496, -14.34966873604960469, 77.91557627198102409 ) ) ;
#89534=CARTESIAN_POINT ( 'NONE',  ( -10.72451020669898014, 18.67979575497178502, 70.41557627198102409 ) ) ;
#89535=CARTESIAN_POINT ( 'NONE',  ( -19.03943276465977164, 0.05219959533909376836, 56.24890960531435979 ) ) ;
#89536=CARTESIAN_POINT ( 'NONE',  ( -21.55341960407610458, -5.719274019375992779, 96.45724293864770971 ) ) ;
#89539=CARTESIAN_POINT ( 'NONE',  ( 5.153800228976335163, 19.02544592524342804, 64.79057627198100988 ) ) ;
#89540=CARTESIAN_POINT ( 'NONE',  ( 4.379528057220339221, -16.55341960407611168, 87.70724293864769550 ) ) ;
#89542=CARTESIAN_POINT ( 'NONE',  ( -16.46253265017160317, 9.564922557960807481, 65.83224293864769550 ) ) ;
#89543=CARTESIAN_POINT ( 'NONE',  ( -13.89961937509957401, -13.97604488694547875, 84.37609039468567573 ) ) ;
#89544=CARTESIAN_POINT ( 'NONE',  ( 8.224510206698953496, -14.34966873604960469, 87.91557627198103830 ) ) ;
#89545=CARTESIAN_POINT ( 'NONE',  ( -10.81492255796105439, 18.62759615963255655, 52.91775706135235424 ) ) ;
#89546=CARTESIAN_POINT ( 'NONE',  ( 16.46253265017160672, -9.564922557960803928, 53.33224293864768839 ) ) ;
#89547=CARTESIAN_POINT ( 'NONE',  ( -18.62759615963255300, -10.81492255796106328, 19.16775706135234714 ) ) ;
#89548=CARTESIAN_POINT ( 'NONE',  ( -16.53943276465976808, 0.05219959533911058130, 106.2489096053143811 ) ) ;
#89550=CARTESIAN_POINT ( 'NONE',  ( -5.153800228976328057, -19.02544592524343514, 62.29057627198100988 ) ) ;
#89552=CARTESIAN_POINT ( 'NONE',  ( 19.05341960407617918, -5.049401038297876454, 111.0427570613523329 ) ) ;
#89553=CARTESIAN_POINT ( 'NONE',  ( -5.049401038298153566, 19.05341960407611168, 115.2072429386477097 ) ) ;
#89554=CARTESIAN_POINT ( 'NONE',  ( 5.823673210054444382, -21.52544592524334988, 50.20942372801901854 ) ) ;
#89555=CARTESIAN_POINT ( 'NONE',  ( -16.51473224551069308, -9.474510206698971260, 101.6655762719810241 ) ) ;
#89556=CARTESIAN_POINT ( 'NONE',  ( 5.153800228976615827, -19.02544592524334988, 80.20942372801901854 ) ) ;
#89557=CARTESIAN_POINT ( 'NONE',  ( 13.97604488694527802, 13.89961937509977652, 64.37390960531436690 ) ) ;
#89558=CARTESIAN_POINT ( 'NONE',  ( 16.53943276465976808, -0.05219959533910856209, 73.74890960531433848 ) ) ;
#89559=CARTESIAN_POINT ( 'NONE',  ( -14.29746914071049879, 8.314922557960819915, 80.83224293864769550 ) ) ;
#89560=CARTESIAN_POINT ( 'NONE',  ( -13.89961937509977652, 13.97604488694528158, 95.62390960531436690 ) ) ;
#89561=CARTESIAN_POINT ( 'NONE',  ( -4.379528057220328563, 16.55341960407611168, 75.20724293864769550 ) ) ;
#89562=CARTESIAN_POINT ( 'NONE',  ( 9.474510206698971260, -16.51473224551069308, 82.91557627198103830 ) ) ;
#89563=CARTESIAN_POINT ( 'NONE',  ( 0.05219959533936267826, -19.03943276465977164, 35.00109039468566863 ) ) ;
#89564=CARTESIAN_POINT ( 'NONE',  ( -16.46253265017160317, 9.564922557960807481, 55.83224293864769550 ) ) ;
#89565=CARTESIAN_POINT ( 'NONE',  ( -0.05219959533910754901, -16.53943276465976808, 32.49890960531435979 ) ) ;
#89566=CARTESIAN_POINT ( 'NONE',  ( 19.02544592524343514, -5.153800228976328945, 28.54057627198102409 ) ) ;
#89568=CARTESIAN_POINT ( 'NONE',  ( 15.80617190586769283, -15.72974639402175789, 50.62609039468568994 ) ) ;
#89569=CARTESIAN_POINT ( 'NONE',  ( 9.564922557961047289, -16.46253265017146816, 85.41775706135233293 ) ) ;
#89570=CARTESIAN_POINT ( 'NONE',  ( 8.224510206698953496, -14.34966873604960469, 37.91557627198102409 ) ) ;
#89571=CARTESIAN_POINT ( 'NONE',  ( -5.823673210054116645, -21.52544592524344225, 92.29057627198103830 ) ) ;
#89572=CARTESIAN_POINT ( 'NONE',  ( -10.72451020669898014, 18.67979575497178502, 30.41557627198101699 ) ) ;
#89573=CARTESIAN_POINT ( 'NONE',  ( 4.483927247898545687, 16.52544592524342804, 64.79057627198103830 ) ) ;
#89574=CARTESIAN_POINT ( 'NONE',  ( 13.97604488694527802, 13.89961937509977652, 44.37390960531435269 ) ) ;
#89575=CARTESIAN_POINT ( 'NONE',  ( -8.224510206698735004, -14.34966873604973081, 104.5844237280190185 ) ) ;
#89576=CARTESIAN_POINT ( 'NONE',  ( 14.29746914071037800, 8.314922557961029526, 66.66775706135234714 ) ) ;
#89577=CARTESIAN_POINT ( 'NONE',  ( 0.05219959533907565091, 21.53943276465977519, 34.99890960531435979 ) ) ;
#89578=CARTESIAN_POINT ( 'NONE',  ( 13.97604488694548053, -13.89961937509957401, 20.62609039468567573 ) ) ;
#89579=CARTESIAN_POINT ( 'NONE',  ( 5.153800228976335163, 19.02544592524342804, 89.79057627198102409 ) ) ;
#89580=CARTESIAN_POINT ( 'NONE',  ( 14.34966873604972726, -8.224510206698740333, 70.83442372801901854 ) ) ;
#89581=CARTESIAN_POINT ( 'NONE',  ( -9.564922557960796823, -16.46253265017161027, 22.08224293864768839 ) ) ;
#89582=CARTESIAN_POINT ( 'NONE',  ( -14.29746914071049879, 8.314922557960819915, 35.83224293864768839 ) ) ;
#89583=CARTESIAN_POINT ( 'NONE',  ( 5.049401038298161559, -19.05341960407611168, 107.7072429386476955 ) ) ;
#89584=CARTESIAN_POINT ( 'NONE',  ( -9.564922557960796823, -16.46253265017161027, 92.08224293864769550 ) ) ;
#89585=CARTESIAN_POINT ( 'NONE',  ( -21.53943276465977519, 0.05219959533907696930, 31.24890960531435979 ) ) ;
#89586=CARTESIAN_POINT ( 'NONE',  ( -4.483927247898539470, -16.52544592524342804, 77.29057627198102409 ) ) ;
#89588=CARTESIAN_POINT ( 'NONE',  ( 12.06949235617757843, -12.14591786802309237, 53.12390960531436690 ) ) ;
#89589=CARTESIAN_POINT ( 'NONE',  ( -8.314922557961024197, 14.29746914071037800, 57.91775706135234714 ) ) ;
#89591=CARTESIAN_POINT ( 'NONE',  ( -19.05341960407617563, 5.049401038297882671, 53.54275706135231871 ) ) ;
#89592=CARTESIAN_POINT ( 'NONE',  ( 13.97604488694527802, 13.89961937509977652, 94.37390960531436690 ) ) ;
#89593=CARTESIAN_POINT ( 'NONE',  ( -19.03943276465977164, -0.05219959533935918106, 68.75109039468566152 ) ) ;
#89595=CARTESIAN_POINT ( 'NONE',  ( 19.03943276465977164, 0.05219959533936151252, 111.2510903946856757 ) ) ;
#89596=CARTESIAN_POINT ( 'NONE',  ( 14.34966873604972726, -8.224510206698740333, 90.83442372801901854 ) ) ;
#89597=CARTESIAN_POINT ( 'NONE',  ( 19.02544592524343514, -5.153800228976328945, 33.54057627198102409 ) ) ;
#89598=CARTESIAN_POINT ( 'NONE',  ( 16.51473224551069308, 9.474510206698969483, 114.1655762719810241 ) ) ;
#89599=CARTESIAN_POINT ( 'NONE',  ( -5.823673210054431948, 21.52544592524334988, 52.70942372801902565 ) ) ;
#89600=CARTESIAN_POINT ( 'NONE',  ( -13.89961937509957401, -13.97604488694547875, 99.37609039468567573 ) ) ;
#89601=CARTESIAN_POINT ( 'NONE',  ( 17.50000000000000711, 4.034393320798373317, 22.04839310049790413 ) ) ;
#89602=CARTESIAN_POINT ( 'NONE',  ( -19.05341960407611168, -5.049401038298163336, 71.45724293864766707 ) ) ;
#89604=CARTESIAN_POINT ( 'NONE',  ( -12.14591786802309592, -12.06949235617757132, 76.87390960531439532 ) ) ;
#89605=CARTESIAN_POINT ( 'NONE',  ( 0.05219959533909260263, 19.03943276465977164, 64.99890960531436690 ) ) ;
#89606=CARTESIAN_POINT ( 'NONE',  ( 5.153800228976335163, 19.02544592524342804, 79.79057627198102409 ) ) ;
#89607=CARTESIAN_POINT ( 'NONE',  ( -5.153800228976607833, 19.02544592524334988, 72.70942372801900433 ) ) ;
#89608=CARTESIAN_POINT ( 'NONE',  ( 21.52544592524344225, -5.823673210054117533, 68.54057627198103830 ) ) ;
#89609=CARTESIAN_POINT ( 'NONE',  ( -12.14591786802309592, -12.06949235617757132, 111.8739096053143669 ) ) ;
#89610=CARTESIAN_POINT ( 'NONE',  ( -0.05219959533936034679, 19.03943276465977164, 52.50109039468566863 ) ) ;
#89611=CARTESIAN_POINT ( 'NONE',  ( 19.02544592524343514, -5.153800228976328945, 58.54057627198102409 ) ) ;
#89612=CARTESIAN_POINT ( 'NONE',  ( -13.89961937509977652, 13.97604488694528158, 95.62390960531436690 ) ) ;
#89613=CARTESIAN_POINT ( 'NONE',  ( 0.05219959533907565091, 21.53943276465977519, 94.99890960531436690 ) ) ;
#89614=CARTESIAN_POINT ( 'NONE',  ( 4.483927247898545687, 16.52544592524342804, 84.79057627198102409 ) ) ;
#89615=CARTESIAN_POINT ( 'NONE',  ( -13.97604488694547697, 13.89961937509957934, 43.12609039468566152 ) ) ;
#89616=CARTESIAN_POINT ( 'NONE',  ( 5.719274019375991003, -21.55341960407610458, 82.70724293864770971 ) ) ;
#89617=CARTESIAN_POINT ( 'NONE',  ( -21.53943276465977519, 0.05219959533907696930, 61.24890960531435979 ) ) ;
#89618=CARTESIAN_POINT ( 'NONE',  ( 4.379528057220339221, -16.55341960407611168, 27.70724293864769905 ) ) ;
#89619=CARTESIAN_POINT ( 'NONE',  ( -21.52544592524334988, -5.823673210054445271, 93.95942372801903275 ) ) ;
#89620=CARTESIAN_POINT ( 'NONE',  ( 9.474510206698971260, -16.51473224551069308, 82.91557627198103830 ) ) ;
#89621=CARTESIAN_POINT ( 'NONE',  ( 13.97604488694527802, 13.89961937509977652, 34.37390960531436690 ) ) ;
#89623=CARTESIAN_POINT ( 'NONE',  ( 21.53943276465977519, 0.05219959533937863772, 41.25109039468568284 ) ) ;
#89624=CARTESIAN_POINT ( 'NONE',  ( 21.52544592524334988, 5.823673210054432836, 46.45942372801901854 ) ) ;
#89625=CARTESIAN_POINT ( 'NONE',  ( -16.51473224551069308, -9.474510206698971260, 51.66557627198102409 ) ) ;
#89626=CARTESIAN_POINT ( 'NONE',  ( 15.72974639402176855, 15.80617190586768217, 21.87609039468567573 ) ) ;
#89627=CARTESIAN_POINT ( 'NONE',  ( 13.89961937509957401, 13.97604488694547697, 66.87609039468567573 ) ) ;
#89628=CARTESIAN_POINT ( 'NONE',  ( 9.474510206698971260, -16.51473224551069308, 42.91557627198103120 ) ) ;
#89629=CARTESIAN_POINT ( 'NONE',  ( -4.483927247898782831, 16.52544592524335698, 22.70942372801901499 ) ) ;
#89631=CARTESIAN_POINT ( 'NONE',  ( -16.52544592524335698, -4.483927247898792601, 68.95942372801901854 ) ) ;
#89632=CARTESIAN_POINT ( 'NONE',  ( 13.97604488694527802, 13.89961937509977652, 39.37390960531435269 ) ) ;
#89634=CARTESIAN_POINT ( 'NONE',  ( -13.89961937509977652, 13.97604488694528158, 90.62390960531432427 ) ) ;
#89635=CARTESIAN_POINT ( 'NONE',  ( -19.03943276465977164, 0.05219959533909376836, 31.24890960531435979 ) ) ;
#89636=CARTESIAN_POINT ( 'NONE',  ( 5.823673210054125526, 21.52544592524343514, 59.79057627198103120 ) ) ;
#89637=CARTESIAN_POINT ( 'NONE',  ( 8.224510206698742110, 14.34966873604972548, 42.08442372801901854 ) ) ;
#89638=CARTESIAN_POINT ( 'NONE',  ( -5.719274019375665041, -21.55341960407619695, 94.79275706135234714 ) ) ;
#89640=CARTESIAN_POINT ( 'NONE',  ( 13.97604488694527802, 13.89961937509977652, 44.37390960531435269 ) ) ;
#89641=CARTESIAN_POINT ( 'NONE',  ( -16.52544592524342804, 4.483927247898546575, 36.04057627198102409 ) ) ;
#89642=CARTESIAN_POINT ( 'NONE',  ( 16.53943276465976808, -0.05219959533910856209, 68.74890960531435269 ) ) ;
#89643=CARTESIAN_POINT ( 'NONE',  ( 16.51473224551069308, 9.474510206698969483, 69.16557627198102409 ) ) ;
#89644=CARTESIAN_POINT ( 'NONE',  ( -15.72974639402176322, -15.80617190586768395, 109.3760903946857042 ) ) ;
#89645=CARTESIAN_POINT ( 'NONE',  ( -18.62759615963255300, -10.81492255796106328, 24.16775706135235424 ) ) ;
#89646=CARTESIAN_POINT ( 'NONE',  ( 13.97604488694527802, 13.89961937509977652, 84.37390960531433848 ) ) ;
#89647=CARTESIAN_POINT ( 'NONE',  ( 0.05219959533937995610, -21.53943276465977519, 85.00109039468568994 ) ) ;
#89648=CARTESIAN_POINT ( 'NONE',  ( 12.06949235617739724, 12.14591786802326823, 51.87609039468568284 ) ) ;
#89649=CARTESIAN_POINT ( 'NONE',  ( -14.29746914071037622, -8.314922557961029526, 29.16775706135234003 ) ) ;
#89650=CARTESIAN_POINT ( 'NONE',  ( -12.14591786802309592, -12.06949235617757132, 86.87390960531438111 ) ) ;
#89651=CARTESIAN_POINT ( 'NONE',  ( -5.719274019375665041, -21.55341960407619695, 99.79275706135234714 ) ) ;
#89654=CARTESIAN_POINT ( 'NONE',  ( -16.55341960407611168, -4.379528057220339221, 36.45724293864768839 ) ) ;
#89655=CARTESIAN_POINT ( 'NONE',  ( 9.564922557960805705, 16.46253265017160317, 24.58224293864769194 ) ) ;
#89656=CARTESIAN_POINT ( 'NONE',  ( -8.224510206698735004, -14.34966873604973081, 49.58442372801901143 ) ) ;
#89657=CARTESIAN_POINT ( 'NONE',  ( -4.483927247898539470, -16.52544592524342804, 57.29057627198103120 ) ) ;
#89658=CARTESIAN_POINT ( 'NONE',  ( 14.29746914071037800, 8.314922557961029526, 96.66775706135234714 ) ) ;
#89659=CARTESIAN_POINT ( 'NONE',  ( 0.05219959533909260263, 19.03943276465977164, 114.9989096053143669 ) ) ;
#89660=CARTESIAN_POINT ( 'NONE',  ( 21.53943276465977519, -0.05219959533907433946, 23.74890960531435269 ) ) ;
#89661=CARTESIAN_POINT ( 'NONE',  ( 21.52544592524334988, 5.823673210054432836, 111.4594237280190328 ) ) ;
#89662=CARTESIAN_POINT ( 'NONE',  ( -0.05219959533910754901, -16.53943276465976808, 92.49890960531436690 ) ) ;
#89663=CARTESIAN_POINT ( 'NONE',  ( -19.03943276465977164, 0.05219959533909376836, 101.2489096053143669 ) ) ;
#89665=CARTESIAN_POINT ( 'NONE',  ( -16.53943276465976808, -0.05219959533934237506, 33.75109039468568284 ) ) ;
#89666=CARTESIAN_POINT ( 'NONE',  ( 5.049401038298161559, -19.05341960407611168, 37.70724293864768839 ) ) ;
#89667=CARTESIAN_POINT ( 'NONE',  ( 12.14591786802327356, -12.06949235617739191, 45.62609039468567573 ) ) ;
#89668=CARTESIAN_POINT ( 'NONE',  ( -5.049401038297874678, -19.05341960407617918, 44.79275706135232582 ) ) ;
#89669=CARTESIAN_POINT ( 'NONE',  ( -9.564922557960796823, -16.46253265017161027, 47.08224293864769550 ) ) ;
#89670=CARTESIAN_POINT ( 'NONE',  ( 12.14591786802327356, -12.06949235617739191, 85.62609039468568994 ) ) ;
#89671=CARTESIAN_POINT ( 'NONE',  ( 19.02544592524334988, 5.153800228976608722, 76.45942372801897591 ) ) ;
#89672=CARTESIAN_POINT ( 'NONE',  ( 5.153800228976615827, -19.02544592524334988, 25.20942372801900433 ) ) ;
#89673=CARTESIAN_POINT ( 'NONE',  ( 13.89961937509977652, -13.97604488694527269, 58.12390960531436690 ) ) ;
#89674=CARTESIAN_POINT ( 'NONE',  ( -16.52544592524342804, 4.483927247898546575, 96.04057627198102409 ) ) ;
#89676=CARTESIAN_POINT ( 'NONE',  ( 16.46253265017146816, 9.564922557961045513, 66.66775706135233293 ) ) ;
#89677=CARTESIAN_POINT ( 'NONE',  ( -21.55341960407610458, -5.719274019375992779, 66.45724293864768129 ) ) ;
#89678=CARTESIAN_POINT ( 'NONE',  ( -0.05219959533936034679, 19.03943276465977164, 22.50109039468566152 ) ) ;
#89679=CARTESIAN_POINT ( 'NONE',  ( 16.46253265017160672, -9.564922557960803928, 98.33224293864769550 ) ) ;
#89681=CARTESIAN_POINT ( 'NONE',  ( -21.52544592524343514, 5.823673210054127303, 81.04057627198102409 ) ) ;
#89683=CARTESIAN_POINT ( 'NONE',  ( 9.474510206698729675, 16.51473224551082808, 107.0844237280190043 ) ) ;
#89685=CARTESIAN_POINT ( 'NONE',  ( -12.14591786802326823, 12.06949235617739902, 33.12609039468569705 ) ) ;
#89686=CARTESIAN_POINT ( 'NONE',  ( 19.02544592524343514, -5.153800228976328945, 38.54057627198103120 ) ) ;
#89687=CARTESIAN_POINT ( 'NONE',  ( -9.474510206698964154, 16.51473224551069663, 105.4155762719810383 ) ) ;
#89688=CARTESIAN_POINT ( 'NONE',  ( 10.81492255796078972, 18.62759615963270932, 89.58224293864768129 ) ) ;
#89689=CARTESIAN_POINT ( 'NONE',  ( 15.72974639402176855, 15.80617190586768217, 56.87609039468568994 ) ) ;
#89690=CARTESIAN_POINT ( 'NONE',  ( -19.02544592524334988, -5.153800228976617603, 108.9594237280189759 ) ) ;
#89691=CARTESIAN_POINT ( 'NONE',  ( 9.564922557961047289, -16.46253265017146816, 20.41775706135233293 ) ) ;
#89692=CARTESIAN_POINT ( 'NONE',  ( 4.379528057220092307, 16.55341960407617563, 107.2927570613523471 ) ) ;
#89693=CARTESIAN_POINT ( 'NONE',  ( 5.823673210054125526, 21.52544592524343514, 104.7905762719810241 ) ) ;
#89694=CARTESIAN_POINT ( 'NONE',  ( 16.55341960407611168, 4.379528057220329451, 43.95724293864769550 ) ) ;
#89695=CARTESIAN_POINT ( 'NONE',  ( 9.474510206698729675, 16.51473224551082808, 77.08442372801900433 ) ) ;
#89696=CARTESIAN_POINT ( 'NONE',  ( -13.89961937509957401, -13.97604488694547875, 59.37609039468566863 ) ) ;
#89697=CARTESIAN_POINT ( 'NONE',  ( -15.80617190586768217, 15.72974639402176855, 68.12609039468567573 ) ) ;
#89698=CARTESIAN_POINT ( 'NONE',  ( 13.97604488694548053, -13.89961937509957401, 35.62609039468567573 ) ) ;
#89699=CARTESIAN_POINT ( 'NONE',  ( 16.53943276465976808, -0.05219959533910856209, 108.7489096053143669 ) ) ;
#89700=CARTESIAN_POINT ( 'NONE',  ( 0.05219959533907565091, 21.53943276465977519, 39.99890960531436690 ) ) ;
#89701=CARTESIAN_POINT ( 'NONE',  ( 4.379528057220339221, -16.55341960407611168, 37.70724293864769550 ) ) ;
#89702=CARTESIAN_POINT ( 'NONE',  ( -18.62759615963255300, -10.81492255796106328, 94.16775706135237556 ) ) ;
#89703=CARTESIAN_POINT ( 'NONE',  ( -16.55341960407617563, 4.379528057220093196, 68.54275706135234714 ) ) ;
#89704=CARTESIAN_POINT ( 'NONE',  ( 4.379528057220339221, -16.55341960407611168, 22.70724293864769194 ) ) ;
#89705=CARTESIAN_POINT ( 'NONE',  ( -15.80617190586768217, 15.72974639402176855, 58.12609039468568994 ) ) ;
#89706=CARTESIAN_POINT ( 'NONE',  ( 15.72974639402176855, 15.80617190586768217, 66.87609039468568994 ) ) ;
#89707=CARTESIAN_POINT ( 'NONE',  ( 15.80617190586746368, 15.72974639402197994, 64.37390960531435269 ) ) ;
#89710=CARTESIAN_POINT ( 'NONE',  ( -9.474510206698964154, 16.51473224551069663, 30.41557627198102054 ) ) ;
#89711=CARTESIAN_POINT ( 'NONE',  ( -21.53943276465977519, -0.05219959533937600094, 48.75109039468568284 ) ) ;
#89712=CARTESIAN_POINT ( 'NONE',  ( 16.51473224551069308, 9.474510206698969483, 24.16557627198102765 ) ) ;
#89713=CARTESIAN_POINT ( 'NONE',  ( 16.51473224551069308, 9.474510206698969483, 34.16557627198102409 ) ) ;
#89714=CARTESIAN_POINT ( 'NONE',  ( 16.52544592524342804, -4.483927247898539470, 73.54057627198102409 ) ) ;
#89715=CARTESIAN_POINT ( 'NONE',  ( 19.05341960407611168, 5.049401038298154454, 83.95724293864766707 ) ) ;
#89716=CARTESIAN_POINT ( 'NONE',  ( -16.55341960407611168, -4.379528057220339221, 21.45724293864769550 ) ) ;
#89717=CARTESIAN_POINT ( 'NONE',  ( 16.53943276465976808, -0.05219959533910856209, 98.74890960531438111 ) ) ;
#89718=CARTESIAN_POINT ( 'NONE',  ( 21.55341960407610458, 5.719274019375980345, 73.95724293864769550 ) ) ;
#89719=CARTESIAN_POINT ( 'NONE',  ( -15.72974639402197994, 15.80617190586746368, 100.6239096053143811 ) ) ;
#89721=CARTESIAN_POINT ( 'NONE',  ( -9.474510206698964154, 16.51473224551069663, 70.41557627198102409 ) ) ;
#89722=CARTESIAN_POINT ( 'NONE',  ( 4.483927247898790824, -16.52544592524335698, 30.20942372801902565 ) ) ;
#89723=CARTESIAN_POINT ( 'NONE',  ( -10.81492255796078084, -18.62759615963271287, 62.08224293864769550 ) ) ;
#89724=CARTESIAN_POINT ( 'NONE',  ( 5.719274019375673035, 21.55341960407619339, 77.29275706135234714 ) ) ;
#89725=CARTESIAN_POINT ( 'NONE',  ( 13.97604488694527802, 13.89961937509977652, 69.37390960531436690 ) ) ;
#89726=CARTESIAN_POINT ( 'NONE',  ( -16.51473224551069308, -9.474510206698971260, 101.6655762719810241 ) ) ;
#89727=CARTESIAN_POINT ( 'NONE',  ( -4.483927247898782831, 16.52544592524335698, 72.70942372801901854 ) ) ;
#89728=CARTESIAN_POINT ( 'NONE',  ( -21.53943276465977519, -0.05219959533937600094, 63.75109039468568284 ) ) ;
#89729=CARTESIAN_POINT ( 'NONE',  ( 21.52544592524334988, 5.823673210054432836, 96.45942372801901854 ) ) ;
#89730=CARTESIAN_POINT ( 'NONE',  ( 0.05219959533937995610, -21.53943276465977519, 20.00109039468568639 ) ) ;
#89731=CARTESIAN_POINT ( 'NONE',  ( -9.564922557960796823, -16.46253265017161027, 22.08224293864768839 ) ) ;
#89732=CARTESIAN_POINT ( 'NONE',  ( -5.823673210054116645, -21.52544592524344225, 87.29057627198103830 ) ) ;
#89733=CARTESIAN_POINT ( 'NONE',  ( -16.46253265017146816, -9.564922557961047289, 44.16775706135232582 ) ) ;
#89734=CARTESIAN_POINT ( 'NONE',  ( 18.62759615963271287, -10.81492255796078972, 38.33224293864768839 ) ) ;
#89735=CARTESIAN_POINT ( 'NONE',  ( 9.474510206698971260, -16.51473224551069308, 77.91557627198103830 ) ) ;
#89736=CARTESIAN_POINT ( 'NONE',  ( -12.14591786802309592, -12.06949235617757132, 31.87390960531435979 ) ) ;
#89737=CARTESIAN_POINT ( 'NONE',  ( -17.49999999999998934, 5.624438216177590988, 65.81670344914645909 ) ) ;
#89739=CARTESIAN_POINT ( 'NONE',  ( 16.46253265017146816, 9.564922557961045513, 101.6677570613523329 ) ) ;
#89740=CARTESIAN_POINT ( 'NONE',  ( -10.81492255796078084, -18.62759615963271287, 67.08224293864770971 ) ) ;
#89741=CARTESIAN_POINT ( 'NONE',  ( 12.06949235617757843, -12.14591786802309237, 48.12390960531436690 ) ) ;
#89742=CARTESIAN_POINT ( 'NONE',  ( -12.06949235617739369, -12.14591786802326823, 29.37609039468568284 ) ) ;
#89743=CARTESIAN_POINT ( 'NONE',  ( 16.51473224551069308, 9.474510206698969483, 44.16557627198103120 ) ) ;
#89744=CARTESIAN_POINT ( 'NONE',  ( 21.52544592524344225, -5.823673210054117533, 108.5405762719810241 ) ) ;
#89745=CARTESIAN_POINT ( 'NONE',  ( -13.97604488694547697, 13.89961937509957934, 88.12609039468563310 ) ) ;
#89746=CARTESIAN_POINT ( 'NONE',  ( -19.03943276465977164, 0.05219959533909376836, 76.24890960531435269 ) ) ;
#89747=CARTESIAN_POINT ( 'NONE',  ( 14.29746914071049879, -8.314922557960816363, 93.33224293864769550 ) ) ;
#89748=CARTESIAN_POINT ( 'NONE',  ( 9.564922557960805705, 16.46253265017160317, 79.58224293864769550 ) ) ;
#89749=CARTESIAN_POINT ( 'NONE',  ( 0.05219959533907565091, 21.53943276465977519, 74.99890960531435269 ) ) ;
#89750=CARTESIAN_POINT ( 'NONE',  ( -5.153800228976328057, -19.02544592524343514, 32.29057627198102409 ) ) ;
#89752=CARTESIAN_POINT ( 'NONE',  ( 14.34966873604960469, 8.224510206698951720, 59.16557627198103120 ) ) ;
#89753=CARTESIAN_POINT ( 'NONE',  ( -5.049401038298153566, 19.05341960407611168, 90.20724293864766707 ) ) ;
#89755=CARTESIAN_POINT ( 'NONE',  ( -0.05219959533936034679, 19.03943276465977164, 57.50109039468566863 ) ) ;
#89756=CARTESIAN_POINT ( 'NONE',  ( 14.29746914071037800, 8.314922557961029526, 66.66775706135234714 ) ) ;
#89757=CARTESIAN_POINT ( 'NONE',  ( 10.81492255796078972, 18.62759615963270932, 74.58224293864768129 ) ) ;
#89758=CARTESIAN_POINT ( 'NONE',  ( -16.51473224551082808, 9.474510206698731452, 38.33442372801899722 ) ) ;
#89759=CARTESIAN_POINT ( 'NONE',  ( 19.03943276465977164, -0.05219959533909143690, 88.74890960531436690 ) ) ;
#89761=CARTESIAN_POINT ( 'NONE',  ( -18.62759615963270932, 10.81492255796079327, 30.83224293864770260 ) ) ;
#89763=CARTESIAN_POINT ( 'NONE',  ( 9.474510206698971260, -16.51473224551069308, 72.91557627198102409 ) ) ;
#89764=CARTESIAN_POINT ( 'NONE',  ( 21.53943276465977519, 0.05219959533937863772, 46.25109039468567573 ) ) ;
#89765=CARTESIAN_POINT ( 'NONE',  ( -19.02544592524342804, 5.153800228976336051, 26.04057627198103120 ) ) ;
#89766=CARTESIAN_POINT ( 'NONE',  ( 10.72451020669871369, 18.67979575497193778, 22.08442372801901143 ) ) ;
#89767=CARTESIAN_POINT ( 'NONE',  ( -16.51473224551069308, -9.474510206698971260, 91.66557627198103830 ) ) ;
#89769=CARTESIAN_POINT ( 'NONE',  ( 10.81492255796106328, -18.62759615963255655, 40.41775706135234714 ) ) ;
#89771=CARTESIAN_POINT ( 'NONE',  ( -16.46253265017160317, 9.564922557960807481, 105.8322429386476955 ) ) ;
#89773=CARTESIAN_POINT ( 'NONE',  ( -5.719274019375978568, 21.55341960407610458, 110.2072429386477239 ) ) ;
#89774=CARTESIAN_POINT ( 'NONE',  ( -9.474510206698964154, 16.51473224551069663, 40.41557627198103120 ) ) ;
#89775=CARTESIAN_POINT ( 'NONE',  ( -12.06949235617739369, -12.14591786802326823, 29.37609039468568284 ) ) ;
#89777=CARTESIAN_POINT ( 'NONE',  ( 10.72451020669871369, 18.67979575497193778, 107.0844237280190043 ) ) ;
#89778=CARTESIAN_POINT ( 'NONE',  ( 0.05219959533909260263, 19.03943276465977164, 39.99890960531436690 ) ) ;
#89779=CARTESIAN_POINT ( 'NONE',  ( -21.55341960407619339, 5.719274019375674811, 93.54275706135234714 ) ) ;
#89780=CARTESIAN_POINT ( 'NONE',  ( -16.51473224551069308, -9.474510206698971260, 86.66557627198102409 ) ) ;
#89781=CARTESIAN_POINT ( 'NONE',  ( -21.52544592524334988, -5.823673210054445271, 63.95942372801901854 ) ) ;
#89783=CARTESIAN_POINT ( 'NONE',  ( -5.049401038298153566, 19.05341960407611168, 105.2072429386476671 ) ) ;
#89784=DIRECTION ( 'NONE',  ( 0.000000000000000000, 0.000000000000000000, 1.000000000000000000 ) ) ;
#89785=CARTESIAN_POINT ( 'NONE',  ( -8.314922557961024197, 14.29746914071037800, 57.91775706135234714 ) ) ;
#89786=CARTESIAN_POINT ( 'NONE',  ( -8.314922557961024197, 14.29746914071037800, 67.91775706135234714 ) ) ;
#89787=CARTESIAN_POINT ( 'NONE',  ( 18.62759615963255655, 10.81492255796105972, 56.66775706135235424 ) ) ;
#89788=CARTESIAN_POINT ( 'NONE',  ( -5.719274019375665041, -21.55341960407619695, 94.79275706135234714 ) ) ;
#89790=CARTESIAN_POINT ( 'NONE',  ( 4.483927247898790824, -16.52544592524335698, 25.20942372801901854 ) ) ;
#89791=CARTESIAN_POINT ( 'NONE',  ( 0.05219959533909260263, 19.03943276465977164, 79.99890960531436690 ) ) ;
#89792=CARTESIAN_POINT ( 'NONE',  ( -16.51473224551069308, -9.474510206698971260, 96.66557627198102409 ) ) ;
#89794=CARTESIAN_POINT ( 'NONE',  ( -16.51473224551069308, -9.474510206698971260, 111.6655762719810383 ) ) ;
#89795=CARTESIAN_POINT ( 'NONE',  ( -5.153800228976328057, -19.02544592524343514, 32.29057627198102409 ) ) ;
#89796=CARTESIAN_POINT ( 'NONE',  ( -10.81492255796078084, -18.62759615963271287, 27.08224293864769550 ) ) ;
#89798=CARTESIAN_POINT ( 'NONE',  ( 4.483927247898790824, -16.52544592524335698, 95.20942372801903275 ) ) ;
#89799=CARTESIAN_POINT ( 'NONE',  ( -16.52544592524342804, 4.483927247898546575, 81.04057627198102409 ) ) ;
#89800=CARTESIAN_POINT ( 'NONE',  ( 19.05341960407611168, 5.049401038298154454, 68.95724293864769550 ) ) ;
#89801=CARTESIAN_POINT ( 'NONE',  ( -18.67979575497193778, 10.72451020669871902, 88.33442372801901854 ) ) ;
#89803=CARTESIAN_POINT ( 'NONE',  ( -16.55341960407617563, 4.379528057220093196, 28.54275706135234358 ) ) ;
#89804=CARTESIAN_POINT ( 'NONE',  ( 4.483927247898545687, 16.52544592524342804, 69.79057627198102409 ) ) ;
#89805=CARTESIAN_POINT ( 'NONE',  ( -5.823673210054431948, 21.52544592524334988, 32.70942372801900433 ) ) ;
#89806=CARTESIAN_POINT ( 'NONE',  ( 21.52544592524344225, -5.823673210054117533, 78.54057627198103830 ) ) ;
#89807=CARTESIAN_POINT ( 'NONE',  ( -0.05219959533936034679, 19.03943276465977164, 37.50109039468567573 ) ) ;
#89808=CARTESIAN_POINT ( 'NONE',  ( -18.22780087662119897, 5.500000000000102141, 46.01763182126894947 ) ) ;
#89809=CARTESIAN_POINT ( 'NONE',  ( 19.02544592524343514, -5.153800228976328945, 83.54057627198100988 ) ) ;
#89810=CARTESIAN_POINT ( 'NONE',  ( 12.14591786802309770, 12.06949235617756955, 44.37390960531435979 ) ) ;
#89812=CARTESIAN_POINT ( 'NONE',  ( -16.53943276465976808, 0.05219959533911058130, 31.24890960531435979 ) ) ;
#89813=CARTESIAN_POINT ( 'NONE',  ( -8.224510206698735004, -14.34966873604973081, 109.5844237280190328 ) ) ;
#89814=CARTESIAN_POINT ( 'NONE',  ( 19.05341960407617918, -5.049401038297876454, 71.04275706135234714 ) ) ;
#89816=CARTESIAN_POINT ( 'NONE',  ( 5.153800228976335163, 19.02544592524342804, 114.7905762719810241 ) ) ;
#89817=CARTESIAN_POINT ( 'NONE',  ( -16.52544592524342804, 4.483927247898546575, 71.04057627198103830 ) ) ;
#89818=CARTESIAN_POINT ( 'NONE',  ( -17.72696623605163424, 5.499999999999873879, 58.59811031808418846 ) ) ;
#89819=CARTESIAN_POINT ( 'NONE',  ( 9.474510206698971260, -16.51473224551069308, 27.91557627198103120 ) ) ;
#89820=CARTESIAN_POINT ( 'NONE',  ( -21.52544592524343514, 5.823673210054127303, 31.04057627198102409 ) ) ;
#89821=CARTESIAN_POINT ( 'NONE',  ( -18.62759615963270932, 10.81492255796079327, 65.83224293864769550 ) ) ;
#89822=CARTESIAN_POINT ( 'NONE',  ( -16.52544592524342804, 4.483927247898546575, 111.0405762719810525 ) ) ;
#89823=CARTESIAN_POINT ( 'NONE',  ( 16.53943276465976808, 0.05219959533934440121, 66.25109039468567573 ) ) ;
#89824=CARTESIAN_POINT ( 'NONE',  ( -13.97604488694527625, -13.89961937509977652, 46.87390960531435979 ) ) ;
#89825=CARTESIAN_POINT ( 'NONE',  ( -5.719274019375665041, -21.55341960407619695, 54.79275706135235424 ) ) ;
#89827=CARTESIAN_POINT ( 'NONE',  ( -12.06949235617756955, 12.14591786802309770, 100.6239096053143811 ) ) ;
#89828=CARTESIAN_POINT ( 'NONE',  ( 17.50000000000000000, -5.499999999999992895, 36.21769037696435589 ) ) ;
#89831=CARTESIAN_POINT ( 'NONE',  ( -10.81492255796078084, -18.62759615963271287, 37.08224293864768129 ) ) ;
#89833=CARTESIAN_POINT ( 'NONE',  ( -18.62759615963255300, -10.81492255796106328, 69.16775706135234714 ) ) ;
#89834=CARTESIAN_POINT ( 'NONE',  ( -8.224510206698735004, -14.34966873604973081, 54.58442372801901143 ) ) ;
#89835=CARTESIAN_POINT ( 'NONE',  ( 4.379528057220339221, -16.55341960407611168, 47.70724293864770260 ) ) ;
#89836=CARTESIAN_POINT ( 'NONE',  ( 21.52544592524344225, -5.823673210054117533, 63.54057627198103830 ) ) ;
#89837=CARTESIAN_POINT ( 'NONE',  ( -5.719274019375978568, 21.55341960407610458, 60.20724293864768839 ) ) ;
#89839=CARTESIAN_POINT ( 'NONE',  ( 13.97604488694548053, -13.89961937509957401, 80.62609039468567573 ) ) ;
#89840=CARTESIAN_POINT ( 'NONE',  ( -19.02544592524342804, 5.153800228976336051, 111.0405762719810099 ) ) ;
#89841=CARTESIAN_POINT ( 'NONE',  ( 0.05219959533909260263, 19.03943276465977164, 49.99890960531435979 ) ) ;
#89842=CARTESIAN_POINT ( 'NONE',  ( 5.049401038298161559, -19.05341960407611168, 22.70724293864769194 ) ) ;
#89843=FACE_BOUND ( 'NONE', #47936, .T. ) ;
#89845=CARTESIAN_POINT ( 'NONE',  ( -12.06949235617739369, -12.14591786802326823, 64.37609039468568994 ) ) ;
#89846=CARTESIAN_POINT ( 'NONE',  ( -5.823673210054116645, -21.52544592524344225, 102.2905762719810383 ) ) ;
#89847=CARTESIAN_POINT ( 'NONE',  ( -19.05341960407611168, -5.049401038298163336, 61.45724293864769550 ) ) ;
#89848=CARTESIAN_POINT ( 'NONE',  ( 15.72974639402176855, 15.80617190586768217, 41.87609039468568284 ) ) ;
#89849=CARTESIAN_POINT ( 'NONE',  ( 19.03943276465977164, -0.05219959533909143690, 98.74890960531436690 ) ) ;
#89852=CARTESIAN_POINT ( 'NONE',  ( -18.62759615963255300, -10.81492255796106328, 34.16775706135234714 ) ) ;
#89853=CARTESIAN_POINT ( 'NONE',  ( -16.46253265017160317, 9.564922557960807481, 110.8322429386476955 ) ) ;
#89854=CARTESIAN_POINT ( 'NONE',  ( -0.05219959533936034679, 19.03943276465977164, 82.50109039468567573 ) ) ;
#89855=CARTESIAN_POINT ( 'NONE',  ( 9.564922557961047289, -16.46253265017146816, 45.41775706135232582 ) ) ;
#89856=CARTESIAN_POINT ( 'NONE',  ( -21.52544592524343514, 5.823673210054127303, 96.04057627198102409 ) ) ;
#89857=CARTESIAN_POINT ( 'NONE',  ( -5.049401038297874678, -19.05341960407617918, 29.79275706135232227 ) ) ;
#89858=CARTESIAN_POINT ( 'NONE',  ( -13.89961937509957401, -13.97604488694547875, 44.37609039468566863 ) ) ;
#89859=CARTESIAN_POINT ( 'NONE',  ( 8.224510206698742110, 14.34966873604972548, 97.08442372801904696 ) ) ;
#89862=CARTESIAN_POINT ( 'NONE',  ( -16.46253265017160317, 9.564922557960807481, 70.83224293864770971 ) ) ;
#89863=CARTESIAN_POINT ( 'NONE',  ( 21.55341960407619695, -5.719274019375665929, 76.04275706135237556 ) ) ;
#89864=CARTESIAN_POINT ( 'NONE',  ( 21.55341960407619695, -5.719274019375665929, 76.04275706135237556 ) ) ;
#89865=CARTESIAN_POINT ( 'NONE',  ( -17.72560187377285246, -5.500000000000057732, 54.07814504131319921 ) ) ;
#89866=CARTESIAN_POINT ( 'NONE',  ( -16.51473224551069308, -9.474510206698971260, 91.66557627198103830 ) ) ;
#89867=CARTESIAN_POINT ( 'NONE',  ( 21.53943276465977519, 0.05219959533937863772, 66.25109039468567573 ) ) ;
#89868=CARTESIAN_POINT ( 'NONE',  ( -0.05219959533936034679, 19.03943276465977164, 107.5010903946856615 ) ) ;
#89869=CARTESIAN_POINT ( 'NONE',  ( -9.474510206698964154, 16.51473224551069663, 65.41557627198102409 ) ) ;
#89870=CARTESIAN_POINT ( 'NONE',  ( 9.474510206698971260, -16.51473224551069308, 107.9155762719810383 ) ) ;
#89871=CARTESIAN_POINT ( 'NONE',  ( -16.51473224551069308, -9.474510206698971260, 76.66557627198103830 ) ) ;
#89872=CARTESIAN_POINT ( 'NONE',  ( 17.50000000000003197, -3.228180402290367290, 22.22094556969252466 ) ) ;
#89873=CARTESIAN_POINT ( 'NONE',  ( -19.03943276465977164, 0.05219959533909376836, 71.24890960531435269 ) ) ;
#89874=CARTESIAN_POINT ( 'NONE',  ( -9.474510206698964154, 16.51473224551069663, 55.41557627198103120 ) ) ;
#89875=CARTESIAN_POINT ( 'NONE',  ( 15.80617190586746368, 15.72974639402197994, 109.3739096053143811 ) ) ;
#89876=CARTESIAN_POINT ( 'NONE',  ( -16.53943276465976808, -0.05219959533934237506, 88.75109039468567573 ) ) ;
#89878=CARTESIAN_POINT ( 'NONE',  ( 9.564922557961047289, -16.46253265017146816, 45.41775706135232582 ) ) ;
#89879=CARTESIAN_POINT ( 'NONE',  ( 16.46253265017160672, -9.564922557960803928, 78.33224293864769550 ) ) ;
#89880=CARTESIAN_POINT ( 'NONE',  ( -14.29746914071049879, 8.314922557960819915, 70.83224293864770971 ) ) ;
#89881=CARTESIAN_POINT ( 'NONE',  ( 16.53943276465976808, -0.05219959533910856209, 103.7489096053143669 ) ) ;
#89882=CARTESIAN_POINT ( 'NONE',  ( -13.97604488694527625, -13.89961937509977652, 111.8739096053143243 ) ) ;
#89883=CARTESIAN_POINT ( 'NONE',  ( -5.049401038298153566, 19.05341960407611168, 110.2072429386476671 ) ) ;
#89884=CARTESIAN_POINT ( 'NONE',  ( -8.224510206698948167, 14.34966873604960824, 85.41557627198102409 ) ) ;
#89886=CARTESIAN_POINT ( 'NONE',  ( -9.564922557961040184, 16.46253265017147172, 27.91775706135232582 ) ) ;
#89887=CARTESIAN_POINT ( 'NONE',  ( 14.34966873604972726, -8.224510206698740333, 90.83442372801901854 ) ) ;
#89888=CARTESIAN_POINT ( 'NONE',  ( -0.05219959533909027116, -19.03943276465977164, 77.49890960531435269 ) ) ;
#89889=CARTESIAN_POINT ( 'NONE',  ( 5.719274019375673035, 21.55341960407619339, 52.29275706135236135 ) ) ;
#89890=CARTESIAN_POINT ( 'NONE',  ( 5.823673210054125526, 21.52544592524343514, 39.79057627198103830 ) ) ;
#89891=CARTESIAN_POINT ( 'NONE',  ( -15.72974639402197994, 15.80617190586746368, 115.6239096053143669 ) ) ;
#89892=CARTESIAN_POINT ( 'NONE',  ( -5.719274019375978568, 21.55341960407610458, 75.20724293864769550 ) ) ;
#89893=CARTESIAN_POINT ( 'NONE',  ( 4.483927247898545687, 16.52544592524342804, 99.79057627198103830 ) ) ;
#89894=CARTESIAN_POINT ( 'NONE',  ( 13.97604488694548053, -13.89961937509957401, 60.62609039468564731 ) ) ;
#89895=CARTESIAN_POINT ( 'NONE',  ( 5.153800228976335163, 19.02544592524342804, 29.79057627198102409 ) ) ;
#89896=CARTESIAN_POINT ( 'NONE',  ( -19.02544592524342804, 5.153800228976336051, 81.04057627198103830 ) ) ;
#89897=CARTESIAN_POINT ( 'NONE',  ( 13.89961937509977652, -13.97604488694527269, 88.12390960531438111 ) ) ;
#89898=CARTESIAN_POINT ( 'NONE',  ( 4.483927247898545687, 16.52544592524342804, 99.79057627198103830 ) ) ;
#89899=CARTESIAN_POINT ( 'NONE',  ( 4.379528057220339221, -16.55341960407611168, 32.70724293864770260 ) ) ;
#89900=CARTESIAN_POINT ( 'NONE',  ( -16.55341960407617563, 4.379528057220093196, 23.54275706135235424 ) ) ;
#89901=CARTESIAN_POINT ( 'NONE',  ( -21.53943276465977519, -0.05219959533937600094, 103.7510903946857042 ) ) ;
#89902=CARTESIAN_POINT ( 'NONE',  ( -19.02544592524342804, 5.153800228976336051, 106.0405762719810241 ) ) ;
#89903=CARTESIAN_POINT ( 'NONE',  ( -5.719274019375665041, -21.55341960407619695, 19.79275706135235069 ) ) ;
#89904=CARTESIAN_POINT ( 'NONE',  ( -19.03943276465977164, 0.05219959533909376836, 46.24890960531435979 ) ) ;
#89905=CARTESIAN_POINT ( 'NONE',  ( 4.483927247898790824, -16.52544592524335698, 50.20942372801901854 ) ) ;
#89906=CARTESIAN_POINT ( 'NONE',  ( -19.05341960407617563, 5.049401038297882671, 113.5427570613523471 ) ) ;
#89907=CARTESIAN_POINT ( 'NONE',  ( 19.02544592524343514, -5.153800228976328945, 38.54057627198103120 ) ) ;
#89909=CARTESIAN_POINT ( 'NONE',  ( -14.29746914071049879, 8.314922557960819915, 95.83224293864770971 ) ) ;
#89910=CARTESIAN_POINT ( 'NONE',  ( 10.81492255796078972, 18.62759615963270932, 99.58224293864770971 ) ) ;
#89911=CARTESIAN_POINT ( 'NONE',  ( 9.564922557961047289, -16.46253265017146816, 75.41775706135234714 ) ) ;
#89913=CARTESIAN_POINT ( 'NONE',  ( -9.564922557960796823, -16.46253265017161027, 87.08224293864769550 ) ) ;
#89914=CARTESIAN_POINT ( 'NONE',  ( 21.53943276465977519, -0.05219959533907433946, 113.7489096053143527 ) ) ;
#89915=CARTESIAN_POINT ( 'NONE',  ( 9.564922557960805705, 16.46253265017160317, 24.58224293864769194 ) ) ;
#89916=CARTESIAN_POINT ( 'NONE',  ( -5.153800228976328057, -19.02544592524343514, 87.29057627198103830 ) ) ;
#89917=CARTESIAN_POINT ( 'NONE',  ( 16.31925111598458500, -7.325300261831533710, 112.6642453896725726 ) ) ;
#89918=CARTESIAN_POINT ( 'NONE',  ( 5.153800228976335163, 19.02544592524342804, 89.79057627198102409 ) ) ;
#89919=CARTESIAN_POINT ( 'NONE',  ( 15.80617190586769283, -15.72974639402175789, 35.62609039468568994 ) ) ;
#89920=CARTESIAN_POINT ( 'NONE',  ( 16.52544592524342804, -4.483927247898539470, 88.54057627198103830 ) ) ;
#89921=CARTESIAN_POINT ( 'NONE',  ( -13.97604488694527625, -13.89961937509977652, 91.87390960531432427 ) ) ;
#89922=CARTESIAN_POINT ( 'NONE',  ( -13.89961937509957401, -13.97604488694547875, 29.37609039468565797 ) ) ;
#89923=CARTESIAN_POINT ( 'NONE',  ( 8.314922557961029526, -14.29746914071037800, 45.41775706135234003 ) ) ;
#89924=CARTESIAN_POINT ( 'NONE',  ( 18.62759615963255655, 10.81492255796105972, 66.66775706135234714 ) ) ;
#89926=CARTESIAN_POINT ( 'NONE',  ( 0.05219959533934541429, -16.53943276465976808, 25.00109039468567218 ) ) ;
#89927=CARTESIAN_POINT ( 'NONE',  ( -5.049401038298153566, 19.05341960407611168, 75.20724293864769550 ) ) ;
#89928=CARTESIAN_POINT ( 'NONE',  ( -16.46253265017146816, -9.564922557961047289, 94.16775706135233293 ) ) ;
#89929=CARTESIAN_POINT ( 'NONE',  ( -0.05219959533934338120, 16.53943276465976808, 67.50109039468568994 ) ) ;
#89930=CARTESIAN_POINT ( 'NONE',  ( -5.823673210054431948, 21.52544592524334988, 107.7094237280190328 ) ) ;
#89931=CARTESIAN_POINT ( 'NONE',  ( 19.03943276465977164, 0.05219959533936151252, 76.25109039468566152 ) ) ;
#89932=CARTESIAN_POINT ( 'NONE',  ( -13.89961937509977652, 13.97604488694528158, 55.62390960531434558 ) ) ;
#89933=CARTESIAN_POINT ( 'NONE',  ( 5.823673210054125526, 21.52544592524343514, 84.79057627198102409 ) ) ;
#89934=CARTESIAN_POINT ( 'NONE',  ( -0.05219959533910754901, -16.53943276465976808, 82.49890960531436690 ) ) ;
#89935=CARTESIAN_POINT ( 'NONE',  ( -13.89961937509957401, -13.97604488694547875, 79.37609039468567573 ) ) ;
#89936=CARTESIAN_POINT ( 'NONE',  ( -19.25918095147779496, -5.499999999999484857, 69.45284276293932635 ) ) ;
#89937=CARTESIAN_POINT ( 'NONE',  ( 9.564922557961047289, -16.46253265017146816, 50.41775706135233293 ) ) ;
#89938=CARTESIAN_POINT ( 'NONE',  ( 8.224510206698742110, 14.34966873604972548, 112.0844237280190185 ) ) ;
#89939=CARTESIAN_POINT ( 'NONE',  ( -14.34966873604960291, -8.224510206698953496, 66.66557627198102409 ) ) ;
#89940=CARTESIAN_POINT ( 'NONE',  ( -5.823673210054431948, 21.52544592524334988, 97.70942372801904696 ) ) ;
#89942=CARTESIAN_POINT ( 'NONE',  ( -18.67979575497178146, -10.72451020669898902, 111.6655762719810525 ) ) ;
#89943=CARTESIAN_POINT ( 'NONE',  ( 16.46253265017160672, -9.564922557960803928, 63.33224293864769550 ) ) ;
#89944=CARTESIAN_POINT ( 'NONE',  ( -21.55341960407619339, 5.719274019375674811, 78.54275706135236135 ) ) ;
#89945=CARTESIAN_POINT ( 'NONE',  ( -16.51473224551069308, -9.474510206698971260, 56.66557627198103120 ) ) ;
#89946=EDGE_LOOP ( 'NONE', ( #182370, #180900, #197336, #78024, #85320, #199399, #88067, #19883 ) ) ;
#89947=CARTESIAN_POINT ( 'NONE',  ( -5.153800228976328057, -19.02544592524343514, 27.29057627198103120 ) ) ;
#89948=CARTESIAN_POINT ( 'NONE',  ( 21.55341960407610458, 5.719274019375980345, 23.95724293864769550 ) ) ;
#89949=CARTESIAN_POINT ( 'NONE',  ( -14.29746914071049879, 8.314922557960819915, 70.83224293864770971 ) ) ;
#89950=CARTESIAN_POINT ( 'NONE',  ( -13.97604488694527625, -13.89961937509977652, 46.87390960531435979 ) ) ;
#89951=CARTESIAN_POINT ( 'NONE',  ( 14.34966873604960469, 8.224510206698951720, 94.16557627198103830 ) ) ;
#89952=CARTESIAN_POINT ( 'NONE',  ( 15.80617190586746368, 15.72974639402197994, 114.3739096053143527 ) ) ;
#89953=CARTESIAN_POINT ( 'NONE',  ( -21.53943276465977519, -0.05219959533937600094, 48.75109039468568284 ) ) ;
#89954=CARTESIAN_POINT ( 'NONE',  ( -19.03943276465977164, 0.05219959533909376836, 26.24890960531435624 ) ) ;
#89955=CARTESIAN_POINT ( 'NONE',  ( 16.53943276465976808, 0.05219959533934440121, 61.25109039468567573 ) ) ;
#89956=CARTESIAN_POINT ( 'NONE',  ( -5.719274019375978568, 21.55341960407610458, 100.2072429386476955 ) ) ;
#89957=CARTESIAN_POINT ( 'NONE',  ( 18.67979575497178502, 10.72451020669898547, 99.16557627198100988 ) ) ;
#89958=CARTESIAN_POINT ( 'NONE',  ( -5.049401038297874678, -19.05341960407617918, 29.79275706135232227 ) ) ;
#89959=CARTESIAN_POINT ( 'NONE',  ( -0.05219959533909027116, -19.03943276465977164, 57.49890960531435979 ) ) ;
#89960=CARTESIAN_POINT ( 'NONE',  ( 18.22780087662123805, -5.499999999999976019, 73.51763182126894947 ) ) ;
#89961=CARTESIAN_POINT ( 'NONE',  ( 21.52544592524334988, 5.823673210054432836, 61.45942372801901854 ) ) ;
#89962=CARTESIAN_POINT ( 'NONE',  ( -15.80617190586745835, -15.72974639402198527, 51.87390960531437401 ) ) ;
#89963=CARTESIAN_POINT ( 'NONE',  ( 16.52544592524342804, -4.483927247898539470, 28.54057627198103120 ) ) ;
#89964=CARTESIAN_POINT ( 'NONE',  ( -0.05219959533937732626, 21.53943276465977519, 82.50109039468568994 ) ) ;
#89965=CARTESIAN_POINT ( 'NONE',  ( 10.72451020669871369, 18.67979575497193778, 102.0844237280190185 ) ) ;
#89966=CARTESIAN_POINT ( 'NONE',  ( -16.46253265017146816, -9.564922557961047289, 44.16775706135232582 ) ) ;
#89967=CARTESIAN_POINT ( 'NONE',  ( 12.14591786802327356, -12.06949235617739191, 95.62609039468568994 ) ) ;
#89968=CARTESIAN_POINT ( 'NONE',  ( -21.52544592524334988, -5.823673210054445271, 58.95942372801902565 ) ) ;
#89969=CARTESIAN_POINT ( 'NONE',  ( 16.51473224551069308, 9.474510206698969483, 54.16557627198103120 ) ) ;
#89970=CARTESIAN_POINT ( 'NONE',  ( -5.153800228976607833, 19.02544592524334988, 37.70942372801899722 ) ) ;
#89971=CARTESIAN_POINT ( 'NONE',  ( 18.62759615963271287, -10.81492255796078972, 43.33224293864769550 ) ) ;
#89972=CARTESIAN_POINT ( 'NONE',  ( -0.05219959533937732626, 21.53943276465977519, 27.50109039468567929 ) ) ;
#89973=CARTESIAN_POINT ( 'NONE',  ( 5.823673210054125526, 21.52544592524343514, 84.79057627198102409 ) ) ;
#89974=CARTESIAN_POINT ( 'NONE',  ( 13.89961937509957401, 13.97604488694547697, 86.87609039468567573 ) ) ;
#89975=CARTESIAN_POINT ( 'NONE',  ( -12.14591786802326823, 12.06949235617739902, 58.12609039468568994 ) ) ;
#89977=CARTESIAN_POINT ( 'NONE',  ( 5.719274019375991003, -21.55341960407610458, 97.70724293864772392 ) ) ;
#89978=CARTESIAN_POINT ( 'NONE',  ( 8.314922557961029526, -14.29746914071037800, 80.41775706135234714 ) ) ;
#89979=CARTESIAN_POINT ( 'NONE',  ( -0.05219959533910754901, -16.53943276465976808, 82.49890960531436690 ) ) ;
#89981=CARTESIAN_POINT ( 'NONE',  ( 13.97604488694548053, -13.89961937509957401, 100.6260903946856615 ) ) ;
#89982=CARTESIAN_POINT ( 'NONE',  ( 18.62759615963271287, -10.81492255796078972, 38.33224293864768839 ) ) ;
#89984=CARTESIAN_POINT ( 'NONE',  ( -16.55341960407617563, 4.379528057220093196, 38.54275706135234714 ) ) ;
#89985=CARTESIAN_POINT ( 'NONE',  ( 18.62759615963271287, -10.81492255796078972, 113.3322429386476955 ) ) ;
#89986=CARTESIAN_POINT ( 'NONE',  ( 5.823673210054125526, 21.52544592524343514, 34.79057627198103120 ) ) ;
#89987=CARTESIAN_POINT ( 'NONE',  ( -8.314922557961024197, 14.29746914071037800, 72.91775706135234714 ) ) ;
#89988=CARTESIAN_POINT ( 'NONE',  ( -9.564922557960796823, -16.46253265017161027, 82.08224293864768129 ) ) ;
#89989=CARTESIAN_POINT ( 'NONE',  ( 5.719274019375673035, 21.55341960407619339, 57.29275706135234714 ) ) ;
#89990=CARTESIAN_POINT ( 'NONE',  ( 19.03943276465977164, -0.05219959533909143690, 23.74890960531435269 ) ) ;
#89991=CARTESIAN_POINT ( 'NONE',  ( 5.719274019375991003, -21.55341960407610458, 22.70724293864769194 ) ) ;
#89992=VERTEX_POINT ( 'NONE', #150105 ) ;
#89993=CARTESIAN_POINT ( 'NONE',  ( 5.153800228976615827, -19.02544592524334988, 35.20942372801899722 ) ) ;
#89994=CARTESIAN_POINT ( 'NONE',  ( 4.379528057220092307, 16.55341960407617563, 52.29275706135236135 ) ) ;
#89995=CARTESIAN_POINT ( 'NONE',  ( -19.02544592524342804, 5.153800228976336051, 111.0405762719810099 ) ) ;
#89996=CARTESIAN_POINT ( 'NONE',  ( -13.97604488694527625, -13.89961937509977652, 71.87390960531433848 ) ) ;
#89997=CARTESIAN_POINT ( 'NONE',  ( -4.483927247898782831, 16.52544592524335698, 102.7094237280190185 ) ) ;
#89998=FACE_OUTER_BOUND ( 'NONE', #62187, .T. ) ;
#89999=CARTESIAN_POINT ( 'NONE',  ( 4.379528057220339221, -16.55341960407611168, 92.70724293864770971 ) ) ;
#90000=CARTESIAN_POINT ( 'NONE',  ( 15.80617190586746368, 15.72974639402197994, 29.37390960531435269 ) ) ;
#90001=CARTESIAN_POINT ( 'NONE',  ( 16.46253265017160672, -9.564922557960803928, 33.33224293864770260 ) ) ;
#90002=CARTESIAN_POINT ( 'NONE',  ( -8.224510206698735004, -14.34966873604973081, 69.58442372801900433 ) ) ;
#90003=CARTESIAN_POINT ( 'NONE',  ( 21.52544592524334988, 5.823673210054432836, 26.45942372801901854 ) ) ;
#90004=CARTESIAN_POINT ( 'NONE',  ( 13.97604488694548053, -13.89961937509957401, 80.62609039468567573 ) ) ;
#90005=CARTESIAN_POINT ( 'NONE',  ( -13.97604488694527625, -13.89961937509977652, 41.87390960531435979 ) ) ;
#90006=CARTESIAN_POINT ( 'NONE',  ( 21.53943276465977519, -0.05219959533907433946, 73.74890960531433848 ) ) ;
#90007=CARTESIAN_POINT ( 'NONE',  ( 13.89961937509977652, -13.97604488694527269, 113.1239096053143527 ) ) ;
#90008=CARTESIAN_POINT ( 'NONE',  ( -10.72451020669870658, -18.67979575497194134, 94.58442372801901854 ) ) ;
#90009=CARTESIAN_POINT ( 'NONE',  ( 16.51473224551069308, 9.474510206698969483, 69.16557627198102409 ) ) ;
#90010=CARTESIAN_POINT ( 'NONE',  ( -8.224510206698735004, -14.34966873604973081, 54.58442372801901143 ) ) ;
#90011=CARTESIAN_POINT ( 'NONE',  ( 21.53943276465977519, 0.05219959533937863772, 81.25109039468568994 ) ) ;
#90012=CARTESIAN_POINT ( 'NONE',  ( 5.153800228976615827, -19.02544592524334988, 35.20942372801899722 ) ) ;
#90013=CARTESIAN_POINT ( 'NONE',  ( -19.05341960407617563, 5.049401038297882671, 53.54275706135231871 ) ) ;
#90015=CARTESIAN_POINT ( 'NONE',  ( -15.72974639402176322, -15.80617190586768395, 49.37609039468569705 ) ) ;
#90017=CARTESIAN_POINT ( 'NONE',  ( -9.564922557961040184, 16.46253265017147172, 42.91775706135234003 ) ) ;
#90018=CARTESIAN_POINT ( 'NONE',  ( 13.97604488694527802, 13.89961937509977652, 94.37390960531436690 ) ) ;
#90019=CARTESIAN_POINT ( 'NONE',  ( -16.51473224551069308, -9.474510206698971260, 76.66557627198103830 ) ) ;
#90020=CARTESIAN_POINT ( 'NONE',  ( -16.55341960407611168, -4.379528057220339221, 41.45724293864769550 ) ) ;
#90021=CARTESIAN_POINT ( 'NONE',  ( 18.67979575497178502, 10.72451020669898547, 34.16557627198102409 ) ) ;
#90024=CARTESIAN_POINT ( 'NONE',  ( -10.72451020669870658, -18.67979575497194134, 104.5844237280190185 ) ) ;
#90026=CARTESIAN_POINT ( 'NONE',  ( -0.05219959533909027116, -19.03943276465977164, 37.49890960531436690 ) ) ;
#90029=CARTESIAN_POINT ( 'NONE',  ( 12.14591786802327356, -12.06949235617739191, 50.62609039468568994 ) ) ;
#90030=CARTESIAN_POINT ( 'NONE',  ( -18.62759615963270932, 10.81492255796079327, 70.83224293864770971 ) ) ;
#90032=CARTESIAN_POINT ( 'NONE',  ( -16.55341960407611168, -4.379528057220339221, 41.45724293864769550 ) ) ;
#90033=CARTESIAN_POINT ( 'NONE',  ( 9.564922557960805705, 16.46253265017160317, 34.58224293864770260 ) ) ;
#90034=CARTESIAN_POINT ( 'NONE',  ( 16.51473224551069308, 9.474510206698969483, 104.1655762719810241 ) ) ;
#90035=CARTESIAN_POINT ( 'NONE',  ( -18.67979575497193778, 10.72451020669871902, 28.33442372801902209 ) ) ;
#90036=CARTESIAN_POINT ( 'NONE',  ( 19.03943276465977164, 0.05219959533936151252, 36.25109039468567573 ) ) ;
#90037=CARTESIAN_POINT ( 'NONE',  ( 14.34966873604960469, 8.224510206698951720, 114.1655762719810383 ) ) ;
#90038=CARTESIAN_POINT ( 'NONE',  ( 21.55341960407619695, -5.719274019375665929, 76.04275706135237556 ) ) ;
#90040=CARTESIAN_POINT ( 'NONE',  ( -8.224510206698948167, 14.34966873604960824, 30.41557627198101699 ) ) ;
#90042=CARTESIAN_POINT ( 'NONE',  ( 0.05219959533907565091, 21.53943276465977519, 24.99890960531435624 ) ) ;
#90043=CARTESIAN_POINT ( 'NONE',  ( 12.06949235617757843, -12.14591786802309237, 93.12390960531436690 ) ) ;
#90045=CARTESIAN_POINT ( 'NONE',  ( -0.05219959533909027116, -19.03943276465977164, 82.49890960531436690 ) ) ;
#90046=CARTESIAN_POINT ( 'NONE',  ( -16.55341960407611168, -4.379528057220339221, 76.45724293864769550 ) ) ;
#90047=CARTESIAN_POINT ( 'NONE',  ( 19.05341960407617918, -5.049401038297876454, 106.0427570613523471 ) ) ;
#90048=CARTESIAN_POINT ( 'NONE',  ( 21.55341960407610458, 5.719274019375980345, 68.95724293864769550 ) ) ;
#90050=CARTESIAN_POINT ( 'NONE',  ( -9.474510206698964154, 16.51473224551069663, 35.41557627198102409 ) ) ;
#90051=CARTESIAN_POINT ( 'NONE',  ( -16.46253265017160317, 9.564922557960807481, 65.83224293864769550 ) ) ;
#90052=CARTESIAN_POINT ( 'NONE',  ( -5.719274019375978568, 21.55341960407610458, 70.20724293864769550 ) ) ;
#90053=CARTESIAN_POINT ( 'NONE',  ( -12.06949235617739369, -12.14591786802326823, 104.3760903946856899 ) ) ;
#90054=CARTESIAN_POINT ( 'NONE',  ( 9.474510206698971260, -16.51473224551069308, 87.91557627198102409 ) ) ;
#90055=CARTESIAN_POINT ( 'NONE',  ( -5.049401038297874678, -19.05341960407617918, 69.79275706135233293 ) ) ;
#90056=CARTESIAN_POINT ( 'NONE',  ( -5.823673210054431948, 21.52544592524334988, 97.70942372801904696 ) ) ;
#90057=CARTESIAN_POINT ( 'NONE',  ( 21.52544592524344225, -5.823673210054117533, 78.54057627198103830 ) ) ;
#90058=CARTESIAN_POINT ( 'NONE',  ( -21.55341960407610458, -5.719274019375992779, 26.45724293864768839 ) ) ;
#90059=CARTESIAN_POINT ( 'NONE',  ( 19.05341960407611168, 5.049401038298154454, 43.95724293864769550 ) ) ;
#90060=CARTESIAN_POINT ( 'NONE',  ( 16.55341960407618274, -4.379528057220086978, 111.0427570613523613 ) ) ;
#90061=CARTESIAN_POINT ( 'NONE',  ( -9.564922557960796823, -16.46253265017161027, 67.08224293864769550 ) ) ;
#90062=CARTESIAN_POINT ( 'NONE',  ( -0.05219959533936034679, 19.03943276465977164, 82.50109039468567573 ) ) ;
#90063=CARTESIAN_POINT ( 'NONE',  ( -18.62759615963255300, -10.81492255796106328, 109.1677570613523613 ) ) ;
#90064=CARTESIAN_POINT ( 'NONE',  ( -4.483927247898539470, -16.52544592524342804, 72.29057627198102409 ) ) ;
#90065=CARTESIAN_POINT ( 'NONE',  ( 0.05219959533907565091, 21.53943276465977519, 109.9989096053143527 ) ) ;
#90066=CARTESIAN_POINT ( 'NONE',  ( 5.823673210054125526, 21.52544592524343514, 99.79057627198103830 ) ) ;
#90068=CARTESIAN_POINT ( 'NONE',  ( 21.53943276465977519, -0.05219959533907433946, 63.74890960531435979 ) ) ;
#90069=CARTESIAN_POINT ( 'NONE',  ( -0.05219959533934338120, 16.53943276465976808, 82.50109039468568994 ) ) ;
#90070=CARTESIAN_POINT ( 'NONE',  ( 16.55341960407611168, 4.379528057220329451, 103.9572429386476813 ) ) ;
#90071=CARTESIAN_POINT ( 'NONE',  ( 16.51473224551069308, 9.474510206698969483, 64.16557627198102409 ) ) ;
#90072=CARTESIAN_POINT ( 'NONE',  ( 4.379528057220092307, 16.55341960407617563, 112.2927570613523471 ) ) ;
#90073=CARTESIAN_POINT ( 'NONE',  ( 18.67979575497194134, -10.72451020669871369, 45.83442372801901854 ) ) ;
#90074=CARTESIAN_POINT ( 'NONE',  ( 9.474510206698971260, -16.51473224551069308, 112.9155762719810383 ) ) ;
#90075=CARTESIAN_POINT ( 'NONE',  ( -0.05219959533937732626, 21.53943276465977519, 87.50109039468568994 ) ) ;
#90076=CARTESIAN_POINT ( 'NONE',  ( 5.049401038298161559, -19.05341960407611168, 32.70724293864768129 ) ) ;
#90077=CARTESIAN_POINT ( 'NONE',  ( 13.97604488694527802, 13.89961937509977652, 39.37390960531435269 ) ) ;
#90079=EDGE_LOOP ( 'NONE', ( #61343, #32622 ) ) ;
#90080=CARTESIAN_POINT ( 'NONE',  ( 21.55341960407619695, -5.719274019375665929, 66.04275706135236135 ) ) ;
#90081=CARTESIAN_POINT ( 'NONE',  ( 19.03943276465977164, -0.05219959533909143690, 103.7489096053143669 ) ) ;
#90082=CARTESIAN_POINT ( 'NONE',  ( 13.97604488694548053, -13.89961937509957401, 75.62609039468564731 ) ) ;
#90083=CARTESIAN_POINT ( 'NONE',  ( 18.67979575497194134, -10.72451020669871369, 40.83442372801901854 ) ) ;
#90084=CARTESIAN_POINT ( 'NONE',  ( 4.483927247898790824, -16.52544592524335698, 20.20942372801900788 ) ) ;
#90085=CARTESIAN_POINT ( 'NONE',  ( 19.02544592524334988, 5.153800228976608722, 76.45942372801897591 ) ) ;
#90086=CARTESIAN_POINT ( 'NONE',  ( 5.049401038298161559, -19.05341960407611168, 57.70724293864769550 ) ) ;
#90087=CARTESIAN_POINT ( 'NONE',  ( 16.46253265017146816, 9.564922557961045513, 81.66775706135233293 ) ) ;
#90088=CARTESIAN_POINT ( 'NONE',  ( 12.06949235617757843, -12.14591786802309237, 28.12390960531435979 ) ) ;
#90089=CARTESIAN_POINT ( 'NONE',  ( 13.97604488694548053, -13.89961937509957401, 95.62609039468563310 ) ) ;
#90090=CARTESIAN_POINT ( 'NONE',  ( 4.483927247898545687, 16.52544592524342804, 39.79057627198103830 ) ) ;
#90091=CARTESIAN_POINT ( 'NONE',  ( 19.02544592524334988, 5.153800228976608722, 61.45942372801900433 ) ) ;
#90092=CARTESIAN_POINT ( 'NONE',  ( 14.29746914071037800, 8.314922557961029526, 41.66775706135235424 ) ) ;
#90093=CARTESIAN_POINT ( 'NONE',  ( 9.564922557961047289, -16.46253265017146816, 20.41775706135233293 ) ) ;
#90094=CARTESIAN_POINT ( 'NONE',  ( 16.46253265017160672, -9.564922557960803928, 48.33224293864769550 ) ) ;
#90095=CARTESIAN_POINT ( 'NONE',  ( -16.62475595723694255, -7.163666690055256581, 64.47286648189536606 ) ) ;
#90096=CARTESIAN_POINT ( 'NONE',  ( -16.52544592524335698, -4.483927247898792601, 48.95942372801902565 ) ) ;
#90097=DIRECTION ( 'NONE',  ( -0.000000000000000000, -0.000000000000000000, 1.000000000000000000 ) ) ;
#90099=CARTESIAN_POINT ( 'NONE',  ( 16.51473224551069308, 9.474510206698969483, 94.16557627198103830 ) ) ;
#90100=DIRECTION ( 'NONE',  ( 0.000000000000000000, 0.000000000000000000, 1.000000000000000000 ) ) ;
#90101=CARTESIAN_POINT ( 'NONE',  ( 19.03943276465977164, 0.05219959533936151252, 86.25109039468567573 ) ) ;
#90102=CARTESIAN_POINT ( 'NONE',  ( 21.55341960407610458, 5.719274019375980345, 23.95724293864769550 ) ) ;
#90103=CARTESIAN_POINT ( 'NONE',  ( 21.55341960407619695, -5.719274019375665929, 111.0427570613523613 ) ) ;
#90104=CARTESIAN_POINT ( 'NONE',  ( 13.97604488694548053, -13.89961937509957401, 100.6260903946856615 ) ) ;
#90105=CARTESIAN_POINT ( 'NONE',  ( 4.483927247898545687, 16.52544592524342804, 109.7905762719810383 ) ) ;
#90106=CARTESIAN_POINT ( 'NONE',  ( 19.03943276465977164, -0.05219959533909143690, 33.74890960531435979 ) ) ;
#90107=CARTESIAN_POINT ( 'NONE',  ( 21.53943276465977519, -0.05219959533907433946, 53.74890960531437401 ) ) ;
#90108=CARTESIAN_POINT ( 'NONE',  ( -19.05341960407611168, -5.049401038298163336, 26.45724293864769550 ) ) ;
#90109=CARTESIAN_POINT ( 'NONE',  ( 17.50000000000000000, 5.499999999999992895, 101.7030961746583131 ) ) ;
#90110=CARTESIAN_POINT ( 'NONE',  ( -19.02544592524334988, -5.153800228976617603, 73.95942372801900433 ) ) ;
#90111=CARTESIAN_POINT ( 'NONE',  ( -4.483927247898539470, -16.52544592524342804, 52.29057627198102409 ) ) ;
#90112=CARTESIAN_POINT ( 'NONE',  ( 5.823673210054125526, 21.52544592524343514, 34.79057627198103120 ) ) ;
#90113=CARTESIAN_POINT ( 'NONE',  ( -18.62759615963255300, -10.81492255796106328, 94.16775706135237556 ) ) ;
#90114=CARTESIAN_POINT ( 'NONE',  ( 0.05219959533907565091, 21.53943276465977519, 89.99890960531438111 ) ) ;
#90115=CARTESIAN_POINT ( 'NONE',  ( -21.55341960407619339, 5.719274019375674811, 58.54275706135235424 ) ) ;
#90116=CARTESIAN_POINT ( 'NONE',  ( -5.823673210054431948, 21.52544592524334988, 67.70942372801901854 ) ) ;
#90117=CARTESIAN_POINT ( 'NONE',  ( 0.05219959533909260263, 19.03943276465977164, 99.99890960531436690 ) ) ;
#90118=CARTESIAN_POINT ( 'NONE',  ( 8.224510206698742110, 14.34966873604972548, 97.08442372801904696 ) ) ;
#90119=CARTESIAN_POINT ( 'NONE',  ( 10.72451020669871369, 18.67979575497193778, 62.08442372801901143 ) ) ;
#90120=CARTESIAN_POINT ( 'NONE',  ( -4.379528057220328563, 16.55341960407611168, 115.2072429386476955 ) ) ;
#90121=CARTESIAN_POINT ( 'NONE',  ( -12.14591786802309592, -12.06949235617757132, 61.87390960531436690 ) ) ;
#90122=CARTESIAN_POINT ( 'NONE',  ( -16.52544592524342804, 4.483927247898546575, 31.04057627198102409 ) ) ;
#90123=CARTESIAN_POINT ( 'NONE',  ( 21.55341960407610458, 5.719274019375980345, 43.95724293864769550 ) ) ;
#90124=CARTESIAN_POINT ( 'NONE',  ( -19.03943276465977164, 0.05219959533909376836, 51.24890960531436690 ) ) ;
#90125=CARTESIAN_POINT ( 'NONE',  ( -18.67979575497178146, -10.72451020669898902, 61.66557627198103120 ) ) ;
#90126=CARTESIAN_POINT ( 'NONE',  ( 19.03943276465977164, 0.05219959533936151252, 51.25109039468567573 ) ) ;
#90128=CARTESIAN_POINT ( 'NONE',  ( 16.52544592524342804, -4.483927247898539470, 43.54057627198103830 ) ) ;
#90129=CARTESIAN_POINT ( 'NONE',  ( 18.62759615963271287, -10.81492255796078972, 28.33224293864769550 ) ) ;
#90130=ORIENTED_EDGE ( 'NONE', *, *, #3863, .T. ) ;
#90132=CARTESIAN_POINT ( 'NONE',  ( 17.78954161113920307, 0.5375896797884988088, 37.50000000000000711 ) ) ;
#90133=CARTESIAN_POINT ( 'NONE',  ( 14.34966873604972726, -8.224510206698740333, 70.83442372801901854 ) ) ;
#90134=CARTESIAN_POINT ( 'NONE',  ( -5.049401038297874678, -19.05341960407617918, 79.79275706135233293 ) ) ;
#90135=CARTESIAN_POINT ( 'NONE',  ( 8.224510206698953496, -14.34966873604960469, 37.91557627198102409 ) ) ;
#90136=CARTESIAN_POINT ( 'NONE',  ( -19.39720447994794839, -5.499999999999978684, 59.66317477297175742 ) ) ;
#90137=CARTESIAN_POINT ( 'NONE',  ( -16.53943276465976808, 0.05219959533911058130, 26.24890960531435624 ) ) ;
#90138=CARTESIAN_POINT ( 'NONE',  ( -16.46253265017160317, 9.564922557960807481, 45.83224293864769550 ) ) ;
#90139=CARTESIAN_POINT ( 'NONE',  ( -13.89961937509977652, 13.97604488694528158, 70.62390960531432427 ) ) ;
#90140=CARTESIAN_POINT ( 'NONE',  ( 5.049401038298161559, -19.05341960407611168, 37.70724293864768839 ) ) ;
#90141=CARTESIAN_POINT ( 'NONE',  ( 18.62759615963255655, 10.81492255796105972, 51.66775706135234714 ) ) ;
#90142=CARTESIAN_POINT ( 'NONE',  ( 9.564922557960805705, 16.46253265017160317, 59.58224293864769550 ) ) ;
#90144=CARTESIAN_POINT ( 'NONE',  ( 0.05219959533909260263, 19.03943276465977164, 59.99890960531436690 ) ) ;
#90145=CARTESIAN_POINT ( 'NONE',  ( -21.55341960407610458, -5.719274019375992779, 41.45724293864769550 ) ) ;
#90147=CARTESIAN_POINT ( 'NONE',  ( -19.02544592524342804, 5.153800228976336051, 36.04057627198100988 ) ) ;
#90148=CARTESIAN_POINT ( 'NONE',  ( -21.55341960407610458, -5.719274019375992779, 36.45724293864768839 ) ) ;
#90149=CARTESIAN_POINT ( 'NONE',  ( 4.483927247898790824, -16.52544592524335698, 90.20942372801903275 ) ) ;
#90151=CARTESIAN_POINT ( 'NONE',  ( 19.03943276465977164, 0.05219959533936151252, 26.25109039468566507 ) ) ;
#90152=CARTESIAN_POINT ( 'NONE',  ( -14.34966873604972548, 8.224510206698743886, 68.33442372801900433 ) ) ;
#90153=CARTESIAN_POINT ( 'NONE',  ( -5.049401038298153566, 19.05341960407611168, 115.2072429386477097 ) ) ;
#90154=CARTESIAN_POINT ( 'NONE',  ( 16.55341960407618274, -4.379528057220086978, 56.04275706135235424 ) ) ;
#90155=CARTESIAN_POINT ( 'NONE',  ( 14.34966873604972726, -8.224510206698740333, 45.83442372801901854 ) ) ;
#90156=CARTESIAN_POINT ( 'NONE',  ( 13.97604488694527802, 13.89961937509977652, 114.3739096053143669 ) ) ;
#90157=CARTESIAN_POINT ( 'NONE',  ( -16.52544592524335698, -4.483927247898792601, 23.95942372801901143 ) ) ;
#90158=CARTESIAN_POINT ( 'NONE',  ( 9.474510206698971260, -16.51473224551069308, 32.91557627198102409 ) ) ;
#90159=CARTESIAN_POINT ( 'NONE',  ( 5.719274019375673035, 21.55341960407619339, 22.29275706135235069 ) ) ;
#90160=CARTESIAN_POINT ( 'NONE',  ( 0.05219959533934541429, -16.53943276465976808, 25.00109039468567218 ) ) ;
#90161=CARTESIAN_POINT ( 'NONE',  ( -14.34966873604972548, 8.224510206698743886, 103.3344237280190043 ) ) ;
#90163=CARTESIAN_POINT ( 'NONE',  ( -5.719274019375665041, -21.55341960407619695, 104.7927570613523898 ) ) ;
#90164=CARTESIAN_POINT ( 'NONE',  ( -5.049401038297874678, -19.05341960407617918, 94.79275706135230450 ) ) ;
#90165=CARTESIAN_POINT ( 'NONE',  ( 16.53943276465976808, -0.05219959533910856209, 53.74890960531437401 ) ) ;
#90166=CARTESIAN_POINT ( 'NONE',  ( 16.46253265017160672, -9.564922557960803928, 28.33224293864769550 ) ) ;
#90167=CARTESIAN_POINT ( 'NONE',  ( -0.05219959533936034679, 19.03943276465977164, 52.50109039468566863 ) ) ;
#90169=CARTESIAN_POINT ( 'NONE',  ( 18.67979575497194134, -10.72451020669871369, 45.83442372801901854 ) ) ;
#90170=CARTESIAN_POINT ( 'NONE',  ( -16.52544592524335698, -4.483927247898792601, 28.95942372801902209 ) ) ;
#90171=CARTESIAN_POINT ( 'NONE',  ( 16.18388926212236711, 7.379444403734555458, 82.93953151366150678 ) ) ;
#90172=CARTESIAN_POINT ( 'NONE',  ( 5.049401038298161559, -19.05341960407611168, 107.7072429386476955 ) ) ;
#90173=CARTESIAN_POINT ( 'NONE',  ( -5.823673210054116645, -21.52544592524344225, 67.29057627198103830 ) ) ;
#90174=CARTESIAN_POINT ( 'NONE',  ( 13.97604488694548053, -13.89961937509957401, 100.6260903946856615 ) ) ;
#90175=CARTESIAN_POINT ( 'NONE',  ( 13.97604488694527802, 13.89961937509977652, 109.3739096053143669 ) ) ;
#90177=CARTESIAN_POINT ( 'NONE',  ( 16.53943276465976808, -0.05219959533910856209, 108.7489096053143669 ) ) ;
#90178=CARTESIAN_POINT ( 'NONE',  ( -5.823673210054431948, 21.52544592524334988, 92.70942372801901854 ) ) ;
#90179=CARTESIAN_POINT ( 'NONE',  ( -19.03943276465977164, 0.05219959533909376836, 46.24890960531435979 ) ) ;
#90180=CARTESIAN_POINT ( 'NONE',  ( 18.62759615963255655, 10.81492255796105972, 56.66775706135235424 ) ) ;
#90182=CARTESIAN_POINT ( 'NONE',  ( 10.81492255796106328, -18.62759615963255655, 90.41775706135236135 ) ) ;
#90183=CARTESIAN_POINT ( 'NONE',  ( -12.06949235617739369, -12.14591786802326823, 109.3760903946857042 ) ) ;
#90184=CARTESIAN_POINT ( 'NONE',  ( 5.153800228976335163, 19.02544592524342804, 74.79057627198103830 ) ) ;
#90185=CARTESIAN_POINT ( 'NONE',  ( -0.05219959533937732626, 21.53943276465977519, 47.50109039468568994 ) ) ;
#90186=CARTESIAN_POINT ( 'NONE',  ( -15.72974639402176322, -15.80617190586768395, 34.37609039468568284 ) ) ;
#90187=CARTESIAN_POINT ( 'NONE',  ( -9.474510206698720793, -16.51473224551083518, 64.58442372801900433 ) ) ;
#90188=CARTESIAN_POINT ( 'NONE',  ( -16.46253265017160317, 9.564922557960807481, 85.83224293864769550 ) ) ;
#90189=CARTESIAN_POINT ( 'NONE',  ( 4.483927247898545687, 16.52544592524342804, 99.79057627198103830 ) ) ;
#90190=CARTESIAN_POINT ( 'NONE',  ( -10.81492255796078084, -18.62759615963271287, 92.08224293864769550 ) ) ;
#90191=CARTESIAN_POINT ( 'NONE',  ( 8.314922557960818139, 14.29746914071049879, 59.58224293864770260 ) ) ;
#90192=CARTESIAN_POINT ( 'NONE',  ( 9.564922557961047289, -16.46253265017146816, 25.41775706135234003 ) ) ;
#90193=CARTESIAN_POINT ( 'NONE',  ( -0.05219959533910754901, -16.53943276465976808, 82.49890960531436690 ) ) ;
#90194=CARTESIAN_POINT ( 'NONE',  ( -16.46253265017160317, 9.564922557960807481, 30.83224293864769550 ) ) ;
#90195=CARTESIAN_POINT ( 'NONE',  ( 9.564922557961047289, -16.46253265017146816, 85.41775706135233293 ) ) ;
#90196=CARTESIAN_POINT ( 'NONE',  ( -4.483927247898539470, -16.52544592524342804, 52.29057627198102409 ) ) ;
#90197=CARTESIAN_POINT ( 'NONE',  ( 5.823673210054444382, -21.52544592524334988, 100.2094237280190043 ) ) ;
#90198=CARTESIAN_POINT ( 'NONE',  ( -16.51473224551069308, -9.474510206698971260, 96.66557627198102409 ) ) ;
#90199=CARTESIAN_POINT ( 'NONE',  ( 0.05219959533936267826, -19.03943276465977164, 75.00109039468566152 ) ) ;
#90200=CARTESIAN_POINT ( 'NONE',  ( -15.72974639402197994, 15.80617190586746368, 80.62390960531438111 ) ) ;
#90201=CARTESIAN_POINT ( 'NONE',  ( -10.81492255796105439, 18.62759615963255655, 27.91775706135234358 ) ) ;
#90202=CARTESIAN_POINT ( 'NONE',  ( -4.483927247898782831, 16.52544592524335698, 27.70942372801901854 ) ) ;
#90203=CARTESIAN_POINT ( 'NONE',  ( 14.29746914071037800, 8.314922557961029526, 91.66775706135234714 ) ) ;
#90204=CARTESIAN_POINT ( 'NONE',  ( -19.03943276465977164, 0.05219959533909376836, 31.24890960531435979 ) ) ;
#90205=CARTESIAN_POINT ( 'NONE',  ( 15.80617190586769283, -15.72974639402175789, 40.62609039468567573 ) ) ;
#90206=CARTESIAN_POINT ( 'NONE',  ( 12.06949235617757843, -12.14591786802309237, 113.1239096053143953 ) ) ;
#90208=CARTESIAN_POINT ( 'NONE',  ( 12.06949235617739724, 12.14591786802326823, 51.87609039468568284 ) ) ;
#90209=CARTESIAN_POINT ( 'NONE',  ( 4.379528057220339221, -16.55341960407611168, 77.70724293864770971 ) ) ;
#90210=CARTESIAN_POINT ( 'NONE',  ( 5.823673210054125526, 21.52544592524343514, 69.79057627198102409 ) ) ;
#90211=CARTESIAN_POINT ( 'NONE',  ( 4.483927247898545687, 16.52544592524342804, 24.79057627198103120 ) ) ;
#90212=CARTESIAN_POINT ( 'NONE',  ( 4.379528057220092307, 16.55341960407617563, 52.29275706135236135 ) ) ;
#90213=CARTESIAN_POINT ( 'NONE',  ( -19.02544592524342804, 5.153800228976336051, 41.04057627198103120 ) ) ;
#90214=CARTESIAN_POINT ( 'NONE',  ( 12.14591786802327356, -12.06949235617739191, 90.62609039468567573 ) ) ;
#90215=CARTESIAN_POINT ( 'NONE',  ( -0.05219959533936034679, 19.03943276465977164, 82.50109039468567573 ) ) ;
#90216=CARTESIAN_POINT ( 'NONE',  ( -15.80617190586745835, -15.72974639402198527, 71.87390960531438111 ) ) ;
#90217=CARTESIAN_POINT ( 'NONE',  ( 4.483927247898790824, -16.52544592524335698, 110.2094237280190185 ) ) ;
#90219=CARTESIAN_POINT ( 'NONE',  ( 9.564922557960805705, 16.46253265017160317, 114.5822429386476955 ) ) ;
#90220=CARTESIAN_POINT ( 'NONE',  ( -5.823673210054116645, -21.52544592524344225, 62.29057627198102409 ) ) ;
#90222=CARTESIAN_POINT ( 'NONE',  ( -12.14591786802326823, 12.06949235617739902, 93.12609039468568994 ) ) ;
#90223=ORIENTED_EDGE ( 'NONE', *, *, #11874, .F. ) ;
#90224=CARTESIAN_POINT ( 'NONE',  ( -9.474510206698964154, 16.51473224551069663, 110.4155762719810383 ) ) ;
#90225=CARTESIAN_POINT ( 'NONE',  ( -18.39443945427639449, 5.500000000000031974, 73.51745347608654413 ) ) ;
#90226=CARTESIAN_POINT ( 'NONE',  ( -18.62759615963270932, 10.81492255796079327, 70.83224293864770971 ) ) ;
#90227=CARTESIAN_POINT ( 'NONE',  ( -4.483927247898782831, 16.52544592524335698, 97.70942372801904696 ) ) ;
#90228=CARTESIAN_POINT ( 'NONE',  ( 14.34966873604972726, -8.224510206698740333, 20.83442372801901143 ) ) ;
#90229=CARTESIAN_POINT ( 'NONE',  ( 13.89961937509977652, -13.97604488694527269, 23.12390960531436335 ) ) ;
#90230=CARTESIAN_POINT ( 'NONE',  ( 16.53943276465976808, 0.05219959533934440121, 31.25109039468568639 ) ) ;
#90231=CARTESIAN_POINT ( 'NONE',  ( -19.05341960407611168, -5.049401038298163336, 51.45724293864770260 ) ) ;
#90234=CARTESIAN_POINT ( 'NONE',  ( 19.03943276465977164, -0.05219959533909143690, 108.7489096053143527 ) ) ;
#90235=CARTESIAN_POINT ( 'NONE',  ( 16.52544592524335698, 4.483927247898782831, 91.45942372801901854 ) ) ;
#90236=CARTESIAN_POINT ( 'NONE',  ( -19.03943276465977164, -0.05219959533935918106, 88.75109039468567573 ) ) ;
#90237=CARTESIAN_POINT ( 'NONE',  ( -19.03943276465977164, -0.05219959533935918106, 23.75109039468566152 ) ) ;
#90238=CARTESIAN_POINT ( 'NONE',  ( -5.823673210054116645, -21.52544592524344225, 72.29057627198102409 ) ) ;
#90239=CARTESIAN_POINT ( 'NONE',  ( 16.53943276465976808, 0.05219959533934440121, 101.2510903946856757 ) ) ;
#90240=CARTESIAN_POINT ( 'NONE',  ( -13.89961937509957401, -13.97604488694547875, 94.37609039468566152 ) ) ;
#90241=CARTESIAN_POINT ( 'NONE',  ( 19.05341960407611168, 5.049401038298154454, 43.95724293864769550 ) ) ;
#90242=CARTESIAN_POINT ( 'NONE',  ( -19.02544592524342804, 5.153800228976336051, 96.04057627198103830 ) ) ;
#90243=CARTESIAN_POINT ( 'NONE',  ( 15.72974639402176855, 15.80617190586768217, 56.87609039468568994 ) ) ;
#90244=CARTESIAN_POINT ( 'NONE',  ( 13.89961937509977652, -13.97604488694527269, 63.12390960531435979 ) ) ;
#90245=CARTESIAN_POINT ( 'NONE',  ( -14.29746914071049879, 8.314922557960819915, 90.83224293864769550 ) ) ;
#90247=CARTESIAN_POINT ( 'NONE',  ( 16.53943276465976808, -0.05219959533910856209, 78.74890960531436690 ) ) ;
#90248=CARTESIAN_POINT ( 'NONE',  ( 0.05219959533907565091, 21.53943276465977519, 69.99890960531435269 ) ) ;
#90249=CARTESIAN_POINT ( 'NONE',  ( -9.474510206698720793, -16.51473224551083518, 94.58442372801900433 ) ) ;
#90251=CARTESIAN_POINT ( 'NONE',  ( -0.05219959533936034679, 19.03943276465977164, 42.50109039468566152 ) ) ;
#90253=CARTESIAN_POINT ( 'NONE',  ( -5.153800228976328057, -19.02544592524343514, 82.29057627198103830 ) ) ;
#90254=CARTESIAN_POINT ( 'NONE',  ( -19.05341960407611168, -5.049401038298163336, 86.45724293864769550 ) ) ;
#90255=CARTESIAN_POINT ( 'NONE',  ( 4.483927247898790824, -16.52544592524335698, 60.20942372801902565 ) ) ;
#90256=CARTESIAN_POINT ( 'NONE',  ( -17.44270441346514033, -5.991230190323107330, 51.36335079264230785 ) ) ;
#90257=CARTESIAN_POINT ( 'NONE',  ( 16.46253265017146816, 9.564922557961045513, 46.66775706135233293 ) ) ;
#90259=CARTESIAN_POINT ( 'NONE',  ( -16.46253265017160317, 9.564922557960807481, 105.8322429386476955 ) ) ;
#90260=CARTESIAN_POINT ( 'NONE',  ( -8.314922557961024197, 14.29746914071037800, 107.9177570613523471 ) ) ;
#90262=CARTESIAN_POINT ( 'NONE',  ( -16.52544592524335698, -4.483927247898792601, 83.95942372801900433 ) ) ;
#90264=CARTESIAN_POINT ( 'NONE',  ( -16.55341960407617563, 4.379528057220093196, 48.54275706135234714 ) ) ;
#90266=CARTESIAN_POINT ( 'NONE',  ( -10.81492255796105439, 18.62759615963255655, 72.91775706135234714 ) ) ;
#90267=CARTESIAN_POINT ( 'NONE',  ( 5.153800228976615827, -19.02544592524334988, 70.20942372801899012 ) ) ;
#90268=CARTESIAN_POINT ( 'NONE',  ( 9.474510206698729675, 16.51473224551082808, 22.08442372801899722 ) ) ;
#90269=CARTESIAN_POINT ( 'NONE',  ( 16.51473224551069308, 9.474510206698969483, 54.16557627198103120 ) ) ;
#90270=CARTESIAN_POINT ( 'NONE',  ( -5.153800228976328057, -19.02544592524343514, 42.29057627198101699 ) ) ;
#90272=CARTESIAN_POINT ( 'NONE',  ( 0.05219959533907565091, 21.53943276465977519, 64.99890960531435269 ) ) ;
#90273=CARTESIAN_POINT ( 'NONE',  ( -19.03943276465977164, 0.05219959533909376836, 111.2489096053143669 ) ) ;
#90274=CARTESIAN_POINT ( 'NONE',  ( -13.97604488694527625, -13.89961937509977652, 21.87390960531435979 ) ) ;
#90275=CARTESIAN_POINT ( 'NONE',  ( -4.483927247898782831, 16.52544592524335698, 47.70942372801902565 ) ) ;
#90276=ORIENTED_EDGE ( 'NONE', *, *, #150999, .F. ) ;
#90277=CARTESIAN_POINT ( 'NONE',  ( -15.80617190586745835, -15.72974639402198527, 111.8739096053143669 ) ) ;
#90278=CARTESIAN_POINT ( 'NONE',  ( 16.53943276465976808, -0.05219959533910856209, 53.74890960531437401 ) ) ;
#90280=CARTESIAN_POINT ( 'NONE',  ( 9.564922557961047289, -16.46253265017146816, 110.4177570613523471 ) ) ;
#90281=CARTESIAN_POINT ( 'NONE',  ( -13.97604488694547697, 13.89961937509957934, 43.12609039468566152 ) ) ;
#90282=CARTESIAN_POINT ( 'NONE',  ( -12.14591786802309592, -12.06949235617757132, 41.87390960531435979 ) ) ;
#90283=CARTESIAN_POINT ( 'NONE',  ( 0.05219959533907565091, 21.53943276465977519, 114.9989096053143669 ) ) ;
#90284=CARTESIAN_POINT ( 'NONE',  ( 16.52216118717206328, 7.221426719304519182, 33.57599021046992505 ) ) ;
#90285=CARTESIAN_POINT ( 'NONE',  ( -0.05219959533907301413, -21.53943276465977519, 67.49890960531436690 ) ) ;
#90286=CARTESIAN_POINT ( 'NONE',  ( 16.46253265017160672, -9.564922557960803928, 88.33224293864769550 ) ) ;
#90287=CARTESIAN_POINT ( 'NONE',  ( 4.379528057220339221, -16.55341960407611168, 62.70724293864769550 ) ) ;
#90288=CARTESIAN_POINT ( 'NONE',  ( -9.474510206698964154, 16.51473224551069663, 105.4155762719810383 ) ) ;
#90290=CARTESIAN_POINT ( 'NONE',  ( 19.03943276465977164, 0.05219959533936151252, 61.25109039468566863 ) ) ;
#90291=CARTESIAN_POINT ( 'NONE',  ( -18.62759615963270932, 10.81492255796079327, 110.8322429386476955 ) ) ;
#90292=CARTESIAN_POINT ( 'NONE',  ( 9.474510206698971260, -16.51473224551069308, 47.91557627198102409 ) ) ;
#90293=CARTESIAN_POINT ( 'NONE',  ( -8.224510206698948167, 14.34966873604960824, 110.4155762719810383 ) ) ;
#90294=CARTESIAN_POINT ( 'NONE',  ( 21.53943276465977519, 0.05219959533937863772, 56.25109039468568284 ) ) ;
#90296=CARTESIAN_POINT ( 'NONE',  ( -0.05219959533910754901, -16.53943276465976808, 32.49890960531435979 ) ) ;
#90297=CARTESIAN_POINT ( 'NONE',  ( 16.46253265017160672, -9.564922557960803928, 43.33224293864769550 ) ) ;
#90298=CARTESIAN_POINT ( 'NONE',  ( -5.049401038298153566, 19.05341960407611168, 105.2072429386476671 ) ) ;
#90299=CARTESIAN_POINT ( 'NONE',  ( -21.53943276465977519, 0.05219959533907696930, 76.24890960531435269 ) ) ;
#90301=CARTESIAN_POINT ( 'NONE',  ( 5.049401038298161559, -19.05341960407611168, 42.70724293864767418 ) ) ;
#90302=CARTESIAN_POINT ( 'NONE',  ( 15.72974639402199770, -15.80617190586745480, 48.12390960531436690 ) ) ;
#90303=CARTESIAN_POINT ( 'NONE',  ( 21.53943276465977519, 0.05219959533937863772, 81.25109039468568994 ) ) ;
#90305=CARTESIAN_POINT ( 'NONE',  ( -16.52544592524335698, -4.483927247898792601, 78.95942372801901854 ) ) ;
#90306=CARTESIAN_POINT ( 'NONE',  ( 4.379528057220339221, -16.55341960407611168, 72.70724293864769550 ) ) ;
#90307=CARTESIAN_POINT ( 'NONE',  ( -19.05341960407611168, -5.049401038298163336, 71.45724293864766707 ) ) ;
#90309=CARTESIAN_POINT ( 'NONE',  ( -5.049401038297874678, -19.05341960407617918, 24.79275706135233648 ) ) ;
#90310=CARTESIAN_POINT ( 'NONE',  ( 0.05219959533934541429, -16.53943276465976808, 90.00109039468567573 ) ) ;
#90311=CARTESIAN_POINT ( 'NONE',  ( -5.823673210054431948, 21.52544592524334988, 112.7094237280190328 ) ) ;
#90312=CARTESIAN_POINT ( 'NONE',  ( -13.89961937509977652, 13.97604488694528158, 70.62390960531432427 ) ) ;
#90313=CARTESIAN_POINT ( 'NONE',  ( 21.53943276465977519, -0.05219959533907433946, 53.74890960531437401 ) ) ;
#90314=CARTESIAN_POINT ( 'NONE',  ( -16.52544592524335698, -4.483927247898792601, 18.95942372801901143 ) ) ;
#90315=CARTESIAN_POINT ( 'NONE',  ( 0.05219959533937995610, -21.53943276465977519, 95.00109039468568994 ) ) ;
#90316=CARTESIAN_POINT ( 'NONE',  ( 4.483927247898790824, -16.52544592524335698, 65.20942372801901854 ) ) ;
#90317=CARTESIAN_POINT ( 'NONE',  ( 15.80617190586746368, 15.72974639402197994, 109.3739096053143811 ) ) ;
#90318=CARTESIAN_POINT ( 'NONE',  ( 14.29746914071037800, 8.314922557961029526, 21.66775706135235069 ) ) ;
#90319=CARTESIAN_POINT ( 'NONE',  ( 16.46253265017160672, -9.564922557960803928, 88.33224293864769550 ) ) ;
#90320=CARTESIAN_POINT ( 'NONE',  ( 4.379528057220092307, 16.55341960407617563, 22.29275706135235069 ) ) ;
#90321=CARTESIAN_POINT ( 'NONE',  ( -5.153800228976328057, -19.02544592524343514, 52.29057627198100988 ) ) ;
#90322=VECTOR ( 'NONE', #51417, 999.9999999999998863 ) ;
#90323=CARTESIAN_POINT ( 'NONE',  ( -4.483927247898782831, 16.52544592524335698, 37.70942372801900433 ) ) ;
#90324=CARTESIAN_POINT ( 'NONE',  ( -8.314922557960811034, -14.29746914071050412, 77.08224293864769550 ) ) ;
#90325=CARTESIAN_POINT ( 'NONE',  ( 16.55341960407618274, -4.379528057220086978, 91.04275706135236135 ) ) ;
#90326=CARTESIAN_POINT ( 'NONE',  ( 21.52544592524334988, 5.823673210054432836, 36.45942372801901143 ) ) ;
#90327=CARTESIAN_POINT ( 'NONE',  ( -16.46253265017160317, 9.564922557960807481, 70.83224293864770971 ) ) ;
#90328=CARTESIAN_POINT ( 'NONE',  ( 9.474510206698971260, -16.51473224551069308, 77.91557627198103830 ) ) ;
#90329=CARTESIAN_POINT ( 'NONE',  ( -12.06949235617739369, -12.14591786802326823, 89.37609039468568994 ) ) ;
#90333=CARTESIAN_POINT ( 'NONE',  ( -16.51473224551082808, 9.474510206698731452, 33.33442372801899722 ) ) ;
#90334=CARTESIAN_POINT ( 'NONE',  ( 13.89961937509977652, -13.97604488694527269, 93.12390960531436690 ) ) ;
#90335=CARTESIAN_POINT ( 'NONE',  ( -9.474510206698964154, 16.51473224551069663, 45.41557627198103120 ) ) ;
#90336=CARTESIAN_POINT ( 'NONE',  ( -9.474510206698964154, 16.51473224551069663, 115.4155762719810241 ) ) ;
#90337=CARTESIAN_POINT ( 'NONE',  ( 16.53943276465976808, 0.05219959533934440121, 46.25109039468567573 ) ) ;
#90338=CARTESIAN_POINT ( 'NONE',  ( 16.46253265017146816, 9.564922557961045513, 56.66775706135233293 ) ) ;
#90339=CARTESIAN_POINT ( 'NONE',  ( 14.29746914071037800, 8.314922557961029526, 41.66775706135235424 ) ) ;
#90340=CARTESIAN_POINT ( 'NONE',  ( -9.474510206698964154, 16.51473224551069663, 105.4155762719810383 ) ) ;
#90341=CARTESIAN_POINT ( 'NONE',  ( -9.474510206698964154, 16.51473224551069663, 75.41557627198103830 ) ) ;
#90342=CARTESIAN_POINT ( 'NONE',  ( -10.81492255796078084, -18.62759615963271287, 97.08224293864770971 ) ) ;
#90343=CARTESIAN_POINT ( 'NONE',  ( -5.153800228976607833, 19.02544592524334988, 67.70942372801900433 ) ) ;
#90344=CARTESIAN_POINT ( 'NONE',  ( -9.564922557960796823, -16.46253265017161027, 87.08224293864769550 ) ) ;
#90346=CARTESIAN_POINT ( 'NONE',  ( -5.049401038298153566, 19.05341960407611168, 70.20724293864769550 ) ) ;
#90347=CARTESIAN_POINT ( 'NONE',  ( 14.29746914071049879, -8.314922557960816363, 33.33224293864769550 ) ) ;
#90348=CARTESIAN_POINT ( 'NONE',  ( 18.22780087662121673, 5.500000000000056843, 68.98459894673892734 ) ) ;
#90349=EDGE_CURVE ( 'NONE', #21815, #72076, #91067, .T. ) ;
#90350=CARTESIAN_POINT ( 'NONE',  ( 9.564922557961047289, -16.46253265017146816, 40.41775706135234003 ) ) ;
#90351=CARTESIAN_POINT ( 'NONE',  ( 16.53943276465976808, -0.05219959533910856209, 78.74890960531436690 ) ) ;
#90352=CARTESIAN_POINT ( 'NONE',  ( -15.80617190586768217, 15.72974639402176855, 98.12609039468570415 ) ) ;
#90353=CARTESIAN_POINT ( 'NONE',  ( 9.564922557960805705, 16.46253265017160317, 34.58224293864770260 ) ) ;
#90354=CARTESIAN_POINT ( 'NONE',  ( 14.34966873604972726, -8.224510206698740333, 55.83442372801901854 ) ) ;
#90355=CARTESIAN_POINT ( 'NONE',  ( -8.314922557960811034, -14.29746914071050412, 42.08224293864769550 ) ) ;
#90356=CARTESIAN_POINT ( 'NONE',  ( 5.823673210054444382, -21.52544592524334988, 105.2094237280190328 ) ) ;
#90357=CARTESIAN_POINT ( 'NONE',  ( 5.049401038298161559, -19.05341960407611168, 97.70724293864766707 ) ) ;
#90358=CARTESIAN_POINT ( 'NONE',  ( 19.02544592524343514, -5.153800228976328945, 88.54057627198102409 ) ) ;
#90359=CARTESIAN_POINT ( 'NONE',  ( 9.564922557960805705, 16.46253265017160317, 24.58224293864769194 ) ) ;
#90360=CARTESIAN_POINT ( 'NONE',  ( 16.55341960407611168, 4.379528057220329451, 108.9572429386476955 ) ) ;
#90361=CARTESIAN_POINT ( 'NONE',  ( -16.53943276465976808, 0.05219959533911058130, 71.24890960531435269 ) ) ;
#90362=CARTESIAN_POINT ( 'NONE',  ( 5.719274019375991003, -21.55341960407610458, 82.70724293864770971 ) ) ;
#90363=CARTESIAN_POINT ( 'NONE',  ( 19.02544592524343514, -5.153800228976328945, 83.54057627198100988 ) ) ;
#90364=CARTESIAN_POINT ( 'NONE',  ( -21.52544592524343514, 5.823673210054127303, 96.04057627198102409 ) ) ;
#90365=CARTESIAN_POINT ( 'NONE',  ( -13.89961937509977652, 13.97604488694528158, 95.62390960531436690 ) ) ;
#90366=CARTESIAN_POINT ( 'NONE',  ( 19.52217212775657984, -5.500000000000105693, 47.43993709005262360 ) ) ;
#90367=CARTESIAN_POINT ( 'NONE',  ( 14.29746914071049879, -8.314922557960816363, 93.33224293864769550 ) ) ;
#90368=CARTESIAN_POINT ( 'NONE',  ( 5.153800228976335163, 19.02544592524342804, 64.79057627198100988 ) ) ;
#90369=CARTESIAN_POINT ( 'NONE',  ( -18.67979575497178146, -10.72451020669898902, 66.66557627198102409 ) ) ;
#90370=DIRECTION ( 'NONE',  ( 0.5150380749100522682, 1.049727191138620051E-16, 0.8571673007021134438 ) ) ;
#90371=CARTESIAN_POINT ( 'NONE',  ( 14.34966873604972726, -8.224510206698740333, 110.8344237280190043 ) ) ;
#90373=CARTESIAN_POINT ( 'NONE',  ( 4.483927247898790824, -16.52544592524335698, 20.20942372801900788 ) ) ;
#90374=CARTESIAN_POINT ( 'NONE',  ( -4.379528057220328563, 16.55341960407611168, 90.20724293864770971 ) ) ;
#90375=CARTESIAN_POINT ( 'NONE',  ( -16.88567814943165502, -6.947325034625643880, 96.29001122652589117 ) ) ;
#90376=CARTESIAN_POINT ( 'NONE',  ( -16.51473224551069308, -9.474510206698971260, 81.66557627198103830 ) ) ;
#90377=CARTESIAN_POINT ( 'NONE',  ( -9.564922557960796823, -16.46253265017161027, 42.08224293864769550 ) ) ;
#90378=CARTESIAN_POINT ( 'NONE',  ( -16.53943276465976808, 0.05219959533911058130, 61.24890960531435979 ) ) ;
#90379=CARTESIAN_POINT ( 'NONE',  ( 16.46253265017160672, -9.564922557960803928, 108.3322429386476955 ) ) ;
#90380=CARTESIAN_POINT ( 'NONE',  ( 13.89961937509957401, 13.97604488694547697, 101.8760903946856331 ) ) ;
#90381=CARTESIAN_POINT ( 'NONE',  ( -21.53943276465977519, -0.05219959533937600094, 58.75109039468568994 ) ) ;
#90382=CARTESIAN_POINT ( 'NONE',  ( 19.05341960407611168, 5.049401038298154454, 93.95724293864769550 ) ) ;
#90383=CARTESIAN_POINT ( 'NONE',  ( -10.81492255796078084, -18.62759615963271287, 77.08224293864769550 ) ) ;
#90384=CARTESIAN_POINT ( 'NONE',  ( -8.224510206698735004, -14.34966873604973081, 64.58442372801900433 ) ) ;
#90386=CARTESIAN_POINT ( 'NONE',  ( -16.46253265017160317, 9.564922557960807481, 70.83224293864770971 ) ) ;
#90387=CARTESIAN_POINT ( 'NONE',  ( -21.53943276465977519, 0.05219959533907696930, 76.24890960531435269 ) ) ;
#90388=CARTESIAN_POINT ( 'NONE',  ( -5.049401038297874678, -19.05341960407617918, 104.7927570613523471 ) ) ;
#90389=CARTESIAN_POINT ( 'NONE',  ( 16.55341960407611168, 4.379528057220329451, 43.95724293864769550 ) ) ;
#90390=CARTESIAN_POINT ( 'NONE',  ( 21.55341960407619695, -5.719274019375665929, 66.04275706135236135 ) ) ;
#90392=CARTESIAN_POINT ( 'NONE',  ( 14.29746914071037800, 8.314922557961029526, 86.66775706135234714 ) ) ;
#90393=CARTESIAN_POINT ( 'NONE',  ( 21.53943276465977519, -0.05219959533907433946, 23.74890960531435269 ) ) ;
#90394=CARTESIAN_POINT ( 'NONE',  ( -5.153800228976328057, -19.02544592524343514, 107.2905762719810383 ) ) ;
#90395=CARTESIAN_POINT ( 'NONE',  ( 17.49999999999999645, -5.500000000000031974, 93.29690382534172954 ) ) ;
#90396=CARTESIAN_POINT ( 'NONE',  ( 16.53943276465976808, 0.05219959533934440121, 111.2510903946856899 ) ) ;
#90397=CARTESIAN_POINT ( 'NONE',  ( -8.314922557961024197, 14.29746914071037800, 42.91775706135235424 ) ) ;
#90398=CARTESIAN_POINT ( 'NONE',  ( 16.51473224551069308, 9.474510206698969483, 59.16557627198102409 ) ) ;
#90399=CARTESIAN_POINT ( 'NONE',  ( 5.049401038298161559, -19.05341960407611168, 67.70724293864769550 ) ) ;
#90400=CARTESIAN_POINT ( 'NONE',  ( -8.224510206698735004, -14.34966873604973081, 64.58442372801900433 ) ) ;
#90401=CARTESIAN_POINT ( 'NONE',  ( 8.314922557960818139, 14.29746914071049879, 44.58224293864769550 ) ) ;
#90402=CARTESIAN_POINT ( 'NONE',  ( 5.153800228976335163, 19.02544592524342804, 59.79057627198100988 ) ) ;
#90403=CARTESIAN_POINT ( 'NONE',  ( -16.51473224551069308, -9.474510206698971260, 46.66557627198102409 ) ) ;
#90404=CARTESIAN_POINT ( 'NONE',  ( -8.224510206698735004, -14.34966873604973081, 44.58442372801901854 ) ) ;
#90405=VERTEX_POINT ( 'NONE', #90395 ) ;
#90406=CARTESIAN_POINT ( 'NONE',  ( -5.153800228976607833, 19.02544592524334988, 97.70942372801900433 ) ) ;
#90407=CARTESIAN_POINT ( 'NONE',  ( 8.224510206698953496, -14.34966873604960469, 92.91557627198103830 ) ) ;
#90408=CARTESIAN_POINT ( 'NONE',  ( -19.05341960407611168, -5.049401038298163336, 71.45724293864766707 ) ) ;
#90409=CARTESIAN_POINT ( 'NONE',  ( 19.03943276465977164, 0.05219959533936151252, 96.25109039468567573 ) ) ;
#90411=CARTESIAN_POINT ( 'NONE',  ( 21.53943276465977519, 0.05219959533937863772, 96.25109039468568994 ) ) ;
#90412=CARTESIAN_POINT ( 'NONE',  ( 8.224510206698742110, 14.34966873604972548, 72.08442372801899012 ) ) ;
#90414=CARTESIAN_POINT ( 'NONE',  ( 21.53943276465977519, -0.05219959533907433946, 58.74890960531436690 ) ) ;
#90415=CARTESIAN_POINT ( 'NONE',  ( 8.224510206698742110, 14.34966873604972548, 47.08442372801901854 ) ) ;
#90416=CARTESIAN_POINT ( 'NONE',  ( -19.03943276465977164, 0.05219959533909376836, 31.24890960531435979 ) ) ;
#90417=CARTESIAN_POINT ( 'NONE',  ( -13.97604488694547697, 13.89961937509957934, 43.12609039468566152 ) ) ;
#90418=CARTESIAN_POINT ( 'NONE',  ( 9.564922557960805705, 16.46253265017160317, 89.58224293864769550 ) ) ;
#90419=CARTESIAN_POINT ( 'NONE',  ( -16.51473224551069308, -9.474510206698971260, 26.66557627198103120 ) ) ;
#90420=CARTESIAN_POINT ( 'NONE',  ( 5.049401038298161559, -19.05341960407611168, 62.70724293864769550 ) ) ;
#90422=CARTESIAN_POINT ( 'NONE',  ( -21.55341960407619339, 5.719274019375674811, 73.54275706135234714 ) ) ;
#90423=CARTESIAN_POINT ( 'NONE',  ( -17.72560187377287022, -5.499999999999974243, 89.07814504131324895 ) ) ;
#90424=CARTESIAN_POINT ( 'NONE',  ( -5.049401038297874678, -19.05341960407617918, 29.79275706135232227 ) ) ;
#90425=CARTESIAN_POINT ( 'NONE',  ( 9.564922557961047289, -16.46253265017146816, 30.41775706135232937 ) ) ;
#90426=CARTESIAN_POINT ( 'NONE',  ( 8.314922557960818139, 14.29746914071049879, 54.58224293864769550 ) ) ;
#90427=CARTESIAN_POINT ( 'NONE',  ( 13.97604488694527802, 13.89961937509977652, 59.37390960531434558 ) ) ;
#90428=CARTESIAN_POINT ( 'NONE',  ( 21.52544592524344225, -5.823673210054117533, 28.54057627198103120 ) ) ;
#90429=CARTESIAN_POINT ( 'NONE',  ( -5.719274019375665041, -21.55341960407619695, 79.79275706135236135 ) ) ;
#90430=CARTESIAN_POINT ( 'NONE',  ( -13.97604488694527625, -13.89961937509977652, 61.87390960531435979 ) ) ;
#90431=CARTESIAN_POINT ( 'NONE',  ( -15.80617190586768217, 15.72974639402176855, 78.12609039468570415 ) ) ;
#90432=CARTESIAN_POINT ( 'NONE',  ( 21.53943276465977519, -0.05219959533907433946, 38.74890960531435979 ) ) ;
#90433=CARTESIAN_POINT ( 'NONE',  ( -13.89961937509977652, 13.97604488694528158, 65.62390960531436690 ) ) ;
#90434=CARTESIAN_POINT ( 'NONE',  ( -0.05219959533937732626, 21.53943276465977519, 37.50109039468568284 ) ) ;
#90435=CARTESIAN_POINT ( 'NONE',  ( -5.153800228976607833, 19.02544592524334988, 57.70942372801899012 ) ) ;
#90436=CARTESIAN_POINT ( 'NONE',  ( 19.03943276465977164, -0.05219959533909143690, 48.74890960531435979 ) ) ;
#90437=CARTESIAN_POINT ( 'NONE',  ( 13.89961937509977652, -13.97604488694527269, 78.12390960531433848 ) ) ;
#90438=CARTESIAN_POINT ( 'NONE',  ( -8.314922557961024197, 14.29746914071037800, 27.91775706135234358 ) ) ;
#90439=CARTESIAN_POINT ( 'NONE',  ( 4.379528057220339221, -16.55341960407611168, 82.70724293864770971 ) ) ;
#90440=CARTESIAN_POINT ( 'NONE',  ( 9.474510206698971260, -16.51473224551069308, 52.91557627198102409 ) ) ;
#90441=CARTESIAN_POINT ( 'NONE',  ( -10.81492255796078084, -18.62759615963271287, 47.08224293864770260 ) ) ;
#90443=CARTESIAN_POINT ( 'NONE',  ( -0.05219959533936034679, 19.03943276465977164, 112.5010903946856757 ) ) ;
#90444=CARTESIAN_POINT ( 'NONE',  ( 15.72974639402176855, 15.80617190586768217, 21.87609039468567573 ) ) ;
#90445=CARTESIAN_POINT ( 'NONE',  ( 18.62759615963255655, 10.81492255796105972, 76.66775706135234714 ) ) ;
#90446=CARTESIAN_POINT ( 'NONE',  ( -0.05219959533934338120, 16.53943276465976808, 67.50109039468568994 ) ) ;
#90447=CARTESIAN_POINT ( 'NONE',  ( 16.52544592524335698, 4.483927247898782831, 71.45942372801901854 ) ) ;
#90449=CARTESIAN_POINT ( 'NONE',  ( 16.46253265017160672, -9.564922557960803928, 63.33224293864769550 ) ) ;
#90450=CARTESIAN_POINT ( 'NONE',  ( -4.379528057220086978, -16.55341960407618274, 94.79275706135234714 ) ) ;
#90451=CARTESIAN_POINT ( 'NONE',  ( 0.05219959533936267826, -19.03943276465977164, 40.00109039468566152 ) ) ;
#90452=CARTESIAN_POINT ( 'NONE',  ( -15.72974639402176322, -15.80617190586768395, 24.37609039468567573 ) ) ;
#90453=CARTESIAN_POINT ( 'NONE',  ( 16.55341960407611168, 4.379528057220329451, 68.95724293864769550 ) ) ;
#90454=CARTESIAN_POINT ( 'NONE',  ( 5.153800228976335163, 19.02544592524342804, 89.79057627198102409 ) ) ;
#90455=CARTESIAN_POINT ( 'NONE',  ( -12.14591786802326823, 12.06949235617739902, 93.12609039468568994 ) ) ;
#90456=CARTESIAN_POINT ( 'NONE',  ( -21.52544592524334988, -5.823673210054445271, 53.95942372801900433 ) ) ;
#90457=CARTESIAN_POINT ( 'NONE',  ( -8.224510206698735004, -14.34966873604973081, 29.58442372801901854 ) ) ;
#90458=CARTESIAN_POINT ( 'NONE',  ( 5.719274019375673035, 21.55341960407619339, 32.29275706135235424 ) ) ;
#90459=CARTESIAN_POINT ( 'NONE',  ( 12.14591786802309770, 12.06949235617756955, 54.37390960531435979 ) ) ;
#90461=CARTESIAN_POINT ( 'NONE',  ( -21.52544592524343514, 5.823673210054127303, 96.04057627198102409 ) ) ;
#90462=CARTESIAN_POINT ( 'NONE',  ( 4.379528057220339221, -16.55341960407611168, 42.70724293864770260 ) ) ;
#90465=CARTESIAN_POINT ( 'NONE',  ( -21.53943276465977519, 0.05219959533907696930, 26.24890960531435624 ) ) ;
#90466=CARTESIAN_POINT ( 'NONE',  ( -18.67979575497193778, 10.72451020669871902, 38.33442372801900433 ) ) ;
#90467=CARTESIAN_POINT ( 'NONE',  ( 16.55341960407611168, 4.379528057220329451, 68.95724293864769550 ) ) ;
#90469=CARTESIAN_POINT ( 'NONE',  ( -9.564922557960796823, -16.46253265017161027, 67.08224293864769550 ) ) ;
#90470=CARTESIAN_POINT ( 'NONE',  ( -13.97604488694527625, -13.89961937509977652, 21.87390960531435979 ) ) ;
#90471=CARTESIAN_POINT ( 'NONE',  ( -16.46253265017146816, -9.564922557961047289, 64.16775706135233293 ) ) ;
#90473=CARTESIAN_POINT ( 'NONE',  ( 18.62759615963271287, -10.81492255796078972, 43.33224293864769550 ) ) ;
#90475=CARTESIAN_POINT ( 'NONE',  ( 5.153800228976335163, 19.02544592524342804, 54.79057627198103120 ) ) ;
#90476=CARTESIAN_POINT ( 'NONE',  ( -0.05219959533934338120, 16.53943276465976808, 37.50109039468568284 ) ) ;
#90477=CARTESIAN_POINT ( 'NONE',  ( 5.823673210054125526, 21.52544592524343514, 114.7905762719810383 ) ) ;
#90478=CARTESIAN_POINT ( 'NONE',  ( -8.314922557960811034, -14.29746914071050412, 47.08224293864770260 ) ) ;
#90479=ORIENTED_EDGE ( 'NONE', *, *, #44009, .T. ) ;
#90480=CARTESIAN_POINT ( 'NONE',  ( 9.474510206698971260, -16.51473224551069308, 92.91557627198103830 ) ) ;
#90481=CARTESIAN_POINT ( 'NONE',  ( 10.81492255796078972, 18.62759615963270932, 74.58224293864768129 ) ) ;
#90482=CARTESIAN_POINT ( 'NONE',  ( -5.823673210054116645, -21.52544592524344225, 112.2905762719810241 ) ) ;
#90483=CARTESIAN_POINT ( 'NONE',  ( -14.34966873604972548, 8.224510206698743886, 43.33442372801901143 ) ) ;
#90484=CARTESIAN_POINT ( 'NONE',  ( 15.72974639402199770, -15.80617190586745480, 43.12390960531435269 ) ) ;
#90485=CARTESIAN_POINT ( 'NONE',  ( 21.52544592524334988, 5.823673210054432836, 106.4594237280190328 ) ) ;
#90486=CARTESIAN_POINT ( 'NONE',  ( -13.97604488694527625, -13.89961937509977652, 96.87390960531433848 ) ) ;
#90487=CARTESIAN_POINT ( 'NONE',  ( -16.51473224551069308, -9.474510206698971260, 46.66557627198102409 ) ) ;
#90488=CARTESIAN_POINT ( 'NONE',  ( -19.05341960407611168, -5.049401038298163336, 96.45724293864769550 ) ) ;
#90489=CARTESIAN_POINT ( 'NONE',  ( -9.564922557960796823, -16.46253265017161027, 82.08224293864768129 ) ) ;
#90490=CARTESIAN_POINT ( 'NONE',  ( 16.81555441253471983, -7.025013491696154411, 88.13685445334212432 ) ) ;
#90491=CARTESIAN_POINT ( 'NONE',  ( 19.02544592524334988, 5.153800228976608722, 61.45942372801900433 ) ) ;
#90492=CARTESIAN_POINT ( 'NONE',  ( 18.67979575497194134, -10.72451020669871369, 105.8344237280190328 ) ) ;
#90493=CARTESIAN_POINT ( 'NONE',  ( 18.67979575497178502, 10.72451020669898547, 34.16557627198102409 ) ) ;
#90494=CARTESIAN_POINT ( 'NONE',  ( -0.05219959533934338120, 16.53943276465976808, 107.5010903946856899 ) ) ;
#90495=CARTESIAN_POINT ( 'NONE',  ( 16.46253265017146816, 9.564922557961045513, 81.66775706135233293 ) ) ;
#90496=CARTESIAN_POINT ( 'NONE',  ( 18.22780087662121673, 5.500000000000056843, 38.98459894673893444 ) ) ;
#90497=CARTESIAN_POINT ( 'NONE',  ( -0.05219959533936034679, 19.03943276465977164, 87.50109039468567573 ) ) ;
#90498=CARTESIAN_POINT ( 'NONE',  ( 13.89961937509957401, 13.97604488694547697, 36.87609039468565442 ) ) ;
#90499=CARTESIAN_POINT ( 'NONE',  ( -16.29526858892878849, -7.335722546920001363, 45.79670597800205201 ) ) ;
#90500=CARTESIAN_POINT ( 'NONE',  ( -19.03943276465977164, 0.05219959533909376836, 46.24890960531435979 ) ) ;
#90501=CARTESIAN_POINT ( 'NONE',  ( -14.29746914071049879, 8.314922557960819915, 50.83224293864770971 ) ) ;
#90502=CARTESIAN_POINT ( 'NONE',  ( -5.049401038298153566, 19.05341960407611168, 25.20724293864768484 ) ) ;
#90503=CARTESIAN_POINT ( 'NONE',  ( -16.52544592524342804, 4.483927247898546575, 26.04057627198103475 ) ) ;
#90505=CARTESIAN_POINT ( 'NONE',  ( -16.52544592524335698, -4.483927247898792601, 88.95942372801901854 ) ) ;
#90506=CARTESIAN_POINT ( 'NONE',  ( 0.05219959533909260263, 19.03943276465977164, 44.99890960531435979 ) ) ;
#90507=CARTESIAN_POINT ( 'NONE',  ( 21.53943276465977519, 0.05219959533937863772, 111.2510903946856899 ) ) ;
#90508=CARTESIAN_POINT ( 'NONE',  ( 16.55341960407618274, -4.379528057220086978, 26.04275706135235779 ) ) ;
#90509=CARTESIAN_POINT ( 'NONE',  ( -15.72974639402176322, -15.80617190586768395, 94.37609039468568994 ) ) ;
#90511=CARTESIAN_POINT ( 'NONE',  ( -5.153800228976328057, -19.02544592524343514, 92.29057627198099567 ) ) ;
#90512=CARTESIAN_POINT ( 'NONE',  ( 9.474510206698971260, -16.51473224551069308, 77.91557627198103830 ) ) ;
#90514=CARTESIAN_POINT ( 'NONE',  ( -18.62759615963270932, 10.81492255796079327, 115.8322429386477097 ) ) ;
#90515=CARTESIAN_POINT ( 'NONE',  ( 16.55341960407611168, 4.379528057220329451, 73.95724293864769550 ) ) ;
#90516=CARTESIAN_POINT ( 'NONE',  ( 21.53943276465977519, -0.05219959533907433946, 68.74890960531435269 ) ) ;
#90517=CARTESIAN_POINT ( 'NONE',  ( 9.564922557960805705, 16.46253265017160317, 54.58224293864769550 ) ) ;
#90518=CARTESIAN_POINT ( 'NONE',  ( 5.719274019375991003, -21.55341960407610458, 97.70724293864772392 ) ) ;
#90519=CARTESIAN_POINT ( 'NONE',  ( -12.06949235617739369, -12.14591786802326823, 94.37609039468568994 ) ) ;
#90521=CARTESIAN_POINT ( 'NONE',  ( -9.474510206698964154, 16.51473224551069663, 60.41557627198102409 ) ) ;
#90522=CARTESIAN_POINT ( 'NONE',  ( -16.55341960407611168, -4.379528057220339221, 86.45724293864770971 ) ) ;
#90524=CARTESIAN_POINT ( 'NONE',  ( 13.97604488694527802, 13.89961937509977652, 69.37390960531436690 ) ) ;
#90525=CARTESIAN_POINT ( 'NONE',  ( -19.02544592524334988, -5.153800228976617603, 83.95942372801901854 ) ) ;
#90526=CARTESIAN_POINT ( 'NONE',  ( -4.379528057220328563, 16.55341960407611168, 80.20724293864769550 ) ) ;
#90527=CARTESIAN_POINT ( 'NONE',  ( -5.719274019375665041, -21.55341960407619695, 64.79275706135234714 ) ) ;
#90528=CARTESIAN_POINT ( 'NONE',  ( -16.51473224551069308, -9.474510206698971260, 41.66557627198103120 ) ) ;
#90529=CARTESIAN_POINT ( 'NONE',  ( 21.52544592524344225, -5.823673210054117533, 113.5405762719810383 ) ) ;
#90530=CARTESIAN_POINT ( 'NONE',  ( -8.314922557960811034, -14.29746914071050412, 107.0822429386476955 ) ) ;
#90532=CARTESIAN_POINT ( 'NONE',  ( 9.474510206698971260, -16.51473224551069308, 62.91557627198102409 ) ) ;
#90533=CARTESIAN_POINT ( 'NONE',  ( 17.12812012977027010, 6.668231424565983723, 113.8594875932314636 ) ) ;
#90534=CARTESIAN_POINT ( 'NONE',  ( -5.153800228976607833, 19.02544592524334988, 92.70942372801901854 ) ) ;
#90535=CARTESIAN_POINT ( 'NONE',  ( 19.03943276465977164, -0.05219959533909143690, 108.7489096053143527 ) ) ;
#90536=CARTESIAN_POINT ( 'NONE',  ( 0.05219959533937995610, -21.53943276465977519, 45.00109039468568284 ) ) ;
#90537=CARTESIAN_POINT ( 'NONE',  ( 13.97604488694527802, 13.89961937509977652, 84.37390960531433848 ) ) ;
#90538=CARTESIAN_POINT ( 'NONE',  ( 5.049401038297881783, 19.05341960407617563, 72.29275706135234714 ) ) ;
#90539=CARTESIAN_POINT ( 'NONE',  ( -13.89961937509977652, 13.97604488694528158, 60.62390960531436690 ) ) ;
#90540=CARTESIAN_POINT ( 'NONE',  ( -4.483927247898539470, -16.52544592524342804, 77.29057627198102409 ) ) ;
#90541=CARTESIAN_POINT ( 'NONE',  ( 4.483927247898545687, 16.52544592524342804, 79.79057627198102409 ) ) ;
#90542=CARTESIAN_POINT ( 'NONE',  ( -19.02544592524342804, 5.153800228976336051, 86.04057627198103830 ) ) ;
#90543=CARTESIAN_POINT ( 'NONE',  ( -14.34966873604960291, -8.224510206698953496, 81.66557627198103830 ) ) ;
#90544=CARTESIAN_POINT ( 'NONE',  ( 5.049401038298161559, -19.05341960407611168, 87.70724293864769550 ) ) ;
#90545=CARTESIAN_POINT ( 'NONE',  ( 9.564922557961047289, -16.46253265017146816, 35.41775706135233293 ) ) ;
#90546=CARTESIAN_POINT ( 'NONE',  ( 5.153800228976335163, 19.02544592524342804, 54.79057627198103120 ) ) ;
#90547=CARTESIAN_POINT ( 'NONE',  ( -12.06949235617756955, 12.14591786802309770, 30.62390960531436335 ) ) ;
#90548=CARTESIAN_POINT ( 'NONE',  ( 14.29746914071049879, -8.314922557960816363, 113.3322429386476955 ) ) ;
#90550=CARTESIAN_POINT ( 'NONE',  ( -15.80617190586768217, 15.72974639402176855, 48.12609039468568284 ) ) ;
#90551=CARTESIAN_POINT ( 'NONE',  ( -16.51473224551082808, 9.474510206698731452, 63.33442372801900433 ) ) ;
#90552=CARTESIAN_POINT ( 'NONE',  ( -16.52544592524342804, 4.483927247898546575, 36.04057627198102409 ) ) ;
#90553=CARTESIAN_POINT ( 'NONE',  ( -5.823673210054116645, -21.52544592524344225, 87.29057627198103830 ) ) ;
#90554=CARTESIAN_POINT ( 'NONE',  ( -13.89961937509977652, 13.97604488694528158, 110.6239096053143243 ) ) ;
#90555=CARTESIAN_POINT ( 'NONE',  ( -4.379528057220328563, 16.55341960407611168, 65.20724293864768129 ) ) ;
#90556=CARTESIAN_POINT ( 'NONE',  ( -16.51473224551069308, -9.474510206698971260, 41.66557627198103120 ) ) ;
#90557=CARTESIAN_POINT ( 'NONE',  ( -9.474510206698720793, -16.51473224551083518, 44.58442372801900433 ) ) ;
#90558=CARTESIAN_POINT ( 'NONE',  ( -12.06949235617739369, -12.14591786802326823, 104.3760903946856899 ) ) ;
#90559=CARTESIAN_POINT ( 'NONE',  ( 12.06949235617739724, 12.14591786802326823, 51.87609039468568284 ) ) ;
#90560=CARTESIAN_POINT ( 'NONE',  ( 18.62759615963271287, -10.81492255796078972, 33.33224293864769550 ) ) ;
#90561=CARTESIAN_POINT ( 'NONE',  ( -5.719274019375665041, -21.55341960407619695, 104.7927570613523898 ) ) ;
#90562=CARTESIAN_POINT ( 'NONE',  ( -19.05341960407611168, -5.049401038298163336, 86.45724293864769550 ) ) ;
#90563=CARTESIAN_POINT ( 'NONE',  ( 4.483927247898790824, -16.52544592524335698, 80.20942372801901854 ) ) ;
#90564=CARTESIAN_POINT ( 'NONE',  ( 14.29746914071049879, -8.314922557960816363, 113.3322429386476955 ) ) ;
#90565=CARTESIAN_POINT ( 'NONE',  ( 4.483927247898545687, 16.52544592524342804, 29.79057627198102409 ) ) ;
#90566=CARTESIAN_POINT ( 'NONE',  ( 16.46253265017160672, -9.564922557960803928, 108.3322429386476955 ) ) ;
#90567=CARTESIAN_POINT ( 'NONE',  ( 19.03943276465977164, -0.05219959533909143690, 88.74890960531436690 ) ) ;
#90568=CARTESIAN_POINT ( 'NONE',  ( 21.52544592524344225, -5.823673210054117533, 33.54057627198102409 ) ) ;
#90569=CARTESIAN_POINT ( 'NONE',  ( 8.224510206698953496, -14.34966873604960469, 67.91557627198102409 ) ) ;
#90571=CARTESIAN_POINT ( 'NONE',  ( 14.29746914071049879, -8.314922557960816363, 53.33224293864769550 ) ) ;
#90573=CARTESIAN_POINT ( 'NONE',  ( -12.14591786802326823, 12.06949235617739902, 58.12609039468568994 ) ) ;
#90574=FACE_OUTER_BOUND ( 'NONE', #163655, .T. ) ;
#90575=CARTESIAN_POINT ( 'NONE',  ( -9.474510206698720793, -16.51473224551083518, 49.58442372801899722 ) ) ;
#90576=CARTESIAN_POINT ( 'NONE',  ( -0.05219959533909027116, -19.03943276465977164, 92.49890960531436690 ) ) ;
#90577=CARTESIAN_POINT ( 'NONE',  ( -13.97604488694547697, 13.89961937509957934, 63.12609039468566152 ) ) ;
#90579=CARTESIAN_POINT ( 'NONE',  ( -13.97604488694547697, 13.89961937509957934, 53.12609039468565442 ) ) ;
#90580=CARTESIAN_POINT ( 'NONE',  ( 9.564922557961047289, -16.46253265017146816, 100.4177570613523329 ) ) ;
#90581=CARTESIAN_POINT ( 'NONE',  ( 8.224510206698742110, 14.34966873604972548, 102.0844237280190185 ) ) ;
#90583=CARTESIAN_POINT ( 'NONE',  ( 19.03943276465977164, -0.05219959533909143690, 28.74890960531435624 ) ) ;
#90584=CARTESIAN_POINT ( 'NONE',  ( 21.53943276465977519, -0.05219959533907433946, 28.74890960531435624 ) ) ;
#90585=CARTESIAN_POINT ( 'NONE',  ( 18.62759615963255655, 10.81492255796105972, 46.66775706135234714 ) ) ;
#90586=CARTESIAN_POINT ( 'NONE',  ( 5.049401038297881783, 19.05341960407617563, 102.2927570613523045 ) ) ;
#90587=DIRECTION ( 'NONE',  ( 0.000000000000000000, 0.000000000000000000, 1.000000000000000000 ) ) ;
#90588=CARTESIAN_POINT ( 'NONE',  ( -5.049401038298153566, 19.05341960407611168, 65.20724293864765286 ) ) ;
#90590=CARTESIAN_POINT ( 'NONE',  ( 12.14591786802309770, 12.06949235617756955, 79.37390960531436690 ) ) ;
#90591=CARTESIAN_POINT ( 'NONE',  ( -19.05341960407611168, -5.049401038298163336, 66.45724293864769550 ) ) ;
#90592=CARTESIAN_POINT ( 'NONE',  ( -13.97604488694527625, -13.89961937509977652, 71.87390960531433848 ) ) ;
#90593=CARTESIAN_POINT ( 'NONE',  ( 19.05341960407617918, -5.049401038297876454, 81.04275706135231871 ) ) ;
#90594=CARTESIAN_POINT ( 'NONE',  ( -21.55341960407610458, -5.719274019375992779, 61.45724293864770260 ) ) ;
#90595=CARTESIAN_POINT ( 'NONE',  ( 16.52544592524342804, -4.483927247898539470, 108.5405762719810241 ) ) ;
#90596=CARTESIAN_POINT ( 'NONE',  ( -13.89961937509957401, -13.97604488694547875, 44.37609039468566863 ) ) ;
#90597=CARTESIAN_POINT ( 'NONE',  ( 19.03943276465977164, -0.05219959533909143690, 78.74890960531436690 ) ) ;
#90598=CARTESIAN_POINT ( 'NONE',  ( 10.81492255796078972, 18.62759615963270932, 84.58224293864769550 ) ) ;
#90599=CARTESIAN_POINT ( 'NONE',  ( 0.05219959533910956823, 16.53943276465976808, 74.99890960531435269 ) ) ;
#90600=CARTESIAN_POINT ( 'NONE',  ( -13.89961937509957401, -13.97604488694547875, 49.37609039468567573 ) ) ;
#90601=CARTESIAN_POINT ( 'NONE',  ( -21.52544592524343514, 5.823673210054127303, 76.04057627198102409 ) ) ;
#90602=CARTESIAN_POINT ( 'NONE',  ( 18.67979575497178502, 10.72451020669898547, 59.16557627198103120 ) ) ;
#90603=CARTESIAN_POINT ( 'NONE',  ( -18.67979575497178146, -10.72451020669898902, 41.66557627198103120 ) ) ;
#90604=CARTESIAN_POINT ( 'NONE',  ( 21.52544592524334988, 5.823673210054432836, 86.45942372801901854 ) ) ;
#90605=CARTESIAN_POINT ( 'NONE',  ( 13.89961937509977652, -13.97604488694527269, 68.12390960531436690 ) ) ;
#90606=CARTESIAN_POINT ( 'NONE',  ( 16.52544592524342804, -4.483927247898539470, 113.5405762719810383 ) ) ;
#90608=CARTESIAN_POINT ( 'NONE',  ( -21.55341960407619339, 5.719274019375674811, 23.54275706135235424 ) ) ;
#90609=CARTESIAN_POINT ( 'NONE',  ( -5.719274019375665041, -21.55341960407619695, 34.79275706135235424 ) ) ;
#90610=CARTESIAN_POINT ( 'NONE',  ( 0.05219959533909260263, 19.03943276465977164, 34.99890960531435979 ) ) ;
#90611=CARTESIAN_POINT ( 'NONE',  ( 21.52544592524344225, -5.823673210054117533, 108.5405762719810241 ) ) ;
#90612=CARTESIAN_POINT ( 'NONE',  ( 19.05341960407617918, -5.049401038297876454, 61.04275706135232582 ) ) ;
#90613=CARTESIAN_POINT ( 'NONE',  ( -9.564922557960796823, -16.46253265017161027, 37.08224293864768839 ) ) ;
#90614=CARTESIAN_POINT ( 'NONE',  ( -16.55341960407617563, 4.379528057220093196, 33.54275706135234714 ) ) ;
#90615=CARTESIAN_POINT ( 'NONE',  ( 16.20063489777861676, -7.373262058553140541, 22.00000000000000711 ) ) ;
#90616=CARTESIAN_POINT ( 'NONE',  ( 14.29746914071037800, 8.314922557961029526, 56.66775706135235424 ) ) ;
#90617=CARTESIAN_POINT ( 'NONE',  ( 16.51473224551069308, 9.474510206698969483, 39.16557627198103120 ) ) ;
#90619=CARTESIAN_POINT ( 'NONE',  ( -0.05219959533909027116, -19.03943276465977164, 87.49890960531436690 ) ) ;
#90620=CARTESIAN_POINT ( 'NONE',  ( -19.05341960407611168, -5.049401038298163336, 21.45724293864768839 ) ) ;
#90621=CARTESIAN_POINT ( 'NONE',  ( -5.719274019375978568, 21.55341960407610458, 55.20724293864770260 ) ) ;
#90622=CARTESIAN_POINT ( 'NONE',  ( -8.314922557961024197, 14.29746914071037800, 47.91775706135234714 ) ) ;
#90623=CARTESIAN_POINT ( 'NONE',  ( 21.52544592524334988, 5.823673210054432836, 106.4594237280190328 ) ) ;
#90624=CARTESIAN_POINT ( 'NONE',  ( 19.02544592524343514, -5.153800228976328945, 38.54057627198103120 ) ) ;
#90625=CARTESIAN_POINT ( 'NONE',  ( -14.29746914071049879, 8.314922557960819915, 25.83224293864769194 ) ) ;
#90626=CARTESIAN_POINT ( 'NONE',  ( -8.314922557960811034, -14.29746914071050412, 57.08224293864769550 ) ) ;
#90627=CARTESIAN_POINT ( 'NONE',  ( 19.03943276465977164, -0.05219959533909143690, 58.74890960531435979 ) ) ;
#90628=CARTESIAN_POINT ( 'NONE',  ( 5.719274019375673035, 21.55341960407619339, 112.2927570613523471 ) ) ;
#90629=CARTESIAN_POINT ( 'NONE',  ( -21.53943276465977519, 0.05219959533907696930, 116.2489096053143669 ) ) ;
#90630=CARTESIAN_POINT ( 'NONE',  ( 21.52544592524334988, 5.823673210054432836, 81.45942372801900433 ) ) ;
#90631=CARTESIAN_POINT ( 'NONE',  ( 4.379528057220092307, 16.55341960407617563, 52.29275706135236135 ) ) ;
#90632=CARTESIAN_POINT ( 'NONE',  ( -12.14591786802326823, 12.06949235617739902, 28.12609039468568284 ) ) ;
#90633=CARTESIAN_POINT ( 'NONE',  ( 4.379528057220339221, -16.55341960407611168, 87.70724293864769550 ) ) ;
#90634=CARTESIAN_POINT ( 'NONE',  ( -21.55341960407619339, 5.719274019375674811, 103.5427570613523613 ) ) ;
#90635=CARTESIAN_POINT ( 'NONE',  ( 16.53943276465976808, -0.05219959533910856209, 33.74890960531436690 ) ) ;
#90636=CARTESIAN_POINT ( 'NONE',  ( -16.51473224551069308, -9.474510206698971260, 31.66557627198102054 ) ) ;
#90637=CARTESIAN_POINT ( 'NONE',  ( 16.52544592524335698, 4.483927247898782831, 41.45942372801901143 ) ) ;
#90638=CARTESIAN_POINT ( 'NONE',  ( -4.379528057220328563, 16.55341960407611168, 55.20724293864770260 ) ) ;
#90639=CARTESIAN_POINT ( 'NONE',  ( 4.483927247898790824, -16.52544592524335698, 90.20942372801903275 ) ) ;
#90640=CARTESIAN_POINT ( 'NONE',  ( 0.05219959533909260263, 19.03943276465977164, 104.9989096053143669 ) ) ;
#90641=CARTESIAN_POINT ( 'NONE',  ( 16.51473224551069308, 9.474510206698969483, 114.1655762719810241 ) ) ;
#90642=CARTESIAN_POINT ( 'NONE',  ( 5.719274019375673035, 21.55341960407619339, 112.2927570613523471 ) ) ;
#90643=CARTESIAN_POINT ( 'NONE',  ( -4.379528057220328563, 16.55341960407611168, 90.20724293864770971 ) ) ;
#90644=CARTESIAN_POINT ( 'NONE',  ( 13.97604488694527802, 13.89961937509977652, 99.37390960531436690 ) ) ;
#90646=CARTESIAN_POINT ( 'NONE',  ( -14.34966873604972548, 8.224510206698743886, 38.33442372801900433 ) ) ;
#90647=CARTESIAN_POINT ( 'NONE',  ( 13.89961937509977652, -13.97604488694527269, 48.12390960531435979 ) ) ;
#90648=CARTESIAN_POINT ( 'NONE',  ( -9.564922557960796823, -16.46253265017161027, 102.0822429386477097 ) ) ;
#90649=CARTESIAN_POINT ( 'NONE',  ( 14.29746914071037800, 8.314922557961029526, 41.66775706135235424 ) ) ;
#90651=CARTESIAN_POINT ( 'NONE',  ( 5.153800228976615827, -19.02544592524334988, 40.20942372801898301 ) ) ;
#90652=CARTESIAN_POINT ( 'NONE',  ( -13.97604488694527625, -13.89961937509977652, 46.87390960531435979 ) ) ;
#90653=CARTESIAN_POINT ( 'NONE',  ( 4.379528057220092307, 16.55341960407617563, 77.29275706135234714 ) ) ;
#90654=CARTESIAN_POINT ( 'NONE',  ( -13.89961937509957401, -13.97604488694547875, 79.37609039468567573 ) ) ;
#90655=CARTESIAN_POINT ( 'NONE',  ( 16.46253265017146816, 9.564922557961045513, 26.66775706135234003 ) ) ;
#90656=CARTESIAN_POINT ( 'NONE',  ( -16.51473224551069308, -9.474510206698971260, 66.66557627198102409 ) ) ;
#90657=CARTESIAN_POINT ( 'NONE',  ( 8.314922557960818139, 14.29746914071049879, 104.5822429386477097 ) ) ;
#90659=CARTESIAN_POINT ( 'NONE',  ( -19.05341960407617563, 5.049401038297882671, 73.54275706135233293 ) ) ;
#90660=CARTESIAN_POINT ( 'NONE',  ( 15.80617190586746368, 15.72974639402197994, 59.37390960531436690 ) ) ;
#90661=CARTESIAN_POINT ( 'NONE',  ( -19.03943276465977164, -0.05219959533935918106, 23.75109039468566152 ) ) ;
#90662=CARTESIAN_POINT ( 'NONE',  ( -9.564922557960796823, -16.46253265017161027, 102.0822429386477097 ) ) ;
#90663=CARTESIAN_POINT ( 'NONE',  ( 10.81492255796078972, 18.62759615963270932, 74.58224293864768129 ) ) ;
#90665=CARTESIAN_POINT ( 'NONE',  ( -13.89961937509957401, -13.97604488694547875, 104.3760903946856757 ) ) ;
#90666=CARTESIAN_POINT ( 'NONE',  ( -19.53037848336981241, 5.499999999999902300, 59.85532783611444785 ) ) ;
#90667=CARTESIAN_POINT ( 'NONE',  ( 14.34966873604972726, -8.224510206698740333, 25.83442372801901499 ) ) ;
#90668=CARTESIAN_POINT ( 'NONE',  ( 9.474510206698971260, -16.51473224551069308, 32.91557627198102409 ) ) ;
#90669=CARTESIAN_POINT ( 'NONE',  ( -13.89961937509977652, 13.97604488694528158, 100.6239096053143669 ) ) ;
#90670=CARTESIAN_POINT ( 'NONE',  ( -18.62759615963270932, 10.81492255796079327, 95.83224293864770971 ) ) ;
#90671=CARTESIAN_POINT ( 'NONE',  ( -5.719274019375665041, -21.55341960407619695, 64.79275706135234714 ) ) ;
#90672=CARTESIAN_POINT ( 'NONE',  ( -9.474510206698720793, -16.51473224551083518, 104.5844237280190043 ) ) ;
#90673=CARTESIAN_POINT ( 'NONE',  ( -19.02544592524334988, -5.153800228976617603, 18.95942372801899722 ) ) ;
#90674=CARTESIAN_POINT ( 'NONE',  ( -12.14591786802326823, 12.06949235617739902, 103.1260903946856757 ) ) ;
#90675=CARTESIAN_POINT ( 'NONE',  ( 21.53943276465977519, -0.05219959533907433946, 98.74890960531438111 ) ) ;
#90676=CARTESIAN_POINT ( 'NONE',  ( 14.34966873604960469, 8.224510206698951720, 34.16557627198102409 ) ) ;
#90677=CARTESIAN_POINT ( 'NONE',  ( -19.03943276465977164, -0.05219959533935918106, 88.75109039468567573 ) ) ;
#90678=CARTESIAN_POINT ( 'NONE',  ( -19.02544592524334988, -5.153800228976617603, 58.95942372801900433 ) ) ;
#90679=CARTESIAN_POINT ( 'NONE',  ( -21.53943276465977519, -0.05219959533937600094, 63.75109039468568284 ) ) ;
#90680=CARTESIAN_POINT ( 'NONE',  ( -9.564922557961040184, 16.46253265017147172, 42.91775706135234003 ) ) ;
#90681=CARTESIAN_POINT ( 'NONE',  ( -4.483927247898539470, -16.52544592524342804, 107.2905762719810525 ) ) ;
#90682=CARTESIAN_POINT ( 'NONE',  ( -18.67979575497178146, -10.72451020669898902, 36.66557627198103120 ) ) ;
#90683=CARTESIAN_POINT ( 'NONE',  ( 0.05219959533910956823, 16.53943276465976808, 39.99890960531436690 ) ) ;
#90684=CARTESIAN_POINT ( 'NONE',  ( -18.67979575497193778, 10.72451020669871902, 93.33442372801901854 ) ) ;
#90685=CARTESIAN_POINT ( 'NONE',  ( 4.379528057220092307, 16.55341960407617563, 72.29275706135236135 ) ) ;
#90686=CARTESIAN_POINT ( 'NONE',  ( -16.53943276465976808, 0.05219959533911058130, 21.24890960531436690 ) ) ;
#90687=CARTESIAN_POINT ( 'NONE',  ( -5.823673210054431948, 21.52544592524334988, 62.70942372801902565 ) ) ;
#90688=CARTESIAN_POINT ( 'NONE',  ( 18.62759615963255655, 10.81492255796105972, 61.66775706135235424 ) ) ;
#90689=CARTESIAN_POINT ( 'NONE',  ( 21.55341960407610458, 5.719274019375980345, 63.95724293864770260 ) ) ;
#90690=CARTESIAN_POINT ( 'NONE',  ( -19.05341960407611168, -5.049401038298163336, 31.45724293864769550 ) ) ;
#90691=CARTESIAN_POINT ( 'NONE',  ( 21.53943276465977519, 0.05219959533937863772, 41.25109039468568284 ) ) ;
#90692=CARTESIAN_POINT ( 'NONE',  ( -0.05219959533909027116, -19.03943276465977164, 22.49890960531436690 ) ) ;
#90693=CARTESIAN_POINT ( 'NONE',  ( -19.05341960407611168, -5.049401038298163336, 36.45724293864766707 ) ) ;
#90694=CARTESIAN_POINT ( 'NONE',  ( -0.05219959533910754901, -16.53943276465976808, 77.49890960531433848 ) ) ;
#90695=CARTESIAN_POINT ( 'NONE',  ( -13.89961937509977652, 13.97604488694528158, 85.62390960531433848 ) ) ;
#90696=CARTESIAN_POINT ( 'NONE',  ( -16.52544592524342804, 4.483927247898546575, 31.04057627198102409 ) ) ;
#90697=CARTESIAN_POINT ( 'NONE',  ( 10.81492255796078972, 18.62759615963270932, 74.58224293864768129 ) ) ;
#90698=CARTESIAN_POINT ( 'NONE',  ( -21.55341960407610458, -5.719274019375992779, 111.4572429386476813 ) ) ;
#90700=CARTESIAN_POINT ( 'NONE',  ( -16.46253265017160317, 9.564922557960807481, 65.83224293864769550 ) ) ;
#90701=CARTESIAN_POINT ( 'NONE',  ( 13.89961937509957401, 13.97604488694547697, 106.8760903946856757 ) ) ;
#90702=CARTESIAN_POINT ( 'NONE',  ( -18.62759615963270932, 10.81492255796079327, 55.83224293864770260 ) ) ;
#90703=CARTESIAN_POINT ( 'NONE',  ( -15.80617190586768217, 15.72974639402176855, 88.12609039468570415 ) ) ;
#90704=CARTESIAN_POINT ( 'NONE',  ( 13.97604488694527802, 13.89961937509977652, 64.37390960531436690 ) ) ;
#90705=CARTESIAN_POINT ( 'NONE',  ( 9.564922557960805705, 16.46253265017160317, 94.58224293864769550 ) ) ;
#90706=CARTESIAN_POINT ( 'NONE',  ( 16.55341960407618274, -4.379528057220086978, 71.04275706135234714 ) ) ;
#90707=CARTESIAN_POINT ( 'NONE',  ( -21.52544592524334988, -5.823673210054445271, 63.95942372801901854 ) ) ;
#90708=CARTESIAN_POINT ( 'NONE',  ( 18.62759615963255655, 10.81492255796105972, 96.66775706135234714 ) ) ;
#90709=CARTESIAN_POINT ( 'NONE',  ( -18.62759615963270932, 10.81492255796079327, 115.8322429386477097 ) ) ;
#90710=CARTESIAN_POINT ( 'NONE',  ( -0.05219959533907301413, -21.53943276465977519, 72.49890960531435269 ) ) ;
#90711=CARTESIAN_POINT ( 'NONE',  ( 0.05219959533936267826, -19.03943276465977164, 50.00109039468566863 ) ) ;
#90712=CARTESIAN_POINT ( 'NONE',  ( -15.80617190586745835, -15.72974639402198527, 36.87390960531435979 ) ) ;
#90713=CARTESIAN_POINT ( 'NONE',  ( -16.51473224551069308, -9.474510206698971260, 86.66557627198102409 ) ) ;
#90714=CARTESIAN_POINT ( 'NONE',  ( -12.14591786802309592, -12.06949235617757132, 36.87390960531435979 ) ) ;
#90717=CARTESIAN_POINT ( 'NONE',  ( -19.02544592524334988, -5.153800228976617603, 98.95942372801900433 ) ) ;
#90718=CARTESIAN_POINT ( 'NONE',  ( -21.53943276465977519, 0.05219959533907696930, 71.24890960531435269 ) ) ;
#90719=CARTESIAN_POINT ( 'NONE',  ( 12.14591786802309770, 12.06949235617756955, 49.37390960531436690 ) ) ;
#90720=CARTESIAN_POINT ( 'NONE',  ( 4.483927247898790824, -16.52544592524335698, 35.20942372801901854 ) ) ;
#90721=CARTESIAN_POINT ( 'NONE',  ( -5.153800228976328057, -19.02544592524343514, 47.29057627198102409 ) ) ;
#90722=CARTESIAN_POINT ( 'NONE',  ( 10.81492255796078972, 18.62759615963270932, 94.58224293864769550 ) ) ;
#90723=CARTESIAN_POINT ( 'NONE',  ( 9.564922557961047289, -16.46253265017146816, 85.41775706135233293 ) ) ;
#90724=CARTESIAN_POINT ( 'NONE',  ( -5.153800228976328057, -19.02544592524343514, 77.29057627198099567 ) ) ;
#90725=CARTESIAN_POINT ( 'NONE',  ( -12.14591786802309592, -12.06949235617757132, 86.87390960531438111 ) ) ;
#90726=CARTESIAN_POINT ( 'NONE',  ( 19.03943276465977164, -0.05219959533909143690, 63.74890960531435979 ) ) ;
#90727=CARTESIAN_POINT ( 'NONE',  ( -12.14591786802309592, -12.06949235617757132, 66.87390960531436690 ) ) ;
#90728=CARTESIAN_POINT ( 'NONE',  ( 16.46253265017160672, -9.564922557960803928, 38.33224293864768839 ) ) ;
#90730=CARTESIAN_POINT ( 'NONE',  ( -12.06949235617756955, 12.14591786802309770, 35.62390960531437401 ) ) ;
#90731=CARTESIAN_POINT ( 'NONE',  ( 5.049401038298161559, -19.05341960407611168, 87.70724293864769550 ) ) ;
#90733=CARTESIAN_POINT ( 'NONE',  ( 13.97604488694548053, -13.89961937509957401, 55.62609039468566863 ) ) ;
#90734=CARTESIAN_POINT ( 'NONE',  ( -16.53943276465976808, -0.05219959533934237506, 53.75109039468568994 ) ) ;
#90735=CARTESIAN_POINT ( 'NONE',  ( 18.67979575497178502, 10.72451020669898547, 74.16557627198102409 ) ) ;
#90736=CARTESIAN_POINT ( 'NONE',  ( 9.564922557961047289, -16.46253265017146816, 35.41775706135233293 ) ) ;
#90737=CARTESIAN_POINT ( 'NONE',  ( 19.05341960407611168, 5.049401038298154454, 88.95724293864769550 ) ) ;
#90739=CARTESIAN_POINT ( 'NONE',  ( 10.72451020669898902, -18.67979575497178502, 22.91557627198102765 ) ) ;
#90740=CARTESIAN_POINT ( 'NONE',  ( 9.564922557960805705, 16.46253265017160317, 59.58224293864769550 ) ) ;
#90741=CARTESIAN_POINT ( 'NONE',  ( 0.05219959533937995610, -21.53943276465977519, 55.00109039468568284 ) ) ;
#90742=CARTESIAN_POINT ( 'NONE',  ( -9.474510206698964154, 16.51473224551069663, 25.41557627198103120 ) ) ;
#90743=CARTESIAN_POINT ( 'NONE',  ( -18.62759615963255300, -10.81492255796106328, 19.16775706135234714 ) ) ;
#90744=CARTESIAN_POINT ( 'NONE',  ( 5.049401038298161559, -19.05341960407611168, 92.70724293864769550 ) ) ;
#90745=EDGE_LOOP ( 'NONE', ( #187287, #198196, #44550, #40859 ) ) ;
#90746=CARTESIAN_POINT ( 'NONE',  ( 5.719274019375673035, 21.55341960407619339, 37.29275706135235424 ) ) ;
#90748=CARTESIAN_POINT ( 'NONE',  ( 9.564922557960805705, 16.46253265017160317, 99.58224293864770971 ) ) ;
#90751=CARTESIAN_POINT ( 'NONE',  ( -21.55341960407610458, -5.719274019375992779, 111.4572429386476813 ) ) ;
#90752=CARTESIAN_POINT ( 'NONE',  ( 19.05341960407611168, 5.049401038298154454, 48.95724293864768129 ) ) ;
#90753=CARTESIAN_POINT ( 'NONE',  ( 8.314922557961029526, -14.29746914071037800, 30.41775706135234358 ) ) ;
#90755=CARTESIAN_POINT ( 'NONE',  ( -21.52544592524334988, -5.823673210054445271, 98.95942372801903275 ) ) ;
#90756=CARTESIAN_POINT ( 'NONE',  ( 13.89961937509977652, -13.97604488694527269, 28.12390960531435624 ) ) ;
#90757=CARTESIAN_POINT ( 'NONE',  ( 18.62759615963255655, 10.81492255796105972, 96.66775706135234714 ) ) ;
#90758=CARTESIAN_POINT ( 'NONE',  ( -5.153800228976328057, -19.02544592524343514, 87.29057627198103830 ) ) ;
#90759=CARTESIAN_POINT ( 'NONE',  ( 21.52544592524334988, 5.823673210054432836, 56.45942372801902565 ) ) ;
#90761=CARTESIAN_POINT ( 'NONE',  ( -5.049401038298153566, 19.05341960407611168, 95.20724293864770971 ) ) ;
#90762=CARTESIAN_POINT ( 'NONE',  ( -17.50000000000000000, 5.076555817581215102, 28.82048507950227290 ) ) ;
#90763=CARTESIAN_POINT ( 'NONE',  ( 16.52544592524335698, 4.483927247898782831, 56.45942372801902565 ) ) ;
#90764=CARTESIAN_POINT ( 'NONE',  ( 8.314922557961029526, -14.29746914071037800, 65.41775706135234714 ) ) ;
#90765=CARTESIAN_POINT ( 'NONE',  ( -18.62759615963255300, -10.81492255796106328, 59.16775706135234714 ) ) ;
#90766=CARTESIAN_POINT ( 'NONE',  ( -5.719274019375665041, -21.55341960407619695, 89.79275706135236135 ) ) ;
#90768=CARTESIAN_POINT ( 'NONE',  ( -4.379528057220086978, -16.55341960407618274, 29.79275706135234358 ) ) ;
#90769=CARTESIAN_POINT ( 'NONE',  ( -0.05219959533909027116, -19.03943276465977164, 77.49890960531435269 ) ) ;
#90770=CARTESIAN_POINT ( 'NONE',  ( 13.97604488694527802, 13.89961937509977652, 104.3739096053143385 ) ) ;
#90771=CARTESIAN_POINT ( 'NONE',  ( -9.564922557960796823, -16.46253265017161027, 32.08224293864769550 ) ) ;
#90772=CARTESIAN_POINT ( 'NONE',  ( 5.719274019375991003, -21.55341960407610458, 32.70724293864770260 ) ) ;
#90773=CARTESIAN_POINT ( 'NONE',  ( -4.483927247898782831, 16.52544592524335698, 97.70942372801904696 ) ) ;
#90774=CARTESIAN_POINT ( 'NONE',  ( -16.55341960407611168, -4.379528057220339221, 66.45724293864768129 ) ) ;
#90775=CARTESIAN_POINT ( 'NONE',  ( -5.153800228976328057, -19.02544592524343514, 67.29057627198102409 ) ) ;
#90776=CARTESIAN_POINT ( 'NONE',  ( 15.80617190586769283, -15.72974639402175789, 90.62609039468567573 ) ) ;
#90778=CARTESIAN_POINT ( 'NONE',  ( 16.51473224551083163, -9.474510206698727899, 110.8344237280190043 ) ) ;
#90779=CARTESIAN_POINT ( 'NONE',  ( -14.34966873604960291, -8.224510206698953496, 81.66557627198103830 ) ) ;
#90780=CARTESIAN_POINT ( 'NONE',  ( -15.72974639402176322, -15.80617190586768395, 34.37609039468568284 ) ) ;
#90781=CARTESIAN_POINT ( 'NONE',  ( 21.55341960407610458, 5.719274019375980345, 78.95724293864769550 ) ) ;
#90782=CARTESIAN_POINT ( 'NONE',  ( 9.474510206698729675, 16.51473224551082808, 32.08442372801900433 ) ) ;
#90784=CARTESIAN_POINT ( 'NONE',  ( 16.46253265017160672, -9.564922557960803928, 88.33224293864769550 ) ) ;
#90785=CARTESIAN_POINT ( 'NONE',  ( 12.14591786802309770, 12.06949235617756955, 54.37390960531435979 ) ) ;
#90786=CARTESIAN_POINT ( 'NONE',  ( -16.52544592524342804, 4.483927247898546575, 31.04057627198102409 ) ) ;
#90787=CARTESIAN_POINT ( 'NONE',  ( 0.05219959533934541429, -16.53943276465976808, 95.00109039468568994 ) ) ;
#90788=CARTESIAN_POINT ( 'NONE',  ( 19.03943276465977164, 0.05219959533936151252, 56.25109039468566863 ) ) ;
#90789=CARTESIAN_POINT ( 'NONE',  ( 17.50000000000000000, 5.499999999999992895, 46.70309617465829888 ) ) ;
#90790=CARTESIAN_POINT ( 'NONE',  ( 13.97604488694527802, 13.89961937509977652, 104.3739096053143385 ) ) ;
#90791=CARTESIAN_POINT ( 'NONE',  ( 16.55341960407611168, 4.379528057220329451, 78.95724293864769550 ) ) ;
#90792=CARTESIAN_POINT ( 'NONE',  ( 17.50000000000000000, 5.499999999999997335, 120.0000000000000142 ) ) ;
#90793=CARTESIAN_POINT ( 'NONE',  ( -19.05341960407611168, -5.049401038298163336, 36.45724293864766707 ) ) ;
#90794=CARTESIAN_POINT ( 'NONE',  ( 10.81492255796078972, 18.62759615963270932, 29.58224293864769905 ) ) ;
#90795=CARTESIAN_POINT ( 'NONE',  ( -21.52544592524343514, 5.823673210054127303, 66.04057627198103830 ) ) ;
#90796=CARTESIAN_POINT ( 'NONE',  ( 5.049401038298161559, -19.05341960407611168, 22.70724293864769194 ) ) ;
#90797=CARTESIAN_POINT ( 'NONE',  ( -4.379528057220086978, -16.55341960407618274, 69.79275706135234714 ) ) ;
#90798=CARTESIAN_POINT ( 'NONE',  ( -5.049401038298153566, 19.05341960407611168, 45.20724293864769550 ) ) ;
#90799=EDGE_CURVE ( 'NONE', #88111, #10027, #61044, .T. ) ;
#90800=CARTESIAN_POINT ( 'NONE',  ( 15.80617190586769283, -15.72974639402175789, 35.62609039468568994 ) ) ;
#90801=CARTESIAN_POINT ( 'NONE',  ( -4.379528057220328563, 16.55341960407611168, 95.20724293864769550 ) ) ;
#90803=CARTESIAN_POINT ( 'NONE',  ( -16.20579543436674896, 7.371946100355232900, 49.43479165828122035 ) ) ;
#90804=CARTESIAN_POINT ( 'NONE',  ( -21.55341960407610458, -5.719274019375992779, 31.45724293864769550 ) ) ;
#90807=CARTESIAN_POINT ( 'NONE',  ( -14.34966873604972548, 8.224510206698743886, 48.33442372801902565 ) ) ;
#90808=CARTESIAN_POINT ( 'NONE',  ( -8.224510206698948167, 14.34966873604960824, 45.41557627198103830 ) ) ;
#90809=CARTESIAN_POINT ( 'NONE',  ( 15.72974639402199770, -15.80617190586745480, 68.12390960531436690 ) ) ;
#90810=CARTESIAN_POINT ( 'NONE',  ( -15.80617190586745835, -15.72974639402198527, 56.87390960531436690 ) ) ;
#90811=PLANE ( 'NONE',  #182307 ) ;
#90812=CARTESIAN_POINT ( 'NONE',  ( -5.153800228976607833, 19.02544592524334988, 77.70942372801900433 ) ) ;
#90813=CARTESIAN_POINT ( 'NONE',  ( 5.049401038298161559, -19.05341960407611168, 97.70724293864766707 ) ) ;
#90814=CARTESIAN_POINT ( 'NONE',  ( -16.51473224551069308, -9.474510206698971260, 51.66557627198102409 ) ) ;
#90815=CARTESIAN_POINT ( 'NONE',  ( -16.55341960407611168, -4.379528057220339221, 111.4572429386476813 ) ) ;
#90818=CARTESIAN_POINT ( 'NONE',  ( -14.34966873604972548, 8.224510206698743886, 68.33442372801900433 ) ) ;
#90819=CARTESIAN_POINT ( 'NONE',  ( -10.81492255796078084, -18.62759615963271287, 102.0822429386476955 ) ) ;
#90820=CARTESIAN_POINT ( 'NONE',  ( 0.05219959533909260263, 19.03943276465977164, 49.99890960531435979 ) ) ;
#90821=CARTESIAN_POINT ( 'NONE',  ( -0.05219959533937732626, 21.53943276465977519, 47.50109039468568994 ) ) ;
#90822=CARTESIAN_POINT ( 'NONE',  ( -13.97604488694527625, -13.89961937509977652, 76.87390960531433848 ) ) ;
#90825=CARTESIAN_POINT ( 'NONE',  ( -15.80617190586768217, 15.72974639402176855, 28.12609039468568284 ) ) ;
#90826=CARTESIAN_POINT ( 'NONE',  ( 5.049401038298161559, -19.05341960407611168, 107.7072429386476955 ) ) ;
#90827=CARTESIAN_POINT ( 'NONE',  ( -9.474510206698720793, -16.51473224551083518, 94.58442372801900433 ) ) ;
#90828=CARTESIAN_POINT ( 'NONE',  ( 13.89961937509957401, 13.97604488694547697, 46.87609039468565442 ) ) ;
#90829=CARTESIAN_POINT ( 'NONE',  ( 5.823673210054125526, 21.52544592524343514, 99.79057627198103830 ) ) ;
#90830=CARTESIAN_POINT ( 'NONE',  ( 19.02544592524334988, 5.153800228976608722, 31.45942372801900433 ) ) ;
#90831=CARTESIAN_POINT ( 'NONE',  ( -9.474510206698720793, -16.51473224551083518, 34.58442372801899722 ) ) ;
#90832=CARTESIAN_POINT ( 'NONE',  ( -16.55341960407617563, 4.379528057220093196, 98.54275706135234714 ) ) ;
#90833=CARTESIAN_POINT ( 'NONE',  ( 13.89961937509977652, -13.97604488694527269, 113.1239096053143527 ) ) ;
#90834=CARTESIAN_POINT ( 'NONE',  ( -16.46253265017160317, 9.564922557960807481, 55.83224293864769550 ) ) ;
#90835=CARTESIAN_POINT ( 'NONE',  ( -21.55341960407619339, 5.719274019375674811, 68.54275706135234714 ) ) ;
#90836=CARTESIAN_POINT ( 'NONE',  ( -15.80617190586768217, 15.72974639402176855, 78.12609039468570415 ) ) ;
#90837=FACE_OUTER_BOUND ( 'NONE', #112349, .T. ) ;
#90838=CARTESIAN_POINT ( 'NONE',  ( 19.02544592524343514, -5.153800228976328945, 83.54057627198100988 ) ) ;
#90839=CARTESIAN_POINT ( 'NONE',  ( 15.80617190586769283, -15.72974639402175789, 65.62609039468568994 ) ) ;
#90840=CARTESIAN_POINT ( 'NONE',  ( -5.049401038297874678, -19.05341960407617918, 99.79275706135234714 ) ) ;
#90841=CARTESIAN_POINT ( 'NONE',  ( 5.153800228976335163, 19.02544592524342804, 69.79057627198103830 ) ) ;
#90842=CARTESIAN_POINT ( 'NONE',  ( 13.89961937509977652, -13.97604488694527269, 98.12390960531433848 ) ) ;
#90843=CARTESIAN_POINT ( 'NONE',  ( 16.51473224551069308, 9.474510206698969483, 74.16557627198103830 ) ) ;
#90844=CARTESIAN_POINT ( 'NONE',  ( 5.049401038298163336, -19.05341960407611168, 77.70724293864768129 ) ) ;
#90845=CARTESIAN_POINT ( 'NONE',  ( -19.02544592524342804, 5.153800228976336051, 61.04057627198103120 ) ) ;
#90846=CARTESIAN_POINT ( 'NONE',  ( -21.53943276465977519, 0.05219959533907696930, 96.24890960531435269 ) ) ;
#90847=CARTESIAN_POINT ( 'NONE',  ( 16.53943276465976808, 0.05219959533934440121, 86.25109039468568994 ) ) ;
#90849=CARTESIAN_POINT ( 'NONE',  ( 19.03943276465977164, 0.05219959533936151252, 41.25109039468566152 ) ) ;
#90850=CARTESIAN_POINT ( 'NONE',  ( 19.03943276465977164, -0.05219959533909143690, 83.74890960531436690 ) ) ;
#90851=CARTESIAN_POINT ( 'NONE',  ( 0.05219959533910956823, 16.53943276465976808, 69.99890960531435269 ) ) ;
#90852=CARTESIAN_POINT ( 'NONE',  ( 16.53943276465976808, -0.05219959533910856209, 113.7489096053143527 ) ) ;
#90853=CARTESIAN_POINT ( 'NONE',  ( 16.46253265017160672, -9.564922557960803928, 108.3322429386476955 ) ) ;
#90854=CARTESIAN_POINT ( 'NONE',  ( 13.97604488694527802, 13.89961937509977652, 109.3739096053143669 ) ) ;
#90855=CARTESIAN_POINT ( 'NONE',  ( -5.153800228976328057, -19.02544592524343514, 82.29057627198102409 ) ) ;
#90856=CARTESIAN_POINT ( 'NONE',  ( 5.049401038297881783, 19.05341960407617563, 37.29275706135232582 ) ) ;
#90857=CARTESIAN_POINT ( 'NONE',  ( -4.379528057220086978, -16.55341960407618274, 89.79275706135236135 ) ) ;
#90858=CARTESIAN_POINT ( 'NONE',  ( -16.51473224551069308, -9.474510206698971260, 71.66557627198102409 ) ) ;
#90859=CARTESIAN_POINT ( 'NONE',  ( 18.67979575497194134, -10.72451020669871369, 55.83442372801901854 ) ) ;
#90860=CARTESIAN_POINT ( 'NONE',  ( 21.52544592524344225, -5.823673210054117533, 28.54057627198103120 ) ) ;
#90861=CARTESIAN_POINT ( 'NONE',  ( 0.05219959533907565091, 21.53943276465977519, 114.9989096053143669 ) ) ;
#90862=CARTESIAN_POINT ( 'NONE',  ( -18.67979575497178146, -10.72451020669898902, 76.66557627198103830 ) ) ;
#90863=CARTESIAN_POINT ( 'NONE',  ( -8.224510206698948167, 14.34966873604960824, 90.41557627198103830 ) ) ;
#90864=CARTESIAN_POINT ( 'NONE',  ( 9.564922557961047289, -16.46253265017146816, 55.41775706135234003 ) ) ;
#90865=CARTESIAN_POINT ( 'NONE',  ( 16.46253265017160672, -9.564922557960803928, 33.33224293864770260 ) ) ;
#90866=CARTESIAN_POINT ( 'NONE',  ( 16.51473224551069308, 9.474510206698969483, 89.16557627198103830 ) ) ;
#90867=CARTESIAN_POINT ( 'NONE',  ( 13.97604488694527802, 13.89961937509977652, 84.37390960531433848 ) ) ;
#90869=CARTESIAN_POINT ( 'NONE',  ( -12.06949235617756955, 12.14591786802309770, 105.6239096053143669 ) ) ;
#90870=VERTEX_POINT ( 'NONE', #74259 ) ;
#90871=CARTESIAN_POINT ( 'NONE',  ( 12.14591786802309770, 12.06949235617756955, 29.37390960531435269 ) ) ;
#90872=CARTESIAN_POINT ( 'NONE',  ( 0.05219959533934541429, -16.53943276465976808, 25.00109039468567218 ) ) ;
#90873=CARTESIAN_POINT ( 'NONE',  ( 21.52544592524334988, 5.823673210054432836, 91.45942372801901854 ) ) ;
#90874=CARTESIAN_POINT ( 'NONE',  ( -13.89961937509977652, 13.97604488694528158, 105.6239096053143527 ) ) ;
#90875=CARTESIAN_POINT ( 'NONE',  ( -0.05219959533937732626, 21.53943276465977519, 22.50109039468567573 ) ) ;
#90876=CARTESIAN_POINT ( 'NONE',  ( -5.153800228976328057, -19.02544592524343514, 42.29057627198101699 ) ) ;
#90877=CARTESIAN_POINT ( 'NONE',  ( 16.55341960407618274, -4.379528057220086978, 41.04275706135236135 ) ) ;
#90879=CARTESIAN_POINT ( 'NONE',  ( -19.03943276465977164, -0.05219959533935918106, 113.7510903946856757 ) ) ;
#90880=CARTESIAN_POINT ( 'NONE',  ( 5.153800228976335163, 19.02544592524342804, 39.79057627198100988 ) ) ;
#90881=CARTESIAN_POINT ( 'NONE',  ( -12.14591786802309592, -12.06949235617757132, 91.87390960531436690 ) ) ;
#90882=CARTESIAN_POINT ( 'NONE',  ( -0.05219959533907301413, -21.53943276465977519, 102.4989096053143811 ) ) ;
#90883=CARTESIAN_POINT ( 'NONE',  ( -13.89961937509957401, -13.97604488694547875, 74.37609039468566152 ) ) ;
#90884=CARTESIAN_POINT ( 'NONE',  ( 0.05219959533937995610, -21.53943276465977519, 25.00109039468567218 ) ) ;
#90885=CARTESIAN_POINT ( 'NONE',  ( 5.153800228976335163, 19.02544592524342804, 94.79057627198103830 ) ) ;
#90887=CARTESIAN_POINT ( 'NONE',  ( 5.049401038298161559, -19.05341960407611168, 82.70724293864770971 ) ) ;
#90888=CARTESIAN_POINT ( 'NONE',  ( -10.72451020669870658, -18.67979575497194134, 34.58442372801900433 ) ) ;
#90889=CARTESIAN_POINT ( 'NONE',  ( -8.224510206698948167, 14.34966873604960824, 80.41557627198103830 ) ) ;
#90890=CARTESIAN_POINT ( 'NONE',  ( -9.564922557960796823, -16.46253265017161027, 77.08224293864769550 ) ) ;
#90891=CARTESIAN_POINT ( 'NONE',  ( -16.55341960407617563, 4.379528057220093196, 48.54275706135234714 ) ) ;
#90892=CARTESIAN_POINT ( 'NONE',  ( 19.02544592524334988, 5.153800228976608722, 51.45942372801900433 ) ) ;
#90893=CARTESIAN_POINT ( 'NONE',  ( -5.823673210054431948, 21.52544592524334988, 67.70942372801901854 ) ) ;
#90894=CARTESIAN_POINT ( 'NONE',  ( -14.29746914071037622, -8.314922557961029526, 29.16775706135234003 ) ) ;
#90895=CARTESIAN_POINT ( 'NONE',  ( -13.97604488694527625, -13.89961937509977652, 66.87390960531436690 ) ) ;
#90896=CARTESIAN_POINT ( 'NONE',  ( -0.05219959533936034679, 19.03943276465977164, 97.50109039468567573 ) ) ;
#90897=CARTESIAN_POINT ( 'NONE',  ( 8.314922557961029526, -14.29746914071037800, 50.41775706135235424 ) ) ;
#90898=CARTESIAN_POINT ( 'NONE',  ( 18.62759615963255655, 10.81492255796105972, 101.6677570613523613 ) ) ;
#90899=CARTESIAN_POINT ( 'NONE',  ( -16.51473224551082808, 9.474510206698731452, 78.33442372801900433 ) ) ;
#90900=CARTESIAN_POINT ( 'NONE',  ( -19.03943276465977164, 0.05219959533909376836, 56.24890960531435979 ) ) ;
#90901=CARTESIAN_POINT ( 'NONE',  ( 5.823673210054125526, 21.52544592524343514, 64.79057627198103830 ) ) ;
#90902=CARTESIAN_POINT ( 'NONE',  ( 14.29746914071049879, -8.314922557960816363, 78.33224293864770971 ) ) ;
#90903=CARTESIAN_POINT ( 'NONE',  ( 16.46253265017146816, 9.564922557961045513, 71.66775706135233293 ) ) ;
#90904=CARTESIAN_POINT ( 'NONE',  ( 16.79531203550644136, -7.028104445595666050, 61.24755011779559055 ) ) ;
#90905=CARTESIAN_POINT ( 'NONE',  ( -0.05219959533936034679, 19.03943276465977164, 47.50109039468566863 ) ) ;
#90907=CARTESIAN_POINT ( 'NONE',  ( 4.483927247898790824, -16.52544592524335698, 105.2094237280190328 ) ) ;
#90908=CARTESIAN_POINT ( 'NONE',  ( -14.29746914071049879, 8.314922557960819915, 65.83224293864769550 ) ) ;
#90909=CARTESIAN_POINT ( 'NONE',  ( 10.72451020669871369, 18.67979575497193778, 97.08442372801904696 ) ) ;
#90911=CARTESIAN_POINT ( 'NONE',  ( -21.52544592524343514, 5.823673210054127303, 111.0405762719810525 ) ) ;
#90912=CARTESIAN_POINT ( 'NONE',  ( -9.474510206698964154, 16.51473224551069663, 65.41557627198102409 ) ) ;
#90913=CARTESIAN_POINT ( 'NONE',  ( -5.823673210054431948, 21.52544592524334988, 77.70942372801900433 ) ) ;
#90914=CARTESIAN_POINT ( 'NONE',  ( -9.564922557960796823, -16.46253265017161027, 62.08224293864769550 ) ) ;
#90915=CARTESIAN_POINT ( 'NONE',  ( 16.52544592524342804, -4.483927247898539470, 113.5405762719810383 ) ) ;
#90916=CARTESIAN_POINT ( 'NONE',  ( 21.52544592524344225, -5.823673210054117533, 33.54057627198102409 ) ) ;
#90917=CARTESIAN_POINT ( 'NONE',  ( -14.34966873604960291, -8.224510206698953496, 61.66557627198103120 ) ) ;
#90918=CARTESIAN_POINT ( 'NONE',  ( 19.05341960407611168, 5.049401038298154454, 48.95724293864768129 ) ) ;
#90919=CARTESIAN_POINT ( 'NONE',  ( 14.29746914071049879, -8.314922557960816363, 98.33224293864769550 ) ) ;
#90920=CARTESIAN_POINT ( 'NONE',  ( -18.67979575497178146, -10.72451020669898902, 106.6655762719810383 ) ) ;
#90921=CARTESIAN_POINT ( 'NONE',  ( -15.80617190586768217, 15.72974639402176855, 48.12609039468568284 ) ) ;
#90922=CARTESIAN_POINT ( 'NONE',  ( -16.46253265017160317, 9.564922557960807481, 30.83224293864769550 ) ) ;
#90923=CARTESIAN_POINT ( 'NONE',  ( 16.53943276465976808, 0.05219959533934440121, 56.25109039468568284 ) ) ;
#90924=CARTESIAN_POINT ( 'NONE',  ( -21.55341960407610458, -5.719274019375992779, 106.4572429386477097 ) ) ;
#90925=CARTESIAN_POINT ( 'NONE',  ( -21.52544592524343514, 5.823673210054127303, 91.04057627198103830 ) ) ;
#90926=CARTESIAN_POINT ( 'NONE',  ( -19.02544592524334988, -5.153800228976617603, 28.95942372801900433 ) ) ;
#90927=CARTESIAN_POINT ( 'NONE',  ( -19.05341960407611168, -5.049401038298163336, 51.45724293864770260 ) ) ;
#90928=CARTESIAN_POINT ( 'NONE',  ( 19.02544592524343514, -5.153800228976328945, 103.5405762719809957 ) ) ;
#90929=CARTESIAN_POINT ( 'NONE',  ( 10.72451020669871369, 18.67979575497193778, 52.08442372801901854 ) ) ;
#90930=CARTESIAN_POINT ( 'NONE',  ( -18.62759615963270932, 10.81492255796079327, 45.83224293864769550 ) ) ;
#90931=CARTESIAN_POINT ( 'NONE',  ( 16.53943276465976808, -0.05219959533910856209, 28.74890960531435624 ) ) ;
#90932=CARTESIAN_POINT ( 'NONE',  ( -21.53943276465977519, -0.05219959533937600094, 68.75109039468568994 ) ) ;
#90933=CARTESIAN_POINT ( 'NONE',  ( -5.719274019375665041, -21.55341960407619695, 94.79275706135234714 ) ) ;
#90934=CARTESIAN_POINT ( 'NONE',  ( 5.153800228976615827, -19.02544592524334988, 45.20942372801901143 ) ) ;
#90935=CARTESIAN_POINT ( 'NONE',  ( 12.14591786802327356, -12.06949235617739191, 105.6260903946856899 ) ) ;
#90936=CARTESIAN_POINT ( 'NONE',  ( -5.719274019375665041, -21.55341960407619695, 49.79275706135234714 ) ) ;
#90937=CARTESIAN_POINT ( 'NONE',  ( -9.474510206698964154, 16.51473224551069663, 65.41557627198102409 ) ) ;
#90938=CARTESIAN_POINT ( 'NONE',  ( -13.97604488694547697, 13.89961937509957934, 23.12609039468565442 ) ) ;
#90939=CARTESIAN_POINT ( 'NONE',  ( -18.67979575497178146, -10.72451020669898902, 21.66557627198102409 ) ) ;
#90940=CARTESIAN_POINT ( 'NONE',  ( 18.67979575497178502, 10.72451020669898547, 114.1655762719810383 ) ) ;
#90941=CARTESIAN_POINT ( 'NONE',  ( -18.67979575497178146, -10.72451020669898902, 91.66557627198103830 ) ) ;
#90942=CARTESIAN_POINT ( 'NONE',  ( 16.53943276465976808, 0.05219959533934440121, 36.25109039468567573 ) ) ;
#90944=CARTESIAN_POINT ( 'NONE',  ( -18.62759615963270932, 10.81492255796079327, 75.83224293864769550 ) ) ;
#90945=CARTESIAN_POINT ( 'NONE',  ( -16.53943276465976808, -0.05219959533934237506, 58.75109039468568994 ) ) ;
#90946=CARTESIAN_POINT ( 'NONE',  ( 4.483927247898545687, 16.52544592524342804, 79.79057627198102409 ) ) ;
#90948=CARTESIAN_POINT ( 'NONE',  ( -19.03943276465977164, -0.05219959533935918106, 108.7510903946856615 ) ) ;
#90949=CARTESIAN_POINT ( 'NONE',  ( -5.823673210054116645, -21.52544592524344225, 32.29057627198102409 ) ) ;
#90951=CARTESIAN_POINT ( 'NONE',  ( -8.314922557961024197, 14.29746914071037800, 37.91775706135235424 ) ) ;
#90952=CARTESIAN_POINT ( 'NONE',  ( -10.72451020669870658, -18.67979575497194134, 19.58442372801901143 ) ) ;
#90953=CARTESIAN_POINT ( 'NONE',  ( -15.72974639402197994, 15.80617190586746368, 35.62390960531437401 ) ) ;
#90954=CARTESIAN_POINT ( 'NONE',  ( -4.379528057220086978, -16.55341960407618274, 74.79275706135234714 ) ) ;
#90955=CARTESIAN_POINT ( 'NONE',  ( -16.46253265017160317, 9.564922557960807481, 80.83224293864769550 ) ) ;
#90956=CARTESIAN_POINT ( 'NONE',  ( 5.823673210054444382, -21.52544592524334988, 60.20942372801902565 ) ) ;
#90957=CARTESIAN_POINT ( 'NONE',  ( 16.51473224551069308, 9.474510206698969483, 24.16557627198102765 ) ) ;
#90958=CARTESIAN_POINT ( 'NONE',  ( -21.55341960407610458, -5.719274019375992779, 26.45724293864768839 ) ) ;
#90960=CARTESIAN_POINT ( 'NONE',  ( -13.89961937509957401, -13.97604488694547875, 39.37609039468566152 ) ) ;
#90961=CARTESIAN_POINT ( 'NONE',  ( -12.14591786802326823, 12.06949235617739902, 58.12609039468568994 ) ) ;
#90962=CARTESIAN_POINT ( 'NONE',  ( 21.53943276465977519, -0.05219959533907433946, 23.74890960531435269 ) ) ;
#90963=CARTESIAN_POINT ( 'NONE',  ( 15.80617190586746368, 15.72974639402197994, 104.3739096053143669 ) ) ;
#90964=CARTESIAN_POINT ( 'NONE',  ( 13.97604488694527802, 13.89961937509977652, 79.37390960531435269 ) ) ;
#90965=CARTESIAN_POINT ( 'NONE',  ( -15.49999999999999822, -5.500000000000000888, 118.0000000000000142 ) ) ;
#90967=CARTESIAN_POINT ( 'NONE',  ( -12.14591786802309592, -12.06949235617757132, 101.8739096053143811 ) ) ;
#90968=CARTESIAN_POINT ( 'NONE',  ( -5.719274019375978568, 21.55341960407610458, 30.20724293864769550 ) ) ;
#90969=CARTESIAN_POINT ( 'NONE',  ( -16.29526858892872454, 7.335722546920266041, 34.20329402199793378 ) ) ;
#90970=CARTESIAN_POINT ( 'NONE',  ( 16.53943276465976808, 0.05219959533934440121, 66.25109039468567573 ) ) ;
#90971=CARTESIAN_POINT ( 'NONE',  ( 5.719274019375673035, 21.55341960407619339, 22.29275706135235069 ) ) ;
#90972=CARTESIAN_POINT ( 'NONE',  ( 0.05219959533936267826, -19.03943276465977164, 80.00109039468567573 ) ) ;
#90973=CARTESIAN_POINT ( 'NONE',  ( -0.05219959533909027116, -19.03943276465977164, 37.49890960531436690 ) ) ;
#90974=CARTESIAN_POINT ( 'NONE',  ( 10.81492255796078972, 18.62759615963270932, 64.58224293864769550 ) ) ;
#90975=CARTESIAN_POINT ( 'NONE',  ( 9.564922557960805705, 16.46253265017160317, 109.5822429386476955 ) ) ;
#90976=CARTESIAN_POINT ( 'NONE',  ( 21.55341960407619695, -5.719274019375665929, 86.04275706135236135 ) ) ;
#90977=CARTESIAN_POINT ( 'NONE',  ( -19.05341960407611168, -5.049401038298163336, 61.45724293864769550 ) ) ;
#90978=CARTESIAN_POINT ( 'NONE',  ( -8.224510206698735004, -14.34966873604973081, 44.58442372801901854 ) ) ;
#90979=CARTESIAN_POINT ( 'NONE',  ( 5.153800228976335163, 19.02544592524342804, 59.79057627198100988 ) ) ;
#90980=CARTESIAN_POINT ( 'NONE',  ( -21.55341960407619339, 5.719274019375674811, 78.54275706135236135 ) ) ;
#90981=CARTESIAN_POINT ( 'NONE',  ( 9.564922557961047289, -16.46253265017146816, 45.41775706135232582 ) ) ;
#90982=CARTESIAN_POINT ( 'NONE',  ( -19.02544592524334988, -5.153800228976617603, 58.95942372801900433 ) ) ;
#90983=CARTESIAN_POINT ( 'NONE',  ( 18.67979575497194134, -10.72451020669871369, 50.83442372801901143 ) ) ;
#90986=CARTESIAN_POINT ( 'NONE',  ( -16.51473224551082808, 9.474510206698731452, 48.33442372801900433 ) ) ;
#90987=CARTESIAN_POINT ( 'NONE',  ( 13.97604488694527802, 13.89961937509977652, 99.37390960531436690 ) ) ;
#90988=CARTESIAN_POINT ( 'NONE',  ( 16.46253265017160672, -9.564922557960803928, 73.33224293864769550 ) ) ;
#90989=CARTESIAN_POINT ( 'NONE',  ( -4.483927247898782831, 16.52544592524335698, 112.7094237280190328 ) ) ;
#90990=CARTESIAN_POINT ( 'NONE',  ( 21.52544592524344225, -5.823673210054117533, 38.54057627198103120 ) ) ;
#90991=CARTESIAN_POINT ( 'NONE',  ( -21.53943276465977519, -0.05219959533937600094, 103.7510903946857042 ) ) ;
#90995=CARTESIAN_POINT ( 'NONE',  ( 18.62759615963255655, 10.81492255796105972, 91.66775706135234714 ) ) ;
#90997=CARTESIAN_POINT ( 'NONE',  ( 0.05219959533910956823, 16.53943276465976808, 114.9989096053143669 ) ) ;
#90998=CARTESIAN_POINT ( 'NONE',  ( -16.46253265017160317, 9.564922557960807481, 115.8322429386477097 ) ) ;
#91000=CARTESIAN_POINT ( 'NONE',  ( -4.483927247898782831, 16.52544592524335698, 52.70942372801902565 ) ) ;
#91001=CARTESIAN_POINT ( 'NONE',  ( -18.67979575497178146, -10.72451020669898902, 71.66557627198100988 ) ) ;
#91002=CARTESIAN_POINT ( 'NONE',  ( -4.483927247898539470, -16.52544592524342804, 42.29057627198103120 ) ) ;
#91003=CARTESIAN_POINT ( 'NONE',  ( -8.314922557960811034, -14.29746914071050412, 107.0822429386476955 ) ) ;
#91004=CARTESIAN_POINT ( 'NONE',  ( -19.03943276465977164, 0.05219959533909376836, 106.2489096053143669 ) ) ;
#91005=CARTESIAN_POINT ( 'NONE',  ( -0.05219959533937732626, 21.53943276465977519, 27.50109039468567929 ) ) ;
#91006=CARTESIAN_POINT ( 'NONE',  ( -19.03943276465977164, -0.05219959533935918106, 38.75109039468566152 ) ) ;
#91007=CARTESIAN_POINT ( 'NONE',  ( -0.05219959533910754901, -16.53943276465976808, 112.4989096053143669 ) ) ;
#91008=CARTESIAN_POINT ( 'NONE',  ( 5.719274019375673035, 21.55341960407619339, 72.29275706135236135 ) ) ;
#91009=CARTESIAN_POINT ( 'NONE',  ( 16.20579543436675252, -7.371946100355225795, 31.93479165828123811 ) ) ;
#91010=CARTESIAN_POINT ( 'NONE',  ( 4.483927247898545687, 16.52544592524342804, 29.79057627198102409 ) ) ;
#91012=CARTESIAN_POINT ( 'NONE',  ( 5.719274019375991003, -21.55341960407610458, 32.70724293864770260 ) ) ;
#91013=CARTESIAN_POINT ( 'NONE',  ( 16.52544592524342804, -4.483927247898539470, 93.54057627198103830 ) ) ;
#91015=CARTESIAN_POINT ( 'NONE',  ( -19.03943276465977164, 0.05219959533909376836, 76.24890960531435269 ) ) ;
#91016=CARTESIAN_POINT ( 'NONE',  ( -8.314922557960811034, -14.29746914071050412, 72.08224293864769550 ) ) ;
#91017=CARTESIAN_POINT ( 'NONE',  ( -13.89961937509957401, -13.97604488694547875, 109.3760903946856331 ) ) ;
#91018=CARTESIAN_POINT ( 'NONE',  ( 0.05219959533907565091, 21.53943276465977519, 44.99890960531435979 ) ) ;
#91020=CARTESIAN_POINT ( 'NONE',  ( 8.314922557960818139, 14.29746914071049879, 114.5822429386477097 ) ) ;
#91021=CARTESIAN_POINT ( 'NONE',  ( 19.02544592524343514, -5.153800228976328945, 68.54057627198103830 ) ) ;
#91022=CARTESIAN_POINT ( 'NONE',  ( 5.719274019375991003, -21.55341960407610458, 72.70724293864769550 ) ) ;
#91023=CARTESIAN_POINT ( 'NONE',  ( -14.29746914071037622, -8.314922557961029526, 109.1677570613523613 ) ) ;
#91024=CARTESIAN_POINT ( 'NONE',  ( 5.153800228976335163, 19.02544592524342804, 84.79057627198099567 ) ) ;
#91025=CARTESIAN_POINT ( 'NONE',  ( 19.05341960407617918, -5.049401038297876454, 71.04275706135234714 ) ) ;
#91026=CARTESIAN_POINT ( 'NONE',  ( 5.719274019375673035, 21.55341960407619339, 92.29275706135236135 ) ) ;
#91027=CARTESIAN_POINT ( 'NONE',  ( 21.52544592524344225, -5.823673210054117533, 63.54057627198103830 ) ) ;
#91028=CARTESIAN_POINT ( 'NONE',  ( 10.72451020669898902, -18.67979575497178502, 27.91557627198103830 ) ) ;
#91029=CARTESIAN_POINT ( 'NONE',  ( -13.97604488694527625, -13.89961937509977652, 31.87390960531435979 ) ) ;
#91030=CARTESIAN_POINT ( 'NONE',  ( 12.14591786802327356, -12.06949235617739191, 105.6260903946856899 ) ) ;
#91031=CARTESIAN_POINT ( 'NONE',  ( 19.05341960407611168, 5.049401038298154454, 68.95724293864769550 ) ) ;
#91032=CARTESIAN_POINT ( 'NONE',  ( -0.05219959533934338120, 16.53943276465976808, 27.50109039468567929 ) ) ;
#91033=CARTESIAN_POINT ( 'NONE',  ( 16.20579543436681647, 7.371946100354975329, 53.06520834171878676 ) ) ;
#91034=CARTESIAN_POINT ( 'NONE',  ( 21.53943276465977519, 0.05219959533937863772, 111.2510903946856899 ) ) ;
#91035=CARTESIAN_POINT ( 'NONE',  ( 16.53943276465976808, -0.05219959533910856209, 73.74890960531433848 ) ) ;
#91036=CARTESIAN_POINT ( 'NONE',  ( 18.67979575497178502, 10.72451020669898547, 104.1655762719810241 ) ) ;
#91037=CARTESIAN_POINT ( 'NONE',  ( -15.80617190586745835, -15.72974639402198527, 96.87390960531436690 ) ) ;
#91039=CARTESIAN_POINT ( 'NONE',  ( -21.52544592524343514, 5.823673210054127303, 41.04057627198103120 ) ) ;
#91040=CARTESIAN_POINT ( 'NONE',  ( -8.224510206698735004, -14.34966873604973081, 84.58442372801903275 ) ) ;
#91041=CARTESIAN_POINT ( 'NONE',  ( 0.05219959533910956823, 16.53943276465976808, 109.9989096053143527 ) ) ;
#91042=CARTESIAN_POINT ( 'NONE',  ( -19.02544592524342804, 5.153800228976336051, 61.04057627198103120 ) ) ;
#91044=CARTESIAN_POINT ( 'NONE',  ( 14.29746914071037800, 8.314922557961029526, 106.6677570613523756 ) ) ;
#91045=CARTESIAN_POINT ( 'NONE',  ( 15.80617190586769283, -15.72974639402175789, 45.62609039468567573 ) ) ;
#91046=CARTESIAN_POINT ( 'NONE',  ( -13.89961937509977652, 13.97604488694528158, 95.62390960531436690 ) ) ;
#91047=CARTESIAN_POINT ( 'NONE',  ( -18.67979575497193778, 10.72451020669871902, 78.33442372801901854 ) ) ;
#91048=CARTESIAN_POINT ( 'NONE',  ( 5.153800228976335163, 19.02544592524342804, 29.79057627198102409 ) ) ;
#91049=CARTESIAN_POINT ( 'NONE',  ( -19.02544592524342804, 5.153800228976336051, 36.04057627198100988 ) ) ;
#91051=CARTESIAN_POINT ( 'NONE',  ( -5.823673210054431948, 21.52544592524334988, 72.70942372801901854 ) ) ;
#91052=CARTESIAN_POINT ( 'NONE',  ( -13.97604488694527625, -13.89961937509977652, 101.8739096053143811 ) ) ;
#91053=CARTESIAN_POINT ( 'NONE',  ( -13.97604488694547697, 13.89961937509957934, 83.12609039468564731 ) ) ;
#91054=CARTESIAN_POINT ( 'NONE',  ( -0.05219959533937732626, 21.53943276465977519, 37.50109039468568284 ) ) ;
#91055=CARTESIAN_POINT ( 'NONE',  ( -4.483927247898782831, 16.52544592524335698, 22.70942372801901499 ) ) ;
#91056=CARTESIAN_POINT ( 'NONE',  ( 13.89961937509957401, 13.97604488694547697, 66.87609039468567573 ) ) ;
#91057=CARTESIAN_POINT ( 'NONE',  ( 16.46253265017160672, -9.564922557960803928, 58.33224293864769550 ) ) ;
#91058=CARTESIAN_POINT ( 'NONE',  ( -16.46253265017146816, -9.564922557961047289, 79.16775706135234714 ) ) ;
#91059=CARTESIAN_POINT ( 'NONE',  ( 8.224510206698953496, -14.34966873604960469, 27.91557627198103830 ) ) ;
#91060=CARTESIAN_POINT ( 'NONE',  ( -19.03943276465977164, -0.05219959533935918106, 78.75109039468567573 ) ) ;
#91061=CARTESIAN_POINT ( 'NONE',  ( 16.52544592524342804, -4.483927247898539470, 38.54057627198103120 ) ) ;
#91062=CARTESIAN_POINT ( 'NONE',  ( 9.474510206698729675, 16.51473224551082808, 62.08442372801899722 ) ) ;
#91063=CARTESIAN_POINT ( 'NONE',  ( 16.53943276465976808, 0.05219959533934440121, 46.25109039468567573 ) ) ;
#91064=CARTESIAN_POINT ( 'NONE',  ( 10.72451020669871369, 18.67979575497193778, 112.0844237280190185 ) ) ;
#91065=CARTESIAN_POINT ( 'NONE',  ( 5.049401038298161559, -19.05341960407611168, 32.70724293864768129 ) ) ;
#91066=CARTESIAN_POINT ( 'NONE',  ( -17.40805194822029378, -6.112264579159361055, 64.16628727489388950 ) ) ;
#91067=B_SPLINE_CURVE_WITH_KNOTS ( 'NONE', 3,
 ( #177454, #130919, #133937, #38924, #85412, #118774, #180462, #24774, #193615, #103600, #166273, #27771, #55087, #163272, #86421, #40925, #94360, #135929, #43911, #44901, #137894, #108544, #138880, #29731, #105573, #171219, #168235, #122716, #30725, #92372, #106558, #156039 ),
 .UNSPECIFIED., .F., .F.,
 ( 4, 2, 2, 2, 2, 2, 2, 2, 2, 2, 2, 2, 2, 2, 2, 4 ),
 ( 2.711112516444420852E-17, 0.0003712461730036987042, 0.0007424923460073703033, 0.001113738519011041794, 0.001484984692014713501, 0.002227477038022075348, 0.002598723211025741851, 0.002969969384029408355, 0.003341215557033074424, 0.003712461730036740928, 0.004083707903040406997, 0.004454954076044073501, 0.004826200249047739137, 0.005197446422051405640, 0.005568692595055072143, 0.005939938768058737779 ),
 .UNSPECIFIED. ) ;
#91068=CARTESIAN_POINT ( 'NONE',  ( 14.34966873604972726, -8.224510206698740333, 50.83442372801901143 ) ) ;
#91071=CARTESIAN_POINT ( 'NONE',  ( 19.03943276465977164, -0.05219959533909143690, 88.74890960531436690 ) ) ;
#91074=CARTESIAN_POINT ( 'NONE',  ( 19.03943276465977164, 0.05219959533936151252, 81.25109039468567573 ) ) ;
#91075=CARTESIAN_POINT ( 'NONE',  ( -18.62759615963270932, 10.81492255796079327, 30.83224293864770260 ) ) ;
#91076=CARTESIAN_POINT ( 'NONE',  ( -10.81492255796105439, 18.62759615963255655, 112.9177570613523329 ) ) ;
#91077=CARTESIAN_POINT ( 'NONE',  ( -9.564922557961040184, 16.46253265017147172, 97.91775706135233293 ) ) ;
#91078=CARTESIAN_POINT ( 'NONE',  ( -0.05219959533910754901, -16.53943276465976808, 107.4989096053143669 ) ) ;
#91079=CARTESIAN_POINT ( 'NONE',  ( -13.97604488694527625, -13.89961937509977652, 31.87390960531435979 ) ) ;
#91080=CARTESIAN_POINT ( 'NONE',  ( 21.52544592524344225, -5.823673210054117533, 63.54057627198103830 ) ) ;
#91081=CARTESIAN_POINT ( 'NONE',  ( 15.72974639402199770, -15.80617190586745480, 53.12390960531436690 ) ) ;
#91082=CARTESIAN_POINT ( 'NONE',  ( -13.97604488694527625, -13.89961937509977652, 21.87390960531435979 ) ) ;
#91084=CARTESIAN_POINT ( 'NONE',  ( 16.51473224551083163, -9.474510206698727899, 65.83442372801900433 ) ) ;
#91085=CARTESIAN_POINT ( 'NONE',  ( 4.379528057220339221, -16.55341960407611168, 42.70724293864770260 ) ) ;
#91086=CARTESIAN_POINT ( 'NONE',  ( -18.67979575497178146, -10.72451020669898902, 26.66557627198103475 ) ) ;
#91087=CARTESIAN_POINT ( 'NONE',  ( 21.55341960407619695, -5.719274019375665929, 91.04275706135236135 ) ) ;
#91088=CARTESIAN_POINT ( 'NONE',  ( -21.55341960407610458, -5.719274019375992779, 81.45724293864769550 ) ) ;
#91089=CARTESIAN_POINT ( 'NONE',  ( 18.67979575497194134, -10.72451020669871369, 60.83442372801901854 ) ) ;
#91090=CARTESIAN_POINT ( 'NONE',  ( -21.53943276465977519, -0.05219959533937600094, 68.75109039468568994 ) ) ;
#91091=CARTESIAN_POINT ( 'NONE',  ( -16.46253265017160317, 9.564922557960807481, 90.83224293864769550 ) ) ;
#91092=CARTESIAN_POINT ( 'NONE',  ( -8.224510206698735004, -14.34966873604973081, 99.58442372801900433 ) ) ;
#91093=CARTESIAN_POINT ( 'NONE',  ( 5.719274019375673035, 21.55341960407619339, 47.29275706135234003 ) ) ;
#91094=CARTESIAN_POINT ( 'NONE',  ( 16.46253265017160672, -9.564922557960803928, 28.33224293864769550 ) ) ;
#91096=CARTESIAN_POINT ( 'NONE',  ( -16.55341960407611168, -4.379528057220339221, 66.45724293864768129 ) ) ;
#91097=CARTESIAN_POINT ( 'NONE',  ( 8.224510206698953496, -14.34966873604960469, 32.91557627198102409 ) ) ;
#91098=CARTESIAN_POINT ( 'NONE',  ( 15.72974639402199770, -15.80617190586745480, 48.12390960531436690 ) ) ;
#91099=CARTESIAN_POINT ( 'NONE',  ( 5.049401038298161559, -19.05341960407611168, 72.70724293864768129 ) ) ;
#91100=CARTESIAN_POINT ( 'NONE',  ( -16.51473224551069308, -9.474510206698971260, 51.66557627198102409 ) ) ;
#91101=CARTESIAN_POINT ( 'NONE',  ( 10.72451020669898902, -18.67979575497178502, 57.91557627198103120 ) ) ;
#91102=CARTESIAN_POINT ( 'NONE',  ( 16.51473224551083163, -9.474510206698727899, 40.83442372801900433 ) ) ;
#91104=CARTESIAN_POINT ( 'NONE',  ( 14.34966873604960469, 8.224510206698951720, 54.16557627198103120 ) ) ;
#91105=CARTESIAN_POINT ( 'NONE',  ( 21.52544592524344225, -5.823673210054117533, 23.54057627198102765 ) ) ;
#91106=ORIENTED_EDGE ( 'NONE', *, *, #42468, .T. ) ;
#91107=CARTESIAN_POINT ( 'NONE',  ( -8.314922557961024197, 14.29746914071037800, 67.91775706135234714 ) ) ;
#91108=CARTESIAN_POINT ( 'NONE',  ( -0.05219959533936034679, 19.03943276465977164, 72.50109039468566152 ) ) ;
#91109=CARTESIAN_POINT ( 'NONE',  ( -16.52544592524342804, 4.483927247898546575, 46.04057627198103830 ) ) ;
#91111=CARTESIAN_POINT ( 'NONE',  ( 12.06949235617757843, -12.14591786802309237, 28.12390960531435979 ) ) ;
#91112=CARTESIAN_POINT ( 'NONE',  ( 9.474510206698971260, -16.51473224551069308, 57.91557627198103120 ) ) ;
#91113=CARTESIAN_POINT ( 'NONE',  ( -19.02544592524342804, 5.153800228976336051, 76.04057627198102409 ) ) ;
#91114=CARTESIAN_POINT ( 'NONE',  ( 13.89961937509977652, -13.97604488694527269, 43.12390960531434558 ) ) ;
#91115=CARTESIAN_POINT ( 'NONE',  ( -5.719274019375665041, -21.55341960407619695, 49.79275706135234714 ) ) ;
#91116=CARTESIAN_POINT ( 'NONE',  ( -9.474510206698964154, 16.51473224551069663, 65.41557627198102409 ) ) ;
#91117=B_SPLINE_CURVE_WITH_KNOTS ( 'NONE', 3,
 ( #19549, #2384, #82179, #81194, #48900, #141884, #190394, #1380, #80213, #142875, #188410, #94388, #64063, #140896, #4355, #49887, #187432, #125733, #67038, #139891, #78220, #111553 ),
 .UNSPECIFIED., .F., .F.,
 ( 4, 2, 2, 2, 2, 2, 2, 2, 2, 2, 4 ),
 ( 2.602085213965210642E-18, 0.001309639967555351406, 0.001964459951333025808, 0.002291869943221863659, 0.002455574939166268490, 0.002619279935110673321, 0.002782984931055078152, 0.002946689926999482550, 0.003274099918888319100, 0.003928919902665989165, 0.005238559870221329295 ),
 .UNSPECIFIED. ) ;
#91119=CARTESIAN_POINT ( 'NONE',  ( 16.51473224551069308, 9.474510206698969483, 59.16557627198102409 ) ) ;
#91120=CARTESIAN_POINT ( 'NONE',  ( -15.80617190586745835, -15.72974639402198527, 36.87390960531435979 ) ) ;
#91121=CARTESIAN_POINT ( 'NONE',  ( -16.46253265017160317, 9.564922557960807481, 25.83224293864769194 ) ) ;
#91122=CARTESIAN_POINT ( 'NONE',  ( 5.823673210054125526, 21.52544592524343514, 29.79057627198102409 ) ) ;
#91123=CARTESIAN_POINT ( 'NONE',  ( 12.14591786802327356, -12.06949235617739191, 85.62609039468568994 ) ) ;
#91124=CARTESIAN_POINT ( 'NONE',  ( -15.72974639402176322, -15.80617190586768395, 109.3760903946857042 ) ) ;
#91125=CARTESIAN_POINT ( 'NONE',  ( -16.55341960407617563, 4.379528057220093196, 63.54275706135234003 ) ) ;
#91126=CARTESIAN_POINT ( 'NONE',  ( 19.02544592524343514, -5.153800228976328945, 113.5405762719810241 ) ) ;
#91127=CARTESIAN_POINT ( 'NONE',  ( -16.52544592524335698, -4.483927247898792601, 58.95942372801902565 ) ) ;
#91128=CARTESIAN_POINT ( 'NONE',  ( 16.55341960407618274, -4.379528057220086978, 46.04275706135234714 ) ) ;
#91129=CARTESIAN_POINT ( 'NONE',  ( 9.564922557960805705, 16.46253265017160317, 114.5822429386476955 ) ) ;
#91130=CARTESIAN_POINT ( 'NONE',  ( -4.483927247898782831, 16.52544592524335698, 27.70942372801901854 ) ) ;
#91131=CARTESIAN_POINT ( 'NONE',  ( -13.97604488694527625, -13.89961937509977652, 31.87390960531435979 ) ) ;
#91132=CARTESIAN_POINT ( 'NONE',  ( 10.81492255796106328, -18.62759615963255655, 25.41775706135235779 ) ) ;
#91133=CARTESIAN_POINT ( 'NONE',  ( 16.53943276465976808, 0.05219959533934440121, 26.25109039468567573 ) ) ;
#91134=CARTESIAN_POINT ( 'NONE',  ( -4.483927247898782831, 16.52544592524335698, 82.70942372801900433 ) ) ;
#91136=CARTESIAN_POINT ( 'NONE',  ( -10.72451020669870658, -18.67979575497194134, 84.58442372801903275 ) ) ;
#91137=CARTESIAN_POINT ( 'NONE',  ( 5.049401038297881783, 19.05341960407617563, 82.29275706135229029 ) ) ;
#91138=EDGE_CURVE ( 'NONE', #45079, #22766, #142128, .T. ) ;
#91139=CARTESIAN_POINT ( 'NONE',  ( 14.29746914071049879, -8.314922557960816363, 58.33224293864768839 ) ) ;
#91140=CARTESIAN_POINT ( 'NONE',  ( -4.379528057220328563, 16.55341960407611168, 110.2072429386477239 ) ) ;
#91141=CARTESIAN_POINT ( 'NONE',  ( 19.02544592524334988, 5.153800228976608722, 51.45942372801900433 ) ) ;
#91142=CARTESIAN_POINT ( 'NONE',  ( 17.97161686093728150, -5.500000000000001776, 53.49637206859166128 ) ) ;
#91143=CARTESIAN_POINT ( 'NONE',  ( -5.719274019375665041, -21.55341960407619695, 49.79275706135234714 ) ) ;
#91144=CARTESIAN_POINT ( 'NONE',  ( -16.51473224551082808, 9.474510206698731452, 103.3344237280190043 ) ) ;
#91145=CARTESIAN_POINT ( 'NONE',  ( 16.88567814943161238, 6.947325034625710494, 83.79001122652586275 ) ) ;
#91146=CARTESIAN_POINT ( 'NONE',  ( 5.153800228976335163, 19.02544592524342804, 104.7905762719809957 ) ) ;
#91147=CARTESIAN_POINT ( 'NONE',  ( -21.55341960407610458, -5.719274019375992779, 76.45724293864769550 ) ) ;
#91148=CARTESIAN_POINT ( 'NONE',  ( 16.51473224551083163, -9.474510206698727899, 90.83442372801900433 ) ) ;
#91149=CARTESIAN_POINT ( 'NONE',  ( 9.564922557960805705, 16.46253265017160317, 99.58224293864770971 ) ) ;
#91151=CARTESIAN_POINT ( 'NONE',  ( -8.314922557960811034, -14.29746914071050412, 112.0822429386477097 ) ) ;
#91152=CARTESIAN_POINT ( 'NONE',  ( -5.719274019375665041, -21.55341960407619695, 94.79275706135234714 ) ) ;
#91153=CARTESIAN_POINT ( 'NONE',  ( 16.46253265017160672, -9.564922557960803928, 38.33224293864768839 ) ) ;
#91154=CARTESIAN_POINT ( 'NONE',  ( -18.67979575497193778, 10.72451020669871902, 58.33442372801901143 ) ) ;
#91155=CARTESIAN_POINT ( 'NONE',  ( 5.719274019375673035, 21.55341960407619339, 82.29275706135234714 ) ) ;
#91156=CARTESIAN_POINT ( 'NONE',  ( -16.55341960407617563, 4.379528057220093196, 108.5427570613523756 ) ) ;
#91157=CARTESIAN_POINT ( 'NONE',  ( -15.72974639402176322, -15.80617190586768395, 39.37609039468567573 ) ) ;
#91158=CARTESIAN_POINT ( 'NONE',  ( 18.67979575497194134, -10.72451020669871369, 40.83442372801901854 ) ) ;
#91159=CARTESIAN_POINT ( 'NONE',  ( -13.97604488694547697, 13.89961937509957934, 63.12609039468566152 ) ) ;
#91160=CARTESIAN_POINT ( 'NONE',  ( 5.153800228976335163, 19.02544592524342804, 89.79057627198102409 ) ) ;
#91161=CARTESIAN_POINT ( 'NONE',  ( -14.34966873604960291, -8.224510206698953496, 101.6655762719810383 ) ) ;
#91162=CARTESIAN_POINT ( 'NONE',  ( -10.81492255796078084, -18.62759615963271287, 87.08224293864769550 ) ) ;
#91163=CARTESIAN_POINT ( 'NONE',  ( 0.05219959533910956823, 16.53943276465976808, 59.99890960531436690 ) ) ;
#91164=CARTESIAN_POINT ( 'NONE',  ( 10.72451020669871369, 18.67979575497193778, 102.0844237280190185 ) ) ;
#91165=CARTESIAN_POINT ( 'NONE',  ( -16.52544592524342804, 4.483927247898546575, 81.04057627198102409 ) ) ;
#91166=CARTESIAN_POINT ( 'NONE',  ( 5.153800228976335163, 19.02544592524342804, 29.79057627198102409 ) ) ;
#91167=CARTESIAN_POINT ( 'NONE',  ( -9.564922557961040184, 16.46253265017147172, 82.91775706135233293 ) ) ;
#91168=CARTESIAN_POINT ( 'NONE',  ( -8.224510206698948167, 14.34966873604960824, 55.41557627198102409 ) ) ;
#91169=CARTESIAN_POINT ( 'NONE',  ( 10.81492255796106328, -18.62759615963255655, 100.4177570613523471 ) ) ;
#91170=CARTESIAN_POINT ( 'NONE',  ( -13.97604488694527625, -13.89961937509977652, 96.87390960531433848 ) ) ;
#91171=CARTESIAN_POINT ( 'NONE',  ( 19.05341960407617918, -5.049401038297876454, 61.04275706135232582 ) ) ;
#91172=CARTESIAN_POINT ( 'NONE',  ( -18.67979575497178146, -10.72451020669898902, 81.66557627198103830 ) ) ;
#91173=CARTESIAN_POINT ( 'NONE',  ( -21.53943276465977519, -0.05219959533937600094, 28.75109039468567929 ) ) ;
#91174=CARTESIAN_POINT ( 'NONE',  ( -8.314922557961024197, 14.29746914071037800, 32.91775706135234714 ) ) ;
#91175=CARTESIAN_POINT ( 'NONE',  ( -12.14591786802326823, 12.06949235617739902, 78.12609039468570415 ) ) ;
#91176=CARTESIAN_POINT ( 'NONE',  ( -5.153800228976328057, -19.02544592524343514, 27.29057627198103120 ) ) ;
#91177=CARTESIAN_POINT ( 'NONE',  ( 0.05219959533907565091, 21.53943276465977519, 114.9989096053143669 ) ) ;
#91178=CARTESIAN_POINT ( 'NONE',  ( 8.224510206698953496, -14.34966873604960469, 112.9155762719810383 ) ) ;
#91180=CARTESIAN_POINT ( 'NONE',  ( -4.483927247898782831, 16.52544592524335698, 42.70942372801901854 ) ) ;
#91181=CARTESIAN_POINT ( 'NONE',  ( -16.53943276465976808, 0.05219959533911058130, 81.24890960531436690 ) ) ;
#91182=CARTESIAN_POINT ( 'NONE',  ( -5.719274019375978568, 21.55341960407610458, 75.20724293864769550 ) ) ;
#91183=CARTESIAN_POINT ( 'NONE',  ( 8.224510206698953496, -14.34966873604960469, 27.91557627198103830 ) ) ;
#91184=CARTESIAN_POINT ( 'NONE',  ( 8.314922557961029526, -14.29746914071037800, 45.41775706135234003 ) ) ;
#91185=CARTESIAN_POINT ( 'NONE',  ( -19.03943276465977164, 0.05219959533909376836, 41.24890960531435269 ) ) ;
#91186=CARTESIAN_POINT ( 'NONE',  ( 8.224510206698742110, 14.34966873604972548, 77.08442372801901854 ) ) ;
#91187=CARTESIAN_POINT ( 'NONE',  ( 19.02544592524334988, 5.153800228976608722, 76.45942372801897591 ) ) ;
#91188=CARTESIAN_POINT ( 'NONE',  ( -18.67979575497178146, -10.72451020669898902, 66.66557627198102409 ) ) ;
#91189=CARTESIAN_POINT ( 'NONE',  ( 0.05219959533934541429, -16.53943276465976808, 110.0010903946856757 ) ) ;
#91191=CARTESIAN_POINT ( 'NONE',  ( -21.53943276465977519, 0.05219959533907696930, 46.24890960531435979 ) ) ;
#91193=CARTESIAN_POINT ( 'NONE',  ( -8.224510206698735004, -14.34966873604973081, 89.58442372801901854 ) ) ;
#91194=ORIENTED_EDGE ( 'NONE', *, *, #177334, .T. ) ;
#91195=CARTESIAN_POINT ( 'NONE',  ( -13.89961937509977652, 13.97604488694528158, 115.6239096053143669 ) ) ;
#91197=CARTESIAN_POINT ( 'NONE',  ( 15.80617190586746368, 15.72974639402197994, 79.37390960531436690 ) ) ;
#91198=CARTESIAN_POINT ( 'NONE',  ( -8.314922557961024197, 14.29746914071037800, 107.9177570613523471 ) ) ;
#91199=CARTESIAN_POINT ( 'NONE',  ( -8.224510206698735004, -14.34966873604973081, 24.58442372801901499 ) ) ;
#91200=CARTESIAN_POINT ( 'NONE',  ( -13.97604488694527625, -13.89961937509977652, 21.87390960531435979 ) ) ;
#91201=CARTESIAN_POINT ( 'NONE',  ( 14.29746914071037800, 8.314922557961029526, 31.66775706135234358 ) ) ;
#91202=CARTESIAN_POINT ( 'NONE',  ( 5.153800228976335163, 19.02544592524342804, 54.79057627198103120 ) ) ;
#91204=CARTESIAN_POINT ( 'NONE',  ( 16.46253265017160672, -9.564922557960803928, 98.33224293864769550 ) ) ;
#91205=CARTESIAN_POINT ( 'NONE',  ( -12.06949235617739369, -12.14591786802326823, 89.37609039468568994 ) ) ;
#91206=CARTESIAN_POINT ( 'NONE',  ( 16.46253265017146816, 9.564922557961045513, 96.66775706135233293 ) ) ;
#91207=CARTESIAN_POINT ( 'NONE',  ( 13.97604488694548053, -13.89961937509957401, 25.62609039468566507 ) ) ;
#91208=CARTESIAN_POINT ( 'NONE',  ( 15.72974639402199770, -15.80617190586745480, 73.12390960531436690 ) ) ;
#91209=CARTESIAN_POINT ( 'NONE',  ( 12.14591786802327356, -12.06949235617739191, 100.6260903946857184 ) ) ;
#91210=CARTESIAN_POINT ( 'NONE',  ( -19.03943276465977164, -0.05219959533935918106, 98.75109039468567573 ) ) ;
#91211=CARTESIAN_POINT ( 'NONE',  ( -16.46253265017160317, 9.564922557960807481, 55.83224293864769550 ) ) ;
#91212=CARTESIAN_POINT ( 'NONE',  ( 19.05341960407611168, 5.049401038298154454, 88.95724293864769550 ) ) ;
#91213=CARTESIAN_POINT ( 'NONE',  ( 10.72451020669871369, 18.67979575497193778, 67.08442372801901854 ) ) ;
#91214=CARTESIAN_POINT ( 'NONE',  ( 0.05219959533909260263, 19.03943276465977164, 49.99890960531435979 ) ) ;
#91215=CARTESIAN_POINT ( 'NONE',  ( -17.50000000000000355, -5.624438216177585659, 84.18329655085358354 ) ) ;
#91216=CARTESIAN_POINT ( 'NONE',  ( -16.53943276465976808, 0.05219959533911058130, 81.24890960531436690 ) ) ;
#91217=CARTESIAN_POINT ( 'NONE',  ( -15.72974639402197994, 15.80617190586746368, 75.62390960531439532 ) ) ;
#91218=CARTESIAN_POINT ( 'NONE',  ( 20.28939339942064279, -0.9295024462021991285, 102.5000000000000284 ) ) ;
#91220=CARTESIAN_POINT ( 'NONE',  ( -19.03943276465977164, -0.05219959533935918106, 48.75109039468566863 ) ) ;
#91222=CARTESIAN_POINT ( 'NONE',  ( 5.049401038298161559, -19.05341960407611168, 82.70724293864770971 ) ) ;
#91223=CARTESIAN_POINT ( 'NONE',  ( 16.46253265017160672, -9.564922557960803928, 83.33224293864768129 ) ) ;
#91224=CARTESIAN_POINT ( 'NONE',  ( 4.379528057220092307, 16.55341960407617563, 62.29275706135236845 ) ) ;
#91225=CARTESIAN_POINT ( 'NONE',  ( -17.50000000000000355, -5.500000000000022204, 66.28230962303567253 ) ) ;
#91226=CARTESIAN_POINT ( 'NONE',  ( 9.564922557961047289, -16.46253265017146816, 25.41775706135234003 ) ) ;
#91228=CARTESIAN_POINT ( 'NONE',  ( -16.52544592524335698, -4.483927247898792601, 83.95942372801900433 ) ) ;
#91230=CARTESIAN_POINT ( 'NONE',  ( 8.224510206698742110, 14.34966873604972548, 77.08442372801901854 ) ) ;
#91232=CARTESIAN_POINT ( 'NONE',  ( 14.29746914071037800, 8.314922557961029526, 56.66775706135235424 ) ) ;
#91234=CARTESIAN_POINT ( 'NONE',  ( 15.80617190586769283, -15.72974639402175789, 65.62609039468568994 ) ) ;
#91235=CARTESIAN_POINT ( 'NONE',  ( 19.02544592524334988, 5.153800228976608722, 81.45942372801897591 ) ) ;
#91236=CARTESIAN_POINT ( 'NONE',  ( 10.72451020669871369, 18.67979575497193778, 102.0844237280190185 ) ) ;
#91237=CARTESIAN_POINT ( 'NONE',  ( -5.153800228976328057, -19.02544592524343514, 52.29057627198100988 ) ) ;
#91238=CARTESIAN_POINT ( 'NONE',  ( 13.89961937509977652, -13.97604488694527269, 38.12390960531436690 ) ) ;
#91240=CARTESIAN_POINT ( 'NONE',  ( 21.55341960407610458, 5.719274019375980345, 63.95724293864770260 ) ) ;
#91241=CARTESIAN_POINT ( 'NONE',  ( 16.51473224551069308, 9.474510206698969483, 114.1655762719810241 ) ) ;
#91242=CARTESIAN_POINT ( 'NONE',  ( -16.51473224551069308, -9.474510206698971260, 26.66557627198103120 ) ) ;
#91243=CARTESIAN_POINT ( 'NONE',  ( 8.224510206698742110, 14.34966873604972548, 52.08442372801901854 ) ) ;
#91245=CARTESIAN_POINT ( 'NONE',  ( -18.62759615963270932, 10.81492255796079327, 110.8322429386476955 ) ) ;
#91246=CARTESIAN_POINT ( 'NONE',  ( 14.34966873604960469, 8.224510206698951720, 49.16557627198102409 ) ) ;
#91248=CARTESIAN_POINT ( 'NONE',  ( -0.05219959533936034679, 19.03943276465977164, 112.5010903946856757 ) ) ;
#91249=CARTESIAN_POINT ( 'NONE',  ( 19.03943276465977164, 0.05219959533936151252, 41.25109039468566152 ) ) ;
#91250=CARTESIAN_POINT ( 'NONE',  ( 16.52544592524342804, -4.483927247898539470, 38.54057627198103120 ) ) ;
#91251=CARTESIAN_POINT ( 'NONE',  ( -5.719274019375665041, -21.55341960407619695, 19.79275706135235069 ) ) ;
#91252=CARTESIAN_POINT ( 'NONE',  ( 16.21995358207305316, 7.366697692864111247, 32.56448998487844193 ) ) ;
#91253=CARTESIAN_POINT ( 'NONE',  ( -5.823673210054116645, -21.52544592524344225, 62.29057627198102409 ) ) ;
#91254=CARTESIAN_POINT ( 'NONE',  ( -5.049401038298153566, 19.05341960407611168, 85.20724293864766707 ) ) ;
#91255=CARTESIAN_POINT ( 'NONE',  ( 4.379528057220339221, -16.55341960407611168, 52.70724293864769550 ) ) ;
#91256=CARTESIAN_POINT ( 'NONE',  ( -9.564922557960796823, -16.46253265017161027, 107.0822429386476955 ) ) ;
#91258=CARTESIAN_POINT ( 'NONE',  ( 16.51473224551083163, -9.474510206698727899, 55.83442372801899722 ) ) ;
#91259=CARTESIAN_POINT ( 'NONE',  ( 18.67979575497178502, 10.72451020669898547, 94.16557627198103830 ) ) ;
#91260=CARTESIAN_POINT ( 'NONE',  ( 9.474510206698971260, -16.51473224551069308, 37.91557627198102409 ) ) ;
#91261=CARTESIAN_POINT ( 'NONE',  ( 19.03943276465977164, -0.05219959533909143690, 23.74890960531435269 ) ) ;
#91263=CARTESIAN_POINT ( 'NONE',  ( 5.823673210054444382, -21.52544592524334988, 55.20942372801902565 ) ) ;
#91265=CARTESIAN_POINT ( 'NONE',  ( 12.14591786802309770, 12.06949235617756955, 29.37390960531435269 ) ) ;
#91266=CARTESIAN_POINT ( 'NONE',  ( 19.02544592524343514, -5.153800228976328945, 53.54057627198102409 ) ) ;
#91267=CARTESIAN_POINT ( 'NONE',  ( -19.03943276465977164, 0.05219959533909376836, 96.24890960531436690 ) ) ;
#91268=CARTESIAN_POINT ( 'NONE',  ( 21.53943276465977519, -0.05219959533907433946, 58.74890960531436690 ) ) ;
#91270=CARTESIAN_POINT ( 'NONE',  ( 19.03943276465977164, -0.05219959533909143690, 43.74890960531435979 ) ) ;
#91271=CARTESIAN_POINT ( 'NONE',  ( 18.62759615963271287, -10.81492255796078972, 58.33224293864768839 ) ) ;
#91272=CARTESIAN_POINT ( 'NONE',  ( -5.719274019375665041, -21.55341960407619695, 84.79275706135234714 ) ) ;
#91274=CARTESIAN_POINT ( 'NONE',  ( -0.05219959533934338120, 16.53943276465976808, 87.50109039468568994 ) ) ;
#91275=CARTESIAN_POINT ( 'NONE',  ( -4.379528057220328563, 16.55341960407611168, 70.20724293864769550 ) ) ;
#91276=CARTESIAN_POINT ( 'NONE',  ( 0.05219959533934541429, -16.53943276465976808, 90.00109039468567573 ) ) ;
#91277=CARTESIAN_POINT ( 'NONE',  ( 13.97604488694527802, 13.89961937509977652, 69.37390960531436690 ) ) ;
#91278=ORIENTED_EDGE ( 'NONE', *, *, #98059, .T. ) ;
#91279=CARTESIAN_POINT ( 'NONE',  ( -0.05219959533936034679, 19.03943276465977164, 27.50109039468566507 ) ) ;
#91280=CARTESIAN_POINT ( 'NONE',  ( -14.29746914071037622, -8.314922557961029526, 84.16775706135234714 ) ) ;
#91281=CARTESIAN_POINT ( 'NONE',  ( 9.474510206698729675, 16.51473224551082808, 22.08442372801899722 ) ) ;
#91282=CARTESIAN_POINT ( 'NONE',  ( 5.049401038298161559, -19.05341960407611168, 77.70724293864765286 ) ) ;
#91283=CARTESIAN_POINT ( 'NONE',  ( -21.53943276465977519, 0.05219959533907696930, 51.24890960531436690 ) ) ;
#91284=CARTESIAN_POINT ( 'NONE',  ( 8.224510206698742110, 14.34966873604972548, 22.08442372801901143 ) ) ;
#91285=CARTESIAN_POINT ( 'NONE',  ( -10.81492255796105439, 18.62759615963255655, 77.91775706135231871 ) ) ;
#91286=CARTESIAN_POINT ( 'NONE',  ( -16.52544592524335698, -4.483927247898792601, 63.95942372801901854 ) ) ;
#91287=CARTESIAN_POINT ( 'NONE',  ( 21.52544592524334988, 5.823673210054432836, 21.45942372801901499 ) ) ;
#91288=CARTESIAN_POINT ( 'NONE',  ( -16.51473224551082808, 9.474510206698731452, 108.3344237280190043 ) ) ;
#91289=CARTESIAN_POINT ( 'NONE',  ( 5.049401038298161559, -19.05341960407611168, 87.70724293864769550 ) ) ;
#91290=CARTESIAN_POINT ( 'NONE',  ( 12.06949235617739724, 12.14591786802326823, 21.87609039468567573 ) ) ;
#91291=CARTESIAN_POINT ( 'NONE',  ( 19.05341960407611168, 5.049401038298154454, 43.95724293864769550 ) ) ;
#91292=CARTESIAN_POINT ( 'NONE',  ( 14.34966873604972726, -8.224510206698740333, 30.83442372801902209 ) ) ;
#91293=CARTESIAN_POINT ( 'NONE',  ( 16.53943276465976808, -0.05219959533910856209, 83.74890960531435269 ) ) ;
#91294=CARTESIAN_POINT ( 'NONE',  ( 4.483927247898790824, -16.52544592524335698, 90.20942372801903275 ) ) ;
#91295=CARTESIAN_POINT ( 'NONE',  ( -21.52544592524334988, -5.823673210054445271, 23.95942372801901143 ) ) ;
#91296=CARTESIAN_POINT ( 'NONE',  ( -16.46253265017160317, 9.564922557960807481, 65.83224293864769550 ) ) ;
#91297=CARTESIAN_POINT ( 'NONE',  ( 0.05219959533909260263, 19.03943276465977164, 64.99890960531436690 ) ) ;
#91298=CARTESIAN_POINT ( 'NONE',  ( 12.06949235617739724, 12.14591786802326823, 81.87609039468568994 ) ) ;
#91302=CARTESIAN_POINT ( 'NONE',  ( 0.05219959533936267826, -19.03943276465977164, 30.00109039468566863 ) ) ;
#91303=CARTESIAN_POINT ( 'NONE',  ( 9.564922557960805705, 16.46253265017160317, 49.58224293864770260 ) ) ;
#91304=CARTESIAN_POINT ( 'NONE',  ( -16.51473224551069308, -9.474510206698971260, 111.6655762719810383 ) ) ;
#91305=VERTEX_POINT ( 'NONE', #101081 ) ;
#91306=CARTESIAN_POINT ( 'NONE',  ( -16.53943276465976808, -0.05219959533934237506, 23.75109039468567929 ) ) ;
#91307=CARTESIAN_POINT ( 'NONE',  ( -19.03943276465977164, -0.05219959533935918106, 63.75109039468566863 ) ) ;
#91308=CARTESIAN_POINT ( 'NONE',  ( 0.05219959533934541429, -16.53943276465976808, 45.00109039468568284 ) ) ;
#91309=CARTESIAN_POINT ( 'NONE',  ( 9.474510206698971260, -16.51473224551069308, 102.9155762719810241 ) ) ;
#91310=CARTESIAN_POINT ( 'NONE',  ( 5.049401038298161559, -19.05341960407611168, 82.70724293864770971 ) ) ;
#91311=CARTESIAN_POINT ( 'NONE',  ( -18.62759615963270932, 10.81492255796079327, 95.83224293864770971 ) ) ;
#91312=CARTESIAN_POINT ( 'NONE',  ( -5.049401038297874678, -19.05341960407617918, 64.79275706135233293 ) ) ;
#91313=CARTESIAN_POINT ( 'NONE',  ( -19.05341960407611168, -5.049401038298163336, 91.45724293864766707 ) ) ;
#91314=CARTESIAN_POINT ( 'NONE',  ( 13.89961937509977652, -13.97604488694527269, 23.12390960531436335 ) ) ;
#91316=CARTESIAN_POINT ( 'NONE',  ( -0.05219959533909027116, -19.03943276465977164, 57.49890960531435979 ) ) ;
#91317=CARTESIAN_POINT ( 'NONE',  ( -14.34966873604972548, 8.224510206698743886, 108.3344237280190185 ) ) ;
#91318=CARTESIAN_POINT ( 'NONE',  ( -5.153800228976328057, -19.02544592524343514, 27.29057627198103120 ) ) ;
#91319=CARTESIAN_POINT ( 'NONE',  ( 19.02544592524334988, 5.153800228976608722, 36.45942372801900433 ) ) ;
#91320=CARTESIAN_POINT ( 'NONE',  ( 16.55341960407611168, 4.379528057220329451, 78.95724293864769550 ) ) ;
#91321=CARTESIAN_POINT ( 'NONE',  ( -21.55341960407619339, 5.719274019375674811, 93.54275706135234714 ) ) ;
#91322=CARTESIAN_POINT ( 'NONE',  ( 19.03943276465977164, -0.05219959533909143690, 38.74890960531436690 ) ) ;
#91323=CARTESIAN_POINT ( 'NONE',  ( -12.14591786802326823, 12.06949235617739902, 53.12609039468568284 ) ) ;
#91324=CARTESIAN_POINT ( 'NONE',  ( -12.14591786802309592, -12.06949235617757132, 41.87390960531435979 ) ) ;
#91325=CARTESIAN_POINT ( 'NONE',  ( 5.823673210054444382, -21.52544592524334988, 90.20942372801903275 ) ) ;
#91326=CARTESIAN_POINT ( 'NONE',  ( 16.51473224551069308, 9.474510206698969483, 89.16557627198103830 ) ) ;
#91327=CARTESIAN_POINT ( 'NONE',  ( -5.049401038298153566, 19.05341960407611168, 100.2072429386476955 ) ) ;
#91328=CARTESIAN_POINT ( 'NONE',  ( -16.53943276465976808, 0.05219959533911058130, 111.2489096053143669 ) ) ;
#91329=CARTESIAN_POINT ( 'NONE',  ( -14.34966873604960291, -8.224510206698953496, 71.66557627198100988 ) ) ;
#91330=CARTESIAN_POINT ( 'NONE',  ( 15.72974639402199770, -15.80617190586745480, 78.12390960531436690 ) ) ;
#91331=CARTESIAN_POINT ( 'NONE',  ( -0.05219959533909027116, -19.03943276465977164, 82.49890960531436690 ) ) ;
#91332=CARTESIAN_POINT ( 'NONE',  ( -18.62759615963270932, 10.81492255796079327, 100.8322429386477097 ) ) ;
#91333=CARTESIAN_POINT ( 'NONE',  ( -16.51473224551069308, -9.474510206698971260, 86.66557627198102409 ) ) ;
#91334=CARTESIAN_POINT ( 'NONE',  ( 19.01533133064927128, -5.499999999999451106, 46.26586590595743331 ) ) ;
#91335=CARTESIAN_POINT ( 'NONE',  ( 16.52544592524342804, -4.483927247898539470, 93.54057627198103830 ) ) ;
#91336=CARTESIAN_POINT ( 'NONE',  ( 19.05341960407611168, 5.049401038298154454, 53.95724293864770260 ) ) ;
#91337=CARTESIAN_POINT ( 'NONE',  ( -10.72451020669898014, 18.67979575497178502, 60.41557627198102409 ) ) ;
#91339=CARTESIAN_POINT ( 'NONE',  ( 17.31747979337950483, -6.344076630960993946, 26.12055131934816998 ) ) ;
#91340=CARTESIAN_POINT ( 'NONE',  ( -0.05219959533910754901, -16.53943276465976808, 22.49890960531436335 ) ) ;
#91342=CARTESIAN_POINT ( 'NONE',  ( 0.05219959533934541429, -16.53943276465976808, 25.00109039468567218 ) ) ;
#91343=CARTESIAN_POINT ( 'NONE',  ( 12.14591786802309770, 12.06949235617756955, 79.37390960531436690 ) ) ;
#91344=CARTESIAN_POINT ( 'NONE',  ( -16.61371651742605238, -7.165104196376108625, 96.14584930007005426 ) ) ;
#91345=CARTESIAN_POINT ( 'NONE',  ( -16.51473224551069308, -9.474510206698971260, 71.66557627198102409 ) ) ;
#91346=CARTESIAN_POINT ( 'NONE',  ( 16.51473224551069308, 9.474510206698969483, 39.16557627198103120 ) ) ;
#91347=CARTESIAN_POINT ( 'NONE',  ( 12.14591786802309770, 12.06949235617756955, 69.37390960531436690 ) ) ;
#91348=CARTESIAN_POINT ( 'NONE',  ( -9.474510206698964154, 16.51473224551069663, 115.4155762719810241 ) ) ;
#91349=CARTESIAN_POINT ( 'NONE',  ( -9.564922557961040184, 16.46253265017147172, 107.9177570613523471 ) ) ;
#91350=CARTESIAN_POINT ( 'NONE',  ( 5.153800228976335163, 19.02544592524342804, 104.7905762719809957 ) ) ;
#91351=CARTESIAN_POINT ( 'NONE',  ( -10.81492255796078084, -18.62759615963271287, 72.08224293864769550 ) ) ;
#91352=CARTESIAN_POINT ( 'NONE',  ( 14.34966873604972726, -8.224510206698740333, 75.83442372801900433 ) ) ;
#91353=CARTESIAN_POINT ( 'NONE',  ( -16.19135201231352639, 7.376712067591987498, 94.81319145947880145 ) ) ;
#91354=CARTESIAN_POINT ( 'NONE',  ( 19.05341960407611168, 5.049401038298154454, 63.95724293864769550 ) ) ;
#91355=CARTESIAN_POINT ( 'NONE',  ( -10.81492255796078084, -18.62759615963271287, 87.08224293864769550 ) ) ;
#91356=CARTESIAN_POINT ( 'NONE',  ( -16.51473224551082808, 9.474510206698731452, 103.3344237280190043 ) ) ;
#91357=VECTOR ( 'NONE', #105001, 1000.000000000000000 ) ;
#91358=CARTESIAN_POINT ( 'NONE',  ( -8.314922557960811034, -14.29746914071050412, 42.08224293864769550 ) ) ;
#91359=CARTESIAN_POINT ( 'NONE',  ( 21.52544592524334988, 5.823673210054432836, 61.45942372801901854 ) ) ;
#91360=CARTESIAN_POINT ( 'NONE',  ( 17.49999999999999289, 5.500000000000007994, 83.78230962303564411 ) ) ;
#91361=CARTESIAN_POINT ( 'NONE',  ( -8.314922557961024197, 14.29746914071037800, 72.91775706135234714 ) ) ;
#91362=CARTESIAN_POINT ( 'NONE',  ( -19.02544592524342804, 5.153800228976336051, 111.0405762719810099 ) ) ;
#91363=CARTESIAN_POINT ( 'NONE',  ( -13.97604488694527625, -13.89961937509977830, 106.8739096053143669 ) ) ;
#91365=CARTESIAN_POINT ( 'NONE',  ( -0.05219959533934338120, 16.53943276465976808, 92.50109039468567573 ) ) ;
#91366=CARTESIAN_POINT ( 'NONE',  ( -4.483927247898782831, 16.52544592524335698, 42.70942372801901854 ) ) ;
#91367=CARTESIAN_POINT ( 'NONE',  ( 16.46253265017160672, -9.564922557960803928, 63.33224293864769550 ) ) ;
#91368=CARTESIAN_POINT ( 'NONE',  ( 13.89961937509977652, -13.97604488694527269, 73.12390960531436690 ) ) ;
#91369=CARTESIAN_POINT ( 'NONE',  ( -15.80617190586768217, 15.72974639402176855, 68.12609039468567573 ) ) ;
#91370=CARTESIAN_POINT ( 'NONE',  ( 14.29746914071037800, 8.314922557961029526, 56.66775706135235424 ) ) ;
#91371=CARTESIAN_POINT ( 'NONE',  ( -8.314922557960811034, -14.29746914071050412, 37.08224293864768129 ) ) ;
#91372=CARTESIAN_POINT ( 'NONE',  ( -19.02544592524342804, 5.153800228976336051, 41.04057627198103120 ) ) ;
#91373=CARTESIAN_POINT ( 'NONE',  ( 0.05219959533909260263, 19.03943276465977164, 34.99890960531435979 ) ) ;
#91374=CARTESIAN_POINT ( 'NONE',  ( 12.14591786802327356, -12.06949235617739191, 40.62609039468567573 ) ) ;
#91377=CARTESIAN_POINT ( 'NONE',  ( -19.02544592524334988, -5.153800228976617603, 88.95942372801897591 ) ) ;
#91378=CARTESIAN_POINT ( 'NONE',  ( 16.55341960407611168, 4.379528057220329451, 98.95724293864770971 ) ) ;
#91379=CARTESIAN_POINT ( 'NONE',  ( -19.05341960407611168, -5.049401038298163336, 51.45724293864770260 ) ) ;
#91380=CARTESIAN_POINT ( 'NONE',  ( -9.564922557961040184, 16.46253265017147172, 87.91775706135233293 ) ) ;
#91382=CARTESIAN_POINT ( 'NONE',  ( 18.67979575497194134, -10.72451020669871369, 85.83442372801901854 ) ) ;
#91383=CARTESIAN_POINT ( 'NONE',  ( 8.314922557961029526, -14.29746914071037800, 60.41775706135235424 ) ) ;
#91384=FACE_OUTER_BOUND ( 'NONE', #76281, .T. ) ;
#91385=CARTESIAN_POINT ( 'NONE',  ( -10.81492255796078084, -18.62759615963271287, 47.08224293864770260 ) ) ;
#91386=CARTESIAN_POINT ( 'NONE',  ( -8.314922557961024197, 14.29746914071037800, 42.91775706135235424 ) ) ;
#91387=CARTESIAN_POINT ( 'NONE',  ( 5.049401038298163336, -19.05341960407611168, 37.70724293864768839 ) ) ;
#91388=CARTESIAN_POINT ( 'NONE',  ( -5.153800228976607833, 19.02544592524334988, 42.70942372801901143 ) ) ;
#91389=CARTESIAN_POINT ( 'NONE',  ( 5.153800228976335163, 19.02544592524342804, 84.79057627198099567 ) ) ;
#91390=CARTESIAN_POINT ( 'NONE',  ( -16.53943276465976808, 0.05219959533911058130, 101.2489096053143669 ) ) ;
#91391=CARTESIAN_POINT ( 'NONE',  ( 13.97604488694527802, 13.89961937509977652, 54.37390960531435979 ) ) ;
#91393=CARTESIAN_POINT ( 'NONE',  ( 15.72974639402176855, 15.80617190586768217, 81.87609039468568994 ) ) ;
#91394=CARTESIAN_POINT ( 'NONE',  ( -17.49999999999999645, -5.499999999999992895, 89.20309617465829888 ) ) ;
#91395=CARTESIAN_POINT ( 'NONE',  ( -9.564922557961040184, 16.46253265017147172, 27.91775706135232582 ) ) ;
#91396=CARTESIAN_POINT ( 'NONE',  ( -10.81492255796105439, 18.62759615963255655, 112.9177570613523329 ) ) ;
#91397=CARTESIAN_POINT ( 'NONE',  ( 16.52544592524342804, -4.483927247898539470, 53.54057627198103120 ) ) ;
#91398=CARTESIAN_POINT ( 'NONE',  ( 5.049401038298161559, -19.05341960407611168, 62.70724293864769550 ) ) ;
#91399=CARTESIAN_POINT ( 'NONE',  ( -16.51473224551069308, -9.474510206698971260, 111.6655762719810383 ) ) ;
#91400=CARTESIAN_POINT ( 'NONE',  ( 5.719274019375673035, 21.55341960407619339, 82.29275706135234714 ) ) ;
#91401=CARTESIAN_POINT ( 'NONE',  ( -19.03943276465977164, 0.05219959533909376836, 61.24890960531436690 ) ) ;
#91403=CARTESIAN_POINT ( 'NONE',  ( 21.52544592524334988, 5.823673210054432836, 86.45942372801901854 ) ) ;
#91404=CARTESIAN_POINT ( 'NONE',  ( -10.81492255796078084, -18.62759615963271287, 42.08224293864769550 ) ) ;
#91405=CARTESIAN_POINT ( 'NONE',  ( -15.72974639402176322, -15.80617190586768395, 34.37609039468568284 ) ) ;
#91406=CARTESIAN_POINT ( 'NONE',  ( 19.02544592524334988, 5.153800228976608722, 56.45942372801898301 ) ) ;
#91407=CARTESIAN_POINT ( 'NONE',  ( 9.474510206698971260, -16.51473224551069308, 27.91557627198103120 ) ) ;
#91408=CARTESIAN_POINT ( 'NONE',  ( -16.51473224551069308, -9.474510206698971260, 71.66557627198102409 ) ) ;
#91409=CARTESIAN_POINT ( 'NONE',  ( -16.52544592524335698, -4.483927247898792601, 23.95942372801901143 ) ) ;
#91410=CARTESIAN_POINT ( 'NONE',  ( 8.224510206698953496, -14.34966873604960469, 87.91557627198103830 ) ) ;
#91411=CARTESIAN_POINT ( 'NONE',  ( -5.049401038298153566, 19.05341960407611168, 60.20724293864768129 ) ) ;
#91412=CARTESIAN_POINT ( 'NONE',  ( 18.62759615963271287, -10.81492255796078972, 43.33224293864769550 ) ) ;
#91414=CARTESIAN_POINT ( 'NONE',  ( 13.89961937509957401, 13.97604488694547697, 111.8760903946856757 ) ) ;
#91415=CARTESIAN_POINT ( 'NONE',  ( 21.52544592524334988, 5.823673210054432836, 21.45942372801901499 ) ) ;
#91416=CARTESIAN_POINT ( 'NONE',  ( 15.80617190586769283, -15.72974639402175789, 75.62609039468567573 ) ) ;
#91417=CARTESIAN_POINT ( 'NONE',  ( 16.55341960407618274, -4.379528057220086978, 76.04275706135237556 ) ) ;
#91418=CARTESIAN_POINT ( 'NONE',  ( 16.55341960407618274, -4.379528057220086978, 71.04275706135234714 ) ) ;
#91419=CARTESIAN_POINT ( 'NONE',  ( 19.05341960407611168, 5.049401038298154454, 63.95724293864769550 ) ) ;
#91420=CARTESIAN_POINT ( 'NONE',  ( -4.483927247898782831, 16.52544592524335698, 87.70942372801901854 ) ) ;
#91421=CARTESIAN_POINT ( 'NONE',  ( -13.97604488694547697, 13.89961937509957934, 43.12609039468566152 ) ) ;
#91422=CARTESIAN_POINT ( 'NONE',  ( 21.52544592524344225, -5.823673210054117533, 113.5405762719810383 ) ) ;
#91423=CARTESIAN_POINT ( 'NONE',  ( 16.55341960407611168, 4.379528057220329451, 63.95724293864770260 ) ) ;
#91424=CARTESIAN_POINT ( 'NONE',  ( -5.049401038298153566, 19.05341960407611168, 85.20724293864766707 ) ) ;
#91425=CARTESIAN_POINT ( 'NONE',  ( 14.34966873604972726, -8.224510206698740333, 85.83442372801901854 ) ) ;
#91426=CARTESIAN_POINT ( 'NONE',  ( 5.823673210054444382, -21.52544592524334988, 60.20942372801902565 ) ) ;
#91427=CARTESIAN_POINT ( 'NONE',  ( 12.06949235617739724, 12.14591786802326823, 36.87609039468568994 ) ) ;
#91428=CARTESIAN_POINT ( 'NONE',  ( 0.05219959533937995610, -21.53943276465977519, 20.00109039468568639 ) ) ;
#91429=CARTESIAN_POINT ( 'NONE',  ( 4.483927247898545687, 16.52544592524342804, 59.79057627198103120 ) ) ;
#91431=CARTESIAN_POINT ( 'NONE',  ( 21.55341960407610458, 5.719274019375980345, 103.9572429386476813 ) ) ;
#91432=CARTESIAN_POINT ( 'NONE',  ( 0.05219959533910956823, 16.53943276465976808, 34.99890960531435979 ) ) ;
#91433=ORIENTED_EDGE ( 'NONE', *, *, #33819, .T. ) ;
#91435=CARTESIAN_POINT ( 'NONE',  ( -18.67979575497178146, -10.72451020669898902, 111.6655762719810525 ) ) ;
#91436=CARTESIAN_POINT ( 'NONE',  ( -9.564922557960796823, -16.46253265017161027, 107.0822429386476955 ) ) ;
#91437=CARTESIAN_POINT ( 'NONE',  ( 5.719274019375673035, 21.55341960407619339, 37.29275706135235424 ) ) ;
#91438=CARTESIAN_POINT ( 'NONE',  ( -12.14591786802309592, -12.06949235617757132, 56.87390960531436690 ) ) ;
#91439=CARTESIAN_POINT ( 'NONE',  ( -19.02544592524342804, 5.153800228976336051, 61.04057627198103120 ) ) ;
#91440=CARTESIAN_POINT ( 'NONE',  ( 5.153800228976615827, -19.02544592524334988, 70.20942372801899012 ) ) ;
#91441=CARTESIAN_POINT ( 'NONE',  ( -16.51473224551069308, -9.474510206698971260, 91.66557627198103830 ) ) ;
#91442=CARTESIAN_POINT ( 'NONE',  ( 10.72451020669898902, -18.67979575497178502, 47.91557627198102409 ) ) ;
#91444=CARTESIAN_POINT ( 'NONE',  ( 9.474510206698971260, -16.51473224551069308, 52.91557627198102409 ) ) ;
#91445=CARTESIAN_POINT ( 'NONE',  ( 8.314922557961029526, -14.29746914071037800, 35.41775706135234003 ) ) ;
#91446=CARTESIAN_POINT ( 'NONE',  ( -9.474510206698720793, -16.51473224551083518, 59.58442372801900433 ) ) ;
#91447=CARTESIAN_POINT ( 'NONE',  ( 10.72451020669898902, -18.67979575497178502, 112.9155762719810383 ) ) ;
#91448=CARTESIAN_POINT ( 'NONE',  ( -4.379528057220328563, 16.55341960407611168, 45.20724293864769550 ) ) ;
#91449=VERTEX_POINT ( 'NONE', #116263 ) ;
#91450=CARTESIAN_POINT ( 'NONE',  ( -13.89961937509977652, 13.97604488694528158, 85.62390960531433848 ) ) ;
#91451=CARTESIAN_POINT ( 'NONE',  ( -21.55341960407610458, -5.719274019375992779, 66.45724293864768129 ) ) ;
#91452=CARTESIAN_POINT ( 'NONE',  ( -15.72974639402197994, 15.80617190586746368, 110.6239096053143669 ) ) ;
#91453=CARTESIAN_POINT ( 'NONE',  ( 4.483927247898790824, -16.52544592524335698, 40.20942372801901854 ) ) ;
#91454=CARTESIAN_POINT ( 'NONE',  ( -5.823673210054116645, -21.52544592524344225, 32.29057627198102409 ) ) ;
#91455=CARTESIAN_POINT ( 'NONE',  ( -21.55341960407619339, 5.719274019375674811, 103.5427570613523613 ) ) ;
#91456=CARTESIAN_POINT ( 'NONE',  ( 0.05219959533909260263, 19.03943276465977164, 84.99890960531436690 ) ) ;
#91457=CARTESIAN_POINT ( 'NONE',  ( 13.89961937509977652, -13.97604488694527269, 38.12390960531436690 ) ) ;
#91458=CARTESIAN_POINT ( 'NONE',  ( 5.153800228976335163, 19.02544592524342804, 94.79057627198103830 ) ) ;
#91459=CARTESIAN_POINT ( 'NONE',  ( -0.05219959533909027116, -19.03943276465977164, 72.49890960531435269 ) ) ;
#91460=CARTESIAN_POINT ( 'NONE',  ( -16.55341960407617563, 4.379528057220093196, 23.54275706135235424 ) ) ;
#91462=CARTESIAN_POINT ( 'NONE',  ( 17.48847506799950935, -5.747544572775296068, 88.32697437843289379 ) ) ;
#91463=CARTESIAN_POINT ( 'NONE',  ( -9.474510206698720793, -16.51473224551083518, 54.58442372801899722 ) ) ;
#91464=CARTESIAN_POINT ( 'NONE',  ( 5.049401038297881783, 19.05341960407617563, 22.29275706135233648 ) ) ;
#91465=CARTESIAN_POINT ( 'NONE',  ( 18.62759615963271287, -10.81492255796078972, 33.33224293864769550 ) ) ;
#91466=CARTESIAN_POINT ( 'NONE',  ( 8.314922557961029526, -14.29746914071037800, 100.4177570613523471 ) ) ;
#91468=CARTESIAN_POINT ( 'NONE',  ( -5.049401038297874678, -19.05341960407617918, 64.79275706135233293 ) ) ;
#91469=CARTESIAN_POINT ( 'NONE',  ( -0.05219959533936034679, 19.03943276465977164, 37.50109039468567573 ) ) ;
#91470=CARTESIAN_POINT ( 'NONE',  ( 17.12812012977026654, 6.668231424565999710, 108.8594875932314494 ) ) ;
#91471=CARTESIAN_POINT ( 'NONE',  ( -16.46253265017160317, 9.564922557960807481, 35.83224293864768839 ) ) ;
#91472=CARTESIAN_POINT ( 'NONE',  ( 16.52544592524342804, -4.483927247898539470, 38.54057627198103120 ) ) ;
#91473=CARTESIAN_POINT ( 'NONE',  ( -13.97604488694527625, -13.89961937509977652, 26.87390960531434558 ) ) ;
#91474=CARTESIAN_POINT ( 'NONE',  ( -14.34966873604960291, -8.224510206698953496, 26.66557627198103475 ) ) ;
#91476=CARTESIAN_POINT ( 'NONE',  ( -8.314922557961024197, 14.29746914071037800, 97.91775706135236135 ) ) ;
#91477=CARTESIAN_POINT ( 'NONE',  ( -0.05219959533909027116, -19.03943276465977164, 52.49890960531436690 ) ) ;
#91478=CARTESIAN_POINT ( 'NONE',  ( 21.52544592524334988, 5.823673210054432836, 111.4594237280190328 ) ) ;
#91479=CARTESIAN_POINT ( 'NONE',  ( 16.52544592524335698, 4.483927247898782831, 26.45942372801901854 ) ) ;
#91480=CARTESIAN_POINT ( 'NONE',  ( 5.823673210054444382, -21.52544592524334988, 80.20942372801901854 ) ) ;
#91482=CARTESIAN_POINT ( 'NONE',  ( 16.51473224551083163, -9.474510206698727899, 60.83442372801900433 ) ) ;
#91483=CARTESIAN_POINT ( 'NONE',  ( -16.46253265017160317, 9.564922557960807481, 85.83224293864769550 ) ) ;
#91484=CARTESIAN_POINT ( 'NONE',  ( -5.049401038298153566, 19.05341960407611168, 80.20724293864769550 ) ) ;
#91486=CARTESIAN_POINT ( 'NONE',  ( -21.52544592524343514, 5.823673210054127303, 111.0405762719810525 ) ) ;
#91487=CARTESIAN_POINT ( 'NONE',  ( -4.483927247898539470, -16.52544592524342804, 72.29057627198102409 ) ) ;
#91488=CARTESIAN_POINT ( 'NONE',  ( -21.52544592524343514, 5.823673210054127303, 66.04057627198103830 ) ) ;
#91489=CARTESIAN_POINT ( 'NONE',  ( -0.05219959533909027116, -19.03943276465977164, 62.49890960531435979 ) ) ;
#91490=CARTESIAN_POINT ( 'NONE',  ( -18.67979575497178146, -10.72451020669898902, 101.6655762719810383 ) ) ;
#91491=CARTESIAN_POINT ( 'NONE',  ( 16.52544592524335698, 4.483927247898782831, 91.45942372801901854 ) ) ;
#91492=VERTEX_POINT ( 'NONE', #68755 ) ;
#91493=CARTESIAN_POINT ( 'NONE',  ( -5.049401038298153566, 19.05341960407611168, 65.20724293864765286 ) ) ;
#91494=CARTESIAN_POINT ( 'NONE',  ( 16.53943276465976808, -0.05219959533910856209, 93.74890960531436690 ) ) ;
#91496=CARTESIAN_POINT ( 'NONE',  ( -19.03943276465977164, 0.05219959533909376836, 56.24890960531435979 ) ) ;
#91497=CARTESIAN_POINT ( 'NONE',  ( 13.97604488694548053, -13.89961937509957401, 85.62609039468568994 ) ) ;
#91498=CARTESIAN_POINT ( 'NONE',  ( 8.224510206698953496, -14.34966873604960469, 82.91557627198103830 ) ) ;
#91499=CARTESIAN_POINT ( 'NONE',  ( -21.55341960407619339, 5.719274019375674811, 58.54275706135235424 ) ) ;
#91500=CARTESIAN_POINT ( 'NONE',  ( -13.89961937509977652, 13.97604488694528158, 40.62390960531435979 ) ) ;
#91501=CARTESIAN_POINT ( 'NONE',  ( -15.80617190586745835, -15.72974639402198527, 106.8739096053143811 ) ) ;
#91502=CARTESIAN_POINT ( 'NONE',  ( 4.379528057220339221, -16.55341960407611168, 107.7072429386476955 ) ) ;
#91504=CARTESIAN_POINT ( 'NONE',  ( -19.02544592524342804, 5.153800228976336051, 61.04057627198103120 ) ) ;
#91506=CARTESIAN_POINT ( 'NONE',  ( -13.89961937509957401, -13.97604488694547875, 99.37609039468567573 ) ) ;
#91507=CARTESIAN_POINT ( 'NONE',  ( 16.46253265017160672, -9.564922557960803928, 108.3322429386476955 ) ) ;
#91508=CARTESIAN_POINT ( 'NONE',  ( 10.81492255796106328, -18.62759615963255655, 40.41775706135234714 ) ) ;
#91509=CARTESIAN_POINT ( 'NONE',  ( -19.05341960407611168, -5.049401038298163336, 81.45724293864769550 ) ) ;
#91510=CARTESIAN_POINT ( 'NONE',  ( 19.05341960407617918, -5.049401038297876454, 66.04275706135233293 ) ) ;
#91511=CARTESIAN_POINT ( 'NONE',  ( -19.03943276465977164, 0.05219959533909376836, 56.24890960531435979 ) ) ;
#91513=CARTESIAN_POINT ( 'NONE',  ( 4.379528057220339221, -16.55341960407611168, 82.70724293864770971 ) ) ;
#91514=CARTESIAN_POINT ( 'NONE',  ( 14.34966873604960469, 8.224510206698951720, 64.16557627198102409 ) ) ;
#91515=CARTESIAN_POINT ( 'NONE',  ( -16.46253265017160317, 9.564922557960807481, 95.83224293864769550 ) ) ;
#91516=CARTESIAN_POINT ( 'NONE',  ( 16.52544592524342804, -4.483927247898539470, 78.54057627198103830 ) ) ;
#91517=CARTESIAN_POINT ( 'NONE',  ( 13.97604488694527802, 13.89961937509977652, 84.37390960531433848 ) ) ;
#91518=CARTESIAN_POINT ( 'NONE',  ( -16.51473224551082808, 9.474510206698731452, 33.33442372801899722 ) ) ;
#91519=CARTESIAN_POINT ( 'NONE',  ( 9.564922557960805705, 16.46253265017160317, 49.58224293864770260 ) ) ;
#91520=CARTESIAN_POINT ( 'NONE',  ( 4.379528057220339221, -16.55341960407611168, 32.70724293864770260 ) ) ;
#91521=CARTESIAN_POINT ( 'NONE',  ( -12.06949235617756955, 12.14591786802309770, 105.6239096053143669 ) ) ;
#91523=CARTESIAN_POINT ( 'NONE',  ( -18.62759615963255300, -10.81492255796106328, 44.16775706135234714 ) ) ;
#91524=CARTESIAN_POINT ( 'NONE',  ( 16.46253265017146816, 9.564922557961045513, 61.66775706135234003 ) ) ;
#91525=CARTESIAN_POINT ( 'NONE',  ( -14.34966873604960291, -8.224510206698953496, 41.66557627198103120 ) ) ;
#91526=CARTESIAN_POINT ( 'NONE',  ( -21.53943276465977519, 0.05219959533907696930, 81.24890960531436690 ) ) ;
#91527=CARTESIAN_POINT ( 'NONE',  ( 13.97604488694527802, 13.89961937509977652, 114.3739096053143669 ) ) ;
#91528=CARTESIAN_POINT ( 'NONE',  ( 16.55341960407611168, 4.379528057220329451, 68.95724293864769550 ) ) ;
#91529=CARTESIAN_POINT ( 'NONE',  ( -0.05219959533909027116, -19.03943276465977164, 47.49890960531435979 ) ) ;
#91530=CARTESIAN_POINT ( 'NONE',  ( 16.46253265017146816, 9.564922557961045513, 26.66775706135234003 ) ) ;
#91531=CARTESIAN_POINT ( 'NONE',  ( -12.14591786802326823, 12.06949235617739902, 103.1260903946856757 ) ) ;
#91532=CARTESIAN_POINT ( 'NONE',  ( -12.06949235617739369, -12.14591786802326823, 54.37609039468568994 ) ) ;
#91533=CARTESIAN_POINT ( 'NONE',  ( -21.53943276465977519, 0.05219959533907696930, 41.24890960531435269 ) ) ;
#91534=CARTESIAN_POINT ( 'NONE',  ( 21.52544592524334988, 5.823673210054432836, 106.4594237280190328 ) ) ;
#91535=CARTESIAN_POINT ( 'NONE',  ( -9.474510206698964154, 16.51473224551069663, 85.41557627198102409 ) ) ;
#91536=CARTESIAN_POINT ( 'NONE',  ( -16.53943276465976808, -0.05219959533934237506, 68.75109039468568994 ) ) ;
#91537=CARTESIAN_POINT ( 'NONE',  ( -5.049401038298153566, 19.05341960407611168, 30.20724293864768839 ) ) ;
#91538=CARTESIAN_POINT ( 'NONE',  ( 4.483927247898545687, 16.52544592524342804, 39.79057627198103830 ) ) ;
#91539=CARTESIAN_POINT ( 'NONE',  ( 9.474510206698971260, -16.51473224551069308, 107.9155762719810383 ) ) ;
#91540=CARTESIAN_POINT ( 'NONE',  ( 9.474510206698971260, -16.51473224551069308, 92.91557627198103830 ) ) ;
#91541=CARTESIAN_POINT ( 'NONE',  ( -5.719274019375978568, 21.55341960407610458, 30.20724293864769550 ) ) ;
#91542=CARTESIAN_POINT ( 'NONE',  ( 12.14591786802309770, 12.06949235617756955, 54.37390960531435979 ) ) ;
#91543=CARTESIAN_POINT ( 'NONE',  ( 8.224510206698953496, -14.34966873604960469, 37.91557627198102409 ) ) ;
#91545=ORIENTED_EDGE ( 'NONE', *, *, #31222, .F. ) ;
#91546=CARTESIAN_POINT ( 'NONE',  ( -12.06949235617756955, 12.14591786802309770, 45.62390960531436690 ) ) ;
#91548=CARTESIAN_POINT ( 'NONE',  ( 8.314922557961029526, -14.29746914071037800, 40.41775706135234714 ) ) ;
#91549=CARTESIAN_POINT ( 'NONE',  ( 0.05219959533936267826, -19.03943276465977164, 60.00109039468566863 ) ) ;
#91550=CARTESIAN_POINT ( 'NONE',  ( -5.153800228976607833, 19.02544592524334988, 47.70942372801900433 ) ) ;
#91551=CARTESIAN_POINT ( 'NONE',  ( -13.89961937509977652, 13.97604488694528158, 90.62390960531432427 ) ) ;
#91552=CARTESIAN_POINT ( 'NONE',  ( 5.049401038297881783, 19.05341960407617563, 62.29275706135234003 ) ) ;
#91554=CARTESIAN_POINT ( 'NONE',  ( 19.02544592524334988, 5.153800228976608722, 56.45942372801898301 ) ) ;
#91555=CARTESIAN_POINT ( 'NONE',  ( -19.05341960407617563, 5.049401038297882671, 98.54275706135233293 ) ) ;
#91556=CARTESIAN_POINT ( 'NONE',  ( 8.224510206698742110, 14.34966873604972548, 77.08442372801901854 ) ) ;
#91558=CARTESIAN_POINT ( 'NONE',  ( -0.05219959533909027116, -19.03943276465977164, 22.49890960531436690 ) ) ;
#91559=CARTESIAN_POINT ( 'NONE',  ( -21.55341960407610458, -5.719274019375992779, 21.45724293864769550 ) ) ;
#91560=CARTESIAN_POINT ( 'NONE',  ( -21.52544592524334988, -5.823673210054445271, 38.95942372801901854 ) ) ;
#91561=CARTESIAN_POINT ( 'NONE',  ( -19.02544592524334988, -5.153800228976617603, 108.9594237280189759 ) ) ;
#91562=CARTESIAN_POINT ( 'NONE',  ( 17.50000000000147793, -3.202012800152252758, 107.4282241602726629 ) ) ;
#91563=CARTESIAN_POINT ( 'NONE',  ( 9.474510206698971260, -16.51473224551069308, 62.91557627198102409 ) ) ;
#91564=CARTESIAN_POINT ( 'NONE',  ( 16.46253265017160672, -9.564922557960803928, 103.3322429386476955 ) ) ;
#91565=CARTESIAN_POINT ( 'NONE',  ( 14.34966873604960469, 8.224510206698951720, 69.16557627198102409 ) ) ;
#91566=CARTESIAN_POINT ( 'NONE',  ( -19.02544592524342804, 5.153800228976336051, 66.04057627198103830 ) ) ;
#91567=CARTESIAN_POINT ( 'NONE',  ( 16.51473224551069308, 9.474510206698969483, 79.16557627198103830 ) ) ;
#91568=CARTESIAN_POINT ( 'NONE',  ( -16.51473224551082808, 9.474510206698731452, 78.33442372801900433 ) ) ;
#91569=CARTESIAN_POINT ( 'NONE',  ( -21.55341960407610458, -5.719274019375992779, 51.45724293864770260 ) ) ;
#91570=CARTESIAN_POINT ( 'NONE',  ( 8.224510206698953496, -14.34966873604960469, 112.9155762719810383 ) ) ;
#91571=CARTESIAN_POINT ( 'NONE',  ( 13.89961937509957401, 13.97604488694547697, 36.87609039468565442 ) ) ;
#91572=CARTESIAN_POINT ( 'NONE',  ( -9.474510206698964154, 16.51473224551069663, 85.41557627198102409 ) ) ;
#91573=CARTESIAN_POINT ( 'NONE',  ( 0.05219959533907565091, 21.53943276465977519, 74.99890960531435269 ) ) ;
#91574=CARTESIAN_POINT ( 'NONE',  ( -4.483927247898539470, -16.52544592524342804, 77.29057627198102409 ) ) ;
#91575=CARTESIAN_POINT ( 'NONE',  ( 9.564922557961047289, -16.46253265017146816, 45.41775706135232582 ) ) ;
#91576=CARTESIAN_POINT ( 'NONE',  ( 21.52544592524344225, -5.823673210054117533, 73.54057627198102409 ) ) ;
#91577=CARTESIAN_POINT ( 'NONE',  ( 10.72451020669898902, -18.67979575497178502, 62.91557627198102409 ) ) ;
#91578=CARTESIAN_POINT ( 'NONE',  ( 18.62759615963271287, -10.81492255796078972, 43.33224293864769550 ) ) ;
#91579=CARTESIAN_POINT ( 'NONE',  ( -10.72451020669870658, -18.67979575497194134, 89.58442372801901854 ) ) ;
#91580=CARTESIAN_POINT ( 'NONE',  ( 13.89961937509977652, -13.97604488694527269, 63.12390960531435979 ) ) ;
#91581=CARTESIAN_POINT ( 'NONE',  ( -5.153800228976328057, -19.02544592524343514, 22.29057627198102765 ) ) ;
#91582=CARTESIAN_POINT ( 'NONE',  ( 15.80617190586769283, -15.72974639402175789, 30.62609039468567929 ) ) ;
#91583=CARTESIAN_POINT ( 'NONE',  ( -18.67979575497193778, 10.72451020669871902, 43.33442372801901143 ) ) ;
#91584=CARTESIAN_POINT ( 'NONE',  ( -9.474510206698964154, 16.51473224551069663, 35.41557627198102409 ) ) ;
#91585=CARTESIAN_POINT ( 'NONE',  ( 0.05219959533907565091, 21.53943276465977519, 104.9989096053143669 ) ) ;
#91586=EDGE_CURVE ( 'NONE', #169038, #114713, #156262, .T. ) ;
#91587=CARTESIAN_POINT ( 'NONE',  ( 9.474510206698729675, 16.51473224551082808, 52.08442372801900433 ) ) ;
#91588=CARTESIAN_POINT ( 'NONE',  ( -9.564922557960796823, -16.46253265017161027, 32.08224293864769550 ) ) ;
#91590=CARTESIAN_POINT ( 'NONE',  ( 17.49999999999998934, -5.500000000000023981, 78.29690382534170112 ) ) ;
#91591=CARTESIAN_POINT ( 'NONE',  ( -16.55341960407617563, 4.379528057220093196, 63.54275706135234003 ) ) ;
#91592=CARTESIAN_POINT ( 'NONE',  ( -19.05341960407611168, -5.049401038298163336, 31.45724293864769550 ) ) ;
#91594=CARTESIAN_POINT ( 'NONE',  ( 13.89961937509977652, -13.97604488694527269, 83.12390960531436690 ) ) ;
#91595=CARTESIAN_POINT ( 'NONE',  ( 14.29746914071049879, -8.314922557960816363, 113.3322429386476955 ) ) ;
#91596=CARTESIAN_POINT ( 'NONE',  ( 21.52544592524344225, -5.823673210054117533, 53.54057627198103120 ) ) ;
#91597=CARTESIAN_POINT ( 'NONE',  ( 0.05219959533934541429, -16.53943276465976808, 50.00109039468568994 ) ) ;
#91598=CARTESIAN_POINT ( 'NONE',  ( 21.53943276465977519, 0.05219959533937863772, 101.2510903946856757 ) ) ;
#91599=CARTESIAN_POINT ( 'NONE',  ( 9.474510206698971260, -16.51473224551069308, 32.91557627198102409 ) ) ;
#91601=CARTESIAN_POINT ( 'NONE',  ( -8.224510206698735004, -14.34966873604973081, 104.5844237280190185 ) ) ;
#91602=CARTESIAN_POINT ( 'NONE',  ( -12.14591786802309592, -12.06949235617757132, 51.87390960531437401 ) ) ;
#91603=CARTESIAN_POINT ( 'NONE',  ( 9.474510206698971260, -16.51473224551069308, 57.91557627198103120 ) ) ;
#91604=CARTESIAN_POINT ( 'NONE',  ( -9.474510206698720793, -16.51473224551083518, 19.58442372801899722 ) ) ;
#91605=CARTESIAN_POINT ( 'NONE',  ( 18.67979575497194134, -10.72451020669871369, 25.83442372801901499 ) ) ;
#91607=CARTESIAN_POINT ( 'NONE',  ( 5.823673210054444382, -21.52544592524334988, 70.20942372801904696 ) ) ;
#91608=CARTESIAN_POINT ( 'NONE',  ( -12.14591786802326823, 12.06949235617739902, 58.12609039468568994 ) ) ;
#91609=CARTESIAN_POINT ( 'NONE',  ( 4.379528057220092307, 16.55341960407617563, 27.29275706135234358 ) ) ;
#91610=CARTESIAN_POINT ( 'NONE',  ( -12.14591786802309592, -12.06949235617757132, 76.87390960531439532 ) ) ;
#91611=CARTESIAN_POINT ( 'NONE',  ( 21.55341960407619695, -5.719274019375665929, 101.0427570613523756 ) ) ;
#91612=CARTESIAN_POINT ( 'NONE',  ( -14.34966873604960291, -8.224510206698953496, 36.66557627198103120 ) ) ;
#91613=CARTESIAN_POINT ( 'NONE',  ( -17.44270441346515810, 5.991230190323032723, 113.6366492073577490 ) ) ;
#91614=CARTESIAN_POINT ( 'NONE',  ( 8.224510206698742110, 14.34966873604972548, 37.08442372801901143 ) ) ;
#91615=CARTESIAN_POINT ( 'NONE',  ( -4.483927247898539470, -16.52544592524342804, 42.29057627198103120 ) ) ;
#91616=CARTESIAN_POINT ( 'NONE',  ( 16.55341960407618274, -4.379528057220086978, 91.04275706135236135 ) ) ;
#91617=CARTESIAN_POINT ( 'NONE',  ( 5.049401038298161559, -19.05341960407611168, 92.70724293864769550 ) ) ;
#91618=CARTESIAN_POINT ( 'NONE',  ( 5.823673210054125526, 21.52544592524343514, 24.79057627198103120 ) ) ;
#91619=CARTESIAN_POINT ( 'NONE',  ( 0.05219959533937995610, -21.53943276465977519, 100.0010903946857042 ) ) ;
#91620=CARTESIAN_POINT ( 'NONE',  ( -14.29746914071037622, -8.314922557961029526, 99.16775706135234714 ) ) ;
#91621=CARTESIAN_POINT ( 'NONE',  ( -14.29746914071049879, 8.314922557960819915, 75.83224293864769550 ) ) ;
#91622=CARTESIAN_POINT ( 'NONE',  ( -13.89961937509977652, 13.97604488694528158, 85.62390960531433848 ) ) ;
#91623=ORIENTED_EDGE ( 'NONE', *, *, #52789, .F. ) ;
#91624=CARTESIAN_POINT ( 'NONE',  ( -8.224510206698735004, -14.34966873604973081, 44.58442372801901854 ) ) ;
#91625=CARTESIAN_POINT ( 'NONE',  ( 13.89961937509977652, -13.97604488694527269, 38.12390960531436690 ) ) ;
#91626=CARTESIAN_POINT ( 'NONE',  ( -13.89961937509977652, 13.97604488694528158, 100.6239096053143669 ) ) ;
#91627=CARTESIAN_POINT ( 'NONE',  ( -16.55341960407617563, 4.379528057220093196, 33.54275706135234714 ) ) ;
#91629=CARTESIAN_POINT ( 'NONE',  ( -13.89961937509957401, -13.97604488694547875, 29.37609039468565797 ) ) ;
#91630=CARTESIAN_POINT ( 'NONE',  ( 16.55341960407618274, -4.379528057220086978, 106.0427570613523471 ) ) ;
#91631=CARTESIAN_POINT ( 'NONE',  ( 16.51473224551069308, 9.474510206698969483, 34.16557627198102409 ) ) ;
#91632=CARTESIAN_POINT ( 'NONE',  ( 16.53943276465976808, 0.05219959533934440121, 71.25109039468568994 ) ) ;
#91633=CARTESIAN_POINT ( 'NONE',  ( 19.02544592524334988, 5.153800228976608722, 81.45942372801897591 ) ) ;
#91634=CARTESIAN_POINT ( 'NONE',  ( 5.153800228976615827, -19.02544592524334988, 35.20942372801899722 ) ) ;
#91635=CARTESIAN_POINT ( 'NONE',  ( -19.05341960407611168, -5.049401038298163336, 61.45724293864769550 ) ) ;
#91636=CARTESIAN_POINT ( 'NONE',  ( -12.06949235617756955, 12.14591786802309770, 80.62390960531438111 ) ) ;
#91637=CARTESIAN_POINT ( 'NONE',  ( 0.05219959533936267826, -19.03943276465977164, 55.00109039468566863 ) ) ;
#91638=CARTESIAN_POINT ( 'NONE',  ( 18.62759615963271287, -10.81492255796078972, 68.33224293864769550 ) ) ;
#91639=CARTESIAN_POINT ( 'NONE',  ( -5.049401038297874678, -19.05341960407617918, 24.79275706135233648 ) ) ;
#91640=CARTESIAN_POINT ( 'NONE',  ( -13.97604488694527625, -13.89961937509977652, 101.8739096053143811 ) ) ;
#91641=CARTESIAN_POINT ( 'NONE',  ( -18.62759615963270932, 10.81492255796079327, 70.83224293864770971 ) ) ;
#91642=CARTESIAN_POINT ( 'NONE',  ( 19.02544592524343514, -5.153800228976328945, 108.5405762719810383 ) ) ;
#91643=CARTESIAN_POINT ( 'NONE',  ( 19.02544592524334988, 5.153800228976608722, 101.4594237280189759 ) ) ;
#91644=CARTESIAN_POINT ( 'NONE',  ( 19.02544592524343514, -5.153800228976328945, 113.5405762719810241 ) ) ;
#91645=CARTESIAN_POINT ( 'NONE',  ( 8.314922557961029526, -14.29746914071037800, 30.41775706135234358 ) ) ;
#91646=CARTESIAN_POINT ( 'NONE',  ( -13.97604488694527625, -13.89961937509977652, 36.87390960531436690 ) ) ;
#91647=CARTESIAN_POINT ( 'NONE',  ( -13.97604488694527625, -13.89961937509977652, 96.87390960531433848 ) ) ;
#91648=CARTESIAN_POINT ( 'NONE',  ( 21.52544592524344225, -5.823673210054117533, 78.54057627198103830 ) ) ;
#91649=CARTESIAN_POINT ( 'NONE',  ( 8.314922557961029526, -14.29746914071037800, 65.41775706135234714 ) ) ;
#91650=CARTESIAN_POINT ( 'NONE',  ( 10.72451020669871369, 18.67979575497193778, 62.08442372801901143 ) ) ;
#91651=CARTESIAN_POINT ( 'NONE',  ( 16.51473224551083163, -9.474510206698727899, 100.8344237280190043 ) ) ;
#91652=CARTESIAN_POINT ( 'NONE',  ( 16.51473224551083163, -9.474510206698727899, 20.83442372801899722 ) ) ;
#91653=CARTESIAN_POINT ( 'NONE',  ( -4.483927247898782831, 16.52544592524335698, 107.7094237280190328 ) ) ;
#91654=CARTESIAN_POINT ( 'NONE',  ( 5.719274019375991003, -21.55341960407610458, 102.7072429386476955 ) ) ;
#91655=CARTESIAN_POINT ( 'NONE',  ( -14.29746914071049879, 8.314922557960819915, 40.83224293864769550 ) ) ;
#91656=CARTESIAN_POINT ( 'NONE',  ( -5.153800228976607833, 19.02544592524334988, 77.70942372801900433 ) ) ;
#91657=CARTESIAN_POINT ( 'NONE',  ( -5.823673210054431948, 21.52544592524334988, 52.70942372801902565 ) ) ;
#91658=CARTESIAN_POINT ( 'NONE',  ( -5.049401038297874678, -19.05341960407617918, 44.79275706135232582 ) ) ;
#91659=CARTESIAN_POINT ( 'NONE',  ( 4.379528057220339221, -16.55341960407611168, 102.7072429386476955 ) ) ;
#91660=CARTESIAN_POINT ( 'NONE',  ( -10.81492255796078084, -18.62759615963271287, 27.08224293864769550 ) ) ;
#91661=CARTESIAN_POINT ( 'NONE',  ( -12.14591786802309592, -12.06949235617757132, 31.87390960531435979 ) ) ;
#91662=CARTESIAN_POINT ( 'NONE',  ( 5.719274019375673035, 21.55341960407619339, 102.2927570613523613 ) ) ;
#91663=CARTESIAN_POINT ( 'NONE',  ( -16.53943276465976808, -0.05219959533934237506, 73.75109039468567573 ) ) ;
#91664=CARTESIAN_POINT ( 'NONE',  ( 16.55341960407611168, 4.379528057220329451, 23.95724293864769550 ) ) ;
#91665=CARTESIAN_POINT ( 'NONE',  ( 21.52544592524334988, 5.823673210054432836, 61.45942372801901854 ) ) ;
#91666=CARTESIAN_POINT ( 'NONE',  ( 10.81492255796106328, -18.62759615963255655, 60.41775706135235424 ) ) ;
#91667=CARTESIAN_POINT ( 'NONE',  ( -9.564922557960796823, -16.46253265017161027, 27.08224293864769550 ) ) ;
#91668=CARTESIAN_POINT ( 'NONE',  ( -15.72974639402176322, -15.80617190586768395, 39.37609039468567573 ) ) ;
#91669=CARTESIAN_POINT ( 'NONE',  ( -0.05219959533910754901, -16.53943276465976808, 112.4989096053143669 ) ) ;
#91670=CARTESIAN_POINT ( 'NONE',  ( 0.05219959533909260263, 19.03943276465977164, 44.99890960531435979 ) ) ;
#91671=CARTESIAN_POINT ( 'NONE',  ( -16.53943276465976808, 0.05219959533911058130, 76.24890960531435269 ) ) ;
#91672=CARTESIAN_POINT ( 'NONE',  ( 19.02544592524343514, -5.153800228976328945, 73.54057627198103830 ) ) ;
#91673=CARTESIAN_POINT ( 'NONE',  ( -8.224510206698948167, 14.34966873604960824, 30.41557627198101699 ) ) ;
#91674=CARTESIAN_POINT ( 'NONE',  ( -21.52544592524343514, 5.823673210054127303, 61.04057627198103120 ) ) ;
#91675=CARTESIAN_POINT ( 'NONE',  ( 8.224510206698953496, -14.34966873604960469, 97.91557627198103830 ) ) ;
#91676=CARTESIAN_POINT ( 'NONE',  ( 15.80617190586746368, 15.72974639402197994, 104.3739096053143669 ) ) ;
#91677=CARTESIAN_POINT ( 'NONE',  ( -13.89961937509977652, 13.97604488694528158, 105.6239096053143527 ) ) ;
#91678=CARTESIAN_POINT ( 'NONE',  ( -9.564922557960796823, -16.46253265017161027, 62.08224293864769550 ) ) ;
#91679=CARTESIAN_POINT ( 'NONE',  ( 19.02544592524334988, 5.153800228976608722, 111.4594237280190043 ) ) ;
#91680=CARTESIAN_POINT ( 'NONE',  ( -5.823673210054116645, -21.52544592524344225, 52.29057627198102409 ) ) ;
#91681=CARTESIAN_POINT ( 'NONE',  ( -15.72974639402176322, -15.80617190586768395, 79.37609039468567573 ) ) ;
#91682=CARTESIAN_POINT ( 'NONE',  ( -5.153800228976328057, -19.02544592524343514, 67.29057627198102409 ) ) ;
#91685=CARTESIAN_POINT ( 'NONE',  ( 5.153800228976335163, 19.02544592524342804, 94.79057627198103830 ) ) ;
#91686=CARTESIAN_POINT ( 'NONE',  ( 16.55341960407618274, -4.379528057220086978, 76.04275706135237556 ) ) ;
#91687=CARTESIAN_POINT ( 'NONE',  ( -21.55341960407619339, 5.719274019375674811, 63.54275706135234003 ) ) ;
#91688=CARTESIAN_POINT ( 'NONE',  ( -21.53943276465977519, -0.05219959533937600094, 83.75109039468568994 ) ) ;
#91689=CARTESIAN_POINT ( 'NONE',  ( 18.62759615963271287, -10.81492255796078972, 108.3322429386477097 ) ) ;
#91690=CARTESIAN_POINT ( 'NONE',  ( -14.34966873604972548, 8.224510206698743886, 78.33442372801901854 ) ) ;
#91691=CARTESIAN_POINT ( 'NONE',  ( -15.72974639402197994, 15.80617190586746368, 80.62390960531438111 ) ) ;
#91692=CARTESIAN_POINT ( 'NONE',  ( 16.46253265017146816, 9.564922557961045513, 46.66775706135233293 ) ) ;
#91693=CARTESIAN_POINT ( 'NONE',  ( -21.53943276465977519, 0.05219959533907696930, 46.24890960531435979 ) ) ;
#91694=CARTESIAN_POINT ( 'NONE',  ( -5.153800228976328057, -19.02544592524343514, 77.29057627198099567 ) ) ;
#91695=CARTESIAN_POINT ( 'NONE',  ( -16.55341960407611168, -4.379528057220339221, 26.45724293864768839 ) ) ;
#91697=CARTESIAN_POINT ( 'NONE',  ( 21.53943276465977519, -0.05219959533907433946, 23.74890960531435269 ) ) ;
#91699=CARTESIAN_POINT ( 'NONE',  ( 19.02544592524334988, 5.153800228976608722, 96.45942372801897591 ) ) ;
#91700=CARTESIAN_POINT ( 'NONE',  ( -15.72974639402197994, 15.80617190586746368, 70.62390960531436690 ) ) ;
#91701=CARTESIAN_POINT ( 'NONE',  ( -16.53943276465976808, 0.05219959533911058130, 51.24890960531436690 ) ) ;
#91702=CARTESIAN_POINT ( 'NONE',  ( 19.02544592524334988, 5.153800228976608722, 106.4594237280190185 ) ) ;
#91703=CARTESIAN_POINT ( 'NONE',  ( -13.89961937509977652, 13.97604488694528158, 50.62390960531435979 ) ) ;
#91704=CARTESIAN_POINT ( 'NONE',  ( -0.05219959533907301413, -21.53943276465977519, 102.4989096053143811 ) ) ;
#91705=CARTESIAN_POINT ( 'NONE',  ( 19.03943276465977164, 0.05219959533936151252, 76.25109039468566152 ) ) ;
#91706=CARTESIAN_POINT ( 'NONE',  ( -5.153800228976328057, -19.02544592524343514, 82.29057627198103830 ) ) ;
#91707=CARTESIAN_POINT ( 'NONE',  ( -0.05219959533910754901, -16.53943276465976808, 92.49890960531436690 ) ) ;
#91708=CARTESIAN_POINT ( 'NONE',  ( -16.46253265017160317, 9.564922557960807481, 60.83224293864769550 ) ) ;
#91709=CARTESIAN_POINT ( 'NONE',  ( -16.52544592524342804, 4.483927247898546575, 61.04057627198103120 ) ) ;
#91710=CARTESIAN_POINT ( 'NONE',  ( -9.474510206698964154, 16.51473224551069663, 35.41557627198102409 ) ) ;
#91712=CARTESIAN_POINT ( 'NONE',  ( -8.224510206698948167, 14.34966873604960824, 45.41557627198103830 ) ) ;
#91713=CARTESIAN_POINT ( 'NONE',  ( -0.05219959533909027116, -19.03943276465977164, 92.49890960531436690 ) ) ;
#91715=CARTESIAN_POINT ( 'NONE',  ( 19.02544592524334988, 5.153800228976608722, 51.45942372801900433 ) ) ;
#91716=CARTESIAN_POINT ( 'NONE',  ( 4.379528057220092307, 16.55341960407617563, 62.29275706135236845 ) ) ;
#91717=CARTESIAN_POINT ( 'NONE',  ( -18.62759615963270932, 10.81492255796079327, 60.83224293864769550 ) ) ;
#91718=CARTESIAN_POINT ( 'NONE',  ( -5.153800228976607833, 19.02544592524334988, 37.70942372801899722 ) ) ;
#91719=CARTESIAN_POINT ( 'NONE',  ( 19.03943276465977164, -0.05219959533909143690, 83.74890960531436690 ) ) ;
#91721=CARTESIAN_POINT ( 'NONE',  ( 15.80617190586746368, 15.72974639402197994, 34.37390960531435979 ) ) ;
#91722=CARTESIAN_POINT ( 'NONE',  ( -13.97604488694527625, -13.89961937509977652, 61.87390960531435979 ) ) ;
#91723=CARTESIAN_POINT ( 'NONE',  ( 15.80617190586769283, -15.72974639402175789, 45.62609039468567573 ) ) ;
#91724=CARTESIAN_POINT ( 'NONE',  ( 5.153800228976335163, 19.02544592524342804, 29.79057627198102409 ) ) ;
#91725=CARTESIAN_POINT ( 'NONE',  ( 5.719274019375991003, -21.55341960407610458, 102.7072429386476955 ) ) ;
#91726=CARTESIAN_POINT ( 'NONE',  ( -9.474510206698964154, 16.51473224551069663, 100.4155762719810241 ) ) ;
#91728=CARTESIAN_POINT ( 'NONE',  ( -15.80617190586768217, 15.72974639402176855, 38.12609039468567573 ) ) ;
#91730=CARTESIAN_POINT ( 'NONE',  ( -16.46253265017160317, 9.564922557960807481, 100.8322429386477097 ) ) ;
#91732=CARTESIAN_POINT ( 'NONE',  ( -21.53943276465977519, 0.05219959533907696930, 106.2489096053143811 ) ) ;
#91733=CARTESIAN_POINT ( 'NONE',  ( -19.03943276465977164, 0.05219959533909376836, 41.24890960531435269 ) ) ;
#91734=CARTESIAN_POINT ( 'NONE',  ( -12.06949235617739369, -12.14591786802326823, 24.37609039468567573 ) ) ;
#91737=CARTESIAN_POINT ( 'NONE',  ( -19.02544592524342804, 5.153800228976336051, 26.04057627198103120 ) ) ;
#91738=CARTESIAN_POINT ( 'NONE',  ( 21.52544592524334988, 5.823673210054432836, 96.45942372801901854 ) ) ;
#91739=CARTESIAN_POINT ( 'NONE',  ( -19.02544592524342804, 5.153800228976336051, 76.04057627198102409 ) ) ;
#91740=CARTESIAN_POINT ( 'NONE',  ( 21.53943276465977519, 0.05219959533937863772, 51.25109039468568994 ) ) ;
#91742=CARTESIAN_POINT ( 'NONE',  ( -13.89961937509977652, 13.97604488694528158, 105.6239096053143527 ) ) ;
#91743=CARTESIAN_POINT ( 'NONE',  ( 19.20446147854529073, 5.499999999999903189, 61.88999695167678539 ) ) ;
#91744=CARTESIAN_POINT ( 'NONE',  ( -16.52544592524335698, -4.483927247898792601, 38.95942372801901854 ) ) ;
#91745=CARTESIAN_POINT ( 'NONE',  ( -8.224510206698735004, -14.34966873604973081, 74.58442372801901854 ) ) ;
#91746=CARTESIAN_POINT ( 'NONE',  ( 21.53943276465977519, 0.05219959533937863772, 56.25109039468568284 ) ) ;
#91747=CARTESIAN_POINT ( 'NONE',  ( 15.80617190586769283, -15.72974639402175789, 95.62609039468568994 ) ) ;
#91749=CARTESIAN_POINT ( 'NONE',  ( -9.474510206698720793, -16.51473224551083518, 104.5844237280190043 ) ) ;
#91750=CARTESIAN_POINT ( 'NONE',  ( -13.97604488694527625, -13.89961937509977652, 71.87390960531433848 ) ) ;
#91751=CARTESIAN_POINT ( 'NONE',  ( 5.049401038298161559, -19.05341960407611168, 102.7072429386476955 ) ) ;
#91753=CARTESIAN_POINT ( 'NONE',  ( 8.314922557960818139, 14.29746914071049879, 109.5822429386476955 ) ) ;
#91754=CARTESIAN_POINT ( 'NONE',  ( 21.53943276465977519, -0.05219959533907433946, 28.74890960531435624 ) ) ;
#91755=CARTESIAN_POINT ( 'NONE',  ( 4.379528057220092307, 16.55341960407617563, 97.29275706135234714 ) ) ;
#91756=CARTESIAN_POINT ( 'NONE',  ( -8.224510206698948167, 14.34966873604960824, 75.41557627198102409 ) ) ;
#91757=CARTESIAN_POINT ( 'NONE',  ( 9.474510206698971260, -16.51473224551069308, 52.91557627198102409 ) ) ;
#91758=CARTESIAN_POINT ( 'NONE',  ( 0.05219959533937995610, -21.53943276465977519, 75.00109039468568994 ) ) ;
#91760=CARTESIAN_POINT ( 'NONE',  ( 19.02544592524334988, 5.153800228976608722, 101.4594237280189759 ) ) ;
#91761=CARTESIAN_POINT ( 'NONE',  ( 14.29746914071049879, -8.314922557960816363, 78.33224293864770971 ) ) ;
#91762=CARTESIAN_POINT ( 'NONE',  ( -5.719274019375665041, -21.55341960407619695, 29.79275706135234358 ) ) ;
#91763=CARTESIAN_POINT ( 'NONE',  ( -18.67979575497178146, -10.72451020669898902, 56.66557627198103830 ) ) ;
#91764=CARTESIAN_POINT ( 'NONE',  ( -16.18388926212238843, -7.379444403734516378, 105.4395315136615636 ) ) ;
#91766=CARTESIAN_POINT ( 'NONE',  ( 0.05219959533909260263, 19.03943276465977164, 79.99890960531436690 ) ) ;
#91767=CARTESIAN_POINT ( 'NONE',  ( 0.05219959533910956823, 16.53943276465976808, 49.99890960531437401 ) ) ;
#91769=CARTESIAN_POINT ( 'NONE',  ( -14.29746914071049879, 8.314922557960819915, 35.83224293864768839 ) ) ;
#91770=CARTESIAN_POINT ( 'NONE',  ( 14.34966873604972726, -8.224510206698740333, 95.83442372801903275 ) ) ;
#91771=CARTESIAN_POINT ( 'NONE',  ( 5.049401038297881783, 19.05341960407617563, 47.29275706135231161 ) ) ;
#91773=CARTESIAN_POINT ( 'NONE',  ( 19.03943276465977164, -0.05219959533909143690, 98.74890960531436690 ) ) ;
#91774=EDGE_CURVE ( 'NONE', #53443, #176653, #170814, .T. ) ;
#91775=CARTESIAN_POINT ( 'NONE',  ( 14.29746914071049879, -8.314922557960816363, 68.33224293864769550 ) ) ;
#91776=CARTESIAN_POINT ( 'NONE',  ( -9.474510206698720793, -16.51473224551083518, 39.58442372801899722 ) ) ;
#91777=CARTESIAN_POINT ( 'NONE',  ( 19.05341960407611168, 5.049401038298154454, 38.95724293864767418 ) ) ;
#91778=CARTESIAN_POINT ( 'NONE',  ( 18.67979575497178502, 10.72451020669898547, 39.16557627198102409 ) ) ;
#91779=CARTESIAN_POINT ( 'NONE',  ( -18.67979575497178146, -10.72451020669898902, 61.66557627198103120 ) ) ;
#91780=CARTESIAN_POINT ( 'NONE',  ( -4.483927247898539470, -16.52544592524342804, 97.29057627198105251 ) ) ;
#91781=CARTESIAN_POINT ( 'NONE',  ( 0.05219959533934541429, -16.53943276465976808, 50.00109039468568994 ) ) ;
#91782=CARTESIAN_POINT ( 'NONE',  ( 10.72451020669871369, 18.67979575497193778, 42.08442372801901854 ) ) ;
#91783=CARTESIAN_POINT ( 'NONE',  ( 16.53943276465976808, -0.05219959533910856209, 98.74890960531438111 ) ) ;
#91785=CARTESIAN_POINT ( 'NONE',  ( -16.29526858892872099, 7.335722546920265152, 49.20329402199791247 ) ) ;
#91786=CARTESIAN_POINT ( 'NONE',  ( 15.80617190586746368, 15.72974639402197994, 34.37390960531435979 ) ) ;
#91789=CARTESIAN_POINT ( 'NONE',  ( -8.224510206698735004, -14.34966873604973081, 44.58442372801901854 ) ) ;
#91790=CARTESIAN_POINT ( 'NONE',  ( -4.483927247898539470, -16.52544592524342804, 32.29057627198102409 ) ) ;
#91791=CARTESIAN_POINT ( 'NONE',  ( -10.72451020669898014, 18.67979575497178502, 65.41557627198102409 ) ) ;
#91792=CARTESIAN_POINT ( 'NONE',  ( -16.46253265017146816, -9.564922557961047289, 84.16775706135233293 ) ) ;
#91793=CARTESIAN_POINT ( 'NONE',  ( 15.80617190586746368, 15.72974639402197994, 64.37390960531435269 ) ) ;
#91795=CARTESIAN_POINT ( 'NONE',  ( -12.06949235617739369, -12.14591786802326823, 54.37609039468568994 ) ) ;
#91796=CARTESIAN_POINT ( 'NONE',  ( 5.153800228976335163, 19.02544592524342804, 34.79057627198102409 ) ) ;
#91797=CARTESIAN_POINT ( 'NONE',  ( -16.46253265017160317, 9.564922557960807481, 95.83224293864769550 ) ) ;
#91798=CARTESIAN_POINT ( 'NONE',  ( 0.05219959533909260263, 19.03943276465977164, 39.99890960531436690 ) ) ;
#91799=CARTESIAN_POINT ( 'NONE',  ( -13.97604488694527625, -13.89961937509977652, 21.87390960531435979 ) ) ;
#91801=CARTESIAN_POINT ( 'NONE',  ( 19.03943276465977164, -0.05219959533909143690, 108.7489096053143527 ) ) ;
#91804=CARTESIAN_POINT ( 'NONE',  ( 14.34966873604972726, -8.224510206698740333, 75.83442372801900433 ) ) ;
#91805=CARTESIAN_POINT ( 'NONE',  ( 10.81492255796078972, 18.62759615963270932, 89.58224293864768129 ) ) ;
#91806=CARTESIAN_POINT ( 'NONE',  ( 9.474510206698971260, -16.51473224551069308, 57.91557627198103120 ) ) ;
#91807=CARTESIAN_POINT ( 'NONE',  ( -18.67979575497193778, 10.72451020669871902, 23.33442372801901499 ) ) ;
#91808=CARTESIAN_POINT ( 'NONE',  ( 16.46253265017160672, -9.564922557960803928, 83.33224293864768129 ) ) ;
#91809=CARTESIAN_POINT ( 'NONE',  ( 19.05341960407611168, 5.049401038298154454, 113.9572429386477097 ) ) ;
#91811=CARTESIAN_POINT ( 'NONE',  ( -21.55341960407619339, 5.719274019375674811, 23.54275706135235424 ) ) ;
#91812=CARTESIAN_POINT ( 'NONE',  ( 16.51473224551069308, 9.474510206698969483, 29.16557627198103475 ) ) ;
#91813=CARTESIAN_POINT ( 'NONE',  ( 9.474510206698971260, -16.51473224551069308, 107.9155762719810383 ) ) ;
#91814=CARTESIAN_POINT ( 'NONE',  ( 5.049401038297881783, 19.05341960407617563, 92.29275706135234714 ) ) ;
#91815=CARTESIAN_POINT ( 'NONE',  ( -13.89961937509957401, -13.97604488694547875, 29.37609039468565797 ) ) ;
#91816=CARTESIAN_POINT ( 'NONE',  ( 21.53943276465977519, -0.05219959533907433946, 93.74890960531436690 ) ) ;
#91817=CARTESIAN_POINT ( 'NONE',  ( -5.049401038297874678, -19.05341960407617918, 29.79275706135232227 ) ) ;
#91818=CARTESIAN_POINT ( 'NONE',  ( -14.29746914071037622, -8.314922557961029526, 84.16775706135234714 ) ) ;
#91819=CARTESIAN_POINT ( 'NONE',  ( -9.474510206698964154, 16.51473224551069663, 100.4155762719810241 ) ) ;
#91820=CARTESIAN_POINT ( 'NONE',  ( 5.153800228976335163, 19.02544592524342804, 54.79057627198103120 ) ) ;
#91821=CARTESIAN_POINT ( 'NONE',  ( 21.52544592524334988, 5.823673210054432836, 71.45942372801901854 ) ) ;
#91822=CARTESIAN_POINT ( 'NONE',  ( -15.72974639402176322, -15.80617190586768395, 84.37609039468570415 ) ) ;
#91823=CARTESIAN_POINT ( 'NONE',  ( -19.03943276465977164, 0.05219959533909376836, 116.2489096053143669 ) ) ;
#91824=CARTESIAN_POINT ( 'NONE',  ( 16.46253265017160672, -9.564922557960803928, 73.33224293864769550 ) ) ;
#91825=CARTESIAN_POINT ( 'NONE',  ( -5.823673210054431948, 21.52544592524334988, 52.70942372801902565 ) ) ;
#91826=CARTESIAN_POINT ( 'NONE',  ( 19.03943276465977164, 0.05219959533936151252, 81.25109039468567573 ) ) ;
#91827=CARTESIAN_POINT ( 'NONE',  ( -9.564922557960796823, -16.46253265017161027, 57.08224293864769550 ) ) ;
#91828=CARTESIAN_POINT ( 'NONE',  ( 16.46253265017160672, -9.564922557960803928, 93.33224293864769550 ) ) ;
#91829=CARTESIAN_POINT ( 'NONE',  ( 16.51473224551069308, 9.474510206698969483, 79.16557627198103830 ) ) ;
#91830=CARTESIAN_POINT ( 'NONE',  ( 17.50000000000003553, -4.509153483536745277, 23.09479828858030359 ) ) ;
#91831=CARTESIAN_POINT ( 'NONE',  ( -19.03943276465977164, 0.05219959533909376836, 51.24890960531436690 ) ) ;
#91832=CARTESIAN_POINT ( 'NONE',  ( 10.81492255796078972, 18.62759615963270932, 104.5822429386477097 ) ) ;
#91833=CARTESIAN_POINT ( 'NONE',  ( 4.379528057220092307, 16.55341960407617563, 87.29275706135236135 ) ) ;
#91834=DIRECTION ( 'NONE',  ( 0.000000000000000000, -3.469446951953611033E-15, 1.000000000000000000 ) ) ;
#91835=CARTESIAN_POINT ( 'NONE',  ( 5.049401038297881783, 19.05341960407617563, 42.29275706135234003 ) ) ;
#91836=CARTESIAN_POINT ( 'NONE',  ( 5.153800228976335163, 19.02544592524342804, 79.79057627198102409 ) ) ;
#91837=CARTESIAN_POINT ( 'NONE',  ( -16.55341960407611168, -4.379528057220339221, 56.45724293864768839 ) ) ;
#91838=CARTESIAN_POINT ( 'NONE',  ( 14.34966873604960469, 8.224510206698951720, 94.16557627198103830 ) ) ;
#91839=CARTESIAN_POINT ( 'NONE',  ( 13.89961937509977652, -13.97604488694527269, 113.1239096053143527 ) ) ;
#91840=CARTESIAN_POINT ( 'NONE',  ( -19.02544592524342804, 5.153800228976336051, 106.0405762719810241 ) ) ;
#91841=CARTESIAN_POINT ( 'NONE',  ( 19.03943276465977164, -0.05219959533909143690, 113.7489096053143669 ) ) ;
#91842=CARTESIAN_POINT ( 'NONE',  ( -13.89961937509957401, -13.97604488694547875, 19.37609039468566507 ) ) ;
#91843=CARTESIAN_POINT ( 'NONE',  ( 8.314922557961029526, -14.29746914071037800, 90.41775706135236135 ) ) ;
#91844=CARTESIAN_POINT ( 'NONE',  ( -5.049401038298153566, 19.05341960407611168, 75.20724293864769550 ) ) ;
#91845=CARTESIAN_POINT ( 'NONE',  ( 21.52544592524334988, 5.823673210054432836, 36.45942372801901143 ) ) ;
#91846=CARTESIAN_POINT ( 'NONE',  ( -21.53943276465977519, 0.05219959533907696930, 31.24890960531435979 ) ) ;
#91847=CARTESIAN_POINT ( 'NONE',  ( -5.823673210054116645, -21.52544592524344225, 112.2905762719810241 ) ) ;
#91848=VERTEX_POINT ( 'NONE', #86928 ) ;
#91849=CARTESIAN_POINT ( 'NONE',  ( -18.62759615963270932, 10.81492255796079327, 65.83224293864769550 ) ) ;
#91850=CARTESIAN_POINT ( 'NONE',  ( -0.05219959533910754901, -16.53943276465976808, 92.49890960531436690 ) ) ;
#91851=CARTESIAN_POINT ( 'NONE',  ( 16.51473224551083163, -9.474510206698727899, 45.83442372801900433 ) ) ;
#91853=CARTESIAN_POINT ( 'NONE',  ( -5.153800228976328057, -19.02544592524343514, 37.29057627198102409 ) ) ;
#91854=CARTESIAN_POINT ( 'NONE',  ( 5.153800228976335163, 19.02544592524342804, 84.79057627198099567 ) ) ;
#91855=CARTESIAN_POINT ( 'NONE',  ( 19.03943276465977164, -0.05219959533909143690, 78.74890960531436690 ) ) ;
#91857=CARTESIAN_POINT ( 'NONE',  ( -16.53943276465976808, 0.05219959533911058130, 101.2489096053143669 ) ) ;
#91858=CARTESIAN_POINT ( 'NONE',  ( -16.52544592524342804, 4.483927247898546575, 31.04057627198102409 ) ) ;
#91859=CARTESIAN_POINT ( 'NONE',  ( 14.34966873604972726, -8.224510206698740333, 20.83442372801901143 ) ) ;
#91860=CARTESIAN_POINT ( 'NONE',  ( -5.823673210054431948, 21.52544592524334988, 87.70942372801901854 ) ) ;
#91861=CARTESIAN_POINT ( 'NONE',  ( 16.51473224551069308, 9.474510206698969483, 104.1655762719810241 ) ) ;
#91862=CARTESIAN_POINT ( 'NONE',  ( 15.80617190586746368, 15.72974639402197994, 114.3739096053143527 ) ) ;
#91863=CARTESIAN_POINT ( 'NONE',  ( -13.89961937509977652, 13.97604488694528158, 40.62390960531435979 ) ) ;
#91864=CARTESIAN_POINT ( 'NONE',  ( 16.52544592524335698, 4.483927247898782831, 46.45942372801901854 ) ) ;
#91866=CARTESIAN_POINT ( 'NONE',  ( 9.474510206698729675, 16.51473224551082808, 107.0844237280190043 ) ) ;
#91867=CARTESIAN_POINT ( 'NONE',  ( -5.823673210054116645, -21.52544592524344225, 102.2905762719810383 ) ) ;
#91868=CARTESIAN_POINT ( 'NONE',  ( 19.02544592524334988, 5.153800228976608722, 61.45942372801900433 ) ) ;
#91869=CARTESIAN_POINT ( 'NONE',  ( 5.153800228976335163, 19.02544592524342804, 24.79057627198102765 ) ) ;
#91870=CARTESIAN_POINT ( 'NONE',  ( -21.53943276465977519, 0.05219959533907696930, 111.2489096053143669 ) ) ;
#91872=CARTESIAN_POINT ( 'NONE',  ( -9.564922557960796823, -16.46253265017161027, 97.08224293864769550 ) ) ;
#91875=CARTESIAN_POINT ( 'NONE',  ( -19.05341960407611168, -5.049401038298163336, 86.45724293864769550 ) ) ;
#91876=CARTESIAN_POINT ( 'NONE',  ( 18.62759615963255655, 10.81492255796105972, 31.66775706135234358 ) ) ;
#91877=CARTESIAN_POINT ( 'NONE',  ( 4.483927247898545687, 16.52544592524342804, 74.79057627198105251 ) ) ;
#91878=CARTESIAN_POINT ( 'NONE',  ( 19.03943276465977164, -0.05219959533909143690, 83.74890960531436690 ) ) ;
#91880=CARTESIAN_POINT ( 'NONE',  ( 8.224510206698742110, 14.34966873604972548, 47.08442372801901854 ) ) ;
#91881=CARTESIAN_POINT ( 'NONE',  ( 13.89961937509957401, 13.97604488694547697, 56.87609039468564731 ) ) ;
#91882=CARTESIAN_POINT ( 'NONE',  ( -10.72451020669870658, -18.67979575497194134, 64.58442372801900433 ) ) ;
#91883=CARTESIAN_POINT ( 'NONE',  ( -16.55341960407617563, 4.379528057220093196, 23.54275706135235424 ) ) ;
#91884=CARTESIAN_POINT ( 'NONE',  ( -9.474510206698964154, 16.51473224551069663, 70.41557627198102409 ) ) ;
#91885=CARTESIAN_POINT ( 'NONE',  ( 13.89961937509957401, 13.97604488694547697, 91.87609039468567573 ) ) ;
#91886=CARTESIAN_POINT ( 'NONE',  ( -0.05219959533934338120, 16.53943276465976808, 52.50109039468567573 ) ) ;
#91887=CARTESIAN_POINT ( 'NONE',  ( -10.72451020669870658, -18.67979575497194134, 94.58442372801901854 ) ) ;
#91888=CARTESIAN_POINT ( 'NONE',  ( 19.05341960407617918, -5.049401038297876454, 81.04275706135231871 ) ) ;
#91889=CARTESIAN_POINT ( 'NONE',  ( 16.51473224551069308, 9.474510206698969483, 44.16557627198103120 ) ) ;
#91890=CARTESIAN_POINT ( 'NONE',  ( -5.823673210054116645, -21.52544592524344225, 77.29057627198102409 ) ) ;
#91891=CARTESIAN_POINT ( 'NONE',  ( -12.14591786802309592, -12.06949235617757132, 81.87390960531435269 ) ) ;
#91892=CARTESIAN_POINT ( 'NONE',  ( -5.153800228976607833, 19.02544592524334988, 82.70942372801897591 ) ) ;
#91893=CARTESIAN_POINT ( 'NONE',  ( -18.39639308325438449, -5.499999999999988454, 71.48252246182195790 ) ) ;
#91894=CARTESIAN_POINT ( 'NONE',  ( -16.46253265017146816, -9.564922557961047289, 39.16775706135234003 ) ) ;
#91895=CARTESIAN_POINT ( 'NONE',  ( -14.29746914071037622, -8.314922557961029526, 109.1677570613523613 ) ) ;
#91896=CARTESIAN_POINT ( 'NONE',  ( -12.06949235617756955, 12.14591786802309770, 60.62390960531437401 ) ) ;
#91897=CARTESIAN_POINT ( 'NONE',  ( 21.55341960407619695, -5.719274019375665929, 101.0427570613523756 ) ) ;
#91899=CARTESIAN_POINT ( 'NONE',  ( 5.719274019375991003, -21.55341960407610458, 112.7072429386476955 ) ) ;
#91900=CARTESIAN_POINT ( 'NONE',  ( 13.97604488694527802, 13.89961937509977652, 69.37390960531436690 ) ) ;
#91901=CARTESIAN_POINT ( 'NONE',  ( 15.80617190586769283, -15.72974639402175789, 85.62609039468568994 ) ) ;
#91902=CARTESIAN_POINT ( 'NONE',  ( 19.05341960407611168, 5.049401038298154454, 63.95724293864769550 ) ) ;
#91904=CARTESIAN_POINT ( 'NONE',  ( -8.224510206698948167, 14.34966873604960824, 115.4155762719810241 ) ) ;
#91905=CARTESIAN_POINT ( 'NONE',  ( -21.52544592524343514, 5.823673210054127303, 36.04057627198102409 ) ) ;
#91906=CARTESIAN_POINT ( 'NONE',  ( -16.52544592524342804, 4.483927247898546575, 61.04057627198103120 ) ) ;
#91907=CARTESIAN_POINT ( 'NONE',  ( -5.049401038298153566, 19.05341960407611168, 40.20724293864768839 ) ) ;
#91908=CARTESIAN_POINT ( 'NONE',  ( -4.379528057220328563, 16.55341960407611168, 90.20724293864770971 ) ) ;
#91910=CARTESIAN_POINT ( 'NONE',  ( 10.72451020669898902, -18.67979575497178502, 112.9155762719810383 ) ) ;
#91911=CARTESIAN_POINT ( 'NONE',  ( 18.62759615963255655, 10.81492255796105972, 51.66775706135234714 ) ) ;
#91913=CARTESIAN_POINT ( 'NONE',  ( 8.314922557961029526, -14.29746914071037800, 45.41775706135234003 ) ) ;
#91914=CARTESIAN_POINT ( 'NONE',  ( -18.62759615963270932, 10.81492255796079327, 95.83224293864770971 ) ) ;
#91915=CARTESIAN_POINT ( 'NONE',  ( -13.89961937509957401, -13.97604488694547875, 24.37609039468565442 ) ) ;
#91916=CARTESIAN_POINT ( 'NONE',  ( 5.049401038298161559, -19.05341960407611168, 42.70724293864767418 ) ) ;
#91917=CARTESIAN_POINT ( 'NONE',  ( -0.05219959533909027116, -19.03943276465977164, 102.4989096053143669 ) ) ;
#91918=CARTESIAN_POINT ( 'NONE',  ( 15.72974639402176855, 15.80617190586768217, 61.87609039468568284 ) ) ;
#91919=EDGE_CURVE ( 'NONE', #49306, #197846, #44416, .T. ) ;
#91920=CARTESIAN_POINT ( 'NONE',  ( 5.823673210054125526, 21.52544592524343514, 44.79057627198103120 ) ) ;
#91921=CARTESIAN_POINT ( 'NONE',  ( 14.29746914071049879, -8.314922557960816363, 28.33224293864769550 ) ) ;
#91922=CARTESIAN_POINT ( 'NONE',  ( -10.72451020669870658, -18.67979575497194134, 64.58442372801900433 ) ) ;
#91923=CARTESIAN_POINT ( 'NONE',  ( -0.05219959533937732626, 21.53943276465977519, 92.50109039468567573 ) ) ;
#91924=CARTESIAN_POINT ( 'NONE',  ( -0.05219959533936034679, 19.03943276465977164, 37.50109039468567573 ) ) ;
#91925=CARTESIAN_POINT ( 'NONE',  ( 4.379528057220092307, 16.55341960407617563, 97.29275706135234714 ) ) ;
#91926=CARTESIAN_POINT ( 'NONE',  ( 15.80617190586769283, -15.72974639402175789, 55.62609039468568284 ) ) ;
#91927=CARTESIAN_POINT ( 'NONE',  ( -13.97604488694527625, -13.89961937509977652, 46.87390960531435979 ) ) ;
#91928=CARTESIAN_POINT ( 'NONE',  ( -18.67979575497193778, 10.72451020669871902, 113.3344237280190328 ) ) ;
#91929=CARTESIAN_POINT ( 'NONE',  ( 16.51473224551069308, 9.474510206698969483, 114.1655762719810241 ) ) ;
#91930=CARTESIAN_POINT ( 'NONE',  ( -5.719274019375665041, -21.55341960407619695, 19.79275706135235069 ) ) ;
#91931=CARTESIAN_POINT ( 'NONE',  ( -15.72974639402197994, 15.80617190586746368, 70.62390960531436690 ) ) ;
#91932=CARTESIAN_POINT ( 'NONE',  ( 0.05219959533934541429, -16.53943276465976808, 40.00109039468567573 ) ) ;
#91934=CARTESIAN_POINT ( 'NONE',  ( -21.52544592524343514, 5.823673210054127303, 76.04057627198102409 ) ) ;
#91935=CARTESIAN_POINT ( 'NONE',  ( -16.52544592524335698, -4.483927247898792601, 68.95942372801901854 ) ) ;
#91936=CARTESIAN_POINT ( 'NONE',  ( -14.29746914071049879, 8.314922557960819915, 80.83224293864769550 ) ) ;
#91938=CARTESIAN_POINT ( 'NONE',  ( 13.97604488694548053, -13.89961937509957401, 105.6260903946856757 ) ) ;
#91939=CARTESIAN_POINT ( 'NONE',  ( 21.55341960407610458, 5.719274019375980345, 28.95724293864769905 ) ) ;
#91941=CARTESIAN_POINT ( 'NONE',  ( -16.55341960407617563, 4.379528057220093196, 33.54275706135234714 ) ) ;
#91942=CARTESIAN_POINT ( 'NONE',  ( 21.52544592524344225, -5.823673210054117533, 113.5405762719810383 ) ) ;
#91943=CARTESIAN_POINT ( 'NONE',  ( -10.81492255796078084, -18.62759615963271287, 32.08224293864769550 ) ) ;
#91944=CARTESIAN_POINT ( 'NONE',  ( 8.224510206698742110, 14.34966873604972548, 57.08442372801901854 ) ) ;
#91945=CARTESIAN_POINT ( 'NONE',  ( 13.97604488694527802, 13.89961937509977652, 79.37390960531435269 ) ) ;
#91946=CARTESIAN_POINT ( 'NONE',  ( -21.53943276465977519, -0.05219959533937600094, 43.75109039468568284 ) ) ;
#91947=CARTESIAN_POINT ( 'NONE',  ( 0.05219959533936267826, -19.03943276465977164, 110.0010903946856757 ) ) ;
#91948=CARTESIAN_POINT ( 'NONE',  ( -21.53943276465977519, 0.05219959533907696930, 26.24890960531435624 ) ) ;
#91949=ORIENTED_EDGE ( 'NONE', *, *, #82460, .T. ) ;
#91950=CARTESIAN_POINT ( 'NONE',  ( 5.049401038297881783, 19.05341960407617563, 27.29275706135232937 ) ) ;
#91951=CARTESIAN_POINT ( 'NONE',  ( -4.483927247898782831, 16.52544592524335698, 42.70942372801901854 ) ) ;
#91952=CARTESIAN_POINT ( 'NONE',  ( -16.51473224551069308, -9.474510206698971260, 106.6655762719810383 ) ) ;
#91953=CARTESIAN_POINT ( 'NONE',  ( -15.80617190586745835, -15.72974639402198527, 101.8739096053143811 ) ) ;
#91954=CARTESIAN_POINT ( 'NONE',  ( -13.97604488694527625, -13.89961937509977652, 66.87390960531436690 ) ) ;
#91955=CARTESIAN_POINT ( 'NONE',  ( -17.12812012977024168, 6.668231424566045895, 23.64051240676857191 ) ) ;
#91956=CARTESIAN_POINT ( 'NONE',  ( -8.224510206698948167, 14.34966873604960824, 85.41557627198102409 ) ) ;
#91957=CARTESIAN_POINT ( 'NONE',  ( -18.67979575497178146, -10.72451020669898902, 31.66557627198102054 ) ) ;
#91958=CARTESIAN_POINT ( 'NONE',  ( -17.48847506799968698, 5.747544572773787053, 35.82697437843280142 ) ) ;
#91959=CARTESIAN_POINT ( 'NONE',  ( 14.29746914071037800, 8.314922557961029526, 66.66775706135234714 ) ) ;
#91960=CARTESIAN_POINT ( 'NONE',  ( -10.81492255796078084, -18.62759615963271287, 112.0822429386477097 ) ) ;
#91961=CARTESIAN_POINT ( 'NONE',  ( -0.05219959533936034679, 19.03943276465977164, 82.50109039468567573 ) ) ;
#91962=CARTESIAN_POINT ( 'NONE',  ( -19.05341960407611168, -5.049401038298163336, 31.45724293864769550 ) ) ;
#91963=CARTESIAN_POINT ( 'NONE',  ( -10.81492255796078084, -18.62759615963271287, 62.08224293864769550 ) ) ;
#91964=CARTESIAN_POINT ( 'NONE',  ( 9.564922557960805705, 16.46253265017160317, 99.58224293864770971 ) ) ;
#91965=CARTESIAN_POINT ( 'NONE',  ( 18.62759615963255655, 10.81492255796105972, 96.66775706135234714 ) ) ;
#91966=CARTESIAN_POINT ( 'NONE',  ( 13.89961937509977652, -13.97604488694527269, 63.12390960531435979 ) ) ;
#91967=CARTESIAN_POINT ( 'NONE',  ( 4.379528057220092307, 16.55341960407617563, 47.29275706135234003 ) ) ;
#91968=CARTESIAN_POINT ( 'NONE',  ( -16.51473224551069308, -9.474510206698971260, 61.66557627198103120 ) ) ;
#91969=CARTESIAN_POINT ( 'NONE',  ( 10.72451020669871369, 18.67979575497193778, 77.08442372801901854 ) ) ;
#91971=CARTESIAN_POINT ( 'NONE',  ( -19.03943276465977164, -0.05219959533935918106, 33.75109039468566863 ) ) ;
#91972=CARTESIAN_POINT ( 'NONE',  ( -5.153800228976607833, 19.02544592524334988, 52.70942372801900433 ) ) ;
#91973=CARTESIAN_POINT ( 'NONE',  ( 5.719274019375673035, 21.55341960407619339, 47.29275706135234003 ) ) ;
#91975=CARTESIAN_POINT ( 'NONE',  ( -5.153800228976607833, 19.02544592524334988, 52.70942372801900433 ) ) ;
#91976=CARTESIAN_POINT ( 'NONE',  ( -5.049401038298153566, 19.05341960407611168, 100.2072429386476955 ) ) ;
#91977=CARTESIAN_POINT ( 'NONE',  ( -9.474510206698964154, 16.51473224551069663, 65.41557627198102409 ) ) ;
#91978=CARTESIAN_POINT ( 'NONE',  ( -12.14591786802309592, -12.06949235617757132, 26.87390960531435979 ) ) ;
#91979=CARTESIAN_POINT ( 'NONE',  ( 18.62759615963271287, -10.81492255796078972, 23.33224293864769194 ) ) ;
#91980=CARTESIAN_POINT ( 'NONE',  ( -5.823673210054431948, 21.52544592524334988, 102.7094237280190185 ) ) ;
#91983=CARTESIAN_POINT ( 'NONE',  ( -18.67979575497193778, 10.72451020669871902, 98.33442372801901854 ) ) ;
#91984=CARTESIAN_POINT ( 'NONE',  ( 16.52216118717208460, -7.221426719304494313, 41.42400978953008206 ) ) ;
#91985=CARTESIAN_POINT ( 'NONE',  ( -8.224510206698948167, 14.34966873604960824, 115.4155762719810241 ) ) ;
#91986=CARTESIAN_POINT ( 'NONE',  ( -18.22780087662122028, 5.500000000000031086, 98.51540105326105845 ) ) ;
#91989=CARTESIAN_POINT ( 'NONE',  ( -16.53943276465976808, -0.05219959533934237506, 48.75109039468568284 ) ) ;
#91990=CARTESIAN_POINT ( 'NONE',  ( 5.719274019375991003, -21.55341960407610458, 72.70724293864769550 ) ) ;
#91991=CARTESIAN_POINT ( 'NONE',  ( -12.06949235617756955, 12.14591786802309770, 45.62390960531436690 ) ) ;
#91992=CARTESIAN_POINT ( 'NONE',  ( -8.224510206698948167, 14.34966873604960824, 105.4155762719810383 ) ) ;
#91993=CARTESIAN_POINT ( 'NONE',  ( 13.97604488694527802, 13.89961937509977652, 94.37390960531436690 ) ) ;
#91994=CARTESIAN_POINT ( 'NONE',  ( 9.564922557961047289, -16.46253265017146816, 40.41775706135234003 ) ) ;
#91995=CARTESIAN_POINT ( 'NONE',  ( -4.483927247898539470, -16.52544592524342804, 112.2905762719810241 ) ) ;
#91996=CARTESIAN_POINT ( 'NONE',  ( -10.81492255796105439, 18.62759615963255655, 72.91775706135234714 ) ) ;
#91997=CARTESIAN_POINT ( 'NONE',  ( -0.05219959533909027116, -19.03943276465977164, 97.49890960531436690 ) ) ;
#91998=CARTESIAN_POINT ( 'NONE',  ( 4.483927247898790824, -16.52544592524335698, 110.2094237280190185 ) ) ;
#92000=CARTESIAN_POINT ( 'NONE',  ( 21.52544592524344225, -5.823673210054117533, 33.54057627198102409 ) ) ;
#92001=CARTESIAN_POINT ( 'NONE',  ( -16.52544592524342804, 4.483927247898546575, 91.04057627198103830 ) ) ;
#92003=CARTESIAN_POINT ( 'NONE',  ( 16.46253265017146816, 9.564922557961045513, 56.66775706135233293 ) ) ;
#92004=CARTESIAN_POINT ( 'NONE',  ( 9.474510206698971260, -16.51473224551069308, 82.91557627198103830 ) ) ;
#92005=CARTESIAN_POINT ( 'NONE',  ( 8.314922557960818139, 14.29746914071049879, 79.58224293864769550 ) ) ;
#92006=CARTESIAN_POINT ( 'NONE',  ( 19.05341960407617918, -5.049401038297876454, 96.04275706135231871 ) ) ;
#92007=CARTESIAN_POINT ( 'NONE',  ( 5.823673210054125526, 21.52544592524343514, 49.79057627198102409 ) ) ;
#92010=CARTESIAN_POINT ( 'NONE',  ( -5.153800228976328057, -19.02544592524343514, 22.29057627198102765 ) ) ;
#92011=CARTESIAN_POINT ( 'NONE',  ( -16.88567814943164791, -6.947325034625600360, 31.29001122652585920 ) ) ;
#92012=CARTESIAN_POINT ( 'NONE',  ( 9.564922557960805705, 16.46253265017160317, 74.58224293864769550 ) ) ;
#92013=CARTESIAN_POINT ( 'NONE',  ( -21.53943276465977519, 0.05219959533907696930, 81.24890960531436690 ) ) ;
#92014=CARTESIAN_POINT ( 'NONE',  ( -14.34966873604972548, 8.224510206698743886, 98.33442372801901854 ) ) ;
#92015=CARTESIAN_POINT ( 'NONE',  ( 13.89961937509977652, -13.97604488694527269, 88.12390960531438111 ) ) ;
#92016=CARTESIAN_POINT ( 'NONE',  ( 13.97604488694548053, -13.89961937509957401, 70.62609039468567573 ) ) ;
#92017=CARTESIAN_POINT ( 'NONE',  ( 18.62759615963255655, 10.81492255796105972, 76.66775706135234714 ) ) ;
#92018=CARTESIAN_POINT ( 'NONE',  ( 5.719274019375991003, -21.55341960407610458, 57.70724293864770260 ) ) ;
#92019=CARTESIAN_POINT ( 'NONE',  ( 9.564922557960805705, 16.46253265017160317, 114.5822429386476955 ) ) ;
#92021=CARTESIAN_POINT ( 'NONE',  ( 19.02544592524343514, -5.153800228976328945, 33.54057627198102409 ) ) ;
#92022=CARTESIAN_POINT ( 'NONE',  ( -8.224510206698735004, -14.34966873604973081, 99.58442372801900433 ) ) ;
#92023=CARTESIAN_POINT ( 'NONE',  ( -19.02544592524342804, 5.153800228976336051, 51.04057627198103120 ) ) ;
#92024=CARTESIAN_POINT ( 'NONE',  ( 16.53943276465976808, 0.05219959533934440121, 26.25109039468567573 ) ) ;
#92025=CARTESIAN_POINT ( 'NONE',  ( -5.153800228976607833, 19.02544592524335343, 82.70942372801899012 ) ) ;
#92026=CARTESIAN_POINT ( 'NONE',  ( 21.55341960407619695, -5.719274019375665929, 111.0427570613523613 ) ) ;
#92027=CIRCLE ( 'NONE', #30713, 2.000000000000001776 ) ;
#92028=CARTESIAN_POINT ( 'NONE',  ( 8.224510206698953496, -14.34966873604960469, 62.91557627198102409 ) ) ;
#92029=CARTESIAN_POINT ( 'NONE',  ( -9.564922557960796823, -16.46253265017161027, 92.08224293864769550 ) ) ;
#92030=CARTESIAN_POINT ( 'NONE',  ( 5.719274019375991003, -21.55341960407610458, 102.7072429386476955 ) ) ;
#92031=CARTESIAN_POINT ( 'NONE',  ( -15.72974639402197994, 15.80617190586746368, 100.6239096053143811 ) ) ;
#92032=DIRECTION ( 'NONE',  ( 0.000000000000000000, 0.000000000000000000, -1.000000000000000000 ) ) ;
#92033=CARTESIAN_POINT ( 'NONE',  ( -21.52544592524343514, 5.823673210054127303, 46.04057627198103830 ) ) ;
#92034=CARTESIAN_POINT ( 'NONE',  ( 14.34966873604972726, -8.224510206698740333, 75.83442372801900433 ) ) ;
#92035=CARTESIAN_POINT ( 'NONE',  ( -8.314922557960811034, -14.29746914071050412, 87.08224293864769550 ) ) ;
#92036=CARTESIAN_POINT ( 'NONE',  ( 9.564922557960805705, 16.46253265017160317, 59.58224293864769550 ) ) ;
#92038=CARTESIAN_POINT ( 'NONE',  ( -15.49999999999999822, -7.500000000000000888, 22.00000000000000711 ) ) ;
#92039=CARTESIAN_POINT ( 'NONE',  ( 12.14591786802327356, -12.06949235617739191, 110.6260903946857042 ) ) ;
#92040=CARTESIAN_POINT ( 'NONE',  ( -18.67979575497193778, 10.72451020669871902, 48.33442372801902565 ) ) ;
#92041=CARTESIAN_POINT ( 'NONE',  ( 13.89961937509977652, -13.97604488694527269, 93.12390960531436690 ) ) ;
#92042=CARTESIAN_POINT ( 'NONE',  ( 18.62759615963255655, 10.81492255796105972, 71.66775706135234714 ) ) ;
#92044=CARTESIAN_POINT ( 'NONE',  ( -13.97604488694527625, -13.89961937509977652, 26.87390960531434558 ) ) ;
#92046=CARTESIAN_POINT ( 'NONE',  ( -5.823673210054431948, 21.52544592524334988, 77.70942372801900433 ) ) ;
#92047=CARTESIAN_POINT ( 'NONE',  ( 16.46253265017160672, -9.564922557960803928, 48.33224293864769550 ) ) ;
#92048=CARTESIAN_POINT ( 'NONE',  ( -5.153800228976328057, -19.02544592524343514, 92.29057627198099567 ) ) ;
#92049=CARTESIAN_POINT ( 'NONE',  ( 5.049401038297881783, 19.05341960407617563, 77.29275706135231871 ) ) ;
#92050=CARTESIAN_POINT ( 'NONE',  ( -15.80617190586768217, 15.72974639402176855, 43.12609039468568284 ) ) ;
#92051=CARTESIAN_POINT ( 'NONE',  ( 13.89961937509957401, 13.97604488694547697, 101.8760903946856331 ) ) ;
#92052=CARTESIAN_POINT ( 'NONE',  ( 16.46253265017146816, 9.564922557961045513, 76.66775706135234714 ) ) ;
#92053=CARTESIAN_POINT ( 'NONE',  ( -16.51473224551069308, -9.474510206698971260, 41.66557627198103120 ) ) ;
#92054=CARTESIAN_POINT ( 'NONE',  ( 13.89961937509957401, 13.97604488694547697, 81.87609039468564731 ) ) ;
#92056=CARTESIAN_POINT ( 'NONE',  ( -14.34966873604972548, 8.224510206698743886, 108.3344237280190185 ) ) ;
#92057=CARTESIAN_POINT ( 'NONE',  ( -0.05219959533936034679, 19.03943276465977164, 72.50109039468566152 ) ) ;
#92058=CARTESIAN_POINT ( 'NONE',  ( 0.05219959533910956823, 16.53943276465976808, 44.99890960531435979 ) ) ;
#92059=CARTESIAN_POINT ( 'NONE',  ( -13.89961937509957401, -13.97604488694547875, 54.37609039468565442 ) ) ;
#92060=CARTESIAN_POINT ( 'NONE',  ( -10.81492255796105439, 18.62759615963255655, 107.9177570613523471 ) ) ;
#92062=CARTESIAN_POINT ( 'NONE',  ( -5.153800228976607833, 19.02544592524334988, 22.70942372801899012 ) ) ;
#92063=CARTESIAN_POINT ( 'NONE',  ( -9.474510206698964154, 16.51473224551069663, 25.41557627198103120 ) ) ;
#92064=CARTESIAN_POINT ( 'NONE',  ( 21.53943276465977519, 0.05219959533937863772, 86.25109039468568994 ) ) ;
#92065=CARTESIAN_POINT ( 'NONE',  ( 14.29746914071037800, 8.314922557961029526, 51.66775706135234714 ) ) ;
#92066=CARTESIAN_POINT ( 'NONE',  ( -19.02544592524342804, 5.153800228976336051, 91.04057627198100988 ) ) ;
#92068=CARTESIAN_POINT ( 'NONE',  ( -16.46253265017160317, 9.564922557960807481, 90.83224293864769550 ) ) ;
#92069=CARTESIAN_POINT ( 'NONE',  ( -17.13100169013222285, 6.664070546374236237, 100.7678983569982734 ) ) ;
#92071=CARTESIAN_POINT ( 'NONE',  ( 16.51473224551083163, -9.474510206698727899, 80.83442372801899012 ) ) ;
#92072=CARTESIAN_POINT ( 'NONE',  ( 18.67979575497178502, 10.72451020669898547, 29.16557627198103120 ) ) ;
#92073=CARTESIAN_POINT ( 'NONE',  ( -9.474510206698720793, -16.51473224551083518, 24.58442372801900078 ) ) ;
#92074=CARTESIAN_POINT ( 'NONE',  ( -19.05341960407617563, 5.049401038297882671, 103.5427570613523329 ) ) ;
#92075=CARTESIAN_POINT ( 'NONE',  ( -14.29746914071049879, 8.314922557960819915, 110.8322429386476955 ) ) ;
#92076=CARTESIAN_POINT ( 'NONE',  ( -19.02544592524342804, 5.153800228976336051, 26.04057627198103120 ) ) ;
#92077=CARTESIAN_POINT ( 'NONE',  ( -5.719274019375978568, 21.55341960407610458, 60.20724293864768839 ) ) ;
#92078=CARTESIAN_POINT ( 'NONE',  ( -5.823673210054116645, -21.52544592524344225, 52.29057627198102409 ) ) ;
#92079=CARTESIAN_POINT ( 'NONE',  ( -5.049401038298153566, 19.05341960407611168, 30.20724293864768839 ) ) ;
#92081=CARTESIAN_POINT ( 'NONE',  ( 9.474510206698729675, 16.51473224551082808, 67.08442372801900433 ) ) ;
#92082=CARTESIAN_POINT ( 'NONE',  ( -14.34966873604960291, -8.224510206698953496, 36.66557627198103120 ) ) ;
#92083=CARTESIAN_POINT ( 'NONE',  ( 18.62759615963271287, -10.81492255796078972, 23.33224293864769194 ) ) ;
#92084=CARTESIAN_POINT ( 'NONE',  ( 5.719274019375673035, 21.55341960407619339, 87.29275706135236135 ) ) ;
#92085=CARTESIAN_POINT ( 'NONE',  ( 5.823673210054125526, 21.52544592524343514, 74.79057627198105251 ) ) ;
#92086=CARTESIAN_POINT ( 'NONE',  ( -10.81492255796105439, 18.62759615963255655, 62.91775706135236135 ) ) ;
#92087=CARTESIAN_POINT ( 'NONE',  ( 21.55341960407619695, -5.719274019375665929, 56.04275706135235424 ) ) ;
#92088=CARTESIAN_POINT ( 'NONE',  ( -9.474510206698964154, 16.51473224551069663, 100.4155762719810241 ) ) ;
#92089=CARTESIAN_POINT ( 'NONE',  ( 14.34966873604972726, -8.224510206698740333, 90.83442372801901854 ) ) ;
#92090=CARTESIAN_POINT ( 'NONE',  ( 8.224510206698953496, -14.34966873604960469, 112.9155762719810383 ) ) ;
#92093=CARTESIAN_POINT ( 'NONE',  ( 16.53943276465976808, -0.05219959533910856209, 73.74890960531433848 ) ) ;
#92094=CARTESIAN_POINT ( 'NONE',  ( -0.05219959533910754901, -16.53943276465976808, 37.49890960531436690 ) ) ;
#92095=CARTESIAN_POINT ( 'NONE',  ( -13.97604488694527625, -13.89961937509977652, 61.87390960531435979 ) ) ;
#92096=CARTESIAN_POINT ( 'NONE',  ( 9.564922557960805705, 16.46253265017160317, 39.58224293864768839 ) ) ;
#92097=CARTESIAN_POINT ( 'NONE',  ( -5.719274019375978568, 21.55341960407610458, 55.20724293864770260 ) ) ;
#92098=CARTESIAN_POINT ( 'NONE',  ( -13.97604488694547697, 13.89961937509957934, 33.12609039468566863 ) ) ;
#92100=CARTESIAN_POINT ( 'NONE',  ( 16.52544592524342804, -4.483927247898539470, 53.54057627198103120 ) ) ;
#92101=CARTESIAN_POINT ( 'NONE',  ( -21.53943276465977519, 0.05219959533907696930, 31.24890960531435979 ) ) ;
#92102=VERTEX_POINT ( 'NONE', #166777 ) ;
#92104=CARTESIAN_POINT ( 'NONE',  ( 14.34966873604972726, -8.224510206698740333, 75.83442372801900433 ) ) ;
#92105=CARTESIAN_POINT ( 'NONE',  ( 16.51473224551083163, -9.474510206698727899, 70.83442372801900433 ) ) ;
#92106=CARTESIAN_POINT ( 'NONE',  ( -16.52544592524342804, 4.483927247898546575, 36.04057627198102409 ) ) ;
#92107=DIRECTION ( 'NONE',  ( 0.000000000000000000, 0.000000000000000000, -1.000000000000000000 ) ) ;
#92108=CARTESIAN_POINT ( 'NONE',  ( 14.34966873604960469, 8.224510206698951720, 29.16557627198103120 ) ) ;
#92109=CARTESIAN_POINT ( 'NONE',  ( 9.564922557960805705, 16.46253265017160317, 49.58224293864770260 ) ) ;
#92110=CARTESIAN_POINT ( 'NONE',  ( 5.049401038298161559, -19.05341960407611168, 72.70724293864768129 ) ) ;
#92111=CARTESIAN_POINT ( 'NONE',  ( 16.51473224551069308, 9.474510206698969483, 34.16557627198102409 ) ) ;
#92112=CARTESIAN_POINT ( 'NONE',  ( 5.823673210054444382, -21.52544592524334988, 50.20942372801901854 ) ) ;
#92113=CARTESIAN_POINT ( 'NONE',  ( -16.51473224551069308, -9.474510206698971260, 61.66557627198103120 ) ) ;
#92115=CARTESIAN_POINT ( 'NONE',  ( -16.51473224551069308, -9.474510206698971260, 46.66557627198102409 ) ) ;
#92117=CARTESIAN_POINT ( 'NONE',  ( 5.823673210054125526, 21.52544592524343514, 29.79057627198102409 ) ) ;
#92118=CARTESIAN_POINT ( 'NONE',  ( 5.719274019375673035, 21.55341960407619339, 72.29275706135236135 ) ) ;
#92119=CARTESIAN_POINT ( 'NONE',  ( -9.564922557960796823, -16.46253265017161027, 27.08224293864769550 ) ) ;
#92120=CARTESIAN_POINT ( 'NONE',  ( -5.823673210054116645, -21.52544592524344225, 32.29057627198102409 ) ) ;
#92121=CARTESIAN_POINT ( 'NONE',  ( -14.34966873604972548, 8.224510206698743886, 88.33442372801901854 ) ) ;
#92122=CARTESIAN_POINT ( 'NONE',  ( 21.52544592524334988, 5.823673210054432836, 101.4594237280190185 ) ) ;
#92123=CARTESIAN_POINT ( 'NONE',  ( 16.55341960407618274, -4.379528057220086978, 61.04275706135234714 ) ) ;
#92124=CARTESIAN_POINT ( 'NONE',  ( 16.51473224551069308, 9.474510206698969483, 104.1655762719810241 ) ) ;
#92126=CARTESIAN_POINT ( 'NONE',  ( -14.29746914071037622, -8.314922557961029526, 54.16775706135235424 ) ) ;
#92127=CARTESIAN_POINT ( 'NONE',  ( -4.379528057220086978, -16.55341960407618274, 39.79275706135235424 ) ) ;
#92128=CARTESIAN_POINT ( 'NONE',  ( 8.224510206698742110, 14.34966873604972548, 92.08442372801901854 ) ) ;
#92129=CARTESIAN_POINT ( 'NONE',  ( 21.55341960407619695, -5.719274019375665929, 56.04275706135235424 ) ) ;
#92130=CARTESIAN_POINT ( 'NONE',  ( 12.06949235617739724, 12.14591786802326823, 21.87609039468567573 ) ) ;
#92131=CARTESIAN_POINT ( 'NONE',  ( -21.53943276465977519, 0.05219959533907696930, 116.2489096053143669 ) ) ;
#92132=CARTESIAN_POINT ( 'NONE',  ( -9.564922557961040184, 16.46253265017147172, 112.9177570613523329 ) ) ;
#92133=CARTESIAN_POINT ( 'NONE',  ( 14.34966873604972726, -8.224510206698740333, 80.83442372801901854 ) ) ;
#92135=CARTESIAN_POINT ( 'NONE',  ( -5.823673210054431948, 21.52544592524334988, 82.70942372801900433 ) ) ;
#92136=CARTESIAN_POINT ( 'NONE',  ( -13.89961937509957401, -13.97604488694547875, 79.37609039468567573 ) ) ;
#92137=CARTESIAN_POINT ( 'NONE',  ( -16.53943276465976808, 0.05219959533911058130, 61.24890960531435979 ) ) ;
#92138=CARTESIAN_POINT ( 'NONE',  ( 0.05219959533910956823, 16.53943276465976808, 39.99890960531436690 ) ) ;
#92139=CARTESIAN_POINT ( 'NONE',  ( -14.29746914071049879, 8.314922557960819915, 100.8322429386477097 ) ) ;
#92140=CARTESIAN_POINT ( 'NONE',  ( 16.51473224551083163, -9.474510206698727899, 40.83442372801900433 ) ) ;
#92142=CARTESIAN_POINT ( 'NONE',  ( 21.55341960407619695, -5.719274019375665929, 51.04275706135234714 ) ) ;
#92143=CARTESIAN_POINT ( 'NONE',  ( -16.52544592524335698, -4.483927247898792601, 18.95942372801901143 ) ) ;
#92145=CARTESIAN_POINT ( 'NONE',  ( 19.05341960407611168, 5.049401038298154454, 103.9572429386476671 ) ) ;
#92146=CARTESIAN_POINT ( 'NONE',  ( -0.05219959533907301413, -21.53943276465977519, 77.49890960531433848 ) ) ;
#92147=CARTESIAN_POINT ( 'NONE',  ( -19.02544592524334988, -5.153800228976617603, 93.95942372801900433 ) ) ;
#92148=CARTESIAN_POINT ( 'NONE',  ( 19.02544592524343514, -5.153800228976328945, 108.5405762719810383 ) ) ;
#92150=CARTESIAN_POINT ( 'NONE',  ( -4.483927247898539470, -16.52544592524342804, 112.2905762719810241 ) ) ;
#92151=CARTESIAN_POINT ( 'NONE',  ( 0.05219959533937995610, -21.53943276465977519, 95.00109039468568994 ) ) ;
#92152=CARTESIAN_POINT ( 'NONE',  ( -19.03943276465977164, 0.05219959533909376836, 31.24890960531435979 ) ) ;
#92153=CARTESIAN_POINT ( 'NONE',  ( -5.823673210054431948, 21.52544592524334988, 47.70942372801902565 ) ) ;
#92154=CARTESIAN_POINT ( 'NONE',  ( -10.72451020669870658, -18.67979575497194134, 84.58442372801903275 ) ) ;
#92155=CARTESIAN_POINT ( 'NONE',  ( -8.314922557961024197, 14.29746914071037800, 87.91775706135234714 ) ) ;
#92156=CARTESIAN_POINT ( 'NONE',  ( -15.80617190586768217, 15.72974639402176855, 43.12609039468568284 ) ) ;
#92157=CARTESIAN_POINT ( 'NONE',  ( 0.05219959533937995610, -21.53943276465977519, 45.00109039468568284 ) ) ;
#92158=CARTESIAN_POINT ( 'NONE',  ( -16.51473224551082808, 9.474510206698731452, 68.33442372801900433 ) ) ;
#92159=CARTESIAN_POINT ( 'NONE',  ( -19.03943276465977164, 0.05219959533909376836, 96.24890960531436690 ) ) ;
#92160=CARTESIAN_POINT ( 'NONE',  ( 8.224510206698953496, -14.34966873604960469, 107.9155762719810241 ) ) ;
#92162=CARTESIAN_POINT ( 'NONE',  ( 21.55341960407610458, 5.719274019375980345, 78.95724293864769550 ) ) ;
#92163=CARTESIAN_POINT ( 'NONE',  ( -0.05219959533910754901, -16.53943276465976808, 62.49890960531436690 ) ) ;
#92164=CARTESIAN_POINT ( 'NONE',  ( 0.05219959533937995610, -21.53943276465977519, 100.0010903946857042 ) ) ;
#92165=CARTESIAN_POINT ( 'NONE',  ( -0.05219959533910754901, -16.53943276465976808, 77.49890960531433848 ) ) ;
#92166=CARTESIAN_POINT ( 'NONE',  ( 9.564922557960805705, 16.46253265017160317, 34.58224293864770260 ) ) ;
#92167=CARTESIAN_POINT ( 'NONE',  ( 16.51473224551083163, -9.474510206698727899, 90.83442372801900433 ) ) ;
#92168=CARTESIAN_POINT ( 'NONE',  ( 8.314922557960818139, 14.29746914071049879, 49.58224293864769550 ) ) ;
#92169=CARTESIAN_POINT ( 'NONE',  ( 5.719274019375673035, 21.55341960407619339, 97.29275706135234714 ) ) ;
#92170=CARTESIAN_POINT ( 'NONE',  ( 19.05341960407611168, 5.049401038298154454, 88.95724293864769550 ) ) ;
#92171=CARTESIAN_POINT ( 'NONE',  ( 19.02544592524334988, 5.153800228976608722, 56.45942372801898301 ) ) ;
#92172=CARTESIAN_POINT ( 'NONE',  ( 10.72451020669898902, -18.67979575497178502, 67.91557627198102409 ) ) ;
#92174=CARTESIAN_POINT ( 'NONE',  ( 10.72451020669898902, -18.67979575497178502, 112.9155762719810383 ) ) ;
#92175=CARTESIAN_POINT ( 'NONE',  ( 8.314922557961029526, -14.29746914071037800, 20.41775706135234714 ) ) ;
#92176=CARTESIAN_POINT ( 'NONE',  ( -4.483927247898782831, 16.52544592524335698, 82.70942372801900433 ) ) ;
#92177=CARTESIAN_POINT ( 'NONE',  ( 0.05219959533909260263, 19.03943276465977164, 24.99890960531435269 ) ) ;
#92178=CARTESIAN_POINT ( 'NONE',  ( 18.67979575497194134, -10.72451020669871369, 25.83442372801901499 ) ) ;
#92180=CARTESIAN_POINT ( 'NONE',  ( -19.03943276465977164, 0.05219959533909376836, 21.24890960531436335 ) ) ;
#92182=CARTESIAN_POINT ( 'NONE',  ( 14.34966873604972726, -8.224510206698740333, 50.83442372801901143 ) ) ;
#92183=CARTESIAN_POINT ( 'NONE',  ( 8.314922557960818139, 14.29746914071049879, 84.58224293864769550 ) ) ;
#92184=CARTESIAN_POINT ( 'NONE',  ( -21.55341960407610458, -5.719274019375992779, 76.45724293864769550 ) ) ;
#92185=CARTESIAN_POINT ( 'NONE',  ( -16.55341960407617563, 4.379528057220093196, 113.5427570613523756 ) ) ;
#92186=CARTESIAN_POINT ( 'NONE',  ( -14.29746914071037622, -8.314922557961029526, 34.16775706135234714 ) ) ;
#92187=CARTESIAN_POINT ( 'NONE',  ( 9.564922557960805705, 16.46253265017160317, 39.58224293864768839 ) ) ;
#92188=CARTESIAN_POINT ( 'NONE',  ( -8.224510206698735004, -14.34966873604973081, 74.58442372801901854 ) ) ;
#92189=CARTESIAN_POINT ( 'NONE',  ( -9.474510206698720793, -16.51473224551083518, 74.58442372801900433 ) ) ;
#92190=CARTESIAN_POINT ( 'NONE',  ( 5.719274019375991003, -21.55341960407610458, 67.70724293864769550 ) ) ;
#92191=CARTESIAN_POINT ( 'NONE',  ( 8.224510206698742110, 14.34966873604972548, 107.0844237280190043 ) ) ;
#92193=CARTESIAN_POINT ( 'NONE',  ( -10.81492255796105439, 18.62759615963255655, 77.91775706135231871 ) ) ;
#92194=CARTESIAN_POINT ( 'NONE',  ( -5.823673210054116645, -21.52544592524344225, 42.29057627198103120 ) ) ;
#92197=CARTESIAN_POINT ( 'NONE',  ( -8.224510206698735004, -14.34966873604973081, 94.58442372801901854 ) ) ;
#92198=CARTESIAN_POINT ( 'NONE',  ( -21.53943276465977519, 0.05219959533907696930, 41.24890960531435269 ) ) ;
#92200=CARTESIAN_POINT ( 'NONE',  ( -0.05219959533909027116, -19.03943276465977164, 107.4989096053143527 ) ) ;
#92201=CARTESIAN_POINT ( 'NONE',  ( 17.49999999999999289, 3.237210098469622377, 107.7876301262046042 ) ) ;
#92202=CARTESIAN_POINT ( 'NONE',  ( -5.049401038298153566, 19.05341960407611168, 30.20724293864768839 ) ) ;
#92203=CARTESIAN_POINT ( 'NONE',  ( -0.05219959533907301413, -21.53943276465977519, 77.49890960531433848 ) ) ;
#92204=CARTESIAN_POINT ( 'NONE',  ( -14.29746914071037622, -8.314922557961029526, 104.1677570613523471 ) ) ;
#92205=CARTESIAN_POINT ( 'NONE',  ( -0.05219959533937732626, 21.53943276465977519, 62.50109039468568284 ) ) ;
#92206=CARTESIAN_POINT ( 'NONE',  ( 12.06949235617739724, 12.14591786802326823, 26.87609039468567218 ) ) ;
#92207=CARTESIAN_POINT ( 'NONE',  ( 16.46253265017160672, -9.564922557960803928, 23.33224293864769194 ) ) ;
#92208=CARTESIAN_POINT ( 'NONE',  ( 4.483927247898790824, -16.52544592524335698, 20.20942372801900788 ) ) ;
#92209=CARTESIAN_POINT ( 'NONE',  ( -19.05341960407611168, -5.049401038298163336, 36.45724293864766707 ) ) ;
#92211=CARTESIAN_POINT ( 'NONE',  ( -9.474510206698964154, 16.51473224551069663, 110.4155762719810383 ) ) ;
#92212=CARTESIAN_POINT ( 'NONE',  ( -14.29746914071037622, -8.314922557961029526, 84.16775706135234714 ) ) ;
#92213=CARTESIAN_POINT ( 'NONE',  ( -0.05219959533936034679, 19.03943276465977164, 82.50109039468567573 ) ) ;
#92214=CARTESIAN_POINT ( 'NONE',  ( -16.46253265017146816, -9.564922557961047289, 29.16775706135232937 ) ) ;
#92215=CARTESIAN_POINT ( 'NONE',  ( 10.81492255796078972, 18.62759615963270932, 74.58224293864768129 ) ) ;
#92216=CARTESIAN_POINT ( 'NONE',  ( -14.29746914071037622, -8.314922557961029526, 99.16775706135234714 ) ) ;
#92217=CARTESIAN_POINT ( 'NONE',  ( 13.97604488694548053, -13.89961937509957401, 95.62609039468563310 ) ) ;
#92218=CARTESIAN_POINT ( 'NONE',  ( 5.153800228976335163, 19.02544592524342804, 54.79057627198103120 ) ) ;
#92219=CARTESIAN_POINT ( 'NONE',  ( 5.049401038298161559, -19.05341960407611168, 87.70724293864769550 ) ) ;
#92220=CARTESIAN_POINT ( 'NONE',  ( -21.53943276465977519, -0.05219959533937600094, 48.75109039468568284 ) ) ;
#92221=CARTESIAN_POINT ( 'NONE',  ( -16.46253265017160317, 9.564922557960807481, 50.83224293864770260 ) ) ;
#92223=CARTESIAN_POINT ( 'NONE',  ( -13.97604488694527625, -13.89961937509977652, 106.8739096053143669 ) ) ;
#92224=CARTESIAN_POINT ( 'NONE',  ( -4.483927247898539470, -16.52544592524342804, 62.29057627198102409 ) ) ;
#92225=CARTESIAN_POINT ( 'NONE',  ( 10.81492255796078972, 18.62759615963270932, 74.58224293864768129 ) ) ;
#92227=CARTESIAN_POINT ( 'NONE',  ( -16.51473224551082808, 9.474510206698731452, 48.33442372801900433 ) ) ;
#92228=CARTESIAN_POINT ( 'NONE',  ( 16.19135201231354415, -7.376712067591905786, 72.31319145947880145 ) ) ;
#92229=CARTESIAN_POINT ( 'NONE',  ( -9.474510206698964154, 16.51473224551069663, 65.41557627198102409 ) ) ;
#92230=CARTESIAN_POINT ( 'NONE',  ( 19.03943276465977164, -0.05219959533909143690, 88.74890960531436690 ) ) ;
#92232=CARTESIAN_POINT ( 'NONE',  ( -12.14591786802326823, 12.06949235617739902, 48.12609039468568284 ) ) ;
#92234=CARTESIAN_POINT ( 'NONE',  ( 0.05219959533936267826, -19.03943276465977164, 25.00109039468566152 ) ) ;
#92236=CARTESIAN_POINT ( 'NONE',  ( 8.314922557961029526, -14.29746914071037800, 95.41775706135234714 ) ) ;
#92238=CARTESIAN_POINT ( 'NONE',  ( 12.14591786802327356, -12.06949235617739191, 80.62609039468567573 ) ) ;
#92239=CARTESIAN_POINT ( 'NONE',  ( -8.314922557961024197, 14.29746914071037800, 52.91775706135235424 ) ) ;
#92240=CARTESIAN_POINT ( 'NONE',  ( -18.67979575497193778, 10.72451020669871902, 113.3344237280190328 ) ) ;
#92241=CARTESIAN_POINT ( 'NONE',  ( -19.03943276465977164, 0.05219959533909376836, 61.24890960531436690 ) ) ;
#92242=CARTESIAN_POINT ( 'NONE',  ( -17.49999999999999645, -5.499999999999992895, 59.20309617465829177 ) ) ;
#92243=CARTESIAN_POINT ( 'NONE',  ( -0.05219959533937732626, 21.53943276465977519, 72.50109039468568994 ) ) ;
#92244=CARTESIAN_POINT ( 'NONE',  ( 16.46253265017146816, 9.564922557961045513, 81.66775706135233293 ) ) ;
#92245=CARTESIAN_POINT ( 'NONE',  ( -15.72974639402176322, -15.80617190586768395, 104.3760903946856899 ) ) ;
#92247=CARTESIAN_POINT ( 'NONE',  ( 13.97604488694527802, 13.89961937509977652, 24.37390960531435624 ) ) ;
#92249=CARTESIAN_POINT ( 'NONE',  ( -18.67979575497178146, -10.72451020669898902, 66.66557627198102409 ) ) ;
#92251=CARTESIAN_POINT ( 'NONE',  ( -15.72974639402197994, 15.80617190586746368, 25.62390960531435624 ) ) ;
#92252=CARTESIAN_POINT ( 'NONE',  ( -16.55341960407611168, -4.379528057220339221, 111.4572429386476813 ) ) ;
#92253=CARTESIAN_POINT ( 'NONE',  ( 12.14591786802327356, -12.06949235617739191, 35.62609039468568994 ) ) ;
#92254=CARTESIAN_POINT ( 'NONE',  ( 12.14591786802309770, 12.06949235617756955, 34.37390960531435979 ) ) ;
#92255=ORIENTED_EDGE ( 'NONE', *, *, #36295, .T. ) ;
#92256=CARTESIAN_POINT ( 'NONE',  ( -5.823673210054116645, -21.52544592524344225, 112.2905762719810241 ) ) ;
#92257=CARTESIAN_POINT ( 'NONE',  ( 8.224510206698953496, -14.34966873604960469, 57.91557627198103120 ) ) ;
#92259=CARTESIAN_POINT ( 'NONE',  ( -19.05341960407617563, 5.049401038297882671, 113.5427570613523471 ) ) ;
#92260=CARTESIAN_POINT ( 'NONE',  ( -19.03943276465977164, -0.05219959533935918106, 28.75109039468566507 ) ) ;
#92261=CARTESIAN_POINT ( 'NONE',  ( 16.52544592524342804, -4.483927247898539470, 43.54057627198103830 ) ) ;
#92262=CARTESIAN_POINT ( 'NONE',  ( 21.52544592524344225, -5.823673210054117533, 108.5405762719810241 ) ) ;
#92264=CARTESIAN_POINT ( 'NONE',  ( -18.62759615963270932, 10.81492255796079327, 65.83224293864769550 ) ) ;
#92265=CARTESIAN_POINT ( 'NONE',  ( -9.474510206698964154, 16.51473224551069663, 75.41557627198103830 ) ) ;
#92266=CARTESIAN_POINT ( 'NONE',  ( -14.29746914071049879, 8.314922557960819915, 50.83224293864770971 ) ) ;
#92267=CARTESIAN_POINT ( 'NONE',  ( 19.02544592524343514, -5.153800228976328945, 98.54057627198100988 ) ) ;
#92269=CARTESIAN_POINT ( 'NONE',  ( 9.564922557961047289, -16.46253265017146816, 60.41775706135233293 ) ) ;
#92270=CARTESIAN_POINT ( 'NONE',  ( 21.53943276465977519, -0.05219959533907433946, 98.74890960531438111 ) ) ;
#92271=CARTESIAN_POINT ( 'NONE',  ( -5.049401038298153566, 19.05341960407611168, 45.20724293864769550 ) ) ;
#92272=CARTESIAN_POINT ( 'NONE',  ( -16.53943276465976808, 0.05219959533911058130, 111.2489096053143669 ) ) ;
#92273=CARTESIAN_POINT ( 'NONE',  ( 5.719274019375673035, 21.55341960407619339, 47.29275706135234003 ) ) ;
#92275=CARTESIAN_POINT ( 'NONE',  ( -12.06949235617756955, 12.14591786802309770, 30.62390960531436335 ) ) ;
#92276=CARTESIAN_POINT ( 'NONE',  ( -19.05341960407611168, -5.049401038298163336, 46.45724293864768129 ) ) ;
#92277=CARTESIAN_POINT ( 'NONE',  ( 9.474510206698971260, -16.51473224551069308, 102.9155762719810241 ) ) ;
#92278=CARTESIAN_POINT ( 'NONE',  ( 5.823673210054125526, 21.52544592524343514, 64.79057627198103830 ) ) ;
#92279=CARTESIAN_POINT ( 'NONE',  ( -19.49149378614658090, 5.499999999999782396, 44.43757513605364551 ) ) ;
#92280=CARTESIAN_POINT ( 'NONE',  ( 5.153800228976335163, 19.02544592524342804, 39.79057627198100988 ) ) ;
#92281=CARTESIAN_POINT ( 'NONE',  ( 10.72451020669898902, -18.67979575497178502, 57.91557627198103120 ) ) ;
#92283=CARTESIAN_POINT ( 'NONE',  ( -10.72451020669870658, -18.67979575497194134, 84.58442372801903275 ) ) ;
#92285=CARTESIAN_POINT ( 'NONE',  ( 8.224510206698742110, 14.34966873604972548, 77.08442372801901854 ) ) ;
#92286=CARTESIAN_POINT ( 'NONE',  ( -14.29746914071037622, -8.314922557961029526, 94.16775706135237556 ) ) ;
#92287=CARTESIAN_POINT ( 'NONE',  ( -16.51473224551069308, -9.474510206698971260, 51.66557627198102409 ) ) ;
#92288=CARTESIAN_POINT ( 'NONE',  ( -16.51473224551069308, -9.474510206698971260, 71.66557627198102409 ) ) ;
#92290=CARTESIAN_POINT ( 'NONE',  ( 0.05219959533936267826, -19.03943276465977164, 25.00109039468566152 ) ) ;
#92291=CARTESIAN_POINT ( 'NONE',  ( -4.379528057220086978, -16.55341960407618274, 79.79275706135236135 ) ) ;
#92292=CARTESIAN_POINT ( 'NONE',  ( 15.80617190586769283, -15.72974639402175789, 110.6260903946857042 ) ) ;
#92293=CARTESIAN_POINT ( 'NONE',  ( 9.474510206698971260, -16.51473224551069308, 72.91557627198102409 ) ) ;
#92294=CARTESIAN_POINT ( 'NONE',  ( 5.823673210054125526, 21.52544592524343514, 54.79057627198104541 ) ) ;
#92295=CARTESIAN_POINT ( 'NONE',  ( 8.314922557961029526, -14.29746914071037800, 30.41775706135234358 ) ) ;
#92296=CARTESIAN_POINT ( 'NONE',  ( -10.72451020669870658, -18.67979575497194134, 84.58442372801903275 ) ) ;
#92297=CARTESIAN_POINT ( 'NONE',  ( -4.379528057220086978, -16.55341960407618274, 44.79275706135234714 ) ) ;
#92298=CARTESIAN_POINT ( 'NONE',  ( -0.05219959533907301413, -21.53943276465977519, 107.4989096053143669 ) ) ;
#92299=CARTESIAN_POINT ( 'NONE',  ( -16.52544592524335698, -4.483927247898792601, 18.95942372801901143 ) ) ;
#92300=CARTESIAN_POINT ( 'NONE',  ( -0.05219959533909027116, -19.03943276465977164, 82.49890960531436690 ) ) ;
#92302=CARTESIAN_POINT ( 'NONE',  ( 14.34966873604972726, -8.224510206698740333, 30.83442372801902209 ) ) ;
#92303=CARTESIAN_POINT ( 'NONE',  ( -19.02544592524342804, 5.153800228976336051, 46.04057627198101699 ) ) ;
#92304=CARTESIAN_POINT ( 'NONE',  ( -16.52544592524335698, -4.483927247898792601, 23.95942372801901143 ) ) ;
#92305=CARTESIAN_POINT ( 'NONE',  ( -16.52544592524342804, 4.483927247898546575, 76.04057627198102409 ) ) ;
#92306=CARTESIAN_POINT ( 'NONE',  ( 14.29746914071037800, 8.314922557961029526, 81.66775706135236135 ) ) ;
#92307=CARTESIAN_POINT ( 'NONE',  ( -21.53943276465977519, -0.05219959533937600094, 28.75109039468567929 ) ) ;
#92308=CARTESIAN_POINT ( 'NONE',  ( 0.05219959533909260263, 19.03943276465977164, 59.99890960531436690 ) ) ;
#92309=CARTESIAN_POINT ( 'NONE',  ( 9.564922557960805705, 16.46253265017160317, 74.58224293864769550 ) ) ;
#92310=CARTESIAN_POINT ( 'NONE',  ( 14.34966873604972726, -8.224510206698740333, 85.83442372801901854 ) ) ;
#92314=CARTESIAN_POINT ( 'NONE',  ( 9.564922557961047289, -16.46253265017146816, 35.41775706135233293 ) ) ;
#92315=CARTESIAN_POINT ( 'NONE',  ( -19.03943276465977164, 0.05219959533909376836, 41.24890960531435269 ) ) ;
#92316=CARTESIAN_POINT ( 'NONE',  ( 19.02544592524343514, -5.153800228976328945, 113.5405762719810241 ) ) ;
#92318=CARTESIAN_POINT ( 'NONE',  ( -12.14591786802326823, 12.06949235617739902, 23.12609039468567573 ) ) ;
#92319=CARTESIAN_POINT ( 'NONE',  ( 16.51473224551083163, -9.474510206698727899, 55.83442372801899722 ) ) ;
#92320=CARTESIAN_POINT ( 'NONE',  ( 16.55341960407618274, -4.379528057220086978, 41.04275706135236135 ) ) ;
#92321=CARTESIAN_POINT ( 'NONE',  ( -13.97604488694527625, -13.89961937509977652, 111.8739096053143243 ) ) ;
#92322=CARTESIAN_POINT ( 'NONE',  ( -16.51473224551069308, -9.474510206698971260, 66.66557627198102409 ) ) ;
#92323=CARTESIAN_POINT ( 'NONE',  ( -5.719274019375978568, 21.55341960407610458, 105.2072429386477097 ) ) ;
#92324=CARTESIAN_POINT ( 'NONE',  ( 19.02544592524343514, -5.153800228976328945, 98.54057627198100988 ) ) ;
#92325=CARTESIAN_POINT ( 'NONE',  ( 9.474510206698971260, -16.51473224551069308, 22.91557627198102765 ) ) ;
#92326=CARTESIAN_POINT ( 'NONE',  ( 9.474510206698971260, -16.51473224551069308, 67.91557627198102409 ) ) ;
#92327=CARTESIAN_POINT ( 'NONE',  ( -16.53943276465976808, 0.05219959533911058130, 26.24890960531435624 ) ) ;
#92328=CARTESIAN_POINT ( 'NONE',  ( 9.564922557960805705, 16.46253265017160317, 29.58224293864769550 ) ) ;
#92329=CARTESIAN_POINT ( 'NONE',  ( -5.049401038297874678, -19.05341960407617918, 39.79275706135232582 ) ) ;
#92330=CARTESIAN_POINT ( 'NONE',  ( -8.314922557960811034, -14.29746914071050412, 57.08224293864769550 ) ) ;
#92331=CARTESIAN_POINT ( 'NONE',  ( -21.52544592524334988, -5.823673210054445271, 103.9594237280190185 ) ) ;
#92332=CARTESIAN_POINT ( 'NONE',  ( 16.46253265017160672, -9.564922557960803928, 38.33224293864768839 ) ) ;
#92333=CARTESIAN_POINT ( 'NONE',  ( 8.314922557961029526, -14.29746914071037800, 50.41775706135235424 ) ) ;
#92334=CARTESIAN_POINT ( 'NONE',  ( 16.55341960407611168, 4.379528057220329451, 38.95724293864768839 ) ) ;
#92335=CARTESIAN_POINT ( 'NONE',  ( 21.52544592524334988, 5.823673210054432836, 86.45942372801901854 ) ) ;
#92336=CARTESIAN_POINT ( 'NONE',  ( 19.05341960407611168, 5.049401038298154454, 78.95724293864769550 ) ) ;
#92337=CARTESIAN_POINT ( 'NONE',  ( -16.51473224551069308, -9.474510206698971260, 96.66557627198102409 ) ) ;
#92338=CARTESIAN_POINT ( 'NONE',  ( 12.14591786802309770, 12.06949235617756955, 104.3739096053143669 ) ) ;
#92339=CARTESIAN_POINT ( 'NONE',  ( 14.34966873604960469, 8.224510206698951720, 74.16557627198102409 ) ) ;
#92340=CARTESIAN_POINT ( 'NONE',  ( -10.72451020669898014, 18.67979575497178502, 90.41557627198103830 ) ) ;
#92341=CARTESIAN_POINT ( 'NONE',  ( 19.03943276465977164, -0.05219959533909143690, 88.74890960531436690 ) ) ;
#92342=CARTESIAN_POINT ( 'NONE',  ( 21.53943276465977519, -0.05219959533907433946, 93.74890960531436690 ) ) ;
#92343=CARTESIAN_POINT ( 'NONE',  ( 16.46253265017146816, 9.564922557961045513, 76.66775706135234714 ) ) ;
#92345=CARTESIAN_POINT ( 'NONE',  ( -16.46253265017146816, -9.564922557961047289, 64.16775706135233293 ) ) ;
#92346=CARTESIAN_POINT ( 'NONE',  ( 16.55341960407611168, 4.379528057220329451, 93.95724293864770971 ) ) ;
#92347=CARTESIAN_POINT ( 'NONE',  ( -16.51473224551069308, -9.474510206698971260, 51.66557627198102409 ) ) ;
#92348=CARTESIAN_POINT ( 'NONE',  ( 5.823673210054125526, 21.52544592524343514, 69.79057627198102409 ) ) ;
#92349=CARTESIAN_POINT ( 'NONE',  ( 17.50000000000000711, -5.622605283950868227, 26.18792689403890606 ) ) ;
#92350=CARTESIAN_POINT ( 'NONE',  ( -16.55341960407617563, 4.379528057220093196, 113.5427570613523756 ) ) ;
#92351=CARTESIAN_POINT ( 'NONE',  ( 14.34966873604972726, -8.224510206698740333, 20.83442372801901143 ) ) ;
#92352=CARTESIAN_POINT ( 'NONE',  ( -12.06949235617756955, 12.14591786802309770, 75.62390960531439532 ) ) ;
#92354=CARTESIAN_POINT ( 'NONE',  ( 16.46253265017160672, -9.564922557960803928, 68.33224293864770971 ) ) ;
#92355=CARTESIAN_POINT ( 'NONE',  ( -0.05219959533909027116, -19.03943276465977164, 37.49890960531436690 ) ) ;
#92356=CARTESIAN_POINT ( 'NONE',  ( 12.14591786802309770, 12.06949235617756955, 64.37390960531435269 ) ) ;
#92357=CARTESIAN_POINT ( 'NONE',  ( -10.72451020669898014, 18.67979575497178502, 25.41557627198103120 ) ) ;
#92358=CARTESIAN_POINT ( 'NONE',  ( -13.97604488694547697, 13.89961937509957934, 93.12609039468566152 ) ) ;
#92359=CARTESIAN_POINT ( 'NONE',  ( 9.564922557960805705, 16.46253265017160317, 104.5822429386476955 ) ) ;
#92360=CARTESIAN_POINT ( 'NONE',  ( -21.52544592524343514, 5.823673210054127303, 71.04057627198103830 ) ) ;
#92361=CARTESIAN_POINT ( 'NONE',  ( 4.483927247898790824, -16.52544592524335698, 65.20942372801901854 ) ) ;
#92362=CARTESIAN_POINT ( 'NONE',  ( -16.79531203550683927, 7.028104445595290350, 93.74755011779544134 ) ) ;
#92363=CARTESIAN_POINT ( 'NONE',  ( 9.564922557960805705, 16.46253265017160317, 64.58224293864769550 ) ) ;
#92364=CARTESIAN_POINT ( 'NONE',  ( -10.81492255796078084, -18.62759615963271287, 62.08224293864769550 ) ) ;
#92365=CARTESIAN_POINT ( 'NONE',  ( -16.52544592524335698, -4.483927247898792601, 18.95942372801901143 ) ) ;
#92366=CARTESIAN_POINT ( 'NONE',  ( -8.224510206698948167, 14.34966873604960824, 35.41557627198102409 ) ) ;
#92367=CARTESIAN_POINT ( 'NONE',  ( 5.823673210054444382, -21.52544592524334988, 65.20942372801901854 ) ) ;
#92369=CARTESIAN_POINT ( 'NONE',  ( 8.224510206698742110, 14.34966873604972548, 72.08442372801899012 ) ) ;
#92370=CARTESIAN_POINT ( 'NONE',  ( -16.46253265017160317, 9.564922557960807481, 105.8322429386476955 ) ) ;
#92371=CARTESIAN_POINT ( 'NONE',  ( 16.46253265017160672, -9.564922557960803928, 103.3322429386476955 ) ) ;
#92372=CARTESIAN_POINT ( 'NONE',  ( -17.48853670773246449, 5.747243402303040760, 78.66671299749995683 ) ) ;
#92373=CARTESIAN_POINT ( 'NONE',  ( -16.52544592524335698, -4.483927247898792601, 93.95942372801903275 ) ) ;
#92374=CARTESIAN_POINT ( 'NONE',  ( -8.314922557961024197, 14.29746914071037800, 52.91775706135235424 ) ) ;
#92375=CARTESIAN_POINT ( 'NONE',  ( 9.474510206698971260, -16.51473224551069308, 52.91557627198102409 ) ) ;
#92376=CARTESIAN_POINT ( 'NONE',  ( -19.05341960407611168, -5.049401038298163336, 76.45724293864769550 ) ) ;
#92377=CARTESIAN_POINT ( 'NONE',  ( 5.719274019375673035, 21.55341960407619339, 52.29275706135236135 ) ) ;
#92378=CARTESIAN_POINT ( 'NONE',  ( 16.55341960407618274, -4.379528057220086978, 56.04275706135235424 ) ) ;
#92379=CARTESIAN_POINT ( 'NONE',  ( 12.06949235617757843, -12.14591786802309237, 28.12390960531435979 ) ) ;
#92380=CARTESIAN_POINT ( 'NONE',  ( -16.51473224551069308, -9.474510206698971260, 36.66557627198102409 ) ) ;
#92381=CARTESIAN_POINT ( 'NONE',  ( -13.97604488694527625, -13.89961937509977652, 31.87390960531435979 ) ) ;
#92382=CARTESIAN_POINT ( 'NONE',  ( -16.52544592524335698, -4.483927247898792601, 33.95942372801901143 ) ) ;
#92383=CARTESIAN_POINT ( 'NONE',  ( 9.474510206698729675, 16.51473224551082808, 82.08442372801899012 ) ) ;
#92384=CARTESIAN_POINT ( 'NONE',  ( 14.29746914071049879, -8.314922557960816363, 78.33224293864770971 ) ) ;
#92385=CARTESIAN_POINT ( 'NONE',  ( -0.05219959533909027116, -19.03943276465977164, 47.49890960531435979 ) ) ;
#92386=CARTESIAN_POINT ( 'NONE',  ( 19.03943276465977164, 0.05219959533936151252, 81.25109039468567573 ) ) ;
#92388=CARTESIAN_POINT ( 'NONE',  ( -10.72451020669870658, -18.67979575497194134, 84.58442372801903275 ) ) ;
#92389=CARTESIAN_POINT ( 'NONE',  ( -16.52544592524335698, -4.483927247898792601, 48.95942372801902565 ) ) ;
#92390=CARTESIAN_POINT ( 'NONE',  ( -17.50000000000003197, 4.640572885337592268, 25.63788164548845572 ) ) ;
#92391=CARTESIAN_POINT ( 'NONE',  ( 10.81492255796078972, 18.62759615963270932, 49.58224293864769550 ) ) ;
#92392=CARTESIAN_POINT ( 'NONE',  ( -12.06949235617739369, -12.14591786802326823, 39.37609039468567573 ) ) ;
#92393=CARTESIAN_POINT ( 'NONE',  ( -19.25663599770060941, 5.499999999999443112, 68.99419308057200340 ) ) ;
#92394=CARTESIAN_POINT ( 'NONE',  ( 13.89961937509957401, 13.97604488694547697, 36.87609039468565442 ) ) ;
#92396=CARTESIAN_POINT ( 'NONE',  ( 5.049401038298161559, -19.05341960407611168, 92.70724293864769550 ) ) ;
#92397=CARTESIAN_POINT ( 'NONE',  ( 13.89961937509977652, -13.97604488694527269, 48.12390960531435979 ) ) ;
#92399=CARTESIAN_POINT ( 'NONE',  ( 5.823673210054444382, -21.52544592524334988, 75.20942372801901854 ) ) ;
#92401=CARTESIAN_POINT ( 'NONE',  ( 19.05341960407617918, -5.049401038297876454, 36.04275706135234003 ) ) ;
#92402=CARTESIAN_POINT ( 'NONE',  ( 5.823673210054444382, -21.52544592524334988, 110.2094237280190185 ) ) ;
#92403=CARTESIAN_POINT ( 'NONE',  ( 4.379528057220339221, -16.55341960407611168, 42.70724293864770260 ) ) ;
#92404=CARTESIAN_POINT ( 'NONE',  ( -5.153800228976328057, -19.02544592524343514, 42.29057627198101699 ) ) ;
#92405=CARTESIAN_POINT ( 'NONE',  ( 19.05341960407611168, 5.049401038298154454, 103.9572429386476671 ) ) ;
#92406=CARTESIAN_POINT ( 'NONE',  ( 21.52544592524334988, 5.823673210054432836, 81.45942372801900433 ) ) ;
#92407=CARTESIAN_POINT ( 'NONE',  ( 9.474510206698971260, -16.51473224551069308, 67.91557627198102409 ) ) ;
#92408=CARTESIAN_POINT ( 'NONE',  ( -18.62759615963255300, -10.81492255796106328, 79.16775706135234714 ) ) ;
#92409=CARTESIAN_POINT ( 'NONE',  ( 0.05219959533907565091, 21.53943276465977519, 34.99890960531435979 ) ) ;
#92410=CARTESIAN_POINT ( 'NONE',  ( -10.72451020669870658, -18.67979575497194134, 24.58442372801901499 ) ) ;
#92411=CARTESIAN_POINT ( 'NONE',  ( -5.049401038297874678, -19.05341960407617918, 44.79275706135232582 ) ) ;
#92412=CARTESIAN_POINT ( 'NONE',  ( 19.02544592524343514, -5.153800228976328945, 23.54057627198102054 ) ) ;
#92413=CARTESIAN_POINT ( 'NONE',  ( 5.153800228976335163, 19.02544592524342804, 69.79057627198103830 ) ) ;
#92414=CARTESIAN_POINT ( 'NONE',  ( 14.29746914071037800, 8.314922557961029526, 26.66775706135235424 ) ) ;
#92415=CARTESIAN_POINT ( 'NONE',  ( 14.34966873604960469, 8.224510206698951720, 89.16557627198102409 ) ) ;
#92416=CARTESIAN_POINT ( 'NONE',  ( -0.05219959533909027116, -19.03943276465977164, 52.49890960531436690 ) ) ;
#92417=CARTESIAN_POINT ( 'NONE',  ( -21.55341960407610458, -5.719274019375992779, 41.45724293864769550 ) ) ;
#92418=CARTESIAN_POINT ( 'NONE',  ( 0.05219959533936267826, -19.03943276465977164, 105.0010903946856615 ) ) ;
#92419=CARTESIAN_POINT ( 'NONE',  ( -21.53943276465977519, 0.05219959533907696930, 111.2489096053143669 ) ) ;
#92420=CARTESIAN_POINT ( 'NONE',  ( 21.52544592524334988, 5.823673210054432836, 56.45942372801902565 ) ) ;
#92421=CARTESIAN_POINT ( 'NONE',  ( 14.34966873604972726, -8.224510206698740333, 70.83442372801901854 ) ) ;
#92422=CARTESIAN_POINT ( 'NONE',  ( -16.55341960407617563, 4.379528057220093196, 63.54275706135234003 ) ) ;
#92423=ORIENTED_EDGE ( 'NONE', *, *, #153922, .F. ) ;
#92424=CARTESIAN_POINT ( 'NONE',  ( -16.46253265017160317, 9.564922557960807481, 65.83224293864769550 ) ) ;
#92425=CARTESIAN_POINT ( 'NONE',  ( -16.52544592524335698, -4.483927247898792601, 88.95942372801901854 ) ) ;
#92426=CARTESIAN_POINT ( 'NONE',  ( -21.53943276465977519, -0.05219959533937600094, 18.75109039468568639 ) ) ;
#92427=CARTESIAN_POINT ( 'NONE',  ( 0.05219959533910956823, 16.53943276465976808, 69.99890960531435269 ) ) ;
#92428=CARTESIAN_POINT ( 'NONE',  ( 16.46253265017160672, -9.564922557960803928, 88.33224293864769550 ) ) ;
#92429=CARTESIAN_POINT ( 'NONE',  ( 16.52544592524335698, 4.483927247898782831, 76.45942372801901854 ) ) ;
#92430=CARTESIAN_POINT ( 'NONE',  ( 15.80617190586769283, -15.72974639402175789, 60.62609039468567573 ) ) ;
#92431=CARTESIAN_POINT ( 'NONE',  ( 13.97604488694548053, -13.89961937509957401, 110.6260903946856615 ) ) ;
#92432=CARTESIAN_POINT ( 'NONE',  ( 0.05219959533907565091, 21.53943276465977519, 114.9989096053143669 ) ) ;
#92433=CARTESIAN_POINT ( 'NONE',  ( 12.14591786802309770, 12.06949235617756955, 59.37390960531436690 ) ) ;
#92436=CARTESIAN_POINT ( 'NONE',  ( 5.719274019375991003, -21.55341960407610458, 87.70724293864769550 ) ) ;
#92437=CARTESIAN_POINT ( 'NONE',  ( 14.29746914071049879, -8.314922557960816363, 38.33224293864768839 ) ) ;
#92440=CARTESIAN_POINT ( 'NONE',  ( 18.67979575497194134, -10.72451020669871369, 20.83442372801901143 ) ) ;
#92441=CARTESIAN_POINT ( 'NONE',  ( -0.05219959533907301413, -21.53943276465977519, 22.49890960531436335 ) ) ;
#92442=CARTESIAN_POINT ( 'NONE',  ( 10.72451020669871369, 18.67979575497193778, 32.08442372801901854 ) ) ;
#92443=CARTESIAN_POINT ( 'NONE',  ( 0.05219959533910956823, 16.53943276465976808, 44.99890960531435979 ) ) ;
#92444=CARTESIAN_POINT ( 'NONE',  ( -4.483927247898782831, 16.52544592524335698, 57.70942372801901143 ) ) ;
#92445=CARTESIAN_POINT ( 'NONE',  ( -19.03943276465977164, 0.05219959533909376836, 61.24890960531436690 ) ) ;
#92446=CARTESIAN_POINT ( 'NONE',  ( 9.564922557961047289, -16.46253265017146816, 60.41775706135233293 ) ) ;
#92447=CARTESIAN_POINT ( 'NONE',  ( -9.564922557960796823, -16.46253265017161027, 92.08224293864769550 ) ) ;
#92448=CARTESIAN_POINT ( 'NONE',  ( 15.80617190586746368, 15.72974639402197994, 54.37390960531435979 ) ) ;
#92450=CARTESIAN_POINT ( 'NONE',  ( -5.153800228976328057, -19.02544592524343514, 52.29057627198100988 ) ) ;
#92451=CARTESIAN_POINT ( 'NONE',  ( -8.224510206698735004, -14.34966873604973081, 39.58442372801901143 ) ) ;
#92452=CARTESIAN_POINT ( 'NONE',  ( -16.51473224551082808, 9.474510206698731452, 58.33442372801900433 ) ) ;
#92453=CARTESIAN_POINT ( 'NONE',  ( 0.05219959533937995610, -21.53943276465977519, 20.00109039468568639 ) ) ;
#92454=CARTESIAN_POINT ( 'NONE',  ( 12.06949235617757843, -12.14591786802309237, 43.12390960531435269 ) ) ;
#92455=CARTESIAN_POINT ( 'NONE',  ( 13.97604488694527802, 13.89961937509977652, 84.37390960531433848 ) ) ;
#92456=CARTESIAN_POINT ( 'NONE',  ( -10.72451020669898014, 18.67979575497178502, 60.41557627198102409 ) ) ;
#92457=CARTESIAN_POINT ( 'NONE',  ( 21.55341960407610458, 5.719274019375980345, 93.95724293864770971 ) ) ;
#92458=CARTESIAN_POINT ( 'NONE',  ( 14.29746914071037800, 8.314922557961029526, 41.66775706135235424 ) ) ;
#92459=CARTESIAN_POINT ( 'NONE',  ( -10.72451020669898014, 18.67979575497178502, 35.41557627198102409 ) ) ;
#92460=CARTESIAN_POINT ( 'NONE',  ( -21.52544592524334988, -5.823673210054445271, 88.95942372801901854 ) ) ;
#92461=CARTESIAN_POINT ( 'NONE',  ( 9.564922557960805705, 16.46253265017160317, 84.58224293864769550 ) ) ;
#92462=CARTESIAN_POINT ( 'NONE',  ( 19.02544592524343514, -5.153800228976328945, 38.54057627198103120 ) ) ;
#92463=CARTESIAN_POINT ( 'NONE',  ( -5.153800228976328057, -19.02544592524343514, 92.29057627198099567 ) ) ;
#92464=CARTESIAN_POINT ( 'NONE',  ( 0.05219959533910956823, 16.53943276465976808, 104.9989096053143669 ) ) ;
#92465=CARTESIAN_POINT ( 'NONE',  ( 9.474510206698971260, -16.51473224551069308, 67.91557627198102409 ) ) ;
#92466=CARTESIAN_POINT ( 'NONE',  ( -16.55341960407617563, 4.379528057220093196, 28.54275706135234358 ) ) ;
#92467=CARTESIAN_POINT ( 'NONE',  ( -9.564922557961040184, 16.46253265017147172, 42.91775706135234003 ) ) ;
#92468=CARTESIAN_POINT ( 'NONE',  ( -0.05219959533936034679, 19.03943276465977164, 57.50109039468566863 ) ) ;
#92469=CARTESIAN_POINT ( 'NONE',  ( 18.62759615963255655, 10.81492255796105972, 101.6677570613523613 ) ) ;
#92470=CARTESIAN_POINT ( 'NONE',  ( 18.62759615963271287, -10.81492255796078972, 28.33224293864769550 ) ) ;
#92471=CARTESIAN_POINT ( 'NONE',  ( 0.05219959533934541429, -16.53943276465976808, 95.00109039468568994 ) ) ;
#92473=CARTESIAN_POINT ( 'NONE',  ( 19.05341960407617918, -5.049401038297876454, 76.04275706135230450 ) ) ;
#92474=CARTESIAN_POINT ( 'NONE',  ( 13.97604488694548053, -13.89961937509957401, 35.62609039468567573 ) ) ;
#92476=CARTESIAN_POINT ( 'NONE',  ( 5.049401038298161559, -19.05341960407611168, 27.70724293864769550 ) ) ;
#92477=CARTESIAN_POINT ( 'NONE',  ( -0.05219959533910754901, -16.53943276465976808, 32.49890960531435979 ) ) ;
#92478=CARTESIAN_POINT ( 'NONE',  ( 5.049401038298161559, -19.05341960407611168, 22.70724293864769194 ) ) ;
#92479=CARTESIAN_POINT ( 'NONE',  ( -4.379528057220328563, 16.55341960407611168, 30.20724293864769550 ) ) ;
#92480=CARTESIAN_POINT ( 'NONE',  ( 17.50000000000000000, -5.500000000000000888, 120.0000000000000142 ) ) ;
#92481=CARTESIAN_POINT ( 'NONE',  ( -0.05219959533934338120, 16.53943276465976808, 97.50109039468567573 ) ) ;
#92482=CARTESIAN_POINT ( 'NONE',  ( -16.46253265017160317, 9.564922557960807481, 40.83224293864769550 ) ) ;
#92483=CARTESIAN_POINT ( 'NONE',  ( 21.55341960407619695, -5.719274019375665929, 101.0427570613523756 ) ) ;
#92484=CARTESIAN_POINT ( 'NONE',  ( -8.224510206698735004, -14.34966873604973081, 24.58442372801901499 ) ) ;
#92485=CARTESIAN_POINT ( 'NONE',  ( -10.81492255796105439, 18.62759615963255655, 82.91775706135234714 ) ) ;
#92486=CARTESIAN_POINT ( 'NONE',  ( -19.02544592524334988, -5.153800228976617603, 58.95942372801900433 ) ) ;
#92487=CARTESIAN_POINT ( 'NONE',  ( -16.51473224551069308, -9.474510206698971260, 96.66557627198102409 ) ) ;
#92488=CARTESIAN_POINT ( 'NONE',  ( -13.97604488694527625, -13.89961937509977652, 86.87390960531436690 ) ) ;
#92489=CARTESIAN_POINT ( 'NONE',  ( 17.40861289039004589, 6.110651285853279546, 73.87232470827433417 ) ) ;
#92490=CARTESIAN_POINT ( 'NONE',  ( -15.80617190586745835, -15.72974639402198527, 111.8739096053143669 ) ) ;
#92492=CARTESIAN_POINT ( 'NONE',  ( -14.34966873604960291, -8.224510206698953496, 61.66557627198103120 ) ) ;
#92493=CARTESIAN_POINT ( 'NONE',  ( 0.05219959533907565091, 21.53943276465977519, 59.99890960531436690 ) ) ;
#92494=CARTESIAN_POINT ( 'NONE',  ( 0.05219959533909260263, 19.03943276465977164, 59.99890960531436690 ) ) ;
#92495=CARTESIAN_POINT ( 'NONE',  ( 15.72974639402199770, -15.80617190586745480, 103.1239096053143811 ) ) ;
#92496=CARTESIAN_POINT ( 'NONE',  ( -16.53943276465976808, -0.05219959533934237506, 93.75109039468567573 ) ) ;
#92497=ORIENTED_EDGE ( 'NONE', *, *, #191495, .F. ) ;
#92498=CARTESIAN_POINT ( 'NONE',  ( 5.049401038298161559, -19.05341960407611168, 47.70724293864770260 ) ) ;
#92499=CARTESIAN_POINT ( 'NONE',  ( 14.29746914071049879, -8.314922557960816363, 88.33224293864769550 ) ) ;
#92501=CARTESIAN_POINT ( 'NONE',  ( -5.153800228976328057, -19.02544592524343514, 47.29057627198102409 ) ) ;
#92502=CARTESIAN_POINT ( 'NONE',  ( 0.05219959533910956823, 16.53943276465976808, 114.9989096053143669 ) ) ;
#92503=CARTESIAN_POINT ( 'NONE',  ( 5.153800228976615827, -19.02544592524334988, 85.20942372801900433 ) ) ;
#92504=CARTESIAN_POINT ( 'NONE',  ( 14.34966873604960469, 8.224510206698951720, 84.16557627198103830 ) ) ;
#92505=CARTESIAN_POINT ( 'NONE',  ( 15.80617190586769283, -15.72974639402175789, 50.62609039468568994 ) ) ;
#92506=CARTESIAN_POINT ( 'NONE',  ( -19.05341960407611168, -5.049401038298163336, 31.45724293864769550 ) ) ;
#92507=CARTESIAN_POINT ( 'NONE',  ( 21.55341960407610458, 5.719274019375980345, 108.9572429386476955 ) ) ;
#92508=CARTESIAN_POINT ( 'NONE',  ( -14.34966873604960291, -8.224510206698953496, 91.66557627198103830 ) ) ;
#92510=CARTESIAN_POINT ( 'NONE',  ( 19.02544592524343514, -5.153800228976328945, 58.54057627198102409 ) ) ;
#92511=CARTESIAN_POINT ( 'NONE',  ( 18.39639308325437028, 5.500000000000037303, 48.98252246182195080 ) ) ;
#92512=CARTESIAN_POINT ( 'NONE',  ( -19.02544592524334988, -5.153800228976617603, 93.95942372801900433 ) ) ;
#92513=CARTESIAN_POINT ( 'NONE',  ( -16.46253265017160317, 9.564922557960807481, 105.8322429386476955 ) ) ;
#92514=CARTESIAN_POINT ( 'NONE',  ( 18.67979575497194134, -10.72451020669871369, 30.83442372801902209 ) ) ;
#92515=CARTESIAN_POINT ( 'NONE',  ( 9.474510206698971260, -16.51473224551069308, 77.91557627198103830 ) ) ;
#92516=CARTESIAN_POINT ( 'NONE',  ( -16.51473224551082808, 9.474510206698731452, 68.33442372801900433 ) ) ;
#92517=CARTESIAN_POINT ( 'NONE',  ( -0.05219959533909027116, -19.03943276465977164, 52.49890960531436690 ) ) ;
#92518=CARTESIAN_POINT ( 'NONE',  ( 4.483927247898545687, 16.52544592524342804, 79.79057627198102409 ) ) ;
#92519=CARTESIAN_POINT ( 'NONE',  ( -14.29746914071049879, 8.314922557960819915, 70.83224293864770971 ) ) ;
#92520=CARTESIAN_POINT ( 'NONE',  ( 0.05219959533909260263, 19.03943276465977164, 94.99890960531436690 ) ) ;
#92521=CARTESIAN_POINT ( 'NONE',  ( 15.80617190586746368, 15.72974639402197994, 104.3739096053143669 ) ) ;
#92522=CARTESIAN_POINT ( 'NONE',  ( 19.03943276465977164, -0.05219959533909143690, 83.74890960531436690 ) ) ;
#92524=CARTESIAN_POINT ( 'NONE',  ( 16.51473224551083163, -9.474510206698727899, 35.83442372801899722 ) ) ;
#92525=CARTESIAN_POINT ( 'NONE',  ( -0.05219959533909027116, -19.03943276465977164, 37.49890960531436690 ) ) ;
#92526=CARTESIAN_POINT ( 'NONE',  ( -14.29746914071049879, 8.314922557960819915, 35.83224293864768839 ) ) ;
#92527=CARTESIAN_POINT ( 'NONE',  ( -14.34966873604960291, -8.224510206698953496, 111.6655762719810525 ) ) ;
#92529=CARTESIAN_POINT ( 'NONE',  ( 21.53943276465977519, 0.05219959533937863772, 31.25109039468568639 ) ) ;
#92530=CARTESIAN_POINT ( 'NONE',  ( -9.474510206698720793, -16.51473224551083518, 64.58442372801900433 ) ) ;
#92531=CARTESIAN_POINT ( 'NONE',  ( -16.55341960407611168, -4.379528057220339221, 41.45724293864769550 ) ) ;
#92532=CARTESIAN_POINT ( 'NONE',  ( 0.05219959533907565091, 21.53943276465977519, 84.99890960531436690 ) ) ;
#92533=CARTESIAN_POINT ( 'NONE',  ( 13.89961937509977652, -13.97604488694527269, 113.1239096053143527 ) ) ;
#92534=CARTESIAN_POINT ( 'NONE',  ( 12.06949235617757843, -12.14591786802309237, 73.12390960531436690 ) ) ;
#92535=CARTESIAN_POINT ( 'NONE',  ( -5.049401038298153566, 19.05341960407611168, 25.20724293864768484 ) ) ;
#92536=CARTESIAN_POINT ( 'NONE',  ( 13.89961937509957401, 13.97604488694547697, 21.87609039468566152 ) ) ;
#92537=CARTESIAN_POINT ( 'NONE',  ( -12.14591786802326823, 12.06949235617739902, 108.1260903946856757 ) ) ;
#92538=CARTESIAN_POINT ( 'NONE',  ( -8.314922557961024197, 14.29746914071037800, 62.91775706135236135 ) ) ;
#92539=CARTESIAN_POINT ( 'NONE',  ( -21.53943276465977519, 0.05219959533907696930, 36.24890960531435979 ) ) ;
#92540=CARTESIAN_POINT ( 'NONE',  ( 15.80617190586769283, -15.72974639402175789, 105.6260903946856899 ) ) ;
#92541=CARTESIAN_POINT ( 'NONE',  ( 16.51473224551069308, 9.474510206698969483, 74.16557627198103830 ) ) ;
#92543=CARTESIAN_POINT ( 'NONE',  ( 14.34966873604972726, -8.224510206698740333, 65.83442372801900433 ) ) ;
#92544=CARTESIAN_POINT ( 'NONE',  ( 5.153800228976335163, 19.02544592524342804, 29.79057627198102409 ) ) ;
#92545=CARTESIAN_POINT ( 'NONE',  ( -0.05219959533910754901, -16.53943276465976808, 37.49890960531436690 ) ) ;
#92546=CARTESIAN_POINT ( 'NONE',  ( -13.89961937509977652, 13.97604488694528158, 110.6239096053143243 ) ) ;
#92547=CARTESIAN_POINT ( 'NONE',  ( -0.05219959533909027116, -19.03943276465977164, 87.49890960531436690 ) ) ;
#92548=CARTESIAN_POINT ( 'NONE',  ( 0.05219959533909260263, 19.03943276465977164, 114.9989096053143669 ) ) ;
#92549=CARTESIAN_POINT ( 'NONE',  ( 8.224510206698953496, -14.34966873604960469, 62.91557627198102409 ) ) ;
#92550=CARTESIAN_POINT ( 'NONE',  ( -14.29746914071049879, 8.314922557960819915, 35.83224293864768839 ) ) ;
#92551=CARTESIAN_POINT ( 'NONE',  ( 4.379528057220339221, -16.55341960407611168, 52.70724293864769550 ) ) ;
#92553=CARTESIAN_POINT ( 'NONE',  ( -4.379528057220086978, -16.55341960407618274, 39.79275706135235424 ) ) ;
#92555=CARTESIAN_POINT ( 'NONE',  ( -16.46253265017146816, -9.564922557961047289, 54.16775706135234003 ) ) ;
#92556=CARTESIAN_POINT ( 'NONE',  ( -0.05219959533909027116, -19.03943276465977164, 77.49890960531435269 ) ) ;
#92557=CARTESIAN_POINT ( 'NONE',  ( -16.46253265017146816, -9.564922557961047289, 69.16775706135233293 ) ) ;
#92559=CARTESIAN_POINT ( 'NONE',  ( -5.049401038297874678, -19.05341960407617918, 49.79275706135231871 ) ) ;
#92560=CARTESIAN_POINT ( 'NONE',  ( -19.03943276465977164, -0.05219959533935918106, 103.7510903946856757 ) ) ;
#92561=CARTESIAN_POINT ( 'NONE',  ( 16.53943276465976808, 0.05219959533934440121, 76.25109039468568994 ) ) ;
#92564=CARTESIAN_POINT ( 'NONE',  ( -13.89961937509977652, 13.97604488694528158, 115.6239096053143669 ) ) ;
#92565=CARTESIAN_POINT ( 'NONE',  ( 5.719274019375673035, 21.55341960407619339, 47.29275706135234003 ) ) ;
#92566=CARTESIAN_POINT ( 'NONE',  ( -19.03943276465977164, -0.05219959533935918106, 108.7510903946856615 ) ) ;
#92567=DIRECTION ( 'NONE',  ( 8.673617379884035472E-16, 1.000000000000000000, 0.000000000000000000 ) ) ;
#92568=CARTESIAN_POINT ( 'NONE',  ( -9.474510206698964154, 16.51473224551069663, 60.41557627198102409 ) ) ;
#92569=CARTESIAN_POINT ( 'NONE',  ( -19.02544592524342804, 5.153800228976336051, 106.0405762719810241 ) ) ;
#92570=CARTESIAN_POINT ( 'NONE',  ( -4.379528057220328563, 16.55341960407611168, 60.20724293864768839 ) ) ;
#92571=CARTESIAN_POINT ( 'NONE',  ( -0.05219959533909027116, -19.03943276465977164, 57.49890960531435979 ) ) ;
#92572=CARTESIAN_POINT ( 'NONE',  ( 16.46253265017160672, -9.564922557960803928, 58.33224293864769550 ) ) ;
#92573=CARTESIAN_POINT ( 'NONE',  ( -9.474510206698720793, -16.51473224551083518, 74.58442372801900433 ) ) ;
#92574=CARTESIAN_POINT ( 'NONE',  ( -5.823673210054116645, -21.52544592524344225, 47.29057627198103120 ) ) ;
#92575=CARTESIAN_POINT ( 'NONE',  ( 16.52544592524342804, -4.483927247898539470, 113.5405762719810383 ) ) ;
#92576=CARTESIAN_POINT ( 'NONE',  ( -19.02544592524334988, -5.153800228976617603, 48.95942372801900433 ) ) ;
#92577=CARTESIAN_POINT ( 'NONE',  ( -9.474510206698964154, 16.51473224551069663, 80.41557627198103830 ) ) ;
#92578=CARTESIAN_POINT ( 'NONE',  ( -21.55341960407610458, -5.719274019375992779, 76.45724293864769550 ) ) ;
#92579=CARTESIAN_POINT ( 'NONE',  ( -4.483927247898539470, -16.52544592524342804, 82.29057627198103830 ) ) ;
#92580=CARTESIAN_POINT ( 'NONE',  ( -16.51473224551082808, 9.474510206698731452, 38.33442372801899722 ) ) ;
#92581=CARTESIAN_POINT ( 'NONE',  ( 21.55341960407610458, 5.719274019375980345, 63.95724293864770260 ) ) ;
#92582=CARTESIAN_POINT ( 'NONE',  ( 18.67979575497178502, 10.72451020669898547, 34.16557627198102409 ) ) ;
#92583=CARTESIAN_POINT ( 'NONE',  ( -18.62759615963255300, -10.81492255796106328, 89.16775706135236135 ) ) ;
#92584=CARTESIAN_POINT ( 'NONE',  ( 5.153800228976335163, 19.02544592524342804, 64.79057627198100988 ) ) ;
#92585=CARTESIAN_POINT ( 'NONE',  ( 16.46253265017160672, -9.564922557960803928, 23.33224293864769194 ) ) ;
#92586=CARTESIAN_POINT ( 'NONE',  ( 5.823673210054444382, -21.52544592524334988, 25.20942372801901854 ) ) ;
#92587=CARTESIAN_POINT ( 'NONE',  ( -17.97058386085787163, -5.500000000000059508, 49.00390968646215839 ) ) ;
#92588=CARTESIAN_POINT ( 'NONE',  ( 0.05219959533937995610, -21.53943276465977519, 40.00109039468567573 ) ) ;
#92589=CARTESIAN_POINT ( 'NONE',  ( 9.474510206698971260, -16.51473224551069308, 37.91557627198102409 ) ) ;
#92590=CARTESIAN_POINT ( 'NONE',  ( -21.52544592524343514, 5.823673210054127303, 106.0405762719810525 ) ) ;
#92591=CARTESIAN_POINT ( 'NONE',  ( 13.97604488694548053, -13.89961937509957401, 50.62609039468566152 ) ) ;
#92594=CARTESIAN_POINT ( 'NONE',  ( 16.55341960407618274, -4.379528057220086978, 61.04275706135234714 ) ) ;
#92595=CARTESIAN_POINT ( 'NONE',  ( 5.049401038298161559, -19.05341960407611168, 22.70724293864769194 ) ) ;
#92597=CARTESIAN_POINT ( 'NONE',  ( 16.46253265017160672, -9.564922557960803928, 78.33224293864769550 ) ) ;
#92598=CARTESIAN_POINT ( 'NONE',  ( 12.06949235617757843, -12.14591786802309237, 108.1239096053143811 ) ) ;
#92599=CARTESIAN_POINT ( 'NONE',  ( -18.67979575497178146, -10.72451020669898902, 56.66557627198103830 ) ) ;
#92600=CARTESIAN_POINT ( 'NONE',  ( 12.06949235617739724, 12.14591786802326823, 36.87609039468568994 ) ) ;
#92601=CARTESIAN_POINT ( 'NONE',  ( 18.62759615963255655, 10.81492255796105972, 101.6677570613523613 ) ) ;
#92602=CARTESIAN_POINT ( 'NONE',  ( -19.03943276465977164, 0.05219959533909376836, 21.24890960531436335 ) ) ;
#92603=CARTESIAN_POINT ( 'NONE',  ( -16.55341960407617563, 4.379528057220093196, 108.5427570613523756 ) ) ;
#92604=CARTESIAN_POINT ( 'NONE',  ( 14.29746914071049879, -8.314922557960816363, 58.33224293864768839 ) ) ;
#92605=CARTESIAN_POINT ( 'NONE',  ( -19.02544592524342804, 5.153800228976336051, 46.04057627198101699 ) ) ;
#92606=CARTESIAN_POINT ( 'NONE',  ( -10.72451020669870658, -18.67979575497194134, 99.58442372801900433 ) ) ;
#92607=CARTESIAN_POINT ( 'NONE',  ( -21.53943276465977519, 0.05219959533907696930, 106.2489096053143811 ) ) ;
#92608=CARTESIAN_POINT ( 'NONE',  ( 21.53943276465977519, 0.05219959533937863772, 76.25109039468568994 ) ) ;
#92609=CARTESIAN_POINT ( 'NONE',  ( -14.29746914071037622, -8.314922557961029526, 49.16775706135234003 ) ) ;
#92610=CARTESIAN_POINT ( 'NONE',  ( -0.05219959533910754901, -16.53943276465976808, 77.49890960531433848 ) ) ;
#92611=CARTESIAN_POINT ( 'NONE',  ( -10.72451020669870658, -18.67979575497194134, 99.58442372801900433 ) ) ;
#92612=CARTESIAN_POINT ( 'NONE',  ( 16.52544592524335698, 4.483927247898782831, 111.4594237280190328 ) ) ;
#92613=CARTESIAN_POINT ( 'NONE',  ( 17.50000000000000000, 5.499999999999992895, 71.70309617465829888 ) ) ;
#92614=CARTESIAN_POINT ( 'NONE',  ( 8.224510206698742110, 14.34966873604972548, 42.08442372801901854 ) ) ;
#92615=CARTESIAN_POINT ( 'NONE',  ( 4.483927247898545687, 16.52544592524342804, 44.79057627198103120 ) ) ;
#92616=CARTESIAN_POINT ( 'NONE',  ( 16.53943276465976808, 0.05219959533934440121, 81.25109039468568994 ) ) ;
#92617=CARTESIAN_POINT ( 'NONE',  ( -13.89961937509977652, 13.97604488694528158, 95.62390960531436690 ) ) ;
#92618=CARTESIAN_POINT ( 'NONE',  ( -15.80617190586745835, -15.72974639402198527, 21.87390960531436690 ) ) ;
#92619=CARTESIAN_POINT ( 'NONE',  ( -5.823673210054431948, 21.52544592524334988, 92.70942372801901854 ) ) ;
#92620=CARTESIAN_POINT ( 'NONE',  ( 16.52544592524335698, 4.483927247898782831, 96.45942372801901854 ) ) ;
#92621=CARTESIAN_POINT ( 'NONE',  ( -8.314922557960811034, -14.29746914071050412, 72.08224293864769550 ) ) ;
#92622=CARTESIAN_POINT ( 'NONE',  ( -13.97604488694527625, -13.89961937509977652, 86.87390960531436690 ) ) ;
#92624=CARTESIAN_POINT ( 'NONE',  ( -4.483927247898782831, 16.52544592524335698, 32.70942372801900433 ) ) ;
#92625=CARTESIAN_POINT ( 'NONE',  ( 9.474510206698971260, -16.51473224551069308, 42.91557627198103120 ) ) ;
#92626=CARTESIAN_POINT ( 'NONE',  ( 0.05219959533909260263, 19.03943276465977164, 89.99890960531436690 ) ) ;
#92627=CARTESIAN_POINT ( 'NONE',  ( -8.314922557961024197, 14.29746914071037800, 32.91775706135234714 ) ) ;
#92629=CARTESIAN_POINT ( 'NONE',  ( -19.03943276465977164, -0.05219959533935918106, 28.75109039468566507 ) ) ;
#92630=CARTESIAN_POINT ( 'NONE',  ( -4.379528057220086978, -16.55341960407618274, 94.79275706135234714 ) ) ;
#92631=CARTESIAN_POINT ( 'NONE',  ( 19.03943276465977164, -0.05219959533909143690, 28.74890960531435624 ) ) ;
#92632=CARTESIAN_POINT ( 'NONE',  ( 16.55341960407618274, -4.379528057220086978, 76.04275706135237556 ) ) ;
#92633=CARTESIAN_POINT ( 'NONE',  ( -8.224510206698735004, -14.34966873604973081, 64.58442372801900433 ) ) ;
#92634=CARTESIAN_POINT ( 'NONE',  ( -19.03943276465977164, -0.05219959533935918106, 88.75109039468567573 ) ) ;
#92635=CARTESIAN_POINT ( 'NONE',  ( -13.89961937509957401, -13.97604488694547875, 34.37609039468566863 ) ) ;
#92636=CARTESIAN_POINT ( 'NONE',  ( 13.97604488694527802, 13.89961937509977652, 49.37390960531434558 ) ) ;
#92637=CARTESIAN_POINT ( 'NONE',  ( -12.14591786802309592, -12.06949235617757132, 91.87390960531436690 ) ) ;
#92639=CARTESIAN_POINT ( 'NONE',  ( 19.02544592524334988, 5.153800228976608722, 51.45942372801900433 ) ) ;
#92640=CARTESIAN_POINT ( 'NONE',  ( 10.81492255796078972, 18.62759615963270932, 54.58224293864769550 ) ) ;
#92641=CARTESIAN_POINT ( 'NONE',  ( -16.51473224551082808, 9.474510206698731452, 28.33442372801900433 ) ) ;
#92642=CARTESIAN_POINT ( 'NONE',  ( 5.049401038298161559, -19.05341960407611168, 107.7072429386476955 ) ) ;
#92643=CARTESIAN_POINT ( 'NONE',  ( 15.72974639402199770, -15.80617190586745480, 78.12390960531436690 ) ) ;
#92644=CARTESIAN_POINT ( 'NONE',  ( 0.05219959533909260263, 19.03943276465977164, 114.9989096053143669 ) ) ;
#92645=CARTESIAN_POINT ( 'NONE',  ( -9.564922557961040184, 16.46253265017147172, 92.91775706135233293 ) ) ;
#92646=CARTESIAN_POINT ( 'NONE',  ( -17.50000000000001776, 4.658240926743198784, 108.9447041781680383 ) ) ;
#92647=CARTESIAN_POINT ( 'NONE',  ( -19.02544592524334988, -5.153800228976617603, 108.9594237280189759 ) ) ;
#92648=CARTESIAN_POINT ( 'NONE',  ( -9.474510206698964154, 16.51473224551069663, 35.41557627198102409 ) ) ;
#92649=CARTESIAN_POINT ( 'NONE',  ( -0.05219959533909027116, -19.03943276465977164, 92.49890960531436690 ) ) ;
#92650=CARTESIAN_POINT ( 'NONE',  ( 10.72451020669898902, -18.67979575497178502, 72.91557627198103830 ) ) ;
#92651=CARTESIAN_POINT ( 'NONE',  ( 8.314922557961029526, -14.29746914071037800, 50.41775706135235424 ) ) ;
#92652=CARTESIAN_POINT ( 'NONE',  ( -10.81492255796105439, 18.62759615963255655, 52.91775706135235424 ) ) ;
#92653=CARTESIAN_POINT ( 'NONE',  ( -13.97604488694547697, 13.89961937509957934, 103.1260903946856473 ) ) ;
#92654=CARTESIAN_POINT ( 'NONE',  ( 18.67979575497194134, -10.72451020669871369, 110.8344237280190043 ) ) ;
#92655=CARTESIAN_POINT ( 'NONE',  ( -4.379528057220086978, -16.55341960407618274, 104.7927570613523898 ) ) ;
#92656=CARTESIAN_POINT ( 'NONE',  ( 19.02544592524343514, -5.153800228976328945, 103.5405762719809957 ) ) ;
#92657=CARTESIAN_POINT ( 'NONE',  ( -15.80617190586745835, -15.72974639402198527, 106.8739096053143811 ) ) ;
#92658=CARTESIAN_POINT ( 'NONE',  ( 0.05219959533910956823, 16.53943276465976808, 29.99890960531435979 ) ) ;
#92659=CARTESIAN_POINT ( 'NONE',  ( -19.05341960407617563, 5.049401038297882671, 83.54275706135233293 ) ) ;
#92660=EDGE_CURVE ( 'NONE', #36339, #155869, #190145, .T. ) ;
#92661=CARTESIAN_POINT ( 'NONE',  ( 10.72451020669871369, 18.67979575497193778, 52.08442372801901854 ) ) ;
#92662=CARTESIAN_POINT ( 'NONE',  ( 19.02544592524334988, 5.153800228976608722, 31.45942372801900433 ) ) ;
#92663=CARTESIAN_POINT ( 'NONE',  ( -0.05219959533910754901, -16.53943276465976808, 107.4989096053143669 ) ) ;
#92664=CARTESIAN_POINT ( 'NONE',  ( 5.719274019375991003, -21.55341960407610458, 27.70724293864769905 ) ) ;
#92665=CARTESIAN_POINT ( 'NONE',  ( 16.52544592524342804, -4.483927247898539470, 23.54057627198102765 ) ) ;
#92666=CARTESIAN_POINT ( 'NONE',  ( 21.53943276465977519, 0.05219959533937863772, 101.2510903946856757 ) ) ;
#92667=CARTESIAN_POINT ( 'NONE',  ( -16.55341960407617563, 4.379528057220093196, 63.54275706135234003 ) ) ;
#92668=CARTESIAN_POINT ( 'NONE',  ( 14.29746914071049879, -8.314922557960816363, 33.33224293864769550 ) ) ;
#92669=CARTESIAN_POINT ( 'NONE',  ( -0.05219959533937732626, 21.53943276465977519, 67.50109039468568994 ) ) ;
#92670=CARTESIAN_POINT ( 'NONE',  ( 0.05219959533937995610, -21.53943276465977519, 50.00109039468568994 ) ) ;
#92672=CARTESIAN_POINT ( 'NONE',  ( -9.474510206698964154, 16.51473224551069663, 25.41557627198103120 ) ) ;
#92673=CARTESIAN_POINT ( 'NONE',  ( 21.53943276465977519, 0.05219959533937863772, 36.25109039468567573 ) ) ;
#92674=CARTESIAN_POINT ( 'NONE',  ( -4.379528057220328563, 16.55341960407611168, 105.2072429386477097 ) ) ;
#92675=CARTESIAN_POINT ( 'NONE',  ( 19.76836671444427651, 4.606730274327740737, 37.50000000000000711 ) ) ;
#92676=CARTESIAN_POINT ( 'NONE',  ( -16.52544592524342804, 4.483927247898546575, 81.04057627198102409 ) ) ;
#92677=CARTESIAN_POINT ( 'NONE',  ( 5.153800228976335163, 19.02544592524342804, 69.79057627198103830 ) ) ;
#92678=CARTESIAN_POINT ( 'NONE',  ( -8.224510206698948167, 14.34966873604960824, 25.41557627198103120 ) ) ;
#92679=CARTESIAN_POINT ( 'NONE',  ( -15.80617190586745835, -15.72974639402198527, 51.87390960531437401 ) ) ;
#92680=CARTESIAN_POINT ( 'NONE',  ( 4.483927247898545687, 16.52544592524342804, 94.79057627198105251 ) ) ;
#92681=CARTESIAN_POINT ( 'NONE',  ( -21.52544592524343514, 5.823673210054127303, 96.04057627198102409 ) ) ;
#92682=CARTESIAN_POINT ( 'NONE',  ( -13.97604488694527625, -13.89961937509977652, 101.8739096053143811 ) ) ;
#92683=CARTESIAN_POINT ( 'NONE',  ( -13.97604488694527625, -13.89961937509977652, 56.87390960531434558 ) ) ;
#92684=CARTESIAN_POINT ( 'NONE',  ( -16.51473224551082808, 9.474510206698731452, 103.3344237280190043 ) ) ;
#92685=CARTESIAN_POINT ( 'NONE',  ( -5.719274019375978568, 21.55341960407610458, 45.20724293864769550 ) ) ;
#92686=CARTESIAN_POINT ( 'NONE',  ( 10.81492255796106328, -18.62759615963255655, 75.41775706135233293 ) ) ;
#92687=CARTESIAN_POINT ( 'NONE',  ( 16.51473224551069308, 9.474510206698969483, 69.16557627198102409 ) ) ;
#92688=CARTESIAN_POINT ( 'NONE',  ( 16.46253265017160672, -9.564922557960803928, 98.33224293864769550 ) ) ;
#92689=CARTESIAN_POINT ( 'NONE',  ( -4.483927247898782831, 16.52544592524335698, 77.70942372801900433 ) ) ;
#92690=CARTESIAN_POINT ( 'NONE',  ( -15.80617190586768217, 15.72974639402176855, 63.12609039468568994 ) ) ;
#92691=CARTESIAN_POINT ( 'NONE',  ( 15.80617190586769283, -15.72974639402175789, 80.62609039468567573 ) ) ;
#92692=CARTESIAN_POINT ( 'NONE',  ( -0.05219959533907301413, -21.53943276465977519, 107.4989096053143669 ) ) ;
#92693=CARTESIAN_POINT ( 'NONE',  ( 0.05219959533934541429, -16.53943276465976808, 80.00109039468568994 ) ) ;
#92694=CARTESIAN_POINT ( 'NONE',  ( -5.823673210054116645, -21.52544592524344225, 82.29057627198103830 ) ) ;
#92695=CARTESIAN_POINT ( 'NONE',  ( 13.89961937509957401, 13.97604488694547697, 51.87609039468566863 ) ) ;
#92696=CARTESIAN_POINT ( 'NONE',  ( -10.81492255796078084, -18.62759615963271287, 37.08224293864768129 ) ) ;
#92697=CARTESIAN_POINT ( 'NONE',  ( 13.89961937509977652, -13.97604488694527269, 78.12390960531433848 ) ) ;
#92698=CARTESIAN_POINT ( 'NONE',  ( 12.06949235617739724, 12.14591786802326823, 111.8760903946856615 ) ) ;
#92699=CARTESIAN_POINT ( 'NONE',  ( -17.26058549869089731, 6.457015423128607878, 63.62254162523936429 ) ) ;
#92700=CARTESIAN_POINT ( 'NONE',  ( -0.05219959533907301413, -21.53943276465977519, 22.49890960531436335 ) ) ;
#92702=CARTESIAN_POINT ( 'NONE',  ( 5.153800228976615827, -19.02544592524334988, 100.2094237280190043 ) ) ;
#92703=CARTESIAN_POINT ( 'NONE',  ( -0.05219959533907301413, -21.53943276465977519, 67.49890960531436690 ) ) ;
#92704=CARTESIAN_POINT ( 'NONE',  ( -12.14591786802309592, -12.06949235617757132, 46.87390960531435979 ) ) ;
#92705=CARTESIAN_POINT ( 'NONE',  ( -16.53943276465976808, -0.05219959533934237506, 18.75109039468568639 ) ) ;
#92706=CARTESIAN_POINT ( 'NONE',  ( 0.05219959533909260263, 19.03943276465977164, 29.99890960531435979 ) ) ;
#92707=CARTESIAN_POINT ( 'NONE',  ( 9.564922557961047289, -16.46253265017146816, 110.4177570613523471 ) ) ;
#92708=CARTESIAN_POINT ( 'NONE',  ( 15.80617190586746368, 15.72974639402197994, 104.3739096053143669 ) ) ;
#92709=CARTESIAN_POINT ( 'NONE',  ( 5.153800228976615827, -19.02544592524334988, 70.20942372801899012 ) ) ;
#92710=CARTESIAN_POINT ( 'NONE',  ( -14.29746914071037622, -8.314922557961029526, 79.16775706135234714 ) ) ;
#92711=CARTESIAN_POINT ( 'NONE',  ( -19.03943276465977164, 0.05219959533909376836, 86.24890960531436690 ) ) ;
#92712=CARTESIAN_POINT ( 'NONE',  ( -16.53943276465976808, 0.05219959533911058130, 71.24890960531435269 ) ) ;
#92713=CARTESIAN_POINT ( 'NONE',  ( -19.03943276465977164, 0.05219959533909376836, 66.24890960531436690 ) ) ;
#92714=CARTESIAN_POINT ( 'NONE',  ( 12.06949235617757843, -12.14591786802309237, 68.12390960531436690 ) ) ;
#92715=CARTESIAN_POINT ( 'NONE',  ( -13.97604488694527625, -13.89961937509977652, 26.87390960531434558 ) ) ;
#92717=CARTESIAN_POINT ( 'NONE',  ( -16.52544592524342804, 4.483927247898546575, 41.04057627198103120 ) ) ;
#92718=CARTESIAN_POINT ( 'NONE',  ( 9.474510206698971260, -16.51473224551069308, 77.91557627198103830 ) ) ;
#92719=DIRECTION ( 'NONE',  ( -0.000000000000000000, -0.000000000000000000, 1.000000000000000000 ) ) ;
#92720=CARTESIAN_POINT ( 'NONE',  ( 19.05341960407617918, -5.049401038297876454, 51.04275706135231871 ) ) ;
#92721=CARTESIAN_POINT ( 'NONE',  ( -12.14591786802326823, 12.06949235617739902, 58.12609039468568994 ) ) ;
#92722=CARTESIAN_POINT ( 'NONE',  ( 21.52544592524344225, -5.823673210054117533, 63.54057627198103830 ) ) ;
#92723=CARTESIAN_POINT ( 'NONE',  ( -19.03943276465977164, -0.05219959533935918106, 28.75109039468566507 ) ) ;
#92724=CARTESIAN_POINT ( 'NONE',  ( 16.51473224551069308, 9.474510206698969483, 84.16557627198102409 ) ) ;
#92726=CARTESIAN_POINT ( 'NONE',  ( 21.52544592524344225, -5.823673210054117533, 33.54057627198102409 ) ) ;
#92727=CARTESIAN_POINT ( 'NONE',  ( 19.05341960407611168, 5.049401038298154454, 63.95724293864769550 ) ) ;
#92728=CARTESIAN_POINT ( 'NONE',  ( 5.719274019375673035, 21.55341960407619339, 57.29275706135234714 ) ) ;
#92729=CARTESIAN_POINT ( 'NONE',  ( 12.06949235617757843, -12.14591786802309237, 103.1239096053143811 ) ) ;
#92731=CARTESIAN_POINT ( 'NONE',  ( 10.72451020669898902, -18.67979575497178502, 97.91557627198103830 ) ) ;
#92732=CARTESIAN_POINT ( 'NONE',  ( -16.46253265017160317, 9.564922557960807481, 100.8322429386477097 ) ) ;
#92734=CARTESIAN_POINT ( 'NONE',  ( -10.81492255796105439, 18.62759615963255655, 37.91775706135235424 ) ) ;
#92735=EDGE_LOOP ( 'NONE', ( #30399, #26780, #121791, #64939 ) ) ;
#92736=CARTESIAN_POINT ( 'NONE',  ( 16.46253265017160672, -9.564922557960803928, 98.33224293864769550 ) ) ;
#92738=CARTESIAN_POINT ( 'NONE',  ( -15.72974639402197994, 15.80617190586746368, 100.6239096053143811 ) ) ;
#92739=CARTESIAN_POINT ( 'NONE',  ( -16.51473224551069308, -9.474510206698971260, 41.66557627198103120 ) ) ;
#92740=CARTESIAN_POINT ( 'NONE',  ( -0.05219959533934338120, 16.53943276465976808, 22.50109039468567573 ) ) ;
#92742=CARTESIAN_POINT ( 'NONE',  ( 9.474510206698971260, -16.51473224551069308, 32.91557627198102409 ) ) ;
#92743=CARTESIAN_POINT ( 'NONE',  ( 5.823673210054444382, -21.52544592524334988, 80.20942372801901854 ) ) ;
#92744=CARTESIAN_POINT ( 'NONE',  ( 13.97604488694527802, 13.89961937509977652, 74.37390960531436690 ) ) ;
#92745=CARTESIAN_POINT ( 'NONE',  ( -10.81492255796105439, 18.62759615963255655, 42.91775706135235424 ) ) ;
#92746=CARTESIAN_POINT ( 'NONE',  ( 18.62759615963255655, 10.81492255796105972, 31.66775706135234358 ) ) ;
#92748=CARTESIAN_POINT ( 'NONE',  ( 19.03943276465977164, -0.05219959533909143690, 93.74890960531435269 ) ) ;
#92750=CARTESIAN_POINT ( 'NONE',  ( -8.224510206698735004, -14.34966873604973081, 39.58442372801901143 ) ) ;
#92751=CARTESIAN_POINT ( 'NONE',  ( -16.52544592524335698, -4.483927247898792601, 68.95942372801901854 ) ) ;
#92752=CARTESIAN_POINT ( 'NONE',  ( -21.55341960407619339, 5.719274019375674811, 58.54275706135235424 ) ) ;
#92753=CARTESIAN_POINT ( 'NONE',  ( -15.72974639402176322, -15.80617190586768395, 79.37609039468567573 ) ) ;
#92755=CARTESIAN_POINT ( 'NONE',  ( 19.05341960407617918, -5.049401038297876454, 111.0427570613523329 ) ) ;
#92756=CARTESIAN_POINT ( 'NONE',  ( 19.03943276465977164, -0.05219959533909143690, 73.74890960531435269 ) ) ;
#92757=CARTESIAN_POINT ( 'NONE',  ( 13.97604488694527802, 13.89961937509977652, 99.37390960531436690 ) ) ;
#92758=CARTESIAN_POINT ( 'NONE',  ( 16.53943276465976808, -0.05219959533910856209, 103.7489096053143669 ) ) ;
#92759=CARTESIAN_POINT ( 'NONE',  ( 12.14591786802309770, 12.06949235617756955, 104.3739096053143669 ) ) ;
#92760=CARTESIAN_POINT ( 'NONE',  ( -5.719274019375978568, 21.55341960407610458, 35.20724293864768839 ) ) ;
#92761=CARTESIAN_POINT ( 'NONE',  ( -16.55341960407617563, 4.379528057220093196, 78.54275706135236135 ) ) ;
#92762=CARTESIAN_POINT ( 'NONE',  ( -16.53943276465976808, 0.05219959533911058130, 71.24890960531435269 ) ) ;
#92763=CARTESIAN_POINT ( 'NONE',  ( -5.153800228976328057, -19.02544592524343514, 57.29057627198103120 ) ) ;
#92764=CARTESIAN_POINT ( 'NONE',  ( -10.81492255796105439, 18.62759615963255655, 72.91775706135234714 ) ) ;
#92765=CARTESIAN_POINT ( 'NONE',  ( -10.81492255796105439, 18.62759615963255655, 72.91775706135234714 ) ) ;
#92766=CARTESIAN_POINT ( 'NONE',  ( 0.05219959533936267826, -19.03943276465977164, 110.0010903946856757 ) ) ;
#92767=CARTESIAN_POINT ( 'NONE',  ( 4.379528057220339221, -16.55341960407611168, 72.70724293864769550 ) ) ;
#92768=CARTESIAN_POINT ( 'NONE',  ( -10.72451020669870658, -18.67979575497194134, 24.58442372801901499 ) ) ;
#92769=CARTESIAN_POINT ( 'NONE',  ( -10.72451020669898014, 18.67979575497178502, 65.41557627198102409 ) ) ;
#92772=CARTESIAN_POINT ( 'NONE',  ( -19.02544592524342804, 5.153800228976336051, 76.04057627198102409 ) ) ;
#92773=CARTESIAN_POINT ( 'NONE',  ( -16.55341960407611168, -4.379528057220339221, 46.45724293864769550 ) ) ;
#92775=CARTESIAN_POINT ( 'NONE',  ( -4.379528057220328563, 16.55341960407611168, 25.20724293864769550 ) ) ;
#92776=CARTESIAN_POINT ( 'NONE',  ( -12.06949235617739369, -12.14591786802326823, 94.37609039468568994 ) ) ;
#92777=CARTESIAN_POINT ( 'NONE',  ( -9.564922557961040184, 16.46253265017147172, 57.91775706135233293 ) ) ;
#92779=CARTESIAN_POINT ( 'NONE',  ( -0.05219959533909027116, -19.03943276465977164, 107.4989096053143527 ) ) ;
#92780=CARTESIAN_POINT ( 'NONE',  ( 14.34966873604960469, 8.224510206698951720, 79.16557627198103830 ) ) ;
#92781=CARTESIAN_POINT ( 'NONE',  ( 9.474510206698729675, 16.51473224551082808, 47.08442372801900433 ) ) ;
#92782=CARTESIAN_POINT ( 'NONE',  ( 0.05219959533909260263, 19.03943276465977164, 34.99890960531435979 ) ) ;
#92783=CARTESIAN_POINT ( 'NONE',  ( -10.81492255796078084, -18.62759615963271287, 37.08224293864768129 ) ) ;
#92784=CARTESIAN_POINT ( 'NONE',  ( 18.62759615963271287, -10.81492255796078972, 48.33224293864770260 ) ) ;
#92785=ORIENTED_EDGE ( 'NONE', *, *, #8686, .F. ) ;
#92786=CARTESIAN_POINT ( 'NONE',  ( 12.14591786802309770, 12.06949235617756955, 104.3739096053143669 ) ) ;
#92787=CARTESIAN_POINT ( 'NONE',  ( 16.52544592524335698, 4.483927247898782831, 46.45942372801901854 ) ) ;
#92788=CARTESIAN_POINT ( 'NONE',  ( -0.05219959533910754901, -16.53943276465976808, 97.49890960531436690 ) ) ;
#92789=CARTESIAN_POINT ( 'NONE',  ( 17.50000000000000000, -5.622605283950865562, 36.18792689403888119 ) ) ;
#92790=CARTESIAN_POINT ( 'NONE',  ( -17.13100169013300089, 6.664070546373151771, 50.76789835699851494 ) ) ;
#92791=CARTESIAN_POINT ( 'NONE',  ( 5.823673210054125526, 21.52544592524343514, 39.79057627198103830 ) ) ;
#92792=CARTESIAN_POINT ( 'NONE',  ( 17.72517630440433223, -5.499999999999963585, 78.42175719257211597 ) ) ;
#92794=CARTESIAN_POINT ( 'NONE',  ( 8.314922557961029526, -14.29746914071037800, 45.41775706135234003 ) ) ;
#92795=CARTESIAN_POINT ( 'NONE',  ( -4.379528057220328563, 16.55341960407611168, 25.20724293864769550 ) ) ;
#92796=CARTESIAN_POINT ( 'NONE',  ( 21.53943276465977519, -0.05219959533907433946, 58.74890960531436690 ) ) ;
#92797=CARTESIAN_POINT ( 'NONE',  ( -19.05341960407617563, 5.049401038297882671, 78.54275706135233293 ) ) ;
#92798=CARTESIAN_POINT ( 'NONE',  ( 18.67979575497178502, 10.72451020669898547, 59.16557627198103120 ) ) ;
#92799=CARTESIAN_POINT ( 'NONE',  ( -0.05219959533937732626, 21.53943276465977519, 77.50109039468567573 ) ) ;
#92801=CARTESIAN_POINT ( 'NONE',  ( -4.483927247898782831, 16.52544592524335698, 42.70942372801901854 ) ) ;
#92802=CARTESIAN_POINT ( 'NONE',  ( -19.03943276465977164, 0.05219959533909376836, 31.24890960531435979 ) ) ;
#92803=CARTESIAN_POINT ( 'NONE',  ( 9.474510206698971260, -16.51473224551069308, 102.9155762719810241 ) ) ;
#92805=CARTESIAN_POINT ( 'NONE',  ( -19.02544592524342804, 5.153800228976336051, 31.04057627198102409 ) ) ;
#92806=CARTESIAN_POINT ( 'NONE',  ( -12.14591786802309592, -12.06949235617757132, 96.87390960531436690 ) ) ;
#92808=FACE_BOUND ( 'NONE', #200065, .T. ) ;
#92810=CARTESIAN_POINT ( 'NONE',  ( -16.53943276465976808, -0.05219959533934237506, 68.75109039468568994 ) ) ;
#92811=CARTESIAN_POINT ( 'NONE',  ( -0.05219959533907301413, -21.53943276465977519, 97.49890960531436690 ) ) ;
#92812=CARTESIAN_POINT ( 'NONE',  ( -16.46253265017160317, 9.564922557960807481, 60.83224293864769550 ) ) ;
#92813=CARTESIAN_POINT ( 'NONE',  ( 5.719274019375673035, 21.55341960407619339, 32.29275706135235424 ) ) ;
#92814=CARTESIAN_POINT ( 'NONE',  ( 13.89961937509977652, -13.97604488694527269, 78.12390960531433848 ) ) ;
#92817=CARTESIAN_POINT ( 'NONE',  ( -5.719274019375665041, -21.55341960407619695, 19.79275706135235069 ) ) ;
#92818=CARTESIAN_POINT ( 'NONE',  ( -5.049401038298153566, 19.05341960407611168, 25.20724293864768484 ) ) ;
#92819=CARTESIAN_POINT ( 'NONE',  ( 19.05341960407611168, 5.049401038298154454, 103.9572429386476671 ) ) ;
#92820=CARTESIAN_POINT ( 'NONE',  ( -0.05219959533936034679, 19.03943276465977164, 72.50109039468566152 ) ) ;
#92821=CARTESIAN_POINT ( 'NONE',  ( -19.03943276465977164, -0.05219959533935918106, 28.75109039468566507 ) ) ;
#92822=CARTESIAN_POINT ( 'NONE',  ( -5.719274019375978568, 21.55341960407610458, 105.2072429386477097 ) ) ;
#92823=CARTESIAN_POINT ( 'NONE',  ( -9.474510206698720793, -16.51473224551083518, 39.58442372801899722 ) ) ;
#92824=CARTESIAN_POINT ( 'NONE',  ( -14.34966873604972548, 8.224510206698743886, 83.33442372801903275 ) ) ;
#92825=CARTESIAN_POINT ( 'NONE',  ( -19.03943276465977164, 0.05219959533909376836, 106.2489096053143669 ) ) ;
#92826=CARTESIAN_POINT ( 'NONE',  ( -5.049401038298153566, 19.05341960407611168, 65.20724293864765286 ) ) ;
#92828=CARTESIAN_POINT ( 'NONE',  ( -18.67979575497193778, 10.72451020669871902, 63.33442372801900433 ) ) ;
#92829=CARTESIAN_POINT ( 'NONE',  ( 15.72974639402176855, 15.80617190586768217, 76.87609039468567573 ) ) ;
#92830=CARTESIAN_POINT ( 'NONE',  ( 5.153800228976335163, 19.02544592524342804, 74.79057627198103830 ) ) ;
#92831=CARTESIAN_POINT ( 'NONE',  ( 0.05219959533937995610, -21.53943276465977519, 50.00109039468568994 ) ) ;
#92832=CARTESIAN_POINT ( 'NONE',  ( -13.89961937509957401, -13.97604488694547875, 84.37609039468567573 ) ) ;
#92833=CARTESIAN_POINT ( 'NONE',  ( 0.05219959533909260263, 19.03943276465977164, 49.99890960531435979 ) ) ;
#92834=CARTESIAN_POINT ( 'NONE',  ( -5.153800228976328057, -19.02544592524343514, 92.29057627198099567 ) ) ;
#92835=CARTESIAN_POINT ( 'NONE',  ( 19.03943276465977164, -0.05219959533909143690, 63.74890960531435979 ) ) ;
#92836=CARTESIAN_POINT ( 'NONE',  ( -17.31747979337952259, -6.344076630960987728, 91.37944868065187620 ) ) ;
#92837=CARTESIAN_POINT ( 'NONE',  ( -0.05219959533909027116, -19.03943276465977164, 47.49890960531435979 ) ) ;
#92838=CARTESIAN_POINT ( 'NONE',  ( 21.53943276465977519, -0.05219959533907433946, 103.7489096053143669 ) ) ;
#92839=CARTESIAN_POINT ( 'NONE',  ( -14.29746914071037622, -8.314922557961029526, 89.16775706135236135 ) ) ;
#92841=CARTESIAN_POINT ( 'NONE',  ( -19.05341960407617563, 5.049401038297882671, 38.54275706135233293 ) ) ;
#92842=CARTESIAN_POINT ( 'NONE',  ( 19.02544592524343514, -5.153800228976328945, 68.54057627198103830 ) ) ;
#92843=CARTESIAN_POINT ( 'NONE',  ( -16.52544592524342804, 4.483927247898546575, 61.04057627198103120 ) ) ;
#92844=CARTESIAN_POINT ( 'NONE',  ( -12.06949235617756955, 12.14591786802309770, 95.62390960531436690 ) ) ;
#92845=CARTESIAN_POINT ( 'NONE',  ( -9.474510206698964154, 16.51473224551069663, 110.4155762719810383 ) ) ;
#92846=CARTESIAN_POINT ( 'NONE',  ( 19.02544592524343514, -5.153800228976328945, 88.54057627198102409 ) ) ;
#92847=CARTESIAN_POINT ( 'NONE',  ( -5.049401038298153566, 19.05341960407611168, 100.2072429386476955 ) ) ;
#92848=CARTESIAN_POINT ( 'NONE',  ( -16.46253265017146816, -9.564922557961047289, 19.16775706135233293 ) ) ;
#92849=CARTESIAN_POINT ( 'NONE',  ( -12.14591786802326823, 12.06949235617739902, 98.12609039468570415 ) ) ;
#92850=CARTESIAN_POINT ( 'NONE',  ( 19.05341960407611168, 5.049401038298154454, 73.95724293864768129 ) ) ;
#92851=CARTESIAN_POINT ( 'NONE',  ( 5.823673210054444382, -21.52544592524334988, 45.20942372801901854 ) ) ;
#92852=CARTESIAN_POINT ( 'NONE',  ( -5.719274019375978568, 21.55341960407610458, 25.20724293864769550 ) ) ;
#92853=CARTESIAN_POINT ( 'NONE',  ( 10.81492255796078972, 18.62759615963270932, 114.5822429386477097 ) ) ;
#92854=CARTESIAN_POINT ( 'NONE',  ( -12.06949235617756955, 12.14591786802309770, 60.62390960531437401 ) ) ;
#92855=CARTESIAN_POINT ( 'NONE',  ( 19.05341960407611168, 5.049401038298154454, 58.95724293864768129 ) ) ;
#92856=CARTESIAN_POINT ( 'NONE',  ( -14.34966873604960291, -8.224510206698953496, 76.66557627198103830 ) ) ;
#92857=CARTESIAN_POINT ( 'NONE',  ( 19.02544592524334988, 5.153800228976608722, 46.45942372801899012 ) ) ;
#92858=CARTESIAN_POINT ( 'NONE',  ( -14.34966873604960291, -8.224510206698953496, 111.6655762719810525 ) ) ;
#92859=CARTESIAN_POINT ( 'NONE',  ( -13.97604488694527625, -13.89961937509977652, 81.87390960531436690 ) ) ;
#92860=CARTESIAN_POINT ( 'NONE',  ( -16.46253265017160317, 9.564922557960807481, 85.83224293864769550 ) ) ;
#92862=CARTESIAN_POINT ( 'NONE',  ( -16.55341960407611168, -4.379528057220339221, 96.45724293864770971 ) ) ;
#92863=VERTEX_POINT ( 'NONE', #49380 ) ;
#92864=CARTESIAN_POINT ( 'NONE',  ( -14.29746914071037622, -8.314922557961029526, 104.1677570613523471 ) ) ;
#92865=CARTESIAN_POINT ( 'NONE',  ( -4.483927247898782831, 16.52544592524335698, 27.70942372801901854 ) ) ;
#92866=CARTESIAN_POINT ( 'NONE',  ( 18.62759615963255655, 10.81492255796105972, 91.66775706135234714 ) ) ;
#92867=CARTESIAN_POINT ( 'NONE',  ( 16.51473224551069308, 9.474510206698969483, 84.16557627198102409 ) ) ;
#92868=CARTESIAN_POINT ( 'NONE',  ( 15.80617190586769283, -15.72974639402175789, 20.62609039468568639 ) ) ;
#92869=CARTESIAN_POINT ( 'NONE',  ( -19.03943276465977164, 0.05219959533909376836, 36.24890960531436690 ) ) ;
#92870=CARTESIAN_POINT ( 'NONE',  ( -14.34966873604972548, 8.224510206698743886, 28.33442372801902209 ) ) ;
#92871=CARTESIAN_POINT ( 'NONE',  ( -16.46253265017146816, -9.564922557961047289, 94.16775706135233293 ) ) ;
#92872=CARTESIAN_POINT ( 'NONE',  ( -15.72974639402197994, 15.80617190586746368, 95.62390960531436690 ) ) ;
#92873=CARTESIAN_POINT ( 'NONE',  ( 16.46253265017146816, 9.564922557961045513, 71.66775706135233293 ) ) ;
#92874=CARTESIAN_POINT ( 'NONE',  ( 0.05219959533909260263, 19.03943276465977164, 24.99890960531435269 ) ) ;
#92875=CARTESIAN_POINT ( 'NONE',  ( 0.05219959533907565091, 21.53943276465977519, 114.9989096053143669 ) ) ;
#92876=CARTESIAN_POINT ( 'NONE',  ( 17.58332526062529411, -7.635886036038496805, 73.42334959558466778 ) ) ;
#92877=CARTESIAN_POINT ( 'NONE',  ( -13.97604488694527625, -13.89961937509977652, 96.87390960531433848 ) ) ;
#92878=CARTESIAN_POINT ( 'NONE',  ( 8.224510206698742110, 14.34966873604972548, 52.08442372801901854 ) ) ;
#92880=CARTESIAN_POINT ( 'NONE',  ( -13.89961937509957401, -13.97604488694547875, 54.37609039468565442 ) ) ;
#92881=CARTESIAN_POINT ( 'NONE',  ( -10.81492255796105439, 18.62759615963255655, 22.91775706135235069 ) ) ;
#92882=CARTESIAN_POINT ( 'NONE',  ( 12.06949235617757843, -12.14591786802309237, 78.12390960531436690 ) ) ;
#92883=CARTESIAN_POINT ( 'NONE',  ( 19.02544592524343514, -5.153800228976328945, 83.54057627198100988 ) ) ;
#92884=CARTESIAN_POINT ( 'NONE',  ( -4.483927247898782831, 16.52544592524335698, 52.70942372801902565 ) ) ;
#92885=CARTESIAN_POINT ( 'NONE',  ( 5.153800228976615827, -19.02544592524334988, 55.20942372801899722 ) ) ;
#92886=CARTESIAN_POINT ( 'NONE',  ( -10.81492255796105439, 18.62759615963255655, 67.91775706135234714 ) ) ;
#92887=CARTESIAN_POINT ( 'NONE',  ( 14.29746914071037800, 8.314922557961029526, 26.66775706135235424 ) ) ;
#92888=CARTESIAN_POINT ( 'NONE',  ( 19.05341960407611168, 5.049401038298154454, 73.95724293864768129 ) ) ;
#92890=CARTESIAN_POINT ( 'NONE',  ( 9.564922557961047289, -16.46253265017146816, 85.41775706135233293 ) ) ;
#92891=CARTESIAN_POINT ( 'NONE',  ( -0.05219959533934338120, 16.53943276465976808, 57.50109039468568994 ) ) ;
#92892=CARTESIAN_POINT ( 'NONE',  ( -5.719274019375665041, -21.55341960407619695, 99.79275706135234714 ) ) ;
#92893=CARTESIAN_POINT ( 'NONE',  ( 19.02544592524334988, 5.153800228976608722, 76.45942372801897591 ) ) ;
#92894=CARTESIAN_POINT ( 'NONE',  ( 13.97604488694527802, 13.89961937509977652, 44.37390960531435269 ) ) ;
#92895=CARTESIAN_POINT ( 'NONE',  ( -10.72451020669898014, 18.67979575497178502, 65.41557627198102409 ) ) ;
#92896=CARTESIAN_POINT ( 'NONE',  ( 4.483927247898545687, 16.52544592524342804, 79.79057627198102409 ) ) ;
#92897=CARTESIAN_POINT ( 'NONE',  ( 0.05219959533936267826, -19.03943276465977164, 75.00109039468566152 ) ) ;
#92898=CARTESIAN_POINT ( 'NONE',  ( 16.36317988757059894, -7.306389748694854802, 61.59789608363229974 ) ) ;
#92899=CARTESIAN_POINT ( 'NONE',  ( -9.564922557961040184, 16.46253265017147172, 47.91775706135233293 ) ) ;
#92900=CARTESIAN_POINT ( 'NONE',  ( -12.14591786802326823, 12.06949235617739902, 93.12609039468568994 ) ) ;
#92901=CARTESIAN_POINT ( 'NONE',  ( 16.52544592524342804, -4.483927247898539470, 73.54057627198102409 ) ) ;
#92902=CARTESIAN_POINT ( 'NONE',  ( 15.72974639402176855, 15.80617190586768217, 101.8760903946857042 ) ) ;
#92904=CARTESIAN_POINT ( 'NONE',  ( 18.67979575497178502, 10.72451020669898547, 104.1655762719810241 ) ) ;
#92905=CARTESIAN_POINT ( 'NONE',  ( 16.51473224551069308, 9.474510206698969483, 59.16557627198102409 ) ) ;
#92906=CARTESIAN_POINT ( 'NONE',  ( 10.72451020669871369, 18.67979575497193778, 82.08442372801901854 ) ) ;
#92907=CARTESIAN_POINT ( 'NONE',  ( -19.02544592524342804, 5.153800228976336051, 56.04057627198100988 ) ) ;
#92908=ORIENTED_EDGE ( 'NONE', *, *, #120239, .T. ) ;
#92909=CARTESIAN_POINT ( 'NONE',  ( -13.89961937509977652, 13.97604488694528158, 30.62390960531435269 ) ) ;
#92910=CARTESIAN_POINT ( 'NONE',  ( -9.474510206698964154, 16.51473224551069663, 110.4155762719810383 ) ) ;
#92911=CARTESIAN_POINT ( 'NONE',  ( 14.34966873604960469, 8.224510206698951720, 69.16557627198102409 ) ) ;
#92912=CARTESIAN_POINT ( 'NONE',  ( -19.02544592524342804, 5.153800228976336051, 31.04057627198102409 ) ) ;
#92913=CARTESIAN_POINT ( 'NONE',  ( 16.55341960407611168, 4.379528057220329451, 83.95724293864770971 ) ) ;
#92915=CARTESIAN_POINT ( 'NONE',  ( -21.55341960407610458, -5.719274019375992779, 91.45724293864769550 ) ) ;
#92916=CARTESIAN_POINT ( 'NONE',  ( -5.823673210054431948, 21.52544592524334988, 42.70942372801901854 ) ) ;
#92917=CARTESIAN_POINT ( 'NONE',  ( -19.05341960407611168, -5.049401038298163336, 21.45724293864768839 ) ) ;
#92918=CARTESIAN_POINT ( 'NONE',  ( 8.314922557961029526, -14.29746914071037800, 50.41775706135235424 ) ) ;
#92919=CARTESIAN_POINT ( 'NONE',  ( 21.52544592524344225, -5.823673210054117533, 98.54057627198105251 ) ) ;
#92920=CARTESIAN_POINT ( 'NONE',  ( -16.51473224551082808, 9.474510206698731452, 28.33442372801900433 ) ) ;
#92921=CARTESIAN_POINT ( 'NONE',  ( 9.474510206698971260, -16.51473224551069308, 112.9155762719810383 ) ) ;
#92922=CARTESIAN_POINT ( 'NONE',  ( 5.823673210054444382, -21.52544592524334988, 45.20942372801901854 ) ) ;
#92923=CARTESIAN_POINT ( 'NONE',  ( -5.823673210054116645, -21.52544592524344225, 42.29057627198103120 ) ) ;
#92924=CARTESIAN_POINT ( 'NONE',  ( 8.224510206698953496, -14.34966873604960469, 27.91557627198103830 ) ) ;
#92925=CARTESIAN_POINT ( 'NONE',  ( -21.55341960407619339, 5.719274019375674811, 68.54275706135234714 ) ) ;
#92926=CARTESIAN_POINT ( 'NONE',  ( 21.55341960407619695, -5.719274019375665929, 101.0427570613523756 ) ) ;
#92927=CARTESIAN_POINT ( 'NONE',  ( 19.02544592524334988, 5.153800228976608722, 26.45942372801899722 ) ) ;
#92928=CARTESIAN_POINT ( 'NONE',  ( 4.379528057220092307, 16.55341960407617563, 82.29275706135234714 ) ) ;
#92929=CARTESIAN_POINT ( 'NONE',  ( -10.72451020669870658, -18.67979575497194134, 54.58442372801901143 ) ) ;
#92930=CARTESIAN_POINT ( 'NONE',  ( -16.46253265017160317, 9.564922557960807481, 40.83224293864769550 ) ) ;
#92931=CARTESIAN_POINT ( 'NONE',  ( 16.51473224551083163, -9.474510206698727899, 20.83442372801899722 ) ) ;
#92932=CARTESIAN_POINT ( 'NONE',  ( -15.80617190586745835, -15.72974639402198527, 26.87390960531435979 ) ) ;
#92933=CARTESIAN_POINT ( 'NONE',  ( -15.72974639402197994, 15.80617190586746368, 115.6239096053143669 ) ) ;
#92934=CARTESIAN_POINT ( 'NONE',  ( 18.62759615963271287, -10.81492255796078972, 73.33224293864769550 ) ) ;
#92935=CARTESIAN_POINT ( 'NONE',  ( -16.55341960407617563, 4.379528057220093196, 43.54275706135235424 ) ) ;
#92937=CARTESIAN_POINT ( 'NONE',  ( -21.52544592524343514, 5.823673210054127303, 86.04057627198102409 ) ) ;
#92938=CARTESIAN_POINT ( 'NONE',  ( -8.224510206698735004, -14.34966873604973081, 64.58442372801900433 ) ) ;
#92939=CARTESIAN_POINT ( 'NONE',  ( 14.29746914071049879, -8.314922557960816363, 68.33224293864769550 ) ) ;
#92941=CARTESIAN_POINT ( 'NONE',  ( -9.474510206698720793, -16.51473224551083518, 104.5844237280190043 ) ) ;
#92942=CARTESIAN_POINT ( 'NONE',  ( 16.51473224551069308, 9.474510206698969483, 114.1655762719810241 ) ) ;
#92943=VECTOR ( 'NONE', #2867, 1000.000000000000000 ) ;
#92945=CARTESIAN_POINT ( 'NONE',  ( 4.379528057220092307, 16.55341960407617563, 42.29275706135235424 ) ) ;
#92946=CARTESIAN_POINT ( 'NONE',  ( -0.05219959533907301413, -21.53943276465977519, 107.4989096053143669 ) ) ;
#92947=CARTESIAN_POINT ( 'NONE',  ( -15.72974639402197994, 15.80617190586746368, 25.62390960531435624 ) ) ;
#92948=CARTESIAN_POINT ( 'NONE',  ( 4.379528057220092307, 16.55341960407617563, 57.29275706135234714 ) ) ;
#92949=CARTESIAN_POINT ( 'NONE',  ( -9.564922557960796823, -16.46253265017161027, 67.08224293864769550 ) ) ;
#92950=CARTESIAN_POINT ( 'NONE',  ( -15.80617190586768217, 15.72974639402176855, 48.12609039468568284 ) ) ;
#92951=CARTESIAN_POINT ( 'NONE',  ( 19.03943276465977164, 0.05219959533936151252, 106.2510903946856615 ) ) ;
#92952=CARTESIAN_POINT ( 'NONE',  ( -21.53943276465977519, 0.05219959533907696930, 31.24890960531435979 ) ) ;
#92954=CARTESIAN_POINT ( 'NONE',  ( 19.05341960407617918, -5.049401038297876454, 26.04275706135233293 ) ) ;
#92955=CARTESIAN_POINT ( 'NONE',  ( 16.52544592524335698, 4.483927247898782831, 41.45942372801901143 ) ) ;
#92956=CARTESIAN_POINT ( 'NONE',  ( 5.153800228976335163, 19.02544592524342804, 94.79057627198103830 ) ) ;
#92957=CARTESIAN_POINT ( 'NONE',  ( -10.72451020669898014, 18.67979575497178502, 100.4155762719810241 ) ) ;
#92958=CARTESIAN_POINT ( 'NONE',  ( 13.89961937509977652, -13.97604488694527269, 73.12390960531436690 ) ) ;
#92959=CARTESIAN_POINT ( 'NONE',  ( -30.00000000000000000, 5.499999999999992895, 102.5000000000000142 ) ) ;
#92960=CARTESIAN_POINT ( 'NONE',  ( -16.53943276465976808, 0.05219959533911058130, 86.24890960531436690 ) ) ;
#92961=CARTESIAN_POINT ( 'NONE',  ( -21.53943276465977519, 0.05219959533907696930, 36.24890960531435979 ) ) ;
#92962=CARTESIAN_POINT ( 'NONE',  ( 16.51473224551069308, 9.474510206698969483, 24.16557627198102765 ) ) ;
#92963=CARTESIAN_POINT ( 'NONE',  ( -14.34966873604972548, 8.224510206698743886, 68.33442372801900433 ) ) ;
#92964=CARTESIAN_POINT ( 'NONE',  ( -18.67979575497178146, -10.72451020669898902, 101.6655762719810383 ) ) ;
#92965=CARTESIAN_POINT ( 'NONE',  ( -19.02544592524334988, -5.153800228976617603, 68.95942372801896170 ) ) ;
#92966=CARTESIAN_POINT ( 'NONE',  ( 15.72974639402199770, -15.80617190586745480, 28.12390960531435979 ) ) ;
#92967=CARTESIAN_POINT ( 'NONE',  ( -19.03943276465977164, 0.05219959533909376836, 21.24890960531436335 ) ) ;
#92968=CARTESIAN_POINT ( 'NONE',  ( 21.53943276465977519, -0.05219959533907433946, 68.74890960531435269 ) ) ;
#92969=CARTESIAN_POINT ( 'NONE',  ( 19.05341960407611168, 5.049401038298154454, 93.95724293864769550 ) ) ;
#92970=CARTESIAN_POINT ( 'NONE',  ( -0.05219959533937732626, 21.53943276465977519, 92.50109039468567573 ) ) ;
#92971=CARTESIAN_POINT ( 'NONE',  ( 19.05341960407611168, 5.049401038298154454, 48.95724293864768129 ) ) ;
#92973=CARTESIAN_POINT ( 'NONE',  ( -16.52544592524335698, -4.483927247898792601, 38.95942372801901854 ) ) ;
#92974=CARTESIAN_POINT ( 'NONE',  ( 19.05341960407611168, 5.049401038298154454, 53.95724293864770260 ) ) ;
#92975=CARTESIAN_POINT ( 'NONE',  ( -0.05219959533937732626, 21.53943276465977519, 82.50109039468568994 ) ) ;
#92977=CARTESIAN_POINT ( 'NONE',  ( 0.05219959533936267826, -19.03943276465977164, 40.00109039468566152 ) ) ;
#92978=CARTESIAN_POINT ( 'NONE',  ( 19.05341960407617918, -5.049401038297876454, 36.04275706135234003 ) ) ;
#92979=CARTESIAN_POINT ( 'NONE',  ( 21.52544592524334988, 5.823673210054432836, 31.45942372801901854 ) ) ;
#92981=CARTESIAN_POINT ( 'NONE',  ( 9.474510206698729675, 16.51473224551082808, 27.08442372801900433 ) ) ;
#92982=CARTESIAN_POINT ( 'NONE',  ( -9.474510206698964154, 16.51473224551069663, 90.41557627198103830 ) ) ;
#92983=CARTESIAN_POINT ( 'NONE',  ( 13.89961937509977652, -13.97604488694527269, 68.12390960531436690 ) ) ;
#92984=CARTESIAN_POINT ( 'NONE',  ( -4.483927247898539470, -16.52544592524342804, 27.29057627198103120 ) ) ;
#92985=CARTESIAN_POINT ( 'NONE',  ( -5.823673210054116645, -21.52544592524344225, 22.29057627198102765 ) ) ;
#92986=CARTESIAN_POINT ( 'NONE',  ( 21.53943276465977519, 0.05219959533937863772, 86.25109039468568994 ) ) ;
#92988=CARTESIAN_POINT ( 'NONE',  ( 17.31728774477272736, 6.344390552232409775, 56.68093348310682700 ) ) ;
#92989=CARTESIAN_POINT ( 'NONE',  ( -15.72974639402176322, -15.80617190586768395, 94.37609039468568994 ) ) ;
#92990=CARTESIAN_POINT ( 'NONE',  ( 17.50000000000000000, -5.500000000000000888, 43.29690382534172244 ) ) ;
#92991=CARTESIAN_POINT ( 'NONE',  ( 4.379528057220339221, -16.55341960407611168, 112.7072429386476955 ) ) ;
#92994=CARTESIAN_POINT ( 'NONE',  ( 14.29746914071037800, 8.314922557961029526, 46.66775706135234714 ) ) ;
#92995=CARTESIAN_POINT ( 'NONE',  ( -10.72451020669898014, 18.67979575497178502, 70.41557627198102409 ) ) ;
#92996=CARTESIAN_POINT ( 'NONE',  ( -12.06949235617756955, 12.14591786802309770, 40.62390960531435269 ) ) ;
#92997=CARTESIAN_POINT ( 'NONE',  ( -0.05219959533910754901, -16.53943276465976808, 112.4989096053143669 ) ) ;
#92998=CARTESIAN_POINT ( 'NONE',  ( 9.564922557960805705, 16.46253265017160317, 89.58224293864769550 ) ) ;
#92999=CARTESIAN_POINT ( 'NONE',  ( -9.564922557961040184, 16.46253265017147172, 22.91775706135233648 ) ) ;
#93000=CARTESIAN_POINT ( 'NONE',  ( -0.05219959533909027116, -19.03943276465977164, 22.49890960531436690 ) ) ;
#93001=CARTESIAN_POINT ( 'NONE',  ( 5.719274019375673035, 21.55341960407619339, 67.29275706135234714 ) ) ;
#93002=CARTESIAN_POINT ( 'NONE',  ( 17.58332526062529411, -7.635886036038496805, 98.42334959558466778 ) ) ;
#93003=CARTESIAN_POINT ( 'NONE',  ( 12.14591786802327356, -12.06949235617739191, 100.6260903946857184 ) ) ;
#93004=CARTESIAN_POINT ( 'NONE',  ( -19.03943276465977164, -0.05219959533935918106, 58.75109039468566863 ) ) ;
#93006=CARTESIAN_POINT ( 'NONE',  ( 18.67979575497178502, 10.72451020669898547, 34.16557627198102409 ) ) ;
#93007=CARTESIAN_POINT ( 'NONE',  ( -16.55341960407611168, -4.379528057220339221, 86.45724293864770971 ) ) ;
#93008=CARTESIAN_POINT ( 'NONE',  ( 5.049401038297881783, 19.05341960407617563, 52.29275706135234003 ) ) ;
#93009=CARTESIAN_POINT ( 'NONE',  ( -13.89961937509977652, 13.97604488694528158, 70.62390960531432427 ) ) ;
#93010=CARTESIAN_POINT ( 'NONE',  ( 8.314922557960818139, 14.29746914071049879, 64.58224293864769550 ) ) ;
#93011=CARTESIAN_POINT ( 'NONE',  ( 9.564922557961047289, -16.46253265017146816, 95.41775706135233293 ) ) ;
#93012=CARTESIAN_POINT ( 'NONE',  ( 10.81492255796078972, 18.62759615963270932, 54.58224293864769550 ) ) ;
#93014=CARTESIAN_POINT ( 'NONE',  ( -8.314922557960811034, -14.29746914071050412, 112.0822429386477097 ) ) ;
#93015=CARTESIAN_POINT ( 'NONE',  ( 17.59860650958994555, -7.585241751806880650, 100.9233701426249183 ) ) ;
#93016=CARTESIAN_POINT ( 'NONE',  ( 5.153800228976335163, 19.02544592524342804, 74.79057627198103830 ) ) ;
#93017=CARTESIAN_POINT ( 'NONE',  ( 15.72974639402199770, -15.80617190586745480, 78.12390960531436690 ) ) ;
#93018=CARTESIAN_POINT ( 'NONE',  ( -8.314922557961024197, 14.29746914071037800, 87.91775706135234714 ) ) ;
#93019=CARTESIAN_POINT ( 'NONE',  ( 9.564922557960805705, 16.46253265017160317, 79.58224293864769550 ) ) ;
#93020=CARTESIAN_POINT ( 'NONE',  ( -16.51473224551082808, 9.474510206698731452, 73.33442372801900433 ) ) ;
#93021=CARTESIAN_POINT ( 'NONE',  ( 15.80617190586769283, -15.72974639402175789, 85.62609039468568994 ) ) ;
#93022=CARTESIAN_POINT ( 'NONE',  ( 10.72451020669898902, -18.67979575497178502, 62.91557627198102409 ) ) ;
#93023=CARTESIAN_POINT ( 'NONE',  ( 16.51473224551069308, 9.474510206698969483, 114.1655762719810241 ) ) ;
#93024=CARTESIAN_POINT ( 'NONE',  ( -19.05341960407611168, -5.049401038298163336, 31.45724293864769550 ) ) ;
#93025=CARTESIAN_POINT ( 'NONE',  ( 16.55341960407618274, -4.379528057220086978, 106.0427570613523471 ) ) ;
#93026=CARTESIAN_POINT ( 'NONE',  ( -13.89961937509977652, 13.97604488694528158, 55.62390960531434558 ) ) ;
#93027=CARTESIAN_POINT ( 'NONE',  ( -4.379528057220086978, -16.55341960407618274, 24.79275706135235779 ) ) ;
#93029=CARTESIAN_POINT ( 'NONE',  ( -18.67979575497193778, 10.72451020669871902, 113.3344237280190328 ) ) ;
#93030=CARTESIAN_POINT ( 'NONE',  ( 4.483927247898545687, 16.52544592524342804, 54.79057627198104541 ) ) ;
#93031=CARTESIAN_POINT ( 'NONE',  ( 15.72974639402199770, -15.80617190586745480, 98.12390960531436690 ) ) ;
#93032=CARTESIAN_POINT ( 'NONE',  ( -21.52544592524343514, 5.823673210054127303, 96.04057627198102409 ) ) ;
#93033=CARTESIAN_POINT ( 'NONE',  ( 16.36317988757059538, -7.306389748694917863, 96.59789608363225000 ) ) ;
#93034=CARTESIAN_POINT ( 'NONE',  ( -18.67979575497178146, -10.72451020669898902, 46.66557627198102409 ) ) ;
#93035=CARTESIAN_POINT ( 'NONE',  ( -16.55341960407617563, 4.379528057220093196, 78.54275706135236135 ) ) ;
#93036=CARTESIAN_POINT ( 'NONE',  ( -12.14591786802309592, -12.06949235617757132, 91.87390960531436690 ) ) ;
#93037=CARTESIAN_POINT ( 'NONE',  ( 19.03943276465977164, -0.05219959533909143690, 53.74890960531436690 ) ) ;
#93040=CARTESIAN_POINT ( 'NONE',  ( -14.29746914071037622, -8.314922557961029526, 104.1677570613523471 ) ) ;
#93041=CARTESIAN_POINT ( 'NONE',  ( -18.62759615963255300, -10.81492255796106328, 39.16775706135235424 ) ) ;
#93042=CARTESIAN_POINT ( 'NONE',  ( 19.05341960407611168, 5.049401038298154454, 93.95724293864769550 ) ) ;
#93043=CARTESIAN_POINT ( 'NONE',  ( -5.823673210054431948, 21.52544592524334988, 62.70942372801902565 ) ) ;
#93046=ORIENTED_EDGE ( 'NONE', *, *, #111151, .F. ) ;
#93047=CARTESIAN_POINT ( 'NONE',  ( 21.55341960407619695, -5.719274019375665929, 61.04275706135234714 ) ) ;
#93048=CARTESIAN_POINT ( 'NONE',  ( 5.049401038298161559, -19.05341960407611168, 47.70724293864770260 ) ) ;
#93049=CARTESIAN_POINT ( 'NONE',  ( 5.049401038298161559, -19.05341960407611168, 112.7072429386476813 ) ) ;
#93050=CARTESIAN_POINT ( 'NONE',  ( -19.05341960407611168, -5.049401038298163336, 86.45724293864769550 ) ) ;
#93051=CARTESIAN_POINT ( 'NONE',  ( 5.049401038297881783, 19.05341960407617563, 67.29275706135234714 ) ) ;
#93052=CARTESIAN_POINT ( 'NONE',  ( -10.81492255796105439, 18.62759615963255655, 47.91775706135234714 ) ) ;
#93053=CARTESIAN_POINT ( 'NONE',  ( -19.03943276465977164, -0.05219959533935918106, 98.75109039468567573 ) ) ;
#93054=CARTESIAN_POINT ( 'NONE',  ( -16.46253265017146816, -9.564922557961047289, 69.16775706135233293 ) ) ;
#93055=CARTESIAN_POINT ( 'NONE',  ( 19.05341960407611168, 5.049401038298154454, 38.95724293864767418 ) ) ;
#93056=CARTESIAN_POINT ( 'NONE',  ( 0.05219959533934541429, -16.53943276465976808, 105.0010903946856757 ) ) ;
#93057=CARTESIAN_POINT ( 'NONE',  ( 19.05341960407617918, -5.049401038297876454, 81.04275706135231871 ) ) ;
#93058=CARTESIAN_POINT ( 'NONE',  ( 8.224510206698953496, -14.34966873604960469, 22.91557627198102765 ) ) ;
#93059=CARTESIAN_POINT ( 'NONE',  ( 9.474510206698729675, 16.51473224551082808, 52.08442372801900433 ) ) ;
#93060=CARTESIAN_POINT ( 'NONE',  ( -10.72451020669870658, -18.67979575497194134, 99.58442372801900433 ) ) ;
#93061=CARTESIAN_POINT ( 'NONE',  ( 5.049401038297881783, 19.05341960407617563, 32.29275706135233293 ) ) ;
#93062=CARTESIAN_POINT ( 'NONE',  ( -9.564922557960796823, -16.46253265017161027, 27.08224293864769550 ) ) ;
#93063=CARTESIAN_POINT ( 'NONE',  ( -21.52544592524334988, -5.823673210054445271, 83.95942372801900433 ) ) ;
#93064=CARTESIAN_POINT ( 'NONE',  ( 0.05219959533934541429, -16.53943276465976808, 30.00109039468568284 ) ) ;
#93065=CARTESIAN_POINT ( 'NONE',  ( -0.05219959533909027116, -19.03943276465977164, 97.49890960531436690 ) ) ;
#93068=CARTESIAN_POINT ( 'NONE',  ( 19.05341960407611168, 5.049401038298154454, 78.95724293864769550 ) ) ;
#93069=CARTESIAN_POINT ( 'NONE',  ( -17.49999999999999289, 5.500000000000036415, 75.79690382534175797 ) ) ;
#93070=VERTEX_POINT ( 'NONE', #30232 ) ;
#93071=CARTESIAN_POINT ( 'NONE',  ( -13.97604488694547697, 13.89961937509957934, 88.12609039468563310 ) ) ;
#93072=CARTESIAN_POINT ( 'NONE',  ( 13.89961937509977652, -13.97604488694527269, 108.1239096053143669 ) ) ;
#93073=CARTESIAN_POINT ( 'NONE',  ( -18.62759615963255300, -10.81492255796106328, 109.1677570613523613 ) ) ;
#93074=CARTESIAN_POINT ( 'NONE',  ( -4.483927247898539470, -16.52544592524342804, 92.29057627198103830 ) ) ;
#93075=B_SPLINE_CURVE_WITH_KNOTS ( 'NONE', 3,
 ( #59463, #118168, #74651, #135340, #58479, #56490, #152473, #167656, #71656, #10994, #87811, #28173, #9996, #197992, #136317, #103991, #121136, #12988, #137305, #133323 ),
 .UNSPECIFIED., .F., .F.,
 ( 4, 2, 2, 2, 2, 2, 2, 2, 2, 4 ),
 ( 0.000000000000000000, 0.0004987090165372347556, 0.0009974180330744695112, 0.001246772541343097894, 0.001496127049611726059, 0.001994836066148982390, 0.002493545082686239155, 0.002742899590954876645, 0.002992254099223514568, 0.003989672132298030700 ),
 .UNSPECIFIED. ) ;
#93077=CARTESIAN_POINT ( 'NONE',  ( 10.81492255796078972, 18.62759615963270932, 64.58224293864769550 ) ) ;
#93078=CARTESIAN_POINT ( 'NONE',  ( -18.62759615963270932, 10.81492255796079327, 35.83224293864768839 ) ) ;
#93079=CARTESIAN_POINT ( 'NONE',  ( 16.53943276465976808, -0.05219959533910856209, 113.7489096053143527 ) ) ;
#93081=CARTESIAN_POINT ( 'NONE',  ( -9.474510206698720793, -16.51473224551083518, 59.58442372801900433 ) ) ;
#93082=CARTESIAN_POINT ( 'NONE',  ( 4.483927247898545687, 16.52544592524342804, 44.79057627198103120 ) ) ;
#93084=CARTESIAN_POINT ( 'NONE',  ( 5.153800228976335163, 19.02544592524342804, 114.7905762719810241 ) ) ;
#93085=CARTESIAN_POINT ( 'NONE',  ( -5.719274019375665041, -21.55341960407619695, 84.79275706135234714 ) ) ;
#93086=CARTESIAN_POINT ( 'NONE',  ( -18.62759615963270932, 10.81492255796079327, 75.83224293864769550 ) ) ;
#93087=CARTESIAN_POINT ( 'NONE',  ( -0.05219959533937732626, 21.53943276465977519, 57.50109039468568994 ) ) ;
#93088=CARTESIAN_POINT ( 'NONE',  ( -5.719274019375665041, -21.55341960407619695, 49.79275706135234714 ) ) ;
#93089=CARTESIAN_POINT ( 'NONE',  ( 16.46253265017160672, -9.564922557960803928, 78.33224293864769550 ) ) ;
#93090=CARTESIAN_POINT ( 'NONE',  ( -16.55341960407617563, 4.379528057220093196, 78.54275706135236135 ) ) ;
#93091=CARTESIAN_POINT ( 'NONE',  ( -16.46253265017160317, 9.564922557960807481, 25.83224293864769194 ) ) ;
#93093=CARTESIAN_POINT ( 'NONE',  ( 14.29746914071049879, -8.314922557960816363, 48.33224293864770260 ) ) ;
#93094=CARTESIAN_POINT ( 'NONE',  ( 14.29746914071049879, -8.314922557960816363, 28.33224293864769550 ) ) ;
#93095=CARTESIAN_POINT ( 'NONE',  ( -9.474510206698964154, 16.51473224551069663, 65.41557627198102409 ) ) ;
#93096=CARTESIAN_POINT ( 'NONE',  ( -16.51473224551069308, -9.474510206698971260, 31.66557627198102054 ) ) ;
#93097=CARTESIAN_POINT ( 'NONE',  ( 21.55341960407610458, 5.719274019375980345, 38.95724293864768839 ) ) ;
#93098=CARTESIAN_POINT ( 'NONE',  ( 19.02544592524334988, 5.153800228976608722, 36.45942372801900433 ) ) ;
#93100=CARTESIAN_POINT ( 'NONE',  ( 4.379528057220339221, -16.55341960407611168, 52.70724293864769550 ) ) ;
#93101=CARTESIAN_POINT ( 'NONE',  ( -19.02544592524342804, 5.153800228976336051, 116.0405762719810383 ) ) ;
#93103=CARTESIAN_POINT ( 'NONE',  ( 12.06949235617739724, 12.14591786802326823, 76.87609039468567573 ) ) ;
#93104=CARTESIAN_POINT ( 'NONE',  ( -5.153800228976607833, 19.02544592524334988, 72.70942372801900433 ) ) ;
#93105=CARTESIAN_POINT ( 'NONE',  ( 4.483927247898545687, 16.52544592524342804, 39.79057627198103830 ) ) ;
#93106=FACE_OUTER_BOUND ( 'NONE', #81697, .T. ) ;
#93107=CARTESIAN_POINT ( 'NONE',  ( 8.224510206698953496, -14.34966873604960469, 32.91557627198102409 ) ) ;
#93108=CARTESIAN_POINT ( 'NONE',  ( 9.474510206698971260, -16.51473224551069308, 42.91557627198103120 ) ) ;
#93109=CARTESIAN_POINT ( 'NONE',  ( -16.46253265017160317, 9.564922557960807481, 60.83224293864769550 ) ) ;
#93110=CARTESIAN_POINT ( 'NONE',  ( -9.564922557960796823, -16.46253265017161027, 42.08224293864769550 ) ) ;
#93111=CARTESIAN_POINT ( 'NONE',  ( -18.67979575497193778, 10.72451020669871902, 28.33442372801902209 ) ) ;
#93112=CARTESIAN_POINT ( 'NONE',  ( -5.153800228976328057, -19.02544592524343514, 57.29057627198103120 ) ) ;
#93114=CARTESIAN_POINT ( 'NONE',  ( -16.51473224551069308, -9.474510206698971260, 41.66557627198103120 ) ) ;
#93115=CARTESIAN_POINT ( 'NONE',  ( -15.72974639402197994, 15.80617190586746368, 35.62390960531437401 ) ) ;
#93116=CARTESIAN_POINT ( 'NONE',  ( -18.67979575497193778, 10.72451020669871902, 63.33442372801900433 ) ) ;
#93117=CARTESIAN_POINT ( 'NONE',  ( 19.02544592524343514, -5.153800228976328945, 28.54057627198102409 ) ) ;
#93118=CARTESIAN_POINT ( 'NONE',  ( 10.72451020669898902, -18.67979575497178502, 22.91557627198102765 ) ) ;
#93119=CARTESIAN_POINT ( 'NONE',  ( 4.379528057220092307, 16.55341960407617563, 97.29275706135234714 ) ) ;
#93120=CARTESIAN_POINT ( 'NONE',  ( -21.53943276465977519, -0.05219959533937600094, 103.7510903946857042 ) ) ;
#93121=CARTESIAN_POINT ( 'NONE',  ( -4.483927247898782831, 16.52544592524335698, 67.70942372801901854 ) ) ;
#93122=CARTESIAN_POINT ( 'NONE',  ( 13.89961937509977652, -13.97604488694527269, 108.1239096053143669 ) ) ;
#93123=CARTESIAN_POINT ( 'NONE',  ( -8.224510206698735004, -14.34966873604973081, 49.58442372801901143 ) ) ;
#93124=CARTESIAN_POINT ( 'NONE',  ( -12.06949235617739369, -12.14591786802326823, 44.37609039468567573 ) ) ;
#93125=CARTESIAN_POINT ( 'NONE',  ( -0.05219959533934338120, 16.53943276465976808, 97.50109039468567573 ) ) ;
#93126=CARTESIAN_POINT ( 'NONE',  ( 18.62759615963255655, 10.81492255796105972, 51.66775706135234714 ) ) ;
#93127=CARTESIAN_POINT ( 'NONE',  ( 14.34966873604972726, -8.224510206698740333, 25.83442372801901499 ) ) ;
#93128=CARTESIAN_POINT ( 'NONE',  ( 21.52544592524344225, -5.823673210054117533, 113.5405762719810383 ) ) ;
#93129=CARTESIAN_POINT ( 'NONE',  ( -16.55341960407617563, 4.379528057220093196, 23.54275706135235424 ) ) ;
#93130=CARTESIAN_POINT ( 'NONE',  ( 16.53943276465976808, 0.05219959533934440121, 91.25109039468568994 ) ) ;
#93131=CARTESIAN_POINT ( 'NONE',  ( -16.31925111598407341, 7.325300261831848125, 45.16424538967171998 ) ) ;
#93132=CARTESIAN_POINT ( 'NONE',  ( -21.52544592524334988, -5.823673210054445271, 93.95942372801903275 ) ) ;
#93133=CARTESIAN_POINT ( 'NONE',  ( 13.89961937509957401, 13.97604488694547697, 81.87609039468564731 ) ) ;
#93134=CARTESIAN_POINT ( 'NONE',  ( -8.224510206698948167, 14.34966873604960824, 65.41557627198102409 ) ) ;
#93135=CARTESIAN_POINT ( 'NONE',  ( -16.55341960407611168, -4.379528057220339221, 46.45724293864769550 ) ) ;
#93136=CARTESIAN_POINT ( 'NONE',  ( -16.55341960407611168, -4.379528057220339221, 111.4572429386476813 ) ) ;
#93137=CARTESIAN_POINT ( 'NONE',  ( -5.153800228976607833, 19.02544592524334988, 47.70942372801900433 ) ) ;
#93139=CARTESIAN_POINT ( 'NONE',  ( -21.52544592524334988, -5.823673210054445271, 43.95942372801902565 ) ) ;
#93140=CARTESIAN_POINT ( 'NONE',  ( -8.224510206698735004, -14.34966873604973081, 19.58442372801901143 ) ) ;
#93141=CARTESIAN_POINT ( 'NONE',  ( -17.49999999999999645, 7.499999999999998224, 120.0000000000000142 ) ) ;
#93142=CARTESIAN_POINT ( 'NONE',  ( -13.97604488694527625, -13.89961937509977652, 101.8739096053143811 ) ) ;
#93143=CARTESIAN_POINT ( 'NONE',  ( -15.80617190586745835, -15.72974639402198527, 66.87390960531436690 ) ) ;
#93144=CARTESIAN_POINT ( 'NONE',  ( -9.474510206698720793, -16.51473224551083518, 99.58442372801900433 ) ) ;
#93146=CARTESIAN_POINT ( 'NONE',  ( 19.02544592524343514, -5.153800228976328945, 98.54057627198100988 ) ) ;
#93147=CARTESIAN_POINT ( 'NONE',  ( -21.52544592524343514, 5.823673210054127303, 61.04057627198103120 ) ) ;
#93148=CARTESIAN_POINT ( 'NONE',  ( -4.379528057220328563, 16.55341960407611168, 110.2072429386477239 ) ) ;
#93149=CARTESIAN_POINT ( 'NONE',  ( 15.80617190586769283, -15.72974639402175789, 95.62609039468568994 ) ) ;
#93150=CARTESIAN_POINT ( 'NONE',  ( 19.03943276465977164, -0.05219959533909143690, 23.74890960531435269 ) ) ;
#93151=CARTESIAN_POINT ( 'NONE',  ( 15.72974639402176855, 15.80617190586768217, 36.87609039468568994 ) ) ;
#93152=CARTESIAN_POINT ( 'NONE',  ( -0.05219959533937732626, 21.53943276465977519, 87.50109039468568994 ) ) ;
#93153=CARTESIAN_POINT ( 'NONE',  ( -12.06949235617739369, -12.14591786802326823, 84.37609039468570415 ) ) ;
#93155=CARTESIAN_POINT ( 'NONE',  ( -10.72451020669870658, -18.67979575497194134, 29.58442372801901854 ) ) ;
#93156=CARTESIAN_POINT ( 'NONE',  ( 21.53943276465977519, 0.05219959533937863772, 41.25109039468568284 ) ) ;
#93157=CARTESIAN_POINT ( 'NONE',  ( 5.049401038297881783, 19.05341960407617563, 62.29275706135234003 ) ) ;
#93158=CARTESIAN_POINT ( 'NONE',  ( -9.474510206698964154, 16.51473224551069663, 85.41557627198102409 ) ) ;
#93159=CARTESIAN_POINT ( 'NONE',  ( 15.80617190586769283, -15.72974639402175789, 85.62609039468568994 ) ) ;
#93160=CARTESIAN_POINT ( 'NONE',  ( 21.52544592524344225, -5.823673210054117533, 78.54057627198103830 ) ) ;
#93161=CARTESIAN_POINT ( 'NONE',  ( 14.29746914071049879, -8.314922557960816363, 58.33224293864768839 ) ) ;
#93162=CARTESIAN_POINT ( 'NONE',  ( 15.72974639402176855, 15.80617190586768217, 106.8760903946856899 ) ) ;
#93163=CARTESIAN_POINT ( 'NONE',  ( -16.53943276465976808, 0.05219959533911058130, 81.24890960531436690 ) ) ;
#93164=CARTESIAN_POINT ( 'NONE',  ( 16.46253265017160672, -9.564922557960803928, 38.33224293864768839 ) ) ;
#93165=CARTESIAN_POINT ( 'NONE',  ( -5.153800228976607833, 19.02544592524334988, 77.70942372801900433 ) ) ;
#93166=CARTESIAN_POINT ( 'NONE',  ( -16.53943276465976808, 0.05219959533911058130, 41.24890960531435269 ) ) ;
#93167=CARTESIAN_POINT ( 'NONE',  ( 0.05219959533937995610, -21.53943276465977519, 100.0010903946857042 ) ) ;
#93168=CARTESIAN_POINT ( 'NONE',  ( -16.46253265017160317, 9.564922557960807481, 90.83224293864769550 ) ) ;
#93169=CARTESIAN_POINT ( 'NONE',  ( 16.46253265017146816, 9.564922557961045513, 66.66775706135233293 ) ) ;
#93170=CARTESIAN_POINT ( 'NONE',  ( 21.53943276465977519, -0.05219959533907433946, 68.74890960531435269 ) ) ;
#93171=CARTESIAN_POINT ( 'NONE',  ( -5.823673210054431948, 21.52544592524334988, 22.70942372801901499 ) ) ;
#93172=CARTESIAN_POINT ( 'NONE',  ( -16.46253265017146816, -9.564922557961047289, 109.1677570613523471 ) ) ;
#93173=CARTESIAN_POINT ( 'NONE',  ( -12.14591786802326823, 12.06949235617739902, 73.12609039468567573 ) ) ;
#93174=CARTESIAN_POINT ( 'NONE',  ( 16.21995358207306737, 7.366697692864131675, 62.56448998487839930 ) ) ;
#93175=CARTESIAN_POINT ( 'NONE',  ( 21.53943276465977519, 0.05219959533937863772, 26.25109039468567573 ) ) ;
#93176=CARTESIAN_POINT ( 'NONE',  ( 0.05219959533910956823, 16.53943276465976808, 99.99890960531436690 ) ) ;
#93178=CARTESIAN_POINT ( 'NONE',  ( -14.34966873604972548, 8.224510206698743886, 53.33442372801901854 ) ) ;
#93179=CARTESIAN_POINT ( 'NONE',  ( 12.06949235617757843, -12.14591786802309237, 78.12390960531436690 ) ) ;
#93180=CARTESIAN_POINT ( 'NONE',  ( 21.53943276465977519, -0.05219959533907433946, 73.74890960531433848 ) ) ;
#93181=CARTESIAN_POINT ( 'NONE',  ( 0.05219959533934541429, -16.53943276465976808, 100.0010903946857042 ) ) ;
#93182=CARTESIAN_POINT ( 'NONE',  ( 0.05219959533934541429, -16.53943276465976808, 40.00109039468567573 ) ) ;
#93183=CARTESIAN_POINT ( 'NONE',  ( -19.05341960407611168, -5.049401038298163336, 41.45724293864769550 ) ) ;
#93184=CARTESIAN_POINT ( 'NONE',  ( -16.52544592524335698, -4.483927247898792601, 73.95942372801901854 ) ) ;
#93185=CARTESIAN_POINT ( 'NONE',  ( -0.05219959533936034679, 19.03943276465977164, 67.50109039468566152 ) ) ;
#93186=CARTESIAN_POINT ( 'NONE',  ( 10.81492255796078972, 18.62759615963270932, 74.58224293864768129 ) ) ;
#93187=CARTESIAN_POINT ( 'NONE',  ( 8.224510206698742110, 14.34966873604972548, 92.08442372801901854 ) ) ;
#93188=CARTESIAN_POINT ( 'NONE',  ( -18.62759615963255300, -10.81492255796106328, 89.16775706135236135 ) ) ;
#93189=CARTESIAN_POINT ( 'NONE',  ( -21.55341960407610458, -5.719274019375992779, 71.45724293864769550 ) ) ;
#93190=CARTESIAN_POINT ( 'NONE',  ( -18.67979575497178146, -10.72451020669898902, 51.66557627198102409 ) ) ;
#93191=VERTEX_POINT ( 'NONE', #174718 ) ;
#93192=CARTESIAN_POINT ( 'NONE',  ( 14.29746914071037800, 8.314922557961029526, 81.66775706135236135 ) ) ;
#93193=CARTESIAN_POINT ( 'NONE',  ( -21.52544592524343514, 5.823673210054127303, 51.04057627198103120 ) ) ;
#93195=CARTESIAN_POINT ( 'NONE',  ( 21.53943276465977519, -0.05219959533907433946, 23.74890960531435269 ) ) ;
#93197=CARTESIAN_POINT ( 'NONE',  ( 19.03943276465977164, -0.05219959533909143690, 28.74890960531435624 ) ) ;
#93198=CARTESIAN_POINT ( 'NONE',  ( 21.52544592524344225, -5.823673210054117533, 78.54057627198103830 ) ) ;
#93199=CARTESIAN_POINT ( 'NONE',  ( 12.06949235617739724, 12.14591786802326823, 101.8760903946857042 ) ) ;
#93200=CARTESIAN_POINT ( 'NONE',  ( 5.823673210054444382, -21.52544592524334988, 45.20942372801901854 ) ) ;
#93201=CARTESIAN_POINT ( 'NONE',  ( -13.97604488694547697, 13.89961937509957934, 113.1260903946856757 ) ) ;
#93202=CARTESIAN_POINT ( 'NONE',  ( -19.02544592524342804, 5.153800228976336051, 26.04057627198103120 ) ) ;
#93203=CARTESIAN_POINT ( 'NONE',  ( -13.89961937509957401, -13.97604488694547875, 109.3760903946856331 ) ) ;
#93204=CARTESIAN_POINT ( 'NONE',  ( -13.89961937509977652, 13.97604488694528158, 35.62390960531435269 ) ) ;
#93206=CARTESIAN_POINT ( 'NONE',  ( 13.89961937509977652, -13.97604488694527269, 108.1239096053143669 ) ) ;
#93207=CARTESIAN_POINT ( 'NONE',  ( -12.14591786802326823, 12.06949235617739902, 88.12609039468570415 ) ) ;
#93208=CARTESIAN_POINT ( 'NONE',  ( -5.049401038297874678, -19.05341960407617918, 84.79275706135233293 ) ) ;
#93209=CARTESIAN_POINT ( 'NONE',  ( 19.02544592524334988, 5.153800228976608722, 26.45942372801899722 ) ) ;
#93210=CARTESIAN_POINT ( 'NONE',  ( 5.823673210054125526, 21.52544592524343514, 64.79057627198103830 ) ) ;
#93211=CARTESIAN_POINT ( 'NONE',  ( -8.224510206698735004, -14.34966873604973081, 89.58442372801901854 ) ) ;
#93212=CARTESIAN_POINT ( 'NONE',  ( 13.89961937509957401, 13.97604488694547697, 76.87609039468566152 ) ) ;
#93213=CARTESIAN_POINT ( 'NONE',  ( 9.564922557960805705, 16.46253265017160317, 49.58224293864770260 ) ) ;
#93214=CARTESIAN_POINT ( 'NONE',  ( -19.05341960407611168, -5.049401038298163336, 86.45724293864769550 ) ) ;
#93215=CARTESIAN_POINT ( 'NONE',  ( 10.81492255796106328, -18.62759615963255655, 45.41775706135234003 ) ) ;
#93216=CARTESIAN_POINT ( 'NONE',  ( -19.02544592524342804, 5.153800228976336051, 46.04057627198101699 ) ) ;
#93218=CARTESIAN_POINT ( 'NONE',  ( 19.05341960407611168, 5.049401038298154454, 103.9572429386476671 ) ) ;
#93219=CARTESIAN_POINT ( 'NONE',  ( 16.55341960407611168, 4.379528057220329451, 63.95724293864770260 ) ) ;
#93220=CARTESIAN_POINT ( 'NONE',  ( 10.72451020669898902, -18.67979575497178502, 62.91557627198102409 ) ) ;
#93222=CARTESIAN_POINT ( 'NONE',  ( 13.89961937509957401, 13.97604488694547697, 41.87609039468566152 ) ) ;
#93224=CARTESIAN_POINT ( 'NONE',  ( -9.474510206698964154, 16.51473224551069663, 60.41557627198102409 ) ) ;
#93225=CARTESIAN_POINT ( 'NONE',  ( -9.564922557960796823, -16.46253265017161027, 77.08224293864769550 ) ) ;
#93226=CARTESIAN_POINT ( 'NONE',  ( 4.483927247898790824, -16.52544592524335698, 50.20942372801901854 ) ) ;
#93227=CARTESIAN_POINT ( 'NONE',  ( -9.474510206698720793, -16.51473224551083518, 79.58442372801899012 ) ) ;
#93229=CARTESIAN_POINT ( 'NONE',  ( 12.06949235617739724, 12.14591786802326823, 91.87609039468568994 ) ) ;
#93231=CARTESIAN_POINT ( 'NONE',  ( 4.483927247898790824, -16.52544592524335698, 80.20942372801901854 ) ) ;
#93232=CARTESIAN_POINT ( 'NONE',  ( -4.379528057220086978, -16.55341960407618274, 54.79275706135235424 ) ) ;
#93233=CARTESIAN_POINT ( 'NONE',  ( 10.72451020669871369, 18.67979575497193778, 112.0844237280190185 ) ) ;
#93234=CARTESIAN_POINT ( 'NONE',  ( 13.97604488694527802, 13.89961937509977652, 49.37390960531434558 ) ) ;
#93236=CARTESIAN_POINT ( 'NONE',  ( -5.823673210054431948, 21.52544592524334988, 52.70942372801902565 ) ) ;
#93237=CARTESIAN_POINT ( 'NONE',  ( -19.03943276465977164, -0.05219959533935918106, 58.75109039468566863 ) ) ;
#93238=CARTESIAN_POINT ( 'NONE',  ( -0.05219959533937732626, 21.53943276465977519, 112.5010903946857042 ) ) ;
#93239=CARTESIAN_POINT ( 'NONE',  ( -5.153800228976328057, -19.02544592524343514, 27.29057627198103120 ) ) ;
#93241=CARTESIAN_POINT ( 'NONE',  ( -5.719274019375978568, 21.55341960407610458, 65.20724293864768129 ) ) ;
#93242=CARTESIAN_POINT ( 'NONE',  ( 19.03943276465977164, -0.05219959533909143690, 113.7489096053143669 ) ) ;
#93243=CARTESIAN_POINT ( 'NONE',  ( -19.03943276465977164, 0.05219959533909376836, 26.24890960531435624 ) ) ;
#93244=CARTESIAN_POINT ( 'NONE',  ( -0.05219959533934338120, 16.53943276465976808, 37.50109039468568284 ) ) ;
#93245=CARTESIAN_POINT ( 'NONE',  ( 16.55341960407611168, 4.379528057220329451, 33.95724293864769550 ) ) ;
#93247=CARTESIAN_POINT ( 'NONE',  ( 21.52544592524334988, 5.823673210054432836, 21.45942372801901499 ) ) ;
#93248=CARTESIAN_POINT ( 'NONE',  ( -12.14591786802309592, -12.06949235617757132, 36.87390960531435979 ) ) ;
#93249=CARTESIAN_POINT ( 'NONE',  ( 9.474510206698971260, -16.51473224551069308, 112.9155762719810383 ) ) ;
#93250=CARTESIAN_POINT ( 'NONE',  ( -5.153800228976607833, 19.02544592524334988, 102.7094237280189759 ) ) ;
#93251=CARTESIAN_POINT ( 'NONE',  ( 9.474510206698729675, 16.51473224551082808, 22.08442372801899722 ) ) ;
#93252=CARTESIAN_POINT ( 'NONE',  ( -16.55341960407611168, -4.379528057220339221, 41.45724293864769550 ) ) ;
#93253=CARTESIAN_POINT ( 'NONE',  ( 18.67979575497178502, 10.72451020669898547, 104.1655762719810241 ) ) ;
#93256=CARTESIAN_POINT ( 'NONE',  ( -10.72451020669898014, 18.67979575497178502, 70.41557627198102409 ) ) ;
#93257=CARTESIAN_POINT ( 'NONE',  ( -19.03943276465977164, 0.05219959533909376836, 71.24890960531435269 ) ) ;
#93258=CARTESIAN_POINT ( 'NONE',  ( 8.314922557960818139, 14.29746914071049879, 44.58224293864769550 ) ) ;
#93259=CARTESIAN_POINT ( 'NONE',  ( -19.03943276465977164, 0.05219959533909376836, 86.24890960531436690 ) ) ;
#93261=CARTESIAN_POINT ( 'NONE',  ( 16.46253265017146816, 9.564922557961045513, 51.66775706135233293 ) ) ;
#93262=CARTESIAN_POINT ( 'NONE',  ( 15.80617190586746368, 15.72974639402197994, 99.37390960531436690 ) ) ;
#93263=CARTESIAN_POINT ( 'NONE',  ( -16.55341960407611168, -4.379528057220339221, 101.4572429386476955 ) ) ;
#93264=CARTESIAN_POINT ( 'NONE',  ( 21.55341960407619695, -5.719274019375665929, 46.04275706135234714 ) ) ;
#93267=CARTESIAN_POINT ( 'NONE',  ( 16.53943276465976808, -0.05219959533910856209, 28.74890960531435624 ) ) ;
#93268=CARTESIAN_POINT ( 'NONE',  ( -19.03943276465977164, 0.05219959533909376836, 36.24890960531436690 ) ) ;
#93269=CARTESIAN_POINT ( 'NONE',  ( 0.05219959533909260263, 19.03943276465977164, 104.9989096053143669 ) ) ;
#93270=CARTESIAN_POINT ( 'NONE',  ( 15.80617190586746368, 15.72974639402197994, 54.37390960531435979 ) ) ;
#93271=CARTESIAN_POINT ( 'NONE',  ( -19.35633801406906684, 5.499999999999782396, 44.13373818172762952 ) ) ;
#93272=CARTESIAN_POINT ( 'NONE',  ( 19.05341960407611168, 5.049401038298154454, 28.95724293864769550 ) ) ;
#93273=CARTESIAN_POINT ( 'NONE',  ( 5.823673210054125526, 21.52544592524343514, 54.79057627198104541 ) ) ;
#93274=CARTESIAN_POINT ( 'NONE',  ( -18.62759615963255300, -10.81492255796106328, 79.16775706135234714 ) ) ;
#93276=CARTESIAN_POINT ( 'NONE',  ( -14.29746914071037622, -8.314922557961029526, 89.16775706135236135 ) ) ;
#93277=CARTESIAN_POINT ( 'NONE',  ( -9.474510206698964154, 16.51473224551069663, 60.41557627198102409 ) ) ;
#93278=CARTESIAN_POINT ( 'NONE',  ( 19.03943276465977164, -0.05219959533909143690, 63.74890960531435979 ) ) ;
#93280=CARTESIAN_POINT ( 'NONE',  ( -16.46253265017146816, -9.564922557961047289, 24.16775706135233648 ) ) ;
#93281=CARTESIAN_POINT ( 'NONE',  ( 16.55341960407618274, -4.379528057220086978, 71.04275706135234714 ) ) ;
#93282=CARTESIAN_POINT ( 'NONE',  ( -21.53943276465977519, -0.05219959533937600094, 103.7510903946857042 ) ) ;
#93283=CARTESIAN_POINT ( 'NONE',  ( 16.51473224551069308, 9.474510206698969483, 74.16557627198103830 ) ) ;
#93284=CARTESIAN_POINT ( 'NONE',  ( -15.80617190586745835, -15.72974639402198527, 31.87390960531435979 ) ) ;
#93285=CARTESIAN_POINT ( 'NONE',  ( -9.564922557961040184, 16.46253265017147172, 107.9177570613523471 ) ) ;
#93286=CARTESIAN_POINT ( 'NONE',  ( -0.05219959533937732626, 21.53943276465977519, 82.50109039468568994 ) ) ;
#93287=CARTESIAN_POINT ( 'NONE',  ( 4.483927247898790824, -16.52544592524335698, 45.20942372801901854 ) ) ;
#93288=CARTESIAN_POINT ( 'NONE',  ( -18.62759615963270932, 10.81492255796079327, 105.8322429386476955 ) ) ;
#93289=CARTESIAN_POINT ( 'NONE',  ( 0.05219959533934541429, -16.53943276465976808, 20.00109039468568639 ) ) ;
#93290=CARTESIAN_POINT ( 'NONE',  ( 9.474510206698971260, -16.51473224551069308, 72.91557627198102409 ) ) ;
#93291=CARTESIAN_POINT ( 'NONE',  ( -8.314922557961024197, 14.29746914071037800, 22.91775706135235069 ) ) ;
#93292=CARTESIAN_POINT ( 'NONE',  ( 0.05219959533909260263, 19.03943276465977164, 39.99890960531436690 ) ) ;
#93293=CARTESIAN_POINT ( 'NONE',  ( 5.153800228976615827, -19.02544592524334988, 110.2094237280189901 ) ) ;
#93294=CARTESIAN_POINT ( 'NONE',  ( 8.314922557960818139, 14.29746914071049879, 69.58224293864769550 ) ) ;
#93295=CARTESIAN_POINT ( 'NONE',  ( 12.14591786802327356, -12.06949235617739191, 75.62609039468567573 ) ) ;
#93296=CARTESIAN_POINT ( 'NONE',  ( -18.67979575497193778, 10.72451020669871902, 33.33442372801900433 ) ) ;
#93297=CARTESIAN_POINT ( 'NONE',  ( 16.51473224551069308, 9.474510206698969483, 49.16557627198102409 ) ) ;
#93298=CARTESIAN_POINT ( 'NONE',  ( -13.89961937509977652, 13.97604488694528158, 75.62390960531438111 ) ) ;
#93299=CARTESIAN_POINT ( 'NONE',  ( -4.483927247898782831, 16.52544592524335698, 77.70942372801900433 ) ) ;
#93304=CARTESIAN_POINT ( 'NONE',  ( -5.823673210054431948, 21.52544592524334988, 107.7094237280190328 ) ) ;
#93305=CARTESIAN_POINT ( 'NONE',  ( -9.474510206698964154, 16.51473224551069663, 40.41557627198103120 ) ) ;
#93306=CARTESIAN_POINT ( 'NONE',  ( 9.564922557960805705, 16.46253265017160317, 114.5822429386476955 ) ) ;
#93308=CARTESIAN_POINT ( 'NONE',  ( -14.34966873604972548, 8.224510206698743886, 28.33442372801902209 ) ) ;
#93310=CARTESIAN_POINT ( 'NONE',  ( -13.89961937509957401, -13.97604488694547875, 59.37609039468566863 ) ) ;
#93311=CARTESIAN_POINT ( 'NONE',  ( 16.53943276465976808, 0.05219959533934440121, 46.25109039468567573 ) ) ;
#93312=CARTESIAN_POINT ( 'NONE',  ( 9.564922557960805705, 16.46253265017160317, 39.58224293864768839 ) ) ;
#93313=CARTESIAN_POINT ( 'NONE',  ( -13.89961937509977652, 13.97604488694528158, 110.6239096053143243 ) ) ;
#93314=CARTESIAN_POINT ( 'NONE',  ( -16.51473224551069308, -9.474510206698971260, 61.66557627198103120 ) ) ;
#93315=CARTESIAN_POINT ( 'NONE',  ( -0.05219959533907301413, -21.53943276465977519, 102.4989096053143811 ) ) ;
#93316=CARTESIAN_POINT ( 'NONE',  ( 16.51473224551069308, 9.474510206698969483, 89.16557627198103830 ) ) ;
#93317=CARTESIAN_POINT ( 'NONE',  ( -13.97604488694527625, -13.89961937509977652, 21.87390960531435979 ) ) ;
#93318=CARTESIAN_POINT ( 'NONE',  ( -9.474510206698964154, 16.51473224551069663, 60.41557627198102409 ) ) ;
#93319=CARTESIAN_POINT ( 'NONE',  ( -0.05219959533934338120, 16.53943276465976808, 107.5010903946856899 ) ) ;
#93320=CARTESIAN_POINT ( 'NONE',  ( -17.49999999999999645, -5.499999999999992895, 59.20309617465829177 ) ) ;
#93321=CARTESIAN_POINT ( 'NONE',  ( -19.05341960407617563, 5.049401038297882671, 98.54275706135233293 ) ) ;
#93322=CARTESIAN_POINT ( 'NONE',  ( -19.02544592524334988, -5.153800228976617603, 28.95942372801900433 ) ) ;
#93323=CARTESIAN_POINT ( 'NONE',  ( -16.52544592524342804, 4.483927247898546575, 56.04057627198102409 ) ) ;
#93324=CARTESIAN_POINT ( 'NONE',  ( 5.719274019375673035, 21.55341960407619339, 102.2927570613523613 ) ) ;
#93325=CARTESIAN_POINT ( 'NONE',  ( 13.97604488694527802, 13.89961937509977652, 34.37390960531436690 ) ) ;
#93326=CARTESIAN_POINT ( 'NONE',  ( -8.224510206698948167, 14.34966873604960824, 40.41557627198103120 ) ) ;
#93327=CARTESIAN_POINT ( 'NONE',  ( 21.53943276465977519, 0.05219959533937863772, 86.25109039468568994 ) ) ;
#93328=CARTESIAN_POINT ( 'NONE',  ( -19.03943276465977164, 0.05219959533909376836, 86.24890960531436690 ) ) ;
#93329=CARTESIAN_POINT ( 'NONE',  ( -9.474510206698964154, 16.51473224551069663, 100.4155762719810241 ) ) ;
#93330=CARTESIAN_POINT ( 'NONE',  ( -8.314922557960811034, -14.29746914071050412, 107.0822429386476955 ) ) ;
#93331=CARTESIAN_POINT ( 'NONE',  ( -14.29746914071049879, 8.314922557960819915, 70.83224293864770971 ) ) ;
#93332=CARTESIAN_POINT ( 'NONE',  ( -10.81492255796078084, -18.62759615963271287, 82.08224293864768129 ) ) ;
#93333=CARTESIAN_POINT ( 'NONE',  ( 9.474510206698971260, -16.51473224551069308, 77.91557627198103830 ) ) ;
#93334=CARTESIAN_POINT ( 'NONE',  ( -10.81492255796078084, -18.62759615963271287, 82.08224293864768129 ) ) ;
#93335=CARTESIAN_POINT ( 'NONE',  ( -13.89961937509957401, -13.97604488694547875, 84.37609039468567573 ) ) ;
#93337=CARTESIAN_POINT ( 'NONE',  ( -16.53943276465976808, 0.05219959533911058130, 96.24890960531435269 ) ) ;
#93338=CARTESIAN_POINT ( 'NONE',  ( 19.02544592524343514, -5.153800228976328945, 58.54057627198102409 ) ) ;
#93339=CARTESIAN_POINT ( 'NONE',  ( -15.72974639402197994, 15.80617190586746368, 65.62390960531436690 ) ) ;
#93341=CARTESIAN_POINT ( 'NONE',  ( -8.314922557961024197, 14.29746914071037800, 107.9177570613523471 ) ) ;
#93342=CARTESIAN_POINT ( 'NONE',  ( -17.49999999999999645, 5.499999999999997335, 120.0000000000000142 ) ) ;
#93343=CARTESIAN_POINT ( 'NONE',  ( 12.14591786802327356, -12.06949235617739191, 25.62609039468567929 ) ) ;
#93344=CARTESIAN_POINT ( 'NONE',  ( -4.379528057220328563, 16.55341960407611168, 75.20724293864769550 ) ) ;
#93346=CARTESIAN_POINT ( 'NONE',  ( 19.02544592524343514, -5.153800228976328945, 78.54057627198099567 ) ) ;
#93347=CARTESIAN_POINT ( 'NONE',  ( 19.03943276465977164, -0.05219959533909143690, 33.74890960531435979 ) ) ;
#93348=CARTESIAN_POINT ( 'NONE',  ( 12.06949235617757843, -12.14591786802309237, 73.12390960531436690 ) ) ;
#93349=CARTESIAN_POINT ( 'NONE',  ( -21.53943276465977519, 0.05219959533907696930, 21.24890960531436690 ) ) ;
#93350=CARTESIAN_POINT ( 'NONE',  ( 5.153800228976615827, -19.02544592524334988, 85.20942372801900433 ) ) ;
#93351=CARTESIAN_POINT ( 'NONE',  ( 19.03943276465977164, -0.05219959533909143690, 73.74890960531435269 ) ) ;
#93352=CARTESIAN_POINT ( 'NONE',  ( -0.05219959533909027116, -19.03943276465977164, 82.49890960531436690 ) ) ;
#93353=CARTESIAN_POINT ( 'NONE',  ( 18.67979575497178502, 10.72451020669898547, 79.16557627198103830 ) ) ;
#93354=CARTESIAN_POINT ( 'NONE',  ( 8.224510206698742110, 14.34966873604972548, 77.08442372801901854 ) ) ;
#93355=CARTESIAN_POINT ( 'NONE',  ( -17.40861289039008497, 6.110651285853112569, 93.62767529172570846 ) ) ;
#93356=CARTESIAN_POINT ( 'NONE',  ( -9.564922557960796823, -16.46253265017161027, 57.08224293864769550 ) ) ;
#93357=CARTESIAN_POINT ( 'NONE',  ( -10.81492255796078084, -18.62759615963271287, 67.08224293864770971 ) ) ;
#93358=CARTESIAN_POINT ( 'NONE',  ( -0.05219959533936034679, 19.03943276465977164, 97.50109039468567573 ) ) ;
#93359=CARTESIAN_POINT ( 'NONE',  ( 12.14591786802309770, 12.06949235617756955, 39.37390960531436690 ) ) ;
#93360=CARTESIAN_POINT ( 'NONE',  ( 21.53943276465977519, 0.05219959533937863772, 51.25109039468568994 ) ) ;
#93361=CARTESIAN_POINT ( 'NONE',  ( -4.483927247898782831, 16.52544592524335698, 77.70942372801900433 ) ) ;
#93362=CARTESIAN_POINT ( 'NONE',  ( 13.97604488694527802, 13.89961937509977652, 104.3739096053143385 ) ) ;
#93365=CARTESIAN_POINT ( 'NONE',  ( -4.379528057220086978, -16.55341960407618274, 99.79275706135234714 ) ) ;
#93366=CARTESIAN_POINT ( 'NONE',  ( -4.483927247898782831, 16.52544592524335698, 47.70942372801902565 ) ) ;
#93367=CARTESIAN_POINT ( 'NONE',  ( -19.05341960407611168, -5.049401038298163336, 56.45724293864768129 ) ) ;
#93368=CARTESIAN_POINT ( 'NONE',  ( 19.03943276465977164, -0.05219959533909143690, 68.74890960531436690 ) ) ;
#93369=CARTESIAN_POINT ( 'NONE',  ( -21.55341960407619339, 5.719274019375674811, 58.54275706135235424 ) ) ;
#93370=CARTESIAN_POINT ( 'NONE',  ( -4.483927247898782831, 16.52544592524335698, 62.70942372801902565 ) ) ;
#93371=CARTESIAN_POINT ( 'NONE',  ( 16.52544592524342804, -4.483927247898539470, 33.54057627198102409 ) ) ;
#93372=CARTESIAN_POINT ( 'NONE',  ( 13.89961937509977652, -13.97604488694527269, 38.12390960531436690 ) ) ;
#93373=CARTESIAN_POINT ( 'NONE',  ( -19.03943276465977164, 0.05219959533909376836, 36.24890960531436690 ) ) ;
#93374=CARTESIAN_POINT ( 'NONE',  ( -0.05219959533934338120, 16.53943276465976808, 22.50109039468567573 ) ) ;
#93376=CARTESIAN_POINT ( 'NONE',  ( 19.02544592524334988, 5.153800228976608722, 86.45942372801900433 ) ) ;
#93377=CARTESIAN_POINT ( 'NONE',  ( -16.52544592524342804, 4.483927247898546575, 86.04057627198102409 ) ) ;
#93378=CARTESIAN_POINT ( 'NONE',  ( -16.51473224551069308, -9.474510206698971260, 51.66557627198102409 ) ) ;
#93379=CARTESIAN_POINT ( 'NONE',  ( -16.51473224551082808, 9.474510206698731452, 88.33442372801900433 ) ) ;
#93381=CARTESIAN_POINT ( 'NONE',  ( 15.72974639402176855, 15.80617190586768217, 96.87609039468568994 ) ) ;
#93382=CARTESIAN_POINT ( 'NONE',  ( 0.05219959533934541429, -16.53943276465976808, 55.00109039468568284 ) ) ;
#93383=CARTESIAN_POINT ( 'NONE',  ( -17.50000000000143530, 3.202012800152433059, 24.92822416027274457 ) ) ;
#93384=CARTESIAN_POINT ( 'NONE',  ( -5.719274019375978568, 21.55341960407610458, 55.20724293864770260 ) ) ;
#93385=CARTESIAN_POINT ( 'NONE',  ( 14.34966873604972726, -8.224510206698740333, 45.83442372801901854 ) ) ;
#93386=CARTESIAN_POINT ( 'NONE',  ( -19.02130022317638236, 5.499999999999802824, 70.78188669246573284 ) ) ;
#93387=CARTESIAN_POINT ( 'NONE',  ( 16.46253265017146816, 9.564922557961045513, 26.66775706135234003 ) ) ;
#93388=CARTESIAN_POINT ( 'NONE',  ( 9.474510206698971260, -16.51473224551069308, 82.91557627198103830 ) ) ;
#93389=CARTESIAN_POINT ( 'NONE',  ( -0.05219959533909027116, -19.03943276465977164, 52.49890960531436690 ) ) ;
#93390=LINE ( 'NONE', #155076, #65768 ) ;
#93391=CARTESIAN_POINT ( 'NONE',  ( 16.46253265017160672, -9.564922557960803928, 63.33224293864769550 ) ) ;
#93392=CARTESIAN_POINT ( 'NONE',  ( -18.87255363501903460, -5.499999999999956479, 56.32513748171827928 ) ) ;
#93393=CARTESIAN_POINT ( 'NONE',  ( -13.97604488694547697, 13.89961937509957934, 38.12609039468566152 ) ) ;
#93394=CARTESIAN_POINT ( 'NONE',  ( -5.823673210054431948, 21.52544592524334988, 107.7094237280190328 ) ) ;
#93395=CARTESIAN_POINT ( 'NONE',  ( -4.379528057220328563, 16.55341960407611168, 35.20724293864768839 ) ) ;
#93396=CARTESIAN_POINT ( 'NONE',  ( 9.564922557960805705, 16.46253265017160317, 39.58224293864768839 ) ) ;
#93398=CARTESIAN_POINT ( 'NONE',  ( -5.153800228976328057, -19.02544592524343514, 112.2905762719810099 ) ) ;
#93399=CARTESIAN_POINT ( 'NONE',  ( -21.53943276465977519, -0.05219959533937600094, 78.75109039468568994 ) ) ;
#93400=CARTESIAN_POINT ( 'NONE',  ( -5.153800228976328057, -19.02544592524343514, 47.29057627198102409 ) ) ;
#93401=CARTESIAN_POINT ( 'NONE',  ( 15.72974639402176855, 15.80617190586768217, 76.87609039468567573 ) ) ;
#93402=CARTESIAN_POINT ( 'NONE',  ( -18.67979575497178146, -10.72451020669898902, 21.66557627198102409 ) ) ;
#93403=CARTESIAN_POINT ( 'NONE',  ( -15.72974639402176322, -15.80617190586768395, 19.37609039468568639 ) ) ;
#93404=CARTESIAN_POINT ( 'NONE',  ( -19.03943276465977164, -0.05219959533935918106, 43.75109039468566863 ) ) ;
#93405=CARTESIAN_POINT ( 'NONE',  ( 9.564922557960805705, 16.46253265017160317, 29.58224293864769550 ) ) ;
#93406=CARTESIAN_POINT ( 'NONE',  ( -13.97604488694527625, -13.89961937509977652, 76.87390960531433848 ) ) ;
#93407=CARTESIAN_POINT ( 'NONE',  ( 14.34966873604972726, -8.224510206698740333, 20.83442372801901143 ) ) ;
#93408=CARTESIAN_POINT ( 'NONE',  ( 12.14591786802309770, 12.06949235617756955, 94.37390960531436690 ) ) ;
#93409=CARTESIAN_POINT ( 'NONE',  ( -18.67979575497178146, -10.72451020669898902, 41.66557627198103120 ) ) ;
#93410=CARTESIAN_POINT ( 'NONE',  ( 19.03943276465977164, 0.05219959533936151252, 101.2510903946856757 ) ) ;
#93411=CARTESIAN_POINT ( 'NONE',  ( -5.719274019375978568, 21.55341960407610458, 100.2072429386476955 ) ) ;
#93412=CARTESIAN_POINT ( 'NONE',  ( 21.53943276465977519, 0.05219959533937863772, 51.25109039468568994 ) ) ;
#93413=CARTESIAN_POINT ( 'NONE',  ( -12.06949235617739369, -12.14591786802326823, 59.37609039468568284 ) ) ;
#93414=CARTESIAN_POINT ( 'NONE',  ( 4.483927247898790824, -16.52544592524335698, 60.20942372801902565 ) ) ;
#93415=CARTESIAN_POINT ( 'NONE',  ( -19.02544592524342804, 5.153800228976336051, 61.04057627198103120 ) ) ;
#93416=CARTESIAN_POINT ( 'NONE',  ( 0.05219959533934541429, -16.53943276465976808, 95.00109039468568994 ) ) ;
#93417=CARTESIAN_POINT ( 'NONE',  ( 21.55341960407610458, 5.719274019375980345, 113.9572429386477239 ) ) ;
#93418=CARTESIAN_POINT ( 'NONE',  ( -16.53943276465976808, 0.05219959533911058130, 51.24890960531436690 ) ) ;
#93419=CARTESIAN_POINT ( 'NONE',  ( -16.51473224551069308, -9.474510206698971260, 86.66557627198102409 ) ) ;
#93420=CARTESIAN_POINT ( 'NONE',  ( 0.05219959533934541429, -16.53943276465976808, 70.00109039468568994 ) ) ;
#93421=CARTESIAN_POINT ( 'NONE',  ( 10.81492255796106328, -18.62759615963255655, 65.41775706135234714 ) ) ;
#93422=CARTESIAN_POINT ( 'NONE',  ( -13.97604488694547697, 13.89961937509957934, 108.1260903946856331 ) ) ;
#93423=CARTESIAN_POINT ( 'NONE',  ( 21.53943276465977519, -0.05219959533907433946, 108.7489096053143669 ) ) ;
#93424=CARTESIAN_POINT ( 'NONE',  ( -12.14591786802309592, -12.06949235617757132, 46.87390960531435979 ) ) ;
#93427=CARTESIAN_POINT ( 'NONE',  ( -17.31747979337950483, 6.344076630961001051, 68.62055131934820906 ) ) ;
#93428=CARTESIAN_POINT ( 'NONE',  ( -18.67979575497178146, -10.72451020669898902, 81.66557627198103830 ) ) ;
#93429=CARTESIAN_POINT ( 'NONE',  ( 12.06949235617757843, -12.14591786802309237, 28.12390960531435979 ) ) ;
#93432=CARTESIAN_POINT ( 'NONE',  ( -15.80617190586745835, -15.72974639402198527, 111.8739096053143669 ) ) ;
#93433=CARTESIAN_POINT ( 'NONE',  ( -19.03943276465977164, 0.05219959533909376836, 116.2489096053143669 ) ) ;
#93434=CARTESIAN_POINT ( 'NONE',  ( -21.53943276465977519, -0.05219959533937600094, 28.75109039468567929 ) ) ;
#93435=CARTESIAN_POINT ( 'NONE',  ( 14.34966873604960469, 8.224510206698951720, 54.16557627198103120 ) ) ;
#93436=CARTESIAN_POINT ( 'NONE',  ( 12.06949235617739724, 12.14591786802326823, 61.87609039468568284 ) ) ;
#93437=CARTESIAN_POINT ( 'NONE',  ( -9.474510206698964154, 16.51473224551069663, 65.41557627198102409 ) ) ;
#93438=CARTESIAN_POINT ( 'NONE',  ( 19.02544592524334988, 5.153800228976608722, 71.45942372801900433 ) ) ;
#93439=CARTESIAN_POINT ( 'NONE',  ( 5.153800228976335163, 19.02544592524342804, 74.79057627198103830 ) ) ;
#93440=CARTESIAN_POINT ( 'NONE',  ( -21.52544592524343514, 5.823673210054127303, 41.04057627198103120 ) ) ;
#93442=CARTESIAN_POINT ( 'NONE',  ( 0.05219959533909260263, 19.03943276465977164, 64.99890960531436690 ) ) ;
#93443=CARTESIAN_POINT ( 'NONE',  ( -8.314922557961024197, 14.29746914071037800, 27.91775706135234358 ) ) ;
#93444=CARTESIAN_POINT ( 'NONE',  ( -5.049401038297874678, -19.05341960407617918, 69.79275706135233293 ) ) ;
#93445=CARTESIAN_POINT ( 'NONE',  ( -15.80617190586745835, -15.72974639402198527, 106.8739096053143811 ) ) ;
#93446=CARTESIAN_POINT ( 'NONE',  ( -0.05219959533910754901, -16.53943276465976808, 32.49890960531435979 ) ) ;
#93447=CARTESIAN_POINT ( 'NONE',  ( 19.02544592524343514, -5.153800228976328945, 88.54057627198102409 ) ) ;
#93448=CARTESIAN_POINT ( 'NONE',  ( 15.80617190586746368, 15.72974639402197994, 59.37390960531436690 ) ) ;
#93449=CARTESIAN_POINT ( 'NONE',  ( -10.81492255796078084, -18.62759615963271287, 92.08224293864769550 ) ) ;
#93450=CARTESIAN_POINT ( 'NONE',  ( -8.224510206698735004, -14.34966873604973081, 44.58442372801901854 ) ) ;
#93451=CARTESIAN_POINT ( 'NONE',  ( -5.823673210054116645, -21.52544592524344225, 42.29057627198103120 ) ) ;
#93452=CARTESIAN_POINT ( 'NONE',  ( 5.719274019375673035, 21.55341960407619339, 87.29275706135236135 ) ) ;
#93453=CARTESIAN_POINT ( 'NONE',  ( -9.474510206698964154, 16.51473224551069663, 85.41557627198102409 ) ) ;
#93455=CARTESIAN_POINT ( 'NONE',  ( -5.049401038298153566, 19.05341960407611168, 45.20724293864769550 ) ) ;
#93456=CARTESIAN_POINT ( 'NONE',  ( -19.03943276465977164, 0.05219959533909376836, 86.24890960531436690 ) ) ;
#93457=CARTESIAN_POINT ( 'NONE',  ( 16.52544592524342804, -4.483927247898539470, 98.54057627198105251 ) ) ;
#93459=CARTESIAN_POINT ( 'NONE',  ( 19.03943276465977164, -0.05219959533909143690, 68.74890960531436690 ) ) ;
#93460=CARTESIAN_POINT ( 'NONE',  ( 16.52544592524335698, 4.483927247898782831, 26.45942372801901854 ) ) ;
#93461=CARTESIAN_POINT ( 'NONE',  ( 13.89961937509957579, 13.97604488694547520, 41.87609039468566152 ) ) ;
#93462=CARTESIAN_POINT ( 'NONE',  ( 21.52544592524334988, 5.823673210054432836, 96.45942372801901854 ) ) ;
#93463=CARTESIAN_POINT ( 'NONE',  ( 19.05341960407611168, 5.049401038298154454, 108.9572429386477097 ) ) ;
#93464=CARTESIAN_POINT ( 'NONE',  ( -16.52544592524335698, -4.483927247898792601, 88.95942372801901854 ) ) ;
#93465=DIRECTION ( 'NONE',  ( -0.000000000000000000, 0.000000000000000000, 1.000000000000000000 ) ) ;
#93466=CARTESIAN_POINT ( 'NONE',  ( 13.97604488694548053, -13.89961937509957401, 75.62609039468564731 ) ) ;
#93467=CARTESIAN_POINT ( 'NONE',  ( -13.97604488694547697, 13.89961937509957934, 28.12609039468565797 ) ) ;
#93468=CARTESIAN_POINT ( 'NONE',  ( -17.44270441346513678, -5.991230190323104665, 46.36335079264228654 ) ) ;
#93469=CARTESIAN_POINT ( 'NONE',  ( 0.05219959533909260263, 19.03943276465977164, 24.99890960531435269 ) ) ;
#93470=CARTESIAN_POINT ( 'NONE',  ( 16.53943276465976808, -0.05219959533910856209, 33.74890960531436690 ) ) ;
#93471=CARTESIAN_POINT ( 'NONE',  ( -16.21995358207306026, -7.366697692864179636, 110.0644899848784206 ) ) ;
#93472=CARTESIAN_POINT ( 'NONE',  ( -12.14591786802309592, -12.06949235617757132, 31.87390960531435979 ) ) ;
#93474=CARTESIAN_POINT ( 'NONE',  ( -4.379528057220086978, -16.55341960407618274, 99.79275706135234714 ) ) ;
#93475=CARTESIAN_POINT ( 'NONE',  ( -19.03943276465977164, 0.05219959533909376836, 36.24890960531436690 ) ) ;
#93476=CARTESIAN_POINT ( 'NONE',  ( -21.53943276465977519, -0.05219959533937600094, 98.75109039468568994 ) ) ;
#93477=CARTESIAN_POINT ( 'NONE',  ( 13.89961937509957401, 13.97604488694547697, 111.8760903946856757 ) ) ;
#93478=CARTESIAN_POINT ( 'NONE',  ( 10.72451020669871369, 18.67979575497193778, 72.08442372801899012 ) ) ;
#93479=CARTESIAN_POINT ( 'NONE',  ( 5.049401038297881783, 19.05341960407617563, 47.29275706135231161 ) ) ;
#93480=CARTESIAN_POINT ( 'NONE',  ( 5.153800228976335163, 19.02544592524342804, 89.79057627198102409 ) ) ;
#93481=CARTESIAN_POINT ( 'NONE',  ( -19.02544592524342804, 5.153800228976336051, 76.04057627198102409 ) ) ;
#93482=CARTESIAN_POINT ( 'NONE',  ( 17.40805194822031865, 6.112264579159365496, 71.66628727489388950 ) ) ;
#93483=CARTESIAN_POINT ( 'NONE',  ( -18.62759615963270932, 10.81492255796079327, 100.8322429386477097 ) ) ;
#93485=CARTESIAN_POINT ( 'NONE',  ( 14.29746914071049879, -8.314922557960816363, 73.33224293864769550 ) ) ;
#93486=CARTESIAN_POINT ( 'NONE',  ( 5.823673210054125526, 21.52544592524343514, 64.79057627198103830 ) ) ;
#93487=CARTESIAN_POINT ( 'NONE',  ( 19.03943276465977164, -0.05219959533909143690, 58.74890960531435979 ) ) ;
#93488=CARTESIAN_POINT ( 'NONE',  ( -5.719274019375978568, 21.55341960407610458, 80.20724293864769550 ) ) ;
#93489=CARTESIAN_POINT ( 'NONE',  ( 8.224510206698742110, 14.34966873604972548, 82.08442372801901854 ) ) ;
#93491=CARTESIAN_POINT ( 'NONE',  ( -9.564922557960796823, -16.46253265017161027, 42.08224293864769550 ) ) ;
#93492=CARTESIAN_POINT ( 'NONE',  ( -8.224510206698948167, 14.34966873604960824, 80.41557627198103830 ) ) ;
#93494=CARTESIAN_POINT ( 'NONE',  ( 19.02544592524343514, -5.153800228976328945, 48.54057627198103120 ) ) ;
#93495=CARTESIAN_POINT ( 'NONE',  ( 13.97604488694527802, 13.89961937509977652, 24.37390960531435624 ) ) ;
#93496=CARTESIAN_POINT ( 'NONE',  ( 5.153800228976615827, -19.02544592524334988, 60.20942372801899012 ) ) ;
#93497=CARTESIAN_POINT ( 'NONE',  ( 0.05219959533910956823, 16.53943276465976808, 89.99890960531438111 ) ) ;
#93498=CARTESIAN_POINT ( 'NONE',  ( -21.53943276465977519, -0.05219959533937600094, 43.75109039468568284 ) ) ;
#93499=EDGE_CURVE ( 'NONE', #4215, #11669, #187304, .T. ) ;
#93500=CARTESIAN_POINT ( 'NONE',  ( -9.564922557960796823, -16.46253265017161027, 42.08224293864769550 ) ) ;
#93501=CARTESIAN_POINT ( 'NONE',  ( -10.81492255796078084, -18.62759615963271287, 107.0822429386476955 ) ) ;
#93503=CARTESIAN_POINT ( 'NONE',  ( 4.379528057220339221, -16.55341960407611168, 92.70724293864770971 ) ) ;
#93505=CARTESIAN_POINT ( 'NONE',  ( -9.564922557960796823, -16.46253265017161027, 47.08224293864769550 ) ) ;
#93506=CARTESIAN_POINT ( 'NONE',  ( 19.53091890409951858, 5.500000000000029310, 47.56097431831422995 ) ) ;
#93507=CARTESIAN_POINT ( 'NONE',  ( 5.153800228976615827, -19.02544592524334988, 90.20942372801900433 ) ) ;
#93508=CARTESIAN_POINT ( 'NONE',  ( 16.51473224551069308, 9.474510206698969483, 99.16557627198102409 ) ) ;
#93509=CARTESIAN_POINT ( 'NONE',  ( 15.80617190586769283, -15.72974639402175789, 35.62609039468568994 ) ) ;
#93510=CARTESIAN_POINT ( 'NONE',  ( -13.97604488694527625, -13.89961937509977652, 86.87390960531436690 ) ) ;
#93511=CARTESIAN_POINT ( 'NONE',  ( 5.153800228976615827, -19.02544592524334988, 75.20942372801896170 ) ) ;
#93512=CARTESIAN_POINT ( 'NONE',  ( -13.97604488694527625, -13.89961937509977652, 46.87390960531435979 ) ) ;
#93513=CARTESIAN_POINT ( 'NONE',  ( -16.55341960407611168, -4.379528057220339221, 71.45724293864769550 ) ) ;
#93514=CARTESIAN_POINT ( 'NONE',  ( -16.55341960407611168, -4.379528057220339221, 71.45724293864769550 ) ) ;
#93515=CARTESIAN_POINT ( 'NONE',  ( -16.51473224551069308, -9.474510206698971260, 81.66557627198103830 ) ) ;
#93516=CARTESIAN_POINT ( 'NONE',  ( -5.719274019375978568, 21.55341960407610458, 105.2072429386477097 ) ) ;
#93517=CARTESIAN_POINT ( 'NONE',  ( -16.51473224551069308, -9.474510206698971260, 71.66557627198102409 ) ) ;
#93518=EDGE_CURVE ( 'NONE', #52144, #99274, #52617, .T. ) ;
#93519=CARTESIAN_POINT ( 'NONE',  ( -18.62759615963255300, -10.81492255796106328, 109.1677570613523613 ) ) ;
#93520=CARTESIAN_POINT ( 'NONE',  ( -19.02544592524342804, 5.153800228976336051, 36.04057627198100988 ) ) ;
#93521=CARTESIAN_POINT ( 'NONE',  ( -8.224510206698948167, 14.34966873604960824, 30.41557627198101699 ) ) ;
#93522=CARTESIAN_POINT ( 'NONE',  ( -4.483927247898539470, -16.52544592524342804, 112.2905762719810241 ) ) ;
#93523=CARTESIAN_POINT ( 'NONE',  ( 13.89961937509957401, 13.97604488694547697, 111.8760903946856757 ) ) ;
#93525=CARTESIAN_POINT ( 'NONE',  ( -21.53943276465977519, -0.05219959533937600094, 33.75109039468568284 ) ) ;
#93526=CARTESIAN_POINT ( 'NONE',  ( 19.05341960407617918, -5.049401038297876454, 66.04275706135233293 ) ) ;
#93527=CARTESIAN_POINT ( 'NONE',  ( -16.55341960407611168, -4.379528057220339221, 21.45724293864769550 ) ) ;
#93528=CARTESIAN_POINT ( 'NONE',  ( -18.62759615963270932, 10.81492255796079327, 85.83224293864768129 ) ) ;
#93529=CARTESIAN_POINT ( 'NONE',  ( -21.53943276465977519, 0.05219959533907696930, 26.24890960531435624 ) ) ;
#93530=CARTESIAN_POINT ( 'NONE',  ( 16.53943276465976808, -0.05219959533910856209, 58.74890960531436690 ) ) ;
#93531=CARTESIAN_POINT ( 'NONE',  ( 19.05341960407611168, 5.049401038298154454, 28.95724293864769550 ) ) ;
#93532=CARTESIAN_POINT ( 'NONE',  ( -9.474510206698720793, -16.51473224551083518, 24.58442372801900078 ) ) ;
#93533=CARTESIAN_POINT ( 'NONE',  ( -16.52544592524335698, -4.483927247898792601, 93.95942372801903275 ) ) ;
#93534=CARTESIAN_POINT ( 'NONE',  ( -16.52544592524335698, -4.483927247898792601, 58.95942372801902565 ) ) ;
#93535=CARTESIAN_POINT ( 'NONE',  ( -15.80617190586745835, -15.72974639402198527, 21.87390960531436690 ) ) ;
#93536=CARTESIAN_POINT ( 'NONE',  ( -16.46253265017146816, -9.564922557961047289, 19.16775706135233293 ) ) ;
#93537=CARTESIAN_POINT ( 'NONE',  ( 16.51473224551069308, 9.474510206698969483, 79.16557627198103830 ) ) ;
#93538=CARTESIAN_POINT ( 'NONE',  ( -12.06949235617739369, -12.14591786802326823, 54.37609039468568994 ) ) ;
#93539=CARTESIAN_POINT ( 'NONE',  ( 13.89961937509977652, -13.97604488694527269, 23.12390960531436335 ) ) ;
#93540=CARTESIAN_POINT ( 'NONE',  ( 4.379528057220339221, -16.55341960407611168, 37.70724293864769550 ) ) ;
#93542=CARTESIAN_POINT ( 'NONE',  ( -0.05219959533937732626, 21.53943276465977519, 72.50109039468568994 ) ) ;
#93543=CARTESIAN_POINT ( 'NONE',  ( -9.474510206698964154, 16.51473224551069663, 90.41557627198103830 ) ) ;
#93544=CARTESIAN_POINT ( 'NONE',  ( 19.02544592524343514, -5.153800228976328945, 73.54057627198103830 ) ) ;
#93545=CARTESIAN_POINT ( 'NONE',  ( -9.474510206698964154, 16.51473224551069663, 105.4155762719810383 ) ) ;
#93546=CARTESIAN_POINT ( 'NONE',  ( -8.224510206698948167, 14.34966873604960824, 60.41557627198102409 ) ) ;
#93547=CARTESIAN_POINT ( 'NONE',  ( -16.55341960407611168, -4.379528057220339221, 31.45724293864769550 ) ) ;
#93548=CARTESIAN_POINT ( 'NONE',  ( 16.53943276465976808, -0.05219959533910856209, 48.74890960531435979 ) ) ;
#93549=CARTESIAN_POINT ( 'NONE',  ( 14.29746914071037800, 8.314922557961029526, 36.66775706135234714 ) ) ;
#93550=CARTESIAN_POINT ( 'NONE',  ( 30.00000000000000000, -5.499999999999992895, 102.5000000000000142 ) ) ;
#93551=CARTESIAN_POINT ( 'NONE',  ( 5.153800228976615827, -19.02544592524334988, 45.20942372801901143 ) ) ;
#93552=CARTESIAN_POINT ( 'NONE',  ( 0.05219959533909260263, 19.03943276465977164, 69.99890960531435269 ) ) ;
#93553=CARTESIAN_POINT ( 'NONE',  ( 19.02544592524334988, 5.153800228976608722, 46.45942372801899012 ) ) ;
#93554=CARTESIAN_POINT ( 'NONE',  ( 13.89961937509957401, 13.97604488694547697, 61.87609039468566863 ) ) ;
#93555=CARTESIAN_POINT ( 'NONE',  ( 13.97604488694548053, -13.89961937509957401, 100.6260903946856615 ) ) ;
#93556=CARTESIAN_POINT ( 'NONE',  ( 12.14591786802327356, -12.06949235617739191, 85.62609039468568994 ) ) ;
#93559=CARTESIAN_POINT ( 'NONE',  ( 5.153800228976335163, 19.02544592524342804, 104.7905762719809957 ) ) ;
#93560=CARTESIAN_POINT ( 'NONE',  ( -10.81492255796105439, 18.62759615963255655, 37.91775706135235424 ) ) ;
#93561=CARTESIAN_POINT ( 'NONE',  ( -5.049401038297874678, -19.05341960407617918, 84.79275706135233293 ) ) ;
#93563=CARTESIAN_POINT ( 'NONE',  ( 5.049401038298161559, -19.05341960407611168, 67.70724293864769550 ) ) ;
#93564=CARTESIAN_POINT ( 'NONE',  ( -5.153800228976328057, -19.02544592524343514, 102.2905762719810383 ) ) ;
#93565=CARTESIAN_POINT ( 'NONE',  ( 8.224510206698953496, -14.34966873604960469, 57.91557627198103120 ) ) ;
#93566=CARTESIAN_POINT ( 'NONE',  ( 19.03943276465977164, -0.05219959533909143690, 63.74890960531435979 ) ) ;
#93567=CARTESIAN_POINT ( 'NONE',  ( -13.97604488694527625, -13.89961937509977652, 56.87390960531434558 ) ) ;
#93568=CARTESIAN_POINT ( 'NONE',  ( -19.02544592524334988, -5.153800228976617603, 63.95942372801899012 ) ) ;
#93569=B_SPLINE_CURVE_WITH_KNOTS ( 'NONE', 3,
 ( #33563, #138743, #46750, #141727, #2221, #31577, #63903, #48740, #172076, #95225, #3217, #156911, #44763, #128536, #97194, #49726, #143713, #19393, #146708, #82017, #113372, #4198, #144709, #100206, #98183, #115390, #85028, #192232, #177078, #37537, #176070, #190231 ),
 .UNSPECIFIED., .F., .F.,
 ( 4, 2, 2, 2, 2, 2, 2, 2, 2, 2, 2, 2, 2, 2, 2, 4 ),
 ( 1.734723475976807094E-18, 0.0003712461730036656360, 0.0007424923460073295373, 0.001113738519010993439, 0.001484984692014657340, 0.002227477038021991648, 0.002598723211025670294, 0.002969969384029348940, 0.003341215557033027587, 0.003712461730036706667, 0.004083707903040384446, 0.004454954076044063092, 0.004826200249047741739, 0.005197446422051420385, 0.005568692595055098164, 0.005939938768058776811 ),
 .UNSPECIFIED. ) ;
#93570=CARTESIAN_POINT ( 'NONE',  ( -10.72451020669898014, 18.67979575497178502, 45.41557627198103830 ) ) ;
#93571=CARTESIAN_POINT ( 'NONE',  ( -13.97604488694547697, 13.89961937509957934, 43.12609039468566152 ) ) ;
#93572=CARTESIAN_POINT ( 'NONE',  ( -5.153800228976328057, -19.02544592524343514, 77.29057627198099567 ) ) ;
#93573=CARTESIAN_POINT ( 'NONE',  ( -5.823673210054116645, -21.52544592524344225, 77.29057627198102409 ) ) ;
#93574=CARTESIAN_POINT ( 'NONE',  ( 16.55341960407611168, 4.379528057220329451, 78.95724293864769550 ) ) ;
#93575=CARTESIAN_POINT ( 'NONE',  ( -13.89961937509957401, -13.97604488694547875, 39.37609039468566152 ) ) ;
#93576=CARTESIAN_POINT ( 'NONE',  ( -21.55341960407610458, -5.719274019375992779, 41.45724293864769550 ) ) ;
#93577=CARTESIAN_POINT ( 'NONE',  ( -0.05219959533907301413, -21.53943276465977519, 42.49890960531435979 ) ) ;
#93578=CARTESIAN_POINT ( 'NONE',  ( -13.97604488694527625, -13.89961937509977652, 66.87390960531436690 ) ) ;
#93579=CARTESIAN_POINT ( 'NONE',  ( -0.05219959533909027116, -19.03943276465977164, 57.49890960531435979 ) ) ;
#93580=CARTESIAN_POINT ( 'NONE',  ( -12.06949235617756955, 12.14591786802309770, 115.6239096053143669 ) ) ;
#93581=CARTESIAN_POINT ( 'NONE',  ( 18.67979575497194134, -10.72451020669871369, 25.83442372801901499 ) ) ;
#93582=CARTESIAN_POINT ( 'NONE',  ( -13.89961937509977652, 13.97604488694528158, 110.6239096053143243 ) ) ;
#93583=CARTESIAN_POINT ( 'NONE',  ( 21.53943276465977519, 0.05219959533937863772, 36.25109039468567573 ) ) ;
#93584=CARTESIAN_POINT ( 'NONE',  ( 19.05341960407611168, 5.049401038298154454, 38.95724293864767418 ) ) ;
#93585=CARTESIAN_POINT ( 'NONE',  ( -18.62759615963270932, 10.81492255796079327, 110.8322429386476955 ) ) ;
#93586=CARTESIAN_POINT ( 'NONE',  ( 16.46253265017146816, 9.564922557961045513, 51.66775706135233293 ) ) ;
#93589=CARTESIAN_POINT ( 'NONE',  ( 16.26219239814447093, -7.340408916676126161, 21.79031256471339617 ) ) ;
#93590=CARTESIAN_POINT ( 'NONE',  ( -0.05219959533934338120, 16.53943276465976808, 62.50109039468568284 ) ) ;
#93591=CARTESIAN_POINT ( 'NONE',  ( 5.153800228976335163, 19.02544592524342804, 24.79057627198102765 ) ) ;
#93593=CARTESIAN_POINT ( 'NONE',  ( 5.049401038298161559, -19.05341960407611168, 67.70724293864769550 ) ) ;
#93594=CARTESIAN_POINT ( 'NONE',  ( 8.314922557960818139, 14.29746914071049879, 109.5822429386476955 ) ) ;
#93595=CARTESIAN_POINT ( 'NONE',  ( 21.53943276465977519, -0.05219959533907433946, 58.74890960531436690 ) ) ;
#93596=CARTESIAN_POINT ( 'NONE',  ( -16.52544592524342804, 4.483927247898546575, 81.04057627198102409 ) ) ;
#93597=CARTESIAN_POINT ( 'NONE',  ( 8.224510206698742110, 14.34966873604972548, 32.08442372801901854 ) ) ;
#93598=CARTESIAN_POINT ( 'NONE',  ( -21.53943276465977519, -0.05219959533937600094, 88.75109039468567573 ) ) ;
#93599=CARTESIAN_POINT ( 'NONE',  ( 9.564922557960805705, 16.46253265017160317, 29.58224293864769550 ) ) ;
#93600=CARTESIAN_POINT ( 'NONE',  ( 14.34966873604960469, 8.224510206698951720, 24.16557627198103120 ) ) ;
#93601=CARTESIAN_POINT ( 'NONE',  ( 12.14591786802309770, 12.06949235617756955, 59.37390960531436690 ) ) ;
#93603=CARTESIAN_POINT ( 'NONE',  ( -13.97604488694527625, -13.89961937509977652, 46.87390960531435979 ) ) ;
#93604=CARTESIAN_POINT ( 'NONE',  ( 10.72451020669871369, 18.67979575497193778, 102.0844237280190185 ) ) ;
#93605=CARTESIAN_POINT ( 'NONE',  ( 5.719274019375991003, -21.55341960407610458, 102.7072429386476955 ) ) ;
#93606=CARTESIAN_POINT ( 'NONE',  ( -10.81492255796105439, 18.62759615963255655, 77.91775706135231871 ) ) ;
#93607=CARTESIAN_POINT ( 'NONE',  ( 12.06949235617739724, 12.14591786802326823, 56.87609039468568994 ) ) ;
#93608=CARTESIAN_POINT ( 'NONE',  ( 8.314922557960818139, 14.29746914071049879, 84.58224293864769550 ) ) ;
#93609=CARTESIAN_POINT ( 'NONE',  ( -18.67979575497193778, 10.72451020669871902, 88.33442372801901854 ) ) ;
#93610=CARTESIAN_POINT ( 'NONE',  ( -4.379528057220086978, -16.55341960407618274, 109.7927570613523613 ) ) ;
#93611=CARTESIAN_POINT ( 'NONE',  ( -16.29526858892874586, 7.335722546920134590, 114.2032940219979906 ) ) ;
#93612=CARTESIAN_POINT ( 'NONE',  ( 16.53943276465976808, 0.05219959533934440121, 41.25109039468568284 ) ) ;
#93613=CARTESIAN_POINT ( 'NONE',  ( -4.379528057220328563, 16.55341960407611168, 45.20724293864769550 ) ) ;
#93614=CARTESIAN_POINT ( 'NONE',  ( -14.29746914071037622, -8.314922557961029526, 84.16775706135234714 ) ) ;
#93615=CARTESIAN_POINT ( 'NONE',  ( 13.97604488694527802, 13.89961937509977652, 104.3739096053143385 ) ) ;
#93616=CARTESIAN_POINT ( 'NONE',  ( 16.46253265017160672, -9.564922557960803928, 108.3322429386476955 ) ) ;
#93617=CARTESIAN_POINT ( 'NONE',  ( 10.72451020669871369, 18.67979575497193778, 97.08442372801904696 ) ) ;
#93618=CARTESIAN_POINT ( 'NONE',  ( 4.379528057220092307, 16.55341960407617563, 102.2927570613523613 ) ) ;
#93619=CARTESIAN_POINT ( 'NONE',  ( 8.224510206698953496, -14.34966873604960469, 77.91557627198102409 ) ) ;
#93620=CARTESIAN_POINT ( 'NONE',  ( -13.97604488694527625, -13.89961937509977652, 76.87390960531433848 ) ) ;
#93621=ORIENTED_EDGE ( 'NONE', *, *, #174158, .F. ) ;
#93622=( BOUNDED_CURVE ( )  B_SPLINE_CURVE ( 2, ( #43610, #163980, #73962, #167941, #41629, #165967, #28464, #149794, #13275, #71951, #27469, #135630, #117454 ),
 .UNSPECIFIED., .F., .F. ) 
 B_SPLINE_CURVE_WITH_KNOTS ( ( 3, 2, 2, 2, 2, 2, 3 ),
 ( 0.2919498004596616791, 0.2938596491228070429, 0.2982456140350877027, 0.3026315789473684181, 0.3070175438596491335, 0.3114035087719298489, 0.3133590372571655180 ),
 .UNSPECIFIED. ) 
 CURVE ( )  GEOMETRIC_REPRESENTATION_ITEM ( )  RATIONAL_B_SPLINE_CURVE ( ( 0.9832469066685285419, 0.9851625545550100060, 1.000000000000000000, 0.9659258262890683122, 1.000000000000000000, 0.9659258262890683122, 1.000000000000000000, 0.9659258262890683122, 1.000000000000000000, 0.9659258262890683122, 1.000000000000000000, 0.9848076720550081875, 0.9831626618144004848 ) ) 
 REPRESENTATION_ITEM ( '' )  );
#93623=CARTESIAN_POINT ( 'NONE',  ( -8.314922557961024197, 14.29746914071037800, 32.91775706135234714 ) ) ;
#93624=CARTESIAN_POINT ( 'NONE',  ( -16.51473224551069308, -9.474510206698971260, 31.66557627198102054 ) ) ;
#93625=CARTESIAN_POINT ( 'NONE',  ( -5.049401038298153566, 19.05341960407611168, 85.20724293864766707 ) ) ;
#93626=CARTESIAN_POINT ( 'NONE',  ( 12.14591786802327356, -12.06949235617739191, 25.62609039468567929 ) ) ;
#93628=CARTESIAN_POINT ( 'NONE',  ( -16.46253265017146816, -9.564922557961047289, 39.16775706135234003 ) ) ;
#93629=CARTESIAN_POINT ( 'NONE',  ( -8.314922557961024197, 14.29746914071037800, 87.91775706135234714 ) ) ;
#93630=CARTESIAN_POINT ( 'NONE',  ( -13.97604488694547697, 13.89961937509957934, 103.1260903946856473 ) ) ;
#93631=CARTESIAN_POINT ( 'NONE',  ( 16.51473224551069308, 9.474510206698969483, 39.16557627198103120 ) ) ;
#93632=CARTESIAN_POINT ( 'NONE',  ( 14.34966873604972726, -8.224510206698740333, 85.83442372801901854 ) ) ;
#93633=CARTESIAN_POINT ( 'NONE',  ( -14.29746914071037622, -8.314922557961029526, 64.16775706135234714 ) ) ;
#93634=CARTESIAN_POINT ( 'NONE',  ( -9.564922557961040184, 16.46253265017147172, 87.91775706135233293 ) ) ;
#93635=CARTESIAN_POINT ( 'NONE',  ( -13.89961937509957401, -13.97604488694547875, 19.37609039468566507 ) ) ;
#93636=CARTESIAN_POINT ( 'NONE',  ( -5.153800228976328057, -19.02544592524343514, 42.29057627198101699 ) ) ;
#93637=CARTESIAN_POINT ( 'NONE',  ( 16.51473224551069308, 9.474510206698969483, 94.16557627198103830 ) ) ;
#93638=CARTESIAN_POINT ( 'NONE',  ( 4.379528057220339221, -16.55341960407611168, 82.70724293864770971 ) ) ;
#93640=CARTESIAN_POINT ( 'NONE',  ( 5.049401038297881783, 19.05341960407617563, 52.29275706135234003 ) ) ;
#93641=CARTESIAN_POINT ( 'NONE',  ( 18.67979575497178502, 10.72451020669898547, 44.16557627198103120 ) ) ;
#93642=CARTESIAN_POINT ( 'NONE',  ( 16.46253265017146816, 9.564922557961045513, 26.66775706135234003 ) ) ;
#93643=CARTESIAN_POINT ( 'NONE',  ( -16.46253265017160317, 9.564922557960807481, 90.83224293864769550 ) ) ;
#93644=CARTESIAN_POINT ( 'NONE',  ( -19.02544592524334988, -5.153800228976617603, 28.95942372801900433 ) ) ;
#93645=CARTESIAN_POINT ( 'NONE',  ( 21.53943276465977519, -0.05219959533907433946, 73.74890960531433848 ) ) ;
#93646=CARTESIAN_POINT ( 'NONE',  ( 19.05341960407611168, 5.049401038298154454, 108.9572429386477097 ) ) ;
#93647=CARTESIAN_POINT ( 'NONE',  ( 19.02544592524334988, 5.153800228976608722, 86.45942372801900433 ) ) ;
#93648=CARTESIAN_POINT ( 'NONE',  ( -17.49999999999999645, 5.499999999999997335, 110.7969038253417295 ) ) ;
#93649=CARTESIAN_POINT ( 'NONE',  ( 19.03943276465977164, 0.05219959533936151252, 106.2510903946856615 ) ) ;
#93650=CARTESIAN_POINT ( 'NONE',  ( 16.46253265017160672, -9.564922557960803928, 28.33224293864769550 ) ) ;
#93651=CARTESIAN_POINT ( 'NONE',  ( -13.89961937509977652, 13.97604488694528158, 95.62390960531436690 ) ) ;
#93652=CARTESIAN_POINT ( 'NONE',  ( -21.53943276465977519, 0.05219959533907696930, 71.24890960531435269 ) ) ;
#93653=CARTESIAN_POINT ( 'NONE',  ( 12.06949235617739724, 12.14591786802326823, 41.87609039468568284 ) ) ;
#93654=CARTESIAN_POINT ( 'NONE',  ( -15.80617190586768217, 15.72974639402176855, 48.12609039468568284 ) ) ;
#93655=CARTESIAN_POINT ( 'NONE',  ( -19.03943276465977164, -0.05219959533935918106, 93.75109039468566152 ) ) ;
#93656=CARTESIAN_POINT ( 'NONE',  ( -15.80617190586768217, 15.72974639402176855, 93.12609039468568994 ) ) ;
#93657=CARTESIAN_POINT ( 'NONE',  ( -12.06949235617739369, -12.14591786802326823, 99.37609039468568994 ) ) ;
#93658=CARTESIAN_POINT ( 'NONE',  ( -5.049401038298153566, 19.05341960407611168, 100.2072429386476955 ) ) ;
#93659=CARTESIAN_POINT ( 'NONE',  ( 12.14591786802309770, 12.06949235617756955, 89.37390960531435269 ) ) ;
#93660=CARTESIAN_POINT ( 'NONE',  ( 16.55341960407611168, 4.379528057220329451, 33.95724293864769550 ) ) ;
#93661=CARTESIAN_POINT ( 'NONE',  ( -0.05219959533936034679, 19.03943276465977164, 67.50109039468566152 ) ) ;
#93662=CARTESIAN_POINT ( 'NONE',  ( 15.72974639402176855, 15.80617190586768217, 56.87609039468568994 ) ) ;
#93663=CARTESIAN_POINT ( 'NONE',  ( 16.51473224551083163, -9.474510206698727899, 30.83442372801900433 ) ) ;
#93664=CARTESIAN_POINT ( 'NONE',  ( -4.379528057220328563, 16.55341960407611168, 110.2072429386477239 ) ) ;
#93665=CARTESIAN_POINT ( 'NONE',  ( -21.55341960407610458, -5.719274019375992779, 26.45724293864768839 ) ) ;
#93666=CARTESIAN_POINT ( 'NONE',  ( 16.55341960407611168, 4.379528057220329451, 23.95724293864769550 ) ) ;
#93667=CARTESIAN_POINT ( 'NONE',  ( 18.62759615963255655, 10.81492255796105972, 96.66775706135234714 ) ) ;
#93668=CARTESIAN_POINT ( 'NONE',  ( 4.483927247898790824, -16.52544592524335698, 60.20942372801902565 ) ) ;
#93669=CARTESIAN_POINT ( 'NONE',  ( 12.14591786802309770, 12.06949235617756955, 24.37390960531435979 ) ) ;
#93670=CARTESIAN_POINT ( 'NONE',  ( 21.52544592524334988, 5.823673210054432836, 46.45942372801901854 ) ) ;
#93671=CARTESIAN_POINT ( 'NONE',  ( -10.72451020669870658, -18.67979575497194134, 49.58442372801901143 ) ) ;
#93672=EDGE_CURVE ( 'NONE', #121093, #78133, #25042, .T. ) ;
#93673=VERTEX_POINT ( 'NONE', #40179 ) ;
#93675=CARTESIAN_POINT ( 'NONE',  ( -21.55341960407619339, 5.719274019375674811, 23.54275706135235424 ) ) ;
#93676=CARTESIAN_POINT ( 'NONE',  ( -14.34966873604960291, -8.224510206698953496, 106.6655762719810383 ) ) ;
#93677=CARTESIAN_POINT ( 'NONE',  ( -16.51473224551069308, -9.474510206698971260, 26.66557627198103120 ) ) ;
#93678=CARTESIAN_POINT ( 'NONE',  ( 14.34966873604960469, 8.224510206698951720, 79.16557627198103830 ) ) ;
#93679=CARTESIAN_POINT ( 'NONE',  ( -5.049401038298153566, 19.05341960407611168, 75.20724293864769550 ) ) ;
#93680=CARTESIAN_POINT ( 'NONE',  ( -8.224510206698735004, -14.34966873604973081, 104.5844237280190185 ) ) ;
#93681=CARTESIAN_POINT ( 'NONE',  ( 21.55341960407610458, 5.719274019375980345, 58.95724293864770971 ) ) ;
#93682=CARTESIAN_POINT ( 'NONE',  ( -8.314922557960811034, -14.29746914071050412, 87.08224293864769550 ) ) ;
#93683=CARTESIAN_POINT ( 'NONE',  ( 0.05219959533907565091, 21.53943276465977519, 89.99890960531438111 ) ) ;
#93684=CARTESIAN_POINT ( 'NONE',  ( 19.05341960407611168, 5.049401038298154454, 103.9572429386476671 ) ) ;
#93685=CARTESIAN_POINT ( 'NONE',  ( -13.89961937509977652, 13.97604488694528158, 50.62390960531435979 ) ) ;
#93686=CARTESIAN_POINT ( 'NONE',  ( 16.51473224551083163, -9.474510206698727899, 110.8344237280190043 ) ) ;
#93687=CARTESIAN_POINT ( 'NONE',  ( 0.05219959533907565091, 21.53943276465977519, 39.99890960531436690 ) ) ;
#93688=CARTESIAN_POINT ( 'NONE',  ( -10.81492255796105439, 18.62759615963255655, 62.91775706135236135 ) ) ;
#93689=CARTESIAN_POINT ( 'NONE',  ( -5.153800228976328057, -19.02544592524343514, 62.29057627198100988 ) ) ;
#93690=CARTESIAN_POINT ( 'NONE',  ( 16.51473224551069308, 9.474510206698969483, 94.16557627198103830 ) ) ;
#93691=CARTESIAN_POINT ( 'NONE',  ( 0.05219959533934541429, -16.53943276465976808, 70.00109039468568994 ) ) ;
#93692=CARTESIAN_POINT ( 'NONE',  ( -5.823673210054431948, 21.52544592524334988, 52.70942372801902565 ) ) ;
#93693=CARTESIAN_POINT ( 'NONE',  ( 5.823673210054444382, -21.52544592524334988, 85.20942372801901854 ) ) ;
#93694=CARTESIAN_POINT ( 'NONE',  ( -5.719274019375978568, 21.55341960407610458, 95.20724293864769550 ) ) ;
#93695=CARTESIAN_POINT ( 'NONE',  ( 18.62759615963255655, 10.81492255796105972, 36.66775706135234714 ) ) ;
#93696=CARTESIAN_POINT ( 'NONE',  ( -16.53943276465976808, -0.05219959533934237506, 73.75109039468567573 ) ) ;
#93697=CARTESIAN_POINT ( 'NONE',  ( -15.80617190586745835, -15.72974639402198527, 76.87390960531439532 ) ) ;
#93698=CARTESIAN_POINT ( 'NONE',  ( -9.474510206698720793, -16.51473224551083518, 39.58442372801899722 ) ) ;
#93699=CARTESIAN_POINT ( 'NONE',  ( -19.03943276465977164, 0.05219959533909376836, 81.24890960531436690 ) ) ;
#93700=CARTESIAN_POINT ( 'NONE',  ( -16.53943276465976808, 0.05219959533911058130, 21.24890960531436690 ) ) ;
#93702=CARTESIAN_POINT ( 'NONE',  ( 16.51473224551069308, 9.474510206698969483, 109.1655762719810383 ) ) ;
#93704=CARTESIAN_POINT ( 'NONE',  ( 13.97604488694548053, -13.89961937509957401, 95.62609039468563310 ) ) ;
#93705=CARTESIAN_POINT ( 'NONE',  ( 15.72974639402199770, -15.80617190586745480, 78.12390960531436690 ) ) ;
#93706=CARTESIAN_POINT ( 'NONE',  ( 16.53943276465976808, -0.05219959533910856209, 38.74890960531435979 ) ) ;
#93707=CARTESIAN_POINT ( 'NONE',  ( 14.34966873604972726, -8.224510206698740333, 20.83442372801901143 ) ) ;
#93708=CARTESIAN_POINT ( 'NONE',  ( -19.02544592524342804, 5.153800228976336051, 26.04057627198103120 ) ) ;
#93709=CARTESIAN_POINT ( 'NONE',  ( -5.153800228976607833, 19.02544592524334988, 112.7094237280190043 ) ) ;
#93710=CARTESIAN_POINT ( 'NONE',  ( -15.72974639402197994, 15.80617190586746368, 100.6239096053143811 ) ) ;
#93711=CARTESIAN_POINT ( 'NONE',  ( 19.02544592524334988, 5.153800228976608722, 71.45942372801900433 ) ) ;
#93712=CARTESIAN_POINT ( 'NONE',  ( 16.52544592524335698, 4.483927247898782831, 81.45942372801900433 ) ) ;
#93713=CARTESIAN_POINT ( 'NONE',  ( -9.564922557960796823, -16.46253265017161027, 72.08224293864770971 ) ) ;
#93714=CARTESIAN_POINT ( 'NONE',  ( 14.34966873604960469, 8.224510206698951720, 74.16557627198102409 ) ) ;
#93715=CARTESIAN_POINT ( 'NONE',  ( 9.564922557960805705, 16.46253265017160317, 59.58224293864769550 ) ) ;
#93716=CARTESIAN_POINT ( 'NONE',  ( 8.224510206698953496, -14.34966873604960469, 67.91557627198102409 ) ) ;
#93719=CARTESIAN_POINT ( 'NONE',  ( -16.55341960407611168, -4.379528057220339221, 41.45724293864769550 ) ) ;
#93720=CARTESIAN_POINT ( 'NONE',  ( 9.474510206698971260, -16.51473224551069308, 82.91557627198103830 ) ) ;
#93722=CARTESIAN_POINT ( 'NONE',  ( 9.564922557961047289, -16.46253265017146816, 55.41775706135234003 ) ) ;
#93723=CARTESIAN_POINT ( 'NONE',  ( 14.34966873604972726, -8.224510206698740333, 55.83442372801901854 ) ) ;
#93724=CARTESIAN_POINT ( 'NONE',  ( -15.80617190586745835, -15.72974639402198527, 61.87390960531436690 ) ) ;
#93725=CARTESIAN_POINT ( 'NONE',  ( -9.474510206698720793, -16.51473224551083518, 19.58442372801899722 ) ) ;
#93726=CARTESIAN_POINT ( 'NONE',  ( -19.05341960407611168, -5.049401038298163336, 81.45724293864769550 ) ) ;
#93728=CARTESIAN_POINT ( 'NONE',  ( -18.67979575497178146, -10.72451020669898902, 21.66557627198102409 ) ) ;
#93729=CARTESIAN_POINT ( 'NONE',  ( 19.02544592524343514, -5.153800228976328945, 58.54057627198102409 ) ) ;
#93730=CARTESIAN_POINT ( 'NONE',  ( -18.67979575497193778, 10.72451020669871902, 33.33442372801900433 ) ) ;
#93732=CARTESIAN_POINT ( 'NONE',  ( 4.379528057220339221, -16.55341960407611168, 107.7072429386476955 ) ) ;
#93733=CARTESIAN_POINT ( 'NONE',  ( -0.05219959533907301413, -21.53943276465977519, 97.49890960531436690 ) ) ;
#93734=CARTESIAN_POINT ( 'NONE',  ( 16.46253265017160672, -9.564922557960803928, 98.33224293864769550 ) ) ;
#93736=CARTESIAN_POINT ( 'NONE',  ( 18.62759615963255655, 10.81492255796105972, 21.66775706135235069 ) ) ;
#93738=CARTESIAN_POINT ( 'NONE',  ( -9.564922557960796823, -16.46253265017161027, 87.08224293864769550 ) ) ;
#93740=CARTESIAN_POINT ( 'NONE',  ( -21.52544592524343514, 5.823673210054127303, 91.04057627198103830 ) ) ;
#93741=CARTESIAN_POINT ( 'NONE',  ( -13.97604488694527625, -13.89961937509977652, 46.87390960531435979 ) ) ;
#93742=CARTESIAN_POINT ( 'NONE',  ( -16.51473224551082808, 9.474510206698731452, 103.3344237280190043 ) ) ;
#93744=CARTESIAN_POINT ( 'NONE',  ( 9.474510206698971260, -16.51473224551069308, 27.91557627198103120 ) ) ;
#93745=CARTESIAN_POINT ( 'NONE',  ( -5.719274019375665041, -21.55341960407619695, 89.79275706135236135 ) ) ;
#93746=CARTESIAN_POINT ( 'NONE',  ( 16.46253265017160672, -9.564922557960803928, 78.33224293864769550 ) ) ;
#93747=CARTESIAN_POINT ( 'NONE',  ( -15.72974639402176322, -15.80617190586768395, 49.37609039468569705 ) ) ;
#93748=CARTESIAN_POINT ( 'NONE',  ( -21.55341960407619339, 5.719274019375674811, 23.54275706135235424 ) ) ;
#93750=CARTESIAN_POINT ( 'NONE',  ( -0.05219959533909027116, -19.03943276465977164, 97.49890960531436690 ) ) ;
#93752=CARTESIAN_POINT ( 'NONE',  ( 12.06949235617739724, 12.14591786802326823, 36.87609039468568994 ) ) ;
#93753=CARTESIAN_POINT ( 'NONE',  ( 10.81492255796078972, 18.62759615963270932, 49.58224293864769550 ) ) ;
#93754=CARTESIAN_POINT ( 'NONE',  ( 18.67979575497194134, -10.72451020669871369, 40.83442372801901854 ) ) ;
#93755=CARTESIAN_POINT ( 'NONE',  ( -10.81492255796105439, 18.62759615963255655, 72.91775706135234714 ) ) ;
#93757=CARTESIAN_POINT ( 'NONE',  ( 0.05219959533934541429, -16.53943276465976808, 20.00109039468568639 ) ) ;
#93758=CARTESIAN_POINT ( 'NONE',  ( -9.564922557960796823, -16.46253265017161027, 57.08224293864769550 ) ) ;
#93759=CARTESIAN_POINT ( 'NONE',  ( 13.89961937509977652, -13.97604488694527269, 93.12390960531436690 ) ) ;
#93760=CARTESIAN_POINT ( 'NONE',  ( 12.14591786802309770, 12.06949235617756955, 104.3739096053143669 ) ) ;
#93761=CARTESIAN_POINT ( 'NONE',  ( 16.55341960407611168, 4.379528057220329451, 108.9572429386476955 ) ) ;
#93762=CARTESIAN_POINT ( 'NONE',  ( -21.52544592524343514, 5.823673210054127303, 36.04057627198102409 ) ) ;
#93763=CARTESIAN_POINT ( 'NONE',  ( 14.34966873604972726, -8.224510206698740333, 85.83442372801901854 ) ) ;
#93764=CARTESIAN_POINT ( 'NONE',  ( -12.06949235617756955, 12.14591786802309770, 65.62390960531436690 ) ) ;
#93765=CARTESIAN_POINT ( 'NONE',  ( 19.03943276465977164, -0.05219959533909143690, 53.74890960531436690 ) ) ;
#93766=CARTESIAN_POINT ( 'NONE',  ( -21.52544592524334988, -5.823673210054445271, 73.95942372801901854 ) ) ;
#93767=CARTESIAN_POINT ( 'NONE',  ( -21.55341960407619339, 5.719274019375674811, 73.54275706135234714 ) ) ;
#93768=CARTESIAN_POINT ( 'NONE',  ( -19.02544592524334988, -5.153800228976617603, 103.9594237280190043 ) ) ;
#93769=CARTESIAN_POINT ( 'NONE',  ( 4.483927247898545687, 16.52544592524342804, 64.79057627198103830 ) ) ;
#93770=CARTESIAN_POINT ( 'NONE',  ( -21.52544592524334988, -5.823673210054445271, 23.95942372801901143 ) ) ;
#93771=CARTESIAN_POINT ( 'NONE',  ( 10.81492255796078972, 18.62759615963270932, 54.58224293864769550 ) ) ;
#93772=CARTESIAN_POINT ( 'NONE',  ( 18.22780087662121673, 5.500000000000056843, 73.98459894673894155 ) ) ;
#93774=CARTESIAN_POINT ( 'NONE',  ( 13.97604488694527802, 13.89961937509977652, 64.37390960531436690 ) ) ;
#93775=CARTESIAN_POINT ( 'NONE',  ( -8.314922557960811034, -14.29746914071050412, 37.08224293864768129 ) ) ;
#93776=CARTESIAN_POINT ( 'NONE',  ( 16.53943276465976808, -0.05219959533910856209, 23.74890960531435269 ) ) ;
#93777=CARTESIAN_POINT ( 'NONE',  ( -12.14591786802326823, 12.06949235617739902, 103.1260903946856757 ) ) ;
#93778=CARTESIAN_POINT ( 'NONE',  ( 19.03943276465977164, 0.05219959533936151252, 51.25109039468567573 ) ) ;
#93780=CARTESIAN_POINT ( 'NONE',  ( -5.049401038298153566, 19.05341960407611168, 105.2072429386476671 ) ) ;
#93781=CARTESIAN_POINT ( 'NONE',  ( 14.34966873604960469, 8.224510206698951720, 74.16557627198102409 ) ) ;
#93782=CARTESIAN_POINT ( 'NONE',  ( 5.153800228976615827, -19.02544592524334988, 40.20942372801898301 ) ) ;
#93783=CARTESIAN_POINT ( 'NONE',  ( -19.02544592524342804, 5.153800228976336051, 31.04057627198102409 ) ) ;
#93784=CARTESIAN_POINT ( 'NONE',  ( 21.53943276465977519, -0.05219959533907433946, 23.74890960531435269 ) ) ;
#93785=CARTESIAN_POINT ( 'NONE',  ( 18.62759615963271287, -10.81492255796078972, 53.33224293864769550 ) ) ;
#93787=CARTESIAN_POINT ( 'NONE',  ( -8.314922557960811034, -14.29746914071050412, 97.08224293864770971 ) ) ;
#93788=CARTESIAN_POINT ( 'NONE',  ( -8.224510206698735004, -14.34966873604973081, 49.58442372801901143 ) ) ;
#93789=CARTESIAN_POINT ( 'NONE',  ( 4.379528057220339221, -16.55341960407611168, 87.70724293864769550 ) ) ;
#93791=CARTESIAN_POINT ( 'NONE',  ( -17.31728774477273092, 6.344390552232386682, 50.81906651689320142 ) ) ;
#93792=CARTESIAN_POINT ( 'NONE',  ( -16.46253265017160317, 9.564922557960807481, 110.8322429386476955 ) ) ;
#93795=CARTESIAN_POINT ( 'NONE',  ( 0.05219959533934541429, -16.53943276465976808, 45.00109039468568284 ) ) ;
#93796=CARTESIAN_POINT ( 'NONE',  ( 16.55341960407611168, 4.379528057220329451, 23.95724293864769550 ) ) ;
#93797=CARTESIAN_POINT ( 'NONE',  ( 15.80617190586746368, 15.72974639402197994, 54.37390960531435979 ) ) ;
#93798=CARTESIAN_POINT ( 'NONE',  ( -9.564922557961040184, 16.46253265017147172, 87.91775706135233293 ) ) ;
#93799=CARTESIAN_POINT ( 'NONE',  ( -15.72974639402197994, 15.80617190586746368, 50.62390960531435979 ) ) ;
#93800=CARTESIAN_POINT ( 'NONE',  ( 21.52544592524334988, 5.823673210054432836, 76.45942372801901854 ) ) ;
#93802=CARTESIAN_POINT ( 'NONE',  ( -16.52544592524335698, -4.483927247898792601, 53.95942372801900433 ) ) ;
#93803=CARTESIAN_POINT ( 'NONE',  ( 13.97604488694527802, 13.89961937509977652, 39.37390960531435269 ) ) ;
#93804=CARTESIAN_POINT ( 'NONE',  ( -13.97604488694527625, -13.89961937509977652, 101.8739096053143811 ) ) ;
#93805=EDGE_CURVE ( 'NONE', #9238, #3778, #96651, .T. ) ;
#93806=CARTESIAN_POINT ( 'NONE',  ( -16.51473224551069308, -9.474510206698971260, 36.66557627198102409 ) ) ;
#93807=CARTESIAN_POINT ( 'NONE',  ( -8.314922557960811034, -14.29746914071050412, 102.0822429386476955 ) ) ;
#93808=CARTESIAN_POINT ( 'NONE',  ( 13.89961937509977652, -13.97604488694527269, 98.12390960531433848 ) ) ;
#93810=CARTESIAN_POINT ( 'NONE',  ( 0.05219959533934541429, -16.53943276465976808, 55.00109039468568284 ) ) ;
#93811=CARTESIAN_POINT ( 'NONE',  ( 15.80617190586746368, 15.72974639402197994, 89.37390960531435269 ) ) ;
#93812=CARTESIAN_POINT ( 'NONE',  ( 19.05341960407611168, 5.049401038298154454, 53.95724293864770260 ) ) ;
#93813=CARTESIAN_POINT ( 'NONE',  ( 15.72974639402176855, 15.80617190586768217, 31.87609039468567929 ) ) ;
#93814=CARTESIAN_POINT ( 'NONE',  ( 5.049401038298161559, -19.05341960407611168, 82.70724293864770971 ) ) ;
#93816=ORIENTED_EDGE ( 'NONE', *, *, #162015, .T. ) ;
#93817=CARTESIAN_POINT ( 'NONE',  ( 5.823673210054444382, -21.52544592524334988, 25.20942372801901854 ) ) ;
#93818=CARTESIAN_POINT ( 'NONE',  ( -19.02544592524342804, 5.153800228976336051, 26.04057627198103120 ) ) ;
#93819=CARTESIAN_POINT ( 'NONE',  ( 9.564922557960805705, 16.46253265017160317, 104.5822429386476955 ) ) ;
#93820=CARTESIAN_POINT ( 'NONE',  ( 9.564922557961047289, -16.46253265017146816, 70.41775706135233293 ) ) ;
#93821=CARTESIAN_POINT ( 'NONE',  ( 5.049401038297881783, 19.05341960407617563, 32.29275706135233293 ) ) ;
#93822=CARTESIAN_POINT ( 'NONE',  ( -18.62759615963270932, 10.81492255796079327, 105.8322429386476955 ) ) ;
#93823=CARTESIAN_POINT ( 'NONE',  ( -13.89961937509957401, -13.97604488694547875, 34.37609039468566863 ) ) ;
#93824=CARTESIAN_POINT ( 'NONE',  ( -16.55341960407617563, 4.379528057220093196, 78.54275706135236135 ) ) ;
#93825=CARTESIAN_POINT ( 'NONE',  ( -19.03943276465977164, 0.05219959533909376836, 101.2489096053143669 ) ) ;
#93826=CARTESIAN_POINT ( 'NONE',  ( -13.97604488694527625, -13.89961937509977652, 56.87390960531434558 ) ) ;
#93827=CARTESIAN_POINT ( 'NONE',  ( -0.05219959533937732626, 21.53943276465977519, 72.50109039468568994 ) ) ;
#93828=CARTESIAN_POINT ( 'NONE',  ( 5.823673210054444382, -21.52544592524334988, 80.20942372801901854 ) ) ;
#93829=CARTESIAN_POINT ( 'NONE',  ( 13.89961937509977652, -13.97604488694527269, 73.12390960531436690 ) ) ;
#93830=CARTESIAN_POINT ( 'NONE',  ( -21.53943276465977519, -0.05219959533937600094, 53.75109039468568994 ) ) ;
#93831=CARTESIAN_POINT ( 'NONE',  ( 5.049401038297881783, 19.05341960407617563, 82.29275706135229029 ) ) ;
#93832=CARTESIAN_POINT ( 'NONE',  ( 16.51473224551069308, 9.474510206698969483, 59.16557627198102409 ) ) ;
#93833=CARTESIAN_POINT ( 'NONE',  ( -5.049401038298153566, 19.05341960407611168, 105.2072429386476671 ) ) ;
#93834=CARTESIAN_POINT ( 'NONE',  ( -5.153800228976328057, -19.02544592524343514, 72.29057627198102409 ) ) ;
#93836=CARTESIAN_POINT ( 'NONE',  ( -0.05219959533909027116, -19.03943276465977164, 57.49890960531435979 ) ) ;
#93837=CARTESIAN_POINT ( 'NONE',  ( -10.81492255796078084, -18.62759615963271287, 97.08224293864770971 ) ) ;
#93838=CARTESIAN_POINT ( 'NONE',  ( 14.29746914071037800, 8.314922557961029526, 76.66775706135234714 ) ) ;
#93841=CARTESIAN_POINT ( 'NONE',  ( 19.05341960407617918, -5.049401038297876454, 46.04275706135233293 ) ) ;
#93842=CARTESIAN_POINT ( 'NONE',  ( -13.89961937509977652, 13.97604488694528158, 65.62390960531436690 ) ) ;
#93843=CARTESIAN_POINT ( 'NONE',  ( -4.379528057220328563, 16.55341960407611168, 55.20724293864770260 ) ) ;
#93844=CARTESIAN_POINT ( 'NONE',  ( -14.29746914071049879, 8.314922557960819915, 90.83224293864769550 ) ) ;
#93845=CARTESIAN_POINT ( 'NONE',  ( -5.049401038298153566, 19.05341960407611168, 105.2072429386476671 ) ) ;
#93846=B_SPLINE_CURVE_WITH_KNOTS ( 'NONE', 3,
 ( #167529, #29024, #8856, #10861, #102857, #70523, #132192, #55348, #72530, #40175, #117018, #9860, #71519, #194877, #118033, #164543, #26035, #134207, #195894, #141148 ),
 .UNSPECIFIED., .F., .F.,
 ( 4, 2, 2, 2, 2, 2, 2, 2, 2, 4 ),
 ( 0.004000878361811913142, 0.004499404418915918698, 0.004997930476019923386, 0.005496456533123928942, 0.005994982590227933630, 0.006244245618779935975, 0.006493508647331939186, 0.006992034704435929997, 0.007490560761539919940, 0.007989086818643910751 ),
 .UNSPECIFIED. ) ;
#93847=CARTESIAN_POINT ( 'NONE',  ( -13.89961937509977652, 13.97604488694528158, 90.62390960531432427 ) ) ;
#93848=CARTESIAN_POINT ( 'NONE',  ( 9.564922557960805705, 16.46253265017160317, 99.58224293864770971 ) ) ;
#93849=CARTESIAN_POINT ( 'NONE',  ( -19.03943276465977164, -0.05219959533935918106, 18.75109039468567218 ) ) ;
#93850=CARTESIAN_POINT ( 'NONE',  ( 8.224510206698742110, 14.34966873604972548, 97.08442372801904696 ) ) ;
#93851=CARTESIAN_POINT ( 'NONE',  ( 13.97604488694527802, 13.89961937509977652, 74.37390960531436690 ) ) ;
#93852=CARTESIAN_POINT ( 'NONE',  ( -21.52544592524334988, -5.823673210054445271, 43.95942372801902565 ) ) ;
#93853=CARTESIAN_POINT ( 'NONE',  ( 21.53943276465977519, -0.05219959533907433946, 33.74890960531436690 ) ) ;
#93854=CARTESIAN_POINT ( 'NONE',  ( 18.62759615963271287, -10.81492255796078972, 98.33224293864769550 ) ) ;
#93855=CARTESIAN_POINT ( 'NONE',  ( -16.53943276465976808, 0.05219959533911058130, 56.24890960531436690 ) ) ;
#93856=CARTESIAN_POINT ( 'NONE',  ( -13.97604488694527625, -13.89961937509977652, 56.87390960531434558 ) ) ;
#93857=CARTESIAN_POINT ( 'NONE',  ( -12.14591786802309592, -12.06949235617757132, 86.87390960531438111 ) ) ;
#93858=CARTESIAN_POINT ( 'NONE',  ( -13.89961937509957401, -13.97604488694547875, 39.37609039468566152 ) ) ;
#93859=CARTESIAN_POINT ( 'NONE',  ( 8.224510206698953496, -14.34966873604960469, 107.9155762719810241 ) ) ;
#93861=CARTESIAN_POINT ( 'NONE',  ( -0.05219959533934338120, 16.53943276465976808, 72.50109039468568994 ) ) ;
#93862=CARTESIAN_POINT ( 'NONE',  ( 19.03943276465977164, -0.05219959533909143690, 73.74890960531435269 ) ) ;
#93864=CARTESIAN_POINT ( 'NONE',  ( 14.29746914071049879, -8.314922557960816363, 93.33224293864769550 ) ) ;
#93865=CARTESIAN_POINT ( 'NONE',  ( 5.719274019375991003, -21.55341960407610458, 37.70724293864769550 ) ) ;
#93866=CARTESIAN_POINT ( 'NONE',  ( -0.05219959533934338120, 16.53943276465976808, 107.5010903946856899 ) ) ;
#93867=CARTESIAN_POINT ( 'NONE',  ( 4.483927247898790824, -16.52544592524335698, 25.20942372801901854 ) ) ;
#93868=CARTESIAN_POINT ( 'NONE',  ( -15.80617190586768217, 15.72974639402176855, 93.12609039468568994 ) ) ;
#93869=CARTESIAN_POINT ( 'NONE',  ( 5.049401038298161559, -19.05341960407611168, 87.70724293864769550 ) ) ;
#93870=CARTESIAN_POINT ( 'NONE',  ( -5.719274019375978568, 21.55341960407610458, 115.2072429386476955 ) ) ;
#93871=CARTESIAN_POINT ( 'NONE',  ( 19.03943276465977164, -0.05219959533909143690, 28.74890960531435624 ) ) ;
#93872=EDGE_CURVE ( 'NONE', #65322, #48812, #12576, .T. ) ;
#93873=CARTESIAN_POINT ( 'NONE',  ( -8.224510206698735004, -14.34966873604973081, 29.58442372801901854 ) ) ;
#93874=CARTESIAN_POINT ( 'NONE',  ( 19.02544592524334988, 5.153800228976608722, 91.45942372801900433 ) ) ;
#93875=CARTESIAN_POINT ( 'NONE',  ( 18.67979575497178502, 10.72451020669898547, 84.16557627198103830 ) ) ;
#93876=CARTESIAN_POINT ( 'NONE',  ( -19.05341960407617563, 5.049401038297882671, 68.54275706135230450 ) ) ;
#93877=CARTESIAN_POINT ( 'NONE',  ( -9.474510206698964154, 16.51473224551069663, 25.41557627198103120 ) ) ;
#93878=CARTESIAN_POINT ( 'NONE',  ( -21.53943276465977519, 0.05219959533907696930, 116.2489096053143669 ) ) ;
#93880=CARTESIAN_POINT ( 'NONE',  ( -16.51473224551069308, -9.474510206698971260, 71.66557627198102409 ) ) ;
#93881=CARTESIAN_POINT ( 'NONE',  ( -4.379528057220086978, -16.55341960407618274, 29.79275706135234358 ) ) ;
#93883=CARTESIAN_POINT ( 'NONE',  ( 13.97604488694548053, -13.89961937509957401, 60.62609039468564731 ) ) ;
#93884=CARTESIAN_POINT ( 'NONE',  ( 0.05219959533937995610, -21.53943276465977519, 20.00109039468568639 ) ) ;
#93885=CARTESIAN_POINT ( 'NONE',  ( 8.224510206698953496, -14.34966873604960469, 82.91557627198103830 ) ) ;
#93886=CARTESIAN_POINT ( 'NONE',  ( -5.049401038298153566, 19.05341960407611168, 85.20724293864766707 ) ) ;
#93887=CARTESIAN_POINT ( 'NONE',  ( -8.314922557961024197, 14.29746914071037800, 42.91775706135235424 ) ) ;
#93888=CARTESIAN_POINT ( 'NONE',  ( 9.564922557961047289, -16.46253265017146816, 45.41775706135232582 ) ) ;
#93889=CARTESIAN_POINT ( 'NONE',  ( 10.72451020669871369, 18.67979575497193778, 62.08442372801901143 ) ) ;
#93890=CARTESIAN_POINT ( 'NONE',  ( -0.05219959533934338120, 16.53943276465976808, 32.50109039468568284 ) ) ;
#93891=CARTESIAN_POINT ( 'NONE',  ( -16.51473224551069308, -9.474510206698971260, 61.66557627198103120 ) ) ;
#93892=CARTESIAN_POINT ( 'NONE',  ( -5.153800228976607833, 19.02544592524334988, 77.70942372801900433 ) ) ;
#93893=CARTESIAN_POINT ( 'NONE',  ( 14.29746914071037800, 8.314922557961029526, 51.66775706135234714 ) ) ;
#93894=CARTESIAN_POINT ( 'NONE',  ( -21.52544592524334988, -5.823673210054445271, 98.95942372801903275 ) ) ;
#93895=CARTESIAN_POINT ( 'NONE',  ( 16.46253265017146816, 9.564922557961045513, 66.66775706135233293 ) ) ;
#93896=CARTESIAN_POINT ( 'NONE',  ( 0.05219959533909260263, 19.03943276465977164, 54.99890960531435979 ) ) ;
#93897=CARTESIAN_POINT ( 'NONE',  ( -18.67979575497178146, -10.72451020669898902, 71.66557627198100988 ) ) ;
#93898=CARTESIAN_POINT ( 'NONE',  ( -16.53943276465976808, 0.05219959533911058130, 61.24890960531435979 ) ) ;
#93899=CARTESIAN_POINT ( 'NONE',  ( 9.564922557961047289, -16.46253265017146816, 65.41775706135233293 ) ) ;
#93900=CARTESIAN_POINT ( 'NONE',  ( -19.19724070472094013, -5.500000000000084377, 71.06193348274381094 ) ) ;
#93901=CARTESIAN_POINT ( 'NONE',  ( 0.05219959533936267826, -19.03943276465977164, 50.00109039468566863 ) ) ;
#93902=CARTESIAN_POINT ( 'NONE',  ( -16.52544592524335698, -4.483927247898792601, 98.95942372801903275 ) ) ;
#93903=CARTESIAN_POINT ( 'NONE',  ( -8.224510206698948167, 14.34966873604960824, 65.41557627198102409 ) ) ;
#93904=CARTESIAN_POINT ( 'NONE',  ( 10.72451020669871369, 18.67979575497193778, 102.0844237280190185 ) ) ;
#93906=CARTESIAN_POINT ( 'NONE',  ( 21.53943276465977519, -0.05219959533907433946, 88.74890960531436690 ) ) ;
#93907=CARTESIAN_POINT ( 'NONE',  ( -5.153800228976328057, -19.02544592524343514, 67.29057627198102409 ) ) ;
#93908=CARTESIAN_POINT ( 'NONE',  ( 10.81492255796106328, -18.62759615963255655, 65.41775706135234714 ) ) ;
#93909=CARTESIAN_POINT ( 'NONE',  ( 5.153800228976335163, 19.02544592524342804, 44.79057627198103830 ) ) ;
#93911=CARTESIAN_POINT ( 'NONE',  ( -13.89961937509977652, 13.97604488694528158, 70.62390960531432427 ) ) ;
#93912=CARTESIAN_POINT ( 'NONE',  ( -9.564922557960796823, -16.46253265017161027, 27.08224293864769550 ) ) ;
#93913=CARTESIAN_POINT ( 'NONE',  ( -19.03943276465977164, 0.05219959533909376836, 111.2489096053143669 ) ) ;
#93914=CARTESIAN_POINT ( 'NONE',  ( -0.05219959533910754901, -16.53943276465976808, 62.49890960531436690 ) ) ;
#93915=CARTESIAN_POINT ( 'NONE',  ( -5.049401038298153566, 19.05341960407611168, 30.20724293864768839 ) ) ;
#93916=CARTESIAN_POINT ( 'NONE',  ( -16.52544592524342804, 4.483927247898546575, 91.04057627198103830 ) ) ;
#93917=CARTESIAN_POINT ( 'NONE',  ( 5.823673210054125526, 21.52544592524343514, 89.79057627198103830 ) ) ;
#93918=CARTESIAN_POINT ( 'NONE',  ( -10.81492255796105439, 18.62759615963255655, 32.91775706135234714 ) ) ;
#93920=CARTESIAN_POINT ( 'NONE',  ( -0.05219959533934338120, 16.53943276465976808, 47.50109039468568994 ) ) ;
#93921=CARTESIAN_POINT ( 'NONE',  ( 10.72451020669898902, -18.67979575497178502, 77.91557627198102409 ) ) ;
#93922=CARTESIAN_POINT ( 'NONE',  ( -19.03943276465977164, -0.05219959533935918106, 28.75109039468566507 ) ) ;
#93923=CARTESIAN_POINT ( 'NONE',  ( -16.51473224551069308, -9.474510206698971260, 106.6655762719810383 ) ) ;
#93924=CARTESIAN_POINT ( 'NONE',  ( -21.52544592524334988, -5.823673210054445271, 38.95942372801901854 ) ) ;
#93925=CARTESIAN_POINT ( 'NONE',  ( 18.62759615963271287, -10.81492255796078972, 43.33224293864769550 ) ) ;
#93926=CARTESIAN_POINT ( 'NONE',  ( -16.55341960407611168, -4.379528057220339221, 21.45724293864769550 ) ) ;
#93927=CARTESIAN_POINT ( 'NONE',  ( -18.67979575497193778, 10.72451020669871902, 68.33442372801900433 ) ) ;
#93928=CARTESIAN_POINT ( 'NONE',  ( -18.62759615963255300, -10.81492255796106328, 104.1677570613523471 ) ) ;
#93929=CARTESIAN_POINT ( 'NONE',  ( 16.51473224551083163, -9.474510206698727899, 35.83442372801899722 ) ) ;
#93930=CARTESIAN_POINT ( 'NONE',  ( -0.05219959533934338120, 16.53943276465976808, 87.50109039468568994 ) ) ;
#93931=CARTESIAN_POINT ( 'NONE',  ( 5.823673210054444382, -21.52544592524334988, 45.20942372801901854 ) ) ;
#93932=CARTESIAN_POINT ( 'NONE',  ( -9.564922557960796823, -16.46253265017161027, 52.08224293864768839 ) ) ;
#93933=CARTESIAN_POINT ( 'NONE',  ( 21.53943276465977519, 0.05219959533937863772, 111.2510903946856899 ) ) ;
#93934=CARTESIAN_POINT ( 'NONE',  ( 10.81492255796078972, 18.62759615963270932, 24.58224293864768839 ) ) ;
#93935=CARTESIAN_POINT ( 'NONE',  ( 21.55341960407619695, -5.719274019375665929, 21.04275706135234714 ) ) ;
#93936=CARTESIAN_POINT ( 'NONE',  ( 0.05219959533907565091, 21.53943276465977519, 74.99890960531435269 ) ) ;
#93937=CARTESIAN_POINT ( 'NONE',  ( -4.379528057220086978, -16.55341960407618274, 39.79275706135235424 ) ) ;
#93939=CARTESIAN_POINT ( 'NONE',  ( 5.823673210054125526, 21.52544592524343514, 84.79057627198102409 ) ) ;
#93940=CARTESIAN_POINT ( 'NONE',  ( 12.06949235617739724, 12.14591786802326823, 61.87609039468568284 ) ) ;
#93941=CARTESIAN_POINT ( 'NONE',  ( 14.29746914071049879, -8.314922557960816363, 63.33224293864770260 ) ) ;
#93943=CARTESIAN_POINT ( 'NONE',  ( 16.46253265017146816, 9.564922557961045513, 86.66775706135233293 ) ) ;
#93945=CARTESIAN_POINT ( 'NONE',  ( -12.06949235617739369, -12.14591786802326823, 34.37609039468568284 ) ) ;
#93946=CARTESIAN_POINT ( 'NONE',  ( -21.53943276465977519, 0.05219959533907696930, 116.2489096053143669 ) ) ;
#93948=CARTESIAN_POINT ( 'NONE',  ( -0.05219959533907301413, -21.53943276465977519, 72.49890960531435269 ) ) ;
#93949=CARTESIAN_POINT ( 'NONE',  ( -5.823673210054116645, -21.52544592524344225, 32.29057627198102409 ) ) ;
#93950=CARTESIAN_POINT ( 'NONE',  ( -4.379528057220086978, -16.55341960407618274, 59.79275706135234714 ) ) ;
#93951=CARTESIAN_POINT ( 'NONE',  ( 19.02544592524343514, -5.153800228976328945, 68.54057627198103830 ) ) ;
#93952=CARTESIAN_POINT ( 'NONE',  ( -18.62759615963255300, -10.81492255796106328, 49.16775706135234003 ) ) ;
#93953=CARTESIAN_POINT ( 'NONE',  ( 16.52544592524335698, 4.483927247898782831, 21.45942372801901499 ) ) ;
#93954=CARTESIAN_POINT ( 'NONE',  ( 19.05341960407611168, 5.049401038298154454, 108.9572429386477097 ) ) ;
#93955=CARTESIAN_POINT ( 'NONE',  ( 19.02544592524334988, 5.153800228976608722, 21.45942372801899012 ) ) ;
#93956=CARTESIAN_POINT ( 'NONE',  ( -16.55341960407617563, 4.379528057220093196, 43.54275706135235424 ) ) ;
#93957=CARTESIAN_POINT ( 'NONE',  ( -13.89961937509977652, 13.97604488694528158, 100.6239096053143669 ) ) ;
#93958=CARTESIAN_POINT ( 'NONE',  ( -15.72974639402197994, 15.80617190586746368, 100.6239096053143811 ) ) ;
#93959=CARTESIAN_POINT ( 'NONE',  ( 5.153800228976335163, 19.02544592524342804, 74.79057627198103830 ) ) ;
#93960=CARTESIAN_POINT ( 'NONE',  ( 16.53943276465976808, -0.05219959533910856209, 83.74890960531435269 ) ) ;
#93961=CARTESIAN_POINT ( 'NONE',  ( -5.719274019375978568, 21.55341960407610458, 25.20724293864769550 ) ) ;
#93962=CARTESIAN_POINT ( 'NONE',  ( 9.474510206698971260, -16.51473224551069308, 22.91557627198102765 ) ) ;
#93963=CARTESIAN_POINT ( 'NONE',  ( 5.823673210054125526, 21.52544592524343514, 99.79057627198103830 ) ) ;
#93964=CARTESIAN_POINT ( 'NONE',  ( -19.05341960407617563, 5.049401038297882671, 63.54275706135234003 ) ) ;
#93965=CARTESIAN_POINT ( 'NONE',  ( 21.55341960407610458, 5.719274019375980345, 28.95724293864769905 ) ) ;
#93966=CARTESIAN_POINT ( 'NONE',  ( -13.89961937509977652, 13.97604488694528158, 30.62390960531435269 ) ) ;
#93967=CARTESIAN_POINT ( 'NONE',  ( -5.719274019375978568, 21.55341960407610458, 65.20724293864768129 ) ) ;
#93968=CARTESIAN_POINT ( 'NONE',  ( 19.02544592524343514, -5.153800228976328945, 103.5405762719809957 ) ) ;
#93969=CARTESIAN_POINT ( 'NONE',  ( -5.823673210054431948, 21.52544592524334988, 87.70942372801901854 ) ) ;
#93970=CARTESIAN_POINT ( 'NONE',  ( -13.97604488694527625, -13.89961937509977652, 51.87390960531436690 ) ) ;
#93971=CARTESIAN_POINT ( 'NONE',  ( 14.34966873604960469, 8.224510206698951720, 89.16557627198102409 ) ) ;
#93972=CARTESIAN_POINT ( 'NONE',  ( 14.34966873604972726, -8.224510206698740333, 30.83442372801902209 ) ) ;
#93973=CARTESIAN_POINT ( 'NONE',  ( -19.02544592524342804, 5.153800228976336051, 56.04057627198100988 ) ) ;
#93974=CARTESIAN_POINT ( 'NONE',  ( 15.80617190586769283, -15.72974639402175789, 85.62609039468568994 ) ) ;
#93975=ORIENTED_EDGE ( 'NONE', *, *, #42127, .T. ) ;
#93976=CARTESIAN_POINT ( 'NONE',  ( 5.049401038297881783, 19.05341960407617563, 27.29275706135232937 ) ) ;
#93977=CARTESIAN_POINT ( 'NONE',  ( 13.97604488694548053, -13.89961937509957401, 35.62609039468567573 ) ) ;
#93978=CARTESIAN_POINT ( 'NONE',  ( 5.823673210054444382, -21.52544592524334988, 35.20942372801901854 ) ) ;
#93980=CARTESIAN_POINT ( 'NONE',  ( -16.51473224551082808, 9.474510206698731452, 28.33442372801900433 ) ) ;
#93981=CARTESIAN_POINT ( 'NONE',  ( -19.02544592524342804, 5.153800228976336051, 81.04057627198103830 ) ) ;
#93982=CARTESIAN_POINT ( 'NONE',  ( 0.05219959533909260263, 19.03943276465977164, 74.99890960531435269 ) ) ;
#93983=CARTESIAN_POINT ( 'NONE',  ( 16.55341960407611168, 4.379528057220329451, 23.95724293864769550 ) ) ;
#93984=CARTESIAN_POINT ( 'NONE',  ( 19.05341960407611168, 5.049401038298154454, 113.9572429386477097 ) ) ;
#93985=CARTESIAN_POINT ( 'NONE',  ( -21.55341960407619339, 5.719274019375674811, 83.54275706135234714 ) ) ;
#93988=CARTESIAN_POINT ( 'NONE',  ( -21.53943276465977519, -0.05219959533937600094, 78.75109039468568994 ) ) ;
#93990=CARTESIAN_POINT ( 'NONE',  ( -19.03943276465977164, 0.05219959533909376836, 96.24890960531436690 ) ) ;
#93992=CARTESIAN_POINT ( 'NONE',  ( -21.52544592524343514, 5.823673210054127303, 71.04057627198103830 ) ) ;
#93993=CARTESIAN_POINT ( 'NONE',  ( -12.14591786802309592, -12.06949235617757132, 26.87390960531435979 ) ) ;
#93994=CARTESIAN_POINT ( 'NONE',  ( -12.14591786802309592, -12.06949235617757132, 111.8739096053143669 ) ) ;
#93995=CARTESIAN_POINT ( 'NONE',  ( -16.46253265017160317, 9.564922557960807481, 100.8322429386477097 ) ) ;
#93996=CARTESIAN_POINT ( 'NONE',  ( 9.474510206698729675, 16.51473224551082808, 27.08442372801900433 ) ) ;
#93997=CARTESIAN_POINT ( 'NONE',  ( 5.153800228976335163, 19.02544592524342804, 24.79057627198102765 ) ) ;
#93998=CARTESIAN_POINT ( 'NONE',  ( -21.52544592524334988, -5.823673210054445271, 63.95942372801901854 ) ) ;
#93999=CARTESIAN_POINT ( 'NONE',  ( 9.564922557960805705, 16.46253265017160317, 109.5822429386476955 ) ) ;
#94000=CARTESIAN_POINT ( 'NONE',  ( 16.53943276465976808, 0.05219959533934440121, 106.2510903946856757 ) ) ;
#94001=CARTESIAN_POINT ( 'NONE',  ( 9.474510206698729675, 16.51473224551082808, 67.08442372801900433 ) ) ;
#94002=CARTESIAN_POINT ( 'NONE',  ( 16.46253265017146816, 9.564922557961045513, 66.66775706135233293 ) ) ;
#94003=CARTESIAN_POINT ( 'NONE',  ( 19.03943276465977164, -0.05219959533909143690, 108.7489096053143527 ) ) ;
#94004=CARTESIAN_POINT ( 'NONE',  ( 4.483927247898545687, 16.52544592524342804, 89.79057627198103830 ) ) ;
#94005=CARTESIAN_POINT ( 'NONE',  ( -5.049401038297874678, -19.05341960407617918, 54.79275706135234003 ) ) ;
#94006=CARTESIAN_POINT ( 'NONE',  ( -9.564922557960796823, -16.46253265017161027, 77.08224293864769550 ) ) ;
#94007=CARTESIAN_POINT ( 'NONE',  ( -12.06949235617756955, 12.14591786802309770, 65.62390960531436690 ) ) ;
#94008=CARTESIAN_POINT ( 'NONE',  ( -13.89961937509957401, -13.97604488694547875, 89.37609039468563310 ) ) ;
#94009=CARTESIAN_POINT ( 'NONE',  ( -18.62759615963270932, 10.81492255796079327, 55.83224293864770260 ) ) ;
#94011=CARTESIAN_POINT ( 'NONE',  ( 0.05219959533910956823, 16.53943276465976808, 109.9989096053143527 ) ) ;
#94013=CARTESIAN_POINT ( 'NONE',  ( -16.51473224551069308, -9.474510206698971260, 66.66557627198102409 ) ) ;
#94014=CARTESIAN_POINT ( 'NONE',  ( -21.55341960407610458, -5.719274019375992779, 81.45724293864769550 ) ) ;
#94015=CARTESIAN_POINT ( 'NONE',  ( 16.53943276465976808, 0.05219959533934440121, 86.25109039468568994 ) ) ;
#94016=CARTESIAN_POINT ( 'NONE',  ( 19.05341960407611168, 5.049401038298154454, 78.95724293864769550 ) ) ;
#94017=CARTESIAN_POINT ( 'NONE',  ( 13.89961937509957401, 13.97604488694547697, 66.87609039468567573 ) ) ;
#94018=CARTESIAN_POINT ( 'NONE',  ( 18.67979575497194134, -10.72451020669871369, 85.83442372801901854 ) ) ;
#94019=CARTESIAN_POINT ( 'NONE',  ( -18.67979575497178146, -10.72451020669898902, 61.66557627198103120 ) ) ;
#94020=CARTESIAN_POINT ( 'NONE',  ( 15.72974639402199770, -15.80617190586745480, 28.12390960531435979 ) ) ;
#94021=CARTESIAN_POINT ( 'NONE',  ( -19.03943276465977164, 0.05219959533909376836, 36.24890960531436690 ) ) ;
#94022=CARTESIAN_POINT ( 'NONE',  ( 14.34966873604972726, -8.224510206698740333, 100.8344237280190185 ) ) ;
#94023=CARTESIAN_POINT ( 'NONE',  ( -16.52544592524335698, -4.483927247898792601, 28.95942372801902209 ) ) ;
#94024=CARTESIAN_POINT ( 'NONE',  ( 19.49190055781010500, 5.500000000000053291, 78.06116087098780554 ) ) ;
#94025=CARTESIAN_POINT ( 'NONE',  ( 21.52544592524334988, 5.823673210054432836, 101.4594237280190185 ) ) ;
#94026=ORIENTED_EDGE ( 'NONE', *, *, #187948, .T. ) ;
#94027=CARTESIAN_POINT ( 'NONE',  ( 8.314922557960818139, 14.29746914071049879, 54.58224293864769550 ) ) ;
#94028=CARTESIAN_POINT ( 'NONE',  ( -0.05219959533907301413, -21.53943276465977519, 92.49890960531436690 ) ) ;
#94029=CARTESIAN_POINT ( 'NONE',  ( 10.81492255796078972, 18.62759615963270932, 104.5822429386477097 ) ) ;
#94031=CARTESIAN_POINT ( 'NONE',  ( -21.53943276465977519, 0.05219959533907696930, 41.24890960531435269 ) ) ;
#94033=CARTESIAN_POINT ( 'NONE',  ( 12.06949235617739724, 12.14591786802326823, 76.87609039468567573 ) ) ;
#94034=CARTESIAN_POINT ( 'NONE',  ( 0.05219959533910956823, 16.53943276465976808, 84.99890960531436690 ) ) ;
#94035=CARTESIAN_POINT ( 'NONE',  ( -0.05219959533909027116, -19.03943276465977164, 42.49890960531435269 ) ) ;
#94036=PRESENTATION_STYLE_ASSIGNMENT (( #16221 ) ) ;
#94038=CARTESIAN_POINT ( 'NONE',  ( -4.379528057220086978, -16.55341960407618274, 89.79275706135236135 ) ) ;
#94039=CARTESIAN_POINT ( 'NONE',  ( -10.72451020669870658, -18.67979575497194134, 39.58442372801901143 ) ) ;
#94040=CARTESIAN_POINT ( 'NONE',  ( 0.05219959533909260263, 19.03943276465977164, 89.99890960531436690 ) ) ;
#94041=CARTESIAN_POINT ( 'NONE',  ( 0.05219959533937995610, -21.53943276465977519, 65.00109039468568994 ) ) ;
#94043=CARTESIAN_POINT ( 'NONE',  ( -5.049401038298153566, 19.05341960407611168, 25.20724293864768484 ) ) ;
#94044=ORIENTED_EDGE ( 'NONE', *, *, #41146, .F. ) ;
#94045=CARTESIAN_POINT ( 'NONE',  ( -0.05219959533937732626, 21.53943276465977519, 62.50109039468568284 ) ) ;
#94046=CARTESIAN_POINT ( 'NONE',  ( -19.03943276465977164, 0.05219959533909376836, 56.24890960531435979 ) ) ;
#94047=CARTESIAN_POINT ( 'NONE',  ( 19.03943276465977164, -0.05219959533909143690, 23.74890960531435269 ) ) ;
#94048=CARTESIAN_POINT ( 'NONE',  ( 13.89961937509977652, -13.97604488694527269, 88.12390960531438111 ) ) ;
#94049=CARTESIAN_POINT ( 'NONE',  ( -0.05219959533936034679, 19.03943276465977164, 62.50109039468566863 ) ) ;
#94050=CARTESIAN_POINT ( 'NONE',  ( -0.05219959533937732626, 21.53943276465977519, 42.50109039468567573 ) ) ;
#94051=CARTESIAN_POINT ( 'NONE',  ( 13.89961937509957401, 13.97604488694547697, 61.87609039468566863 ) ) ;
#94052=CARTESIAN_POINT ( 'NONE',  ( 5.153800228976335163, 19.02544592524342804, 44.79057627198103830 ) ) ;
#94053=CARTESIAN_POINT ( 'NONE',  ( 16.52544592524335698, 4.483927247898782831, 111.4594237280190328 ) ) ;
#94054=CARTESIAN_POINT ( 'NONE',  ( 19.03943276465977164, 0.05219959533936151252, 76.25109039468566152 ) ) ;
#94055=CARTESIAN_POINT ( 'NONE',  ( -4.483927247898539470, -16.52544592524342804, 22.29057627198102765 ) ) ;
#94056=CARTESIAN_POINT ( 'NONE',  ( 0.05219959533936267826, -19.03943276465977164, 55.00109039468566863 ) ) ;
#94057=CARTESIAN_POINT ( 'NONE',  ( -5.153800228976328057, -19.02544592524343514, 97.29057627198099567 ) ) ;
#94058=CARTESIAN_POINT ( 'NONE',  ( 18.67979575497194134, -10.72451020669871369, 110.8344237280190043 ) ) ;
#94059=CARTESIAN_POINT ( 'NONE',  ( 13.97604488694548053, -13.89961937509957401, 25.62609039468566507 ) ) ;
#94060=CARTESIAN_POINT ( 'NONE',  ( -5.049401038298153566, 19.05341960407611168, 35.20724293864768839 ) ) ;
#94061=CARTESIAN_POINT ( 'NONE',  ( 18.67979575497194134, -10.72451020669871369, 90.83442372801901854 ) ) ;
#94062=CARTESIAN_POINT ( 'NONE',  ( 8.224510206698742110, 14.34966873604972548, 37.08442372801901143 ) ) ;
#94063=CARTESIAN_POINT ( 'NONE',  ( -13.97604488694527625, -13.89961937509977652, 91.87390960531432427 ) ) ;
#94065=CARTESIAN_POINT ( 'NONE',  ( -16.46253265017160317, 9.564922557960807481, 75.83224293864769550 ) ) ;
#94066=CARTESIAN_POINT ( 'NONE',  ( 0.05219959533936267826, -19.03943276465977164, 90.00109039468567573 ) ) ;
#94068=CARTESIAN_POINT ( 'NONE',  ( 19.05341960407611168, 5.049401038298154454, 103.9572429386476671 ) ) ;
#94069=CARTESIAN_POINT ( 'NONE',  ( 18.62759615963255655, 10.81492255796105972, 101.6677570613523613 ) ) ;
#94070=CARTESIAN_POINT ( 'NONE',  ( -12.06949235617756955, 12.14591786802309770, 100.6239096053143811 ) ) ;
#94071=CARTESIAN_POINT ( 'NONE',  ( 19.03943276465977164, -0.05219959533909143690, 23.74890960531435269 ) ) ;
#94072=CARTESIAN_POINT ( 'NONE',  ( -0.05219959533907301413, -21.53943276465977519, 42.49890960531435979 ) ) ;
#94073=CARTESIAN_POINT ( 'NONE',  ( -5.823673210054116645, -21.52544592524344225, 37.29057627198102409 ) ) ;
#94074=CARTESIAN_POINT ( 'NONE',  ( 9.474510206698971260, -16.51473224551069308, 27.91557627198103120 ) ) ;
#94076=CARTESIAN_POINT ( 'NONE',  ( -19.02544592524334988, -5.153800228976617603, 63.95942372801899012 ) ) ;
#94077=CARTESIAN_POINT ( 'NONE',  ( 8.314922557960818139, 14.29746914071049879, 44.58224293864769550 ) ) ;
#94078=CARTESIAN_POINT ( 'NONE',  ( 13.89961937509977652, -13.97604488694527269, 113.1239096053143527 ) ) ;
#94079=CARTESIAN_POINT ( 'NONE',  ( -15.72974639402176322, -15.80617190586768395, 84.37609039468570415 ) ) ;
#94080=CARTESIAN_POINT ( 'NONE',  ( -18.67979575497178146, -10.72451020669898902, 71.66557627198100988 ) ) ;
#94081=CARTESIAN_POINT ( 'NONE',  ( -15.72974639402176322, -15.80617190586768395, 49.37609039468569705 ) ) ;
#94082=CARTESIAN_POINT ( 'NONE',  ( -21.53943276465977519, 0.05219959533907696930, 96.24890960531435269 ) ) ;
#94083=CARTESIAN_POINT ( 'NONE',  ( 21.53943276465977519, 0.05219959533937863772, 51.25109039468568994 ) ) ;
#94084=CARTESIAN_POINT ( 'NONE',  ( 0.05219959533909260263, 19.03943276465977164, 29.99890960531435979 ) ) ;
#94085=CARTESIAN_POINT ( 'NONE',  ( -13.89961937509977652, 13.97604488694528158, 85.62390960531433848 ) ) ;
#94086=CARTESIAN_POINT ( 'NONE',  ( 12.14591786802327356, -12.06949235617739191, 75.62609039468567573 ) ) ;
#94087=CARTESIAN_POINT ( 'NONE',  ( -12.06949235617756955, 12.14591786802309770, 110.6239096053143669 ) ) ;
#94088=CARTESIAN_POINT ( 'NONE',  ( -19.02544592524342804, 5.153800228976336051, 116.0405762719810383 ) ) ;
#94089=CARTESIAN_POINT ( 'NONE',  ( -14.34966873604960291, -8.224510206698953496, 51.66557627198102409 ) ) ;
#94090=CARTESIAN_POINT ( 'NONE',  ( 12.14591786802309770, 12.06949235617756955, 24.37390960531435979 ) ) ;
#94091=CARTESIAN_POINT ( 'NONE',  ( -19.03943276465977164, 0.05219959533909376836, 71.24890960531435269 ) ) ;
#94092=CARTESIAN_POINT ( 'NONE',  ( 9.564922557960805705, 16.46253265017160317, 29.58224293864769550 ) ) ;
#94093=CARTESIAN_POINT ( 'NONE',  ( -18.67979575497178146, -10.72451020669898902, 46.66557627198102409 ) ) ;
#94094=CARTESIAN_POINT ( 'NONE',  ( -5.153800228976607833, 19.02544592524334988, 37.70942372801899722 ) ) ;
#94096=CARTESIAN_POINT ( 'NONE',  ( -12.14591786802309592, -12.06949235617757132, 36.87390960531435979 ) ) ;
#94097=CARTESIAN_POINT ( 'NONE',  ( 19.05341960407611168, 5.049401038298154454, 108.9572429386477097 ) ) ;
#94098=CARTESIAN_POINT ( 'NONE',  ( 0.05219959533937995610, -21.53943276465977519, 60.00109039468568284 ) ) ;
#94100=CARTESIAN_POINT ( 'NONE',  ( 16.53943276465976808, 0.05219959533934440121, 71.25109039468568994 ) ) ;
#94102=CARTESIAN_POINT ( 'NONE',  ( 5.049401038297881783, 19.05341960407617563, 62.29275706135234003 ) ) ;
#94103=CARTESIAN_POINT ( 'NONE',  ( -8.314922557960811034, -14.29746914071050412, 47.08224293864770260 ) ) ;
#94104=CARTESIAN_POINT ( 'NONE',  ( -18.56399227203343116, -5.499999999999928058, 73.97830131249904184 ) ) ;
#94105=CARTESIAN_POINT ( 'NONE',  ( 16.53943276465976808, -0.05219959533910856209, 28.74890960531435624 ) ) ;
#94106=CARTESIAN_POINT ( 'NONE',  ( -16.51473224551069308, -9.474510206698971260, 36.66557627198102409 ) ) ;
#94107=CARTESIAN_POINT ( 'NONE',  ( 9.474510206698971260, -16.51473224551069308, 57.91557627198103120 ) ) ;
#94108=CARTESIAN_POINT ( 'NONE',  ( 4.483927247898545687, 16.52544592524342804, 114.7905762719810383 ) ) ;
#94109=CARTESIAN_POINT ( 'NONE',  ( -21.52544592524334988, -5.823673210054445271, 33.95942372801901143 ) ) ;
#94110=CARTESIAN_POINT ( 'NONE',  ( 9.564922557960805705, 16.46253265017160317, 54.58224293864769550 ) ) ;
#94112=CARTESIAN_POINT ( 'NONE',  ( -9.474510206698964154, 16.51473224551069663, 50.41557627198102409 ) ) ;
#94113=CARTESIAN_POINT ( 'NONE',  ( -5.823673210054116645, -21.52544592524344225, 32.29057627198102409 ) ) ;
#94114=CARTESIAN_POINT ( 'NONE',  ( -10.72451020669870658, -18.67979575497194134, 54.58442372801901143 ) ) ;
#94115=CARTESIAN_POINT ( 'NONE',  ( -9.474510206698964154, 16.51473224551069663, 25.41557627198103120 ) ) ;
#94116=CARTESIAN_POINT ( 'NONE',  ( 10.72451020669898902, -18.67979575497178502, 32.91557627198102409 ) ) ;
#94117=CARTESIAN_POINT ( 'NONE',  ( 8.224510206698742110, 14.34966873604972548, 92.08442372801901854 ) ) ;
#94118=CARTESIAN_POINT ( 'NONE',  ( 21.53943276465977519, 0.05219959533937863772, 106.2510903946856757 ) ) ;
#94119=CARTESIAN_POINT ( 'NONE',  ( -16.55341960407617563, 4.379528057220093196, 73.54275706135234714 ) ) ;
#94120=CARTESIAN_POINT ( 'NONE',  ( 16.46253265017160672, -9.564922557960803928, 108.3322429386476955 ) ) ;
#94121=CARTESIAN_POINT ( 'NONE',  ( -16.55341960407617563, 4.379528057220093196, 53.54275706135234714 ) ) ;
#94122=CARTESIAN_POINT ( 'NONE',  ( -8.224510206698735004, -14.34966873604973081, 29.58442372801901854 ) ) ;
#94123=CARTESIAN_POINT ( 'NONE',  ( 4.379528057220092307, 16.55341960407617563, 102.2927570613523613 ) ) ;
#94124=CARTESIAN_POINT ( 'NONE',  ( -5.823673210054431948, 21.52544592524334988, 52.70942372801902565 ) ) ;
#94125=CARTESIAN_POINT ( 'NONE',  ( 19.02544592524334988, 5.153800228976608722, 106.4594237280190185 ) ) ;
#94126=CARTESIAN_POINT ( 'NONE',  ( -15.72974639402197994, 15.80617190586746368, 110.6239096053143669 ) ) ;
#94127=CARTESIAN_POINT ( 'NONE',  ( 8.314922557961029526, -14.29746914071037800, 25.41775706135235779 ) ) ;
#94128=CARTESIAN_POINT ( 'NONE',  ( 4.483927247898790824, -16.52544592524335698, 80.20942372801901854 ) ) ;
#94130=CARTESIAN_POINT ( 'NONE',  ( -5.823673210054431948, 21.52544592524334988, 87.70942372801901854 ) ) ;
#94131=CARTESIAN_POINT ( 'NONE',  ( 13.97604488694548053, -13.89961937509957401, 80.62609039468567573 ) ) ;
#94132=CARTESIAN_POINT ( 'NONE',  ( -16.53943276465976808, 0.05219959533911058130, 46.24890960531435979 ) ) ;
#94133=CARTESIAN_POINT ( 'NONE',  ( 8.224510206698953496, -14.34966873604960469, 37.91557627198102409 ) ) ;
#94134=CARTESIAN_POINT ( 'NONE',  ( -4.379528057220328563, 16.55341960407611168, 105.2072429386477097 ) ) ;
#94135=CARTESIAN_POINT ( 'NONE',  ( -19.02544592524334988, -5.153800228976617603, 43.95942372801899012 ) ) ;
#94136=CARTESIAN_POINT ( 'NONE',  ( 18.22780087662123805, -5.499999999999989342, 53.51763182126895657 ) ) ;
#94137=CARTESIAN_POINT ( 'NONE',  ( 15.80617190586769283, -15.72974639402175789, 40.62609039468567573 ) ) ;
#94138=CARTESIAN_POINT ( 'NONE',  ( -5.153800228976607833, 19.02544592524334988, 112.7094237280190043 ) ) ;
#94140=CARTESIAN_POINT ( 'NONE',  ( 19.03943276465977164, -0.05219959533909143690, 98.74890960531436690 ) ) ;
#94141=CARTESIAN_POINT ( 'NONE',  ( 21.53943276465977519, -0.05219959533907433946, 53.74890960531437401 ) ) ;
#94142=CARTESIAN_POINT ( 'NONE',  ( 9.564922557961047289, -16.46253265017146816, 100.4177570613523329 ) ) ;
#94143=CARTESIAN_POINT ( 'NONE',  ( -0.05219959533909027116, -19.03943276465977164, 87.49890960531436690 ) ) ;
#94144=CARTESIAN_POINT ( 'NONE',  ( 18.67979575497178502, 10.72451020669898547, 54.16557627198103120 ) ) ;
#94145=CARTESIAN_POINT ( 'NONE',  ( 12.06949235617757843, -12.14591786802309237, 103.1239096053143811 ) ) ;
#94146=CARTESIAN_POINT ( 'NONE',  ( 19.03943276465977164, -0.05219959533909143690, 63.74890960531435979 ) ) ;
#94147=CARTESIAN_POINT ( 'NONE',  ( -16.46253265017160317, 9.564922557960807481, 35.83224293864768839 ) ) ;
#94148=CARTESIAN_POINT ( 'NONE',  ( -15.80617190586768217, 15.72974639402176855, 33.12609039468569705 ) ) ;
#94149=CARTESIAN_POINT ( 'NONE',  ( -10.72451020669870658, -18.67979575497194134, 79.58442372801903275 ) ) ;
#94150=CARTESIAN_POINT ( 'NONE',  ( -12.06949235617739369, -12.14591786802326823, 94.37609039468568994 ) ) ;
#94151=CARTESIAN_POINT ( 'NONE',  ( -10.72451020669870658, -18.67979575497194134, 24.58442372801901499 ) ) ;
#94152=CARTESIAN_POINT ( 'NONE',  ( -18.62759615963255300, -10.81492255796106328, 24.16775706135235424 ) ) ;
#94153=CARTESIAN_POINT ( 'NONE',  ( 19.03943276465977164, 0.05219959533936151252, 61.25109039468566863 ) ) ;
#94154=CARTESIAN_POINT ( 'NONE',  ( 19.02544592524343514, -5.153800228976328945, 83.54057627198100988 ) ) ;
#94155=CARTESIAN_POINT ( 'NONE',  ( -15.80617190586768217, 15.72974639402176855, 88.12609039468570415 ) ) ;
#94156=CARTESIAN_POINT ( 'NONE',  ( 5.823673210054125526, 21.52544592524343514, 79.79057627198102409 ) ) ;
#94157=CARTESIAN_POINT ( 'NONE',  ( -14.34966873604960291, -8.224510206698953496, 61.66557627198103120 ) ) ;
#94158=CARTESIAN_POINT ( 'NONE',  ( -5.719274019375665041, -21.55341960407619695, 99.79275706135234714 ) ) ;
#94159=CARTESIAN_POINT ( 'NONE',  ( 16.55341960407611168, 4.379528057220329451, 88.95724293864769550 ) ) ;
#94160=CARTESIAN_POINT ( 'NONE',  ( -19.02544592524342804, 5.153800228976336051, 31.04057627198102409 ) ) ;
#94161=CARTESIAN_POINT ( 'NONE',  ( -5.153800228976607833, 19.02544592524334988, 72.70942372801900433 ) ) ;
#94162=CARTESIAN_POINT ( 'NONE',  ( -14.34966873604960291, -8.224510206698953496, 41.66557627198103120 ) ) ;
#94163=CARTESIAN_POINT ( 'NONE',  ( -5.823673210054431948, 21.52544592524334988, 97.70942372801904696 ) ) ;
#94164=CARTESIAN_POINT ( 'NONE',  ( 19.05341960407611168, 5.049401038298154454, 93.95724293864769550 ) ) ;
#94165=CARTESIAN_POINT ( 'NONE',  ( -19.03943276465977164, -0.05219959533935918106, 58.75109039468566863 ) ) ;
#94166=CARTESIAN_POINT ( 'NONE',  ( -21.53943276465977519, 0.05219959533907696930, 66.24890960531436690 ) ) ;
#94167=CARTESIAN_POINT ( 'NONE',  ( -21.52544592524334988, -5.823673210054445271, 23.95942372801901143 ) ) ;
#94168=CARTESIAN_POINT ( 'NONE',  ( 0.05219959533936267826, -19.03943276465977164, 105.0010903946856615 ) ) ;
#94169=CARTESIAN_POINT ( 'NONE',  ( -8.224510206698735004, -14.34966873604973081, 79.58442372801903275 ) ) ;
#94171=CARTESIAN_POINT ( 'NONE',  ( 21.52544592524334988, 5.823673210054432836, 26.45942372801901854 ) ) ;
#94172=CARTESIAN_POINT ( 'NONE',  ( 8.224510206698953496, -14.34966873604960469, 97.91557627198103830 ) ) ;
#94174=CARTESIAN_POINT ( 'NONE',  ( -12.06949235617739369, -12.14591786802326823, 39.37609039468567573 ) ) ;
#94175=CARTESIAN_POINT ( 'NONE',  ( 10.81492255796078972, 18.62759615963270932, 59.58224293864770260 ) ) ;
#94176=CARTESIAN_POINT ( 'NONE',  ( 16.53943276465976808, 0.05219959533934440121, 101.2510903946856757 ) ) ;
#94177=CARTESIAN_POINT ( 'NONE',  ( 14.29746914071037800, 8.314922557961029526, 41.66775706135235424 ) ) ;
#94178=CARTESIAN_POINT ( 'NONE',  ( -0.05219959533909027116, -19.03943276465977164, 32.49890960531435979 ) ) ;
#94179=CARTESIAN_POINT ( 'NONE',  ( -4.379528057220086978, -16.55341960407618274, 84.79275706135234714 ) ) ;
#94180=CARTESIAN_POINT ( 'NONE',  ( -0.05219959533936034679, 19.03943276465977164, 72.50109039468566152 ) ) ;
#94181=CARTESIAN_POINT ( 'NONE',  ( -5.823673210054116645, -21.52544592524344225, 67.29057627198103830 ) ) ;
#94182=CARTESIAN_POINT ( 'NONE',  ( 0.05219959533934541429, -16.53943276465976808, 95.00109039468568994 ) ) ;
#94183=CARTESIAN_POINT ( 'NONE',  ( 10.81492255796106328, -18.62759615963255655, 85.41775706135236135 ) ) ;
#94184=CARTESIAN_POINT ( 'NONE',  ( -21.53943276465977519, 0.05219959533907696930, 66.24890960531436690 ) ) ;
#94185=CARTESIAN_POINT ( 'NONE',  ( -0.05219959533907301413, -21.53943276465977519, 47.49890960531435979 ) ) ;
#94187=CARTESIAN_POINT ( 'NONE',  ( -4.483927247898782831, 16.52544592524335698, 77.70942372801900433 ) ) ;
#94188=CARTESIAN_POINT ( 'NONE',  ( -15.80617190586745835, -15.72974639402198527, 46.87390960531435979 ) ) ;
#94190=CARTESIAN_POINT ( 'NONE',  ( -9.474510206698964154, 16.51473224551069663, 115.4155762719810241 ) ) ;
#94192=CARTESIAN_POINT ( 'NONE',  ( -8.224510206698948167, 14.34966873604960824, 115.4155762719810241 ) ) ;
#94193=CARTESIAN_POINT ( 'NONE',  ( -18.67979575497178146, -10.72451020669898902, 56.66557627198103830 ) ) ;
#94194=CARTESIAN_POINT ( 'NONE',  ( 16.53943276465976808, 0.05219959533934440121, 106.2510903946856757 ) ) ;
#94195=CARTESIAN_POINT ( 'NONE',  ( -18.67979575497193778, 10.72451020669871902, 48.33442372801902565 ) ) ;
#94196=CARTESIAN_POINT ( 'NONE',  ( -19.03943276465977164, -0.05219959533935918106, 98.75109039468567573 ) ) ;
#94197=CARTESIAN_POINT ( 'NONE',  ( -16.55341960407611168, -4.379528057220339221, 111.4572429386476813 ) ) ;
#94198=CARTESIAN_POINT ( 'NONE',  ( 16.46253265017146816, 9.564922557961045513, 106.6677570613523471 ) ) ;
#94199=CARTESIAN_POINT ( 'NONE',  ( -9.564922557960796823, -16.46253265017161027, 42.08224293864769550 ) ) ;
#94201=CARTESIAN_POINT ( 'NONE',  ( -19.02544592524342804, 5.153800228976336051, 91.04057627198100988 ) ) ;
#94202=CARTESIAN_POINT ( 'NONE',  ( -12.06949235617739369, -12.14591786802326823, 79.37609039468567573 ) ) ;
#94203=CARTESIAN_POINT ( 'NONE',  ( -5.153800228976607833, 19.02544592524334988, 72.70942372801900433 ) ) ;
#94204=CARTESIAN_POINT ( 'NONE',  ( 9.474510206698729675, 16.51473224551082808, 27.08442372801900433 ) ) ;
#94205=CARTESIAN_POINT ( 'NONE',  ( 5.719274019375991003, -21.55341960407610458, 57.70724293864770260 ) ) ;
#94206=EDGE_CURVE ( 'NONE', #61533, #22005, #152564, .T. ) ;
#94207=CARTESIAN_POINT ( 'NONE',  ( 16.55341960407618274, -4.379528057220086978, 81.04275706135236135 ) ) ;
#94208=CARTESIAN_POINT ( 'NONE',  ( 13.97604488694548053, -13.89961937509957401, 75.62609039468564731 ) ) ;
#94209=CARTESIAN_POINT ( 'NONE',  ( -13.97604488694527625, -13.89961937509977652, 41.87390960531435979 ) ) ;
#94210=CARTESIAN_POINT ( 'NONE',  ( 16.46253265017160672, -9.564922557960803928, 83.33224293864768129 ) ) ;
#94211=CARTESIAN_POINT ( 'NONE',  ( -15.72974639402176322, -15.80617190586768395, 49.37609039468569705 ) ) ;
#94212=CARTESIAN_POINT ( 'NONE',  ( -19.03943276465977164, 0.05219959533909376836, 46.24890960531435979 ) ) ;
#94213=CARTESIAN_POINT ( 'NONE',  ( 19.03943276465977164, 0.05219959533936151252, 76.25109039468566152 ) ) ;
#94215=CARTESIAN_POINT ( 'NONE',  ( -19.05341960407611168, -5.049401038298163336, 106.4572429386476955 ) ) ;
#94216=CARTESIAN_POINT ( 'NONE',  ( 14.34966873604960469, 8.224510206698951720, 59.16557627198103120 ) ) ;
#94217=CARTESIAN_POINT ( 'NONE',  ( -21.52544592524343514, 5.823673210054127303, 61.04057627198103120 ) ) ;
#94219=CARTESIAN_POINT ( 'NONE',  ( -9.474510206698720793, -16.51473224551083518, 49.58442372801899722 ) ) ;
#94220=CARTESIAN_POINT ( 'NONE',  ( -17.97182807773871716, 5.500000000000055955, 88.53038844047284783 ) ) ;
#94221=CARTESIAN_POINT ( 'NONE',  ( 16.46253265017160672, -9.564922557960803928, 68.33224293864770971 ) ) ;
#94222=CARTESIAN_POINT ( 'NONE',  ( -5.153800228976328057, -19.02544592524343514, 67.29057627198102409 ) ) ;
#94223=CARTESIAN_POINT ( 'NONE',  ( 4.483927247898790824, -16.52544592524335698, 55.20942372801902565 ) ) ;
#94226=CARTESIAN_POINT ( 'NONE',  ( 12.14591786802327356, -12.06949235617739191, 95.62609039468568994 ) ) ;
#94228=CARTESIAN_POINT ( 'NONE',  ( -0.05219959533934338120, 16.53943276465976808, 72.50109039468568994 ) ) ;
#94229=CARTESIAN_POINT ( 'NONE',  ( -0.05219959533934338120, 16.53943276465976808, 37.50109039468568284 ) ) ;
#94230=CARTESIAN_POINT ( 'NONE',  ( -13.97604488694547697, 13.89961937509957934, 23.12609039468565442 ) ) ;
#94231=CARTESIAN_POINT ( 'NONE',  ( -16.51473224551069308, -9.474510206698971260, 56.66557627198103120 ) ) ;
#94233=CARTESIAN_POINT ( 'NONE',  ( -5.823673210054431948, 21.52544592524334988, 47.70942372801902565 ) ) ;
#94234=CARTESIAN_POINT ( 'NONE',  ( -19.03943276465977164, -0.05219959533935918106, 68.75109039468566152 ) ) ;
#94235=CARTESIAN_POINT ( 'NONE',  ( -21.53943276465977519, -0.05219959533937600094, 103.7510903946857042 ) ) ;
#94236=CARTESIAN_POINT ( 'NONE',  ( 5.153800228976335163, 19.02544592524342804, 29.79057627198102409 ) ) ;
#94238=CARTESIAN_POINT ( 'NONE',  ( 0.05219959533907565091, 21.53943276465977519, 59.99890960531436690 ) ) ;
#94239=ADVANCED_FACE ( 'NONE', ( #78472 ), #103448, .T. ) ;
#94240=CARTESIAN_POINT ( 'NONE',  ( -18.67979575497178146, -10.72451020669898902, 21.66557627198102409 ) ) ;
#94241=CARTESIAN_POINT ( 'NONE',  ( -14.34966873604960291, -8.224510206698953496, 96.66557627198102409 ) ) ;
#94242=CARTESIAN_POINT ( 'NONE',  ( 8.314922557961029526, -14.29746914071037800, 40.41775706135234714 ) ) ;
#94243=CARTESIAN_POINT ( 'NONE',  ( 12.14591786802309770, 12.06949235617756955, 29.37390960531435269 ) ) ;
#94244=VERTEX_POINT ( 'NONE', #61837 ) ;
#94245=CARTESIAN_POINT ( 'NONE',  ( 21.55341960407610458, 5.719274019375980345, 113.9572429386477239 ) ) ;
#94246=CARTESIAN_POINT ( 'NONE',  ( 16.53943276465976808, -0.05219959533910856209, 33.74890960531436690 ) ) ;
#94247=CARTESIAN_POINT ( 'NONE',  ( 19.02544592524343514, -5.153800228976328945, 108.5405762719810383 ) ) ;
#94249=CARTESIAN_POINT ( 'NONE',  ( 9.474510206698729675, 16.51473224551082808, 102.0844237280190043 ) ) ;
#94250=CARTESIAN_POINT ( 'NONE',  ( 13.89961937509957401, 13.97604488694547697, 31.87609039468566863 ) ) ;
#94251=CARTESIAN_POINT ( 'NONE',  ( -16.53943276465976808, 0.05219959533911058130, 26.24890960531435624 ) ) ;
#94252=CARTESIAN_POINT ( 'NONE',  ( -15.80617190586745835, -15.72974639402198527, 106.8739096053143811 ) ) ;
#94253=CARTESIAN_POINT ( 'NONE',  ( -5.719274019375978568, 21.55341960407610458, 70.20724293864769550 ) ) ;
#94254=CARTESIAN_POINT ( 'NONE',  ( 5.049401038298161559, -19.05341960407611168, 82.70724293864770971 ) ) ;
#94255=CARTESIAN_POINT ( 'NONE',  ( 16.53943276465976808, -0.05219959533910856209, 53.74890960531437401 ) ) ;
#94256=CARTESIAN_POINT ( 'NONE',  ( -16.51473224551069308, -9.474510206698971260, 96.66557627198102409 ) ) ;
#94258=CARTESIAN_POINT ( 'NONE',  ( -0.05219959533936034679, 19.03943276465977164, 52.50109039468566863 ) ) ;
#94259=CARTESIAN_POINT ( 'NONE',  ( -21.53943276465977519, 0.05219959533907696930, 96.24890960531435269 ) ) ;
#94260=CARTESIAN_POINT ( 'NONE',  ( 16.53943276465976808, -0.05219959533910856209, 98.74890960531438111 ) ) ;
#94261=CARTESIAN_POINT ( 'NONE',  ( -18.62759615963255300, -10.81492255796106328, 34.16775706135234714 ) ) ;
#94263=EDGE_CURVE ( 'NONE', #141307, #53672, #184214, .T. ) ;
#94264=CARTESIAN_POINT ( 'NONE',  ( -8.314922557960811034, -14.29746914071050412, 27.08224293864769550 ) ) ;
#94265=CARTESIAN_POINT ( 'NONE',  ( -19.03943276465977164, 0.05219959533909376836, 31.24890960531435979 ) ) ;
#94266=CARTESIAN_POINT ( 'NONE',  ( 9.564922557960805705, 16.46253265017160317, 84.58224293864769550 ) ) ;
#94267=CARTESIAN_POINT ( 'NONE',  ( -10.72451020669898014, 18.67979575497178502, 60.41557627198102409 ) ) ;
#94269=CARTESIAN_POINT ( 'NONE',  ( 16.51473224551069308, 9.474510206698969483, 34.16557627198102409 ) ) ;
#94270=CARTESIAN_POINT ( 'NONE',  ( -15.72974639402197994, 15.80617190586746368, 55.62390960531436690 ) ) ;
#94271=CARTESIAN_POINT ( 'NONE',  ( 21.55341960407619695, -5.719274019375665929, 71.04275706135234714 ) ) ;
#94273=CARTESIAN_POINT ( 'NONE',  ( -12.06949235617739369, -12.14591786802326823, 74.37609039468568994 ) ) ;
#94274=CARTESIAN_POINT ( 'NONE',  ( 13.89961937509977652, -13.97604488694527269, 63.12390960531435979 ) ) ;
#94275=CARTESIAN_POINT ( 'NONE',  ( -16.46253265017160317, 9.564922557960807481, 65.83224293864769550 ) ) ;
#94277=CARTESIAN_POINT ( 'NONE',  ( -21.52544592524334988, -5.823673210054445271, 108.9594237280190185 ) ) ;
#94278=CARTESIAN_POINT ( 'NONE',  ( 12.14591786802327356, -12.06949235617739191, 80.62609039468567573 ) ) ;
#94279=CARTESIAN_POINT ( 'NONE',  ( -5.823673210054431948, 21.52544592524334988, 92.70942372801901854 ) ) ;
#94280=CARTESIAN_POINT ( 'NONE',  ( -5.153800228976328057, -19.02544592524343514, 77.29057627198099567 ) ) ;
#94281=CARTESIAN_POINT ( 'NONE',  ( 0.05219959533907565091, 21.53943276465977519, 29.99890960531435979 ) ) ;
#94282=CARTESIAN_POINT ( 'NONE',  ( -5.049401038297874678, -19.05341960407617918, 104.7927570613523471 ) ) ;
#94283=CARTESIAN_POINT ( 'NONE',  ( -21.52544592524334988, -5.823673210054445271, 88.95942372801901854 ) ) ;
#94284=CARTESIAN_POINT ( 'NONE',  ( 14.29746914071037800, 8.314922557961029526, 46.66775706135234714 ) ) ;
#94285=CARTESIAN_POINT ( 'NONE',  ( 5.823673210054125526, 21.52544592524343514, 99.79057627198103830 ) ) ;
#94286=CARTESIAN_POINT ( 'NONE',  ( -5.049401038297874678, -19.05341960407617918, 99.79275706135234714 ) ) ;
#94287=CARTESIAN_POINT ( 'NONE',  ( 5.153800228976335163, 19.02544592524342804, 74.79057627198103830 ) ) ;
#94288=CARTESIAN_POINT ( 'NONE',  ( 19.05341960407617918, -5.049401038297876454, 111.0427570613523329 ) ) ;
#94289=CARTESIAN_POINT ( 'NONE',  ( -19.02544592524342804, 5.153800228976336051, 36.04057627198100988 ) ) ;
#94290=CARTESIAN_POINT ( 'NONE',  ( -12.06949235617739369, -12.14591786802326823, 24.37609039468567573 ) ) ;
#94291=CARTESIAN_POINT ( 'NONE',  ( 12.14591786802309770, 12.06949235617756955, 64.37390960531435269 ) ) ;
#94292=CARTESIAN_POINT ( 'NONE',  ( -12.06949235617739369, -12.14591786802326823, 79.37609039468567573 ) ) ;
#94293=CARTESIAN_POINT ( 'NONE',  ( 5.719274019375673035, 21.55341960407619339, 32.29275706135235424 ) ) ;
#94294=CARTESIAN_POINT ( 'NONE',  ( -9.564922557960796823, -16.46253265017161027, 57.08224293864769550 ) ) ;
#94295=CARTESIAN_POINT ( 'NONE',  ( -0.05219959533909027116, -19.03943276465977164, 72.49890960531435269 ) ) ;
#94296=EDGE_CURVE ( 'NONE', #76130, #149451, #169395, .T. ) ;
#94297=CARTESIAN_POINT ( 'NONE',  ( 16.55341960407618274, -4.379528057220086978, 71.04275706135234714 ) ) ;
#94300=CARTESIAN_POINT ( 'NONE',  ( -21.55341960407619339, 5.719274019375674811, 113.5427570613523756 ) ) ;
#94301=CARTESIAN_POINT ( 'NONE',  ( -19.03943276465977164, 0.05219959533909376836, 31.24890960531435979 ) ) ;
#94302=CARTESIAN_POINT ( 'NONE',  ( -13.89961937509977652, 13.97604488694528158, 105.6239096053143527 ) ) ;
#94303=ORIENTED_EDGE ( 'NONE', *, *, #165511, .F. ) ;
#94304=CARTESIAN_POINT ( 'NONE',  ( -16.52544592524335698, -4.483927247898792601, 33.95942372801901143 ) ) ;
#94305=CARTESIAN_POINT ( 'NONE',  ( 5.049401038297881783, 19.05341960407617563, 42.29275706135234003 ) ) ;
#94306=CARTESIAN_POINT ( 'NONE',  ( -16.52544592524335698, -4.483927247898792601, 48.95942372801902565 ) ) ;
#94307=CARTESIAN_POINT ( 'NONE',  ( 13.97604488694527802, 13.89961937509977652, 44.37390960531435269 ) ) ;
#94308=CARTESIAN_POINT ( 'NONE',  ( 0.05219959533909260263, 19.03943276465977164, 104.9989096053143669 ) ) ;
#94309=CARTESIAN_POINT ( 'NONE',  ( 16.46253265017160672, -9.564922557960803928, 58.33224293864769550 ) ) ;
#94310=CARTESIAN_POINT ( 'NONE',  ( -5.719274019375978568, 21.55341960407610458, 100.2072429386476955 ) ) ;
#94311=CARTESIAN_POINT ( 'NONE',  ( -5.049401038298153566, 19.05341960407611168, 90.20724293864766707 ) ) ;
#94312=CARTESIAN_POINT ( 'NONE',  ( 5.049401038298161559, -19.05341960407611168, 112.7072429386476813 ) ) ;
#94313=CARTESIAN_POINT ( 'NONE',  ( 13.97604488694527802, 13.89961937509977652, 64.37390960531436690 ) ) ;
#94314=CARTESIAN_POINT ( 'NONE',  ( 16.52544592524335698, 4.483927247898782831, 111.4594237280190328 ) ) ;
#94316=CARTESIAN_POINT ( 'NONE',  ( -0.05219959533936034679, 19.03943276465977164, 102.5010903946856757 ) ) ;
#94317=CARTESIAN_POINT ( 'NONE',  ( -13.89961937509957401, -13.97604488694547875, 24.37609039468565442 ) ) ;
#94318=CARTESIAN_POINT ( 'NONE',  ( -4.379528057220328563, 16.55341960407611168, 60.20724293864768839 ) ) ;
#94319=CARTESIAN_POINT ( 'NONE',  ( -21.52544592524334988, -5.823673210054445271, 78.95942372801901854 ) ) ;
#94320=CARTESIAN_POINT ( 'NONE',  ( 16.51473224551069308, 9.474510206698969483, 24.16557627198102765 ) ) ;
#94321=CARTESIAN_POINT ( 'NONE',  ( -4.483927247898539470, -16.52544592524342804, 32.29057627198102409 ) ) ;
#94322=CARTESIAN_POINT ( 'NONE',  ( 15.72974639402176855, 15.80617190586768217, 96.87609039468568994 ) ) ;
#94323=CARTESIAN_POINT ( 'NONE',  ( 16.51473224551069308, 9.474510206698969483, 79.16557627198103830 ) ) ;
#94324=CARTESIAN_POINT ( 'NONE',  ( -0.05219959533937732626, 21.53943276465977519, 47.50109039468568994 ) ) ;
#94325=CARTESIAN_POINT ( 'NONE',  ( -13.97604488694527625, -13.89961937509977652, 96.87390960531433848 ) ) ;
#94326=CARTESIAN_POINT ( 'NONE',  ( 0.05219959533910956823, 16.53943276465976808, 94.99890960531436690 ) ) ;
#94327=CARTESIAN_POINT ( 'NONE',  ( -16.52544592524342804, 4.483927247898546575, 66.04057627198103830 ) ) ;
#94328=CARTESIAN_POINT ( 'NONE',  ( 21.52544592524344225, -5.823673210054117533, 73.54057627198102409 ) ) ;
#94329=CARTESIAN_POINT ( 'NONE',  ( -16.51473224551069308, -9.474510206698971260, 76.66557627198103830 ) ) ;
#94330=CARTESIAN_POINT ( 'NONE',  ( -21.55341960407610458, -5.719274019375992779, 81.45724293864769550 ) ) ;
#94331=CARTESIAN_POINT ( 'NONE',  ( -5.049401038297874678, -19.05341960407617918, 79.79275706135233293 ) ) ;
#94332=CARTESIAN_POINT ( 'NONE',  ( 19.05341960407618274, -5.049401038297876454, 31.04275706135232582 ) ) ;
#94333=CARTESIAN_POINT ( 'NONE',  ( 4.483927247898545687, 16.52544592524342804, 84.79057627198102409 ) ) ;
#94334=CARTESIAN_POINT ( 'NONE',  ( -19.03943276465977164, 0.05219959533909376836, 56.24890960531435979 ) ) ;
#94335=CARTESIAN_POINT ( 'NONE',  ( 5.719274019375991003, -21.55341960407610458, 62.70724293864769550 ) ) ;
#94336=CARTESIAN_POINT ( 'NONE',  ( 16.61371651742598843, -7.165104196376272938, 26.35415069992996706 ) ) ;
#94337=CARTESIAN_POINT ( 'NONE',  ( -0.05219959533934338120, 16.53943276465976808, 107.5010903946856899 ) ) ;
#94338=CARTESIAN_POINT ( 'NONE',  ( -5.153800228976607833, 19.02544592524334988, 102.7094237280189759 ) ) ;
#94339=CARTESIAN_POINT ( 'NONE',  ( -16.52544592524342804, 4.483927247898546575, 86.04057627198102409 ) ) ;
#94340=CARTESIAN_POINT ( 'NONE',  ( -18.56101223717332260, -5.500000000000006217, 96.44978406935675252 ) ) ;
#94341=CARTESIAN_POINT ( 'NONE',  ( -5.049401038298153566, 19.05341960407611168, 75.20724293864769550 ) ) ;
#94342=CARTESIAN_POINT ( 'NONE',  ( -19.05341960407611168, -5.049401038298163336, 36.45724293864766707 ) ) ;
#94343=CARTESIAN_POINT ( 'NONE',  ( -4.379528057220328563, 16.55341960407611168, 70.20724293864769550 ) ) ;
#94344=CARTESIAN_POINT ( 'NONE',  ( 5.049401038298161559, -19.05341960407611168, 97.70724293864766707 ) ) ;
#94345=CARTESIAN_POINT ( 'NONE',  ( 9.474510206698729675, 16.51473224551082808, 92.08442372801900433 ) ) ;
#94346=CARTESIAN_POINT ( 'NONE',  ( -9.564922557960796823, -16.46253265017161027, 62.08224293864769550 ) ) ;
#94347=CARTESIAN_POINT ( 'NONE',  ( 19.03943276465977164, -0.05219959533909143690, 83.74890960531436690 ) ) ;
#94348=CARTESIAN_POINT ( 'NONE',  ( -15.72974639402197994, 15.80617190586746368, 75.62390960531439532 ) ) ;
#94349=CARTESIAN_POINT ( 'NONE',  ( 16.53943276465976808, 0.05219959533934440121, 71.25109039468568994 ) ) ;
#94350=CARTESIAN_POINT ( 'NONE',  ( -17.44270441346520073, 5.991230190322872851, 93.63664920735774899 ) ) ;
#94351=CARTESIAN_POINT ( 'NONE',  ( -5.049401038298153566, 19.05341960407611168, 60.20724293864768129 ) ) ;
#94352=CARTESIAN_POINT ( 'NONE',  ( 5.719274019375991003, -21.55341960407610458, 72.70724293864769550 ) ) ;
#94353=CARTESIAN_POINT ( 'NONE',  ( -13.89961937509957401, -13.97604488694547875, 89.37609039468563310 ) ) ;
#94354=CARTESIAN_POINT ( 'NONE',  ( -8.224510206698948167, 14.34966873604960824, 40.41557627198103120 ) ) ;
#94355=CARTESIAN_POINT ( 'NONE',  ( -15.72974639402176322, -15.80617190586768395, 49.37609039468569705 ) ) ;
#94356=CARTESIAN_POINT ( 'NONE',  ( 9.474510206698729675, 16.51473224551082808, 72.08442372801900433 ) ) ;
#94357=CARTESIAN_POINT ( 'NONE',  ( 4.379528057220092307, 16.55341960407617563, 77.29275706135234714 ) ) ;
#94358=CARTESIAN_POINT ( 'NONE',  ( 19.05341960407611168, 5.049401038298154454, 108.9572429386477097 ) ) ;
#94359=CARTESIAN_POINT ( 'NONE',  ( 19.02544592524343514, -5.153800228976328945, 103.5405762719810099 ) ) ;
#94360=CARTESIAN_POINT ( 'NONE',  ( -16.20579543436678449, 7.371946100355091680, 79.43479165828127009 ) ) ;
#94361=CARTESIAN_POINT ( 'NONE',  ( -14.29746914071037622, -8.314922557961029526, 89.16775706135236135 ) ) ;
#94362=CARTESIAN_POINT ( 'NONE',  ( -16.53943276465976808, -0.05219959533934237506, 48.75109039468568284 ) ) ;
#94363=CARTESIAN_POINT ( 'NONE',  ( 5.153800228976335163, 19.02544592524342804, 59.79057627198100988 ) ) ;
#94364=CARTESIAN_POINT ( 'NONE',  ( 5.153800228976335163, 19.02544592524342804, 59.79057627198100988 ) ) ;
#94365=CARTESIAN_POINT ( 'NONE',  ( 18.62759615963255655, 10.81492255796105972, 56.66775706135235424 ) ) ;
#94366=CARTESIAN_POINT ( 'NONE',  ( 4.483927247898790824, -16.52544592524335698, 60.20942372801902565 ) ) ;
#94367=CARTESIAN_POINT ( 'NONE',  ( -4.483927247898539470, -16.52544592524342804, 37.29057627198102409 ) ) ;
#94368=CARTESIAN_POINT ( 'NONE',  ( -9.564922557960796823, -16.46253265017161027, 47.08224293864769550 ) ) ;
#94369=CARTESIAN_POINT ( 'NONE',  ( 9.564922557960805705, 16.46253265017160317, 39.58224293864768839 ) ) ;
#94370=CARTESIAN_POINT ( 'NONE',  ( -12.06949235617739369, -12.14591786802326823, 34.37609039468568284 ) ) ;
#94371=CARTESIAN_POINT ( 'NONE',  ( 13.97604488694548053, -13.89961937509957401, 75.62609039468564731 ) ) ;
#94372=CARTESIAN_POINT ( 'NONE',  ( -8.314922557960811034, -14.29746914071050412, 87.08224293864769550 ) ) ;
#94373=CARTESIAN_POINT ( 'NONE',  ( 19.03943276465977164, -0.05219959533909143690, 48.74890960531435979 ) ) ;
#94374=CARTESIAN_POINT ( 'NONE',  ( -13.97604488694547697, 13.89961937509957934, 83.12609039468564731 ) ) ;
#94376=CARTESIAN_POINT ( 'NONE',  ( 5.719274019375673035, 21.55341960407619339, 92.29275706135236135 ) ) ;
#94377=CARTESIAN_POINT ( 'NONE',  ( -16.52544592524335698, -4.483927247898792601, 58.95942372801902565 ) ) ;
#94378=CARTESIAN_POINT ( 'NONE',  ( 17.12812012977024878, 6.668231424566068988, 38.85948759323144941 ) ) ;
#94379=CARTESIAN_POINT ( 'NONE',  ( 18.62759615963271287, -10.81492255796078972, 48.33224293864770260 ) ) ;
#94380=CARTESIAN_POINT ( 'NONE',  ( -8.224510206698735004, -14.34966873604973081, 39.58442372801901143 ) ) ;
#94381=CARTESIAN_POINT ( 'NONE',  ( 18.22780087662121673, 5.500000000000056843, 88.98459894673892734 ) ) ;
#94382=CARTESIAN_POINT ( 'NONE',  ( 0.05219959533936267826, -19.03943276465977164, 25.00109039468566152 ) ) ;
#94383=CARTESIAN_POINT ( 'NONE',  ( -5.153800228976328057, -19.02544592524343514, 77.29057627198099567 ) ) ;
#94385=CARTESIAN_POINT ( 'NONE',  ( 13.89961937509977652, -13.97604488694527269, 53.12390960531434558 ) ) ;
#94387=CARTESIAN_POINT ( 'NONE',  ( -0.05219959533909027116, -19.03943276465977164, 67.49890960531436690 ) ) ;
#94388=CARTESIAN_POINT ( 'NONE',  ( 17.49999999999999645, -3.209263204892621513, 112.2619682560626444 ) ) ;
#94389=CARTESIAN_POINT ( 'NONE',  ( 5.153800228976615827, -19.02544592524334988, 40.20942372801898301 ) ) ;
#94390=CARTESIAN_POINT ( 'NONE',  ( 0.05219959533936267826, -19.03943276465977164, 20.00109039468567218 ) ) ;
#94391=CARTESIAN_POINT ( 'NONE',  ( 16.53943276465976808, -0.05219959533910856209, 38.74890960531435979 ) ) ;
#94392=CARTESIAN_POINT ( 'NONE',  ( -16.51473224551069308, -9.474510206698971260, 41.66557627198103120 ) ) ;
#94393=CARTESIAN_POINT ( 'NONE',  ( -16.46253265017160317, 9.564922557960807481, 100.8322429386477097 ) ) ;
#94394=CARTESIAN_POINT ( 'NONE',  ( 10.72451020669871369, 18.67979575497193778, 72.08442372801899012 ) ) ;
#94395=CARTESIAN_POINT ( 'NONE',  ( -9.564922557960796823, -16.46253265017161027, 52.08224293864768839 ) ) ;
#94396=CARTESIAN_POINT ( 'NONE',  ( 21.53943276465977519, 0.05219959533937863772, 86.25109039468568994 ) ) ;
#94397=CARTESIAN_POINT ( 'NONE',  ( 16.46253265017160672, -9.564922557960803928, 113.3322429386476955 ) ) ;
#94398=CARTESIAN_POINT ( 'NONE',  ( -5.049401038298153566, 19.05341960407611168, 35.20724293864768839 ) ) ;
#94399=CARTESIAN_POINT ( 'NONE',  ( 5.719274019375673035, 21.55341960407619339, 27.29275706135234358 ) ) ;
#94400=CARTESIAN_POINT ( 'NONE',  ( -19.03943276465977164, -0.05219959533935918106, 53.75109039468566863 ) ) ;
#94401=CARTESIAN_POINT ( 'NONE',  ( 16.46253265017160672, -9.564922557960803928, 28.33224293864769550 ) ) ;
#94402=CARTESIAN_POINT ( 'NONE',  ( 19.02544592524343514, -5.153800228976328945, 73.54057627198103830 ) ) ;
#94403=CARTESIAN_POINT ( 'NONE',  ( 9.474510206698729675, 16.51473224551082808, 107.0844237280190043 ) ) ;
#94404=CARTESIAN_POINT ( 'NONE',  ( 0.05219959533910956823, 16.53943276465976808, 74.99890960531435269 ) ) ;
#94405=CARTESIAN_POINT ( 'NONE',  ( 15.72974639402199770, -15.80617190586745480, 33.12390960531435979 ) ) ;
#94406=CARTESIAN_POINT ( 'NONE',  ( 5.153800228976615827, -19.02544592524334988, 100.2094237280190043 ) ) ;
#94407=CARTESIAN_POINT ( 'NONE',  ( -0.05219959533907301413, -21.53943276465977519, 102.4989096053143811 ) ) ;
#94408=CARTESIAN_POINT ( 'NONE',  ( 0.05219959533937995610, -21.53943276465977519, 60.00109039468568284 ) ) ;
#94409=CARTESIAN_POINT ( 'NONE',  ( 12.14591786802327356, -12.06949235617739191, 50.62609039468568994 ) ) ;
#94410=CARTESIAN_POINT ( 'NONE',  ( 16.55341960407618274, -4.379528057220086978, 51.04275706135234714 ) ) ;
#94411=CARTESIAN_POINT ( 'NONE',  ( 15.80617190586746368, 15.72974639402197994, 69.37390960531436690 ) ) ;
#94413=CARTESIAN_POINT ( 'NONE',  ( 13.97604488694527802, 13.89961937509977652, 44.37390960531435269 ) ) ;
#94414=CARTESIAN_POINT ( 'NONE',  ( -4.483927247898782831, 16.52544592524335698, 82.70942372801900433 ) ) ;
#94415=CARTESIAN_POINT ( 'NONE',  ( 18.62759615963271287, -10.81492255796078972, 108.3322429386477097 ) ) ;
#94416=CARTESIAN_POINT ( 'NONE',  ( 16.52544592524342804, -4.483927247898539470, 48.54057627198103120 ) ) ;
#94417=CARTESIAN_POINT ( 'NONE',  ( 16.51473224551069308, 9.474510206698969483, 79.16557627198103830 ) ) ;
#94418=CARTESIAN_POINT ( 'NONE',  ( 4.379528057220092307, 16.55341960407617563, 72.29275706135236135 ) ) ;
#94419=CARTESIAN_POINT ( 'NONE',  ( 0.05219959533934541429, -16.53943276465976808, 20.00109039468568639 ) ) ;
#94420=CARTESIAN_POINT ( 'NONE',  ( 0.05219959533907565091, 21.53943276465977519, 109.9989096053143527 ) ) ;
#94421=CARTESIAN_POINT ( 'NONE',  ( -14.34966873604960291, -8.224510206698953496, 41.66557627198103120 ) ) ;
#94423=CARTESIAN_POINT ( 'NONE',  ( -16.29526858892874941, 7.335722546920117715, 74.20329402199800484 ) ) ;
#94424=CARTESIAN_POINT ( 'NONE',  ( 21.52544592524344225, -5.823673210054117533, 88.54057627198103830 ) ) ;
#94425=CARTESIAN_POINT ( 'NONE',  ( -14.34966873604960291, -8.224510206698953496, 31.66557627198102054 ) ) ;
#94428=CARTESIAN_POINT ( 'NONE',  ( -21.53943276465977519, 0.05219959533907696930, 106.2489096053143811 ) ) ;
#94429=CARTESIAN_POINT ( 'NONE',  ( -19.03943276465977164, 0.05219959533909376836, 111.2489096053143669 ) ) ;
#94430=CARTESIAN_POINT ( 'NONE',  ( -21.55341960407619339, 5.719274019375674811, 23.54275706135235424 ) ) ;
#94431=CARTESIAN_POINT ( 'NONE',  ( -0.05219959533910754901, -16.53943276465976808, 57.49890960531435979 ) ) ;
#94432=CARTESIAN_POINT ( 'NONE',  ( -16.53943276465976808, -0.05219959533934237506, 53.75109039468568994 ) ) ;
#94433=CARTESIAN_POINT ( 'NONE',  ( 9.564922557960805705, 16.46253265017160317, 59.58224293864769550 ) ) ;
#94434=CARTESIAN_POINT ( 'NONE',  ( -13.97604488694547697, 13.89961937509957934, 48.12609039468566863 ) ) ;
#94435=CARTESIAN_POINT ( 'NONE',  ( -9.474510206698964154, 16.51473224551069663, 85.41557627198102409 ) ) ;
#94436=CARTESIAN_POINT ( 'NONE',  ( -21.53943276465977519, 0.05219959533907696930, 31.24890960531435979 ) ) ;
#94438=CARTESIAN_POINT ( 'NONE',  ( -5.153800228976328057, -19.02544592524343514, 47.29057627198102409 ) ) ;
#94439=CARTESIAN_POINT ( 'NONE',  ( -12.14591786802326823, 12.06949235617739902, 28.12609039468568284 ) ) ;
#94440=CARTESIAN_POINT ( 'NONE',  ( -5.049401038297874678, -19.05341960407617918, 64.79275706135233293 ) ) ;
#94441=CARTESIAN_POINT ( 'NONE',  ( -21.55341960407610458, -5.719274019375992779, 101.4572429386476955 ) ) ;
#94443=CARTESIAN_POINT ( 'NONE',  ( 4.379528057220339221, -16.55341960407611168, 27.70724293864769905 ) ) ;
#94444=CARTESIAN_POINT ( 'NONE',  ( 13.97604488694527802, 13.89961937509977652, 89.37390960531436690 ) ) ;
#94445=CARTESIAN_POINT ( 'NONE',  ( -15.72974639402197994, 15.80617190586746368, 55.62390960531436690 ) ) ;
#94446=CARTESIAN_POINT ( 'NONE',  ( -21.53943276465977519, 0.05219959533907696930, 91.24890960531436690 ) ) ;
#94447=CARTESIAN_POINT ( 'NONE',  ( 12.06949235617739724, 12.14591786802326823, 26.87609039468567218 ) ) ;
#94448=CARTESIAN_POINT ( 'NONE',  ( 5.823673210054125526, 21.52544592524343514, 29.79057627198102409 ) ) ;
#94449=CARTESIAN_POINT ( 'NONE',  ( 5.719274019375673035, 21.55341960407619339, 92.29275706135236135 ) ) ;
#94450=CARTESIAN_POINT ( 'NONE',  ( -0.05219959533909027116, -19.03943276465977164, 87.49890960531436690 ) ) ;
#94451=CARTESIAN_POINT ( 'NONE',  ( 13.97604488694527802, 13.89961937509977652, 29.37390960531435979 ) ) ;
#94452=CARTESIAN_POINT ( 'NONE',  ( 16.51473224551069308, 9.474510206698969483, 84.16557627198102409 ) ) ;
#94453=CARTESIAN_POINT ( 'NONE',  ( -16.53943276465976808, 0.05219959533911058130, 101.2489096053143669 ) ) ;
#94454=CARTESIAN_POINT ( 'NONE',  ( 5.049401038298161559, -19.05341960407611168, 67.70724293864769550 ) ) ;
#94455=CARTESIAN_POINT ( 'NONE',  ( -19.03943276465977164, -0.05219959533935918106, 113.7510903946856757 ) ) ;
#94457=CARTESIAN_POINT ( 'NONE',  ( -18.67979575497193778, 10.72451020669871902, 93.33442372801901854 ) ) ;
#94458=CARTESIAN_POINT ( 'NONE',  ( 19.03943276465977164, -0.05219959533909143690, 108.7489096053143527 ) ) ;
#94459=CARTESIAN_POINT ( 'NONE',  ( 16.55341960407618274, -4.379528057220086978, 91.04275706135236135 ) ) ;
#94461=CARTESIAN_POINT ( 'NONE',  ( -9.564922557961040184, 16.46253265017147172, 67.91775706135233293 ) ) ;
#94462=CARTESIAN_POINT ( 'NONE',  ( 19.03943276465977164, 0.05219959533936151252, 26.25109039468566507 ) ) ;
#94464=CARTESIAN_POINT ( 'NONE',  ( -5.153800228976328057, -19.02544592524343514, 22.29057627198102765 ) ) ;
#94465=CARTESIAN_POINT ( 'NONE',  ( -4.379528057220328563, 16.55341960407611168, 30.20724293864769550 ) ) ;
#94466=CARTESIAN_POINT ( 'NONE',  ( -9.564922557960796823, -16.46253265017161027, 22.08224293864768839 ) ) ;
#94467=CARTESIAN_POINT ( 'NONE',  ( 4.379528057220092307, 16.55341960407617563, 112.2927570613523471 ) ) ;
#94468=CARTESIAN_POINT ( 'NONE',  ( -18.56101223717332971, -5.500000000000068390, 86.44978406935680937 ) ) ;
#94469=CARTESIAN_POINT ( 'NONE',  ( -16.53943276465976808, -0.05219959533934237506, 93.75109039468567573 ) ) ;
#94470=CARTESIAN_POINT ( 'NONE',  ( 9.564922557960805705, 16.46253265017160317, 39.58224293864768839 ) ) ;
#94471=CARTESIAN_POINT ( 'NONE',  ( 15.72974639402176855, 15.80617190586768217, 91.87609039468568994 ) ) ;
#94472=CARTESIAN_POINT ( 'NONE',  ( 19.03943276465977164, 0.05219959533936151252, 106.2510903946856615 ) ) ;
#94473=CARTESIAN_POINT ( 'NONE',  ( -5.719274019375665041, -21.55341960407619695, 79.79275706135236135 ) ) ;
#94474=CARTESIAN_POINT ( 'NONE',  ( 5.049401038297881783, 19.05341960407617563, 52.29275706135234003 ) ) ;
#94475=CARTESIAN_POINT ( 'NONE',  ( 13.97604488694527802, 13.89961937509977652, 89.37390960531436690 ) ) ;
#94476=CARTESIAN_POINT ( 'NONE',  ( 0.05219959533909260263, 19.03943276465977164, 74.99890960531435269 ) ) ;
#94477=CARTESIAN_POINT ( 'NONE',  ( 17.31728774477274158, 6.344390552232410663, 71.68093348310685542 ) ) ;
#94478=CARTESIAN_POINT ( 'NONE',  ( 4.379528057220339221, -16.55341960407611168, 67.70724293864769550 ) ) ;
#94479=CARTESIAN_POINT ( 'NONE',  ( 0.05219959533907565091, 21.53943276465977519, 54.99890960531435269 ) ) ;
#94480=CARTESIAN_POINT ( 'NONE',  ( 19.05341960407611168, 5.049401038298154454, 48.95724293864768129 ) ) ;
#94481=CARTESIAN_POINT ( 'NONE',  ( -5.823673210054116645, -21.52544592524344225, 82.29057627198103830 ) ) ;
#94482=CARTESIAN_POINT ( 'NONE',  ( 16.52544592524335698, 4.483927247898782831, 76.45942372801901854 ) ) ;
#94484=CARTESIAN_POINT ( 'NONE',  ( -19.05341960407611168, -5.049401038298163336, 46.45724293864768129 ) ) ;
#94485=CARTESIAN_POINT ( 'NONE',  ( -8.224510206698948167, 14.34966873604960824, 75.41557627198102409 ) ) ;
#94487=CARTESIAN_POINT ( 'NONE',  ( -9.474510206698964154, 16.51473224551069663, 55.41557627198103120 ) ) ;
#94488=CARTESIAN_POINT ( 'NONE',  ( -5.153800228976328057, -19.02544592524343514, 27.29057627198103120 ) ) ;
#94489=CARTESIAN_POINT ( 'NONE',  ( 9.474510206698729675, 16.51473224551082808, 67.08442372801900433 ) ) ;
#94490=CARTESIAN_POINT ( 'NONE',  ( -12.06949235617756955, 12.14591786802309770, 75.62390960531439532 ) ) ;
#94491=CARTESIAN_POINT ( 'NONE',  ( 18.62759615963255655, 10.81492255796105972, 51.66775706135234714 ) ) ;
#94492=CARTESIAN_POINT ( 'NONE',  ( -0.05219959533909027116, -19.03943276465977164, 37.49890960531436690 ) ) ;
#94493=CARTESIAN_POINT ( 'NONE',  ( 21.53943276465977519, -0.05219959533907433946, 108.7489096053143669 ) ) ;
#94494=FACE_OUTER_BOUND ( 'NONE', #162410, .T. ) ;
#94495=CARTESIAN_POINT ( 'NONE',  ( 0.05219959533910956823, 16.53943276465976808, 89.99890960531438111 ) ) ;
#94497=CARTESIAN_POINT ( 'NONE',  ( 5.049401038298161559, -19.05341960407611168, 42.70724293864767418 ) ) ;
#94499=CARTESIAN_POINT ( 'NONE',  ( -9.474510206698720793, -16.51473224551083518, 94.58442372801900433 ) ) ;
#94500=CARTESIAN_POINT ( 'NONE',  ( 0.05219959533909260263, 19.03943276465977164, 104.9989096053143669 ) ) ;
#94501=CARTESIAN_POINT ( 'NONE',  ( -5.823673210054431948, 21.52544592524334988, 32.70942372801900433 ) ) ;
#94502=CARTESIAN_POINT ( 'NONE',  ( 5.049401038298161559, -19.05341960407611168, 77.70724293864765286 ) ) ;
#94503=CARTESIAN_POINT ( 'NONE',  ( 19.03943276465977164, 0.05219959533936151252, 76.25109039468566152 ) ) ;
#94504=CARTESIAN_POINT ( 'NONE',  ( -13.89961937509977652, 13.97604488694528158, 40.62390960531435979 ) ) ;
#94505=CARTESIAN_POINT ( 'NONE',  ( -16.53943276465976808, 0.05219959533911058130, 66.24890960531436690 ) ) ;
#94506=CARTESIAN_POINT ( 'NONE',  ( 14.29746914071049879, -8.314922557960816363, 63.33224293864770260 ) ) ;
#94507=CARTESIAN_POINT ( 'NONE',  ( -5.049401038298153566, 19.05341960407611168, 75.20724293864769550 ) ) ;
#94508=CARTESIAN_POINT ( 'NONE',  ( -10.72451020669898014, 18.67979575497178502, 105.4155762719810383 ) ) ;
#94509=CARTESIAN_POINT ( 'NONE',  ( -9.474510206698964154, 16.51473224551069663, 65.41557627198102409 ) ) ;
#94510=CARTESIAN_POINT ( 'NONE',  ( -19.03943276465977164, -0.05219959533935918106, 18.75109039468567218 ) ) ;
#94511=CARTESIAN_POINT ( 'NONE',  ( 16.51473224551069308, 9.474510206698969483, 34.16557627198102409 ) ) ;
#94512=CARTESIAN_POINT ( 'NONE',  ( 8.224510206698953496, -14.34966873604960469, 22.91557627198102765 ) ) ;
#94513=CARTESIAN_POINT ( 'NONE',  ( -16.55341960407611168, -4.379528057220339221, 111.4572429386476813 ) ) ;
#94514=CARTESIAN_POINT ( 'NONE',  ( 16.46253265017146816, 9.564922557961045513, 106.6677570613523471 ) ) ;
#94516=CARTESIAN_POINT ( 'NONE',  ( 15.72974639402176855, 15.80617190586768217, 26.87609039468567218 ) ) ;
#94517=CARTESIAN_POINT ( 'NONE',  ( -16.46253265017146816, -9.564922557961047289, 69.16775706135233293 ) ) ;
#94518=CARTESIAN_POINT ( 'NONE',  ( 16.55341960407618274, -4.379528057220086978, 111.0427570613523613 ) ) ;
#94519=CARTESIAN_POINT ( 'NONE',  ( 21.52544592524344225, -5.823673210054117533, 78.54057627198103830 ) ) ;
#94520=CARTESIAN_POINT ( 'NONE',  ( -18.67979575497178146, -10.72451020669898902, 26.66557627198103475 ) ) ;
#94521=CARTESIAN_POINT ( 'NONE',  ( -14.29746914071049879, 8.314922557960819915, 50.83224293864770971 ) ) ;
#94522=CARTESIAN_POINT ( 'NONE',  ( 19.02544592524343514, -5.153800228976328945, 33.54057627198102409 ) ) ;
#94523=CARTESIAN_POINT ( 'NONE',  ( -9.474510206698964154, 16.51473224551069663, 35.41557627198102409 ) ) ;
#94524=CARTESIAN_POINT ( 'NONE',  ( 16.51473224551083163, -9.474510206698727899, 25.83442372801900078 ) ) ;
#94525=CARTESIAN_POINT ( 'NONE',  ( 4.379528057220092307, 16.55341960407617563, 92.29275706135236135 ) ) ;
#94526=CARTESIAN_POINT ( 'NONE',  ( -16.52544592524335698, -4.483927247898792601, 53.95942372801900433 ) ) ;
#94527=CARTESIAN_POINT ( 'NONE',  ( 18.62759615963271287, -10.81492255796078972, 23.33224293864769194 ) ) ;
#94528=CARTESIAN_POINT ( 'NONE',  ( 13.97604488694527802, 13.89961937509977652, 54.37390960531435979 ) ) ;
#94529=CARTESIAN_POINT ( 'NONE',  ( 5.719274019375673035, 21.55341960407619339, 107.2927570613523471 ) ) ;
#94530=CARTESIAN_POINT ( 'NONE',  ( 19.02544592524343514, -5.153800228976328945, 83.54057627198100988 ) ) ;
#94531=CARTESIAN_POINT ( 'NONE',  ( -12.14591786802326823, 12.06949235617739902, 58.12609039468568994 ) ) ;
#94532=CARTESIAN_POINT ( 'NONE',  ( -16.52544592524342804, 4.483927247898546575, 111.0405762719810525 ) ) ;
#94533=CARTESIAN_POINT ( 'NONE',  ( -16.52544592524342804, 4.483927247898546575, 26.04057627198103475 ) ) ;
#94535=CARTESIAN_POINT ( 'NONE',  ( -21.53943276465977519, -0.05219959533937600094, 73.75109039468567573 ) ) ;
#94536=CARTESIAN_POINT ( 'NONE',  ( -5.153800228976328057, -19.02544592524343514, 87.29057627198103830 ) ) ;
#94537=CARTESIAN_POINT ( 'NONE',  ( 19.05341960407611168, 5.049401038298154454, 73.95724293864768129 ) ) ;
#94538=CARTESIAN_POINT ( 'NONE',  ( 13.89961937509977652, -13.97604488694527269, 113.1239096053143527 ) ) ;
#94540=CARTESIAN_POINT ( 'NONE',  ( -12.14591786802309592, -12.06949235617757132, 61.87390960531436690 ) ) ;
#94541=CARTESIAN_POINT ( 'NONE',  ( -12.14591786802326823, 12.06949235617739902, 113.1260903946856899 ) ) ;
#94543=CARTESIAN_POINT ( 'NONE',  ( 16.55341960407611168, 4.379528057220329451, 33.95724293864769550 ) ) ;
#94544=CARTESIAN_POINT ( 'NONE',  ( 16.55341960407618274, -4.379528057220086978, 41.04275706135236135 ) ) ;
#94546=CARTESIAN_POINT ( 'NONE',  ( 13.89961937509957401, 13.97604488694547697, 36.87609039468565442 ) ) ;
#94547=CARTESIAN_POINT ( 'NONE',  ( 16.51473224551069308, 9.474510206698969483, 79.16557627198103830 ) ) ;
#94548=CARTESIAN_POINT ( 'NONE',  ( 0.05219959533936267826, -19.03943276465977164, 55.00109039468566863 ) ) ;
#94549=CARTESIAN_POINT ( 'NONE',  ( 19.05341960407617918, -5.049401038297876454, 61.04275706135232582 ) ) ;
#94550=CARTESIAN_POINT ( 'NONE',  ( -16.51473224551082808, 9.474510206698731452, 103.3344237280190043 ) ) ;
#94551=CARTESIAN_POINT ( 'NONE',  ( 4.379528057220092307, 16.55341960407617563, 87.29275706135236135 ) ) ;
#94552=CARTESIAN_POINT ( 'NONE',  ( -13.89961937509977652, 13.97604488694528158, 25.62390960531434558 ) ) ;
#94554=CARTESIAN_POINT ( 'NONE',  ( -19.03943276465977164, 0.05219959533909376836, 101.2489096053143669 ) ) ;
#94555=CARTESIAN_POINT ( 'NONE',  ( -21.52544592524334988, -5.823673210054445271, 43.95942372801902565 ) ) ;
#94557=CARTESIAN_POINT ( 'NONE',  ( -5.049401038297874678, -19.05341960407617918, 94.79275706135230450 ) ) ;
#94559=CARTESIAN_POINT ( 'NONE',  ( -9.564922557960796823, -16.46253265017161027, 47.08224293864769550 ) ) ;
#94560=CARTESIAN_POINT ( 'NONE',  ( 16.51473224551069308, 9.474510206698969483, 99.16557627198102409 ) ) ;
#94561=CARTESIAN_POINT ( 'NONE',  ( -4.483927247898539470, -16.52544592524342804, 57.29057627198103120 ) ) ;
#94562=CARTESIAN_POINT ( 'NONE',  ( -19.02544592524342804, 5.153800228976336051, 46.04057627198101699 ) ) ;
#94563=CARTESIAN_POINT ( 'NONE',  ( 0.05219959533909260263, 19.03943276465977164, 64.99890960531436690 ) ) ;
#94564=CARTESIAN_POINT ( 'NONE',  ( -19.05341960407617563, 5.049401038297882671, 58.54275706135234003 ) ) ;
#94565=CARTESIAN_POINT ( 'NONE',  ( -16.46253265017146816, -9.564922557961047289, 29.16775706135232937 ) ) ;
#94566=CARTESIAN_POINT ( 'NONE',  ( -19.02544592524334988, -5.153800228976617603, 43.95942372801899012 ) ) ;
#94567=CARTESIAN_POINT ( 'NONE',  ( 19.05341960407611168, 5.049401038298154454, 83.95724293864766707 ) ) ;
#94569=CARTESIAN_POINT ( 'NONE',  ( 15.80617190586746368, 15.72974639402197994, 74.37390960531436690 ) ) ;
#94570=CARTESIAN_POINT ( 'NONE',  ( 14.29746914071049879, -8.314922557960816363, 63.33224293864770260 ) ) ;
#94571=CARTESIAN_POINT ( 'NONE',  ( -5.153800228976607833, 19.02544592524334988, 37.70942372801899722 ) ) ;
#94572=CARTESIAN_POINT ( 'NONE',  ( -5.823673210054116645, -21.52544592524344225, 52.29057627198102409 ) ) ;
#94573=CARTESIAN_POINT ( 'NONE',  ( 18.67979575497178502, 10.72451020669898547, 39.16557627198102409 ) ) ;
#94574=CARTESIAN_POINT ( 'NONE',  ( 13.97604488694527802, 13.89961937509977652, 69.37390960531436690 ) ) ;
#94575=CARTESIAN_POINT ( 'NONE',  ( 9.564922557960805705, 16.46253265017160317, 39.58224293864768839 ) ) ;
#94576=CARTESIAN_POINT ( 'NONE',  ( -14.29746914071049879, 8.314922557960819915, 115.8322429386477097 ) ) ;
#94577=CARTESIAN_POINT ( 'NONE',  ( 5.823673210054125526, 21.52544592524343514, 104.7905762719810241 ) ) ;
#94578=CARTESIAN_POINT ( 'NONE',  ( 13.97604488694527802, 13.89961937509977652, 109.3739096053143669 ) ) ;
#94579=CARTESIAN_POINT ( 'NONE',  ( -0.05219959533937732626, 21.53943276465977519, 27.50109039468567929 ) ) ;
#94580=CARTESIAN_POINT ( 'NONE',  ( -13.89961937509977652, 13.97604488694528158, 30.62390960531435269 ) ) ;
#94581=CARTESIAN_POINT ( 'NONE',  ( 0.05219959533907565091, 21.53943276465977519, 99.99890960531436690 ) ) ;
#94582=CARTESIAN_POINT ( 'NONE',  ( 13.89961937509957401, 13.97604488694547697, 51.87609039468566863 ) ) ;
#94583=CARTESIAN_POINT ( 'NONE',  ( -13.97604488694527625, -13.89961937509977652, 21.87390960531435979 ) ) ;
#94584=CARTESIAN_POINT ( 'NONE',  ( 5.153800228976335163, 19.02544592524342804, 29.79057627198102409 ) ) ;
#94586=CARTESIAN_POINT ( 'NONE',  ( -4.483927247898782831, 16.52544592524335698, 62.70942372801902565 ) ) ;
#94587=CARTESIAN_POINT ( 'NONE',  ( 9.474510206698971260, -16.51473224551069308, 27.91557627198103120 ) ) ;
#94589=CARTESIAN_POINT ( 'NONE',  ( 5.049401038298161559, -19.05341960407611168, 72.70724293864768129 ) ) ;
#94590=CARTESIAN_POINT ( 'NONE',  ( -12.06949235617756955, 12.14591786802309770, 105.6239096053143669 ) ) ;
#94592=CARTESIAN_POINT ( 'NONE',  ( -21.55341960407610458, -5.719274019375992779, 41.45724293864769550 ) ) ;
#94593=CARTESIAN_POINT ( 'NONE',  ( 16.53943276465976808, -0.05219959533910856209, 78.74890960531436690 ) ) ;
#94594=CARTESIAN_POINT ( 'NONE',  ( 16.55341960407618274, -4.379528057220086978, 36.04275706135234714 ) ) ;
#94595=CARTESIAN_POINT ( 'NONE',  ( 21.53943276465977519, 0.05219959533937863772, 81.25109039468568994 ) ) ;
#94596=CARTESIAN_POINT ( 'NONE',  ( 19.02544592524343514, -5.153800228976328945, 23.54057627198102054 ) ) ;
#94597=CARTESIAN_POINT ( 'NONE',  ( 14.29746914071049879, -8.314922557960816363, 23.33224293864769194 ) ) ;
#94598=CARTESIAN_POINT ( 'NONE',  ( -16.52544592524342804, 4.483927247898546575, 56.04057627198102409 ) ) ;
#94599=CARTESIAN_POINT ( 'NONE',  ( 0.05219959533909260263, 19.03943276465977164, 49.99890960531435979 ) ) ;
#94600=CARTESIAN_POINT ( 'NONE',  ( -21.55341960407619339, 5.719274019375674811, 98.54275706135234714 ) ) ;
#94601=CARTESIAN_POINT ( 'NONE',  ( -21.55341960407610458, -5.719274019375992779, 111.4572429386476813 ) ) ;
#94602=CARTESIAN_POINT ( 'NONE',  ( -0.05219959533937732626, 21.53943276465977519, 72.50109039468568994 ) ) ;
#94603=CARTESIAN_POINT ( 'NONE',  ( 14.34966873604972726, -8.224510206698740333, 35.83442372801901143 ) ) ;
#94604=CARTESIAN_POINT ( 'NONE',  ( -16.52544592524342804, 4.483927247898546575, 76.04057627198102409 ) ) ;
#94605=CARTESIAN_POINT ( 'NONE',  ( 21.55341960407619695, -5.719274019375665929, 81.04275706135236135 ) ) ;
#94606=CARTESIAN_POINT ( 'NONE',  ( -16.55341960407617563, 4.379528057220093196, 108.5427570613523756 ) ) ;
#94607=CARTESIAN_POINT ( 'NONE',  ( -16.31925111598458145, 7.325300261831528381, 115.1642453896725584 ) ) ;
#94608=CARTESIAN_POINT ( 'NONE',  ( -0.05219959533934338120, 16.53943276465976808, 37.50109039468568284 ) ) ;
#94609=CARTESIAN_POINT ( 'NONE',  ( 4.379528057220339221, -16.55341960407611168, 42.70724293864770260 ) ) ;
#94610=CARTESIAN_POINT ( 'NONE',  ( -4.379528057220086978, -16.55341960407618274, 84.79275706135234714 ) ) ;
#94611=CARTESIAN_POINT ( 'NONE',  ( -5.049401038298153566, 19.05341960407611168, 105.2072429386476671 ) ) ;
#94612=CARTESIAN_POINT ( 'NONE',  ( 5.049401038298161559, -19.05341960407611168, 97.70724293864766707 ) ) ;
#94613=CARTESIAN_POINT ( 'NONE',  ( -21.55341960407619339, 5.719274019375674811, 98.54275706135234714 ) ) ;
#94614=CARTESIAN_POINT ( 'NONE',  ( 16.55341960407618274, -4.379528057220086978, 101.0427570613523756 ) ) ;
#94615=CARTESIAN_POINT ( 'NONE',  ( -8.314922557960811034, -14.29746914071050412, 77.08224293864769550 ) ) ;
#94616=CARTESIAN_POINT ( 'NONE',  ( -16.51473224551069308, -9.474510206698971260, 86.66557627198102409 ) ) ;
#94618=CARTESIAN_POINT ( 'NONE',  ( 14.29746914071037800, 8.314922557961029526, 21.66775706135235069 ) ) ;
#94619=CARTESIAN_POINT ( 'NONE',  ( -0.05219959533909027116, -19.03943276465977164, 22.49890960531436690 ) ) ;
#94620=CARTESIAN_POINT ( 'NONE',  ( 19.05341960407611168, 5.049401038298154454, 93.95724293864769550 ) ) ;
#94621=CARTESIAN_POINT ( 'NONE',  ( 16.55341960407618274, -4.379528057220086978, 31.04275706135234714 ) ) ;
#94623=CARTESIAN_POINT ( 'NONE',  ( 16.46253265017146816, 9.564922557961045513, 31.66775706135232937 ) ) ;
#94624=CARTESIAN_POINT ( 'NONE',  ( -14.29746914071037622, -8.314922557961029526, 99.16775706135234714 ) ) ;
#94625=CARTESIAN_POINT ( 'NONE',  ( 16.51473224551083163, -9.474510206698727899, 105.8344237280190043 ) ) ;
#94626=CARTESIAN_POINT ( 'NONE',  ( 19.05341960407611168, 5.049401038298154454, 33.95724293864769550 ) ) ;
#94627=CARTESIAN_POINT ( 'NONE',  ( -4.379528057220086978, -16.55341960407618274, 79.79275706135236135 ) ) ;
#94628=CARTESIAN_POINT ( 'NONE',  ( -12.14591786802326823, 12.06949235617739902, 68.12609039468567573 ) ) ;
#94629=CARTESIAN_POINT ( 'NONE',  ( -9.474510206698964154, 16.51473224551069663, 30.41557627198102054 ) ) ;
#94630=CARTESIAN_POINT ( 'NONE',  ( 5.153800228976615827, -19.02544592524334988, 70.20942372801899012 ) ) ;
#94631=CARTESIAN_POINT ( 'NONE',  ( -5.823673210054431948, 21.52544592524334988, 107.7094237280190328 ) ) ;
#94632=CARTESIAN_POINT ( 'NONE',  ( 19.02544592524343514, -5.153800228976328945, 53.54057627198102409 ) ) ;
#94633=CARTESIAN_POINT ( 'NONE',  ( 5.049401038298161559, -19.05341960407611168, 92.70724293864769550 ) ) ;
#94634=CARTESIAN_POINT ( 'NONE',  ( -16.52544592524342804, 4.483927247898546575, 86.04057627198102409 ) ) ;
#94635=CARTESIAN_POINT ( 'NONE',  ( -16.46253265017146816, -9.564922557961047289, 59.16775706135233293 ) ) ;
#94636=CARTESIAN_POINT ( 'NONE',  ( 0.05219959533907565091, 21.53943276465977519, 49.99890960531437401 ) ) ;
#94637=CARTESIAN_POINT ( 'NONE',  ( 16.51473224551083163, -9.474510206698727899, 20.83442372801899722 ) ) ;
#94638=CARTESIAN_POINT ( 'NONE',  ( -13.97604488694527625, -13.89961937509977652, 96.87390960531433848 ) ) ;
#94639=CARTESIAN_POINT ( 'NONE',  ( -0.05219959533936034679, 19.03943276465977164, 27.50109039468566507 ) ) ;
#94640=CARTESIAN_POINT ( 'NONE',  ( 21.55341960407610458, 5.719274019375980345, 63.95724293864770260 ) ) ;
#94641=CARTESIAN_POINT ( 'NONE',  ( -13.97604488694527625, -13.89961937509977652, 106.8739096053143669 ) ) ;
#94642=CARTESIAN_POINT ( 'NONE',  ( -13.97604488694547697, 13.89961937509957934, 83.12609039468564731 ) ) ;
#94643=CARTESIAN_POINT ( 'NONE',  ( -13.89961937509977652, 13.97604488694528158, 115.6239096053143669 ) ) ;
#94645=CARTESIAN_POINT ( 'NONE',  ( 5.153800228976615827, -19.02544592524334988, 105.2094237280190185 ) ) ;
#94646=CARTESIAN_POINT ( 'NONE',  ( 4.379528057220339221, -16.55341960407611168, 112.7072429386476955 ) ) ;
#94647=CARTESIAN_POINT ( 'NONE',  ( -16.46253265017160317, 9.564922557960807481, 95.83224293864769550 ) ) ;
#94648=CARTESIAN_POINT ( 'NONE',  ( 15.80617190586746368, 15.72974639402197994, 79.37390960531436690 ) ) ;
#94649=CARTESIAN_POINT ( 'NONE',  ( -14.34966873604972548, 8.224510206698743886, 48.33442372801902565 ) ) ;
#94650=CARTESIAN_POINT ( 'NONE',  ( -21.52544592524334988, -5.823673210054445271, 48.95942372801902565 ) ) ;
#94651=CARTESIAN_POINT ( 'NONE',  ( -21.53943276465977519, -0.05219959533937600094, 98.75109039468568994 ) ) ;
#94652=CARTESIAN_POINT ( 'NONE',  ( 12.14591786802327356, -12.06949235617739191, 95.62609039468568994 ) ) ;
#94653=CARTESIAN_POINT ( 'NONE',  ( 9.564922557960805705, 16.46253265017160317, 84.58224293864769550 ) ) ;
#94654=CARTESIAN_POINT ( 'NONE',  ( 16.52544592524342804, -4.483927247898539470, 93.54057627198103830 ) ) ;
#94655=CARTESIAN_POINT ( 'NONE',  ( -16.55341960407611168, -4.379528057220339221, 31.45724293864769550 ) ) ;
#94656=CARTESIAN_POINT ( 'NONE',  ( -9.474510206698720793, -16.51473224551083518, 64.58442372801900433 ) ) ;
#94657=CARTESIAN_POINT ( 'NONE',  ( -5.719274019375665041, -21.55341960407619695, 59.79275706135234714 ) ) ;
#94658=CARTESIAN_POINT ( 'NONE',  ( 0.05219959533936267826, -19.03943276465977164, 20.00109039468567218 ) ) ;
#94660=CARTESIAN_POINT ( 'NONE',  ( -12.06949235617756955, 12.14591786802309770, 90.62390960531436690 ) ) ;
#94661=CARTESIAN_POINT ( 'NONE',  ( -21.55341960407610458, -5.719274019375992779, 31.45724293864769550 ) ) ;
#94662=CARTESIAN_POINT ( 'NONE',  ( 0.05219959533934541429, -16.53943276465976808, 110.0010903946856757 ) ) ;
#94663=CARTESIAN_POINT ( 'NONE',  ( 0.05219959533937995610, -21.53943276465977519, 80.00109039468568994 ) ) ;
#94664=CARTESIAN_POINT ( 'NONE',  ( -14.34966873604972548, 8.224510206698743886, 53.33442372801901854 ) ) ;
#94665=CARTESIAN_POINT ( 'NONE',  ( 12.14591786802327356, -12.06949235617739191, 110.6260903946857042 ) ) ;
#94666=CARTESIAN_POINT ( 'NONE',  ( -21.52544592524334988, -5.823673210054445271, 48.95942372801902565 ) ) ;
#94668=CARTESIAN_POINT ( 'NONE',  ( 5.719274019375673035, 21.55341960407619339, 32.29275706135235424 ) ) ;
#94669=CARTESIAN_POINT ( 'NONE',  ( 12.14591786802309770, 12.06949235617756955, 104.3739096053143669 ) ) ;
#94670=CARTESIAN_POINT ( 'NONE',  ( -5.153800228976328057, -19.02544592524343514, 22.29057627198102765 ) ) ;
#94671=CARTESIAN_POINT ( 'NONE',  ( -8.224510206698948167, 14.34966873604960824, 70.41557627198102409 ) ) ;
#94672=CARTESIAN_POINT ( 'NONE',  ( 19.02544592524343514, -5.153800228976328945, 78.54057627198099567 ) ) ;
#94673=CARTESIAN_POINT ( 'NONE',  ( -4.483927247898782831, 16.52544592524335698, 102.7094237280190185 ) ) ;
#94674=CARTESIAN_POINT ( 'NONE',  ( -15.72974639402197994, 15.80617190586746368, 60.62390960531437401 ) ) ;
#94675=CARTESIAN_POINT ( 'NONE',  ( -14.34966873604960291, -8.224510206698953496, 96.66557627198102409 ) ) ;
#94676=CARTESIAN_POINT ( 'NONE',  ( 21.53943276465977519, -0.05219959533907433946, 93.74890960531436690 ) ) ;
#94677=CARTESIAN_POINT ( 'NONE',  ( -19.02544592524342804, 5.153800228976336051, 96.04057627198103830 ) ) ;
#94678=CARTESIAN_POINT ( 'NONE',  ( 5.049401038298161559, -19.05341960407611168, 52.70724293864767418 ) ) ;
#94679=CARTESIAN_POINT ( 'NONE',  ( 0.05219959533936267826, -19.03943276465977164, 110.0010903946856757 ) ) ;
#94680=CARTESIAN_POINT ( 'NONE',  ( -21.52544592524343514, 5.823673210054127303, 46.04057627198103830 ) ) ;
#94681=CARTESIAN_POINT ( 'NONE',  ( -0.05219959533937732626, 21.53943276465977519, 62.50109039468568284 ) ) ;
#94682=CARTESIAN_POINT ( 'NONE',  ( 13.89961937509977652, -13.97604488694527269, 48.12390960531435979 ) ) ;
#94683=CARTESIAN_POINT ( 'NONE',  ( -19.05341960407611168, -5.049401038298163336, 81.45724293864769550 ) ) ;
#94684=CARTESIAN_POINT ( 'NONE',  ( -8.224510206698735004, -14.34966873604973081, 64.58442372801900433 ) ) ;
#94685=CARTESIAN_POINT ( 'NONE',  ( 21.55341960407619695, -5.719274019375665929, 41.04275706135236135 ) ) ;
#94687=CARTESIAN_POINT ( 'NONE',  ( -21.52544592524334988, -5.823673210054445271, 88.95942372801901854 ) ) ;
#94688=CARTESIAN_POINT ( 'NONE',  ( 5.823673210054125526, 21.52544592524343514, 99.79057627198103830 ) ) ;
#94689=CARTESIAN_POINT ( 'NONE',  ( -15.80617190586768217, 15.72974639402176855, 43.12609039468568284 ) ) ;
#94690=CARTESIAN_POINT ( 'NONE',  ( -14.29746914071037622, -8.314922557961029526, 59.16775706135234714 ) ) ;
#94691=CARTESIAN_POINT ( 'NONE',  ( 18.67979575497178502, 10.72451020669898547, 79.16557627198103830 ) ) ;
#94692=CARTESIAN_POINT ( 'NONE',  ( -0.05219959533936034679, 19.03943276465977164, 37.50109039468567573 ) ) ;
#94693=CARTESIAN_POINT ( 'NONE',  ( -13.89961937509977652, 13.97604488694528158, 65.62390960531436690 ) ) ;
#94694=CARTESIAN_POINT ( 'NONE',  ( -12.14591786802326823, 12.06949235617739902, 113.1260903946856899 ) ) ;
#94695=CARTESIAN_POINT ( 'NONE',  ( 17.49999999999999645, -5.500000000000031086, 83.29690382534172954 ) ) ;
#94696=CARTESIAN_POINT ( 'NONE',  ( 19.02544592524343514, -5.153800228976328945, 98.54057627198100988 ) ) ;
#94698=CARTESIAN_POINT ( 'NONE',  ( 19.02544592524334988, 5.153800228976608722, 86.45942372801900433 ) ) ;
#94699=CARTESIAN_POINT ( 'NONE',  ( -21.53943276465977519, 0.05219959533907696930, 56.24890960531436690 ) ) ;
#94700=CARTESIAN_POINT ( 'NONE',  ( -8.224510206698948167, 14.34966873604960824, 35.41557627198102409 ) ) ;
#94701=CARTESIAN_POINT ( 'NONE',  ( -14.29746914071037622, -8.314922557961029526, 19.16775706135234714 ) ) ;
#94702=CARTESIAN_POINT ( 'NONE',  ( -13.97604488694527625, -13.89961937509977652, 31.87390960531435979 ) ) ;
#94703=CARTESIAN_POINT ( 'NONE',  ( 16.46253265017146816, 9.564922557961045513, 111.6677570613523329 ) ) ;
#94704=CARTESIAN_POINT ( 'NONE',  ( -15.72974639402197994, 15.80617190586746368, 95.62390960531436690 ) ) ;
#94705=CARTESIAN_POINT ( 'NONE',  ( -0.05219959533936034679, 19.03943276465977164, 77.50109039468566152 ) ) ;
#94706=CARTESIAN_POINT ( 'NONE',  ( -14.34966873604972548, 8.224510206698743886, 78.33442372801901854 ) ) ;
#94707=CARTESIAN_POINT ( 'NONE',  ( -5.153800228976328057, -19.02544592524343514, 72.29057627198102409 ) ) ;
#94708=CARTESIAN_POINT ( 'NONE',  ( -14.29746914071049879, 8.314922557960819915, 80.83224293864769550 ) ) ;
#94709=CARTESIAN_POINT ( 'NONE',  ( 16.46253265017160672, -9.564922557960803928, 58.33224293864769550 ) ) ;
#94710=CARTESIAN_POINT ( 'NONE',  ( 12.14591786802309770, 12.06949235617756955, 69.37390960531436690 ) ) ;
#94711=FACE_OUTER_BOUND ( 'NONE', #142791, .T. ) ;
#94713=CARTESIAN_POINT ( 'NONE',  ( 16.53943276465976808, -0.05219959533910856209, 43.74890960531435979 ) ) ;
#94714=CARTESIAN_POINT ( 'NONE',  ( -19.02544592524342804, 5.153800228976336051, 71.04057627198099567 ) ) ;
#94716=CARTESIAN_POINT ( 'NONE',  ( 13.97604488694548053, -13.89961937509957401, 40.62609039468564731 ) ) ;
#94717=CARTESIAN_POINT ( 'NONE',  ( 16.52544592524335698, 4.483927247898782831, 41.45942372801901143 ) ) ;
#94718=CARTESIAN_POINT ( 'NONE',  ( -15.72974639402197994, 15.80617190586746368, 65.62390960531436690 ) ) ;
#94719=CARTESIAN_POINT ( 'NONE',  ( 5.049401038297881783, 19.05341960407617563, 22.29275706135233648 ) ) ;
#94720=CARTESIAN_POINT ( 'NONE',  ( 0.05219959533909260263, 19.03943276465977164, 79.99890960531436690 ) ) ;
#94722=CARTESIAN_POINT ( 'NONE',  ( 5.153800228976335163, 19.02544592524342804, 109.7905762719810099 ) ) ;
#94723=CARTESIAN_POINT ( 'NONE',  ( -0.05219959533937732626, 21.53943276465977519, 32.50109039468568284 ) ) ;
#94724=CARTESIAN_POINT ( 'NONE',  ( -12.14591786802309592, -12.06949235617757132, 101.8739096053143811 ) ) ;
#94725=CARTESIAN_POINT ( 'NONE',  ( 18.67979575497178502, 10.72451020669898547, 104.1655762719810241 ) ) ;
#94726=CARTESIAN_POINT ( 'NONE',  ( -19.03943276465977164, 0.05219959533909376836, 86.24890960531436690 ) ) ;
#94727=EDGE_LOOP ( 'NONE', ( #190854, #54285, #188000, #66105 ) ) ;
#94728=CARTESIAN_POINT ( 'NONE',  ( 15.72974639402176855, 15.80617190586768217, 26.87609039468567218 ) ) ;
#94729=ORIENTED_EDGE ( 'NONE', *, *, #194696, .F. ) ;
#94730=CARTESIAN_POINT ( 'NONE',  ( -19.05341960407611168, -5.049401038298163336, 81.45724293864769550 ) ) ;
#94732=CARTESIAN_POINT ( 'NONE',  ( -18.22780087662123094, -5.499999999999984901, 76.48459894673894155 ) ) ;
#94733=CARTESIAN_POINT ( 'NONE',  ( 0.05219959533907565091, 21.53943276465977519, 94.99890960531436690 ) ) ;
#94734=CARTESIAN_POINT ( 'NONE',  ( 19.02544592524343514, -5.153800228976328945, 28.54057627198102409 ) ) ;
#94735=CARTESIAN_POINT ( 'NONE',  ( 9.564922557961047289, -16.46253265017146816, 100.4177570613523329 ) ) ;
#94737=CARTESIAN_POINT ( 'NONE',  ( 19.03943276465977164, -0.05219959533909143690, 33.74890960531435979 ) ) ;
#94738=CARTESIAN_POINT ( 'NONE',  ( -0.05219959533937732626, 21.53943276465977519, 87.50109039468568994 ) ) ;
#94739=CARTESIAN_POINT ( 'NONE',  ( -19.05341960407611168, -5.049401038298163336, 76.45724293864769550 ) ) ;
#94740=CARTESIAN_POINT ( 'NONE',  ( -15.72974639402176322, -15.80617190586768395, 44.37609039468567573 ) ) ;
#94741=CARTESIAN_POINT ( 'NONE',  ( 5.823673210054444382, -21.52544592524334988, 20.20942372801900788 ) ) ;
#94743=CARTESIAN_POINT ( 'NONE',  ( 5.153800228976335163, 19.02544592524342804, 89.79057627198102409 ) ) ;
#94745=CARTESIAN_POINT ( 'NONE',  ( 12.06949235617739724, 12.14591786802326823, 41.87609039468568284 ) ) ;
#94746=CARTESIAN_POINT ( 'NONE',  ( -0.05219959533907301413, -21.53943276465977519, 42.49890960531435979 ) ) ;
#94747=CARTESIAN_POINT ( 'NONE',  ( 21.55341960407619695, -5.719274019375665929, 51.04275706135234714 ) ) ;
#94748=CARTESIAN_POINT ( 'NONE',  ( -21.53943276465977519, -0.05219959533937600094, 78.75109039468568994 ) ) ;
#94750=CARTESIAN_POINT ( 'NONE',  ( 14.34966873604972726, -8.224510206698740333, 20.83442372801901143 ) ) ;
#94751=CARTESIAN_POINT ( 'NONE',  ( -9.474510206698964154, 16.51473224551069663, 60.41557627198102409 ) ) ;
#94752=CARTESIAN_POINT ( 'NONE',  ( 13.97604488694527802, 13.89961937509977652, 79.37390960531435269 ) ) ;
#94753=CARTESIAN_POINT ( 'NONE',  ( 16.55341960407611168, 4.379528057220329451, 108.9572429386476955 ) ) ;
#94754=CARTESIAN_POINT ( 'NONE',  ( 12.14591786802309770, 12.06949235617756955, 109.3739096053143811 ) ) ;
#94755=CARTESIAN_POINT ( 'NONE',  ( 13.97604488694527802, 13.89961937509977652, 109.3739096053143669 ) ) ;
#94756=CARTESIAN_POINT ( 'NONE',  ( -16.53943276465976808, -0.05219959533934237506, 78.75109039468568994 ) ) ;
#94757=CARTESIAN_POINT ( 'NONE',  ( 12.06949235617757843, -12.14591786802309237, 68.12390960531436690 ) ) ;
#94758=CARTESIAN_POINT ( 'NONE',  ( 19.02544592524343514, -5.153800228976328945, 48.54057627198103120 ) ) ;
#94759=CARTESIAN_POINT ( 'NONE',  ( -10.81492255796105439, 18.62759615963255655, 82.91775706135234714 ) ) ;
#94760=CARTESIAN_POINT ( 'NONE',  ( -10.72451020669870658, -18.67979575497194134, 69.58442372801900433 ) ) ;
#94761=CARTESIAN_POINT ( 'NONE',  ( -5.153800228976607833, 19.02544592524334988, 107.7094237280189759 ) ) ;
#94762=CARTESIAN_POINT ( 'NONE',  ( 12.14591786802309770, 12.06949235617756955, 64.37390960531435269 ) ) ;
#94763=CARTESIAN_POINT ( 'NONE',  ( 15.80617190586746368, 15.72974639402197994, 109.3739096053143811 ) ) ;
#94764=CARTESIAN_POINT ( 'NONE',  ( -15.80617190586745835, -15.72974639402198527, 56.87390960531436690 ) ) ;
#94765=CARTESIAN_POINT ( 'NONE',  ( -17.48847506799970120, -5.747544572773739979, 104.1730256215672341 ) ) ;
#94767=CARTESIAN_POINT ( 'NONE',  ( -19.02544592524342804, 5.153800228976336051, 66.04057627198103830 ) ) ;
#94768=CARTESIAN_POINT ( 'NONE',  ( 12.06949235617757843, -12.14591786802309237, 33.12390960531435979 ) ) ;
#94769=CARTESIAN_POINT ( 'NONE',  ( 0.05219959533910956823, 16.53943276465976808, 24.99890960531435624 ) ) ;
#94770=CARTESIAN_POINT ( 'NONE',  ( 16.52544592524335698, 4.483927247898782831, 101.4594237280190185 ) ) ;
#94771=CARTESIAN_POINT ( 'NONE',  ( -19.02544592524334988, -5.153800228976617603, 58.95942372801900433 ) ) ;
#94773=CARTESIAN_POINT ( 'NONE',  ( 17.49999999999999289, 5.500000000000006217, 48.78230962303565121 ) ) ;
#94774=CARTESIAN_POINT ( 'NONE',  ( -19.05341960407611168, -5.049401038298163336, 101.4572429386476955 ) ) ;
#94775=CARTESIAN_POINT ( 'NONE',  ( 12.06949235617757843, -12.14591786802309237, 63.12390960531435979 ) ) ;
#94776=CARTESIAN_POINT ( 'NONE',  ( -5.153800228976328057, -19.02544592524343514, 22.29057627198102765 ) ) ;
#94777=CARTESIAN_POINT ( 'NONE',  ( -9.564922557960796823, -16.46253265017161027, 112.0822429386476955 ) ) ;
#94778=CARTESIAN_POINT ( 'NONE',  ( -5.719274019375978568, 21.55341960407610458, 55.20724293864770260 ) ) ;
#94779=VERTEX_POINT ( 'NONE', #125519 ) ;
#94780=CARTESIAN_POINT ( 'NONE',  ( -12.14591786802309592, -12.06949235617757132, 96.87390960531436690 ) ) ;
#94781=CARTESIAN_POINT ( 'NONE',  ( 14.34966873604972726, -8.224510206698740333, 45.83442372801901854 ) ) ;
#94782=CARTESIAN_POINT ( 'NONE',  ( -12.14591786802309592, -12.06949235617757132, 86.87390960531438111 ) ) ;
#94784=CARTESIAN_POINT ( 'NONE',  ( 16.46253265017146816, 9.564922557961045513, 81.66775706135233293 ) ) ;
#94785=CARTESIAN_POINT ( 'NONE',  ( 16.46253265017160672, -9.564922557960803928, 113.3322429386476955 ) ) ;
#94787=CARTESIAN_POINT ( 'NONE',  ( -18.22780087662121673, -5.500000000000062172, 41.48459894673893444 ) ) ;
#94789=CARTESIAN_POINT ( 'NONE',  ( 12.14591786802327356, -12.06949235617739191, 40.62609039468567573 ) ) ;
#94790=CARTESIAN_POINT ( 'NONE',  ( -0.05219959533910754901, -16.53943276465976808, 32.49890960531435979 ) ) ;
#94791=CARTESIAN_POINT ( 'NONE',  ( -18.67979575497178146, -10.72451020669898902, 56.66557627198103830 ) ) ;
#94793=CARTESIAN_POINT ( 'NONE',  ( 5.153800228976615827, -19.02544592524334988, 85.20942372801900433 ) ) ;
#94794=CARTESIAN_POINT ( 'NONE',  ( 0.05219959533907565091, 21.53943276465977519, 44.99890960531435979 ) ) ;
#94795=CARTESIAN_POINT ( 'NONE',  ( 10.72451020669871369, 18.67979575497193778, 87.08442372801901854 ) ) ;
#94797=CARTESIAN_POINT ( 'NONE',  ( 16.52544592524335698, 4.483927247898782831, 41.45942372801901143 ) ) ;
#94798=CARTESIAN_POINT ( 'NONE',  ( 9.564922557960805705, 16.46253265017160317, 39.58224293864768839 ) ) ;
#94799=CARTESIAN_POINT ( 'NONE',  ( -13.89961937509977652, 13.97604488694528158, 100.6239096053143669 ) ) ;
#94800=CARTESIAN_POINT ( 'NONE',  ( -19.03943276465977164, 0.05219959533909376836, 31.24890960531435979 ) ) ;
#94801=CARTESIAN_POINT ( 'NONE',  ( 0.05219959533910956823, 16.53943276465976808, 94.99890960531436690 ) ) ;
#94803=CARTESIAN_POINT ( 'NONE',  ( -19.05341960407611168, -5.049401038298163336, 106.4572429386476955 ) ) ;
#94805=CARTESIAN_POINT ( 'NONE',  ( 14.29746914071037800, 8.314922557961029526, 56.66775706135235424 ) ) ;
#94806=CARTESIAN_POINT ( 'NONE',  ( -0.05219959533907301413, -21.53943276465977519, 92.49890960531436690 ) ) ;
#94807=CARTESIAN_POINT ( 'NONE',  ( 19.03943276465977164, -0.05219959533909143690, 43.74890960531435979 ) ) ;
#94808=CARTESIAN_POINT ( 'NONE',  ( 21.53943276465977519, 0.05219959533937863772, 21.25109039468567218 ) ) ;
#94809=CARTESIAN_POINT ( 'NONE',  ( 13.89961937509977652, -13.97604488694527269, 88.12390960531438111 ) ) ;
#94811=EDGE_CURVE ( 'NONE', #20950, #129974, #62835, .T. ) ;
#94813=CARTESIAN_POINT ( 'NONE',  ( 16.55341960407618274, -4.379528057220086978, 51.04275706135234714 ) ) ;
#94814=CARTESIAN_POINT ( 'NONE',  ( -15.80617190586745835, -15.72974639402198527, 111.8739096053143669 ) ) ;
#94815=CARTESIAN_POINT ( 'NONE',  ( 8.224510206698953496, -14.34966873604960469, 107.9155762719810241 ) ) ;
#94816=CARTESIAN_POINT ( 'NONE',  ( -13.97604488694527625, -13.89961937509977652, 96.87390960531433848 ) ) ;
#94817=CARTESIAN_POINT ( 'NONE',  ( 19.02544592524334988, 5.153800228976608722, 81.45942372801897591 ) ) ;
#94818=CARTESIAN_POINT ( 'NONE',  ( -5.153800228976607833, 19.02544592524334988, 22.70942372801899012 ) ) ;
#94819=CARTESIAN_POINT ( 'NONE',  ( 0.05219959533907565091, 21.53943276465977519, 89.99890960531438111 ) ) ;
#94820=CARTESIAN_POINT ( 'NONE',  ( 16.51473224551083163, -9.474510206698727899, 30.83442372801900433 ) ) ;
#94821=CARTESIAN_POINT ( 'NONE',  ( -14.29746914071037622, -8.314922557961029526, 79.16775706135234714 ) ) ;
#94822=CARTESIAN_POINT ( 'NONE',  ( 19.02544592524343514, -5.153800228976328945, 103.5405762719809957 ) ) ;
#94824=CARTESIAN_POINT ( 'NONE',  ( -19.05341960407611168, -5.049401038298163336, 56.45724293864768129 ) ) ;
#94825=CARTESIAN_POINT ( 'NONE',  ( -5.823673210054431948, 21.52544592524334988, 72.70942372801901854 ) ) ;
#94826=CARTESIAN_POINT ( 'NONE',  ( -21.52544592524334988, -5.823673210054445271, 63.95942372801901854 ) ) ;
#94827=CARTESIAN_POINT ( 'NONE',  ( 9.564922557960805705, 16.46253265017160317, 74.58224293864769550 ) ) ;
#94828=CARTESIAN_POINT ( 'NONE',  ( -21.52544592524334988, -5.823673210054445271, 43.95942372801902565 ) ) ;
#94829=CARTESIAN_POINT ( 'NONE',  ( -16.51473224551082808, 9.474510206698731452, 93.33442372801900433 ) ) ;
#94830=CARTESIAN_POINT ( 'NONE',  ( -5.049401038298153566, 19.05341960407611168, 50.20724293864770260 ) ) ;
#94831=CARTESIAN_POINT ( 'NONE',  ( -19.02544592524342804, 5.153800228976336051, 96.04057627198103830 ) ) ;
#94832=CARTESIAN_POINT ( 'NONE',  ( -9.474510206698964154, 16.51473224551069663, 65.41557627198102409 ) ) ;
#94833=CARTESIAN_POINT ( 'NONE',  ( 17.50000000000000000, -5.500000000000000888, 113.2969038253417153 ) ) ;
#94834=CARTESIAN_POINT ( 'NONE',  ( -19.02544592524342804, 5.153800228976336051, 51.04057627198103120 ) ) ;
#94835=CARTESIAN_POINT ( 'NONE',  ( -21.52544592524343514, 5.823673210054127303, 96.04057627198102409 ) ) ;
#94836=CARTESIAN_POINT ( 'NONE',  ( -16.52544592524335698, -4.483927247898792601, 73.95942372801901854 ) ) ;
#94838=CARTESIAN_POINT ( 'NONE',  ( 5.153800228976615827, -19.02544592524334988, 30.20942372801900433 ) ) ;
#94839=CARTESIAN_POINT ( 'NONE',  ( 16.51473224551069308, 9.474510206698969483, 69.16557627198102409 ) ) ;
#94840=CARTESIAN_POINT ( 'NONE',  ( 16.52544592524342804, -4.483927247898539470, 58.54057627198103120 ) ) ;
#94841=CARTESIAN_POINT ( 'NONE',  ( -4.379528057220328563, 16.55341960407611168, 95.20724293864769550 ) ) ;
#94842=CARTESIAN_POINT ( 'NONE',  ( 13.89961937509977652, -13.97604488694527269, 103.1239096053143527 ) ) ;
#94843=CARTESIAN_POINT ( 'NONE',  ( -5.049401038298153566, 19.05341960407611168, 95.20724293864770971 ) ) ;
#94844=CARTESIAN_POINT ( 'NONE',  ( 10.81492255796106328, -18.62759615963255655, 45.41775706135234003 ) ) ;
#94845=CARTESIAN_POINT ( 'NONE',  ( -16.51473224551069308, -9.474510206698971260, 111.6655762719810383 ) ) ;
#94846=CARTESIAN_POINT ( 'NONE',  ( -21.53943276465977519, -0.05219959533937600094, 113.7510903946856757 ) ) ;
#94847=CARTESIAN_POINT ( 'NONE',  ( 14.29746914071037800, 8.314922557961029526, 76.66775706135234714 ) ) ;
#94848=CARTESIAN_POINT ( 'NONE',  ( 10.81492255796106328, -18.62759615963255655, 35.41775706135234003 ) ) ;
#94849=CARTESIAN_POINT ( 'NONE',  ( -18.62759615963270932, 10.81492255796079327, 25.83224293864769194 ) ) ;
#94850=CARTESIAN_POINT ( 'NONE',  ( -21.52544592524343514, 5.823673210054127303, 106.0405762719810525 ) ) ;
#94851=CARTESIAN_POINT ( 'NONE',  ( -12.14591786802309592, -12.06949235617757132, 56.87390960531436690 ) ) ;
#94852=CARTESIAN_POINT ( 'NONE',  ( -13.89961937509977652, 13.97604488694528158, 50.62390960531435979 ) ) ;
#94853=CARTESIAN_POINT ( 'NONE',  ( 12.06949235617757843, -12.14591786802309237, 78.12390960531436690 ) ) ;
#94854=CARTESIAN_POINT ( 'NONE',  ( 21.52544592524344225, -5.823673210054117533, 48.54057627198103120 ) ) ;
#94855=CARTESIAN_POINT ( 'NONE',  ( -19.05341960407617563, 5.049401038297882671, 48.54275706135233293 ) ) ;
#94856=CARTESIAN_POINT ( 'NONE',  ( 19.05341960407611168, 5.049401038298154454, 23.95724293864769194 ) ) ;
#94858=CARTESIAN_POINT ( 'NONE',  ( -16.52544592524335698, -4.483927247898792601, 68.95942372801901854 ) ) ;
#94859=CARTESIAN_POINT ( 'NONE',  ( -5.049401038298153566, 19.05341960407611168, 65.20724293864765286 ) ) ;
#94861=CARTESIAN_POINT ( 'NONE',  ( 12.14591786802309770, 12.06949235617756955, 84.37390960531438111 ) ) ;
#94862=CARTESIAN_POINT ( 'NONE',  ( 10.72451020669898902, -18.67979575497178502, 32.91557627198102409 ) ) ;
#94864=CARTESIAN_POINT ( 'NONE',  ( 14.34966873604972726, -8.224510206698740333, 110.8344237280190043 ) ) ;
#94865=CARTESIAN_POINT ( 'NONE',  ( -9.474510206698720793, -16.51473224551083518, 104.5844237280190043 ) ) ;
#94866=CARTESIAN_POINT ( 'NONE',  ( 15.72974639402176855, 15.80617190586768217, 96.87609039468568994 ) ) ;
#94867=CARTESIAN_POINT ( 'NONE',  ( 5.049401038298161559, -19.05341960407611168, 82.70724293864770971 ) ) ;
#94868=CARTESIAN_POINT ( 'NONE',  ( -0.05219959533907301413, -21.53943276465977519, 102.4989096053143811 ) ) ;
#94869=CARTESIAN_POINT ( 'NONE',  ( -4.483927247898782831, 16.52544592524335698, 57.70942372801901143 ) ) ;
#94870=CARTESIAN_POINT ( 'NONE',  ( 19.03943276465977164, -0.05219959533909143690, 33.74890960531435979 ) ) ;
#94871=CARTESIAN_POINT ( 'NONE',  ( -12.14591786802326823, 12.06949235617739902, 28.12609039468568284 ) ) ;
#94872=CARTESIAN_POINT ( 'NONE',  ( -19.03943276465977164, -0.05219959533935918106, 88.75109039468567573 ) ) ;
#94874=CARTESIAN_POINT ( 'NONE',  ( 0.05219959533907565091, 21.53943276465977519, 89.99890960531438111 ) ) ;
#94875=CARTESIAN_POINT ( 'NONE',  ( -16.51473224551082808, 9.474510206698731452, 73.33442372801900433 ) ) ;
#94876=CARTESIAN_POINT ( 'NONE',  ( 19.02130022317637525, -5.499999999999793943, 88.28188669246574705 ) ) ;
#94877=CARTESIAN_POINT ( 'NONE',  ( -10.81492255796078084, -18.62759615963271287, 102.0822429386476955 ) ) ;
#94879=CARTESIAN_POINT ( 'NONE',  ( 5.153800228976335163, 19.02544592524342804, 79.79057627198102409 ) ) ;
#94880=CARTESIAN_POINT ( 'NONE',  ( -8.314922557961024197, 14.29746914071037800, 37.91775706135235424 ) ) ;
#94882=CARTESIAN_POINT ( 'NONE',  ( 13.89961937509957401, 13.97604488694547697, 56.87609039468564731 ) ) ;
#94883=CARTESIAN_POINT ( 'NONE',  ( -21.52544592524334988, -5.823673210054445271, 18.95942372801901143 ) ) ;
#94884=CARTESIAN_POINT ( 'NONE',  ( 16.52544592524342804, -4.483927247898539470, 58.54057627198103120 ) ) ;
#94885=CARTESIAN_POINT ( 'NONE',  ( -16.46253265017160317, 9.564922557960807481, 80.83224293864769550 ) ) ;
#94886=CARTESIAN_POINT ( 'NONE',  ( 4.379528057220092307, 16.55341960407617563, 32.29275706135235424 ) ) ;
#94887=CARTESIAN_POINT ( 'NONE',  ( 16.51473224551083163, -9.474510206698727899, 40.83442372801900433 ) ) ;
#94888=CARTESIAN_POINT ( 'NONE',  ( -0.05219959533937732626, 21.53943276465977519, 47.50109039468568994 ) ) ;
#94889=CARTESIAN_POINT ( 'NONE',  ( -12.06949235617739369, -12.14591786802326823, 19.37609039468568639 ) ) ;
#94890=CARTESIAN_POINT ( 'NONE',  ( -9.474510206698964154, 16.51473224551069663, 55.41557627198103120 ) ) ;
#94891=CARTESIAN_POINT ( 'NONE',  ( 19.05341960407617918, -5.049401038297876454, 81.04275706135231871 ) ) ;
#94892=CARTESIAN_POINT ( 'NONE',  ( -18.62759615963255300, -10.81492255796106328, 94.16775706135237556 ) ) ;
#94893=CARTESIAN_POINT ( 'NONE',  ( -19.05341960407617563, 5.049401038297882671, 68.54275706135230450 ) ) ;
#94894=CARTESIAN_POINT ( 'NONE',  ( -5.153800228976328057, -19.02544592524343514, 37.29057627198102409 ) ) ;
#94895=CARTESIAN_POINT ( 'NONE',  ( -10.72451020669898014, 18.67979575497178502, 70.41557627198102409 ) ) ;
#94896=CARTESIAN_POINT ( 'NONE',  ( -14.34966873604960291, -8.224510206698953496, 61.66557627198103120 ) ) ;
#94897=CARTESIAN_POINT ( 'NONE',  ( -9.564922557961040184, 16.46253265017147172, 67.91775706135233293 ) ) ;
#94899=CARTESIAN_POINT ( 'NONE',  ( -19.02544592524334988, -5.153800228976617603, 48.95942372801900433 ) ) ;
#94900=CARTESIAN_POINT ( 'NONE',  ( -8.314922557961024197, 14.29746914071037800, 92.91775706135236135 ) ) ;
#94901=CARTESIAN_POINT ( 'NONE',  ( 8.224510206698953496, -14.34966873604960469, 57.91557627198103120 ) ) ;
#94902=CARTESIAN_POINT ( 'NONE',  ( -21.52544592524334988, -5.823673210054445271, 83.95942372801900433 ) ) ;
#94904=CARTESIAN_POINT ( 'NONE',  ( 5.823673210054125526, 21.52544592524343514, 94.79057627198105251 ) ) ;
#94905=CARTESIAN_POINT ( 'NONE',  ( -5.049401038298153566, 19.05341960407611168, 50.20724293864770260 ) ) ;
#94906=CARTESIAN_POINT ( 'NONE',  ( 21.55341960407619695, -5.719274019375665929, 66.04275706135236135 ) ) ;
#94907=CARTESIAN_POINT ( 'NONE',  ( -0.05219959533909027116, -19.03943276465977164, 47.49890960531435979 ) ) ;
#94908=CARTESIAN_POINT ( 'NONE',  ( 13.97604488694527802, 13.89961937509977652, 59.37390960531434558 ) ) ;
#94909=CARTESIAN_POINT ( 'NONE',  ( -14.34966873604960291, -8.224510206698953496, 101.6655762719810383 ) ) ;
#94910=CARTESIAN_POINT ( 'NONE',  ( -18.67979575497178146, -10.72451020669898902, 21.66557627198102409 ) ) ;
#94911=CARTESIAN_POINT ( 'NONE',  ( 16.55341960407611168, 4.379528057220329451, 53.95724293864770260 ) ) ;
#94912=CARTESIAN_POINT ( 'NONE',  ( -19.05341960407611168, -5.049401038298163336, 36.45724293864766707 ) ) ;
#94913=CARTESIAN_POINT ( 'NONE',  ( 16.53943276465976808, -0.05219959533910856209, 78.74890960531436690 ) ) ;
#94914=CARTESIAN_POINT ( 'NONE',  ( 0.05219959533907565091, 21.53943276465977519, 99.99890960531436690 ) ) ;
#94915=CARTESIAN_POINT ( 'NONE',  ( -10.72451020669870658, -18.67979575497194134, 29.58442372801901854 ) ) ;
#94916=CARTESIAN_POINT ( 'NONE',  ( 9.474510206698971260, -16.51473224551069308, 22.91557627198102765 ) ) ;
#94917=CARTESIAN_POINT ( 'NONE',  ( -12.06949235617739369, -12.14591786802326823, 44.37609039468567573 ) ) ;
#94918=CARTESIAN_POINT ( 'NONE',  ( 15.80617190586746368, 15.72974639402197994, 79.37390960531436690 ) ) ;
#94920=CARTESIAN_POINT ( 'NONE',  ( 5.719274019375673035, 21.55341960407619339, 107.2927570613523471 ) ) ;
#94921=CARTESIAN_POINT ( 'NONE',  ( -0.05219959533909027116, -19.03943276465977164, 112.4989096053143669 ) ) ;
#94922=CARTESIAN_POINT ( 'NONE',  ( 18.62759615963255655, 10.81492255796105972, 41.66775706135235424 ) ) ;
#94923=CARTESIAN_POINT ( 'NONE',  ( -15.72974639402197994, 15.80617190586746368, 45.62390960531436690 ) ) ;
#94924=CARTESIAN_POINT ( 'NONE',  ( 4.379528057220092307, 16.55341960407617563, 107.2927570613523471 ) ) ;
#94925=CARTESIAN_POINT ( 'NONE',  ( -5.823673210054431948, 21.52544592524334988, 57.70942372801901143 ) ) ;
#94926=CARTESIAN_POINT ( 'NONE',  ( 5.823673210054444382, -21.52544592524334988, 85.20942372801901854 ) ) ;
#94927=CARTESIAN_POINT ( 'NONE',  ( 19.02544592524334988, 5.153800228976608722, 31.45942372801900433 ) ) ;
#94928=CARTESIAN_POINT ( 'NONE',  ( -16.52544592524335698, -4.483927247898792601, 93.95942372801903275 ) ) ;
#94929=CARTESIAN_POINT ( 'NONE',  ( -21.52544592524334988, -5.823673210054445271, 38.95942372801901854 ) ) ;
#94930=CARTESIAN_POINT ( 'NONE',  ( -9.474510206698964154, 16.51473224551069663, 45.41557627198103120 ) ) ;
#94931=CARTESIAN_POINT ( 'NONE',  ( -0.05219959533936034679, 19.03943276465977164, 22.50109039468566152 ) ) ;
#94932=CARTESIAN_POINT ( 'NONE',  ( 15.72974639402199770, -15.80617190586745480, 28.12390960531435979 ) ) ;
#94933=CARTESIAN_POINT ( 'NONE',  ( 21.53943276465977519, 0.05219959533937863772, 21.25109039468567218 ) ) ;
#94934=CARTESIAN_POINT ( 'NONE',  ( -0.05219959533907301413, -21.53943276465977519, 77.49890960531433848 ) ) ;
#94935=CARTESIAN_POINT ( 'NONE',  ( -17.49999999999998579, 5.500000000000032863, 60.79690382534172244 ) ) ;
#94936=CARTESIAN_POINT ( 'NONE',  ( -10.72451020669898014, 18.67979575497178502, 60.41557627198102409 ) ) ;
#94937=CARTESIAN_POINT ( 'NONE',  ( -12.14591786802326823, 12.06949235617739902, 63.12609039468568994 ) ) ;
#94938=CARTESIAN_POINT ( 'NONE',  ( 12.14591786802309770, 12.06949235617756955, 64.37390960531435269 ) ) ;
#94940=CARTESIAN_POINT ( 'NONE',  ( 19.05341960407617918, -5.049401038297876454, 91.04275706135234714 ) ) ;
#94943=CARTESIAN_POINT ( 'NONE',  ( -12.14591786802326823, 12.06949235617739902, 33.12609039468569705 ) ) ;
#94944=CARTESIAN_POINT ( 'NONE',  ( -5.719274019375978568, 21.55341960407610458, 95.20724293864769550 ) ) ;
#94945=CARTESIAN_POINT ( 'NONE',  ( 21.53943276465977519, -0.05219959533907433946, 78.74890960531436690 ) ) ;
#94946=CARTESIAN_POINT ( 'NONE',  ( 21.55341960407610458, 5.719274019375980345, 23.95724293864769550 ) ) ;
#94947=CARTESIAN_POINT ( 'NONE',  ( -12.14591786802326823, 12.06949235617739902, 53.12609039468568284 ) ) ;
#94948=CARTESIAN_POINT ( 'NONE',  ( -19.02544592524342804, 5.153800228976336051, 66.04057627198103830 ) ) ;
#94949=CARTESIAN_POINT ( 'NONE',  ( 21.53943276465977519, 0.05219959533937863772, 46.25109039468567573 ) ) ;
#94950=CARTESIAN_POINT ( 'NONE',  ( -4.483927247898782831, 16.52544592524335698, 22.70942372801901499 ) ) ;
#94951=CARTESIAN_POINT ( 'NONE',  ( 19.05341960407611168, 5.049401038298154454, 113.9572429386477097 ) ) ;
#94952=CARTESIAN_POINT ( 'NONE',  ( 19.03943276465977164, 0.05219959533936151252, 21.25109039468565797 ) ) ;
#94953=CARTESIAN_POINT ( 'NONE',  ( -19.05341960407611168, -5.049401038298163336, 101.4572429386476955 ) ) ;
#94954=CARTESIAN_POINT ( 'NONE',  ( -21.55341960407610458, -5.719274019375992779, 106.4572429386477097 ) ) ;
#94955=CARTESIAN_POINT ( 'NONE',  ( 0.05219959533909260263, 19.03943276465977164, 64.99890960531436690 ) ) ;
#94957=CARTESIAN_POINT ( 'NONE',  ( 16.52544592524342804, -4.483927247898539470, 88.54057627198103830 ) ) ;
#94958=CARTESIAN_POINT ( 'NONE',  ( 13.89961937509977652, -13.97604488694527269, 113.1239096053143527 ) ) ;
#94959=CARTESIAN_POINT ( 'NONE',  ( -0.05219959533909027116, -19.03943276465977164, 22.49890960531436690 ) ) ;
#94960=CARTESIAN_POINT ( 'NONE',  ( 21.52544592524344225, -5.823673210054117533, 103.5405762719810383 ) ) ;
#94961=CARTESIAN_POINT ( 'NONE',  ( 0.05219959533936267826, -19.03943276465977164, 65.00109039468567573 ) ) ;
#94962=CARTESIAN_POINT ( 'NONE',  ( 5.153800228976335163, 19.02544592524342804, 109.7905762719810099 ) ) ;
#94963=CARTESIAN_POINT ( 'NONE',  ( 19.02544592524343514, -5.153800228976328945, 28.54057627198102409 ) ) ;
#94964=CARTESIAN_POINT ( 'NONE',  ( -5.719274019375978568, 21.55341960407610458, 55.20724293864770260 ) ) ;
#94966=CARTESIAN_POINT ( 'NONE',  ( -5.049401038298153566, 19.05341960407611168, 100.2072429386476955 ) ) ;
#94967=CARTESIAN_POINT ( 'NONE',  ( -18.67979575497193778, 10.72451020669871902, 73.33442372801901854 ) ) ;
#94968=CARTESIAN_POINT ( 'NONE',  ( -13.89961937509977652, 13.97604488694528158, 45.62390960531433848 ) ) ;
#94969=CARTESIAN_POINT ( 'NONE',  ( 14.29746914071049879, -8.314922557960816363, 93.33224293864769550 ) ) ;
#94970=CARTESIAN_POINT ( 'NONE',  ( 8.224510206698742110, 14.34966873604972548, 37.08442372801901143 ) ) ;
#94971=CARTESIAN_POINT ( 'NONE',  ( -5.823673210054431948, 21.52544592524334988, 62.70942372801902565 ) ) ;
#94973=CARTESIAN_POINT ( 'NONE',  ( -16.51473224551082808, 9.474510206698731452, 28.33442372801900433 ) ) ;
#94974=CARTESIAN_POINT ( 'NONE',  ( -16.51473224551082808, 9.474510206698731452, 73.33442372801900433 ) ) ;
#94975=CARTESIAN_POINT ( 'NONE',  ( -19.02544592524334988, -5.153800228976617603, 38.95942372801900433 ) ) ;
#94977=CARTESIAN_POINT ( 'NONE',  ( -21.53943276465977519, -0.05219959533937600094, 38.75109039468567573 ) ) ;
#94978=CARTESIAN_POINT ( 'NONE',  ( -19.01529144963332385, -5.500000000000167866, 46.23431955728440101 ) ) ;
#94979=CARTESIAN_POINT ( 'NONE',  ( -16.51473224551082808, 9.474510206698731452, 38.33442372801899722 ) ) ;
#94980=CARTESIAN_POINT ( 'NONE',  ( 5.049401038298161559, -19.05341960407611168, 62.70724293864769550 ) ) ;
#94981=CARTESIAN_POINT ( 'NONE',  ( -4.483927247898539470, -16.52544592524342804, 22.29057627198102765 ) ) ;
#94982=CARTESIAN_POINT ( 'NONE',  ( 10.81492255796078972, 18.62759615963270932, 24.58224293864768839 ) ) ;
#94983=CARTESIAN_POINT ( 'NONE',  ( -18.62759615963255300, -10.81492255796106328, 84.16775706135234714 ) ) ;
#94986=CARTESIAN_POINT ( 'NONE',  ( -0.05219959533937732626, 21.53943276465977519, 82.50109039468568994 ) ) ;
#94987=CARTESIAN_POINT ( 'NONE',  ( 16.79531203550645557, -7.028104445595743321, 41.24755011779557634 ) ) ;
#94988=CARTESIAN_POINT ( 'NONE',  ( -16.46253265017160317, 9.564922557960807481, 105.8322429386476955 ) ) ;
#94990=CARTESIAN_POINT ( 'NONE',  ( -13.89961937509977652, 13.97604488694528158, 50.62390960531435979 ) ) ;
#94991=CARTESIAN_POINT ( 'NONE',  ( 10.81492255796078972, 18.62759615963270932, 59.58224293864770260 ) ) ;
#94992=CARTESIAN_POINT ( 'NONE',  ( -8.314922557961024197, 14.29746914071037800, 112.9177570613523329 ) ) ;
#94993=CARTESIAN_POINT ( 'NONE',  ( 12.14591786802309770, 12.06949235617756955, 114.3739096053143527 ) ) ;
#94994=CARTESIAN_POINT ( 'NONE',  ( 16.46253265017160672, -9.564922557960803928, 93.33224293864769550 ) ) ;
#94995=CARTESIAN_POINT ( 'NONE',  ( -19.05341960407617563, 5.049401038297882671, 28.54275706135232937 ) ) ;
#94996=CARTESIAN_POINT ( 'NONE',  ( 12.14591786802309770, 12.06949235617756955, 99.37390960531436690 ) ) ;
#94997=CARTESIAN_POINT ( 'NONE',  ( -0.05219959533937732626, 21.53943276465977519, 72.50109039468568994 ) ) ;
#94998=CARTESIAN_POINT ( 'NONE',  ( -19.02544592524342804, 5.153800228976336051, 116.0405762719810383 ) ) ;
#94999=CARTESIAN_POINT ( 'NONE',  ( 14.34966873604972726, -8.224510206698740333, 110.8344237280190043 ) ) ;
#95000=CARTESIAN_POINT ( 'NONE',  ( -5.049401038297874678, -19.05341960407617918, 69.79275706135233293 ) ) ;
#95001=CARTESIAN_POINT ( 'NONE',  ( -16.46253265017160317, 9.564922557960807481, 115.8322429386477097 ) ) ;
#95002=CARTESIAN_POINT ( 'NONE',  ( 16.55341960407611168, 4.379528057220329451, 78.95724293864769550 ) ) ;
#95003=CARTESIAN_POINT ( 'NONE',  ( -5.153800228976607833, 19.02544592524334988, 52.70942372801900433 ) ) ;
#95004=CARTESIAN_POINT ( 'NONE',  ( 13.97604488694527802, 13.89961937509977652, 69.37390960531436690 ) ) ;
#95005=CARTESIAN_POINT ( 'NONE',  ( 16.52544592524342804, -4.483927247898539470, 58.54057627198103120 ) ) ;
#95006=CARTESIAN_POINT ( 'NONE',  ( 0.05219959533936267826, -19.03943276465977164, 95.00109039468567573 ) ) ;
#95007=CARTESIAN_POINT ( 'NONE',  ( -21.53943276465977519, 0.05219959533907696930, 56.24890960531436690 ) ) ;
#95009=CARTESIAN_POINT ( 'NONE',  ( 8.314922557960818139, 14.29746914071049879, 109.5822429386476955 ) ) ;
#95010=CARTESIAN_POINT ( 'NONE',  ( -5.049401038297874678, -19.05341960407618274, 99.79275706135233293 ) ) ;
#95011=CARTESIAN_POINT ( 'NONE',  ( 16.51473224551069308, 9.474510206698969483, 54.16557627198103120 ) ) ;
#95012=CARTESIAN_POINT ( 'NONE',  ( 0.05219959533907565091, 21.53943276465977519, 59.99890960531436690 ) ) ;
#95013=CARTESIAN_POINT ( 'NONE',  ( 8.314922557961029526, -14.29746914071037800, 95.41775706135234714 ) ) ;
#95014=CARTESIAN_POINT ( 'NONE',  ( -16.46253265017160317, 9.564922557960807481, 70.83224293864770971 ) ) ;
#95015=CARTESIAN_POINT ( 'NONE',  ( -19.05341960407617563, 5.049401038297882671, 58.54275706135234003 ) ) ;
#95016=CARTESIAN_POINT ( 'NONE',  ( -21.55341960407619339, 5.719274019375674811, 83.54275706135234714 ) ) ;
#95017=CARTESIAN_POINT ( 'NONE',  ( 10.72451020669898902, -18.67979575497178502, 67.91557627198102409 ) ) ;
#95018=CARTESIAN_POINT ( 'NONE',  ( -5.049401038298153566, 19.05341960407611168, 110.2072429386476671 ) ) ;
#95019=CARTESIAN_POINT ( 'NONE',  ( 13.89961937509977652, -13.97604488694527269, 38.12390960531436690 ) ) ;
#95020=CARTESIAN_POINT ( 'NONE',  ( 16.55341960407618274, -4.379528057220086978, 96.04275706135236135 ) ) ;
#95021=CARTESIAN_POINT ( 'NONE',  ( -5.153800228976607833, 19.02544592524334988, 112.7094237280190043 ) ) ;
#95022=CARTESIAN_POINT ( 'NONE',  ( 17.44270441346514744, 5.991230190323102889, 53.86335079264230785 ) ) ;
#95023=CARTESIAN_POINT ( 'NONE',  ( -21.55341960407619339, 5.719274019375674811, 98.54275706135234714 ) ) ;
#95024=CARTESIAN_POINT ( 'NONE',  ( -8.224510206698948167, 14.34966873604960824, 65.41557627198102409 ) ) ;
#95025=CARTESIAN_POINT ( 'NONE',  ( 8.224510206698953496, -14.34966873604960469, 67.91557627198102409 ) ) ;
#95026=CARTESIAN_POINT ( 'NONE',  ( 21.53943276465977519, -0.05219959533907433946, 88.74890960531436690 ) ) ;
#95027=CARTESIAN_POINT ( 'NONE',  ( -15.72974639402197994, 15.80617190586746368, 90.62390960531436690 ) ) ;
#95028=CARTESIAN_POINT ( 'NONE',  ( 17.50000000000000000, -5.499999999999992895, 96.21769037696437010 ) ) ;
#95029=CARTESIAN_POINT ( 'NONE',  ( -21.53943276465977519, 0.05219959533907696930, 51.24890960531436690 ) ) ;
#95030=CARTESIAN_POINT ( 'NONE',  ( -14.29746914071037622, -8.314922557961029526, 64.16775706135234714 ) ) ;
#95031=CARTESIAN_POINT ( 'NONE',  ( 8.314922557960818139, 14.29746914071049879, 94.58224293864769550 ) ) ;
#95032=CARTESIAN_POINT ( 'NONE',  ( 16.51473224551069308, 9.474510206698969483, 49.16557627198102409 ) ) ;
#95033=LINE ( 'NONE', #40348, #144578 ) ;
#95034=CARTESIAN_POINT ( 'NONE',  ( -14.29746914071037622, -8.314922557961029526, 94.16775706135237556 ) ) ;
#95035=CARTESIAN_POINT ( 'NONE',  ( -0.05219959533937732626, 21.53943276465977519, 37.50109039468568284 ) ) ;
#95036=CARTESIAN_POINT ( 'NONE',  ( -5.049401038298153566, 19.05341960407611168, 100.2072429386476955 ) ) ;
#95037=CARTESIAN_POINT ( 'NONE',  ( -10.81492255796105439, 18.62759615963255655, 72.91775706135234714 ) ) ;
#95038=DIRECTION ( 'NONE',  ( 0.000000000000000000, -1.000000000000000000, 0.000000000000000000 ) ) ;
#95039=CARTESIAN_POINT ( 'NONE',  ( 5.049401038298161559, -19.05341960407611168, 27.70724293864769550 ) ) ;
#95042=EDGE_LOOP ( 'NONE', ( #85664, #189454, #147460, #71637, #99412, #1969, #92908, #198642, #149220, #40062, #151170, #31539, #66316, #163336, #124127, #83288 ) ) ;
#95043=CARTESIAN_POINT ( 'NONE',  ( 18.67979575497194134, -10.72451020669871369, 55.83442372801901854 ) ) ;
#95044=CARTESIAN_POINT ( 'NONE',  ( 9.564922557960805705, 16.46253265017160317, 39.58224293864768839 ) ) ;
#95045=CARTESIAN_POINT ( 'NONE',  ( -5.153800228976328057, -19.02544592524343514, 22.29057627198102765 ) ) ;
#95046=CARTESIAN_POINT ( 'NONE',  ( -19.02544592524342804, 5.153800228976336051, 91.04057627198100988 ) ) ;
#95047=CARTESIAN_POINT ( 'NONE',  ( -19.02544592524334988, -5.153800228976617603, 63.95942372801899012 ) ) ;
#95048=CARTESIAN_POINT ( 'NONE',  ( 10.81492255796106328, -18.62759615963255655, 35.41775706135234003 ) ) ;
#95049=CARTESIAN_POINT ( 'NONE',  ( -0.05219959533936034679, 19.03943276465977164, 57.50109039468566863 ) ) ;
#95050=CARTESIAN_POINT ( 'NONE',  ( -19.03943276465977164, 0.05219959533909376836, 41.24890960531435269 ) ) ;
#95051=CARTESIAN_POINT ( 'NONE',  ( 0.05219959533934541429, -16.53943276465976808, 100.0010903946857042 ) ) ;
#95052=CARTESIAN_POINT ( 'NONE',  ( 19.05341960407617918, -5.049401038297876454, 76.04275706135230450 ) ) ;
#95053=CARTESIAN_POINT ( 'NONE',  ( 16.53943276465976808, -0.05219959533910856209, 23.74890960531435269 ) ) ;
#95054=CARTESIAN_POINT ( 'NONE',  ( 19.03943276465977164, 0.05219959533936151252, 56.25109039468566863 ) ) ;
#95055=CARTESIAN_POINT ( 'NONE',  ( 19.02544592524343514, -5.153800228976328945, 98.54057627198100988 ) ) ;
#95056=CARTESIAN_POINT ( 'NONE',  ( 18.62759615963255655, 10.81492255796105972, 101.6677570613523613 ) ) ;
#95057=CARTESIAN_POINT ( 'NONE',  ( 5.823673210054444382, -21.52544592524334988, 105.2094237280190328 ) ) ;
#95058=CARTESIAN_POINT ( 'NONE',  ( -19.02544592524342804, 5.153800228976336051, 26.04057627198103120 ) ) ;
#95059=CARTESIAN_POINT ( 'NONE',  ( -15.72974639402176322, -15.80617190586768395, 89.37609039468568994 ) ) ;
#95060=CARTESIAN_POINT ( 'NONE',  ( 16.53943276465976808, 0.05219959533934440121, 31.25109039468568639 ) ) ;
#95062=CARTESIAN_POINT ( 'NONE',  ( 5.153800228976335163, 19.02544592524342804, 94.79057627198103830 ) ) ;
#95064=CARTESIAN_POINT ( 'NONE',  ( -13.97604488694527625, -13.89961937509977652, 76.87390960531433848 ) ) ;
#95067=CARTESIAN_POINT ( 'NONE',  ( 19.02544592524334988, 5.153800228976608722, 66.45942372801899012 ) ) ;
#95068=CARTESIAN_POINT ( 'NONE',  ( 5.049401038298161559, -19.05341960407611168, 102.7072429386476955 ) ) ;
#95069=CARTESIAN_POINT ( 'NONE',  ( 21.55341960407619695, -5.719274019375665929, 96.04275706135236135 ) ) ;
#95070=CARTESIAN_POINT ( 'NONE',  ( -4.483927247898539470, -16.52544592524342804, 102.2905762719810383 ) ) ;
#95071=CARTESIAN_POINT ( 'NONE',  ( 21.52544592524344225, -5.823673210054117533, 48.54057627198103120 ) ) ;
#95072=CARTESIAN_POINT ( 'NONE',  ( 21.53943276465977519, -0.05219959533907433946, 33.74890960531436690 ) ) ;
#95073=CARTESIAN_POINT ( 'NONE',  ( 4.379528057220339221, -16.55341960407611168, 102.7072429386476955 ) ) ;
#95075=CARTESIAN_POINT ( 'NONE',  ( 13.89961937509957401, 13.97604488694547697, 61.87609039468566863 ) ) ;
#95076=CARTESIAN_POINT ( 'NONE',  ( -16.53943276465976808, 0.05219959533911058130, 36.24890960531435979 ) ) ;
#95077=CARTESIAN_POINT ( 'NONE',  ( -5.049401038298153566, 19.05341960407611168, 110.2072429386476671 ) ) ;
#95078=CARTESIAN_POINT ( 'NONE',  ( -5.719274019375665041, -21.55341960407619695, 79.79275706135236135 ) ) ;
#95079=CARTESIAN_POINT ( 'NONE',  ( -21.55341960407610458, -5.719274019375992779, 71.45724293864769550 ) ) ;
#95080=CARTESIAN_POINT ( 'NONE',  ( 18.62759615963255655, 10.81492255796105972, 46.66775706135234714 ) ) ;
#95081=CARTESIAN_POINT ( 'NONE',  ( -21.52544592524343514, 5.823673210054127303, 101.0405762719810383 ) ) ;
#95082=CARTESIAN_POINT ( 'NONE',  ( -10.81492255796105439, 18.62759615963255655, 52.91775706135235424 ) ) ;
#95083=CARTESIAN_POINT ( 'NONE',  ( -19.03943276465977164, 0.05219959533909376836, 21.24890960531436335 ) ) ;
#95084=CARTESIAN_POINT ( 'NONE',  ( 19.02544592524343514, -5.153800228976328945, 83.54057627198100988 ) ) ;
#95085=CARTESIAN_POINT ( 'NONE',  ( -16.53943276465976808, -0.05219959533934237506, 83.75109039468568994 ) ) ;
#95086=CARTESIAN_POINT ( 'NONE',  ( 16.53943276465976808, -0.05219959533910856209, 108.7489096053143669 ) ) ;
#95087=CARTESIAN_POINT ( 'NONE',  ( -19.03943276465977164, 0.05219959533909376836, 106.2489096053143669 ) ) ;
#95088=CARTESIAN_POINT ( 'NONE',  ( -0.05219959533910754901, -16.53943276465976808, 52.49890960531435979 ) ) ;
#95089=CARTESIAN_POINT ( 'NONE',  ( -8.314922557961024197, 14.29746914071037800, 112.9177570613523329 ) ) ;
#95090=CARTESIAN_POINT ( 'NONE',  ( -16.51473224551069308, -9.474510206698971260, 66.66557627198102409 ) ) ;
#95091=CARTESIAN_POINT ( 'NONE',  ( 5.049401038298161559, -19.05341960407611168, 37.70724293864768839 ) ) ;
#95092=CARTESIAN_POINT ( 'NONE',  ( 21.55341960407610458, 5.719274019375980345, 43.95724293864769550 ) ) ;
#95093=CARTESIAN_POINT ( 'NONE',  ( 13.97604488694548053, -13.89961937509957401, 40.62609039468564731 ) ) ;
#95094=CARTESIAN_POINT ( 'NONE',  ( -17.60779699588841751, -5.499999999999946709, 86.34981316670108242 ) ) ;
#95095=CARTESIAN_POINT ( 'NONE',  ( -8.224510206698948167, 14.34966873604960824, 30.41557627198101699 ) ) ;
#95096=CARTESIAN_POINT ( 'NONE',  ( -9.564922557960796823, -16.46253265017161027, 102.0822429386477097 ) ) ;
#95097=CARTESIAN_POINT ( 'NONE',  ( -18.67979575497193778, 10.72451020669871902, 53.33442372801901854 ) ) ;
#95099=CARTESIAN_POINT ( 'NONE',  ( 16.55341960407618274, -4.379528057220086978, 56.04275706135235424 ) ) ;
#95100=CARTESIAN_POINT ( 'NONE',  ( 16.51473224551083163, -9.474510206698727899, 55.83442372801899722 ) ) ;
#95101=CARTESIAN_POINT ( 'NONE',  ( 4.483927247898545687, 16.52544592524342804, 24.79057627198103120 ) ) ;
#95102=CARTESIAN_POINT ( 'NONE',  ( 22.00000000000000000, -5.510910596163089556E-15, 45.00000000000000000 ) ) ;
#95103=CARTESIAN_POINT ( 'NONE',  ( 12.06949235617739724, 12.14591786802326823, 111.8760903946856615 ) ) ;
#95104=CARTESIAN_POINT ( 'NONE',  ( 16.51473224551069308, 9.474510206698969483, 39.16557627198103120 ) ) ;
#95105=CARTESIAN_POINT ( 'NONE',  ( -19.03943276465977164, 0.05219959533909376836, 61.24890960531436690 ) ) ;
#95106=CARTESIAN_POINT ( 'NONE',  ( 0.05219959533909260263, 19.03943276465977164, 24.99890960531435269 ) ) ;
#95107=CARTESIAN_POINT ( 'NONE',  ( 15.72974639402176855, 15.80617190586768217, 36.87609039468568994 ) ) ;
#95108=CARTESIAN_POINT ( 'NONE',  ( 19.02544592524343514, -5.153800228976328945, 43.54057627198103120 ) ) ;
#95109=CARTESIAN_POINT ( 'NONE',  ( -19.03943276465977164, 0.05219959533909376836, 116.2489096053143669 ) ) ;
#95110=CARTESIAN_POINT ( 'NONE',  ( 19.02544592524343514, -5.153800228976328945, 48.54057627198103120 ) ) ;
#95111=CARTESIAN_POINT ( 'NONE',  ( -16.46253265017160317, 9.564922557960807481, 115.8322429386477097 ) ) ;
#95112=CARTESIAN_POINT ( 'NONE',  ( 15.80617190586769283, -15.72974639402175789, 65.62609039468568994 ) ) ;
#95113=CARTESIAN_POINT ( 'NONE',  ( -16.51473224551069308, -9.474510206698971260, 21.66557627198102765 ) ) ;
#95114=CARTESIAN_POINT ( 'NONE',  ( -21.52544592524343514, 5.823673210054127303, 31.04057627198102409 ) ) ;
#95115=CARTESIAN_POINT ( 'NONE',  ( 4.483927247898790824, -16.52544592524335698, 80.20942372801901854 ) ) ;
#95116=CARTESIAN_POINT ( 'NONE',  ( 15.80617190586769283, -15.72974639402175789, 100.6260903946857184 ) ) ;
#95117=CARTESIAN_POINT ( 'NONE',  ( 16.55341960407618274, -4.379528057220086978, 51.04275706135234714 ) ) ;
#95118=CARTESIAN_POINT ( 'NONE',  ( 19.03943276465977164, -0.05219959533909143690, 93.74890960531435269 ) ) ;
#95119=CARTESIAN_POINT ( 'NONE',  ( 16.52544592524335698, 4.483927247898782831, 36.45942372801901143 ) ) ;
#95120=CARTESIAN_POINT ( 'NONE',  ( 14.34966873604972726, -8.224510206698740333, 25.83442372801901499 ) ) ;
#95121=CARTESIAN_POINT ( 'NONE',  ( 16.55341960407618274, -4.379528057220086978, 96.04275706135236135 ) ) ;
#95122=CARTESIAN_POINT ( 'NONE',  ( -15.80617190586768217, 15.72974639402176855, 53.12609039468568284 ) ) ;
#95123=CARTESIAN_POINT ( 'NONE',  ( 0.05219959533936267826, -19.03943276465977164, 105.0010903946856615 ) ) ;
#95124=CARTESIAN_POINT ( 'NONE',  ( -18.62759615963270932, 10.81492255796079327, 115.8322429386477097 ) ) ;
#95125=CARTESIAN_POINT ( 'NONE',  ( 14.34966873604960469, 8.224510206698951720, 99.16557627198100988 ) ) ;
#95126=CARTESIAN_POINT ( 'NONE',  ( -16.51473224551082808, 9.474510206698731452, 108.3344237280190043 ) ) ;
#95127=CARTESIAN_POINT ( 'NONE',  ( -16.52544592524335698, -4.483927247898792601, 73.95942372801901854 ) ) ;
#95128=CARTESIAN_POINT ( 'NONE',  ( -16.88567814943193568, 6.947325034625407625, 43.70998877347406619 ) ) ;
#95129=CARTESIAN_POINT ( 'NONE',  ( -9.474510206698720793, -16.51473224551083518, 89.58442372801900433 ) ) ;
#95130=CARTESIAN_POINT ( 'NONE',  ( -4.379528057220328563, 16.55341960407611168, 40.20724293864769550 ) ) ;
#95131=CARTESIAN_POINT ( 'NONE',  ( -16.52544592524342804, 4.483927247898546575, 41.04057627198103120 ) ) ;
#95132=CARTESIAN_POINT ( 'NONE',  ( 16.53943276465976808, -0.05219959533910856209, 103.7489096053143669 ) ) ;
#95133=CARTESIAN_POINT ( 'NONE',  ( 5.153800228976615827, -19.02544592524334988, 40.20942372801898301 ) ) ;
#95134=CARTESIAN_POINT ( 'NONE',  ( -17.49999999999999645, 5.499999999999992895, 93.71769037696437010 ) ) ;
#95135=CARTESIAN_POINT ( 'NONE',  ( 21.55341960407619695, -5.719274019375665929, 31.04275706135234714 ) ) ;
#95136=CARTESIAN_POINT ( 'NONE',  ( 0.05219959533936267826, -19.03943276465977164, 105.0010903946856615 ) ) ;
#95138=CARTESIAN_POINT ( 'NONE',  ( 19.05341960407611168, 5.049401038298154454, 93.95724293864769550 ) ) ;
#95139=CARTESIAN_POINT ( 'NONE',  ( -5.049401038298153566, 19.05341960407611168, 95.20724293864770971 ) ) ;
#95140=CARTESIAN_POINT ( 'NONE',  ( 0.05219959533907565091, 21.53943276465977519, 54.99890960531435269 ) ) ;
#95141=CARTESIAN_POINT ( 'NONE',  ( 8.224510206698953496, -14.34966873604960469, 97.91557627198103830 ) ) ;
#95142=CARTESIAN_POINT ( 'NONE',  ( 16.46253265017160672, -9.564922557960803928, 68.33224293864770971 ) ) ;
#95143=CARTESIAN_POINT ( 'NONE',  ( 0.05219959533909260263, 19.03943276465977164, 29.99890960531435979 ) ) ;
#95144=CARTESIAN_POINT ( 'NONE',  ( 21.55341960407619695, -5.719274019375665929, 41.04275706135236135 ) ) ;
#95145=CARTESIAN_POINT ( 'NONE',  ( 18.67979575497194134, -10.72451020669871369, 70.83442372801901854 ) ) ;
#95146=CARTESIAN_POINT ( 'NONE',  ( -14.34966873604972548, 8.224510206698743886, 93.33442372801901854 ) ) ;
#95147=CARTESIAN_POINT ( 'NONE',  ( 0.05219959533937995610, -21.53943276465977519, 35.00109039468568284 ) ) ;
#95148=CARTESIAN_POINT ( 'NONE',  ( -10.81492255796105439, 18.62759615963255655, 27.91775706135234358 ) ) ;
#95149=CARTESIAN_POINT ( 'NONE',  ( 13.89961937509957401, 13.97604488694547697, 56.87609039468564731 ) ) ;
#95150=CARTESIAN_POINT ( 'NONE',  ( -13.97604488694527625, -13.89961937509977652, 81.87390960531436690 ) ) ;
#95151=CARTESIAN_POINT ( 'NONE',  ( 15.72974639402176855, 15.80617190586768217, 81.87609039468568994 ) ) ;
#95153=CARTESIAN_POINT ( 'NONE',  ( 18.67979575497178502, 10.72451020669898547, 84.16557627198103830 ) ) ;
#95154=CARTESIAN_POINT ( 'NONE',  ( -16.55341960407611168, -4.379528057220339221, 46.45724293864769550 ) ) ;
#95155=CARTESIAN_POINT ( 'NONE',  ( -5.719274019375665041, -21.55341960407619695, 109.7927570613523613 ) ) ;
#95156=CARTESIAN_POINT ( 'NONE',  ( 19.03943276465977164, 0.05219959533936151252, 46.25109039468566863 ) ) ;
#95157=CARTESIAN_POINT ( 'NONE',  ( -0.05219959533910754901, -16.53943276465976808, 72.49890960531435269 ) ) ;
#95158=CARTESIAN_POINT ( 'NONE',  ( -5.049401038298153566, 19.05341960407611168, 25.20724293864768484 ) ) ;
#95159=CARTESIAN_POINT ( 'NONE',  ( -19.05341960407617563, 5.049401038297882671, 73.54275706135233293 ) ) ;
#95160=CARTESIAN_POINT ( 'NONE',  ( 14.29746914071049879, -8.314922557960816363, 38.33224293864768839 ) ) ;
#95161=CARTESIAN_POINT ( 'NONE',  ( -10.72451020669870658, -18.67979575497194134, 79.58442372801903275 ) ) ;
#95162=CARTESIAN_POINT ( 'NONE',  ( 0.05219959533909260263, 19.03943276465977164, 79.99890960531436690 ) ) ;
#95163=CARTESIAN_POINT ( 'NONE',  ( -13.89961937509957401, -13.97604488694547875, 64.37609039468567573 ) ) ;
#95164=CARTESIAN_POINT ( 'NONE',  ( -18.62759615963270932, 10.81492255796079327, 60.83224293864769550 ) ) ;
#95165=CARTESIAN_POINT ( 'NONE',  ( -21.53943276465977519, 0.05219959533907696930, 116.2489096053143669 ) ) ;
#95166=CARTESIAN_POINT ( 'NONE',  ( -12.06949235617739369, -12.14591786802326823, 19.37609039468568639 ) ) ;
#95167=CARTESIAN_POINT ( 'NONE',  ( -8.314922557961024197, 14.29746914071037800, 82.91775706135234714 ) ) ;
#95168=CARTESIAN_POINT ( 'NONE',  ( 17.12812012977025589, 6.668231424566066323, 63.85948759323147073 ) ) ;
#95169=CARTESIAN_POINT ( 'NONE',  ( 21.55341960407619695, -5.719274019375665929, 26.04275706135235779 ) ) ;
#95170=CARTESIAN_POINT ( 'NONE',  ( -4.379528057220328563, 16.55341960407611168, 100.2072429386476955 ) ) ;
#95172=CARTESIAN_POINT ( 'NONE',  ( -8.314922557961024197, 14.29746914071037800, 37.91775706135235424 ) ) ;
#95174=CARTESIAN_POINT ( 'NONE',  ( -5.719274019375978568, 21.55341960407610458, 60.20724293864768839 ) ) ;
#95175=CARTESIAN_POINT ( 'NONE',  ( 14.34966873604972726, -8.224510206698740333, 105.8344237280190328 ) ) ;
#95176=CARTESIAN_POINT ( 'NONE',  ( -8.314922557961024197, 14.29746914071037800, 37.91775706135235424 ) ) ;
#95177=CARTESIAN_POINT ( 'NONE',  ( -13.97604488694527625, -13.89961937509977652, 31.87390960531435979 ) ) ;
#95178=CARTESIAN_POINT ( 'NONE',  ( 16.55341960407618274, -4.379528057220086978, 86.04275706135236135 ) ) ;
#95179=CARTESIAN_POINT ( 'NONE',  ( -0.05219959533936034679, 19.03943276465977164, 77.50109039468566152 ) ) ;
#95182=CARTESIAN_POINT ( 'NONE',  ( -10.81492255796078084, -18.62759615963271287, 57.08224293864769550 ) ) ;
#95183=CARTESIAN_POINT ( 'NONE',  ( -16.52544592524335698, -4.483927247898792601, 103.9594237280190185 ) ) ;
#95184=CARTESIAN_POINT ( 'NONE',  ( -0.05219959533937732626, 21.53943276465977519, 77.50109039468567573 ) ) ;
#95185=CARTESIAN_POINT ( 'NONE',  ( -10.81492255796078084, -18.62759615963271287, 52.08224293864768839 ) ) ;
#95186=CARTESIAN_POINT ( 'NONE',  ( 18.67979575497178502, 10.72451020669898547, 54.16557627198103120 ) ) ;
#95187=CARTESIAN_POINT ( 'NONE',  ( 12.06949235617739724, 12.14591786802326823, 76.87609039468567573 ) ) ;
#95188=CARTESIAN_POINT ( 'NONE',  ( -10.81492255796078084, -18.62759615963271287, 52.08224293864768839 ) ) ;
#95189=ORIENTED_EDGE ( 'NONE', *, *, #26316, .T. ) ;
#95190=CARTESIAN_POINT ( 'NONE',  ( 5.153800228976335163, 19.02544592524342804, 104.7905762719809957 ) ) ;
#95192=CARTESIAN_POINT ( 'NONE',  ( -0.05219959533909027116, -19.03943276465977164, 32.49890960531435979 ) ) ;
#95193=CARTESIAN_POINT ( 'NONE',  ( 10.72451020669898902, -18.67979575497178502, 57.91557627198103120 ) ) ;
#95194=CARTESIAN_POINT ( 'NONE',  ( -12.06949235617739369, -12.14591786802326823, 94.37609039468568994 ) ) ;
#95195=CARTESIAN_POINT ( 'NONE',  ( 10.81492255796106328, -18.62759615963255655, 50.41775706135235424 ) ) ;
#95196=CARTESIAN_POINT ( 'NONE',  ( -5.153800228976607833, 19.02544592524334988, 102.7094237280189759 ) ) ;
#95197=CARTESIAN_POINT ( 'NONE',  ( 16.52544592524342804, -4.483927247898539470, 108.5405762719810241 ) ) ;
#95198=CARTESIAN_POINT ( 'NONE',  ( -13.89961937509957401, -13.97604488694547875, 104.3760903946856757 ) ) ;
#95200=CARTESIAN_POINT ( 'NONE',  ( 19.05341960407611168, 5.049401038298154454, 38.95724293864767418 ) ) ;
#95201=CARTESIAN_POINT ( 'NONE',  ( 22.00000000000000000, -5.510910596163089556E-15, 45.00000000000000000 ) ) ;
#95202=CARTESIAN_POINT ( 'NONE',  ( -9.474510206698964154, 16.51473224551069663, 85.41557627198102409 ) ) ;
#95203=CARTESIAN_POINT ( 'NONE',  ( -4.483927247898782831, 16.52544592524335698, 77.70942372801900433 ) ) ;
#95204=CARTESIAN_POINT ( 'NONE',  ( -15.80617190586768217, 15.72974639402176855, 108.1260903946856757 ) ) ;
#95205=CARTESIAN_POINT ( 'NONE',  ( -15.80617190586745835, -15.72974639402198527, 66.87390960531436690 ) ) ;
#95206=CARTESIAN_POINT ( 'NONE',  ( -14.29746914071037622, -8.314922557961029526, 89.16775706135236135 ) ) ;
#95207=CARTESIAN_POINT ( 'NONE',  ( -9.474510206698720793, -16.51473224551083518, 74.58442372801900433 ) ) ;
#95208=CARTESIAN_POINT ( 'NONE',  ( 5.049401038298161559, -19.05341960407611168, 42.70724293864767418 ) ) ;
#95209=CARTESIAN_POINT ( 'NONE',  ( -19.05341960407611168, -5.049401038298163336, 76.45724293864769550 ) ) ;
#95211=CARTESIAN_POINT ( 'NONE',  ( -5.719274019375665041, -21.55341960407619695, 44.79275706135234714 ) ) ;
#95212=CARTESIAN_POINT ( 'NONE',  ( -19.05341960407611168, -5.049401038298163336, 51.45724293864770260 ) ) ;
#95213=CARTESIAN_POINT ( 'NONE',  ( 13.89961937509957401, 13.97604488694547697, 76.87609039468566152 ) ) ;
#95215=CARTESIAN_POINT ( 'NONE',  ( 16.46253265017160672, -9.564922557960803928, 113.3322429386476955 ) ) ;
#95216=CARTESIAN_POINT ( 'NONE',  ( 14.29746914071049879, -8.314922557960816363, 68.33224293864769550 ) ) ;
#95217=CARTESIAN_POINT ( 'NONE',  ( -21.53943276465977519, 0.05219959533907696930, 66.24890960531436690 ) ) ;
#95219=CARTESIAN_POINT ( 'NONE',  ( -16.51473224551082808, 9.474510206698731452, 23.33442372801900078 ) ) ;
#95221=CARTESIAN_POINT ( 'NONE',  ( -13.89961937509977652, 13.97604488694528158, 70.62390960531432427 ) ) ;
#95222=CARTESIAN_POINT ( 'NONE',  ( 5.049401038298161559, -19.05341960407611168, 77.70724293864765286 ) ) ;
#95223=CARTESIAN_POINT ( 'NONE',  ( 8.224510206698742110, 14.34966873604972548, 57.08442372801901854 ) ) ;
#95225=CARTESIAN_POINT ( 'NONE',  ( -16.81555441253554051, 7.025013491695463408, 110.6368544533425791 ) ) ;
#95226=CARTESIAN_POINT ( 'NONE',  ( 8.224510206698742110, 14.34966873604972548, 92.08442372801901854 ) ) ;
#95227=CARTESIAN_POINT ( 'NONE',  ( 17.50000000000000711, 5.499999999999976907, 93.78230962303565832 ) ) ;
#95228=CARTESIAN_POINT ( 'NONE',  ( -0.05219959533934338120, 16.53943276465976808, 67.50109039468568994 ) ) ;
#95229=CARTESIAN_POINT ( 'NONE',  ( 0.05219959533934541429, -16.53943276465976808, 45.00109039468568284 ) ) ;
#95230=CARTESIAN_POINT ( 'NONE',  ( 19.05341960407611168, 5.049401038298154454, 53.95724293864770260 ) ) ;
#95232=CARTESIAN_POINT ( 'NONE',  ( 21.52544592524334988, 5.823673210054432836, 56.45942372801902565 ) ) ;
#95233=CARTESIAN_POINT ( 'NONE',  ( -0.05219959533936034679, 19.03943276465977164, 57.50109039468566863 ) ) ;
#95234=CARTESIAN_POINT ( 'NONE',  ( -10.81492255796105439, 18.62759615963255655, 112.9177570613523329 ) ) ;
#95235=CARTESIAN_POINT ( 'NONE',  ( -13.89961937509977652, 13.97604488694528158, 30.62390960531435269 ) ) ;
#95236=CARTESIAN_POINT ( 'NONE',  ( 16.23956094088878288, 7.360292434722755850, 22.49130789039435641 ) ) ;
#95237=CARTESIAN_POINT ( 'NONE',  ( 10.72451020669898902, -18.67979575497178502, 47.91557627198102409 ) ) ;
#95238=CARTESIAN_POINT ( 'NONE',  ( -13.89961937509977652, 13.97604488694528158, 105.6239096053143527 ) ) ;
#95239=CARTESIAN_POINT ( 'NONE',  ( -0.05219959533910754901, -16.53943276465976808, 107.4989096053143669 ) ) ;
#95240=CARTESIAN_POINT ( 'NONE',  ( -4.379528057220086978, -16.55341960407618274, 34.79275706135235424 ) ) ;
#95241=EDGE_CURVE ( 'NONE', #3778, #9238, #54682, .T. ) ;
#95242=CARTESIAN_POINT ( 'NONE',  ( -8.314922557960811034, -14.29746914071050412, 27.08224293864769550 ) ) ;
#95243=ORIENTED_EDGE ( 'NONE', *, *, #93518, .T. ) ;
#95244=CARTESIAN_POINT ( 'NONE',  ( -0.05219959533907301413, -21.53943276465977519, 97.49890960531436690 ) ) ;
#95245=CARTESIAN_POINT ( 'NONE',  ( 8.224510206698953496, -14.34966873604960469, 32.91557627198102409 ) ) ;
#95246=CARTESIAN_POINT ( 'NONE',  ( 16.51473224551069308, 9.474510206698969483, 114.1655762719810241 ) ) ;
#95247=CARTESIAN_POINT ( 'NONE',  ( -0.05219959533936034679, 19.03943276465977164, 92.50109039468566152 ) ) ;
#95248=CARTESIAN_POINT ( 'NONE',  ( -5.153800228976607833, 19.02544592524334988, 27.70942372801899722 ) ) ;
#95249=CARTESIAN_POINT ( 'NONE',  ( -16.55341960407611168, -4.379528057220339221, 26.45724293864768839 ) ) ;
#95250=CARTESIAN_POINT ( 'NONE',  ( -10.81492255796078084, -18.62759615963271287, 97.08224293864770971 ) ) ;
#95251=CARTESIAN_POINT ( 'NONE',  ( -21.55341960407610458, -5.719274019375992779, 56.45724293864768839 ) ) ;
#95252=CARTESIAN_POINT ( 'NONE',  ( 19.05341960407611168, 5.049401038298154454, 78.95724293864769550 ) ) ;
#95253=CARTESIAN_POINT ( 'NONE',  ( 16.52544592524342804, -4.483927247898539470, 53.54057627198103120 ) ) ;
#95254=CARTESIAN_POINT ( 'NONE',  ( 19.05341960407611168, 5.049401038298154454, 93.95724293864769550 ) ) ;
#95257=CARTESIAN_POINT ( 'NONE',  ( 18.22780087662123805, -5.499999999999989342, 63.51763182126896368 ) ) ;
#95258=CARTESIAN_POINT ( 'NONE',  ( -19.05341960407617563, 5.049401038297882671, 43.54275706135232582 ) ) ;
#95259=CARTESIAN_POINT ( 'NONE',  ( 18.62759615963271287, -10.81492255796078972, 93.33224293864769550 ) ) ;
#95260=CARTESIAN_POINT ( 'NONE',  ( 8.314922557960818139, 14.29746914071049879, 94.58224293864769550 ) ) ;
#95261=CARTESIAN_POINT ( 'NONE',  ( 15.72974639402176855, 15.80617190586768217, 31.87609039468567929 ) ) ;
#95263=CARTESIAN_POINT ( 'NONE',  ( -8.314922557961024197, 14.29746914071037800, 102.9177570613523756 ) ) ;
#95264=CARTESIAN_POINT ( 'NONE',  ( 9.474510206698971260, -16.51473224551069308, 37.91557627198102409 ) ) ;
#95265=CARTESIAN_POINT ( 'NONE',  ( 0.05219959533909260263, 19.03943276465977164, 89.99890960531436690 ) ) ;
#95266=CARTESIAN_POINT ( 'NONE',  ( -19.46398650005389541, 5.499999999999948486, 45.18269651486372851 ) ) ;
#95267=CARTESIAN_POINT ( 'NONE',  ( 19.03943276465977164, -0.05219959533909143690, 28.74890960531435624 ) ) ;
#95268=CARTESIAN_POINT ( 'NONE',  ( 8.224510206698953496, -14.34966873604960469, 37.91557627198102409 ) ) ;
#95269=CARTESIAN_POINT ( 'NONE',  ( -10.72451020669870658, -18.67979575497194134, 79.58442372801903275 ) ) ;
#95271=CARTESIAN_POINT ( 'NONE',  ( -0.05219959533934338120, 16.53943276465976808, 72.50109039468568994 ) ) ;
#95272=CARTESIAN_POINT ( 'NONE',  ( -19.05341960407611168, -5.049401038298163336, 61.45724293864769550 ) ) ;
#95273=CARTESIAN_POINT ( 'NONE',  ( -13.97604488694527625, -13.89961937509977652, 61.87390960531435979 ) ) ;
#95275=CARTESIAN_POINT ( 'NONE',  ( -21.55341960407619339, 5.719274019375674811, 103.5427570613523613 ) ) ;
#95276=CARTESIAN_POINT ( 'NONE',  ( -16.55341960407617563, 4.379528057220093196, 73.54275706135234714 ) ) ;
#95277=CARTESIAN_POINT ( 'NONE',  ( -10.81492255796105439, 18.62759615963255655, 102.9177570613523756 ) ) ;
#95278=CARTESIAN_POINT ( 'NONE',  ( -16.51473224551069308, -9.474510206698971260, 66.66557627198102409 ) ) ;
#95279=CARTESIAN_POINT ( 'NONE',  ( -18.67979575497178146, -10.72451020669898902, 36.66557627198103120 ) ) ;
#95280=CARTESIAN_POINT ( 'NONE',  ( 19.02544592524334988, 5.153800228976608722, 101.4594237280189759 ) ) ;
#95281=CARTESIAN_POINT ( 'NONE',  ( -5.719274019375665041, -21.55341960407619695, 84.79275706135234714 ) ) ;
#95282=CARTESIAN_POINT ( 'NONE',  ( -8.224510206698735004, -14.34966873604973081, 49.58442372801901143 ) ) ;
#95283=CARTESIAN_POINT ( 'NONE',  ( -18.62759615963270932, 10.81492255796079327, 100.8322429386477097 ) ) ;
#95284=CARTESIAN_POINT ( 'NONE',  ( 19.02544592524334988, 5.153800228976608722, 101.4594237280189759 ) ) ;
#95285=CARTESIAN_POINT ( 'NONE',  ( -9.564922557960796823, -16.46253265017161027, 82.08224293864768129 ) ) ;
#95286=CARTESIAN_POINT ( 'NONE',  ( 19.03943276465977164, 0.05219959533936151252, 106.2510903946856615 ) ) ;
#95287=CARTESIAN_POINT ( 'NONE',  ( 14.34966873604972726, -8.224510206698740333, 25.83442372801901499 ) ) ;
#95288=CARTESIAN_POINT ( 'NONE',  ( -14.34966873604960291, -8.224510206698953496, 71.66557627198100988 ) ) ;
#95289=CARTESIAN_POINT ( 'NONE',  ( -14.34966873604972548, 8.224510206698743886, 68.33442372801900433 ) ) ;
#95290=CARTESIAN_POINT ( 'NONE',  ( 15.80617190586769283, -15.72974639402175789, 20.62609039468568639 ) ) ;
#95291=CARTESIAN_POINT ( 'NONE',  ( -0.05219959533909027116, -19.03943276465977164, 57.49890960531435979 ) ) ;
#95292=CARTESIAN_POINT ( 'NONE',  ( 5.153800228976335163, 19.02544592524342804, 74.79057627198103830 ) ) ;
#95293=CARTESIAN_POINT ( 'NONE',  ( -14.29746914071037622, -8.314922557961029526, 79.16775706135234714 ) ) ;
#95296=CARTESIAN_POINT ( 'NONE',  ( 21.52544592524334988, 5.823673210054432836, 106.4594237280190328 ) ) ;
#95297=CARTESIAN_POINT ( 'NONE',  ( -9.564922557960796823, -16.46253265017161027, 42.08224293864769550 ) ) ;
#95299=CARTESIAN_POINT ( 'NONE',  ( -0.05219959533934338120, 16.53943276465976808, 27.50109039468567929 ) ) ;
#95300=CARTESIAN_POINT ( 'NONE',  ( -9.474510206698720793, -16.51473224551083518, 49.58442372801899722 ) ) ;
#95301=CARTESIAN_POINT ( 'NONE',  ( -4.379528057220086978, -16.55341960407618274, 34.79275706135235424 ) ) ;
#95302=CARTESIAN_POINT ( 'NONE',  ( 5.049401038298161559, -19.05341960407611168, 42.70724293864767418 ) ) ;
#95303=CARTESIAN_POINT ( 'NONE',  ( -16.46253265017160317, 9.564922557960807481, 65.83224293864769550 ) ) ;
#95304=CARTESIAN_POINT ( 'NONE',  ( 0.05219959533907565091, 21.53943276465977519, 89.99890960531438111 ) ) ;
#95305=CARTESIAN_POINT ( 'NONE',  ( -19.05341960407611168, -5.049401038298163336, 106.4572429386476955 ) ) ;
#95306=CARTESIAN_POINT ( 'NONE',  ( 9.474510206698971260, -16.51473224551069308, 47.91557627198102409 ) ) ;
#95308=CARTESIAN_POINT ( 'NONE',  ( -5.049401038297874678, -19.05341960407617918, 94.79275706135230450 ) ) ;
#95309=CARTESIAN_POINT ( 'NONE',  ( 21.55341960407610458, 5.719274019375980345, 73.95724293864769550 ) ) ;
#95310=CARTESIAN_POINT ( 'NONE',  ( -21.53943276465977519, -0.05219959533937600094, 113.7510903946856757 ) ) ;
#95311=CARTESIAN_POINT ( 'NONE',  ( -8.224510206698948167, 14.34966873604960824, 60.41557627198102409 ) ) ;
#95312=CARTESIAN_POINT ( 'NONE',  ( 18.67979575497194134, -10.72451020669871369, 85.83442372801901854 ) ) ;
#95313=CARTESIAN_POINT ( 'NONE',  ( 5.153800228976335163, 19.02544592524342804, 24.79057627198102765 ) ) ;
#95314=CARTESIAN_POINT ( 'NONE',  ( 14.29746914071049879, -8.314922557960816363, 33.33224293864769550 ) ) ;
#95315=CARTESIAN_POINT ( 'NONE',  ( -5.719274019375665041, -21.55341960407619695, 89.79275706135236135 ) ) ;
#95316=CARTESIAN_POINT ( 'NONE',  ( 9.474510206698971260, -16.51473224551069308, 77.91557627198103830 ) ) ;
#95317=CARTESIAN_POINT ( 'NONE',  ( 10.72451020669871369, 18.67979575497193778, 42.08442372801901854 ) ) ;
#95318=CARTESIAN_POINT ( 'NONE',  ( -9.564922557960796823, -16.46253265017161027, 87.08224293864769550 ) ) ;
#95319=CARTESIAN_POINT ( 'NONE',  ( 14.34966873604960469, 8.224510206698951720, 89.16557627198102409 ) ) ;
#95320=CARTESIAN_POINT ( 'NONE',  ( 16.53943276465976808, -0.05219959533910856209, 63.74890960531435979 ) ) ;
#95321=CARTESIAN_POINT ( 'NONE',  ( 0.05219959533907565091, 21.53943276465977519, 69.99890960531435269 ) ) ;
#95322=CARTESIAN_POINT ( 'NONE',  ( -5.153800228976328057, -19.02544592524343514, 77.29057627198099567 ) ) ;
#95323=CARTESIAN_POINT ( 'NONE',  ( 5.719274019375991003, -21.55341960407610458, 87.70724293864769550 ) ) ;
#95325=CARTESIAN_POINT ( 'NONE',  ( 0.05219959533936267826, -19.03943276465977164, 75.00109039468566152 ) ) ;
#95326=CARTESIAN_POINT ( 'NONE',  ( -19.03943276465977164, -0.05219959533935918106, 28.75109039468566507 ) ) ;
#95327=CARTESIAN_POINT ( 'NONE',  ( -4.379528057220328563, 16.55341960407611168, 70.20724293864769550 ) ) ;
#95328=CARTESIAN_POINT ( 'NONE',  ( 10.72451020669898902, -18.67979575497178502, 52.91557627198103830 ) ) ;
#95330=CARTESIAN_POINT ( 'NONE',  ( 8.314922557961029526, -14.29746914071037800, 100.4177570613523471 ) ) ;
#95332=CARTESIAN_POINT ( 'NONE',  ( 9.564922557961047289, -16.46253265017146816, 100.4177570613523329 ) ) ;
#95333=CARTESIAN_POINT ( 'NONE',  ( -16.53943276465976808, 0.05219959533911058130, 81.24890960531436690 ) ) ;
#95334=CARTESIAN_POINT ( 'NONE',  ( -19.53091890409951858, -5.499999999999991118, 95.06097431831415179 ) ) ;
#95335=CARTESIAN_POINT ( 'NONE',  ( 9.474510206698971260, -16.51473224551069308, 67.91557627198102409 ) ) ;
#95336=CARTESIAN_POINT ( 'NONE',  ( -9.474510206698964154, 16.51473224551069663, 35.41557627198102409 ) ) ;
#95337=CARTESIAN_POINT ( 'NONE',  ( 16.53943276465976808, -0.05219959533910856209, 48.74890960531435979 ) ) ;
#95338=CARTESIAN_POINT ( 'NONE',  ( -9.474510206698964154, 16.51473224551069663, 105.4155762719810383 ) ) ;
#95339=CARTESIAN_POINT ( 'NONE',  ( 9.474510206698729675, 16.51473224551082808, 87.08442372801900433 ) ) ;
#95340=CARTESIAN_POINT ( 'NONE',  ( 13.89961937509977652, -13.97604488694527269, 63.12390960531435979 ) ) ;
#95341=CARTESIAN_POINT ( 'NONE',  ( 8.224510206698742110, 14.34966873604972548, 32.08442372801901854 ) ) ;
#95342=CARTESIAN_POINT ( 'NONE',  ( -19.05341960407611168, -5.049401038298163336, 86.45724293864769550 ) ) ;
#95343=CARTESIAN_POINT ( 'NONE',  ( -15.72974639402197994, 15.80617190586746368, 60.62390960531437401 ) ) ;
#95344=CARTESIAN_POINT ( 'NONE',  ( -14.29746914071037622, -8.314922557961029526, 59.16775706135234714 ) ) ;
#95346=CARTESIAN_POINT ( 'NONE',  ( 19.03943276465977164, 0.05219959533936151252, 111.2510903946856757 ) ) ;
#95347=CARTESIAN_POINT ( 'NONE',  ( 13.89961937509977652, -13.97604488694527269, 63.12390960531435979 ) ) ;
#95348=CARTESIAN_POINT ( 'NONE',  ( 15.72974639402199770, -15.80617190586745480, 63.12390960531435979 ) ) ;
#95349=CARTESIAN_POINT ( 'NONE',  ( -19.05341960407617563, 5.049401038297882671, 88.54275706135230450 ) ) ;
#95350=CARTESIAN_POINT ( 'NONE',  ( -4.483927247898539470, -16.52544592524342804, 22.29057627198102765 ) ) ;
#95351=CARTESIAN_POINT ( 'NONE',  ( 10.81492255796106328, -18.62759615963255655, 50.41775706135235424 ) ) ;
#95353=CARTESIAN_POINT ( 'NONE',  ( -12.14591786802326823, 12.06949235617739902, 68.12609039468567573 ) ) ;
#95354=CARTESIAN_POINT ( 'NONE',  ( 0.05219959533934541429, -16.53943276465976808, 90.00109039468567573 ) ) ;
#95355=CARTESIAN_POINT ( 'NONE',  ( -17.72696623605160227, 5.500000000000055955, 73.59811031808419557 ) ) ;
#95356=CARTESIAN_POINT ( 'NONE',  ( -16.55341960407617563, 4.379528057220093196, 98.54275706135234714 ) ) ;
#95357=CARTESIAN_POINT ( 'NONE',  ( 16.52544592524335698, 4.483927247898782831, 31.45942372801901854 ) ) ;
#95358=CARTESIAN_POINT ( 'NONE',  ( -9.474510206698964154, 16.51473224551069663, 45.41557627198103120 ) ) ;
#95359=CARTESIAN_POINT ( 'NONE',  ( -9.564922557960796823, -16.46253265017161027, 52.08224293864768839 ) ) ;
#95360=CARTESIAN_POINT ( 'NONE',  ( 13.97604488694527802, 13.89961937509977652, 54.37390960531435979 ) ) ;
#95361=CARTESIAN_POINT ( 'NONE',  ( 18.62759615963255655, 10.81492255796105972, 46.66775706135234714 ) ) ;
#95362=CARTESIAN_POINT ( 'NONE',  ( 16.55341960407618274, -4.379528057220086978, 51.04275706135234714 ) ) ;
#95363=CARTESIAN_POINT ( 'NONE',  ( -16.53943276465976808, 0.05219959533911058130, 31.24890960531435979 ) ) ;
#95364=CARTESIAN_POINT ( 'NONE',  ( 5.049401038298161559, -19.05341960407611168, 47.70724293864770260 ) ) ;
#95365=CARTESIAN_POINT ( 'NONE',  ( 19.02544592524343514, -5.153800228976328945, 33.54057627198102409 ) ) ;
#95366=CARTESIAN_POINT ( 'NONE',  ( -14.34966873604972548, 8.224510206698743886, 33.33442372801900433 ) ) ;
#95367=CARTESIAN_POINT ( 'NONE',  ( 5.153800228976615827, -19.02544592524334988, 85.20942372801900433 ) ) ;
#95368=CARTESIAN_POINT ( 'NONE',  ( 0.05219959533910956823, 16.53943276465976808, 79.99890960531435269 ) ) ;
#95369=CARTESIAN_POINT ( 'NONE',  ( 13.89961937509977652, -13.97604488694527269, 58.12390960531436690 ) ) ;
#95370=CARTESIAN_POINT ( 'NONE',  ( -9.564922557961040184, 16.46253265017147172, 92.91775706135233293 ) ) ;
#95372=CARTESIAN_POINT ( 'NONE',  ( -18.67979575497193778, 10.72451020669871902, 83.33442372801903275 ) ) ;
#95373=CARTESIAN_POINT ( 'NONE',  ( -4.483927247898782831, 16.52544592524335698, 57.70942372801901143 ) ) ;
#95374=CARTESIAN_POINT ( 'NONE',  ( -17.49999999999998579, 3.345213924137300232, 24.58768623094359640 ) ) ;
#95375=CARTESIAN_POINT ( 'NONE',  ( -21.55341960407610458, -5.719274019375992779, 46.45724293864769550 ) ) ;
#95376=CARTESIAN_POINT ( 'NONE',  ( -16.53943276465976808, -0.05219959533934237506, 43.75109039468568284 ) ) ;
#95377=CARTESIAN_POINT ( 'NONE',  ( -19.03943276465977164, 0.05219959533909376836, 26.24890960531435624 ) ) ;
#95378=CARTESIAN_POINT ( 'NONE',  ( -9.564922557961040184, 16.46253265017147172, 22.91775706135233648 ) ) ;
#95380=CARTESIAN_POINT ( 'NONE',  ( -5.049401038298153566, 19.05341960407611168, 50.20724293864770260 ) ) ;
#95382=CARTESIAN_POINT ( 'NONE',  ( -13.89961937509977652, 13.97604488694528158, 75.62390960531438111 ) ) ;
#95383=CARTESIAN_POINT ( 'NONE',  ( -17.72517630440429315, 5.500000000000143885, 65.92175719257210176 ) ) ;
#95385=CARTESIAN_POINT ( 'NONE',  ( -19.05341960407617563, 5.049401038297882671, 23.54275706135233648 ) ) ;
#95386=CARTESIAN_POINT ( 'NONE',  ( -4.483927247898539470, -16.52544592524342804, 37.29057627198102409 ) ) ;
#95387=CARTESIAN_POINT ( 'NONE',  ( 13.97604488694527802, 13.89961937509977652, 49.37390960531434558 ) ) ;
#95388=CARTESIAN_POINT ( 'NONE',  ( 16.51473224551069308, 9.474510206698969483, 99.16557627198102409 ) ) ;
#95389=CARTESIAN_POINT ( 'NONE',  ( -18.62759615963255300, -10.81492255796106328, 74.16775706135231871 ) ) ;
#95390=CARTESIAN_POINT ( 'NONE',  ( -16.51473224551069308, -9.474510206698971260, 56.66557627198103120 ) ) ;
#95391=CARTESIAN_POINT ( 'NONE',  ( -5.719274019375665041, -21.55341960407619695, 64.79275706135234714 ) ) ;
#95392=CARTESIAN_POINT ( 'NONE',  ( 13.89961937509977652, -13.97604488694527269, 113.1239096053143527 ) ) ;
#95393=CARTESIAN_POINT ( 'NONE',  ( 9.564922557960805705, 16.46253265017160317, 34.58224293864770260 ) ) ;
#95394=CARTESIAN_POINT ( 'NONE',  ( -21.55341960407619339, 5.719274019375674811, 28.54275706135234358 ) ) ;
#95395=CARTESIAN_POINT ( 'NONE',  ( 5.153800228976615827, -19.02544592524334988, 50.20942372801897591 ) ) ;
#95396=CARTESIAN_POINT ( 'NONE',  ( 13.89961937509977652, -13.97604488694527269, 28.12390960531435624 ) ) ;
#95397=CARTESIAN_POINT ( 'NONE',  ( 5.049401038298161559, -19.05341960407611168, 57.70724293864769550 ) ) ;
#95398=CARTESIAN_POINT ( 'NONE',  ( 9.564922557961047289, -16.46253265017146816, 110.4177570613523471 ) ) ;
#95399=CARTESIAN_POINT ( 'NONE',  ( -12.06949235617756955, 12.14591786802309770, 80.62390960531438111 ) ) ;
#95400=CARTESIAN_POINT ( 'NONE',  ( -18.67979575497178146, -10.72451020669898902, 31.66557627198102054 ) ) ;
#95401=CARTESIAN_POINT ( 'NONE',  ( -9.564922557961040184, 16.46253265017147172, 102.9177570613523329 ) ) ;
#95402=CARTESIAN_POINT ( 'NONE',  ( -10.72451020669898014, 18.67979575497178502, 100.4155762719810241 ) ) ;
#95403=CARTESIAN_POINT ( 'NONE',  ( 10.81492255796106328, -18.62759615963255655, 60.41775706135235424 ) ) ;
#95404=CARTESIAN_POINT ( 'NONE',  ( 8.224510206698742110, 14.34966873604972548, 62.08442372801901143 ) ) ;
#95405=CARTESIAN_POINT ( 'NONE',  ( -16.52544592524335698, -4.483927247898792601, 53.95942372801900433 ) ) ;
#95406=CARTESIAN_POINT ( 'NONE',  ( 10.81492255796078972, 18.62759615963270932, 54.58224293864769550 ) ) ;
#95407=CARTESIAN_POINT ( 'NONE',  ( -16.51473224551069308, -9.474510206698971260, 41.66557627198103120 ) ) ;
#95408=CARTESIAN_POINT ( 'NONE',  ( 14.29746914071037800, 8.314922557961029526, 71.66775706135234714 ) ) ;
#95410=CARTESIAN_POINT ( 'NONE',  ( 15.80617190586746368, 15.72974639402197994, 99.37390960531436690 ) ) ;
#95411=CARTESIAN_POINT ( 'NONE',  ( -8.224510206698948167, 14.34966873604960824, 50.41557627198103120 ) ) ;
#95412=CARTESIAN_POINT ( 'NONE',  ( 13.97604488694527802, 13.89961937509977652, 69.37390960531436690 ) ) ;
#95413=CARTESIAN_POINT ( 'NONE',  ( 14.29746914071037800, 8.314922557961029526, 81.66775706135236135 ) ) ;
#95414=CARTESIAN_POINT ( 'NONE',  ( 9.564922557961047289, -16.46253265017146816, 110.4177570613523471 ) ) ;
#95415=CARTESIAN_POINT ( 'NONE',  ( 18.67979575497178502, 10.72451020669898547, 109.1655762719810383 ) ) ;
#95416=CARTESIAN_POINT ( 'NONE',  ( -8.224510206698948167, 14.34966873604960824, 50.41557627198103120 ) ) ;
#95418=CARTESIAN_POINT ( 'NONE',  ( 19.35633801406909171, -5.499999999999671374, 91.63373818172765084 ) ) ;
#95419=CARTESIAN_POINT ( 'NONE',  ( -15.80617190586745835, -15.72974639402198527, 91.87390960531436690 ) ) ;
#95421=CARTESIAN_POINT ( 'NONE',  ( -16.53943276465976808, 0.05219959533911058130, 26.24890960531435624 ) ) ;
#95422=VERTEX_POINT ( 'NONE', #6140 ) ;
#95424=CARTESIAN_POINT ( 'NONE',  ( 21.55341960407610458, 5.719274019375980345, 103.9572429386476813 ) ) ;
#95425=CARTESIAN_POINT ( 'NONE',  ( 19.05341960407611168, 5.049401038298154454, 108.9572429386477097 ) ) ;
#95426=CARTESIAN_POINT ( 'NONE',  ( -21.53943276465977519, 0.05219959533907696930, 116.2489096053143669 ) ) ;
#95427=CARTESIAN_POINT ( 'NONE',  ( -8.314922557960811034, -14.29746914071050412, 47.08224293864770260 ) ) ;
#95428=CARTESIAN_POINT ( 'NONE',  ( -8.314922557961024197, 14.29746914071037800, 47.91775706135234714 ) ) ;
#95429=CARTESIAN_POINT ( 'NONE',  ( 19.05341960407611168, 5.049401038298154454, 48.95724293864768129 ) ) ;
#95430=CARTESIAN_POINT ( 'NONE',  ( -9.564922557961040184, 16.46253265017147172, 47.91775706135233293 ) ) ;
#95431=CARTESIAN_POINT ( 'NONE',  ( 0.05219959533909260263, 19.03943276465977164, 84.99890960531436690 ) ) ;
#95433=CARTESIAN_POINT ( 'NONE',  ( -21.53943276465977519, 0.05219959533907696930, 36.24890960531435979 ) ) ;
#95435=CARTESIAN_POINT ( 'NONE',  ( -4.483927247898782831, 16.52544592524335698, 27.70942372801901854 ) ) ;
#95436=CARTESIAN_POINT ( 'NONE',  ( 13.89961937509957401, 13.97604488694547697, 66.87609039468567573 ) ) ;
#95437=CARTESIAN_POINT ( 'NONE',  ( 10.72451020669898902, -18.67979575497178502, 102.9155762719810383 ) ) ;
#95438=CARTESIAN_POINT ( 'NONE',  ( -12.14591786802309592, -12.06949235617757132, 36.87390960531435979 ) ) ;
#95439=CARTESIAN_POINT ( 'NONE',  ( -16.51473224551069308, -9.474510206698971260, 76.66557627198103830 ) ) ;
#95440=CARTESIAN_POINT ( 'NONE',  ( -18.67979575497178146, -10.72451020669898902, 56.66557627198103830 ) ) ;
#95441=CARTESIAN_POINT ( 'NONE',  ( -5.823673210054116645, -21.52544592524344225, 92.29057627198103830 ) ) ;
#95442=CARTESIAN_POINT ( 'NONE',  ( 0.05219959533934541429, -16.53943276465976808, 20.00109039468568639 ) ) ;
#95443=CARTESIAN_POINT ( 'NONE',  ( 16.51473224551069308, 9.474510206698969483, 114.1655762719810241 ) ) ;
#95444=CARTESIAN_POINT ( 'NONE',  ( -21.52544592524334988, -5.823673210054445271, 93.95942372801903275 ) ) ;
#95445=CARTESIAN_POINT ( 'NONE',  ( -5.049401038298153566, 19.05341960407611168, 90.20724293864766707 ) ) ;
#95446=CARTESIAN_POINT ( 'NONE',  ( -13.89961937509977652, 13.97604488694528158, 25.62390960531434558 ) ) ;
#95447=CARTESIAN_POINT ( 'NONE',  ( -0.05219959533909027116, -19.03943276465977164, 77.49890960531435269 ) ) ;
#95448=CARTESIAN_POINT ( 'NONE',  ( -12.14591786802309592, -12.06949235617757132, 106.8739096053143811 ) ) ;
#95449=CARTESIAN_POINT ( 'NONE',  ( -5.049401038298153566, 19.05341960407611168, 60.20724293864768129 ) ) ;
#95450=CARTESIAN_POINT ( 'NONE',  ( 16.55341960407618274, -4.379528057220086978, 26.04275706135235779 ) ) ;
#95452=CARTESIAN_POINT ( 'NONE',  ( 19.03943276465977164, -0.05219959533909143690, 73.74890960531435269 ) ) ;
#95453=CARTESIAN_POINT ( 'NONE',  ( -18.67979575497193778, 10.72451020669871902, 103.3344237280190043 ) ) ;
#95454=CARTESIAN_POINT ( 'NONE',  ( 9.474510206698971260, -16.51473224551069308, 112.9155762719810383 ) ) ;
#95455=CARTESIAN_POINT ( 'NONE',  ( -16.55341960407617563, 4.379528057220093196, 93.54275706135234714 ) ) ;
#95457=CARTESIAN_POINT ( 'NONE',  ( 5.153800228976615827, -19.02544592524334988, 65.20942372801900433 ) ) ;
#95458=CARTESIAN_POINT ( 'NONE',  ( -16.46253265017146816, -9.564922557961047289, 24.16775706135233648 ) ) ;
#95460=CARTESIAN_POINT ( 'NONE',  ( -0.05219959533909027116, -19.03943276465977164, 27.49890960531435624 ) ) ;
#95461=CARTESIAN_POINT ( 'NONE',  ( -14.29746914071049879, 8.314922557960819915, 35.83224293864768839 ) ) ;
#95463=CARTESIAN_POINT ( 'NONE',  ( 0.05219959533934541429, -16.53943276465976808, 105.0010903946856757 ) ) ;
#95465=CARTESIAN_POINT ( 'NONE',  ( 8.314922557961029526, -14.29746914071037800, 85.41775706135236135 ) ) ;
#95466=CARTESIAN_POINT ( 'NONE',  ( -13.97604488694527625, -13.89961937509977652, 31.87390960531435979 ) ) ;
#95467=CARTESIAN_POINT ( 'NONE',  ( 0.05219959533937995610, -21.53943276465977519, 95.00109039468568994 ) ) ;
#95468=CARTESIAN_POINT ( 'NONE',  ( 19.02544592524334988, 5.153800228976608722, 96.45942372801897591 ) ) ;
#95469=CARTESIAN_POINT ( 'NONE',  ( 15.80617190586769283, -15.72974639402175789, 75.62609039468567573 ) ) ;
#95470=CARTESIAN_POINT ( 'NONE',  ( -13.89961937509957401, -13.97604488694547875, 54.37609039468565442 ) ) ;
#95471=CARTESIAN_POINT ( 'NONE',  ( 13.97604488694527802, 13.89961937509977652, 74.37390960531436690 ) ) ;
#95472=CARTESIAN_POINT ( 'NONE',  ( -19.03943276465977164, 0.05219959533909376836, 71.24890960531435269 ) ) ;
#95473=CARTESIAN_POINT ( 'NONE',  ( 17.48853670773246449, 5.747243402303058524, 73.83328700250008580 ) ) ;
#95474=CARTESIAN_POINT ( 'NONE',  ( -4.483927247898539470, -16.52544592524342804, 67.29057627198103830 ) ) ;
#95475=CARTESIAN_POINT ( 'NONE',  ( 15.80617190586746368, 15.72974639402197994, 64.37390960531435269 ) ) ;
#95476=CARTESIAN_POINT ( 'NONE',  ( -19.02544592524342804, 5.153800228976336051, 41.04057627198103120 ) ) ;
#95477=CARTESIAN_POINT ( 'NONE',  ( -0.05219959533907301413, -21.53943276465977519, 82.49890960531436690 ) ) ;
#95478=CARTESIAN_POINT ( 'NONE',  ( -16.52544592524335698, -4.483927247898792601, 73.95942372801901854 ) ) ;
#95479=EDGE_CURVE ( 'NONE', #10184, #165187, #2864, .T. ) ;
#95480=ORIENTED_EDGE ( 'NONE', *, *, #163889, .T. ) ;
#95481=CARTESIAN_POINT ( 'NONE',  ( 14.34966873604960469, 8.224510206698951720, 84.16557627198103830 ) ) ;
#95483=CARTESIAN_POINT ( 'NONE',  ( -8.314922557961024197, 14.29746914071037800, 37.91775706135235424 ) ) ;
#95484=CARTESIAN_POINT ( 'NONE',  ( -14.34966873604960291, -8.224510206698953496, 111.6655762719810525 ) ) ;
#95485=CARTESIAN_POINT ( 'NONE',  ( 19.05341960407617918, -5.049401038297876454, 71.04275706135234714 ) ) ;
#95486=CARTESIAN_POINT ( 'NONE',  ( 4.379528057220339221, -16.55341960407611168, 67.70724293864769550 ) ) ;
#95487=CARTESIAN_POINT ( 'NONE',  ( -10.72451020669870658, -18.67979575497194134, 39.58442372801901143 ) ) ;
#95488=CARTESIAN_POINT ( 'NONE',  ( -5.153800228976328057, -19.02544592524343514, 22.29057627198102765 ) ) ;
#95489=CARTESIAN_POINT ( 'NONE',  ( 5.719274019375991003, -21.55341960407610458, 107.7072429386476955 ) ) ;
#95491=CARTESIAN_POINT ( 'NONE',  ( -12.14591786802309592, -12.06949235617757132, 86.87390960531438111 ) ) ;
#95493=CARTESIAN_POINT ( 'NONE',  ( -9.564922557960796823, -16.46253265017161027, 52.08224293864768839 ) ) ;
#95495=CARTESIAN_POINT ( 'NONE',  ( 13.97604488694548053, -13.89961937509957401, 80.62609039468567573 ) ) ;
#95496=CARTESIAN_POINT ( 'NONE',  ( 10.72451020669871369, 18.67979575497193778, 42.08442372801901854 ) ) ;
#95497=CARTESIAN_POINT ( 'NONE',  ( -5.049401038298153566, 19.05341960407611168, 75.20724293864769550 ) ) ;
#95498=CARTESIAN_POINT ( 'NONE',  ( 13.97604488694548053, -13.89961937509957401, 60.62609039468564731 ) ) ;
#95499=CARTESIAN_POINT ( 'NONE',  ( -16.46253265017160317, 9.564922557960807481, 45.83224293864769550 ) ) ;
#95500=CARTESIAN_POINT ( 'NONE',  ( 16.55341960407611168, 4.379528057220329451, 58.95724293864770971 ) ) ;
#95501=CARTESIAN_POINT ( 'NONE',  ( -16.52544592524342804, 4.483927247898546575, 61.04057627198103120 ) ) ;
#95502=CARTESIAN_POINT ( 'NONE',  ( 19.02544592524343514, -5.153800228976328945, 78.54057627198099567 ) ) ;
#95503=CARTESIAN_POINT ( 'NONE',  ( 15.72974639402199770, -15.80617190586745480, 103.1239096053143811 ) ) ;
#95504=CARTESIAN_POINT ( 'NONE',  ( -9.564922557960796823, -16.46253265017161027, 72.08224293864770971 ) ) ;
#95505=CARTESIAN_POINT ( 'NONE',  ( -15.72974639402197994, 15.80617190586746368, 85.62390960531436690 ) ) ;
#95506=CARTESIAN_POINT ( 'NONE',  ( 10.72451020669871369, 18.67979575497193778, 107.0844237280190043 ) ) ;
#95507=CARTESIAN_POINT ( 'NONE',  ( -9.564922557960796823, -16.46253265017161027, 32.08224293864769550 ) ) ;
#95508=CARTESIAN_POINT ( 'NONE',  ( 0.05219959533934541429, -16.53943276465976808, 105.0010903946856757 ) ) ;
#95509=CARTESIAN_POINT ( 'NONE',  ( -14.34966873604960291, -8.224510206698953496, 91.66557627198103830 ) ) ;
#95510=CARTESIAN_POINT ( 'NONE',  ( 9.564922557961047289, -16.46253265017146816, 100.4177570613523329 ) ) ;
#95512=CARTESIAN_POINT ( 'NONE',  ( -5.823673210054431948, 21.52544592524334988, 37.70942372801900433 ) ) ;
#95513=CARTESIAN_POINT ( 'NONE',  ( 13.89961937509957401, 13.97604488694547697, 56.87609039468564731 ) ) ;
#95514=CARTESIAN_POINT ( 'NONE',  ( -14.34966873604960291, -8.224510206698953496, 26.66557627198103475 ) ) ;
#95515=CARTESIAN_POINT ( 'NONE',  ( -15.80617190586745835, -15.72974639402198527, 66.87390960531436690 ) ) ;
#95516=CARTESIAN_POINT ( 'NONE',  ( -16.51473224551069308, -9.474510206698971260, 96.66557627198102409 ) ) ;
#95517=CARTESIAN_POINT ( 'NONE',  ( -4.379528057220328563, 16.55341960407611168, 60.20724293864768839 ) ) ;
#95518=CARTESIAN_POINT ( 'NONE',  ( 13.97604488694527802, 13.89961937509977652, 34.37390960531436690 ) ) ;
#95519=CARTESIAN_POINT ( 'NONE',  ( -16.46253265017160317, 9.564922557960807481, 30.83224293864769550 ) ) ;
#95520=CARTESIAN_POINT ( 'NONE',  ( -5.049401038297874678, -19.05341960407617918, 24.79275706135233648 ) ) ;
#95521=CARTESIAN_POINT ( 'NONE',  ( 16.55341960407618274, -4.379528057220086978, 91.04275706135236135 ) ) ;
#95522=CARTESIAN_POINT ( 'NONE',  ( -18.67979575497193778, 10.72451020669871902, 48.33442372801902565 ) ) ;
#95523=CARTESIAN_POINT ( 'NONE',  ( -16.55341960407617563, 4.379528057220093196, 48.54275706135234714 ) ) ;
#95524=CARTESIAN_POINT ( 'NONE',  ( -18.62759615963270932, 10.81492255796079327, 25.83224293864769194 ) ) ;
#95525=CARTESIAN_POINT ( 'NONE',  ( -5.049401038298153566, 19.05341960407611168, 50.20724293864770260 ) ) ;
#95526=CARTESIAN_POINT ( 'NONE',  ( 21.55341960407619695, -5.719274019375665929, 101.0427570613523756 ) ) ;
#95527=CARTESIAN_POINT ( 'NONE',  ( 0.05219959533909260263, 19.03943276465977164, 79.99890960531436690 ) ) ;
#95528=CARTESIAN_POINT ( 'NONE',  ( 8.314922557961029526, -14.29746914071037800, 65.41775706135234714 ) ) ;
#95529=CARTESIAN_POINT ( 'NONE',  ( -12.14591786802309592, -12.06949235617757132, 101.8739096053143811 ) ) ;
#95530=CARTESIAN_POINT ( 'NONE',  ( 8.224510206698742110, 14.34966873604972548, 112.0844237280190185 ) ) ;
#95531=CARTESIAN_POINT ( 'NONE',  ( -17.97182807773875624, 5.499999999999873879, 38.53038844047286915 ) ) ;
#95532=CARTESIAN_POINT ( 'NONE',  ( 5.719274019375673035, 21.55341960407619339, 67.29275706135234714 ) ) ;
#95533=CARTESIAN_POINT ( 'NONE',  ( -16.46253265017160317, 9.564922557960807481, 85.83224293864769550 ) ) ;
#95534=CARTESIAN_POINT ( 'NONE',  ( -0.05219959533909027116, -19.03943276465977164, 72.49890960531435269 ) ) ;
#95535=CARTESIAN_POINT ( 'NONE',  ( 9.564922557960805705, 16.46253265017160317, 104.5822429386476955 ) ) ;
#95536=CARTESIAN_POINT ( 'NONE',  ( -8.314922557960811034, -14.29746914071050412, 62.08224293864769550 ) ) ;
#95537=CARTESIAN_POINT ( 'NONE',  ( 14.34966873604960469, 8.224510206698951720, 24.16557627198103120 ) ) ;
#95538=CARTESIAN_POINT ( 'NONE',  ( -4.379528057220328563, 16.55341960407611168, 35.20724293864768839 ) ) ;
#95540=CARTESIAN_POINT ( 'NONE',  ( -16.51473224551082808, 9.474510206698731452, 33.33442372801899722 ) ) ;
#95541=CARTESIAN_POINT ( 'NONE',  ( 16.46253265017160672, -9.564922557960803928, 73.33224293864769550 ) ) ;
#95542=CARTESIAN_POINT ( 'NONE',  ( -5.049401038297874678, -19.05341960407617918, 54.79275706135234003 ) ) ;
#95545=CARTESIAN_POINT ( 'NONE',  ( 13.89961937509957401, 13.97604488694547697, 86.87609039468567573 ) ) ;
#95546=CARTESIAN_POINT ( 'NONE',  ( -8.314922557961024197, 14.29746914071037800, 82.91775706135234714 ) ) ;
#95547=CARTESIAN_POINT ( 'NONE',  ( 17.50000000000002132, 5.622605283950872668, 93.81207310596117566 ) ) ;
#95548=CARTESIAN_POINT ( 'NONE',  ( 19.05341960407611168, 5.049401038298154454, 98.95724293864766707 ) ) ;
#95549=CARTESIAN_POINT ( 'NONE',  ( -21.53943276465977519, -0.05219959533937600094, 28.75109039468567929 ) ) ;
#95550=CARTESIAN_POINT ( 'NONE',  ( 9.564922557961047289, -16.46253265017146816, 90.41775706135234714 ) ) ;
#95552=CARTESIAN_POINT ( 'NONE',  ( 19.02544592524343514, -5.153800228976328945, 48.54057627198103120 ) ) ;
#95553=CARTESIAN_POINT ( 'NONE',  ( -5.049401038298153566, 19.05341960407611168, 105.2072429386476671 ) ) ;
#95554=CARTESIAN_POINT ( 'NONE',  ( -16.55341960407611168, -4.379528057220339221, 61.45724293864770260 ) ) ;
#95555=CARTESIAN_POINT ( 'NONE',  ( 9.564922557960805705, 16.46253265017160317, 44.58224293864769550 ) ) ;
#95556=CARTESIAN_POINT ( 'NONE',  ( 19.05341960407611168, 5.049401038298154454, 63.95724293864769550 ) ) ;
#95557=CARTESIAN_POINT ( 'NONE',  ( 13.97604488694548053, -13.89961937509957401, 70.62609039468567573 ) ) ;
#95558=CARTESIAN_POINT ( 'NONE',  ( -0.05219959533936034679, 19.03943276465977164, 27.50109039468566507 ) ) ;
#95559=CARTESIAN_POINT ( 'NONE',  ( -19.03943276465977164, 0.05219959533909376836, 66.24890960531436690 ) ) ;
#95560=CARTESIAN_POINT ( 'NONE',  ( 5.719274019375991003, -21.55341960407610458, 72.70724293864769550 ) ) ;
#95561=CARTESIAN_POINT ( 'NONE',  ( 0.05219959533910956823, 16.53943276465976808, 64.99890960531435269 ) ) ;
#95562=CARTESIAN_POINT ( 'NONE',  ( 13.97604488694548053, -13.89961937509957401, 40.62609039468564731 ) ) ;
#95564=CARTESIAN_POINT ( 'NONE',  ( -21.53943276465977519, 0.05219959533907696930, 41.24890960531435269 ) ) ;
#95566=CARTESIAN_POINT ( 'NONE',  ( -10.72451020669898014, 18.67979575497178502, 25.41557627198103120 ) ) ;
#95567=CARTESIAN_POINT ( 'NONE',  ( -19.03943276465977164, 0.05219959533909376836, 56.24890960531435979 ) ) ;
#95568=CARTESIAN_POINT ( 'NONE',  ( -9.474510206698964154, 16.51473224551069663, 40.41557627198103120 ) ) ;
#95569=CARTESIAN_POINT ( 'NONE',  ( -14.34966873604960291, -8.224510206698953496, 106.6655762719810383 ) ) ;
#95570=CARTESIAN_POINT ( 'NONE',  ( 21.55341960407610458, 5.719274019375980345, 113.9572429386477239 ) ) ;
#95571=CARTESIAN_POINT ( 'NONE',  ( 0.05219959533909260263, 19.03943276465977164, 114.9989096053143669 ) ) ;
#95572=CARTESIAN_POINT ( 'NONE',  ( 21.55341960407619695, -5.719274019375665929, 31.04275706135234714 ) ) ;
#95573=CARTESIAN_POINT ( 'NONE',  ( 19.02544592524343514, -5.153800228976328945, 23.54057627198102054 ) ) ;
#95574=CARTESIAN_POINT ( 'NONE',  ( -21.55341960407610458, -5.719274019375992779, 96.45724293864770971 ) ) ;
#95575=CARTESIAN_POINT ( 'NONE',  ( -0.05219959533936034679, 19.03943276465977164, 42.50109039468566152 ) ) ;
#95576=CARTESIAN_POINT ( 'NONE',  ( -0.05219959533909027116, -19.03943276465977164, 27.49890960531435624 ) ) ;
#95577=CARTESIAN_POINT ( 'NONE',  ( 5.049401038298161559, -19.05341960407611168, 27.70724293864769550 ) ) ;
#95579=CARTESIAN_POINT ( 'NONE',  ( 8.224510206698742110, 14.34966873604972548, 52.08442372801901854 ) ) ;
#95580=CARTESIAN_POINT ( 'NONE',  ( -8.224510206698948167, 14.34966873604960824, 115.4155762719810241 ) ) ;
#95581=CARTESIAN_POINT ( 'NONE',  ( 30.00000000000000000, -1.163414459189985801E-14, 92.50000000000000000 ) ) ;
#95582=CARTESIAN_POINT ( 'NONE',  ( 16.46253265017160672, -9.564922557960803928, 68.33224293864770971 ) ) ;
#95583=CARTESIAN_POINT ( 'NONE',  ( -16.52544592524342804, 4.483927247898546575, 111.0405762719810525 ) ) ;
#95585=CARTESIAN_POINT ( 'NONE',  ( 0.05219959533907565091, 21.53943276465977519, 39.99890960531436690 ) ) ;
#95586=CARTESIAN_POINT ( 'NONE',  ( 4.483927247898545687, 16.52544592524342804, 84.79057627198102409 ) ) ;
#95587=CARTESIAN_POINT ( 'NONE',  ( 0.05219959533934541429, -16.53943276465976808, 40.00109039468567573 ) ) ;
#95588=CARTESIAN_POINT ( 'NONE',  ( 5.823673210054444382, -21.52544592524334988, 85.20942372801901854 ) ) ;
#95590=CARTESIAN_POINT ( 'NONE',  ( 16.53943276465976808, 0.05219959533934440121, 106.2510903946856757 ) ) ;
#95591=CARTESIAN_POINT ( 'NONE',  ( -4.379528057220328563, 16.55341960407611168, 45.20724293864769550 ) ) ;
#95592=CARTESIAN_POINT ( 'NONE',  ( -19.03943276465977164, 0.05219959533909376836, 51.24890960531436690 ) ) ;
#95593=CARTESIAN_POINT ( 'NONE',  ( -10.81492255796105439, 18.62759615963255655, 97.91775706135236135 ) ) ;
#95594=CARTESIAN_POINT ( 'NONE',  ( -5.719274019375978568, 21.55341960407610458, 105.2072429386477097 ) ) ;
#95595=CARTESIAN_POINT ( 'NONE',  ( -5.719274019375665041, -21.55341960407619695, 74.79275706135234714 ) ) ;
#95596=CARTESIAN_POINT ( 'NONE',  ( -16.53943276465976808, -0.05219959533934237506, 38.75109039468567573 ) ) ;
#95597=CARTESIAN_POINT ( 'NONE',  ( 16.55341960407611168, 4.379528057220329451, 68.95724293864769550 ) ) ;
#95598=CARTESIAN_POINT ( 'NONE',  ( -0.05219959533937732626, 21.53943276465977519, 82.50109039468568994 ) ) ;
#95599=CARTESIAN_POINT ( 'NONE',  ( -16.53943276465976808, -0.05219959533934237506, 113.7510903946856757 ) ) ;
#95600=CARTESIAN_POINT ( 'NONE',  ( -16.81555441253555117, 7.025013491695454526, 115.6368544533426075 ) ) ;
#95602=CARTESIAN_POINT ( 'NONE',  ( -16.55341960407611168, -4.379528057220339221, 41.45724293864769550 ) ) ;
#95603=CARTESIAN_POINT ( 'NONE',  ( -8.224510206698735004, -14.34966873604973081, 79.58442372801903275 ) ) ;
#95604=CARTESIAN_POINT ( 'NONE',  ( -5.153800228976328057, -19.02544592524343514, 82.29057627198103830 ) ) ;
#95605=CARTESIAN_POINT ( 'NONE',  ( -9.474510206698964154, 16.51473224551069663, 105.4155762719810383 ) ) ;
#95606=CARTESIAN_POINT ( 'NONE',  ( 10.81492255796106328, -18.62759615963255655, 105.4177570613523613 ) ) ;
#95607=CARTESIAN_POINT ( 'NONE',  ( 14.29746914071037800, 8.314922557961029526, 101.6677570613523613 ) ) ;
#95608=CARTESIAN_POINT ( 'NONE',  ( -4.483927247898539470, -16.52544592524342804, 67.29057627198103830 ) ) ;
#95609=CARTESIAN_POINT ( 'NONE',  ( -9.474510206698964154, 16.51473224551069663, 85.41557627198102409 ) ) ;
#95610=ORIENTED_EDGE ( 'NONE', *, *, #106006, .T. ) ;
#95611=CARTESIAN_POINT ( 'NONE',  ( 12.14591786802327356, -12.06949235617739191, 25.62609039468567929 ) ) ;
#95612=CARTESIAN_POINT ( 'NONE',  ( 19.02544592524343514, -5.153800228976328945, 23.54057627198102054 ) ) ;
#95613=CARTESIAN_POINT ( 'NONE',  ( 5.049401038298161559, -19.05341960407611168, 92.70724293864769550 ) ) ;
#95614=CARTESIAN_POINT ( 'NONE',  ( 4.379528057220092307, 16.55341960407617563, 27.29275706135234358 ) ) ;
#95616=CARTESIAN_POINT ( 'NONE',  ( -9.474510206698720793, -16.51473224551083518, 19.58442372801899722 ) ) ;
#95617=CARTESIAN_POINT ( 'NONE',  ( 12.14591786802327356, -12.06949235617739191, 90.62609039468567573 ) ) ;
#95618=CARTESIAN_POINT ( 'NONE',  ( 16.46253265017146816, 9.564922557961045513, 101.6677570613523329 ) ) ;
#95619=CARTESIAN_POINT ( 'NONE',  ( 9.474510206698971260, -16.51473224551069308, 32.91557627198102409 ) ) ;
#95620=CARTESIAN_POINT ( 'NONE',  ( 0.05219959533934541429, -16.53943276465976808, 85.00109039468568994 ) ) ;
#95621=CARTESIAN_POINT ( 'NONE',  ( -4.379528057220086978, -16.55341960407618274, 64.79275706135234714 ) ) ;
#95622=CARTESIAN_POINT ( 'NONE',  ( 9.564922557960805705, 16.46253265017160317, 24.58224293864769194 ) ) ;
#95623=CARTESIAN_POINT ( 'NONE',  ( -9.474510206698720793, -16.51473224551083518, 64.58442372801900433 ) ) ;
#95624=CARTESIAN_POINT ( 'NONE',  ( 5.823673210054444382, -21.52544592524334988, 105.2094237280190328 ) ) ;
#95625=CARTESIAN_POINT ( 'NONE',  ( 19.05341960407611168, 5.049401038298154454, 43.95724293864769550 ) ) ;
#95626=CARTESIAN_POINT ( 'NONE',  ( -19.02544592524342804, 5.153800228976336051, 96.04057627198103830 ) ) ;
#95627=CARTESIAN_POINT ( 'NONE',  ( -14.29746914071049879, 8.314922557960819915, 90.83224293864769550 ) ) ;
#95628=CARTESIAN_POINT ( 'NONE',  ( -19.02544592524334988, -5.153800228976617603, 53.95942372801898301 ) ) ;
#95629=CARTESIAN_POINT ( 'NONE',  ( 21.52544592524344225, -5.823673210054117533, 48.54057627198103120 ) ) ;
#95630=CARTESIAN_POINT ( 'NONE',  ( 21.55341960407619695, -5.719274019375665929, 106.0427570613523471 ) ) ;
#95631=CARTESIAN_POINT ( 'NONE',  ( 16.51473224551069308, 9.474510206698969483, 94.16557627198103830 ) ) ;
#95632=CARTESIAN_POINT ( 'NONE',  ( 18.62759615963255655, 10.81492255796105972, 101.6677570613523613 ) ) ;
#95633=CARTESIAN_POINT ( 'NONE',  ( 0.05219959533907565091, 21.53943276465977519, 64.99890960531435269 ) ) ;
#95634=CARTESIAN_POINT ( 'NONE',  ( 9.474510206698971260, -16.51473224551069308, 97.91557627198102409 ) ) ;
#95635=CARTESIAN_POINT ( 'NONE',  ( -19.02544592524334988, -5.153800228976617603, 93.95942372801900433 ) ) ;
#95636=CARTESIAN_POINT ( 'NONE',  ( 16.46253265017160672, -9.564922557960803928, 113.3322429386476955 ) ) ;
#95637=CARTESIAN_POINT ( 'NONE',  ( -16.46253265017146816, -9.564922557961047289, 109.1677570613523471 ) ) ;
#95638=CARTESIAN_POINT ( 'NONE',  ( -14.34966873604960291, -8.224510206698953496, 111.6655762719810525 ) ) ;
#95639=CARTESIAN_POINT ( 'NONE',  ( -9.564922557960796823, -16.46253265017161027, 82.08224293864768129 ) ) ;
#95640=CARTESIAN_POINT ( 'NONE',  ( -5.823673210054116645, -21.52544592524344225, 77.29057627198102409 ) ) ;
#95641=CARTESIAN_POINT ( 'NONE',  ( 4.379528057220092307, 16.55341960407617563, 52.29275706135236135 ) ) ;
#95642=CARTESIAN_POINT ( 'NONE',  ( 21.52544592524334988, 5.823673210054432836, 46.45942372801901854 ) ) ;
#95643=CARTESIAN_POINT ( 'NONE',  ( -21.55341960407619339, 5.719274019375674811, 98.54275706135234714 ) ) ;
#95644=CARTESIAN_POINT ( 'NONE',  ( -8.314922557961024197, 14.29746914071037800, 92.91775706135236135 ) ) ;
#95645=CARTESIAN_POINT ( 'NONE',  ( -5.153800228976328057, -19.02544592524343514, 82.29057627198103830 ) ) ;
#95646=CARTESIAN_POINT ( 'NONE',  ( 16.52544592524342804, -4.483927247898539470, 88.54057627198103830 ) ) ;
#95647=CARTESIAN_POINT ( 'NONE',  ( 16.52544592524342804, -4.483927247898539470, 28.54057627198103120 ) ) ;
#95648=CARTESIAN_POINT ( 'NONE',  ( 19.05341960407617918, -5.049401038297876454, 66.04275706135233293 ) ) ;
#95649=CARTESIAN_POINT ( 'NONE',  ( -15.72974639402176322, -15.80617190586768395, 44.37609039468567573 ) ) ;
#95650=CARTESIAN_POINT ( 'NONE',  ( -19.03943276465977164, -0.05219959533935918106, 23.75109039468566152 ) ) ;
#95651=CARTESIAN_POINT ( 'NONE',  ( 4.379528057220339221, -16.55341960407611168, 97.70724293864772392 ) ) ;
#95652=CARTESIAN_POINT ( 'NONE',  ( -9.564922557960796823, -16.46253265017161027, 112.0822429386476955 ) ) ;
#95653=CARTESIAN_POINT ( 'NONE',  ( -12.06949235617756955, 12.14591786802309770, 25.62390960531435624 ) ) ;
#95654=CARTESIAN_POINT ( 'NONE',  ( -10.72451020669870658, -18.67979575497194134, 79.58442372801903275 ) ) ;
#95655=CARTESIAN_POINT ( 'NONE',  ( -16.53943276465976808, -0.05219959533934237506, 53.75109039468568994 ) ) ;
#95656=CARTESIAN_POINT ( 'NONE',  ( 12.14591786802327356, -12.06949235617739191, 100.6260903946857184 ) ) ;
#95657=CARTESIAN_POINT ( 'NONE',  ( 15.72974639402176855, 15.80617190586768217, 56.87609039468568994 ) ) ;
#95659=CARTESIAN_POINT ( 'NONE',  ( -15.72974639402176322, -15.80617190586768395, 34.37609039468568284 ) ) ;
#95660=CARTESIAN_POINT ( 'NONE',  ( 14.29746914071049879, -8.314922557960816363, 103.3322429386476955 ) ) ;
#95662=CARTESIAN_POINT ( 'NONE',  ( 5.153800228976335163, 19.02544592524342804, 29.79057627198102409 ) ) ;
#95663=CARTESIAN_POINT ( 'NONE',  ( 14.29746914071049879, -8.314922557960816363, 63.33224293864770260 ) ) ;
#95664=CARTESIAN_POINT ( 'NONE',  ( -5.049401038298153566, 19.05341960407611168, 70.20724293864769550 ) ) ;
#95665=CARTESIAN_POINT ( 'NONE',  ( -8.314922557961024197, 14.29746914071037800, 102.9177570613523756 ) ) ;
#95666=CARTESIAN_POINT ( 'NONE',  ( 19.02544592524343514, -5.153800228976328945, 33.54057627198102409 ) ) ;
#95667=CARTESIAN_POINT ( 'NONE',  ( 21.55341960407610458, 5.719274019375980345, 53.95724293864770260 ) ) ;
#95668=CARTESIAN_POINT ( 'NONE',  ( -8.224510206698948167, 14.34966873604960824, 90.41557627198103830 ) ) ;
#95670=CARTESIAN_POINT ( 'NONE',  ( -5.719274019375978568, 21.55341960407610458, 95.20724293864769550 ) ) ;
#95671=CARTESIAN_POINT ( 'NONE',  ( 13.89961937509977652, -13.97604488694527269, 98.12390960531433848 ) ) ;
#95672=CARTESIAN_POINT ( 'NONE',  ( 16.46253265017160672, -9.564922557960803928, 53.33224293864768839 ) ) ;
#95673=CARTESIAN_POINT ( 'NONE',  ( 13.97604488694548053, -13.89961937509957401, 95.62609039468563310 ) ) ;
#95675=CARTESIAN_POINT ( 'NONE',  ( -5.719274019375978568, 21.55341960407610458, 50.20724293864769550 ) ) ;
#95676=CARTESIAN_POINT ( 'NONE',  ( -10.81492255796105439, 18.62759615963255655, 67.91775706135234714 ) ) ;
#95677=CARTESIAN_POINT ( 'NONE',  ( -0.05219959533909027116, -19.03943276465977164, 52.49890960531436690 ) ) ;
#95678=CARTESIAN_POINT ( 'NONE',  ( 16.51473224551069308, 9.474510206698969483, 89.16557627198103830 ) ) ;
#95679=CARTESIAN_POINT ( 'NONE',  ( 16.55341960407618274, -4.379528057220086978, 66.04275706135236135 ) ) ;
#95680=CARTESIAN_POINT ( 'NONE',  ( -21.55341960407619339, 5.719274019375674811, 38.54275706135234714 ) ) ;
#95681=CARTESIAN_POINT ( 'NONE',  ( -21.52544592524334988, -5.823673210054445271, 83.95942372801900433 ) ) ;
#95682=CARTESIAN_POINT ( 'NONE',  ( -18.62759615963270932, 10.81492255796079327, 95.83224293864770971 ) ) ;
#95683=CARTESIAN_POINT ( 'NONE',  ( -21.52544592524334988, -5.823673210054445271, 38.95942372801901854 ) ) ;
#95684=CARTESIAN_POINT ( 'NONE',  ( 8.224510206698742110, 14.34966873604972548, 67.08442372801901854 ) ) ;
#95685=CARTESIAN_POINT ( 'NONE',  ( 18.67979575497178502, 10.72451020669898547, 64.16557627198102409 ) ) ;
#95686=CARTESIAN_POINT ( 'NONE',  ( -13.89961937509957401, -13.97604488694547875, 29.37609039468565797 ) ) ;
#95687=CARTESIAN_POINT ( 'NONE',  ( 13.89961937509977652, -13.97604488694527269, 63.12390960531435979 ) ) ;
#95688=CARTESIAN_POINT ( 'NONE',  ( 16.55341960407611168, 4.379528057220329451, 28.95724293864769905 ) ) ;
#95690=CARTESIAN_POINT ( 'NONE',  ( -16.51473224551069308, -9.474510206698971260, 106.6655762719810383 ) ) ;
#95691=LINE ( 'NONE', #80518, #89499 ) ;
#95692=CARTESIAN_POINT ( 'NONE',  ( -13.97604488694547697, 13.89961937509957934, 78.12609039468567573 ) ) ;
#95693=CARTESIAN_POINT ( 'NONE',  ( 18.62759615963271287, -10.81492255796078972, 58.33224293864768839 ) ) ;
#95694=CARTESIAN_POINT ( 'NONE',  ( 4.483927247898545687, 16.52544592524342804, 39.79057627198103830 ) ) ;
#95695=CARTESIAN_POINT ( 'NONE',  ( -19.05341960407617563, 5.049401038297882671, 113.5427570613523471 ) ) ;
#95696=CARTESIAN_POINT ( 'NONE',  ( -5.153800228976328057, -19.02544592524343514, 32.29057627198102409 ) ) ;
#95697=CARTESIAN_POINT ( 'NONE',  ( 16.46253265017146816, 9.564922557961045513, 106.6677570613523471 ) ) ;
#95698=CARTESIAN_POINT ( 'NONE',  ( 18.62759615963271287, -10.81492255796078972, 93.33224293864769550 ) ) ;
#95699=CARTESIAN_POINT ( 'NONE',  ( 16.46253265017146816, 9.564922557961045513, 66.66775706135233293 ) ) ;
#95700=CARTESIAN_POINT ( 'NONE',  ( 8.224510206698742110, 14.34966873604972548, 82.08442372801901854 ) ) ;
#95701=CARTESIAN_POINT ( 'NONE',  ( 19.03943276465977164, -0.05219959533909143690, 68.74890960531436690 ) ) ;
#95702=CARTESIAN_POINT ( 'NONE',  ( 8.314922557960818139, 14.29746914071049879, 79.58224293864769550 ) ) ;
#95703=CARTESIAN_POINT ( 'NONE',  ( -19.05341960407611168, -5.049401038298163336, 41.45724293864769550 ) ) ;
#95704=CARTESIAN_POINT ( 'NONE',  ( 16.53943276465976808, -0.05219959533910856209, 53.74890960531437401 ) ) ;
#95707=CARTESIAN_POINT ( 'NONE',  ( 16.55341960407611168, 4.379528057220329451, 28.95724293864769905 ) ) ;
#95708=CARTESIAN_POINT ( 'NONE',  ( -9.474510206698964154, 16.51473224551069663, 80.41557627198103830 ) ) ;
#95709=CARTESIAN_POINT ( 'NONE',  ( 17.50000000000002132, 5.499999999999984013, 98.78230962303568674 ) ) ;
#95710=CARTESIAN_POINT ( 'NONE',  ( -9.474510206698720793, -16.51473224551083518, 34.58442372801899722 ) ) ;
#95711=CARTESIAN_POINT ( 'NONE',  ( 14.34966873604972726, -8.224510206698740333, 40.83442372801901854 ) ) ;
#95713=CARTESIAN_POINT ( 'NONE',  ( 5.719274019375991003, -21.55341960407610458, 67.70724293864769550 ) ) ;
#95714=CARTESIAN_POINT ( 'NONE',  ( 5.153800228976615827, -19.02544592524334988, 25.20942372801900433 ) ) ;
#95715=CARTESIAN_POINT ( 'NONE',  ( 16.51473224551069308, 9.474510206698969483, 79.16557627198103830 ) ) ;
#95717=CARTESIAN_POINT ( 'NONE',  ( 5.049401038298161559, -19.05341960407611168, 112.7072429386476813 ) ) ;
#95718=CARTESIAN_POINT ( 'NONE',  ( 21.53943276465977519, 0.05219959533937863772, 36.25109039468567573 ) ) ;
#95720=CARTESIAN_POINT ( 'NONE',  ( -16.52544592524342804, 4.483927247898546575, 106.0405762719810525 ) ) ;
#95721=CARTESIAN_POINT ( 'NONE',  ( -10.72451020669898014, 18.67979575497178502, 100.4155762719810241 ) ) ;
#95722=CARTESIAN_POINT ( 'NONE',  ( -13.89961937509977652, 13.97604488694528158, 75.62390960531438111 ) ) ;
#95724=CARTESIAN_POINT ( 'NONE',  ( 18.67979575497194134, -10.72451020669871369, 25.83442372801901499 ) ) ;
#95725=VERTEX_POINT ( 'NONE', #44475 ) ;
#95726=CARTESIAN_POINT ( 'NONE',  ( -16.46253265017160317, 9.564922557960807481, 85.83224293864769550 ) ) ;
#95728=CARTESIAN_POINT ( 'NONE',  ( 16.46253265017160672, -9.564922557960803928, 28.33224293864769550 ) ) ;
#95729=CARTESIAN_POINT ( 'NONE',  ( -0.05219959533936034679, 19.03943276465977164, 112.5010903946856757 ) ) ;
#95731=CARTESIAN_POINT ( 'NONE',  ( -14.29746914071049879, 8.314922557960819915, 110.8322429386476955 ) ) ;
#95732=CARTESIAN_POINT ( 'NONE',  ( -21.55341960407619339, 5.719274019375674811, 88.54275706135236135 ) ) ;
#95733=CARTESIAN_POINT ( 'NONE',  ( 19.02544592524343514, -5.153800228976328945, 73.54057627198103830 ) ) ;
#95734=CARTESIAN_POINT ( 'NONE',  ( -21.53943276465977519, -0.05219959533937600094, 48.75109039468568284 ) ) ;
#95735=CARTESIAN_POINT ( 'NONE',  ( -15.72974639402176322, -15.80617190586768395, 24.37609039468567573 ) ) ;
#95737=CARTESIAN_POINT ( 'NONE',  ( 16.46253265017160672, -9.564922557960803928, 83.33224293864768129 ) ) ;
#95739=CARTESIAN_POINT ( 'NONE',  ( 0.05219959533934541429, -16.53943276465976808, 45.00109039468568284 ) ) ;
#95740=CARTESIAN_POINT ( 'NONE',  ( -5.823673210054116645, -21.52544592524344225, 37.29057627198102409 ) ) ;
#95741=CARTESIAN_POINT ( 'NONE',  ( -5.719274019375665041, -21.55341960407619695, 74.79275706135234714 ) ) ;
#95744=CARTESIAN_POINT ( 'NONE',  ( 5.049401038297881783, 19.05341960407617563, 107.2927570613523187 ) ) ;
#95745=CARTESIAN_POINT ( 'NONE',  ( 19.05341960407611168, 5.049401038298154454, 53.95724293864770260 ) ) ;
#95746=CARTESIAN_POINT ( 'NONE',  ( 19.02544592524343514, -5.153800228976328945, 88.54057627198102409 ) ) ;
#95747=CARTESIAN_POINT ( 'NONE',  ( -12.14591786802309592, -12.06949235617757132, 101.8739096053143811 ) ) ;
#95748=CARTESIAN_POINT ( 'NONE',  ( -16.55341960407611168, -4.379528057220339221, 106.4572429386477097 ) ) ;
#95749=CARTESIAN_POINT ( 'NONE',  ( -5.153800228976328057, -19.02544592524343514, 107.2905762719810383 ) ) ;
#95750=CARTESIAN_POINT ( 'NONE',  ( -14.29746914071037622, -8.314922557961029526, 84.16775706135234714 ) ) ;
#95751=CARTESIAN_POINT ( 'NONE',  ( -12.06949235617756955, 12.14591786802309770, 60.62390960531437401 ) ) ;
#95752=CARTESIAN_POINT ( 'NONE',  ( 0.05219959533909260263, 19.03943276465977164, 59.99890960531436690 ) ) ;
#95753=CARTESIAN_POINT ( 'NONE',  ( -15.80617190586768217, 15.72974639402176855, 83.12609039468568994 ) ) ;
#95754=CARTESIAN_POINT ( 'NONE',  ( -21.53943276465977519, -0.05219959533937600094, 73.75109039468567573 ) ) ;
#95755=CARTESIAN_POINT ( 'NONE',  ( 0.05219959533936267826, -19.03943276465977164, 95.00109039468567573 ) ) ;
#95756=CARTESIAN_POINT ( 'NONE',  ( 16.52544592524342804, -4.483927247898539470, 58.54057627198103120 ) ) ;
#95757=CARTESIAN_POINT ( 'NONE',  ( 18.67979575497178502, 10.72451020669898547, 109.1655762719810383 ) ) ;
#95758=CARTESIAN_POINT ( 'NONE',  ( 10.72451020669898902, -18.67979575497178502, 62.91557627198102409 ) ) ;
#95761=CARTESIAN_POINT ( 'NONE',  ( -16.46253265017160317, 9.564922557960807481, 70.83224293864770971 ) ) ;
#95762=CARTESIAN_POINT ( 'NONE',  ( 4.379528057220339221, -16.55341960407611168, 42.70724293864770260 ) ) ;
#95763=CARTESIAN_POINT ( 'NONE',  ( 16.55341960407611168, 4.379528057220329451, 23.95724293864769550 ) ) ;
#95764=CARTESIAN_POINT ( 'NONE',  ( -14.34966873604972548, 8.224510206698743886, 78.33442372801901854 ) ) ;
#95765=CARTESIAN_POINT ( 'NONE',  ( -13.97604488694547697, 13.89961937509957934, 43.12609039468566152 ) ) ;
#95767=CARTESIAN_POINT ( 'NONE',  ( 16.46253265017160672, -9.564922557960803928, 98.33224293864769550 ) ) ;
#95768=CARTESIAN_POINT ( 'NONE',  ( 16.52544592524342804, -4.483927247898539470, 58.54057627198103120 ) ) ;
#95769=CARTESIAN_POINT ( 'NONE',  ( 16.19135201231366139, -7.376712067591918220, 102.3131914594797252 ) ) ;
#95770=CARTESIAN_POINT ( 'NONE',  ( -19.03943276465977164, 0.05219959533909376836, 111.2489096053143669 ) ) ;
#95771=CARTESIAN_POINT ( 'NONE',  ( -21.55341960407610458, -5.719274019375992779, 51.45724293864770260 ) ) ;
#95773=CARTESIAN_POINT ( 'NONE',  ( 4.379528057220339221, -16.55341960407611168, 102.7072429386476955 ) ) ;
#95774=CARTESIAN_POINT ( 'NONE',  ( -4.483927247898782831, 16.52544592524335698, 52.70942372801902565 ) ) ;
#95775=CARTESIAN_POINT ( 'NONE',  ( -0.05219959533910754901, -16.53943276465976808, 77.49890960531433848 ) ) ;
#95776=EDGE_CURVE ( 'NONE', #73688, #179909, #145398, .T. ) ;
#95777=CARTESIAN_POINT ( 'NONE',  ( -19.46398650005389896, 5.499999999999950262, 65.18269651486376404 ) ) ;
#95778=CARTESIAN_POINT ( 'NONE',  ( -0.05219959533936034679, 19.03943276465977164, 82.50109039468567573 ) ) ;
#95779=CARTESIAN_POINT ( 'NONE',  ( -9.474510206698964154, 16.51473224551069663, 115.4155762719810241 ) ) ;
#95782=CARTESIAN_POINT ( 'NONE',  ( -12.14591786802326823, 12.06949235617739902, 28.12609039468568284 ) ) ;
#95783=CARTESIAN_POINT ( 'NONE',  ( -14.34966873604960291, -8.224510206698953496, 26.66557627198103475 ) ) ;
#95784=CARTESIAN_POINT ( 'NONE',  ( -5.823673210054116645, -21.52544592524344225, 52.29057627198102409 ) ) ;
#95785=CARTESIAN_POINT ( 'NONE',  ( 5.153800228976615827, -19.02544592524334988, 90.20942372801900433 ) ) ;
#95786=CARTESIAN_POINT ( 'NONE',  ( -5.823673210054116645, -21.52544592524344225, 42.29057627198103120 ) ) ;
#95787=CARTESIAN_POINT ( 'NONE',  ( -15.80617190586768217, 15.72974639402176855, 88.12609039468570415 ) ) ;
#95789=CARTESIAN_POINT ( 'NONE',  ( 14.29746914071037800, 8.314922557961029526, 36.66775706135234714 ) ) ;
#95790=CARTESIAN_POINT ( 'NONE',  ( 13.89961937509977652, -13.97604488694527269, 43.12390960531434558 ) ) ;
#95791=CARTESIAN_POINT ( 'NONE',  ( 16.51473224551069308, 9.474510206698969483, 84.16557627198102409 ) ) ;
#95792=CARTESIAN_POINT ( 'NONE',  ( -5.049401038298153566, 19.05341960407611168, 35.20724293864768839 ) ) ;
#95793=CARTESIAN_POINT ( 'NONE',  ( 4.483927247898545687, 16.52544592524342804, 99.79057627198103830 ) ) ;
#95795=CARTESIAN_POINT ( 'NONE',  ( -13.89961937509977652, 13.97604488694528158, 100.6239096053143669 ) ) ;
#95796=ORIENTED_EDGE ( 'NONE', *, *, #45960, .F. ) ;
#95797=CARTESIAN_POINT ( 'NONE',  ( 16.55341960407618274, -4.379528057220086978, 56.04275706135235424 ) ) ;
#95798=CARTESIAN_POINT ( 'NONE',  ( 21.53943276465977519, -0.05219959533907433946, 93.74890960531436690 ) ) ;
#95799=CARTESIAN_POINT ( 'NONE',  ( 13.89961937509977652, -13.97604488694527269, 38.12390960531436690 ) ) ;
#95800=CARTESIAN_POINT ( 'NONE',  ( -16.51473224551082808, 9.474510206698731452, 73.33442372801900433 ) ) ;
#95801=CARTESIAN_POINT ( 'NONE',  ( -10.72451020669870658, -18.67979575497194134, 29.58442372801901854 ) ) ;
#95802=CARTESIAN_POINT ( 'NONE',  ( -13.89961937509977652, 13.97604488694528158, 65.62390960531436690 ) ) ;
#95803=CARTESIAN_POINT ( 'NONE',  ( -19.05341960407611168, -5.049401038298163336, 101.4572429386476955 ) ) ;
#95804=ORIENTED_EDGE ( 'NONE', *, *, #138549, .F. ) ;
#95805=CARTESIAN_POINT ( 'NONE',  ( 16.52544592524335698, 4.483927247898782831, 36.45942372801901143 ) ) ;
#95806=CARTESIAN_POINT ( 'NONE',  ( -10.81492255796105439, 18.62759615963255655, 22.91775706135235069 ) ) ;
#95807=CARTESIAN_POINT ( 'NONE',  ( -8.224510206698948167, 14.34966873604960824, 110.4155762719810383 ) ) ;
#95808=CARTESIAN_POINT ( 'NONE',  ( 19.03943276465977164, -0.05219959533909143690, 98.74890960531436690 ) ) ;
#95809=CARTESIAN_POINT ( 'NONE',  ( -19.03943276465977164, -0.05219959533935918106, 78.75109039468567573 ) ) ;
#95810=CARTESIAN_POINT ( 'NONE',  ( 15.72974639402199770, -15.80617190586745480, 88.12390960531436690 ) ) ;
#95811=CARTESIAN_POINT ( 'NONE',  ( 0.05219959533910956823, 16.53943276465976808, 39.99890960531436690 ) ) ;
#95812=CARTESIAN_POINT ( 'NONE',  ( 19.03943276465977164, 0.05219959533936151252, 21.25109039468565797 ) ) ;
#95813=CARTESIAN_POINT ( 'NONE',  ( 16.55341960407618274, -4.379528057220086978, 76.04275706135237556 ) ) ;
#95814=CARTESIAN_POINT ( 'NONE',  ( 5.153800228976335163, 19.02544592524342804, 99.79057627198102409 ) ) ;
#95815=CARTESIAN_POINT ( 'NONE',  ( -0.05219959533909027116, -19.03943276465977164, 47.49890960531435979 ) ) ;
#95817=CARTESIAN_POINT ( 'NONE',  ( 21.55341960407619695, -5.719274019375665929, 56.04275706135235424 ) ) ;
#95818=CARTESIAN_POINT ( 'NONE',  ( 21.53943276465977519, 0.05219959533937863772, 66.25109039468567573 ) ) ;
#95819=CARTESIAN_POINT ( 'NONE',  ( 19.02544592524343514, -5.153800228976328945, 68.54057627198103830 ) ) ;
#95820=CARTESIAN_POINT ( 'NONE',  ( -15.80617190586768217, 15.72974639402176855, 48.12609039468568284 ) ) ;
#95821=CARTESIAN_POINT ( 'NONE',  ( -9.564922557961040184, 16.46253265017147172, 87.91775706135233293 ) ) ;
#95822=CARTESIAN_POINT ( 'NONE',  ( -9.564922557960796823, -16.46253265017161027, 47.08224293864769550 ) ) ;
#95823=CARTESIAN_POINT ( 'NONE',  ( 0.05219959533934541429, -16.53943276465976808, 90.00109039468567573 ) ) ;
#95824=CARTESIAN_POINT ( 'NONE',  ( -5.049401038298153566, 19.05341960407611168, 65.20724293864765286 ) ) ;
#95825=CARTESIAN_POINT ( 'NONE',  ( -19.02544592524342804, 5.153800228976336051, 116.0405762719810383 ) ) ;
#95826=CARTESIAN_POINT ( 'NONE',  ( -9.564922557960796823, -16.46253265017161027, 52.08224293864768839 ) ) ;
#95827=EDGE_CURVE ( 'NONE', #149451, #199515, #29391, .T. ) ;
#95828=CARTESIAN_POINT ( 'NONE',  ( -15.80617190586745835, -15.72974639402198527, 91.87390960531436690 ) ) ;
#95829=CARTESIAN_POINT ( 'NONE',  ( -4.379528057220086978, -16.55341960407618274, 79.79275706135236135 ) ) ;
#95831=CARTESIAN_POINT ( 'NONE',  ( -16.46253265017146816, -9.564922557961047289, 34.16775706135233293 ) ) ;
#95832=CARTESIAN_POINT ( 'NONE',  ( -13.89961937509977652, 13.97604488694528158, 70.62390960531432427 ) ) ;
#95833=CARTESIAN_POINT ( 'NONE',  ( -4.379528057220328563, 16.55341960407611168, 60.20724293864768839 ) ) ;
#95834=CARTESIAN_POINT ( 'NONE',  ( 16.53943276465976808, -0.05219959533910856209, 93.74890960531436690 ) ) ;
#95835=CARTESIAN_POINT ( 'NONE',  ( -9.474510206698964154, 16.51473224551069663, 105.4155762719810383 ) ) ;
#95836=CARTESIAN_POINT ( 'NONE',  ( -13.89961937509977652, 13.97604488694528158, 95.62390960531436690 ) ) ;
#95837=CARTESIAN_POINT ( 'NONE',  ( -21.52544592524334988, -5.823673210054445271, 43.95942372801902565 ) ) ;
#95838=CARTESIAN_POINT ( 'NONE',  ( -9.474510206698964154, 16.51473224551069663, 110.4155762719810383 ) ) ;
#95839=CARTESIAN_POINT ( 'NONE',  ( 18.67979575497194134, -10.72451020669871369, 110.8344237280190043 ) ) ;
#95840=CARTESIAN_POINT ( 'NONE',  ( -12.06949235617739369, -12.14591786802326823, 79.37609039468567573 ) ) ;
#95841=CARTESIAN_POINT ( 'NONE',  ( 5.823673210054444382, -21.52544592524334988, 40.20942372801901854 ) ) ;
#95842=CARTESIAN_POINT ( 'NONE',  ( -9.474510206698964154, 16.51473224551069663, 110.4155762719810383 ) ) ;
#95843=CARTESIAN_POINT ( 'NONE',  ( -5.823673210054116645, -21.52544592524344225, 97.29057627198105251 ) ) ;
#95844=CARTESIAN_POINT ( 'NONE',  ( 4.379528057220339221, -16.55341960407611168, 57.70724293864770260 ) ) ;
#95845=CARTESIAN_POINT ( 'NONE',  ( -13.89961937509977652, 13.97604488694528158, 55.62390960531434558 ) ) ;
#95846=CARTESIAN_POINT ( 'NONE',  ( 16.53943276465976808, -0.05219959533910856209, 83.74890960531435269 ) ) ;
#95847=CARTESIAN_POINT ( 'NONE',  ( -10.72451020669898014, 18.67979575497178502, 40.41557627198103120 ) ) ;
#95848=CARTESIAN_POINT ( 'NONE',  ( 19.03943276465977164, 0.05219959533936151252, 46.25109039468566863 ) ) ;
#95849=CARTESIAN_POINT ( 'NONE',  ( -5.153800228976328057, -19.02544592524343514, 22.29057627198102765 ) ) ;
#95850=ORIENTED_EDGE ( 'NONE', *, *, #11874, .T. ) ;
#95851=CARTESIAN_POINT ( 'NONE',  ( -4.483927247898782831, 16.52544592524335698, 67.70942372801901854 ) ) ;
#95852=CARTESIAN_POINT ( 'NONE',  ( -5.049401038298153566, 19.05341960407611168, 70.20724293864769550 ) ) ;
#95854=CARTESIAN_POINT ( 'NONE',  ( -12.06949235617756955, 12.14591786802309770, 85.62390960531436690 ) ) ;
#95855=CARTESIAN_POINT ( 'NONE',  ( 18.62759615963271287, -10.81492255796078972, 43.33224293864769550 ) ) ;
#95857=CARTESIAN_POINT ( 'NONE',  ( 8.224510206698742110, 14.34966873604972548, 112.0844237280190185 ) ) ;
#95858=CARTESIAN_POINT ( 'NONE',  ( -4.379528057220086978, -16.55341960407618274, 19.79275706135235069 ) ) ;
#95859=CARTESIAN_POINT ( 'NONE',  ( 5.823673210054444382, -21.52544592524334988, 80.20942372801901854 ) ) ;
#95860=CARTESIAN_POINT ( 'NONE',  ( -9.474510206698964154, 16.51473224551069663, 85.41557627198102409 ) ) ;
#95861=CARTESIAN_POINT ( 'NONE',  ( 15.80617190586746368, 15.72974639402197994, 99.37390960531436690 ) ) ;
#95862=CARTESIAN_POINT ( 'NONE',  ( -8.224510206698735004, -14.34966873604973081, 49.58442372801901143 ) ) ;
#95863=CARTESIAN_POINT ( 'NONE',  ( 13.89961937509977652, -13.97604488694527269, 33.12390960531434558 ) ) ;
#95865=CARTESIAN_POINT ( 'NONE',  ( 4.379528057220092307, 16.55341960407617563, 37.29275706135235424 ) ) ;
#95866=CARTESIAN_POINT ( 'NONE',  ( -13.89961937509957401, -13.97604488694547875, 99.37609039468567573 ) ) ;
#95867=CARTESIAN_POINT ( 'NONE',  ( -10.81492255796078084, -18.62759615963271287, 87.08224293864769550 ) ) ;
#95868=CARTESIAN_POINT ( 'NONE',  ( 5.153800228976615827, -19.02544592524334988, 60.20942372801899012 ) ) ;
#95869=CARTESIAN_POINT ( 'NONE',  ( 19.52837319214027545, -5.499999999999890754, 87.10471352585537375 ) ) ;
#95870=CARTESIAN_POINT ( 'NONE',  ( 18.62759615963271287, -10.81492255796078972, 98.33224293864769550 ) ) ;
#95872=CARTESIAN_POINT ( 'NONE',  ( 13.89961937509977652, -13.97604488694527269, 73.12390960531436690 ) ) ;
#95873=CARTESIAN_POINT ( 'NONE',  ( -4.379528057220086978, -16.55341960407618274, 39.79275706135235424 ) ) ;
#95875=CARTESIAN_POINT ( 'NONE',  ( -9.474510206698720793, -16.51473224551083518, 59.58442372801900433 ) ) ;
#95876=CARTESIAN_POINT ( 'NONE',  ( -5.719274019375978568, 21.55341960407610458, 115.2072429386476955 ) ) ;
#95877=CARTESIAN_POINT ( 'NONE',  ( 12.06949235617757843, -12.14591786802309237, 68.12390960531436690 ) ) ;
#95878=CARTESIAN_POINT ( 'NONE',  ( 5.049401038298161559, -19.05341960407611168, 72.70724293864768129 ) ) ;
#95879=CARTESIAN_POINT ( 'NONE',  ( 14.29746914071037800, 8.314922557961029526, 31.66775706135234358 ) ) ;
#95880=CARTESIAN_POINT ( 'NONE',  ( 16.46253265017146816, 9.564922557961045513, 36.66775706135233293 ) ) ;
#95881=CARTESIAN_POINT ( 'NONE',  ( -15.80617190586768217, 15.72974639402176855, 53.12609039468568284 ) ) ;
#95882=CARTESIAN_POINT ( 'NONE',  ( 5.049401038297881783, 19.05341960407617563, 112.2927570613523471 ) ) ;
#95883=CARTESIAN_POINT ( 'NONE',  ( -5.049401038298153566, 19.05341960407611168, 60.20724293864768129 ) ) ;
#95884=CARTESIAN_POINT ( 'NONE',  ( 16.46253265017146816, 9.564922557961045513, 86.66775706135233293 ) ) ;
#95885=CARTESIAN_POINT ( 'NONE',  ( 10.81492255796106328, -18.62759615963255655, 90.41775706135236135 ) ) ;
#95886=CARTESIAN_POINT ( 'NONE',  ( 13.89961937509957401, 13.97604488694547697, 61.87609039468566863 ) ) ;
#95887=CARTESIAN_POINT ( 'NONE',  ( -16.46253265017160317, 9.564922557960807481, 30.83224293864769550 ) ) ;
#95888=CARTESIAN_POINT ( 'NONE',  ( 0.05219959533907565091, 21.53943276465977519, 54.99890960531435269 ) ) ;
#95889=CARTESIAN_POINT ( 'NONE',  ( 4.483927247898545687, 16.52544592524342804, 64.79057627198103830 ) ) ;
#95890=CARTESIAN_POINT ( 'NONE',  ( -16.51473224551082808, 9.474510206698731452, 68.33442372801900433 ) ) ;
#95891=CARTESIAN_POINT ( 'NONE',  ( -18.09918380851993192, -5.500000000000014211, 101.4861830733561163 ) ) ;
#95892=CARTESIAN_POINT ( 'NONE',  ( 13.97604488694548053, -13.89961937509957401, 30.62609039468566863 ) ) ;
#95893=CARTESIAN_POINT ( 'NONE',  ( 0.05219959533934541429, -16.53943276465976808, 95.00109039468568994 ) ) ;
#95894=CARTESIAN_POINT ( 'NONE',  ( 16.52544592524342804, -4.483927247898539470, 48.54057627198103120 ) ) ;
#95895=CARTESIAN_POINT ( 'NONE',  ( -0.05219959533937732626, 21.53943276465977519, 92.50109039468567573 ) ) ;
#95897=CARTESIAN_POINT ( 'NONE',  ( -18.67979575497178146, -10.72451020669898902, 91.66557627198103830 ) ) ;
#95898=CARTESIAN_POINT ( 'NONE',  ( 5.153800228976335163, 19.02544592524342804, 49.79057627198100988 ) ) ;
#95899=CARTESIAN_POINT ( 'NONE',  ( 18.67979575497194134, -10.72451020669871369, 65.83442372801900433 ) ) ;
#95900=CARTESIAN_POINT ( 'NONE',  ( -9.564922557960796823, -16.46253265017161027, 47.08224293864769550 ) ) ;
#95901=CARTESIAN_POINT ( 'NONE',  ( -16.46253265017160317, 9.564922557960807481, 65.83224293864769550 ) ) ;
#95902=CARTESIAN_POINT ( 'NONE',  ( 16.53943276465976808, -0.05219959533910856209, 108.7489096053143669 ) ) ;
#95903=CARTESIAN_POINT ( 'NONE',  ( 5.049401038298161559, -19.05341960407611168, 112.7072429386476813 ) ) ;
#95904=CARTESIAN_POINT ( 'NONE',  ( -12.06949235617756955, 12.14591786802309770, 50.62390960531435979 ) ) ;
#95905=CARTESIAN_POINT ( 'NONE',  ( -9.564922557960796823, -16.46253265017161027, 32.08224293864769550 ) ) ;
#95906=CARTESIAN_POINT ( 'NONE',  ( -16.52544592524342804, 4.483927247898546575, 81.04057627198102409 ) ) ;
#95907=CARTESIAN_POINT ( 'NONE',  ( -10.81492255796078084, -18.62759615963271287, 92.08224293864769550 ) ) ;
#95908=CARTESIAN_POINT ( 'NONE',  ( -15.72974639402176322, -15.80617190586768395, 39.37609039468567573 ) ) ;
#95910=CARTESIAN_POINT ( 'NONE',  ( 8.314922557961029526, -14.29746914071037800, 40.41775706135234714 ) ) ;
#95911=CARTESIAN_POINT ( 'NONE',  ( -10.81492255796078084, -18.62759615963271287, 82.08224293864768129 ) ) ;
#95912=CARTESIAN_POINT ( 'NONE',  ( -19.03943276465977164, -0.05219959533935918106, 18.75109039468567218 ) ) ;
#95913=CARTESIAN_POINT ( 'NONE',  ( 0.05219959533909260263, 19.03943276465977164, 99.99890960531436690 ) ) ;
#95914=CARTESIAN_POINT ( 'NONE',  ( 5.719274019375673035, 21.55341960407619339, 42.29275706135235424 ) ) ;
#95915=CARTESIAN_POINT ( 'NONE',  ( -0.05219959533907301413, -21.53943276465977519, 27.49890960531435269 ) ) ;
#95916=CARTESIAN_POINT ( 'NONE',  ( -4.483927247898782831, 16.52544592524335698, 107.7094237280190328 ) ) ;
#95917=CARTESIAN_POINT ( 'NONE',  ( 15.80617190586769283, -15.72974639402175789, 55.62609039468568284 ) ) ;
#95918=CARTESIAN_POINT ( 'NONE',  ( 5.719274019375673035, 21.55341960407619339, 82.29275706135234714 ) ) ;
#95919=CARTESIAN_POINT ( 'NONE',  ( 16.51473224551083163, -9.474510206698727899, 25.83442372801900078 ) ) ;
#95920=CARTESIAN_POINT ( 'NONE',  ( -12.14591786802326823, 12.06949235617739902, 93.12609039468568994 ) ) ;
#95921=CARTESIAN_POINT ( 'NONE',  ( 18.62759615963255655, 10.81492255796105972, 36.66775706135234714 ) ) ;
#95922=CARTESIAN_POINT ( 'NONE',  ( 9.564922557960805705, 16.46253265017160317, 49.58224293864770260 ) ) ;
#95923=CARTESIAN_POINT ( 'NONE',  ( -10.72451020669870658, -18.67979575497194134, 104.5844237280190185 ) ) ;
#95924=CARTESIAN_POINT ( 'NONE',  ( -16.51473224551069308, -9.474510206698971260, 111.6655762719810383 ) ) ;
#95925=CARTESIAN_POINT ( 'NONE',  ( -10.81492255796078084, -18.62759615963271287, 107.0822429386476955 ) ) ;
#95926=CARTESIAN_POINT ( 'NONE',  ( -15.72974639402197994, 15.80617190586746368, 55.62390960531436690 ) ) ;
#95928=CARTESIAN_POINT ( 'NONE',  ( -10.72451020669898014, 18.67979575497178502, 70.41557627198102409 ) ) ;
#95929=CARTESIAN_POINT ( 'NONE',  ( -4.379528057220086978, -16.55341960407618274, 49.79275706135234714 ) ) ;
#95930=CARTESIAN_POINT ( 'NONE',  ( 12.06949235617757843, -12.14591786802309237, 68.12390960531436690 ) ) ;
#95932=CARTESIAN_POINT ( 'NONE',  ( -19.05341960407617563, 5.049401038297882671, 93.54275706135234714 ) ) ;
#95934=CARTESIAN_POINT ( 'NONE',  ( -14.34966873604972548, 8.224510206698743886, 28.33442372801902209 ) ) ;
#95935=CARTESIAN_POINT ( 'NONE',  ( 21.53943276465977519, -0.05219959533907433946, 93.74890960531436690 ) ) ;
#95936=CARTESIAN_POINT ( 'NONE',  ( -5.719274019375978568, 21.55341960407610458, 75.20724293864769550 ) ) ;
#95937=CARTESIAN_POINT ( 'NONE',  ( -5.049401038298153566, 19.05341960407611168, 115.2072429386477097 ) ) ;
#95938=CARTESIAN_POINT ( 'NONE',  ( -8.314922557961024197, 14.29746914071037800, 62.91775706135236135 ) ) ;
#95939=CARTESIAN_POINT ( 'NONE',  ( -19.02544592524342804, 5.153800228976336051, 71.04057627198099567 ) ) ;
#95940=CARTESIAN_POINT ( 'NONE',  ( -10.81492255796105439, 18.62759615963255655, 37.91775706135235424 ) ) ;
#95941=CARTESIAN_POINT ( 'NONE',  ( 9.564922557961047289, -16.46253265017146816, 105.4177570613523471 ) ) ;
#95943=CARTESIAN_POINT ( 'NONE',  ( -13.97604488694527625, -13.89961937509977652, 101.8739096053143811 ) ) ;
#95944=CARTESIAN_POINT ( 'NONE',  ( -13.89961937509977652, 13.97604488694528158, 90.62390960531432427 ) ) ;
#95945=CARTESIAN_POINT ( 'NONE',  ( 0.05219959533907565091, 21.53943276465977519, 94.99890960531436690 ) ) ;
#95946=CARTESIAN_POINT ( 'NONE',  ( 13.89961937509977652, -13.97604488694527269, 53.12390960531434558 ) ) ;
#95948=CARTESIAN_POINT ( 'NONE',  ( 14.29746914071049879, -8.314922557960816363, 73.33224293864769550 ) ) ;
#95950=CARTESIAN_POINT ( 'NONE',  ( -19.03943276465977164, 0.05219959533909376836, 111.2489096053143669 ) ) ;
#95952=CARTESIAN_POINT ( 'NONE',  ( 10.72451020669898902, -18.67979575497178502, 107.9155762719810241 ) ) ;
#95953=CARTESIAN_POINT ( 'NONE',  ( -19.05341960407617563, 5.049401038297882671, 68.54275706135230450 ) ) ;
#95954=CARTESIAN_POINT ( 'NONE',  ( 18.62759615963271287, -10.81492255796078972, 23.33224293864769194 ) ) ;
#95955=CARTESIAN_POINT ( 'NONE',  ( -19.05341960407611168, -5.049401038298163336, 21.45724293864768839 ) ) ;
#95956=CARTESIAN_POINT ( 'NONE',  ( 18.62759615963271287, -10.81492255796078972, 58.33224293864768839 ) ) ;
#95958=CARTESIAN_POINT ( 'NONE',  ( -16.51473224551069308, -9.474510206698971260, 101.6655762719810241 ) ) ;
#95959=CARTESIAN_POINT ( 'NONE',  ( 15.72974639402176855, 15.80617190586768217, 81.87609039468568994 ) ) ;
#95960=CARTESIAN_POINT ( 'NONE',  ( -9.474510206698964154, 16.51473224551069663, 55.41557627198103120 ) ) ;
#95961=CARTESIAN_POINT ( 'NONE',  ( -12.06949235617756955, 12.14591786802309770, 85.62390960531436690 ) ) ;
#95962=CARTESIAN_POINT ( 'NONE',  ( 4.483927247898790824, -16.52544592524335698, 35.20942372801901854 ) ) ;
#95963=CARTESIAN_POINT ( 'NONE',  ( 0.05219959533937995610, -21.53943276465977519, 60.00109039468568284 ) ) ;
#95964=ORIENTED_EDGE ( 'NONE', *, *, #53248, .T. ) ;
#95965=CARTESIAN_POINT ( 'NONE',  ( 19.05341960407617918, -5.049401038297876454, 26.04275706135233293 ) ) ;
#95966=CARTESIAN_POINT ( 'NONE',  ( 16.51473224551083163, -9.474510206698727899, 80.83442372801899012 ) ) ;
#95967=CARTESIAN_POINT ( 'NONE',  ( -16.46253265017146816, -9.564922557961047289, 44.16775706135232582 ) ) ;
#95968=CARTESIAN_POINT ( 'NONE',  ( 18.22780087662121673, 5.500000000000056843, 88.98459894673892734 ) ) ;
#95969=CARTESIAN_POINT ( 'NONE',  ( -18.62759615963255300, -10.81492255796106328, 34.16775706135234714 ) ) ;
#95971=CARTESIAN_POINT ( 'NONE',  ( -19.49671883438229614, -5.499999999999982236, 44.89279849105685116 ) ) ;
#95972=CARTESIAN_POINT ( 'NONE',  ( -9.474510206698720793, -16.51473224551083518, 29.58442372801900433 ) ) ;
#95973=CARTESIAN_POINT ( 'NONE',  ( -19.02544592524342804, 5.153800228976336051, 51.04057627198103120 ) ) ;
#95974=CARTESIAN_POINT ( 'NONE',  ( 16.46253265017146816, 9.564922557961045513, 31.66775706135232937 ) ) ;
#95975=CARTESIAN_POINT ( 'NONE',  ( 4.483927247898790824, -16.52544592524335698, 105.2094237280190328 ) ) ;
#95976=CARTESIAN_POINT ( 'NONE',  ( -19.03943276465977164, 0.05219959533909376836, 111.2489096053143669 ) ) ;
#95977=CARTESIAN_POINT ( 'NONE',  ( 21.53943276465977519, 0.05219959533937863772, 91.25109039468568994 ) ) ;
#95979=CARTESIAN_POINT ( 'NONE',  ( -17.50000000000014921, -3.417042746626747896, 34.82619603767538052 ) ) ;
#95980=CARTESIAN_POINT ( 'NONE',  ( -5.719274019375665041, -21.55341960407619695, 89.79275706135236135 ) ) ;
#95982=CARTESIAN_POINT ( 'NONE',  ( 19.05341960407611168, 5.049401038298154454, 93.95724293864769550 ) ) ;
#95984=CARTESIAN_POINT ( 'NONE',  ( -19.03943276465977164, 0.05219959533909376836, 56.24890960531435979 ) ) ;
#95985=CARTESIAN_POINT ( 'NONE',  ( -18.67979575497178146, -10.72451020669898902, 56.66557627198103830 ) ) ;
#95986=CARTESIAN_POINT ( 'NONE',  ( -14.34966873604972548, 8.224510206698743886, 113.3344237280190328 ) ) ;
#95987=CARTESIAN_POINT ( 'NONE',  ( 8.314922557960818139, 14.29746914071049879, 94.58224293864769550 ) ) ;
#95988=CARTESIAN_POINT ( 'NONE',  ( 0.05219959533909260263, 19.03943276465977164, 94.99890960531436690 ) ) ;
#95989=CARTESIAN_POINT ( 'NONE',  ( 13.97604488694548053, -13.89961937509957401, 25.62609039468566507 ) ) ;
#95990=CARTESIAN_POINT ( 'NONE',  ( 8.224510206698953496, -14.34966873604960469, 107.9155762719810241 ) ) ;
#95991=CARTESIAN_POINT ( 'NONE',  ( 10.81492255796106328, -18.62759615963255655, 60.41775706135235424 ) ) ;
#95992=CARTESIAN_POINT ( 'NONE',  ( -8.224510206698735004, -14.34966873604973081, 104.5844237280190185 ) ) ;
#95993=CARTESIAN_POINT ( 'NONE',  ( 19.05341960407617918, -5.049401038297876454, 71.04275706135234714 ) ) ;
#95995=CARTESIAN_POINT ( 'NONE',  ( 19.03943276465977164, -0.05219959533909143690, 113.7489096053143669 ) ) ;
#95996=CARTESIAN_POINT ( 'NONE',  ( -4.379528057220328563, 16.55341960407611168, 70.20724293864769550 ) ) ;
#95997=CARTESIAN_POINT ( 'NONE',  ( -19.02544592524334988, -5.153800228976617603, 53.95942372801898301 ) ) ;
#95999=CARTESIAN_POINT ( 'NONE',  ( -16.51473224551069308, -9.474510206698971260, 56.66557627198103120 ) ) ;
#96000=CARTESIAN_POINT ( 'NONE',  ( -12.14591786802309592, -12.06949235617757132, 61.87390960531436690 ) ) ;
#96001=CARTESIAN_POINT ( 'NONE',  ( 5.049401038297881783, 19.05341960407617563, 97.29275706135233293 ) ) ;
#96002=CARTESIAN_POINT ( 'NONE',  ( -18.62759615963270932, 10.81492255796079327, 30.83224293864770260 ) ) ;
#96003=ORIENTED_EDGE ( 'NONE', *, *, #20112, .F. ) ;
#96004=CARTESIAN_POINT ( 'NONE',  ( -14.29746914071049879, 8.314922557960819915, 95.83224293864770971 ) ) ;
#96005=CARTESIAN_POINT ( 'NONE',  ( -17.49999999999999645, -5.500000000000000888, 29.20309617465828467 ) ) ;
#96006=CARTESIAN_POINT ( 'NONE',  ( -5.049401038298153566, 19.05341960407611168, 60.20724293864768129 ) ) ;
#96007=CARTESIAN_POINT ( 'NONE',  ( 15.80617190586746368, 15.72974639402197994, 59.37390960531436690 ) ) ;
#96008=CARTESIAN_POINT ( 'NONE',  ( 9.564922557960805705, 16.46253265017160317, 44.58224293864769550 ) ) ;
#96009=CARTESIAN_POINT ( 'NONE',  ( -8.224510206698735004, -14.34966873604973081, 94.58442372801901854 ) ) ;
#96010=CARTESIAN_POINT ( 'NONE',  ( 19.02544592524343514, -5.153800228976328945, 78.54057627198099567 ) ) ;
#96011=CARTESIAN_POINT ( 'NONE',  ( -0.05219959533936034679, 19.03943276465977164, 47.50109039468566863 ) ) ;
#96012=CARTESIAN_POINT ( 'NONE',  ( -0.05219959533937732626, 21.53943276465977519, 82.50109039468568994 ) ) ;
#96013=CARTESIAN_POINT ( 'NONE',  ( 18.67979575497178502, 10.72451020669898547, 54.16557627198103120 ) ) ;
#96014=CARTESIAN_POINT ( 'NONE',  ( 16.46253265017160672, -9.564922557960803928, 108.3322429386476955 ) ) ;
#96015=CARTESIAN_POINT ( 'NONE',  ( -13.89961937509977652, 13.97604488694528158, 25.62390960531434558 ) ) ;
#96016=CARTESIAN_POINT ( 'NONE',  ( -16.53943276465976808, -0.05219959533934237506, 93.75109039468567573 ) ) ;
#96017=CARTESIAN_POINT ( 'NONE',  ( -5.049401038297874678, -19.05341960407617918, 104.7927570613523471 ) ) ;
#96018=CARTESIAN_POINT ( 'NONE',  ( -16.51473224551069308, -9.474510206698971260, 21.66557627198102765 ) ) ;
#96019=CARTESIAN_POINT ( 'NONE',  ( 19.39056639909674118, 5.500000000000052403, 78.28948781074343799 ) ) ;
#96020=CARTESIAN_POINT ( 'NONE',  ( 18.62759615963255655, 10.81492255796105972, 101.6677570613523613 ) ) ;
#96021=CARTESIAN_POINT ( 'NONE',  ( -12.14591786802309592, -12.06949235617757132, 56.87390960531436690 ) ) ;
#96022=CARTESIAN_POINT ( 'NONE',  ( 4.483927247898545687, 16.52544592524342804, 64.79057627198103830 ) ) ;
#96023=CARTESIAN_POINT ( 'NONE',  ( 21.53943276465977519, -0.05219959533907433946, 93.74890960531436690 ) ) ;
#96024=CARTESIAN_POINT ( 'NONE',  ( 5.719274019375991003, -21.55341960407610458, 87.70724293864769550 ) ) ;
#96025=CARTESIAN_POINT ( 'NONE',  ( 17.40805194822031865, -6.112264579159335298, 98.33371272510615313 ) ) ;
#96026=CARTESIAN_POINT ( 'NONE',  ( -5.719274019375978568, 21.55341960407610458, 30.20724293864769550 ) ) ;
#96027=CARTESIAN_POINT ( 'NONE',  ( -0.05219959533934338120, 16.53943276465976808, 62.50109039468568284 ) ) ;
#96028=CARTESIAN_POINT ( 'NONE',  ( 4.483927247898545687, 16.52544592524342804, 84.79057627198102409 ) ) ;
#96029=CARTESIAN_POINT ( 'NONE',  ( 19.05341960407611168, 5.049401038298154454, 43.95724293864769550 ) ) ;
#96031=CARTESIAN_POINT ( 'NONE',  ( 16.55341960407618274, -4.379528057220086978, 91.04275706135236135 ) ) ;
#96032=CARTESIAN_POINT ( 'NONE',  ( 0.05219959533937995610, -21.53943276465977519, 40.00109039468567573 ) ) ;
#96033=CARTESIAN_POINT ( 'NONE',  ( 16.46253265017160672, -9.564922557960803928, 83.33224293864768129 ) ) ;
#96034=CARTESIAN_POINT ( 'NONE',  ( -21.52544592524334988, -5.823673210054445271, 73.95942372801901854 ) ) ;
#96036=CARTESIAN_POINT ( 'NONE',  ( -13.89961937509977652, 13.97604488694528158, 25.62390960531434558 ) ) ;
#96038=CARTESIAN_POINT ( 'NONE',  ( 21.52544592524334988, 5.823673210054432836, 56.45942372801902565 ) ) ;
#96039=CARTESIAN_POINT ( 'NONE',  ( -16.51473224551069308, -9.474510206698971260, 36.66557627198102409 ) ) ;
#96040=CARTESIAN_POINT ( 'NONE',  ( 16.46253265017160672, -9.564922557960803928, 23.33224293864769194 ) ) ;
#96041=CARTESIAN_POINT ( 'NONE',  ( 5.153800228976335163, 19.02544592524342804, 94.79057627198103830 ) ) ;
#96042=CARTESIAN_POINT ( 'NONE',  ( -0.05219959533936034679, 19.03943276465977164, 72.50109039468566152 ) ) ;
#96043=CARTESIAN_POINT ( 'NONE',  ( -15.80617190586768217, 15.72974639402176855, 23.12609039468567573 ) ) ;
#96044=CARTESIAN_POINT ( 'NONE',  ( 9.564922557961047289, -16.46253265017146816, 65.41775706135233293 ) ) ;
#96045=CARTESIAN_POINT ( 'NONE',  ( 19.02544592524343514, -5.153800228976328945, 43.54057627198103120 ) ) ;
#96046=CARTESIAN_POINT ( 'NONE',  ( -14.29746914071037622, -8.314922557961029526, 104.1677570613523471 ) ) ;
#96047=CARTESIAN_POINT ( 'NONE',  ( -9.474510206698720793, -16.51473224551083518, 64.58442372801900433 ) ) ;
#96048=CARTESIAN_POINT ( 'NONE',  ( -8.314922557960811034, -14.29746914071050412, 32.08224293864769550 ) ) ;
#96049=CARTESIAN_POINT ( 'NONE',  ( -16.46253265017146816, -9.564922557961047289, 49.16775706135233293 ) ) ;
#96050=CARTESIAN_POINT ( 'NONE',  ( -13.97604488694527625, -13.89961937509977652, 81.87390960531436690 ) ) ;
#96051=CARTESIAN_POINT ( 'NONE',  ( 10.81492255796106328, -18.62759615963255655, 95.41775706135234714 ) ) ;
#96052=CARTESIAN_POINT ( 'NONE',  ( 18.62759615963255655, 10.81492255796105972, 101.6677570613523613 ) ) ;
#96054=CARTESIAN_POINT ( 'NONE',  ( -0.05219959533937732626, 21.53943276465977519, 82.50109039468568994 ) ) ;
#96055=CARTESIAN_POINT ( 'NONE',  ( 16.55341960407618274, -4.379528057220086978, 26.04275706135235779 ) ) ;
#96056=CARTESIAN_POINT ( 'NONE',  ( 19.03943276465977164, -0.05219959533909143690, 88.74890960531436690 ) ) ;
#96058=CARTESIAN_POINT ( 'NONE',  ( 16.51473224551069308, 9.474510206698969483, 79.16557627198103830 ) ) ;
#96059=CARTESIAN_POINT ( 'NONE',  ( -17.40861289039008497, 6.110651285853115233, 98.62767529172569425 ) ) ;
#96060=CARTESIAN_POINT ( 'NONE',  ( -19.03943276465977164, -0.05219959533935918106, 68.75109039468566152 ) ) ;
#96061=CARTESIAN_POINT ( 'NONE',  ( 16.51473224551069308, 9.474510206698969483, 104.1655762719810241 ) ) ;
#96062=CARTESIAN_POINT ( 'NONE',  ( 10.81492255796106328, -18.62759615963255655, 100.4177570613523471 ) ) ;
#96063=CARTESIAN_POINT ( 'NONE',  ( 4.483927247898545687, 16.52544592524342804, 104.7905762719810241 ) ) ;
#96064=CARTESIAN_POINT ( 'NONE',  ( -10.72451020669898014, 18.67979575497178502, 50.41557627198103120 ) ) ;
#96065=CARTESIAN_POINT ( 'NONE',  ( 15.72974639402199770, -15.80617190586745480, 43.12390960531435269 ) ) ;
#96066=CARTESIAN_POINT ( 'NONE',  ( -8.224510206698948167, 14.34966873604960824, 110.4155762719810383 ) ) ;
#96068=CARTESIAN_POINT ( 'NONE',  ( -9.564922557961040184, 16.46253265017147172, 57.91775706135233293 ) ) ;
#96069=CARTESIAN_POINT ( 'NONE',  ( -14.34966873604960291, -8.224510206698953496, 26.66557627198103475 ) ) ;
#96070=CARTESIAN_POINT ( 'NONE',  ( 16.51473224551069308, 9.474510206698969483, 104.1655762719810241 ) ) ;
#96071=CARTESIAN_POINT ( 'NONE',  ( 21.55341960407619695, -5.719274019375665929, 81.04275706135236135 ) ) ;
#96072=CARTESIAN_POINT ( 'NONE',  ( 0.05219959533907565091, 21.53943276465977519, 74.99890960531435269 ) ) ;
#96074=CARTESIAN_POINT ( 'NONE',  ( -18.62759615963255300, -10.81492255796106328, 44.16775706135234714 ) ) ;
#96075=CARTESIAN_POINT ( 'NONE',  ( -18.62759615963270932, 10.81492255796079327, 90.83224293864769550 ) ) ;
#96076=CARTESIAN_POINT ( 'NONE',  ( -21.52544592524334988, -5.823673210054445271, 48.95942372801902565 ) ) ;
#96077=CARTESIAN_POINT ( 'NONE',  ( 13.89961937509977652, -13.97604488694527269, 28.12390960531435624 ) ) ;
#96078=CARTESIAN_POINT ( 'NONE',  ( 13.97604488694527802, 13.89961937509977652, 79.37390960531435269 ) ) ;
#96079=CARTESIAN_POINT ( 'NONE',  ( -16.53943276465976808, -0.05219959533934237506, 78.75109039468568994 ) ) ;
#96080=CARTESIAN_POINT ( 'NONE',  ( 16.55341960407611168, 4.379528057220329451, 108.9572429386476955 ) ) ;
#96081=CARTESIAN_POINT ( 'NONE',  ( -0.05219959533909027116, -19.03943276465977164, 102.4989096053143669 ) ) ;
#96082=CARTESIAN_POINT ( 'NONE',  ( 0.05219959533910956823, 16.53943276465976808, 49.99890960531437401 ) ) ;
#96083=CARTESIAN_POINT ( 'NONE',  ( -16.52544592524335698, -4.483927247898792601, 108.9594237280190185 ) ) ;
#96084=CARTESIAN_POINT ( 'NONE',  ( 13.97604488694527802, 13.89961937509977652, 49.37390960531434558 ) ) ;
#96085=CARTESIAN_POINT ( 'NONE',  ( -5.049401038298153566, 19.05341960407611168, 30.20724293864768839 ) ) ;
#96086=CARTESIAN_POINT ( 'NONE',  ( -15.72974639402197994, 15.80617190586746368, 40.62390960531435269 ) ) ;
#96087=CARTESIAN_POINT ( 'NONE',  ( -13.89961937509957401, -13.97604488694547875, 29.37609039468565797 ) ) ;
#96088=AXIS2_PLACEMENT_3D ( 'NONE', #5479, #67162, #68154 ) ;
#96089=CARTESIAN_POINT ( 'NONE',  ( -16.52216118717207394, -7.221426719304522734, 41.07599021046991794 ) ) ;
#96090=CARTESIAN_POINT ( 'NONE',  ( -16.53943276465976808, 0.05219959533911058130, 41.24890960531435269 ) ) ;
#96091=CARTESIAN_POINT ( 'NONE',  ( -18.67979575497193778, 10.72451020669871902, 48.33442372801902565 ) ) ;
#96092=CARTESIAN_POINT ( 'NONE',  ( 0.05219959533909260263, 19.03943276465977164, 114.9989096053143669 ) ) ;
#96093=CARTESIAN_POINT ( 'NONE',  ( 12.14591786802327356, -12.06949235617739191, 60.62609039468567573 ) ) ;
#96094=CARTESIAN_POINT ( 'NONE',  ( -13.97604488694547697, 13.89961937509957934, 68.12609039468563310 ) ) ;
#96095=CARTESIAN_POINT ( 'NONE',  ( 12.14591786802309770, 12.06949235617756955, 24.37390960531435979 ) ) ;
#96096=CARTESIAN_POINT ( 'NONE',  ( -4.483927247898782831, 16.52544592524335698, 112.7094237280190328 ) ) ;
#96097=CARTESIAN_POINT ( 'NONE',  ( -19.05341960407611168, -5.049401038298163336, 41.45724293864769550 ) ) ;
#96098=CARTESIAN_POINT ( 'NONE',  ( -16.46253265017160317, 9.564922557960807481, 65.83224293864769550 ) ) ;
#96099=CARTESIAN_POINT ( 'NONE',  ( 0.05219959533909260263, 19.03943276465977164, 29.99890960531435979 ) ) ;
#96100=CARTESIAN_POINT ( 'NONE',  ( -5.823673210054431948, 21.52544592524334988, 27.70942372801901854 ) ) ;
#96101=CARTESIAN_POINT ( 'NONE',  ( 16.46253265017160672, -9.564922557960803928, 48.33224293864769550 ) ) ;
#96103=CARTESIAN_POINT ( 'NONE',  ( -9.474510206698964154, 16.51473224551069663, 45.41557627198103120 ) ) ;
#96104=CARTESIAN_POINT ( 'NONE',  ( -19.02544592524342804, 5.153800228976336051, 116.0405762719810383 ) ) ;
#96105=CARTESIAN_POINT ( 'NONE',  ( -5.823673210054431948, 21.52544592524334988, 62.70942372801902565 ) ) ;
#96106=CARTESIAN_POINT ( 'NONE',  ( -0.05219959533910754901, -16.53943276465976808, 107.4989096053143669 ) ) ;
#96107=CARTESIAN_POINT ( 'NONE',  ( -9.474510206698964154, 16.51473224551069663, 110.4155762719810383 ) ) ;
#96108=CARTESIAN_POINT ( 'NONE',  ( 14.34966873604972726, -8.224510206698740333, 80.83442372801901854 ) ) ;
#96109=CARTESIAN_POINT ( 'NONE',  ( 15.80617190586769283, -15.72974639402175789, 90.62609039468567573 ) ) ;
#96111=CARTESIAN_POINT ( 'NONE',  ( -4.379528057220086978, -16.55341960407618274, 49.79275706135234714 ) ) ;
#96112=CARTESIAN_POINT ( 'NONE',  ( -13.89961937509977652, 13.97604488694528158, 90.62390960531432427 ) ) ;
#96113=CARTESIAN_POINT ( 'NONE',  ( -8.314922557961024197, 14.29746914071037800, 42.91775706135235424 ) ) ;
#96114=CARTESIAN_POINT ( 'NONE',  ( 4.483927247898790824, -16.52544592524335698, 25.20942372801901854 ) ) ;
#96115=CARTESIAN_POINT ( 'NONE',  ( 12.06949235617739724, 12.14591786802326823, 101.8760903946857042 ) ) ;
#96116=CARTESIAN_POINT ( 'NONE',  ( 9.564922557961047289, -16.46253265017146816, 110.4177570613523471 ) ) ;
#96117=CARTESIAN_POINT ( 'NONE',  ( -18.62759615963270932, 10.81492255796079327, 105.8322429386476955 ) ) ;
#96118=CARTESIAN_POINT ( 'NONE',  ( 8.224510206698953496, -14.34966873604960469, 107.9155762719810241 ) ) ;
#96119=CARTESIAN_POINT ( 'NONE',  ( 19.03943276465977164, 0.05219959533936151252, 101.2510903946856757 ) ) ;
#96120=CARTESIAN_POINT ( 'NONE',  ( -16.53943276465976808, -0.05219959533934237506, 73.75109039468567573 ) ) ;
#96122=CARTESIAN_POINT ( 'NONE',  ( 5.049401038297881783, 19.05341960407617563, 72.29275706135234714 ) ) ;
#96123=CARTESIAN_POINT ( 'NONE',  ( 12.14591786802309770, 12.06949235617756955, 39.37390960531436690 ) ) ;
#96124=CARTESIAN_POINT ( 'NONE',  ( 14.29746914071049879, -8.314922557960816363, 38.33224293864768839 ) ) ;
#96125=CARTESIAN_POINT ( 'NONE',  ( 12.06949235617757843, -12.14591786802309237, 93.12390960531436690 ) ) ;
#96126=CARTESIAN_POINT ( 'NONE',  ( 19.05341960407617918, -5.049401038297876454, 31.04275706135232227 ) ) ;
#96127=CARTESIAN_POINT ( 'NONE',  ( -16.21995358207303894, 7.366697692864242697, 89.93551001512156517 ) ) ;
#96128=CARTESIAN_POINT ( 'NONE',  ( -5.719274019375665041, -21.55341960407619695, 34.79275706135235424 ) ) ;
#96129=CARTESIAN_POINT ( 'NONE',  ( 19.05341960407617918, -5.049401038297876454, 96.04275706135231871 ) ) ;
#96131=CARTESIAN_POINT ( 'NONE',  ( -9.564922557960796823, -16.46253265017161027, 92.08224293864769550 ) ) ;
#96132=CARTESIAN_POINT ( 'NONE',  ( -19.03943276465977164, 0.05219959533909376836, 91.24890960531436690 ) ) ;
#96133=CARTESIAN_POINT ( 'NONE',  ( -21.55341960407610458, -5.719274019375992779, 56.45724293864768839 ) ) ;
#96134=CARTESIAN_POINT ( 'NONE',  ( 14.34966873604960469, 8.224510206698951720, 89.16557627198102409 ) ) ;
#96135=CARTESIAN_POINT ( 'NONE',  ( -13.89961937509977652, 13.97604488694528158, 70.62390960531432427 ) ) ;
#96136=CARTESIAN_POINT ( 'NONE',  ( -5.153800228976328057, -19.02544592524343514, 27.29057627198103120 ) ) ;
#96137=CARTESIAN_POINT ( 'NONE',  ( -0.05219959533937732626, 21.53943276465977519, 42.50109039468567573 ) ) ;
#96138=CARTESIAN_POINT ( 'NONE',  ( 18.62759615963255655, 10.81492255796105972, 81.66775706135236135 ) ) ;
#96139=CARTESIAN_POINT ( 'NONE',  ( 5.153800228976335163, 19.02544592524342804, 59.79057627198100988 ) ) ;
#96140=CARTESIAN_POINT ( 'NONE',  ( 4.483927247898790824, -16.52544592524335698, 85.20942372801901854 ) ) ;
#96141=CARTESIAN_POINT ( 'NONE',  ( -18.62759615963255300, -10.81492255796106328, 34.16775706135234714 ) ) ;
#96142=CARTESIAN_POINT ( 'NONE',  ( 18.62759615963255655, 10.81492255796105972, 31.66775706135234358 ) ) ;
#96143=CARTESIAN_POINT ( 'NONE',  ( -13.89961937509957401, -13.97604488694547875, 49.37609039468567573 ) ) ;
#96144=CARTESIAN_POINT ( 'NONE',  ( -13.89961937509977652, 13.97604488694528158, 85.62390960531433848 ) ) ;
#96145=CARTESIAN_POINT ( 'NONE',  ( -9.564922557961040184, 16.46253265017147172, 32.91775706135233293 ) ) ;
#96146=CARTESIAN_POINT ( 'NONE',  ( 15.72974639402176855, 15.80617190586768217, 86.87609039468568994 ) ) ;
#96147=CARTESIAN_POINT ( 'NONE',  ( -21.53943276465977519, 0.05219959533907696930, 76.24890960531435269 ) ) ;
#96148=CARTESIAN_POINT ( 'NONE',  ( 4.483927247898545687, 16.52544592524342804, 44.79057627198103120 ) ) ;
#96149=CARTESIAN_POINT ( 'NONE',  ( -0.05219959533937732626, 21.53943276465977519, 92.50109039468567573 ) ) ;
#96150=CARTESIAN_POINT ( 'NONE',  ( 13.89961937509957401, 13.97604488694547697, 26.87609039468566507 ) ) ;
#96151=CARTESIAN_POINT ( 'NONE',  ( -12.14591786802309592, -12.06949235617757132, 71.87390960531438111 ) ) ;
#96152=CARTESIAN_POINT ( 'NONE',  ( -13.89961937509977652, 13.97604488694528158, 25.62390960531434558 ) ) ;
#96153=CARTESIAN_POINT ( 'NONE',  ( 9.474510206698729675, 16.51473224551082808, 67.08442372801900433 ) ) ;
#96154=CARTESIAN_POINT ( 'NONE',  ( 12.14591786802309770, 12.06949235617756955, 34.37390960531435979 ) ) ;
#96155=CARTESIAN_POINT ( 'NONE',  ( -18.67979575497193778, 10.72451020669871902, 83.33442372801903275 ) ) ;
#96156=CARTESIAN_POINT ( 'NONE',  ( 9.564922557960805705, 16.46253265017160317, 74.58224293864769550 ) ) ;
#96157=CARTESIAN_POINT ( 'NONE',  ( -5.049401038297874678, -19.05341960407617918, 49.79275706135231871 ) ) ;
#96158=CARTESIAN_POINT ( 'NONE',  ( 15.72974639402199770, -15.80617190586745480, 48.12390960531436690 ) ) ;
#96159=CARTESIAN_POINT ( 'NONE',  ( -10.81492255796105439, 18.62759615963255655, 22.91775706135235069 ) ) ;
#96160=CARTESIAN_POINT ( 'NONE',  ( 19.02544592524334988, 5.153800228976608722, 106.4594237280190185 ) ) ;
#96161=CARTESIAN_POINT ( 'NONE',  ( -4.379528057220086978, -16.55341960407618274, 69.79275706135234714 ) ) ;
#96162=CARTESIAN_POINT ( 'NONE',  ( 16.61371651742603817, 7.165104196376034018, 63.64584930006999741 ) ) ;
#96163=CARTESIAN_POINT ( 'NONE',  ( -15.80617190586745835, -15.72974639402198527, 106.8739096053143811 ) ) ;
#96164=CARTESIAN_POINT ( 'NONE',  ( 12.14591786802309770, 12.06949235617756955, 109.3739096053143811 ) ) ;
#96165=CARTESIAN_POINT ( 'NONE',  ( -17.50000000000149214, -3.254303733634606566, 29.97604106928586987 ) ) ;
#96166=CARTESIAN_POINT ( 'NONE',  ( 4.379528057220092307, 16.55341960407617563, 37.29275706135235424 ) ) ;
#96167=CARTESIAN_POINT ( 'NONE',  ( 21.52544592524344225, -5.823673210054117533, 63.54057627198103830 ) ) ;
#96168=CARTESIAN_POINT ( 'NONE',  ( -8.314922557961024197, 14.29746914071037800, 102.9177570613523756 ) ) ;
#96169=CARTESIAN_POINT ( 'NONE',  ( 19.03943276465977164, -0.05219959533909143690, 33.74890960531435979 ) ) ;
#96170=CARTESIAN_POINT ( 'NONE',  ( -0.05219959533934338120, 16.53943276465976808, 72.50109039468568994 ) ) ;
#96171=CARTESIAN_POINT ( 'NONE',  ( -19.05341960407617563, 5.049401038297882671, 63.54275706135234003 ) ) ;
#96172=CARTESIAN_POINT ( 'NONE',  ( -10.81492255796105439, 18.62759615963255655, 42.91775706135235424 ) ) ;
#96173=CARTESIAN_POINT ( 'NONE',  ( -18.62759615963270932, 10.81492255796079327, 60.83224293864769550 ) ) ;
#96174=CARTESIAN_POINT ( 'NONE',  ( -8.314922557961024197, 14.29746914071037800, 102.9177570613523756 ) ) ;
#96175=CARTESIAN_POINT ( 'NONE',  ( 10.72451020669871369, 18.67979575497193778, 87.08442372801901854 ) ) ;
#96177=CARTESIAN_POINT ( 'NONE',  ( -15.72974639402197994, 15.80617190586746368, 50.62390960531435979 ) ) ;
#96178=CARTESIAN_POINT ( 'NONE',  ( 10.72451020669898902, -18.67979575497178502, 32.91557627198102409 ) ) ;
#96179=ORIENTED_EDGE ( 'NONE', *, *, #152995, .F. ) ;
#96180=CARTESIAN_POINT ( 'NONE',  ( 4.379528057220092307, 16.55341960407617563, 82.29275706135234714 ) ) ;
#96181=CARTESIAN_POINT ( 'NONE',  ( -18.62759615963270932, 10.81492255796079327, 45.83224293864769550 ) ) ;
#96182=VERTEX_POINT ( 'NONE', #150672 ) ;
#96183=CARTESIAN_POINT ( 'NONE',  ( 16.46253265017160672, -9.564922557960803928, 93.33224293864769550 ) ) ;
#96185=CARTESIAN_POINT ( 'NONE',  ( 13.97604488694527802, 13.89961937509977652, 29.37390960531435979 ) ) ;
#96186=CARTESIAN_POINT ( 'NONE',  ( -18.67979575497178146, -10.72451020669898902, 66.66557627198102409 ) ) ;
#96187=CARTESIAN_POINT ( 'NONE',  ( 14.29746914071037800, 8.314922557961029526, 86.66775706135234714 ) ) ;
#96188=CARTESIAN_POINT ( 'NONE',  ( -5.719274019375665041, -21.55341960407619695, 49.79275706135234714 ) ) ;
#96189=CARTESIAN_POINT ( 'NONE',  ( -5.049401038297874678, -19.05341960407617918, 109.7927570613523187 ) ) ;
#96190=CARTESIAN_POINT ( 'NONE',  ( -0.05219959533910754901, -16.53943276465976808, 107.4989096053143669 ) ) ;
#96191=CARTESIAN_POINT ( 'NONE',  ( 16.46253265017146816, 9.564922557961045513, 111.6677570613523329 ) ) ;
#96192=CARTESIAN_POINT ( 'NONE',  ( 16.51473224551069308, 9.474510206698969483, 44.16557627198103120 ) ) ;
#96194=CARTESIAN_POINT ( 'NONE',  ( -16.51473224551069308, -9.474510206698971260, 91.66557627198103830 ) ) ;
#96195=CARTESIAN_POINT ( 'NONE',  ( -12.14591786802326823, 12.06949235617739902, 78.12609039468570415 ) ) ;
#96196=CARTESIAN_POINT ( 'NONE',  ( -15.72974639402176322, -15.80617190586768395, 109.3760903946857042 ) ) ;
#96197=CARTESIAN_POINT ( 'NONE',  ( 21.53943276465977519, -0.05219959533907433946, 58.74890960531436690 ) ) ;
#96198=CARTESIAN_POINT ( 'NONE',  ( -16.55341960407617563, 4.379528057220093196, 93.54275706135234714 ) ) ;
#96199=CARTESIAN_POINT ( 'NONE',  ( -19.05341960407617563, 5.049401038297882671, 73.54275706135233293 ) ) ;
#96200=CARTESIAN_POINT ( 'NONE',  ( -5.153800228976328057, -19.02544592524343514, 32.29057627198102409 ) ) ;
#96201=CARTESIAN_POINT ( 'NONE',  ( 0.05219959533909260263, 19.03943276465977164, 79.99890960531436690 ) ) ;
#96202=CARTESIAN_POINT ( 'NONE',  ( -16.51473224551069308, -9.474510206698971260, 31.66557627198102054 ) ) ;
#96203=CARTESIAN_POINT ( 'NONE',  ( -19.05341960407617563, 5.049401038297882671, 68.54275706135230450 ) ) ;
#96205=CARTESIAN_POINT ( 'NONE',  ( -13.89961937509977652, 13.97604488694528158, 105.6239096053143527 ) ) ;
#96206=CARTESIAN_POINT ( 'NONE',  ( -12.06949235617756955, 12.14591786802309770, 60.62390960531437401 ) ) ;
#96207=CARTESIAN_POINT ( 'NONE',  ( 18.67979575497178502, 10.72451020669898547, 64.16557627198102409 ) ) ;
#96208=CARTESIAN_POINT ( 'NONE',  ( -17.49999999999998934, 4.640572885337569176, 105.6378816454884060 ) ) ;
#96209=CARTESIAN_POINT ( 'NONE',  ( -5.049401038297874678, -19.05341960407617918, 34.79275706135233293 ) ) ;
#96211=CARTESIAN_POINT ( 'NONE',  ( -5.153800228976328057, -19.02544592524343514, 67.29057627198102409 ) ) ;
#96212=CARTESIAN_POINT ( 'NONE',  ( 19.03943276465977164, -0.05219959533909143690, 68.74890960531436690 ) ) ;
#96213=CARTESIAN_POINT ( 'NONE',  ( 16.55341960407618274, -4.379528057220086978, 46.04275706135234714 ) ) ;
#96216=CARTESIAN_POINT ( 'NONE',  ( 12.06949235617739724, 12.14591786802326823, 81.87609039468568994 ) ) ;
#96217=CARTESIAN_POINT ( 'NONE',  ( 14.34966873604972726, -8.224510206698740333, 60.83442372801901854 ) ) ;
#96218=CARTESIAN_POINT ( 'NONE',  ( -12.14591786802326823, 12.06949235617739902, 38.12609039468567573 ) ) ;
#96219=CARTESIAN_POINT ( 'NONE',  ( -16.51473224551069308, -9.474510206698971260, 51.66557627198102409 ) ) ;
#96221=CARTESIAN_POINT ( 'NONE',  ( -15.80617190586768217, 15.72974639402176855, 53.12609039468568284 ) ) ;
#96222=CARTESIAN_POINT ( 'NONE',  ( 13.89961937509957401, 13.97604488694547697, 66.87609039468567573 ) ) ;
#96223=CARTESIAN_POINT ( 'NONE',  ( -15.80617190586768217, 15.72974639402176855, 93.12609039468568994 ) ) ;
#96224=CARTESIAN_POINT ( 'NONE',  ( 13.89961937509977652, -13.97604488694527269, 28.12390960531435624 ) ) ;
#96225=CARTESIAN_POINT ( 'NONE',  ( 19.49671883438229614, 5.499999999999975131, 42.39279849105686537 ) ) ;
#96226=CARTESIAN_POINT ( 'NONE',  ( 15.80617190586746368, 15.72974639402197994, 59.37390960531436690 ) ) ;
#96227=AXIS2_PLACEMENT_3D ( 'NONE', #26346, #87986, #70837 ) ;
#96228=CARTESIAN_POINT ( 'NONE',  ( -9.564922557960796823, -16.46253265017161027, 102.0822429386477097 ) ) ;
#96229=CARTESIAN_POINT ( 'NONE',  ( -16.53943276465976808, 0.05219959533911058130, 106.2489096053143811 ) ) ;
#96230=CARTESIAN_POINT ( 'NONE',  ( -8.224510206698735004, -14.34966873604973081, 34.58442372801900433 ) ) ;
#96231=CARTESIAN_POINT ( 'NONE',  ( -16.55341960407617563, 4.379528057220093196, 113.5427570613523756 ) ) ;
#96233=CARTESIAN_POINT ( 'NONE',  ( -10.81492255796078084, -18.62759615963271287, 107.0822429386476955 ) ) ;
#96234=CARTESIAN_POINT ( 'NONE',  ( 4.379528057220339221, -16.55341960407611168, 32.70724293864770260 ) ) ;
#96235=CARTESIAN_POINT ( 'NONE',  ( 19.02544592524343514, -5.153800228976328945, 113.5405762719810241 ) ) ;
#96236=CARTESIAN_POINT ( 'NONE',  ( 13.89961937509957401, 13.97604488694547697, 91.87609039468567573 ) ) ;
#96237=CARTESIAN_POINT ( 'NONE',  ( 0.05219959533936267826, -19.03943276465977164, 30.00109039468566863 ) ) ;
#96238=CARTESIAN_POINT ( 'NONE',  ( 4.379528057220339221, -16.55341960407611168, 32.70724293864770260 ) ) ;
#96239=CARTESIAN_POINT ( 'NONE',  ( 21.53943276465977519, -0.05219959533907433946, 88.74890960531436690 ) ) ;
#96240=CARTESIAN_POINT ( 'NONE',  ( -21.55341960407610458, -5.719274019375992779, 46.45724293864769550 ) ) ;
#96241=CARTESIAN_POINT ( 'NONE',  ( 16.46253265017160672, -9.564922557960803928, 83.33224293864768129 ) ) ;
#96242=CARTESIAN_POINT ( 'NONE',  ( 4.483927247898545687, 16.52544592524342804, 39.79057627198103830 ) ) ;
#96243=CARTESIAN_POINT ( 'NONE',  ( -16.51473224551069308, -9.474510206698971260, 86.66557627198102409 ) ) ;
#96244=CARTESIAN_POINT ( 'NONE',  ( 19.39720447994797325, 5.499999999999975131, 57.16317477297181426 ) ) ;
#96245=CARTESIAN_POINT ( 'NONE',  ( -5.049401038297874678, -19.05341960407617918, 44.79275706135232582 ) ) ;
#96246=CARTESIAN_POINT ( 'NONE',  ( -5.823673210054116645, -21.52544592524344225, 82.29057627198103830 ) ) ;
#96247=CARTESIAN_POINT ( 'NONE',  ( -16.55341960407611168, -4.379528057220339221, 106.4572429386477097 ) ) ;
#96248=CARTESIAN_POINT ( 'NONE',  ( -18.62759615963255300, -10.81492255796106328, 39.16775706135235424 ) ) ;
#96251=CARTESIAN_POINT ( 'NONE',  ( -14.34966873604972548, 8.224510206698743886, 103.3344237280190043 ) ) ;
#96252=CARTESIAN_POINT ( 'NONE',  ( -5.049401038298153566, 19.05341960407611168, 40.20724293864768839 ) ) ;
#96253=CARTESIAN_POINT ( 'NONE',  ( -9.564922557960796823, -16.46253265017161027, 92.08224293864769550 ) ) ;
#96255=CARTESIAN_POINT ( 'NONE',  ( -0.05219959533909027116, -19.03943276465977164, 32.49890960531435979 ) ) ;
#96256=CARTESIAN_POINT ( 'NONE',  ( 16.53943276465976808, -0.05219959533910856209, 43.74890960531435979 ) ) ;
#96258=CARTESIAN_POINT ( 'NONE',  ( -5.719274019375665041, -21.55341960407619695, 79.79275706135236135 ) ) ;
#96260=CARTESIAN_POINT ( 'NONE',  ( 8.314922557961029526, -14.29746914071037800, 75.41775706135233293 ) ) ;
#96261=CARTESIAN_POINT ( 'NONE',  ( 9.564922557960805705, 16.46253265017160317, 54.58224293864769550 ) ) ;
#96262=CARTESIAN_POINT ( 'NONE',  ( 5.153800228976335163, 19.02544592524342804, 64.79057627198100988 ) ) ;
#96264=CARTESIAN_POINT ( 'NONE',  ( 5.823673210054444382, -21.52544592524334988, 105.2094237280190328 ) ) ;
#96265=CARTESIAN_POINT ( 'NONE',  ( -4.483927247898782831, 16.52544592524335698, 72.70942372801901854 ) ) ;
#96266=CARTESIAN_POINT ( 'NONE',  ( 0.05219959533937995610, -21.53943276465977519, 105.0010903946856757 ) ) ;
#96267=CARTESIAN_POINT ( 'NONE',  ( -0.05219959533909027116, -19.03943276465977164, 57.49890960531435979 ) ) ;
#96268=CARTESIAN_POINT ( 'NONE',  ( -18.67979575497178146, -10.72451020669898902, 31.66557627198102054 ) ) ;
#96269=CARTESIAN_POINT ( 'NONE',  ( 9.474510206698729675, 16.51473224551082808, 107.0844237280190043 ) ) ;
#96270=CARTESIAN_POINT ( 'NONE',  ( 15.72974639402176855, 15.80617190586768217, 66.87609039468568994 ) ) ;
#96271=CARTESIAN_POINT ( 'NONE',  ( -4.483927247898782831, 16.52544592524335698, 52.70942372801902565 ) ) ;
#96272=CARTESIAN_POINT ( 'NONE',  ( 15.80617190586746368, 15.72974639402197994, 99.37390960531436690 ) ) ;
#96273=CARTESIAN_POINT ( 'NONE',  ( 0.05219959533936267826, -19.03943276465977164, 100.0010903946856757 ) ) ;
#96274=CARTESIAN_POINT ( 'NONE',  ( 16.51473224551069308, 9.474510206698969483, 84.16557627198102409 ) ) ;
#96275=CARTESIAN_POINT ( 'NONE',  ( 19.02544592524334988, 5.153800228976608722, 106.4594237280190185 ) ) ;
#96276=CARTESIAN_POINT ( 'NONE',  ( 16.53943276465976808, 0.05219959533934440121, 26.25109039468567573 ) ) ;
#96277=CARTESIAN_POINT ( 'NONE',  ( -12.06949235617756955, 12.14591786802309770, 65.62390960531436690 ) ) ;
#96278=CARTESIAN_POINT ( 'NONE',  ( 8.314922557961029526, -14.29746914071037800, 80.41775706135234714 ) ) ;
#96279=CARTESIAN_POINT ( 'NONE',  ( -0.05219959533907301413, -21.53943276465977519, 112.4989096053143669 ) ) ;
#96280=CARTESIAN_POINT ( 'NONE',  ( -16.51473224551069308, -9.474510206698971260, 51.66557627198102409 ) ) ;
#96281=CARTESIAN_POINT ( 'NONE',  ( -5.153800228976328057, -19.02544592524343514, 57.29057627198103120 ) ) ;
#96282=CARTESIAN_POINT ( 'NONE',  ( -12.14591786802326823, 12.06949235617739902, 78.12609039468570415 ) ) ;
#96285=CARTESIAN_POINT ( 'NONE',  ( -18.67979575497193778, 10.72451020669871902, 113.3344237280190328 ) ) ;
#96286=CARTESIAN_POINT ( 'NONE',  ( 19.05341960407611168, 5.049401038298154454, 33.95724293864769550 ) ) ;
#96288=CARTESIAN_POINT ( 'NONE',  ( 16.52544592524335698, 4.483927247898782831, 21.45942372801901499 ) ) ;
#96289=CARTESIAN_POINT ( 'NONE',  ( 9.564922557961047289, -16.46253265017146816, 50.41775706135233293 ) ) ;
#96290=CARTESIAN_POINT ( 'NONE',  ( 14.29746914071037800, 8.314922557961029526, 31.66775706135234358 ) ) ;
#96291=CARTESIAN_POINT ( 'NONE',  ( -16.46253265017160317, 9.564922557960807481, 40.83224293864769550 ) ) ;
#96292=CARTESIAN_POINT ( 'NONE',  ( -13.89961937509977652, 13.97604488694528158, 70.62390960531432427 ) ) ;
#96293=CARTESIAN_POINT ( 'NONE',  ( -5.823673210054116645, -21.52544592524344225, 92.29057627198103830 ) ) ;
#96294=CARTESIAN_POINT ( 'NONE',  ( -5.049401038298153566, 19.05341960407611168, 115.2072429386477097 ) ) ;
#96296=CARTESIAN_POINT ( 'NONE',  ( 13.97604488694527802, 13.89961937509977652, 54.37390960531435979 ) ) ;
#96298=CARTESIAN_POINT ( 'NONE',  ( 13.97604488694548053, -13.89961937509957401, 100.6260903946856615 ) ) ;
#96299=CARTESIAN_POINT ( 'NONE',  ( 12.06949235617757843, -12.14591786802309237, 68.12390960531436690 ) ) ;
#96300=CARTESIAN_POINT ( 'NONE',  ( -19.03943276465977164, -0.05219959533935918106, 28.75109039468566507 ) ) ;
#96301=CARTESIAN_POINT ( 'NONE',  ( 16.52544592524342804, -4.483927247898539470, 63.54057627198103830 ) ) ;
#96302=CARTESIAN_POINT ( 'NONE',  ( -18.62759615963255300, -10.81492255796106328, 89.16775706135236135 ) ) ;
#96303=CARTESIAN_POINT ( 'NONE',  ( -13.97604488694527625, -13.89961937509977652, 26.87390960531434558 ) ) ;
#96304=CARTESIAN_POINT ( 'NONE',  ( 15.72974639402176855, 15.80617190586768217, 86.87609039468568994 ) ) ;
#96305=CARTESIAN_POINT ( 'NONE',  ( -4.379528057220328563, 16.55341960407611168, 30.20724293864769550 ) ) ;
#96306=CARTESIAN_POINT ( 'NONE',  ( 21.53943276465977519, 0.05219959533937863772, 71.25109039468568994 ) ) ;
#96307=CARTESIAN_POINT ( 'NONE',  ( 9.564922557960805705, 16.46253265017160317, 79.58224293864769550 ) ) ;
#96308=CARTESIAN_POINT ( 'NONE',  ( -21.53943276465977519, -0.05219959533937600094, 38.75109039468567573 ) ) ;
#96309=CARTESIAN_POINT ( 'NONE',  ( 16.46253265017160672, -9.564922557960803928, 83.33224293864768129 ) ) ;
#96310=CARTESIAN_POINT ( 'NONE',  ( 14.34966873604960469, 8.224510206698951720, 99.16557627198100988 ) ) ;
#96311=CARTESIAN_POINT ( 'NONE',  ( 16.55341960407611168, 4.379528057220329451, 63.95724293864770260 ) ) ;
#96312=CARTESIAN_POINT ( 'NONE',  ( 10.72451020669898902, -18.67979575497178502, 67.91557627198102409 ) ) ;
#96313=CARTESIAN_POINT ( 'NONE',  ( 13.97604488694527802, 13.89961937509977652, 79.37390960531435269 ) ) ;
#96314=CARTESIAN_POINT ( 'NONE',  ( -18.62759615963270932, 10.81492255796079327, 80.83224293864769550 ) ) ;
#96315=CARTESIAN_POINT ( 'NONE',  ( 9.474510206698729675, 16.51473224551082808, 62.08442372801899722 ) ) ;
#96316=CARTESIAN_POINT ( 'NONE',  ( 5.049401038297881783, 19.05341960407617918, 37.29275706135232582 ) ) ;
#96317=CARTESIAN_POINT ( 'NONE',  ( -14.29746914071049879, 8.314922557960819915, 75.83224293864769550 ) ) ;
#96318=CARTESIAN_POINT ( 'NONE',  ( 21.52544592524344225, -5.823673210054117533, 53.54057627198103120 ) ) ;
#96320=CARTESIAN_POINT ( 'NONE',  ( -8.314922557961024197, 14.29746914071037800, 92.91775706135236135 ) ) ;
#96322=CARTESIAN_POINT ( 'NONE',  ( 16.51473224551083163, -9.474510206698727899, 100.8344237280190043 ) ) ;
#96323=CARTESIAN_POINT ( 'NONE',  ( 8.314922557960818139, 14.29746914071049879, 64.58224293864769550 ) ) ;
#96325=CARTESIAN_POINT ( 'NONE',  ( 13.97604488694527802, 13.89961937509977652, 64.37390960531436690 ) ) ;
#96326=CARTESIAN_POINT ( 'NONE',  ( -4.379528057220328563, 16.55341960407611168, 60.20724293864768839 ) ) ;
#96327=CARTESIAN_POINT ( 'NONE',  ( -19.03943276465977164, 0.05219959533909376836, 106.2489096053143669 ) ) ;
#96328=CARTESIAN_POINT ( 'NONE',  ( 9.564922557961047289, -16.46253265017146816, 85.41775706135233293 ) ) ;
#96329=CARTESIAN_POINT ( 'NONE',  ( 13.97604488694527802, 13.89961937509977652, 69.37390960531436690 ) ) ;
#96330=CARTESIAN_POINT ( 'NONE',  ( 9.564922557960805705, 16.46253265017160317, 79.58224293864769550 ) ) ;
#96331=CARTESIAN_POINT ( 'NONE',  ( -19.02544592524342804, 5.153800228976336051, 91.04057627198100988 ) ) ;
#96332=CARTESIAN_POINT ( 'NONE',  ( 10.72451020669898902, -18.67979575497178502, 57.91557627198103120 ) ) ;
#96333=CARTESIAN_POINT ( 'NONE',  ( -16.53943276465976808, -0.05219959533934237506, 63.75109039468568284 ) ) ;
#96334=CARTESIAN_POINT ( 'NONE',  ( -19.03943276465977164, -0.05219959533935918106, 103.7510903946856757 ) ) ;
#96335=CARTESIAN_POINT ( 'NONE',  ( -16.51473224551069308, -9.474510206698971260, 51.66557627198102409 ) ) ;
#96336=CARTESIAN_POINT ( 'NONE',  ( 21.55341960407610458, 5.719274019375980345, 68.95724293864769550 ) ) ;
#96337=CARTESIAN_POINT ( 'NONE',  ( 9.474510206698729675, 16.51473224551082808, 97.08442372801900433 ) ) ;
#96338=CARTESIAN_POINT ( 'NONE',  ( 14.29746914071037800, 8.314922557961029526, 111.6677570613523613 ) ) ;
#96339=CARTESIAN_POINT ( 'NONE',  ( -15.80617190586768217, 15.72974639402176855, 43.12609039468568284 ) ) ;
#96340=CARTESIAN_POINT ( 'NONE',  ( -19.03943276465977164, -0.05219959533935918106, 38.75109039468566152 ) ) ;
#96341=CARTESIAN_POINT ( 'NONE',  ( 14.34966873604972726, -8.224510206698740333, 55.83442372801901854 ) ) ;
#96342=CARTESIAN_POINT ( 'NONE',  ( 14.34966873604972726, -8.224510206698740333, 95.83442372801903275 ) ) ;
#96344=CARTESIAN_POINT ( 'NONE',  ( 12.06949235617739724, 12.14591786802326823, 76.87609039468567573 ) ) ;
#96345=CARTESIAN_POINT ( 'NONE',  ( -12.06949235617739369, -12.14591786802326823, 34.37609039468568284 ) ) ;
#96346=CARTESIAN_POINT ( 'NONE',  ( -5.153800228976328057, -19.02544592524343514, 47.29057627198102409 ) ) ;
#96347=CARTESIAN_POINT ( 'NONE',  ( 19.05341960407611168, 5.049401038298154454, 48.95724293864768129 ) ) ;
#96348=CARTESIAN_POINT ( 'NONE',  ( 16.51473224551069308, 9.474510206698969483, 64.16557627198102409 ) ) ;
#96349=CARTESIAN_POINT ( 'NONE',  ( 18.67979575497194134, -10.72451020669871369, 55.83442372801901854 ) ) ;
#96350=CARTESIAN_POINT ( 'NONE',  ( 16.53943276465976808, 0.05219959533934440121, 51.25109039468568994 ) ) ;
#96351=CARTESIAN_POINT ( 'NONE',  ( 16.53943276465976808, -0.05219959533910856209, 23.74890960531435269 ) ) ;
#96352=CARTESIAN_POINT ( 'NONE',  ( -19.05341960407611168, -5.049401038298163336, 26.45724293864769550 ) ) ;
#96353=CARTESIAN_POINT ( 'NONE',  ( -15.80617190586768217, 15.72974639402176855, 113.1260903946856899 ) ) ;
#96354=CARTESIAN_POINT ( 'NONE',  ( -16.53943276465976808, -0.05219959533934237506, 23.75109039468567929 ) ) ;
#96355=CARTESIAN_POINT ( 'NONE',  ( 13.89961937509957401, 13.97604488694547697, 86.87609039468567573 ) ) ;
#96356=CARTESIAN_POINT ( 'NONE',  ( 16.53943276465976808, -0.05219959533910856209, 83.74890960531435269 ) ) ;
#96357=CARTESIAN_POINT ( 'NONE',  ( 13.89961937509977652, -13.97604488694527269, 33.12390960531434558 ) ) ;
#96358=CARTESIAN_POINT ( 'NONE',  ( -19.03943276465977164, -0.05219959533935918106, 73.75109039468566152 ) ) ;
#96359=CARTESIAN_POINT ( 'NONE',  ( 17.26172910966778673, 6.454744622555869782, 76.69353091350774321 ) ) ;
#96360=CARTESIAN_POINT ( 'NONE',  ( -5.719274019375665041, -21.55341960407619695, 74.79275706135234714 ) ) ;
#96361=CARTESIAN_POINT ( 'NONE',  ( 16.55341960407618274, -4.379528057220086978, 46.04275706135234714 ) ) ;
#96362=CARTESIAN_POINT ( 'NONE',  ( 16.19135201231368981, 7.376712067591805422, 37.68680854052031037 ) ) ;
#96363=CARTESIAN_POINT ( 'NONE',  ( 5.823673210054125526, 21.52544592524343514, 34.79057627198103120 ) ) ;
#96364=CARTESIAN_POINT ( 'NONE',  ( 4.379528057220092307, 16.55341960407617563, 32.29275706135235424 ) ) ;
#96365=CARTESIAN_POINT ( 'NONE',  ( 16.46253265017160672, -9.564922557960803928, 28.33224293864769550 ) ) ;
#96366=CARTESIAN_POINT ( 'NONE',  ( 5.049401038297881783, 19.05341960407617563, 27.29275706135232937 ) ) ;
#96368=CARTESIAN_POINT ( 'NONE',  ( 5.153800228976335163, 19.02544592524342804, 44.79057627198103830 ) ) ;
#96370=CARTESIAN_POINT ( 'NONE',  ( -19.05341960407611168, -5.049401038298163336, 71.45724293864766707 ) ) ;
#96371=CARTESIAN_POINT ( 'NONE',  ( -19.49671883438229258, -5.499999999999978684, 54.89279849105684406 ) ) ;
#96372=EDGE_CURVE ( 'NONE', #98417, #121093, #127249, .T. ) ;
#96373=CARTESIAN_POINT ( 'NONE',  ( -13.89961937509957401, -13.97604488694547875, 24.37609039468565442 ) ) ;
#96374=CARTESIAN_POINT ( 'NONE',  ( -8.314922557960811034, -14.29746914071050412, 37.08224293864768129 ) ) ;
#96375=CARTESIAN_POINT ( 'NONE',  ( -19.03943276465977164, 0.05219959533909376836, 41.24890960531435269 ) ) ;
#96376=CARTESIAN_POINT ( 'NONE',  ( -0.05219959533909027116, -19.03943276465977164, 92.49890960531436690 ) ) ;
#96377=CARTESIAN_POINT ( 'NONE',  ( -15.72974639402176322, -15.80617190586768395, 64.37609039468568994 ) ) ;
#96378=CARTESIAN_POINT ( 'NONE',  ( 13.97604488694527802, 13.89961937509977652, 49.37390960531434558 ) ) ;
#96379=CARTESIAN_POINT ( 'NONE',  ( 15.80617190586769283, -15.72974639402175789, 60.62609039468567573 ) ) ;
#96380=CARTESIAN_POINT ( 'NONE',  ( -21.53943276465977519, 0.05219959533907696930, 21.24890960531436690 ) ) ;
#96381=CARTESIAN_POINT ( 'NONE',  ( -19.02544592524342804, 5.153800228976336051, 41.04057627198103120 ) ) ;
#96382=CARTESIAN_POINT ( 'NONE',  ( 10.81492255796106328, -18.62759615963255655, 30.41775706135234358 ) ) ;
#96383=CARTESIAN_POINT ( 'NONE',  ( 0.05219959533936267826, -19.03943276465977164, 45.00109039468566863 ) ) ;
#96384=CARTESIAN_POINT ( 'NONE',  ( -12.14591786802309592, -12.06949235617757132, 111.8739096053143669 ) ) ;
#96385=CARTESIAN_POINT ( 'NONE',  ( 16.46253265017160672, -9.564922557960803928, 58.33224293864769550 ) ) ;
#96386=CARTESIAN_POINT ( 'NONE',  ( 19.02544592524334988, 5.153800228976608722, 106.4594237280190185 ) ) ;
#96387=CARTESIAN_POINT ( 'NONE',  ( 12.06949235617757843, -12.14591786802309237, 78.12390960531436690 ) ) ;
#96388=CARTESIAN_POINT ( 'NONE',  ( 19.03943276465977164, -0.05219959533909143690, 113.7489096053143669 ) ) ;
#96389=CARTESIAN_POINT ( 'NONE',  ( -19.03943276465977164, -0.05219959533935918106, 98.75109039468567573 ) ) ;
#96390=CARTESIAN_POINT ( 'NONE',  ( -5.823673210054116645, -21.52544592524344225, 102.2905762719810383 ) ) ;
#96391=CARTESIAN_POINT ( 'NONE',  ( 21.52544592524334988, 5.823673210054432836, 61.45942372801901854 ) ) ;
#96392=CARTESIAN_POINT ( 'NONE',  ( -16.53943276465976808, -0.05219959533934237506, 58.75109039468568994 ) ) ;
#96393=CARTESIAN_POINT ( 'NONE',  ( 4.483927247898790824, -16.52544592524335698, 55.20942372801902565 ) ) ;
#96394=CARTESIAN_POINT ( 'NONE',  ( -5.719274019375978568, 21.55341960407610458, 50.20724293864769550 ) ) ;
#96395=CARTESIAN_POINT ( 'NONE',  ( 13.89961937509977652, -13.97604488694527269, 43.12390960531434558 ) ) ;
#96396=CARTESIAN_POINT ( 'NONE',  ( 8.314922557961029526, -14.29746914071037800, 70.41775706135236135 ) ) ;
#96397=AXIS2_PLACEMENT_3D ( 'NONE', #157882, #142695, #68853 ) ;
#96398=CARTESIAN_POINT ( 'NONE',  ( 21.55341960407610458, 5.719274019375980345, 98.95724293864770971 ) ) ;
#96399=CARTESIAN_POINT ( 'NONE',  ( 14.29746914071049879, -8.314922557960816363, 58.33224293864768839 ) ) ;
#96400=CARTESIAN_POINT ( 'NONE',  ( 19.02544592524343514, -5.153800228976328945, 78.54057627198099567 ) ) ;
#96401=CARTESIAN_POINT ( 'NONE',  ( -12.06949235617739369, -12.14591786802326823, 74.37609039468568994 ) ) ;
#96402=CARTESIAN_POINT ( 'NONE',  ( -5.049401038297874678, -19.05341960407617918, 104.7927570613523471 ) ) ;
#96403=CARTESIAN_POINT ( 'NONE',  ( 18.67979575497178502, 10.72451020669898547, 104.1655762719810241 ) ) ;
#96404=CARTESIAN_POINT ( 'NONE',  ( 12.14591786802309770, 12.06949235617756955, 44.37390960531435979 ) ) ;
#96406=CARTESIAN_POINT ( 'NONE',  ( -16.88567814943163015, 6.947325034625698947, 73.70998877347417988 ) ) ;
#96407=CARTESIAN_POINT ( 'NONE',  ( 21.53943276465977519, -0.05219959533907433946, 83.74890960531435269 ) ) ;
#96408=CARTESIAN_POINT ( 'NONE',  ( 12.14591786802309770, 12.06949235617756955, 24.37390960531435979 ) ) ;
#96411=CARTESIAN_POINT ( 'NONE',  ( -21.55341960407610458, -5.719274019375992779, 96.45724293864770971 ) ) ;
#96412=CARTESIAN_POINT ( 'NONE',  ( 13.97604488694527802, 13.89961937509977652, 94.37390960531436690 ) ) ;
#96413=CARTESIAN_POINT ( 'NONE',  ( -18.62759615963255300, -10.81492255796106328, 29.16775706135234003 ) ) ;
#96414=CARTESIAN_POINT ( 'NONE',  ( 14.34966873604960469, 8.224510206698951720, 44.16557627198103120 ) ) ;
#96415=CARTESIAN_POINT ( 'NONE',  ( 16.52544592524335698, 4.483927247898782831, 51.45942372801901854 ) ) ;
#96416=CARTESIAN_POINT ( 'NONE',  ( -16.51473224551069308, -9.474510206698971260, 41.66557627198103120 ) ) ;
#96417=CARTESIAN_POINT ( 'NONE',  ( 19.05341960407617918, -5.049401038297876454, 56.04275706135234714 ) ) ;
#96418=CARTESIAN_POINT ( 'NONE',  ( -9.564922557960796823, -16.46253265017161027, 77.08224293864769550 ) ) ;
#96420=CARTESIAN_POINT ( 'NONE',  ( 15.80617190586746368, 15.72974639402197994, 29.37390960531435269 ) ) ;
#96422=CARTESIAN_POINT ( 'NONE',  ( 4.379528057220092307, 16.55341960407617563, 27.29275706135234358 ) ) ;
#96423=CARTESIAN_POINT ( 'NONE',  ( 9.564922557961047289, -16.46253265017146816, 55.41775706135234003 ) ) ;
#96424=CARTESIAN_POINT ( 'NONE',  ( -21.55341960407610458, -5.719274019375992779, 106.4572429386477097 ) ) ;
#96425=CARTESIAN_POINT ( 'NONE',  ( 12.06949235617757843, -12.14591786802309237, 38.12390960531436690 ) ) ;
#96426=CARTESIAN_POINT ( 'NONE',  ( -13.89961937509977652, 13.97604488694528158, 80.62390960531436690 ) ) ;
#96427=CARTESIAN_POINT ( 'NONE',  ( 18.67979575497178502, 10.72451020669898547, 54.16557627198103120 ) ) ;
#96428=CARTESIAN_POINT ( 'NONE',  ( 18.67979575497178502, 10.72451020669898547, 89.16557627198102409 ) ) ;
#96429=CARTESIAN_POINT ( 'NONE',  ( -8.224510206698735004, -14.34966873604973081, 29.58442372801901854 ) ) ;
#96430=CARTESIAN_POINT ( 'NONE',  ( 10.72451020669898902, -18.67979575497178502, 22.91557627198102765 ) ) ;
#96431=CARTESIAN_POINT ( 'NONE',  ( -10.81492255796105439, 18.62759615963255655, 87.91775706135234714 ) ) ;
#96432=CARTESIAN_POINT ( 'NONE',  ( -9.564922557960796823, -16.46253265017161027, 72.08224293864770971 ) ) ;
#96433=CARTESIAN_POINT ( 'NONE',  ( 19.02544592524343514, -5.153800228976328945, 28.54057627198102409 ) ) ;
#96434=CARTESIAN_POINT ( 'NONE',  ( 19.03943276465977164, -0.05219959533909143690, 83.74890960531436690 ) ) ;
#96435=CARTESIAN_POINT ( 'NONE',  ( -0.05219959533910754901, -16.53943276465976808, 102.4989096053143811 ) ) ;
#96436=CARTESIAN_POINT ( 'NONE',  ( 13.97604488694548053, -13.89961937509957401, 100.6260903946856615 ) ) ;
#96438=CARTESIAN_POINT ( 'NONE',  ( 9.474510206698971260, -16.51473224551069308, 67.91557627198102409 ) ) ;
#96439=CARTESIAN_POINT ( 'NONE',  ( 18.67979575497194134, -10.72451020669871369, 95.83442372801903275 ) ) ;
#96440=CARTESIAN_POINT ( 'NONE',  ( 19.02544592524343514, -5.153800228976328945, 113.5405762719810241 ) ) ;
#96441=CARTESIAN_POINT ( 'NONE',  ( 4.379528057220092307, 16.55341960407617563, 92.29275706135236135 ) ) ;
#96443=CARTESIAN_POINT ( 'NONE',  ( -0.05219959533936034679, 19.03943276465977164, 62.50109039468566863 ) ) ;
#96444=CARTESIAN_POINT ( 'NONE',  ( 19.03943276465977164, 0.05219959533936151252, 21.25109039468565797 ) ) ;
#96446=CARTESIAN_POINT ( 'NONE',  ( -13.97604488694527625, -13.89961937509977652, 31.87390960531435979 ) ) ;
#96447=CARTESIAN_POINT ( 'NONE',  ( 16.52544592524335698, 4.483927247898782831, 111.4594237280190328 ) ) ;
#96448=DIRECTION ( 'NONE',  ( -1.000000000000000000, -0.000000000000000000, -0.000000000000000000 ) ) ;
#96449=CARTESIAN_POINT ( 'NONE',  ( 14.34966873604972726, -8.224510206698740333, 105.8344237280190328 ) ) ;
#96451=CARTESIAN_POINT ( 'NONE',  ( 8.224510206698742110, 14.34966873604972548, 77.08442372801901854 ) ) ;
#96452=CARTESIAN_POINT ( 'NONE',  ( 5.049401038298161559, -19.05341960407611168, 37.70724293864768839 ) ) ;
#96453=CARTESIAN_POINT ( 'NONE',  ( 0.05219959533937995610, -21.53943276465977519, 100.0010903946857042 ) ) ;
#96454=CARTESIAN_POINT ( 'NONE',  ( 16.46253265017146816, 9.564922557961045513, 106.6677570613523471 ) ) ;
#96455=CARTESIAN_POINT ( 'NONE',  ( 18.67979575497194134, -10.72451020669871369, 65.83442372801900433 ) ) ;
#96456=CARTESIAN_POINT ( 'NONE',  ( -16.51473224551082808, 9.474510206698731452, 53.33442372801900433 ) ) ;
#96457=CARTESIAN_POINT ( 'NONE',  ( -5.049401038298153566, 19.05341960407611168, 80.20724293864769550 ) ) ;
#96458=CARTESIAN_POINT ( 'NONE',  ( -5.049401038298153566, 19.05341960407611168, 65.20724293864765286 ) ) ;
#96459=CARTESIAN_POINT ( 'NONE',  ( 17.50000000000000000, 5.499999999999992895, 71.70309617465829888 ) ) ;
#96460=CARTESIAN_POINT ( 'NONE',  ( -0.05219959533907301413, -21.53943276465977519, 42.49890960531435979 ) ) ;
#96461=CARTESIAN_POINT ( 'NONE',  ( -13.89961937509977652, 13.97604488694528158, 40.62390960531435979 ) ) ;
#96462=CARTESIAN_POINT ( 'NONE',  ( -18.62759615963270932, 10.81492255796079327, 80.83224293864769550 ) ) ;
#96463=CARTESIAN_POINT ( 'NONE',  ( 16.55341960407618274, -4.379528057220086978, 76.04275706135237556 ) ) ;
#96464=VERTEX_POINT ( 'NONE', #94935 ) ;
#96465=CARTESIAN_POINT ( 'NONE',  ( 12.14591786802309770, 12.06949235617756955, 74.37390960531436690 ) ) ;
#96467=CARTESIAN_POINT ( 'NONE',  ( -14.29746914071037622, -8.314922557961029526, 34.16775706135234714 ) ) ;
#96468=CARTESIAN_POINT ( 'NONE',  ( 13.89961937509977652, -13.97604488694527269, 23.12390960531436335 ) ) ;
#96469=CARTESIAN_POINT ( 'NONE',  ( -13.97604488694547697, 13.89961937509957934, 63.12609039468566152 ) ) ;
#96470=CARTESIAN_POINT ( 'NONE',  ( 8.314922557960818139, 14.29746914071049879, 74.58224293864768129 ) ) ;
#96471=CARTESIAN_POINT ( 'NONE',  ( 10.72451020669871369, 18.67979575497193778, 47.08442372801901854 ) ) ;
#96472=CARTESIAN_POINT ( 'NONE',  ( -13.97604488694527625, -13.89961937509977652, 21.87390960531435979 ) ) ;
#96473=CARTESIAN_POINT ( 'NONE',  ( -10.81492255796078084, -18.62759615963271287, 92.08224293864769550 ) ) ;
#96475=CARTESIAN_POINT ( 'NONE',  ( -16.52544592524342804, 4.483927247898546575, 71.04057627198103830 ) ) ;
#96477=CARTESIAN_POINT ( 'NONE',  ( 13.89961937509977652, -13.97604488694527269, 48.12390960531435979 ) ) ;
#96479=CARTESIAN_POINT ( 'NONE',  ( 19.02544592524334988, 5.153800228976608722, 81.45942372801897591 ) ) ;
#96480=CARTESIAN_POINT ( 'NONE',  ( -18.67979575497193778, 10.72451020669871902, 23.33442372801901499 ) ) ;
#96481=CARTESIAN_POINT ( 'NONE',  ( 19.03943276465977164, -0.05219959533909143690, 73.74890960531435269 ) ) ;
#96482=CARTESIAN_POINT ( 'NONE',  ( 16.51473224551083163, -9.474510206698727899, 50.83442372801899722 ) ) ;
#96483=CARTESIAN_POINT ( 'NONE',  ( -19.02544592524342804, 5.153800228976336051, 41.04057627198103120 ) ) ;
#96484=CARTESIAN_POINT ( 'NONE',  ( 14.34966873604960469, 8.224510206698951720, 64.16557627198102409 ) ) ;
#96485=CARTESIAN_POINT ( 'NONE',  ( 0.05219959533910956823, 16.53943276465976808, 49.99890960531437401 ) ) ;
#96486=CARTESIAN_POINT ( 'NONE',  ( -19.03943276465977164, 0.05219959533909376836, 76.24890960531435269 ) ) ;
#96487=CARTESIAN_POINT ( 'NONE',  ( -10.81492255796078084, -18.62759615963271287, 102.0822429386476955 ) ) ;
#96488=CARTESIAN_POINT ( 'NONE',  ( -16.46253265017160317, 9.564922557960807481, 75.83224293864769550 ) ) ;
#96489=CARTESIAN_POINT ( 'NONE',  ( 0.05219959533907565091, 21.53943276465977519, 74.99890960531435269 ) ) ;
#96490=CARTESIAN_POINT ( 'NONE',  ( 9.564922557961047289, -16.46253265017146816, 20.41775706135233293 ) ) ;
#96491=CARTESIAN_POINT ( 'NONE',  ( 5.153800228976335163, 19.02544592524342804, 24.79057627198102765 ) ) ;
#96492=CARTESIAN_POINT ( 'NONE',  ( -0.05219959533934338120, 16.53943276465976808, 112.5010903946857042 ) ) ;
#96493=CARTESIAN_POINT ( 'NONE',  ( 8.224510206698953496, -14.34966873604960469, 97.91557627198103830 ) ) ;
#96494=CARTESIAN_POINT ( 'NONE',  ( 9.564922557961047289, -16.46253265017146816, 105.4177570613523471 ) ) ;
#96496=CARTESIAN_POINT ( 'NONE',  ( -21.55341960407619339, 5.719274019375674811, 28.54275706135234358 ) ) ;
#96497=CARTESIAN_POINT ( 'NONE',  ( 16.46253265017146816, 9.564922557961045513, 46.66775706135233293 ) ) ;
#96498=CARTESIAN_POINT ( 'NONE',  ( -12.14591786802309592, -12.06949235617757132, 21.87390960531436690 ) ) ;
#96499=CARTESIAN_POINT ( 'NONE',  ( -21.55341960407610458, -5.719274019375992779, 71.45724293864769550 ) ) ;
#96500=CARTESIAN_POINT ( 'NONE',  ( 16.46253265017160672, -9.564922557960803928, 103.3322429386476955 ) ) ;
#96501=CARTESIAN_POINT ( 'NONE',  ( 14.34966873604960469, 8.224510206698951720, 59.16557627198103120 ) ) ;
#96502=CARTESIAN_POINT ( 'NONE',  ( 0.05219959533909260263, 19.03943276465977164, 34.99890960531435979 ) ) ;
#96503=CARTESIAN_POINT ( 'NONE',  ( 5.049401038298161559, -19.05341960407611168, 27.70724293864769550 ) ) ;
#96504=CARTESIAN_POINT ( 'NONE',  ( 15.80617190586769283, -15.72974639402175789, 105.6260903946856899 ) ) ;
#96505=CARTESIAN_POINT ( 'NONE',  ( 8.224510206698742110, 14.34966873604972548, 87.08442372801901854 ) ) ;
#96506=CARTESIAN_POINT ( 'NONE',  ( -15.72974639402176322, -15.80617190586768395, 44.37609039468567573 ) ) ;
#96507=CARTESIAN_POINT ( 'NONE',  ( 4.483927247898790824, -16.52544592524335698, 40.20942372801901854 ) ) ;
#96508=CARTESIAN_POINT ( 'NONE',  ( -0.05219959533907301413, -21.53943276465977519, 22.49890960531436335 ) ) ;
#96509=CARTESIAN_POINT ( 'NONE',  ( -13.97604488694527625, -13.89961937509977652, 51.87390960531436690 ) ) ;
#96510=CARTESIAN_POINT ( 'NONE',  ( -13.97604488694527625, -13.89961937509977652, 66.87390960531436690 ) ) ;
#96511=CARTESIAN_POINT ( 'NONE',  ( 16.53943276465976808, 0.05219959533934440121, 66.25109039468567573 ) ) ;
#96512=CARTESIAN_POINT ( 'NONE',  ( 0.05219959533910956823, 16.53943276465976808, 99.99890960531436690 ) ) ;
#96513=CARTESIAN_POINT ( 'NONE',  ( 8.314922557960818139, 14.29746914071049879, 24.58224293864768839 ) ) ;
#96515=CARTESIAN_POINT ( 'NONE',  ( 5.823673210054444382, -21.52544592524334988, 60.20942372801902565 ) ) ;
#96516=CARTESIAN_POINT ( 'NONE',  ( -0.05219959533909027116, -19.03943276465977164, 92.49890960531436690 ) ) ;
#96517=CARTESIAN_POINT ( 'NONE',  ( 9.474510206698971260, -16.51473224551069308, 77.91557627198103830 ) ) ;
#96518=CARTESIAN_POINT ( 'NONE',  ( 13.89961937509977652, -13.97604488694527269, 103.1239096053143527 ) ) ;
#96519=CARTESIAN_POINT ( 'NONE',  ( 12.06949235617757843, -12.14591786802309237, 43.12390960531435269 ) ) ;
#96520=CARTESIAN_POINT ( 'NONE',  ( -16.53943276465976808, 0.05219959533911058130, 26.24890960531435624 ) ) ;
#96521=CARTESIAN_POINT ( 'NONE',  ( 4.483927247898545687, 16.52544592524342804, 44.79057627198103120 ) ) ;
#96523=CARTESIAN_POINT ( 'NONE',  ( 9.474510206698729675, 16.51473224551082808, 32.08442372801900433 ) ) ;
#96524=CARTESIAN_POINT ( 'NONE',  ( -5.049401038298153566, 19.05341960407611168, 80.20724293864769550 ) ) ;
#96525=CARTESIAN_POINT ( 'NONE',  ( -5.049401038297874678, -19.05341960407617918, 49.79275706135231871 ) ) ;
#96528=CARTESIAN_POINT ( 'NONE',  ( -0.05219959533936034679, 19.03943276465977164, 87.50109039468567573 ) ) ;
#96529=CARTESIAN_POINT ( 'NONE',  ( -8.224510206698735004, -14.34966873604973081, 69.58442372801900433 ) ) ;
#96531=CARTESIAN_POINT ( 'NONE',  ( -5.153800228976328057, -19.02544592524343514, 107.2905762719810383 ) ) ;
#96532=CARTESIAN_POINT ( 'NONE',  ( -18.67979575497193778, 10.72451020669871902, 33.33442372801900433 ) ) ;
#96533=CARTESIAN_POINT ( 'NONE',  ( 13.89961937509957401, 13.97604488694547697, 96.87609039468566152 ) ) ;
#96534=CARTESIAN_POINT ( 'NONE',  ( 16.46253265017160672, -9.564922557960803928, 113.3322429386476955 ) ) ;
#96535=CARTESIAN_POINT ( 'NONE',  ( 16.51473224551069308, 9.474510206698969483, 54.16557627198103120 ) ) ;
#96536=EDGE_CURVE ( 'NONE', #44580, #199831, #44089, .T. ) ;
#96537=CARTESIAN_POINT ( 'NONE',  ( -5.153800228976328057, -19.02544592524343514, 87.29057627198103830 ) ) ;
#96538=CARTESIAN_POINT ( 'NONE',  ( 12.06949235617757843, -12.14591786802309237, 63.12390960531435979 ) ) ;
#96539=CARTESIAN_POINT ( 'NONE',  ( 5.153800228976335163, 19.02544592524342804, 49.79057627198100988 ) ) ;
#96540=CARTESIAN_POINT ( 'NONE',  ( 16.51473224551069308, 9.474510206698969483, 64.16557627198102409 ) ) ;
#96541=CARTESIAN_POINT ( 'NONE',  ( 19.03943276465977164, 0.05219959533936151252, 66.25109039468567573 ) ) ;
#96542=CARTESIAN_POINT ( 'NONE',  ( 9.564922557961047289, -16.46253265017146816, 35.41775706135233293 ) ) ;
#96543=CARTESIAN_POINT ( 'NONE',  ( -0.05219959533909027116, -19.03943276465977164, 62.49890960531435979 ) ) ;
#96544=( BOUNDED_SURFACE ( )  B_SPLINE_SURFACE ( 3, 2, ( 
 ( #101895, #163577, #103897, #194916, #9899, #121039, #152382, #87716, #150418, #102894, #151405, #72570, #182737, #195931, #181742, #118073, #136225, #29059, #43223, #137209, #134245, #135249, #74558, #119078, #44221, #41233, #105879, #165577, #198896, #164579, #196921, #149402, #26073, #180760, #27076, #11913, #73576, #167566, #104891, #166580, #76532, #126019, #157358, #187714, #108857, #106866, #62339, #107848, #199890, #63351, #49186, #91677, #79514, #110844, #139194, #60364, #32026, #15864, #169533, #93684, #669, #1673, #138208, #18852, #183726, #124009, #14871, #140180, #31033, #92682, #122036, #142171, #125028, #61354, #186724, #185707, #123025, #80498, #45212, #17858, #171534, #168540, #30038, #170536, #172528, #47197, #34014, #95671, #48195, #16856, #153369, #184710, #155367, #46195, #78507, #109849, #33022, #94677, #141184, #154370, #77522, #156356, #2673, #64350, #98641, #66328, #19829, #97631, #7637, #23831, #127989, #54162, #38993, #99650, #175506, #173528, #159320, #96653, #68316, #158340, #53146, #174517, #188700, #36980, #85481, #162330, #3655, #145155, #65333, #126993, #190678, #81470, #111839, #146150, #177524, #35984, #160336, #189692, #176518, #20815, #84472, #82472, #6638, #50182, #22826, #115835, #129967, #100649, #144157, #21825, #161334, #5642, #69321, #51164, #130987, #52154, #34998, #143156, #83477, #67319, #112825, #128980, #113811, #191667, #4637, #192679, #114825, #37995, #163345, #12664, #43982, #74332, #195698, #193687, #149180, #194686, #86490, #148175, #70332, #119831, #182502, #58164, #28828, #165348, #42005, #134007, #104662, #147170, #57170, #181516, #42995, #105643, #39982, #103670, #26842, #88482, #180531, #27845, #151176, #120802, #72332, #118848, #167332, #150178, #8659, #73344, #131999, #55155, #166347, #116825, #117837, #132995, #178516, #11679, #89486, #101653, #24841, #179530, #9667, #71333, #135998, #10668, #135017, #56156, #197669, #41000, #196694, #59134, #102667, #164352, #25848, #87491, #121797, #29803, #184478, #63106, #90469, #44974, #30796, #198663, #31788, #1427, #62105, #152152, #93437, #139937, #186483, #125776, #15625, #156114, #108617, #79271, #16617, #136974, #17612, #123768, #45957, #61115, #122789, #107612, #169290, #168306, #124784, #185468, #92445, #91439, #140942, #60129, #75302, #183490, #138952, #47959, #94433, #155124, #110598, #77282, #46958, #109610, #106633, #154132, #13635, #153127, #170295, #431, #14630, #78265, #171295, #76287, #137967, #199649, #32781, #172280, #2430, #64109, #187477, #48945, #188454, #141927, #176278, #7398, #4400, #5400, #19595, #6398, #189452, #52904, #22587, #112587, #33769, #67084, #50930, #81237, #128743, #174281, #175268, #111600, #192441, #157113, #35750, #49935, #113574, #66085, #142918, #95429, #115598, #98397, #173284, #36734, #159082, #34758, #53923, #18610, #191428, #144915, #80257, #130749, #143919, #161092, #20576, #84235, #145913, #21581, #190439, #3418, #65093, #82229, #158102, #97396, #51915, #68077, #160095, #114580, #127751, #126752, #129731, #83240, #37749, #99410, #96416, #69082, #71089, #181279, #197433, #101404, #27604, #12429, #73102, #148936, #146929, #132756, #70091, #41760, #131760, #26597, #147938, #42756, #23590, #162095, #164110, #58899, #118602, #177286, #38757, #25608, #193442, #85238, #119596, #150936, #9424, #10426, #163098, #149925, #194443, #57925, #55914, #180292, #100414, #196455, #89243, #103425, #74092, #117588, #195453, #134772, #179289, #104419, #39742, #166102, #87252, #135762, #8419, #56927, #40754, #24601, #86248, #102422, #72084, #54918, #116590, #178279, #165104, #133758, #88240, #11432, #186243, #169049, #167091, #122553, #168071, #59891, #123535, #109372, #151913, #93202, #45724, #185229, #15388, #183253, #136732, #14386, #124546, #140704, #44734, #171054, #155877, #16385, #92207, #90229, #76052, #13402, #46720, #75066, #170059, #91200, #47721, #28592, #105406 ),
 ( #77045, #79029, #121557, #43744, #154887, #17374, #31550, #2194, #138716, #197, #107377, #78032, #120565, #30555, #139701, #1187, #182259, #198414, #61866, #108383, #62864, #153891, #32544, #94197, #106390, #29569, #152890, #137728, #199412, #60876, #184243, #99175, #125547, #98158, #48713, #34530, #49699, #95197, #174052, #6169, #187243, #160865, #96190, #18380, #22355, #129504, #65850, #158854, #84007, #67849, #110366, #66848, #20342, #189224, #128511, #21351, #172048, #156883, #3192, #157879, #36504, #63876, #80032, #4172, #33535, #5165, #175039, #35521, #141701, #190206, #113347, #159858, #145685, #50702, #191204, #81991, #52679, #51685, #64865, #114342, #97169, #19368, #81017, #142692, #127520, #112361, #126527, #83009, #143684, #144684, #188226, #111364, #176045, #37513, #173053, #29086, #198922, #86017, #7167, #179052, #162859, #54680, #40520, #147706, #151433, #85001, #168568, #130509, #9194, #161862, #89747, #178043, #116354, #68850, #91707, #74584, #146682, #12920, #132528, #8177, #30066, #192205, #167591, #121070, #53687, #106895, #117356, #137238, #194217, #60391, #122063, #197928, #163879, #115364, #177054, #55682, #131521, #70859, #28108, #182764, #102191, #90725, #39511, #38524, #44248, #136252, #59396, #105905, #69853, #23356, #101171, #13895, #100180, #193207, #183755, #45241, #152408, #75562, #24366, #108888, #46226, #17890, #107879, #2704, #124041, #157390, #199919, #138236, #140211, #35030, #94708, #153401, #14899, #1705, #169567, #61383, #95702, #127025, #185740, #125058, #139225, #126049, #170567, #34045, #32057, #156385, #76560, #172559, #65364, #79544, #50217, #47229, #171563, #49216, #155396, #18883, #15895, #80529, #63381, #188732, #123055, #33053, #93714, #700, #77553, #62372, #16886, #111871, #110874, #142203, #141214, #31064, #3686, #173561, #184741, #186755, #92712, #78537, #48225, #154400, #109879, #64381, #187745, #53182, #55188, #97665, #19862, #69353, #132030, #7669, #178548, #114858, #191699, #83509, #54194, #96685, #145186, #131022, #192711, #193720, #189724, #176552, #38028, #99684, #129999, #177556, #100680, #70363, #21858, #6670, #116857, #161368, #158373, #22859, #81502, #143189, #115867, #4669, #67352, #82508, #128022, #68348, #39025, #66361, #51197, #129012, #112858, #174549, #162362, #98674, #84506, #36016, #23863, #159354, #146184, #85514, #147202, #8693, #20850, #144190, #5676, #190712, #52185, #113843, #175539, #37013, #160368, #148206, #181546, #151206, #11710, #40014, #43024, #89516, #136026, #75334, #165380, #105677, #58193, #28861, #166379, #86522, #167363, #73377, #195731, #10701, #72364, #57204, #134038, #117871, #12694, #135049, #118879, #41031, #90501, #9699, #24873, #71364, #88517, #74360, #44016, #104691, #60160, #26874, #196725, #197700, #133028, #180563, #101687, #194718, #119861, #42037, #163376, #27875, #59166, #164385, #25878, #120834, #182534, #103701, #150213, #152183, #179561, #56188, #13667, #137004, #87522, #102697, #198693, #121829, #149210, #107645, #33801, #18642, #79304, #155157, #153160, #138984, #76321, #47990, #137999, #32814, #154165, #187509, #29835, #168339, #170327, #65125, #124816, #183523, #45006, #31819, #199683, #91472, #125807, #157147, #15657, #16649, #169322, #156146, #462, #64143, #62137, #186516, #106666, #2461, #95461, #109643, #80288, #77316, #1459, #140973, #185499, #48976, #45990, #110631, #93470, #141960, #14661, #63137, #123801, #30829, #92477, #46990, #108649, #3449, #172312, #61148, #171326, #122820, #184510, #78296, #139970, #94465, #17644, #128775, #174312, #66118, #129762, #115629, #158134, #145948, #177318, #5433, #126783, #98430, #82261, #35782, #160127, #67117, #68110, #4430, #85270, #49968, #190474, #81268, #6428, #97429, #159115, #188489, #8449, #191458, #127783, #52936, #51947, #189483, #146961, #111632, #84267, #37780, #173317, #23622, #36767, #53953, #113607, #38789, #100446 ),
 ( #99444, #175301, #114610, #21615, #50961, #20609, #83273, #144947, #176308, #112620, #34792, #96447, #161124, #142949, #22620, #143953, #7429, #19626, #69113, #130779, #192471, #162126, #195484, #9459, #28623, #70122, #27637, #181311, #90260, #167123, #180324, #197465, #56959, #58931, #120599, #57957, #26629, #151943, #131793, #118633, #194476, #10458, #88272, #42789, #41792, #150968, #102455, #101438, #104452, #103459, #134807, #165137, #132789, #86280, #164143, #74123, #193473, #55948, #182294, #105438, #166135, #149960, #39774, #25640, #163129, #196487, #24632, #119628, #40786, #135794, #116622, #54950, #11466, #178311, #73137, #147971, #71123, #89278, #117624, #179322, #12463, #43774, #87284, #148969, #72119, #133792, #169078, #94226, #92236, #154914, #13432, #32573, #125574, #78059, #110395, #107405, #31578, #109402, #15416, #17403, #76079, #155907, #226, #187272, #95226, #93229, #184270, #199439, #137755, #60907, #122583, #172077, #171082, #79060, #16412, #29597, #140733, #33564, #2222, #61894, #59920, #77074, #45753, #152919, #139727, #63904, #44765, #48741, #75096, #153921, #136763, #185259, #30584, #198448, #123564, #46751, #121588, #106418, #138744, #183283, #168099, #170085, #108410, #91228, #1216, #62893, #124574, #186270, #14415, #47749, #112387, #5193, #66875, #96216, #173080, #143714, #37538, #81043, #157905, #18409, #4199, #98184, #113373, #115391, #19394, #80058, #129529, #192233, #67875, #38550, #175064, #51710, #128537, #114366, #156912, #190232, #191229, #52703, #53714, #49727, #36530, #159888, #21376, #83035, #99202, #160890, #130535, #82018, #144710, #177079, #6195, #141728, #176071, #3218, #64892, #22382, #126553, #127551, #142719, #188253, #84032, #145710, #111395, #34557, #189252, #65877, #50729, #7192, #158881, #68876, #174079, #35548, #97195, #20370, #56723, #25404, #164901, #57722, #23382, #131550, #39537, #194243, #72897, #100207, #54708, #40550, #8206, #41556, #11222, #71879, #161887, #103219, #149722, #196253, #135558, #87046, #165894, #118394, #89037, #26395, #146709, #27391, #133549, #55710, #70887, #132555, #117382, #179079, #178070, #134565, #195239, #102219, #101195, #150727, #69881, #85029, #193235, #148731, #119392, #104213, #88034, #116380, #181075, #180088, #10219, #42550, #12226, #162886, #24395, #86044, #163908, #73889, #147733, #9220, #197231, #58692, #120362, #182055, #107171, #43538, #76838, #123328, #169849, #124334, #122345, #77830, #153683, #139497, #195428, #151712, #16175, #168842, #75845, #91000, #152686, #137521, #14175, #59683, #185022, #30347, #199203, #183047, #979, #90029, #13205, #74868, #45516, #108168, #62655, #138509, #109168, #184034, #91989, #31343, #136530, #60670, #105204, #198211, #15179, #61660, #28391, #46508, #92994, #167869, #29369, #154680, #186030, #47512, #166891, #121354, #44531, #106186, #70020, #26527, #71021, #196385, #193370, #194377, #8345, #195379, #178208, #103356, #101334, #164041, #22516, #41691, #134702, #87184, #119526, #116520, #40682, #118532, #24529, #88171, #85164, #165034, #9356, #57854, #104346, #102352, #54846, #131689, #146852, #39672, #163023, #181209, #180221, #149855, #25540, #38687, #11360, #42685, #73030, #132689, #69009, #86180, #147870, #162022, #148865, #84163, #53852, #145843, #7325, #55844, #130675, #117518, #179216, #10356, #72013, #192369, #133686, #115526, #56857, #177214, #100343, #23518, #13330, #199339, #106315, #107301, #43670, #124470, #89171, #44662, #120494, #45650, #136660, #74995, #27530, #47649, #30478, #105332, #168973, #91130, #167020, #186167, #166030, #123462, #76971, #150863, #62789, #75979, #93127, #152820, #154812, #16310, #153817, #122477, #12357, #74020, #14314, #90157, #168001, #184168, #138642, #137652, #46644, #198341, #197362, #123, #60804, #92130, #15312, #28521, #182185, #59816, #169984, #135690, #151840, #77960, #1115, #61792, #185154, #58827, #121486, #183180, #108304 ),
 ( #31475, #29497, #139627, #170979, #156813, #50624, #65776, #67772, #110295, #32472, #81913, #144608, #20267, #191127, #127445, #4097, #96116, #66772, #109300, #157804, #143606, #5090, #6093, #2121, #189151, #112285, #173975, #142618, #190130, #113269, #82930, #34457, #19295, #129429, #35443, #94125, #97095, #155804, #17302, #128433, #78956, #79961, #95123, #140631, #80943, #51605, #63803, #174961, #36425, #125476, #187172, #158779, #98080, #159778, #21273, #48643, #171977, #33465, #18305, #141630, #3120, #64795, #126456, #188154, #49627, #111289, #172979, #37436, #23279, #38445, #83927, #162780, #195135, #114263, #102112, #11116, #145608, #160788, #118290, #54602, #147626, #72791, #56616, #175967, #55604, #9114, #177966, #117278, #10115, #99096, #7087, #192125, #146603, #25299, #52601, #68768, #193129, #22276, #194140, #163797, #24288, #130426, #178972, #86941, #148625, #87931, #39434, #179981, #70781, #41449, #40439, #53606, #103114, #85937, #8096, #84923, #69774, #131442, #116276, #115282, #71775, #132449, #101094, #176975, #164795, #100100, #161784, #133445, #26290, #149618, #134461, #137419, #16075, #182947, #29268, #153579, #88936, #166790, #57618, #165792, #152585, #28291, #119286, #14076, #45417, #120261, #181953, #15077, #76738, #151612, #44430, #106084, #135459, #12123, #150627, #75742, #74769, #91888, #180969, #43435, #199099, #60566, #154579, #197128, #42446, #168741, #31243, #107070, #77733, #122242, #90899, #167770, #138413, #196146, #183932, #104110, #200093, #108064, #30245, #92893, #89931, #61561, #123230, #198112, #184921, #58595, #46405, #169748, #27289, #73787, #105104, #13104, #136431, #59579, #121253, #63567, #97848, #96866, #4857, #19062, #155573, #66542, #36194, #128206, #187923, #185928, #141396, #186939, #78722, #142387, #126228, #189903, #159537, #170748, #18072, #139399, #111055, #94893, #48410, #172743, #79727, #80709, #17068, #21035, #62556, #2884, #93895, #3866, #110066, #171746, #881, #124232, #65545, #140398, #127204, #64563, #1886, #47413, #109069, #158550, #50396, #32237, #125241, #49392, #51378, #34224, #113039, #174731, #188918, #95886, #33235, #156577, #157569, #112056, #173744, #35213, #20040, #81683, #143365, #115044, #114024, #55366, #7854, #147387, #177734, #145370, #98856, #176736, #86699, #102873, #6852, #133204, #118052, #178731, #54373, #52367, #38209, #175721, #8875, #37200, #132211, #53366, #148384, #129193, #67535, #69541, #164558, #24045, #82688, #144372, #9878, #130186, #71538, #131205, #56369, #99865, #116045, #68531, #117036, #161549, #163556, #23042, #85701, #160551, #39203, #100859, #162541, #70543, #25056, #194895, #179742, #192896, #193902, #41212, #40194, #5859, #101874, #190891, #22041, #83692, #191882, #84687, #146367, #57385, #136204, #168522, #87696, #75514, #184691, #119058, #134225, #91658, #28057, #121016, #46175, #30020, #149381, #29040, #182714, #151384, #90680, #183707, #10877, #180740, #165557, #120034, #198875, #26052, #42216, #166558, #195910, #167545, #137188, #197879, #72547, #152362, #60342, #122016, #61334, #12874, #153347, #44199, #14849, #13847, #103877, #76511, #59348, #181720, #196900, #58367, #43202, #104869, #27054, #45193, #105858, #89698, #88700, #138187, #150396, #11892, #73555, #74539, #106847, #199870, #123005, #107828, #135228, #2654, #129701, #62319, #140161, #31012, #139172, #125999, #1653, #92662, #187696, #18833, #93663, #155348, #191398, #52875, #125009, #17838, #79496, #108836, #185687, #123989, #49166, #48176, #65314, #154350, #16837, #110825, #172507, #130717, #170517, #15843, #142152, #7366, #80478, #53892, #33994, #64331, #156338, #114547, #169512, #141165, #3636, #176246, #69051, #77502, #95650, #649, #157338, #47177, #32006, #37717, #78488, #99379, #161062, #145883, #63331, #22557, #186705, #84203, #109832, #192410, #171515, #33004, #94658, #134740, #27571, #180259, #12397, #9394, #133725 ),
 ( #39710, #74059, #73068, #181247, #195417, #131729, #42724, #135730, #104386, #164079, #162062, #117557, #163063, #54886, #118569, #102391, #166069, #197401, #146895, #194414, #115567, #87222, #71060, #24569, #148904, #55884, #56895, #193411, #177254, #38726, #179257, #70061, #41729, #86218, #147908, #100384, #23558, #103393, #116560, #165071, #40722, #178249, #85206, #8386, #196422, #26565, #101373, #132726, #25578, #89210, #10394, #150903, #72051, #88208, #149892, #11399, #57892, #119564, #183220, #199378, #15353, #31514, #30517, #139665, #91169, #90197, #93167, #184207, #123500, #153855, #121525, #75034, #152858, #62828, #78995, #44701, #109338, #94163, #154852, #92169, #28560, #14353, #151880, #185193, #13370, #108343, #29536, #124511, #105372, #162, #120533, #46684, #155842, #182226, #16350, #43711, #76018, #106355, #136700, #169013, #1153, #167059, #170024, #17339, #198381, #59858, #186206, #60842, #77009, #140669, #47688, #168039, #61830, #138681, #45689, #77998, #171020, #137693, #122517, #107340, #32511, #58867, #2161, #156849, #142658, #110332, #143646, #113310, #174014, #63839, #5129, #51646, #98123, #37478, #127485, #67815, #20306, #191169, #128474, #48680, #129470, #35485, #157844, #173018, #34497, #19335, #96155, #79999, #175001, #97134, #80983, #3159, #52642, #172013, #187209, #33502, #50664, #36466, #6132, #66812, #22317, #189190, #158818, #159820, #95161, #4137, #125512, #18344, #81954, #65816, #141667, #190170, #21315, #126494, #188192, #82973, #144649, #112324, #114307, #176009, #64832, #49664, #111328, #99140, #160829, #83968, #7128, #193169, #86980, #102152, #104149, #146644, #68810, #118329, #181012, #56656, #27328, #163837, #40480, #132490, #103154, #145648, #194179, #180022, #41489, #42486, #38485, #25339, #148667, #10155, #179012, #26331, #149659, #119325, #70821, #55643, #165831, #162819, #116316, #23318, #164835, #71815, #39472, #8137, #134501, #192167, #130469, #53647, #117316, #87971, #11157, #133483, #115325, #195175, #72831, #196187, #100142, #178005, #177016, #161823, #57659, #101133, #84962, #69815, #131482, #54641, #24328, #85977, #147667, #9155, #137458, #199137, #28329, #105142, #181992, #168778, #167806, #184957, #150664, #136468, #30280, #45454, #47449, #89968, #12162, #61597, #124269, #200128, #170784, #107108, #183967, #75780, #46441, #88974, #60604, #123266, #108100, #185964, #43474, #91926, #153618, #15114, #122279, #169785, #92929, #62591, #14113, #76775, #109105, #138447, #73827, #31278, #135497, #197167, #154615, #58633, #59618, #74805, #120299, #16110, #77768, #166828, #139435, #151648, #13143, #198148, #917, #90936, #121291, #182984, #44468, #106122, #29306, #152622, #157606, #96902, #189937, #155610, #63603, #171782, #126263, #4893, #32274, #186976, #172781, #140434, #173782, #143404, #3903, #93931, #35249, #81719, #128240, #67570, #19097, #97882, #50433, #21071, #158586, #78757, #159573, #65583, #187960, #2921, #64599, #17105, #80746, #156614, #34262, #188956, #66575, #127242, #113072, #49430, #125279, #51412, #142424, #20075, #112092, #94929, #48446, #111091, #36230, #52402, #18109, #82727, #129228, #174764, #144408, #1924, #95921, #110103, #5894, #33270, #190925, #114061, #79763, #141434, #160585, #162575, #57418, #117069, #175758, #37235, #179776, #23076, #41245, #24078, #149414, #146399, #147421, #161582, #148417, #131240, #56404, #54406, #178765, #98891, #194929, #87729, #40230, #72583, #69574, #193936, #71572, #177766, #102907, #38242, #118086, #85734, #10910, #22074, #55399, #7888, #84721, #99897, #192928, #116078, #134257, #133237, #164591, #101907, #191916, #26085, #195944, #83725, #8908, #145404, #39235, #100891, #115078, #163589, #70576, #6886, #68564, #130221, #132244, #53400, #25090, #86732, #9912, #176770, #59380, #60374, #196932, #77532, #42248, #197910, #73588, #198906, #89730, #166591, #180773, #679, #183736, #58400, #122046 ),
 ( #165590, #184721, #90709, #44232, #46205, #137219, #107859, #45222, #27088, #169544, #152392, #74568, #151416, #12904, #136236, #121052, #120066, #30048, #13878, #182747, #181754, #31043, #88734, #103909, #150429, #167576, #153379, #123035, #106877, #139204, #105889, #75545, #76542, #11924, #29070, #135260, #43236, #168550, #91689, #104902, #14881, #138218, #92692, #28091, #199900, #61364, #119091, #154380, #15874, #62350, #66340, #109859, #128002, #110854, #35996, #33032, #34024, #48205, #35010, #17869, #143169, #141194, #3666, #124020, #81482, #174529, #127004, #159332, #156366, #80509, #158352, #64360, #189704, #125038, #4649, #49196, #97643, #144169, #142182, #94688, #171544, #186734, #79524, #2683, #20829, #19841, #51177, #65344, #78517, #112837, #82485, #185717, #172539, #108867, #126029, #187725, #1683, #188712, #95682, #47208, #170546, #93694, #157369, #32037, #18863, #50195, #111851, #173541, #96665, #155377, #140191, #16866, #63361, #84486, #160348, #85494, #176532, #53160, #67331, #87502, #70344, #83490, #147182, #130999, #145167, #164363, #5655, #163357, #116838, #25858, #102678, #86502, #38008, #36993, #178528, #192691, #132011, #100661, #68329, #21837, #99663, #9680, #128993, #129979, #56168, #41011, #101667, #190691, #52166, #115847, #54174, #193698, #98654, #55167, #161348, #71345, #113823, #175518, #177536, #6651, #8671, #191679, #114838, #133008, #22839, #194699, #39006, #179542, #146163, #162343, #7649, #39995, #69333, #148186, #23844, #24853, #117849, #168318, #61127, #13646, #45969, #43005, #167343, #44986, #151186, #153139, #11690, #29815, #136007, #122800, #30807, #28840, #119841, #135029, #73356, #196704, #58174, #107623, #106646, #14641, #90481, #165360, #76301, #169301, #137979, #197679, #195710, #12674, #181526, #88495, #152163, #59144, #199661, #149190, #180542, #27856, #10679, #120814, #104672, #166358, #182514, #89496, #75313, #26854, #72344, #134018, #74341, #103681, #136984, #43993, #105655, #57182, #118859, #198673, #150192, #60140, #121807, #183503, #42016, #91451, #184490, #3428, #50940, #189462, #2440, #19605, #79283, #81247, #142929, #80267, #48955, #112598, #154144, #140953, #16629, #32792, #110608, #65104, #64122, #170306, #174290, #15636, #171306, #46969, #172291, #63117, #139949, #77293, #92456, #157124, #31799, #33780, #17624, #93448, #138964, #442, #49947, #126762, #62117, #123780, #125787, #4410, #187489, #66095, #127762, #141937, #95440, #185479, #108628, #18620, #78276, #94445, #188465, #111611, #173296, #34770, #124796, #155135, #96427, #158113, #1439, #186494, #47970, #109622, #156125, #39752, #55925, #160104, #86258, #71099, #131769, #194454, #20587, #145924, #84244, #100423, #128753, #85247, #6406, #101414, #82239, #143929, #22597, #117599, #177295, #35760, #97406, #163107, #83250, #24610, #7407, #9434, #68087, #69090, #21591, #8428, #191437, #116600, #114589, #38766, #159093, #54927, #147948, #162104, #132766, #129740, #53931, #193451, #37758, #5411, #98408, #178288, #130757, #67094, #190450, #115606, #52913, #144925, #176286, #99419, #161102, #51925, #113585, #175279, #23601, #36744, #192449, #146938, #70100, #27616, #25618, #181290, #26608, #118613, #182271, #166113, #170819, #78792, #10437, #57936, #179300, #150947, #134784, #88251, #12441, #119607, #120578, #72097, #154652, #104430, #46478, #74103, #41771, #195464, #73115, #186002, #1959, #103436, #32311, #17140, #77802, #140470, #164120, #89255, #135773, #108138, #133769, #31313, #149937, #47483, #87262, #148947, #197444, #63638, #169822, #40764, #102433, #109140, #11443, #93965, #58910, #155645, #196466, #92966, #165116, #16147, #42768, #62626, #139471, #951, #56939, #124304, #180303, #189968, #22106, #19128, #143437, #21104, #127274, #129261, #187991, #5925, #112122, #37266, #6918, #4924, #95954, #111123, #49461, #172813, #34293, #83756, #82759, #190956, #66606, #141469, #52433 ),
 ( #188988, #20106, #145435, #114091, #187010, #128270, #81750, #50463, #51443, #144439, #48480, #156647, #64632, #80778, #97914, #125314, #79796, #65614, #33303, #113103, #36260, #96934, #110136, #174794, #159605, #67602, #160616, #173814, #175792, #98924, #171815, #94962, #18143, #2953, #158616, #142456, #157639, #3934, #35279, #126294, #146431, #179806, #101940, #162608, #116109, #9944, #25122, #27117, #69606, #191947, #41275, #103938, #102937, #150457, #86766, #163621, #55431, #26116, #68596, #117102, #164622, #87759, #165618, #161613, #148449, #71603, #133269, #194960, #149444, #72613, #42280, #193968, #178797, #88764, #56437, #130252, #118118, #53433, #115109, #10940, #134288, #176801, #38274, #99928, #40266, #195975, #23107, #57447, #84753, #7921, #131272, #119120, #70610, #180801, #192960, #54439, #177797, #39267, #100923, #24112, #85767, #147453, #8941, #132277, #151445, #105917, #184753, #11952, #166618, #152420, #120094, #153413, #123067, #183767, #73616, #14912, #61395, #107892, #47242, #137250, #77565, #30078, #712, #138248, #58427, #139237, #45253, #167603, #182777, #44260, #29098, #90737, #89759, #46238, #106907, #13908, #12932, #62384, #181782, #196959, #43263, #60403, #169579, #15907, #76573, #32070, #198936, #168580, #31077, #104931, #75574, #74596, #136264, #135287, #92724, #28120, #91719, #154413, #197939, #59408, #124054, #185753, #122075, #199932, #108900, #121082, #170579, #93726, #35042, #34057, #51209, #16898, #3698, #65377, #94720, #171576, #48237, #96696, #95715, #112870, #78549, #2716, #158385, #111883, #113855, #156398, #140224, #128034, #190724, #66374, #37026, #173573, #50229, #142215, #174561, #155408, #127037, #189736, #36028, #52197, #109892, #19874, #81514, #143201, #188744, #97677, #159366, #129023, #80541, #4682, #175551, #20863, #1717, #82520, #63393, #125070, #144202, #5688, #186767, #33065, #17902, #67364, #79557, #141225, #64393, #126061, #187758, #49228, #110886, #157402, #172571, #18895, #9711, #98687, #193731, #147213, #39035, #55199, #24884, #21871, #130011, #176564, #7680, #40024, #160381, #38039, #177567, #191710, #116868, #163387, #8704, #83521, #178559, #86533, #71375, #164396, #162372, #117881, #101697, #179572, #148217, #53194, #56199, #70374, #115877, #131033, #192722, #100691, #54206, #99695, #133039, #132042, #23874, #22870, #41042, #114869, #161379, #84517, #85525, #194729, #102707, #145199, #6682, #68360, #146195, #69364, #172212, #49863, #157044, #18541, #140869, #113504, #2358, #97328, #128673, #3351, #65026, #98323, #160023, #34690, #21510, #111529, #110531, #51845, #4331, #143851, #174212, #141860, #95359, #173214, #83171, #99339, #126682, #129660, #114503, #175199, #37674, #64039, #189383, #127683, #5330, #33696, #190370, #96347, #144845, #125709, #187408, #66015, #161022, #20507, #79200, #48876, #6328, #188386, #68008, #50860, #52834, #158034, #112518, #19525, #36664, #81170, #191356, #142852, #82155, #80188, #176205, #35680, #67014, #159014, #57315, #27989, #89628, #152295, #75446, #76439, #134154, #136137, #197813, #59278, #74472, #121945, #45120, #14779, #166491, #151316, #138116, #182647, #102810, #167476, #199797, #164495, #120948, #105790, #122934, #25988, #72481, #12805, #183638, #87631, #90613, #61264, #195842, #149317, #106778, #43133, #44131, #41147, #168453, #10811, #28971, #13779, #137121, #198807, #60272, #118991, #180674, #42150, #135160, #29950, #103810, #165490, #181654, #26986, #91588, #153278, #88631, #150327, #11822, #73487, #196833, #58301, #119968, #104802, #2577, #173435, #110749, #30945, #50087, #156261, #140086, #155273, #16762, #1578, #78410, #62247, #95576, #17764, #143064, #185615, #107758, #157262, #19738, #18757, #66236, #64257, #96560, #170442, #576, #171441, #32928, #80404, #142076, #81379, #77431, #79420, #141090, #125924, #187622, #65240, #188606, #158248, #109757, #94583, #4542, #49092, #46103 ) ),
 .UNSPECIFIED., .T., .F., .F. ) 
 B_SPLINE_SURFACE_WITH_KNOTS ( ( 4, 3, 4 ),
 ( 3, 2, 2, 2, 2, 2, 2, 2, 2, 2, 2, 2, 2, 2, 2, 2, 2, 2, 2, 2, 2, 2, 2, 2, 2, 2, 2, 2, 2, 2, 2, 2, 2, 2, 2, 2, 2, 2, 2, 2, 2, 2, 2, 2, 2, 2, 2, 2, 2, 2, 2, 2, 2, 2, 2, 2, 2, 2, 2, 2, 2, 2, 2, 2, 2, 2, 2, 2, 2, 2, 2, 2, 2, 2, 2, 2, 2, 2, 2, 2, 2, 2, 2, 2, 2, 2, 2, 2, 2, 2, 2, 2, 2, 2, 2, 2, 2, 2, 2, 2, 2, 2, 2, 2, 2, 2, 2, 2, 2, 2, 2, 2, 2, 2, 2, 2, 2, 2, 2, 2, 2, 2, 2, 2, 2, 2, 2, 2, 2, 2, 2, 2, 2, 2, 2, 2, 2, 2, 2, 2, 2, 2, 2, 2, 2, 2, 2, 2, 2, 2, 2, 2, 2, 2, 2, 2, 2, 2, 2, 2, 2, 2, 2, 2, 2, 2, 2, 2, 2, 2, 2, 2, 2, 2, 2, 2, 2, 2, 2, 2, 2, 2, 2, 2, 2, 2, 2, 2, 2, 2, 2, 2, 2, 2, 2, 2, 2, 2, 2, 2, 2, 2, 2, 2, 2, 2, 2, 2, 2, 2, 2, 2, 2, 2, 2, 2, 2, 2, 2, 2, 2, 2, 2, 2, 2, 2, 2, 2, 3 ),
 ( 0.000000000000000000, 0.5000000000000000000, 1.000000000000000000 ),
 ( 0.000000000000000000, 0.004385964912280701511, 0.008771929824561403022, 0.01315789473684210453, 0.01754385964912280604, 0.02192982456140350755, 0.02631578947368420907, 0.03070175438596491058, 0.03508771929824561209, 0.03947368421052631360, 0.04385964912280701511, 0.04824561403508771662, 0.05263157894736841813, 0.05701754385964911964, 0.06140350877192982115, 0.06578947368421052266, 0.07017543859649122417, 0.07456140350877192569, 0.07894736842105262720, 0.08333333333333332871, 0.08771929824561403022, 0.09210526315789473173, 0.09649122807017543324, 0.1008771929824561348, 0.1052631578947368363, 0.1096491228070175378, 0.1140350877192982393, 0.1184210526315789408, 0.1228070175438596423, 0.1271929824561403577, 0.1315789473684210453, 0.1359649122807017607, 0.1403508771929824483, 0.1447368421052631637, 0.1491228070175438514, 0.1535087719298245668, 0.1578947368421052544, 0.1622807017543859698, 0.1666666666666666574, 0.1710526315789473728, 0.1754385964912280604, 0.1798245614035087758, 0.1842105263157894635, 0.1885964912280701788, 0.1929824561403508665, 0.1973684210526315819, 0.2017543859649122695, 0.2061403508771929849, 0.2105263157894736725, 0.2149122807017543879, 0.2192982456140350755, 0.2236842105263157909, 0.2280701754385964786, 0.2324561403508771940, 0.2368421052631578816, 0.2412280701754385970, 0.2456140350877192846, 0.2500000000000000000, 0.2543859649122807154, 0.2587719298245614308, 0.2631578947368420907, 0.2675438596491228060, 0.2719298245614035214, 0.2763157894736842368, 0.2807017543859648967, 0.2850877192982456121, 0.2894736842105263275, 0.2938596491228070429, 0.2982456140350877027, 0.3026315789473684181, 0.3070175438596491335, 0.3114035087719298489, 0.3157894736842105088, 0.3201754385964912242, 0.3245614035087719396, 0.3289473684210526550, 0.3333333333333333148, 0.3377192982456140302, 0.3421052631578947456, 0.3464912280701754610, 0.3508771929824561209, 0.3552631578947368363, 0.3596491228070175517, 0.3640350877192982670, 0.3684210526315789269, 0.3728070175438596423, 0.3771929824561403577, 0.3815789473684210731, 0.3859649122807017330, 0.3903508771929824483, 0.3947368421052631637, 0.3991228070175438791, 0.4035087719298245390, 0.4078947368421052544, 0.4122807017543859698, 0.4166666666666666852, 0.4210526315789473450, 0.4254385964912280604, 0.4298245614035087758, 0.4342105263157894912, 0.4385964912280701511, 0.4429824561403508665, 0.4473684210526315819, 0.4517543859649122973, 0.4561403508771929571, 0.4605263157894736725, 0.4649122807017543879, 0.4692982456140351033, 0.4736842105263157632, 0.4780701754385964786, 0.4824561403508771940, 0.4868421052631579093, 0.4912280701754385692, 0.4956140350877192846, 0.5000000000000000000, 0.5043859649122807154, 0.5087719298245614308, 0.5131578947368421462, 0.5175438596491228616, 0.5219298245614034659, 0.5263157894736841813, 0.5307017543859648967, 0.5350877192982456121, 0.5394736842105263275, 0.5438596491228070429, 0.5482456140350877583, 0.5526315789473684736, 0.5570175438596490780, 0.5614035087719297934, 0.5657894736842105088, 0.5701754385964912242, 0.5745614035087719396, 0.5789473684210526550, 0.5833333333333333703, 0.5877192982456140857, 0.5921052631578946901, 0.5964912280701754055, 0.6008771929824561209, 0.6052631578947368363, 0.6096491228070175517, 0.6140350877192982670, 0.6184210526315789824, 0.6228070175438596978, 0.6271929824561403022, 0.6315789473684210176, 0.6359649122807017330, 0.6403508771929824483, 0.6447368421052631637, 0.6491228070175438791, 0.6535087719298245945, 0.6578947368421053099, 0.6622807017543859143, 0.6666666666666666297, 0.6710526315789473450, 0.6754385964912280604, 0.6798245614035087758, 0.6842105263157894912, 0.6885964912280702066, 0.6929824561403509220, 0.6973684210526315264, 0.7017543859649122417, 0.7061403508771929571, 0.7105263157894736725, 0.7149122807017543879, 0.7192982456140351033, 0.7236842105263158187, 0.7280701754385965341, 0.7324561403508771384, 0.7368421052631578538, 0.7412280701754385692, 0.7456140350877192846, 0.7500000000000000000, 0.7543859649122807154, 0.7587719298245614308, 0.7631578947368421462, 0.7675438596491228616, 0.7719298245614034659, 0.7763157894736841813, 0.7807017543859648967, 0.7850877192982456121, 0.7894736842105263275, 0.7938596491228070429, 0.7982456140350877583, 0.8026315789473684736, 0.8070175438596490780, 0.8114035087719297934, 0.8157894736842105088, 0.8201754385964912242, 0.8245614035087719396, 0.8289473684210526550, 0.8333333333333333703, 0.8377192982456140857, 0.8421052631578946901, 0.8464912280701754055, 0.8508771929824561209, 0.8552631578947368363, 0.8596491228070175517, 0.8640350877192982670, 0.8684210526315789824, 0.8728070175438596978, 0.8771929824561403022, 0.8815789473684210176, 0.8859649122807017330, 0.8903508771929824483, 0.8947368421052631637, 0.8991228070175438791, 0.9035087719298245945, 0.9078947368421053099, 0.9122807017543859143, 0.9166666666666666297, 0.9210526315789473450, 0.9254385964912280604, 0.9298245614035087758, 0.9342105263157894912, 0.9385964912280702066, 0.9429824561403509220, 0.9473684210526315264, 0.9517543859649122417, 0.9561403508771929571, 0.9605263157894736725, 0.9649122807017543879, 0.9692982456140351033, 0.9736842105263158187, 0.9780701754385965341, 0.9824561403508771384, 0.9868421052631578538, 0.9912280701754385692, 0.9956140350877192846, 1.000000000000000000 ),
 .UNSPECIFIED. ) 
 GEOMETRIC_REPRESENTATION_ITEM ( )  RATIONAL_B_SPLINE_SURFACE ( (
 ( 1.000000000000000000, 0.9659258262890683122, 1.000000000000000000, 0.9659258262890683122, 1.000000000000000000, 0.9659258262890683122, 1.000000000000000000, 0.9659258262890683122, 1.000000000000000000, 0.9659258262890683122, 1.000000000000000000, 0.9659258262890683122, 1.000000000000000000, 0.9659258262890683122, 1.000000000000000000, 0.9659258262890683122, 1.000000000000000000, 0.9659258262890683122, 1.000000000000000000, 0.9659258262890683122, 1.000000000000000000, 0.9659258262890683122, 1.000000000000000000, 0.9659258262890683122, 1.000000000000000000, 0.9659258262890683122, 1.000000000000000000, 0.9659258262890683122, 1.000000000000000000, 0.9659258262890683122, 1.000000000000000000, 0.9659258262890683122, 1.000000000000000000, 0.9659258262890683122, 1.000000000000000000, 0.9659258262890683122, 1.000000000000000000, 0.9659258262890683122, 1.000000000000000000, 0.9659258262890683122, 1.000000000000000000, 0.9659258262890683122, 1.000000000000000000, 0.9659258262890683122, 1.000000000000000000, 0.9659258262890683122, 1.000000000000000000, 0.9659258262890683122, 1.000000000000000000, 0.9659258262890683122, 1.000000000000000000, 0.9659258262890683122, 1.000000000000000000, 0.9659258262890683122, 1.000000000000000000, 0.9659258262890683122, 1.000000000000000000, 0.9659258262890683122, 1.000000000000000000, 0.9659258262890683122, 1.000000000000000000, 0.9659258262890683122, 1.000000000000000000, 0.9659258262890683122, 1.000000000000000000, 0.9659258262890683122, 1.000000000000000000, 0.9659258262890683122, 1.000000000000000000, 0.9659258262890683122, 1.000000000000000000, 0.9659258262890683122, 1.000000000000000000, 0.9659258262890683122, 1.000000000000000000, 0.9659258262890683122, 1.000000000000000000, 0.9659258262890683122, 1.000000000000000000, 0.9659258262890683122, 1.000000000000000000, 0.9659258262890683122, 1.000000000000000000, 0.9659258262890683122, 1.000000000000000000, 0.9659258262890683122, 1.000000000000000000, 0.9659258262890683122, 1.000000000000000000, 0.9659258262890683122, 1.000000000000000000, 0.9659258262890683122, 1.000000000000000000, 0.9659258262890683122, 1.000000000000000000, 0.9659258262890683122, 1.000000000000000000, 0.9659258262890683122, 1.000000000000000000, 0.9659258262890683122, 1.000000000000000000, 0.9659258262890683122, 1.000000000000000000, 0.9659258262890683122, 1.000000000000000000, 0.9659258262890683122, 1.000000000000000000, 0.9659258262890683122, 1.000000000000000000, 0.9659258262890683122, 1.000000000000000000, 0.9659258262890683122, 1.000000000000000000, 0.9659258262890683122, 1.000000000000000000, 0.9659258262890683122, 1.000000000000000000, 0.9659258262890683122, 1.000000000000000000, 0.9659258262890683122, 1.000000000000000000, 0.9659258262890683122, 1.000000000000000000, 0.9659258262890683122, 1.000000000000000000, 0.9659258262890683122, 1.000000000000000000, 0.9659258262890683122, 1.000000000000000000, 0.9659258262890683122, 1.000000000000000000, 0.9659258262890683122, 1.000000000000000000, 0.9659258262890683122, 1.000000000000000000, 0.9659258262890683122, 1.000000000000000000, 0.9659258262890683122, 1.000000000000000000, 0.9659258262890683122, 1.000000000000000000, 0.9659258262890683122, 1.000000000000000000, 0.9659258262890683122, 1.000000000000000000, 0.9659258262890683122, 1.000000000000000000, 0.9659258262890683122, 1.000000000000000000, 0.9659258262890683122, 1.000000000000000000, 0.9659258262890683122, 1.000000000000000000, 0.9659258262890683122, 1.000000000000000000, 0.9659258262890683122, 1.000000000000000000, 0.9659258262890683122, 1.000000000000000000, 0.9659258262890683122, 1.000000000000000000, 0.9659258262890683122, 1.000000000000000000, 0.9659258262890683122, 1.000000000000000000, 0.9659258262890683122, 1.000000000000000000, 0.9659258262890683122, 1.000000000000000000, 0.9659258262890683122, 1.000000000000000000, 0.9659258262890683122, 1.000000000000000000, 0.9659258262890683122, 1.000000000000000000, 0.9659258262890683122, 1.000000000000000000, 0.9659258262890683122, 1.000000000000000000, 0.9659258262890683122, 1.000000000000000000, 0.9659258262890683122, 1.000000000000000000, 0.9659258262890683122, 1.000000000000000000, 0.9659258262890683122, 1.000000000000000000, 0.9659258262890683122, 1.000000000000000000, 0.9659258262890683122, 1.000000000000000000, 0.9659258262890683122, 1.000000000000000000, 0.9659258262890683122, 1.000000000000000000, 0.9659258262890683122, 1.000000000000000000, 0.9659258262890683122, 1.000000000000000000, 0.9659258262890683122, 1.000000000000000000, 0.9659258262890683122, 1.000000000000000000, 0.9659258262890683122, 1.000000000000000000, 0.9659258262890683122, 1.000000000000000000, 0.9659258262890683122, 1.000000000000000000, 0.9659258262890683122, 1.000000000000000000, 0.9659258262890683122, 1.000000000000000000, 0.9659258262890683122, 1.000000000000000000, 0.9659258262890683122, 1.000000000000000000, 0.9659258262890683122, 1.000000000000000000, 0.9659258262890683122, 1.000000000000000000, 0.9659258262890683122, 1.000000000000000000, 0.9659258262890683122, 1.000000000000000000, 0.9659258262890683122, 1.000000000000000000, 0.9659258262890683122, 1.000000000000000000, 0.9659258262890683122, 1.000000000000000000, 0.9659258262890683122, 1.000000000000000000, 0.9659258262890683122, 1.000000000000000000, 0.9659258262890683122, 1.000000000000000000, 0.9659258262890683122, 1.000000000000000000, 0.9659258262890683122, 1.000000000000000000, 0.9659258262890683122, 1.000000000000000000, 0.9659258262890683122, 1.000000000000000000, 0.9659258262890683122, 1.000000000000000000, 0.9659258262890683122, 1.000000000000000000, 0.9659258262890683122, 1.000000000000000000, 0.9659258262890683122, 1.000000000000000000, 0.9659258262890683122, 1.000000000000000000, 0.9659258262890683122, 1.000000000000000000, 0.9659258262890683122, 1.000000000000000000, 0.9659258262890683122, 1.000000000000000000, 0.9659258262890683122, 1.000000000000000000, 0.9659258262890683122, 1.000000000000000000, 0.9659258262890683122, 1.000000000000000000, 0.9659258262890683122, 1.000000000000000000, 0.9659258262890683122, 1.000000000000000000, 0.9659258262890683122, 1.000000000000000000, 0.9659258262890683122, 1.000000000000000000, 0.9659258262890683122, 1.000000000000000000, 0.9659258262890683122, 1.000000000000000000, 0.9659258262890683122, 1.000000000000000000, 0.9659258262890683122, 1.000000000000000000, 0.9659258262890683122, 1.000000000000000000, 0.9659258262890683122, 1.000000000000000000, 0.9659258262890683122, 1.000000000000000000, 0.9659258262890683122, 1.000000000000000000, 0.9659258262890683122, 1.000000000000000000, 0.9659258262890683122, 1.000000000000000000, 0.9659258262890683122, 1.000000000000000000, 0.9659258262890683122, 1.000000000000000000, 0.9659258262890683122, 1.000000000000000000, 0.9659258262890683122, 1.000000000000000000, 0.9659258262890683122, 1.000000000000000000, 0.9659258262890683122, 1.000000000000000000, 0.9659258262890683122, 1.000000000000000000, 0.9659258262890683122, 1.000000000000000000, 0.9659258262890683122, 1.000000000000000000, 0.9659258262890683122, 1.000000000000000000, 0.9659258262890683122, 1.000000000000000000, 0.9659258262890683122, 1.000000000000000000, 0.9659258262890683122, 1.000000000000000000, 0.9659258262890683122, 1.000000000000000000, 0.9659258262890683122, 1.000000000000000000, 0.9659258262890683122, 1.000000000000000000, 0.9659258262890683122, 1.000000000000000000, 0.9659258262890683122, 1.000000000000000000, 0.9659258262890683122, 1.000000000000000000, 0.9659258262890683122, 1.000000000000000000, 0.9659258262890683122, 1.000000000000000000, 0.9659258262890683122, 1.000000000000000000, 0.9659258262890683122, 1.000000000000000000, 0.9659258262890683122, 1.000000000000000000, 0.9659258262890683122, 1.000000000000000000, 0.9659258262890683122, 1.000000000000000000, 0.9659258262890683122, 1.000000000000000000, 0.9659258262890683122, 1.000000000000000000, 0.9659258262890683122, 1.000000000000000000, 0.9659258262890683122, 1.000000000000000000, 0.9659258262890683122, 1.000000000000000000, 0.9659258262890683122, 1.000000000000000000, 0.9659258262890683122, 1.000000000000000000, 0.9659258262890683122, 1.000000000000000000, 0.9659258262890683122, 1.000000000000000000, 0.9659258262890683122, 1.000000000000000000, 0.9659258262890683122, 1.000000000000000000, 0.9659258262890683122, 1.000000000000000000, 0.9659258262890683122, 1.000000000000000000, 0.9659258262890683122, 1.000000000000000000, 0.9659258262890683122, 1.000000000000000000, 0.9659258262890683122, 1.000000000000000000, 0.9659258262890683122, 1.000000000000000000, 0.9659258262890683122, 1.000000000000000000, 0.9659258262890683122, 1.000000000000000000, 0.9659258262890683122, 1.000000000000000000, 0.9659258262890683122, 1.000000000000000000, 0.9659258262890683122, 1.000000000000000000, 0.9659258262890683122, 1.000000000000000000, 0.9659258262890683122, 1.000000000000000000, 0.9659258262890683122, 1.000000000000000000, 0.9659258262890683122, 1.000000000000000000, 0.9659258262890683122, 1.000000000000000000, 0.9659258262890683122, 1.000000000000000000, 0.9659258262890683122, 1.000000000000000000, 0.9659258262890683122, 1.000000000000000000, 0.9659258262890683122, 1.000000000000000000, 0.9659258262890683122, 1.000000000000000000, 0.9659258262890683122, 1.000000000000000000, 0.9659258262890683122, 1.000000000000000000, 0.9659258262890683122, 1.000000000000000000, 0.9659258262890683122, 1.000000000000000000, 0.9659258262890683122, 1.000000000000000000, 0.9659258262890683122, 1.000000000000000000, 0.9659258262890683122, 1.000000000000000000, 0.9659258262890683122, 1.000000000000000000, 0.9659258262890683122, 1.000000000000000000, 0.9659258262890683122, 1.000000000000000000, 0.9659258262890683122, 1.000000000000000000, 0.9659258262890683122, 1.000000000000000000, 0.9659258262890683122, 1.000000000000000000, 0.9659258262890683122, 1.000000000000000000, 0.9659258262890683122, 1.000000000000000000, 0.9659258262890683122, 1.000000000000000000, 0.9659258262890683122, 1.000000000000000000, 0.9659258262890683122, 1.000000000000000000, 0.9659258262890683122, 1.000000000000000000, 0.9659258262890683122, 1.000000000000000000, 0.9659258262890683122, 1.000000000000000000, 0.9659258262890683122, 1.000000000000000000, 0.9659258262890683122, 1.000000000000000000),
 ( 0.3333333333333333703, 0.3219752754296894559, 0.3333333333333333703, 0.3219752754296894559, 0.3333333333333333703, 0.3219752754296894559, 0.3333333333333333703, 0.3219752754296894559, 0.3333333333333333703, 0.3219752754296894559, 0.3333333333333333703, 0.3219752754296894559, 0.3333333333333333703, 0.3219752754296894559, 0.3333333333333333703, 0.3219752754296894559, 0.3333333333333333703, 0.3219752754296894559, 0.3333333333333333703, 0.3219752754296894559, 0.3333333333333333703, 0.3219752754296894559, 0.3333333333333333703, 0.3219752754296894559, 0.3333333333333333703, 0.3219752754296894559, 0.3333333333333333703, 0.3219752754296894559, 0.3333333333333333703, 0.3219752754296894559, 0.3333333333333333703, 0.3219752754296894559, 0.3333333333333333703, 0.3219752754296894559, 0.3333333333333333703, 0.3219752754296894559, 0.3333333333333333703, 0.3219752754296894559, 0.3333333333333333703, 0.3219752754296894559, 0.3333333333333333703, 0.3219752754296894559, 0.3333333333333333703, 0.3219752754296894559, 0.3333333333333333703, 0.3219752754296894559, 0.3333333333333333703, 0.3219752754296894559, 0.3333333333333333703, 0.3219752754296894559, 0.3333333333333333703, 0.3219752754296894559, 0.3333333333333333703, 0.3219752754296894559, 0.3333333333333333703, 0.3219752754296894559, 0.3333333333333333703, 0.3219752754296894559, 0.3333333333333333703, 0.3219752754296894559, 0.3333333333333333703, 0.3219752754296894559, 0.3333333333333333703, 0.3219752754296894559, 0.3333333333333333703, 0.3219752754296894559, 0.3333333333333333703, 0.3219752754296894559, 0.3333333333333333703, 0.3219752754296894559, 0.3333333333333333703, 0.3219752754296894559, 0.3333333333333333703, 0.3219752754296894559, 0.3333333333333333703, 0.3219752754296894559, 0.3333333333333333703, 0.3219752754296894559, 0.3333333333333333703, 0.3219752754296894559, 0.3333333333333333703, 0.3219752754296894559, 0.3333333333333333703, 0.3219752754296894559, 0.3333333333333333703, 0.3219752754296894559, 0.3333333333333333703, 0.3219752754296894559, 0.3333333333333333703, 0.3219752754296894559, 0.3333333333333333703, 0.3219752754296894559, 0.3333333333333333703, 0.3219752754296894559, 0.3333333333333333703, 0.3219752754296894559, 0.3333333333333333703, 0.3219752754296894559, 0.3333333333333333703, 0.3219752754296894559, 0.3333333333333333703, 0.3219752754296894559, 0.3333333333333333703, 0.3219752754296894559, 0.3333333333333333703, 0.3219752754296894559, 0.3333333333333333703, 0.3219752754296894559, 0.3333333333333333703, 0.3219752754296894559, 0.3333333333333333703, 0.3219752754296894559, 0.3333333333333333703, 0.3219752754296894559, 0.3333333333333333703, 0.3219752754296894559, 0.3333333333333333703, 0.3219752754296894559, 0.3333333333333333703, 0.3219752754296894559, 0.3333333333333333703, 0.3219752754296894559, 0.3333333333333333703, 0.3219752754296894559, 0.3333333333333333703, 0.3219752754296894559, 0.3333333333333333703, 0.3219752754296894559, 0.3333333333333333703, 0.3219752754296894559, 0.3333333333333333703, 0.3219752754296894559, 0.3333333333333333703, 0.3219752754296894559, 0.3333333333333333703, 0.3219752754296894559, 0.3333333333333333703, 0.3219752754296894559, 0.3333333333333333703, 0.3219752754296894559, 0.3333333333333333703, 0.3219752754296894559, 0.3333333333333333703, 0.3219752754296894559, 0.3333333333333333703, 0.3219752754296894559, 0.3333333333333333703, 0.3219752754296894559, 0.3333333333333333703, 0.3219752754296894559, 0.3333333333333333703, 0.3219752754296894559, 0.3333333333333333703, 0.3219752754296894559, 0.3333333333333333703, 0.3219752754296894559, 0.3333333333333333703, 0.3219752754296894559, 0.3333333333333333703, 0.3219752754296894559, 0.3333333333333333703, 0.3219752754296894559, 0.3333333333333333703, 0.3219752754296894559, 0.3333333333333333703, 0.3219752754296894559, 0.3333333333333333703, 0.3219752754296894559, 0.3333333333333333703, 0.3219752754296894559, 0.3333333333333333703, 0.3219752754296894559, 0.3333333333333333703, 0.3219752754296894559, 0.3333333333333333703, 0.3219752754296894559, 0.3333333333333333703, 0.3219752754296894559, 0.3333333333333333703, 0.3219752754296894559, 0.3333333333333333703, 0.3219752754296894559, 0.3333333333333333703, 0.3219752754296894559, 0.3333333333333333703, 0.3219752754296894559, 0.3333333333333333703, 0.3219752754296894559, 0.3333333333333333703, 0.3219752754296894559, 0.3333333333333333703, 0.3219752754296894559, 0.3333333333333333703, 0.3219752754296894559, 0.3333333333333333703, 0.3219752754296894559, 0.3333333333333333703, 0.3219752754296894559, 0.3333333333333333703, 0.3219752754296894559, 0.3333333333333333703, 0.3219752754296894559, 0.3333333333333333703, 0.3219752754296894559, 0.3333333333333333703, 0.3219752754296894559, 0.3333333333333333703, 0.3219752754296894559, 0.3333333333333333703, 0.3219752754296894559, 0.3333333333333333703, 0.3219752754296894559, 0.3333333333333333703, 0.3219752754296894559, 0.3333333333333333703, 0.3219752754296894559, 0.3333333333333333703, 0.3219752754296894559, 0.3333333333333333703, 0.3219752754296894559, 0.3333333333333333703, 0.3219752754296894559, 0.3333333333333333703, 0.3219752754296894559, 0.3333333333333333703, 0.3219752754296894559, 0.3333333333333333703, 0.3219752754296894559, 0.3333333333333333703, 0.3219752754296894559, 0.3333333333333333703, 0.3219752754296894559, 0.3333333333333333703, 0.3219752754296894559, 0.3333333333333333703, 0.3219752754296894559, 0.3333333333333333703, 0.3219752754296894559, 0.3333333333333333703, 0.3219752754296894559, 0.3333333333333333703, 0.3219752754296894559, 0.3333333333333333703, 0.3219752754296894559, 0.3333333333333333703, 0.3219752754296894559, 0.3333333333333333703, 0.3219752754296894559, 0.3333333333333333703, 0.3219752754296894559, 0.3333333333333333703, 0.3219752754296894559, 0.3333333333333333703, 0.3219752754296894559, 0.3333333333333333703, 0.3219752754296894559, 0.3333333333333333703, 0.3219752754296894559, 0.3333333333333333703, 0.3219752754296894559, 0.3333333333333333703, 0.3219752754296894559, 0.3333333333333333703, 0.3219752754296894559, 0.3333333333333333703, 0.3219752754296894559, 0.3333333333333333703, 0.3219752754296894559, 0.3333333333333333703, 0.3219752754296894559, 0.3333333333333333703, 0.3219752754296894559, 0.3333333333333333703, 0.3219752754296894559, 0.3333333333333333703, 0.3219752754296894559, 0.3333333333333333703, 0.3219752754296894559, 0.3333333333333333703, 0.3219752754296894559, 0.3333333333333333703, 0.3219752754296894559, 0.3333333333333333703, 0.3219752754296894559, 0.3333333333333333703, 0.3219752754296894559, 0.3333333333333333703, 0.3219752754296894559, 0.3333333333333333703, 0.3219752754296894559, 0.3333333333333333703, 0.3219752754296894559, 0.3333333333333333703, 0.3219752754296894559, 0.3333333333333333703, 0.3219752754296894559, 0.3333333333333333703, 0.3219752754296894559, 0.3333333333333333703, 0.3219752754296894559, 0.3333333333333333703, 0.3219752754296894559, 0.3333333333333333703, 0.3219752754296894559, 0.3333333333333333703, 0.3219752754296894559, 0.3333333333333333703, 0.3219752754296894559, 0.3333333333333333703, 0.3219752754296894559, 0.3333333333333333703, 0.3219752754296894559, 0.3333333333333333703, 0.3219752754296894559, 0.3333333333333333703, 0.3219752754296894559, 0.3333333333333333703, 0.3219752754296894559, 0.3333333333333333703, 0.3219752754296894559, 0.3333333333333333703, 0.3219752754296894559, 0.3333333333333333703, 0.3219752754296894559, 0.3333333333333333703, 0.3219752754296894559, 0.3333333333333333703, 0.3219752754296894559, 0.3333333333333333703, 0.3219752754296894559, 0.3333333333333333703, 0.3219752754296894559, 0.3333333333333333703, 0.3219752754296894559, 0.3333333333333333703, 0.3219752754296894559, 0.3333333333333333703, 0.3219752754296894559, 0.3333333333333333703, 0.3219752754296894559, 0.3333333333333333703, 0.3219752754296894559, 0.3333333333333333703, 0.3219752754296894559, 0.3333333333333333703, 0.3219752754296894559, 0.3333333333333333703, 0.3219752754296894559, 0.3333333333333333703, 0.3219752754296894559, 0.3333333333333333703, 0.3219752754296894559, 0.3333333333333333703, 0.3219752754296894559, 0.3333333333333333703, 0.3219752754296894559, 0.3333333333333333703, 0.3219752754296894559, 0.3333333333333333703, 0.3219752754296894559, 0.3333333333333333703, 0.3219752754296894559, 0.3333333333333333703, 0.3219752754296894559, 0.3333333333333333703, 0.3219752754296894559, 0.3333333333333333703, 0.3219752754296894559, 0.3333333333333333703, 0.3219752754296894559, 0.3333333333333333703, 0.3219752754296894559, 0.3333333333333333703, 0.3219752754296894559, 0.3333333333333333703, 0.3219752754296894559, 0.3333333333333333703, 0.3219752754296894559, 0.3333333333333333703, 0.3219752754296894559, 0.3333333333333333703, 0.3219752754296894559, 0.3333333333333333703, 0.3219752754296894559, 0.3333333333333333703, 0.3219752754296894559, 0.3333333333333333703, 0.3219752754296894559, 0.3333333333333333703, 0.3219752754296894559, 0.3333333333333333703, 0.3219752754296894559, 0.3333333333333333703, 0.3219752754296894559, 0.3333333333333333703, 0.3219752754296894559, 0.3333333333333333703, 0.3219752754296894559, 0.3333333333333333703, 0.3219752754296894559, 0.3333333333333333703, 0.3219752754296894559, 0.3333333333333333703, 0.3219752754296894559, 0.3333333333333333703, 0.3219752754296894559, 0.3333333333333333703, 0.3219752754296894559, 0.3333333333333333703, 0.3219752754296894559, 0.3333333333333333703, 0.3219752754296894559, 0.3333333333333333703, 0.3219752754296894559, 0.3333333333333333703, 0.3219752754296894559, 0.3333333333333333703, 0.3219752754296894559, 0.3333333333333333703, 0.3219752754296894559, 0.3333333333333333703, 0.3219752754296894559, 0.3333333333333333703, 0.3219752754296894559, 0.3333333333333333703, 0.3219752754296894559, 0.3333333333333333703, 0.3219752754296894559, 0.3333333333333333703, 0.3219752754296894559, 0.3333333333333333703, 0.3219752754296894559, 0.3333333333333333703, 0.3219752754296894559, 0.3333333333333333703, 0.3219752754296894559, 0.3333333333333333703, 0.3219752754296894559, 0.3333333333333333703, 0.3219752754296894559, 0.3333333333333333703, 0.3219752754296894559, 0.3333333333333333703, 0.3219752754296894559, 0.3333333333333333703, 0.3219752754296894559, 0.3333333333333333703, 0.3219752754296894559, 0.3333333333333333703, 0.3219752754296894559, 0.3333333333333333703, 0.3219752754296894559, 0.3333333333333333703, 0.3219752754296894559, 0.3333333333333333703, 0.3219752754296894559, 0.3333333333333333703),
 ( 0.3333333333333333703, 0.3219752754296894559, 0.3333333333333333703, 0.3219752754296894559, 0.3333333333333333703, 0.3219752754296894559, 0.3333333333333333703, 0.3219752754296894559, 0.3333333333333333703, 0.3219752754296894559, 0.3333333333333333703, 0.3219752754296894559, 0.3333333333333333703, 0.3219752754296894559, 0.3333333333333333703, 0.3219752754296894559, 0.3333333333333333703, 0.3219752754296894559, 0.3333333333333333703, 0.3219752754296894559, 0.3333333333333333703, 0.3219752754296894559, 0.3333333333333333703, 0.3219752754296894559, 0.3333333333333333703, 0.3219752754296894559, 0.3333333333333333703, 0.3219752754296894559, 0.3333333333333333703, 0.3219752754296894559, 0.3333333333333333703, 0.3219752754296894559, 0.3333333333333333703, 0.3219752754296894559, 0.3333333333333333703, 0.3219752754296894559, 0.3333333333333333703, 0.3219752754296894559, 0.3333333333333333703, 0.3219752754296894559, 0.3333333333333333703, 0.3219752754296894559, 0.3333333333333333703, 0.3219752754296894559, 0.3333333333333333703, 0.3219752754296894559, 0.3333333333333333703, 0.3219752754296894559, 0.3333333333333333703, 0.3219752754296894559, 0.3333333333333333703, 0.3219752754296894559, 0.3333333333333333703, 0.3219752754296894559, 0.3333333333333333703, 0.3219752754296894559, 0.3333333333333333703, 0.3219752754296894559, 0.3333333333333333703, 0.3219752754296894559, 0.3333333333333333703, 0.3219752754296894559, 0.3333333333333333703, 0.3219752754296894559, 0.3333333333333333703, 0.3219752754296894559, 0.3333333333333333703, 0.3219752754296894559, 0.3333333333333333703, 0.3219752754296894559, 0.3333333333333333703, 0.3219752754296894559, 0.3333333333333333703, 0.3219752754296894559, 0.3333333333333333703, 0.3219752754296894559, 0.3333333333333333703, 0.3219752754296894559, 0.3333333333333333703, 0.3219752754296894559, 0.3333333333333333703, 0.3219752754296894559, 0.3333333333333333703, 0.3219752754296894559, 0.3333333333333333703, 0.3219752754296894559, 0.3333333333333333703, 0.3219752754296894559, 0.3333333333333333703, 0.3219752754296894559, 0.3333333333333333703, 0.3219752754296894559, 0.3333333333333333703, 0.3219752754296894559, 0.3333333333333333703, 0.3219752754296894559, 0.3333333333333333703, 0.3219752754296894559, 0.3333333333333333703, 0.3219752754296894559, 0.3333333333333333703, 0.3219752754296894559, 0.3333333333333333703, 0.3219752754296894559, 0.3333333333333333703, 0.3219752754296894559, 0.3333333333333333703, 0.3219752754296894559, 0.3333333333333333703, 0.3219752754296894559, 0.3333333333333333703, 0.3219752754296894559, 0.3333333333333333703, 0.3219752754296894559, 0.3333333333333333703, 0.3219752754296894559, 0.3333333333333333703, 0.3219752754296894559, 0.3333333333333333703, 0.3219752754296894559, 0.3333333333333333703, 0.3219752754296894559, 0.3333333333333333703, 0.3219752754296894559, 0.3333333333333333703, 0.3219752754296894559, 0.3333333333333333703, 0.3219752754296894559, 0.3333333333333333703, 0.3219752754296894559, 0.3333333333333333703, 0.3219752754296894559, 0.3333333333333333703, 0.3219752754296894559, 0.3333333333333333703, 0.3219752754296894559, 0.3333333333333333703, 0.3219752754296894559, 0.3333333333333333703, 0.3219752754296894559, 0.3333333333333333703, 0.3219752754296894559, 0.3333333333333333703, 0.3219752754296894559, 0.3333333333333333703, 0.3219752754296894559, 0.3333333333333333703, 0.3219752754296894559, 0.3333333333333333703, 0.3219752754296894559, 0.3333333333333333703, 0.3219752754296894559, 0.3333333333333333703, 0.3219752754296894559, 0.3333333333333333703, 0.3219752754296894559, 0.3333333333333333703, 0.3219752754296894559, 0.3333333333333333703, 0.3219752754296894559, 0.3333333333333333703, 0.3219752754296894559, 0.3333333333333333703, 0.3219752754296894559, 0.3333333333333333703, 0.3219752754296894559, 0.3333333333333333703, 0.3219752754296894559, 0.3333333333333333703, 0.3219752754296894559, 0.3333333333333333703, 0.3219752754296894559, 0.3333333333333333703, 0.3219752754296894559, 0.3333333333333333703, 0.3219752754296894559, 0.3333333333333333703, 0.3219752754296894559, 0.3333333333333333703, 0.3219752754296894559, 0.3333333333333333703, 0.3219752754296894559, 0.3333333333333333703, 0.3219752754296894559, 0.3333333333333333703, 0.3219752754296894559, 0.3333333333333333703, 0.3219752754296894559, 0.3333333333333333703, 0.3219752754296894559, 0.3333333333333333703, 0.3219752754296894559, 0.3333333333333333703, 0.3219752754296894559, 0.3333333333333333703, 0.3219752754296894559, 0.3333333333333333703, 0.3219752754296894559, 0.3333333333333333703, 0.3219752754296894559, 0.3333333333333333703, 0.3219752754296894559, 0.3333333333333333703, 0.3219752754296894559, 0.3333333333333333703, 0.3219752754296894559, 0.3333333333333333703, 0.3219752754296894559, 0.3333333333333333703, 0.3219752754296894559, 0.3333333333333333703, 0.3219752754296894559, 0.3333333333333333703, 0.3219752754296894559, 0.3333333333333333703, 0.3219752754296894559, 0.3333333333333333703, 0.3219752754296894559, 0.3333333333333333703, 0.3219752754296894559, 0.3333333333333333703, 0.3219752754296894559, 0.3333333333333333703, 0.3219752754296894559, 0.3333333333333333703, 0.3219752754296894559, 0.3333333333333333703, 0.3219752754296894559, 0.3333333333333333703, 0.3219752754296894559, 0.3333333333333333703, 0.3219752754296894559, 0.3333333333333333703, 0.3219752754296894559, 0.3333333333333333703, 0.3219752754296894559, 0.3333333333333333703, 0.3219752754296894559, 0.3333333333333333703, 0.3219752754296894559, 0.3333333333333333703, 0.3219752754296894559, 0.3333333333333333703, 0.3219752754296894559, 0.3333333333333333703, 0.3219752754296894559, 0.3333333333333333703, 0.3219752754296894559, 0.3333333333333333703, 0.3219752754296894559, 0.3333333333333333703, 0.3219752754296894559, 0.3333333333333333703, 0.3219752754296894559, 0.3333333333333333703, 0.3219752754296894559, 0.3333333333333333703, 0.3219752754296894559, 0.3333333333333333703, 0.3219752754296894559, 0.3333333333333333703, 0.3219752754296894559, 0.3333333333333333703, 0.3219752754296894559, 0.3333333333333333703, 0.3219752754296894559, 0.3333333333333333703, 0.3219752754296894559, 0.3333333333333333703, 0.3219752754296894559, 0.3333333333333333703, 0.3219752754296894559, 0.3333333333333333703, 0.3219752754296894559, 0.3333333333333333703, 0.3219752754296894559, 0.3333333333333333703, 0.3219752754296894559, 0.3333333333333333703, 0.3219752754296894559, 0.3333333333333333703, 0.3219752754296894559, 0.3333333333333333703, 0.3219752754296894559, 0.3333333333333333703, 0.3219752754296894559, 0.3333333333333333703, 0.3219752754296894559, 0.3333333333333333703, 0.3219752754296894559, 0.3333333333333333703, 0.3219752754296894559, 0.3333333333333333703, 0.3219752754296894559, 0.3333333333333333703, 0.3219752754296894559, 0.3333333333333333703, 0.3219752754296894559, 0.3333333333333333703, 0.3219752754296894559, 0.3333333333333333703, 0.3219752754296894559, 0.3333333333333333703, 0.3219752754296894559, 0.3333333333333333703, 0.3219752754296894559, 0.3333333333333333703, 0.3219752754296894559, 0.3333333333333333703, 0.3219752754296894559, 0.3333333333333333703, 0.3219752754296894559, 0.3333333333333333703, 0.3219752754296894559, 0.3333333333333333703, 0.3219752754296894559, 0.3333333333333333703, 0.3219752754296894559, 0.3333333333333333703, 0.3219752754296894559, 0.3333333333333333703, 0.3219752754296894559, 0.3333333333333333703, 0.3219752754296894559, 0.3333333333333333703, 0.3219752754296894559, 0.3333333333333333703, 0.3219752754296894559, 0.3333333333333333703, 0.3219752754296894559, 0.3333333333333333703, 0.3219752754296894559, 0.3333333333333333703, 0.3219752754296894559, 0.3333333333333333703, 0.3219752754296894559, 0.3333333333333333703, 0.3219752754296894559, 0.3333333333333333703, 0.3219752754296894559, 0.3333333333333333703, 0.3219752754296894559, 0.3333333333333333703, 0.3219752754296894559, 0.3333333333333333703, 0.3219752754296894559, 0.3333333333333333703, 0.3219752754296894559, 0.3333333333333333703, 0.3219752754296894559, 0.3333333333333333703, 0.3219752754296894559, 0.3333333333333333703, 0.3219752754296894559, 0.3333333333333333703, 0.3219752754296894559, 0.3333333333333333703, 0.3219752754296894559, 0.3333333333333333703, 0.3219752754296894559, 0.3333333333333333703, 0.3219752754296894559, 0.3333333333333333703, 0.3219752754296894559, 0.3333333333333333703, 0.3219752754296894559, 0.3333333333333333703, 0.3219752754296894559, 0.3333333333333333703, 0.3219752754296894559, 0.3333333333333333703, 0.3219752754296894559, 0.3333333333333333703, 0.3219752754296894559, 0.3333333333333333703, 0.3219752754296894559, 0.3333333333333333703, 0.3219752754296894559, 0.3333333333333333703, 0.3219752754296894559, 0.3333333333333333703, 0.3219752754296894559, 0.3333333333333333703, 0.3219752754296894559, 0.3333333333333333703, 0.3219752754296894559, 0.3333333333333333703, 0.3219752754296894559, 0.3333333333333333703, 0.3219752754296894559, 0.3333333333333333703, 0.3219752754296894559, 0.3333333333333333703, 0.3219752754296894559, 0.3333333333333333703, 0.3219752754296894559, 0.3333333333333333703, 0.3219752754296894559, 0.3333333333333333703, 0.3219752754296894559, 0.3333333333333333703, 0.3219752754296894559, 0.3333333333333333703, 0.3219752754296894559, 0.3333333333333333703, 0.3219752754296894559, 0.3333333333333333703, 0.3219752754296894559, 0.3333333333333333703, 0.3219752754296894559, 0.3333333333333333703, 0.3219752754296894559, 0.3333333333333333703, 0.3219752754296894559, 0.3333333333333333703, 0.3219752754296894559, 0.3333333333333333703, 0.3219752754296894559, 0.3333333333333333703, 0.3219752754296894559, 0.3333333333333333703, 0.3219752754296894559, 0.3333333333333333703, 0.3219752754296894559, 0.3333333333333333703, 0.3219752754296894559, 0.3333333333333333703, 0.3219752754296894559, 0.3333333333333333703, 0.3219752754296894559, 0.3333333333333333703, 0.3219752754296894559, 0.3333333333333333703, 0.3219752754296894559, 0.3333333333333333703, 0.3219752754296894559, 0.3333333333333333703, 0.3219752754296894559, 0.3333333333333333703, 0.3219752754296894559, 0.3333333333333333703, 0.3219752754296894559, 0.3333333333333333703, 0.3219752754296894559, 0.3333333333333333703, 0.3219752754296894559, 0.3333333333333333703, 0.3219752754296894559, 0.3333333333333333703, 0.3219752754296894559, 0.3333333333333333703, 0.3219752754296894559, 0.3333333333333333703, 0.3219752754296894559, 0.3333333333333333703, 0.3219752754296894559, 0.3333333333333333703),
 ( 1.000000000000000000, 0.9659258262890683122, 1.000000000000000000, 0.9659258262890683122, 1.000000000000000000, 0.9659258262890683122, 1.000000000000000000, 0.9659258262890683122, 1.000000000000000000, 0.9659258262890683122, 1.000000000000000000, 0.9659258262890683122, 1.000000000000000000, 0.9659258262890683122, 1.000000000000000000, 0.9659258262890683122, 1.000000000000000000, 0.9659258262890683122, 1.000000000000000000, 0.9659258262890683122, 1.000000000000000000, 0.9659258262890683122, 1.000000000000000000, 0.9659258262890683122, 1.000000000000000000, 0.9659258262890683122, 1.000000000000000000, 0.9659258262890683122, 1.000000000000000000, 0.9659258262890683122, 1.000000000000000000, 0.9659258262890683122, 1.000000000000000000, 0.9659258262890683122, 1.000000000000000000, 0.9659258262890683122, 1.000000000000000000, 0.9659258262890683122, 1.000000000000000000, 0.9659258262890683122, 1.000000000000000000, 0.9659258262890683122, 1.000000000000000000, 0.9659258262890683122, 1.000000000000000000, 0.9659258262890683122, 1.000000000000000000, 0.9659258262890683122, 1.000000000000000000, 0.9659258262890683122, 1.000000000000000000, 0.9659258262890683122, 1.000000000000000000, 0.9659258262890683122, 1.000000000000000000, 0.9659258262890683122, 1.000000000000000000, 0.9659258262890683122, 1.000000000000000000, 0.9659258262890683122, 1.000000000000000000, 0.9659258262890683122, 1.000000000000000000, 0.9659258262890683122, 1.000000000000000000, 0.9659258262890683122, 1.000000000000000000, 0.9659258262890683122, 1.000000000000000000, 0.9659258262890683122, 1.000000000000000000, 0.9659258262890683122, 1.000000000000000000, 0.9659258262890683122, 1.000000000000000000, 0.9659258262890683122, 1.000000000000000000, 0.9659258262890683122, 1.000000000000000000, 0.9659258262890683122, 1.000000000000000000, 0.9659258262890683122, 1.000000000000000000, 0.9659258262890683122, 1.000000000000000000, 0.9659258262890683122, 1.000000000000000000, 0.9659258262890683122, 1.000000000000000000, 0.9659258262890683122, 1.000000000000000000, 0.9659258262890683122, 1.000000000000000000, 0.9659258262890683122, 1.000000000000000000, 0.9659258262890683122, 1.000000000000000000, 0.9659258262890683122, 1.000000000000000000, 0.9659258262890683122, 1.000000000000000000, 0.9659258262890683122, 1.000000000000000000, 0.9659258262890683122, 1.000000000000000000, 0.9659258262890683122, 1.000000000000000000, 0.9659258262890683122, 1.000000000000000000, 0.9659258262890683122, 1.000000000000000000, 0.9659258262890683122, 1.000000000000000000, 0.9659258262890683122, 1.000000000000000000, 0.9659258262890683122, 1.000000000000000000, 0.9659258262890683122, 1.000000000000000000, 0.9659258262890683122, 1.000000000000000000, 0.9659258262890683122, 1.000000000000000000, 0.9659258262890683122, 1.000000000000000000, 0.9659258262890683122, 1.000000000000000000, 0.9659258262890683122, 1.000000000000000000, 0.9659258262890683122, 1.000000000000000000, 0.9659258262890683122, 1.000000000000000000, 0.9659258262890683122, 1.000000000000000000, 0.9659258262890683122, 1.000000000000000000, 0.9659258262890683122, 1.000000000000000000, 0.9659258262890683122, 1.000000000000000000, 0.9659258262890683122, 1.000000000000000000, 0.9659258262890683122, 1.000000000000000000, 0.9659258262890683122, 1.000000000000000000, 0.9659258262890683122, 1.000000000000000000, 0.9659258262890683122, 1.000000000000000000, 0.9659258262890683122, 1.000000000000000000, 0.9659258262890683122, 1.000000000000000000, 0.9659258262890683122, 1.000000000000000000, 0.9659258262890683122, 1.000000000000000000, 0.9659258262890683122, 1.000000000000000000, 0.9659258262890683122, 1.000000000000000000, 0.9659258262890683122, 1.000000000000000000, 0.9659258262890683122, 1.000000000000000000, 0.9659258262890683122, 1.000000000000000000, 0.9659258262890683122, 1.000000000000000000, 0.9659258262890683122, 1.000000000000000000, 0.9659258262890683122, 1.000000000000000000, 0.9659258262890683122, 1.000000000000000000, 0.9659258262890683122, 1.000000000000000000, 0.9659258262890683122, 1.000000000000000000, 0.9659258262890683122, 1.000000000000000000, 0.9659258262890683122, 1.000000000000000000, 0.9659258262890683122, 1.000000000000000000, 0.9659258262890683122, 1.000000000000000000, 0.9659258262890683122, 1.000000000000000000, 0.9659258262890683122, 1.000000000000000000, 0.9659258262890683122, 1.000000000000000000, 0.9659258262890683122, 1.000000000000000000, 0.9659258262890683122, 1.000000000000000000, 0.9659258262890683122, 1.000000000000000000, 0.9659258262890683122, 1.000000000000000000, 0.9659258262890683122, 1.000000000000000000, 0.9659258262890683122, 1.000000000000000000, 0.9659258262890683122, 1.000000000000000000, 0.9659258262890683122, 1.000000000000000000, 0.9659258262890683122, 1.000000000000000000, 0.9659258262890683122, 1.000000000000000000, 0.9659258262890683122, 1.000000000000000000, 0.9659258262890683122, 1.000000000000000000, 0.9659258262890683122, 1.000000000000000000, 0.9659258262890683122, 1.000000000000000000, 0.9659258262890683122, 1.000000000000000000, 0.9659258262890683122, 1.000000000000000000, 0.9659258262890683122, 1.000000000000000000, 0.9659258262890683122, 1.000000000000000000, 0.9659258262890683122, 1.000000000000000000, 0.9659258262890683122, 1.000000000000000000, 0.9659258262890683122, 1.000000000000000000, 0.9659258262890683122, 1.000000000000000000, 0.9659258262890683122, 1.000000000000000000, 0.9659258262890683122, 1.000000000000000000, 0.9659258262890683122, 1.000000000000000000, 0.9659258262890683122, 1.000000000000000000, 0.9659258262890683122, 1.000000000000000000, 0.9659258262890683122, 1.000000000000000000, 0.9659258262890683122, 1.000000000000000000, 0.9659258262890683122, 1.000000000000000000, 0.9659258262890683122, 1.000000000000000000, 0.9659258262890683122, 1.000000000000000000, 0.9659258262890683122, 1.000000000000000000, 0.9659258262890683122, 1.000000000000000000, 0.9659258262890683122, 1.000000000000000000, 0.9659258262890683122, 1.000000000000000000, 0.9659258262890683122, 1.000000000000000000, 0.9659258262890683122, 1.000000000000000000, 0.9659258262890683122, 1.000000000000000000, 0.9659258262890683122, 1.000000000000000000, 0.9659258262890683122, 1.000000000000000000, 0.9659258262890683122, 1.000000000000000000, 0.9659258262890683122, 1.000000000000000000, 0.9659258262890683122, 1.000000000000000000, 0.9659258262890683122, 1.000000000000000000, 0.9659258262890683122, 1.000000000000000000, 0.9659258262890683122, 1.000000000000000000, 0.9659258262890683122, 1.000000000000000000, 0.9659258262890683122, 1.000000000000000000, 0.9659258262890683122, 1.000000000000000000, 0.9659258262890683122, 1.000000000000000000, 0.9659258262890683122, 1.000000000000000000, 0.9659258262890683122, 1.000000000000000000, 0.9659258262890683122, 1.000000000000000000, 0.9659258262890683122, 1.000000000000000000, 0.9659258262890683122, 1.000000000000000000, 0.9659258262890683122, 1.000000000000000000, 0.9659258262890683122, 1.000000000000000000, 0.9659258262890683122, 1.000000000000000000, 0.9659258262890683122, 1.000000000000000000, 0.9659258262890683122, 1.000000000000000000, 0.9659258262890683122, 1.000000000000000000, 0.9659258262890683122, 1.000000000000000000, 0.9659258262890683122, 1.000000000000000000, 0.9659258262890683122, 1.000000000000000000, 0.9659258262890683122, 1.000000000000000000, 0.9659258262890683122, 1.000000000000000000, 0.9659258262890683122, 1.000000000000000000, 0.9659258262890683122, 1.000000000000000000, 0.9659258262890683122, 1.000000000000000000, 0.9659258262890683122, 1.000000000000000000, 0.9659258262890683122, 1.000000000000000000, 0.9659258262890683122, 1.000000000000000000, 0.9659258262890683122, 1.000000000000000000, 0.9659258262890683122, 1.000000000000000000, 0.9659258262890683122, 1.000000000000000000, 0.9659258262890683122, 1.000000000000000000, 0.9659258262890683122, 1.000000000000000000, 0.9659258262890683122, 1.000000000000000000, 0.9659258262890683122, 1.000000000000000000, 0.9659258262890683122, 1.000000000000000000, 0.9659258262890683122, 1.000000000000000000, 0.9659258262890683122, 1.000000000000000000, 0.9659258262890683122, 1.000000000000000000, 0.9659258262890683122, 1.000000000000000000, 0.9659258262890683122, 1.000000000000000000, 0.9659258262890683122, 1.000000000000000000, 0.9659258262890683122, 1.000000000000000000, 0.9659258262890683122, 1.000000000000000000, 0.9659258262890683122, 1.000000000000000000, 0.9659258262890683122, 1.000000000000000000, 0.9659258262890683122, 1.000000000000000000, 0.9659258262890683122, 1.000000000000000000, 0.9659258262890683122, 1.000000000000000000, 0.9659258262890683122, 1.000000000000000000, 0.9659258262890683122, 1.000000000000000000, 0.9659258262890683122, 1.000000000000000000, 0.9659258262890683122, 1.000000000000000000, 0.9659258262890683122, 1.000000000000000000, 0.9659258262890683122, 1.000000000000000000, 0.9659258262890683122, 1.000000000000000000, 0.9659258262890683122, 1.000000000000000000, 0.9659258262890683122, 1.000000000000000000, 0.9659258262890683122, 1.000000000000000000, 0.9659258262890683122, 1.000000000000000000, 0.9659258262890683122, 1.000000000000000000, 0.9659258262890683122, 1.000000000000000000, 0.9659258262890683122, 1.000000000000000000, 0.9659258262890683122, 1.000000000000000000, 0.9659258262890683122, 1.000000000000000000, 0.9659258262890683122, 1.000000000000000000, 0.9659258262890683122, 1.000000000000000000, 0.9659258262890683122, 1.000000000000000000, 0.9659258262890683122, 1.000000000000000000, 0.9659258262890683122, 1.000000000000000000, 0.9659258262890683122, 1.000000000000000000, 0.9659258262890683122, 1.000000000000000000, 0.9659258262890683122, 1.000000000000000000, 0.9659258262890683122, 1.000000000000000000, 0.9659258262890683122, 1.000000000000000000, 0.9659258262890683122, 1.000000000000000000, 0.9659258262890683122, 1.000000000000000000, 0.9659258262890683122, 1.000000000000000000, 0.9659258262890683122, 1.000000000000000000, 0.9659258262890683122, 1.000000000000000000, 0.9659258262890683122, 1.000000000000000000, 0.9659258262890683122, 1.000000000000000000, 0.9659258262890683122, 1.000000000000000000, 0.9659258262890683122, 1.000000000000000000, 0.9659258262890683122, 1.000000000000000000, 0.9659258262890683122, 1.000000000000000000),
 ( 0.3333333333333333703, 0.3219752754296894559, 0.3333333333333333703, 0.3219752754296894559, 0.3333333333333333703, 0.3219752754296894559, 0.3333333333333333703, 0.3219752754296894559, 0.3333333333333333703, 0.3219752754296894559, 0.3333333333333333703, 0.3219752754296894559, 0.3333333333333333703, 0.3219752754296894559, 0.3333333333333333703, 0.3219752754296894559, 0.3333333333333333703, 0.3219752754296894559, 0.3333333333333333703, 0.3219752754296894559, 0.3333333333333333703, 0.3219752754296894559, 0.3333333333333333703, 0.3219752754296894559, 0.3333333333333333703, 0.3219752754296894559, 0.3333333333333333703, 0.3219752754296894559, 0.3333333333333333703, 0.3219752754296894559, 0.3333333333333333703, 0.3219752754296894559, 0.3333333333333333703, 0.3219752754296894559, 0.3333333333333333703, 0.3219752754296894559, 0.3333333333333333703, 0.3219752754296894559, 0.3333333333333333703, 0.3219752754296894559, 0.3333333333333333703, 0.3219752754296894559, 0.3333333333333333703, 0.3219752754296894559, 0.3333333333333333703, 0.3219752754296894559, 0.3333333333333333703, 0.3219752754296894559, 0.3333333333333333703, 0.3219752754296894559, 0.3333333333333333703, 0.3219752754296894559, 0.3333333333333333703, 0.3219752754296894559, 0.3333333333333333703, 0.3219752754296894559, 0.3333333333333333703, 0.3219752754296894559, 0.3333333333333333703, 0.3219752754296894559, 0.3333333333333333703, 0.3219752754296894559, 0.3333333333333333703, 0.3219752754296894559, 0.3333333333333333703, 0.3219752754296894559, 0.3333333333333333703, 0.3219752754296894559, 0.3333333333333333703, 0.3219752754296894559, 0.3333333333333333703, 0.3219752754296894559, 0.3333333333333333703, 0.3219752754296894559, 0.3333333333333333703, 0.3219752754296894559, 0.3333333333333333703, 0.3219752754296894559, 0.3333333333333333703, 0.3219752754296894559, 0.3333333333333333703, 0.3219752754296894559, 0.3333333333333333703, 0.3219752754296894559, 0.3333333333333333703, 0.3219752754296894559, 0.3333333333333333703, 0.3219752754296894559, 0.3333333333333333703, 0.3219752754296894559, 0.3333333333333333703, 0.3219752754296894559, 0.3333333333333333703, 0.3219752754296894559, 0.3333333333333333703, 0.3219752754296894559, 0.3333333333333333703, 0.3219752754296894559, 0.3333333333333333703, 0.3219752754296894559, 0.3333333333333333703, 0.3219752754296894559, 0.3333333333333333703, 0.3219752754296894559, 0.3333333333333333703, 0.3219752754296894559, 0.3333333333333333703, 0.3219752754296894559, 0.3333333333333333703, 0.3219752754296894559, 0.3333333333333333703, 0.3219752754296894559, 0.3333333333333333703, 0.3219752754296894559, 0.3333333333333333703, 0.3219752754296894559, 0.3333333333333333703, 0.3219752754296894559, 0.3333333333333333703, 0.3219752754296894559, 0.3333333333333333703, 0.3219752754296894559, 0.3333333333333333703, 0.3219752754296894559, 0.3333333333333333703, 0.3219752754296894559, 0.3333333333333333703, 0.3219752754296894559, 0.3333333333333333703, 0.3219752754296894559, 0.3333333333333333703, 0.3219752754296894559, 0.3333333333333333703, 0.3219752754296894559, 0.3333333333333333703, 0.3219752754296894559, 0.3333333333333333703, 0.3219752754296894559, 0.3333333333333333703, 0.3219752754296894559, 0.3333333333333333703, 0.3219752754296894559, 0.3333333333333333703, 0.3219752754296894559, 0.3333333333333333703, 0.3219752754296894559, 0.3333333333333333703, 0.3219752754296894559, 0.3333333333333333703, 0.3219752754296894559, 0.3333333333333333703, 0.3219752754296894559, 0.3333333333333333703, 0.3219752754296894559, 0.3333333333333333703, 0.3219752754296894559, 0.3333333333333333703, 0.3219752754296894559, 0.3333333333333333703, 0.3219752754296894559, 0.3333333333333333703, 0.3219752754296894559, 0.3333333333333333703, 0.3219752754296894559, 0.3333333333333333703, 0.3219752754296894559, 0.3333333333333333703, 0.3219752754296894559, 0.3333333333333333703, 0.3219752754296894559, 0.3333333333333333703, 0.3219752754296894559, 0.3333333333333333703, 0.3219752754296894559, 0.3333333333333333703, 0.3219752754296894559, 0.3333333333333333703, 0.3219752754296894559, 0.3333333333333333703, 0.3219752754296894559, 0.3333333333333333703, 0.3219752754296894559, 0.3333333333333333703, 0.3219752754296894559, 0.3333333333333333703, 0.3219752754296894559, 0.3333333333333333703, 0.3219752754296894559, 0.3333333333333333703, 0.3219752754296894559, 0.3333333333333333703, 0.3219752754296894559, 0.3333333333333333703, 0.3219752754296894559, 0.3333333333333333703, 0.3219752754296894559, 0.3333333333333333703, 0.3219752754296894559, 0.3333333333333333703, 0.3219752754296894559, 0.3333333333333333703, 0.3219752754296894559, 0.3333333333333333703, 0.3219752754296894559, 0.3333333333333333703, 0.3219752754296894559, 0.3333333333333333703, 0.3219752754296894559, 0.3333333333333333703, 0.3219752754296894559, 0.3333333333333333703, 0.3219752754296894559, 0.3333333333333333703, 0.3219752754296894559, 0.3333333333333333703, 0.3219752754296894559, 0.3333333333333333703, 0.3219752754296894559, 0.3333333333333333703, 0.3219752754296894559, 0.3333333333333333703, 0.3219752754296894559, 0.3333333333333333703, 0.3219752754296894559, 0.3333333333333333703, 0.3219752754296894559, 0.3333333333333333703, 0.3219752754296894559, 0.3333333333333333703, 0.3219752754296894559, 0.3333333333333333703, 0.3219752754296894559, 0.3333333333333333703, 0.3219752754296894559, 0.3333333333333333703, 0.3219752754296894559, 0.3333333333333333703, 0.3219752754296894559, 0.3333333333333333703, 0.3219752754296894559, 0.3333333333333333703, 0.3219752754296894559, 0.3333333333333333703, 0.3219752754296894559, 0.3333333333333333703, 0.3219752754296894559, 0.3333333333333333703, 0.3219752754296894559, 0.3333333333333333703, 0.3219752754296894559, 0.3333333333333333703, 0.3219752754296894559, 0.3333333333333333703, 0.3219752754296894559, 0.3333333333333333703, 0.3219752754296894559, 0.3333333333333333703, 0.3219752754296894559, 0.3333333333333333703, 0.3219752754296894559, 0.3333333333333333703, 0.3219752754296894559, 0.3333333333333333703, 0.3219752754296894559, 0.3333333333333333703, 0.3219752754296894559, 0.3333333333333333703, 0.3219752754296894559, 0.3333333333333333703, 0.3219752754296894559, 0.3333333333333333703, 0.3219752754296894559, 0.3333333333333333703, 0.3219752754296894559, 0.3333333333333333703, 0.3219752754296894559, 0.3333333333333333703, 0.3219752754296894559, 0.3333333333333333703, 0.3219752754296894559, 0.3333333333333333703, 0.3219752754296894559, 0.3333333333333333703, 0.3219752754296894559, 0.3333333333333333703, 0.3219752754296894559, 0.3333333333333333703, 0.3219752754296894559, 0.3333333333333333703, 0.3219752754296894559, 0.3333333333333333703, 0.3219752754296894559, 0.3333333333333333703, 0.3219752754296894559, 0.3333333333333333703, 0.3219752754296894559, 0.3333333333333333703, 0.3219752754296894559, 0.3333333333333333703, 0.3219752754296894559, 0.3333333333333333703, 0.3219752754296894559, 0.3333333333333333703, 0.3219752754296894559, 0.3333333333333333703, 0.3219752754296894559, 0.3333333333333333703, 0.3219752754296894559, 0.3333333333333333703, 0.3219752754296894559, 0.3333333333333333703, 0.3219752754296894559, 0.3333333333333333703, 0.3219752754296894559, 0.3333333333333333703, 0.3219752754296894559, 0.3333333333333333703, 0.3219752754296894559, 0.3333333333333333703, 0.3219752754296894559, 0.3333333333333333703, 0.3219752754296894559, 0.3333333333333333703, 0.3219752754296894559, 0.3333333333333333703, 0.3219752754296894559, 0.3333333333333333703, 0.3219752754296894559, 0.3333333333333333703, 0.3219752754296894559, 0.3333333333333333703, 0.3219752754296894559, 0.3333333333333333703, 0.3219752754296894559, 0.3333333333333333703, 0.3219752754296894559, 0.3333333333333333703, 0.3219752754296894559, 0.3333333333333333703, 0.3219752754296894559, 0.3333333333333333703, 0.3219752754296894559, 0.3333333333333333703, 0.3219752754296894559, 0.3333333333333333703, 0.3219752754296894559, 0.3333333333333333703, 0.3219752754296894559, 0.3333333333333333703, 0.3219752754296894559, 0.3333333333333333703, 0.3219752754296894559, 0.3333333333333333703, 0.3219752754296894559, 0.3333333333333333703, 0.3219752754296894559, 0.3333333333333333703, 0.3219752754296894559, 0.3333333333333333703, 0.3219752754296894559, 0.3333333333333333703, 0.3219752754296894559, 0.3333333333333333703, 0.3219752754296894559, 0.3333333333333333703, 0.3219752754296894559, 0.3333333333333333703, 0.3219752754296894559, 0.3333333333333333703, 0.3219752754296894559, 0.3333333333333333703, 0.3219752754296894559, 0.3333333333333333703, 0.3219752754296894559, 0.3333333333333333703, 0.3219752754296894559, 0.3333333333333333703, 0.3219752754296894559, 0.3333333333333333703, 0.3219752754296894559, 0.3333333333333333703, 0.3219752754296894559, 0.3333333333333333703, 0.3219752754296894559, 0.3333333333333333703, 0.3219752754296894559, 0.3333333333333333703, 0.3219752754296894559, 0.3333333333333333703, 0.3219752754296894559, 0.3333333333333333703, 0.3219752754296894559, 0.3333333333333333703, 0.3219752754296894559, 0.3333333333333333703, 0.3219752754296894559, 0.3333333333333333703, 0.3219752754296894559, 0.3333333333333333703, 0.3219752754296894559, 0.3333333333333333703, 0.3219752754296894559, 0.3333333333333333703, 0.3219752754296894559, 0.3333333333333333703, 0.3219752754296894559, 0.3333333333333333703, 0.3219752754296894559, 0.3333333333333333703, 0.3219752754296894559, 0.3333333333333333703, 0.3219752754296894559, 0.3333333333333333703, 0.3219752754296894559, 0.3333333333333333703, 0.3219752754296894559, 0.3333333333333333703, 0.3219752754296894559, 0.3333333333333333703, 0.3219752754296894559, 0.3333333333333333703, 0.3219752754296894559, 0.3333333333333333703, 0.3219752754296894559, 0.3333333333333333703, 0.3219752754296894559, 0.3333333333333333703, 0.3219752754296894559, 0.3333333333333333703, 0.3219752754296894559, 0.3333333333333333703, 0.3219752754296894559, 0.3333333333333333703, 0.3219752754296894559, 0.3333333333333333703, 0.3219752754296894559, 0.3333333333333333703, 0.3219752754296894559, 0.3333333333333333703, 0.3219752754296894559, 0.3333333333333333703, 0.3219752754296894559, 0.3333333333333333703, 0.3219752754296894559, 0.3333333333333333703, 0.3219752754296894559, 0.3333333333333333703, 0.3219752754296894559, 0.3333333333333333703, 0.3219752754296894559, 0.3333333333333333703, 0.3219752754296894559, 0.3333333333333333703, 0.3219752754296894559, 0.3333333333333333703, 0.3219752754296894559, 0.3333333333333333703),
 ( 0.3333333333333333703, 0.3219752754296894559, 0.3333333333333333703, 0.3219752754296894559, 0.3333333333333333703, 0.3219752754296894559, 0.3333333333333333703, 0.3219752754296894559, 0.3333333333333333703, 0.3219752754296894559, 0.3333333333333333703, 0.3219752754296894559, 0.3333333333333333703, 0.3219752754296894559, 0.3333333333333333703, 0.3219752754296894559, 0.3333333333333333703, 0.3219752754296894559, 0.3333333333333333703, 0.3219752754296894559, 0.3333333333333333703, 0.3219752754296894559, 0.3333333333333333703, 0.3219752754296894559, 0.3333333333333333703, 0.3219752754296894559, 0.3333333333333333703, 0.3219752754296894559, 0.3333333333333333703, 0.3219752754296894559, 0.3333333333333333703, 0.3219752754296894559, 0.3333333333333333703, 0.3219752754296894559, 0.3333333333333333703, 0.3219752754296894559, 0.3333333333333333703, 0.3219752754296894559, 0.3333333333333333703, 0.3219752754296894559, 0.3333333333333333703, 0.3219752754296894559, 0.3333333333333333703, 0.3219752754296894559, 0.3333333333333333703, 0.3219752754296894559, 0.3333333333333333703, 0.3219752754296894559, 0.3333333333333333703, 0.3219752754296894559, 0.3333333333333333703, 0.3219752754296894559, 0.3333333333333333703, 0.3219752754296894559, 0.3333333333333333703, 0.3219752754296894559, 0.3333333333333333703, 0.3219752754296894559, 0.3333333333333333703, 0.3219752754296894559, 0.3333333333333333703, 0.3219752754296894559, 0.3333333333333333703, 0.3219752754296894559, 0.3333333333333333703, 0.3219752754296894559, 0.3333333333333333703, 0.3219752754296894559, 0.3333333333333333703, 0.3219752754296894559, 0.3333333333333333703, 0.3219752754296894559, 0.3333333333333333703, 0.3219752754296894559, 0.3333333333333333703, 0.3219752754296894559, 0.3333333333333333703, 0.3219752754296894559, 0.3333333333333333703, 0.3219752754296894559, 0.3333333333333333703, 0.3219752754296894559, 0.3333333333333333703, 0.3219752754296894559, 0.3333333333333333703, 0.3219752754296894559, 0.3333333333333333703, 0.3219752754296894559, 0.3333333333333333703, 0.3219752754296894559, 0.3333333333333333703, 0.3219752754296894559, 0.3333333333333333703, 0.3219752754296894559, 0.3333333333333333703, 0.3219752754296894559, 0.3333333333333333703, 0.3219752754296894559, 0.3333333333333333703, 0.3219752754296894559, 0.3333333333333333703, 0.3219752754296894559, 0.3333333333333333703, 0.3219752754296894559, 0.3333333333333333703, 0.3219752754296894559, 0.3333333333333333703, 0.3219752754296894559, 0.3333333333333333703, 0.3219752754296894559, 0.3333333333333333703, 0.3219752754296894559, 0.3333333333333333703, 0.3219752754296894559, 0.3333333333333333703, 0.3219752754296894559, 0.3333333333333333703, 0.3219752754296894559, 0.3333333333333333703, 0.3219752754296894559, 0.3333333333333333703, 0.3219752754296894559, 0.3333333333333333703, 0.3219752754296894559, 0.3333333333333333703, 0.3219752754296894559, 0.3333333333333333703, 0.3219752754296894559, 0.3333333333333333703, 0.3219752754296894559, 0.3333333333333333703, 0.3219752754296894559, 0.3333333333333333703, 0.3219752754296894559, 0.3333333333333333703, 0.3219752754296894559, 0.3333333333333333703, 0.3219752754296894559, 0.3333333333333333703, 0.3219752754296894559, 0.3333333333333333703, 0.3219752754296894559, 0.3333333333333333703, 0.3219752754296894559, 0.3333333333333333703, 0.3219752754296894559, 0.3333333333333333703, 0.3219752754296894559, 0.3333333333333333703, 0.3219752754296894559, 0.3333333333333333703, 0.3219752754296894559, 0.3333333333333333703, 0.3219752754296894559, 0.3333333333333333703, 0.3219752754296894559, 0.3333333333333333703, 0.3219752754296894559, 0.3333333333333333703, 0.3219752754296894559, 0.3333333333333333703, 0.3219752754296894559, 0.3333333333333333703, 0.3219752754296894559, 0.3333333333333333703, 0.3219752754296894559, 0.3333333333333333703, 0.3219752754296894559, 0.3333333333333333703, 0.3219752754296894559, 0.3333333333333333703, 0.3219752754296894559, 0.3333333333333333703, 0.3219752754296894559, 0.3333333333333333703, 0.3219752754296894559, 0.3333333333333333703, 0.3219752754296894559, 0.3333333333333333703, 0.3219752754296894559, 0.3333333333333333703, 0.3219752754296894559, 0.3333333333333333703, 0.3219752754296894559, 0.3333333333333333703, 0.3219752754296894559, 0.3333333333333333703, 0.3219752754296894559, 0.3333333333333333703, 0.3219752754296894559, 0.3333333333333333703, 0.3219752754296894559, 0.3333333333333333703, 0.3219752754296894559, 0.3333333333333333703, 0.3219752754296894559, 0.3333333333333333703, 0.3219752754296894559, 0.3333333333333333703, 0.3219752754296894559, 0.3333333333333333703, 0.3219752754296894559, 0.3333333333333333703, 0.3219752754296894559, 0.3333333333333333703, 0.3219752754296894559, 0.3333333333333333703, 0.3219752754296894559, 0.3333333333333333703, 0.3219752754296894559, 0.3333333333333333703, 0.3219752754296894559, 0.3333333333333333703, 0.3219752754296894559, 0.3333333333333333703, 0.3219752754296894559, 0.3333333333333333703, 0.3219752754296894559, 0.3333333333333333703, 0.3219752754296894559, 0.3333333333333333703, 0.3219752754296894559, 0.3333333333333333703, 0.3219752754296894559, 0.3333333333333333703, 0.3219752754296894559, 0.3333333333333333703, 0.3219752754296894559, 0.3333333333333333703, 0.3219752754296894559, 0.3333333333333333703, 0.3219752754296894559, 0.3333333333333333703, 0.3219752754296894559, 0.3333333333333333703, 0.3219752754296894559, 0.3333333333333333703, 0.3219752754296894559, 0.3333333333333333703, 0.3219752754296894559, 0.3333333333333333703, 0.3219752754296894559, 0.3333333333333333703, 0.3219752754296894559, 0.3333333333333333703, 0.3219752754296894559, 0.3333333333333333703, 0.3219752754296894559, 0.3333333333333333703, 0.3219752754296894559, 0.3333333333333333703, 0.3219752754296894559, 0.3333333333333333703, 0.3219752754296894559, 0.3333333333333333703, 0.3219752754296894559, 0.3333333333333333703, 0.3219752754296894559, 0.3333333333333333703, 0.3219752754296894559, 0.3333333333333333703, 0.3219752754296894559, 0.3333333333333333703, 0.3219752754296894559, 0.3333333333333333703, 0.3219752754296894559, 0.3333333333333333703, 0.3219752754296894559, 0.3333333333333333703, 0.3219752754296894559, 0.3333333333333333703, 0.3219752754296894559, 0.3333333333333333703, 0.3219752754296894559, 0.3333333333333333703, 0.3219752754296894559, 0.3333333333333333703, 0.3219752754296894559, 0.3333333333333333703, 0.3219752754296894559, 0.3333333333333333703, 0.3219752754296894559, 0.3333333333333333703, 0.3219752754296894559, 0.3333333333333333703, 0.3219752754296894559, 0.3333333333333333703, 0.3219752754296894559, 0.3333333333333333703, 0.3219752754296894559, 0.3333333333333333703, 0.3219752754296894559, 0.3333333333333333703, 0.3219752754296894559, 0.3333333333333333703, 0.3219752754296894559, 0.3333333333333333703, 0.3219752754296894559, 0.3333333333333333703, 0.3219752754296894559, 0.3333333333333333703, 0.3219752754296894559, 0.3333333333333333703, 0.3219752754296894559, 0.3333333333333333703, 0.3219752754296894559, 0.3333333333333333703, 0.3219752754296894559, 0.3333333333333333703, 0.3219752754296894559, 0.3333333333333333703, 0.3219752754296894559, 0.3333333333333333703, 0.3219752754296894559, 0.3333333333333333703, 0.3219752754296894559, 0.3333333333333333703, 0.3219752754296894559, 0.3333333333333333703, 0.3219752754296894559, 0.3333333333333333703, 0.3219752754296894559, 0.3333333333333333703, 0.3219752754296894559, 0.3333333333333333703, 0.3219752754296894559, 0.3333333333333333703, 0.3219752754296894559, 0.3333333333333333703, 0.3219752754296894559, 0.3333333333333333703, 0.3219752754296894559, 0.3333333333333333703, 0.3219752754296894559, 0.3333333333333333703, 0.3219752754296894559, 0.3333333333333333703, 0.3219752754296894559, 0.3333333333333333703, 0.3219752754296894559, 0.3333333333333333703, 0.3219752754296894559, 0.3333333333333333703, 0.3219752754296894559, 0.3333333333333333703, 0.3219752754296894559, 0.3333333333333333703, 0.3219752754296894559, 0.3333333333333333703, 0.3219752754296894559, 0.3333333333333333703, 0.3219752754296894559, 0.3333333333333333703, 0.3219752754296894559, 0.3333333333333333703, 0.3219752754296894559, 0.3333333333333333703, 0.3219752754296894559, 0.3333333333333333703, 0.3219752754296894559, 0.3333333333333333703, 0.3219752754296894559, 0.3333333333333333703, 0.3219752754296894559, 0.3333333333333333703, 0.3219752754296894559, 0.3333333333333333703, 0.3219752754296894559, 0.3333333333333333703, 0.3219752754296894559, 0.3333333333333333703, 0.3219752754296894559, 0.3333333333333333703, 0.3219752754296894559, 0.3333333333333333703, 0.3219752754296894559, 0.3333333333333333703, 0.3219752754296894559, 0.3333333333333333703, 0.3219752754296894559, 0.3333333333333333703, 0.3219752754296894559, 0.3333333333333333703, 0.3219752754296894559, 0.3333333333333333703, 0.3219752754296894559, 0.3333333333333333703, 0.3219752754296894559, 0.3333333333333333703, 0.3219752754296894559, 0.3333333333333333703, 0.3219752754296894559, 0.3333333333333333703, 0.3219752754296894559, 0.3333333333333333703, 0.3219752754296894559, 0.3333333333333333703, 0.3219752754296894559, 0.3333333333333333703, 0.3219752754296894559, 0.3333333333333333703, 0.3219752754296894559, 0.3333333333333333703, 0.3219752754296894559, 0.3333333333333333703, 0.3219752754296894559, 0.3333333333333333703, 0.3219752754296894559, 0.3333333333333333703, 0.3219752754296894559, 0.3333333333333333703, 0.3219752754296894559, 0.3333333333333333703, 0.3219752754296894559, 0.3333333333333333703, 0.3219752754296894559, 0.3333333333333333703, 0.3219752754296894559, 0.3333333333333333703, 0.3219752754296894559, 0.3333333333333333703, 0.3219752754296894559, 0.3333333333333333703, 0.3219752754296894559, 0.3333333333333333703, 0.3219752754296894559, 0.3333333333333333703, 0.3219752754296894559, 0.3333333333333333703, 0.3219752754296894559, 0.3333333333333333703, 0.3219752754296894559, 0.3333333333333333703, 0.3219752754296894559, 0.3333333333333333703, 0.3219752754296894559, 0.3333333333333333703, 0.3219752754296894559, 0.3333333333333333703, 0.3219752754296894559, 0.3333333333333333703, 0.3219752754296894559, 0.3333333333333333703, 0.3219752754296894559, 0.3333333333333333703, 0.3219752754296894559, 0.3333333333333333703, 0.3219752754296894559, 0.3333333333333333703, 0.3219752754296894559, 0.3333333333333333703, 0.3219752754296894559, 0.3333333333333333703, 0.3219752754296894559, 0.3333333333333333703, 0.3219752754296894559, 0.3333333333333333703),
 ( 1.000000000000000000, 0.9659258262890683122, 1.000000000000000000, 0.9659258262890683122, 1.000000000000000000, 0.9659258262890683122, 1.000000000000000000, 0.9659258262890683122, 1.000000000000000000, 0.9659258262890683122, 1.000000000000000000, 0.9659258262890683122, 1.000000000000000000, 0.9659258262890683122, 1.000000000000000000, 0.9659258262890683122, 1.000000000000000000, 0.9659258262890683122, 1.000000000000000000, 0.9659258262890683122, 1.000000000000000000, 0.9659258262890683122, 1.000000000000000000, 0.9659258262890683122, 1.000000000000000000, 0.9659258262890683122, 1.000000000000000000, 0.9659258262890683122, 1.000000000000000000, 0.9659258262890683122, 1.000000000000000000, 0.9659258262890683122, 1.000000000000000000, 0.9659258262890683122, 1.000000000000000000, 0.9659258262890683122, 1.000000000000000000, 0.9659258262890683122, 1.000000000000000000, 0.9659258262890683122, 1.000000000000000000, 0.9659258262890683122, 1.000000000000000000, 0.9659258262890683122, 1.000000000000000000, 0.9659258262890683122, 1.000000000000000000, 0.9659258262890683122, 1.000000000000000000, 0.9659258262890683122, 1.000000000000000000, 0.9659258262890683122, 1.000000000000000000, 0.9659258262890683122, 1.000000000000000000, 0.9659258262890683122, 1.000000000000000000, 0.9659258262890683122, 1.000000000000000000, 0.9659258262890683122, 1.000000000000000000, 0.9659258262890683122, 1.000000000000000000, 0.9659258262890683122, 1.000000000000000000, 0.9659258262890683122, 1.000000000000000000, 0.9659258262890683122, 1.000000000000000000, 0.9659258262890683122, 1.000000000000000000, 0.9659258262890683122, 1.000000000000000000, 0.9659258262890683122, 1.000000000000000000, 0.9659258262890683122, 1.000000000000000000, 0.9659258262890683122, 1.000000000000000000, 0.9659258262890683122, 1.000000000000000000, 0.9659258262890683122, 1.000000000000000000, 0.9659258262890683122, 1.000000000000000000, 0.9659258262890683122, 1.000000000000000000, 0.9659258262890683122, 1.000000000000000000, 0.9659258262890683122, 1.000000000000000000, 0.9659258262890683122, 1.000000000000000000, 0.9659258262890683122, 1.000000000000000000, 0.9659258262890683122, 1.000000000000000000, 0.9659258262890683122, 1.000000000000000000, 0.9659258262890683122, 1.000000000000000000, 0.9659258262890683122, 1.000000000000000000, 0.9659258262890683122, 1.000000000000000000, 0.9659258262890683122, 1.000000000000000000, 0.9659258262890683122, 1.000000000000000000, 0.9659258262890683122, 1.000000000000000000, 0.9659258262890683122, 1.000000000000000000, 0.9659258262890683122, 1.000000000000000000, 0.9659258262890683122, 1.000000000000000000, 0.9659258262890683122, 1.000000000000000000, 0.9659258262890683122, 1.000000000000000000, 0.9659258262890683122, 1.000000000000000000, 0.9659258262890683122, 1.000000000000000000, 0.9659258262890683122, 1.000000000000000000, 0.9659258262890683122, 1.000000000000000000, 0.9659258262890683122, 1.000000000000000000, 0.9659258262890683122, 1.000000000000000000, 0.9659258262890683122, 1.000000000000000000, 0.9659258262890683122, 1.000000000000000000, 0.9659258262890683122, 1.000000000000000000, 0.9659258262890683122, 1.000000000000000000, 0.9659258262890683122, 1.000000000000000000, 0.9659258262890683122, 1.000000000000000000, 0.9659258262890683122, 1.000000000000000000, 0.9659258262890683122, 1.000000000000000000, 0.9659258262890683122, 1.000000000000000000, 0.9659258262890683122, 1.000000000000000000, 0.9659258262890683122, 1.000000000000000000, 0.9659258262890683122, 1.000000000000000000, 0.9659258262890683122, 1.000000000000000000, 0.9659258262890683122, 1.000000000000000000, 0.9659258262890683122, 1.000000000000000000, 0.9659258262890683122, 1.000000000000000000, 0.9659258262890683122, 1.000000000000000000, 0.9659258262890683122, 1.000000000000000000, 0.9659258262890683122, 1.000000000000000000, 0.9659258262890683122, 1.000000000000000000, 0.9659258262890683122, 1.000000000000000000, 0.9659258262890683122, 1.000000000000000000, 0.9659258262890683122, 1.000000000000000000, 0.9659258262890683122, 1.000000000000000000, 0.9659258262890683122, 1.000000000000000000, 0.9659258262890683122, 1.000000000000000000, 0.9659258262890683122, 1.000000000000000000, 0.9659258262890683122, 1.000000000000000000, 0.9659258262890683122, 1.000000000000000000, 0.9659258262890683122, 1.000000000000000000, 0.9659258262890683122, 1.000000000000000000, 0.9659258262890683122, 1.000000000000000000, 0.9659258262890683122, 1.000000000000000000, 0.9659258262890683122, 1.000000000000000000, 0.9659258262890683122, 1.000000000000000000, 0.9659258262890683122, 1.000000000000000000, 0.9659258262890683122, 1.000000000000000000, 0.9659258262890683122, 1.000000000000000000, 0.9659258262890683122, 1.000000000000000000, 0.9659258262890683122, 1.000000000000000000, 0.9659258262890683122, 1.000000000000000000, 0.9659258262890683122, 1.000000000000000000, 0.9659258262890683122, 1.000000000000000000, 0.9659258262890683122, 1.000000000000000000, 0.9659258262890683122, 1.000000000000000000, 0.9659258262890683122, 1.000000000000000000, 0.9659258262890683122, 1.000000000000000000, 0.9659258262890683122, 1.000000000000000000, 0.9659258262890683122, 1.000000000000000000, 0.9659258262890683122, 1.000000000000000000, 0.9659258262890683122, 1.000000000000000000, 0.9659258262890683122, 1.000000000000000000, 0.9659258262890683122, 1.000000000000000000, 0.9659258262890683122, 1.000000000000000000, 0.9659258262890683122, 1.000000000000000000, 0.9659258262890683122, 1.000000000000000000, 0.9659258262890683122, 1.000000000000000000, 0.9659258262890683122, 1.000000000000000000, 0.9659258262890683122, 1.000000000000000000, 0.9659258262890683122, 1.000000000000000000, 0.9659258262890683122, 1.000000000000000000, 0.9659258262890683122, 1.000000000000000000, 0.9659258262890683122, 1.000000000000000000, 0.9659258262890683122, 1.000000000000000000, 0.9659258262890683122, 1.000000000000000000, 0.9659258262890683122, 1.000000000000000000, 0.9659258262890683122, 1.000000000000000000, 0.9659258262890683122, 1.000000000000000000, 0.9659258262890683122, 1.000000000000000000, 0.9659258262890683122, 1.000000000000000000, 0.9659258262890683122, 1.000000000000000000, 0.9659258262890683122, 1.000000000000000000, 0.9659258262890683122, 1.000000000000000000, 0.9659258262890683122, 1.000000000000000000, 0.9659258262890683122, 1.000000000000000000, 0.9659258262890683122, 1.000000000000000000, 0.9659258262890683122, 1.000000000000000000, 0.9659258262890683122, 1.000000000000000000, 0.9659258262890683122, 1.000000000000000000, 0.9659258262890683122, 1.000000000000000000, 0.9659258262890683122, 1.000000000000000000, 0.9659258262890683122, 1.000000000000000000, 0.9659258262890683122, 1.000000000000000000, 0.9659258262890683122, 1.000000000000000000, 0.9659258262890683122, 1.000000000000000000, 0.9659258262890683122, 1.000000000000000000, 0.9659258262890683122, 1.000000000000000000, 0.9659258262890683122, 1.000000000000000000, 0.9659258262890683122, 1.000000000000000000, 0.9659258262890683122, 1.000000000000000000, 0.9659258262890683122, 1.000000000000000000, 0.9659258262890683122, 1.000000000000000000, 0.9659258262890683122, 1.000000000000000000, 0.9659258262890683122, 1.000000000000000000, 0.9659258262890683122, 1.000000000000000000, 0.9659258262890683122, 1.000000000000000000, 0.9659258262890683122, 1.000000000000000000, 0.9659258262890683122, 1.000000000000000000, 0.9659258262890683122, 1.000000000000000000, 0.9659258262890683122, 1.000000000000000000, 0.9659258262890683122, 1.000000000000000000, 0.9659258262890683122, 1.000000000000000000, 0.9659258262890683122, 1.000000000000000000, 0.9659258262890683122, 1.000000000000000000, 0.9659258262890683122, 1.000000000000000000, 0.9659258262890683122, 1.000000000000000000, 0.9659258262890683122, 1.000000000000000000, 0.9659258262890683122, 1.000000000000000000, 0.9659258262890683122, 1.000000000000000000, 0.9659258262890683122, 1.000000000000000000, 0.9659258262890683122, 1.000000000000000000, 0.9659258262890683122, 1.000000000000000000, 0.9659258262890683122, 1.000000000000000000, 0.9659258262890683122, 1.000000000000000000, 0.9659258262890683122, 1.000000000000000000, 0.9659258262890683122, 1.000000000000000000, 0.9659258262890683122, 1.000000000000000000, 0.9659258262890683122, 1.000000000000000000, 0.9659258262890683122, 1.000000000000000000, 0.9659258262890683122, 1.000000000000000000, 0.9659258262890683122, 1.000000000000000000, 0.9659258262890683122, 1.000000000000000000, 0.9659258262890683122, 1.000000000000000000, 0.9659258262890683122, 1.000000000000000000, 0.9659258262890683122, 1.000000000000000000, 0.9659258262890683122, 1.000000000000000000, 0.9659258262890683122, 1.000000000000000000, 0.9659258262890683122, 1.000000000000000000, 0.9659258262890683122, 1.000000000000000000, 0.9659258262890683122, 1.000000000000000000, 0.9659258262890683122, 1.000000000000000000, 0.9659258262890683122, 1.000000000000000000, 0.9659258262890683122, 1.000000000000000000, 0.9659258262890683122, 1.000000000000000000, 0.9659258262890683122, 1.000000000000000000, 0.9659258262890683122, 1.000000000000000000, 0.9659258262890683122, 1.000000000000000000, 0.9659258262890683122, 1.000000000000000000, 0.9659258262890683122, 1.000000000000000000, 0.9659258262890683122, 1.000000000000000000, 0.9659258262890683122, 1.000000000000000000, 0.9659258262890683122, 1.000000000000000000, 0.9659258262890683122, 1.000000000000000000, 0.9659258262890683122, 1.000000000000000000, 0.9659258262890683122, 1.000000000000000000, 0.9659258262890683122, 1.000000000000000000, 0.9659258262890683122, 1.000000000000000000, 0.9659258262890683122, 1.000000000000000000, 0.9659258262890683122, 1.000000000000000000, 0.9659258262890683122, 1.000000000000000000, 0.9659258262890683122, 1.000000000000000000, 0.9659258262890683122, 1.000000000000000000, 0.9659258262890683122, 1.000000000000000000, 0.9659258262890683122, 1.000000000000000000, 0.9659258262890683122, 1.000000000000000000, 0.9659258262890683122, 1.000000000000000000, 0.9659258262890683122, 1.000000000000000000, 0.9659258262890683122, 1.000000000000000000, 0.9659258262890683122, 1.000000000000000000, 0.9659258262890683122, 1.000000000000000000, 0.9659258262890683122, 1.000000000000000000, 0.9659258262890683122, 1.000000000000000000) ) ) 
 REPRESENTATION_ITEM ( '' )  SURFACE ( )  );
#96545=CARTESIAN_POINT ( 'NONE',  ( -21.52544592524343514, 5.823673210054127303, 66.04057627198103830 ) ) ;
#96546=CARTESIAN_POINT ( 'NONE',  ( -16.53943276465976808, 0.05219959533911058130, 71.24890960531435269 ) ) ;
#96547=CARTESIAN_POINT ( 'NONE',  ( -10.81492255796105439, 18.62759615963255655, 112.9177570613523329 ) ) ;
#96549=CARTESIAN_POINT ( 'NONE',  ( 5.823673210054125526, 21.52544592524343514, 29.79057627198102409 ) ) ;
#96550=CARTESIAN_POINT ( 'NONE',  ( -19.02544592524342804, 5.153800228976336051, 56.04057627198100988 ) ) ;
#96551=CARTESIAN_POINT ( 'NONE',  ( 19.02544592524343514, -5.153800228976328945, 33.54057627198102409 ) ) ;
#96552=CARTESIAN_POINT ( 'NONE',  ( -4.379528057220328563, 16.55341960407611168, 105.2072429386477097 ) ) ;
#96553=CARTESIAN_POINT ( 'NONE',  ( 18.62759615963271287, -10.81492255796078972, 113.3322429386476955 ) ) ;
#96555=CARTESIAN_POINT ( 'NONE',  ( -21.53943276465977519, -0.05219959533937600094, 28.75109039468567929 ) ) ;
#96556=CARTESIAN_POINT ( 'NONE',  ( 13.89961937509977652, -13.97604488694527269, 23.12390960531436335 ) ) ;
#96557=CARTESIAN_POINT ( 'NONE',  ( 10.72451020669871369, 18.67979575497193778, 82.08442372801901854 ) ) ;
#96558=CARTESIAN_POINT ( 'NONE',  ( 21.55341960407610458, 5.719274019375980345, 98.95724293864770971 ) ) ;
#96559=CARTESIAN_POINT ( 'NONE',  ( -19.03943276465977164, -0.05219959533935918106, 33.75109039468566863 ) ) ;
#96560=CARTESIAN_POINT ( 'NONE',  ( -9.474510206698964154, 16.51473224551069663, 25.41557627198103120 ) ) ;
#96562=CARTESIAN_POINT ( 'NONE',  ( -17.58332526062525858, 7.635886036038558977, 60.92334959558466778 ) ) ;
#96563=CARTESIAN_POINT ( 'NONE',  ( 14.34966873604972726, -8.224510206698740333, 45.83442372801901854 ) ) ;
#96564=CARTESIAN_POINT ( 'NONE',  ( -14.29746914071049879, 8.314922557960819915, 105.8322429386476955 ) ) ;
#96566=CARTESIAN_POINT ( 'NONE',  ( -19.02544592524342804, 5.153800228976336051, 66.04057627198103830 ) ) ;
#96567=CARTESIAN_POINT ( 'NONE',  ( -0.05219959533910754901, -16.53943276465976808, 87.49890960531436690 ) ) ;
#96568=CARTESIAN_POINT ( 'NONE',  ( -10.81492255796078084, -18.62759615963271287, 52.08224293864768839 ) ) ;
#96569=CARTESIAN_POINT ( 'NONE',  ( -0.05219959533910754901, -16.53943276465976808, 67.49890960531436690 ) ) ;
#96570=CARTESIAN_POINT ( 'NONE',  ( -12.14591786802326823, 12.06949235617739902, 38.12609039468567573 ) ) ;
#96571=CARTESIAN_POINT ( 'NONE',  ( 10.81492255796106328, -18.62759615963255655, 90.41775706135236135 ) ) ;
#96572=CARTESIAN_POINT ( 'NONE',  ( -0.05219959533936034679, 19.03943276465977164, 62.50109039468566863 ) ) ;
#96573=CARTESIAN_POINT ( 'NONE',  ( -14.34966873604972548, 8.224510206698743886, 98.33442372801901854 ) ) ;
#96574=CARTESIAN_POINT ( 'NONE',  ( 4.483927247898545687, 16.52544592524342804, 39.79057627198103830 ) ) ;
#96575=CARTESIAN_POINT ( 'NONE',  ( 19.05341960407611168, 5.049401038298154454, 43.95724293864769550 ) ) ;
#96576=CARTESIAN_POINT ( 'NONE',  ( -10.72451020669870658, -18.67979575497194134, 94.58442372801901854 ) ) ;
#96577=CARTESIAN_POINT ( 'NONE',  ( 21.53943276465977519, -0.05219959533907433946, 103.7489096053143669 ) ) ;
#96578=CARTESIAN_POINT ( 'NONE',  ( -15.72974639402176322, -15.80617190586768395, 64.37609039468568994 ) ) ;
#96579=CARTESIAN_POINT ( 'NONE',  ( 16.53943276465976808, 0.05219959533934440121, 41.25109039468568284 ) ) ;
#96580=CARTESIAN_POINT ( 'NONE',  ( -16.53943276465976808, 0.05219959533911058130, 66.24890960531436690 ) ) ;
#96581=CARTESIAN_POINT ( 'NONE',  ( 21.52544592524334988, 5.823673210054432836, 81.45942372801900433 ) ) ;
#96582=CARTESIAN_POINT ( 'NONE',  ( 8.314922557960818139, 14.29746914071049879, 24.58224293864768839 ) ) ;
#96583=CARTESIAN_POINT ( 'NONE',  ( 16.20579543436680936, 7.371946100354974440, 28.06520834171877965 ) ) ;
#96585=CARTESIAN_POINT ( 'NONE',  ( -12.06949235617756955, 12.14591786802309770, 25.62390960531435624 ) ) ;
#96586=CARTESIAN_POINT ( 'NONE',  ( -8.314922557961024197, 14.29746914071037800, 77.91775706135231871 ) ) ;
#96587=CARTESIAN_POINT ( 'NONE',  ( -16.51473224551069308, -9.474510206698971260, 86.66557627198102409 ) ) ;
#96588=CARTESIAN_POINT ( 'NONE',  ( -16.46253265017160317, 9.564922557960807481, 100.8322429386477097 ) ) ;
#96589=CARTESIAN_POINT ( 'NONE',  ( -10.81492255796105439, 18.62759615963255655, 87.91775706135234714 ) ) ;
#96590=CARTESIAN_POINT ( 'NONE',  ( 16.53943276465976808, 0.05219959533934440121, 86.25109039468568994 ) ) ;
#96591=CARTESIAN_POINT ( 'NONE',  ( -4.379528057220328563, 16.55341960407611168, 60.20724293864768839 ) ) ;
#96592=CARTESIAN_POINT ( 'NONE',  ( -16.51473224551069308, -9.474510206698971260, 71.66557627198102409 ) ) ;
#96594=CARTESIAN_POINT ( 'NONE',  ( -8.314922557961024197, 14.29746914071037800, 22.91775706135235069 ) ) ;
#96595=CARTESIAN_POINT ( 'NONE',  ( 9.474510206698971260, -16.51473224551069308, 22.91557627198102765 ) ) ;
#96596=CARTESIAN_POINT ( 'NONE',  ( -19.05341960407611168, -5.049401038298163336, 96.45724293864769550 ) ) ;
#96597=CARTESIAN_POINT ( 'NONE',  ( -0.05219959533934338120, 16.53943276465976808, 22.50109039468567573 ) ) ;
#96599=CARTESIAN_POINT ( 'NONE',  ( -16.46253265017146816, -9.564922557961047289, 24.16775706135233648 ) ) ;
#96600=CARTESIAN_POINT ( 'NONE',  ( 4.483927247898790824, -16.52544592524335698, 95.20942372801903275 ) ) ;
#96601=CARTESIAN_POINT ( 'NONE',  ( -16.46253265017146816, -9.564922557961047289, 109.1677570613523471 ) ) ;
#96602=CARTESIAN_POINT ( 'NONE',  ( -13.89961937509977652, 13.97604488694528158, 25.62390960531434558 ) ) ;
#96603=CARTESIAN_POINT ( 'NONE',  ( -12.14591786802326823, 12.06949235617739902, 73.12609039468567573 ) ) ;
#96604=CARTESIAN_POINT ( 'NONE',  ( 16.52544592524335698, 4.483927247898782831, 56.45942372801902565 ) ) ;
#96605=CARTESIAN_POINT ( 'NONE',  ( -16.51473224551069308, -9.474510206698971260, 21.66557627198102765 ) ) ;
#96606=CARTESIAN_POINT ( 'NONE',  ( -9.564922557961040184, 16.46253265017147172, 67.91775706135233293 ) ) ;
#96607=CARTESIAN_POINT ( 'NONE',  ( 10.81492255796106328, -18.62759615963255655, 110.4177570613523756 ) ) ;
#96608=CARTESIAN_POINT ( 'NONE',  ( 19.03943276465977164, -0.05219959533909143690, 43.74890960531435979 ) ) ;
#96609=CARTESIAN_POINT ( 'NONE',  ( -0.05219959533909027116, -19.03943276465977164, 77.49890960531435269 ) ) ;
#96610=CARTESIAN_POINT ( 'NONE',  ( 4.379528057220339221, -16.55341960407611168, 72.70724293864769550 ) ) ;
#96611=EDGE_CURVE ( 'NONE', #27205, #20950, #76783, .T. ) ;
#96612=CARTESIAN_POINT ( 'NONE',  ( 0.05219959533936267826, -19.03943276465977164, 45.00109039468566863 ) ) ;
#96613=CARTESIAN_POINT ( 'NONE',  ( -21.53943276465977519, 0.05219959533907696930, 31.24890960531435979 ) ) ;
#96614=CARTESIAN_POINT ( 'NONE',  ( -5.719274019375665041, -21.55341960407619695, 109.7927570613523613 ) ) ;
#96615=CARTESIAN_POINT ( 'NONE',  ( -5.049401038298153566, 19.05341960407611168, 90.20724293864766707 ) ) ;
#96616=CARTESIAN_POINT ( 'NONE',  ( -10.72451020669870658, -18.67979575497194134, 104.5844237280190185 ) ) ;
#96617=CARTESIAN_POINT ( 'NONE',  ( 0.05219959533907565091, 21.53943276465977519, 69.99890960531435269 ) ) ;
#96618=CARTESIAN_POINT ( 'NONE',  ( -13.97604488694527625, -13.89961937509977652, 91.87390960531432427 ) ) ;
#96619=CARTESIAN_POINT ( 'NONE',  ( 16.46253265017146816, 9.564922557961045513, 91.66775706135234714 ) ) ;
#96620=CARTESIAN_POINT ( 'NONE',  ( -9.474510206698964154, 16.51473224551069663, 105.4155762719810383 ) ) ;
#96621=CARTESIAN_POINT ( 'NONE',  ( -14.29746914071037622, -8.314922557961029526, 19.16775706135234714 ) ) ;
#96622=CARTESIAN_POINT ( 'NONE',  ( -9.474510206698964154, 16.51473224551069663, 25.41557627198103120 ) ) ;
#96623=CARTESIAN_POINT ( 'NONE',  ( -5.049401038298153566, 19.05341960407611168, 90.20724293864766707 ) ) ;
#96624=CARTESIAN_POINT ( 'NONE',  ( -21.53943276465977519, 0.05219959533907696930, 61.24890960531435979 ) ) ;
#96626=CARTESIAN_POINT ( 'NONE',  ( 16.55341960407618274, -4.379528057220086978, 41.04275706135236135 ) ) ;
#96627=CARTESIAN_POINT ( 'NONE',  ( 21.53943276465977519, 0.05219959533937863772, 41.25109039468568284 ) ) ;
#96628=CARTESIAN_POINT ( 'NONE',  ( -21.55341960407619339, 5.719274019375674811, 93.54275706135234714 ) ) ;
#96629=CARTESIAN_POINT ( 'NONE',  ( -8.224510206698735004, -14.34966873604973081, 99.58442372801900433 ) ) ;
#96630=CARTESIAN_POINT ( 'NONE',  ( 5.049401038298161559, -19.05341960407611168, 92.70724293864769550 ) ) ;
#96631=CARTESIAN_POINT ( 'NONE',  ( -16.52544592524342804, 4.483927247898546575, 86.04057627198102409 ) ) ;
#96632=CARTESIAN_POINT ( 'NONE',  ( 12.06949235617739724, 12.14591786802326823, 111.8760903946856615 ) ) ;
#96633=CARTESIAN_POINT ( 'NONE',  ( 19.02544592524334988, 5.153800228976608722, 66.45942372801899012 ) ) ;
#96634=CARTESIAN_POINT ( 'NONE',  ( 0.05219959533937995610, -21.53943276465977519, 40.00109039468567573 ) ) ;
#96635=CARTESIAN_POINT ( 'NONE',  ( -14.29746914071049879, 8.314922557960819915, 85.83224293864768129 ) ) ;
#96636=CARTESIAN_POINT ( 'NONE',  ( -5.153800228976328057, -19.02544592524343514, 107.2905762719810383 ) ) ;
#96637=CARTESIAN_POINT ( 'NONE',  ( -4.379528057220086978, -16.55341960407618274, 109.7927570613523613 ) ) ;
#96638=CARTESIAN_POINT ( 'NONE',  ( -10.72451020669870658, -18.67979575497194134, 84.58442372801903275 ) ) ;
#96639=CARTESIAN_POINT ( 'NONE',  ( -8.224510206698735004, -14.34966873604973081, 59.58442372801901854 ) ) ;
#96640=CARTESIAN_POINT ( 'NONE',  ( 15.80617190586769283, -15.72974639402175789, 40.62609039468567573 ) ) ;
#96642=CARTESIAN_POINT ( 'NONE',  ( 10.72451020669871369, 18.67979575497193778, 32.08442372801901854 ) ) ;
#96643=CARTESIAN_POINT ( 'NONE',  ( 4.483927247898545687, 16.52544592524342804, 104.7905762719810241 ) ) ;
#96644=CARTESIAN_POINT ( 'NONE',  ( 9.474510206698971260, -16.51473224551069308, 22.91557627198102765 ) ) ;
#96645=CARTESIAN_POINT ( 'NONE',  ( -4.379528057220328563, 16.55341960407611168, 70.20724293864769550 ) ) ;
#96646=CARTESIAN_POINT ( 'NONE',  ( 5.153800228976335163, 19.02544592524342804, 54.79057627198103120 ) ) ;
#96647=CARTESIAN_POINT ( 'NONE',  ( 4.379528057220092307, 16.55341960407617563, 107.2927570613523471 ) ) ;
#96648=CARTESIAN_POINT ( 'NONE',  ( -19.02544592524342804, 5.153800228976336051, 36.04057627198100988 ) ) ;
#96649=CARTESIAN_POINT ( 'NONE',  ( 10.72451020669898902, -18.67979575497178502, 37.91557627198102409 ) ) ;
#96650=CARTESIAN_POINT ( 'NONE',  ( -0.05219959533910754901, -16.53943276465976808, 82.49890960531436690 ) ) ;
#96651=CIRCLE ( 'NONE', #161332, 2.500000000000002220 ) ;
#96652=CARTESIAN_POINT ( 'NONE',  ( -15.80617190586745835, -15.72974639402198527, 91.87390960531436690 ) ) ;
#96653=CARTESIAN_POINT ( 'NONE',  ( -13.97604488694527625, -13.89961937509977652, 91.87390960531432427 ) ) ;
#96654=CARTESIAN_POINT ( 'NONE',  ( -16.51473224551069308, -9.474510206698971260, 51.66557627198102409 ) ) ;
#96655=CARTESIAN_POINT ( 'NONE',  ( 19.05341960407617918, -5.049401038297876454, 91.04275706135234714 ) ) ;
#96656=CARTESIAN_POINT ( 'NONE',  ( -21.55341960407610458, -5.719274019375992779, 46.45724293864769550 ) ) ;
#96657=CARTESIAN_POINT ( 'NONE',  ( 15.80617190586769283, -15.72974639402175789, 70.62609039468567573 ) ) ;
#96658=CARTESIAN_POINT ( 'NONE',  ( 13.89961937509977652, -13.97604488694527269, 53.12390960531434558 ) ) ;
#96659=CARTESIAN_POINT ( 'NONE',  ( -9.564922557960796823, -16.46253265017161027, 87.08224293864769550 ) ) ;
#96661=CARTESIAN_POINT ( 'NONE',  ( -8.224510206698735004, -14.34966873604973081, 69.58442372801900433 ) ) ;
#96662=CARTESIAN_POINT ( 'NONE',  ( -15.80617190586768217, 15.72974639402176855, 43.12609039468568284 ) ) ;
#96663=CARTESIAN_POINT ( 'NONE',  ( -10.72451020669870658, -18.67979575497194134, 79.58442372801903275 ) ) ;
#96664=CARTESIAN_POINT ( 'NONE',  ( 18.67979575497178502, 10.72451020669898547, 24.16557627198103120 ) ) ;
#96665=CARTESIAN_POINT ( 'NONE',  ( 21.53943276465977519, -0.05219959533907433946, 93.74890960531436690 ) ) ;
#96666=CARTESIAN_POINT ( 'NONE',  ( 21.55341960407619695, -5.719274019375665929, 36.04275706135234714 ) ) ;
#96667=CARTESIAN_POINT ( 'NONE',  ( 4.483927247898790824, -16.52544592524335698, 70.20942372801904696 ) ) ;
#96668=CARTESIAN_POINT ( 'NONE',  ( -15.80617190586745835, -15.72974639402198527, 61.87390960531436690 ) ) ;
#96669=CARTESIAN_POINT ( 'NONE',  ( 16.46253265017146816, 9.564922557961045513, 31.66775706135232937 ) ) ;
#96670=CARTESIAN_POINT ( 'NONE',  ( 16.46253265017160672, -9.564922557960803928, 68.33224293864770971 ) ) ;
#96671=CARTESIAN_POINT ( 'NONE',  ( -8.314922557961024197, 14.29746914071037800, 102.9177570613523756 ) ) ;
#96673=CARTESIAN_POINT ( 'NONE',  ( -0.05219959533909027116, -19.03943276465977164, 102.4989096053143669 ) ) ;
#96675=CARTESIAN_POINT ( 'NONE',  ( 5.049401038297881783, 19.05341960407617563, 77.29275706135231871 ) ) ;
#96676=CARTESIAN_POINT ( 'NONE',  ( 18.62759615963271287, -10.81492255796078972, 63.33224293864770260 ) ) ;
#96677=CARTESIAN_POINT ( 'NONE',  ( -16.55341960407611168, -4.379528057220339221, 41.45724293864769550 ) ) ;
#96678=CARTESIAN_POINT ( 'NONE',  ( 0.05219959533936267826, -19.03943276465977164, 95.00109039468567573 ) ) ;
#96679=CARTESIAN_POINT ( 'NONE',  ( 13.97604488694527802, 13.89961937509977652, 34.37390960531436690 ) ) ;
#96680=CARTESIAN_POINT ( 'NONE',  ( -8.224510206698735004, -14.34966873604973081, 19.58442372801901143 ) ) ;
#96681=CARTESIAN_POINT ( 'NONE',  ( 5.719274019375991003, -21.55341960407610458, 87.70724293864769550 ) ) ;
#96682=CARTESIAN_POINT ( 'NONE',  ( -16.46253265017146816, -9.564922557961047289, 54.16775706135234003 ) ) ;
#96683=CARTESIAN_POINT ( 'NONE',  ( -16.53943276465976808, -0.05219959533934237506, 78.75109039468568994 ) ) ;
#96684=CARTESIAN_POINT ( 'NONE',  ( -13.97604488694527625, -13.89961937509977652, 71.87390960531433848 ) ) ;
#96685=CARTESIAN_POINT ( 'NONE',  ( -4.483927247898539470, -16.52544592524342804, 67.29057627198103830 ) ) ;
#96686=CARTESIAN_POINT ( 'NONE',  ( -5.153800228976328057, -19.02544592524343514, 42.29057627198101699 ) ) ;
#96687=CARTESIAN_POINT ( 'NONE',  ( 12.14591786802309770, 12.06949235617756955, 54.37390960531435979 ) ) ;
#96688=CARTESIAN_POINT ( 'NONE',  ( -19.02544592524342804, 5.153800228976336051, 26.04057627198103120 ) ) ;
#96690=CARTESIAN_POINT ( 'NONE',  ( 16.55341960407611168, 4.379528057220329451, 33.95724293864769550 ) ) ;
#96691=CARTESIAN_POINT ( 'NONE',  ( -19.02544592524342804, 5.153800228976336051, 76.04057627198102409 ) ) ;
#96692=CARTESIAN_POINT ( 'NONE',  ( 19.02544592524334988, 5.153800228976608722, 36.45942372801900433 ) ) ;
#96693=CARTESIAN_POINT ( 'NONE',  ( -4.483927247898782831, 16.52544592524335698, 42.70942372801901854 ) ) ;
#96694=CARTESIAN_POINT ( 'NONE',  ( -15.80617190586745835, -15.72974639402198527, 46.87390960531435979 ) ) ;
#96695=CARTESIAN_POINT ( 'NONE',  ( -19.03943276465977164, -0.05219959533935918106, 18.75109039468567218 ) ) ;
#96696=CARTESIAN_POINT ( 'NONE',  ( 13.97604488694527802, 13.89961937509977652, 79.37390960531435269 ) ) ;
#96697=CARTESIAN_POINT ( 'NONE',  ( 19.05341960407611168, 5.049401038298154454, 113.9572429386477097 ) ) ;
#96698=CARTESIAN_POINT ( 'NONE',  ( -5.049401038298153566, 19.05341960407611168, 110.2072429386476671 ) ) ;
#96699=CARTESIAN_POINT ( 'NONE',  ( -18.67979575497193778, 10.72451020669871902, 43.33442372801901143 ) ) ;
#96700=CARTESIAN_POINT ( 'NONE',  ( -16.52544592524342804, 4.483927247898546575, 101.0405762719810383 ) ) ;
#96701=CARTESIAN_POINT ( 'NONE',  ( -18.67979575497178146, -10.72451020669898902, 81.66557627198103830 ) ) ;
#96702=CARTESIAN_POINT ( 'NONE',  ( -13.89961937509977652, 13.97604488694528158, 80.62390960531436690 ) ) ;
#96704=CARTESIAN_POINT ( 'NONE',  ( 5.719274019375673035, 21.55341960407619339, 22.29275706135235069 ) ) ;
#96706=CARTESIAN_POINT ( 'NONE',  ( -5.153800228976328057, -19.02544592524343514, 92.29057627198099567 ) ) ;
#96707=EDGE_CURVE ( 'NONE', #149451, #23056, #61604, .T. ) ;
#96709=CARTESIAN_POINT ( 'NONE',  ( 9.564922557960805705, 16.46253265017160317, 29.58224293864769550 ) ) ;
#96710=CARTESIAN_POINT ( 'NONE',  ( -0.05219959533909027116, -19.03943276465977164, 37.49890960531436690 ) ) ;
#96711=CARTESIAN_POINT ( 'NONE',  ( 19.05341960407617918, -5.049401038297876454, 106.0427570613523471 ) ) ;
#96713=CARTESIAN_POINT ( 'NONE',  ( -0.05219959533910754901, -16.53943276465976808, 107.4989096053143669 ) ) ;
#96714=CARTESIAN_POINT ( 'NONE',  ( -10.72451020669870658, -18.67979575497194134, 89.58442372801901854 ) ) ;
#96715=CARTESIAN_POINT ( 'NONE',  ( -9.474510206698964154, 16.51473224551069663, 65.41557627198102409 ) ) ;
#96716=CARTESIAN_POINT ( 'NONE',  ( 10.72451020669871369, 18.67979575497193778, 27.08442372801901854 ) ) ;
#96717=CARTESIAN_POINT ( 'NONE',  ( -5.823673210054431948, 21.52544592524334988, 27.70942372801901854 ) ) ;
#96719=CARTESIAN_POINT ( 'NONE',  ( 16.51473224551069308, 9.474510206698969483, 89.16557627198103830 ) ) ;
#96721=CARTESIAN_POINT ( 'NONE',  ( 14.34966873604972726, -8.224510206698740333, 30.83442372801902209 ) ) ;
#96722=CARTESIAN_POINT ( 'NONE',  ( -18.62759615963270932, 10.81492255796079327, 45.83224293864769550 ) ) ;
#96723=CARTESIAN_POINT ( 'NONE',  ( 15.80617190586769283, -15.72974639402175789, 80.62609039468567573 ) ) ;
#96724=CARTESIAN_POINT ( 'NONE',  ( -13.89961937509977652, 13.97604488694528158, 115.6239096053143669 ) ) ;
#96725=CARTESIAN_POINT ( 'NONE',  ( 5.153800228976615827, -19.02544592524334988, 95.20942372801897591 ) ) ;
#96726=CARTESIAN_POINT ( 'NONE',  ( -5.153800228976328057, -19.02544592524343514, 57.29057627198103120 ) ) ;
#96727=CARTESIAN_POINT ( 'NONE',  ( -0.05219959533909027116, -19.03943276465977164, 87.49890960531436690 ) ) ;
#96728=CARTESIAN_POINT ( 'NONE',  ( -16.53943276465976808, 0.05219959533911058130, 96.24890960531435269 ) ) ;
#96729=CARTESIAN_POINT ( 'NONE',  ( -8.314922557960811034, -14.29746914071050412, 102.0822429386476955 ) ) ;
#96730=CARTESIAN_POINT ( 'NONE',  ( -18.67979575497178146, -10.72451020669898902, 21.66557627198102409 ) ) ;
#96731=CARTESIAN_POINT ( 'NONE',  ( -8.314922557960811034, -14.29746914071050412, 52.08224293864768839 ) ) ;
#96732=CARTESIAN_POINT ( 'NONE',  ( 13.97604488694527802, 13.89961937509977652, 39.37390960531435269 ) ) ;
#96733=CARTESIAN_POINT ( 'NONE',  ( 0.05219959533937995610, -21.53943276465977519, 70.00109039468568994 ) ) ;
#96734=CARTESIAN_POINT ( 'NONE',  ( -13.97604488694547697, 13.89961937509957934, 88.12609039468563310 ) ) ;
#96735=CARTESIAN_POINT ( 'NONE',  ( -16.55341960407611168, -4.379528057220339221, 66.45724293864768129 ) ) ;
#96736=CARTESIAN_POINT ( 'NONE',  ( -10.72451020669898014, 18.67979575497178502, 110.4155762719810383 ) ) ;
#96737=CARTESIAN_POINT ( 'NONE',  ( -15.80617190586745835, -15.72974639402198527, 46.87390960531435979 ) ) ;
#96738=CARTESIAN_POINT ( 'NONE',  ( 9.564922557960805705, 16.46253265017160317, 109.5822429386476955 ) ) ;
#96740=CARTESIAN_POINT ( 'NONE',  ( -13.97604488694527625, -13.89961937509977652, 71.87390960531433848 ) ) ;
#96741=CARTESIAN_POINT ( 'NONE',  ( -12.06949235617756955, 12.14591786802309770, 40.62390960531435269 ) ) ;
#96742=CARTESIAN_POINT ( 'NONE',  ( -16.52544592524335698, -4.483927247898792601, 108.9594237280190185 ) ) ;
#96743=CARTESIAN_POINT ( 'NONE',  ( 12.06949235617739724, 12.14591786802326823, 81.87609039468568994 ) ) ;
#96744=CARTESIAN_POINT ( 'NONE',  ( 0.05219959533936267826, -19.03943276465977164, 45.00109039468566863 ) ) ;
#96746=CARTESIAN_POINT ( 'NONE',  ( -19.02544592524342804, 5.153800228976336051, 91.04057627198100988 ) ) ;
#96747=CARTESIAN_POINT ( 'NONE',  ( 19.03943276465977164, -0.05219959533909143690, 53.74890960531436690 ) ) ;
#96748=CARTESIAN_POINT ( 'NONE',  ( -4.379528057220328563, 16.55341960407611168, 55.20724293864770260 ) ) ;
#96749=CARTESIAN_POINT ( 'NONE',  ( 13.89961937509977652, -13.97604488694527269, 23.12390960531436335 ) ) ;
#96750=CARTESIAN_POINT ( 'NONE',  ( -10.72451020669898014, 18.67979575497178502, 25.41557627198103120 ) ) ;
#96751=CARTESIAN_POINT ( 'NONE',  ( -0.05219959533907301413, -21.53943276465977519, 47.49890960531435979 ) ) ;
#96752=CARTESIAN_POINT ( 'NONE',  ( -14.34966873604960291, -8.224510206698953496, 86.66557627198102409 ) ) ;
#96753=CARTESIAN_POINT ( 'NONE',  ( 16.52544592524335698, 4.483927247898782831, 41.45942372801901143 ) ) ;
#96754=CARTESIAN_POINT ( 'NONE',  ( 14.34966873604960469, 8.224510206698951720, 74.16557627198102409 ) ) ;
#96756=CARTESIAN_POINT ( 'NONE',  ( -19.05341960407617563, 5.049401038297882671, 83.54275706135233293 ) ) ;
#96757=CARTESIAN_POINT ( 'NONE',  ( 16.51473224551069308, 9.474510206698969483, 114.1655762719810241 ) ) ;
#96761=CARTESIAN_POINT ( 'NONE',  ( 14.34966873604972726, -8.224510206698740333, 25.83442372801901499 ) ) ;
#96762=CARTESIAN_POINT ( 'NONE',  ( -16.52544592524335698, -4.483927247898792601, 108.9594237280190185 ) ) ;
#96763=CARTESIAN_POINT ( 'NONE',  ( -5.153800228976607833, 19.02544592524334988, 72.70942372801900433 ) ) ;
#96764=CARTESIAN_POINT ( 'NONE',  ( -21.53943276465977519, 0.05219959533907696930, 51.24890960531436690 ) ) ;
#96765=CARTESIAN_POINT ( 'NONE',  ( -0.05219959533937732626, 21.53943276465977519, 62.50109039468568284 ) ) ;
#96767=CARTESIAN_POINT ( 'NONE',  ( -8.314922557961024197, 14.29746914071037800, 37.91775706135235424 ) ) ;
#96769=CARTESIAN_POINT ( 'NONE',  ( -0.05219959533909027116, -19.03943276465977164, 82.49890960531436690 ) ) ;
#96771=CARTESIAN_POINT ( 'NONE',  ( -12.14591786802309592, -12.06949235617757132, 101.8739096053143811 ) ) ;
#96773=CARTESIAN_POINT ( 'NONE',  ( -13.89961937509977652, 13.97604488694528158, 105.6239096053143527 ) ) ;
#96775=CARTESIAN_POINT ( 'NONE',  ( -16.53943276465976808, -0.05219959533934237506, 53.75109039468568994 ) ) ;
#96776=CARTESIAN_POINT ( 'NONE',  ( 19.05341960407617918, -5.049401038297876454, 106.0427570613523471 ) ) ;
#96777=CARTESIAN_POINT ( 'NONE',  ( 18.67979575497178502, 10.72451020669898547, 74.16557627198102409 ) ) ;
#96778=CARTESIAN_POINT ( 'NONE',  ( -13.97604488694527625, -13.89961937509977652, 36.87390960531436690 ) ) ;
#96779=CARTESIAN_POINT ( 'NONE',  ( -19.03943276465977164, -0.05219959533935918106, 68.75109039468566152 ) ) ;
#96780=CARTESIAN_POINT ( 'NONE',  ( 18.67979575497178502, 10.72451020669898547, 109.1655762719810383 ) ) ;
#96781=CARTESIAN_POINT ( 'NONE',  ( 5.153800228976335163, 19.02544592524342804, 69.79057627198103830 ) ) ;
#96782=CARTESIAN_POINT ( 'NONE',  ( 5.153800228976335163, 19.02544592524342804, 99.79057627198102409 ) ) ;
#96784=CARTESIAN_POINT ( 'NONE',  ( 4.379528057220092307, 16.55341960407617563, 32.29275706135235424 ) ) ;
#96785=CARTESIAN_POINT ( 'NONE',  ( 21.53943276465977519, -0.05219959533907433946, 108.7489096053143669 ) ) ;
#96786=CARTESIAN_POINT ( 'NONE',  ( -14.34966873604960291, -8.224510206698953496, 106.6655762719810383 ) ) ;
#96787=CARTESIAN_POINT ( 'NONE',  ( 0.05219959533909260263, 19.03943276465977164, 94.99890960531436690 ) ) ;
#96788=CARTESIAN_POINT ( 'NONE',  ( 13.89961937509957401, 13.97604488694547697, 76.87609039468566152 ) ) ;
#96789=CARTESIAN_POINT ( 'NONE',  ( -10.72451020669898014, 18.67979575497178502, 90.41557627198103830 ) ) ;
#96790=CARTESIAN_POINT ( 'NONE',  ( -8.224510206698948167, 14.34966873604960824, 50.41557627198103120 ) ) ;
#96791=CARTESIAN_POINT ( 'NONE',  ( 5.153800228976615827, -19.02544592524334988, 25.20942372801900433 ) ) ;
#96792=CARTESIAN_POINT ( 'NONE',  ( 12.06949235617739724, 12.14591786802326823, 61.87609039468568284 ) ) ;
#96793=CARTESIAN_POINT ( 'NONE',  ( 16.46253265017160672, -9.564922557960803928, 98.33224293864769550 ) ) ;
#96795=CARTESIAN_POINT ( 'NONE',  ( 19.02544592524343514, -5.153800228976328945, 48.54057627198103120 ) ) ;
#96797=CARTESIAN_POINT ( 'NONE',  ( 21.53943276465977519, 0.05219959533937863772, 51.25109039468568994 ) ) ;
#96798=CARTESIAN_POINT ( 'NONE',  ( -10.72451020669870658, -18.67979575497194134, 64.58442372801900433 ) ) ;
#96799=CARTESIAN_POINT ( 'NONE',  ( -16.46253265017160317, 9.564922557960807481, 65.83224293864769550 ) ) ;
#96800=CARTESIAN_POINT ( 'NONE',  ( 15.80617190586769283, -15.72974639402175789, 40.62609039468567573 ) ) ;
#96801=CARTESIAN_POINT ( 'NONE',  ( -13.89961937509957401, -13.97604488694547875, 79.37609039468567573 ) ) ;
#96804=CARTESIAN_POINT ( 'NONE',  ( -9.474510206698964154, 16.51473224551069663, 45.41557627198103120 ) ) ;
#96805=CARTESIAN_POINT ( 'NONE',  ( 16.53943276465976808, 0.05219959533934440121, 91.25109039468568994 ) ) ;
#96806=CARTESIAN_POINT ( 'NONE',  ( 19.03943276465977164, -0.05219959533909143690, 53.74890960531436690 ) ) ;
#96807=CARTESIAN_POINT ( 'NONE',  ( 5.049401038298161559, -19.05341960407611168, 107.7072429386476955 ) ) ;
#96808=CARTESIAN_POINT ( 'NONE',  ( 5.153800228976335163, 19.02544592524342804, 34.79057627198102409 ) ) ;
#96809=CARTESIAN_POINT ( 'NONE',  ( -0.05219959533907301413, -21.53943276465977519, 92.49890960531436690 ) ) ;
#96810=CARTESIAN_POINT ( 'NONE',  ( 16.53943276465976808, 0.05219959533934440121, 76.25109039468568994 ) ) ;
#96812=CARTESIAN_POINT ( 'NONE',  ( 5.049401038297881783, 19.05341960407617563, 37.29275706135232582 ) ) ;
#96813=CARTESIAN_POINT ( 'NONE',  ( 9.474510206698971260, -16.51473224551069308, 72.91557627198102409 ) ) ;
#96814=CARTESIAN_POINT ( 'NONE',  ( -4.379528057220328563, 16.55341960407611168, 50.20724293864769550 ) ) ;
#96815=CARTESIAN_POINT ( 'NONE',  ( 14.29746914071049879, -8.314922557960816363, 78.33224293864770971 ) ) ;
#96816=B_SPLINE_CURVE_WITH_KNOTS ( 'NONE', 3,
 ( #163041, #99357, #69028, #52851, #180239, #179234 ),
 .UNSPECIFIED., .F., .F.,
 ( 4, 2, 4 ),
 ( 3.469446951953614189E-18, 0.0003837532665635135821, 0.0007675065331270236949 ),
 .UNSPECIFIED. ) ;
#96817=CARTESIAN_POINT ( 'NONE',  ( 5.049401038298161559, -19.05341960407611168, 102.7072429386476955 ) ) ;
#96818=CARTESIAN_POINT ( 'NONE',  ( 19.05341960407611168, 5.049401038298154454, 88.95724293864769550 ) ) ;
#96819=CARTESIAN_POINT ( 'NONE',  ( -18.62759615963255300, -10.81492255796106328, 49.16775706135234003 ) ) ;
#96820=CARTESIAN_POINT ( 'NONE',  ( 13.97604488694527802, 13.89961937509977652, 99.37390960531436690 ) ) ;
#96821=CARTESIAN_POINT ( 'NONE',  ( 21.55341960407619695, -5.719274019375665929, 96.04275706135236135 ) ) ;
#96822=CARTESIAN_POINT ( 'NONE',  ( -14.29746914071037622, -8.314922557961029526, 84.16775706135234714 ) ) ;
#96823=CARTESIAN_POINT ( 'NONE',  ( 21.53943276465977519, 0.05219959533937863772, 26.25109039468567573 ) ) ;
#96824=CARTESIAN_POINT ( 'NONE',  ( -9.564922557960796823, -16.46253265017161027, 107.0822429386476955 ) ) ;
#96825=CARTESIAN_POINT ( 'NONE',  ( 21.55341960407610458, 5.719274019375980345, 108.9572429386476955 ) ) ;
#96826=CARTESIAN_POINT ( 'NONE',  ( -16.52544592524342804, 4.483927247898546575, 61.04057627198103120 ) ) ;
#96827=CARTESIAN_POINT ( 'NONE',  ( -9.474510206698964154, 16.51473224551069663, 40.41557627198103120 ) ) ;
#96828=CARTESIAN_POINT ( 'NONE',  ( 8.314922557960818139, 14.29746914071049879, 69.58224293864769550 ) ) ;
#96829=CARTESIAN_POINT ( 'NONE',  ( -18.62759615963270932, 10.81492255796079327, 35.83224293864768839 ) ) ;
#96830=CARTESIAN_POINT ( 'NONE',  ( 0.05219959533936267826, -19.03943276465977164, 25.00109039468566152 ) ) ;
#96831=CARTESIAN_POINT ( 'NONE',  ( 0.05219959533910956823, 16.53943276465976808, 109.9989096053143527 ) ) ;
#96833=CARTESIAN_POINT ( 'NONE',  ( 12.14591786802327356, -12.06949235617739191, 60.62609039468567573 ) ) ;
#96834=CARTESIAN_POINT ( 'NONE',  ( -13.97604488694527625, -13.89961937509977652, 66.87390960531436690 ) ) ;
#96836=CARTESIAN_POINT ( 'NONE',  ( 0.05219959533910956823, 16.53943276465976808, 84.99890960531436690 ) ) ;
#96837=CARTESIAN_POINT ( 'NONE',  ( 21.55341960407610458, 5.719274019375980345, 38.95724293864768839 ) ) ;
#96838=CARTESIAN_POINT ( 'NONE',  ( -16.52544592524335698, -4.483927247898792601, 108.9594237280190185 ) ) ;
#96839=CARTESIAN_POINT ( 'NONE',  ( 19.05341960407617918, -5.049401038297876454, 106.0427570613523471 ) ) ;
#96840=CARTESIAN_POINT ( 'NONE',  ( -21.55341960407619339, 5.719274019375674811, 78.54275706135236135 ) ) ;
#96841=CARTESIAN_POINT ( 'NONE',  ( -5.153800228976328057, -19.02544592524343514, 82.29057627198103830 ) ) ;
#96842=CARTESIAN_POINT ( 'NONE',  ( 21.55341960407610458, 5.719274019375980345, 108.9572429386476955 ) ) ;
#96843=CARTESIAN_POINT ( 'NONE',  ( -4.379528057220086978, -16.55341960407618274, 49.79275706135234714 ) ) ;
#96844=CARTESIAN_POINT ( 'NONE',  ( -19.02544592524342804, 5.153800228976336051, 26.04057627198103120 ) ) ;
#96845=CARTESIAN_POINT ( 'NONE',  ( 8.314922557961029526, -14.29746914071037800, 25.41775706135235779 ) ) ;
#96846=CARTESIAN_POINT ( 'NONE',  ( -16.51473224551082808, 9.474510206698731452, 93.33442372801900433 ) ) ;
#96847=CARTESIAN_POINT ( 'NONE',  ( -21.55341960407610458, -5.719274019375992779, 96.45724293864770971 ) ) ;
#96848=CARTESIAN_POINT ( 'NONE',  ( 16.51473224551083163, -9.474510206698727899, 55.83442372801899722 ) ) ;
#96849=CARTESIAN_POINT ( 'NONE',  ( 19.35633801406910592, -5.499999999999574563, 86.63373818172766505 ) ) ;
#96850=CARTESIAN_POINT ( 'NONE',  ( 18.67979575497178502, 10.72451020669898547, 99.16557627198100988 ) ) ;
#96851=CARTESIAN_POINT ( 'NONE',  ( 18.22780087662126647, 5.499999999999818812, 61.48236817873107185 ) ) ;
#96852=CARTESIAN_POINT ( 'NONE',  ( 16.46253265017160672, -9.564922557960803928, 83.33224293864768129 ) ) ;
#96854=CARTESIAN_POINT ( 'NONE',  ( 8.224510206698742110, 14.34966873604972548, 37.08442372801901143 ) ) ;
#96856=CARTESIAN_POINT ( 'NONE',  ( -21.52544592524343514, 5.823673210054127303, 111.0405762719810525 ) ) ;
#96857=CARTESIAN_POINT ( 'NONE',  ( 12.06949235617757843, -12.14591786802309237, 63.12390960531435979 ) ) ;
#96858=CARTESIAN_POINT ( 'NONE',  ( 0.05219959533909260263, 19.03943276465977164, 64.99890960531436690 ) ) ;
#96859=CARTESIAN_POINT ( 'NONE',  ( 8.224510206698742110, 14.34966873604972548, 37.08442372801901143 ) ) ;
#96860=CARTESIAN_POINT ( 'NONE',  ( -16.46253265017146816, -9.564922557961047289, 44.16775706135232582 ) ) ;
#96861=CARTESIAN_POINT ( 'NONE',  ( -21.55341960407619339, 5.719274019375674811, 53.54275706135234714 ) ) ;
#96862=CARTESIAN_POINT ( 'NONE',  ( 13.97604488694548053, -13.89961937509957401, 110.6260903946856615 ) ) ;
#96863=CARTESIAN_POINT ( 'NONE',  ( 13.97604488694527802, 13.89961937509977652, 54.37390960531435979 ) ) ;
#96864=CARTESIAN_POINT ( 'NONE',  ( -13.89961937509957401, -13.97604488694547875, 79.37609039468567573 ) ) ;
#96865=CARTESIAN_POINT ( 'NONE',  ( -15.72974639402176322, -15.80617190586768395, 89.37609039468568994 ) ) ;
#96866=CARTESIAN_POINT ( 'NONE',  ( -5.153800228976607833, 19.02544592524334988, 72.70942372801900433 ) ) ;
#96867=CARTESIAN_POINT ( 'NONE',  ( -9.564922557960796823, -16.46253265017161027, 42.08224293864769550 ) ) ;
#96868=CARTESIAN_POINT ( 'NONE',  ( 18.67979575497178502, 10.72451020669898547, 54.16557627198103120 ) ) ;
#96869=CARTESIAN_POINT ( 'NONE',  ( 16.53943276465976808, -0.05219959533910856209, 58.74890960531436690 ) ) ;
#96870=CARTESIAN_POINT ( 'NONE',  ( -18.22780087662122028, -5.500000000000014211, 101.4845989467389273 ) ) ;
#96871=CARTESIAN_POINT ( 'NONE',  ( -19.03943276465977164, -0.05219959533935918106, 33.75109039468566863 ) ) ;
#96872=CARTESIAN_POINT ( 'NONE',  ( -14.29746914071037622, -8.314922557961029526, 104.1677570613523471 ) ) ;
#96873=CARTESIAN_POINT ( 'NONE',  ( -12.14591786802309592, -12.06949235617757132, 51.87390960531437401 ) ) ;
#96874=CARTESIAN_POINT ( 'NONE',  ( -18.67979575497193778, 10.72451020669871902, 93.33442372801901854 ) ) ;
#96876=CARTESIAN_POINT ( 'NONE',  ( 15.72974639402176855, 15.80617190586768217, 91.87609039468568994 ) ) ;
#96877=CARTESIAN_POINT ( 'NONE',  ( 21.52544592524344225, -5.823673210054117533, 88.54057627198103830 ) ) ;
#96878=CARTESIAN_POINT ( 'NONE',  ( -13.89961937509977652, 13.97604488694528158, 55.62390960531434558 ) ) ;
#96879=CARTESIAN_POINT ( 'NONE',  ( -18.62759615963255300, -10.81492255796106328, 74.16775706135231871 ) ) ;
#96880=CARTESIAN_POINT ( 'NONE',  ( -19.05341960407611168, -5.049401038298163336, 46.45724293864768129 ) ) ;
#96882=CARTESIAN_POINT ( 'NONE',  ( -5.153800228976328057, -19.02544592524343514, 62.29057627198100988 ) ) ;
#96883=CARTESIAN_POINT ( 'NONE',  ( 16.55341960407611168, 4.379528057220329451, 103.9572429386476813 ) ) ;
#96884=CARTESIAN_POINT ( 'NONE',  ( -15.80617190586745835, -15.72974639402198527, 21.87390960531436690 ) ) ;
#96885=CARTESIAN_POINT ( 'NONE',  ( 16.55341960407611168, 4.379528057220329451, 58.95724293864770971 ) ) ;
#96886=CARTESIAN_POINT ( 'NONE',  ( -19.02544592524342804, 5.153800228976336051, 26.04057627198103120 ) ) ;
#96887=CARTESIAN_POINT ( 'NONE',  ( -0.05219959533910754901, -16.53943276465976808, 77.49890960531433848 ) ) ;
#96888=CARTESIAN_POINT ( 'NONE',  ( 18.62759615963271287, -10.81492255796078972, 88.33224293864769550 ) ) ;
#96889=CARTESIAN_POINT ( 'NONE',  ( -15.72974639402176322, -15.80617190586768395, 34.37609039468568284 ) ) ;
#96891=CARTESIAN_POINT ( 'NONE',  ( 16.53943276465976808, 0.05219959533934440121, 31.25109039468568639 ) ) ;
#96892=CARTESIAN_POINT ( 'NONE',  ( 10.81492255796078972, 18.62759615963270932, 84.58224293864769550 ) ) ;
#96893=CARTESIAN_POINT ( 'NONE',  ( 21.55341960407619695, -5.719274019375665929, 106.0427570613523471 ) ) ;
#96894=CARTESIAN_POINT ( 'NONE',  ( -16.46253265017160317, 9.564922557960807481, 95.83224293864769550 ) ) ;
#96895=CARTESIAN_POINT ( 'NONE',  ( 15.72974639402176855, 15.80617190586768217, 41.87609039468568284 ) ) ;
#96896=CARTESIAN_POINT ( 'NONE',  ( 21.55341960407610458, 5.719274019375980345, 23.95724293864769550 ) ) ;
#96897=CARTESIAN_POINT ( 'NONE',  ( 16.52544592524335698, 4.483927247898782831, 106.4594237280190328 ) ) ;
#96898=CARTESIAN_POINT ( 'NONE',  ( -15.72974639402176322, -15.80617190586768395, 44.37609039468567573 ) ) ;
#96899=CARTESIAN_POINT ( 'NONE',  ( 5.719274019375673035, 21.55341960407619339, 87.29275706135236135 ) ) ;
#96900=CARTESIAN_POINT ( 'NONE',  ( 19.03943276465977164, 0.05219959533936151252, 21.25109039468565797 ) ) ;
#96901=CARTESIAN_POINT ( 'NONE',  ( -12.14591786802326823, 12.06949235617739902, 83.12609039468568994 ) ) ;
#96902=CARTESIAN_POINT ( 'NONE',  ( -15.80617190586768217, 15.72974639402176855, 48.12609039468568284 ) ) ;
#96903=CARTESIAN_POINT ( 'NONE',  ( 5.153800228976335163, 19.02544592524342804, 34.79057627198102409 ) ) ;
#96904=CARTESIAN_POINT ( 'NONE',  ( 10.72451020669871369, 18.67979575497193778, 107.0844237280190043 ) ) ;
#96905=CARTESIAN_POINT ( 'NONE',  ( -9.564922557960796823, -16.46253265017161027, 107.0822429386476955 ) ) ;
#96906=CARTESIAN_POINT ( 'NONE',  ( -10.81492255796078084, -18.62759615963271287, 97.08224293864770971 ) ) ;
#96908=CARTESIAN_POINT ( 'NONE',  ( 19.39056639909674118, 5.500000000000051514, 83.28948781074343799 ) ) ;
#96909=CARTESIAN_POINT ( 'NONE',  ( -18.67979575497178146, -10.72451020669898902, 66.66557627198102409 ) ) ;
#96910=CARTESIAN_POINT ( 'NONE',  ( -4.483927247898782831, 16.52544592524335698, 57.70942372801901143 ) ) ;
#96911=CARTESIAN_POINT ( 'NONE',  ( 16.55341960407611168, 4.379528057220329451, 63.95724293864770260 ) ) ;
#96912=CARTESIAN_POINT ( 'NONE',  ( 19.08440550902509258, -5.500000000000005329, 101.3294784629314762 ) ) ;
#96913=CARTESIAN_POINT ( 'NONE',  ( -16.51473224551082808, 9.474510206698731452, 93.33442372801900433 ) ) ;
#96916=CARTESIAN_POINT ( 'NONE',  ( 16.55341960407618274, -4.379528057220086978, 26.04275706135235779 ) ) ;
#96917=CARTESIAN_POINT ( 'NONE',  ( -15.80617190586745835, -15.72974639402198527, 91.87390960531436690 ) ) ;
#96918=CARTESIAN_POINT ( 'NONE',  ( 5.719274019375991003, -21.55341960407610458, 72.70724293864769550 ) ) ;
#96919=CARTESIAN_POINT ( 'NONE',  ( 5.049401038298161559, -19.05341960407611168, 112.7072429386476813 ) ) ;
#96920=CARTESIAN_POINT ( 'NONE',  ( -16.52544592524335698, -4.483927247898792601, 48.95942372801902565 ) ) ;
#96921=CARTESIAN_POINT ( 'NONE',  ( -0.05219959533909027116, -19.03943276465977164, 72.49890960531435269 ) ) ;
#96922=CARTESIAN_POINT ( 'NONE',  ( -21.52544592524334988, -5.823673210054445271, 33.95942372801901143 ) ) ;
#96923=CARTESIAN_POINT ( 'NONE',  ( -16.46253265017146816, -9.564922557961047289, 99.16775706135233293 ) ) ;
#96924=CARTESIAN_POINT ( 'NONE',  ( 13.97604488694527802, 13.89961937509977652, 114.3739096053143669 ) ) ;
#96925=CARTESIAN_POINT ( 'NONE',  ( -19.02544592524342804, 5.153800228976336051, 86.04057627198103830 ) ) ;
#96926=CARTESIAN_POINT ( 'NONE',  ( 18.62759615963271287, -10.81492255796078972, 83.33224293864769550 ) ) ;
#96927=CARTESIAN_POINT ( 'NONE',  ( -9.474510206698964154, 16.51473224551069663, 60.41557627198102409 ) ) ;
#96929=CARTESIAN_POINT ( 'NONE',  ( 8.224510206698953496, -14.34966873604960469, 62.91557627198102409 ) ) ;
#96930=CARTESIAN_POINT ( 'NONE',  ( -18.67979575497178146, -10.72451020669898902, 26.66557627198103475 ) ) ;
#96932=CARTESIAN_POINT ( 'NONE',  ( 18.67979575497178502, 10.72451020669898547, 99.16557627198100988 ) ) ;
#96933=CARTESIAN_POINT ( 'NONE',  ( -19.05341960407617563, 5.049401038297882671, 58.54275706135234003 ) ) ;
#96934=CARTESIAN_POINT ( 'NONE',  ( -13.97604488694527625, -13.89961937509977652, 111.8739096053143243 ) ) ;
#96935=CARTESIAN_POINT ( 'NONE',  ( 19.01529144963336648, 5.499999999999972466, 68.73431955728435128 ) ) ;
#96936=CARTESIAN_POINT ( 'NONE',  ( -18.67979575497178146, -10.72451020669898902, 61.66557627198103120 ) ) ;
#96938=CARTESIAN_POINT ( 'NONE',  ( 0.05219959533909260263, 19.03943276465977164, 84.99890960531436690 ) ) ;
#96939=CARTESIAN_POINT ( 'NONE',  ( 18.67979575497194134, -10.72451020669871369, 80.83442372801901854 ) ) ;
#96940=CARTESIAN_POINT ( 'NONE',  ( -16.46253265017160317, 9.564922557960807481, 50.83224293864770260 ) ) ;
#96941=CARTESIAN_POINT ( 'NONE',  ( 8.314922557960818139, 14.29746914071049879, 84.58224293864769550 ) ) ;
#96942=CARTESIAN_POINT ( 'NONE',  ( -16.55341960407617563, 4.379528057220093196, 33.54275706135234714 ) ) ;
#96943=CARTESIAN_POINT ( 'NONE',  ( 15.72974639402176855, 15.80617190586768217, 71.87609039468568994 ) ) ;
#96945=CARTESIAN_POINT ( 'NONE',  ( 16.51473224551083163, -9.474510206698727899, 20.83442372801899722 ) ) ;
#96946=CARTESIAN_POINT ( 'NONE',  ( -19.02544592524334988, -5.153800228976617603, 78.95942372801900433 ) ) ;
#96949=CARTESIAN_POINT ( 'NONE',  ( 5.719274019375673035, 21.55341960407619339, 32.29275706135235424 ) ) ;
#96951=CARTESIAN_POINT ( 'NONE',  ( -19.05341960407617563, 5.049401038297882671, 33.54275706135231871 ) ) ;
#96952=CARTESIAN_POINT ( 'NONE',  ( 19.03943276465977164, -0.05219959533909143690, 58.74890960531435979 ) ) ;
#96953=CARTESIAN_POINT ( 'NONE',  ( -9.474510206698720793, -16.51473224551083518, 24.58442372801900078 ) ) ;
#96954=CARTESIAN_POINT ( 'NONE',  ( -4.379528057220086978, -16.55341960407618274, 104.7927570613523898 ) ) ;
#96955=CARTESIAN_POINT ( 'NONE',  ( 13.89961937509977652, -13.97604488694527269, 98.12390960531433848 ) ) ;
#96956=CARTESIAN_POINT ( 'NONE',  ( 5.719274019375673035, 21.55341960407619339, 87.29275706135236135 ) ) ;
#96958=CARTESIAN_POINT ( 'NONE',  ( -17.49999999999999645, 5.499999999999992895, 98.71769037696435589 ) ) ;
#96959=CARTESIAN_POINT ( 'NONE',  ( -21.53943276465977519, -0.05219959533937600094, 83.75109039468568994 ) ) ;
#96961=CARTESIAN_POINT ( 'NONE',  ( -9.564922557960796823, -16.46253265017161027, 102.0822429386477097 ) ) ;
#96963=CARTESIAN_POINT ( 'NONE',  ( -0.05219959533909027116, -19.03943276465977164, 52.49890960531436690 ) ) ;
#96964=CARTESIAN_POINT ( 'NONE',  ( 5.823673210054125526, 21.52544592524343514, 59.79057627198103120 ) ) ;
#96965=CARTESIAN_POINT ( 'NONE',  ( 4.379528057220339221, -16.55341960407611168, 32.70724293864770260 ) ) ;
#96966=CARTESIAN_POINT ( 'NONE',  ( -12.14591786802309592, -12.06949235617757132, 101.8739096053143811 ) ) ;
#96967=CARTESIAN_POINT ( 'NONE',  ( -19.02544592524342804, 5.153800228976336051, 76.04057627198102409 ) ) ;
#96968=CARTESIAN_POINT ( 'NONE',  ( 18.62759615963255655, 10.81492255796105972, 111.6677570613523613 ) ) ;
#96969=CARTESIAN_POINT ( 'NONE',  ( -9.474510206698964154, 16.51473224551069663, 40.41557627198103120 ) ) ;
#96970=CARTESIAN_POINT ( 'NONE',  ( 8.314922557960818139, 14.29746914071049879, 104.5822429386477097 ) ) ;
#96971=CARTESIAN_POINT ( 'NONE',  ( 5.719274019375673035, 21.55341960407619339, 57.29275706135234714 ) ) ;
#96972=CARTESIAN_POINT ( 'NONE',  ( -21.53943276465977519, 0.05219959533907696930, 81.24890960531436690 ) ) ;
#96973=CARTESIAN_POINT ( 'NONE',  ( 19.05341960407617918, -5.049401038297876454, 66.04275706135233293 ) ) ;
#96975=CARTESIAN_POINT ( 'NONE',  ( 9.564922557960805705, 16.46253265017160317, 109.5822429386476955 ) ) ;
#96976=CARTESIAN_POINT ( 'NONE',  ( -4.483927247898539470, -16.52544592524342804, 77.29057627198102409 ) ) ;
#96977=CARTESIAN_POINT ( 'NONE',  ( 19.02544592524334988, 5.153800228976608722, 41.45942372801900433 ) ) ;
#96978=CARTESIAN_POINT ( 'NONE',  ( 16.51473224551069308, 9.474510206698969483, 64.16557627198102409 ) ) ;
#96979=CARTESIAN_POINT ( 'NONE',  ( -8.224510206698948167, 14.34966873604960824, 60.41557627198102409 ) ) ;
#96980=CARTESIAN_POINT ( 'NONE',  ( -5.049401038297874678, -19.05341960407617918, 74.79275706135231871 ) ) ;
#96982=CARTESIAN_POINT ( 'NONE',  ( -21.52544592524343514, 5.823673210054127303, 31.04057627198102409 ) ) ;
#96983=ORIENTED_EDGE ( 'NONE', *, *, #177098, .F. ) ;
#96984=CARTESIAN_POINT ( 'NONE',  ( 16.55341960407611168, 4.379528057220329451, 98.95724293864770971 ) ) ;
#96985=CARTESIAN_POINT ( 'NONE',  ( -17.49999999999997158, -3.512728167237161081, 24.77190004818871572 ) ) ;
#96986=CARTESIAN_POINT ( 'NONE',  ( 13.89961937509977652, -13.97604488694527269, 53.12390960531434558 ) ) ;
#96987=CARTESIAN_POINT ( 'NONE',  ( -18.67979575497178146, -10.72451020669898902, 56.66557627198103830 ) ) ;
#96988=CARTESIAN_POINT ( 'NONE',  ( -0.05219959533909027116, -19.03943276465977164, 37.49890960531436690 ) ) ;
#96989=CARTESIAN_POINT ( 'NONE',  ( -16.52544592524335698, -4.483927247898792601, 83.95942372801900433 ) ) ;
#96990=CARTESIAN_POINT ( 'NONE',  ( 16.51473224551069308, 9.474510206698969483, 79.16557627198103830 ) ) ;
#96991=CARTESIAN_POINT ( 'NONE',  ( -13.97604488694547697, 13.89961937509957934, 58.12609039468566863 ) ) ;
#96992=CARTESIAN_POINT ( 'NONE',  ( 5.719274019375673035, 21.55341960407619339, 67.29275706135234714 ) ) ;
#96993=CARTESIAN_POINT ( 'NONE',  ( -10.81492255796078084, -18.62759615963271287, 52.08224293864768839 ) ) ;
#96994=CARTESIAN_POINT ( 'NONE',  ( -16.53943276465976808, 0.05219959533911058130, 116.2489096053143669 ) ) ;
#96995=CARTESIAN_POINT ( 'NONE',  ( -16.55341960407617563, 4.379528057220093196, 93.54275706135234714 ) ) ;
#96996=CARTESIAN_POINT ( 'NONE',  ( -19.03943276465977164, -0.05219959533935918106, 103.7510903946856757 ) ) ;
#96997=CARTESIAN_POINT ( 'NONE',  ( 18.22780087662123805, -5.499999999999976019, 78.51763182126894947 ) ) ;
#96998=CARTESIAN_POINT ( 'NONE',  ( 18.56399227203342406, 5.500000000000001776, 76.47830131249902763 ) ) ;
#96999=CARTESIAN_POINT ( 'NONE',  ( 5.823673210054444382, -21.52544592524334988, 95.20942372801903275 ) ) ;
#97001=CARTESIAN_POINT ( 'NONE',  ( -16.55341960407611168, -4.379528057220339221, 41.45724293864769550 ) ) ;
#97002=CARTESIAN_POINT ( 'NONE',  ( -4.379528057220328563, 16.55341960407611168, 75.20724293864769550 ) ) ;
#97003=CARTESIAN_POINT ( 'NONE',  ( -10.72451020669898014, 18.67979575497178502, 95.41557627198102409 ) ) ;
#97004=CARTESIAN_POINT ( 'NONE',  ( 10.81492255796078972, 18.62759615963270932, 89.58224293864768129 ) ) ;
#97006=CARTESIAN_POINT ( 'NONE',  ( -21.53943276465977519, 0.05219959533907696930, 31.24890960531435979 ) ) ;
#97007=CARTESIAN_POINT ( 'NONE',  ( 4.379528057220092307, 16.55341960407617563, 72.29275706135236135 ) ) ;
#97008=CARTESIAN_POINT ( 'NONE',  ( -16.55341960407611168, -4.379528057220339221, 81.45724293864769550 ) ) ;
#97009=CARTESIAN_POINT ( 'NONE',  ( 9.564922557960805705, 16.46253265017160317, 44.58224293864769550 ) ) ;
#97012=CARTESIAN_POINT ( 'NONE',  ( 0.05219959533934541429, -16.53943276465976808, 95.00109039468568994 ) ) ;
#97013=CARTESIAN_POINT ( 'NONE',  ( 5.719274019375991003, -21.55341960407610458, 112.7072429386476955 ) ) ;
#97014=CARTESIAN_POINT ( 'NONE',  ( 19.05341960407611168, 5.049401038298154454, 83.95724293864766707 ) ) ;
#97015=CARTESIAN_POINT ( 'NONE',  ( -0.05219959533937732626, 21.53943276465977519, 57.50109039468568994 ) ) ;
#97016=CARTESIAN_POINT ( 'NONE',  ( -19.02544592524342804, 5.153800228976336051, 106.0405762719810241 ) ) ;
#97019=CARTESIAN_POINT ( 'NONE',  ( -21.52544592524334988, -5.823673210054445271, 53.95942372801900433 ) ) ;
#97020=CARTESIAN_POINT ( 'NONE',  ( -5.153800228976328057, -19.02544592524343514, 37.29057627198102409 ) ) ;
#97021=CARTESIAN_POINT ( 'NONE',  ( 9.564922557960805705, 16.46253265017160317, 24.58224293864769194 ) ) ;
#97022=CARTESIAN_POINT ( 'NONE',  ( 0.05219959533936267826, -19.03943276465977164, 70.00109039468566152 ) ) ;
#97023=CARTESIAN_POINT ( 'NONE',  ( -18.62759615963255300, -10.81492255796106328, 24.16775706135235424 ) ) ;
#97024=CARTESIAN_POINT ( 'NONE',  ( -9.474510206698720793, -16.51473224551083518, 59.58442372801900433 ) ) ;
#97025=CARTESIAN_POINT ( 'NONE',  ( 19.05341960407611168, 5.049401038298154454, 28.95724293864769550 ) ) ;
#97026=CARTESIAN_POINT ( 'NONE',  ( -8.314922557961024197, 14.29746914071037800, 87.91775706135234714 ) ) ;
#97027=CARTESIAN_POINT ( 'NONE',  ( -5.153800228976607833, 19.02544592524334988, 62.70942372801899722 ) ) ;
#97028=CARTESIAN_POINT ( 'NONE',  ( 8.224510206698742110, 14.34966873604972548, 112.0844237280190185 ) ) ;
#97030=CARTESIAN_POINT ( 'NONE',  ( -13.89961937509977652, 13.97604488694528158, 80.62390960531436690 ) ) ;
#97031=CARTESIAN_POINT ( 'NONE',  ( -21.52544592524334988, -5.823673210054445271, 88.95942372801901854 ) ) ;
#97032=CARTESIAN_POINT ( 'NONE',  ( 18.62759615963255655, 10.81492255796105972, 106.6677570613523756 ) ) ;
#97034=CARTESIAN_POINT ( 'NONE',  ( -15.80617190586768217, 15.72974639402176855, 73.12609039468567573 ) ) ;
#97035=CARTESIAN_POINT ( 'NONE',  ( 14.29746914071037800, 8.314922557961029526, 31.66775706135234358 ) ) ;
#97037=CARTESIAN_POINT ( 'NONE',  ( 13.97604488694527802, 13.89961937509977652, 74.37390960531436690 ) ) ;
#97038=CARTESIAN_POINT ( 'NONE',  ( -21.55341960407610458, -5.719274019375992779, 36.45724293864768839 ) ) ;
#97039=CARTESIAN_POINT ( 'NONE',  ( -19.02544592524342804, 5.153800228976336051, 81.04057627198103830 ) ) ;
#97040=CARTESIAN_POINT ( 'NONE',  ( -18.22780087662121673, -5.500000000000063061, 41.48459894673893444 ) ) ;
#97041=CARTESIAN_POINT ( 'NONE',  ( 19.05341960407617918, -5.049401038297876454, 76.04275706135230450 ) ) ;
#97042=CARTESIAN_POINT ( 'NONE',  ( -19.05341960407611168, -5.049401038298163336, 106.4572429386476955 ) ) ;
#97043=CARTESIAN_POINT ( 'NONE',  ( -15.72974639402176322, -15.80617190586768395, 99.37609039468568994 ) ) ;
#97044=CARTESIAN_POINT ( 'NONE',  ( -16.55341960407611168, -4.379528057220339221, 81.45724293864769550 ) ) ;
#97045=CARTESIAN_POINT ( 'NONE',  ( -21.52544592524343514, 5.823673210054127303, 51.04057627198103120 ) ) ;
#97046=CARTESIAN_POINT ( 'NONE',  ( -21.52544592524343514, 5.823673210054127303, 36.04057627198102409 ) ) ;
#97047=CARTESIAN_POINT ( 'NONE',  ( -8.224510206698948167, 14.34966873604960824, 100.4155762719810241 ) ) ;
#97049=CARTESIAN_POINT ( 'NONE',  ( 5.153800228976615827, -19.02544592524334988, 60.20942372801899012 ) ) ;
#97050=CARTESIAN_POINT ( 'NONE',  ( -14.34966873604960291, -8.224510206698953496, 31.66557627198102054 ) ) ;
#97051=CARTESIAN_POINT ( 'NONE',  ( -19.03943276465977164, 0.05219959533909376836, 96.24890960531436690 ) ) ;
#97052=CARTESIAN_POINT ( 'NONE',  ( -15.80617190586768217, 15.72974639402176855, 73.12609039468567573 ) ) ;
#97053=CARTESIAN_POINT ( 'NONE',  ( 18.67979575497178502, 10.72451020669898547, 64.16557627198102409 ) ) ;
#97054=CARTESIAN_POINT ( 'NONE',  ( 21.52544592524334988, 5.823673210054432836, 51.45942372801901854 ) ) ;
#97055=CARTESIAN_POINT ( 'NONE',  ( -21.55341960407610458, -5.719274019375992779, 96.45724293864770971 ) ) ;
#97056=CARTESIAN_POINT ( 'NONE',  ( -18.62759615963255300, -10.81492255796106328, 39.16775706135235424 ) ) ;
#97057=CARTESIAN_POINT ( 'NONE',  ( -4.379528057220328563, 16.55341960407611168, 115.2072429386476955 ) ) ;
#97059=CARTESIAN_POINT ( 'NONE',  ( -16.46253265017160317, 9.564922557960807481, 85.83224293864769550 ) ) ;
#97060=CARTESIAN_POINT ( 'NONE',  ( 0.05219959533910956823, 16.53943276465976808, 99.99890960531436690 ) ) ;
#97061=CARTESIAN_POINT ( 'NONE',  ( -19.05341960407611168, -5.049401038298163336, 111.4572429386476671 ) ) ;
#97062=CARTESIAN_POINT ( 'NONE',  ( 16.52544592524342804, -4.483927247898539470, 58.54057627198103120 ) ) ;
#97063=CARTESIAN_POINT ( 'NONE',  ( -4.483927247898782831, 16.52544592524335698, 112.7094237280190328 ) ) ;
#97064=CARTESIAN_POINT ( 'NONE',  ( -13.97604488694527625, -13.89961937509977652, 46.87390960531435979 ) ) ;
#97065=CARTESIAN_POINT ( 'NONE',  ( 16.55341960407611168, 4.379528057220329451, 113.9572429386477239 ) ) ;
#97066=CARTESIAN_POINT ( 'NONE',  ( -18.62759615963270932, 10.81492255796079327, 45.83224293864769550 ) ) ;
#97067=CARTESIAN_POINT ( 'NONE',  ( -16.51473224551082808, 9.474510206698731452, 23.33442372801900078 ) ) ;
#97068=CARTESIAN_POINT ( 'NONE',  ( -18.09918380851993902, -5.499999999999988454, 86.48618307335611632 ) ) ;
#97069=CARTESIAN_POINT ( 'NONE',  ( -4.483927247898539470, -16.52544592524342804, 37.29057627198102409 ) ) ;
#97071=CARTESIAN_POINT ( 'NONE',  ( -18.67979575497193778, 10.72451020669871902, 43.33442372801901143 ) ) ;
#97072=DIRECTION ( 'NONE',  ( -1.000000000000000000, 0.000000000000000000, 0.000000000000000000 ) ) ;
#97073=CARTESIAN_POINT ( 'NONE',  ( -0.05219959533934338120, 16.53943276465976808, 62.50109039468568284 ) ) ;
#97074=CARTESIAN_POINT ( 'NONE',  ( -16.51473224551082808, 9.474510206698731452, 68.33442372801900433 ) ) ;
#97075=CARTESIAN_POINT ( 'NONE',  ( -14.34966873604960291, -8.224510206698953496, 26.66557627198103475 ) ) ;
#97076=CARTESIAN_POINT ( 'NONE',  ( -16.55341960407617563, 4.379528057220093196, 108.5427570613523756 ) ) ;
#97077=CARTESIAN_POINT ( 'NONE',  ( 13.97604488694527802, 13.89961937509977652, 34.37390960531436690 ) ) ;
#97078=CARTESIAN_POINT ( 'NONE',  ( 13.97604488694527802, 13.89961937509977652, 59.37390960531434558 ) ) ;
#97079=CARTESIAN_POINT ( 'NONE',  ( -16.46253265017160317, 9.564922557960807481, 30.83224293864769550 ) ) ;
#97080=CARTESIAN_POINT ( 'NONE',  ( -18.62759615963255300, -10.81492255796106328, 39.16775706135235424 ) ) ;
#97081=CARTESIAN_POINT ( 'NONE',  ( -9.564922557960796823, -16.46253265017161027, 47.08224293864769550 ) ) ;
#97083=CARTESIAN_POINT ( 'NONE',  ( -16.51473224551069308, -9.474510206698971260, 36.66557627198102409 ) ) ;
#97084=CARTESIAN_POINT ( 'NONE',  ( 0.05219959533907565091, 21.53943276465977519, 24.99890960531435624 ) ) ;
#97085=CARTESIAN_POINT ( 'NONE',  ( 21.53943276465977519, 0.05219959533937863772, 56.25109039468568284 ) ) ;
#97086=CARTESIAN_POINT ( 'NONE',  ( -8.314922557960811034, -14.29746914071050412, 107.0822429386476955 ) ) ;
#97087=CARTESIAN_POINT ( 'NONE',  ( -13.89961937509977652, 13.97604488694528158, 105.6239096053143527 ) ) ;
#97088=CARTESIAN_POINT ( 'NONE',  ( -4.483927247898782831, 16.52544592524335698, 77.70942372801900433 ) ) ;
#97089=CARTESIAN_POINT ( 'NONE',  ( -18.67979575497193778, 10.72451020669871902, 88.33442372801901854 ) ) ;
#97090=CARTESIAN_POINT ( 'NONE',  ( -8.224510206698735004, -14.34966873604973081, 54.58442372801901143 ) ) ;
#97091=CARTESIAN_POINT ( 'NONE',  ( -19.02544592524342804, 5.153800228976336051, 96.04057627198103830 ) ) ;
#97092=CARTESIAN_POINT ( 'NONE',  ( 14.29746914071037800, 8.314922557961029526, 46.66775706135234714 ) ) ;
#97093=CARTESIAN_POINT ( 'NONE',  ( -8.314922557961024197, 14.29746914071037800, 22.91775706135235069 ) ) ;
#97094=CARTESIAN_POINT ( 'NONE',  ( -12.14591786802326823, 12.06949235617739902, 83.12609039468568994 ) ) ;
#97095=CARTESIAN_POINT ( 'NONE',  ( 19.03943276465977164, 0.05219959533936151252, 106.2510903946856615 ) ) ;
#97096=CARTESIAN_POINT ( 'NONE',  ( -21.53943276465977519, 0.05219959533907696930, 101.2489096053143669 ) ) ;
#97097=CARTESIAN_POINT ( 'NONE',  ( 8.224510206698953496, -14.34966873604960469, 102.9155762719810383 ) ) ;
#97098=CARTESIAN_POINT ( 'NONE',  ( -5.049401038297874678, -19.05341960407617918, 104.7927570613523471 ) ) ;
#97099=CARTESIAN_POINT ( 'NONE',  ( 14.29746914071037800, 8.314922557961029526, 66.66775706135234714 ) ) ;
#97100=CARTESIAN_POINT ( 'NONE',  ( -16.36317988757095421, 7.306389748694863684, 44.09789608363175972 ) ) ;
#97101=CARTESIAN_POINT ( 'NONE',  ( -13.89961937509957401, -13.97604488694547875, 64.37609039468567573 ) ) ;
#97102=CARTESIAN_POINT ( 'NONE',  ( -12.14591786802309592, -12.06949235617757132, 51.87390960531437401 ) ) ;
#97103=CARTESIAN_POINT ( 'NONE',  ( 14.29746914071049879, -8.314922557960816363, 33.33224293864769550 ) ) ;
#97104=CARTESIAN_POINT ( 'NONE',  ( 8.224510206698953496, -14.34966873604960469, 87.91557627198103830 ) ) ;
#97105=CARTESIAN_POINT ( 'NONE',  ( 16.46253265017146816, 9.564922557961045513, 36.66775706135233293 ) ) ;
#97106=CARTESIAN_POINT ( 'NONE',  ( -17.31747979337945154, 6.344076630961115626, 88.62055131934820906 ) ) ;
#97107=CARTESIAN_POINT ( 'NONE',  ( 10.72451020669871369, 18.67979575497193778, 42.08442372801901854 ) ) ;
#97108=CARTESIAN_POINT ( 'NONE',  ( 13.97604488694548053, -13.89961937509957401, 100.6260903946856615 ) ) ;
#97109=CARTESIAN_POINT ( 'NONE',  ( 19.03943276465977164, -0.05219959533909143690, 113.7489096053143669 ) ) ;
#97110=CARTESIAN_POINT ( 'NONE',  ( -16.51473224551069308, -9.474510206698971260, 86.66557627198102409 ) ) ;
#97111=CARTESIAN_POINT ( 'NONE',  ( -9.474510206698964154, 16.51473224551069663, 90.41557627198103830 ) ) ;
#97112=CARTESIAN_POINT ( 'NONE',  ( -21.55341960407610458, -5.719274019375992779, 61.45724293864770260 ) ) ;
#97113=CARTESIAN_POINT ( 'NONE',  ( 12.06949235617757843, -12.14591786802309237, 98.12390960531436690 ) ) ;
#97114=CARTESIAN_POINT ( 'NONE',  ( -13.97604488694527625, -13.89961937509977652, 66.87390960531436690 ) ) ;
#97115=CARTESIAN_POINT ( 'NONE',  ( 16.53943276465976808, -0.05219959533910856209, 108.7489096053143669 ) ) ;
#97116=CARTESIAN_POINT ( 'NONE',  ( -21.55341960407619339, 5.719274019375674811, 43.54275706135235424 ) ) ;
#97117=CARTESIAN_POINT ( 'NONE',  ( 18.67979575497194134, -10.72451020669871369, 75.83442372801900433 ) ) ;
#97118=CARTESIAN_POINT ( 'NONE',  ( -9.474510206698964154, 16.51473224551069663, 60.41557627198102409 ) ) ;
#97119=CARTESIAN_POINT ( 'NONE',  ( 16.52544592524335698, 4.483927247898782831, 76.45942372801901854 ) ) ;
#97120=CARTESIAN_POINT ( 'NONE',  ( -10.72451020669870658, -18.67979575497194134, 34.58442372801900433 ) ) ;
#97121=CARTESIAN_POINT ( 'NONE',  ( -21.52544592524334988, -5.823673210054445271, 28.95942372801902209 ) ) ;
#97122=CARTESIAN_POINT ( 'NONE',  ( 19.02544592524334988, 5.153800228976608722, 46.45942372801899012 ) ) ;
#97123=CARTESIAN_POINT ( 'NONE',  ( -9.474510206698964154, 16.51473224551069663, 75.41557627198103830 ) ) ;
#97124=CARTESIAN_POINT ( 'NONE',  ( -0.05219959533936034679, 19.03943276465977164, 27.50109039468566507 ) ) ;
#97125=CARTESIAN_POINT ( 'NONE',  ( 0.05219959533937995610, -21.53943276465977519, 80.00109039468568994 ) ) ;
#97126=CARTESIAN_POINT ( 'NONE',  ( -10.72451020669898014, 18.67979575497178502, 70.41557627198102409 ) ) ;
#97127=CARTESIAN_POINT ( 'NONE',  ( -14.29746914071049879, 8.314922557960819915, 50.83224293864770971 ) ) ;
#97128=CARTESIAN_POINT ( 'NONE',  ( -21.53943276465977519, -0.05219959533937600094, 93.75109039468567573 ) ) ;
#97129=CARTESIAN_POINT ( 'NONE',  ( -19.05341960407617563, 5.049401038297882671, 33.54275706135231871 ) ) ;
#97130=CARTESIAN_POINT ( 'NONE',  ( 14.34966873604960469, 8.224510206698951720, 64.16557627198102409 ) ) ;
#97131=CARTESIAN_POINT ( 'NONE',  ( 16.46253265017160672, -9.564922557960803928, 23.33224293864769194 ) ) ;
#97132=CARTESIAN_POINT ( 'NONE',  ( 16.46253265017146816, 9.564922557961045513, 56.66775706135233293 ) ) ;
#97133=CARTESIAN_POINT ( 'NONE',  ( 16.52544592524342804, -4.483927247898539470, 33.54057627198102409 ) ) ;
#97134=CARTESIAN_POINT ( 'NONE',  ( -5.823673210054431948, 21.52544592524334988, 82.70942372801900433 ) ) ;
#97136=CARTESIAN_POINT ( 'NONE',  ( -16.51473224551069308, -9.474510206698971260, 81.66557627198103830 ) ) ;
#97137=CARTESIAN_POINT ( 'NONE',  ( 19.05341960407617918, -5.049401038297876454, 46.04275706135233293 ) ) ;
#97138=CARTESIAN_POINT ( 'NONE',  ( -5.823673210054116645, -21.52544592524344225, 47.29057627198103120 ) ) ;
#97139=CARTESIAN_POINT ( 'NONE',  ( 21.52544592524334988, 5.823673210054432836, 51.45942372801901854 ) ) ;
#97140=CARTESIAN_POINT ( 'NONE',  ( -18.67979575497178146, -10.72451020669898902, 101.6655762719810383 ) ) ;
#97141=CARTESIAN_POINT ( 'NONE',  ( -5.049401038297874678, -19.05341960407617918, 94.79275706135230450 ) ) ;
#97142=CARTESIAN_POINT ( 'NONE',  ( -14.29746914071037622, -8.314922557961029526, 64.16775706135234714 ) ) ;
#97144=CARTESIAN_POINT ( 'NONE',  ( -10.81492255796078084, -18.62759615963271287, 107.0822429386476955 ) ) ;
#97145=CARTESIAN_POINT ( 'NONE',  ( -12.14591786802309592, -12.06949235617757132, 101.8739096053143811 ) ) ;
#97147=CARTESIAN_POINT ( 'NONE',  ( 12.14591786802327356, -12.06949235617739191, 40.62609039468567573 ) ) ;
#97148=CARTESIAN_POINT ( 'NONE',  ( 21.52544592524344225, -5.823673210054117533, 68.54057627198103830 ) ) ;
#97149=CARTESIAN_POINT ( 'NONE',  ( -12.14591786802326823, 12.06949235617739902, 103.1260903946856757 ) ) ;
#97150=CARTESIAN_POINT ( 'NONE',  ( -9.564922557960796823, -16.46253265017161027, 32.08224293864769550 ) ) ;
#97151=CARTESIAN_POINT ( 'NONE',  ( -4.483927247898782831, 16.52544592524335698, 62.70942372801902565 ) ) ;
#97152=CARTESIAN_POINT ( 'NONE',  ( 5.049401038297881783, 19.05341960407617563, 57.29275706135231871 ) ) ;
#97153=CARTESIAN_POINT ( 'NONE',  ( 18.67979575497194134, -10.72451020669871369, 40.83442372801901854 ) ) ;
#97154=CARTESIAN_POINT ( 'NONE',  ( 15.72974639402199770, -15.80617190586745480, 53.12390960531436690 ) ) ;
#97155=CARTESIAN_POINT ( 'NONE',  ( 0.05219959533934541429, -16.53943276465976808, 100.0010903946857042 ) ) ;
#97156=CARTESIAN_POINT ( 'NONE',  ( -0.05219959533937732626, 21.53943276465977519, 67.50109039468568994 ) ) ;
#97157=CARTESIAN_POINT ( 'NONE',  ( 21.52544592524344225, -5.823673210054117533, 58.54057627198103120 ) ) ;
#97158=CARTESIAN_POINT ( 'NONE',  ( 15.72974639402199770, -15.80617190586745480, 28.12390960531435979 ) ) ;
#97159=CARTESIAN_POINT ( 'NONE',  ( 8.224510206698742110, 14.34966873604972548, 77.08442372801901854 ) ) ;
#97160=CARTESIAN_POINT ( 'NONE',  ( -15.72974639402197994, 15.80617190586746368, 30.62390960531436335 ) ) ;
#97161=CARTESIAN_POINT ( 'NONE',  ( -16.51473224551069308, -9.474510206698971260, 96.66557627198102409 ) ) ;
#97162=CARTESIAN_POINT ( 'NONE',  ( 16.53943276465976808, 0.05219959533934440121, 111.2510903946856899 ) ) ;
#97164=CARTESIAN_POINT ( 'NONE',  ( 16.55341960407611168, 4.379528057220329451, 103.9572429386476813 ) ) ;
#97165=CARTESIAN_POINT ( 'NONE',  ( 18.62759615963271287, -10.81492255796078972, 63.33224293864770260 ) ) ;
#97166=CARTESIAN_POINT ( 'NONE',  ( -14.34966873604972548, 8.224510206698743886, 88.33442372801901854 ) ) ;
#97167=CARTESIAN_POINT ( 'NONE',  ( 18.67979575497194134, -10.72451020669871369, 50.83442372801901143 ) ) ;
#97168=CARTESIAN_POINT ( 'NONE',  ( 13.97604488694548053, -13.89961937509957401, 100.6260903946856615 ) ) ;
#97169=CARTESIAN_POINT ( 'NONE',  ( 8.314922557960818139, 14.29746914071049879, 99.58224293864770971 ) ) ;
#97170=CARTESIAN_POINT ( 'NONE',  ( -5.049401038298153566, 19.05341960407611168, 60.20724293864768129 ) ) ;
#97171=CARTESIAN_POINT ( 'NONE',  ( 19.03943276465977164, -0.05219959533909143690, 28.74890960531435624 ) ) ;
#97173=CARTESIAN_POINT ( 'NONE',  ( -5.153800228976328057, -19.02544592524343514, 92.29057627198099567 ) ) ;
#97174=CARTESIAN_POINT ( 'NONE',  ( 4.483927247898790824, -16.52544592524335698, 80.20942372801901854 ) ) ;
#97175=CARTESIAN_POINT ( 'NONE',  ( 18.62759615963255655, 10.81492255796105972, 106.6677570613523756 ) ) ;
#97176=CARTESIAN_POINT ( 'NONE',  ( -15.80617190586745835, -15.72974639402198527, 56.87390960531436690 ) ) ;
#97177=CARTESIAN_POINT ( 'NONE',  ( -16.53943276465976808, -0.05219959533934237506, 83.75109039468568994 ) ) ;
#97178=CARTESIAN_POINT ( 'NONE',  ( -16.46253265017146816, -9.564922557961047289, 79.16775706135234714 ) ) ;
#97179=CARTESIAN_POINT ( 'NONE',  ( -19.02544592524342804, 5.153800228976336051, 41.04057627198103120 ) ) ;
#97180=CARTESIAN_POINT ( 'NONE',  ( -0.05219959533909027116, -19.03943276465977164, 82.49890960531436690 ) ) ;
#97181=CARTESIAN_POINT ( 'NONE',  ( -5.153800228976328057, -19.02544592524343514, 32.29057627198102409 ) ) ;
#97182=CARTESIAN_POINT ( 'NONE',  ( 9.564922557961047289, -16.46253265017146816, 75.41775706135234714 ) ) ;
#97184=CARTESIAN_POINT ( 'NONE',  ( 13.97604488694527802, 13.89961937509977652, 94.37390960531436690 ) ) ;
#97185=CARTESIAN_POINT ( 'NONE',  ( -4.379528057220328563, 16.55341960407611168, 45.20724293864769550 ) ) ;
#97186=CARTESIAN_POINT ( 'NONE',  ( -18.62759615963270932, 10.81492255796079327, 65.83224293864769550 ) ) ;
#97187=CARTESIAN_POINT ( 'NONE',  ( -17.49999999999999645, 3.189878218039158497, 104.8705143742874810 ) ) ;
#97188=CARTESIAN_POINT ( 'NONE',  ( 9.564922557961047289, -16.46253265017146816, 35.41775706135233293 ) ) ;
#97190=CARTESIAN_POINT ( 'NONE',  ( -0.05219959533909027116, -19.03943276465977164, 47.49890960531435979 ) ) ;
#97191=CARTESIAN_POINT ( 'NONE',  ( -16.46253265017160317, 9.564922557960807481, 70.83224293864770971 ) ) ;
#97192=CARTESIAN_POINT ( 'NONE',  ( 4.483927247898790824, -16.52544592524335698, 35.20942372801901854 ) ) ;
#97193=CARTESIAN_POINT ( 'NONE',  ( -17.49999999999999645, -5.500000000000000888, 120.0000000000000142 ) ) ;
#97194=CARTESIAN_POINT ( 'NONE',  ( -16.19135201231366850, 7.376712067591920885, 109.8131914594797252 ) ) ;
#97195=CARTESIAN_POINT ( 'NONE',  ( -8.224510206698735004, -14.34966873604973081, 69.58442372801900433 ) ) ;
#97196=CARTESIAN_POINT ( 'NONE',  ( 5.823673210054125526, 21.52544592524343514, 89.79057627198103830 ) ) ;
#97197=CARTESIAN_POINT ( 'NONE',  ( 8.224510206698742110, 14.34966873604972548, 47.08442372801901854 ) ) ;
#97198=CARTESIAN_POINT ( 'NONE',  ( -16.46253265017160317, 9.564922557960807481, 40.83224293864769550 ) ) ;
#97199=CARTESIAN_POINT ( 'NONE',  ( 17.50000000000000000, 5.499999999999992895, 81.70309617465829888 ) ) ;
#97200=CARTESIAN_POINT ( 'NONE',  ( 10.72451020669871369, 18.67979575497193778, 57.08442372801901854 ) ) ;
#97201=CARTESIAN_POINT ( 'NONE',  ( 19.03943276465977164, 0.05219959533936151252, 61.25109039468566863 ) ) ;
#97202=CARTESIAN_POINT ( 'NONE',  ( -21.53943276465977519, -0.05219959533937600094, 88.75109039468567573 ) ) ;
#97204=CARTESIAN_POINT ( 'NONE',  ( -4.379528057220328563, 16.55341960407611168, 45.20724293864769550 ) ) ;
#97206=CARTESIAN_POINT ( 'NONE',  ( 21.53943276465977519, -0.05219959533907433946, 58.74890960531436690 ) ) ;
#97208=CARTESIAN_POINT ( 'NONE',  ( 16.51473224551069308, 9.474510206698969483, 109.1655762719810383 ) ) ;
#97209=CARTESIAN_POINT ( 'NONE',  ( 0.05219959533910956823, 16.53943276465976808, 99.99890960531436690 ) ) ;
#97210=CARTESIAN_POINT ( 'NONE',  ( 12.06949235617739724, 12.14591786802326823, 21.87609039468567573 ) ) ;
#97211=CARTESIAN_POINT ( 'NONE',  ( -16.53943276465976808, -0.05219959533934237506, 113.7510903946856757 ) ) ;
#97212=ORIENTED_EDGE ( 'NONE', *, *, #91919, .T. ) ;
#97213=CARTESIAN_POINT ( 'NONE',  ( -21.52544592524343514, 5.823673210054127303, 96.04057627198102409 ) ) ;
#97214=CARTESIAN_POINT ( 'NONE',  ( -16.53943276465976808, 0.05219959533911058130, 26.24890960531435624 ) ) ;
#97216=CARTESIAN_POINT ( 'NONE',  ( -0.05219959533936034679, 19.03943276465977164, 87.50109039468567573 ) ) ;
#97217=CARTESIAN_POINT ( 'NONE',  ( 15.72974639402176855, 15.80617190586768217, 106.8760903946856899 ) ) ;
#97218=CARTESIAN_POINT ( 'NONE',  ( 4.483927247898545687, 16.52544592524342804, 29.79057627198102409 ) ) ;
#97219=CARTESIAN_POINT ( 'NONE',  ( -5.823673210054116645, -21.52544592524344225, 92.29057627198103830 ) ) ;
#97220=CARTESIAN_POINT ( 'NONE',  ( 15.72974639402199770, -15.80617190586745480, 48.12390960531436690 ) ) ;
#97221=CARTESIAN_POINT ( 'NONE',  ( -5.049401038298153566, 19.05341960407611168, 60.20724293864768129 ) ) ;
#97222=CARTESIAN_POINT ( 'NONE',  ( 4.483927247898545687, 16.52544592524342804, 29.79057627198102409 ) ) ;
#97223=CARTESIAN_POINT ( 'NONE',  ( -5.153800228976328057, -19.02544592524343514, 97.29057627198099567 ) ) ;
#97224=CARTESIAN_POINT ( 'NONE',  ( 18.22780087662126647, 5.499999999999818812, 56.48236817873107185 ) ) ;
#97225=CARTESIAN_POINT ( 'NONE',  ( 9.474510206698729675, 16.51473224551082808, 47.08442372801900433 ) ) ;
#97226=CARTESIAN_POINT ( 'NONE',  ( 15.80617190586746368, 15.72974639402197994, 79.37390960531436690 ) ) ;
#97227=CARTESIAN_POINT ( 'NONE',  ( 8.224510206698953496, -14.34966873604960469, 102.9155762719810383 ) ) ;
#97228=CARTESIAN_POINT ( 'NONE',  ( -10.72451020669870658, -18.67979575497194134, 39.58442372801901143 ) ) ;
#97230=CARTESIAN_POINT ( 'NONE',  ( -16.55341960407617563, 4.379528057220093196, 103.5427570613523613 ) ) ;
#97231=CARTESIAN_POINT ( 'NONE',  ( -13.97604488694527625, -13.89961937509977652, 36.87390960531436690 ) ) ;
#97232=CARTESIAN_POINT ( 'NONE',  ( -19.05341960407611168, -5.049401038298163336, 86.45724293864769550 ) ) ;
#97234=CARTESIAN_POINT ( 'NONE',  ( 16.46253265017160672, -9.564922557960803928, 33.33224293864770260 ) ) ;
#97235=CARTESIAN_POINT ( 'NONE',  ( -12.14591786802309592, -12.06949235617757132, 41.87390960531435979 ) ) ;
#97236=CARTESIAN_POINT ( 'NONE',  ( -18.67979575497193778, 10.72451020669871902, 78.33442372801901854 ) ) ;
#97238=CARTESIAN_POINT ( 'NONE',  ( 16.52544592524335698, 4.483927247898782831, 66.45942372801903275 ) ) ;
#97239=CARTESIAN_POINT ( 'NONE',  ( -9.564922557960796823, -16.46253265017161027, 47.08224293864769550 ) ) ;
#97240=CARTESIAN_POINT ( 'NONE',  ( -19.03943276465977164, 0.05219959533909376836, 46.24890960531435979 ) ) ;
#97242=CARTESIAN_POINT ( 'NONE',  ( -15.80617190586768217, 15.72974639402176855, 108.1260903946856757 ) ) ;
#97243=CARTESIAN_POINT ( 'NONE',  ( -4.379528057220086978, -16.55341960407618274, 59.79275706135234714 ) ) ;
#97244=CARTESIAN_POINT ( 'NONE',  ( -5.823673210054431948, 21.52544592524334988, 102.7094237280190185 ) ) ;
#97245=CARTESIAN_POINT ( 'NONE',  ( 15.72974639402199770, -15.80617190586745480, 38.12390960531436690 ) ) ;
#97246=CARTESIAN_POINT ( 'NONE',  ( 13.89961937509957401, 13.97604488694547697, 111.8760903946856757 ) ) ;
#97247=CARTESIAN_POINT ( 'NONE',  ( -18.62759615963255300, -10.81492255796106328, 74.16775706135231871 ) ) ;
#97248=CARTESIAN_POINT ( 'NONE',  ( 12.14591786802327356, -12.06949235617739191, 35.62609039468568994 ) ) ;
#97249=CARTESIAN_POINT ( 'NONE',  ( -18.67979575497178146, -10.72451020669898902, 101.6655762719810383 ) ) ;
#97250=CARTESIAN_POINT ( 'NONE',  ( 5.153800228976615827, -19.02544592524334988, 100.2094237280190043 ) ) ;
#97251=CARTESIAN_POINT ( 'NONE',  ( 19.02544592524343514, -5.153800228976328945, 68.54057627198103830 ) ) ;
#97252=CARTESIAN_POINT ( 'NONE',  ( 13.89961937509957401, 13.97604488694547697, 111.8760903946856757 ) ) ;
#97253=CARTESIAN_POINT ( 'NONE',  ( 19.02544592524334988, 5.153800228976608722, 106.4594237280190185 ) ) ;
#97254=CARTESIAN_POINT ( 'NONE',  ( -8.224510206698948167, 14.34966873604960824, 70.41557627198102409 ) ) ;
#97255=CARTESIAN_POINT ( 'NONE',  ( -16.53943276465976808, -0.05219959533934237506, 73.75109039468567573 ) ) ;
#97256=CARTESIAN_POINT ( 'NONE',  ( 10.72451020669871369, 18.67979575497193778, 22.08442372801901143 ) ) ;
#97257=CARTESIAN_POINT ( 'NONE',  ( 5.049401038298161559, -19.05341960407611168, 52.70724293864767418 ) ) ;
#97258=CARTESIAN_POINT ( 'NONE',  ( -13.89961937509977652, 13.97604488694528158, 60.62390960531436690 ) ) ;
#97259=CARTESIAN_POINT ( 'NONE',  ( 8.314922557961029526, -14.29746914071037800, 70.41775706135236135 ) ) ;
#97261=DIRECTION ( 'NONE',  ( 0.000000000000000000, 0.000000000000000000, -1.000000000000000000 ) ) ;
#97263=CARTESIAN_POINT ( 'NONE',  ( -9.564922557961040184, 16.46253265017147172, 22.91775706135233648 ) ) ;
#97264=CARTESIAN_POINT ( 'NONE',  ( 19.03943276465977164, -0.05219959533909143690, 23.74890960531435269 ) ) ;
#97266=CARTESIAN_POINT ( 'NONE',  ( -5.049401038297874678, -19.05341960407617918, 109.7927570613523187 ) ) ;
#97267=CARTESIAN_POINT ( 'NONE',  ( -5.719274019375978568, 21.55341960407610458, 50.20724293864769550 ) ) ;
#97268=CARTESIAN_POINT ( 'NONE',  ( 0.05219959533936267826, -19.03943276465977164, 50.00109039468566863 ) ) ;
#97269=CARTESIAN_POINT ( 'NONE',  ( 12.14591786802327356, -12.06949235617739191, 25.62609039468567929 ) ) ;
#97270=CARTESIAN_POINT ( 'NONE',  ( -19.02544592524342804, 5.153800228976336051, 46.04057627198101699 ) ) ;
#97271=CARTESIAN_POINT ( 'NONE',  ( 0.05219959533909260263, 19.03943276465977164, 54.99890960531435979 ) ) ;
#97272=CARTESIAN_POINT ( 'NONE',  ( -21.52544592524343514, 5.823673210054127303, 91.04057627198103830 ) ) ;
#97274=CARTESIAN_POINT ( 'NONE',  ( -19.05341960407611168, -5.049401038298163336, 56.45724293864768129 ) ) ;
#97276=CARTESIAN_POINT ( 'NONE',  ( 0.05219959533936267826, -19.03943276465977164, 95.00109039468567573 ) ) ;
#97277=CARTESIAN_POINT ( 'NONE',  ( -8.314922557960811034, -14.29746914071050412, 62.08224293864769550 ) ) ;
#97278=CARTESIAN_POINT ( 'NONE',  ( -16.46253265017146816, -9.564922557961047289, 24.16775706135233648 ) ) ;
#97279=CARTESIAN_POINT ( 'NONE',  ( -21.52544592524343514, 5.823673210054127303, 96.04057627198102409 ) ) ;
#97280=CARTESIAN_POINT ( 'NONE',  ( -18.67979575497193778, 10.72451020669871902, 88.33442372801901854 ) ) ;
#97281=CARTESIAN_POINT ( 'NONE',  ( -16.51473224551069308, -9.474510206698971260, 26.66557627198103120 ) ) ;
#97282=CARTESIAN_POINT ( 'NONE',  ( 21.55341960407619695, -5.719274019375665929, 81.04275706135236135 ) ) ;
#97284=CARTESIAN_POINT ( 'NONE',  ( -12.06949235617756955, 12.14591786802309770, 30.62390960531436335 ) ) ;
#97285=CARTESIAN_POINT ( 'NONE',  ( 10.81492255796106328, -18.62759615963255655, 80.41775706135234714 ) ) ;
#97286=CARTESIAN_POINT ( 'NONE',  ( -19.02544592524342804, 5.153800228976336051, 66.04057627198103830 ) ) ;
#97287=CARTESIAN_POINT ( 'NONE',  ( 0.05219959533937995610, -21.53943276465977519, 45.00109039468568284 ) ) ;
#97288=CARTESIAN_POINT ( 'NONE',  ( 19.02544592524343514, -5.153800228976328945, 78.54057627198099567 ) ) ;
#97289=CARTESIAN_POINT ( 'NONE',  ( -8.314922557960811034, -14.29746914071050412, 92.08224293864769550 ) ) ;
#97290=CARTESIAN_POINT ( 'NONE',  ( -12.06949235617756955, 12.14591786802309770, 55.62390960531436690 ) ) ;
#97291=CARTESIAN_POINT ( 'NONE',  ( -10.81492255796078084, -18.62759615963271287, 72.08224293864769550 ) ) ;
#97293=CARTESIAN_POINT ( 'NONE',  ( -9.474510206698964154, 16.51473224551069663, 55.41557627198103120 ) ) ;
#97294=CARTESIAN_POINT ( 'NONE',  ( 21.52544592524344225, -5.823673210054117533, 83.54057627198102409 ) ) ;
#97295=CARTESIAN_POINT ( 'NONE',  ( 9.564922557961047289, -16.46253265017146816, 65.41775706135233293 ) ) ;
#97296=CARTESIAN_POINT ( 'NONE',  ( 16.51473224551083163, -9.474510206698727899, 35.83442372801899722 ) ) ;
#97297=CARTESIAN_POINT ( 'NONE',  ( -0.05219959533910754901, -16.53943276465976808, 82.49890960531436690 ) ) ;
#97298=CARTESIAN_POINT ( 'NONE',  ( -5.823673210054116645, -21.52544592524344225, 47.29057627198103120 ) ) ;
#97299=CARTESIAN_POINT ( 'NONE',  ( 17.48847506799969409, 5.747544572773783500, 101.6730256215672057 ) ) ;
#97300=CARTESIAN_POINT ( 'NONE',  ( 16.55341960407618274, -4.379528057220086978, 96.04275706135236135 ) ) ;
#97302=CARTESIAN_POINT ( 'NONE',  ( 19.02544592524334988, 5.153800228976608722, 96.45942372801897591 ) ) ;
#97303=CARTESIAN_POINT ( 'NONE',  ( 0.05219959533910956823, 16.53943276465976808, 64.99890960531435269 ) ) ;
#97304=CARTESIAN_POINT ( 'NONE',  ( -17.49999999999999289, 5.068104630630395846, 35.72818405340028391 ) ) ;
#97305=CARTESIAN_POINT ( 'NONE',  ( -9.564922557960796823, -16.46253265017161027, 62.08224293864769550 ) ) ;
#97306=CARTESIAN_POINT ( 'NONE',  ( 16.52544592524342804, -4.483927247898539470, 53.54057627198103120 ) ) ;
#97307=CARTESIAN_POINT ( 'NONE',  ( -19.05341960407611168, -5.049401038298163336, 101.4572429386476955 ) ) ;
#97308=CARTESIAN_POINT ( 'NONE',  ( -5.049401038297874678, -19.05341960407617918, 74.79275706135231871 ) ) ;
#97309=CARTESIAN_POINT ( 'NONE',  ( -13.97604488694527625, -13.89961937509977652, 71.87390960531433848 ) ) ;
#97310=CARTESIAN_POINT ( 'NONE',  ( -5.049401038298153566, 19.05341960407611168, 90.20724293864766707 ) ) ;
#97311=CARTESIAN_POINT ( 'NONE',  ( -13.97604488694527625, -13.89961937509977652, 81.87390960531436690 ) ) ;
#97312=CARTESIAN_POINT ( 'NONE',  ( 21.52544592524344225, -5.823673210054117533, 68.54057627198103830 ) ) ;
#97313=CARTESIAN_POINT ( 'NONE',  ( 12.14591786802327356, -12.06949235617739191, 55.62609039468568284 ) ) ;
#97314=CARTESIAN_POINT ( 'NONE',  ( -9.564922557961040184, 16.46253265017147172, 102.9177570613523329 ) ) ;
#97315=CARTESIAN_POINT ( 'NONE',  ( -9.564922557960796823, -16.46253265017161027, 47.08224293864769550 ) ) ;
#97316=CARTESIAN_POINT ( 'NONE',  ( 10.81492255796078972, 18.62759615963270932, 54.58224293864769550 ) ) ;
#97317=CARTESIAN_POINT ( 'NONE',  ( -9.564922557961040184, 16.46253265017147172, 97.91775706135233293 ) ) ;
#97318=CARTESIAN_POINT ( 'NONE',  ( 4.379528057220339221, -16.55341960407611168, 22.70724293864769194 ) ) ;
#97319=CARTESIAN_POINT ( 'NONE',  ( 21.53943276465977519, 0.05219959533937863772, 41.25109039468568284 ) ) ;
#97320=CARTESIAN_POINT ( 'NONE',  ( -19.03943276465977164, -0.05219959533935918106, 33.75109039468566863 ) ) ;
#97321=CARTESIAN_POINT ( 'NONE',  ( -16.55341960407617563, 4.379528057220093196, 53.54275706135234714 ) ) ;
#97322=CARTESIAN_POINT ( 'NONE',  ( -16.52544592524335698, -4.483927247898792601, 88.95942372801901854 ) ) ;
#97323=CARTESIAN_POINT ( 'NONE',  ( -18.22780087662122028, 5.500000000000031086, 73.51540105326107266 ) ) ;
#97324=CARTESIAN_POINT ( 'NONE',  ( -8.224510206698735004, -14.34966873604973081, 79.58442372801903275 ) ) ;
#97325=CARTESIAN_POINT ( 'NONE',  ( 10.72451020669898902, -18.67979575497178502, 22.91557627198102765 ) ) ;
#97326=CARTESIAN_POINT ( 'NONE',  ( -8.314922557961024197, 14.29746914071037800, 32.91775706135234714 ) ) ;
#97327=CARTESIAN_POINT ( 'NONE',  ( -19.05341960407611168, -5.049401038298163336, 51.45724293864770260 ) ) ;
#97328=CARTESIAN_POINT ( 'NONE',  ( -5.049401038298153566, 19.05341960407611168, 55.20724293864769550 ) ) ;
#97329=CARTESIAN_POINT ( 'NONE',  ( -0.05219959533909027116, -19.03943276465977164, 57.49890960531435979 ) ) ;
#97330=CARTESIAN_POINT ( 'NONE',  ( 18.62759615963255655, 10.81492255796105972, 41.66775706135235424 ) ) ;
#97331=CARTESIAN_POINT ( 'NONE',  ( -4.483927247898782831, 16.52544592524335698, 42.70942372801901854 ) ) ;
#97332=CARTESIAN_POINT ( 'NONE',  ( -12.14591786802326823, 12.06949235617739902, 108.1260903946856757 ) ) ;
#97333=CARTESIAN_POINT ( 'NONE',  ( 5.153800228976335163, 19.02544592524342804, 29.79057627198102409 ) ) ;
#97334=CARTESIAN_POINT ( 'NONE',  ( -9.564922557961040184, 16.46253265017147172, 22.91775706135233648 ) ) ;
#97335=CARTESIAN_POINT ( 'NONE',  ( -5.049401038297874678, -19.05341960407617918, 109.7927570613523187 ) ) ;
#97336=CARTESIAN_POINT ( 'NONE',  ( 0.05219959533936267826, -19.03943276465977164, 75.00109039468566152 ) ) ;
#97337=CARTESIAN_POINT ( 'NONE',  ( 4.483927247898545687, 16.52544592524342804, 64.79057627198103830 ) ) ;
#97338=CARTESIAN_POINT ( 'NONE',  ( 9.564922557960805705, 16.46253265017160317, 39.58224293864768839 ) ) ;
#97339=CARTESIAN_POINT ( 'NONE',  ( -13.89961937509957401, -13.97604488694547875, 74.37609039468566152 ) ) ;
#97340=CARTESIAN_POINT ( 'NONE',  ( 16.29526858892876362, -7.335722546920113274, 91.70329402199793378 ) ) ;
#97341=CARTESIAN_POINT ( 'NONE',  ( -18.67979575497193778, 10.72451020669871902, 73.33442372801901854 ) ) ;
#97342=CARTESIAN_POINT ( 'NONE',  ( 16.53943276465976808, 0.05219959533934440121, 46.25109039468567573 ) ) ;
#97344=CARTESIAN_POINT ( 'NONE',  ( -10.72451020669898014, 18.67979575497178502, 30.41557627198101699 ) ) ;
#97345=CARTESIAN_POINT ( 'NONE',  ( -12.06949235617739369, -12.14591786802326823, 29.37609039468568284 ) ) ;
#97346=CARTESIAN_POINT ( 'NONE',  ( -5.153800228976328057, -19.02544592524343514, 22.29057627198102765 ) ) ;
#97347=CARTESIAN_POINT ( 'NONE',  ( -19.02544592524334988, -5.153800228976617603, 23.95942372801900078 ) ) ;
#97349=CARTESIAN_POINT ( 'NONE',  ( -5.049401038298153566, 19.05341960407611168, 40.20724293864768839 ) ) ;
#97351=CARTESIAN_POINT ( 'NONE',  ( 13.97604488694527802, 13.89961937509977652, 64.37390960531436690 ) ) ;
#97352=CARTESIAN_POINT ( 'NONE',  ( -17.60728821186566506, 5.500000000000031974, 65.86690927743006796 ) ) ;
#97353=CARTESIAN_POINT ( 'NONE',  ( 5.153800228976615827, -19.02544592524334988, 20.20942372801899722 ) ) ;
#97354=CARTESIAN_POINT ( 'NONE',  ( -8.224510206698948167, 14.34966873604960824, 25.41557627198103120 ) ) ;
#97355=CARTESIAN_POINT ( 'NONE',  ( 13.89961937509977652, -13.97604488694527269, 33.12390960531434558 ) ) ;
#97356=CARTESIAN_POINT ( 'NONE',  ( 16.51473224551069308, 9.474510206698969483, 94.16557627198103830 ) ) ;
#97357=CARTESIAN_POINT ( 'NONE',  ( -5.719274019375665041, -21.55341960407619695, 64.79275706135234714 ) ) ;
#97358=CARTESIAN_POINT ( 'NONE',  ( 9.564922557960805705, 16.46253265017160317, 49.58224293864770260 ) ) ;
#97359=CARTESIAN_POINT ( 'NONE',  ( -5.823673210054431948, 21.52544592524334988, 62.70942372801902565 ) ) ;
#97360=CARTESIAN_POINT ( 'NONE',  ( -19.02544592524334988, -5.153800228976617603, 88.95942372801897591 ) ) ;
#97361=CARTESIAN_POINT ( 'NONE',  ( 15.72974639402199770, -15.80617190586745480, 28.12390960531435979 ) ) ;
#97362=CARTESIAN_POINT ( 'NONE',  ( 9.474510206698971260, -16.51473224551069308, 37.91557627198102409 ) ) ;
#97363=CARTESIAN_POINT ( 'NONE',  ( 15.72974639402199770, -15.80617190586745480, 113.1239096053143953 ) ) ;
#97364=CARTESIAN_POINT ( 'NONE',  ( 0.05219959533936267826, -19.03943276465977164, 35.00109039468566863 ) ) ;
#97365=CARTESIAN_POINT ( 'NONE',  ( 4.483927247898545687, 16.52544592524342804, 104.7905762719810241 ) ) ;
#97366=CARTESIAN_POINT ( 'NONE',  ( 5.049401038298161559, -19.05341960407611168, 62.70724293864769550 ) ) ;
#97367=CARTESIAN_POINT ( 'NONE',  ( 16.51473224551083163, -9.474510206698727899, 110.8344237280190043 ) ) ;
#97368=CARTESIAN_POINT ( 'NONE',  ( -16.53943276465976808, 0.05219959533911058130, 81.24890960531436690 ) ) ;
#97369=CARTESIAN_POINT ( 'NONE',  ( -19.02544592524342804, 5.153800228976336051, 116.0405762719810383 ) ) ;
#97370=CARTESIAN_POINT ( 'NONE',  ( -19.02544592524334988, -5.153800228976617603, 83.95942372801901854 ) ) ;
#97371=CARTESIAN_POINT ( 'NONE',  ( -15.72974639402197994, 15.80617190586746368, 90.62390960531436690 ) ) ;
#97372=CARTESIAN_POINT ( 'NONE',  ( -18.67979575497193778, 10.72451020669871902, 38.33442372801900433 ) ) ;
#97373=CARTESIAN_POINT ( 'NONE',  ( -8.224510206698735004, -14.34966873604973081, 54.58442372801901143 ) ) ;
#97374=CARTESIAN_POINT ( 'NONE',  ( 16.52544592524335698, 4.483927247898782831, 51.45942372801901854 ) ) ;
#97375=CARTESIAN_POINT ( 'NONE',  ( 21.53943276465977519, 0.05219959533937863772, 51.25109039468568994 ) ) ;
#97376=CARTESIAN_POINT ( 'NONE',  ( 15.80617190586746368, 15.72974639402197994, 49.37390960531436690 ) ) ;
#97377=CARTESIAN_POINT ( 'NONE',  ( 19.02544592524343514, -5.153800228976328945, 53.54057627198102409 ) ) ;
#97379=CARTESIAN_POINT ( 'NONE',  ( -14.34966873604972548, 8.224510206698743886, 78.33442372801901854 ) ) ;
#97380=CARTESIAN_POINT ( 'NONE',  ( -21.55341960407610458, -5.719274019375992779, 106.4572429386477097 ) ) ;
#97381=CARTESIAN_POINT ( 'NONE',  ( 4.379528057220339221, -16.55341960407611168, 47.70724293864770260 ) ) ;
#97382=CARTESIAN_POINT ( 'NONE',  ( -16.55341960407617563, 4.379528057220093196, 58.54275706135235424 ) ) ;
#97383=CARTESIAN_POINT ( 'NONE',  ( -9.474510206698720793, -16.51473224551083518, 99.58442372801900433 ) ) ;
#97384=CARTESIAN_POINT ( 'NONE',  ( -0.05219959533907301413, -21.53943276465977519, 92.49890960531436690 ) ) ;
#97385=CARTESIAN_POINT ( 'NONE',  ( 8.314922557960818139, 14.29746914071049879, 49.58224293864769550 ) ) ;
#97387=CARTESIAN_POINT ( 'NONE',  ( -17.05116617787824396, 6.768360034955816396, 68.65675553259198693 ) ) ;
#97388=CARTESIAN_POINT ( 'NONE',  ( -18.67979575497178146, -10.72451020669898902, 71.66557627198100988 ) ) ;
#97389=CARTESIAN_POINT ( 'NONE',  ( -8.314922557960811034, -14.29746914071050412, 27.08224293864769550 ) ) ;
#97392=CARTESIAN_POINT ( 'NONE',  ( -5.823673210054116645, -21.52544592524344225, 107.2905762719810525 ) ) ;
#97393=CARTESIAN_POINT ( 'NONE',  ( 18.67979575497178502, 10.72451020669898547, 114.1655762719810383 ) ) ;
#97394=CARTESIAN_POINT ( 'NONE',  ( -0.05219959533910754901, -16.53943276465976808, 32.49890960531435979 ) ) ;
#97395=CARTESIAN_POINT ( 'NONE',  ( -12.14591786802326823, 12.06949235617739902, 48.12609039468568284 ) ) ;
#97396=CARTESIAN_POINT ( 'NONE',  ( 19.05341960407611168, 5.049401038298154454, 43.95724293864769550 ) ) ;
#97397=CARTESIAN_POINT ( 'NONE',  ( -19.03943276465977164, 0.05219959533909376836, 81.24890960531436690 ) ) ;
#97398=CARTESIAN_POINT ( 'NONE',  ( -10.72451020669898014, 18.67979575497178502, 35.41557627198102409 ) ) ;
#97400=CARTESIAN_POINT ( 'NONE',  ( -14.29746914071037622, -8.314922557961029526, 19.16775706135234714 ) ) ;
#97401=CARTESIAN_POINT ( 'NONE',  ( 19.05341960407617918, -5.049401038297876454, 46.04275706135233293 ) ) ;
#97402=CARTESIAN_POINT ( 'NONE',  ( -10.72451020669898014, 18.67979575497178502, 95.41557627198102409 ) ) ;
#97403=CARTESIAN_POINT ( 'NONE',  ( -16.53943276465976808, 0.05219959533911058130, 36.24890960531435979 ) ) ;
#97404=VECTOR ( 'NONE', #195315, 1000.000000000000000 ) ;
#97405=CARTESIAN_POINT ( 'NONE',  ( 16.46253265017160672, -9.564922557960803928, 83.33224293864768129 ) ) ;
#97406=CARTESIAN_POINT ( 'NONE',  ( 18.62759615963271287, -10.81492255796078972, 48.33224293864770260 ) ) ;
#97407=CARTESIAN_POINT ( 'NONE',  ( 10.72451020669898902, -18.67979575497178502, 87.91557627198103830 ) ) ;
#97408=CARTESIAN_POINT ( 'NONE',  ( 16.55341960407618274, -4.379528057220086978, 31.04275706135234714 ) ) ;
#97409=CARTESIAN_POINT ( 'NONE',  ( 10.72451020669898902, -18.67979575497178502, 27.91557627198103830 ) ) ;
#97410=CARTESIAN_POINT ( 'NONE',  ( -15.80617190586768217, 15.72974639402176855, 73.12609039468567573 ) ) ;
#97411=CARTESIAN_POINT ( 'NONE',  ( 9.564922557960805705, 16.46253265017160317, 69.58224293864770971 ) ) ;
#97412=CARTESIAN_POINT ( 'NONE',  ( 16.51473224551069308, 9.474510206698969483, 24.16557627198102765 ) ) ;
#97413=CARTESIAN_POINT ( 'NONE',  ( -9.474510206698964154, 16.51473224551069663, 80.41557627198103830 ) ) ;
#97414=CARTESIAN_POINT ( 'NONE',  ( 12.14591786802309770, 12.06949235617756955, 94.37390960531436690 ) ) ;
#97416=CARTESIAN_POINT ( 'NONE',  ( 16.51473224551083163, -9.474510206698727899, 105.8344237280190043 ) ) ;
#97419=CARTESIAN_POINT ( 'NONE',  ( 0.05219959533909260263, 19.03943276465977164, 69.99890960531435269 ) ) ;
#97420=CARTESIAN_POINT ( 'NONE',  ( -10.81492255796105439, 18.62759615963255655, 87.91775706135234714 ) ) ;
#97421=CARTESIAN_POINT ( 'NONE',  ( -18.67979575497178146, -10.72451020669898902, 21.66557627198102409 ) ) ;
#97422=CARTESIAN_POINT ( 'NONE',  ( -16.52544592524335698, -4.483927247898792601, 78.95942372801901854 ) ) ;
#97423=CARTESIAN_POINT ( 'NONE',  ( -17.13100169013300089, -6.664070546373138448, 74.23210164300155611 ) ) ;
#97424=CARTESIAN_POINT ( 'NONE',  ( 9.564922557961047289, -16.46253265017146816, 55.41775706135234003 ) ) ;
#97425=CARTESIAN_POINT ( 'NONE',  ( -9.564922557961040184, 16.46253265017147172, 22.91775706135233648 ) ) ;
#97427=CARTESIAN_POINT ( 'NONE',  ( -19.03943276465977164, 0.05219959533909376836, 21.24890960531436335 ) ) ;
#97429=CARTESIAN_POINT ( 'NONE',  ( -4.379528057220328563, 16.55341960407611168, 25.20724293864769550 ) ) ;
#97431=CARTESIAN_POINT ( 'NONE',  ( -4.379528057220086978, -16.55341960407618274, 99.79275706135234714 ) ) ;
#97432=CARTESIAN_POINT ( 'NONE',  ( -19.20446147854523744, -5.500000000000000888, 84.38999695167674986 ) ) ;
#97433=CARTESIAN_POINT ( 'NONE',  ( 0.05219959533934541429, -16.53943276465976808, 85.00109039468568994 ) ) ;
#97434=CARTESIAN_POINT ( 'NONE',  ( -19.03943276465977164, 0.05219959533909376836, 21.24890960531436335 ) ) ;
#97435=CARTESIAN_POINT ( 'NONE',  ( 21.55341960407619695, -5.719274019375665929, 91.04275706135236135 ) ) ;
#97436=CARTESIAN_POINT ( 'NONE',  ( -19.03943276465977164, -0.05219959533935918106, 108.7510903946856615 ) ) ;
#97437=CARTESIAN_POINT ( 'NONE',  ( 10.72451020669871369, 18.67979575497193778, 62.08442372801901143 ) ) ;
#97438=CARTESIAN_POINT ( 'NONE',  ( 9.474510206698729675, 16.51473224551082808, 42.08442372801900433 ) ) ;
#97439=CARTESIAN_POINT ( 'NONE',  ( 5.049401038298161559, -19.05341960407611168, 77.70724293864765286 ) ) ;
#97440=CARTESIAN_POINT ( 'NONE',  ( -9.474510206698964154, 16.51473224551069663, 75.41557627198103830 ) ) ;
#97442=CARTESIAN_POINT ( 'NONE',  ( 15.72974639402199770, -15.80617190586745480, 53.12390960531436690 ) ) ;
#97443=CARTESIAN_POINT ( 'NONE',  ( -19.05341960407611168, -5.049401038298163336, 51.45724293864770260 ) ) ;
#97444=CARTESIAN_POINT ( 'NONE',  ( 0.05219959533934541429, -16.53943276465976808, 80.00109039468568994 ) ) ;
#97445=ORIENTED_EDGE ( 'NONE', *, *, #64444, .T. ) ;
#97446=CARTESIAN_POINT ( 'NONE',  ( -16.55341960407611168, -4.379528057220339221, 76.45724293864769550 ) ) ;
#97448=CARTESIAN_POINT ( 'NONE',  ( -14.34966873604972548, 8.224510206698743886, 33.33442372801900433 ) ) ;
#97449=CARTESIAN_POINT ( 'NONE',  ( -4.483927247898539470, -16.52544592524342804, 107.2905762719810525 ) ) ;
#97450=CARTESIAN_POINT ( 'NONE',  ( -9.564922557961040184, 16.46253265017147172, 67.91775706135233293 ) ) ;
#97451=CARTESIAN_POINT ( 'NONE',  ( -12.14591786802309592, -12.06949235617757132, 76.87390960531439532 ) ) ;
#97452=CARTESIAN_POINT ( 'NONE',  ( -15.80617190586768217, 15.72974639402176855, 33.12609039468569705 ) ) ;
#97453=CARTESIAN_POINT ( 'NONE',  ( -15.49999999999999822, 0.000000000000000000, 118.0000000000000142 ) ) ;
#97454=CARTESIAN_POINT ( 'NONE',  ( 15.80617190586746368, 15.72974639402197994, 89.37390960531435269 ) ) ;
#97455=CARTESIAN_POINT ( 'NONE',  ( 13.97604488694527802, 13.89961937509977652, 104.3739096053143385 ) ) ;
#97456=CARTESIAN_POINT ( 'NONE',  ( 8.314922557960818139, 14.29746914071049879, 69.58224293864769550 ) ) ;
#97458=CARTESIAN_POINT ( 'NONE',  ( 9.474510206698971260, -16.51473224551069308, 47.91557627198102409 ) ) ;
#97460=CARTESIAN_POINT ( 'NONE',  ( 19.03943276465977164, 0.05219959533936151252, 86.25109039468567573 ) ) ;
#97461=CARTESIAN_POINT ( 'NONE',  ( 21.52544592524334988, 5.823673210054432836, 21.45942372801901499 ) ) ;
#97462=CARTESIAN_POINT ( 'NONE',  ( 19.05341960407611168, 5.049401038298154454, 73.95724293864768129 ) ) ;
#97463=CARTESIAN_POINT ( 'NONE',  ( -9.564922557961040184, 16.46253265017147172, 57.91775706135233293 ) ) ;
#97464=CARTESIAN_POINT ( 'NONE',  ( -16.46253265017160317, 9.564922557960807481, 40.83224293864769550 ) ) ;
#97466=CARTESIAN_POINT ( 'NONE',  ( 12.06949235617757843, -12.14591786802309237, 63.12390960531435979 ) ) ;
#97467=CARTESIAN_POINT ( 'NONE',  ( 4.379528057220339221, -16.55341960407611168, 47.70724293864770260 ) ) ;
#97468=CARTESIAN_POINT ( 'NONE',  ( 19.05341960407611168, 5.049401038298154454, 73.95724293864768129 ) ) ;
#97469=CARTESIAN_POINT ( 'NONE',  ( -18.67979575497178146, -10.72451020669898902, 81.66557627198103830 ) ) ;
#97470=CARTESIAN_POINT ( 'NONE',  ( 0.05219959533909260263, 19.03943276465977164, 69.99890960531435269 ) ) ;
#97471=CARTESIAN_POINT ( 'NONE',  ( -21.55341960407610458, -5.719274019375992779, 76.45724293864769550 ) ) ;
#97472=CARTESIAN_POINT ( 'NONE',  ( 18.67979575497194134, -10.72451020669871369, 110.8344237280190043 ) ) ;
#97474=CARTESIAN_POINT ( 'NONE',  ( 12.06949235617739724, 12.14591786802326823, 111.8760903946856615 ) ) ;
#97475=CARTESIAN_POINT ( 'NONE',  ( -0.05219959533910754901, -16.53943276465976808, 92.49890960531436690 ) ) ;
#97476=CARTESIAN_POINT ( 'NONE',  ( 13.97604488694548053, -13.89961937509957401, 100.6260903946856615 ) ) ;
#97478=CARTESIAN_POINT ( 'NONE',  ( 18.62759615963271287, -10.81492255796078972, 113.3322429386476955 ) ) ;
#97479=CARTESIAN_POINT ( 'NONE',  ( -9.474510206698720793, -16.51473224551083518, 59.58442372801900433 ) ) ;
#97480=CARTESIAN_POINT ( 'NONE',  ( 16.53943276465976808, -0.05219959533910856209, 28.74890960531435624 ) ) ;
#97481=CARTESIAN_POINT ( 'NONE',  ( -19.02544592524334988, -5.153800228976617603, 43.95942372801899012 ) ) ;
#97482=CARTESIAN_POINT ( 'NONE',  ( -16.46253265017160317, 9.564922557960807481, 95.83224293864769550 ) ) ;
#97483=CARTESIAN_POINT ( 'NONE',  ( -16.52544592524342804, 4.483927247898546575, 56.04057627198102409 ) ) ;
#97485=CARTESIAN_POINT ( 'NONE',  ( 19.05341960407611168, 5.049401038298154454, 33.95724293864769550 ) ) ;
#97486=CARTESIAN_POINT ( 'NONE',  ( -5.823673210054431948, 21.52544592524334988, 107.7094237280190328 ) ) ;
#97487=CARTESIAN_POINT ( 'NONE',  ( -0.05219959533934338120, 16.53943276465976808, 87.50109039468568994 ) ) ;
#97488=CARTESIAN_POINT ( 'NONE',  ( -5.823673210054431948, 21.52544592524334988, 47.70942372801902565 ) ) ;
#97489=CARTESIAN_POINT ( 'NONE',  ( 4.379528057220092307, 16.55341960407617563, 42.29275706135235424 ) ) ;
#97490=CARTESIAN_POINT ( 'NONE',  ( 5.153800228976335163, 19.02544592524342804, 114.7905762719810241 ) ) ;
#97491=CARTESIAN_POINT ( 'NONE',  ( 5.153800228976335163, 19.02544592524342804, 49.79057627198100988 ) ) ;
#97492=CARTESIAN_POINT ( 'NONE',  ( 9.564922557960805705, 16.46253265017160317, 59.58224293864769550 ) ) ;
#97493=CARTESIAN_POINT ( 'NONE',  ( -4.483927247898782831, 16.52544592524335698, 47.70942372801902565 ) ) ;
#97494=CARTESIAN_POINT ( 'NONE',  ( 16.52544592524342804, -4.483927247898539470, 103.5405762719810383 ) ) ;
#97495=CARTESIAN_POINT ( 'NONE',  ( -14.34966873604972548, 8.224510206698743886, 108.3344237280190185 ) ) ;
#97497=CARTESIAN_POINT ( 'NONE',  ( -5.719274019375665041, -21.55341960407619695, 54.79275706135235424 ) ) ;
#97498=CARTESIAN_POINT ( 'NONE',  ( 13.97604488694527802, 13.89961937509977652, 89.37390960531436690 ) ) ;
#97499=CARTESIAN_POINT ( 'NONE',  ( -5.153800228976328057, -19.02544592524343514, 82.29057627198103830 ) ) ;
#97500=CARTESIAN_POINT ( 'NONE',  ( 16.46253265017160672, -9.564922557960803928, 98.33224293864769550 ) ) ;
#97501=CARTESIAN_POINT ( 'NONE',  ( -4.379528057220328563, 16.55341960407611168, 40.20724293864769550 ) ) ;
#97502=CARTESIAN_POINT ( 'NONE',  ( 16.55341960407611168, 4.379528057220329451, 23.95724293864769550 ) ) ;
#97503=CARTESIAN_POINT ( 'NONE',  ( 8.224510206698953496, -14.34966873604960469, 37.91557627198102409 ) ) ;
#97504=ORIENTED_EDGE ( 'NONE', *, *, #96536, .T. ) ;
#97505=CARTESIAN_POINT ( 'NONE',  ( 17.72560187377285601, 5.500000000000050626, 56.57814504131319921 ) ) ;
#97506=CARTESIAN_POINT ( 'NONE',  ( -9.564922557961040184, 16.46253265017147172, 42.91775706135234003 ) ) ;
#97507=CARTESIAN_POINT ( 'NONE',  ( 13.89961937509977652, -13.97604488694527269, 58.12390960531436690 ) ) ;
#97508=CARTESIAN_POINT ( 'NONE',  ( 19.02544592524334988, 5.153800228976608722, 56.45942372801898301 ) ) ;
#97511=CARTESIAN_POINT ( 'NONE',  ( -19.05341960407617563, 5.049401038297882671, 83.54275706135233293 ) ) ;
#97512=CARTESIAN_POINT ( 'NONE',  ( 8.224510206698742110, 14.34966873604972548, 72.08442372801899012 ) ) ;
#97513=PLANE ( 'NONE',  #85195 ) ;
#97514=CARTESIAN_POINT ( 'NONE',  ( 19.05341960407611168, 5.049401038298154454, 108.9572429386477097 ) ) ;
#97515=CARTESIAN_POINT ( 'NONE',  ( -15.80617190586768217, 15.72974639402176855, 23.12609039468567573 ) ) ;
#97516=CARTESIAN_POINT ( 'NONE',  ( 5.153800228976615827, -19.02544592524334988, 85.20942372801900433 ) ) ;
#97517=CARTESIAN_POINT ( 'NONE',  ( 17.49999999999999645, 5.624438216177603422, 86.68329655085356933 ) ) ;
#97518=CARTESIAN_POINT ( 'NONE',  ( 16.46253265017160672, -9.564922557960803928, 43.33224293864769550 ) ) ;
#97519=CARTESIAN_POINT ( 'NONE',  ( 13.97604488694527802, 13.89961937509977652, 94.37390960531436690 ) ) ;
#97520=CARTESIAN_POINT ( 'NONE',  ( 14.29746914071049879, -8.314922557960816363, 53.33224293864769550 ) ) ;
#97521=CARTESIAN_POINT ( 'NONE',  ( -5.153800228976328057, -19.02544592524343514, 47.29057627198102409 ) ) ;
#97522=CARTESIAN_POINT ( 'NONE',  ( 13.97604488694548053, -13.89961937509957401, 60.62609039468564731 ) ) ;
#97523=CARTESIAN_POINT ( 'NONE',  ( 16.46253265017146816, 9.564922557961045513, 31.66775706135232937 ) ) ;
#97524=CARTESIAN_POINT ( 'NONE',  ( -16.46253265017160317, 9.564922557960807481, 65.83224293864769550 ) ) ;
#97526=CARTESIAN_POINT ( 'NONE',  ( 15.72974639402199770, -15.80617190586745480, 58.12390960531435979 ) ) ;
#97527=CARTESIAN_POINT ( 'NONE',  ( -14.34966873604960291, -8.224510206698953496, 66.66557627198102409 ) ) ;
#97528=CARTESIAN_POINT ( 'NONE',  ( 9.474510206698729675, 16.51473224551082808, 22.08442372801899722 ) ) ;
#97529=CARTESIAN_POINT ( 'NONE',  ( -9.564922557960796823, -16.46253265017161027, 102.0822429386477097 ) ) ;
#97530=CARTESIAN_POINT ( 'NONE',  ( -15.72974639402197994, 15.80617190586746368, 30.62390960531436335 ) ) ;
#97531=CARTESIAN_POINT ( 'NONE',  ( -5.049401038298153566, 19.05341960407611168, 50.20724293864770260 ) ) ;
#97532=CARTESIAN_POINT ( 'NONE',  ( 13.89961937509977652, -13.97604488694527269, 33.12390960531434558 ) ) ;
#97533=CARTESIAN_POINT ( 'NONE',  ( -14.29746914071049879, 8.314922557960819915, 95.83224293864770971 ) ) ;
#97534=CARTESIAN_POINT ( 'NONE',  ( -15.72974639402197994, 15.80617190586746368, 115.6239096053143669 ) ) ;
#97535=CARTESIAN_POINT ( 'NONE',  ( 5.049401038298161559, -19.05341960407611168, 112.7072429386476813 ) ) ;
#97536=CARTESIAN_POINT ( 'NONE',  ( -21.55341960407619339, 5.719274019375674811, 28.54275706135234358 ) ) ;
#97537=CARTESIAN_POINT ( 'NONE',  ( 19.05341960407611168, 5.049401038298154454, 108.9572429386477097 ) ) ;
#97538=CARTESIAN_POINT ( 'NONE',  ( -4.379528057220328563, 16.55341960407611168, 115.2072429386476955 ) ) ;
#97539=CARTESIAN_POINT ( 'NONE',  ( -5.823673210054431948, 21.52544592524334988, 72.70942372801901854 ) ) ;
#97540=CARTESIAN_POINT ( 'NONE',  ( 15.80617190586746368, 15.72974639402197994, 94.37390960531436690 ) ) ;
#97543=CARTESIAN_POINT ( 'NONE',  ( -13.89961937509977830, 13.97604488694528158, 60.62390960531436690 ) ) ;
#97544=CARTESIAN_POINT ( 'NONE',  ( 12.06949235617739724, 12.14591786802326823, 46.87609039468568994 ) ) ;
#97545=CARTESIAN_POINT ( 'NONE',  ( 16.53943276465976808, -0.05219959533910856209, 103.7489096053143669 ) ) ;
#97547=CARTESIAN_POINT ( 'NONE',  ( -19.05341960407611168, -5.049401038298163336, 61.45724293864769550 ) ) ;
#97548=CARTESIAN_POINT ( 'NONE',  ( -16.55341960407611168, -4.379528057220339221, 96.45724293864770971 ) ) ;
#97549=CARTESIAN_POINT ( 'NONE',  ( -0.05219959533907301413, -21.53943276465977519, 52.49890960531435979 ) ) ;
#97550=CARTESIAN_POINT ( 'NONE',  ( 4.483927247898545687, 16.52544592524342804, 59.79057627198103120 ) ) ;
#97551=CARTESIAN_POINT ( 'NONE',  ( -0.05219959533936034679, 19.03943276465977164, 112.5010903946856757 ) ) ;
#97552=CARTESIAN_POINT ( 'NONE',  ( 18.67979575497194134, -10.72451020669871369, 85.83442372801901854 ) ) ;
#97553=CARTESIAN_POINT ( 'NONE',  ( 17.05116617787825462, -6.768360034955811066, 76.15675553259197272 ) ) ;
#97554=CARTESIAN_POINT ( 'NONE',  ( -12.14591786802326823, 12.06949235617739902, 93.12609039468568994 ) ) ;
#97555=CARTESIAN_POINT ( 'NONE',  ( 12.06949235617757843, -12.14591786802309237, 38.12390960531436690 ) ) ;
#97556=CARTESIAN_POINT ( 'NONE',  ( -0.05219959533909027116, -19.03943276465977164, 32.49890960531435979 ) ) ;
#97557=CARTESIAN_POINT ( 'NONE',  ( -9.474510206698964154, 16.51473224551069663, 90.41557627198103830 ) ) ;
#97558=CARTESIAN_POINT ( 'NONE',  ( -15.80617190586745835, -15.72974639402198527, 96.87390960531436690 ) ) ;
#97559=CARTESIAN_POINT ( 'NONE',  ( -14.34966873604972548, 8.224510206698743886, 33.33442372801900433 ) ) ;
#97560=CARTESIAN_POINT ( 'NONE',  ( 0.05219959533910956823, 16.53943276465976808, 69.99890960531435269 ) ) ;
#97561=CARTESIAN_POINT ( 'NONE',  ( 5.719274019375673035, 21.55341960407619339, 92.29275706135236135 ) ) ;
#97562=CARTESIAN_POINT ( 'NONE',  ( 12.14591786802327356, -12.06949235617739191, 95.62609039468568994 ) ) ;
#97563=CARTESIAN_POINT ( 'NONE',  ( 17.05116617787848554, -6.768360034955523297, 46.15675553259190877 ) ) ;
#97564=DIRECTION ( 'NONE',  ( -1.000000000000000000, 0.000000000000000000, 0.000000000000000000 ) ) ;
#97565=CARTESIAN_POINT ( 'NONE',  ( -4.483927247898539470, -16.52544592524342804, 27.29057627198103120 ) ) ;
#97566=CARTESIAN_POINT ( 'NONE',  ( -12.06949235617739369, -12.14591786802326823, 74.37609039468568994 ) ) ;
#97567=CARTESIAN_POINT ( 'NONE',  ( -9.564922557960796823, -16.46253265017161027, 82.08224293864768129 ) ) ;
#97568=CARTESIAN_POINT ( 'NONE',  ( -9.474510206698964154, 16.51473224551069663, 100.4155762719810241 ) ) ;
#97569=CARTESIAN_POINT ( 'NONE',  ( 15.80617190586769283, -15.72974639402175789, 90.62609039468567573 ) ) ;
#97570=CARTESIAN_POINT ( 'NONE',  ( -12.06949235617739369, -12.14591786802326823, 94.37609039468568994 ) ) ;
#97571=CARTESIAN_POINT ( 'NONE',  ( -8.224510206698948167, 14.34966873604960824, 65.41557627198102409 ) ) ;
#97572=CARTESIAN_POINT ( 'NONE',  ( 19.03943276465977164, -0.05219959533909143690, 63.74890960531435979 ) ) ;
#97574=CARTESIAN_POINT ( 'NONE',  ( -19.05341960407617563, 5.049401038297882671, 113.5427570613523471 ) ) ;
#97575=CARTESIAN_POINT ( 'NONE',  ( -13.97604488694527625, -13.89961937509977652, 26.87390960531434558 ) ) ;
#97576=CARTESIAN_POINT ( 'NONE',  ( 19.05341960407611168, 5.049401038298154454, 78.95724293864769550 ) ) ;
#97577=CARTESIAN_POINT ( 'NONE',  ( 8.224510206698742110, 14.34966873604972548, 22.08442372801901143 ) ) ;
#97579=CARTESIAN_POINT ( 'NONE',  ( 19.03943276465977164, 0.05219959533936151252, 26.25109039468566507 ) ) ;
#97580=CARTESIAN_POINT ( 'NONE',  ( 16.53943276465976808, 0.05219959533934440121, 81.25109039468568994 ) ) ;
#97581=CARTESIAN_POINT ( 'NONE',  ( -13.89961937509957401, -13.97604488694547875, 109.3760903946856331 ) ) ;
#97582=CARTESIAN_POINT ( 'NONE',  ( -14.34966873604960291, -8.224510206698953496, 111.6655762719810525 ) ) ;
#97583=CARTESIAN_POINT ( 'NONE',  ( 8.314922557961029526, -14.29746914071037800, 60.41775706135235424 ) ) ;
#97584=CARTESIAN_POINT ( 'NONE',  ( 14.34966873604972726, -8.224510206698740333, 50.83442372801901143 ) ) ;
#97585=CARTESIAN_POINT ( 'NONE',  ( -0.05219959533909027116, -19.03943276465977164, 27.49890960531435624 ) ) ;
#97586=CARTESIAN_POINT ( 'NONE',  ( 9.474510206698729675, 16.51473224551082808, 67.08442372801900433 ) ) ;
#97587=CARTESIAN_POINT ( 'NONE',  ( 13.97604488694548053, -13.89961937509957401, 20.62609039468567573 ) ) ;
#97588=CARTESIAN_POINT ( 'NONE',  ( 16.51473224551069308, 9.474510206698969483, 29.16557627198103475 ) ) ;
#97589=CARTESIAN_POINT ( 'NONE',  ( 19.05341960407611168, 5.049401038298154454, 73.95724293864768129 ) ) ;
#97590=CARTESIAN_POINT ( 'NONE',  ( 0.05219959533910956823, 16.53943276465976808, 74.99890960531435269 ) ) ;
#97591=CARTESIAN_POINT ( 'NONE',  ( 16.51473224551083163, -9.474510206698727899, 35.83442372801899722 ) ) ;
#97592=CARTESIAN_POINT ( 'NONE',  ( 5.823673210054125526, 21.52544592524343514, 39.79057627198103830 ) ) ;
#97593=CARTESIAN_POINT ( 'NONE',  ( -21.53943276465977519, -0.05219959533937600094, 113.7510903946856757 ) ) ;
#97594=CARTESIAN_POINT ( 'NONE',  ( -19.05341960407611168, -5.049401038298163336, 91.45724293864766707 ) ) ;
#97595=CARTESIAN_POINT ( 'NONE',  ( 5.823673210054444382, -21.52544592524334988, 110.2094237280190185 ) ) ;
#97596=CARTESIAN_POINT ( 'NONE',  ( 5.823673210054125526, 21.52544592524343514, 59.79057627198103120 ) ) ;
#97597=CARTESIAN_POINT ( 'NONE',  ( 13.89961937509977652, -13.97604488694527269, 98.12390960531433848 ) ) ;
#97598=CARTESIAN_POINT ( 'NONE',  ( 0.05219959533936267826, -19.03943276465977164, 80.00109039468567573 ) ) ;
#97599=CARTESIAN_POINT ( 'NONE',  ( 5.049401038298161559, -19.05341960407611168, 97.70724293864766707 ) ) ;
#97600=CARTESIAN_POINT ( 'NONE',  ( -19.05341960407617563, 5.049401038297882671, 93.54275706135234714 ) ) ;
#97601=CARTESIAN_POINT ( 'NONE',  ( -14.34966873604972548, 8.224510206698743886, 53.33442372801901854 ) ) ;
#97602=CARTESIAN_POINT ( 'NONE',  ( 16.46253265017160672, -9.564922557960803928, 23.33224293864769194 ) ) ;
#97603=CARTESIAN_POINT ( 'NONE',  ( -19.02544592524342804, 5.153800228976336051, 81.04057627198103830 ) ) ;
#97604=CARTESIAN_POINT ( 'NONE',  ( 15.72974639402199770, -15.80617190586745480, 58.12390960531435979 ) ) ;
#97605=CARTESIAN_POINT ( 'NONE',  ( -8.224510206698735004, -14.34966873604973081, 29.58442372801901854 ) ) ;
#97606=CARTESIAN_POINT ( 'NONE',  ( -18.62759615963255300, -10.81492255796106328, 29.16775706135234003 ) ) ;
#97607=CARTESIAN_POINT ( 'NONE',  ( 5.823673210054444382, -21.52544592524334988, 100.2094237280190043 ) ) ;
#97608=CARTESIAN_POINT ( 'NONE',  ( -0.05219959533934338120, 16.53943276465976808, 97.50109039468567573 ) ) ;
#97609=CARTESIAN_POINT ( 'NONE',  ( -19.03943276465977164, 0.05219959533909376836, 86.24890960531436690 ) ) ;
#97610=CARTESIAN_POINT ( 'NONE',  ( -16.53943276465976808, 0.05219959533911058130, 96.24890960531435269 ) ) ;
#97611=CARTESIAN_POINT ( 'NONE',  ( -16.55341960407617563, 4.379528057220093196, 113.5427570613523756 ) ) ;
#97612=CARTESIAN_POINT ( 'NONE',  ( 0.05219959533936267826, -19.03943276465977164, 75.00109039468566152 ) ) ;
#97613=CARTESIAN_POINT ( 'NONE',  ( -5.823673210054431948, 21.52544592524334988, 42.70942372801901854 ) ) ;
#97614=CARTESIAN_POINT ( 'NONE',  ( 8.224510206698953496, -14.34966873604960469, 87.91557627198103830 ) ) ;
#97615=CARTESIAN_POINT ( 'NONE',  ( -0.05219959533907301413, -21.53943276465977519, 22.49890960531436335 ) ) ;
#97616=CARTESIAN_POINT ( 'NONE',  ( 14.29746914071037800, 8.314922557961029526, 101.6677570613523613 ) ) ;
#97617=CARTESIAN_POINT ( 'NONE',  ( 21.53943276465977519, 0.05219959533937863772, 81.25109039468568994 ) ) ;
#97618=CARTESIAN_POINT ( 'NONE',  ( -16.55341960407617563, 4.379528057220093196, 43.54275706135235424 ) ) ;
#97619=CARTESIAN_POINT ( 'NONE',  ( 15.80617190586769283, -15.72974639402175789, 35.62609039468568994 ) ) ;
#97621=CARTESIAN_POINT ( 'NONE',  ( 21.55341960407610458, 5.719274019375980345, 113.9572429386477239 ) ) ;
#97622=CARTESIAN_POINT ( 'NONE',  ( -4.379528057220328563, 16.55341960407611168, 90.20724293864770971 ) ) ;
#97623=CARTESIAN_POINT ( 'NONE',  ( 17.50000000000001776, -3.345213924137293127, 27.08768623094348271 ) ) ;
#97624=CARTESIAN_POINT ( 'NONE',  ( -16.53943276465976808, 0.05219959533911058130, 71.24890960531435269 ) ) ;
#97625=CARTESIAN_POINT ( 'NONE',  ( -5.153800228976328057, -19.02544592524343514, 52.29057627198100988 ) ) ;
#97626=CARTESIAN_POINT ( 'NONE',  ( -4.379528057220086978, -16.55341960407618274, 109.7927570613523613 ) ) ;
#97627=CARTESIAN_POINT ( 'NONE',  ( 13.97604488694527802, 13.89961937509977652, 39.37390960531435269 ) ) ;
#97628=CARTESIAN_POINT ( 'NONE',  ( 15.80617190586746368, 15.72974639402197994, 49.37390960531436690 ) ) ;
#97629=CARTESIAN_POINT ( 'NONE',  ( 12.06949235617757843, -12.14591786802309237, 73.12390960531436690 ) ) ;
#97630=CARTESIAN_POINT ( 'NONE',  ( -21.55341960407610458, -5.719274019375992779, 86.45724293864770971 ) ) ;
#97631=CARTESIAN_POINT ( 'NONE',  ( 19.05341960407611168, 5.049401038298154454, 93.95724293864769550 ) ) ;
#97632=CARTESIAN_POINT ( 'NONE',  ( -9.564922557960796823, -16.46253265017161027, 32.08224293864769550 ) ) ;
#97633=CARTESIAN_POINT ( 'NONE',  ( -5.153800228976607833, 19.02544592524334988, 92.70942372801901854 ) ) ;
#97634=CARTESIAN_POINT ( 'NONE',  ( -10.72451020669898014, 18.67979575497178502, 35.41557627198102409 ) ) ;
#97635=CARTESIAN_POINT ( 'NONE',  ( 21.55341960407619695, -5.719274019375665929, 66.04275706135236135 ) ) ;
#97636=CARTESIAN_POINT ( 'NONE',  ( -19.05341960407611168, -5.049401038298163336, 56.45724293864768129 ) ) ;
#97637=CARTESIAN_POINT ( 'NONE',  ( 0.05219959533909260263, 19.03943276465977164, 89.99890960531436690 ) ) ;
#97639=CARTESIAN_POINT ( 'NONE',  ( -4.483927247898782831, 16.52544592524335698, 57.70942372801901143 ) ) ;
#97640=CARTESIAN_POINT ( 'NONE',  ( 10.81492255796106328, -18.62759615963255655, 45.41775706135234003 ) ) ;
#97641=CARTESIAN_POINT ( 'NONE',  ( -21.55341960407619339, 5.719274019375674811, 73.54275706135234714 ) ) ;
#97642=CARTESIAN_POINT ( 'NONE',  ( -9.474510206698964154, 16.51473224551069663, 115.4155762719810241 ) ) ;
#97643=CARTESIAN_POINT ( 'NONE',  ( -10.72451020669898014, 18.67979575497178502, 100.4155762719810241 ) ) ;
#97644=CARTESIAN_POINT ( 'NONE',  ( -5.823673210054431948, 21.52544592524334988, 42.70942372801901854 ) ) ;
#97645=CARTESIAN_POINT ( 'NONE',  ( -16.55341960407617563, 4.379528057220093196, 68.54275706135234714 ) ) ;
#97646=CARTESIAN_POINT ( 'NONE',  ( -10.81492255796078084, -18.62759615963271287, 67.08224293864770971 ) ) ;
#97647=CARTESIAN_POINT ( 'NONE',  ( 16.51473224551083163, -9.474510206698727899, 35.83442372801899722 ) ) ;
#97648=CARTESIAN_POINT ( 'NONE',  ( 5.153800228976335163, 19.02544592524342804, 69.79057627198103830 ) ) ;
#97649=CARTESIAN_POINT ( 'NONE',  ( -0.05219959533934338120, 16.53943276465976808, 107.5010903946856899 ) ) ;
#97650=CARTESIAN_POINT ( 'NONE',  ( 17.60728821186569704, -5.500000000000036415, 83.36690927743002533 ) ) ;
#97651=CARTESIAN_POINT ( 'NONE',  ( 5.049401038298161559, -19.05341960407611168, 102.7072429386476955 ) ) ;
#97652=CARTESIAN_POINT ( 'NONE',  ( -16.53943276465976808, -0.05219959533934237506, 43.75109039468568284 ) ) ;
#97655=CARTESIAN_POINT ( 'NONE',  ( -19.05341960407617563, 5.049401038297882671, 83.54275706135233293 ) ) ;
#97656=CARTESIAN_POINT ( 'NONE',  ( 15.80617190586746368, 15.72974639402197994, 59.37390960531436690 ) ) ;
#97657=CARTESIAN_POINT ( 'NONE',  ( -16.52544592524342804, 4.483927247898546575, 31.04057627198102409 ) ) ;
#97658=CARTESIAN_POINT ( 'NONE',  ( -9.474510206698720793, -16.51473224551083518, 99.58442372801900433 ) ) ;
#97660=CARTESIAN_POINT ( 'NONE',  ( 16.51473224551083163, -9.474510206698727899, 95.83442372801900433 ) ) ;
#97661=CARTESIAN_POINT ( 'NONE',  ( -21.55341960407610458, -5.719274019375992779, 91.45724293864769550 ) ) ;
#97662=CARTESIAN_POINT ( 'NONE',  ( -19.02544592524334988, -5.153800228976617603, 53.95942372801898301 ) ) ;
#97664=CARTESIAN_POINT ( 'NONE',  ( 9.564922557960805705, 16.46253265017160317, 69.58224293864770971 ) ) ;
#97665=CARTESIAN_POINT ( 'NONE',  ( 12.14591786802309770, 12.06949235617756955, 69.37390960531436690 ) ) ;
#97666=CARTESIAN_POINT ( 'NONE',  ( -0.05219959533909027116, -19.03943276465977164, 52.49890960531436690 ) ) ;
#97667=CARTESIAN_POINT ( 'NONE',  ( -8.314922557960811034, -14.29746914071050412, 47.08224293864770260 ) ) ;
#97670=CARTESIAN_POINT ( 'NONE',  ( -8.224510206698948167, 14.34966873604960824, 30.41557627198101699 ) ) ;
#97671=CARTESIAN_POINT ( 'NONE',  ( -19.02544592524342804, 5.153800228976336051, 61.04057627198103120 ) ) ;
#97673=CARTESIAN_POINT ( 'NONE',  ( -13.97604488694547697, 13.89961937509957934, 38.12609039468566152 ) ) ;
#97674=CARTESIAN_POINT ( 'NONE',  ( 4.379528057220092307, 16.55341960407617563, 42.29275706135235424 ) ) ;
#97675=CARTESIAN_POINT ( 'NONE',  ( 18.62759615963271287, -10.81492255796078972, 53.33224293864769550 ) ) ;
#97676=CARTESIAN_POINT ( 'NONE',  ( 18.67979575497194134, -10.72451020669871369, 100.8344237280190185 ) ) ;
#97677=CARTESIAN_POINT ( 'NONE',  ( 19.02544592524343514, -5.153800228976328945, 73.54057627198103830 ) ) ;
#97679=CARTESIAN_POINT ( 'NONE',  ( 16.51473224551069308, 9.474510206698969483, 109.1655762719810383 ) ) ;
#97681=CARTESIAN_POINT ( 'NONE',  ( 15.80617190586769283, -15.72974639402175789, 35.62609039468568994 ) ) ;
#97682=CARTESIAN_POINT ( 'NONE',  ( -8.314922557960811034, -14.29746914071050412, 97.08224293864770971 ) ) ;
#97683=CARTESIAN_POINT ( 'NONE',  ( 18.67979575497178502, 10.72451020669898547, 89.16557627198102409 ) ) ;
#97684=CARTESIAN_POINT ( 'NONE',  ( -5.153800228976328057, -19.02544592524343514, 77.29057627198099567 ) ) ;
#97686=CARTESIAN_POINT ( 'NONE',  ( -0.05219959533909027116, -19.03943276465977164, 87.49890960531436690 ) ) ;
#97687=CARTESIAN_POINT ( 'NONE',  ( 10.81492255796106328, -18.62759615963255655, 20.41775706135234714 ) ) ;
#97689=CARTESIAN_POINT ( 'NONE',  ( 19.03943276465977164, -0.05219959533909143690, 93.74890960531435269 ) ) ;
#97691=CARTESIAN_POINT ( 'NONE',  ( -13.89961937509977652, 13.97604488694528158, 30.62390960531435269 ) ) ;
#97692=CARTESIAN_POINT ( 'NONE',  ( -19.02544592524342804, 5.153800228976336051, 31.04057627198102409 ) ) ;
#97693=CARTESIAN_POINT ( 'NONE',  ( 19.05341960407617918, -5.049401038297876454, 111.0427570613523329 ) ) ;
#97695=CARTESIAN_POINT ( 'NONE',  ( -5.153800228976328057, -19.02544592524343514, 22.29057627198102765 ) ) ;
#97696=CARTESIAN_POINT ( 'NONE',  ( -21.52544592524334988, -5.823673210054445271, 68.95942372801901854 ) ) ;
#97697=CARTESIAN_POINT ( 'NONE',  ( 5.049401038298161559, -19.05341960407611168, 67.70724293864769550 ) ) ;
#97698=CARTESIAN_POINT ( 'NONE',  ( 15.80617190586769283, -15.72974639402175789, 30.62609039468567929 ) ) ;
#97699=CARTESIAN_POINT ( 'NONE',  ( 21.52544592524344225, -5.823673210054117533, 108.5405762719810241 ) ) ;
#97701=CARTESIAN_POINT ( 'NONE',  ( -13.89961937509977652, 13.97604488694528158, 85.62390960531433848 ) ) ;
#97703=CARTESIAN_POINT ( 'NONE',  ( -0.05219959533934338120, 16.53943276465976808, 22.50109039468567573 ) ) ;
#97704=CARTESIAN_POINT ( 'NONE',  ( 21.52544592524344225, -5.823673210054117533, 48.54057627198103120 ) ) ;
#97705=CARTESIAN_POINT ( 'NONE',  ( -18.67979575497193778, 10.72451020669871902, 68.33442372801900433 ) ) ;
#97706=CARTESIAN_POINT ( 'NONE',  ( -13.89961937509977652, 13.97604488694528158, 110.6239096053143243 ) ) ;
#97707=CARTESIAN_POINT ( 'NONE',  ( 9.564922557961047289, -16.46253265017146816, 90.41775706135234714 ) ) ;
#97708=CARTESIAN_POINT ( 'NONE',  ( -19.02544592524342804, 5.153800228976336051, 66.04057627198103830 ) ) ;
#97709=CARTESIAN_POINT ( 'NONE',  ( -19.03943276465977164, 0.05219959533909376836, 86.24890960531436690 ) ) ;
#97710=CARTESIAN_POINT ( 'NONE',  ( 8.224510206698953496, -14.34966873604960469, 87.91557627198103830 ) ) ;
#97711=CARTESIAN_POINT ( 'NONE',  ( -16.55341960407611168, -4.379528057220339221, 86.45724293864770971 ) ) ;
#97712=CARTESIAN_POINT ( 'NONE',  ( 5.719274019375991003, -21.55341960407610458, 22.70724293864769194 ) ) ;
#97713=CARTESIAN_POINT ( 'NONE',  ( -16.52544592524342804, 4.483927247898546575, 56.04057627198102409 ) ) ;
#97714=( BOUNDED_CURVE ( )  B_SPLINE_CURVE ( 2, ( #160196, #142031, #21686, #126854, #99512, #51027, #83339, #161193, #22689, #188560, #50039, #84336, #112688 ),
 .UNSPECIFIED., .F., .F. ) 
 B_SPLINE_CURVE_WITH_KNOTS ( ( 3, 2, 2, 2, 2, 2, 3 ),
 ( 0.6866409627428347040, 0.6885964912280702066, 0.6929824561403509220, 0.6973684210526315264, 0.7017543859649122417, 0.7061403508771929571, 0.7080501995403384319 ),
 .UNSPECIFIED. ) 
 CURVE ( )  GEOMETRIC_REPRESENTATION_ITEM ( )  RATIONAL_B_SPLINE_CURVE ( ( 0.9831626618144007068, 0.9848076720550096308, 1.000000000000000000, 0.9659258262890683122, 1.000000000000000000, 0.9659258262890683122, 1.000000000000000000, 0.9659258262890683122, 1.000000000000000000, 0.9659258262890683122, 1.000000000000000000, 0.9851625545550091179, 0.9832469066685282089 ) ) 
 REPRESENTATION_ITEM ( '' )  );
#97715=CARTESIAN_POINT ( 'NONE',  ( -5.153800228976328057, -19.02544592524343514, 37.29057627198102409 ) ) ;
#97716=CARTESIAN_POINT ( 'NONE',  ( -21.52544592524334988, -5.823673210054445271, 63.95942372801901854 ) ) ;
#97717=CARTESIAN_POINT ( 'NONE',  ( 9.474510206698729675, 16.51473224551082808, 87.08442372801900433 ) ) ;
#97718=CARTESIAN_POINT ( 'NONE',  ( -16.53943276465976808, 0.05219959533911058130, 61.24890960531435979 ) ) ;
#97719=CARTESIAN_POINT ( 'NONE',  ( -21.53943276465977519, 0.05219959533907696930, 111.2489096053143669 ) ) ;
#97720=CARTESIAN_POINT ( 'NONE',  ( 5.823673210054125526, 21.52544592524343514, 44.79057627198103120 ) ) ;
#97721=CARTESIAN_POINT ( 'NONE',  ( 19.02544592524343514, -5.153800228976328945, 113.5405762719810241 ) ) ;
#97723=CARTESIAN_POINT ( 'NONE',  ( -16.46253265017160317, 9.564922557960807481, 60.83224293864769550 ) ) ;
#97724=CARTESIAN_POINT ( 'NONE',  ( 8.224510206698953496, -14.34966873604960469, 32.91557627198102409 ) ) ;
#97725=CARTESIAN_POINT ( 'NONE',  ( -12.14591786802326823, 12.06949235617739902, 98.12609039468570415 ) ) ;
#97726=CARTESIAN_POINT ( 'NONE',  ( -16.53943276465976808, -0.05219959533934237506, 83.75109039468568994 ) ) ;
#97727=CARTESIAN_POINT ( 'NONE',  ( -5.153800228976607833, 19.02544592524334988, 42.70942372801901143 ) ) ;
#97729=CARTESIAN_POINT ( 'NONE',  ( -13.97604488694527625, -13.89961937509977652, 91.87390960531432427 ) ) ;
#97730=CARTESIAN_POINT ( 'NONE',  ( -19.05341960407611168, -5.049401038298163336, 46.45724293864768129 ) ) ;
#97732=CARTESIAN_POINT ( 'NONE',  ( -0.05219959533910754901, -16.53943276465976808, 57.49890960531435979 ) ) ;
#97733=CARTESIAN_POINT ( 'NONE',  ( 19.02544592524343514, -5.153800228976328945, 23.54057627198102054 ) ) ;
#97734=CARTESIAN_POINT ( 'NONE',  ( 19.03943276465977164, -0.05219959533909143690, 113.7489096053143669 ) ) ;
#97735=CARTESIAN_POINT ( 'NONE',  ( 18.62759615963271287, -10.81492255796078972, 43.33224293864769550 ) ) ;
#97736=CARTESIAN_POINT ( 'NONE',  ( 4.483927247898545687, 16.52544592524342804, 84.79057627198102409 ) ) ;
#97737=CARTESIAN_POINT ( 'NONE',  ( 0.05219959533934541429, -16.53943276465976808, 45.00109039468568284 ) ) ;
#97739=CARTESIAN_POINT ( 'NONE',  ( 16.53943276465976808, -0.05219959533910856209, 78.74890960531436690 ) ) ;
#97741=CARTESIAN_POINT ( 'NONE',  ( -19.03943276465977164, -0.05219959533935918106, 78.75109039468567573 ) ) ;
#97742=CARTESIAN_POINT ( 'NONE',  ( -5.153800228976328057, -19.02544592524343514, 112.2905762719810099 ) ) ;
#97745=CARTESIAN_POINT ( 'NONE',  ( 18.52568451169417685, 5.499999999999960920, 101.4787647167951548 ) ) ;
#97746=CARTESIAN_POINT ( 'NONE',  ( -16.53943276465976808, -0.05219959533934237506, 23.75109039468567929 ) ) ;
#97747=CARTESIAN_POINT ( 'NONE',  ( -12.06949235617739369, -12.14591786802326823, 104.3760903946856899 ) ) ;
#97748=CARTESIAN_POINT ( 'NONE',  ( 0.05219959533936267826, -19.03943276465977164, 75.00109039468566152 ) ) ;
#97749=CARTESIAN_POINT ( 'NONE',  ( -10.72451020669898014, 18.67979575497178502, 50.41557627198103120 ) ) ;
#97750=CARTESIAN_POINT ( 'NONE',  ( 21.55341960407619695, -5.719274019375665929, 71.04275706135234714 ) ) ;
#97752=CARTESIAN_POINT ( 'NONE',  ( -16.52544592524335698, -4.483927247898792601, 28.95942372801902209 ) ) ;
#97753=CARTESIAN_POINT ( 'NONE',  ( -0.05219959533909027116, -19.03943276465977164, 27.49890960531435624 ) ) ;
#97754=CARTESIAN_POINT ( 'NONE',  ( 19.03943276465977164, -0.05219959533909143690, 93.74890960531435269 ) ) ;
#97755=CARTESIAN_POINT ( 'NONE',  ( 13.97604488694527802, 13.89961937509977652, 24.37390960531435624 ) ) ;
#97756=CARTESIAN_POINT ( 'NONE',  ( -12.14591786802309592, -12.06949235617757132, 91.87390960531436690 ) ) ;
#97758=CARTESIAN_POINT ( 'NONE',  ( -19.03943276465977164, 0.05219959533909376836, 101.2489096053143669 ) ) ;
#97760=CARTESIAN_POINT ( 'NONE',  ( 13.97604488694548053, -13.89961937509957401, 110.6260903946856615 ) ) ;
#97761=CARTESIAN_POINT ( 'NONE',  ( -10.81492255796078084, -18.62759615963271287, 72.08224293864769550 ) ) ;
#97762=CARTESIAN_POINT ( 'NONE',  ( -16.51473224551069308, -9.474510206698971260, 46.66557627198102409 ) ) ;
#97763=CARTESIAN_POINT ( 'NONE',  ( 9.474510206698729675, 16.51473224551082808, 72.08442372801900433 ) ) ;
#97764=CARTESIAN_POINT ( 'NONE',  ( -21.52544592524343514, 5.823673210054127303, 111.0405762719810525 ) ) ;
#97765=CARTESIAN_POINT ( 'NONE',  ( -5.049401038298153566, 19.05341960407611168, 75.20724293864769550 ) ) ;
#97766=CARTESIAN_POINT ( 'NONE',  ( -0.05219959533909027116, -19.03943276465977164, 107.4989096053143527 ) ) ;
#97768=CARTESIAN_POINT ( 'NONE',  ( 8.314922557961029526, -14.29746914071037800, 35.41775706135234003 ) ) ;
#97769=CARTESIAN_POINT ( 'NONE',  ( -15.80617190586745835, -15.72974639402198527, 96.87390960531436690 ) ) ;
#97770=CARTESIAN_POINT ( 'NONE',  ( -14.29746914071049879, 8.314922557960819915, 105.8322429386476955 ) ) ;
#97771=CARTESIAN_POINT ( 'NONE',  ( 0.05219959533909260263, 19.03943276465977164, 99.99890960531436690 ) ) ;
#97772=CARTESIAN_POINT ( 'NONE',  ( 19.03943276465977164, 0.05219959533936151252, 56.25109039468566863 ) ) ;
#97773=CARTESIAN_POINT ( 'NONE',  ( 15.72974639402199770, -15.80617190586745480, 93.12390960531436690 ) ) ;
#97774=CARTESIAN_POINT ( 'NONE',  ( -8.314922557960811034, -14.29746914071050412, 42.08224293864769550 ) ) ;
#97775=CARTESIAN_POINT ( 'NONE',  ( 16.46253265017146816, 9.564922557961045513, 21.66775706135233648 ) ) ;
#97776=CARTESIAN_POINT ( 'NONE',  ( -14.34966873604972548, 8.224510206698743886, 68.33442372801900433 ) ) ;
#97777=CARTESIAN_POINT ( 'NONE',  ( 19.02544592524343514, -5.153800228976328945, 88.54057627198102409 ) ) ;
#97778=CARTESIAN_POINT ( 'NONE',  ( 9.474510206698971260, -16.51473224551069308, 47.91557627198102409 ) ) ;
#97779=CARTESIAN_POINT ( 'NONE',  ( -21.55341960407619339, 5.719274019375674811, 48.54275706135234714 ) ) ;
#97780=CARTESIAN_POINT ( 'NONE',  ( 15.72974639402176855, 15.80617190586768217, 66.87609039468568994 ) ) ;
#97781=CARTESIAN_POINT ( 'NONE',  ( -16.51473224551069308, -9.474510206698971260, 56.66557627198103120 ) ) ;
#97782=CARTESIAN_POINT ( 'NONE',  ( 18.62759615963255655, 10.81492255796105972, 36.66775706135234714 ) ) ;
#97783=CARTESIAN_POINT ( 'NONE',  ( -19.05341960407617563, 5.049401038297882671, 68.54275706135230450 ) ) ;
#97784=CARTESIAN_POINT ( 'NONE',  ( -19.05341960407617563, 5.049401038297882671, 78.54275706135233293 ) ) ;
#97785=CARTESIAN_POINT ( 'NONE',  ( -16.46253265017160317, 9.564922557960807481, 45.83224293864769550 ) ) ;
#97786=CARTESIAN_POINT ( 'NONE',  ( -0.05219959533934338120, 16.53943276465976808, 92.50109039468567573 ) ) ;
#97787=CARTESIAN_POINT ( 'NONE',  ( 13.97604488694527802, 13.89961937509977652, 49.37390960531434558 ) ) ;
#97788=CARTESIAN_POINT ( 'NONE',  ( 9.474510206698971260, -16.51473224551069308, 22.91557627198102765 ) ) ;
#97789=CARTESIAN_POINT ( 'NONE',  ( -19.05341960407611168, -5.049401038298163336, 101.4572429386476955 ) ) ;
#97790=CARTESIAN_POINT ( 'NONE',  ( 9.474510206698971260, -16.51473224551069308, 32.91557627198102409 ) ) ;
#97791=CARTESIAN_POINT ( 'NONE',  ( -10.72451020669898014, 18.67979575497178502, 90.41557627198103830 ) ) ;
#97792=CARTESIAN_POINT ( 'NONE',  ( -16.55341960407617563, 4.379528057220093196, 78.54275706135236135 ) ) ;
#97794=CARTESIAN_POINT ( 'NONE',  ( 19.03943276465977164, 0.05219959533936151252, 26.25109039468566507 ) ) ;
#97795=CARTESIAN_POINT ( 'NONE',  ( -19.03943276465977164, 0.05219959533909376836, 56.24890960531435979 ) ) ;
#97796=CARTESIAN_POINT ( 'NONE',  ( -14.29746914071049879, 8.314922557960819915, 40.83224293864769550 ) ) ;
#97797=CARTESIAN_POINT ( 'NONE',  ( 0.05219959533910956823, 16.53943276465976808, 74.99890960531435269 ) ) ;
#97798=CARTESIAN_POINT ( 'NONE',  ( -16.51473224551069308, -9.474510206698971260, 96.66557627198102409 ) ) ;
#97799=CARTESIAN_POINT ( 'NONE',  ( 13.97604488694527802, 13.89961937509977652, 79.37390960531435269 ) ) ;
#97800=CARTESIAN_POINT ( 'NONE',  ( -15.80617190586768217, 15.72974639402176855, 48.12609039468568284 ) ) ;
#97801=CARTESIAN_POINT ( 'NONE',  ( -13.89961937509977652, 13.97604488694528158, 90.62390960531432427 ) ) ;
#97802=CARTESIAN_POINT ( 'NONE',  ( 0.05219959533937995610, -21.53943276465977519, 105.0010903946856757 ) ) ;
#97803=CARTESIAN_POINT ( 'NONE',  ( 16.55341960407618274, -4.379528057220086978, 76.04275706135237556 ) ) ;
#97804=CARTESIAN_POINT ( 'NONE',  ( -21.52544592524334988, -5.823673210054445271, 23.95942372801901143 ) ) ;
#97805=CARTESIAN_POINT ( 'NONE',  ( 15.80617190586746368, 15.72974639402197994, 84.37390960531438111 ) ) ;
#97806=CARTESIAN_POINT ( 'NONE',  ( 8.224510206698953496, -14.34966873604960469, 52.91557627198103830 ) ) ;
#97807=CARTESIAN_POINT ( 'NONE',  ( -9.564922557960796823, -16.46253265017161027, 42.08224293864769550 ) ) ;
#97808=CARTESIAN_POINT ( 'NONE',  ( -16.53943276465976808, 0.05219959533911058130, 71.24890960531435269 ) ) ;
#97809=CARTESIAN_POINT ( 'NONE',  ( -15.72974639402197994, 15.80617190586746368, 30.62390960531436335 ) ) ;
#97810=CARTESIAN_POINT ( 'NONE',  ( 16.51473224551083163, -9.474510206698727899, 35.83442372801899722 ) ) ;
#97811=CARTESIAN_POINT ( 'NONE',  ( 16.52544592524342804, -4.483927247898539470, 103.5405762719810383 ) ) ;
#97812=ORIENTED_EDGE ( 'NONE', *, *, #85603, .T. ) ;
#97813=CARTESIAN_POINT ( 'NONE',  ( 12.06949235617739724, 12.14591786802326823, 61.87609039468568284 ) ) ;
#97814=CARTESIAN_POINT ( 'NONE',  ( -19.02544592524342804, 5.153800228976336051, 71.04057627198099567 ) ) ;
#97816=CARTESIAN_POINT ( 'NONE',  ( -18.67979575497178146, -10.72451020669898902, 36.66557627198103120 ) ) ;
#97817=CARTESIAN_POINT ( 'NONE',  ( 12.06949235617739724, 12.14591786802326823, 96.87609039468568994 ) ) ;
#97818=CARTESIAN_POINT ( 'NONE',  ( 0.05219959533934541429, -16.53943276465976808, 20.00109039468568639 ) ) ;
#97819=CARTESIAN_POINT ( 'NONE',  ( -21.53943276465977519, -0.05219959533937600094, 78.75109039468568994 ) ) ;
#97820=CARTESIAN_POINT ( 'NONE',  ( -19.03943276465977164, 0.05219959533909376836, 76.24890960531435269 ) ) ;
#97821=CARTESIAN_POINT ( 'NONE',  ( 18.62759615963271287, -10.81492255796078972, 108.3322429386477097 ) ) ;
#97822=CARTESIAN_POINT ( 'NONE',  ( 4.483927247898790824, -16.52544592524335698, 55.20942372801902565 ) ) ;
#97823=CARTESIAN_POINT ( 'NONE',  ( 4.379528057220339221, -16.55341960407611168, 112.7072429386476955 ) ) ;
#97824=CARTESIAN_POINT ( 'NONE',  ( 0.05219959533934541429, -16.53943276465976808, 20.00109039468568639 ) ) ;
#97825=CARTESIAN_POINT ( 'NONE',  ( 5.049401038297881783, 19.05341960407617563, 82.29275706135229029 ) ) ;
#97826=EDGE_CURVE ( 'NONE', #53699, #123077, #109237, .T. ) ;
#97827=CARTESIAN_POINT ( 'NONE',  ( 0.05219959533907565091, 21.53943276465977519, 74.99890960531435269 ) ) ;
#97828=CARTESIAN_POINT ( 'NONE',  ( 19.02544592524334988, 5.153800228976608722, 56.45942372801898301 ) ) ;
#97830=CARTESIAN_POINT ( 'NONE',  ( 0.05219959533907565091, 21.53943276465977519, 109.9989096053143527 ) ) ;
#97832=CARTESIAN_POINT ( 'NONE',  ( 19.03943276465977164, -0.05219959533909143690, 78.74890960531436690 ) ) ;
#97834=CARTESIAN_POINT ( 'NONE',  ( 12.06949235617739724, 12.14591786802326823, 36.87609039468568994 ) ) ;
#97836=CARTESIAN_POINT ( 'NONE',  ( 18.67979575497178502, 10.72451020669898547, 104.1655762719810241 ) ) ;
#97837=CARTESIAN_POINT ( 'NONE',  ( 16.53943276465976808, -0.05219959533910856209, 63.74890960531435979 ) ) ;
#97838=CARTESIAN_POINT ( 'NONE',  ( 19.03943276465977164, -0.05219959533909143690, 63.74890960531435979 ) ) ;
#97839=CARTESIAN_POINT ( 'NONE',  ( -21.55341960407619339, 5.719274019375674811, 93.54275706135234714 ) ) ;
#97840=CARTESIAN_POINT ( 'NONE',  ( -4.483927247898782831, 16.52544592524335698, 32.70942372801900433 ) ) ;
#97841=CARTESIAN_POINT ( 'NONE',  ( 5.153800228976615827, -19.02544592524334988, 40.20942372801898301 ) ) ;
#97842=CARTESIAN_POINT ( 'NONE',  ( 15.72974639402176855, 15.80617190586768217, 46.87609039468568994 ) ) ;
#97843=CARTESIAN_POINT ( 'NONE',  ( 21.55341960407610458, 5.719274019375980345, 63.95724293864770260 ) ) ;
#97844=CARTESIAN_POINT ( 'NONE',  ( -19.05341960407617563, 5.049401038297882671, 113.5427570613523471 ) ) ;
#97845=CARTESIAN_POINT ( 'NONE',  ( -9.564922557960796823, -16.46253265017161027, 62.08224293864769550 ) ) ;
#97846=CARTESIAN_POINT ( 'NONE',  ( 16.51473224551083163, -9.474510206698727899, 65.83442372801900433 ) ) ;
#97847=CARTESIAN_POINT ( 'NONE',  ( -0.05219959533937732626, 21.53943276465977519, 82.50109039468568994 ) ) ;
#97848=CARTESIAN_POINT ( 'NONE',  ( -9.564922557961040184, 16.46253265017147172, 72.91775706135233293 ) ) ;
#97849=CARTESIAN_POINT ( 'NONE',  ( -9.564922557960796823, -16.46253265017161027, 32.08224293864769550 ) ) ;
#97850=CARTESIAN_POINT ( 'NONE',  ( 10.81492255796078972, 18.62759615963270932, 54.58224293864769550 ) ) ;
#97851=CARTESIAN_POINT ( 'NONE',  ( -16.53943276465976808, 0.05219959533911058130, 66.24890960531436690 ) ) ;
#97853=CARTESIAN_POINT ( 'NONE',  ( -19.05341960407617563, 5.049401038297882671, 33.54275706135231871 ) ) ;
#97854=CARTESIAN_POINT ( 'NONE',  ( -4.379528057220086978, -16.55341960407618274, 84.79275706135234714 ) ) ;
#97855=CARTESIAN_POINT ( 'NONE',  ( 14.29746914071049879, -8.314922557960816363, 48.33224293864770260 ) ) ;
#97856=CARTESIAN_POINT ( 'NONE',  ( -18.67979575497193778, 10.72451020669871902, 88.33442372801901854 ) ) ;
#97857=CARTESIAN_POINT ( 'NONE',  ( -5.823673210054431948, 21.52544592524334988, 82.70942372801900433 ) ) ;
#97858=CARTESIAN_POINT ( 'NONE',  ( 5.823673210054125526, 21.52544592524343514, 89.79057627198103830 ) ) ;
#97859=CARTESIAN_POINT ( 'NONE',  ( -5.153800228976328057, -19.02544592524343514, 47.29057627198102409 ) ) ;
#97860=CARTESIAN_POINT ( 'NONE',  ( 5.719274019375673035, 21.55341960407619339, 52.29275706135236135 ) ) ;
#97861=CARTESIAN_POINT ( 'NONE',  ( 9.474510206698971260, -16.51473224551069308, 37.91557627198102409 ) ) ;
#97862=CARTESIAN_POINT ( 'NONE',  ( -9.474510206698964154, 16.51473224551069663, 70.41557627198102409 ) ) ;
#97863=CARTESIAN_POINT ( 'NONE',  ( 8.314922557960818139, 14.29746914071049879, 109.5822429386476955 ) ) ;
#97864=CARTESIAN_POINT ( 'NONE',  ( 13.89961937509977652, -13.97604488694527269, 98.12390960531433848 ) ) ;
#97865=CARTESIAN_POINT ( 'NONE',  ( 16.55341960407611168, 4.379528057220329451, 48.95724293864770971 ) ) ;
#97866=CARTESIAN_POINT ( 'NONE',  ( 14.34966873604960469, 8.224510206698951720, 109.1655762719810383 ) ) ;
#97867=CARTESIAN_POINT ( 'NONE',  ( 21.55341960407610458, 5.719274019375980345, 83.95724293864770971 ) ) ;
#97868=CARTESIAN_POINT ( 'NONE',  ( 15.72974639402176855, 15.80617190586768217, 36.87609039468568994 ) ) ;
#97870=CARTESIAN_POINT ( 'NONE',  ( -4.483927247898782831, 16.52544592524335698, 42.70942372801901854 ) ) ;
#97871=CARTESIAN_POINT ( 'NONE',  ( 10.81492255796078972, 18.62759615963270932, 79.58224293864769550 ) ) ;
#97872=CARTESIAN_POINT ( 'NONE',  ( 18.62759615963255655, 10.81492255796105972, 101.6677570613523613 ) ) ;
#97873=CARTESIAN_POINT ( 'NONE',  ( 9.564922557960805705, 16.46253265017160317, 94.58224293864769550 ) ) ;
#97874=CARTESIAN_POINT ( 'NONE',  ( 21.53943276465977519, 0.05219959533937863772, 31.25109039468568639 ) ) ;
#97876=CARTESIAN_POINT ( 'NONE',  ( 5.719274019375991003, -21.55341960407610458, 32.70724293864770260 ) ) ;
#97877=CARTESIAN_POINT ( 'NONE',  ( 14.34966873604972726, -8.224510206698740333, 100.8344237280190185 ) ) ;
#97878=CARTESIAN_POINT ( 'NONE',  ( -10.81492255796105439, 18.62759615963255655, 47.91775706135234714 ) ) ;
#97879=CARTESIAN_POINT ( 'NONE',  ( -18.62759615963255300, -10.81492255796106328, 79.16775706135234714 ) ) ;
#97880=CARTESIAN_POINT ( 'NONE',  ( 15.80617190586769283, -15.72974639402175789, 110.6260903946857042 ) ) ;
#97881=CARTESIAN_POINT ( 'NONE',  ( -16.52544592524335698, -4.483927247898792601, 78.95942372801901854 ) ) ;
#97882=CARTESIAN_POINT ( 'NONE',  ( -21.52544592524334988, -5.823673210054445271, 43.95942372801902565 ) ) ;
#97883=CARTESIAN_POINT ( 'NONE',  ( 16.46253265017160672, -9.564922557960803928, 28.33224293864769550 ) ) ;
#97884=CARTESIAN_POINT ( 'NONE',  ( -0.05219959533937732626, 21.53943276465977519, 97.50109039468567573 ) ) ;
#97885=CARTESIAN_POINT ( 'NONE',  ( -9.474510206698964154, 16.51473224551069663, 100.4155762719810241 ) ) ;
#97886=CARTESIAN_POINT ( 'NONE',  ( 15.72974639402199770, -15.80617190586745480, 103.1239096053143811 ) ) ;
#97888=CARTESIAN_POINT ( 'NONE',  ( 21.53943276465977519, -0.05219959533907433946, 68.74890960531435269 ) ) ;
#97889=CARTESIAN_POINT ( 'NONE',  ( 14.29746914071037800, 8.314922557961029526, 56.66775706135235424 ) ) ;
#97890=CARTESIAN_POINT ( 'NONE',  ( 16.55341960407611168, 4.379528057220329451, 48.95724293864770971 ) ) ;
#97892=CARTESIAN_POINT ( 'NONE',  ( 16.51473224551083163, -9.474510206698727899, 90.83442372801900433 ) ) ;
#97895=CARTESIAN_POINT ( 'NONE',  ( -12.14591786802326823, 12.06949235617739902, 28.12609039468568284 ) ) ;
#97896=CARTESIAN_POINT ( 'NONE',  ( 5.719274019375991003, -21.55341960407610458, 97.70724293864772392 ) ) ;
#97897=CARTESIAN_POINT ( 'NONE',  ( -18.62759615963270932, 10.81492255796079327, 75.83224293864769550 ) ) ;
#97898=CARTESIAN_POINT ( 'NONE',  ( 19.05341960407611168, 5.049401038298154454, 113.9572429386477097 ) ) ;
#97899=CARTESIAN_POINT ( 'NONE',  ( 16.53943276465976808, 0.05219959533934440121, 41.25109039468568284 ) ) ;
#97900=CARTESIAN_POINT ( 'NONE',  ( -13.89961937509977652, 13.97604488694528158, 60.62390960531436690 ) ) ;
#97901=CARTESIAN_POINT ( 'NONE',  ( 0.05219959533937995610, -21.53943276465977519, 35.00109039468568284 ) ) ;
#97902=CARTESIAN_POINT ( 'NONE',  ( 0.05219959533936267826, -19.03943276465977164, 100.0010903946856757 ) ) ;
#97903=CARTESIAN_POINT ( 'NONE',  ( -9.474510206698964154, 16.51473224551069663, 110.4155762719810383 ) ) ;
#97904=CARTESIAN_POINT ( 'NONE',  ( -19.03943276465977164, 0.05219959533909376836, 81.24890960531436690 ) ) ;
#97905=CARTESIAN_POINT ( 'NONE',  ( -10.81492255796078084, -18.62759615963271287, 92.08224293864769550 ) ) ;
#97906=CARTESIAN_POINT ( 'NONE',  ( -0.05219959533909027116, -19.03943276465977164, 57.49890960531435979 ) ) ;
#97908=CARTESIAN_POINT ( 'NONE',  ( -14.29746914071049879, 8.314922557960819915, 70.83224293864770971 ) ) ;
#97909=CARTESIAN_POINT ( 'NONE',  ( -19.05341960407611168, -5.049401038298163336, 101.4572429386476955 ) ) ;
#97911=CARTESIAN_POINT ( 'NONE',  ( 5.049401038297881783, 19.05341960407617563, 72.29275706135234714 ) ) ;
#97912=CARTESIAN_POINT ( 'NONE',  ( 10.72451020669898902, -18.67979575497178502, 87.91557627198103830 ) ) ;
#97913=CARTESIAN_POINT ( 'NONE',  ( 19.05341960407617918, -5.049401038297876454, 56.04275706135234714 ) ) ;
#97914=CARTESIAN_POINT ( 'NONE',  ( 16.46253265017160672, -9.564922557960803928, 113.3322429386476955 ) ) ;
#97916=CARTESIAN_POINT ( 'NONE',  ( -21.53943276465977519, 0.05219959533907696930, 51.24890960531436690 ) ) ;
#97917=CARTESIAN_POINT ( 'NONE',  ( 5.153800228976335163, 19.02544592524342804, 84.79057627198099567 ) ) ;
#97918=CARTESIAN_POINT ( 'NONE',  ( 0.05219959533937995610, -21.53943276465977519, 80.00109039468568994 ) ) ;
#97919=CARTESIAN_POINT ( 'NONE',  ( -19.02544592524342804, 5.153800228976336051, 41.04057627198103120 ) ) ;
#97920=EDGE_CURVE ( 'NONE', #86773, #2480, #7894, .T. ) ;
#97921=CARTESIAN_POINT ( 'NONE',  ( 16.55341960407611168, 4.379528057220329451, 68.95724293864769550 ) ) ;
#97922=CARTESIAN_POINT ( 'NONE',  ( -16.52544592524335698, -4.483927247898792601, 28.95942372801902209 ) ) ;
#97923=CARTESIAN_POINT ( 'NONE',  ( 18.67979575497194134, -10.72451020669871369, 60.83442372801901854 ) ) ;
#97925=CARTESIAN_POINT ( 'NONE',  ( -16.46253265017146816, -9.564922557961047289, 24.16775706135233648 ) ) ;
#97926=CARTESIAN_POINT ( 'NONE',  ( 0.05219959533936267826, -19.03943276465977164, 75.00109039468566152 ) ) ;
#97928=CARTESIAN_POINT ( 'NONE',  ( 18.67979575497194134, -10.72451020669871369, 20.83442372801901143 ) ) ;
#97929=CARTESIAN_POINT ( 'NONE',  ( -19.34837522270366250, -5.499999999999742428, 45.86337684832577111 ) ) ;
#97930=CARTESIAN_POINT ( 'NONE',  ( 9.564922557961047289, -16.46253265017146816, 25.41775706135234003 ) ) ;
#97931=CARTESIAN_POINT ( 'NONE',  ( -9.474510206698964154, 16.51473224551069663, 55.41557627198103120 ) ) ;
#97932=CARTESIAN_POINT ( 'NONE',  ( -9.474510206698720793, -16.51473224551083518, 29.58442372801900433 ) ) ;
#97933=CARTESIAN_POINT ( 'NONE',  ( 8.224510206698742110, 14.34966873604972548, 102.0844237280190185 ) ) ;
#97934=CARTESIAN_POINT ( 'NONE',  ( 9.474510206698971260, -16.51473224551069308, 97.91557627198102409 ) ) ;
#97935=CARTESIAN_POINT ( 'NONE',  ( -15.80617190586768217, 15.72974639402176855, 68.12609039468567573 ) ) ;
#97938=CARTESIAN_POINT ( 'NONE',  ( -5.823673210054431948, 21.52544592524334988, 87.70942372801901854 ) ) ;
#97939=CARTESIAN_POINT ( 'NONE',  ( 21.53943276465977519, 0.05219959533937863772, 106.2510903946856757 ) ) ;
#97942=CARTESIAN_POINT ( 'NONE',  ( -0.05219959533909027116, -19.03943276465977164, 102.4989096053143669 ) ) ;
#97943=CARTESIAN_POINT ( 'NONE',  ( 16.51473224551083163, -9.474510206698727899, 20.83442372801899722 ) ) ;
#97944=SPHERICAL_SURFACE ( 'NONE', #50200, 2.000000000000000000 ) ;
#97945=CARTESIAN_POINT ( 'NONE',  ( 19.02544592524343514, -5.153800228976328945, 38.54057627198103120 ) ) ;
#97946=CARTESIAN_POINT ( 'NONE',  ( -18.67979575497178146, -10.72451020669898902, 61.66557627198103120 ) ) ;
#97947=CARTESIAN_POINT ( 'NONE',  ( 14.29746914071049879, -8.314922557960816363, 23.33224293864769194 ) ) ;
#97948=CARTESIAN_POINT ( 'NONE',  ( -12.14591786802309592, -12.06949235617757132, 91.87390960531436690 ) ) ;
#97949=CARTESIAN_POINT ( 'NONE',  ( -19.02544592524342804, 5.153800228976336051, 81.04057627198103830 ) ) ;
#97950=CARTESIAN_POINT ( 'NONE',  ( 0.05219959533937995610, -21.53943276465977519, 110.0010903946856757 ) ) ;
#97951=CARTESIAN_POINT ( 'NONE',  ( 16.46253265017160672, -9.564922557960803928, 43.33224293864769550 ) ) ;
#97952=CARTESIAN_POINT ( 'NONE',  ( -14.29746914071049879, 8.314922557960819915, 105.8322429386476955 ) ) ;
#97953=CARTESIAN_POINT ( 'NONE',  ( 5.823673210054444382, -21.52544592524334988, 55.20942372801902565 ) ) ;
#97954=CARTESIAN_POINT ( 'NONE',  ( 5.719274019375991003, -21.55341960407610458, 92.70724293864770971 ) ) ;
#97955=CARTESIAN_POINT ( 'NONE',  ( 5.049401038297881783, 19.05341960407617563, 57.29275706135231871 ) ) ;
#97957=CARTESIAN_POINT ( 'NONE',  ( -19.02544592524342804, 5.153800228976336051, 116.0405762719810383 ) ) ;
#97958=CARTESIAN_POINT ( 'NONE',  ( 16.52544592524342804, -4.483927247898539470, 78.54057627198103830 ) ) ;
#97959=CARTESIAN_POINT ( 'NONE',  ( 16.51473224551083163, -9.474510206698727899, 50.83442372801899722 ) ) ;
#97960=CARTESIAN_POINT ( 'NONE',  ( 13.97604488694527802, 13.89961937509977652, 59.37390960531434558 ) ) ;
#97961=CARTESIAN_POINT ( 'NONE',  ( -14.29746914071049879, 8.314922557960819915, 50.83224293864770971 ) ) ;
#97962=CARTESIAN_POINT ( 'NONE',  ( -5.049401038297874678, -19.05341960407617918, 84.79275706135233293 ) ) ;
#97963=CARTESIAN_POINT ( 'NONE',  ( -18.22780087662122028, 5.500000000000031086, 83.51540105326107266 ) ) ;
#97964=CARTESIAN_POINT ( 'NONE',  ( -10.81492255796078084, -18.62759615963271287, 32.08224293864769550 ) ) ;
#97965=CARTESIAN_POINT ( 'NONE',  ( -16.53943276465976808, 0.05219959533911058130, 106.2489096053143811 ) ) ;
#97967=CARTESIAN_POINT ( 'NONE',  ( 0.05219959533909260263, 19.03943276465977164, 59.99890960531436690 ) ) ;
#97968=CARTESIAN_POINT ( 'NONE',  ( -0.05219959533907301413, -21.53943276465977519, 62.49890960531436690 ) ) ;
#97969=CARTESIAN_POINT ( 'NONE',  ( -16.46253265017160317, 9.564922557960807481, 25.83224293864769194 ) ) ;
#97970=CARTESIAN_POINT ( 'NONE',  ( -16.52544592524335698, -4.483927247898792601, 78.95942372801901854 ) ) ;
#97971=CARTESIAN_POINT ( 'NONE',  ( 16.51473224551069308, 9.474510206698969483, 59.16557627198102409 ) ) ;
#97972=CARTESIAN_POINT ( 'NONE',  ( 0.05219959533936267826, -19.03943276465977164, 60.00109039468566863 ) ) ;
#97973=CARTESIAN_POINT ( 'NONE',  ( 18.62759615963255655, 10.81492255796105972, 71.66775706135234714 ) ) ;
#97974=CARTESIAN_POINT ( 'NONE',  ( 18.62759615963271287, -10.81492255796078972, 43.33224293864769550 ) ) ;
#97975=CARTESIAN_POINT ( 'NONE',  ( 16.51473224551069308, 9.474510206698969483, 24.16557627198102765 ) ) ;
#97976=CARTESIAN_POINT ( 'NONE',  ( 16.55341960407618274, -4.379528057220086978, 86.04275706135236135 ) ) ;
#97977=CARTESIAN_POINT ( 'NONE',  ( 5.153800228976615827, -19.02544592524334988, 100.2094237280190043 ) ) ;
#97978=CARTESIAN_POINT ( 'NONE',  ( -13.97604488694527625, -13.89961937509977652, 26.87390960531434558 ) ) ;
#97980=CARTESIAN_POINT ( 'NONE',  ( -0.05219959533907301413, -21.53943276465977519, 57.49890960531435979 ) ) ;
#97981=CARTESIAN_POINT ( 'NONE',  ( 0.05219959533937995610, -21.53943276465977519, 100.0010903946857042 ) ) ;
#97982=CARTESIAN_POINT ( 'NONE',  ( -8.314922557960811034, -14.29746914071050412, 42.08224293864769550 ) ) ;
#97983=CARTESIAN_POINT ( 'NONE',  ( -16.53943276465976808, 0.05219959533911058130, 61.24890960531435979 ) ) ;
#97984=CARTESIAN_POINT ( 'NONE',  ( 21.55341960407610458, 5.719274019375980345, 78.95724293864769550 ) ) ;
#97985=CARTESIAN_POINT ( 'NONE',  ( 10.81492255796078972, 18.62759615963270932, 84.58224293864769550 ) ) ;
#97987=CARTESIAN_POINT ( 'NONE',  ( -15.72974639402197994, 15.80617190586746368, 30.62390960531436335 ) ) ;
#97988=CARTESIAN_POINT ( 'NONE',  ( -8.224510206698735004, -14.34966873604973081, 69.58442372801900433 ) ) ;
#97989=CARTESIAN_POINT ( 'NONE',  ( 8.314922557960818139, 14.29746914071049879, 84.58224293864769550 ) ) ;
#97990=CARTESIAN_POINT ( 'NONE',  ( 16.51473224551069308, 9.474510206698969483, 34.16557627198102409 ) ) ;
#97993=CARTESIAN_POINT ( 'NONE',  ( -16.53943276465976808, -0.05219959533934237506, 98.75109039468568994 ) ) ;
#97994=CARTESIAN_POINT ( 'NONE',  ( 18.62759615963271287, -10.81492255796078972, 113.3322429386476955 ) ) ;
#97995=CARTESIAN_POINT ( 'NONE',  ( 16.46253265017160672, -9.564922557960803928, 88.33224293864769550 ) ) ;
#97996=CARTESIAN_POINT ( 'NONE',  ( 0.05219959533937995610, -21.53943276465977519, 50.00109039468568994 ) ) ;
#97997=CARTESIAN_POINT ( 'NONE',  ( -13.89961937509977652, 13.97604488694528158, 105.6239096053143527 ) ) ;
#97998=CARTESIAN_POINT ( 'NONE',  ( -18.22780087662126647, -5.499999999999827693, 48.98236817873107185 ) ) ;
#97999=ORIENTED_EDGE ( 'NONE', *, *, #125462, .F. ) ;
#98000=CARTESIAN_POINT ( 'NONE',  ( -10.72451020669870658, -18.67979575497194134, 44.58442372801901854 ) ) ;
#98001=CARTESIAN_POINT ( 'NONE',  ( -9.474510206698964154, 16.51473224551069663, 40.41557627198103120 ) ) ;
#98002=CARTESIAN_POINT ( 'NONE',  ( -5.153800228976328057, -19.02544592524343514, 102.2905762719810383 ) ) ;
#98003=CARTESIAN_POINT ( 'NONE',  ( 5.049401038297881783, 19.05341960407617563, 52.29275706135234003 ) ) ;
#98004=CARTESIAN_POINT ( 'NONE',  ( 18.62759615963255655, 10.81492255796105972, 31.66775706135234358 ) ) ;
#98005=CARTESIAN_POINT ( 'NONE',  ( -19.03943276465977164, -0.05219959533935918106, 63.75109039468566863 ) ) ;
#98006=CARTESIAN_POINT ( 'NONE',  ( -14.34966873604972548, 8.224510206698743886, 93.33442372801901854 ) ) ;
#98007=CARTESIAN_POINT ( 'NONE',  ( -0.05219959533936034679, 19.03943276465977164, 57.50109039468566863 ) ) ;
#98008=CARTESIAN_POINT ( 'NONE',  ( 4.483927247898790824, -16.52544592524335698, 110.2094237280190185 ) ) ;
#98009=CARTESIAN_POINT ( 'NONE',  ( 18.09867054820430710, 5.500000000000000000, 86.48393025253589883 ) ) ;
#98010=CARTESIAN_POINT ( 'NONE',  ( -9.564922557960796823, -16.46253265017161027, 82.08224293864768129 ) ) ;
#98011=CARTESIAN_POINT ( 'NONE',  ( 21.52544592524334988, 5.823673210054432836, 86.45942372801901854 ) ) ;
#98012=CARTESIAN_POINT ( 'NONE',  ( -5.719274019375665041, -21.55341960407619695, 109.7927570613523613 ) ) ;
#98014=CARTESIAN_POINT ( 'NONE',  ( 0.05219959533909260263, 19.03943276465977164, 99.99890960531436690 ) ) ;
#98015=CARTESIAN_POINT ( 'NONE',  ( -5.719274019375665041, -21.55341960407619695, 69.79275706135234714 ) ) ;
#98016=CARTESIAN_POINT ( 'NONE',  ( 5.049401038297881783, 19.05341960407617563, 112.2927570613523471 ) ) ;
#98017=CARTESIAN_POINT ( 'NONE',  ( -19.03943276465977164, 0.05219959533909376836, 81.24890960531436690 ) ) ;
#98018=CARTESIAN_POINT ( 'NONE',  ( 5.823673210054125526, 21.52544592524343514, 34.79057627198103120 ) ) ;
#98020=CARTESIAN_POINT ( 'NONE',  ( -19.03943276465977164, 0.05219959533909376836, 96.24890960531436690 ) ) ;
#98022=CARTESIAN_POINT ( 'NONE',  ( -9.474510206698964154, 16.51473224551069663, 75.41557627198103830 ) ) ;
#98023=CARTESIAN_POINT ( 'NONE',  ( -16.46253265017160317, 9.564922557960807481, 65.83224293864769550 ) ) ;
#98024=CARTESIAN_POINT ( 'NONE',  ( -4.379528057220086978, -16.55341960407618274, 109.7927570613523613 ) ) ;
#98025=CARTESIAN_POINT ( 'NONE',  ( -19.39720447994796260, -5.499999999999982236, 39.66317477297176453 ) ) ;
#98026=CARTESIAN_POINT ( 'NONE',  ( -9.564922557961040184, 16.46253265017147172, 72.91775706135233293 ) ) ;
#98027=CARTESIAN_POINT ( 'NONE',  ( 16.51473224551069308, 9.474510206698969483, 89.16557627198103830 ) ) ;
#98028=CARTESIAN_POINT ( 'NONE',  ( 4.483927247898545687, 16.52544592524342804, 84.79057627198102409 ) ) ;
#98029=CARTESIAN_POINT ( 'NONE',  ( -0.05219959533907301413, -21.53943276465977519, 52.49890960531435979 ) ) ;
#98030=CARTESIAN_POINT ( 'NONE',  ( 18.67979575497178502, 10.72451020669898547, 24.16557627198103120 ) ) ;
#98031=CARTESIAN_POINT ( 'NONE',  ( -14.29746914071049879, 8.314922557960819915, 105.8322429386476955 ) ) ;
#98033=CARTESIAN_POINT ( 'NONE',  ( 0.05219959533936267826, -19.03943276465977164, 50.00109039468566863 ) ) ;
#98034=CARTESIAN_POINT ( 'NONE',  ( 14.34966873604960469, 8.224510206698951720, 29.16557627198103120 ) ) ;
#98035=CARTESIAN_POINT ( 'NONE',  ( -19.03943276465977164, 0.05219959533909376836, 101.2489096053143669 ) ) ;
#98036=CARTESIAN_POINT ( 'NONE',  ( 5.719274019375673035, 21.55341960407619339, 62.29275706135236845 ) ) ;
#98037=CARTESIAN_POINT ( 'NONE',  ( 15.72974639402199770, -15.80617190586745480, 63.12390960531435979 ) ) ;
#98038=CARTESIAN_POINT ( 'NONE',  ( -18.67979575497193778, 10.72451020669871902, 43.33442372801901143 ) ) ;
#98039=CARTESIAN_POINT ( 'NONE',  ( -21.53943276465977519, 0.05219959533907696930, 101.2489096053143669 ) ) ;
#98040=CARTESIAN_POINT ( 'NONE',  ( 21.55341960407619695, -5.719274019375665929, 36.04275706135234714 ) ) ;
#98041=CARTESIAN_POINT ( 'NONE',  ( -12.14591786802309592, -12.06949235617757132, 111.8739096053143669 ) ) ;
#98042=CARTESIAN_POINT ( 'NONE',  ( 9.474510206698729675, 16.51473224551082808, 77.08442372801900433 ) ) ;
#98043=CARTESIAN_POINT ( 'NONE',  ( 13.97604488694527802, 13.89961937509977652, 39.37390960531435269 ) ) ;
#98044=CARTESIAN_POINT ( 'NONE',  ( -0.05219959533910754901, -16.53943276465976808, 102.4989096053143811 ) ) ;
#98045=CARTESIAN_POINT ( 'NONE',  ( -19.02544592524342804, 5.153800228976336051, 111.0405762719810099 ) ) ;
#98046=CARTESIAN_POINT ( 'NONE',  ( 14.29746914071049879, -8.314922557960816363, 38.33224293864768839 ) ) ;
#98047=CARTESIAN_POINT ( 'NONE',  ( -14.29746914071037622, -8.314922557961029526, 109.1677570613523613 ) ) ;
#98048=CARTESIAN_POINT ( 'NONE',  ( -19.05341960407611168, -5.049401038298163336, 51.45724293864770260 ) ) ;
#98049=CARTESIAN_POINT ( 'NONE',  ( -8.224510206698948167, 14.34966873604960824, 115.4155762719810241 ) ) ;
#98050=CARTESIAN_POINT ( 'NONE',  ( -19.05341960407617563, 5.049401038297882671, 28.54275706135232937 ) ) ;
#98052=CARTESIAN_POINT ( 'NONE',  ( 12.14591786802309770, 12.06949235617756955, 39.37390960531436690 ) ) ;
#98053=CARTESIAN_POINT ( 'NONE',  ( 5.719274019375673035, 21.55341960407619339, 52.29275706135236135 ) ) ;
#98055=CARTESIAN_POINT ( 'NONE',  ( 0.05219959533934541429, -16.53943276465976808, 55.00109039468568284 ) ) ;
#98056=CARTESIAN_POINT ( 'NONE',  ( -8.314922557960811034, -14.29746914071050412, 32.08224293864769550 ) ) ;
#98057=CARTESIAN_POINT ( 'NONE',  ( 12.06949235617739724, 12.14591786802326823, 101.8760903946857042 ) ) ;
#98058=CARTESIAN_POINT ( 'NONE',  ( -0.05219959533934338120, 16.53943276465976808, 32.50109039468568284 ) ) ;
#98059=EDGE_CURVE ( 'NONE', #120648, #109472, #63406, .T. ) ;
#98060=CARTESIAN_POINT ( 'NONE',  ( -13.97604488694527625, -13.89961937509977652, 41.87390960531435979 ) ) ;
#98061=CARTESIAN_POINT ( 'NONE',  ( -5.049401038298153566, 19.05341960407611168, 30.20724293864768839 ) ) ;
#98062=CARTESIAN_POINT ( 'NONE',  ( 10.81492255796106328, -18.62759615963255655, 20.41775706135234714 ) ) ;
#98063=CARTESIAN_POINT ( 'NONE',  ( 19.05341960407611168, 5.049401038298154454, 43.95724293864769550 ) ) ;
#98064=CARTESIAN_POINT ( 'NONE',  ( 19.02544592524343514, -5.153800228976328945, 113.5405762719810241 ) ) ;
#98065=CARTESIAN_POINT ( 'NONE',  ( -0.05219959533909027116, -19.03943276465977164, 32.49890960531435979 ) ) ;
#98066=CARTESIAN_POINT ( 'NONE',  ( -21.55341960407610458, -5.719274019375992779, 21.45724293864769550 ) ) ;
#98067=CARTESIAN_POINT ( 'NONE',  ( -17.44279575226826040, -5.990770900252400999, 34.16442432485683156 ) ) ;
#98068=CARTESIAN_POINT ( 'NONE',  ( -18.62759615963255300, -10.81492255796106328, 44.16775706135234714 ) ) ;
#98069=CARTESIAN_POINT ( 'NONE',  ( 16.52544592524342804, -4.483927247898539470, 103.5405762719810383 ) ) ;
#98070=CARTESIAN_POINT ( 'NONE',  ( 13.97604488694527802, 13.89961937509977652, 104.3739096053143385 ) ) ;
#98072=CARTESIAN_POINT ( 'NONE',  ( 16.52544592524335698, 4.483927247898782831, 76.45942372801901854 ) ) ;
#98074=CARTESIAN_POINT ( 'NONE',  ( 21.55341960407619695, -5.719274019375665929, 96.04275706135236135 ) ) ;
#98075=CARTESIAN_POINT ( 'NONE',  ( -16.53943276465976808, -0.05219959533934237506, 58.75109039468568994 ) ) ;
#98076=CARTESIAN_POINT ( 'NONE',  ( -16.46253265017160317, 9.564922557960807481, 90.83224293864769550 ) ) ;
#98077=CARTESIAN_POINT ( 'NONE',  ( 12.06949235617739724, 12.14591786802326823, 41.87609039468568284 ) ) ;
#98078=CARTESIAN_POINT ( 'NONE',  ( -4.483927247898782831, 16.52544592524335698, 22.70942372801901499 ) ) ;
#98079=CARTESIAN_POINT ( 'NONE',  ( -16.52544592524335698, -4.483927247898792601, 88.95942372801901854 ) ) ;
#98080=CARTESIAN_POINT ( 'NONE',  ( -9.564922557961040184, 16.46253265017147172, 102.9177570613523329 ) ) ;
#98081=CARTESIAN_POINT ( 'NONE',  ( 19.02544592524343514, -5.153800228976328945, 73.54057627198103830 ) ) ;
#98082=CARTESIAN_POINT ( 'NONE',  ( -10.81492255796078084, -18.62759615963271287, 97.08224293864770971 ) ) ;
#98083=CARTESIAN_POINT ( 'NONE',  ( 16.52544592524342804, -4.483927247898539470, 108.5405762719810241 ) ) ;
#98084=CARTESIAN_POINT ( 'NONE',  ( 19.02544592524334988, 5.153800228976608722, 101.4594237280189759 ) ) ;
#98085=CARTESIAN_POINT ( 'NONE',  ( -16.53943276465976808, -0.05219959533934237506, 68.75109039468568994 ) ) ;
#98087=CARTESIAN_POINT ( 'NONE',  ( -19.03943276465977164, -0.05219959533935918106, 68.75109039468566152 ) ) ;
#98088=CARTESIAN_POINT ( 'NONE',  ( 12.06949235617757843, -12.14591786802309237, 43.12390960531435269 ) ) ;
#98089=CARTESIAN_POINT ( 'NONE',  ( 0.05219959533910956823, 16.53943276465976808, 99.99890960531436690 ) ) ;
#98090=CARTESIAN_POINT ( 'NONE',  ( 16.51473224551083163, -9.474510206698727899, 35.83442372801899722 ) ) ;
#98091=CARTESIAN_POINT ( 'NONE',  ( -16.38665767535054840, 7.295008042176050367, 90.26400864214551234 ) ) ;
#98092=CARTESIAN_POINT ( 'NONE',  ( 10.72451020669871369, 18.67979575497193778, 37.08442372801901143 ) ) ;
#98093=CARTESIAN_POINT ( 'NONE',  ( -16.51473224551082808, 9.474510206698731452, 93.33442372801900433 ) ) ;
#98094=CARTESIAN_POINT ( 'NONE',  ( -9.474510206698964154, 16.51473224551069663, 115.4155762719810241 ) ) ;
#98095=CARTESIAN_POINT ( 'NONE',  ( 16.51473224551069308, 9.474510206698969483, 89.16557627198103830 ) ) ;
#98096=CARTESIAN_POINT ( 'NONE',  ( -16.46253265017146816, -9.564922557961047289, 19.16775706135233293 ) ) ;
#98097=CARTESIAN_POINT ( 'NONE',  ( 19.03943276465977164, -0.05219959533909143690, 93.74890960531435269 ) ) ;
#98098=CARTESIAN_POINT ( 'NONE',  ( 5.823673210054125526, 21.52544592524343514, 39.79057627198103830 ) ) ;
#98099=CARTESIAN_POINT ( 'NONE',  ( -16.53943276465976808, 0.05219959533911058130, 96.24890960531435269 ) ) ;
#98100=CARTESIAN_POINT ( 'NONE',  ( 13.97604488694527802, 13.89961937509977652, 54.37390960531435979 ) ) ;
#98101=CARTESIAN_POINT ( 'NONE',  ( -4.483927247898539470, -16.52544592524342804, 107.2905762719810525 ) ) ;
#98103=CARTESIAN_POINT ( 'NONE',  ( -21.53943276465977519, -0.05219959533937600094, 23.75109039468567929 ) ) ;
#98104=B_SPLINE_CURVE_WITH_KNOTS ( 'NONE', 3,
 ( #193504, #8478, #163159, #23651, #53985, #25670 ),
 .UNSPECIFIED., .F., .F.,
 ( 4, 2, 4 ),
 ( 0.007228050697041374893, 0.007608510107494848712, 0.007988969517948321664 ),
 .UNSPECIFIED. ) ;
#98105=CARTESIAN_POINT ( 'NONE',  ( 5.719274019375673035, 21.55341960407619339, 72.29275706135236135 ) ) ;
#98106=CARTESIAN_POINT ( 'NONE',  ( -13.89961937509977652, 13.97604488694528158, 50.62390960531435979 ) ) ;
#98107=CARTESIAN_POINT ( 'NONE',  ( 16.52544592524335698, 4.483927247898782831, 71.45942372801901854 ) ) ;
#98108=CARTESIAN_POINT ( 'NONE',  ( -21.53943276465977519, 0.05219959533907696930, 116.2489096053143669 ) ) ;
#98110=CARTESIAN_POINT ( 'NONE',  ( -5.823673210054431948, 21.52544592524334988, 22.70942372801901499 ) ) ;
#98111=CARTESIAN_POINT ( 'NONE',  ( 9.564922557961047289, -16.46253265017146816, 50.41775706135233293 ) ) ;
#98112=CARTESIAN_POINT ( 'NONE',  ( -16.51473224551069308, -9.474510206698971260, 66.66557627198102409 ) ) ;
#98113=CARTESIAN_POINT ( 'NONE',  ( 5.153800228976615827, -19.02544592524334988, 30.20942372801900433 ) ) ;
#98114=CARTESIAN_POINT ( 'NONE',  ( 15.80617190586769283, -15.72974639402175789, 75.62609039468567573 ) ) ;
#98115=CARTESIAN_POINT ( 'NONE',  ( -5.823673210054116645, -21.52544592524344225, 67.29057627198103830 ) ) ;
#98116=CARTESIAN_POINT ( 'NONE',  ( 14.29746914071049879, -8.314922557960816363, 48.33224293864770260 ) ) ;
#98117=CARTESIAN_POINT ( 'NONE',  ( -10.72451020669870658, -18.67979575497194134, 89.58442372801901854 ) ) ;
#98118=CARTESIAN_POINT ( 'NONE',  ( -0.05219959533936034679, 19.03943276465977164, 22.50109039468566152 ) ) ;
#98119=CARTESIAN_POINT ( 'NONE',  ( 0.05219959533910956823, 16.53943276465976808, 69.99890960531435269 ) ) ;
#98120=CARTESIAN_POINT ( 'NONE',  ( 19.02544592524343514, -5.153800228976328945, 23.54057627198102054 ) ) ;
#98121=CARTESIAN_POINT ( 'NONE',  ( -13.97604488694547697, 13.89961937509957934, 53.12609039468565442 ) ) ;
#98122=CARTESIAN_POINT ( 'NONE',  ( 12.14591786802309770, 12.06949235617756955, 24.37390960531435979 ) ) ;
#98123=CARTESIAN_POINT ( 'NONE',  ( 21.53943276465977519, 0.05219959533937863772, 86.25109039468568994 ) ) ;
#98124=CARTESIAN_POINT ( 'NONE',  ( 0.05219959533909260263, 19.03943276465977164, 84.99890960531436690 ) ) ;
#98125=CARTESIAN_POINT ( 'NONE',  ( -19.02544592524334988, -5.153800228976617603, 53.95942372801898301 ) ) ;
#98126=CARTESIAN_POINT ( 'NONE',  ( -5.719274019375978568, 21.55341960407610458, 45.20724293864769550 ) ) ;
#98127=CARTESIAN_POINT ( 'NONE',  ( -21.53943276465977519, -0.05219959533937600094, 43.75109039468568284 ) ) ;
#98128=CARTESIAN_POINT ( 'NONE',  ( 5.823673210054125526, 21.52544592524343514, 104.7905762719810241 ) ) ;
#98129=CARTESIAN_POINT ( 'NONE',  ( 9.474510206698729675, 16.51473224551082808, 102.0844237280190043 ) ) ;
#98130=CARTESIAN_POINT ( 'NONE',  ( 16.53943276465976808, 0.05219959533934440121, 66.25109039468567573 ) ) ;
#98132=CARTESIAN_POINT ( 'NONE',  ( -0.05219959533907301413, -21.53943276465977519, 107.4989096053143669 ) ) ;
#98133=CARTESIAN_POINT ( 'NONE',  ( -16.55341960407611168, -4.379528057220339221, 86.45724293864770971 ) ) ;
#98134=CARTESIAN_POINT ( 'NONE',  ( -17.26172910966779028, -6.454744622555857347, 99.19353091350777163 ) ) ;
#98135=CARTESIAN_POINT ( 'NONE',  ( -12.06949235617739369, -12.14591786802326823, 29.37609039468568284 ) ) ;
#98136=CARTESIAN_POINT ( 'NONE',  ( 15.72974639402199770, -15.80617190586745480, 58.12390960531435979 ) ) ;
#98137=CARTESIAN_POINT ( 'NONE',  ( -12.06949235617739369, -12.14591786802326823, 94.37609039468568994 ) ) ;
#98138=CARTESIAN_POINT ( 'NONE',  ( -19.05341960407611168, -5.049401038298163336, 26.45724293864769550 ) ) ;
#98139=CARTESIAN_POINT ( 'NONE',  ( 8.314922557961029526, -14.29746914071037800, 65.41775706135234714 ) ) ;
#98140=CARTESIAN_POINT ( 'NONE',  ( -10.72451020669870658, -18.67979575497194134, 39.58442372801901143 ) ) ;
#98141=CARTESIAN_POINT ( 'NONE',  ( 18.67979575497178502, 10.72451020669898547, 59.16557627198103120 ) ) ;
#98142=CARTESIAN_POINT ( 'NONE',  ( -8.314922557961024197, 14.29746914071037800, 87.91775706135234714 ) ) ;
#98143=CARTESIAN_POINT ( 'NONE',  ( -15.80617190586768217, 15.72974639402176855, 63.12609039468568994 ) ) ;
#98144=CARTESIAN_POINT ( 'NONE',  ( 10.81492255796078972, 18.62759615963270932, 59.58224293864770260 ) ) ;
#98145=CARTESIAN_POINT ( 'NONE',  ( -10.72451020669898014, 18.67979575497178502, 35.41557627198102409 ) ) ;
#98146=CARTESIAN_POINT ( 'NONE',  ( 14.29746914071037800, 8.314922557961029526, 66.66775706135234714 ) ) ;
#98147=CARTESIAN_POINT ( 'NONE',  ( 15.80617190586746368, 15.72974639402197994, 29.37390960531435269 ) ) ;
#98148=ORIENTED_EDGE ( 'NONE', *, *, #62447, .T. ) ;
#98149=CARTESIAN_POINT ( 'NONE',  ( 16.46253265017160672, -9.564922557960803928, 98.33224293864769550 ) ) ;
#98150=CARTESIAN_POINT ( 'NONE',  ( 12.06949235617757843, -12.14591786802309237, 23.12390960531436335 ) ) ;
#98152=CARTESIAN_POINT ( 'NONE',  ( 14.34966873604960469, 8.224510206698951720, 104.1655762719810241 ) ) ;
#98153=CARTESIAN_POINT ( 'NONE',  ( -5.823673210054116645, -21.52544592524344225, 67.29057627198103830 ) ) ;
#98154=CARTESIAN_POINT ( 'NONE',  ( -13.89961937509977652, 13.97604488694528158, 40.62390960531435979 ) ) ;
#98155=CARTESIAN_POINT ( 'NONE',  ( -12.14591786802326823, 12.06949235617739902, 93.12609039468568994 ) ) ;
#98156=CARTESIAN_POINT ( 'NONE',  ( -10.72451020669870658, -18.67979575497194134, 39.58442372801901143 ) ) ;
#98157=CARTESIAN_POINT ( 'NONE',  ( -19.05341960407617563, 5.049401038297882671, 108.5427570613523187 ) ) ;
#98158=CARTESIAN_POINT ( 'NONE',  ( 12.14591786802309770, 12.06949235617756955, 109.3739096053143811 ) ) ;
#98159=CARTESIAN_POINT ( 'NONE',  ( 19.03943276465977164, -0.05219959533909143690, 48.74890960531435979 ) ) ;
#98160=CARTESIAN_POINT ( 'NONE',  ( -13.97604488694527625, -13.89961937509977652, 21.87390960531435979 ) ) ;
#98162=CARTESIAN_POINT ( 'NONE',  ( 0.05219959533909260263, 19.03943276465977164, 89.99890960531436690 ) ) ;
#98164=CARTESIAN_POINT ( 'NONE',  ( 16.52544592524335698, 4.483927247898782831, 76.45942372801901854 ) ) ;
#98165=CARTESIAN_POINT ( 'NONE',  ( -10.72451020669870658, -18.67979575497194134, 99.58442372801900433 ) ) ;
#98166=CARTESIAN_POINT ( 'NONE',  ( -15.80617190586745835, -15.72974639402198527, 46.87390960531435979 ) ) ;
#98167=CARTESIAN_POINT ( 'NONE',  ( -16.53943276465976808, -0.05219959533934237506, 78.75109039468568994 ) ) ;
#98168=CARTESIAN_POINT ( 'NONE',  ( -5.153800228976607833, 19.02544592524334988, 67.70942372801900433 ) ) ;
#98169=CARTESIAN_POINT ( 'NONE',  ( 5.823673210054444382, -21.52544592524334988, 60.20942372801902565 ) ) ;
#98170=CARTESIAN_POINT ( 'NONE',  ( -16.51473224551069308, -9.474510206698971260, 76.66557627198103830 ) ) ;
#98171=CARTESIAN_POINT ( 'NONE',  ( -5.049401038298153566, 19.05341960407611168, 35.20724293864768839 ) ) ;
#98172=CARTESIAN_POINT ( 'NONE',  ( 5.153800228976615827, -19.02544592524334988, 60.20942372801899012 ) ) ;
#98174=CARTESIAN_POINT ( 'NONE',  ( -19.03943276465977164, 0.05219959533909376836, 91.24890960531436690 ) ) ;
#98175=CARTESIAN_POINT ( 'NONE',  ( -16.52544592524342804, 4.483927247898546575, 46.04057627198103830 ) ) ;
#98176=CARTESIAN_POINT ( 'NONE',  ( -15.72974639402197994, 15.80617190586746368, 50.62390960531435979 ) ) ;
#98178=CARTESIAN_POINT ( 'NONE',  ( -16.46253265017146816, -9.564922557961047289, 24.16775706135233648 ) ) ;
#98179=CARTESIAN_POINT ( 'NONE',  ( -16.38665767535055906, -7.295008042176049479, 79.73599135785454450 ) ) ;
#98180=CARTESIAN_POINT ( 'NONE',  ( 13.97604488694527802, 13.89961937509977652, 49.37390960531434558 ) ) ;
#98181=CARTESIAN_POINT ( 'NONE',  ( 12.06949235617739724, 12.14591786802326823, 41.87609039468568284 ) ) ;
#98183=CARTESIAN_POINT ( 'NONE',  ( -17.12812012977027010, 6.668231424565978394, 108.6405124067685790 ) ) ;
#98184=CARTESIAN_POINT ( 'NONE',  ( 4.483927247898790824, -16.52544592524335698, 80.20942372801901854 ) ) ;
#98185=CARTESIAN_POINT ( 'NONE',  ( 10.72451020669898902, -18.67979575497178502, 102.9155762719810383 ) ) ;
#98187=CARTESIAN_POINT ( 'NONE',  ( -0.05219959533909027116, -19.03943276465977164, 37.49890960531436690 ) ) ;
#98189=CARTESIAN_POINT ( 'NONE',  ( -18.62759615963255300, -10.81492255796106328, 44.16775706135234714 ) ) ;
#98190=CARTESIAN_POINT ( 'NONE',  ( -19.05341960407617563, 5.049401038297882671, 53.54275706135231871 ) ) ;
#98191=CARTESIAN_POINT ( 'NONE',  ( 19.03943276465977164, -0.05219959533909143690, 53.74890960531436690 ) ) ;
#98192=CARTESIAN_POINT ( 'NONE',  ( 21.52544592524334988, 5.823673210054432836, 91.45942372801901854 ) ) ;
#98193=CARTESIAN_POINT ( 'NONE',  ( 16.81555441253554051, 7.025013491695493606, 96.86314554665749199 ) ) ;
#98194=CARTESIAN_POINT ( 'NONE',  ( -8.314922557960811034, -14.29746914071050412, 42.08224293864769550 ) ) ;
#98196=CARTESIAN_POINT ( 'NONE',  ( 5.719274019375991003, -21.55341960407610458, 57.70724293864770260 ) ) ;
#98198=CARTESIAN_POINT ( 'NONE',  ( 13.89961937509977652, -13.97604488694527269, 103.1239096053143527 ) ) ;
#98199=CARTESIAN_POINT ( 'NONE',  ( -0.05219959533910754901, -16.53943276465976808, 97.49890960531436690 ) ) ;
#98200=CARTESIAN_POINT ( 'NONE',  ( -13.97604488694547697, 13.89961937509957934, 113.1260903946856757 ) ) ;
#98201=CARTESIAN_POINT ( 'NONE',  ( -16.53943276465976808, 0.05219959533911058130, 21.24890960531436690 ) ) ;
#98203=CARTESIAN_POINT ( 'NONE',  ( -19.05341960407611168, -5.049401038298163336, 96.45724293864769550 ) ) ;
#98204=CARTESIAN_POINT ( 'NONE',  ( 15.72974639402199770, -15.80617190586745480, 103.1239096053143811 ) ) ;
#98205=CARTESIAN_POINT ( 'NONE',  ( -14.34966873604960291, -8.224510206698953496, 31.66557627198102054 ) ) ;
#98206=CARTESIAN_POINT ( 'NONE',  ( 19.05341960407611168, 5.049401038298154454, 98.95724293864766707 ) ) ;
#98207=CARTESIAN_POINT ( 'NONE',  ( -19.05341960407617563, 5.049401038297882671, 93.54275706135234714 ) ) ;
#98208=CARTESIAN_POINT ( 'NONE',  ( -15.72974639402176322, -15.80617190586768395, 109.3760903946857042 ) ) ;
#98209=CARTESIAN_POINT ( 'NONE',  ( 15.80617190586746368, 15.72974639402197994, 84.37390960531438111 ) ) ;
#98210=CARTESIAN_POINT ( 'NONE',  ( -15.80617190586745835, -15.72974639402198527, 51.87390960531437401 ) ) ;
#98212=CARTESIAN_POINT ( 'NONE',  ( 5.153800228976335163, 19.02544592524342804, 69.79057627198103830 ) ) ;
#98213=CARTESIAN_POINT ( 'NONE',  ( 12.14591786802309770, 12.06949235617756955, 29.37390960531435269 ) ) ;
#98214=CARTESIAN_POINT ( 'NONE',  ( -13.97604488694527625, -13.89961937509977652, 71.87390960531433848 ) ) ;
#98216=CARTESIAN_POINT ( 'NONE',  ( 18.56197773271730611, -5.500000000000111910, 61.05066217314453070 ) ) ;
#98217=CARTESIAN_POINT ( 'NONE',  ( -5.153800228976607833, 19.02544592524334988, 37.70942372801899722 ) ) ;
#98218=CARTESIAN_POINT ( 'NONE',  ( -15.80617190586745835, -15.72974639402198527, 81.87390960531435269 ) ) ;
#98219=CARTESIAN_POINT ( 'NONE',  ( -16.55341960407611168, -4.379528057220339221, 91.45724293864769550 ) ) ;
#98220=CARTESIAN_POINT ( 'NONE',  ( -21.53943276465977519, -0.05219959533937600094, 43.75109039468568284 ) ) ;
#98222=CARTESIAN_POINT ( 'NONE',  ( -4.483927247898782831, 16.52544592524335698, 102.7094237280190185 ) ) ;
#98223=CARTESIAN_POINT ( 'NONE',  ( -9.474510206698964154, 16.51473224551069663, 25.41557627198103120 ) ) ;
#98224=CARTESIAN_POINT ( 'NONE',  ( 16.51473224551069308, 9.474510206698969483, 84.16557627198102409 ) ) ;
#98225=CARTESIAN_POINT ( 'NONE',  ( 17.72696623605160582, -5.500000000000045297, 71.09811031808418136 ) ) ;
#98227=CARTESIAN_POINT ( 'NONE',  ( 0.05219959533910956823, 16.53943276465976808, 39.99890960531436690 ) ) ;
#98228=CARTESIAN_POINT ( 'NONE',  ( 21.53943276465977519, 0.05219959533937863772, 66.25109039468567573 ) ) ;
#98230=CARTESIAN_POINT ( 'NONE',  ( 5.049401038298161559, -19.05341960407611168, 47.70724293864770260 ) ) ;
#98231=CARTESIAN_POINT ( 'NONE',  ( 19.03943276465977164, -0.05219959533909143690, 48.74890960531435979 ) ) ;
#98232=ORIENTED_EDGE ( 'NONE', *, *, #184834, .F. ) ;
#98233=CARTESIAN_POINT ( 'NONE',  ( -19.03943276465977164, -0.05219959533935918106, 18.75109039468567218 ) ) ;
#98234=CARTESIAN_POINT ( 'NONE',  ( 14.29746914071037800, 8.314922557961029526, 61.66775706135235424 ) ) ;
#98235=CARTESIAN_POINT ( 'NONE',  ( 5.719274019375673035, 21.55341960407619339, 92.29275706135236135 ) ) ;
#98236=CARTESIAN_POINT ( 'NONE',  ( -19.03943276465977164, 0.05219959533909376836, 111.2489096053143669 ) ) ;
#98237=CARTESIAN_POINT ( 'NONE',  ( 19.03943276465977164, 0.05219959533936151252, 96.25109039468567573 ) ) ;
#98238=CARTESIAN_POINT ( 'NONE',  ( -15.80617190586768217, 15.72974639402176855, 73.12609039468567573 ) ) ;
#98239=CARTESIAN_POINT ( 'NONE',  ( 4.483927247898790824, -16.52544592524335698, 30.20942372801902565 ) ) ;
#98240=CARTESIAN_POINT ( 'NONE',  ( 21.52544592524344225, -5.823673210054117533, 83.54057627198102409 ) ) ;
#98241=CARTESIAN_POINT ( 'NONE',  ( -19.02544592524334988, -5.153800228976617603, 93.95942372801900433 ) ) ;
#98242=CARTESIAN_POINT ( 'NONE',  ( -16.46253265017160317, 9.564922557960807481, 60.83224293864769550 ) ) ;
#98243=CARTESIAN_POINT ( 'NONE',  ( 16.55341960407618274, -4.379528057220086978, 21.04275706135234714 ) ) ;
#98244=CIRCLE ( 'NONE', #156451, 2.500000000000002220 ) ;
#98245=CARTESIAN_POINT ( 'NONE',  ( -13.89961937509957401, -13.97604488694547875, 104.3760903946856757 ) ) ;
#98246=CARTESIAN_POINT ( 'NONE',  ( -14.34966873604960291, -8.224510206698953496, 46.66557627198102409 ) ) ;
#98247=CARTESIAN_POINT ( 'NONE',  ( 5.049401038297881783, 19.05341960407617563, 77.29275706135231871 ) ) ;
#98248=CARTESIAN_POINT ( 'NONE',  ( -14.34966873604972548, 8.224510206698743886, 58.33442372801901143 ) ) ;
#98249=CARTESIAN_POINT ( 'NONE',  ( 18.62759615963271287, -10.81492255796078972, 113.3322429386476955 ) ) ;
#98250=CARTESIAN_POINT ( 'NONE',  ( 16.51473224551069308, 9.474510206698969483, 39.16557627198103120 ) ) ;
#98251=CARTESIAN_POINT ( 'NONE',  ( -13.97604488694527625, -13.89961937509977652, 51.87390960531436690 ) ) ;
#98252=CARTESIAN_POINT ( 'NONE',  ( -16.52544592524335698, -4.483927247898792601, 58.95942372801902565 ) ) ;
#98253=CARTESIAN_POINT ( 'NONE',  ( -17.97161686094258215, 5.499999999999975131, 45.99637206859247840 ) ) ;
#98255=CARTESIAN_POINT ( 'NONE',  ( -9.474510206698964154, 16.51473224551069663, 100.4155762719810241 ) ) ;
#98256=EDGE_CURVE ( 'NONE', #93673, #199515, #74734, .T. ) ;
#98257=CARTESIAN_POINT ( 'NONE',  ( -19.03943276465977164, 0.05219959533909376836, 26.24890960531435624 ) ) ;
#98259=CARTESIAN_POINT ( 'NONE',  ( 14.34966873604972726, -8.224510206698740333, 20.83442372801901143 ) ) ;
#98260=CARTESIAN_POINT ( 'NONE',  ( -10.72451020669898014, 18.67979575497178502, 55.41557627198102409 ) ) ;
#98261=CARTESIAN_POINT ( 'NONE',  ( -19.05341960407617563, 5.049401038297882671, 43.54275706135232582 ) ) ;
#98262=CARTESIAN_POINT ( 'NONE',  ( 0.05219959533934541429, -16.53943276465976808, 35.00109039468568284 ) ) ;
#98263=CARTESIAN_POINT ( 'NONE',  ( -19.02544592524342804, 5.153800228976336051, 26.04057627198103120 ) ) ;
#98264=CARTESIAN_POINT ( 'NONE',  ( -5.049401038298153566, 19.05341960407611168, 50.20724293864770260 ) ) ;
#98265=CARTESIAN_POINT ( 'NONE',  ( 5.823673210054125526, 21.52544592524343514, 84.79057627198102409 ) ) ;
#98266=CARTESIAN_POINT ( 'NONE',  ( 0.05219959533909260263, 19.03943276465977164, 114.9989096053143669 ) ) ;
#98267=CARTESIAN_POINT ( 'NONE',  ( -16.51473224551069308, -9.474510206698971260, 51.66557627198102409 ) ) ;
#98269=CARTESIAN_POINT ( 'NONE',  ( -19.05341960407617563, 5.049401038297882671, 78.54275706135233293 ) ) ;
#98270=CARTESIAN_POINT ( 'NONE',  ( -8.224510206698948167, 14.34966873604960824, 60.41557627198102409 ) ) ;
#98271=CARTESIAN_POINT ( 'NONE',  ( 21.53943276465977519, 0.05219959533937863772, 101.2510903946856757 ) ) ;
#98273=CARTESIAN_POINT ( 'NONE',  ( -15.80617190586745835, -15.72974639402198527, 101.8739096053143811 ) ) ;
#98274=CARTESIAN_POINT ( 'NONE',  ( 5.823673210054444382, -21.52544592524334988, 80.20942372801901854 ) ) ;
#98275=CARTESIAN_POINT ( 'NONE',  ( 19.05341960407611168, 5.049401038298154454, 28.95724293864769550 ) ) ;
#98276=CARTESIAN_POINT ( 'NONE',  ( 15.72974639402176855, 15.80617190586768217, 71.87609039468568994 ) ) ;
#98277=CARTESIAN_POINT ( 'NONE',  ( 9.564922557960805705, 16.46253265017160317, 109.5822429386476955 ) ) ;
#98278=CARTESIAN_POINT ( 'NONE',  ( 16.55341960407618274, -4.379528057220086978, 101.0427570613523756 ) ) ;
#98279=CARTESIAN_POINT ( 'NONE',  ( -5.719274019375665041, -21.55341960407619695, 79.79275706135236135 ) ) ;
#98280=CARTESIAN_POINT ( 'NONE',  ( -9.564922557960796823, -16.46253265017161027, 62.08224293864769550 ) ) ;
#98281=CARTESIAN_POINT ( 'NONE',  ( -10.81492255796105439, 18.62759615963255655, 42.91775706135235424 ) ) ;
#98282=CARTESIAN_POINT ( 'NONE',  ( 19.05341960407611168, 5.049401038298154454, 83.95724293864766707 ) ) ;
#98283=CARTESIAN_POINT ( 'NONE',  ( -8.224510206698948167, 14.34966873604960824, 100.4155762719810241 ) ) ;
#98284=CARTESIAN_POINT ( 'NONE',  ( 4.379528057220339221, -16.55341960407611168, 57.70724293864770260 ) ) ;
#98285=CARTESIAN_POINT ( 'NONE',  ( -5.719274019375978568, 21.55341960407610458, 65.20724293864768129 ) ) ;
#98286=CARTESIAN_POINT ( 'NONE',  ( -16.51473224551069308, -9.474510206698971260, 56.66557627198103120 ) ) ;
#98287=CARTESIAN_POINT ( 'NONE',  ( -18.67979575497178146, -10.72451020669898902, 71.66557627198100988 ) ) ;
#98288=CARTESIAN_POINT ( 'NONE',  ( -13.89961937509957401, -13.97604488694547875, 59.37609039468566863 ) ) ;
#98289=CARTESIAN_POINT ( 'NONE',  ( -5.153800228976607833, 19.02544592524335343, 27.70942372801900078 ) ) ;
#98290=CARTESIAN_POINT ( 'NONE',  ( 14.34966873604960469, 8.224510206698951720, 74.16557627198102409 ) ) ;
#98291=CARTESIAN_POINT ( 'NONE',  ( -15.72974639402197994, 15.80617190586746368, 55.62390960531436690 ) ) ;
#98292=CARTESIAN_POINT ( 'NONE',  ( 17.50000000000000000, 5.499999999999992895, 101.7030961746583131 ) ) ;
#98293=CARTESIAN_POINT ( 'NONE',  ( -0.05219959533934338120, 16.53943276465976808, 97.50109039468567573 ) ) ;
#98295=CARTESIAN_POINT ( 'NONE',  ( -13.89961937509957401, -13.97604488694547875, 104.3760903946856757 ) ) ;
#98296=CARTESIAN_POINT ( 'NONE',  ( -12.06949235617756955, 12.14591786802309770, 70.62390960531436690 ) ) ;
#98298=CARTESIAN_POINT ( 'NONE',  ( -0.05219959533909027116, -19.03943276465977164, 67.49890960531436690 ) ) ;
#98299=CARTESIAN_POINT ( 'NONE',  ( -16.55341960407611168, -4.379528057220339221, 51.45724293864770260 ) ) ;
#98301=CARTESIAN_POINT ( 'NONE',  ( 0.05219959533909260263, 19.03943276465977164, 104.9989096053143669 ) ) ;
#98303=CARTESIAN_POINT ( 'NONE',  ( -13.89961937509957401, -13.97604488694547875, 79.37609039468567573 ) ) ;
#98304=CARTESIAN_POINT ( 'NONE',  ( -5.153800228976328057, -19.02544592524343514, 62.29057627198100988 ) ) ;
#98305=CARTESIAN_POINT ( 'NONE',  ( -16.51473224551069308, -9.474510206698971260, 86.66557627198102409 ) ) ;
#98306=CARTESIAN_POINT ( 'NONE',  ( 5.153800228976335163, 19.02544592524342804, 74.79057627198103830 ) ) ;
#98307=CARTESIAN_POINT ( 'NONE',  ( 10.81492255796078972, 18.62759615963270932, 69.58224293864769550 ) ) ;
#98308=CARTESIAN_POINT ( 'NONE',  ( 4.379528057220092307, 16.55341960407617563, 57.29275706135234714 ) ) ;
#98309=CARTESIAN_POINT ( 'NONE',  ( 13.89961937509957579, 13.97604488694547520, 101.8760903946856615 ) ) ;
#98310=CARTESIAN_POINT ( 'NONE',  ( -5.049401038298153566, 19.05341960407611168, 50.20724293864770260 ) ) ;
#98311=CARTESIAN_POINT ( 'NONE',  ( -0.05219959533907301413, -21.53943276465977519, 52.49890960531435979 ) ) ;
#98312=CARTESIAN_POINT ( 'NONE',  ( 19.03943276465977164, 0.05219959533936151252, 76.25109039468566152 ) ) ;
#98313=CARTESIAN_POINT ( 'NONE',  ( -8.314922557961024197, 14.29746914071037800, 112.9177570613523329 ) ) ;
#98314=CARTESIAN_POINT ( 'NONE',  ( 21.55341960407619695, -5.719274019375665929, 31.04275706135234714 ) ) ;
#98315=CARTESIAN_POINT ( 'NONE',  ( 19.03943276465977164, 0.05219959533936151252, 36.25109039468567573 ) ) ;
#98316=CARTESIAN_POINT ( 'NONE',  ( 8.314922557961029526, -14.29746914071037800, 65.41775706135234714 ) ) ;
#98317=CARTESIAN_POINT ( 'NONE',  ( 14.34966873604972726, -8.224510206698740333, 90.83442372801901854 ) ) ;
#98319=CARTESIAN_POINT ( 'NONE',  ( -12.14591786802326823, 12.06949235617739902, 78.12609039468570415 ) ) ;
#98320=CARTESIAN_POINT ( 'NONE',  ( -13.89961937509977652, 13.97604488694528158, 115.6239096053143669 ) ) ;
#98321=CARTESIAN_POINT ( 'NONE',  ( -8.224510206698735004, -14.34966873604973081, 39.58442372801901143 ) ) ;
#98322=CARTESIAN_POINT ( 'NONE',  ( -13.97604488694527625, -13.89961937509977652, 51.87390960531436690 ) ) ;
#98323=CARTESIAN_POINT ( 'NONE',  ( 13.97604488694527802, 13.89961937509977652, 54.37390960531435979 ) ) ;
#98324=CARTESIAN_POINT ( 'NONE',  ( 19.03943276465977164, -0.05219959533909143690, 63.74890960531435979 ) ) ;
#98325=CARTESIAN_POINT ( 'NONE',  ( -15.80617190586768217, 15.72974639402176855, 38.12609039468567573 ) ) ;
#98326=CARTESIAN_POINT ( 'NONE',  ( 12.14591786802327356, -12.06949235617739191, 50.62609039468568994 ) ) ;
#98327=CARTESIAN_POINT ( 'NONE',  ( -8.224510206698735004, -14.34966873604973081, 109.5844237280190328 ) ) ;
#98328=CARTESIAN_POINT ( 'NONE',  ( 19.05341960407611168, 5.049401038298154454, 28.95724293864769550 ) ) ;
#98329=CARTESIAN_POINT ( 'NONE',  ( -19.03943276465977164, -0.05219959533935918106, 23.75109039468566152 ) ) ;
#98330=CARTESIAN_POINT ( 'NONE',  ( 14.29746914071037800, 8.314922557961029526, 21.66775706135235069 ) ) ;
#98332=CARTESIAN_POINT ( 'NONE',  ( -5.153800228976607833, 19.02544592524334988, 62.70942372801899722 ) ) ;
#98333=CARTESIAN_POINT ( 'NONE',  ( 16.52544592524342804, -4.483927247898539470, 68.54057627198103830 ) ) ;
#98334=CARTESIAN_POINT ( 'NONE',  ( -13.97604488694527625, -13.89961937509977652, 41.87390960531435979 ) ) ;
#98335=CARTESIAN_POINT ( 'NONE',  ( 0.05219959533936267826, -19.03943276465977164, 80.00109039468567573 ) ) ;
#98336=CARTESIAN_POINT ( 'NONE',  ( 17.05587630539785238, -6.762274262135687053, 93.24180309037312497 ) ) ;
#98337=CARTESIAN_POINT ( 'NONE',  ( 15.72974639402176855, 15.80617190586768217, 76.87609039468567573 ) ) ;
#98338=CARTESIAN_POINT ( 'NONE',  ( -4.379528057220086978, -16.55341960407618274, 44.79275706135234714 ) ) ;
#98339=CARTESIAN_POINT ( 'NONE',  ( 18.87580814761072645, -5.500000000000034639, 58.37172394265762421 ) ) ;
#98340=CARTESIAN_POINT ( 'NONE',  ( 21.55341960407610458, 5.719274019375980345, 38.95724293864768839 ) ) ;
#98341=CARTESIAN_POINT ( 'NONE',  ( -4.483927247898782831, 16.52544592524335698, 27.70942372801901854 ) ) ;
#98342=CARTESIAN_POINT ( 'NONE',  ( 19.05341960407611168, 5.049401038298154454, 28.95724293864769550 ) ) ;
#98343=CARTESIAN_POINT ( 'NONE',  ( 18.67979575497194134, -10.72451020669871369, 105.8344237280190328 ) ) ;
#98344=CARTESIAN_POINT ( 'NONE',  ( 17.72696623605164490, -5.499999999999867661, 66.09811031808418136 ) ) ;
#98345=CARTESIAN_POINT ( 'NONE',  ( -9.564922557960796823, -16.46253265017161027, 32.08224293864769550 ) ) ;
#98347=CARTESIAN_POINT ( 'NONE',  ( -5.153800228976328057, -19.02544592524343514, 57.29057627198103120 ) ) ;
#98348=CARTESIAN_POINT ( 'NONE',  ( 5.823673210054444382, -21.52544592524334988, 70.20942372801904696 ) ) ;
#98349=CARTESIAN_POINT ( 'NONE',  ( -9.474510206698720793, -16.51473224551083518, 24.58442372801900078 ) ) ;
#98350=CARTESIAN_POINT ( 'NONE',  ( 12.14591786802327356, -12.06949235617739191, 110.6260903946857042 ) ) ;
#98351=CARTESIAN_POINT ( 'NONE',  ( -5.049401038298153566, 19.05341960407611168, 35.20724293864768839 ) ) ;
#98353=CARTESIAN_POINT ( 'NONE',  ( -19.05341960407611168, -5.049401038298163336, 91.45724293864766707 ) ) ;
#98354=CARTESIAN_POINT ( 'NONE',  ( 21.55341960407619695, -5.719274019375665929, 76.04275706135237556 ) ) ;
#98355=CARTESIAN_POINT ( 'NONE',  ( 9.564922557960805705, 16.46253265017160317, 34.58224293864770260 ) ) ;
#98356=CARTESIAN_POINT ( 'NONE',  ( -5.823673210054431948, 21.52544592524334988, 67.70942372801901854 ) ) ;
#98357=CARTESIAN_POINT ( 'NONE',  ( -0.05219959533936034679, 19.03943276465977164, 92.50109039468566152 ) ) ;
#98358=CARTESIAN_POINT ( 'NONE',  ( -19.05341960407611168, -5.049401038298163336, 101.4572429386476955 ) ) ;
#98359=CARTESIAN_POINT ( 'NONE',  ( 16.46253265017160672, -9.564922557960803928, 38.33224293864768839 ) ) ;
#98360=CARTESIAN_POINT ( 'NONE',  ( 18.67979575497178502, 10.72451020669898547, 104.1655762719810241 ) ) ;
#98361=CARTESIAN_POINT ( 'NONE',  ( -19.03943276465977164, -0.05219959533935918106, 38.75109039468566152 ) ) ;
#98362=CARTESIAN_POINT ( 'NONE',  ( -16.52544592524342804, 4.483927247898546575, 111.0405762719810525 ) ) ;
#98363=CARTESIAN_POINT ( 'NONE',  ( 19.05341960407611168, 5.049401038298154454, 63.95724293864769550 ) ) ;
#98364=CARTESIAN_POINT ( 'NONE',  ( -9.474510206698720793, -16.51473224551083518, 99.58442372801900433 ) ) ;
#98365=VECTOR ( 'NONE', #121947, 1000.000000000000000 ) ;
#98366=CARTESIAN_POINT ( 'NONE',  ( 4.483927247898545687, 16.52544592524342804, 64.79057627198103830 ) ) ;
#98367=CARTESIAN_POINT ( 'NONE',  ( 10.72451020669898902, -18.67979575497178502, 22.91557627198102765 ) ) ;
#98368=CARTESIAN_POINT ( 'NONE',  ( 16.46253265017146816, 9.564922557961045513, 81.66775706135233293 ) ) ;
#98369=CARTESIAN_POINT ( 'NONE',  ( -21.53943276465977519, 0.05219959533907696930, 86.24890960531436690 ) ) ;
#98370=CARTESIAN_POINT ( 'NONE',  ( 10.81492255796106328, -18.62759615963255655, 45.41775706135234003 ) ) ;
#98371=CARTESIAN_POINT ( 'NONE',  ( 0.05219959533934541429, -16.53943276465976808, 45.00109039468568284 ) ) ;
#98372=CARTESIAN_POINT ( 'NONE',  ( 8.314922557961029526, -14.29746914071037800, 40.41775706135234714 ) ) ;
#98373=CARTESIAN_POINT ( 'NONE',  ( -21.52544592524334988, -5.823673210054445271, 48.95942372801902565 ) ) ;
#98374=CARTESIAN_POINT ( 'NONE',  ( 10.72451020669898902, -18.67979575497178502, 57.91557627198103120 ) ) ;
#98376=CARTESIAN_POINT ( 'NONE',  ( 19.05341960407611168, 5.049401038298154454, 38.95724293864767418 ) ) ;
#98378=CARTESIAN_POINT ( 'NONE',  ( 4.379528057220092307, 16.55341960407617563, 72.29275706135236135 ) ) ;
#98379=CARTESIAN_POINT ( 'NONE',  ( -10.72451020669898014, 18.67979575497178502, 100.4155762719810241 ) ) ;
#98380=CARTESIAN_POINT ( 'NONE',  ( 16.52544592524342804, -4.483927247898539470, 38.54057627198103120 ) ) ;
#98381=CARTESIAN_POINT ( 'NONE',  ( 14.29746914071037800, 8.314922557961029526, 56.66775706135235424 ) ) ;
#98382=CARTESIAN_POINT ( 'NONE',  ( 0.05219959533936267826, -19.03943276465977164, 95.00109039468567573 ) ) ;
#98383=CARTESIAN_POINT ( 'NONE',  ( -5.719274019375978568, 21.55341960407610458, 95.20724293864769550 ) ) ;
#98384=CARTESIAN_POINT ( 'NONE',  ( 0.05219959533910956823, 16.53943276465976808, 29.99890960531435979 ) ) ;
#98386=CARTESIAN_POINT ( 'NONE',  ( 14.29746914071037800, 8.314922557961029526, 81.66775706135236135 ) ) ;
#98388=CARTESIAN_POINT ( 'NONE',  ( -15.80617190586745835, -15.72974639402198527, 71.87390960531438111 ) ) ;
#98389=CARTESIAN_POINT ( 'NONE',  ( 16.52544592524335698, 4.483927247898782831, 106.4594237280190328 ) ) ;
#98390=ORIENTED_EDGE ( 'NONE', *, *, #16822, .F. ) ;
#98391=CARTESIAN_POINT ( 'NONE',  ( -17.49999999999999645, -5.499999999999992895, 54.20309617465830598 ) ) ;
#98392=CARTESIAN_POINT ( 'NONE',  ( 21.55341960407610458, 5.719274019375980345, 98.95724293864770971 ) ) ;
#98393=CARTESIAN_POINT ( 'NONE',  ( -0.05219959533907301413, -21.53943276465977519, 107.4989096053143669 ) ) ;
#98394=CARTESIAN_POINT ( 'NONE',  ( -12.14591786802309592, -12.06949235617757132, 41.87390960531435979 ) ) ;
#98396=CARTESIAN_POINT ( 'NONE',  ( -4.483927247898782831, 16.52544592524335698, 42.70942372801901854 ) ) ;
#98397=CARTESIAN_POINT ( 'NONE',  ( 19.02544592524343514, -5.153800228976328945, 48.54057627198103120 ) ) ;
#98398=EDGE_CURVE ( 'NONE', #84229, #30776, #198426, .T. ) ;
#98399=CARTESIAN_POINT ( 'NONE',  ( 9.474510206698971260, -16.51473224551069308, 72.91557627198102409 ) ) ;
#98401=CARTESIAN_POINT ( 'NONE',  ( 9.474510206698971260, -16.51473224551069308, 112.9155762719810383 ) ) ;
#98403=CARTESIAN_POINT ( 'NONE',  ( -0.05219959533936034679, 19.03943276465977164, 107.5010903946856615 ) ) ;
#98404=CARTESIAN_POINT ( 'NONE',  ( 9.474510206698729675, 16.51473224551082808, 57.08442372801900433 ) ) ;
#98405=CARTESIAN_POINT ( 'NONE',  ( -21.53943276465977519, 0.05219959533907696930, 86.24890960531436690 ) ) ;
#98406=CARTESIAN_POINT ( 'NONE',  ( -16.53943276465976808, -0.05219959533934237506, 113.7510903946856757 ) ) ;
#98407=CARTESIAN_POINT ( 'NONE',  ( 19.03943276465977164, -0.05219959533909143690, 73.74890960531435269 ) ) ;
#98408=CARTESIAN_POINT ( 'NONE',  ( 18.62759615963271287, -10.81492255796078972, 43.33224293864769550 ) ) ;
#98409=CARTESIAN_POINT ( 'NONE',  ( -18.67979575497178146, -10.72451020669898902, 76.66557627198103830 ) ) ;
#98410=CARTESIAN_POINT ( 'NONE',  ( 4.379528057220092307, 16.55341960407617563, 27.29275706135234358 ) ) ;
#98411=CARTESIAN_POINT ( 'NONE',  ( 19.02544592524343514, -5.153800228976328945, 113.5405762719810241 ) ) ;
#98412=CARTESIAN_POINT ( 'NONE',  ( 15.80617190586769283, -15.72974639402175789, 80.62609039468567573 ) ) ;
#98413=CARTESIAN_POINT ( 'NONE',  ( 19.03943276465977164, -0.05219959533909143690, 78.74890960531436690 ) ) ;
#98414=CARTESIAN_POINT ( 'NONE',  ( -13.97604488694527625, -13.89961937509977652, 21.87390960531435979 ) ) ;
#98415=CARTESIAN_POINT ( 'NONE',  ( 16.46253265017160672, -9.564922557960803928, 68.33224293864770971 ) ) ;
#98416=CARTESIAN_POINT ( 'NONE',  ( 8.224510206698953496, -14.34966873604960469, 87.91557627198103830 ) ) ;
#98417=VERTEX_POINT ( 'NONE', #7401 ) ;
#98418=CARTESIAN_POINT ( 'NONE',  ( -13.97604488694547697, 13.89961937509957934, 98.12609039468566152 ) ) ;
#98419=CARTESIAN_POINT ( 'NONE',  ( 22.00000000000000000, -1.163414459189985801E-14, 92.50000000000000000 ) ) ;
#98420=CARTESIAN_POINT ( 'NONE',  ( -13.89961937509977652, 13.97604488694528158, 75.62390960531438111 ) ) ;
#98421=CARTESIAN_POINT ( 'NONE',  ( 5.823673210054444382, -21.52544592524334988, 90.20942372801903275 ) ) ;
#98422=CARTESIAN_POINT ( 'NONE',  ( 19.02544592524343514, -5.153800228976328945, 98.54057627198100988 ) ) ;
#98423=CARTESIAN_POINT ( 'NONE',  ( 16.53943276465976808, 0.05219959533934440121, 81.25109039468568994 ) ) ;
#98424=CARTESIAN_POINT ( 'NONE',  ( -16.19135201231366494, -7.376712067591931543, 75.18680854052030327 ) ) ;
#98425=CARTESIAN_POINT ( 'NONE',  ( 19.03943276465977164, 0.05219959533936151252, 61.25109039468566863 ) ) ;
#98426=CARTESIAN_POINT ( 'NONE',  ( 5.049401038297881783, 19.05341960407617563, 22.29275706135233648 ) ) ;
#98430=CARTESIAN_POINT ( 'NONE',  ( 4.379528057220339221, -16.55341960407611168, 27.70724293864769905 ) ) ;
#98433=CARTESIAN_POINT ( 'NONE',  ( -16.55341960407617563, 4.379528057220093196, 103.5427570613523613 ) ) ;
#98434=CARTESIAN_POINT ( 'NONE',  ( 17.26058549869092928, 6.457015423128506626, 68.87745837476070676 ) ) ;
#98435=CARTESIAN_POINT ( 'NONE',  ( 4.379528057220092307, 16.55341960407617563, 82.29275706135234714 ) ) ;
#98437=CARTESIAN_POINT ( 'NONE',  ( -15.80617190586768217, 15.72974639402176855, 83.12609039468568994 ) ) ;
#98438=CARTESIAN_POINT ( 'NONE',  ( -5.153800228976607833, 19.02544592524334988, 107.7094237280189759 ) ) ;
#98439=CARTESIAN_POINT ( 'NONE',  ( -18.62759615963255300, -10.81492255796106328, 64.16775706135234714 ) ) ;
#98440=CARTESIAN_POINT ( 'NONE',  ( -19.03943276465977164, -0.05219959533935918106, 33.75109039468566863 ) ) ;
#98441=CARTESIAN_POINT ( 'NONE',  ( -13.89961937509977652, 13.97604488694528158, 75.62390960531438111 ) ) ;
#98442=CARTESIAN_POINT ( 'NONE',  ( 16.46253265017160672, -9.564922557960803928, 53.33224293864768839 ) ) ;
#98443=EDGE_CURVE ( 'NONE', #24966, #176032, #193685, .T. ) ;
#98444=CARTESIAN_POINT ( 'NONE',  ( -19.02130022317637170, 5.499999999999601208, 40.78188669246577547 ) ) ;
#98445=CARTESIAN_POINT ( 'NONE',  ( 0.05219959533907565091, 21.53943276465977519, 99.99890960531436690 ) ) ;
#98446=CARTESIAN_POINT ( 'NONE',  ( 10.81492255796078972, 18.62759615963270932, 49.58224293864769550 ) ) ;
#98447=CARTESIAN_POINT ( 'NONE',  ( 19.03943276465977164, -0.05219959533909143690, 48.74890960531435979 ) ) ;
#98448=CARTESIAN_POINT ( 'NONE',  ( -16.52544592524335698, -4.483927247898792601, 58.95942372801902565 ) ) ;
#98450=ORIENTED_EDGE ( 'NONE', *, *, #176690, .F. ) ;
#98451=CARTESIAN_POINT ( 'NONE',  ( -21.52544592524334988, -5.823673210054445271, 38.95942372801901854 ) ) ;
#98452=CARTESIAN_POINT ( 'NONE',  ( -12.06949235617756955, 12.14591786802309770, 60.62390960531437401 ) ) ;
#98454=CARTESIAN_POINT ( 'NONE',  ( 16.53943276465976808, 0.05219959533934440121, 41.25109039468568284 ) ) ;
#98455=CARTESIAN_POINT ( 'NONE',  ( -0.05219959533910754901, -16.53943276465976808, 97.49890960531436690 ) ) ;
#98456=CARTESIAN_POINT ( 'NONE',  ( 5.049401038297881783, 19.05341960407617563, 47.29275706135231161 ) ) ;
#98457=CARTESIAN_POINT ( 'NONE',  ( 12.14591786802309770, 12.06949235617756955, 74.37390960531436690 ) ) ;
#98458=CARTESIAN_POINT ( 'NONE',  ( 21.53943276465977519, 0.05219959533937863772, 26.25109039468567573 ) ) ;
#98459=CARTESIAN_POINT ( 'NONE',  ( 19.02544592524343514, -5.153800228976328945, 23.54057627198102054 ) ) ;
#98460=CARTESIAN_POINT ( 'NONE',  ( -10.72451020669898014, 18.67979575497178502, 85.41557627198102409 ) ) ;
#98461=CARTESIAN_POINT ( 'NONE',  ( 0.05219959533909260263, 19.03943276465977164, 104.9989096053143669 ) ) ;
#98462=CARTESIAN_POINT ( 'NONE',  ( 12.06949235617757843, -12.14591786802309237, 78.12390960531436690 ) ) ;
#98465=CARTESIAN_POINT ( 'NONE',  ( -0.05219959533936034679, 19.03943276465977164, 87.50109039468567573 ) ) ;
#98466=CARTESIAN_POINT ( 'NONE',  ( 10.72451020669871369, 18.67979575497193778, 27.08442372801901854 ) ) ;
#98467=CARTESIAN_POINT ( 'NONE',  ( -13.89961937509977652, 13.97604488694528158, 65.62390960531436690 ) ) ;
#98468=CARTESIAN_POINT ( 'NONE',  ( -16.46253265017146816, -9.564922557961047289, 54.16775706135234003 ) ) ;
#98469=CARTESIAN_POINT ( 'NONE',  ( -5.153800228976328057, -19.02544592524343514, 37.29057627198102409 ) ) ;
#98471=CARTESIAN_POINT ( 'NONE',  ( -4.483927247898539470, -16.52544592524342804, 57.29057627198103120 ) ) ;
#98472=CARTESIAN_POINT ( 'NONE',  ( 8.224510206698953496, -14.34966873604960469, 57.91557627198103120 ) ) ;
#98473=CARTESIAN_POINT ( 'NONE',  ( -19.03943276465977164, 0.05219959533909376836, 61.24890960531436690 ) ) ;
#98475=CARTESIAN_POINT ( 'NONE',  ( -5.823673210054116645, -21.52544592524344225, 87.29057627198103830 ) ) ;
#98476=CARTESIAN_POINT ( 'NONE',  ( -13.89961937509977652, 13.97604488694528158, 60.62390960531436690 ) ) ;
#98477=CARTESIAN_POINT ( 'NONE',  ( -15.80617190586745835, -15.72974639402198527, 81.87390960531435269 ) ) ;
#98478=CARTESIAN_POINT ( 'NONE',  ( -21.55341960407619339, 5.719274019375674811, 98.54275706135234714 ) ) ;
#98479=CARTESIAN_POINT ( 'NONE',  ( 13.89961937509977652, -13.97604488694527269, 23.12390960531436335 ) ) ;
#98480=CARTESIAN_POINT ( 'NONE',  ( -16.55341960407611168, -4.379528057220339221, 21.45724293864769550 ) ) ;
#98481=CARTESIAN_POINT ( 'NONE',  ( 0.05219959533910956823, 16.53943276465976808, 94.99890960531436690 ) ) ;
#98482=CARTESIAN_POINT ( 'NONE',  ( 19.03943276465977164, 0.05219959533936151252, 86.25109039468567573 ) ) ;
#98484=CARTESIAN_POINT ( 'NONE',  ( 18.67979575497194134, -10.72451020669871369, 20.83442372801901143 ) ) ;
#98485=CARTESIAN_POINT ( 'NONE',  ( -5.153800228976607833, 19.02544592524334988, 52.70942372801900433 ) ) ;
#98486=CARTESIAN_POINT ( 'NONE',  ( -4.379528057220086978, -16.55341960407618274, 99.79275706135234714 ) ) ;
#98487=CARTESIAN_POINT ( 'NONE',  ( 19.02544592524334988, 5.153800228976608722, 26.45942372801899722 ) ) ;
#98488=CARTESIAN_POINT ( 'NONE',  ( -16.51473224551069308, -9.474510206698971260, 106.6655762719810383 ) ) ;
#98489=CARTESIAN_POINT ( 'NONE',  ( -10.72451020669898014, 18.67979575497178502, 65.41557627198102409 ) ) ;
#98491=CARTESIAN_POINT ( 'NONE',  ( 9.474510206698971260, -16.51473224551069308, 37.91557627198102409 ) ) ;
#98492=CARTESIAN_POINT ( 'NONE',  ( 21.53943276465977519, 0.05219959533937863772, 111.2510903946856899 ) ) ;
#98493=CARTESIAN_POINT ( 'NONE',  ( -8.314922557961024197, 14.29746914071037800, 77.91775706135231871 ) ) ;
#98494=CARTESIAN_POINT ( 'NONE',  ( 21.52544592524334988, 5.823673210054432836, 26.45942372801901854 ) ) ;
#98495=CARTESIAN_POINT ( 'NONE',  ( 16.52544592524335698, 4.483927247898782831, 41.45942372801901143 ) ) ;
#98496=CARTESIAN_POINT ( 'NONE',  ( 16.46253265017160672, -9.564922557960803928, 108.3322429386476955 ) ) ;
#98497=CARTESIAN_POINT ( 'NONE',  ( 9.564922557960805705, 16.46253265017160317, 59.58224293864769550 ) ) ;
#98498=CARTESIAN_POINT ( 'NONE',  ( 19.03943276465977164, -0.05219959533909143690, 68.74890960531436690 ) ) ;
#98499=CARTESIAN_POINT ( 'NONE',  ( -8.314922557961024197, 14.29746914071037800, 47.91775706135234714 ) ) ;
#98500=CARTESIAN_POINT ( 'NONE',  ( -16.52544592524342804, 4.483927247898546575, 106.0405762719810525 ) ) ;
#98501=CARTESIAN_POINT ( 'NONE',  ( -8.314922557961024197, 14.29746914071037800, 107.9177570613523471 ) ) ;
#98502=CARTESIAN_POINT ( 'NONE',  ( -15.72974639402176322, -15.80617190586768395, 59.37609039468568284 ) ) ;
#98503=CARTESIAN_POINT ( 'NONE',  ( -9.564922557960796823, -16.46253265017161027, 72.08224293864770971 ) ) ;
#98504=CARTESIAN_POINT ( 'NONE',  ( -19.02544592524342804, 5.153800228976336051, 71.04057627198099567 ) ) ;
#98505=CARTESIAN_POINT ( 'NONE',  ( -9.564922557960796823, -16.46253265017161027, 92.08224293864769550 ) ) ;
#98506=CARTESIAN_POINT ( 'NONE',  ( -4.483927247898539470, -16.52544592524342804, 47.29057627198103120 ) ) ;
#98507=CARTESIAN_POINT ( 'NONE',  ( 8.224510206698953496, -14.34966873604960469, 22.91557627198102765 ) ) ;
#98508=CARTESIAN_POINT ( 'NONE',  ( 4.483927247898545687, 16.52544592524342804, 39.79057627198103830 ) ) ;
#98510=CARTESIAN_POINT ( 'NONE',  ( -19.03943276465977164, -0.05219959533935918106, 48.75109039468566863 ) ) ;
#98513=CARTESIAN_POINT ( 'NONE',  ( -0.05219959533909027116, -19.03943276465977164, 67.49890960531436690 ) ) ;
#98514=CARTESIAN_POINT ( 'NONE',  ( -9.564922557961040184, 16.46253265017147172, 32.91775706135233293 ) ) ;
#98518=CARTESIAN_POINT ( 'NONE',  ( -19.05341960407617563, 5.049401038297882671, 78.54275706135233293 ) ) ;
#98519=CARTESIAN_POINT ( 'NONE',  ( 14.34966873604972726, -8.224510206698740333, 65.83442372801900433 ) ) ;
#98520=CARTESIAN_POINT ( 'NONE',  ( 17.49999999999999645, 5.624438216177590100, 91.68329655085358354 ) ) ;
#98521=CARTESIAN_POINT ( 'NONE',  ( -19.02544592524342804, 5.153800228976336051, 91.04057627198100988 ) ) ;
#98522=CARTESIAN_POINT ( 'NONE',  ( -21.52544592524334988, -5.823673210054445271, 23.95942372801901143 ) ) ;
#98523=CARTESIAN_POINT ( 'NONE',  ( 5.153800228976615827, -19.02544592524334988, 75.20942372801896170 ) ) ;
#98524=CARTESIAN_POINT ( 'NONE',  ( 17.31747979337950127, 6.344076630961020591, 88.87944868065186199 ) ) ;
#98525=CARTESIAN_POINT ( 'NONE',  ( 5.049401038298161559, -19.05341960407611168, 52.70724293864767418 ) ) ;
#98526=CARTESIAN_POINT ( 'NONE',  ( 16.51473224551069308, 9.474510206698969483, 84.16557627198102409 ) ) ;
#98527=CARTESIAN_POINT ( 'NONE',  ( 14.29746914071049879, -8.314922557960816363, 48.33224293864770260 ) ) ;
#98528=CARTESIAN_POINT ( 'NONE',  ( 19.02544592524343514, -5.153800228976328945, 48.54057627198103120 ) ) ;
#98529=CARTESIAN_POINT ( 'NONE',  ( 9.474510206698729675, 16.51473224551082808, 47.08442372801900433 ) ) ;
#98530=CARTESIAN_POINT ( 'NONE',  ( 14.29746914071049879, -8.314922557960816363, 88.33224293864769550 ) ) ;
#98531=CARTESIAN_POINT ( 'NONE',  ( -19.02544592524334988, -5.153800228976617603, 28.95942372801900433 ) ) ;
#98532=CARTESIAN_POINT ( 'NONE',  ( -19.02544592524342804, 5.153800228976336051, 61.04057627198103120 ) ) ;
#98533=CARTESIAN_POINT ( 'NONE',  ( -15.80617190586745835, -15.72974639402198527, 56.87390960531436690 ) ) ;
#98534=CARTESIAN_POINT ( 'NONE',  ( -4.379528057220328563, 16.55341960407611168, 70.20724293864769550 ) ) ;
#98535=CARTESIAN_POINT ( 'NONE',  ( 13.97604488694548053, -13.89961937509957401, 20.62609039468567573 ) ) ;
#98536=CARTESIAN_POINT ( 'NONE',  ( -19.05341960407611168, -5.049401038298163336, 111.4572429386476671 ) ) ;
#98537=CARTESIAN_POINT ( 'NONE',  ( 18.62759615963271287, -10.81492255796078972, 28.33224293864769550 ) ) ;
#98538=CARTESIAN_POINT ( 'NONE',  ( -5.153800228976328057, -19.02544592524343514, 47.29057627198102409 ) ) ;
#98539=CARTESIAN_POINT ( 'NONE',  ( 16.51473224551069308, 9.474510206698969483, 44.16557627198103120 ) ) ;
#98540=CARTESIAN_POINT ( 'NONE',  ( 8.224510206698953496, -14.34966873604960469, 97.91557627198103830 ) ) ;
#98542=CARTESIAN_POINT ( 'NONE',  ( -15.80617190586745835, -15.72974639402198527, 111.8739096053143669 ) ) ;
#98543=CARTESIAN_POINT ( 'NONE',  ( -19.03943276465977164, 0.05219959533909376836, 106.2489096053143669 ) ) ;
#98544=CARTESIAN_POINT ( 'NONE',  ( 15.72974639402199770, -15.80617190586745480, 113.1239096053143953 ) ) ;
#98545=CARTESIAN_POINT ( 'NONE',  ( 19.05341960407611168, 5.049401038298154454, 103.9572429386476671 ) ) ;
#98546=CARTESIAN_POINT ( 'NONE',  ( 9.474510206698971260, -16.51473224551069308, 27.91557627198103120 ) ) ;
#98547=CARTESIAN_POINT ( 'NONE',  ( -18.62759615963255300, -10.81492255796106328, 84.16775706135234714 ) ) ;
#98548=CARTESIAN_POINT ( 'NONE',  ( -21.52544592524343514, 5.823673210054127303, 91.04057627198103830 ) ) ;
#98550=CARTESIAN_POINT ( 'NONE',  ( 19.26498983726237668, -5.499999999999793943, 78.05319577422000066 ) ) ;
#98552=CARTESIAN_POINT ( 'NONE',  ( -16.53943276465976808, -0.05219959533934237506, 48.75109039468568284 ) ) ;
#98553=CARTESIAN_POINT ( 'NONE',  ( 8.314922557960818139, 14.29746914071049879, 114.5822429386477097 ) ) ;
#98555=CARTESIAN_POINT ( 'NONE',  ( 9.474510206698971260, -16.51473224551069308, 57.91557627198103120 ) ) ;
#98556=CARTESIAN_POINT ( 'NONE',  ( -16.53943276465976808, 0.05219959533911058130, 96.24890960531435269 ) ) ;
#98557=CARTESIAN_POINT ( 'NONE',  ( 15.80617190586746368, 15.72974639402197994, 49.37390960531436690 ) ) ;
#98558=CARTESIAN_POINT ( 'NONE',  ( -4.379528057220328563, 16.55341960407611168, 65.20724293864768129 ) ) ;
#98559=CARTESIAN_POINT ( 'NONE',  ( 16.53943276465976808, 0.05219959533934440121, 26.25109039468567573 ) ) ;
#98560=CARTESIAN_POINT ( 'NONE',  ( 15.72974639402176855, 15.80617190586768217, 76.87609039468567573 ) ) ;
#98561=CARTESIAN_POINT ( 'NONE',  ( 13.89961937509957579, 13.97604488694547520, 61.87609039468566863 ) ) ;
#98562=CARTESIAN_POINT ( 'NONE',  ( -16.52544592524335698, -4.483927247898792601, 98.95942372801903275 ) ) ;
#98563=CARTESIAN_POINT ( 'NONE',  ( 16.52544592524342804, -4.483927247898539470, 43.54057627198103830 ) ) ;
#98564=CARTESIAN_POINT ( 'NONE',  ( -13.97604488694527625, -13.89961937509977652, 36.87390960531436690 ) ) ;
#98565=CARTESIAN_POINT ( 'NONE',  ( 5.153800228976335163, 19.02544592524342804, 94.79057627198103830 ) ) ;
#98566=CARTESIAN_POINT ( 'NONE',  ( 15.72974639402199770, -15.80617190586745480, 88.12390960531436690 ) ) ;
#98567=CARTESIAN_POINT ( 'NONE',  ( -12.14591786802326823, 12.06949235617739902, 43.12609039468568284 ) ) ;
#98568=CARTESIAN_POINT ( 'NONE',  ( -0.05219959533910754901, -16.53943276465976808, 62.49890960531436690 ) ) ;
#98569=CARTESIAN_POINT ( 'NONE',  ( -15.72974639402176322, -15.80617190586768395, 69.37609039468567573 ) ) ;
#98570=CARTESIAN_POINT ( 'NONE',  ( 8.224510206698742110, 14.34966873604972548, 102.0844237280190185 ) ) ;
#98573=CARTESIAN_POINT ( 'NONE',  ( 12.14591786802309770, 12.06949235617756955, 24.37390960531435979 ) ) ;
#98574=CARTESIAN_POINT ( 'NONE',  ( -14.34966873604972548, 8.224510206698743886, 68.33442372801900433 ) ) ;
#98575=CARTESIAN_POINT ( 'NONE',  ( 9.474510206698971260, -16.51473224551069308, 87.91557627198102409 ) ) ;
#98576=CARTESIAN_POINT ( 'NONE',  ( -13.89961937509977652, 13.97604488694528158, 100.6239096053143669 ) ) ;
#98577=CARTESIAN_POINT ( 'NONE',  ( 18.67979575497194134, -10.72451020669871369, 90.83442372801901854 ) ) ;
#98578=CARTESIAN_POINT ( 'NONE',  ( 12.06949235617739724, 12.14591786802326823, 91.87609039468568994 ) ) ;
#98579=CARTESIAN_POINT ( 'NONE',  ( 16.55341960407611168, 4.379528057220329451, 53.95724293864770260 ) ) ;
#98580=CARTESIAN_POINT ( 'NONE',  ( -5.153800228976328057, -19.02544592524343514, 72.29057627198102409 ) ) ;
#98582=CARTESIAN_POINT ( 'NONE',  ( 13.97604488694548053, -13.89961937509957401, 105.6260903946856757 ) ) ;
#98583=CARTESIAN_POINT ( 'NONE',  ( -14.29746914071049879, 8.314922557960819915, 105.8322429386476955 ) ) ;
#98584=CARTESIAN_POINT ( 'NONE',  ( 9.474510206698971260, -16.51473224551069308, 77.91557627198103830 ) ) ;
#98585=CARTESIAN_POINT ( 'NONE',  ( -14.29746914071037622, -8.314922557961029526, 24.16775706135235424 ) ) ;
#98587=CARTESIAN_POINT ( 'NONE',  ( 15.72974639402176855, 15.80617190586768217, 111.8760903946856615 ) ) ;
#98588=CARTESIAN_POINT ( 'NONE',  ( 16.53943276465976808, 0.05219959533934440121, 86.25109039468568994 ) ) ;
#98589=CARTESIAN_POINT ( 'NONE',  ( -9.474510206698720793, -16.51473224551083518, 89.58442372801900433 ) ) ;
#98590=CARTESIAN_POINT ( 'NONE',  ( -5.153800228976328057, -19.02544592524343514, 22.29057627198102765 ) ) ;
#98591=CARTESIAN_POINT ( 'NONE',  ( 8.314922557961029526, -14.29746914071037800, 65.41775706135234714 ) ) ;
#98592=CARTESIAN_POINT ( 'NONE',  ( -8.224510206698735004, -14.34966873604973081, 54.58442372801901143 ) ) ;
#98594=CARTESIAN_POINT ( 'NONE',  ( -16.46253265017146816, -9.564922557961047289, 69.16775706135233293 ) ) ;
#98596=CARTESIAN_POINT ( 'NONE',  ( -21.55341960407619339, 5.719274019375674811, 103.5427570613523613 ) ) ;
#98597=CARTESIAN_POINT ( 'NONE',  ( -13.89961937509977652, 13.97604488694528158, 35.62390960531435269 ) ) ;
#98598=CARTESIAN_POINT ( 'NONE',  ( -13.89961937509977652, 13.97604488694528158, 80.62390960531436690 ) ) ;
#98599=CARTESIAN_POINT ( 'NONE',  ( -12.14591786802309592, -12.06949235617757132, 76.87390960531439532 ) ) ;
#98600=CARTESIAN_POINT ( 'NONE',  ( 5.719274019375673035, 21.55341960407619339, 92.29275706135236135 ) ) ;
#98601=CARTESIAN_POINT ( 'NONE',  ( 16.51473224551083163, -9.474510206698727899, 45.83442372801900433 ) ) ;
#98602=CARTESIAN_POINT ( 'NONE',  ( 5.719274019375991003, -21.55341960407610458, 42.70724293864770260 ) ) ;
#98603=CARTESIAN_POINT ( 'NONE',  ( 13.97604488694548053, -13.89961937509957401, 20.62609039468567573 ) ) ;
#98604=CARTESIAN_POINT ( 'NONE',  ( -9.564922557960796823, -16.46253265017161027, 77.08224293864769550 ) ) ;
#98605=CARTESIAN_POINT ( 'NONE',  ( -15.72974639402176322, -15.80617190586768395, 109.3760903946857042 ) ) ;
#98606=CARTESIAN_POINT ( 'NONE',  ( 21.52544592524344225, -5.823673210054117533, 63.54057627198103830 ) ) ;
#98607=CARTESIAN_POINT ( 'NONE',  ( -19.05341960407611168, -5.049401038298163336, 96.45724293864769550 ) ) ;
#98608=CARTESIAN_POINT ( 'NONE',  ( -16.46253265017146816, -9.564922557961047289, 79.16775706135234714 ) ) ;
#98609=CARTESIAN_POINT ( 'NONE',  ( -16.51473224551069308, -9.474510206698971260, 96.66557627198102409 ) ) ;
#98610=CARTESIAN_POINT ( 'NONE',  ( 13.89961937509957401, 13.97604488694547697, 91.87609039468567573 ) ) ;
#98611=CARTESIAN_POINT ( 'NONE',  ( -16.52544592524335698, -4.483927247898792601, 48.95942372801902565 ) ) ;
#98612=CARTESIAN_POINT ( 'NONE',  ( 16.51473224551069308, 9.474510206698969483, 24.16557627198102765 ) ) ;
#98613=CARTESIAN_POINT ( 'NONE',  ( -13.97604488694527625, -13.89961937509977652, 81.87390960531436690 ) ) ;
#98614=CARTESIAN_POINT ( 'NONE',  ( 10.72451020669898902, -18.67979575497178502, 67.91557627198102409 ) ) ;
#98615=CARTESIAN_POINT ( 'NONE',  ( 4.379528057220092307, 16.55341960407617563, 27.29275706135234358 ) ) ;
#98616=CARTESIAN_POINT ( 'NONE',  ( -15.80617190586768217, 15.72974639402176855, 28.12609039468568284 ) ) ;
#98617=CARTESIAN_POINT ( 'NONE',  ( 0.05219959533937995610, -21.53943276465977519, 80.00109039468568994 ) ) ;
#98618=CARTESIAN_POINT ( 'NONE',  ( -12.06949235617739369, -12.14591786802326823, 84.37609039468570415 ) ) ;
#98619=CARTESIAN_POINT ( 'NONE',  ( 5.049401038298161559, -19.05341960407611168, 87.70724293864769550 ) ) ;
#98620=CARTESIAN_POINT ( 'NONE',  ( 8.224510206698953496, -14.34966873604960469, 72.91557627198103830 ) ) ;
#98621=CARTESIAN_POINT ( 'NONE',  ( -12.06949235617756955, 12.14591786802309770, 25.62390960531435624 ) ) ;
#98622=CARTESIAN_POINT ( 'NONE',  ( -5.049401038297874678, -19.05341960407617918, 54.79275706135234003 ) ) ;
#98623=CARTESIAN_POINT ( 'NONE',  ( -21.52544592524334988, -5.823673210054445271, 48.95942372801902565 ) ) ;
#98624=CARTESIAN_POINT ( 'NONE',  ( 8.224510206698953496, -14.34966873604960469, 92.91557627198103830 ) ) ;
#98625=CARTESIAN_POINT ( 'NONE',  ( -9.474510206698964154, 16.51473224551069663, 115.4155762719810241 ) ) ;
#98626=CARTESIAN_POINT ( 'NONE',  ( -16.53943276465976808, -0.05219959533934237506, 98.75109039468568994 ) ) ;
#98627=CARTESIAN_POINT ( 'NONE',  ( 18.67979575497194134, -10.72451020669871369, 85.83442372801901854 ) ) ;
#98628=CARTESIAN_POINT ( 'NONE',  ( 14.29746914071037800, 8.314922557961029526, 46.66775706135234714 ) ) ;
#98629=CARTESIAN_POINT ( 'NONE',  ( -10.81492255796105439, 18.62759615963255655, 42.91775706135235424 ) ) ;
#98631=CARTESIAN_POINT ( 'NONE',  ( 18.62759615963271287, -10.81492255796078972, 113.3322429386476955 ) ) ;
#98632=CARTESIAN_POINT ( 'NONE',  ( 8.224510206698953496, -14.34966873604960469, 87.91557627198103830 ) ) ;
#98633=CARTESIAN_POINT ( 'NONE',  ( -18.39639308325436673, -5.500000000000040856, 51.48252246182197922 ) ) ;
#98634=CARTESIAN_POINT ( 'NONE',  ( 14.29746914071049879, -8.314922557960816363, 68.33224293864769550 ) ) ;
#98635=CARTESIAN_POINT ( 'NONE',  ( 0.05219959533934541429, -16.53943276465976808, 95.00109039468568994 ) ) ;
#98636=CARTESIAN_POINT ( 'NONE',  ( -19.02544592524342804, 5.153800228976336051, 41.04057627198103120 ) ) ;
#98637=CARTESIAN_POINT ( 'NONE',  ( -5.719274019375978568, 21.55341960407610458, 45.20724293864769550 ) ) ;
#98638=CARTESIAN_POINT ( 'NONE',  ( -12.14591786802309592, -12.06949235617757132, 71.87390960531438111 ) ) ;
#98640=CARTESIAN_POINT ( 'NONE',  ( 5.823673210054125526, 21.52544592524343514, 74.79057627198105251 ) ) ;
#98641=CARTESIAN_POINT ( 'NONE',  ( 9.564922557960805705, 16.46253265017160317, 94.58224293864769550 ) ) ;
#98642=ADVANCED_FACE ( 'NONE', ( #39746 ), #138278, .T. ) ;
#98643=CARTESIAN_POINT ( 'NONE',  ( 9.564922557960805705, 16.46253265017160317, 44.58224293864769550 ) ) ;
#98644=CARTESIAN_POINT ( 'NONE',  ( 9.564922557961047289, -16.46253265017146816, 90.41775706135234714 ) ) ;
#98645=CARTESIAN_POINT ( 'NONE',  ( -10.81492255796078084, -18.62759615963271287, 32.08224293864769550 ) ) ;
#98646=CARTESIAN_POINT ( 'NONE',  ( 5.823673210054444382, -21.52544592524334988, 60.20942372801902565 ) ) ;
#98647=CARTESIAN_POINT ( 'NONE',  ( 19.05341960407611168, 5.049401038298154454, 58.95724293864768129 ) ) ;
#98648=CARTESIAN_POINT ( 'NONE',  ( -16.46253265017160317, 9.564922557960807481, 90.83224293864769550 ) ) ;
#98650=CARTESIAN_POINT ( 'NONE',  ( 0.05219959533934541429, -16.53943276465976808, 45.00109039468568284 ) ) ;
#98651=CARTESIAN_POINT ( 'NONE',  ( 18.62759615963255655, 10.81492255796105972, 41.66775706135235424 ) ) ;
#98652=CARTESIAN_POINT ( 'NONE',  ( -21.53943276465977519, -0.05219959533937600094, 73.75109039468567573 ) ) ;
#98653=CARTESIAN_POINT ( 'NONE',  ( 9.474510206698971260, -16.51473224551069308, 112.9155762719810383 ) ) ;
#98654=CARTESIAN_POINT ( 'NONE',  ( 10.81492255796078972, 18.62759615963270932, 84.58224293864769550 ) ) ;
#98655=CARTESIAN_POINT ( 'NONE',  ( -18.67979575497193778, 10.72451020669871902, 28.33442372801902209 ) ) ;
#98656=CARTESIAN_POINT ( 'NONE',  ( 16.53943276465976808, 0.05219959533934440121, 66.25109039468567573 ) ) ;
#98657=CARTESIAN_POINT ( 'NONE',  ( -18.67979575497178146, -10.72451020669898902, 61.66557627198103120 ) ) ;
#98658=CARTESIAN_POINT ( 'NONE',  ( 18.62759615963255655, 10.81492255796105972, 111.6677570613523613 ) ) ;
#98659=CARTESIAN_POINT ( 'NONE',  ( 16.51473224551069308, 9.474510206698969483, 74.16557627198103830 ) ) ;
#98660=CARTESIAN_POINT ( 'NONE',  ( -16.55341960407617563, 4.379528057220093196, 108.5427570613523756 ) ) ;
#98662=CARTESIAN_POINT ( 'NONE',  ( -19.03943276465977164, 0.05219959533909376836, 91.24890960531436690 ) ) ;
#98663=CARTESIAN_POINT ( 'NONE',  ( -16.51473224551082808, 9.474510206698731452, 53.33442372801900433 ) ) ;
#98664=CARTESIAN_POINT ( 'NONE',  ( -5.153800228976607833, 19.02544592524334988, 82.70942372801897591 ) ) ;
#98665=CARTESIAN_POINT ( 'NONE',  ( 21.52544592524344225, -5.823673210054117533, 53.54057627198103120 ) ) ;
#98666=CARTESIAN_POINT ( 'NONE',  ( -0.05219959533934338120, 16.53943276465976808, 112.5010903946857042 ) ) ;
#98667=CARTESIAN_POINT ( 'NONE',  ( -13.89961937509957401, -13.97604488694547875, 104.3760903946856757 ) ) ;
#98668=CARTESIAN_POINT ( 'NONE',  ( 19.03943276465977164, -0.05219959533909143690, 23.74890960531435269 ) ) ;
#98669=CARTESIAN_POINT ( 'NONE',  ( -5.153800228976607833, 19.02544592524334988, 102.7094237280189759 ) ) ;
#98670=CARTESIAN_POINT ( 'NONE',  ( 10.81492255796078972, 18.62759615963270932, 89.58224293864768129 ) ) ;
#98671=CARTESIAN_POINT ( 'NONE',  ( 16.51473224551083163, -9.474510206698727899, 55.83442372801899722 ) ) ;
#98672=CARTESIAN_POINT ( 'NONE',  ( 17.48847506799970120, 5.747544572773734650, 106.6730256215672341 ) ) ;
#98673=CARTESIAN_POINT ( 'NONE',  ( 19.03943276465977164, -0.05219959533909143690, 48.74890960531435979 ) ) ;
#98674=CARTESIAN_POINT ( 'NONE',  ( -4.379528057220328563, 16.55341960407611168, 60.20724293864768839 ) ) ;
#98676=CARTESIAN_POINT ( 'NONE',  ( 16.51473224551069308, 9.474510206698969483, 44.16557627198103120 ) ) ;
#98677=CARTESIAN_POINT ( 'NONE',  ( -8.224510206698948167, 14.34966873604960824, 55.41557627198102409 ) ) ;
#98680=CARTESIAN_POINT ( 'NONE',  ( 8.224510206698953496, -14.34966873604960469, 27.91557627198103830 ) ) ;
#98681=CARTESIAN_POINT ( 'NONE',  ( -16.46253265017160317, 9.564922557960807481, 65.83224293864769550 ) ) ;
#98683=CARTESIAN_POINT ( 'NONE',  ( -13.89961937509957401, -13.97604488694547875, 34.37609039468566863 ) ) ;
#98684=CARTESIAN_POINT ( 'NONE',  ( -12.06949235617739369, -12.14591786802326823, 49.37609039468569705 ) ) ;
#98685=CARTESIAN_POINT ( 'NONE',  ( 10.81492255796078972, 18.62759615963270932, 44.58224293864769550 ) ) ;
#98686=CARTESIAN_POINT ( 'NONE',  ( 0.05219959533937995610, -21.53943276465977519, 105.0010903946856757 ) ) ;
#98687=CARTESIAN_POINT ( 'NONE',  ( 5.049401038298161559, -19.05341960407611168, 67.70724293864769550 ) ) ;
#98689=CARTESIAN_POINT ( 'NONE',  ( -16.51473224551069308, -9.474510206698971260, 96.66557627198102409 ) ) ;
#98691=CARTESIAN_POINT ( 'NONE',  ( 5.719274019375673035, 21.55341960407619339, 22.29275706135235069 ) ) ;
#98693=CARTESIAN_POINT ( 'NONE',  ( 16.55341960407611168, 4.379528057220329451, 88.95724293864769550 ) ) ;
#98694=CARTESIAN_POINT ( 'NONE',  ( 5.823673210054125526, 21.52544592524343514, 84.79057627198102409 ) ) ;
#98695=CARTESIAN_POINT ( 'NONE',  ( 13.97604488694527802, 13.89961937509977652, 79.37390960531435269 ) ) ;
#98696=CARTESIAN_POINT ( 'NONE',  ( 19.05341960407611168, 5.049401038298154454, 88.95724293864769550 ) ) ;
#98697=CARTESIAN_POINT ( 'NONE',  ( -21.55341960407610458, -5.719274019375992779, 106.4572429386477097 ) ) ;
#98699=CARTESIAN_POINT ( 'NONE',  ( 16.46253265017160672, -9.564922557960803928, 78.33224293864769550 ) ) ;
#98700=CARTESIAN_POINT ( 'NONE',  ( 19.49149378614659867, -5.499999999999673150, 96.93757513605366682 ) ) ;
#98701=CARTESIAN_POINT ( 'NONE',  ( -16.52544592524342804, 4.483927247898546575, 106.0405762719810525 ) ) ;
#98702=CARTESIAN_POINT ( 'NONE',  ( -9.474510206698964154, 16.51473224551069663, 35.41557627198102409 ) ) ;
#98703=CARTESIAN_POINT ( 'NONE',  ( -19.02544592524334988, -5.153800228976617603, 98.95942372801900433 ) ) ;
#98704=CARTESIAN_POINT ( 'NONE',  ( -4.379528057220328563, 16.55341960407611168, 115.2072429386476955 ) ) ;
#98705=CARTESIAN_POINT ( 'NONE',  ( -15.80617190586768217, 15.72974639402176855, 73.12609039468567573 ) ) ;
#98706=CARTESIAN_POINT ( 'NONE',  ( -13.97604488694527625, -13.89961937509977652, 66.87390960531436690 ) ) ;
#98707=CARTESIAN_POINT ( 'NONE',  ( -18.67979575497193778, 10.72451020669871902, 33.33442372801900433 ) ) ;
#98708=CARTESIAN_POINT ( 'NONE',  ( -5.719274019375978568, 21.55341960407610458, 115.2072429386476955 ) ) ;
#98710=CARTESIAN_POINT ( 'NONE',  ( -19.02544592524342804, 5.153800228976336051, 91.04057627198100988 ) ) ;
#98712=CARTESIAN_POINT ( 'NONE',  ( 8.314922557961029526, -14.29746914071037800, 30.41775706135234358 ) ) ;
#98713=CARTESIAN_POINT ( 'NONE',  ( -21.53943276465977519, 0.05219959533907696930, 36.24890960531435979 ) ) ;
#98714=CARTESIAN_POINT ( 'NONE',  ( 21.53943276465977519, 0.05219959533937863772, 66.25109039468567573 ) ) ;
#98715=CARTESIAN_POINT ( 'NONE',  ( -19.03943276465977164, 0.05219959533909376836, 106.2489096053143669 ) ) ;
#98716=CARTESIAN_POINT ( 'NONE',  ( 0.05219959533936267826, -19.03943276465977164, 100.0010903946856757 ) ) ;
#98717=CARTESIAN_POINT ( 'NONE',  ( 16.51473224551069308, 9.474510206698969483, 49.16557627198102409 ) ) ;
#98718=CARTESIAN_POINT ( 'NONE',  ( 5.153800228976335163, 19.02544592524342804, 79.79057627198102409 ) ) ;
#98719=CARTESIAN_POINT ( 'NONE',  ( 16.52544592524342804, -4.483927247898539470, 98.54057627198105251 ) ) ;
#98720=CARTESIAN_POINT ( 'NONE',  ( 5.049401038298163336, -19.05341960407611168, 97.70724293864768129 ) ) ;
#98721=CARTESIAN_POINT ( 'NONE',  ( 16.52544592524342804, -4.483927247898539470, 88.54057627198103830 ) ) ;
#98722=CARTESIAN_POINT ( 'NONE',  ( -9.474510206698964154, 16.51473224551069663, 115.4155762719810241 ) ) ;
#98723=CARTESIAN_POINT ( 'NONE',  ( -12.14591786802309592, -12.06949235617757132, 61.87390960531436690 ) ) ;
#98724=CARTESIAN_POINT ( 'NONE',  ( 19.05341960407611168, 5.049401038298154454, 38.95724293864767418 ) ) ;
#98725=CARTESIAN_POINT ( 'NONE',  ( -5.719274019375665041, -21.55341960407619695, 59.79275706135234714 ) ) ;
#98726=CARTESIAN_POINT ( 'NONE',  ( 5.049401038297881783, 19.05341960407617563, 92.29275706135234714 ) ) ;
#98727=CARTESIAN_POINT ( 'NONE',  ( 4.379528057220339221, -16.55341960407611168, 47.70724293864770260 ) ) ;
#98728=CARTESIAN_POINT ( 'NONE',  ( -21.53943276465977519, -0.05219959533937600094, 18.75109039468568639 ) ) ;
#98729=CARTESIAN_POINT ( 'NONE',  ( -21.55341960407610458, -5.719274019375992779, 51.45724293864770260 ) ) ;
#98731=CARTESIAN_POINT ( 'NONE',  ( -9.564922557960796823, -16.46253265017161027, 112.0822429386476955 ) ) ;
#98733=CARTESIAN_POINT ( 'NONE',  ( -13.89961937509977652, 13.97604488694528158, 50.62390960531435979 ) ) ;
#98734=CARTESIAN_POINT ( 'NONE',  ( -16.53943276465976808, 0.05219959533911058130, 21.24890960531436690 ) ) ;
#98735=CARTESIAN_POINT ( 'NONE',  ( 4.483927247898790824, -16.52544592524335698, 105.2094237280190328 ) ) ;
#98736=CARTESIAN_POINT ( 'NONE',  ( -12.06949235617739369, -12.14591786802326823, 84.37609039468570415 ) ) ;
#98737=CARTESIAN_POINT ( 'NONE',  ( -19.03943276465977164, -0.05219959533935918106, 38.75109039468566152 ) ) ;
#98739=CARTESIAN_POINT ( 'NONE',  ( 9.474510206698971260, -16.51473224551069308, 87.91557627198102409 ) ) ;
#98740=CARTESIAN_POINT ( 'NONE',  ( 13.97604488694527802, 13.89961937509977652, 54.37390960531435979 ) ) ;
#98741=CARTESIAN_POINT ( 'NONE',  ( 12.14591786802309770, 12.06949235617756955, 64.37390960531435269 ) ) ;
#98742=CARTESIAN_POINT ( 'NONE',  ( -17.49999999999999645, 5.499999999999992895, 88.71769037696435589 ) ) ;
#98743=CARTESIAN_POINT ( 'NONE',  ( -19.03943276465977164, 0.05219959533909376836, 101.2489096053143669 ) ) ;
#98744=CARTESIAN_POINT ( 'NONE',  ( -0.05219959533907301413, -21.53943276465977519, 37.49890960531436690 ) ) ;
#98745=CARTESIAN_POINT ( 'NONE',  ( -4.379528057220328563, 16.55341960407611168, 85.20724293864770971 ) ) ;
#98746=CARTESIAN_POINT ( 'NONE',  ( -8.314922557961024197, 14.29746914071037800, 37.91775706135235424 ) ) ;
#98747=CARTESIAN_POINT ( 'NONE',  ( -16.52544592524342804, 4.483927247898546575, 81.04057627198102409 ) ) ;
#98749=CARTESIAN_POINT ( 'NONE',  ( 13.89961937509957401, 13.97604488694547697, 81.87609039468564731 ) ) ;
#98750=CARTESIAN_POINT ( 'NONE',  ( 16.46253265017160672, -9.564922557960803928, 108.3322429386476955 ) ) ;
#98751=CARTESIAN_POINT ( 'NONE',  ( 19.02544592524334988, 5.153800228976608722, 81.45942372801897591 ) ) ;
#98753=CARTESIAN_POINT ( 'NONE',  ( -8.224510206698735004, -14.34966873604973081, 34.58442372801900433 ) ) ;
#98754=CARTESIAN_POINT ( 'NONE',  ( -16.53943276465976808, -0.05219959533934237506, 108.7510903946857042 ) ) ;
#98755=CARTESIAN_POINT ( 'NONE',  ( -19.03943276465977164, -0.05219959533935918106, 73.75109039468566152 ) ) ;
#98756=CARTESIAN_POINT ( 'NONE',  ( 5.823673210054125526, 21.52544592524343514, 39.79057627198103830 ) ) ;
#98757=CARTESIAN_POINT ( 'NONE',  ( -15.80617190586768217, 15.72974639402176855, 73.12609039468567573 ) ) ;
#98759=CARTESIAN_POINT ( 'NONE',  ( -14.29746914071037622, -8.314922557961029526, 34.16775706135234714 ) ) ;
#98760=CARTESIAN_POINT ( 'NONE',  ( 19.02544592524343514, -5.153800228976328945, 23.54057627198102054 ) ) ;
#98761=CARTESIAN_POINT ( 'NONE',  ( 5.153800228976335163, 19.02544592524342804, 89.79057627198102409 ) ) ;
#98762=CARTESIAN_POINT ( 'NONE',  ( 19.05341960407611168, 5.049401038298154454, 28.95724293864769550 ) ) ;
#98763=CARTESIAN_POINT ( 'NONE',  ( 4.483927247898545687, 16.52544592524342804, 89.79057627198103830 ) ) ;
#98765=CARTESIAN_POINT ( 'NONE',  ( -19.02544592524342804, 5.153800228976336051, 91.04057627198100988 ) ) ;
#98766=CARTESIAN_POINT ( 'NONE',  ( -19.05341960407617563, 5.049401038297882671, 98.54275706135233293 ) ) ;
#98767=CARTESIAN_POINT ( 'NONE',  ( -5.719274019375978568, 21.55341960407610458, 80.20724293864769550 ) ) ;
#98768=CARTESIAN_POINT ( 'NONE',  ( -5.153800228976328057, -19.02544592524343514, 42.29057627198101699 ) ) ;
#98769=CARTESIAN_POINT ( 'NONE',  ( -9.474510206698720793, -16.51473224551083518, 74.58442372801900433 ) ) ;
#98770=CARTESIAN_POINT ( 'NONE',  ( 15.80617190586769283, -15.72974639402175789, 20.62609039468568639 ) ) ;
#98771=CARTESIAN_POINT ( 'NONE',  ( -16.46253265017160317, 9.564922557960807481, 70.83224293864770971 ) ) ;
#98772=CARTESIAN_POINT ( 'NONE',  ( 19.03943276465977164, -0.05219959533909143690, 103.7489096053143669 ) ) ;
#98774=CARTESIAN_POINT ( 'NONE',  ( -12.14591786802326823, 12.06949235617739902, 33.12609039468569705 ) ) ;
#98775=CARTESIAN_POINT ( 'NONE',  ( -18.62759615963270932, 10.81492255796079327, 105.8322429386476955 ) ) ;
#98776=CARTESIAN_POINT ( 'NONE',  ( 16.55341960407611168, 4.379528057220329451, 103.9572429386476813 ) ) ;
#98777=CARTESIAN_POINT ( 'NONE',  ( 5.049401038298161559, -19.05341960407611168, 87.70724293864769550 ) ) ;
#98778=CARTESIAN_POINT ( 'NONE',  ( -16.51473224551082808, 9.474510206698731452, 63.33442372801900433 ) ) ;
#98779=CARTESIAN_POINT ( 'NONE',  ( 21.55341960407610458, 5.719274019375980345, 83.95724293864770971 ) ) ;
#98780=CARTESIAN_POINT ( 'NONE',  ( -10.81492255796078084, -18.62759615963271287, 87.08224293864769550 ) ) ;
#98781=CARTESIAN_POINT ( 'NONE',  ( -4.379528057220328563, 16.55341960407611168, 45.20724293864769550 ) ) ;
#98782=CARTESIAN_POINT ( 'NONE',  ( -0.05219959533936034679, 19.03943276465977164, 27.50109039468566507 ) ) ;
#98783=CARTESIAN_POINT ( 'NONE',  ( 16.52544592524335698, 4.483927247898782831, 71.45942372801901854 ) ) ;
#98785=CARTESIAN_POINT ( 'NONE',  ( -13.97604488694527625, -13.89961937509977652, 86.87390960531436690 ) ) ;
#98786=CARTESIAN_POINT ( 'NONE',  ( 16.51473224551069308, 9.474510206698969483, 44.16557627198103120 ) ) ;
#98787=CARTESIAN_POINT ( 'NONE',  ( 18.62759615963255655, 10.81492255796105972, 56.66775706135235424 ) ) ;
#98788=CARTESIAN_POINT ( 'NONE',  ( 10.72451020669871369, 18.67979575497193778, 67.08442372801901854 ) ) ;
#98789=CARTESIAN_POINT ( 'NONE',  ( 5.049401038298161559, -19.05341960407611168, 62.70724293864769550 ) ) ;
#98790=CARTESIAN_POINT ( 'NONE',  ( -18.62759615963255300, -10.81492255796106328, 29.16775706135234003 ) ) ;
#98791=CARTESIAN_POINT ( 'NONE',  ( -13.89961937509957401, -13.97604488694547875, 74.37609039468566152 ) ) ;
#98792=CARTESIAN_POINT ( 'NONE',  ( -13.89961937509957401, -13.97604488694547875, 74.37609039468566152 ) ) ;
#98793=CARTESIAN_POINT ( 'NONE',  ( 9.564922557960805705, 16.46253265017160317, 44.58224293864769550 ) ) ;
#98794=CARTESIAN_POINT ( 'NONE',  ( 0.05219959533934541429, -16.53943276465976808, 85.00109039468568994 ) ) ;
#98795=CARTESIAN_POINT ( 'NONE',  ( 13.97604488694527802, 13.89961937509977652, 59.37390960531434558 ) ) ;
#98797=CARTESIAN_POINT ( 'NONE',  ( -9.474510206698964154, 16.51473224551069663, 95.41557627198102409 ) ) ;
#98798=CARTESIAN_POINT ( 'NONE',  ( -9.564922557960796823, -16.46253265017161027, 32.08224293864769550 ) ) ;
#98799=CARTESIAN_POINT ( 'NONE',  ( -21.52544592524343514, 5.823673210054127303, 91.04057627198103830 ) ) ;
#98800=CARTESIAN_POINT ( 'NONE',  ( 14.34966873604972726, -8.224510206698740333, 60.83442372801901854 ) ) ;
#98801=CARTESIAN_POINT ( 'NONE',  ( 13.97604488694548053, -13.89961937509957401, 30.62609039468566863 ) ) ;
#98802=CARTESIAN_POINT ( 'NONE',  ( 9.474510206698971260, -16.51473224551069308, 52.91557627198102409 ) ) ;
#98803=CARTESIAN_POINT ( 'NONE',  ( -16.53943276465976808, 0.05219959533911058130, 51.24890960531436690 ) ) ;
#98804=CARTESIAN_POINT ( 'NONE',  ( 14.34966873604960469, 8.224510206698951720, 79.16557627198103830 ) ) ;
#98805=CARTESIAN_POINT ( 'NONE',  ( 16.51473224551069308, 9.474510206698969483, 74.16557627198103830 ) ) ;
#98806=CARTESIAN_POINT ( 'NONE',  ( 21.52544592524334988, 5.823673210054432836, 41.45942372801901143 ) ) ;
#98807=CARTESIAN_POINT ( 'NONE',  ( -16.51473224551069308, -9.474510206698971260, 86.66557627198102409 ) ) ;
#98808=CARTESIAN_POINT ( 'NONE',  ( -10.81492255796105439, 18.62759615963255655, 97.91775706135236135 ) ) ;
#98809=CARTESIAN_POINT ( 'NONE',  ( 12.14591786802327356, -12.06949235617739191, 75.62609039468567573 ) ) ;
#98811=CARTESIAN_POINT ( 'NONE',  ( -21.55341960407619339, 5.719274019375674811, 23.54275706135235424 ) ) ;
#98812=CARTESIAN_POINT ( 'NONE',  ( 21.53943276465977519, -0.05219959533907433946, 93.74890960531436690 ) ) ;
#98813=CARTESIAN_POINT ( 'NONE',  ( 4.379528057220339221, -16.55341960407611168, 42.70724293864770260 ) ) ;
#98814=CARTESIAN_POINT ( 'NONE',  ( -16.46253265017160317, 9.564922557960807481, 45.83224293864769550 ) ) ;
#98815=CARTESIAN_POINT ( 'NONE',  ( -16.53943276465976808, 0.05219959533911058130, 66.24890960531436690 ) ) ;
#98816=CARTESIAN_POINT ( 'NONE',  ( -21.52544592524343514, 5.823673210054127303, 36.04057627198102409 ) ) ;
#98817=CARTESIAN_POINT ( 'NONE',  ( -5.049401038297874678, -19.05341960407617918, 34.79275706135233293 ) ) ;
#98818=CARTESIAN_POINT ( 'NONE',  ( -16.55341960407611168, -4.379528057220339221, 106.4572429386477097 ) ) ;
#98819=CARTESIAN_POINT ( 'NONE',  ( 9.474510206698971260, -16.51473224551069308, 107.9155762719810383 ) ) ;
#98821=CARTESIAN_POINT ( 'NONE',  ( -12.14591786802326823, 12.06949235617739902, 48.12609039468568284 ) ) ;
#98822=CARTESIAN_POINT ( 'NONE',  ( 16.51473224551069308, 9.474510206698969483, 54.16557627198103120 ) ) ;
#98823=CARTESIAN_POINT ( 'NONE',  ( -17.30380112737341136, -6.006629661696645250, 21.28751624816027288 ) ) ;
#98824=CARTESIAN_POINT ( 'NONE',  ( -14.34966873604972548, 8.224510206698743886, 88.33442372801901854 ) ) ;
#98825=CARTESIAN_POINT ( 'NONE',  ( -5.049401038297874678, -19.05341960407617918, 109.7927570613523187 ) ) ;
#98826=CARTESIAN_POINT ( 'NONE',  ( -5.823673210054431948, 21.52544592524334988, 82.70942372801900433 ) ) ;
#98827=CARTESIAN_POINT ( 'NONE',  ( -9.564922557960796823, -16.46253265017161027, 77.08224293864769550 ) ) ;
#98828=CARTESIAN_POINT ( 'NONE',  ( 21.53943276465977519, -0.05219959533907433946, 108.7489096053143669 ) ) ;
#98829=CARTESIAN_POINT ( 'NONE',  ( 8.224510206698742110, 14.34966873604972548, 52.08442372801901854 ) ) ;
#98830=CARTESIAN_POINT ( 'NONE',  ( -16.51473224551069308, -9.474510206698971260, 21.66557627198102765 ) ) ;
#98832=CARTESIAN_POINT ( 'NONE',  ( -4.379528057220086978, -16.55341960407618274, 19.79275706135235069 ) ) ;
#98833=CARTESIAN_POINT ( 'NONE',  ( 0.05219959533936267826, -19.03943276465977164, 80.00109039468567573 ) ) ;
#98834=CARTESIAN_POINT ( 'NONE',  ( 21.52544592524344225, -5.823673210054117533, 83.54057627198102409 ) ) ;
#98835=CARTESIAN_POINT ( 'NONE',  ( -19.03943276465977164, -0.05219959533935918106, 53.75109039468566863 ) ) ;
#98836=CARTESIAN_POINT ( 'NONE',  ( 18.22780087662123805, -5.499999999999976019, 88.51763182126893525 ) ) ;
#98837=CARTESIAN_POINT ( 'NONE',  ( -5.719274019375978568, 21.55341960407610458, 105.2072429386477097 ) ) ;
#98838=CARTESIAN_POINT ( 'NONE',  ( 18.09867054820433907, 5.499999999999818812, 61.48393025253584909 ) ) ;
#98839=CARTESIAN_POINT ( 'NONE',  ( 16.46253265017160672, -9.564922557960803928, 68.33224293864770971 ) ) ;
#98841=CARTESIAN_POINT ( 'NONE',  ( -8.224510206698735004, -14.34966873604973081, 24.58442372801901499 ) ) ;
#98843=CARTESIAN_POINT ( 'NONE',  ( 10.81492255796106328, -18.62759615963255655, 55.41775706135234714 ) ) ;
#98844=CARTESIAN_POINT ( 'NONE',  ( 0.05219959533907565091, 21.53943276465977519, 104.9989096053143669 ) ) ;
#98845=CARTESIAN_POINT ( 'NONE',  ( 0.05219959533910956823, 16.53943276465976808, 59.99890960531436690 ) ) ;
#98846=CARTESIAN_POINT ( 'NONE',  ( 19.02544592524343514, -5.153800228976328945, 68.54057627198103830 ) ) ;
#98847=CARTESIAN_POINT ( 'NONE',  ( -21.53943276465977519, -0.05219959533937600094, 78.75109039468568994 ) ) ;
#98848=CARTESIAN_POINT ( 'NONE',  ( -0.05219959533934338120, 16.53943276465976808, 27.50109039468567929 ) ) ;
#98849=CARTESIAN_POINT ( 'NONE',  ( 19.02544592524334988, 5.153800228976608722, 31.45942372801900433 ) ) ;
#98850=CARTESIAN_POINT ( 'NONE',  ( -5.823673210054431948, 21.52544592524334988, 52.70942372801902565 ) ) ;
#98851=CARTESIAN_POINT ( 'NONE',  ( 21.55341960407610458, 5.719274019375980345, 113.9572429386477239 ) ) ;
#98852=CARTESIAN_POINT ( 'NONE',  ( 0.05219959533907565091, 21.53943276465977519, 59.99890960531436690 ) ) ;
#98853=CARTESIAN_POINT ( 'NONE',  ( -5.049401038297874678, -19.05341960407617918, 94.79275706135230450 ) ) ;
#98854=CARTESIAN_POINT ( 'NONE',  ( -13.97604488694547697, 13.89961937509957934, 73.12609039468568994 ) ) ;
#98855=CARTESIAN_POINT ( 'NONE',  ( -18.62759615963255300, -10.81492255796106328, 79.16775706135234714 ) ) ;
#98856=CARTESIAN_POINT ( 'NONE',  ( -16.51473224551082808, 9.474510206698731452, 58.33442372801900433 ) ) ;
#98857=CARTESIAN_POINT ( 'NONE',  ( -13.97604488694527625, -13.89961937509977652, 36.87390960531436690 ) ) ;
#98858=CARTESIAN_POINT ( 'NONE',  ( -21.53943276465977519, 0.05219959533907696930, 56.24890960531436690 ) ) ;
#98859=CARTESIAN_POINT ( 'NONE',  ( -16.52544592524342804, 4.483927247898546575, 51.04057627198103120 ) ) ;
#98860=CARTESIAN_POINT ( 'NONE',  ( -17.44279575226824619, -5.990770900252396558, 24.16442432485681735 ) ) ;
#98861=CARTESIAN_POINT ( 'NONE',  ( 13.97604488694548053, -13.89961937509957401, 35.62609039468567573 ) ) ;
#98862=CARTESIAN_POINT ( 'NONE',  ( -14.29746914071037622, -8.314922557961029526, 84.16775706135234714 ) ) ;
#98863=CARTESIAN_POINT ( 'NONE',  ( -14.34966873604960291, -8.224510206698953496, 56.66557627198103830 ) ) ;
#98864=CARTESIAN_POINT ( 'NONE',  ( -21.52544592524334988, -5.823673210054445271, 93.95942372801903275 ) ) ;
#98865=CARTESIAN_POINT ( 'NONE',  ( -18.67979575497193778, 10.72451020669871902, 83.33442372801903275 ) ) ;
#98866=CARTESIAN_POINT ( 'NONE',  ( -15.72974639402197994, 15.80617190586746368, 85.62390960531436690 ) ) ;
#98867=CARTESIAN_POINT ( 'NONE',  ( -0.05219959533909027116, -19.03943276465977164, 57.49890960531435979 ) ) ;
#98868=CARTESIAN_POINT ( 'NONE',  ( 10.81492255796106328, -18.62759615963255655, 55.41775706135234714 ) ) ;
#98869=CARTESIAN_POINT ( 'NONE',  ( -0.05219959533909027116, -19.03943276465977164, 32.49890960531435979 ) ) ;
#98870=CARTESIAN_POINT ( 'NONE',  ( -5.153800228976328057, -19.02544592524343514, 52.29057627198100988 ) ) ;
#98871=CARTESIAN_POINT ( 'NONE',  ( 8.314922557960818139, 14.29746914071049879, 104.5822429386477097 ) ) ;
#98872=CARTESIAN_POINT ( 'NONE',  ( 19.03943276465977164, -0.05219959533909143690, 98.74890960531436690 ) ) ;
#98873=CARTESIAN_POINT ( 'NONE',  ( -14.34966873604960291, -8.224510206698953496, 56.66557627198103830 ) ) ;
#98874=CARTESIAN_POINT ( 'NONE',  ( 8.314922557960818139, 14.29746914071049879, 109.5822429386476955 ) ) ;
#98875=CARTESIAN_POINT ( 'NONE',  ( -21.53943276465977519, 0.05219959533907696930, 86.24890960531436690 ) ) ;
#98877=CARTESIAN_POINT ( 'NONE',  ( 21.55341960407610458, 5.719274019375980345, 113.9572429386477239 ) ) ;
#98880=CARTESIAN_POINT ( 'NONE',  ( 16.53943276465976808, 0.05219959533934440121, 41.25109039468568284 ) ) ;
#98881=ORIENTED_EDGE ( 'NONE', *, *, #34959, .F. ) ;
#98882=CARTESIAN_POINT ( 'NONE',  ( 10.81492255796078972, 18.62759615963270932, 69.58224293864769550 ) ) ;
#98883=CARTESIAN_POINT ( 'NONE',  ( -10.81492255796105439, 18.62759615963255655, 107.9177570613523471 ) ) ;
#98884=CARTESIAN_POINT ( 'NONE',  ( -19.05341960407611168, -5.049401038298163336, 91.45724293864766707 ) ) ;
#98885=CARTESIAN_POINT ( 'NONE',  ( 5.719274019375673035, 21.55341960407619339, 32.29275706135235424 ) ) ;
#98886=CARTESIAN_POINT ( 'NONE',  ( 5.719274019375991003, -21.55341960407610458, 27.70724293864769905 ) ) ;
#98887=CARTESIAN_POINT ( 'NONE',  ( 8.224510206698742110, 14.34966873604972548, 107.0844237280190043 ) ) ;
#98888=CARTESIAN_POINT ( 'NONE',  ( 5.823673210054444382, -21.52544592524334988, 90.20942372801903275 ) ) ;
#98889=CARTESIAN_POINT ( 'NONE',  ( 18.62759615963255655, 10.81492255796105972, 106.6677570613523756 ) ) ;
#98890=CARTESIAN_POINT ( 'NONE',  ( -16.55341960407617563, 4.379528057220093196, 68.54275706135234714 ) ) ;
#98891=CARTESIAN_POINT ( 'NONE',  ( 21.55341960407619695, -5.719274019375665929, 31.04275706135234714 ) ) ;
#98892=CARTESIAN_POINT ( 'NONE',  ( 19.03943276465977164, -0.05219959533909143690, 33.74890960531435979 ) ) ;
#98893=CARTESIAN_POINT ( 'NONE',  ( 5.719274019375673035, 21.55341960407619339, 107.2927570613523471 ) ) ;
#98894=CARTESIAN_POINT ( 'NONE',  ( -19.05341960407611168, -5.049401038298163336, 111.4572429386476671 ) ) ;
#98895=CARTESIAN_POINT ( 'NONE',  ( -18.67979575497178146, -10.72451020669898902, 101.6655762719810383 ) ) ;
#98897=CARTESIAN_POINT ( 'NONE',  ( 21.55341960407610458, 5.719274019375980345, 68.95724293864769550 ) ) ;
#98898=CARTESIAN_POINT ( 'NONE',  ( 12.14591786802327356, -12.06949235617739191, 55.62609039468568284 ) ) ;
#98899=CARTESIAN_POINT ( 'NONE',  ( -16.53943276465976808, 0.05219959533911058130, 51.24890960531436690 ) ) ;
#98900=CARTESIAN_POINT ( 'NONE',  ( 18.59930490233255540, -5.499999999999989342, 101.0584990050579250 ) ) ;
#98901=CARTESIAN_POINT ( 'NONE',  ( 19.02544592524334988, 5.153800228976608722, 76.45942372801897591 ) ) ;
#98902=CARTESIAN_POINT ( 'NONE',  ( -16.21995358207305316, 7.366697692864160985, 104.9355100151216220 ) ) ;
#98903=CARTESIAN_POINT ( 'NONE',  ( -4.483927247898782831, 16.52544592524335698, 27.70942372801901854 ) ) ;
#98905=CARTESIAN_POINT ( 'NONE',  ( 18.62759615963271287, -10.81492255796078972, 98.33224293864769550 ) ) ;
#98906=CARTESIAN_POINT ( 'NONE',  ( -14.29746914071049879, 8.314922557960819915, 60.83224293864769550 ) ) ;
#98907=CARTESIAN_POINT ( 'NONE',  ( 19.03943276465977164, -0.05219959533909143690, 113.7489096053143669 ) ) ;
#98908=CARTESIAN_POINT ( 'NONE',  ( 14.29746914071037800, 8.314922557961029526, 41.66775706135235424 ) ) ;
#98909=CARTESIAN_POINT ( 'NONE',  ( -19.03943276465977164, 0.05219959533909376836, 61.24890960531436690 ) ) ;
#98910=CARTESIAN_POINT ( 'NONE',  ( -21.52544592524334988, -5.823673210054445271, 28.95942372801902209 ) ) ;
#98911=CARTESIAN_POINT ( 'NONE',  ( -13.97604488694547697, 13.89961937509957934, 98.12609039468566152 ) ) ;
#98912=CARTESIAN_POINT ( 'NONE',  ( -5.049401038298153566, 19.05341960407611168, 95.20724293864770971 ) ) ;
#98914=CARTESIAN_POINT ( 'NONE',  ( 19.03943276465977164, -0.05219959533909143690, 88.74890960531436690 ) ) ;
#98915=CARTESIAN_POINT ( 'NONE',  ( 21.53943276465977519, -0.05219959533907433946, 88.74890960531436690 ) ) ;
#98916=CARTESIAN_POINT ( 'NONE',  ( 9.474510206698971260, -16.51473224551069308, 42.91557627198103120 ) ) ;
#98917=CARTESIAN_POINT ( 'NONE',  ( -16.38665767535053774, -7.295008042176054808, 59.73599135785457293 ) ) ;
#98918=CARTESIAN_POINT ( 'NONE',  ( 16.52544592524342804, -4.483927247898539470, 68.54057627198103830 ) ) ;
#98919=CARTESIAN_POINT ( 'NONE',  ( 19.05341960407611168, 5.049401038298154454, 103.9572429386476671 ) ) ;
#98921=CARTESIAN_POINT ( 'NONE',  ( 5.153800228976615827, -19.02544592524334988, 85.20942372801900433 ) ) ;
#98922=CARTESIAN_POINT ( 'NONE',  ( -15.80617190586745835, -15.72974639402198527, 96.87390960531436690 ) ) ;
#98923=CARTESIAN_POINT ( 'NONE',  ( 13.89961937509957401, 13.97604488694547697, 51.87609039468566863 ) ) ;
#98924=CARTESIAN_POINT ( 'NONE',  ( -5.049401038298153566, 19.05341960407611168, 110.2072429386476671 ) ) ;
#98926=CARTESIAN_POINT ( 'NONE',  ( -10.72451020669898014, 18.67979575497178502, 50.41557627198103120 ) ) ;
#98927=CARTESIAN_POINT ( 'NONE',  ( -19.05341960407611168, -5.049401038298163336, 86.45724293864769550 ) ) ;
#98928=CARTESIAN_POINT ( 'NONE',  ( -15.72974639402176322, -15.80617190586768395, 74.37609039468568994 ) ) ;
#98929=CARTESIAN_POINT ( 'NONE',  ( -5.153800228976328057, -19.02544592524343514, 42.29057627198101699 ) ) ;
#98930=CARTESIAN_POINT ( 'NONE',  ( 12.14591786802309770, 12.06949235617756955, 74.37390960531436690 ) ) ;
#98931=CARTESIAN_POINT ( 'NONE',  ( -4.483927247898782831, 16.52544592524335698, 27.70942372801901854 ) ) ;
#98932=CARTESIAN_POINT ( 'NONE',  ( -10.72451020669870658, -18.67979575497194134, 64.58442372801900433 ) ) ;
#98933=EDGE_LOOP ( 'NONE', ( #89320, #123949, #40034 ) ) ;
#98934=CARTESIAN_POINT ( 'NONE',  ( 19.03943276465977164, -0.05219959533909143690, 113.7489096053143669 ) ) ;
#98935=CARTESIAN_POINT ( 'NONE',  ( 9.474510206698729675, 16.51473224551082808, 77.08442372801900433 ) ) ;
#98937=CARTESIAN_POINT ( 'NONE',  ( -21.53943276465977519, -0.05219959533937600094, 28.75109039468567929 ) ) ;
#98939=CARTESIAN_POINT ( 'NONE',  ( -16.46253265017146816, -9.564922557961047289, 19.16775706135233293 ) ) ;
#98940=CARTESIAN_POINT ( 'NONE',  ( 16.46253265017160672, -9.564922557960803928, 58.33224293864769550 ) ) ;
#98941=CARTESIAN_POINT ( 'NONE',  ( 21.52544592524334988, 5.823673210054432836, 106.4594237280190328 ) ) ;
#98942=CARTESIAN_POINT ( 'NONE',  ( 8.224510206698742110, 14.34966873604972548, 107.0844237280190043 ) ) ;
#98943=CARTESIAN_POINT ( 'NONE',  ( 9.474510206698971260, -16.51473224551069308, 102.9155762719810241 ) ) ;
#98944=CARTESIAN_POINT ( 'NONE',  ( 15.72974639402176855, 15.80617190586768217, 76.87609039468567573 ) ) ;
#98945=B_SPLINE_CURVE_WITH_KNOTS ( 'NONE', 3,
 ( #38845, #127837, #190529, #51015, #130837, #54011, #115685, #82319, #144009, #5490, #52003, #36824, #160183, #186076, #46554, #107215, #185066, #45561, #40840, #132844 ),
 .UNSPECIFIED., .F., .F.,
 ( 4, 2, 2, 2, 2, 2, 2, 2, 2, 4 ),
 ( 0.004000878361811842886, 0.004499404418915854513, 0.004997930476019866140, 0.005496456533123877768, 0.005994982590227890262, 0.006244245618779896076, 0.006493508647331901022, 0.006992034704435916986, 0.007490560761539932083, 0.007989086818643948915 ),
 .UNSPECIFIED. ) ;
#98948=CARTESIAN_POINT ( 'NONE',  ( -18.10062525802553424, 5.500000000000031086, 78.51383468041922242 ) ) ;
#98949=CARTESIAN_POINT ( 'NONE',  ( 5.823673210054444382, -21.52544592524334988, 75.20942372801901854 ) ) ;
#98950=CARTESIAN_POINT ( 'NONE',  ( -21.53943276465977519, -0.05219959533937600094, 98.75109039468568994 ) ) ;
#98952=CARTESIAN_POINT ( 'NONE',  ( 9.474510206698971260, -16.51473224551069308, 92.91557627198103830 ) ) ;
#98953=CARTESIAN_POINT ( 'NONE',  ( -21.55341960407619339, 5.719274019375674811, 113.5427570613523756 ) ) ;
#98955=CARTESIAN_POINT ( 'NONE',  ( -13.89961937509977652, 13.97604488694528158, 35.62390960531435269 ) ) ;
#98956=CARTESIAN_POINT ( 'NONE',  ( -15.80617190586745835, -15.72974639402198527, 51.87390960531437401 ) ) ;
#98957=CARTESIAN_POINT ( 'NONE',  ( 16.53943276465976808, 0.05219959533934440121, 101.2510903946856757 ) ) ;
#98958=CARTESIAN_POINT ( 'NONE',  ( 16.52544592524342804, -4.483927247898539470, 103.5405762719810383 ) ) ;
#98959=CARTESIAN_POINT ( 'NONE',  ( -9.474510206698964154, 16.51473224551069663, 85.41557627198102409 ) ) ;
#98960=CARTESIAN_POINT ( 'NONE',  ( -10.81492255796105439, 18.62759615963255655, 97.91775706135236135 ) ) ;
#98961=CARTESIAN_POINT ( 'NONE',  ( 13.97604488694527802, 13.89961937509977652, 34.37390960531436690 ) ) ;
#98962=CARTESIAN_POINT ( 'NONE',  ( 14.29746914071049879, -8.314922557960816363, 103.3322429386476955 ) ) ;
#98963=CARTESIAN_POINT ( 'NONE',  ( -15.72974639402176322, -15.80617190586768395, 54.37609039468568994 ) ) ;
#98964=CARTESIAN_POINT ( 'NONE',  ( -21.55341960407610458, -5.719274019375992779, 86.45724293864770971 ) ) ;
#98965=CARTESIAN_POINT ( 'NONE',  ( 16.46253265017146816, 9.564922557961045513, 46.66775706135233293 ) ) ;
#98966=CARTESIAN_POINT ( 'NONE',  ( 5.049401038298163336, -19.05341960407611168, 47.70724293864769550 ) ) ;
#98967=CARTESIAN_POINT ( 'NONE',  ( -19.03943276465977164, 0.05219959533909376836, 96.24890960531436690 ) ) ;
#98968=CARTESIAN_POINT ( 'NONE',  ( 12.06949235617757843, -12.14591786802309237, 73.12390960531436690 ) ) ;
#98969=CARTESIAN_POINT ( 'NONE',  ( 13.89961937509957401, 13.97604488694547697, 41.87609039468566152 ) ) ;
#98970=CARTESIAN_POINT ( 'NONE',  ( -0.05219959533909027116, -19.03943276465977164, 57.49890960531435979 ) ) ;
#98971=CARTESIAN_POINT ( 'NONE',  ( 16.53943276465976808, -0.05219959533910856209, 43.74890960531435979 ) ) ;
#98972=CARTESIAN_POINT ( 'NONE',  ( 19.02544592524334988, 5.153800228976608722, 81.45942372801897591 ) ) ;
#98974=CARTESIAN_POINT ( 'NONE',  ( 5.719274019375991003, -21.55341960407610458, 32.70724293864770260 ) ) ;
#98975=CARTESIAN_POINT ( 'NONE',  ( 8.224510206698953496, -14.34966873604960469, 102.9155762719810383 ) ) ;
#98976=CARTESIAN_POINT ( 'NONE',  ( -17.49999999999996447, -4.640572885337702402, 24.36211835451159402 ) ) ;
#98977=CARTESIAN_POINT ( 'NONE',  ( 16.46253265017160672, -9.564922557960803928, 58.33224293864769550 ) ) ;
#98978=CARTESIAN_POINT ( 'NONE',  ( -18.67979575497178146, -10.72451020669898902, 61.66557627198103120 ) ) ;
#98979=CARTESIAN_POINT ( 'NONE',  ( 9.564922557960805705, 16.46253265017160317, 29.58224293864769550 ) ) ;
#98980=CARTESIAN_POINT ( 'NONE',  ( 16.52544592524335698, 4.483927247898782831, 81.45942372801900433 ) ) ;
#98981=CARTESIAN_POINT ( 'NONE',  ( -9.474510206698964154, 16.51473224551069663, 65.41557627198102409 ) ) ;
#98982=CARTESIAN_POINT ( 'NONE',  ( -5.049401038297874678, -19.05341960407617918, 39.79275706135232582 ) ) ;
#98983=CARTESIAN_POINT ( 'NONE',  ( 21.55341960407619695, -5.719274019375665929, 71.04275706135234714 ) ) ;
#98985=CARTESIAN_POINT ( 'NONE',  ( -0.05219959533907301413, -21.53943276465977519, 47.49890960531435979 ) ) ;
#98986=CARTESIAN_POINT ( 'NONE',  ( -0.05219959533909027116, -19.03943276465977164, 27.49890960531435624 ) ) ;
#98987=CARTESIAN_POINT ( 'NONE',  ( 8.224510206698742110, 14.34966873604972548, 92.08442372801901854 ) ) ;
#98988=CARTESIAN_POINT ( 'NONE',  ( -5.049401038297874678, -19.05341960407617918, 99.79275706135234714 ) ) ;
#98989=CARTESIAN_POINT ( 'NONE',  ( -19.05341960407611168, -5.049401038298163336, 21.45724293864768839 ) ) ;
#98991=CARTESIAN_POINT ( 'NONE',  ( 5.719274019375991003, -21.55341960407610458, 47.70724293864770260 ) ) ;
#98992=CARTESIAN_POINT ( 'NONE',  ( -21.55341960407619339, 5.719274019375674811, 83.54275706135234714 ) ) ;
#98993=CARTESIAN_POINT ( 'NONE',  ( 12.14591786802309770, 12.06949235617756955, 49.37390960531436690 ) ) ;
#98994=CARTESIAN_POINT ( 'NONE',  ( -12.14591786802309592, -12.06949235617757132, 56.87390960531436690 ) ) ;
#98995=CARTESIAN_POINT ( 'NONE',  ( 18.67979575497178502, 10.72451020669898547, 84.16557627198103830 ) ) ;
#98996=CARTESIAN_POINT ( 'NONE',  ( 15.80617190586746368, 15.72974639402197994, 74.37390960531436690 ) ) ;
#98998=CARTESIAN_POINT ( 'NONE',  ( -10.81492255796078084, -18.62759615963271287, 32.08224293864769550 ) ) ;
#98999=CARTESIAN_POINT ( 'NONE',  ( -16.53943276465976808, -0.05219959533934237506, 68.75109039468568994 ) ) ;
#99000=CARTESIAN_POINT ( 'NONE',  ( 14.34966873604960469, 8.224510206698951720, 74.16557627198102409 ) ) ;
#99001=CARTESIAN_POINT ( 'NONE',  ( -9.564922557960796823, -16.46253265017161027, 32.08224293864769550 ) ) ;
#99002=DIRECTION ( 'NONE',  ( 0.000000000000000000, 1.000000000000000000, 0.000000000000000000 ) ) ;
#99003=ORIENTED_EDGE ( 'NONE', *, *, #146110, .T. ) ;
#99004=CARTESIAN_POINT ( 'NONE',  ( 16.53943276465976808, 0.05219959533934440121, 86.25109039468568994 ) ) ;
#99005=CARTESIAN_POINT ( 'NONE',  ( 15.72974639402176855, 15.80617190586768217, 21.87609039468567573 ) ) ;
#99006=CARTESIAN_POINT ( 'NONE',  ( -0.05219959533909027116, -19.03943276465977164, 82.49890960531436690 ) ) ;
#99007=CARTESIAN_POINT ( 'NONE',  ( 21.55341960407619695, -5.719274019375665929, 51.04275706135234714 ) ) ;
#99008=CARTESIAN_POINT ( 'NONE',  ( -5.049401038298153566, 19.05341960407611168, 105.2072429386476671 ) ) ;
#99010=ORIENTED_EDGE ( 'NONE', *, *, #128971, .F. ) ;
#99011=CARTESIAN_POINT ( 'NONE',  ( -0.05219959533937732626, 21.53943276465977519, 42.50109039468567573 ) ) ;
#99012=CARTESIAN_POINT ( 'NONE',  ( -19.02544592524342804, 5.153800228976336051, 36.04057627198100988 ) ) ;
#99013=CARTESIAN_POINT ( 'NONE',  ( -19.03943276465977164, 0.05219959533909376836, 106.2489096053143669 ) ) ;
#99014=CARTESIAN_POINT ( 'NONE',  ( -19.05341960407617563, 5.049401038297882671, 48.54275706135233293 ) ) ;
#99015=CARTESIAN_POINT ( 'NONE',  ( 10.72451020669871369, 18.67979575497193778, 27.08442372801901854 ) ) ;
#99016=CARTESIAN_POINT ( 'NONE',  ( 13.89961937509957401, 13.97604488694547697, 46.87609039468565442 ) ) ;
#99017=CARTESIAN_POINT ( 'NONE',  ( 0.05219959533909260263, 19.03943276465977164, 24.99890960531435269 ) ) ;
#99018=CARTESIAN_POINT ( 'NONE',  ( -8.224510206698735004, -14.34966873604973081, 94.58442372801901854 ) ) ;
#99019=CARTESIAN_POINT ( 'NONE',  ( 0.05219959533936267826, -19.03943276465977164, 60.00109039468566863 ) ) ;
#99020=CARTESIAN_POINT ( 'NONE',  ( 12.14591786802327356, -12.06949235617739191, 105.6260903946856899 ) ) ;
#99022=CARTESIAN_POINT ( 'NONE',  ( -16.51473224551069308, -9.474510206698971260, 86.66557627198102409 ) ) ;
#99024=CARTESIAN_POINT ( 'NONE',  ( 10.72451020669871369, 18.67979575497193778, 92.08442372801901854 ) ) ;
#99025=CARTESIAN_POINT ( 'NONE',  ( -15.72974639402176322, -15.80617190586768395, 109.3760903946857042 ) ) ;
#99027=CARTESIAN_POINT ( 'NONE',  ( 19.05341960407611168, 5.049401038298154454, 103.9572429386476671 ) ) ;
#99028=CARTESIAN_POINT ( 'NONE',  ( 5.823673210054444382, -21.52544592524334988, 70.20942372801904696 ) ) ;
#99029=CARTESIAN_POINT ( 'NONE',  ( 13.89961937509957401, 13.97604488694547697, 111.8760903946856757 ) ) ;
#99030=CARTESIAN_POINT ( 'NONE',  ( -5.049401038298153566, 19.05341960407611168, 85.20724293864766707 ) ) ;
#99031=CARTESIAN_POINT ( 'NONE',  ( 18.67979575497178502, 10.72451020669898547, 34.16557627198102409 ) ) ;
#99032=CARTESIAN_POINT ( 'NONE',  ( 16.51473224551069308, 9.474510206698969483, 94.16557627198103830 ) ) ;
#99033=CARTESIAN_POINT ( 'NONE',  ( -16.62475595723696387, -7.163666690055378261, 89.47286648189532343 ) ) ;
#99034=CARTESIAN_POINT ( 'NONE',  ( -0.05219959533909027116, -19.03943276465977164, 72.49890960531435269 ) ) ;
#99035=CARTESIAN_POINT ( 'NONE',  ( 19.02544592524343514, -5.153800228976328945, 68.54057627198103830 ) ) ;
#99036=CARTESIAN_POINT ( 'NONE',  ( 14.29746914071037800, 8.314922557961029526, 101.6677570613523613 ) ) ;
#99037=CARTESIAN_POINT ( 'NONE',  ( -16.38665767534994444, 7.295008042176405638, 100.2640086421446597 ) ) ;
#99038=CARTESIAN_POINT ( 'NONE',  ( 0.05219959533936267826, -19.03943276465977164, 70.00109039468566152 ) ) ;
#99039=CARTESIAN_POINT ( 'NONE',  ( -5.153800228976328057, -19.02544592524343514, 87.29057627198103830 ) ) ;
#99040=CARTESIAN_POINT ( 'NONE',  ( 8.224510206698953496, -14.34966873604960469, 82.91557627198103830 ) ) ;
#99041=CARTESIAN_POINT ( 'NONE',  ( -18.62759615963270932, 10.81492255796079327, 35.83224293864768839 ) ) ;
#99042=CARTESIAN_POINT ( 'NONE',  ( -19.02544592524342804, 5.153800228976336051, 116.0405762719810383 ) ) ;
#99043=CARTESIAN_POINT ( 'NONE',  ( -0.05219959533910754901, -16.53943276465976808, 107.4989096053143669 ) ) ;
#99045=CARTESIAN_POINT ( 'NONE',  ( 5.049401038297881783, 19.05341960407617563, 47.29275706135231161 ) ) ;
#99046=CARTESIAN_POINT ( 'NONE',  ( -4.379528057220328563, 16.55341960407611168, 25.20724293864769550 ) ) ;
#99047=CARTESIAN_POINT ( 'NONE',  ( 5.049401038298161559, -19.05341960407611168, 102.7072429386476955 ) ) ;
#99049=CARTESIAN_POINT ( 'NONE',  ( -21.53943276465977519, -0.05219959533937600094, 63.75109039468568284 ) ) ;
#99050=CARTESIAN_POINT ( 'NONE',  ( -21.53943276465977519, 0.05219959533907696930, 56.24890960531436690 ) ) ;
#99051=CARTESIAN_POINT ( 'NONE',  ( 15.72974639402176855, 15.80617190586768217, 36.87609039468568994 ) ) ;
#99052=CARTESIAN_POINT ( 'NONE',  ( 21.52544592524344225, -5.823673210054117533, 88.54057627198103830 ) ) ;
#99053=CARTESIAN_POINT ( 'NONE',  ( 21.52544592524334988, 5.823673210054432836, 36.45942372801901143 ) ) ;
#99055=CARTESIAN_POINT ( 'NONE',  ( -12.06949235617756955, 12.14591786802309770, 110.6239096053143669 ) ) ;
#99056=CARTESIAN_POINT ( 'NONE',  ( 19.03943276465977164, 0.05219959533936151252, 66.25109039468567573 ) ) ;
#99057=CARTESIAN_POINT ( 'NONE',  ( 16.51473224551069308, 9.474510206698969483, 44.16557627198103120 ) ) ;
#99058=CARTESIAN_POINT ( 'NONE',  ( -14.34966873604960291, -8.224510206698953496, 86.66557627198102409 ) ) ;
#99059=CARTESIAN_POINT ( 'NONE',  ( 0.05219959533909260263, 19.03943276465977164, 94.99890960531436690 ) ) ;
#99060=CARTESIAN_POINT ( 'NONE',  ( 16.51473224551069308, 9.474510206698969483, 114.1655762719810241 ) ) ;
#99061=CARTESIAN_POINT ( 'NONE',  ( 19.03943276465977164, -0.05219959533909143690, 28.74890960531435624 ) ) ;
#99062=CARTESIAN_POINT ( 'NONE',  ( -14.34966873604960291, -8.224510206698953496, 36.66557627198103120 ) ) ;
#99063=CARTESIAN_POINT ( 'NONE',  ( 8.314922557961029526, -14.29746914071037800, 100.4177570613523471 ) ) ;
#99064=CARTESIAN_POINT ( 'NONE',  ( -9.564922557960796823, -16.46253265017161027, 52.08224293864768839 ) ) ;
#99065=CARTESIAN_POINT ( 'NONE',  ( -19.03943276465977164, 0.05219959533909376836, 26.24890960531435624 ) ) ;
#99066=CARTESIAN_POINT ( 'NONE',  ( 5.049401038297881783, 19.05341960407617563, 27.29275706135232937 ) ) ;
#99067=CARTESIAN_POINT ( 'NONE',  ( 13.97604488694527802, 13.89961937509977652, 114.3739096053143669 ) ) ;
#99068=CARTESIAN_POINT ( 'NONE',  ( -4.483927247898782831, 16.52544592524335698, 112.7094237280190328 ) ) ;
#99069=CARTESIAN_POINT ( 'NONE',  ( 21.55341960407619695, -5.719274019375665929, 41.04275706135236135 ) ) ;
#99071=CARTESIAN_POINT ( 'NONE',  ( -0.05219959533934338120, 16.53943276465976808, 57.50109039468568994 ) ) ;
#99072=CARTESIAN_POINT ( 'NONE',  ( 14.29746914071049879, -8.314922557960816363, 33.33224293864769550 ) ) ;
#99073=CARTESIAN_POINT ( 'NONE',  ( -5.153800228976328057, -19.02544592524343514, 42.29057627198101699 ) ) ;
#99074=CARTESIAN_POINT ( 'NONE',  ( -16.52544592524335698, -4.483927247898792601, 108.9594237280190185 ) ) ;
#99075=CARTESIAN_POINT ( 'NONE',  ( 16.55341960407618274, -4.379528057220086978, 21.04275706135234714 ) ) ;
#99076=CARTESIAN_POINT ( 'NONE',  ( 13.97604488694527802, 13.89961937509977652, 54.37390960531435979 ) ) ;
#99077=CARTESIAN_POINT ( 'NONE',  ( 12.06949235617757843, -12.14591786802309237, 103.1239096053143811 ) ) ;
#99078=CARTESIAN_POINT ( 'NONE',  ( 5.823673210054444382, -21.52544592524334988, 20.20942372801900788 ) ) ;
#99079=CARTESIAN_POINT ( 'NONE',  ( 5.049401038298161559, -19.05341960407611168, 47.70724293864770260 ) ) ;
#99081=CARTESIAN_POINT ( 'NONE',  ( -19.05341960407611168, -5.049401038298163336, 26.45724293864769550 ) ) ;
#99082=CARTESIAN_POINT ( 'NONE',  ( -15.80617190586745835, -15.72974639402198527, 26.87390960531435979 ) ) ;
#99084=CARTESIAN_POINT ( 'NONE',  ( 13.97604488694527802, 13.89961937509977652, 94.37390960531436690 ) ) ;
#99085=CARTESIAN_POINT ( 'NONE',  ( 21.55341960407619695, -5.719274019375665929, 46.04275706135234714 ) ) ;
#99086=CARTESIAN_POINT ( 'NONE',  ( 8.224510206698953496, -14.34966873604960469, 97.91557627198103830 ) ) ;
#99087=CARTESIAN_POINT ( 'NONE',  ( 0.05219959533909260263, 19.03943276465977164, 114.9989096053143669 ) ) ;
#99089=CARTESIAN_POINT ( 'NONE',  ( -16.52544592524335698, -4.483927247898792601, 58.95942372801902565 ) ) ;
#99090=CARTESIAN_POINT ( 'NONE',  ( -21.53943276465977519, -0.05219959533937600094, 88.75109039468567573 ) ) ;
#99091=CARTESIAN_POINT ( 'NONE',  ( -4.379528057220086978, -16.55341960407618274, 54.79275706135235424 ) ) ;
#99092=CARTESIAN_POINT ( 'NONE',  ( 5.153800228976335163, 19.02544592524342804, 99.79057627198102409 ) ) ;
#99093=CARTESIAN_POINT ( 'NONE',  ( 12.14591786802327356, -12.06949235617739191, 45.62609039468567573 ) ) ;
#99094=CARTESIAN_POINT ( 'NONE',  ( -16.46253265017146816, -9.564922557961047289, 109.1677570613523471 ) ) ;
#99095=CARTESIAN_POINT ( 'NONE',  ( 16.53943276465976808, 0.05219959533934440121, 81.25109039468568994 ) ) ;
#99096=CARTESIAN_POINT ( 'NONE',  ( 5.153800228976615827, -19.02544592524334988, 95.20942372801897591 ) ) ;
#99097=CARTESIAN_POINT ( 'NONE',  ( -9.474510206698964154, 16.51473224551069663, 70.41557627198102409 ) ) ;
#99098=CARTESIAN_POINT ( 'NONE',  ( 5.719274019375991003, -21.55341960407610458, 102.7072429386476955 ) ) ;
#99099=CARTESIAN_POINT ( 'NONE',  ( 8.224510206698953496, -14.34966873604960469, 87.91557627198103830 ) ) ;
#99100=CARTESIAN_POINT ( 'NONE',  ( 16.51473224551083163, -9.474510206698727899, 110.8344237280190043 ) ) ;
#99101=CARTESIAN_POINT ( 'NONE',  ( 12.06949235617739724, 12.14591786802326823, 76.87609039468567573 ) ) ;
#99103=CARTESIAN_POINT ( 'NONE',  ( 9.564922557961047289, -16.46253265017146816, 70.41775706135233293 ) ) ;
#99104=CARTESIAN_POINT ( 'NONE',  ( 8.224510206698953496, -14.34966873604960469, 37.91557627198102409 ) ) ;
#99105=CARTESIAN_POINT ( 'NONE',  ( 0.05219959533910956823, 16.53943276465976808, 94.99890960531436690 ) ) ;
#99106=CARTESIAN_POINT ( 'NONE',  ( 19.02544592524334988, 5.153800228976608722, 36.45942372801900433 ) ) ;
#99108=CARTESIAN_POINT ( 'NONE',  ( 10.81492255796106328, -18.62759615963255655, 25.41775706135235779 ) ) ;
#99109=CARTESIAN_POINT ( 'NONE',  ( 9.474510206698729675, 16.51473224551082808, 97.08442372801900433 ) ) ;
#99111=CARTESIAN_POINT ( 'NONE',  ( -9.564922557960796823, -16.46253265017161027, 97.08224293864769550 ) ) ;
#99112=CARTESIAN_POINT ( 'NONE',  ( 10.81492255796106328, -18.62759615963255655, 100.4177570613523471 ) ) ;
#99113=CARTESIAN_POINT ( 'NONE',  ( 5.049401038298161559, -19.05341960407611168, 72.70724293864768129 ) ) ;
#99114=CARTESIAN_POINT ( 'NONE',  ( -10.81492255796078084, -18.62759615963271287, 37.08224293864768129 ) ) ;
#99115=CARTESIAN_POINT ( 'NONE',  ( -8.224510206698948167, 14.34966873604960824, 100.4155762719810241 ) ) ;
#99116=CARTESIAN_POINT ( 'NONE',  ( -0.05219959533909027116, -19.03943276465977164, 52.49890960531436690 ) ) ;
#99117=CARTESIAN_POINT ( 'NONE',  ( -4.379528057220328563, 16.55341960407611168, 105.2072429386477097 ) ) ;
#99119=CARTESIAN_POINT ( 'NONE',  ( 10.72451020669871369, 18.67979575497193778, 22.08442372801901143 ) ) ;
#99120=CARTESIAN_POINT ( 'NONE',  ( -5.719274019375665041, -21.55341960407619695, 59.79275706135234714 ) ) ;
#99121=CARTESIAN_POINT ( 'NONE',  ( -5.049401038298153566, 19.05341960407611168, 40.20724293864768839 ) ) ;
#99123=CARTESIAN_POINT ( 'NONE',  ( -16.55341960407617563, 4.379528057220093196, 73.54275706135234714 ) ) ;
#99124=CARTESIAN_POINT ( 'NONE',  ( 21.52544592524334988, 5.823673210054432836, 21.45942372801901499 ) ) ;
#99126=CARTESIAN_POINT ( 'NONE',  ( -15.72974639402197994, 15.80617190586746368, 115.6239096053143669 ) ) ;
#99127=CARTESIAN_POINT ( 'NONE',  ( 9.564922557961047289, -16.46253265017146816, 55.41775706135234003 ) ) ;
#99128=CARTESIAN_POINT ( 'NONE',  ( 5.049401038298161559, -19.05341960407611168, 67.70724293864769550 ) ) ;
#99129=CARTESIAN_POINT ( 'NONE',  ( -19.02544592524334988, -5.153800228976617603, 33.95942372801897591 ) ) ;
#99130=CARTESIAN_POINT ( 'NONE',  ( 21.52544592524334988, 5.823673210054432836, 66.45942372801903275 ) ) ;
#99131=CARTESIAN_POINT ( 'NONE',  ( 15.72974639402199770, -15.80617190586745480, 73.12390960531436690 ) ) ;
#99132=CARTESIAN_POINT ( 'NONE',  ( 12.06949235617757843, -12.14591786802309237, 53.12390960531436690 ) ) ;
#99133=CARTESIAN_POINT ( 'NONE',  ( 15.80617190586769283, -15.72974639402175789, 85.62609039468568994 ) ) ;
#99134=CARTESIAN_POINT ( 'NONE',  ( 9.564922557961047289, -16.46253265017146816, 25.41775706135234003 ) ) ;
#99135=CARTESIAN_POINT ( 'NONE',  ( -16.53943276465976808, 0.05219959533911058130, 66.24890960531436690 ) ) ;
#99136=CARTESIAN_POINT ( 'NONE',  ( 13.89961937509977652, -13.97604488694527269, 23.12390960531436335 ) ) ;
#99137=CARTESIAN_POINT ( 'NONE',  ( 13.89961937509957401, 13.97604488694547697, 51.87609039468566863 ) ) ;
#99138=CARTESIAN_POINT ( 'NONE',  ( -4.379528057220086978, -16.55341960407618274, 109.7927570613523613 ) ) ;
#99140=CARTESIAN_POINT ( 'NONE',  ( 15.80617190586769283, -15.72974639402175789, 75.62609039468567573 ) ) ;
#99141=CARTESIAN_POINT ( 'NONE',  ( 19.03943276465977164, 0.05219959533936151252, 51.25109039468567573 ) ) ;
#99142=CARTESIAN_POINT ( 'NONE',  ( -18.62759615963270932, 10.81492255796079327, 55.83224293864770260 ) ) ;
#99143=CARTESIAN_POINT ( 'NONE',  ( 15.72974639402176855, 15.80617190586768217, 41.87609039468568284 ) ) ;
#99144=CARTESIAN_POINT ( 'NONE',  ( -10.72451020669898014, 18.67979575497178502, 95.41557627198102409 ) ) ;
#99145=CARTESIAN_POINT ( 'NONE',  ( 5.153800228976615827, -19.02544592524334988, 100.2094237280190043 ) ) ;
#99146=CARTESIAN_POINT ( 'NONE',  ( -8.314922557961024197, 14.29746914071037800, 72.91775706135234714 ) ) ;
#99148=CARTESIAN_POINT ( 'NONE',  ( -18.67979575497178146, -10.72451020669898902, 106.6655762719810383 ) ) ;
#99149=CARTESIAN_POINT ( 'NONE',  ( 12.06949235617757843, -12.14591786802309237, 88.12390960531436690 ) ) ;
#99150=CARTESIAN_POINT ( 'NONE',  ( -17.13100169013299734, -6.664070546373157100, 99.23210164300155611 ) ) ;
#99151=CARTESIAN_POINT ( 'NONE',  ( -16.52544592524335698, -4.483927247898792601, 23.95942372801901143 ) ) ;
#99152=CARTESIAN_POINT ( 'NONE',  ( 0.05219959533907565091, 21.53943276465977519, 54.99890960531435269 ) ) ;
#99153=CARTESIAN_POINT ( 'NONE',  ( 16.53943276465976808, 0.05219959533934440121, 86.25109039468568994 ) ) ;
#99155=CARTESIAN_POINT ( 'NONE',  ( 16.52544592524335698, 4.483927247898782831, 66.45942372801903275 ) ) ;
#99156=CARTESIAN_POINT ( 'NONE',  ( -15.72974639402176322, -15.80617190586768395, 44.37609039468567573 ) ) ;
#99157=CARTESIAN_POINT ( 'NONE',  ( 21.55341960407610458, 5.719274019375980345, 63.95724293864770260 ) ) ;
#99158=CARTESIAN_POINT ( 'NONE',  ( 0.05219959533934541429, -16.53943276465976808, 85.00109039468568994 ) ) ;
#99159=CARTESIAN_POINT ( 'NONE',  ( 5.823673210054444382, -21.52544592524334988, 65.20942372801901854 ) ) ;
#99160=CARTESIAN_POINT ( 'NONE',  ( 10.72451020669898902, -18.67979575497178502, 47.91557627198102409 ) ) ;
#99161=CARTESIAN_POINT ( 'NONE',  ( -10.72451020669898014, 18.67979575497178502, 40.41557627198103120 ) ) ;
#99163=CARTESIAN_POINT ( 'NONE',  ( 8.224510206698742110, 14.34966873604972548, 67.08442372801901854 ) ) ;
#99164=CARTESIAN_POINT ( 'NONE',  ( -5.823673210054116645, -21.52544592524344225, 37.29057627198102409 ) ) ;
#99166=CARTESIAN_POINT ( 'NONE',  ( 5.049401038298161559, -19.05341960407611168, 97.70724293864766707 ) ) ;
#99167=CARTESIAN_POINT ( 'NONE',  ( 16.55341960407618274, -4.379528057220086978, 111.0427570613523613 ) ) ;
#99168=CARTESIAN_POINT ( 'NONE',  ( 18.22780087662121673, 5.500000000000056843, 73.98459894673894155 ) ) ;
#99169=CARTESIAN_POINT ( 'NONE',  ( 8.314922557960818139, 14.29746914071049879, 109.5822429386476955 ) ) ;
#99170=CARTESIAN_POINT ( 'NONE',  ( 10.72451020669898902, -18.67979575497178502, 42.91557627198103120 ) ) ;
#99171=CARTESIAN_POINT ( 'NONE',  ( -19.05341960407611168, -5.049401038298163336, 46.45724293864768129 ) ) ;
#99172=CARTESIAN_POINT ( 'NONE',  ( 8.314922557961029526, -14.29746914071037800, 90.41775706135236135 ) ) ;
#99173=CARTESIAN_POINT ( 'NONE',  ( -15.80617190586768217, 15.72974639402176855, 28.12609039468568284 ) ) ;
#99174=CARTESIAN_POINT ( 'NONE',  ( 5.153800228976615827, -19.02544592524334988, 90.20942372801900433 ) ) ;
#99175=CARTESIAN_POINT ( 'NONE',  ( 4.483927247898545687, 16.52544592524342804, 109.7905762719810383 ) ) ;
#99176=CARTESIAN_POINT ( 'NONE',  ( 19.02544592524343514, -5.153800228976328945, 53.54057627198102409 ) ) ;
#99177=AXIS2_PLACEMENT_3D ( 'NONE', #90965, #190949, #36254 ) ;
#99178=CARTESIAN_POINT ( 'NONE',  ( 19.02544592524343514, -5.153800228976328945, 33.54057627198102409 ) ) ;
#99180=CARTESIAN_POINT ( 'NONE',  ( 5.153800228976335163, 19.02544592524342804, 74.79057627198103830 ) ) ;
#99181=CARTESIAN_POINT ( 'NONE',  ( 4.483927247898790824, -16.52544592524335698, 60.20942372801902565 ) ) ;
#99182=CARTESIAN_POINT ( 'NONE',  ( 5.719274019375673035, 21.55341960407619339, 102.2927570613523613 ) ) ;
#99183=CARTESIAN_POINT ( 'NONE',  ( 21.55341960407610458, 5.719274019375980345, 48.95724293864770971 ) ) ;
#99184=CARTESIAN_POINT ( 'NONE',  ( 14.29746914071037800, 8.314922557961029526, 76.66775706135234714 ) ) ;
#99185=CARTESIAN_POINT ( 'NONE',  ( -9.564922557961040184, 16.46253265017147172, 52.91775706135233293 ) ) ;
#99186=CARTESIAN_POINT ( 'NONE',  ( -0.05219959533936034679, 19.03943276465977164, 62.50109039468566863 ) ) ;
#99188=CARTESIAN_POINT ( 'NONE',  ( -21.53943276465977519, -0.05219959533937600094, 58.75109039468568994 ) ) ;
#99189=CARTESIAN_POINT ( 'NONE',  ( -19.05341960407611168, -5.049401038298163336, 61.45724293864769550 ) ) ;
#99190=CARTESIAN_POINT ( 'NONE',  ( -5.049401038298153566, 19.05341960407611168, 40.20724293864768839 ) ) ;
#99191=CARTESIAN_POINT ( 'NONE',  ( 13.97604488694548053, -13.89961937509957401, 65.62609039468567573 ) ) ;
#99192=CARTESIAN_POINT ( 'NONE',  ( 16.46253265017160672, -9.564922557960803928, 108.3322429386476955 ) ) ;
#99193=CARTESIAN_POINT ( 'NONE',  ( 19.03943276465977164, -0.05219959533909143690, 98.74890960531436690 ) ) ;
#99194=CARTESIAN_POINT ( 'NONE',  ( -14.34966873604960291, -8.224510206698953496, 56.66557627198103830 ) ) ;
#99195=CARTESIAN_POINT ( 'NONE',  ( -0.05219959533907301413, -21.53943276465977519, 42.49890960531435979 ) ) ;
#99197=CARTESIAN_POINT ( 'NONE',  ( -9.474510206698720793, -16.51473224551083518, 34.58442372801899722 ) ) ;
#99199=CARTESIAN_POINT ( 'NONE',  ( 16.51473224551069308, 9.474510206698969483, 44.16557627198103120 ) ) ;
#99202=CARTESIAN_POINT ( 'NONE',  ( 8.314922557961029526, -14.29746914071037800, 75.41775706135233293 ) ) ;
#99203=CARTESIAN_POINT ( 'NONE',  ( 21.52544592524344225, -5.823673210054117533, 98.54057627198105251 ) ) ;
#99204=CARTESIAN_POINT ( 'NONE',  ( -16.55341960407611168, -4.379528057220339221, 56.45724293864768839 ) ) ;
#99205=CARTESIAN_POINT ( 'NONE',  ( 19.03943276465977164, -0.05219959533909143690, 43.74890960531435979 ) ) ;
#99207=CARTESIAN_POINT ( 'NONE',  ( 5.823673210054444382, -21.52544592524334988, 45.20942372801901854 ) ) ;
#99208=CARTESIAN_POINT ( 'NONE',  ( 13.97604488694548053, -13.89961937509957401, 50.62609039468566152 ) ) ;
#99209=CARTESIAN_POINT ( 'NONE',  ( -5.049401038298153566, 19.05341960407611168, 45.20724293864769550 ) ) ;
#99210=CARTESIAN_POINT ( 'NONE',  ( -21.53943276465977519, -0.05219959533937600094, 93.75109039468567573 ) ) ;
#99211=CARTESIAN_POINT ( 'NONE',  ( 17.12812012977027365, 6.668231424565989940, 98.85948759323144941 ) ) ;
#99212=CARTESIAN_POINT ( 'NONE',  ( -0.05219959533910754901, -16.53943276465976808, 42.49890960531435979 ) ) ;
#99214=CARTESIAN_POINT ( 'NONE',  ( 5.823673210054125526, 21.52544592524343514, 44.79057627198103120 ) ) ;
#99216=CARTESIAN_POINT ( 'NONE',  ( -0.05219959533909027116, -19.03943276465977164, 102.4989096053143669 ) ) ;
#99217=CARTESIAN_POINT ( 'NONE',  ( -4.483927247898539470, -16.52544592524342804, 87.29057627198103830 ) ) ;
#99218=CARTESIAN_POINT ( 'NONE',  ( 0.05219959533934541429, -16.53943276465976808, 25.00109039468567218 ) ) ;
#99219=CARTESIAN_POINT ( 'NONE',  ( -8.314922557961024197, 14.29746914071037800, 102.9177570613523756 ) ) ;
#99222=CARTESIAN_POINT ( 'NONE',  ( -5.049401038298153566, 19.05341960407611168, 95.20724293864770971 ) ) ;
#99223=CARTESIAN_POINT ( 'NONE',  ( 21.52544592524344225, -5.823673210054117533, 98.54057627198105251 ) ) ;
#99224=CARTESIAN_POINT ( 'NONE',  ( 16.55341960407611168, 4.379528057220329451, 23.95724293864769550 ) ) ;
#99225=CARTESIAN_POINT ( 'NONE',  ( 9.564922557960805705, 16.46253265017160317, 94.58224293864769550 ) ) ;
#99226=CARTESIAN_POINT ( 'NONE',  ( 19.02544592524334988, 5.153800228976608722, 91.45942372801900433 ) ) ;
#99227=CARTESIAN_POINT ( 'NONE',  ( 10.72451020669871369, 18.67979575497193778, 107.0844237280190043 ) ) ;
#99228=CARTESIAN_POINT ( 'NONE',  ( 21.52544592524344225, -5.823673210054117533, 83.54057627198102409 ) ) ;
#99229=CARTESIAN_POINT ( 'NONE',  ( -10.72451020669898014, 18.67979575497178502, 50.41557627198103120 ) ) ;
#99230=CARTESIAN_POINT ( 'NONE',  ( -13.89961937509977652, 13.97604488694528158, 60.62390960531436690 ) ) ;
#99231=CARTESIAN_POINT ( 'NONE',  ( 16.52544592524342804, -4.483927247898539470, 38.54057627198103120 ) ) ;
#99232=CARTESIAN_POINT ( 'NONE',  ( 13.97604488694527802, 13.89961937509977652, 79.37390960531435269 ) ) ;
#99234=CARTESIAN_POINT ( 'NONE',  ( 18.87075004821569379, -5.500000000000108358, 61.17408112101048090 ) ) ;
#99235=CARTESIAN_POINT ( 'NONE',  ( 13.97604488694548053, -13.89961937509957401, 40.62609039468564731 ) ) ;
#99236=CARTESIAN_POINT ( 'NONE',  ( -16.53943276465976808, 0.05219959533911058130, 86.24890960531436690 ) ) ;
#99237=CARTESIAN_POINT ( 'NONE',  ( -0.05219959533937732626, 21.53943276465977519, 22.50109039468567573 ) ) ;
#99239=CARTESIAN_POINT ( 'NONE',  ( -12.14591786802326823, 12.06949235617739902, 103.1260903946856757 ) ) ;
#99240=CARTESIAN_POINT ( 'NONE',  ( 8.224510206698953496, -14.34966873604960469, 112.9155762719810383 ) ) ;
#99241=CARTESIAN_POINT ( 'NONE',  ( -9.474510206698964154, 16.51473224551069663, 75.41557627198103830 ) ) ;
#99242=DIRECTION ( 'NONE',  ( 0.000000000000000000, 0.000000000000000000, 1.000000000000000000 ) ) ;
#99243=CARTESIAN_POINT ( 'NONE',  ( 5.049401038298161559, -19.05341960407611168, 22.70724293864769194 ) ) ;
#99244=CARTESIAN_POINT ( 'NONE',  ( 14.34966873604960469, 8.224510206698951720, 44.16557627198103120 ) ) ;
#99245=CARTESIAN_POINT ( 'NONE',  ( -10.72451020669870658, -18.67979575497194134, 54.58442372801901143 ) ) ;
#99247=CARTESIAN_POINT ( 'NONE',  ( 5.719274019375673035, 21.55341960407619339, 92.29275706135236135 ) ) ;
#99248=CARTESIAN_POINT ( 'NONE',  ( 16.51473224551069308, 9.474510206698969483, 44.16557627198103120 ) ) ;
#99249=CARTESIAN_POINT ( 'NONE',  ( -9.474510206698964154, 16.51473224551069663, 55.41557627198103120 ) ) ;
#99251=CARTESIAN_POINT ( 'NONE',  ( -10.81492255796105439, 18.62759615963255655, 97.91775706135236135 ) ) ;
#99252=CARTESIAN_POINT ( 'NONE',  ( 14.29746914071037800, 8.314922557961029526, 56.66775706135235424 ) ) ;
#99253=CARTESIAN_POINT ( 'NONE',  ( 10.72451020669871369, 18.67979575497193778, 82.08442372801901854 ) ) ;
#99254=CARTESIAN_POINT ( 'NONE',  ( 18.62759615963271287, -10.81492255796078972, 23.33224293864769194 ) ) ;
#99255=CARTESIAN_POINT ( 'NONE',  ( -19.02544592524334988, -5.153800228976617603, 88.95942372801897591 ) ) ;
#99256=CARTESIAN_POINT ( 'NONE',  ( 10.72451020669871369, 18.67979575497193778, 72.08442372801899012 ) ) ;
#99257=CARTESIAN_POINT ( 'NONE',  ( -12.14591786802326823, 12.06949235617739902, 38.12609039468567573 ) ) ;
#99258=CARTESIAN_POINT ( 'NONE',  ( -21.52544592524343514, 5.823673210054127303, 91.04057627198103830 ) ) ;
#99259=CARTESIAN_POINT ( 'NONE',  ( -9.474510206698720793, -16.51473224551083518, 84.58442372801900433 ) ) ;
#99260=CARTESIAN_POINT ( 'NONE',  ( 19.05341960407611168, 5.049401038298154454, 58.95724293864768129 ) ) ;
#99261=CARTESIAN_POINT ( 'NONE',  ( 0.05219959533936267826, -19.03943276465977164, 100.0010903946856757 ) ) ;
#99263=CARTESIAN_POINT ( 'NONE',  ( 9.474510206698729675, 16.51473224551082808, 97.08442372801900433 ) ) ;
#99264=CARTESIAN_POINT ( 'NONE',  ( -16.55341960407611168, -4.379528057220339221, 51.45724293864770260 ) ) ;
#99265=CARTESIAN_POINT ( 'NONE',  ( 16.46253265017146816, 9.564922557961045513, 71.66775706135233293 ) ) ;
#99266=CARTESIAN_POINT ( 'NONE',  ( 12.14591786802327356, -12.06949235617739191, 60.62609039468567573 ) ) ;
#99267=CARTESIAN_POINT ( 'NONE',  ( 19.02544592524343514, -5.153800228976328945, 43.54057627198103120 ) ) ;
#99268=CARTESIAN_POINT ( 'NONE',  ( -19.02544592524342804, 5.153800228976336051, 51.04057627198103120 ) ) ;
#99269=CARTESIAN_POINT ( 'NONE',  ( -4.483927247898782831, 16.52544592524335698, 62.70942372801902565 ) ) ;
#99272=CARTESIAN_POINT ( 'NONE',  ( -13.89961937509977652, 13.97604488694528158, 110.6239096053143243 ) ) ;
#99273=CARTESIAN_POINT ( 'NONE',  ( -13.97604488694527625, -13.89961937509977652, 26.87390960531434558 ) ) ;
#99274=VERTEX_POINT ( 'NONE', #124456 ) ;
#99275=CARTESIAN_POINT ( 'NONE',  ( 9.564922557961047289, -16.46253265017146816, 110.4177570613523471 ) ) ;
#99276=CARTESIAN_POINT ( 'NONE',  ( 10.72451020669898902, -18.67979575497178502, 37.91557627198102409 ) ) ;
#99277=CARTESIAN_POINT ( 'NONE',  ( -13.97604488694547697, 13.89961937509957934, 33.12609039468566863 ) ) ;
#99278=CARTESIAN_POINT ( 'NONE',  ( 14.29746914071037800, 8.314922557961029526, 26.66775706135235424 ) ) ;
#99279=CARTESIAN_POINT ( 'NONE',  ( 19.02544592524343514, -5.153800228976328945, 28.54057627198102409 ) ) ;
#99280=CARTESIAN_POINT ( 'NONE',  ( -5.153800228976328057, -19.02544592524343514, 57.29057627198103120 ) ) ;
#99281=CARTESIAN_POINT ( 'NONE',  ( 0.05219959533907565091, 21.53943276465977519, 84.99890960531436690 ) ) ;
#99282=CARTESIAN_POINT ( 'NONE',  ( 0.05219959533909260263, 19.03943276465977164, 104.9989096053143669 ) ) ;
#99283=CARTESIAN_POINT ( 'NONE',  ( -16.46253265017160317, 9.564922557960807481, 55.83224293864769550 ) ) ;
#99285=CARTESIAN_POINT ( 'NONE',  ( 5.153800228976615827, -19.02544592524334988, 90.20942372801900433 ) ) ;
#99286=CARTESIAN_POINT ( 'NONE',  ( -8.224510206698948167, 14.34966873604960824, 70.41557627198102409 ) ) ;
#99288=CARTESIAN_POINT ( 'NONE',  ( 21.53943276465977519, -0.05219959533907433946, 43.74890960531435979 ) ) ;
#99289=CARTESIAN_POINT ( 'NONE',  ( 21.55341960407619695, -5.719274019375665929, 101.0427570613523756 ) ) ;
#99290=CARTESIAN_POINT ( 'NONE',  ( -21.53943276465977519, 0.05219959533907696930, 96.24890960531435269 ) ) ;
#99291=CARTESIAN_POINT ( 'NONE',  ( -18.67979575497193778, 10.72451020669871902, 78.33442372801901854 ) ) ;
#99292=CARTESIAN_POINT ( 'NONE',  ( 21.52544592524334988, 5.823673210054432836, 71.45942372801901854 ) ) ;
#99293=CARTESIAN_POINT ( 'NONE',  ( 19.05341960407611168, 5.049401038298154454, 108.9572429386477097 ) ) ;
#99294=CARTESIAN_POINT ( 'NONE',  ( -4.483927247898782831, 16.52544592524335698, 107.7094237280190328 ) ) ;
#99295=CARTESIAN_POINT ( 'NONE',  ( -15.80617190586768217, 15.72974639402176855, 73.12609039468567573 ) ) ;
#99296=CARTESIAN_POINT ( 'NONE',  ( 13.89961937509977652, -13.97604488694527269, 68.12390960531436690 ) ) ;
#99298=CARTESIAN_POINT ( 'NONE',  ( 21.55341960407619695, -5.719274019375665929, 31.04275706135234714 ) ) ;
#99299=CARTESIAN_POINT ( 'NONE',  ( 0.05219959533909260263, 19.03943276465977164, 69.99890960531435269 ) ) ;
#99300=CARTESIAN_POINT ( 'NONE',  ( -16.55341960407611168, -4.379528057220339221, 86.45724293864770971 ) ) ;
#99301=CARTESIAN_POINT ( 'NONE',  ( -16.55341960407611168, -4.379528057220339221, 51.45724293864770260 ) ) ;
#99302=CARTESIAN_POINT ( 'NONE',  ( 18.62759615963271287, -10.81492255796078972, 58.33224293864768839 ) ) ;
#99303=CARTESIAN_POINT ( 'NONE',  ( -5.049401038298153566, 19.05341960407611168, 60.20724293864768129 ) ) ;
#99304=CARTESIAN_POINT ( 'NONE',  ( -21.52544592524343514, 5.823673210054127303, 76.04057627198102409 ) ) ;
#99305=CARTESIAN_POINT ( 'NONE',  ( 13.97604488694548053, -13.89961937509957401, 70.62609039468567573 ) ) ;
#99306=CARTESIAN_POINT ( 'NONE',  ( 5.049401038297881783, 19.05341960407617918, 22.29275706135233648 ) ) ;
#99307=CARTESIAN_POINT ( 'NONE',  ( -12.06949235617756955, 12.14591786802309770, 75.62390960531439532 ) ) ;
#99309=CARTESIAN_POINT ( 'NONE',  ( -10.81492255796078084, -18.62759615963271287, 57.08224293864769550 ) ) ;
#99312=CARTESIAN_POINT ( 'NONE',  ( -16.55341960407617563, 4.379528057220093196, 93.54275706135234714 ) ) ;
#99314=CARTESIAN_POINT ( 'NONE',  ( 19.02544592524334988, 5.153800228976608722, 86.45942372801900433 ) ) ;
#99315=ADVANCED_FACE ( 'NONE', ( #139613 ), #197349, .F. ) ;
#99316=CARTESIAN_POINT ( 'NONE',  ( 4.379528057220339221, -16.55341960407611168, 62.70724293864769550 ) ) ;
#99317=CARTESIAN_POINT ( 'NONE',  ( -17.50000000000000000, 5.499999999999992895, 33.71769037696435589 ) ) ;
#99318=CARTESIAN_POINT ( 'NONE',  ( 16.51473224551069308, 9.474510206698969483, 64.16557627198102409 ) ) ;
#99319=CARTESIAN_POINT ( 'NONE',  ( -8.314922557960811034, -14.29746914071050412, 57.08224293864769550 ) ) ;
#99320=CARTESIAN_POINT ( 'NONE',  ( -9.474510206698964154, 16.51473224551069663, 85.41557627198102409 ) ) ;
#99321=CARTESIAN_POINT ( 'NONE',  ( 9.474510206698729675, 16.51473224551082808, 77.08442372801900433 ) ) ;
#99322=CARTESIAN_POINT ( 'NONE',  ( -5.049401038298153566, 19.05341960407611168, 55.20724293864769550 ) ) ;
#99323=CARTESIAN_POINT ( 'NONE',  ( 16.46253265017160672, -9.564922557960803928, 83.33224293864768129 ) ) ;
#99324=CARTESIAN_POINT ( 'NONE',  ( -5.153800228976328057, -19.02544592524343514, 72.29057627198102409 ) ) ;
#99325=CARTESIAN_POINT ( 'NONE',  ( -5.719274019375978568, 21.55341960407610458, 60.20724293864768839 ) ) ;
#99326=CARTESIAN_POINT ( 'NONE',  ( -8.314922557961024197, 14.29746914071037800, 62.91775706135236135 ) ) ;
#99327=CARTESIAN_POINT ( 'NONE',  ( 17.58332526062525147, 7.635886036038630920, 101.5766504044153322 ) ) ;
#99328=CARTESIAN_POINT ( 'NONE',  ( -19.05341960407611168, -5.049401038298163336, 51.45724293864770260 ) ) ;
#99329=CARTESIAN_POINT ( 'NONE',  ( 18.62759615963271287, -10.81492255796078972, 53.33224293864769550 ) ) ;
#99330=CARTESIAN_POINT ( 'NONE',  ( -19.02544592524334988, -5.153800228976617603, 78.95942372801900433 ) ) ;
#99331=CARTESIAN_POINT ( 'NONE',  ( -14.34966873604960291, -8.224510206698953496, 21.66557627198102409 ) ) ;
#99332=CARTESIAN_POINT ( 'NONE',  ( -13.89961937509957401, -13.97604488694547875, 34.37609039468566863 ) ) ;
#99333=CARTESIAN_POINT ( 'NONE',  ( -12.14591786802326823, 12.06949235617739902, 58.12609039468568994 ) ) ;
#99334=CARTESIAN_POINT ( 'NONE',  ( 4.483927247898790824, -16.52544592524335698, 90.20942372801903275 ) ) ;
#99336=CARTESIAN_POINT ( 'NONE',  ( 8.224510206698742110, 14.34966873604972548, 82.08442372801901854 ) ) ;
#99337=CARTESIAN_POINT ( 'NONE',  ( -21.53943276465977519, 0.05219959533907696930, 31.24890960531435979 ) ) ;
#99338=CARTESIAN_POINT ( 'NONE',  ( 9.564922557960805705, 16.46253265017160317, 39.58224293864768839 ) ) ;
#99339=CARTESIAN_POINT ( 'NONE',  ( -19.05341960407611168, -5.049401038298163336, 51.45724293864770260 ) ) ;
#99340=CARTESIAN_POINT ( 'NONE',  ( -16.46253265017160317, 9.564922557960807481, 40.83224293864769550 ) ) ;
#99341=CARTESIAN_POINT ( 'NONE',  ( -21.55341960407619339, 5.719274019375674811, 33.54275706135234714 ) ) ;
#99342=CARTESIAN_POINT ( 'NONE',  ( 14.29746914071037800, 8.314922557961029526, 46.66775706135234714 ) ) ;
#99343=CARTESIAN_POINT ( 'NONE',  ( -14.34966873604960291, -8.224510206698953496, 26.66557627198103475 ) ) ;
#99344=CARTESIAN_POINT ( 'NONE',  ( 19.03943276465977164, -0.05219959533909143690, 23.74890960531435269 ) ) ;
#99345=CARTESIAN_POINT ( 'NONE',  ( -16.51473224551082808, 9.474510206698731452, 23.33442372801900078 ) ) ;
#99346=CARTESIAN_POINT ( 'NONE',  ( 0.05219959533934541429, -16.53943276465976808, 20.00109039468568639 ) ) ;
#99347=CARTESIAN_POINT ( 'NONE',  ( 13.89961937509957401, 13.97604488694547697, 66.87609039468567573 ) ) ;
#99348=CARTESIAN_POINT ( 'NONE',  ( 16.52544592524342804, -4.483927247898539470, 73.54057627198102409 ) ) ;
#99349=CARTESIAN_POINT ( 'NONE',  ( 19.05341960407611168, 5.049401038298154454, 43.95724293864769550 ) ) ;
#99350=CARTESIAN_POINT ( 'NONE',  ( -5.049401038297874678, -19.05341960407617918, 69.79275706135233293 ) ) ;
#99352=CARTESIAN_POINT ( 'NONE',  ( 15.72974639402176855, 15.80617190586768217, 71.87609039468568994 ) ) ;
#99353=CARTESIAN_POINT ( 'NONE',  ( 12.06949235617739724, 12.14591786802326823, 46.87609039468568994 ) ) ;
#99355=CARTESIAN_POINT ( 'NONE',  ( -21.52544592524343514, 5.823673210054127303, 36.04057627198102409 ) ) ;
#99356=CARTESIAN_POINT ( 'NONE',  ( -14.29746914071037622, -8.314922557961029526, 24.16775706135235424 ) ) ;
#99357=CARTESIAN_POINT ( 'NONE',  ( 18.09805431107249518, -5.499999999999974243, 98.51606229291887473 ) ) ;
#99359=CARTESIAN_POINT ( 'NONE',  ( 19.05341960407611168, 5.049401038298154454, 38.95724293864767418 ) ) ;
#99360=CARTESIAN_POINT ( 'NONE',  ( -9.564922557961040184, 16.46253265017147172, 57.91775706135233293 ) ) ;
#99361=CARTESIAN_POINT ( 'NONE',  ( -19.02544592524342804, 5.153800228976336051, 51.04057627198103120 ) ) ;
#99362=CARTESIAN_POINT ( 'NONE',  ( 5.823673210054444382, -21.52544592524334988, 65.20942372801901854 ) ) ;
#99363=CARTESIAN_POINT ( 'NONE',  ( -18.67979575497193778, 10.72451020669871902, 113.3344237280190328 ) ) ;
#99364=CARTESIAN_POINT ( 'NONE',  ( -16.55341960407611168, -4.379528057220339221, 26.45724293864768839 ) ) ;
#99365=CARTESIAN_POINT ( 'NONE',  ( -5.153800228976328057, -19.02544592524343514, 32.29057627198102409 ) ) ;
#99366=CARTESIAN_POINT ( 'NONE',  ( -5.153800228976328057, -19.02544592524343514, 87.29057627198103830 ) ) ;
#99367=CARTESIAN_POINT ( 'NONE',  ( -21.53943276465977519, -0.05219959533937600094, 53.75109039468568994 ) ) ;
#99368=CARTESIAN_POINT ( 'NONE',  ( -19.02544592524342804, 5.153800228976336051, 41.04057627198103120 ) ) ;
#99369=CARTESIAN_POINT ( 'NONE',  ( 21.55341960407619695, -5.719274019375665929, 71.04275706135234714 ) ) ;
#99370=CARTESIAN_POINT ( 'NONE',  ( -19.03943276465977164, -0.05219959533935918106, 98.75109039468567573 ) ) ;
#99371=CARTESIAN_POINT ( 'NONE',  ( 16.51473224551069308, 9.474510206698969483, 104.1655762719810241 ) ) ;
#99372=CARTESIAN_POINT ( 'NONE',  ( -19.05341960407611168, -5.049401038298163336, 26.45724293864769550 ) ) ;
#99373=CARTESIAN_POINT ( 'NONE',  ( 21.52544592524344225, -5.823673210054117533, 108.5405762719810241 ) ) ;
#99374=CARTESIAN_POINT ( 'NONE',  ( 19.02544592524334988, 5.153800228976608722, 36.45942372801900433 ) ) ;
#99375=CARTESIAN_POINT ( 'NONE',  ( 12.06949235617757843, -12.14591786802309237, 108.1239096053143811 ) ) ;
#99376=CARTESIAN_POINT ( 'NONE',  ( 19.03943276465977164, -0.05219959533909143690, 63.74890960531435979 ) ) ;
#99377=CARTESIAN_POINT ( 'NONE',  ( -16.46253265017146816, -9.564922557961047289, 104.1677570613523329 ) ) ;
#99378=CARTESIAN_POINT ( 'NONE',  ( -4.379528057220328563, 16.55341960407611168, 60.20724293864768839 ) ) ;
#99379=CARTESIAN_POINT ( 'NONE',  ( 5.049401038297881783, 19.05341960407617563, 22.29275706135233648 ) ) ;
#99380=CARTESIAN_POINT ( 'NONE',  ( -18.67979575497178146, -10.72451020669898902, 26.66557627198103475 ) ) ;
#99381=CARTESIAN_POINT ( 'NONE',  ( -5.049401038297874678, -19.05341960407617918, 89.79275706135230450 ) ) ;
#99382=CARTESIAN_POINT ( 'NONE',  ( -21.55341960407610458, -5.719274019375992779, 91.45724293864769550 ) ) ;
#99383=CARTESIAN_POINT ( 'NONE',  ( -15.80617190586768217, 15.72974639402176855, 48.12609039468568284 ) ) ;
#99384=CARTESIAN_POINT ( 'NONE',  ( 16.55341960407618274, -4.379528057220086978, 41.04275706135236135 ) ) ;
#99385=CARTESIAN_POINT ( 'NONE',  ( 12.06949235617739724, 12.14591786802326823, 111.8760903946856615 ) ) ;
#99386=CARTESIAN_POINT ( 'NONE',  ( 14.34966873604972726, -8.224510206698740333, 35.83442372801901143 ) ) ;
#99387=CARTESIAN_POINT ( 'NONE',  ( 18.62759615963255655, 10.81492255796105972, 51.66775706135234714 ) ) ;
#99388=CARTESIAN_POINT ( 'NONE',  ( 15.72974639402199770, -15.80617190586745480, 53.12390960531436690 ) ) ;
#99389=CARTESIAN_POINT ( 'NONE',  ( 5.049401038298161559, -19.05341960407611168, 32.70724293864768129 ) ) ;
#99391=CARTESIAN_POINT ( 'NONE',  ( -4.379528057220086978, -16.55341960407618274, 74.79275706135234714 ) ) ;
#99392=CARTESIAN_POINT ( 'NONE',  ( 15.72974639402199770, -15.80617190586745480, 93.12390960531436690 ) ) ;
#99393=CARTESIAN_POINT ( 'NONE',  ( 8.314922557960818139, 14.29746914071049879, 34.58224293864770260 ) ) ;
#99394=CARTESIAN_POINT ( 'NONE',  ( -0.05219959533934338120, 16.53943276465976808, 62.50109039468568284 ) ) ;
#99395=CARTESIAN_POINT ( 'NONE',  ( -5.049401038297874678, -19.05341960407617918, 99.79275706135234714 ) ) ;
#99396=CARTESIAN_POINT ( 'NONE',  ( -10.81492255796078084, -18.62759615963271287, 102.0822429386476955 ) ) ;
#99397=CARTESIAN_POINT ( 'NONE',  ( -12.06949235617756955, 12.14591786802309770, 25.62390960531435624 ) ) ;
#99399=CARTESIAN_POINT ( 'NONE',  ( -16.55341960407617563, 4.379528057220093196, 78.54275706135236135 ) ) ;
#99401=CARTESIAN_POINT ( 'NONE',  ( -21.52544592524343514, 5.823673210054127303, 76.04057627198102409 ) ) ;
#99402=CARTESIAN_POINT ( 'NONE',  ( 12.06949235617739724, 12.14591786802326823, 111.8760903946856615 ) ) ;
#99404=CARTESIAN_POINT ( 'NONE',  ( 19.25176906914651198, 5.499999999999741540, 88.49927264242276692 ) ) ;
#99405=CARTESIAN_POINT ( 'NONE',  ( 15.72974639402199770, -15.80617190586745480, 83.12390960531436690 ) ) ;
#99406=CARTESIAN_POINT ( 'NONE',  ( 10.81492255796078972, 18.62759615963270932, 104.5822429386477097 ) ) ;
#99407=CARTESIAN_POINT ( 'NONE',  ( -8.314922557960811034, -14.29746914071050412, 42.08224293864769550 ) ) ;
#99408=CARTESIAN_POINT ( 'NONE',  ( -16.52544592524335698, -4.483927247898792601, 38.95942372801901854 ) ) ;
#99409=CIRCLE ( 'NONE', #5734, 2.000000000000000000 ) ;
#99410=CARTESIAN_POINT ( 'NONE',  ( -13.97604488694527625, -13.89961937509977652, 41.87390960531435979 ) ) ;
#99411=CARTESIAN_POINT ( 'NONE',  ( -13.89961937509977652, 13.97604488694528158, 60.62390960531436690 ) ) ;
#99412=ORIENTED_EDGE ( 'NONE', *, *, #141141, .T. ) ;
#99413=CARTESIAN_POINT ( 'NONE',  ( -0.05219959533907301413, -21.53943276465977519, 27.49890960531435269 ) ) ;
#99414=CARTESIAN_POINT ( 'NONE',  ( -5.049401038298153566, 19.05341960407611168, 115.2072429386477097 ) ) ;
#99415=CARTESIAN_POINT ( 'NONE',  ( -19.02544592524334988, -5.153800228976617603, 103.9594237280190043 ) ) ;
#99416=CARTESIAN_POINT ( 'NONE',  ( -0.05219959533936034679, 19.03943276465977164, 47.50109039468566863 ) ) ;
#99417=CARTESIAN_POINT ( 'NONE',  ( 18.62759615963271287, -10.81492255796078972, 83.33224293864769550 ) ) ;
#99418=CARTESIAN_POINT ( 'NONE',  ( -4.483927247898782831, 16.52544592524335698, 107.7094237280190328 ) ) ;
#99419=CARTESIAN_POINT ( 'NONE',  ( -21.55341960407610458, -5.719274019375992779, 41.45724293864769550 ) ) ;
#99420=CARTESIAN_POINT ( 'NONE',  ( -21.53943276465977519, 0.05219959533907696930, 76.24890960531435269 ) ) ;
#99421=CARTESIAN_POINT ( 'NONE',  ( 13.97604488694548053, -13.89961937509957401, 100.6260903946856615 ) ) ;
#99423=CARTESIAN_POINT ( 'NONE',  ( 0.05219959533909260263, 19.03943276465977164, 99.99890960531436690 ) ) ;
#99424=CARTESIAN_POINT ( 'NONE',  ( -18.67979575497193778, 10.72451020669871902, 73.33442372801901854 ) ) ;
#99425=CARTESIAN_POINT ( 'NONE',  ( -13.89961937509977652, 13.97604488694528158, 70.62390960531432427 ) ) ;
#99427=CARTESIAN_POINT ( 'NONE',  ( -9.564922557960796823, -16.46253265017161027, 77.08224293864769550 ) ) ;
#99428=CARTESIAN_POINT ( 'NONE',  ( -16.52544592524342804, 4.483927247898546575, 86.04057627198102409 ) ) ;
#99429=ORIENTED_EDGE ( 'NONE', *, *, #26797, .T. ) ;
#99430=CARTESIAN_POINT ( 'NONE',  ( 19.02544592524334988, 5.153800228976608722, 106.4594237280190185 ) ) ;
#99431=CARTESIAN_POINT ( 'NONE',  ( 17.05587630539788080, -6.762274262135693270, 83.24180309037316761 ) ) ;
#99432=CARTESIAN_POINT ( 'NONE',  ( -16.51473224551069308, -9.474510206698971260, 71.66557627198102409 ) ) ;
#99434=CARTESIAN_POINT ( 'NONE',  ( -15.80617190586768217, 15.72974639402176855, 83.12609039468568994 ) ) ;
#99435=CARTESIAN_POINT ( 'NONE',  ( -19.05341960407611168, -5.049401038298163336, 101.4572429386476955 ) ) ;
#99436=CARTESIAN_POINT ( 'NONE',  ( -8.314922557961024197, 14.29746914071037800, 72.91775706135234714 ) ) ;
#99438=CARTESIAN_POINT ( 'NONE',  ( -17.44279575226822843, -5.990770900252439191, 74.16442432485679603 ) ) ;
#99439=CARTESIAN_POINT ( 'NONE',  ( -16.51473224551082808, 9.474510206698731452, 53.33442372801900433 ) ) ;
#99440=CARTESIAN_POINT ( 'NONE',  ( -15.72974639402176322, -15.80617190586768395, 109.3760903946857042 ) ) ;
#99444=CARTESIAN_POINT ( 'NONE',  ( -16.53943276465976808, -0.05219959533934237506, 113.7510903946856757 ) ) ;
#99446=CARTESIAN_POINT ( 'NONE',  ( 4.379528057220092307, 16.55341960407617563, 97.29275706135234714 ) ) ;
#99448=CARTESIAN_POINT ( 'NONE',  ( -4.483927247898782831, 16.52544592524335698, 62.70942372801902565 ) ) ;
#99449=CARTESIAN_POINT ( 'NONE',  ( -0.05219959533937732626, 21.53943276465977519, 77.50109039468567573 ) ) ;
#99450=CARTESIAN_POINT ( 'NONE',  ( 0.05219959533936267826, -19.03943276465977164, 95.00109039468567573 ) ) ;
#99451=CARTESIAN_POINT ( 'NONE',  ( -19.05341960407617563, 5.049401038297882671, 38.54275706135233293 ) ) ;
#99452=CARTESIAN_POINT ( 'NONE',  ( 13.89961937509977652, -13.97604488694527269, 73.12390960531436690 ) ) ;
#99453=CARTESIAN_POINT ( 'NONE',  ( 19.03943276465977164, -0.05219959533909143690, 53.74890960531436690 ) ) ;
#99454=CARTESIAN_POINT ( 'NONE',  ( 13.89961937509978007, -13.97604488694527269, 88.12390960531436690 ) ) ;
#99455=CARTESIAN_POINT ( 'NONE',  ( 21.53943276465977519, -0.05219959533907433946, 93.74890960531436690 ) ) ;
#99456=CARTESIAN_POINT ( 'NONE',  ( -15.80617190586745835, -15.72974639402198527, 46.87390960531435979 ) ) ;
#99457=CARTESIAN_POINT ( 'NONE',  ( -16.51473224551069308, -9.474510206698971260, 31.66557627198102054 ) ) ;
#99458=CARTESIAN_POINT ( 'NONE',  ( -8.224510206698735004, -14.34966873604973081, 64.58442372801900433 ) ) ;
#99459=VERTEX_POINT ( 'NONE', #185139 ) ;
#99461=CARTESIAN_POINT ( 'NONE',  ( -15.72974639402176322, -15.80617190586768395, 44.37609039468567573 ) ) ;
#99462=CARTESIAN_POINT ( 'NONE',  ( 16.52544592524342804, -4.483927247898539470, 63.54057627198103830 ) ) ;
#99464=CARTESIAN_POINT ( 'NONE',  ( -12.06949235617739369, -12.14591786802326823, 44.37609039468567573 ) ) ;
#99465=CARTESIAN_POINT ( 'NONE',  ( -16.55341960407611168, -4.379528057220339221, 101.4572429386476955 ) ) ;
#99466=CARTESIAN_POINT ( 'NONE',  ( 16.46253265017146816, 9.564922557961045513, 46.66775706135233293 ) ) ;
#99467=CARTESIAN_POINT ( 'NONE',  ( 14.29746914071049879, -8.314922557960816363, 63.33224293864770260 ) ) ;
#99468=CARTESIAN_POINT ( 'NONE',  ( 5.719274019375673035, 21.55341960407619339, 32.29275706135235424 ) ) ;
#99470=CARTESIAN_POINT ( 'NONE',  ( -10.81492255796078084, -18.62759615963271287, 97.08224293864770971 ) ) ;
#99471=CARTESIAN_POINT ( 'NONE',  ( 19.05341960407611168, 5.049401038298154454, 98.95724293864766707 ) ) ;
#99472=CARTESIAN_POINT ( 'NONE',  ( -16.53943276465976808, 0.05219959533911058130, 76.24890960531435269 ) ) ;
#99473=CARTESIAN_POINT ( 'NONE',  ( -9.564922557960796823, -16.46253265017161027, 112.0822429386476955 ) ) ;
#99475=CARTESIAN_POINT ( 'NONE',  ( -9.564922557961040184, 16.46253265017147172, 87.91775706135233293 ) ) ;
#99476=CARTESIAN_POINT ( 'NONE',  ( -18.67979575497193778, 10.72451020669871902, 28.33442372801902209 ) ) ;
#99477=CARTESIAN_POINT ( 'NONE',  ( -0.05219959533909027116, -19.03943276465977164, 67.49890960531436690 ) ) ;
#99478=CARTESIAN_POINT ( 'NONE',  ( 19.05341960407617918, -5.049401038297876454, 56.04275706135234714 ) ) ;
#99479=CARTESIAN_POINT ( 'NONE',  ( 13.97604488694527802, 13.89961937509977652, 34.37390960531436690 ) ) ;
#99480=CARTESIAN_POINT ( 'NONE',  ( -5.719274019375665041, -21.55341960407619695, 59.79275706135234714 ) ) ;
#99482=CARTESIAN_POINT ( 'NONE',  ( 14.29746914071049879, -8.314922557960816363, 53.33224293864769550 ) ) ;
#99483=CARTESIAN_POINT ( 'NONE',  ( -5.153800228976328057, -19.02544592524343514, 67.29057627198102409 ) ) ;
#99484=CARTESIAN_POINT ( 'NONE',  ( 15.72974639402199770, -15.80617190586745480, 88.12390960531436690 ) ) ;
#99485=CARTESIAN_POINT ( 'NONE',  ( -5.153800228976328057, -19.02544592524343514, 52.29057627198100988 ) ) ;
#99486=ORIENTED_EDGE ( 'NONE', *, *, #155971, .T. ) ;
#99487=CARTESIAN_POINT ( 'NONE',  ( 10.72451020669898902, -18.67979575497178502, 77.91557627198102409 ) ) ;
#99488=CARTESIAN_POINT ( 'NONE',  ( 5.823673210054444382, -21.52544592524334988, 95.20942372801903275 ) ) ;
#99489=CARTESIAN_POINT ( 'NONE',  ( -5.153800228976328057, -19.02544592524343514, 27.29057627198103120 ) ) ;
#99490=CARTESIAN_POINT ( 'NONE',  ( -16.55341960407617563, 4.379528057220093196, 93.54275706135234714 ) ) ;
#99491=CARTESIAN_POINT ( 'NONE',  ( 12.14591786802309770, 12.06949235617756955, 99.37390960531436690 ) ) ;
#99492=CARTESIAN_POINT ( 'NONE',  ( -19.02544592524334988, -5.153800228976617603, 88.95942372801897591 ) ) ;
#99494=CARTESIAN_POINT ( 'NONE',  ( -21.53943276465977519, -0.05219959533937600094, 23.75109039468567929 ) ) ;
#99495=CARTESIAN_POINT ( 'NONE',  ( 16.51473224551083163, -9.474510206698727899, 50.83442372801899722 ) ) ;
#99496=CARTESIAN_POINT ( 'NONE',  ( -0.05219959533934338120, 16.53943276465976808, 97.50109039468567573 ) ) ;
#99497=CARTESIAN_POINT ( 'NONE',  ( 16.46253265017146816, 9.564922557961045513, 26.66775706135234003 ) ) ;
#99498=CARTESIAN_POINT ( 'NONE',  ( 13.89961937509977652, -13.97604488694527269, 98.12390960531433848 ) ) ;
#99499=CARTESIAN_POINT ( 'NONE',  ( -15.72974639402197994, 15.80617190586746368, 65.62390960531436690 ) ) ;
#99501=CARTESIAN_POINT ( 'NONE',  ( -19.03943276465977164, 0.05219959533909376836, 26.24890960531435624 ) ) ;
#99502=CARTESIAN_POINT ( 'NONE',  ( 18.62759615963255655, 10.81492255796105972, 106.6677570613523756 ) ) ;
#99503=CARTESIAN_POINT ( 'NONE',  ( -4.379528057220086978, -16.55341960407618274, 69.79275706135234714 ) ) ;
#99504=CARTESIAN_POINT ( 'NONE',  ( -21.55341960407619339, 5.719274019375674811, 23.54275706135235424 ) ) ;
#99505=CARTESIAN_POINT ( 'NONE',  ( 12.06949235617739724, 12.14591786802326823, 46.87609039468568994 ) ) ;
#99506=CARTESIAN_POINT ( 'NONE',  ( 16.46253265017160672, -9.564922557960803928, 103.3322429386476955 ) ) ;
#99507=CARTESIAN_POINT ( 'NONE',  ( -0.05219959533909027116, -19.03943276465977164, 42.49890960531435269 ) ) ;
#99508=CARTESIAN_POINT ( 'NONE',  ( -19.05341960407611168, -5.049401038298163336, 66.45724293864769550 ) ) ;
#99509=CARTESIAN_POINT ( 'NONE',  ( -0.05219959533934338120, 16.53943276465976808, 42.50109039468567573 ) ) ;
#99510=CARTESIAN_POINT ( 'NONE',  ( -16.52544592524342804, 4.483927247898546575, 91.04057627198103830 ) ) ;
#99511=CARTESIAN_POINT ( 'NONE',  ( -4.379528057220086978, -16.55341960407618274, 104.7927570613523898 ) ) ;
#99512=CARTESIAN_POINT ( 'NONE',  ( -9.474510206698964154, 16.51473224551069663, 50.41557627198102409 ) ) ;
#99513=CARTESIAN_POINT ( 'NONE',  ( 0.05219959533937995610, -21.53943276465977519, 55.00109039468568284 ) ) ;
#99514=CARTESIAN_POINT ( 'NONE',  ( 16.46253265017160672, -9.564922557960803928, 83.33224293864768129 ) ) ;
#99515=CARTESIAN_POINT ( 'NONE',  ( 16.46253265017160672, -9.564922557960803928, 63.33224293864769550 ) ) ;
#99516=CARTESIAN_POINT ( 'NONE',  ( 9.564922557960805705, 16.46253265017160317, 89.58224293864769550 ) ) ;
#99517=CARTESIAN_POINT ( 'NONE',  ( 16.52544592524342804, -4.483927247898539470, 48.54057627198103120 ) ) ;
#99518=CARTESIAN_POINT ( 'NONE',  ( 12.14591786802327356, -12.06949235617739191, 95.62609039468568994 ) ) ;
#99519=CARTESIAN_POINT ( 'NONE',  ( 8.314922557960818139, 14.29746914071049879, 24.58224293864768839 ) ) ;
#99521=CARTESIAN_POINT ( 'NONE',  ( -5.049401038297874678, -19.05341960407617918, 44.79275706135232582 ) ) ;
#99522=CARTESIAN_POINT ( 'NONE',  ( 9.474510206698971260, -16.51473224551069308, 112.9155762719810383 ) ) ;
#99523=CARTESIAN_POINT ( 'NONE',  ( 9.474510206698971260, -16.51473224551069308, 57.91557627198103120 ) ) ;
#99524=CARTESIAN_POINT ( 'NONE',  ( -16.51473224551082808, 9.474510206698731452, 33.33442372801899722 ) ) ;
#99527=CARTESIAN_POINT ( 'NONE',  ( -5.049401038297874678, -19.05341960407617918, 79.79275706135233293 ) ) ;
#99528=CARTESIAN_POINT ( 'NONE',  ( 12.14591786802327356, -12.06949235617739191, 70.62609039468567573 ) ) ;
#99529=CARTESIAN_POINT ( 'NONE',  ( 16.38665767535053064, 7.295008042176115204, 92.23599135785453029 ) ) ;
#99530=CARTESIAN_POINT ( 'NONE',  ( -9.474510206698964154, 16.51473224551069663, 85.41557627198102409 ) ) ;
#99531=CARTESIAN_POINT ( 'NONE',  ( -21.55341960407619339, 5.719274019375674811, 33.54275706135234714 ) ) ;
#99532=CARTESIAN_POINT ( 'NONE',  ( 16.51473224551083163, -9.474510206698727899, 70.83442372801900433 ) ) ;
#99533=CARTESIAN_POINT ( 'NONE',  ( 17.48853670773247870, 5.747243402303060300, 88.83328700250011423 ) ) ;
#99534=CARTESIAN_POINT ( 'NONE',  ( -16.46253265017160317, 9.564922557960807481, 30.83224293864769550 ) ) ;
#99535=CARTESIAN_POINT ( 'NONE',  ( 19.05341960407611168, 5.049401038298154454, 88.95724293864769550 ) ) ;
#99536=CARTESIAN_POINT ( 'NONE',  ( -4.483927247898539470, -16.52544592524342804, 47.29057627198103120 ) ) ;
#99537=CARTESIAN_POINT ( 'NONE',  ( 16.51473224551069308, 9.474510206698969483, 39.16557627198103120 ) ) ;
#99538=CARTESIAN_POINT ( 'NONE',  ( 19.05341960407617918, -5.049401038297876454, 46.04275706135233293 ) ) ;
#99540=CARTESIAN_POINT ( 'NONE',  ( -8.314922557960811034, -14.29746914071050412, 82.08224293864768129 ) ) ;
#99541=CARTESIAN_POINT ( 'NONE',  ( -9.474510206698720793, -16.51473224551083518, 34.58442372801899722 ) ) ;
#99542=CARTESIAN_POINT ( 'NONE',  ( -9.564922557960796823, -16.46253265017161027, 62.08224293864769550 ) ) ;
#99543=CARTESIAN_POINT ( 'NONE',  ( -21.53943276465977519, 0.05219959533907696930, 61.24890960531435979 ) ) ;
#99544=CARTESIAN_POINT ( 'NONE',  ( 12.14591786802309770, 12.06949235617756955, 49.37390960531436690 ) ) ;
#99545=CARTESIAN_POINT ( 'NONE',  ( -0.05219959533936034679, 19.03943276465977164, 22.50109039468566152 ) ) ;
#99546=CARTESIAN_POINT ( 'NONE',  ( -0.05219959533909027116, -19.03943276465977164, 112.4989096053143669 ) ) ;
#99547=CARTESIAN_POINT ( 'NONE',  ( -0.05219959533907301413, -21.53943276465977519, 22.49890960531436335 ) ) ;
#99548=CARTESIAN_POINT ( 'NONE',  ( -5.049401038298153566, 19.05341960407611168, 55.20724293864769550 ) ) ;
#99549=CARTESIAN_POINT ( 'NONE',  ( 9.474510206698971260, -16.51473224551069308, 22.91557627198102765 ) ) ;
#99550=CARTESIAN_POINT ( 'NONE',  ( -8.224510206698948167, 14.34966873604960824, 85.41557627198102409 ) ) ;
#99551=CARTESIAN_POINT ( 'NONE',  ( 18.62759615963271287, -10.81492255796078972, 103.3322429386476955 ) ) ;
#99552=CARTESIAN_POINT ( 'NONE',  ( -9.564922557960796823, -16.46253265017161027, 102.0822429386477097 ) ) ;
#99553=CARTESIAN_POINT ( 'NONE',  ( 21.52544592524344225, -5.823673210054117533, 108.5405762719810241 ) ) ;
#99554=CARTESIAN_POINT ( 'NONE',  ( 5.049401038298161559, -19.05341960407611168, 107.7072429386476955 ) ) ;
#99555=CARTESIAN_POINT ( 'NONE',  ( -0.05219959533909027116, -19.03943276465977164, 22.49890960531436690 ) ) ;
#99556=CARTESIAN_POINT ( 'NONE',  ( -21.55341960407619339, 5.719274019375674811, 83.54275706135234714 ) ) ;
#99557=CARTESIAN_POINT ( 'NONE',  ( -0.05219959533907301413, -21.53943276465977519, 97.49890960531436690 ) ) ;
#99559=CARTESIAN_POINT ( 'NONE',  ( 18.87580814761076908, -5.500000000000053291, 78.37172394265758157 ) ) ;
#99561=CARTESIAN_POINT ( 'NONE',  ( 8.314922557961029526, -14.29746914071037800, 40.41775706135234714 ) ) ;
#99563=CARTESIAN_POINT ( 'NONE',  ( 4.483927247898545687, 16.52544592524342804, 109.7905762719810383 ) ) ;
#99565=CARTESIAN_POINT ( 'NONE',  ( 19.05341960407611168, 5.049401038298154454, 53.95724293864770260 ) ) ;
#99566=CARTESIAN_POINT ( 'NONE',  ( -8.224510206698948167, 14.34966873604960824, 90.41557627198103830 ) ) ;
#99567=CARTESIAN_POINT ( 'NONE',  ( 10.72451020669898902, -18.67979575497178502, 32.91557627198102409 ) ) ;
#99568=CARTESIAN_POINT ( 'NONE',  ( -12.14591786802309592, -12.06949235617757132, 61.87390960531436690 ) ) ;
#99569=CARTESIAN_POINT ( 'NONE',  ( 19.03943276465977164, 0.05219959533936151252, 111.2510903946856757 ) ) ;
#99570=CARTESIAN_POINT ( 'NONE',  ( -0.05219959533937732626, 21.53943276465977519, 77.50109039468567573 ) ) ;
#99571=CARTESIAN_POINT ( 'NONE',  ( 17.49999999999999645, -5.624438216177592764, 78.31670344914645909 ) ) ;
#99572=CARTESIAN_POINT ( 'NONE',  ( 8.314922557961029526, -14.29746914071037800, 100.4177570613523471 ) ) ;
#99573=CARTESIAN_POINT ( 'NONE',  ( 5.153800228976335163, 19.02544592524342804, 39.79057627198100988 ) ) ;
#99574=CARTESIAN_POINT ( 'NONE',  ( 13.89961937509977652, -13.97604488694527269, 88.12390960531438111 ) ) ;
#99575=CARTESIAN_POINT ( 'NONE',  ( 21.52544592524344225, -5.823673210054117533, 93.54057627198103830 ) ) ;
#99576=CARTESIAN_POINT ( 'NONE',  ( 16.55341960407618274, -4.379528057220086978, 26.04275706135235779 ) ) ;
#99577=CARTESIAN_POINT ( 'NONE',  ( 12.14591786802309770, 12.06949235617756955, 69.37390960531436690 ) ) ;
#99578=CARTESIAN_POINT ( 'NONE',  ( 15.72974639402176855, 15.80617190586768217, 71.87609039468568994 ) ) ;
#99580=CARTESIAN_POINT ( 'NONE',  ( -16.52544592524335698, -4.483927247898792601, 93.95942372801903275 ) ) ;
#99581=CARTESIAN_POINT ( 'NONE',  ( 17.50000000000000355, -5.624438216177558125, 48.31670344914645199 ) ) ;
#99582=CARTESIAN_POINT ( 'NONE',  ( -19.39720447994795549, -5.499999999999980460, 64.66317477297177163 ) ) ;
#99583=CARTESIAN_POINT ( 'NONE',  ( 14.29746914071049879, -8.314922557960816363, 28.33224293864769550 ) ) ;
#99584=CARTESIAN_POINT ( 'NONE',  ( -0.05219959533934338120, 16.53943276465976808, 77.50109039468567573 ) ) ;
#99585=CARTESIAN_POINT ( 'NONE',  ( -13.89961937509977652, 13.97604488694528158, 80.62390960531436690 ) ) ;
#99586=CARTESIAN_POINT ( 'NONE',  ( -19.05341960407611168, -5.049401038298163336, 91.45724293864766707 ) ) ;
#99587=CARTESIAN_POINT ( 'NONE',  ( 21.52544592524334988, 5.823673210054432836, 91.45942372801901854 ) ) ;
#99588=EDGE_CURVE ( 'NONE', #147783, #85848, #55873, .T. ) ;
#99589=CARTESIAN_POINT ( 'NONE',  ( 4.483927247898790824, -16.52544592524335698, 85.20942372801901854 ) ) ;
#99590=CARTESIAN_POINT ( 'NONE',  ( -14.29746914071049879, 8.314922557960819915, 65.83224293864769550 ) ) ;
#99591=CARTESIAN_POINT ( 'NONE',  ( -13.89961937509977652, 13.97604488694528158, 70.62390960531432427 ) ) ;
#99593=CARTESIAN_POINT ( 'NONE',  ( 0.05219959533934541429, -16.53943276465976808, 20.00109039468568639 ) ) ;
#99594=CARTESIAN_POINT ( 'NONE',  ( 4.483927247898545687, 16.52544592524342804, 104.7905762719810241 ) ) ;
#99595=CARTESIAN_POINT ( 'NONE',  ( -5.153800228976328057, -19.02544592524343514, 77.29057627198099567 ) ) ;
#99596=CARTESIAN_POINT ( 'NONE',  ( -9.474510206698720793, -16.51473224551083518, 109.5844237280190043 ) ) ;
#99598=CARTESIAN_POINT ( 'NONE',  ( 13.89961937509957401, 13.97604488694547697, 26.87609039468566507 ) ) ;
#99599=CARTESIAN_POINT ( 'NONE',  ( -4.379528057220086978, -16.55341960407618274, 84.79275706135234714 ) ) ;
#99600=CARTESIAN_POINT ( 'NONE',  ( 9.474510206698729675, 16.51473224551082808, 92.08442372801900433 ) ) ;
#99601=CARTESIAN_POINT ( 'NONE',  ( -16.55341960407611168, -4.379528057220339221, 111.4572429386476813 ) ) ;
#99602=CARTESIAN_POINT ( 'NONE',  ( -4.483927247898782831, 16.52544592524335698, 62.70942372801902565 ) ) ;
#99603=CARTESIAN_POINT ( 'NONE',  ( -0.05219959533934338120, 16.53943276465976808, 52.50109039468567573 ) ) ;
#99604=CARTESIAN_POINT ( 'NONE',  ( -13.97604488694527625, -13.89961937509977652, 21.87390960531435979 ) ) ;
#99605=CARTESIAN_POINT ( 'NONE',  ( 13.97604488694548053, -13.89961937509957401, 55.62609039468566863 ) ) ;
#99606=CARTESIAN_POINT ( 'NONE',  ( 21.52544592524334988, 5.823673210054432836, 91.45942372801901854 ) ) ;
#99607=CARTESIAN_POINT ( 'NONE',  ( -16.46253265017160317, 9.564922557960807481, 40.83224293864769550 ) ) ;
#99608=CARTESIAN_POINT ( 'NONE',  ( -19.03943276465977164, 0.05219959533909376836, 76.24890960531435269 ) ) ;
#99609=CARTESIAN_POINT ( 'NONE',  ( 12.14591786802309770, 12.06949235617756955, 74.37390960531436690 ) ) ;
#99610=CARTESIAN_POINT ( 'NONE',  ( 18.67979575497194134, -10.72451020669871369, 85.83442372801901854 ) ) ;
#99611=CARTESIAN_POINT ( 'NONE',  ( 9.564922557961047289, -16.46253265017146816, 55.41775706135234003 ) ) ;
#99612=CARTESIAN_POINT ( 'NONE',  ( -0.05219959533936034679, 19.03943276465977164, 47.50109039468566863 ) ) ;
#99613=CARTESIAN_POINT ( 'NONE',  ( -21.55341960407610458, -5.719274019375992779, 31.45724293864769550 ) ) ;
#99614=CARTESIAN_POINT ( 'NONE',  ( 18.62759615963255655, 10.81492255796105972, 96.66775706135234714 ) ) ;
#99615=CARTESIAN_POINT ( 'NONE',  ( -5.049401038298153566, 19.05341960407611168, 75.20724293864769550 ) ) ;
#99616=CARTESIAN_POINT ( 'NONE',  ( -5.719274019375665041, -21.55341960407619695, 109.7927570613523613 ) ) ;
#99617=CARTESIAN_POINT ( 'NONE',  ( 18.62759615963271287, -10.81492255796078972, 48.33224293864770260 ) ) ;
#99618=CARTESIAN_POINT ( 'NONE',  ( 0.05219959533909260263, 19.03943276465977164, 94.99890960531436690 ) ) ;
#99619=CARTESIAN_POINT ( 'NONE',  ( -0.05219959533936034679, 19.03943276465977164, 77.50109039468566152 ) ) ;
#99620=CARTESIAN_POINT ( 'NONE',  ( -16.51473224551069308, -9.474510206698971260, 101.6655762719810241 ) ) ;
#99621=CARTESIAN_POINT ( 'NONE',  ( -9.474510206698720793, -16.51473224551083518, 99.58442372801900433 ) ) ;
#99622=CARTESIAN_POINT ( 'NONE',  ( -16.53943276465976808, -0.05219959533934237506, 38.75109039468567573 ) ) ;
#99623=CARTESIAN_POINT ( 'NONE',  ( 16.55341960407611168, 4.379528057220329451, 103.9572429386476813 ) ) ;
#99624=CARTESIAN_POINT ( 'NONE',  ( 9.474510206698971260, -16.51473224551069308, 87.91557627198102409 ) ) ;
#99625=CARTESIAN_POINT ( 'NONE',  ( -18.62759615963270932, 10.81492255796079327, 65.83224293864769550 ) ) ;
#99626=CARTESIAN_POINT ( 'NONE',  ( -8.314922557961024197, 14.29746914071037800, 37.91775706135235424 ) ) ;
#99627=CARTESIAN_POINT ( 'NONE',  ( -5.719274019375665041, -21.55341960407619695, 34.79275706135235424 ) ) ;
#99628=CARTESIAN_POINT ( 'NONE',  ( -21.55341960407619339, 5.719274019375674811, 78.54275706135236135 ) ) ;
#99629=CARTESIAN_POINT ( 'NONE',  ( 8.224510206698742110, 14.34966873604972548, 77.08442372801901854 ) ) ;
#99630=CARTESIAN_POINT ( 'NONE',  ( -5.049401038298153566, 19.05341960407611168, 70.20724293864769550 ) ) ;
#99631=CARTESIAN_POINT ( 'NONE',  ( -12.14591786802309592, -12.06949235617757132, 76.87390960531439532 ) ) ;
#99632=CARTESIAN_POINT ( 'NONE',  ( -0.05219959533910754901, -16.53943276465976808, 27.49890960531435269 ) ) ;
#99633=CARTESIAN_POINT ( 'NONE',  ( 19.05341960407617918, -5.049401038297876454, 61.04275706135232582 ) ) ;
#99634=CARTESIAN_POINT ( 'NONE',  ( 18.62759615963255655, 10.81492255796105972, 26.66775706135235424 ) ) ;
#99635=CARTESIAN_POINT ( 'NONE',  ( -0.05219959533910754901, -16.53943276465976808, 72.49890960531435269 ) ) ;
#99636=CARTESIAN_POINT ( 'NONE',  ( 19.02544592524343514, -5.153800228976328945, 113.5405762719810241 ) ) ;
#99637=CARTESIAN_POINT ( 'NONE',  ( 16.52544592524335698, 4.483927247898782831, 101.4594237280190185 ) ) ;
#99638=CARTESIAN_POINT ( 'NONE',  ( -5.719274019375665041, -21.55341960407619695, 74.79275706135234714 ) ) ;
#99639=CARTESIAN_POINT ( 'NONE',  ( 4.483927247898790824, -16.52544592524335698, 50.20942372801901854 ) ) ;
#99640=CARTESIAN_POINT ( 'NONE',  ( 21.53943276465977519, 0.05219959533937863772, 36.25109039468567573 ) ) ;
#99642=CARTESIAN_POINT ( 'NONE',  ( 10.81492255796078972, 18.62759615963270932, 114.5822429386477097 ) ) ;
#99643=CARTESIAN_POINT ( 'NONE',  ( 12.14591786802309770, 12.06949235617756955, 89.37390960531435269 ) ) ;
#99645=CARTESIAN_POINT ( 'NONE',  ( -12.14591786802309592, -12.06949235617757132, 46.87390960531435979 ) ) ;
#99646=CARTESIAN_POINT ( 'NONE',  ( -19.03943276465977164, 0.05219959533909376836, 26.24890960531435624 ) ) ;
#99647=CARTESIAN_POINT ( 'NONE',  ( 0.05219959533907565091, 21.53943276465977519, 44.99890960531435979 ) ) ;
#99648=CARTESIAN_POINT ( 'NONE',  ( 0.05219959533910956823, 16.53943276465976808, 74.99890960531435269 ) ) ;
#99649=CARTESIAN_POINT ( 'NONE',  ( 21.53943276465977519, -0.05219959533907433946, 78.74890960531436690 ) ) ;
#99650=CARTESIAN_POINT ( 'NONE',  ( 5.049401038298161559, -19.05341960407611168, 92.70724293864769550 ) ) ;
#99651=CARTESIAN_POINT ( 'NONE',  ( 5.153800228976335163, 19.02544592524342804, 44.79057627198103830 ) ) ;
#99652=CARTESIAN_POINT ( 'NONE',  ( 9.564922557961047289, -16.46253265017146816, 95.41775706135233293 ) ) ;
#99653=CARTESIAN_POINT ( 'NONE',  ( 5.823673210054125526, 21.52544592524343514, 29.79057627198102409 ) ) ;
#99654=CARTESIAN_POINT ( 'NONE',  ( 21.52544592524334988, 5.823673210054432836, 56.45942372801902565 ) ) ;
#99655=CARTESIAN_POINT ( 'NONE',  ( -10.81492255796078084, -18.62759615963271287, 67.08224293864770971 ) ) ;
#99656=CARTESIAN_POINT ( 'NONE',  ( -0.05219959533909027116, -19.03943276465977164, 37.49890960531436690 ) ) ;
#99657=CARTESIAN_POINT ( 'NONE',  ( 5.153800228976335163, 19.02544592524342804, 74.79057627198103830 ) ) ;
#99659=CARTESIAN_POINT ( 'NONE',  ( 16.52544592524335698, 4.483927247898782831, 46.45942372801901854 ) ) ;
#99660=CARTESIAN_POINT ( 'NONE',  ( -21.53943276465977519, -0.05219959533937600094, 28.75109039468567929 ) ) ;
#99661=CARTESIAN_POINT ( 'NONE',  ( -18.62759615963255300, -10.81492255796106328, 69.16775706135234714 ) ) ;
#99662=CARTESIAN_POINT ( 'NONE',  ( -5.719274019375978568, 21.55341960407610458, 25.20724293864769550 ) ) ;
#99663=CARTESIAN_POINT ( 'NONE',  ( -10.81492255796078084, -18.62759615963271287, 87.08224293864769550 ) ) ;
#99664=CARTESIAN_POINT ( 'NONE',  ( -10.81492255796105439, 18.62759615963255655, 22.91775706135235069 ) ) ;
#99665=CARTESIAN_POINT ( 'NONE',  ( 8.314922557961029526, -14.29746914071037800, 50.41775706135235424 ) ) ;
#99667=CARTESIAN_POINT ( 'NONE',  ( -18.67979575497178146, -10.72451020669898902, 56.66557627198103830 ) ) ;
#99668=CARTESIAN_POINT ( 'NONE',  ( 13.97604488694548053, -13.89961937509957401, 20.62609039468567573 ) ) ;
#99669=CARTESIAN_POINT ( 'NONE',  ( 13.97604488694527802, 13.89961937509977652, 49.37390960531434558 ) ) ;
#99670=CARTESIAN_POINT ( 'NONE',  ( 19.05341960407611168, 5.049401038298154454, 113.9572429386477097 ) ) ;
#99671=CARTESIAN_POINT ( 'NONE',  ( -19.03943276465977164, 0.05219959533909376836, 96.24890960531436690 ) ) ;
#99673=CARTESIAN_POINT ( 'NONE',  ( 19.02544592524334988, 5.153800228976608722, 66.45942372801899012 ) ) ;
#99674=CARTESIAN_POINT ( 'NONE',  ( 18.62759615963271287, -10.81492255796078972, 48.33224293864770260 ) ) ;
#99675=CARTESIAN_POINT ( 'NONE',  ( -14.29746914071049879, 8.314922557960819915, 25.83224293864769194 ) ) ;
#99676=CARTESIAN_POINT ( 'NONE',  ( 9.564922557961047289, -16.46253265017146816, 95.41775706135233293 ) ) ;
#99677=CARTESIAN_POINT ( 'NONE',  ( -19.05341960407611168, -5.049401038298163336, 21.45724293864768839 ) ) ;
#99678=CARTESIAN_POINT ( 'NONE',  ( 16.46253265017146816, 9.564922557961045513, 26.66775706135234003 ) ) ;
#99679=CARTESIAN_POINT ( 'NONE',  ( -16.46253265017146816, -9.564922557961047289, 99.16775706135233293 ) ) ;
#99680=CARTESIAN_POINT ( 'NONE',  ( -0.05219959533907301413, -21.53943276465977519, 87.49890960531436690 ) ) ;
#99681=CARTESIAN_POINT ( 'NONE',  ( 16.46253265017146816, 9.564922557961045513, 61.66775706135234003 ) ) ;
#99683=CARTESIAN_POINT ( 'NONE',  ( -13.89961937509977652, 13.97604488694528158, 55.62390960531434558 ) ) ;
#99684=CARTESIAN_POINT ( 'NONE',  ( -12.06949235617756955, 12.14591786802309770, 65.62390960531436690 ) ) ;
#99685=CARTESIAN_POINT ( 'NONE',  ( 16.51473224551069308, 9.474510206698969483, 49.16557627198102409 ) ) ;
#99686=CARTESIAN_POINT ( 'NONE',  ( 8.224510206698953496, -14.34966873604960469, 57.91557627198103120 ) ) ;
#99688=CARTESIAN_POINT ( 'NONE',  ( -12.06949235617756955, 12.14591786802309770, 25.62390960531435624 ) ) ;
#99689=CARTESIAN_POINT ( 'NONE',  ( 16.51473224551069308, 9.474510206698969483, 69.16557627198102409 ) ) ;
#99690=CARTESIAN_POINT ( 'NONE',  ( -13.89961937509957401, -13.97604488694547875, 29.37609039468565797 ) ) ;
#99691=CARTESIAN_POINT ( 'NONE',  ( 12.06949235617739724, 12.14591786802326823, 31.87609039468567929 ) ) ;
#99692=CARTESIAN_POINT ( 'NONE',  ( -21.55341960407610458, -5.719274019375992779, 46.45724293864769550 ) ) ;
#99693=CARTESIAN_POINT ( 'NONE',  ( -21.53943276465977519, -0.05219959533937600094, 98.75109039468568994 ) ) ;
#99695=CARTESIAN_POINT ( 'NONE',  ( -5.049401038298153566, 19.05341960407611168, 60.20724293864768129 ) ) ;
#99697=CARTESIAN_POINT ( 'NONE',  ( 5.049401038298161559, -19.05341960407611168, 92.70724293864769550 ) ) ;
#99699=CARTESIAN_POINT ( 'NONE',  ( -15.72974639402176322, -15.80617190586768395, 29.37609039468568284 ) ) ;
#99700=CARTESIAN_POINT ( 'NONE',  ( -8.314922557960811034, -14.29746914071050412, 92.08224293864769550 ) ) ;
#99701=CARTESIAN_POINT ( 'NONE',  ( 18.67979575497178502, 10.72451020669898547, 94.16557627198103830 ) ) ;
#99702=CARTESIAN_POINT ( 'NONE',  ( 19.02544592524343514, -5.153800228976328945, 68.54057627198103830 ) ) ;
#99703=CARTESIAN_POINT ( 'NONE',  ( 13.97604488694527802, 13.89961937509977652, 89.37390960531436690 ) ) ;
#99704=CARTESIAN_POINT ( 'NONE',  ( -18.67979575497178146, -10.72451020669898902, 111.6655762719810525 ) ) ;
#99706=CARTESIAN_POINT ( 'NONE',  ( -9.474510206698964154, 16.51473224551069663, 70.41557627198102409 ) ) ;
#99707=DIRECTION ( 'NONE',  ( -1.000000000000000000, -0.000000000000000000, -0.000000000000000000 ) ) ;
#99708=CARTESIAN_POINT ( 'NONE',  ( -12.06949235617756955, 12.14591786802309770, 110.6239096053143669 ) ) ;
#99710=CARTESIAN_POINT ( 'NONE',  ( 13.89961937509957401, 13.97604488694547697, 91.87609039468567573 ) ) ;
#99711=CARTESIAN_POINT ( 'NONE',  ( 16.52544592524342804, -4.483927247898539470, 113.5405762719810383 ) ) ;
#99712=CARTESIAN_POINT ( 'NONE',  ( 15.72974639402176855, 15.80617190586768217, 76.87609039468567573 ) ) ;
#99713=CARTESIAN_POINT ( 'NONE',  ( 5.153800228976335163, 19.02544592524342804, 64.79057627198100988 ) ) ;
#99714=CARTESIAN_POINT ( 'NONE',  ( 21.55341960407619695, -5.719274019375665929, 31.04275706135234714 ) ) ;
#99715=CARTESIAN_POINT ( 'NONE',  ( -21.55341960407610458, -5.719274019375992779, 111.4572429386476813 ) ) ;
#99717=CARTESIAN_POINT ( 'NONE',  ( -5.049401038298153566, 19.05341960407611168, 70.20724293864769550 ) ) ;
#99719=CARTESIAN_POINT ( 'NONE',  ( -4.483927247898782831, 16.52544592524335698, 27.70942372801901854 ) ) ;
#99720=CARTESIAN_POINT ( 'NONE',  ( -10.72451020669898014, 18.67979575497178502, 25.41557627198103120 ) ) ;
#99721=CARTESIAN_POINT ( 'NONE',  ( -15.80617190586768217, 15.72974639402176855, 58.12609039468568994 ) ) ;
#99722=CARTESIAN_POINT ( 'NONE',  ( -19.05341960407611168, -5.049401038298163336, 111.4572429386476671 ) ) ;
#99723=CARTESIAN_POINT ( 'NONE',  ( -5.153800228976607833, 19.02544592524334988, 97.70942372801900433 ) ) ;
#99724=CARTESIAN_POINT ( 'NONE',  ( -16.46253265017160317, 9.564922557960807481, 50.83224293864770260 ) ) ;
#99725=CARTESIAN_POINT ( 'NONE',  ( -9.564922557960796823, -16.46253265017161027, 72.08224293864770971 ) ) ;
#99726=CARTESIAN_POINT ( 'NONE',  ( -14.29746914071049879, 8.314922557960819915, 90.83224293864769550 ) ) ;
#99727=CARTESIAN_POINT ( 'NONE',  ( -9.564922557960796823, -16.46253265017161027, 107.0822429386476955 ) ) ;
#99728=CARTESIAN_POINT ( 'NONE',  ( 0.05219959533910956823, 16.53943276465976808, 89.99890960531438111 ) ) ;
#99729=CARTESIAN_POINT ( 'NONE',  ( 16.46253265017160672, -9.564922557960803928, 98.33224293864769550 ) ) ;
#99730=CARTESIAN_POINT ( 'NONE',  ( 16.52544592524342804, -4.483927247898539470, 58.54057627198103120 ) ) ;
#99731=CARTESIAN_POINT ( 'NONE',  ( 16.46253265017160672, -9.564922557960803928, 38.33224293864768839 ) ) ;
#99732=CARTESIAN_POINT ( 'NONE',  ( -15.80617190586768217, 15.72974639402176855, 63.12609039468568994 ) ) ;
#99733=CARTESIAN_POINT ( 'NONE',  ( -9.474510206698720793, -16.51473224551083518, 94.58442372801900433 ) ) ;
#99734=CARTESIAN_POINT ( 'NONE',  ( 8.314922557960818139, 14.29746914071049879, 44.58224293864769550 ) ) ;
#99735=CARTESIAN_POINT ( 'NONE',  ( 18.62759615963271287, -10.81492255796078972, 98.33224293864769550 ) ) ;
#99736=CARTESIAN_POINT ( 'NONE',  ( -0.05219959533907301413, -21.53943276465977519, 47.49890960531435979 ) ) ;
#99737=CARTESIAN_POINT ( 'NONE',  ( 9.564922557960805705, 16.46253265017160317, 114.5822429386476955 ) ) ;
#99738=CARTESIAN_POINT ( 'NONE',  ( 14.34966873604960469, 8.224510206698951720, 84.16557627198103830 ) ) ;
#99740=CARTESIAN_POINT ( 'NONE',  ( -9.474510206698964154, 16.51473224551069663, 55.41557627198103120 ) ) ;
#99741=CARTESIAN_POINT ( 'NONE',  ( -12.14591786802309592, -12.06949235617757132, 26.87390960531435979 ) ) ;
#99742=CARTESIAN_POINT ( 'NONE',  ( 12.06949235617739724, 12.14591786802326823, 96.87609039468568994 ) ) ;
#99743=CARTESIAN_POINT ( 'NONE',  ( -4.483927247898782831, 16.52544592524335698, 77.70942372801900433 ) ) ;
#99744=CARTESIAN_POINT ( 'NONE',  ( 9.474510206698729675, 16.51473224551082808, 42.08442372801900433 ) ) ;
#99745=CARTESIAN_POINT ( 'NONE',  ( -16.38665767535050577, 7.295008042176172047, 70.26400864214545550 ) ) ;
#99746=CARTESIAN_POINT ( 'NONE',  ( 9.564922557960805705, 16.46253265017160317, 109.5822429386476955 ) ) ;
#99747=CARTESIAN_POINT ( 'NONE',  ( 13.97604488694527802, 13.89961937509977652, 84.37390960531433848 ) ) ;
#99748=CARTESIAN_POINT ( 'NONE',  ( 16.46253265017160672, -9.564922557960803928, 43.33224293864769550 ) ) ;
#99749=CARTESIAN_POINT ( 'NONE',  ( 4.483927247898545687, 16.52544592524342804, 44.79057627198103120 ) ) ;
#99751=CARTESIAN_POINT ( 'NONE',  ( -5.049401038298153566, 19.05341960407611168, 110.2072429386476671 ) ) ;
#99752=CARTESIAN_POINT ( 'NONE',  ( 5.823673210054125526, 21.52544592524343514, 34.79057627198103120 ) ) ;
#99753=CARTESIAN_POINT ( 'NONE',  ( 14.29746914071049879, -8.314922557960816363, 88.33224293864769550 ) ) ;
#99754=CARTESIAN_POINT ( 'NONE',  ( 14.34966873604972726, -8.224510206698740333, 40.83442372801901854 ) ) ;
#99755=CARTESIAN_POINT ( 'NONE',  ( -0.05219959533910754901, -16.53943276465976808, 72.49890960531435269 ) ) ;
#99757=CARTESIAN_POINT ( 'NONE',  ( 9.564922557961047289, -16.46253265017146816, 70.41775706135233293 ) ) ;
#99758=CARTESIAN_POINT ( 'NONE',  ( 19.02544592524343514, -5.153800228976328945, 103.5405762719809957 ) ) ;
#99759=CARTESIAN_POINT ( 'NONE',  ( 9.474510206698729675, 16.51473224551082808, 82.08442372801899012 ) ) ;
#99760=CARTESIAN_POINT ( 'NONE',  ( 0.05219959533936267826, -19.03943276465977164, 95.00109039468567573 ) ) ;
#99761=CARTESIAN_POINT ( 'NONE',  ( -4.379528057220086978, -16.55341960407618274, 29.79275706135234358 ) ) ;
#99762=CARTESIAN_POINT ( 'NONE',  ( -14.29746914071037622, -8.314922557961029526, 109.1677570613523613 ) ) ;
#99763=CARTESIAN_POINT ( 'NONE',  ( -0.05219959533936034679, 19.03943276465977164, 77.50109039468566152 ) ) ;
#99764=CARTESIAN_POINT ( 'NONE',  ( 5.823673210054125526, 21.52544592524343514, 34.79057627198103120 ) ) ;
#99765=CARTESIAN_POINT ( 'NONE',  ( 5.719274019375673035, 21.55341960407619339, 67.29275706135234714 ) ) ;
#99767=CARTESIAN_POINT ( 'NONE',  ( 5.049401038297881783, 19.05341960407617563, 112.2927570613523471 ) ) ;
#99768=CARTESIAN_POINT ( 'NONE',  ( 9.474510206698971260, -16.51473224551069308, 22.91557627198102765 ) ) ;
#99769=CARTESIAN_POINT ( 'NONE',  ( 13.97604488694527802, 13.89961937509977652, 84.37390960531433848 ) ) ;
#99770=CARTESIAN_POINT ( 'NONE',  ( -0.05219959533909027116, -19.03943276465977164, 27.49890960531435624 ) ) ;
#99771=CARTESIAN_POINT ( 'NONE',  ( -16.55341960407611168, -4.379528057220339221, 81.45724293864769550 ) ) ;
#99772=CARTESIAN_POINT ( 'NONE',  ( 19.05341960407611168, 5.049401038298154454, 78.95724293864769550 ) ) ;
#99774=CARTESIAN_POINT ( 'NONE',  ( -13.97604488694527625, -13.89961937509977652, 91.87390960531432427 ) ) ;
#99775=VERTEX_POINT ( 'NONE', #188140 ) ;
#99776=CARTESIAN_POINT ( 'NONE',  ( -5.153800228976607833, 19.02544592524334988, 97.70942372801900433 ) ) ;
#99777=CARTESIAN_POINT ( 'NONE',  ( -15.80617190586745835, -15.72974639402198527, 81.87390960531435269 ) ) ;
#99778=CARTESIAN_POINT ( 'NONE',  ( 9.564922557960805705, 16.46253265017160317, 29.58224293864769550 ) ) ;
#99779=CARTESIAN_POINT ( 'NONE',  ( -16.46253265017146816, -9.564922557961047289, 74.16775706135234714 ) ) ;
#99780=CARTESIAN_POINT ( 'NONE',  ( -21.55341960407610458, -5.719274019375992779, 111.4572429386476813 ) ) ;
#99781=CARTESIAN_POINT ( 'NONE',  ( -19.03943276465977164, 0.05219959533909376836, 76.24890960531435269 ) ) ;
#99782=CARTESIAN_POINT ( 'NONE',  ( 13.89961937509977652, -13.97604488694527269, 108.1239096053143669 ) ) ;
#99784=CARTESIAN_POINT ( 'NONE',  ( -15.80617190586745835, -15.72974639402198527, 106.8739096053143811 ) ) ;
#99785=CARTESIAN_POINT ( 'NONE',  ( -16.52544592524342804, 4.483927247898546575, 96.04057627198102409 ) ) ;
#99786=CARTESIAN_POINT ( 'NONE',  ( -13.97604488694527625, -13.89961937509977652, 81.87390960531436690 ) ) ;
#99787=CARTESIAN_POINT ( 'NONE',  ( -13.97604488694547697, 13.89961937509957934, 68.12609039468563310 ) ) ;
#99788=CARTESIAN_POINT ( 'NONE',  ( 5.719274019375991003, -21.55341960407610458, 87.70724293864769550 ) ) ;
#99789=CARTESIAN_POINT ( 'NONE',  ( -5.823673210054116645, -21.52544592524344225, 72.29057627198102409 ) ) ;
#99790=CARTESIAN_POINT ( 'NONE',  ( 16.55341960407611168, 4.379528057220329451, 48.95724293864770971 ) ) ;
#99791=CARTESIAN_POINT ( 'NONE',  ( -19.05341960407617563, 5.049401038297882671, 23.54275706135233648 ) ) ;
#99792=CARTESIAN_POINT ( 'NONE',  ( -12.06949235617739369, -12.14591786802326823, 64.37609039468568994 ) ) ;
#99793=CARTESIAN_POINT ( 'NONE',  ( -13.89961937509977652, 13.97604488694528158, 95.62390960531436690 ) ) ;
#99794=CARTESIAN_POINT ( 'NONE',  ( -5.049401038298153566, 19.05341960407611168, 40.20724293864768839 ) ) ;
#99795=CARTESIAN_POINT ( 'NONE',  ( 18.62759615963255655, 10.81492255796105972, 46.66775706135234714 ) ) ;
#99797=CARTESIAN_POINT ( 'NONE',  ( -21.55341960407619339, 5.719274019375674811, 48.54275706135234714 ) ) ;
#99798=CARTESIAN_POINT ( 'NONE',  ( 13.97604488694527802, 13.89961937509977652, 59.37390960531434558 ) ) ;
#99799=CARTESIAN_POINT ( 'NONE',  ( 5.719274019375673035, 21.55341960407619339, 37.29275706135235424 ) ) ;
#99800=CARTESIAN_POINT ( 'NONE',  ( -16.46253265017146816, -9.564922557961047289, 74.16775706135234714 ) ) ;
#99801=CARTESIAN_POINT ( 'NONE',  ( -13.97604488694547697, 13.89961937509957934, 68.12609039468563310 ) ) ;
#99802=CARTESIAN_POINT ( 'NONE',  ( 16.46253265017160672, -9.564922557960803928, 38.33224293864768839 ) ) ;
#99803=CARTESIAN_POINT ( 'NONE',  ( -14.34966873604972548, 8.224510206698743886, 93.33442372801901854 ) ) ;
#99804=CARTESIAN_POINT ( 'NONE',  ( 19.03943276465977164, -0.05219959533909143690, 48.74890960531435979 ) ) ;
#99806=CARTESIAN_POINT ( 'NONE',  ( 16.51473224551069308, 9.474510206698969483, 94.16557627198103830 ) ) ;
#99807=CARTESIAN_POINT ( 'NONE',  ( 5.153800228976335163, 19.02544592524342804, 39.79057627198100988 ) ) ;
#99808=CARTESIAN_POINT ( 'NONE',  ( 15.72974639402199770, -15.80617190586745480, 73.12390960531436690 ) ) ;
#99809=CARTESIAN_POINT ( 'NONE',  ( 4.379528057220092307, 16.55341960407617563, 67.29275706135234714 ) ) ;
#99810=CARTESIAN_POINT ( 'NONE',  ( 21.53943276465977519, 0.05219959533937863772, 111.2510903946856899 ) ) ;
#99811=CARTESIAN_POINT ( 'NONE',  ( -16.46253265017160317, 9.564922557960807481, 55.83224293864769550 ) ) ;
#99812=CARTESIAN_POINT ( 'NONE',  ( 0.05219959533910956823, 16.53943276465976808, 44.99890960531435979 ) ) ;
#99813=CARTESIAN_POINT ( 'NONE',  ( -8.224510206698948167, 14.34966873604960824, 80.41557627198103830 ) ) ;
#99815=CARTESIAN_POINT ( 'NONE',  ( -5.153800228976328057, -19.02544592524343514, 72.29057627198102409 ) ) ;
#99816=CARTESIAN_POINT ( 'NONE',  ( 15.72974639402176855, 15.80617190586768217, 31.87609039468567929 ) ) ;
#99817=CARTESIAN_POINT ( 'NONE',  ( 5.049401038298161559, -19.05341960407611168, 97.70724293864766707 ) ) ;
#99818=CARTESIAN_POINT ( 'NONE',  ( 21.53943276465977519, 0.05219959533937863772, 101.2510903946856757 ) ) ;
#99819=CARTESIAN_POINT ( 'NONE',  ( 0.05219959533934541429, -16.53943276465976808, 70.00109039468568994 ) ) ;
#99820=CARTESIAN_POINT ( 'NONE',  ( 15.80617190586769283, -15.72974639402175789, 25.62609039468567929 ) ) ;
#99821=CARTESIAN_POINT ( 'NONE',  ( -19.03943276465977164, 0.05219959533909376836, 106.2489096053143669 ) ) ;
#99822=CARTESIAN_POINT ( 'NONE',  ( -5.719274019375978568, 21.55341960407610458, 90.20724293864770971 ) ) ;
#99823=CARTESIAN_POINT ( 'NONE',  ( -16.52544592524342804, 4.483927247898546575, 41.04057627198103120 ) ) ;
#99824=CARTESIAN_POINT ( 'NONE',  ( -19.03943276465977164, 0.05219959533909376836, 41.24890960531435269 ) ) ;
#99825=CARTESIAN_POINT ( 'NONE',  ( 12.14591786802309770, 12.06949235617756955, 74.37390960531436690 ) ) ;
#99826=CARTESIAN_POINT ( 'NONE',  ( 10.81492255796078972, 18.62759615963270932, 24.58224293864768839 ) ) ;
#99827=CARTESIAN_POINT ( 'NONE',  ( -9.474510206698720793, -16.51473224551083518, 29.58442372801900433 ) ) ;
#99829=CARTESIAN_POINT ( 'NONE',  ( 16.55341960407611168, 4.379528057220329451, 103.9572429386476813 ) ) ;
#99830=CARTESIAN_POINT ( 'NONE',  ( -19.05341960407611168, -5.049401038298163336, 111.4572429386476671 ) ) ;
#99832=CARTESIAN_POINT ( 'NONE',  ( 8.314922557961029526, -14.29746914071037800, 55.41775706135234714 ) ) ;
#99833=CARTESIAN_POINT ( 'NONE',  ( -9.474510206698964154, 16.51473224551069663, 50.41557627198102409 ) ) ;
#99835=CARTESIAN_POINT ( 'NONE',  ( -4.379528057220086978, -16.55341960407618274, 99.79275706135234714 ) ) ;
#99836=CARTESIAN_POINT ( 'NONE',  ( -19.05341960407617563, 5.049401038297882671, 93.54275706135234714 ) ) ;
#99837=CARTESIAN_POINT ( 'NONE',  ( -5.719274019375665041, -21.55341960407619695, 69.79275706135234714 ) ) ;
#99838=CARTESIAN_POINT ( 'NONE',  ( -5.153800228976328057, -19.02544592524343514, 77.29057627198099567 ) ) ;
#99839=CARTESIAN_POINT ( 'NONE',  ( -10.81492255796078084, -18.62759615963271287, 87.08224293864769550 ) ) ;
#99840=CARTESIAN_POINT ( 'NONE',  ( 16.55341960407618274, -4.379528057220086978, 41.04275706135236135 ) ) ;
#99841=CARTESIAN_POINT ( 'NONE',  ( -5.153800228976328057, -19.02544592524343514, 22.29057627198102765 ) ) ;
#99842=CARTESIAN_POINT ( 'NONE',  ( 16.46253265017146816, 9.564922557961045513, 76.66775706135234714 ) ) ;
#99843=CARTESIAN_POINT ( 'NONE',  ( -21.52544592524343514, 5.823673210054127303, 76.04057627198102409 ) ) ;
#99844=CARTESIAN_POINT ( 'NONE',  ( 9.564922557961047289, -16.46253265017146816, 55.41775706135234003 ) ) ;
#99845=CARTESIAN_POINT ( 'NONE',  ( 19.35543954521081034, 5.499999999999523936, 97.08901960356452321 ) ) ;
#99846=CARTESIAN_POINT ( 'NONE',  ( 18.62759615963271287, -10.81492255796078972, 88.33224293864769550 ) ) ;
#99847=CARTESIAN_POINT ( 'NONE',  ( 17.50000000000014211, 3.292511757969722730, 27.43479729789468990 ) ) ;
#99848=CARTESIAN_POINT ( 'NONE',  ( -5.153800228976328057, -19.02544592524343514, 62.29057627198100988 ) ) ;
#99849=CARTESIAN_POINT ( 'NONE',  ( 17.50000000000000000, 5.499999999999992895, 56.70309617465829888 ) ) ;
#99850=CARTESIAN_POINT ( 'NONE',  ( -14.29746914071037622, -8.314922557961029526, 19.16775706135234714 ) ) ;
#99852=CARTESIAN_POINT ( 'NONE',  ( -19.05341960407611168, -5.049401038298163336, 41.45724293864769550 ) ) ;
#99853=CARTESIAN_POINT ( 'NONE',  ( -18.62759615963270932, 10.81492255796079327, 105.8322429386476955 ) ) ;
#99854=CARTESIAN_POINT ( 'NONE',  ( 16.55341960407611168, 4.379528057220329451, 48.95724293864770971 ) ) ;
#99855=CARTESIAN_POINT ( 'NONE',  ( -9.564922557960796823, -16.46253265017161027, 67.08224293864769550 ) ) ;
#99856=CARTESIAN_POINT ( 'NONE',  ( -10.72451020669870658, -18.67979575497194134, 74.58442372801901854 ) ) ;
#99857=CARTESIAN_POINT ( 'NONE',  ( -16.53943276465976808, -0.05219959533934237506, 18.75109039468568639 ) ) ;
#99858=CARTESIAN_POINT ( 'NONE',  ( -0.05219959533936034679, 19.03943276465977164, 32.50109039468566863 ) ) ;
#99859=CARTESIAN_POINT ( 'NONE',  ( -18.67979575497193778, 10.72451020669871902, 38.33442372801900433 ) ) ;
#99860=CARTESIAN_POINT ( 'NONE',  ( 10.72451020669871369, 18.67979575497193778, 22.08442372801901143 ) ) ;
#99861=CARTESIAN_POINT ( 'NONE',  ( -5.823673210054116645, -21.52544592524344225, 62.29057627198102409 ) ) ;
#99862=CARTESIAN_POINT ( 'NONE',  ( -0.05219959533936034679, 19.03943276465977164, 92.50109039468566152 ) ) ;
#99863=CARTESIAN_POINT ( 'NONE',  ( -13.97604488694547697, 13.89961937509957934, 63.12609039468566152 ) ) ;
#99864=CARTESIAN_POINT ( 'NONE',  ( 5.719274019375673035, 21.55341960407619339, 82.29275706135234714 ) ) ;
#99865=CARTESIAN_POINT ( 'NONE',  ( 5.049401038297881783, 19.05341960407617563, 52.29275706135234003 ) ) ;
#99866=CARTESIAN_POINT ( 'NONE',  ( -9.474510206698964154, 16.51473224551069663, 25.41557627198103120 ) ) ;
#99867=CARTESIAN_POINT ( 'NONE',  ( 21.53943276465977519, -0.05219959533907433946, 53.74890960531437401 ) ) ;
#99868=CARTESIAN_POINT ( 'NONE',  ( -16.53943276465976808, 0.05219959533911058130, 51.24890960531436690 ) ) ;
#99870=CARTESIAN_POINT ( 'NONE',  ( 13.89961937509957401, 13.97604488694547697, 31.87609039468566863 ) ) ;
#99871=CARTESIAN_POINT ( 'NONE',  ( -4.483927247898782831, 16.52544592524335698, 82.70942372801900433 ) ) ;
#99872=CARTESIAN_POINT ( 'NONE',  ( -14.34966873604960291, -8.224510206698953496, 46.66557627198102409 ) ) ;
#99873=CARTESIAN_POINT ( 'NONE',  ( -0.05219959533937732626, 21.53943276465977519, 77.50109039468567573 ) ) ;
#99874=CARTESIAN_POINT ( 'NONE',  ( 15.72974639402176855, 15.80617190586768217, 86.87609039468568994 ) ) ;
#99875=CARTESIAN_POINT ( 'NONE',  ( -21.52544592524343514, 5.823673210054127303, 86.04057627198102409 ) ) ;
#99876=CARTESIAN_POINT ( 'NONE',  ( 5.049401038298161559, -19.05341960407611168, 37.70724293864768839 ) ) ;
#99877=CARTESIAN_POINT ( 'NONE',  ( -15.72974639402176322, -15.80617190586768395, 59.37609039468568284 ) ) ;
#99878=CARTESIAN_POINT ( 'NONE',  ( -16.46253265017160317, 9.564922557960807481, 30.83224293864769550 ) ) ;
#99879=CARTESIAN_POINT ( 'NONE',  ( -5.153800228976328057, -19.02544592524343514, 57.29057627198103120 ) ) ;
#99880=CARTESIAN_POINT ( 'NONE',  ( 16.52544592524342804, -4.483927247898539470, 98.54057627198105251 ) ) ;
#99881=CARTESIAN_POINT ( 'NONE',  ( 9.564922557960805705, 16.46253265017160317, 99.58224293864770971 ) ) ;
#99882=CARTESIAN_POINT ( 'NONE',  ( -14.29746914071049879, 8.314922557960819915, 45.83224293864769550 ) ) ;
#99883=CARTESIAN_POINT ( 'NONE',  ( -8.314922557960811034, -14.29746914071050412, 107.0822429386476955 ) ) ;
#99884=CARTESIAN_POINT ( 'NONE',  ( 10.81492255796078972, 18.62759615963270932, 89.58224293864768129 ) ) ;
#99885=CARTESIAN_POINT ( 'NONE',  ( 18.67979575497194134, -10.72451020669871369, 25.83442372801901499 ) ) ;
#99887=CARTESIAN_POINT ( 'NONE',  ( 16.55341960407618274, -4.379528057220086978, 41.04275706135236135 ) ) ;
#99888=CARTESIAN_POINT ( 'NONE',  ( -15.80617190586745835, -15.72974639402198527, 71.87390960531438111 ) ) ;
#99889=CARTESIAN_POINT ( 'NONE',  ( -21.52544592524334988, -5.823673210054445271, 98.95942372801903275 ) ) ;
#99890=CARTESIAN_POINT ( 'NONE',  ( -16.46253265017160317, 9.564922557960807481, 90.83224293864769550 ) ) ;
#99891=CARTESIAN_POINT ( 'NONE',  ( 21.53943276465977519, 0.05219959533937863772, 26.25109039468567573 ) ) ;
#99892=CARTESIAN_POINT ( 'NONE',  ( -10.81492255796078084, -18.62759615963271287, 32.08224293864769550 ) ) ;
#99893=CARTESIAN_POINT ( 'NONE',  ( -4.483927247898782831, 16.52544592524335698, 92.70942372801901854 ) ) ;
#99894=CARTESIAN_POINT ( 'NONE',  ( 10.81492255796106328, -18.62759615963255655, 65.41775706135234714 ) ) ;
#99895=CARTESIAN_POINT ( 'NONE',  ( 19.05341960407617918, -5.049401038297876454, 21.04275706135232582 ) ) ;
#99896=CARTESIAN_POINT ( 'NONE',  ( 14.34966873604972726, -8.224510206698740333, 70.83442372801901854 ) ) ;
#99897=CARTESIAN_POINT ( 'NONE',  ( 5.719274019375673035, 21.55341960407619339, 27.29275706135234358 ) ) ;
#99898=CARTESIAN_POINT ( 'NONE',  ( 13.89961937509977652, -13.97604488694527269, 28.12390960531435624 ) ) ;
#99899=CARTESIAN_POINT ( 'NONE',  ( 21.55341960407619695, -5.719274019375665929, 106.0427570613523471 ) ) ;
#99900=CARTESIAN_POINT ( 'NONE',  ( -16.46253265017160317, 9.564922557960807481, 110.8322429386476955 ) ) ;
#99901=CARTESIAN_POINT ( 'NONE',  ( -5.823673210054116645, -21.52544592524344225, 97.29057627198105251 ) ) ;
#99903=CARTESIAN_POINT ( 'NONE',  ( -21.55341960407610458, -5.719274019375992779, 56.45724293864768839 ) ) ;
#99904=CARTESIAN_POINT ( 'NONE',  ( 8.314922557961029526, -14.29746914071037800, 50.41775706135235424 ) ) ;
#99905=CARTESIAN_POINT ( 'NONE',  ( -14.34966873604960291, -8.224510206698953496, 51.66557627198102409 ) ) ;
#99907=CARTESIAN_POINT ( 'NONE',  ( 19.02544592524334988, 5.153800228976608722, 81.45942372801897591 ) ) ;
#99908=CARTESIAN_POINT ( 'NONE',  ( -17.40861289039001392, 6.110651285853331949, 103.6276752917256943 ) ) ;
#99909=CARTESIAN_POINT ( 'NONE',  ( 16.51473224551083163, -9.474510206698727899, 105.8344237280190043 ) ) ;
#99910=CARTESIAN_POINT ( 'NONE',  ( -5.719274019375978568, 21.55341960407610458, 80.20724293864769550 ) ) ;
#99911=CARTESIAN_POINT ( 'NONE',  ( -0.05219959533910754901, -16.53943276465976808, 67.49890960531436690 ) ) ;
#99912=CARTESIAN_POINT ( 'NONE',  ( 9.474510206698971260, -16.51473224551069308, 97.91557627198102409 ) ) ;
#99913=CARTESIAN_POINT ( 'NONE',  ( 16.52544592524335698, 4.483927247898782831, 46.45942372801901854 ) ) ;
#99914=CARTESIAN_POINT ( 'NONE',  ( -16.51473224551069308, -9.474510206698971260, 61.66557627198103120 ) ) ;
#99915=CARTESIAN_POINT ( 'NONE',  ( 5.719274019375673035, 21.55341960407619339, 32.29275706135235424 ) ) ;
#99916=CARTESIAN_POINT ( 'NONE',  ( -9.474510206698720793, -16.51473224551083518, 104.5844237280190043 ) ) ;
#99917=CARTESIAN_POINT ( 'NONE',  ( -16.46253265017160317, 9.564922557960807481, 95.83224293864769550 ) ) ;
#99918=CARTESIAN_POINT ( 'NONE',  ( -19.05341960407611168, -5.049401038298163336, 86.45724293864769550 ) ) ;
#99919=CARTESIAN_POINT ( 'NONE',  ( -10.72451020669898014, 18.67979575497178502, 85.41557627198102409 ) ) ;
#99920=CARTESIAN_POINT ( 'NONE',  ( -19.02544592524342804, 5.153800228976336051, 41.04057627198103120 ) ) ;
#99921=CARTESIAN_POINT ( 'NONE',  ( -16.79531203550651242, -7.028104445595497296, 61.25244988220445919 ) ) ;
#99922=CARTESIAN_POINT ( 'NONE',  ( 4.483927247898545687, 16.52544592524342804, 64.79057627198103830 ) ) ;
#99923=CARTESIAN_POINT ( 'NONE',  ( 0.05219959533909260263, 19.03943276465977164, 109.9989096053143669 ) ) ;
#99925=CARTESIAN_POINT ( 'NONE',  ( 5.049401038297881783, 19.05341960407617563, 62.29275706135234003 ) ) ;
#99926=CARTESIAN_POINT ( 'NONE',  ( -18.62759615963270932, 10.81492255796079327, 85.83224293864768129 ) ) ;
#99927=CARTESIAN_POINT ( 'NONE',  ( 19.03943276465977164, 0.05219959533936151252, 56.25109039468566863 ) ) ;
#99928=CARTESIAN_POINT ( 'NONE',  ( 19.05341960407611168, 5.049401038298154454, 98.95724293864766707 ) ) ;
#99929=CARTESIAN_POINT ( 'NONE',  ( 19.53091890409951503, 5.500000000000028422, 67.56097431831419442 ) ) ;
#99930=CARTESIAN_POINT ( 'NONE',  ( -10.81492255796078084, -18.62759615963271287, 37.08224293864768129 ) ) ;
#99931=CARTESIAN_POINT ( 'NONE',  ( -13.89961937509977652, 13.97604488694528158, 90.62390960531432427 ) ) ;
#99932=CARTESIAN_POINT ( 'NONE',  ( -10.72451020669870658, -18.67979575497194134, 59.58442372801901854 ) ) ;
#99933=CARTESIAN_POINT ( 'NONE',  ( -5.153800228976328057, -19.02544592524343514, 32.29057627198102409 ) ) ;
#99934=CARTESIAN_POINT ( 'NONE',  ( -4.483927247898539470, -16.52544592524342804, 72.29057627198102409 ) ) ;
#99935=CARTESIAN_POINT ( 'NONE',  ( 14.29746914071037800, 8.314922557961029526, 21.66775706135235069 ) ) ;
#99936=CARTESIAN_POINT ( 'NONE',  ( 0.05219959533937995610, -21.53943276465977519, 50.00109039468568994 ) ) ;
#99938=FACE_OUTER_BOUND ( 'NONE', #90745, .T. ) ;
#99939=CARTESIAN_POINT ( 'NONE',  ( -0.05219959533936034679, 19.03943276465977164, 62.50109039468566863 ) ) ;
#99941=CARTESIAN_POINT ( 'NONE',  ( -0.05219959533937732626, 21.53943276465977519, 22.50109039468567573 ) ) ;
#99943=CARTESIAN_POINT ( 'NONE',  ( 19.03943276465977164, 0.05219959533936151252, 21.25109039468565797 ) ) ;
#99944=CARTESIAN_POINT ( 'NONE',  ( 13.89961937509977652, -13.97604488694527269, 58.12390960531436690 ) ) ;
#99945=CARTESIAN_POINT ( 'NONE',  ( -21.55341960407619339, 5.719274019375674811, 113.5427570613523756 ) ) ;
#99946=CARTESIAN_POINT ( 'NONE',  ( -16.52544592524335698, -4.483927247898792601, 108.9594237280190185 ) ) ;
#99947=CARTESIAN_POINT ( 'NONE',  ( 13.89961937509977652, -13.97604488694527269, 103.1239096053143527 ) ) ;
#99948=CARTESIAN_POINT ( 'NONE',  ( 21.53943276465977519, 0.05219959533937863772, 76.25109039468568994 ) ) ;
#99949=VECTOR ( 'NONE', #59797, 1000.000000000000000 ) ;
#99952=CARTESIAN_POINT ( 'NONE',  ( -14.29746914071037622, -8.314922557961029526, 69.16775706135234714 ) ) ;
#99953=CARTESIAN_POINT ( 'NONE',  ( -10.72451020669870658, -18.67979575497194134, 69.58442372801900433 ) ) ;
#99954=CARTESIAN_POINT ( 'NONE',  ( -21.53943276465977519, -0.05219959533937600094, 103.7510903946857042 ) ) ;
#99956=CARTESIAN_POINT ( 'NONE',  ( 19.05341960407611168, 5.049401038298154454, 83.95724293864766707 ) ) ;
#99958=FACE_OUTER_BOUND ( 'NONE', #7954, .T. ) ;
#99959=EDGE_LOOP ( 'NONE', ( #55692, #12331, #60000, #50511 ) ) ;
#99960=CARTESIAN_POINT ( 'NONE',  ( -22.00000000000000000, -5.510910596163089556E-15, 45.00000000000000000 ) ) ;
#99961=CARTESIAN_POINT ( 'NONE',  ( 19.02544592524343514, -5.153800228976328945, 33.54057627198102409 ) ) ;
#99962=CARTESIAN_POINT ( 'NONE',  ( 21.55341960407610458, 5.719274019375980345, 38.95724293864768839 ) ) ;
#99963=CARTESIAN_POINT ( 'NONE',  ( 16.52544592524335698, 4.483927247898782831, 106.4594237280190328 ) ) ;
#99964=CARTESIAN_POINT ( 'NONE',  ( -8.224510206698948167, 14.34966873604960824, 100.4155762719810241 ) ) ;
#99965=CARTESIAN_POINT ( 'NONE',  ( -13.89961937509977652, 13.97604488694528158, 80.62390960531436690 ) ) ;
#99966=CARTESIAN_POINT ( 'NONE',  ( 21.52544592524334988, 5.823673210054432836, 106.4594237280190328 ) ) ;
#99967=CARTESIAN_POINT ( 'NONE',  ( 5.153800228976335163, 19.02544592524342804, 39.79057627198100988 ) ) ;
#99968=CARTESIAN_POINT ( 'NONE',  ( -8.224510206698948167, 14.34966873604960824, 90.41557627198103830 ) ) ;
#99969=CARTESIAN_POINT ( 'NONE',  ( -21.55341960407619339, 5.719274019375674811, 53.54275706135234714 ) ) ;
#99970=CARTESIAN_POINT ( 'NONE',  ( 15.72974639402199770, -15.80617190586745480, 93.12390960531436690 ) ) ;
#99971=CARTESIAN_POINT ( 'NONE',  ( -5.153800228976607833, 19.02544592524334988, 52.70942372801900433 ) ) ;
#99973=CARTESIAN_POINT ( 'NONE',  ( -13.89961937509977652, 13.97604488694528158, 90.62390960531432427 ) ) ;
#99974=CARTESIAN_POINT ( 'NONE',  ( -12.14591786802309592, -12.06949235617757132, 61.87390960531436690 ) ) ;
#99975=CARTESIAN_POINT ( 'NONE',  ( -13.89961937509957401, -13.97604488694547875, 49.37609039468567573 ) ) ;
#99976=CARTESIAN_POINT ( 'NONE',  ( -0.05219959533910754901, -16.53943276465976808, 42.49890960531435979 ) ) ;
#99977=CARTESIAN_POINT ( 'NONE',  ( -13.97604488694547697, 13.89961937509957934, 83.12609039468564731 ) ) ;
#99978=CARTESIAN_POINT ( 'NONE',  ( -13.89961937509957401, -13.97604488694547697, 89.37609039468564731 ) ) ;
#99979=CARTESIAN_POINT ( 'NONE',  ( -18.62759615963270932, 10.81492255796079327, 35.83224293864768839 ) ) ;
#99980=CARTESIAN_POINT ( 'NONE',  ( 4.379528057220339221, -16.55341960407611168, 107.7072429386476955 ) ) ;
#99981=CARTESIAN_POINT ( 'NONE',  ( -17.50000000000001421, -5.499999999999956479, 26.28230962303566542 ) ) ;
#99982=CARTESIAN_POINT ( 'NONE',  ( -16.51473224551069308, -9.474510206698971260, 51.66557627198102409 ) ) ;
#99983=CARTESIAN_POINT ( 'NONE',  ( 15.80617190586746368, 15.72974639402197994, 49.37390960531436690 ) ) ;
#99984=CARTESIAN_POINT ( 'NONE',  ( 19.05341960407611168, 5.049401038298154454, 28.95724293864769550 ) ) ;
#99985=CARTESIAN_POINT ( 'NONE',  ( -14.29746914071037622, -8.314922557961029526, 74.16775706135231871 ) ) ;
#99986=CARTESIAN_POINT ( 'NONE',  ( 0.05219959533909260263, 19.03943276465977164, 64.99890960531436690 ) ) ;
#99987=CARTESIAN_POINT ( 'NONE',  ( 19.03943276465977164, 0.05219959533936151252, 36.25109039468567573 ) ) ;
#99988=CARTESIAN_POINT ( 'NONE',  ( -15.72974639402176322, -15.80617190586768395, 64.37609039468568994 ) ) ;
#99989=CARTESIAN_POINT ( 'NONE',  ( -21.55341960407610458, -5.719274019375992779, 51.45724293864770260 ) ) ;
#99990=CARTESIAN_POINT ( 'NONE',  ( 5.049401038298161559, -19.05341960407611168, 22.70724293864769194 ) ) ;
#99991=CARTESIAN_POINT ( 'NONE',  ( -13.97604488694547697, 13.89961937509957934, 98.12609039468566152 ) ) ;
#99993=CARTESIAN_POINT ( 'NONE',  ( 17.49999999999999289, 3.270424329314900014, 37.45773515054982283 ) ) ;
#99994=CARTESIAN_POINT ( 'NONE',  ( -5.823673210054116645, -21.52544592524344225, 47.29057627198103120 ) ) ;
#99995=CARTESIAN_POINT ( 'NONE',  ( 19.03943276465977164, -0.05219959533909143690, 28.74890960531435624 ) ) ;
#99996=CARTESIAN_POINT ( 'NONE',  ( -15.72974639402176322, -15.80617190586768395, 84.37609039468570415 ) ) ;
#99997=CARTESIAN_POINT ( 'NONE',  ( -16.53943276465976808, 0.05219959533911058130, 46.24890960531435979 ) ) ;
#99998=CARTESIAN_POINT ( 'NONE',  ( -4.483927247898539470, -16.52544592524342804, 62.29057627198102409 ) ) ;
#99999=CARTESIAN_POINT ( 'NONE',  ( -5.719274019375978568, 21.55341960407610458, 85.20724293864770971 ) ) ;
#100000=CARTESIAN_POINT ( 'NONE',  ( -15.80617190586745835, -15.72974639402198527, 81.87390960531435269 ) ) ;
#100002=CARTESIAN_POINT ( 'NONE',  ( 21.53943276465977519, -0.05219959533907433946, 33.74890960531436690 ) ) ;
#100003=CARTESIAN_POINT ( 'NONE',  ( 16.55341960407618274, -4.379528057220086978, 51.04275706135234714 ) ) ;
#100004=CARTESIAN_POINT ( 'NONE',  ( -16.52544592524342804, 4.483927247898546575, 81.04057627198102409 ) ) ;
#100005=CARTESIAN_POINT ( 'NONE',  ( -9.564922557960796823, -16.46253265017161027, 57.08224293864769550 ) ) ;
#100006=CARTESIAN_POINT ( 'NONE',  ( 13.89961937509977652, -13.97604488694527269, 38.12390960531436690 ) ) ;
#100009=CARTESIAN_POINT ( 'NONE',  ( -0.05219959533934338120, 16.53943276465976808, 77.50109039468567573 ) ) ;
#100010=CARTESIAN_POINT ( 'NONE',  ( 21.55341960407619695, -5.719274019375665929, 26.04275706135235779 ) ) ;
#100011=CARTESIAN_POINT ( 'NONE',  ( -9.474510206698964154, 16.51473224551069663, 75.41557627198103830 ) ) ;
#100012=CARTESIAN_POINT ( 'NONE',  ( 21.55341960407619695, -5.719274019375665929, 61.04275706135234714 ) ) ;
#100013=CARTESIAN_POINT ( 'NONE',  ( 0.05219959533909260263, 19.03943276465977164, 114.9989096053143669 ) ) ;
#100016=CARTESIAN_POINT ( 'NONE',  ( -18.62759615963255300, -10.81492255796106328, 39.16775706135235424 ) ) ;
#100017=CARTESIAN_POINT ( 'NONE',  ( 9.564922557960805705, 16.46253265017160317, 24.58224293864769194 ) ) ;
#100018=CARTESIAN_POINT ( 'NONE',  ( 0.05219959533909260263, 19.03943276465977164, 99.99890960531436690 ) ) ;
#100019=CARTESIAN_POINT ( 'NONE',  ( -13.97604488694547697, 13.89961937509957934, 48.12609039468566863 ) ) ;
#100020=CARTESIAN_POINT ( 'NONE',  ( 21.55341960407619695, -5.719274019375665929, 21.04275706135234714 ) ) ;
#100021=CARTESIAN_POINT ( 'NONE',  ( -5.153800228976607833, 19.02544592524334988, 47.70942372801900433 ) ) ;
#100022=CARTESIAN_POINT ( 'NONE',  ( 19.03943276465977164, -0.05219959533909143690, 28.74890960531435624 ) ) ;
#100023=CARTESIAN_POINT ( 'NONE',  ( 8.314922557961029526, -14.29746914071037800, 95.41775706135234714 ) ) ;
#100024=CARTESIAN_POINT ( 'NONE',  ( 19.03943276465977164, 0.05219959533936151252, 56.25109039468566863 ) ) ;
#100025=CARTESIAN_POINT ( 'NONE',  ( -16.53943276465976808, -0.05219959533934237506, 98.75109039468568994 ) ) ;
#100028=CARTESIAN_POINT ( 'NONE',  ( 5.153800228976335163, 19.02544592524342804, 84.79057627198099567 ) ) ;
#100029=CARTESIAN_POINT ( 'NONE',  ( -15.72974639402176322, -15.80617190586768395, 89.37609039468568994 ) ) ;
#100030=CARTESIAN_POINT ( 'NONE',  ( -10.81492255796105439, 18.62759615963255655, 92.91775706135236135 ) ) ;
#100032=CARTESIAN_POINT ( 'NONE',  ( -16.51473224551069308, -9.474510206698971260, 21.66557627198102765 ) ) ;
#100033=CARTESIAN_POINT ( 'NONE',  ( -0.05219959533909027116, -19.03943276465977164, 102.4989096053143669 ) ) ;
#100034=CARTESIAN_POINT ( 'NONE',  ( 15.80617190586769283, -15.72974639402175789, 75.62609039468567573 ) ) ;
#100035=CARTESIAN_POINT ( 'NONE',  ( -9.474510206698720793, -16.51473224551083518, 109.5844237280190043 ) ) ;
#100036=CARTESIAN_POINT ( 'NONE',  ( 19.03943276465977164, -0.05219959533909143690, 83.74890960531436690 ) ) ;
#100037=CARTESIAN_POINT ( 'NONE',  ( 10.81492255796078972, 18.62759615963270932, 34.58224293864770260 ) ) ;
#100038=CARTESIAN_POINT ( 'NONE',  ( -19.05341960407611168, -5.049401038298163336, 96.45724293864769550 ) ) ;
#100039=CARTESIAN_POINT ( 'NONE',  ( -16.18388926212238488, -7.379444403734532365, 90.43953151366152099 ) ) ;
#100040=CARTESIAN_POINT ( 'NONE',  ( -19.05341960407611168, -5.049401038298163336, 81.45724293864769550 ) ) ;
#100041=CARTESIAN_POINT ( 'NONE',  ( 5.049401038298161559, -19.05341960407611168, 67.70724293864769550 ) ) ;
#100042=CARTESIAN_POINT ( 'NONE',  ( 8.314922557961029526, -14.29746914071037800, 100.4177570613523471 ) ) ;
#100044=CARTESIAN_POINT ( 'NONE',  ( 5.153800228976615827, -19.02544592524334988, 55.20942372801899722 ) ) ;
#100045=CARTESIAN_POINT ( 'NONE',  ( 19.03943276465977164, -0.05219959533909143690, 98.74890960531436690 ) ) ;
#100046=CARTESIAN_POINT ( 'NONE',  ( -16.52544592524342804, 4.483927247898546575, 86.04057627198102409 ) ) ;
#100047=CARTESIAN_POINT ( 'NONE',  ( -10.72451020669898014, 18.67979575497178502, 35.41557627198102409 ) ) ;
#100048=CARTESIAN_POINT ( 'NONE',  ( -15.80617190586745835, -15.72974639402198527, 26.87390960531435979 ) ) ;
#100049=CARTESIAN_POINT ( 'NONE',  ( -14.29746914071049879, 8.314922557960819915, 85.83224293864768129 ) ) ;
#100050=CARTESIAN_POINT ( 'NONE',  ( -17.05587630539785948, 6.762274262135695047, 55.74180309037311787 ) ) ;
#100051=CARTESIAN_POINT ( 'NONE',  ( 19.05341960407617918, -5.049401038297876454, 46.04275706135233293 ) ) ;
#100052=CARTESIAN_POINT ( 'NONE',  ( 4.379528057220092307, 16.55341960407617563, 112.2927570613523471 ) ) ;
#100053=CARTESIAN_POINT ( 'NONE',  ( 13.97604488694527802, 13.89961937509977652, 104.3739096053143385 ) ) ;
#100054=CARTESIAN_POINT ( 'NONE',  ( 0.05219959533937995610, -21.53943276465977519, 65.00109039468568994 ) ) ;
#100055=CARTESIAN_POINT ( 'NONE',  ( -15.80617190586745835, -15.72974639402198527, 51.87390960531437401 ) ) ;
#100056=CARTESIAN_POINT ( 'NONE',  ( 18.67979575497194134, -10.72451020669871369, 30.83442372801902209 ) ) ;
#100057=ORIENTED_EDGE ( 'NONE', *, *, #124931, .T. ) ;
#100058=CARTESIAN_POINT ( 'NONE',  ( -21.52544592524343514, 5.823673210054127303, 81.04057627198102409 ) ) ;
#100059=CARTESIAN_POINT ( 'NONE',  ( -18.67979575497193778, 10.72451020669871902, 38.33442372801900433 ) ) ;
#100060=CARTESIAN_POINT ( 'NONE',  ( -16.55341960407611168, -4.379528057220339221, 111.4572429386476813 ) ) ;
#100061=CARTESIAN_POINT ( 'NONE',  ( 16.46253265017146816, 9.564922557961045513, 76.66775706135234714 ) ) ;
#100062=CARTESIAN_POINT ( 'NONE',  ( 16.46253265017160672, -9.564922557960803928, 38.33224293864768839 ) ) ;
#100063=CARTESIAN_POINT ( 'NONE',  ( -0.05219959533910754901, -16.53943276465976808, 97.49890960531436690 ) ) ;
#100064=CARTESIAN_POINT ( 'NONE',  ( 19.05341960407611168, 5.049401038298154454, 98.95724293864766707 ) ) ;
#100065=CARTESIAN_POINT ( 'NONE',  ( 5.153800228976335163, 19.02544592524342804, 89.79057627198102409 ) ) ;
#100066=CARTESIAN_POINT ( 'NONE',  ( 19.03943276465977164, -0.05219959533909143690, 23.74890960531435269 ) ) ;
#100067=CARTESIAN_POINT ( 'NONE',  ( 0.05219959533910956823, 16.53943276465976808, 34.99890960531435979 ) ) ;
#100068=CARTESIAN_POINT ( 'NONE',  ( 16.55341960407618274, -4.379528057220086978, 101.0427570613523756 ) ) ;
#100069=CARTESIAN_POINT ( 'NONE',  ( 16.46253265017160672, -9.564922557960803928, 53.33224293864768839 ) ) ;
#100070=CARTESIAN_POINT ( 'NONE',  ( -16.46253265017160317, 9.564922557960807481, 25.83224293864769194 ) ) ;
#100071=CARTESIAN_POINT ( 'NONE',  ( -9.474510206698720793, -16.51473224551083518, 24.58442372801900078 ) ) ;
#100072=DIRECTION ( 'NONE',  ( 1.000000000000000000, 0.000000000000000000, 0.000000000000000000 ) ) ;
#100073=CARTESIAN_POINT ( 'NONE',  ( -14.34966873604972548, 8.224510206698743886, 113.3344237280190328 ) ) ;
#100074=CARTESIAN_POINT ( 'NONE',  ( -10.81492255796105439, 18.62759615963255655, 47.91775706135234714 ) ) ;
#100075=CARTESIAN_POINT ( 'NONE',  ( 13.97604488694527802, 13.89961937509977652, 99.37390960531436690 ) ) ;
#100076=CARTESIAN_POINT ( 'NONE',  ( -14.34966873604972548, 8.224510206698743886, 43.33442372801901143 ) ) ;
#100077=CARTESIAN_POINT ( 'NONE',  ( 12.14591786802327356, -12.06949235617739191, 105.6260903946856899 ) ) ;
#100078=CARTESIAN_POINT ( 'NONE',  ( 14.29746914071037800, 8.314922557961029526, 91.66775706135234714 ) ) ;
#100079=CARTESIAN_POINT ( 'NONE',  ( -4.379528057220086978, -16.55341960407618274, 19.79275706135235069 ) ) ;
#100080=CARTESIAN_POINT ( 'NONE',  ( 0.05219959533909260263, 19.03943276465977164, 49.99890960531435979 ) ) ;
#100081=CARTESIAN_POINT ( 'NONE',  ( -8.314922557960811034, -14.29746914071050412, 102.0822429386476955 ) ) ;
#100082=CARTESIAN_POINT ( 'NONE',  ( -5.719274019375665041, -21.55341960407619695, 19.79275706135235069 ) ) ;
#100083=CARTESIAN_POINT ( 'NONE',  ( -19.02544592524342804, 5.153800228976336051, 31.04057627198102409 ) ) ;
#100084=CARTESIAN_POINT ( 'NONE',  ( -9.564922557960796823, -16.46253265017161027, 102.0822429386477097 ) ) ;
#100085=CARTESIAN_POINT ( 'NONE',  ( 19.02544592524343514, -5.153800228976328945, 33.54057627198102409 ) ) ;
#100086=CARTESIAN_POINT ( 'NONE',  ( -19.05341960407611168, -5.049401038298163336, 106.4572429386476955 ) ) ;
#100088=AXIS2_PLACEMENT_3D ( 'NONE', #52188, #9703, #176556 ) ;
#100089=CARTESIAN_POINT ( 'NONE',  ( -13.97604488694527625, -13.89961937509977652, 91.87390960531432427 ) ) ;
#100090=CARTESIAN_POINT ( 'NONE',  ( 0.05219959533937995610, -21.53943276465977519, 45.00109039468568284 ) ) ;
#100091=CARTESIAN_POINT ( 'NONE',  ( -14.29746914071049879, 8.314922557960819915, 105.8322429386476955 ) ) ;
#100092=CARTESIAN_POINT ( 'NONE',  ( -5.153800228976328057, -19.02544592524343514, 112.2905762719810099 ) ) ;
#100094=CARTESIAN_POINT ( 'NONE',  ( 16.53943276465976808, 0.05219959533934440121, 61.25109039468567573 ) ) ;
#100095=CARTESIAN_POINT ( 'NONE',  ( -10.81492255796105439, 18.62759615963255655, 92.91775706135236135 ) ) ;
#100096=CARTESIAN_POINT ( 'NONE',  ( 8.224510206698742110, 14.34966873604972548, 42.08442372801901854 ) ) ;
#100097=CARTESIAN_POINT ( 'NONE',  ( -13.97604488694527625, -13.89961937509977652, 81.87390960531436690 ) ) ;
#100098=CARTESIAN_POINT ( 'NONE',  ( -19.05341960407617563, 5.049401038297882671, 113.5427570613523471 ) ) ;
#100099=CARTESIAN_POINT ( 'NONE',  ( 12.14591786802327356, -12.06949235617739191, 80.62609039468567573 ) ) ;
#100100=CARTESIAN_POINT ( 'NONE',  ( -5.153800228976607833, 19.02544592524334988, 87.70942372801897591 ) ) ;
#100101=CARTESIAN_POINT ( 'NONE',  ( 13.89961937509977652, -13.97604488694527269, 83.12390960531436690 ) ) ;
#100102=CARTESIAN_POINT ( 'NONE',  ( 5.823673210054125526, 21.52544592524343514, 99.79057627198103830 ) ) ;
#100103=CARTESIAN_POINT ( 'NONE',  ( -14.29746914071049879, 8.314922557960819915, 90.83224293864769550 ) ) ;
#100104=CARTESIAN_POINT ( 'NONE',  ( 5.153800228976615827, -19.02544592524334988, 85.20942372801900433 ) ) ;
#100105=CARTESIAN_POINT ( 'NONE',  ( -12.06949235617739369, -12.14591786802326823, 64.37609039468568994 ) ) ;
#100107=CARTESIAN_POINT ( 'NONE',  ( -9.474510206698720793, -16.51473224551083518, 69.58442372801901854 ) ) ;
#100108=CARTESIAN_POINT ( 'NONE',  ( 4.379528057220339221, -16.55341960407611168, 27.70724293864769905 ) ) ;
#100109=CARTESIAN_POINT ( 'NONE',  ( 4.379528057220339221, -16.55341960407611168, 92.70724293864770971 ) ) ;
#100110=CARTESIAN_POINT ( 'NONE',  ( 0.05219959533936267826, -19.03943276465977164, 25.00109039468566152 ) ) ;
#100111=CARTESIAN_POINT ( 'NONE',  ( 9.564922557961047289, -16.46253265017146816, 45.41775706135232582 ) ) ;
#100112=CARTESIAN_POINT ( 'NONE',  ( -15.72974639402176322, -15.80617190586768395, 24.37609039468567573 ) ) ;
#100114=CARTESIAN_POINT ( 'NONE',  ( -13.89961937509977652, 13.97604488694528158, 115.6239096053143669 ) ) ;
#100115=CARTESIAN_POINT ( 'NONE',  ( -16.51473224551069308, -9.474510206698971260, 71.66557627198102409 ) ) ;
#100116=CARTESIAN_POINT ( 'NONE',  ( -5.719274019375665041, -21.55341960407619695, 94.79275706135234714 ) ) ;
#100117=CARTESIAN_POINT ( 'NONE',  ( -5.049401038298153566, 19.05341960407611168, 70.20724293864769550 ) ) ;
#100118=CARTESIAN_POINT ( 'NONE',  ( -21.52544592524343514, 5.823673210054127303, 41.04057627198103120 ) ) ;
#100119=CARTESIAN_POINT ( 'NONE',  ( -16.53943276465976808, 0.05219959533911058130, 81.24890960531436690 ) ) ;
#100120=CARTESIAN_POINT ( 'NONE',  ( -16.46253265017160317, 9.564922557960807481, 50.83224293864770260 ) ) ;
#100121=CARTESIAN_POINT ( 'NONE',  ( -16.53943276465976808, 0.05219959533911058130, 116.2489096053143669 ) ) ;
#100122=CARTESIAN_POINT ( 'NONE',  ( 10.81492255796106328, -18.62759615963255655, 30.41775706135234358 ) ) ;
#100124=CARTESIAN_POINT ( 'NONE',  ( -0.05219959533937732626, 21.53943276465977519, 57.50109039468568994 ) ) ;
#100125=CARTESIAN_POINT ( 'NONE',  ( -16.46253265017160317, 9.564922557960807481, 45.83224293864769550 ) ) ;
#100126=CARTESIAN_POINT ( 'NONE',  ( -4.483927247898782831, 16.52544592524335698, 77.70942372801900433 ) ) ;
#100127=CARTESIAN_POINT ( 'NONE',  ( 15.80617190586769283, -15.72974639402175789, 20.62609039468568639 ) ) ;
#100128=EDGE_LOOP ( 'NONE', ( #22589, #23138, #173416, #144002 ) ) ;
#100129=CARTESIAN_POINT ( 'NONE',  ( 0.05219959533907565091, 21.53943276465977519, 104.9989096053143669 ) ) ;
#100130=CARTESIAN_POINT ( 'NONE',  ( -13.97604488694547697, 13.89961937509957934, 38.12609039468566152 ) ) ;
#100131=CARTESIAN_POINT ( 'NONE',  ( 19.05341960407611168, 5.049401038298154454, 68.95724293864769550 ) ) ;
#100132=CARTESIAN_POINT ( 'NONE',  ( -16.46253265017146816, -9.564922557961047289, 34.16775706135233293 ) ) ;
#100133=CARTESIAN_POINT ( 'NONE',  ( -18.67979575497193778, 10.72451020669871902, 73.33442372801901854 ) ) ;
#100134=CARTESIAN_POINT ( 'NONE',  ( 15.80617190586746368, 15.72974639402197994, 64.37390960531435269 ) ) ;
#100135=CARTESIAN_POINT ( 'NONE',  ( 16.52544592524342804, -4.483927247898539470, 38.54057627198103120 ) ) ;
#100136=CARTESIAN_POINT ( 'NONE',  ( 18.67979575497194134, -10.72451020669871369, 95.83442372801903275 ) ) ;
#100137=CARTESIAN_POINT ( 'NONE',  ( -13.97604488694547697, 13.89961937509957934, 33.12609039468566863 ) ) ;
#100138=CARTESIAN_POINT ( 'NONE',  ( -16.55341960407611168, -4.379528057220339221, 61.45724293864770260 ) ) ;
#100139=CARTESIAN_POINT ( 'NONE',  ( 8.224510206698953496, -14.34966873604960469, 107.9155762719810241 ) ) ;
#100140=CARTESIAN_POINT ( 'NONE',  ( -16.46253265017146816, -9.564922557961047289, 59.16775706135233293 ) ) ;
#100141=CARTESIAN_POINT ( 'NONE',  ( -8.224510206698948167, 14.34966873604960824, 25.41557627198103120 ) ) ;
#100142=CARTESIAN_POINT ( 'NONE',  ( -10.72451020669870658, -18.67979575497194134, 64.58442372801900433 ) ) ;
#100143=CARTESIAN_POINT ( 'NONE',  ( -19.03943276465977164, 0.05219959533909376836, 76.24890960531435269 ) ) ;
#100144=CARTESIAN_POINT ( 'NONE',  ( 19.02544592524334988, 5.153800228976608722, 46.45942372801899012 ) ) ;
#100145=CARTESIAN_POINT ( 'NONE',  ( -15.72974639402197994, 15.80617190586746368, 50.62390960531435979 ) ) ;
#100146=CARTESIAN_POINT ( 'NONE',  ( -5.823673210054431948, 21.52544592524334988, 47.70942372801902565 ) ) ;
#100147=CARTESIAN_POINT ( 'NONE',  ( 10.72451020669898902, -18.67979575497178502, 107.9155762719810241 ) ) ;
#100148=CARTESIAN_POINT ( 'NONE',  ( 0.05219959533936267826, -19.03943276465977164, 100.0010903946856757 ) ) ;
#100149=CARTESIAN_POINT ( 'NONE',  ( 16.55341960407618274, -4.379528057220086978, 71.04275706135234714 ) ) ;
#100151=CARTESIAN_POINT ( 'NONE',  ( 15.80617190586746368, 15.72974639402197994, 104.3739096053143669 ) ) ;
#100152=CARTESIAN_POINT ( 'NONE',  ( 12.14591786802309770, 12.06949235617756955, 94.37390960531436690 ) ) ;
#100153=CARTESIAN_POINT ( 'NONE',  ( -16.18388926212238843, -7.379444403734542135, 100.4395315136615494 ) ) ;
#100154=CARTESIAN_POINT ( 'NONE',  ( -16.52544592524335698, -4.483927247898792601, 28.95942372801902209 ) ) ;
#100155=CARTESIAN_POINT ( 'NONE',  ( -5.823673210054116645, -21.52544592524344225, 42.29057627198103120 ) ) ;
#100156=CARTESIAN_POINT ( 'NONE',  ( 14.29746914071037800, 8.314922557961029526, 91.66775706135234714 ) ) ;
#100157=CARTESIAN_POINT ( 'NONE',  ( 5.049401038298161559, -19.05341960407611168, 22.70724293864769194 ) ) ;
#100158=CARTESIAN_POINT ( 'NONE',  ( 8.224510206698742110, 14.34966873604972548, 62.08442372801901143 ) ) ;
#100159=CARTESIAN_POINT ( 'NONE',  ( -21.52544592524334988, -5.823673210054445271, 33.95942372801901143 ) ) ;
#100160=CARTESIAN_POINT ( 'NONE',  ( 0.05219959533907565091, 21.53943276465977519, 39.99890960531436690 ) ) ;
#100161=CARTESIAN_POINT ( 'NONE',  ( -14.34966873604972548, 8.224510206698743886, 83.33442372801903275 ) ) ;
#100162=CARTESIAN_POINT ( 'NONE',  ( -16.51473224551069308, -9.474510206698971260, 91.66557627198103830 ) ) ;
#100163=CARTESIAN_POINT ( 'NONE',  ( -15.80617190586768217, 15.72974639402176855, 73.12609039468567573 ) ) ;
#100164=CARTESIAN_POINT ( 'NONE',  ( 10.81492255796078972, 18.62759615963270932, 34.58224293864770260 ) ) ;
#100165=CARTESIAN_POINT ( 'NONE',  ( 15.72974639402199770, -15.80617190586745480, 33.12390960531435979 ) ) ;
#100166=ORIENTED_EDGE ( 'NONE', *, *, #143807, .F. ) ;
#100167=CARTESIAN_POINT ( 'NONE',  ( 9.474510206698729675, 16.51473224551082808, 47.08442372801900433 ) ) ;
#100168=CARTESIAN_POINT ( 'NONE',  ( 16.52544592524335698, 4.483927247898782831, 66.45942372801903275 ) ) ;
#100169=CARTESIAN_POINT ( 'NONE',  ( -21.53943276465977519, 0.05219959533907696930, 31.24890960531435979 ) ) ;
#100171=CARTESIAN_POINT ( 'NONE',  ( 19.03943276465977164, -0.05219959533909143690, 88.74890960531436690 ) ) ;
#100172=CARTESIAN_POINT ( 'NONE',  ( -8.314922557960811034, -14.29746914071050412, 27.08224293864769550 ) ) ;
#100173=CARTESIAN_POINT ( 'NONE',  ( -18.22780087662121673, -5.500000000000063061, 56.48459894673892734 ) ) ;
#100174=CARTESIAN_POINT ( 'NONE',  ( 14.34966873604960469, 8.224510206698951720, 114.1655762719810383 ) ) ;
#100175=CARTESIAN_POINT ( 'NONE',  ( -5.823673210054116645, -21.52544592524344225, 47.29057627198103120 ) ) ;
#100176=CARTESIAN_POINT ( 'NONE',  ( 9.564922557960805705, 16.46253265017160317, 49.58224293864770260 ) ) ;
#100177=CARTESIAN_POINT ( 'NONE',  ( -14.29746914071037622, -8.314922557961029526, 79.16775706135234714 ) ) ;
#100178=CARTESIAN_POINT ( 'NONE',  ( -18.62759615963255300, -10.81492255796106328, 39.16775706135235424 ) ) ;
#100179=CARTESIAN_POINT ( 'NONE',  ( -13.89961937509957401, -13.97604488694547875, 84.37609039468567573 ) ) ;
#100180=CARTESIAN_POINT ( 'NONE',  ( 8.314922557960818139, 14.29746914071049879, 84.58224293864769550 ) ) ;
#100181=CARTESIAN_POINT ( 'NONE',  ( 16.46253265017160672, -9.564922557960803928, 58.33224293864769550 ) ) ;
#100182=CARTESIAN_POINT ( 'NONE',  ( -16.51473224551069308, -9.474510206698971260, 31.66557627198102054 ) ) ;
#100183=CARTESIAN_POINT ( 'NONE',  ( 10.81492255796106328, -18.62759615963255655, 100.4177570613523471 ) ) ;
#100184=CARTESIAN_POINT ( 'NONE',  ( -19.02544592524342804, 5.153800228976336051, 76.04057627198102409 ) ) ;
#100185=CARTESIAN_POINT ( 'NONE',  ( 8.314922557961029526, -14.29746914071037800, 65.41775706135234714 ) ) ;
#100186=CARTESIAN_POINT ( 'NONE',  ( -15.72974639402176322, -15.80617190586768395, 99.37609039468568994 ) ) ;
#100187=CARTESIAN_POINT ( 'NONE',  ( 18.67979575497178502, 10.72451020669898547, 54.16557627198103120 ) ) ;
#100188=CARTESIAN_POINT ( 'NONE',  ( -16.53943276465976808, -0.05219959533934237506, 68.75109039468568994 ) ) ;
#100189=CARTESIAN_POINT ( 'NONE',  ( 5.153800228976615827, -19.02544592524334988, 50.20942372801897591 ) ) ;
#100190=CARTESIAN_POINT ( 'NONE',  ( 9.564922557961047289, -16.46253265017146816, 70.41775706135233293 ) ) ;
#100192=CARTESIAN_POINT ( 'NONE',  ( 15.72974639402176855, 15.80617190586768217, 56.87609039468568994 ) ) ;
#100193=CARTESIAN_POINT ( 'NONE',  ( -16.51473224551069308, -9.474510206698971260, 61.66557627198103120 ) ) ;
#100194=CARTESIAN_POINT ( 'NONE',  ( -16.46253265017160317, 9.564922557960807481, 35.83224293864768839 ) ) ;
#100195=CARTESIAN_POINT ( 'NONE',  ( 0.05219959533936267826, -19.03943276465977164, 60.00109039468566863 ) ) ;
#100196=CARTESIAN_POINT ( 'NONE',  ( -0.05219959533909027116, -19.03943276465977164, 107.4989096053143527 ) ) ;
#100197=CARTESIAN_POINT ( 'NONE',  ( -16.46253265017160317, 9.564922557960807481, 95.83224293864769550 ) ) ;
#100198=CARTESIAN_POINT ( 'NONE',  ( -14.29746914071049879, 8.314922557960819915, 55.83224293864770260 ) ) ;
#100199=CARTESIAN_POINT ( 'NONE',  ( 21.52544592524344225, -5.823673210054117533, 48.54057627198103120 ) ) ;
#100201=CARTESIAN_POINT ( 'NONE',  ( 10.81492255796106328, -18.62759615963255655, 110.4177570613523756 ) ) ;
#100202=CARTESIAN_POINT ( 'NONE',  ( -16.52216118717208104, -7.221426719304496089, 81.07599021046993926 ) ) ;
#100203=CARTESIAN_POINT ( 'NONE',  ( -19.05341960407611168, -5.049401038298163336, 46.45724293864768129 ) ) ;
#100206=CARTESIAN_POINT ( 'NONE',  ( -17.05116617787824396, 6.768360034955808402, 108.6567555325920296 ) ) ;
#100207=CARTESIAN_POINT ( 'NONE',  ( 4.379528057220092307, 16.55341960407617563, 67.29275706135234714 ) ) ;
#100208=CARTESIAN_POINT ( 'NONE',  ( -15.80617190586745835, -15.72974639402198527, 91.87390960531436690 ) ) ;
#100209=CARTESIAN_POINT ( 'NONE',  ( -8.314922557960811034, -14.29746914071050412, 47.08224293864770260 ) ) ;
#100210=CARTESIAN_POINT ( 'NONE',  ( 19.02544592524343514, -5.153800228976328945, 43.54057627198103120 ) ) ;
#100212=CARTESIAN_POINT ( 'NONE',  ( 18.67979575497194134, -10.72451020669871369, 35.83442372801901143 ) ) ;
#100213=CARTESIAN_POINT ( 'NONE',  ( 19.03943276465977164, 0.05219959533936151252, 51.25109039468567573 ) ) ;
#100214=CARTESIAN_POINT ( 'NONE',  ( -19.05341960407611168, -5.049401038298163336, 36.45724293864766707 ) ) ;
#100215=CARTESIAN_POINT ( 'NONE',  ( 21.52544592524334988, 5.823673210054432836, 101.4594237280190185 ) ) ;
#100217=CARTESIAN_POINT ( 'NONE',  ( -14.34966873604960291, -8.224510206698953496, 41.66557627198103120 ) ) ;
#100219=CARTESIAN_POINT ( 'NONE',  ( -21.55341960407610458, -5.719274019375992779, 36.45724293864768839 ) ) ;
#100221=CARTESIAN_POINT ( 'NONE',  ( 5.153800228976335163, 19.02544592524342804, 84.79057627198099567 ) ) ;
#100222=CARTESIAN_POINT ( 'NONE',  ( 16.52544592524342804, -4.483927247898539470, 83.54057627198102409 ) ) ;
#100223=CARTESIAN_POINT ( 'NONE',  ( 16.52544592524335698, 4.483927247898782831, 26.45942372801901854 ) ) ;
#100224=CARTESIAN_POINT ( 'NONE',  ( -8.314922557961024197, 14.29746914071037800, 112.9177570613523329 ) ) ;
#100226=CARTESIAN_POINT ( 'NONE',  ( -9.474510206698964154, 16.51473224551069663, 105.4155762719810383 ) ) ;
#100227=CARTESIAN_POINT ( 'NONE',  ( -10.81492255796078084, -18.62759615963271287, 87.08224293864769550 ) ) ;
#100228=CARTESIAN_POINT ( 'NONE',  ( -8.314922557960811034, -14.29746914071050412, 22.08224293864769194 ) ) ;
#100229=CARTESIAN_POINT ( 'NONE',  ( -16.51473224551069308, -9.474510206698971260, 101.6655762719810241 ) ) ;
#100230=CARTESIAN_POINT ( 'NONE',  ( -19.02544592524334988, -5.153800228976617603, 78.95942372801900433 ) ) ;
#100231=CARTESIAN_POINT ( 'NONE',  ( 21.55341960407619695, -5.719274019375665929, 106.0427570613523471 ) ) ;
#100232=CARTESIAN_POINT ( 'NONE',  ( 18.67979575497178502, 10.72451020669898547, 84.16557627198103830 ) ) ;
#100233=CARTESIAN_POINT ( 'NONE',  ( 18.62759615963271287, -10.81492255796078972, 38.33224293864768839 ) ) ;
#100234=CARTESIAN_POINT ( 'NONE',  ( -13.89961937509977652, 13.97604488694528158, 65.62390960531436690 ) ) ;
#100235=CARTESIAN_POINT ( 'NONE',  ( -14.29746914071049879, 8.314922557960819915, 30.83224293864770260 ) ) ;
#100236=CARTESIAN_POINT ( 'NONE',  ( -0.05219959533909027116, -19.03943276465977164, 72.49890960531435269 ) ) ;
#100239=CARTESIAN_POINT ( 'NONE',  ( 5.049401038297881783, 19.05341960407617563, 32.29275706135233293 ) ) ;
#100240=CARTESIAN_POINT ( 'NONE',  ( -0.05219959533910754901, -16.53943276465976808, 87.49890960531436690 ) ) ;
#100241=CARTESIAN_POINT ( 'NONE',  ( 21.52544592524334988, 5.823673210054432836, 26.45942372801901854 ) ) ;
#100243=CARTESIAN_POINT ( 'NONE',  ( 10.72451020669898902, -18.67979575497178502, 77.91557627198102409 ) ) ;
#100244=CARTESIAN_POINT ( 'NONE',  ( -14.29746914071037622, -8.314922557961029526, 94.16775706135237556 ) ) ;
#100245=CARTESIAN_POINT ( 'NONE',  ( 9.474510206698971260, -16.51473224551069308, 27.91557627198103120 ) ) ;
#100246=CARTESIAN_POINT ( 'NONE',  ( 19.05341960407611168, 5.049401038298154454, 68.95724293864769550 ) ) ;
#100248=CARTESIAN_POINT ( 'NONE',  ( 19.05341960407611168, 5.049401038298154454, 23.95724293864769194 ) ) ;
#100249=CARTESIAN_POINT ( 'NONE',  ( -12.06949235617756955, 12.14591786802309770, 25.62390960531435624 ) ) ;
#100250=CARTESIAN_POINT ( 'NONE',  ( -10.72451020669870658, -18.67979575497194134, 59.58442372801901854 ) ) ;
#100252=CARTESIAN_POINT ( 'NONE',  ( -0.05219959533937732626, 21.53943276465977519, 97.50109039468567573 ) ) ;
#100253=CARTESIAN_POINT ( 'NONE',  ( 19.02544592524343514, -5.153800228976328945, 43.54057627198103120 ) ) ;
#100254=CARTESIAN_POINT ( 'NONE',  ( -16.46253265017160317, 9.564922557960807481, 55.83224293864769550 ) ) ;
#100256=CARTESIAN_POINT ( 'NONE',  ( -21.52544592524334988, -5.823673210054445271, 88.95942372801901854 ) ) ;
#100257=CARTESIAN_POINT ( 'NONE',  ( 16.52544592524335698, 4.483927247898782831, 66.45942372801903275 ) ) ;
#100258=CARTESIAN_POINT ( 'NONE',  ( -10.81492255796105439, 18.62759615963255655, 82.91775706135234714 ) ) ;
#100259=CARTESIAN_POINT ( 'NONE',  ( -10.81492255796078084, -18.62759615963271287, 27.08224293864769550 ) ) ;
#100260=CARTESIAN_POINT ( 'NONE',  ( -19.05341960407617563, 5.049401038297882671, 98.54275706135233293 ) ) ;
#100261=CARTESIAN_POINT ( 'NONE',  ( -10.81492255796105439, 18.62759615963255655, 67.91775706135234714 ) ) ;
#100262=CARTESIAN_POINT ( 'NONE',  ( -16.53943276465976808, -0.05219959533934237506, 38.75109039468567573 ) ) ;
#100263=CARTESIAN_POINT ( 'NONE',  ( 5.719274019375991003, -21.55341960407610458, 82.70724293864770971 ) ) ;
#100264=CARTESIAN_POINT ( 'NONE',  ( 13.97604488694548053, -13.89961937509957401, 90.62609039468567573 ) ) ;
#100265=CARTESIAN_POINT ( 'NONE',  ( 0.05219959533909260263, 19.03943276465977164, 64.99890960531436690 ) ) ;
#100266=CARTESIAN_POINT ( 'NONE',  ( 5.153800228976615827, -19.02544592524334988, 90.20942372801900433 ) ) ;
#100267=CARTESIAN_POINT ( 'NONE',  ( 19.03943276465977164, 0.05219959533936151252, 101.2510903946856757 ) ) ;
#100268=CARTESIAN_POINT ( 'NONE',  ( -0.05219959533910754901, -16.53943276465976808, 57.49890960531435979 ) ) ;
#100269=CARTESIAN_POINT ( 'NONE',  ( -5.049401038297874678, -19.05341960407617918, 74.79275706135231871 ) ) ;
#100270=ORIENTED_EDGE ( 'NONE', *, *, #164449, .T. ) ;
#100271=CARTESIAN_POINT ( 'NONE',  ( -0.05219959533934338120, 16.53943276465976808, 62.50109039468568284 ) ) ;
#100272=ADVANCED_FACE ( 'NONE', ( #127431 ), #109548, .T. ) ;
#100273=CARTESIAN_POINT ( 'NONE',  ( 5.153800228976335163, 19.02544592524342804, 44.79057627198103830 ) ) ;
#100274=CARTESIAN_POINT ( 'NONE',  ( 13.97604488694527802, 13.89961937509977652, 59.37390960531434558 ) ) ;
#100275=CARTESIAN_POINT ( 'NONE',  ( -14.29746914071037622, -8.314922557961029526, 59.16775706135234714 ) ) ;
#100278=CARTESIAN_POINT ( 'NONE',  ( 0.05219959533909260263, 19.03943276465977164, 104.9989096053143669 ) ) ;
#100279=CARTESIAN_POINT ( 'NONE',  ( 0.05219959533909260263, 19.03943276465977164, 24.99890960531435269 ) ) ;
#100280=ORIENTED_EDGE ( 'NONE', *, *, #11460, .F. ) ;
#100281=CARTESIAN_POINT ( 'NONE',  ( -13.97604488694547697, 13.89961937509957934, 103.1260903946856473 ) ) ;
#100282=EDGE_CURVE ( 'NONE', #110833, #88111, #73265, .T. ) ;
#100283=CARTESIAN_POINT ( 'NONE',  ( -21.55341960407610458, -5.719274019375992779, 31.45724293864769550 ) ) ;
#100284=CARTESIAN_POINT ( 'NONE',  ( -5.153800228976607833, 19.02544592524334988, 37.70942372801899722 ) ) ;
#100285=CARTESIAN_POINT ( 'NONE',  ( 0.05219959533934541429, -16.53943276465976808, 20.00109039468568639 ) ) ;
#100286=CARTESIAN_POINT ( 'NONE',  ( -13.89961937509977652, 13.97604488694528158, 30.62390960531435269 ) ) ;
#100287=CARTESIAN_POINT ( 'NONE',  ( 5.153800228976335163, 19.02544592524342804, 54.79057627198103120 ) ) ;
#100288=CARTESIAN_POINT ( 'NONE',  ( -5.823673210054116645, -21.52544592524344225, 72.29057627198102409 ) ) ;
#100289=CARTESIAN_POINT ( 'NONE',  ( 19.05341960407611168, 5.049401038298154454, 98.95724293864766707 ) ) ;
#100290=CARTESIAN_POINT ( 'NONE',  ( -19.05341960407611168, -5.049401038298163336, 36.45724293864766707 ) ) ;
#100292=CARTESIAN_POINT ( 'NONE',  ( -9.564922557961040184, 16.46253265017147172, 77.91775706135234714 ) ) ;
#100293=CARTESIAN_POINT ( 'NONE',  ( 16.53943276465976808, -0.05219959533910856209, 63.74890960531435979 ) ) ;
#100294=CARTESIAN_POINT ( 'NONE',  ( -15.80617190586745835, -15.72974639402198527, 51.87390960531437401 ) ) ;
#100295=CARTESIAN_POINT ( 'NONE',  ( 18.67979575497194134, -10.72451020669871369, 105.8344237280190328 ) ) ;
#100296=CARTESIAN_POINT ( 'NONE',  ( 10.81492255796078972, 18.62759615963270932, 94.58224293864769550 ) ) ;
#100297=CARTESIAN_POINT ( 'NONE',  ( -10.81492255796105439, 18.62759615963255655, 67.91775706135234714 ) ) ;
#100298=CARTESIAN_POINT ( 'NONE',  ( 0.05219959533937995610, -21.53943276465977519, 75.00109039468568994 ) ) ;
#100299=CARTESIAN_POINT ( 'NONE',  ( -13.89961937509977652, 13.97604488694528158, 110.6239096053143243 ) ) ;
#100300=CARTESIAN_POINT ( 'NONE',  ( 12.14591786802327356, -12.06949235617739191, 110.6260903946857042 ) ) ;
#100301=CARTESIAN_POINT ( 'NONE',  ( -15.80617190586768217, 15.72974639402176855, 78.12609039468570415 ) ) ;
#100302=CARTESIAN_POINT ( 'NONE',  ( -9.474510206698964154, 16.51473224551069663, 70.41557627198102409 ) ) ;
#100303=CARTESIAN_POINT ( 'NONE',  ( -16.51473224551082808, 9.474510206698731452, 38.33442372801899722 ) ) ;
#100304=CARTESIAN_POINT ( 'NONE',  ( -10.72451020669870658, -18.67979575497194134, 24.58442372801901499 ) ) ;
#100305=CARTESIAN_POINT ( 'NONE',  ( -5.153800228976328057, -19.02544592524343514, 62.29057627198100988 ) ) ;
#100306=CARTESIAN_POINT ( 'NONE',  ( 4.483927247898545687, 16.52544592524342804, 84.79057627198102409 ) ) ;
#100307=CARTESIAN_POINT ( 'NONE',  ( 16.53943276465976808, -0.05219959533910856209, 48.74890960531435979 ) ) ;
#100308=CARTESIAN_POINT ( 'NONE',  ( -15.80617190586745835, -15.72974639402198527, 56.87390960531436690 ) ) ;
#100309=CARTESIAN_POINT ( 'NONE',  ( 19.02544592524343514, -5.153800228976328945, 58.54057627198102409 ) ) ;
#100310=CARTESIAN_POINT ( 'NONE',  ( 5.823673210054125526, 21.52544592524343514, 69.79057627198102409 ) ) ;
#100311=CARTESIAN_POINT ( 'NONE',  ( -13.97604488694547697, 13.89961937509957934, 58.12609039468566863 ) ) ;
#100312=CARTESIAN_POINT ( 'NONE',  ( 0.05219959533910956823, 16.53943276465976808, 64.99890960531435269 ) ) ;
#100313=CARTESIAN_POINT ( 'NONE',  ( -21.53943276465977519, 0.05219959533907696930, 46.24890960531435979 ) ) ;
#100316=CARTESIAN_POINT ( 'NONE',  ( 16.52544592524335698, 4.483927247898782831, 86.45942372801901854 ) ) ;
#100318=CARTESIAN_POINT ( 'NONE',  ( -13.97604488694547697, 13.89961937509957934, 83.12609039468564731 ) ) ;
#100319=CARTESIAN_POINT ( 'NONE',  ( -4.483927247898539470, -16.52544592524342804, 57.29057627198103120 ) ) ;
#100320=CARTESIAN_POINT ( 'NONE',  ( -19.34837522270366250, -5.499999999999742428, 60.86337684832576400 ) ) ;
#100321=CARTESIAN_POINT ( 'NONE',  ( 13.89961937509977652, -13.97604488694527269, 48.12390960531435979 ) ) ;
#100322=CARTESIAN_POINT ( 'NONE',  ( -14.34966873604960291, -8.224510206698953496, 36.66557627198103120 ) ) ;
#100323=CARTESIAN_POINT ( 'NONE',  ( 0.05219959533909260263, 19.03943276465977164, 84.99890960531436690 ) ) ;
#100324=CARTESIAN_POINT ( 'NONE',  ( 5.153800228976615827, -19.02544592524334988, 75.20942372801896170 ) ) ;
#100325=CARTESIAN_POINT ( 'NONE',  ( -9.564922557960796823, -16.46253265017161027, 57.08224293864769550 ) ) ;
#100326=CARTESIAN_POINT ( 'NONE',  ( 0.05219959533937995610, -21.53943276465977519, 65.00109039468568994 ) ) ;
#100327=CARTESIAN_POINT ( 'NONE',  ( -19.03943276465977164, 0.05219959533909376836, 86.24890960531436690 ) ) ;
#100328=CARTESIAN_POINT ( 'NONE',  ( 0.05219959533909260263, 19.03943276465977164, 24.99890960531435269 ) ) ;
#100329=CARTESIAN_POINT ( 'NONE',  ( -19.02544592524342804, 5.153800228976336051, 76.04057627198102409 ) ) ;
#100330=CARTESIAN_POINT ( 'NONE',  ( 0.05219959533907565091, 21.53943276465977519, 54.99890960531435269 ) ) ;
#100332=CARTESIAN_POINT ( 'NONE',  ( 19.03943276465977164, -0.05219959533909143690, 43.74890960531435979 ) ) ;
#100333=CARTESIAN_POINT ( 'NONE',  ( -21.55341960407610458, -5.719274019375992779, 56.45724293864768839 ) ) ;
#100334=CARTESIAN_POINT ( 'NONE',  ( -19.03943276465977164, -0.05219959533935918106, 83.75109039468567573 ) ) ;
#100335=CARTESIAN_POINT ( 'NONE',  ( -0.05219959533934338120, 16.53943276465976808, 102.5010903946856899 ) ) ;
#100336=CARTESIAN_POINT ( 'NONE',  ( 16.51473224551083163, -9.474510206698727899, 30.83442372801900433 ) ) ;
#100337=CARTESIAN_POINT ( 'NONE',  ( 16.55341960407618274, -4.379528057220086978, 56.04275706135235424 ) ) ;
#100338=CARTESIAN_POINT ( 'NONE',  ( -16.53943276465976808, -0.05219959533934237506, 78.75109039468568994 ) ) ;
#100339=CARTESIAN_POINT ( 'NONE',  ( -17.49999999999999645, 5.499999999999992895, 68.71769037696435589 ) ) ;
#100340=CARTESIAN_POINT ( 'NONE',  ( -4.379528057220086978, -16.55341960407618274, 69.79275706135234714 ) ) ;
#100341=CARTESIAN_POINT ( 'NONE',  ( -10.72451020669898014, 18.67979575497178502, 25.41557627198103120 ) ) ;
#100342=CARTESIAN_POINT ( 'NONE',  ( -9.564922557960796823, -16.46253265017161027, 32.08224293864769550 ) ) ;
#100343=CARTESIAN_POINT ( 'NONE',  ( 14.29746914071037800, 8.314922557961029526, 31.66775706135234358 ) ) ;
#100344=CARTESIAN_POINT ( 'NONE',  ( -16.46253265017160317, 9.564922557960807481, 50.83224293864770260 ) ) ;
#100345=CARTESIAN_POINT ( 'NONE',  ( -21.52544592524334988, -5.823673210054445271, 38.95942372801901854 ) ) ;
#100346=CARTESIAN_POINT ( 'NONE',  ( 4.483927247898790824, -16.52544592524335698, 30.20942372801902565 ) ) ;
#100347=CARTESIAN_POINT ( 'NONE',  ( -14.29746914071049879, 8.314922557960819915, 25.83224293864769194 ) ) ;
#100348=CARTESIAN_POINT ( 'NONE',  ( -17.72662750342728089, -5.500000000000023093, 71.40179492283743912 ) ) ;
#100349=CARTESIAN_POINT ( 'NONE',  ( -0.05219959533937732626, 21.53943276465977519, 112.5010903946857042 ) ) ;
#100350=CARTESIAN_POINT ( 'NONE',  ( 9.474510206698729675, 16.51473224551082808, 107.0844237280190043 ) ) ;
#100351=CARTESIAN_POINT ( 'NONE',  ( 9.474510206698729675, 16.51473224551082808, 67.08442372801900433 ) ) ;
#100352=CARTESIAN_POINT ( 'NONE',  ( 0.05219959533910956823, 16.53943276465976808, 64.99890960531435269 ) ) ;
#100353=CARTESIAN_POINT ( 'NONE',  ( 9.564922557960805705, 16.46253265017160317, 44.58224293864769550 ) ) ;
#100354=CARTESIAN_POINT ( 'NONE',  ( -0.05219959533936034679, 19.03943276465977164, 72.50109039468566152 ) ) ;
#100356=CARTESIAN_POINT ( 'NONE',  ( -18.62759615963255300, -10.81492255796106328, 64.16775706135234714 ) ) ;
#100357=CARTESIAN_POINT ( 'NONE',  ( -14.29746914071037622, -8.314922557961029526, 44.16775706135234714 ) ) ;
#100358=CARTESIAN_POINT ( 'NONE',  ( 19.25663599770062362, -5.499999999999449329, 56.49419308057201761 ) ) ;
#100359=CARTESIAN_POINT ( 'NONE',  ( 5.719274019375991003, -21.55341960407610458, 42.70724293864770260 ) ) ;
#100360=CARTESIAN_POINT ( 'NONE',  ( 16.55341960407618274, -4.379528057220086978, 21.04275706135234714 ) ) ;
#100361=CARTESIAN_POINT ( 'NONE',  ( 13.89961937509977652, -13.97604488694527269, 113.1239096053143527 ) ) ;
#100363=CARTESIAN_POINT ( 'NONE',  ( -13.89961937509977652, 13.97604488694528158, 35.62390960531435269 ) ) ;
#100364=CARTESIAN_POINT ( 'NONE',  ( -10.81492255796105439, 18.62759615963255655, 112.9177570613523329 ) ) ;
#100365=CARTESIAN_POINT ( 'NONE',  ( -19.03943276465977164, 0.05219959533909376836, 56.24890960531435979 ) ) ;
#100366=CARTESIAN_POINT ( 'NONE',  ( -5.823673210054431948, 21.52544592524334988, 67.70942372801901854 ) ) ;
#100367=CARTESIAN_POINT ( 'NONE',  ( 15.72974639402176855, 15.80617190586768217, 101.8760903946857042 ) ) ;
#100368=CARTESIAN_POINT ( 'NONE',  ( 16.53943276465976808, -0.05219959533910856209, 23.74890960531435269 ) ) ;
#100369=CARTESIAN_POINT ( 'NONE',  ( -5.153800228976328057, -19.02544592524343514, 27.29057627198103120 ) ) ;
#100370=CARTESIAN_POINT ( 'NONE',  ( -5.153800228976328057, -19.02544592524343514, 92.29057627198099567 ) ) ;
#100371=CARTESIAN_POINT ( 'NONE',  ( 15.72974639402176855, 15.80617190586768217, 56.87609039468568994 ) ) ;
#100372=CARTESIAN_POINT ( 'NONE',  ( 13.97604488694527802, 13.89961937509977652, 39.37390960531435269 ) ) ;
#100373=EDGE_CURVE ( 'NONE', #63341, #11857, #174061, .T. ) ;
#100374=CARTESIAN_POINT ( 'NONE',  ( -15.80617190586768217, 15.72974639402176855, 53.12609039468568284 ) ) ;
#100375=CARTESIAN_POINT ( 'NONE',  ( 9.564922557961047289, -16.46253265017146816, 95.41775706135233293 ) ) ;
#100376=CARTESIAN_POINT ( 'NONE',  ( 9.564922557960805705, 16.46253265017160317, 99.58224293864770971 ) ) ;
#100377=CARTESIAN_POINT ( 'NONE',  ( 4.483927247898545687, 16.52544592524342804, 114.7905762719810383 ) ) ;
#100378=CARTESIAN_POINT ( 'NONE',  ( 15.80617190586746368, 15.72974639402197994, 114.3739096053143527 ) ) ;
#100379=CARTESIAN_POINT ( 'NONE',  ( -16.51473224551082808, 9.474510206698731452, 33.33442372801899722 ) ) ;
#100380=CARTESIAN_POINT ( 'NONE',  ( -19.05341960407611168, -5.049401038298163336, 21.45724293864768839 ) ) ;
#100381=CARTESIAN_POINT ( 'NONE',  ( -19.02544592524342804, 5.153800228976336051, 51.04057627198103120 ) ) ;
#100382=CARTESIAN_POINT ( 'NONE',  ( -19.02544592524334988, -5.153800228976617603, 103.9594237280190043 ) ) ;
#100383=CARTESIAN_POINT ( 'NONE',  ( 12.06949235617757843, -12.14591786802309237, 58.12390960531435979 ) ) ;
#100384=CARTESIAN_POINT ( 'NONE',  ( 21.52544592524334988, 5.823673210054432836, 106.4594237280190328 ) ) ;
#100385=CARTESIAN_POINT ( 'NONE',  ( -10.81492255796078084, -18.62759615963271287, 22.08224293864769194 ) ) ;
#100386=CARTESIAN_POINT ( 'NONE',  ( 16.51473224551083163, -9.474510206698727899, 85.83442372801900433 ) ) ;
#100387=CARTESIAN_POINT ( 'NONE',  ( 0.05219959533907565091, 21.53943276465977519, 94.99890960531436690 ) ) ;
#100388=CARTESIAN_POINT ( 'NONE',  ( 0.05219959533937995610, -21.53943276465977519, 50.00109039468568994 ) ) ;
#100389=CARTESIAN_POINT ( 'NONE',  ( 8.224510206698742110, 14.34966873604972548, 47.08442372801901854 ) ) ;
#100390=CARTESIAN_POINT ( 'NONE',  ( 12.14591786802327356, -12.06949235617739191, 105.6260903946856899 ) ) ;
#100391=CARTESIAN_POINT ( 'NONE',  ( 4.379528057220092307, 16.55341960407617563, 42.29275706135235424 ) ) ;
#100392=CARTESIAN_POINT ( 'NONE',  ( 18.67979575497194134, -10.72451020669871369, 55.83442372801901854 ) ) ;
#100393=CARTESIAN_POINT ( 'NONE',  ( 18.67979575497178502, 10.72451020669898547, 44.16557627198103120 ) ) ;
#100394=CARTESIAN_POINT ( 'NONE',  ( -13.89961937509977652, 13.97604488694528158, 35.62390960531435269 ) ) ;
#100396=CARTESIAN_POINT ( 'NONE',  ( 8.224510206698742110, 14.34966873604972548, 67.08442372801901854 ) ) ;
#100397=CARTESIAN_POINT ( 'NONE',  ( 10.81492255796078972, 18.62759615963270932, 94.58224293864769550 ) ) ;
#100398=CARTESIAN_POINT ( 'NONE',  ( -4.379528057220328563, 16.55341960407611168, 40.20724293864769550 ) ) ;
#100399=CARTESIAN_POINT ( 'NONE',  ( 16.53943276465976808, 0.05219959533934440121, 56.25109039468568284 ) ) ;
#100400=CARTESIAN_POINT ( 'NONE',  ( -19.02544592524334988, -5.153800228976617603, 98.95942372801900433 ) ) ;
#100401=CARTESIAN_POINT ( 'NONE',  ( 10.81492255796078972, 18.62759615963270932, 104.5822429386477097 ) ) ;
#100402=CARTESIAN_POINT ( 'NONE',  ( -0.05219959533910754901, -16.53943276465976808, 37.49890960531436690 ) ) ;
#100404=CARTESIAN_POINT ( 'NONE',  ( -14.29746914071037622, -8.314922557961029526, 74.16775706135231871 ) ) ;
#100406=CARTESIAN_POINT ( 'NONE',  ( -21.55341960407610458, -5.719274019375992779, 76.45724293864769550 ) ) ;
#100407=CARTESIAN_POINT ( 'NONE',  ( 14.29746914071037800, 8.314922557961029526, 101.6677570613523613 ) ) ;
#100410=CARTESIAN_POINT ( 'NONE',  ( -18.67979575497178146, -10.72451020669898902, 91.66557627198103830 ) ) ;
#100411=CARTESIAN_POINT ( 'NONE',  ( -21.52544592524343514, 5.823673210054127303, 111.0405762719810525 ) ) ;
#100412=CARTESIAN_POINT ( 'NONE',  ( 12.14591786802309770, 12.06949235617756955, 34.37390960531435979 ) ) ;
#100413=CARTESIAN_POINT ( 'NONE',  ( -12.06949235617739369, -12.14591786802326823, 39.37609039468567573 ) ) ;
#100414=CARTESIAN_POINT ( 'NONE',  ( 19.03943276465977164, -0.05219959533909143690, 33.74890960531435979 ) ) ;
#100415=CARTESIAN_POINT ( 'NONE',  ( -0.05219959533909027116, -19.03943276465977164, 72.49890960531435269 ) ) ;
#100417=CARTESIAN_POINT ( 'NONE',  ( -5.823673210054116645, -21.52544592524344225, 22.29057627198102765 ) ) ;
#100418=CARTESIAN_POINT ( 'NONE',  ( -16.51473224551069308, -9.474510206698971260, 111.6655762719810383 ) ) ;
#100419=CARTESIAN_POINT ( 'NONE',  ( 16.46253265017146816, 9.564922557961045513, 101.6677570613523329 ) ) ;
#100420=CARTESIAN_POINT ( 'NONE',  ( 16.46253265017146816, 9.564922557961045513, 36.66775706135233293 ) ) ;
#100421=CARTESIAN_POINT ( 'NONE',  ( 10.81492255796078972, 18.62759615963270932, 89.58224293864768129 ) ) ;
#100422=CARTESIAN_POINT ( 'NONE',  ( 4.483927247898545687, 16.52544592524342804, 24.79057627198103120 ) ) ;
#100423=CARTESIAN_POINT ( 'NONE',  ( -15.72974639402197994, 15.80617190586746368, 50.62390960531435979 ) ) ;
#100424=CARTESIAN_POINT ( 'NONE',  ( -21.53943276465977519, 0.05219959533907696930, 81.24890960531436690 ) ) ;
#100425=CARTESIAN_POINT ( 'NONE',  ( 13.97604488694548053, -13.89961937509957401, 105.6260903946856757 ) ) ;
#100426=CARTESIAN_POINT ( 'NONE',  ( 19.03943276465977164, -0.05219959533909143690, 103.7489096053143669 ) ) ;
#100427=CARTESIAN_POINT ( 'NONE',  ( -5.719274019375665041, -21.55341960407619695, 74.79275706135234714 ) ) ;
#100428=CARTESIAN_POINT ( 'NONE',  ( 5.049401038298161559, -19.05341960407611168, 67.70724293864769550 ) ) ;
#100429=CARTESIAN_POINT ( 'NONE',  ( 16.52544592524342804, -4.483927247898539470, 98.54057627198105251 ) ) ;
#100431=CARTESIAN_POINT ( 'NONE',  ( 5.153800228976335163, 19.02544592524342804, 64.79057627198100988 ) ) ;
#100432=CARTESIAN_POINT ( 'NONE',  ( -4.379528057220328563, 16.55341960407611168, 85.20724293864770971 ) ) ;
#100434=CARTESIAN_POINT ( 'NONE',  ( 13.97604488694548053, -13.89961937509957401, 105.6260903946856757 ) ) ;
#100436=CARTESIAN_POINT ( 'NONE',  ( -5.049401038298153566, 19.05341960407611168, 55.20724293864769550 ) ) ;
#100437=CARTESIAN_POINT ( 'NONE',  ( 5.719274019375673035, 21.55341960407619339, 82.29275706135234714 ) ) ;
#100438=CARTESIAN_POINT ( 'NONE',  ( 13.97604488694527802, 13.89961937509977652, 104.3739096053143385 ) ) ;
#100439=EDGE_CURVE ( 'NONE', #45079, #119772, #145936, .T. ) ;
#100440=CARTESIAN_POINT ( 'NONE',  ( 12.06949235617739724, 12.14591786802326823, 81.87609039468568994 ) ) ;
#100441=CARTESIAN_POINT ( 'NONE',  ( -17.49999999999999645, -5.499999999999992895, 74.20309617465828467 ) ) ;
#100442=CARTESIAN_POINT ( 'NONE',  ( 16.46253265017146816, 9.564922557961045513, 56.66775706135233293 ) ) ;
#100443=CARTESIAN_POINT ( 'NONE',  ( -21.55341960407619339, 5.719274019375674811, 93.54275706135234714 ) ) ;
#100446=CARTESIAN_POINT ( 'NONE',  ( -16.53943276465976808, 0.05219959533911058130, 21.24890960531436690 ) ) ;
#100448=CARTESIAN_POINT ( 'NONE',  ( -12.06949235617739369, -12.14591786802326823, 89.37609039468568994 ) ) ;
#100450=CARTESIAN_POINT ( 'NONE',  ( -4.379528057220086978, -16.55341960407618274, 64.79275706135234714 ) ) ;
#100451=CARTESIAN_POINT ( 'NONE',  ( 21.52544592524334988, 5.823673210054432836, 86.45942372801901854 ) ) ;
#100452=CARTESIAN_POINT ( 'NONE',  ( -9.564922557961040184, 16.46253265017147172, 87.91775706135233293 ) ) ;
#100453=CARTESIAN_POINT ( 'NONE',  ( 19.05341960407617918, -5.049401038297876454, 46.04275706135233293 ) ) ;
#100454=CARTESIAN_POINT ( 'NONE',  ( -0.05219959533909027116, -19.03943276465977164, 67.49890960531436690 ) ) ;
#100455=CARTESIAN_POINT ( 'NONE',  ( -19.03943276465977164, 0.05219959533909376836, 51.24890960531436690 ) ) ;
#100456=CARTESIAN_POINT ( 'NONE',  ( -17.59860650958991002, -7.585241751807008548, 86.57662985737509587 ) ) ;
#100457=CARTESIAN_POINT ( 'NONE',  ( 21.52544592524344225, -5.823673210054117533, 78.54057627198103830 ) ) ;
#100458=CARTESIAN_POINT ( 'NONE',  ( 5.823673210054125526, 21.52544592524343514, 49.79057627198102409 ) ) ;
#100459=CARTESIAN_POINT ( 'NONE',  ( -5.153800228976328057, -19.02544592524343514, 37.29057627198102409 ) ) ;
#100460=CARTESIAN_POINT ( 'NONE',  ( 16.55341960407618274, -4.379528057220086978, 61.04275706135234714 ) ) ;
#100461=ADVANCED_FACE ( 'NONE', ( #145830 ), #161010, .T. ) ;
#100464=CARTESIAN_POINT ( 'NONE',  ( -21.52544592524334988, -5.823673210054445271, 43.95942372801902565 ) ) ;
#100465=CARTESIAN_POINT ( 'NONE',  ( -0.05219959533910754901, -16.53943276465976808, 67.49890960531436690 ) ) ;
#100467=CARTESIAN_POINT ( 'NONE',  ( -4.483927247898782831, 16.52544592524335698, 27.70942372801901854 ) ) ;
#100468=CARTESIAN_POINT ( 'NONE',  ( -9.474510206698720793, -16.51473224551083518, 59.58442372801900433 ) ) ;
#100469=CARTESIAN_POINT ( 'NONE',  ( -16.55341960407611168, -4.379528057220339221, 61.45724293864770260 ) ) ;
#100470=CARTESIAN_POINT ( 'NONE',  ( -21.53943276465977519, -0.05219959533937600094, 38.75109039468567573 ) ) ;
#100471=CARTESIAN_POINT ( 'NONE',  ( 17.59860650958990647, 7.585241751807016541, 99.07662985737508166 ) ) ;
#100472=CARTESIAN_POINT ( 'NONE',  ( 15.72974639402199770, -15.80617190586745480, 93.12390960531436690 ) ) ;
#100473=CARTESIAN_POINT ( 'NONE',  ( 19.05341960407611168, 5.049401038298154454, 103.9572429386476671 ) ) ;
#100474=CARTESIAN_POINT ( 'NONE',  ( 4.483927247898545687, 16.52544592524342804, 74.79057627198105251 ) ) ;
#100475=CARTESIAN_POINT ( 'NONE',  ( -19.03943276465977164, 0.05219959533909376836, 111.2489096053143669 ) ) ;
#100477=CARTESIAN_POINT ( 'NONE',  ( -19.05341960407617563, 5.049401038297882671, 68.54275706135230450 ) ) ;
#100478=CARTESIAN_POINT ( 'NONE',  ( -18.62759615963270932, 10.81492255796079327, 115.8322429386477097 ) ) ;
#100479=CARTESIAN_POINT ( 'NONE',  ( -13.89961937509977652, 13.97604488694528158, 60.62390960531436690 ) ) ;
#100480=CARTESIAN_POINT ( 'NONE',  ( 9.474510206698729675, 16.51473224551082808, 42.08442372801900433 ) ) ;
#100481=CARTESIAN_POINT ( 'NONE',  ( -19.02544592524342804, 5.153800228976336051, 36.04057627198100988 ) ) ;
#100482=CARTESIAN_POINT ( 'NONE',  ( -15.80617190586768217, 15.72974639402176855, 63.12609039468568994 ) ) ;
#100483=CARTESIAN_POINT ( 'NONE',  ( -17.44270441346519718, -5.991230190322950122, 71.36335079264232206 ) ) ;
#100484=CARTESIAN_POINT ( 'NONE',  ( 12.14591786802309770, 12.06949235617756955, 59.37390960531436690 ) ) ;
#100485=CARTESIAN_POINT ( 'NONE',  ( 13.97604488694527802, 13.89961937509977652, 59.37390960531434558 ) ) ;
#100486=CARTESIAN_POINT ( 'NONE',  ( -0.05219959533907301413, -21.53943276465977519, 92.49890960531436690 ) ) ;
#100487=CARTESIAN_POINT ( 'NONE',  ( -16.51473224551069308, -9.474510206698971260, 61.66557627198103120 ) ) ;
#100489=CARTESIAN_POINT ( 'NONE',  ( 0.05219959533907565091, 21.53943276465977519, 69.99890960531435269 ) ) ;
#100490=CARTESIAN_POINT ( 'NONE',  ( -5.823673210054431948, 21.52544592524334988, 102.7094237280190185 ) ) ;
#100491=CARTESIAN_POINT ( 'NONE',  ( 13.97604488694527802, 13.89961937509977652, 24.37390960531435624 ) ) ;
#100492=CARTESIAN_POINT ( 'NONE',  ( -14.34966873604972548, 8.224510206698743886, 93.33442372801901854 ) ) ;
#100493=CARTESIAN_POINT ( 'NONE',  ( 8.224510206698953496, -14.34966873604960469, 77.91557627198102409 ) ) ;
#100494=CARTESIAN_POINT ( 'NONE',  ( -5.153800228976607833, 19.02544592524334988, 97.70942372801900433 ) ) ;
#100496=CARTESIAN_POINT ( 'NONE',  ( -5.719274019375665041, -21.55341960407619695, 19.79275706135235069 ) ) ;
#100497=CARTESIAN_POINT ( 'NONE',  ( -13.97604488694547697, 13.89961937509957934, 38.12609039468566152 ) ) ;
#100498=CARTESIAN_POINT ( 'NONE',  ( -16.53943276465976808, -0.05219959533934237506, 98.75109039468568994 ) ) ;
#100499=CARTESIAN_POINT ( 'NONE',  ( -13.89961937509957401, -13.97604488694547875, 24.37609039468565442 ) ) ;
#100500=CARTESIAN_POINT ( 'NONE',  ( -16.51473224551069308, -9.474510206698971260, 86.66557627198102409 ) ) ;
#100501=CARTESIAN_POINT ( 'NONE',  ( 21.55341960407610458, 5.719274019375980345, 63.95724293864770260 ) ) ;
#100502=CARTESIAN_POINT ( 'NONE',  ( -5.153800228976328057, -19.02544592524343514, 22.29057627198102765 ) ) ;
#100503=CARTESIAN_POINT ( 'NONE',  ( 16.52544592524342804, -4.483927247898539470, 113.5405762719810383 ) ) ;
#100504=CARTESIAN_POINT ( 'NONE',  ( -9.474510206698720793, -16.51473224551083518, 19.58442372801899722 ) ) ;
#100505=CARTESIAN_POINT ( 'NONE',  ( 14.29746914071037800, 8.314922557961029526, 81.66775706135236135 ) ) ;
#100506=CARTESIAN_POINT ( 'NONE',  ( -21.55341960407619339, 5.719274019375674811, 33.54275706135234714 ) ) ;
#100507=CARTESIAN_POINT ( 'NONE',  ( -16.53943276465976808, -0.05219959533934237506, 28.75109039468567929 ) ) ;
#100508=CARTESIAN_POINT ( 'NONE',  ( -5.153800228976328057, -19.02544592524343514, 102.2905762719810383 ) ) ;
#100509=CARTESIAN_POINT ( 'NONE',  ( -0.05219959533909027116, -19.03943276465977164, 37.49890960531436690 ) ) ;
#100510=CARTESIAN_POINT ( 'NONE',  ( -9.564922557960796823, -16.46253265017161027, 67.08224293864769550 ) ) ;
#100511=CARTESIAN_POINT ( 'NONE',  ( 12.14591786802327356, -12.06949235617739191, 50.62609039468568994 ) ) ;
#100512=CARTESIAN_POINT ( 'NONE',  ( -0.05219959533910754901, -16.53943276465976808, 97.49890960531436690 ) ) ;
#100513=CARTESIAN_POINT ( 'NONE',  ( 14.29746914071037800, 8.314922557961029526, 96.66775706135234714 ) ) ;
#100514=CARTESIAN_POINT ( 'NONE',  ( 18.62759615963255655, 10.81492255796105972, 51.66775706135234714 ) ) ;
#100515=CARTESIAN_POINT ( 'NONE',  ( 19.03943276465977164, -0.05219959533909143690, 73.74890960531435269 ) ) ;
#100516=CARTESIAN_POINT ( 'NONE',  ( 19.05341960407611168, 5.049401038298154454, 58.95724293864768129 ) ) ;
#100517=CARTESIAN_POINT ( 'NONE',  ( 5.153800228976335163, 19.02544592524342804, 99.79057627198102409 ) ) ;
#100518=CARTESIAN_POINT ( 'NONE',  ( -16.52544592524342804, 4.483927247898546575, 46.04057627198103830 ) ) ;
#100519=CARTESIAN_POINT ( 'NONE',  ( 12.14591786802327356, -12.06949235617739191, 105.6260903946856899 ) ) ;
#100521=CARTESIAN_POINT ( 'NONE',  ( -0.05219959533936034679, 19.03943276465977164, 42.50109039468566152 ) ) ;
#100522=CARTESIAN_POINT ( 'NONE',  ( -19.03943276465977164, 0.05219959533909376836, 111.2489096053143669 ) ) ;
#100523=CARTESIAN_POINT ( 'NONE',  ( 5.049401038298161559, -19.05341960407611168, 57.70724293864769550 ) ) ;
#100524=CARTESIAN_POINT ( 'NONE',  ( 16.46253265017146816, 9.564922557961045513, 36.66775706135233293 ) ) ;
#100527=CARTESIAN_POINT ( 'NONE',  ( -16.52544592524335698, -4.483927247898792601, 58.95942372801902565 ) ) ;
#100528=CARTESIAN_POINT ( 'NONE',  ( -5.049401038297874678, -19.05341960407617918, 69.79275706135233293 ) ) ;
#100529=CARTESIAN_POINT ( 'NONE',  ( -16.52544592524335698, -4.483927247898792601, 68.95942372801901854 ) ) ;
#100531=CARTESIAN_POINT ( 'NONE',  ( -5.153800228976328057, -19.02544592524343514, 92.29057627198099567 ) ) ;
#100532=CARTESIAN_POINT ( 'NONE',  ( -5.823673210054116645, -21.52544592524344225, 112.2905762719810241 ) ) ;
#100533=CARTESIAN_POINT ( 'NONE',  ( 0.05219959533936267826, -19.03943276465977164, 80.00109039468567573 ) ) ;
#100534=CARTESIAN_POINT ( 'NONE',  ( 13.97604488694527802, 13.89961937509977652, 99.37390960531436690 ) ) ;
#100535=CARTESIAN_POINT ( 'NONE',  ( 19.02544592524343514, -5.153800228976328945, 33.54057627198102409 ) ) ;
#100536=CARTESIAN_POINT ( 'NONE',  ( 13.89961937509977652, -13.97604488694527269, 93.12390960531436690 ) ) ;
#100537=CARTESIAN_POINT ( 'NONE',  ( -14.29746914071049879, 8.314922557960819915, 45.83224293864769550 ) ) ;
#100538=CARTESIAN_POINT ( 'NONE',  ( -16.51473224551069308, -9.474510206698971260, 41.66557627198103120 ) ) ;
#100539=CARTESIAN_POINT ( 'NONE',  ( -9.474510206698720793, -16.51473224551083518, 54.58442372801899722 ) ) ;
#100540=CARTESIAN_POINT ( 'NONE',  ( -16.53943276465976808, 0.05219959533911058130, 86.24890960531436690 ) ) ;
#100541=CARTESIAN_POINT ( 'NONE',  ( -21.55341960407619339, 5.719274019375674811, 108.5427570613523756 ) ) ;
#100542=CARTESIAN_POINT ( 'NONE',  ( -16.46253265017160317, 9.564922557960807481, 50.83224293864770260 ) ) ;
#100543=CARTESIAN_POINT ( 'NONE',  ( 5.719274019375991003, -21.55341960407610458, 62.70724293864769550 ) ) ;
#100544=CARTESIAN_POINT ( 'NONE',  ( -16.53943276465976808, 0.05219959533911058130, 56.24890960531436690 ) ) ;
#100545=CARTESIAN_POINT ( 'NONE',  ( 15.80617190586769283, -15.72974639402175789, 110.6260903946857042 ) ) ;
#100546=CARTESIAN_POINT ( 'NONE',  ( 13.97604488694527802, 13.89961937509977652, 109.3739096053143669 ) ) ;
#100547=CARTESIAN_POINT ( 'NONE',  ( 19.05341960407611168, 5.049401038298154454, 113.9572429386477097 ) ) ;
#100548=CARTESIAN_POINT ( 'NONE',  ( -16.51473224551069308, -9.474510206698971260, 36.66557627198102409 ) ) ;
#100549=CARTESIAN_POINT ( 'NONE',  ( -16.52544592524342804, 4.483927247898546575, 116.0405762719810383 ) ) ;
#100550=CARTESIAN_POINT ( 'NONE',  ( -4.483927247898539470, -16.52544592524342804, 82.29057627198103830 ) ) ;
#100551=CARTESIAN_POINT ( 'NONE',  ( 5.719274019375991003, -21.55341960407610458, 97.70724293864772392 ) ) ;
#100552=CARTESIAN_POINT ( 'NONE',  ( -16.51473224551069308, -9.474510206698971260, 101.6655762719810241 ) ) ;
#100553=CARTESIAN_POINT ( 'NONE',  ( 21.53943276465977519, -0.05219959533907433946, 108.7489096053143669 ) ) ;
#100554=CARTESIAN_POINT ( 'NONE',  ( 9.474510206698971260, -16.51473224551069308, 102.9155762719810241 ) ) ;
#100555=CARTESIAN_POINT ( 'NONE',  ( 8.314922557960818139, 14.29746914071049879, 104.5822429386477097 ) ) ;
#100556=CARTESIAN_POINT ( 'NONE',  ( 0.05219959533937995610, -21.53943276465977519, 85.00109039468568994 ) ) ;
#100557=CARTESIAN_POINT ( 'NONE',  ( -0.05219959533907301413, -21.53943276465977519, 77.49890960531433848 ) ) ;
#100558=CARTESIAN_POINT ( 'NONE',  ( 16.88567814943162304, -6.947325034625676743, 106.2099887734741372 ) ) ;
#100559=CARTESIAN_POINT ( 'NONE',  ( -0.05219959533909027116, -19.03943276465977164, 52.49890960531436690 ) ) ;
#100561=CARTESIAN_POINT ( 'NONE',  ( -8.224510206698735004, -14.34966873604973081, 34.58442372801900433 ) ) ;
#100562=CARTESIAN_POINT ( 'NONE',  ( 12.14591786802309770, 12.06949235617756955, 114.3739096053143527 ) ) ;
#100564=CARTESIAN_POINT ( 'NONE',  ( 0.05219959533909260263, 19.03943276465977164, 59.99890960531436690 ) ) ;
#100565=CARTESIAN_POINT ( 'NONE',  ( 16.52544592524342804, -4.483927247898539470, 88.54057627198103830 ) ) ;
#100566=CARTESIAN_POINT ( 'NONE',  ( 15.72974639402199770, -15.80617190586745480, 28.12390960531435979 ) ) ;
#100567=CARTESIAN_POINT ( 'NONE',  ( -8.314922557960811034, -14.29746914071050412, 67.08224293864770971 ) ) ;
#100568=CARTESIAN_POINT ( 'NONE',  ( 9.474510206698729675, 16.51473224551082808, 112.0844237280190043 ) ) ;
#100569=CARTESIAN_POINT ( 'NONE',  ( 15.80617190586769283, -15.72974639402175789, 75.62609039468567573 ) ) ;
#100571=CARTESIAN_POINT ( 'NONE',  ( 9.474510206698971260, -16.51473224551069308, 112.9155762719810383 ) ) ;
#100572=CARTESIAN_POINT ( 'NONE',  ( 8.224510206698742110, 14.34966873604972548, 82.08442372801901854 ) ) ;
#100573=CARTESIAN_POINT ( 'NONE',  ( 16.51473224551069308, 9.474510206698969483, 34.16557627198102409 ) ) ;
#100574=CARTESIAN_POINT ( 'NONE',  ( -19.02544592524342804, 5.153800228976336051, 86.04057627198103830 ) ) ;
#100575=CARTESIAN_POINT ( 'NONE',  ( -0.05219959533907301413, -21.53943276465977519, 97.49890960531436690 ) ) ;
#100576=CARTESIAN_POINT ( 'NONE',  ( -16.52544592524335698, -4.483927247898792601, 28.95942372801902209 ) ) ;
#100577=CARTESIAN_POINT ( 'NONE',  ( -14.29746914071049879, 8.314922557960819915, 45.83224293864769550 ) ) ;
#100578=CARTESIAN_POINT ( 'NONE',  ( 10.72451020669871369, 18.67979575497193778, 67.08442372801901854 ) ) ;
#100579=CARTESIAN_POINT ( 'NONE',  ( -16.52544592524335698, -4.483927247898792601, 98.95942372801903275 ) ) ;
#100580=CARTESIAN_POINT ( 'NONE',  ( 16.31925111598457079, 7.325300261831474202, 27.33575461032749843 ) ) ;
#100582=CARTESIAN_POINT ( 'NONE',  ( -14.29746914071049879, 8.314922557960819915, 30.83224293864770260 ) ) ;
#100583=CARTESIAN_POINT ( 'NONE',  ( 8.314922557961029526, -14.29746914071037800, 55.41775706135234714 ) ) ;
#100584=CARTESIAN_POINT ( 'NONE',  ( -5.049401038298153566, 19.05341960407611168, 75.20724293864769550 ) ) ;
#100585=CARTESIAN_POINT ( 'NONE',  ( -13.97604488694527625, -13.89961937509977652, 91.87390960531432427 ) ) ;
#100586=CARTESIAN_POINT ( 'NONE',  ( 0.05219959533937995610, -21.53943276465977519, 85.00109039468568994 ) ) ;
#100587=CARTESIAN_POINT ( 'NONE',  ( -14.34966873604972548, 8.224510206698743886, 93.33442372801901854 ) ) ;
#100588=CARTESIAN_POINT ( 'NONE',  ( -0.05219959533910754901, -16.53943276465976808, 62.49890960531436690 ) ) ;
#100589=CARTESIAN_POINT ( 'NONE',  ( 0.05219959533909260263, 19.03943276465977164, 69.99890960531435269 ) ) ;
#100591=CARTESIAN_POINT ( 'NONE',  ( -9.474510206698720793, -16.51473224551083518, 109.5844237280190043 ) ) ;
#100592=CARTESIAN_POINT ( 'NONE',  ( -16.55341960407611168, -4.379528057220339221, 106.4572429386477097 ) ) ;
#100593=CARTESIAN_POINT ( 'NONE',  ( 16.51473224551069308, 9.474510206698969483, 79.16557627198103830 ) ) ;
#100594=CARTESIAN_POINT ( 'NONE',  ( -5.153800228976607833, 19.02544592524334988, 107.7094237280189759 ) ) ;
#100596=CARTESIAN_POINT ( 'NONE',  ( 18.67979575497194134, -10.72451020669871369, 105.8344237280190328 ) ) ;
#100597=CARTESIAN_POINT ( 'NONE',  ( -4.483927247898782831, 16.52544592524335698, 82.70942372801900433 ) ) ;
#100598=CARTESIAN_POINT ( 'NONE',  ( 13.97604488694548053, -13.89961937509957401, 90.62609039468567573 ) ) ;
#100599=CARTESIAN_POINT ( 'NONE',  ( 13.97604488694527802, 13.89961937509977652, 24.37390960531435624 ) ) ;
#100600=CARTESIAN_POINT ( 'NONE',  ( -0.05219959533934338120, 16.53943276465976808, 62.50109039468568284 ) ) ;
#100602=CARTESIAN_POINT ( 'NONE',  ( -13.97604488694547697, 13.89961937509957934, 58.12609039468566863 ) ) ;
#100603=CARTESIAN_POINT ( 'NONE',  ( -21.53943276465977519, -0.05219959533937600094, 98.75109039468568994 ) ) ;
#100604=CARTESIAN_POINT ( 'NONE',  ( -19.02544592524342804, 5.153800228976336051, 36.04057627198100988 ) ) ;
#100605=CARTESIAN_POINT ( 'NONE',  ( 13.97604488694527802, 13.89961937509977652, 84.37390960531433848 ) ) ;
#100606=CARTESIAN_POINT ( 'NONE',  ( -16.55341960407611168, -4.379528057220339221, 71.45724293864769550 ) ) ;
#100607=CARTESIAN_POINT ( 'NONE',  ( 15.80617190586769283, -15.72974639402175789, 95.62609039468568994 ) ) ;
#100608=CARTESIAN_POINT ( 'NONE',  ( 19.02544592524334988, 5.153800228976608722, 41.45942372801900433 ) ) ;
#100609=CARTESIAN_POINT ( 'NONE',  ( -5.153800228976607833, 19.02544592524334988, 37.70942372801899722 ) ) ;
#100610=CARTESIAN_POINT ( 'NONE',  ( -21.53943276465977519, 0.05219959533907696930, 41.24890960531435269 ) ) ;
#100611=CARTESIAN_POINT ( 'NONE',  ( 15.80617190586769283, -15.72974639402175789, 95.62609039468568994 ) ) ;
#100612=CARTESIAN_POINT ( 'NONE',  ( 16.46253265017160672, -9.564922557960803928, 73.33224293864769550 ) ) ;
#100614=CARTESIAN_POINT ( 'NONE',  ( -5.823673210054431948, 21.52544592524334988, 87.70942372801901854 ) ) ;
#100615=CARTESIAN_POINT ( 'NONE',  ( -18.67979575497178146, -10.72451020669898902, 56.66557627198103830 ) ) ;
#100616=CARTESIAN_POINT ( 'NONE',  ( 0.05219959533909260263, 19.03943276465977164, 84.99890960531436690 ) ) ;
#100617=CARTESIAN_POINT ( 'NONE',  ( -9.474510206698720793, -16.51473224551083518, 74.58442372801900433 ) ) ;
#100618=CARTESIAN_POINT ( 'NONE',  ( 19.02544592524343514, -5.153800228976328945, 103.5405762719809957 ) ) ;
#100619=CARTESIAN_POINT ( 'NONE',  ( 5.049401038297881783, 19.05341960407617563, 92.29275706135234714 ) ) ;
#100620=CARTESIAN_POINT ( 'NONE',  ( -8.314922557961024197, 14.29746914071037800, 42.91775706135235424 ) ) ;
#100621=CARTESIAN_POINT ( 'NONE',  ( 14.29746914071049879, -8.314922557960816363, 103.3322429386476955 ) ) ;
#100622=CARTESIAN_POINT ( 'NONE',  ( -9.564922557960796823, -16.46253265017161027, 67.08224293864769550 ) ) ;
#100623=CARTESIAN_POINT ( 'NONE',  ( 15.72974639402199770, -15.80617190586745480, 63.12390960531435979 ) ) ;
#100624=CARTESIAN_POINT ( 'NONE',  ( -4.483927247898782831, 16.52544592524335698, 37.70942372801900433 ) ) ;
#100625=CARTESIAN_POINT ( 'NONE',  ( 21.55341960407619695, -5.719274019375665929, 36.04275706135234714 ) ) ;
#100626=CARTESIAN_POINT ( 'NONE',  ( -10.81492255796105439, 18.62759615963255655, 82.91775706135234714 ) ) ;
#100627=B_SPLINE_CURVE_WITH_KNOTS ( 'NONE', 3,
 ( #65041, #124728, #172227, #171237, #157059, #3366, #123715, #18556, #185412, #189398, #46903, #49879, #34705, #156058, #96362, #108563, #186426, #112533, #174227, #35696, #20522, #47902, #109556, #32726, #94378, #79215, #140884, #160038, #101349, #9371, #70035, #113520 ),
 .UNSPECIFIED., .F., .F.,
 ( 4, 2, 2, 2, 2, 2, 2, 2, 2, 2, 2, 2, 2, 2, 2, 4 ),
 ( 2.195984522899319715E-17, 0.0003712461730036923074, 0.0007424923460073627138, 0.001113738519011033120, 0.001484984692014703310, 0.002227477038022051062, 0.002598723211025731009, 0.002969969384029411390, 0.003341215557033091772, 0.003712461730036772153, 0.004083707903040452100, 0.004454954076044132481, 0.004826200249047811995, 0.005197446422051492376, 0.005568692595055172757, 0.005939938768058853139 ),
 .UNSPECIFIED. ) ;
#100628=CARTESIAN_POINT ( 'NONE',  ( -14.34966873604972548, 8.224510206698743886, 83.33442372801903275 ) ) ;
#100629=CARTESIAN_POINT ( 'NONE',  ( -0.05219959533909027116, -19.03943276465977164, 77.49890960531435269 ) ) ;
#100630=CARTESIAN_POINT ( 'NONE',  ( -14.34966873604960291, -8.224510206698953496, 71.66557627198100988 ) ) ;
#100631=CARTESIAN_POINT ( 'NONE',  ( 4.379528057220092307, 16.55341960407617563, 107.2927570613523471 ) ) ;
#100632=CARTESIAN_POINT ( 'NONE',  ( 0.05219959533936267826, -19.03943276465977164, 55.00109039468566863 ) ) ;
#100633=CARTESIAN_POINT ( 'NONE',  ( -15.80617190586768217, 15.72974639402176855, 28.12609039468568284 ) ) ;
#100634=CARTESIAN_POINT ( 'NONE',  ( 0.05219959533910956823, 16.53943276465976808, 79.99890960531435269 ) ) ;
#100635=CARTESIAN_POINT ( 'NONE',  ( 16.51473224551069308, 9.474510206698969483, 104.1655762719810241 ) ) ;
#100636=CARTESIAN_POINT ( 'NONE',  ( -4.483927247898782831, 16.52544592524335698, 97.70942372801904696 ) ) ;
#100637=CARTESIAN_POINT ( 'NONE',  ( -21.52544592524334988, -5.823673210054445271, 73.95942372801901854 ) ) ;
#100638=CARTESIAN_POINT ( 'NONE',  ( -4.483927247898782831, 16.52544592524335698, 42.70942372801901854 ) ) ;
#100639=CARTESIAN_POINT ( 'NONE',  ( 18.62759615963255655, 10.81492255796105972, 36.66775706135234714 ) ) ;
#100640=CARTESIAN_POINT ( 'NONE',  ( -8.224510206698948167, 14.34966873604960824, 70.41557627198102409 ) ) ;
#100642=CARTESIAN_POINT ( 'NONE',  ( 21.53943276465977519, -0.05219959533907433946, 113.7489096053143527 ) ) ;
#100643=CARTESIAN_POINT ( 'NONE',  ( 17.49999999999999289, -4.640572885337604703, 28.13788164548842374 ) ) ;
#100644=CARTESIAN_POINT ( 'NONE',  ( 16.53943276465976808, -0.05219959533910856209, 48.74890960531435979 ) ) ;
#100645=CARTESIAN_POINT ( 'NONE',  ( -19.05341960407611168, -5.049401038298163336, 21.45724293864768839 ) ) ;
#100646=CARTESIAN_POINT ( 'NONE',  ( -0.05219959533907301413, -21.53943276465977519, 42.49890960531435979 ) ) ;
#100647=CARTESIAN_POINT ( 'NONE',  ( -4.379528057220328563, 16.55341960407611168, 80.20724293864769550 ) ) ;
#100648=CARTESIAN_POINT ( 'NONE',  ( 10.81492255796078972, 18.62759615963270932, 79.58224293864769550 ) ) ;
#100649=CARTESIAN_POINT ( 'NONE',  ( -13.89961937509977652, 13.97604488694528158, 85.62390960531433848 ) ) ;
#100650=CARTESIAN_POINT ( 'NONE',  ( -5.153800228976328057, -19.02544592524343514, 37.29057627198102409 ) ) ;
#100651=CARTESIAN_POINT ( 'NONE',  ( -13.97604488694547697, 13.89961937509957934, 78.12609039468567573 ) ) ;
#100652=CARTESIAN_POINT ( 'NONE',  ( 15.80617190586769283, -15.72974639402175789, 60.62609039468567573 ) ) ;
#100653=CARTESIAN_POINT ( 'NONE',  ( 18.62759615963271287, -10.81492255796078972, 58.33224293864768839 ) ) ;
#100654=CARTESIAN_POINT ( 'NONE',  ( 16.51473224551069308, 9.474510206698969483, 34.16557627198102409 ) ) ;
#100655=CARTESIAN_POINT ( 'NONE',  ( 13.97604488694527802, 13.89961937509977652, 74.37390960531436690 ) ) ;
#100657=CARTESIAN_POINT ( 'NONE',  ( 16.53943276465976808, 0.05219959533934440121, 51.25109039468568994 ) ) ;
#100658=CARTESIAN_POINT ( 'NONE',  ( 21.53943276465977519, 0.05219959533937863772, 31.25109039468568639 ) ) ;
#100659=CARTESIAN_POINT ( 'NONE',  ( -5.719274019375665041, -21.55341960407619695, 64.79275706135234714 ) ) ;
#100660=CARTESIAN_POINT ( 'NONE',  ( 13.97604488694527802, 13.89961937509977652, 109.3739096053143669 ) ) ;
#100661=CARTESIAN_POINT ( 'NONE',  ( 5.719274019375991003, -21.55341960407610458, 87.70724293864769550 ) ) ;
#100662=CARTESIAN_POINT ( 'NONE',  ( -10.81492255796105439, 18.62759615963255655, 27.91775706135234358 ) ) ;
#100663=CARTESIAN_POINT ( 'NONE',  ( -12.14591786802326823, 12.06949235617739902, 48.12609039468568284 ) ) ;
#100664=CARTESIAN_POINT ( 'NONE',  ( -15.72974639402197994, 15.80617190586746368, 55.62390960531436690 ) ) ;
#100665=CARTESIAN_POINT ( 'NONE',  ( -18.62759615963255300, -10.81492255796106328, 109.1677570613523613 ) ) ;
#100666=CARTESIAN_POINT ( 'NONE',  ( 16.46253265017160672, -9.564922557960803928, 58.33224293864769550 ) ) ;
#100667=CARTESIAN_POINT ( 'NONE',  ( -13.89961937509977652, 13.97604488694528158, 105.6239096053143527 ) ) ;
#100668=CARTESIAN_POINT ( 'NONE',  ( 19.02544592524343514, -5.153800228976328945, 93.54057627198102409 ) ) ;
#100669=CARTESIAN_POINT ( 'NONE',  ( 17.50000000000001066, 4.601506711240531899, 103.5269151853245262 ) ) ;
#100670=CARTESIAN_POINT ( 'NONE',  ( 19.02544592524334988, 5.153800228976608722, 71.45942372801900433 ) ) ;
#100671=CARTESIAN_POINT ( 'NONE',  ( 21.52544592524344225, -5.823673210054117533, 38.54057627198103120 ) ) ;
#100672=CARTESIAN_POINT ( 'NONE',  ( 16.55341960407611168, 4.379528057220329451, 23.95724293864769550 ) ) ;
#100673=CARTESIAN_POINT ( 'NONE',  ( -19.02544592524334988, -5.153800228976617603, 103.9594237280190043 ) ) ;
#100675=CARTESIAN_POINT ( 'NONE',  ( 13.97604488694548053, -13.89961937509957401, 20.62609039468567573 ) ) ;
#100676=CARTESIAN_POINT ( 'NONE',  ( 9.474510206698729675, 16.51473224551082808, 102.0844237280190043 ) ) ;
#100677=CARTESIAN_POINT ( 'NONE',  ( 9.564922557961047289, -16.46253265017146816, 40.41775706135234003 ) ) ;
#100679=CARTESIAN_POINT ( 'NONE',  ( -16.51473224551069308, -9.474510206698971260, 51.66557627198102409 ) ) ;
#100680=CARTESIAN_POINT ( 'NONE',  ( 0.05219959533910956823, 16.53943276465976808, 64.99890960531435269 ) ) ;
#100681=CARTESIAN_POINT ( 'NONE',  ( 9.564922557960805705, 16.46253265017160317, 39.58224293864768839 ) ) ;
#100682=CARTESIAN_POINT ( 'NONE',  ( -12.14591786802309592, -12.06949235617757132, 46.87390960531435979 ) ) ;
#100684=CARTESIAN_POINT ( 'NONE',  ( -8.314922557961024197, 14.29746914071037800, 102.9177570613523756 ) ) ;
#100685=CARTESIAN_POINT ( 'NONE',  ( -19.02544592524342804, 5.153800228976336051, 66.04057627198103830 ) ) ;
#100686=CARTESIAN_POINT ( 'NONE',  ( 19.05341960407617918, -5.049401038297876454, 31.04275706135232227 ) ) ;
#100687=CARTESIAN_POINT ( 'NONE',  ( 4.483927247898790824, -16.52544592524335698, 40.20942372801901854 ) ) ;
#100688=CARTESIAN_POINT ( 'NONE',  ( 15.80617190586746368, 15.72974639402197994, 54.37390960531435979 ) ) ;
#100689=CARTESIAN_POINT ( 'NONE',  ( 10.81492255796106328, -18.62759615963255655, 110.4177570613523756 ) ) ;
#100691=CARTESIAN_POINT ( 'NONE',  ( -13.89961937509977652, 13.97604488694528158, 60.62390960531436690 ) ) ;
#100692=CARTESIAN_POINT ( 'NONE',  ( 19.02544592524343514, -5.153800228976328945, 108.5405762719810383 ) ) ;
#100693=CARTESIAN_POINT ( 'NONE',  ( -5.153800228976328057, -19.02544592524343514, 97.29057627198099567 ) ) ;
#100695=CARTESIAN_POINT ( 'NONE',  ( 21.55341960407619695, -5.719274019375665929, 31.04275706135234714 ) ) ;
#100696=CARTESIAN_POINT ( 'NONE',  ( 14.29746914071049879, -8.314922557960816363, 98.33224293864769550 ) ) ;
#100697=CARTESIAN_POINT ( 'NONE',  ( -21.53943276465977519, 0.05219959533907696930, 91.24890960531436690 ) ) ;
#100698=CARTESIAN_POINT ( 'NONE',  ( 13.97604488694527802, 13.89961937509977652, 64.37390960531436690 ) ) ;
#100699=CARTESIAN_POINT ( 'NONE',  ( 9.474510206698971260, -16.51473224551069308, 77.91557627198103830 ) ) ;
#100700=CARTESIAN_POINT ( 'NONE',  ( -5.719274019375978568, 21.55341960407610458, 115.2072429386476955 ) ) ;
#100702=ORIENTED_EDGE ( 'NONE', *, *, #43792, .F. ) ;
#100703=CARTESIAN_POINT ( 'NONE',  ( 0.05219959533909260263, 19.03943276465977164, 79.99890960531436690 ) ) ;
#100705=CARTESIAN_POINT ( 'NONE',  ( 4.483927247898545687, 16.52544592524342804, 99.79057627198103830 ) ) ;
#100707=CARTESIAN_POINT ( 'NONE',  ( 16.46253265017146816, 9.564922557961045513, 91.66775706135234714 ) ) ;
#100708=CARTESIAN_POINT ( 'NONE',  ( 4.483927247898545687, 16.52544592524342804, 99.79057627198103830 ) ) ;
#100709=CARTESIAN_POINT ( 'NONE',  ( -18.62759615963255300, -10.81492255796106328, 74.16775706135231871 ) ) ;
#100710=CARTESIAN_POINT ( 'NONE',  ( 5.049401038298161559, -19.05341960407611168, 57.70724293864769550 ) ) ;
#100711=CARTESIAN_POINT ( 'NONE',  ( -18.67979575497193778, 10.72451020669871902, 28.33442372801902209 ) ) ;
#100712=CARTESIAN_POINT ( 'NONE',  ( -21.52544592524334988, -5.823673210054445271, 18.95942372801901143 ) ) ;
#100714=CARTESIAN_POINT ( 'NONE',  ( -16.51473224551069308, -9.474510206698971260, 76.66557627198103830 ) ) ;
#100715=CARTESIAN_POINT ( 'NONE',  ( -17.49999999999999645, -5.500000000000000888, 120.0000000000000142 ) ) ;
#100716=CARTESIAN_POINT ( 'NONE',  ( -19.05341960407617563, 5.049401038297882671, 113.5427570613523471 ) ) ;
#100717=CARTESIAN_POINT ( 'NONE',  ( 5.719274019375991003, -21.55341960407610458, 32.70724293864770260 ) ) ;
#100718=CARTESIAN_POINT ( 'NONE',  ( 10.72451020669871369, 18.67979575497193778, 57.08442372801901854 ) ) ;
#100719=CARTESIAN_POINT ( 'NONE',  ( -13.97604488694527625, -13.89961937509977652, 91.87390960531432427 ) ) ;
#100720=CARTESIAN_POINT ( 'NONE',  ( -19.05341960407617563, 5.049401038297882671, 93.54275706135234714 ) ) ;
#100721=CARTESIAN_POINT ( 'NONE',  ( 19.03943276465977164, -0.05219959533909143690, 43.74890960531435979 ) ) ;
#100722=CARTESIAN_POINT ( 'NONE',  ( 9.564922557960805705, 16.46253265017160317, 69.58224293864770971 ) ) ;
#100723=CARTESIAN_POINT ( 'NONE',  ( 14.29746914071049879, -8.314922557960816363, 93.33224293864769550 ) ) ;
#100724=CARTESIAN_POINT ( 'NONE',  ( -19.02544592524342804, 5.153800228976336051, 106.0405762719810241 ) ) ;
#100725=CARTESIAN_POINT ( 'NONE',  ( -8.314922557960811034, -14.29746914071050412, 92.08224293864769550 ) ) ;
#100726=CARTESIAN_POINT ( 'NONE',  ( 19.02544592524343514, -5.153800228976328945, 103.5405762719809957 ) ) ;
#100727=CARTESIAN_POINT ( 'NONE',  ( -8.224510206698948167, 14.34966873604960824, 40.41557627198103120 ) ) ;
#100728=CARTESIAN_POINT ( 'NONE',  ( -19.03943276465977164, 0.05219959533909376836, 46.24890960531435979 ) ) ;
#100730=CARTESIAN_POINT ( 'NONE',  ( 18.67979575497194134, -10.72451020669871369, 60.83442372801901854 ) ) ;
#100731=CARTESIAN_POINT ( 'NONE',  ( -19.05341960407617563, 5.049401038297882671, 83.54275706135233293 ) ) ;
#100732=CARTESIAN_POINT ( 'NONE',  ( -0.05219959533910754901, -16.53943276465976808, 47.49890960531435979 ) ) ;
#100733=CARTESIAN_POINT ( 'NONE',  ( 21.55341960407610458, 5.719274019375980345, 98.95724293864770971 ) ) ;
#100734=CARTESIAN_POINT ( 'NONE',  ( 21.53943276465977519, -0.05219959533907433946, 38.74890960531435979 ) ) ;
#100735=CARTESIAN_POINT ( 'NONE',  ( 8.224510206698953496, -14.34966873604960469, 77.91557627198102409 ) ) ;
#100736=CARTESIAN_POINT ( 'NONE',  ( -16.46253265017160317, 9.564922557960807481, 50.83224293864770260 ) ) ;
#100737=CARTESIAN_POINT ( 'NONE',  ( 16.55341960407611168, 4.379528057220329451, 28.95724293864769905 ) ) ;
#100738=CARTESIAN_POINT ( 'NONE',  ( 12.06949235617739724, 12.14591786802326823, 101.8760903946857042 ) ) ;
#100739=CARTESIAN_POINT ( 'NONE',  ( 8.224510206698742110, 14.34966873604972548, 72.08442372801899012 ) ) ;
#100740=CARTESIAN_POINT ( 'NONE',  ( 5.049401038297881783, 19.05341960407617563, 22.29275706135233648 ) ) ;
#100742=CARTESIAN_POINT ( 'NONE',  ( -13.97604488694527625, -13.89961937509977652, 106.8739096053143669 ) ) ;
#100743=CARTESIAN_POINT ( 'NONE',  ( -5.153800228976328057, -19.02544592524343514, 72.29057627198102409 ) ) ;
#100744=CARTESIAN_POINT ( 'NONE',  ( -16.51473224551069308, -9.474510206698971260, 31.66557627198102054 ) ) ;
#100745=CARTESIAN_POINT ( 'NONE',  ( -12.14591786802309592, -12.06949235617757132, 41.87390960531435979 ) ) ;
#100747=CARTESIAN_POINT ( 'NONE',  ( -5.049401038298153566, 19.05341960407611168, 100.2072429386476955 ) ) ;
#100748=CARTESIAN_POINT ( 'NONE',  ( -5.719274019375978568, 21.55341960407610458, 40.20724293864769550 ) ) ;
#100749=CARTESIAN_POINT ( 'NONE',  ( -16.53943276465976808, 0.05219959533911058130, 81.24890960531436690 ) ) ;
#100750=CARTESIAN_POINT ( 'NONE',  ( -14.29746914071037622, -8.314922557961029526, 24.16775706135235424 ) ) ;
#100751=CARTESIAN_POINT ( 'NONE',  ( 12.14591786802309770, 12.06949235617756955, 64.37390960531435269 ) ) ;
#100753=CARTESIAN_POINT ( 'NONE',  ( -0.05219959533936034679, 19.03943276465977164, 67.50109039468566152 ) ) ;
#100754=CARTESIAN_POINT ( 'NONE',  ( 19.03943276465977164, -0.05219959533909143690, 103.7489096053143669 ) ) ;
#100755=CARTESIAN_POINT ( 'NONE',  ( -19.05341960407617563, 5.049401038297882671, 78.54275706135233293 ) ) ;
#100757=CARTESIAN_POINT ( 'NONE',  ( -19.03943276465977164, -0.05219959533935918106, 108.7510903946856615 ) ) ;
#100758=CARTESIAN_POINT ( 'NONE',  ( 16.52544592524335698, 4.483927247898782831, 111.4594237280190328 ) ) ;
#100759=CARTESIAN_POINT ( 'NONE',  ( -5.153800228976607833, 19.02544592524334988, 67.70942372801900433 ) ) ;
#100760=CARTESIAN_POINT ( 'NONE',  ( -5.823673210054116645, -21.52544592524344225, 37.29057627198102409 ) ) ;
#100761=CARTESIAN_POINT ( 'NONE',  ( 0.05219959533937995610, -21.53943276465977519, 65.00109039468568994 ) ) ;
#100763=CARTESIAN_POINT ( 'NONE',  ( -8.224510206698735004, -14.34966873604973081, 19.58442372801901143 ) ) ;
#100764=CARTESIAN_POINT ( 'NONE',  ( 17.50000000000001066, 3.583808971632316265, 22.23472503527400690 ) ) ;
#100765=CARTESIAN_POINT ( 'NONE',  ( -19.02544592524342804, 5.153800228976336051, 81.04057627198103830 ) ) ;
#100767=CARTESIAN_POINT ( 'NONE',  ( 0.05219959533910956823, 16.53943276465976808, 84.99890960531436690 ) ) ;
#100768=CARTESIAN_POINT ( 'NONE',  ( 5.153800228976335163, 19.02544592524342804, 79.79057627198102409 ) ) ;
#100769=CARTESIAN_POINT ( 'NONE',  ( 5.049401038298161559, -19.05341960407611168, 92.70724293864769550 ) ) ;
#100770=CARTESIAN_POINT ( 'NONE',  ( -16.46253265017146816, -9.564922557961047289, 89.16775706135234714 ) ) ;
#100771=CARTESIAN_POINT ( 'NONE',  ( -21.52544592524343514, 5.823673210054127303, 81.04057627198102409 ) ) ;
#100772=CARTESIAN_POINT ( 'NONE',  ( 5.153800228976335163, 19.02544592524342804, 24.79057627198102765 ) ) ;
#100773=CARTESIAN_POINT ( 'NONE',  ( -9.564922557961040184, 16.46253265017147172, 62.91775706135233293 ) ) ;
#100774=CARTESIAN_POINT ( 'NONE',  ( -16.51473224551069308, -9.474510206698971260, 61.66557627198103120 ) ) ;
#100775=CARTESIAN_POINT ( 'NONE',  ( 13.89961937509977652, -13.97604488694527269, 98.12390960531433848 ) ) ;
#100776=ORIENTED_EDGE ( 'NONE', *, *, #175843, .T. ) ;
#100777=CARTESIAN_POINT ( 'NONE',  ( 10.81492255796078972, 18.62759615963270932, 104.5822429386477097 ) ) ;
#100778=CARTESIAN_POINT ( 'NONE',  ( 4.379528057220339221, -16.55341960407611168, 97.70724293864772392 ) ) ;
#100779=CARTESIAN_POINT ( 'NONE',  ( -19.02544592524342804, 5.153800228976336051, 81.04057627198103830 ) ) ;
#100780=CARTESIAN_POINT ( 'NONE',  ( -9.564922557961040184, 16.46253265017147172, 62.91775706135233293 ) ) ;
#100781=CARTESIAN_POINT ( 'NONE',  ( -18.62759615963270932, 10.81492255796079327, 85.83224293864768129 ) ) ;
#100782=CARTESIAN_POINT ( 'NONE',  ( -15.80617190586745835, -15.72974639402198527, 66.87390960531436690 ) ) ;
#100783=CARTESIAN_POINT ( 'NONE',  ( -16.55341960407611168, -4.379528057220339221, 36.45724293864768839 ) ) ;
#100784=CARTESIAN_POINT ( 'NONE',  ( -21.53943276465977519, -0.05219959533937600094, 108.7510903946857042 ) ) ;
#100785=CARTESIAN_POINT ( 'NONE',  ( 4.483927247898790824, -16.52544592524335698, 70.20942372801904696 ) ) ;
#100786=CARTESIAN_POINT ( 'NONE',  ( 0.05219959533909260263, 19.03943276465977164, 94.99890960531436690 ) ) ;
#100787=CARTESIAN_POINT ( 'NONE',  ( 19.05341960407611168, 5.049401038298154454, 28.95724293864769550 ) ) ;
#100788=CARTESIAN_POINT ( 'NONE',  ( -21.53943276465977519, -0.05219959533937600094, 38.75109039468567573 ) ) ;
#100789=CARTESIAN_POINT ( 'NONE',  ( -10.81492255796105439, 18.62759615963255655, 57.91775706135234714 ) ) ;
#100790=CARTESIAN_POINT ( 'NONE',  ( -19.02544592524342804, 5.153800228976336051, 56.04057627198100988 ) ) ;
#100791=CARTESIAN_POINT ( 'NONE',  ( -0.05219959533937732626, 21.53943276465977519, 32.50109039468568284 ) ) ;
#100792=CARTESIAN_POINT ( 'NONE',  ( 13.89961937509957401, 13.97604488694547697, 76.87609039468566152 ) ) ;
#100793=CARTESIAN_POINT ( 'NONE',  ( -13.89961937509957401, -13.97604488694547875, 69.37609039468564731 ) ) ;
#100794=CARTESIAN_POINT ( 'NONE',  ( -5.049401038298153566, 19.05341960407611168, 45.20724293864769550 ) ) ;
#100795=CARTESIAN_POINT ( 'NONE',  ( 0.05219959533934541429, -16.53943276465976808, 70.00109039468568994 ) ) ;
#100796=CARTESIAN_POINT ( 'NONE',  ( -5.153800228976328057, -19.02544592524343514, 52.29057627198100988 ) ) ;
#100798=CARTESIAN_POINT ( 'NONE',  ( -5.049401038298153566, 19.05341960407611168, 100.2072429386476955 ) ) ;
#100799=CARTESIAN_POINT ( 'NONE',  ( -0.05219959533909027116, -19.03943276465977164, 37.49890960531436690 ) ) ;
#100800=CARTESIAN_POINT ( 'NONE',  ( 21.52544592524344225, -5.823673210054117533, 73.54057627198102409 ) ) ;
#100801=CARTESIAN_POINT ( 'NONE',  ( -4.379528057220086978, -16.55341960407618274, 64.79275706135234714 ) ) ;
#100802=CARTESIAN_POINT ( 'NONE',  ( -0.05219959533937732626, 21.53943276465977519, 112.5010903946857042 ) ) ;
#100803=EDGE_CURVE ( 'NONE', #70081, #35831, #39415, .T. ) ;
#100804=CARTESIAN_POINT ( 'NONE',  ( -0.05219959533909027116, -19.03943276465977164, 57.49890960531435979 ) ) ;
#100805=CARTESIAN_POINT ( 'NONE',  ( 8.224510206698953496, -14.34966873604960469, 42.91557627198103120 ) ) ;
#100806=CARTESIAN_POINT ( 'NONE',  ( -16.55341960407611168, -4.379528057220339221, 76.45724293864769550 ) ) ;
#100807=CARTESIAN_POINT ( 'NONE',  ( 19.02544592524343514, -5.153800228976328945, 78.54057627198099567 ) ) ;
#100808=CARTESIAN_POINT ( 'NONE',  ( 15.80617190586769283, -15.72974639402175789, 35.62609039468568994 ) ) ;
#100809=CARTESIAN_POINT ( 'NONE',  ( -13.97604488694527625, -13.89961937509977652, 91.87390960531432427 ) ) ;
#100810=CARTESIAN_POINT ( 'NONE',  ( -5.823673210054431948, 21.52544592524334988, 97.70942372801904696 ) ) ;
#100811=CARTESIAN_POINT ( 'NONE',  ( 14.34966873604972726, -8.224510206698740333, 60.83442372801901854 ) ) ;
#100812=CARTESIAN_POINT ( 'NONE',  ( -5.153800228976328057, -19.02544592524343514, 107.2905762719810383 ) ) ;
#100814=CARTESIAN_POINT ( 'NONE',  ( -10.72451020669898014, 18.67979575497178502, 95.41557627198102409 ) ) ;
#100815=CARTESIAN_POINT ( 'NONE',  ( -4.483927247898539470, -16.52544592524342804, 42.29057627198103120 ) ) ;
#100816=CARTESIAN_POINT ( 'NONE',  ( 9.474510206698971260, -16.51473224551069308, 37.91557627198102409 ) ) ;
#100817=CARTESIAN_POINT ( 'NONE',  ( 12.06949235617739724, 12.14591786802326823, 46.87609039468568994 ) ) ;
#100818=CARTESIAN_POINT ( 'NONE',  ( -14.34966873604960291, -8.224510206698953496, 61.66557627198103120 ) ) ;
#100819=CARTESIAN_POINT ( 'NONE',  ( 19.03943276465977164, -0.05219959533909143690, 108.7489096053143527 ) ) ;
#100820=CARTESIAN_POINT ( 'NONE',  ( -18.62759615963270932, 10.81492255796079327, 25.83224293864769194 ) ) ;
#100821=CARTESIAN_POINT ( 'NONE',  ( 0.05219959533936267826, -19.03943276465977164, 30.00109039468566863 ) ) ;
#100822=CARTESIAN_POINT ( 'NONE',  ( -0.05219959533910754901, -16.53943276465976808, 102.4989096053143811 ) ) ;
#100823=CARTESIAN_POINT ( 'NONE',  ( 9.474510206698971260, -16.51473224551069308, 102.9155762719810241 ) ) ;
#100824=ORIENTED_EDGE ( 'NONE', *, *, #82301, .F. ) ;
#100825=CARTESIAN_POINT ( 'NONE',  ( -4.379528057220086978, -16.55341960407618274, 54.79275706135235424 ) ) ;
#100826=CARTESIAN_POINT ( 'NONE',  ( 9.474510206698971260, -16.51473224551069308, 57.91557627198103120 ) ) ;
#100828=CARTESIAN_POINT ( 'NONE',  ( -13.89961937509957401, -13.97604488694547875, 59.37609039468566863 ) ) ;
#100829=CARTESIAN_POINT ( 'NONE',  ( 16.53943276465976808, 0.05219959533934440121, 91.25109039468568994 ) ) ;
#100830=CARTESIAN_POINT ( 'NONE',  ( 13.89961937509957401, 13.97604488694547697, 91.87609039468567573 ) ) ;
#100831=CARTESIAN_POINT ( 'NONE',  ( 18.67979575497194134, -10.72451020669871369, 65.83442372801900433 ) ) ;
#100832=CARTESIAN_POINT ( 'NONE',  ( -0.05219959533909027116, -19.03943276465977164, 72.49890960531435269 ) ) ;
#100833=CARTESIAN_POINT ( 'NONE',  ( -18.62759615963270932, 10.81492255796079327, 95.83224293864770971 ) ) ;
#100834=CARTESIAN_POINT ( 'NONE',  ( 16.52544592524342804, -4.483927247898539470, 108.5405762719810241 ) ) ;
#100835=CARTESIAN_POINT ( 'NONE',  ( 9.564922557961047289, -16.46253265017146816, 75.41775706135234714 ) ) ;
#100836=CARTESIAN_POINT ( 'NONE',  ( 5.719274019375991003, -21.55341960407610458, 82.70724293864770971 ) ) ;
#100837=CARTESIAN_POINT ( 'NONE',  ( -13.97604488694547697, 13.89961937509957934, 43.12609039468566152 ) ) ;
#100838=CARTESIAN_POINT ( 'NONE',  ( 18.56399227203342406, 5.499999999999960920, 96.47830131249901342 ) ) ;
#100840=CARTESIAN_POINT ( 'NONE',  ( -21.53943276465977519, 0.05219959533907696930, 86.24890960531436690 ) ) ;
#100842=CARTESIAN_POINT ( 'NONE',  ( 0.05219959533909260263, 19.03943276465977164, 64.99890960531436690 ) ) ;
#100844=CARTESIAN_POINT ( 'NONE',  ( 16.51473224551083163, -9.474510206698727899, 110.8344237280190043 ) ) ;
#100846=CARTESIAN_POINT ( 'NONE',  ( -13.97604488694527625, -13.89961937509977652, 41.87390960531435979 ) ) ;
#100847=CARTESIAN_POINT ( 'NONE',  ( -21.53943276465977519, 0.05219959533907696930, 106.2489096053143811 ) ) ;
#100848=CARTESIAN_POINT ( 'NONE',  ( 16.53943276465976808, -0.05219959533910856209, 48.74890960531435979 ) ) ;
#100849=CARTESIAN_POINT ( 'NONE',  ( 5.823673210054444382, -21.52544592524334988, 75.20942372801901854 ) ) ;
#100850=CARTESIAN_POINT ( 'NONE',  ( 16.52544592524335698, 4.483927247898782831, 21.45942372801901499 ) ) ;
#100851=CARTESIAN_POINT ( 'NONE',  ( -9.474510206698720793, -16.51473224551083518, 34.58442372801899722 ) ) ;
#100852=CARTESIAN_POINT ( 'NONE',  ( 14.34966873604960469, 8.224510206698951720, 24.16557627198103120 ) ) ;
#100853=CARTESIAN_POINT ( 'NONE',  ( -21.55341960407619339, 5.719274019375674811, 33.54275706135234714 ) ) ;
#100854=CARTESIAN_POINT ( 'NONE',  ( -21.52544592524334988, -5.823673210054445271, 18.95942372801901143 ) ) ;
#100855=CARTESIAN_POINT ( 'NONE',  ( 18.67979575497178502, 10.72451020669898547, 64.16557627198102409 ) ) ;
#100856=CARTESIAN_POINT ( 'NONE',  ( -5.049401038297874678, -19.05341960407617918, 89.79275706135230450 ) ) ;
#100857=CARTESIAN_POINT ( 'NONE',  ( -13.97604488694547697, 13.89961937509957934, 68.12609039468563310 ) ) ;
#100858=CARTESIAN_POINT ( 'NONE',  ( -5.823673210054431948, 21.52544592524334988, 77.70942372801900433 ) ) ;
#100859=CARTESIAN_POINT ( 'NONE',  ( 5.153800228976615827, -19.02544592524334988, 50.20942372801897591 ) ) ;
#100860=CARTESIAN_POINT ( 'NONE',  ( 4.483927247898545687, 16.52544592524342804, 114.7905762719810383 ) ) ;
#100861=CARTESIAN_POINT ( 'NONE',  ( 18.62759615963271287, -10.81492255796078972, 43.33224293864769550 ) ) ;
#100862=CARTESIAN_POINT ( 'NONE',  ( 14.34966873604960469, 8.224510206698951720, 49.16557627198102409 ) ) ;
#100863=CARTESIAN_POINT ( 'NONE',  ( -18.22780087662123805, 5.499999999999981348, 96.01763182126897789 ) ) ;
#100864=CARTESIAN_POINT ( 'NONE',  ( -9.474510206698720793, -16.51473224551083518, 19.58442372801899722 ) ) ;
#100865=CARTESIAN_POINT ( 'NONE',  ( -16.53943276465976808, -0.05219959533934237506, 83.75109039468568994 ) ) ;
#100866=CARTESIAN_POINT ( 'NONE',  ( 4.379528057220339221, -16.55341960407611168, 37.70724293864769550 ) ) ;
#100867=CARTESIAN_POINT ( 'NONE',  ( 21.52544592524334988, 5.823673210054432836, 76.45942372801901854 ) ) ;
#100868=CARTESIAN_POINT ( 'NONE',  ( 15.72974639402176855, 15.80617190586768217, 81.87609039468568994 ) ) ;
#100869=CARTESIAN_POINT ( 'NONE',  ( -10.72451020669898014, 18.67979575497178502, 85.41557627198102409 ) ) ;
#100870=CARTESIAN_POINT ( 'NONE',  ( 9.474510206698971260, -16.51473224551069308, 32.91557627198102409 ) ) ;
#100871=CARTESIAN_POINT ( 'NONE',  ( -18.67979575497193778, 10.72451020669871902, 58.33442372801901143 ) ) ;
#100872=CARTESIAN_POINT ( 'NONE',  ( 5.049401038298161559, -19.05341960407611168, 37.70724293864768839 ) ) ;
#100873=CARTESIAN_POINT ( 'NONE',  ( -16.46253265017160317, 9.564922557960807481, 50.83224293864770260 ) ) ;
#100874=CARTESIAN_POINT ( 'NONE',  ( -12.06949235617756955, 12.14591786802309770, 95.62390960531436690 ) ) ;
#100875=CARTESIAN_POINT ( 'NONE',  ( -13.97604488694527625, -13.89961937509977652, 96.87390960531433848 ) ) ;
#100876=CARTESIAN_POINT ( 'NONE',  ( 16.55341960407611168, 4.379528057220329451, 43.95724293864769550 ) ) ;
#100877=CARTESIAN_POINT ( 'NONE',  ( 8.314922557960818139, 14.29746914071049879, 114.5822429386477097 ) ) ;
#100878=CARTESIAN_POINT ( 'NONE',  ( -18.62759615963270932, 10.81492255796079327, 80.83224293864769550 ) ) ;
#100879=CARTESIAN_POINT ( 'NONE',  ( -5.823673210054431948, 21.52544592524334988, 27.70942372801901854 ) ) ;
#100881=CARTESIAN_POINT ( 'NONE',  ( 12.14591786802327356, -12.06949235617739191, 20.62609039468568639 ) ) ;
#100882=CARTESIAN_POINT ( 'NONE',  ( -10.72451020669898014, 18.67979575497178502, 70.41557627198102409 ) ) ;
#100883=CARTESIAN_POINT ( 'NONE',  ( -5.719274019375665041, -21.55341960407619695, 99.79275706135234714 ) ) ;
#100884=CARTESIAN_POINT ( 'NONE',  ( -5.049401038298153566, 19.05341960407611168, 85.20724293864766707 ) ) ;
#100885=CARTESIAN_POINT ( 'NONE',  ( 15.80617190586769283, -15.72974639402175789, 35.62609039468568994 ) ) ;
#100886=CARTESIAN_POINT ( 'NONE',  ( 5.153800228976335163, 19.02544592524342804, 109.7905762719810099 ) ) ;
#100887=CARTESIAN_POINT ( 'NONE',  ( 8.314922557961029526, -14.29746914071037800, 85.41775706135236135 ) ) ;
#100888=CARTESIAN_POINT ( 'NONE',  ( 0.05219959533937995610, -21.53943276465977519, 75.00109039468568994 ) ) ;
#100889=CARTESIAN_POINT ( 'NONE',  ( -0.05219959533937732626, 21.53943276465977519, 112.5010903946857042 ) ) ;
#100890=CARTESIAN_POINT ( 'NONE',  ( 16.55341960407618274, -4.379528057220086978, 81.04275706135236135 ) ) ;
#100891=CARTESIAN_POINT ( 'NONE',  ( -15.72974639402176322, -15.80617190586768395, 24.37609039468567573 ) ) ;
#100892=CARTESIAN_POINT ( 'NONE',  ( 19.05341960407611168, 5.049401038298154454, 28.95724293864769550 ) ) ;
#100893=CARTESIAN_POINT ( 'NONE',  ( 21.53943276465977519, 0.05219959533937863772, 86.25109039468568994 ) ) ;
#100894=CARTESIAN_POINT ( 'NONE',  ( 0.05219959533909260263, 19.03943276465977164, 89.99890960531436690 ) ) ;
#100895=CARTESIAN_POINT ( 'NONE',  ( 18.67979575497178502, 10.72451020669898547, 84.16557627198103830 ) ) ;
#100896=CARTESIAN_POINT ( 'NONE',  ( -16.46253265017146816, -9.564922557961047289, 54.16775706135234003 ) ) ;
#100897=CARTESIAN_POINT ( 'NONE',  ( 17.72517630441461378, -5.499999999999979572, 88.42175719257600974 ) ) ;
#100898=CARTESIAN_POINT ( 'NONE',  ( 21.53943276465977519, -0.05219959533907433946, 48.74890960531435979 ) ) ;
#100899=CARTESIAN_POINT ( 'NONE',  ( -13.97604488694527625, -13.89961937509977652, 91.87390960531432427 ) ) ;
#100900=CARTESIAN_POINT ( 'NONE',  ( -0.05219959533910754901, -16.53943276465976808, 47.49890960531435979 ) ) ;
#100902=CARTESIAN_POINT ( 'NONE',  ( -16.51473224551082808, 9.474510206698731452, 73.33442372801900433 ) ) ;
#100903=CARTESIAN_POINT ( 'NONE',  ( -17.44279575226824264, 5.990770900252420539, 105.8355756751431755 ) ) ;
#100904=CARTESIAN_POINT ( 'NONE',  ( -5.153800228976607833, 19.02544592524334988, 107.7094237280189759 ) ) ;
#100905=CARTESIAN_POINT ( 'NONE',  ( -10.72451020669898014, 18.67979575497178502, 90.41557627198103830 ) ) ;
#100906=CARTESIAN_POINT ( 'NONE',  ( -4.483927247898539470, -16.52544592524342804, 67.29057627198103830 ) ) ;
#100907=CARTESIAN_POINT ( 'NONE',  ( -19.05341960407611168, -5.049401038298163336, 96.45724293864769550 ) ) ;
#100908=CARTESIAN_POINT ( 'NONE',  ( -8.224510206698735004, -14.34966873604973081, 44.58442372801901854 ) ) ;
#100909=CARTESIAN_POINT ( 'NONE',  ( 9.564922557960805705, 16.46253265017160317, 59.58224293864769550 ) ) ;
#100910=CARTESIAN_POINT ( 'NONE',  ( 10.81492255796106328, -18.62759615963255655, 25.41775706135235779 ) ) ;
#100911=CARTESIAN_POINT ( 'NONE',  ( -19.02544592524334988, -5.153800228976617603, 93.95942372801900433 ) ) ;
#100912=CARTESIAN_POINT ( 'NONE',  ( -16.46253265017160317, 9.564922557960807481, 90.83224293864769550 ) ) ;
#100913=CARTESIAN_POINT ( 'NONE',  ( -16.46253265017160317, 9.564922557960807481, 75.83224293864769550 ) ) ;
#100914=CARTESIAN_POINT ( 'NONE',  ( -15.80617190586745835, -15.72974639402198527, 81.87390960531435269 ) ) ;
#100915=CARTESIAN_POINT ( 'NONE',  ( 19.03943276465977164, -0.05219959533909143690, 43.74890960531435979 ) ) ;
#100917=CARTESIAN_POINT ( 'NONE',  ( -16.53943276465976808, 0.05219959533911058130, 51.24890960531436690 ) ) ;
#100918=CARTESIAN_POINT ( 'NONE',  ( 19.02544592524343514, -5.153800228976328945, 103.5405762719809957 ) ) ;
#100919=LINE ( 'NONE', #181778, #115366 ) ;
#100920=CARTESIAN_POINT ( 'NONE',  ( 16.46253265017146816, 9.564922557961045513, 71.66775706135233293 ) ) ;
#100921=CARTESIAN_POINT ( 'NONE',  ( 21.53943276465977519, -0.05219959533907433946, 93.74890960531436690 ) ) ;
#100922=CARTESIAN_POINT ( 'NONE',  ( 16.51473224551083163, -9.474510206698727899, 45.83442372801900433 ) ) ;
#100923=CARTESIAN_POINT ( 'NONE',  ( -16.46253265017160317, 9.564922557960807481, 95.83224293864769550 ) ) ;
#100924=CARTESIAN_POINT ( 'NONE',  ( 17.97058386085786097, 5.500000000000042633, 76.50390968646217971 ) ) ;
#100925=CARTESIAN_POINT ( 'NONE',  ( -0.05219959533907301413, -21.53943276465977519, 42.49890960531435979 ) ) ;
#100926=CARTESIAN_POINT ( 'NONE',  ( -16.51473224551069308, -9.474510206698971260, 91.66557627198103830 ) ) ;
#100927=EDGE_CURVE ( 'NONE', #167324, #197337, #107101, .T. ) ;
#100928=CARTESIAN_POINT ( 'NONE',  ( 18.62759615963255655, 10.81492255796105972, 61.66775706135235424 ) ) ;
#100929=CARTESIAN_POINT ( 'NONE',  ( 5.153800228976335163, 19.02544592524342804, 34.79057627198102409 ) ) ;
#100930=CARTESIAN_POINT ( 'NONE',  ( 16.53943276465976808, -0.05219959533910856209, 73.74890960531433848 ) ) ;
#100932=CARTESIAN_POINT ( 'NONE',  ( -14.34966873604972548, 8.224510206698743886, 28.33442372801902209 ) ) ;
#100933=CARTESIAN_POINT ( 'NONE',  ( 18.62759615963255655, 10.81492255796105972, 46.66775706135234714 ) ) ;
#100934=EDGE_LOOP ( 'NONE', ( #66905, #117342, #77811, #45498, #74370, #130546, #69374, #95850 ) ) ;
#100935=CARTESIAN_POINT ( 'NONE',  ( -16.51473224551069308, -9.474510206698971260, 111.6655762719810383 ) ) ;
#100936=CARTESIAN_POINT ( 'NONE',  ( 0.05219959533936267826, -19.03943276465977164, 65.00109039468567573 ) ) ;
#100938=CARTESIAN_POINT ( 'NONE',  ( 15.72974639402176855, 15.80617190586768217, 21.87609039468567573 ) ) ;
#100939=CARTESIAN_POINT ( 'NONE',  ( -5.049401038298153566, 19.05341960407611168, 55.20724293864769550 ) ) ;
#100941=CARTESIAN_POINT ( 'NONE',  ( 13.89961937509957401, 13.97604488694547697, 21.87609039468566152 ) ) ;
#100942=CARTESIAN_POINT ( 'NONE',  ( 13.97604488694527802, 13.89961937509977652, 44.37390960531435269 ) ) ;
#100943=CARTESIAN_POINT ( 'NONE',  ( -9.564922557961040184, 16.46253265017147172, 22.91775706135233648 ) ) ;
#100944=CARTESIAN_POINT ( 'NONE',  ( 4.483927247898790824, -16.52544592524335698, 95.20942372801903275 ) ) ;
#100945=CARTESIAN_POINT ( 'NONE',  ( -13.97604488694527625, -13.89961937509977652, 106.8739096053143669 ) ) ;
#100946=CARTESIAN_POINT ( 'NONE',  ( 10.81492255796106328, -18.62759615963255655, 70.41775706135236135 ) ) ;
#100948=CARTESIAN_POINT ( 'NONE',  ( 19.05341960407611168, 5.049401038298154454, 113.9572429386477097 ) ) ;
#100950=CARTESIAN_POINT ( 'NONE',  ( 4.483927247898790824, -16.52544592524335698, 70.20942372801904696 ) ) ;
#100951=CARTESIAN_POINT ( 'NONE',  ( 21.52544592524334988, 5.823673210054432836, 71.45942372801901854 ) ) ;
#100952=CARTESIAN_POINT ( 'NONE',  ( 15.80617190586769283, -15.72974639402175789, 105.6260903946856899 ) ) ;
#100954=CARTESIAN_POINT ( 'NONE',  ( 16.53943276465976808, 0.05219959533934440121, 41.25109039468568284 ) ) ;
#100955=CARTESIAN_POINT ( 'NONE',  ( -0.05219959533909027116, -19.03943276465977164, 92.49890960531436690 ) ) ;
#100956=CARTESIAN_POINT ( 'NONE',  ( 5.153800228976335163, 19.02544592524342804, 104.7905762719809957 ) ) ;
#100958=CARTESIAN_POINT ( 'NONE',  ( 16.20579543436682002, 7.371946100354975329, 43.06520834171879386 ) ) ;
#100959=CARTESIAN_POINT ( 'NONE',  ( 16.46253265017160672, -9.564922557960803928, 43.33224293864769550 ) ) ;
#100960=CARTESIAN_POINT ( 'NONE',  ( 21.53943276465977519, -0.05219959533907433946, 38.74890960531435979 ) ) ;
#100962=CARTESIAN_POINT ( 'NONE',  ( 16.53943276465976808, 0.05219959533934440121, 111.2510903946856899 ) ) ;
#100963=CARTESIAN_POINT ( 'NONE',  ( -4.483927247898539470, -16.52544592524342804, 77.29057627198102409 ) ) ;
#100964=CARTESIAN_POINT ( 'NONE',  ( -9.564922557960796823, -16.46253265017161027, 77.08224293864769550 ) ) ;
#100965=CARTESIAN_POINT ( 'NONE',  ( -21.55341960407619339, 5.719274019375674811, 108.5427570613523756 ) ) ;
#100966=CARTESIAN_POINT ( 'NONE',  ( -19.02544592524342804, 5.153800228976336051, 31.04057627198102409 ) ) ;
#100967=CARTESIAN_POINT ( 'NONE',  ( 16.52544592524342804, -4.483927247898539470, 83.54057627198102409 ) ) ;
#100968=CARTESIAN_POINT ( 'NONE',  ( -21.53943276465977519, -0.05219959533937600094, 43.75109039468568284 ) ) ;
#100969=CARTESIAN_POINT ( 'NONE',  ( 21.53943276465977519, -0.05219959533907433946, 88.74890960531436690 ) ) ;
#100970=CARTESIAN_POINT ( 'NONE',  ( -0.05219959533936034679, 19.03943276465977164, 57.50109039468566863 ) ) ;
#100972=CARTESIAN_POINT ( 'NONE',  ( 13.97604488694527802, 13.89961937509977652, 94.37390960531436690 ) ) ;
#100973=CARTESIAN_POINT ( 'NONE',  ( 8.314922557960818139, 14.29746914071049879, 59.58224293864770260 ) ) ;
#100975=CARTESIAN_POINT ( 'NONE',  ( -14.29746914071049879, 8.314922557960819915, 45.83224293864769550 ) ) ;
#100976=CARTESIAN_POINT ( 'NONE',  ( 16.52544592524342804, -4.483927247898539470, 28.54057627198103120 ) ) ;
#100977=CARTESIAN_POINT ( 'NONE',  ( 13.97604488694548053, -13.89961937509957401, 85.62609039468568994 ) ) ;
#100978=CARTESIAN_POINT ( 'NONE',  ( 18.22780087662122384, -5.500000000000022204, 101.0154010532610869 ) ) ;
#100979=CARTESIAN_POINT ( 'NONE',  ( -21.52544592524343514, 5.823673210054127303, 26.04057627198103475 ) ) ;
#100980=CARTESIAN_POINT ( 'NONE',  ( -12.06949235617756955, 12.14591786802309770, 90.62390960531436690 ) ) ;
#100982=CARTESIAN_POINT ( 'NONE',  ( -13.89961937509977652, 13.97604488694528158, 50.62390960531435979 ) ) ;
#100983=CARTESIAN_POINT ( 'NONE',  ( -5.719274019375978568, 21.55341960407610458, 50.20724293864769550 ) ) ;
#100984=CARTESIAN_POINT ( 'NONE',  ( -19.03943276465977164, 0.05219959533909376836, 31.24890960531435979 ) ) ;
#100985=CARTESIAN_POINT ( 'NONE',  ( -14.34966873604972548, 8.224510206698743886, 78.33442372801901854 ) ) ;
#100986=CARTESIAN_POINT ( 'NONE',  ( -16.51473224551069308, -9.474510206698971260, 66.66557627198102409 ) ) ;
#100987=CARTESIAN_POINT ( 'NONE',  ( 13.89961937509957401, 13.97604488694547697, 41.87609039468566152 ) ) ;
#100988=CARTESIAN_POINT ( 'NONE',  ( 18.62759615963255655, 10.81492255796105972, 66.66775706135234714 ) ) ;
#100989=CARTESIAN_POINT ( 'NONE',  ( 10.81492255796078972, 18.62759615963270932, 34.58224293864770260 ) ) ;
#100990=CARTESIAN_POINT ( 'NONE',  ( -16.55341960407611168, -4.379528057220339221, 106.4572429386477097 ) ) ;
#100991=CARTESIAN_POINT ( 'NONE',  ( 9.474510206698729675, 16.51473224551082808, 87.08442372801900433 ) ) ;
#100994=CARTESIAN_POINT ( 'NONE',  ( 18.62759615963271287, -10.81492255796078972, 53.33224293864769550 ) ) ;
#100995=CARTESIAN_POINT ( 'NONE',  ( -13.97604488694527625, -13.89961937509977652, 21.87390960531435979 ) ) ;
#100996=CARTESIAN_POINT ( 'NONE',  ( -18.62759615963255300, -10.81492255796106328, 89.16775706135236135 ) ) ;
#100997=CARTESIAN_POINT ( 'NONE',  ( -16.55341960407611168, -4.379528057220339221, 46.45724293864769550 ) ) ;
#100998=CARTESIAN_POINT ( 'NONE',  ( 4.483927247898790824, -16.52544592524335698, 65.20942372801901854 ) ) ;
#100999=CARTESIAN_POINT ( 'NONE',  ( -4.379528057220328563, 16.55341960407611168, 50.20724293864769550 ) ) ;
#101000=CARTESIAN_POINT ( 'NONE',  ( -21.52544592524343514, 5.823673210054127303, 76.04057627198102409 ) ) ;
#101001=CARTESIAN_POINT ( 'NONE',  ( 15.72974639402199770, -15.80617190586745480, 73.12390960531436690 ) ) ;
#101003=CARTESIAN_POINT ( 'NONE',  ( 5.153800228976335163, 19.02544592524342804, 109.7905762719810099 ) ) ;
#101004=CARTESIAN_POINT ( 'NONE',  ( 12.14591786802309770, 12.06949235617756955, 84.37390960531438111 ) ) ;
#101005=CARTESIAN_POINT ( 'NONE',  ( 9.564922557960805705, 16.46253265017160317, 59.58224293864769550 ) ) ;
#101006=CARTESIAN_POINT ( 'NONE',  ( -19.03943276465977164, 0.05219959533909376836, 31.24890960531435979 ) ) ;
#101009=VERTEX_POINT ( 'NONE', #2010 ) ;
#101010=CARTESIAN_POINT ( 'NONE',  ( 16.53943276465976808, 0.05219959533934440121, 76.25109039468568994 ) ) ;
#101011=CARTESIAN_POINT ( 'NONE',  ( -18.62759615963270932, 10.81492255796079327, 115.8322429386477097 ) ) ;
#101012=CARTESIAN_POINT ( 'NONE',  ( 5.049401038298161559, -19.05341960407611168, 72.70724293864768129 ) ) ;
#101013=CARTESIAN_POINT ( 'NONE',  ( -10.81492255796105439, 18.62759615963255655, 52.91775706135235424 ) ) ;
#101014=CARTESIAN_POINT ( 'NONE',  ( -13.97604488694527625, -13.89961937509977652, 106.8739096053143669 ) ) ;
#101016=VERTEX_POINT ( 'NONE', #157689 ) ;
#101017=CARTESIAN_POINT ( 'NONE',  ( 18.67979575497194134, -10.72451020669871369, 50.83442372801901143 ) ) ;
#101018=CARTESIAN_POINT ( 'NONE',  ( -19.02544592524342804, 5.153800228976336051, 116.0405762719810383 ) ) ;
#101019=CARTESIAN_POINT ( 'NONE',  ( 16.51473224551069308, 9.474510206698969483, 99.16557627198102409 ) ) ;
#101020=CARTESIAN_POINT ( 'NONE',  ( 9.474510206698729675, 16.51473224551082808, 52.08442372801900433 ) ) ;
#101021=CARTESIAN_POINT ( 'NONE',  ( 15.72974639402199770, -15.80617190586745480, 108.1239096053143811 ) ) ;
#101022=CARTESIAN_POINT ( 'NONE',  ( -5.049401038297874678, -19.05341960407617918, 39.79275706135232582 ) ) ;
#101023=CARTESIAN_POINT ( 'NONE',  ( 16.51473224551083163, -9.474510206698727899, 55.83442372801899722 ) ) ;
#101024=CARTESIAN_POINT ( 'NONE',  ( 4.379528057220092307, 16.55341960407617563, 102.2927570613523613 ) ) ;
#101026=ORIENTED_EDGE ( 'NONE', *, *, #171652, .F. ) ;
#101027=CARTESIAN_POINT ( 'NONE',  ( 16.51473224551069308, 9.474510206698969483, 74.16557627198103830 ) ) ;
#101028=CARTESIAN_POINT ( 'NONE',  ( -5.719274019375665041, -21.55341960407619695, 84.79275706135234714 ) ) ;
#101029=CARTESIAN_POINT ( 'NONE',  ( -21.53943276465977519, -0.05219959533937600094, 88.75109039468567573 ) ) ;
#101031=CARTESIAN_POINT ( 'NONE',  ( -5.153800228976328057, -19.02544592524343514, 97.29057627198099567 ) ) ;
#101032=CARTESIAN_POINT ( 'NONE',  ( 5.719274019375673035, 21.55341960407619339, 77.29275706135234714 ) ) ;
#101033=CARTESIAN_POINT ( 'NONE',  ( -4.483927247898782831, 16.52544592524335698, 22.70942372801901499 ) ) ;
#101034=CARTESIAN_POINT ( 'NONE',  ( -19.02544592524342804, 5.153800228976336051, 76.04057627198102409 ) ) ;
#101035=CARTESIAN_POINT ( 'NONE',  ( 18.67979575497178502, 10.72451020669898547, 24.16557627198103120 ) ) ;
#101036=CARTESIAN_POINT ( 'NONE',  ( 19.03943276465977164, -0.05219959533909143690, 93.74890960531435269 ) ) ;
#101038=CARTESIAN_POINT ( 'NONE',  ( -16.51473224551069308, -9.474510206698971260, 81.66557627198103830 ) ) ;
#101039=CARTESIAN_POINT ( 'NONE',  ( 19.03943276465977164, -0.05219959533909143690, 63.74890960531435979 ) ) ;
#101040=CARTESIAN_POINT ( 'NONE',  ( 10.72451020669898902, -18.67979575497178502, 107.9155762719810241 ) ) ;
#101041=CARTESIAN_POINT ( 'NONE',  ( -8.224510206698735004, -14.34966873604973081, 94.58442372801901854 ) ) ;
#101042=LINE ( 'NONE', #195078, #176000 ) ;
#101043=CARTESIAN_POINT ( 'NONE',  ( 19.02544592524334988, 5.153800228976608722, 56.45942372801898301 ) ) ;
#101044=CARTESIAN_POINT ( 'NONE',  ( 9.474510206698971260, -16.51473224551069308, 87.91557627198102409 ) ) ;
#101045=CARTESIAN_POINT ( 'NONE',  ( 14.29746914071049879, -8.314922557960816363, 88.33224293864769550 ) ) ;
#101046=CARTESIAN_POINT ( 'NONE',  ( -10.81492255796078084, -18.62759615963271287, 27.08224293864769550 ) ) ;
#101048=CARTESIAN_POINT ( 'NONE',  ( -21.52544592524343514, 5.823673210054127303, 26.04057627198103475 ) ) ;
#101049=CARTESIAN_POINT ( 'NONE',  ( -8.314922557960811034, -14.29746914071050412, 92.08224293864769550 ) ) ;
#101050=CARTESIAN_POINT ( 'NONE',  ( -17.44279575226822843, 5.990770900252464060, 55.83557567514321107 ) ) ;
#101051=CARTESIAN_POINT ( 'NONE',  ( 9.564922557961047289, -16.46253265017146816, 45.41775706135232582 ) ) ;
#101052=CARTESIAN_POINT ( 'NONE',  ( 8.224510206698742110, 14.34966873604972548, 107.0844237280190043 ) ) ;
#101053=CARTESIAN_POINT ( 'NONE',  ( -9.564922557960796823, -16.46253265017161027, 92.08224293864769550 ) ) ;
#101054=CARTESIAN_POINT ( 'NONE',  ( 10.72451020669871369, 18.67979575497193778, 67.08442372801901854 ) ) ;
#101055=CARTESIAN_POINT ( 'NONE',  ( 21.52544592524344225, -5.823673210054117533, 63.54057627198103830 ) ) ;
#101056=CARTESIAN_POINT ( 'NONE',  ( 10.81492255796106328, -18.62759615963255655, 30.41775706135234358 ) ) ;
#101057=CARTESIAN_POINT ( 'NONE',  ( -0.05219959533907301413, -21.53943276465977519, 82.49890960531436690 ) ) ;
#101058=CARTESIAN_POINT ( 'NONE',  ( -0.05219959533910754901, -16.53943276465976808, 112.4989096053143669 ) ) ;
#101059=CARTESIAN_POINT ( 'NONE',  ( 9.474510206698729675, 16.51473224551082808, 67.08442372801900433 ) ) ;
#101060=CARTESIAN_POINT ( 'NONE',  ( -5.153800228976328057, -19.02544592524343514, 42.29057627198101699 ) ) ;
#101061=CARTESIAN_POINT ( 'NONE',  ( -13.89961937509977652, 13.97604488694528158, 95.62390960531436690 ) ) ;
#101062=CARTESIAN_POINT ( 'NONE',  ( 19.03943276465977164, -0.05219959533909143690, 88.74890960531436690 ) ) ;
#101063=CARTESIAN_POINT ( 'NONE',  ( 16.53943276465976808, -0.05219959533910856209, 113.7489096053143527 ) ) ;
#101064=CARTESIAN_POINT ( 'NONE',  ( 0.05219959533910956823, 16.53943276465976808, 44.99890960531435979 ) ) ;
#101065=CARTESIAN_POINT ( 'NONE',  ( 16.53943276465976808, 0.05219959533934440121, 41.25109039468568284 ) ) ;
#101066=CARTESIAN_POINT ( 'NONE',  ( 5.719274019375673035, 21.55341960407619339, 112.2927570613523471 ) ) ;
#101068=CARTESIAN_POINT ( 'NONE',  ( -8.314922557960811034, -14.29746914071050412, 22.08224293864769194 ) ) ;
#101069=CARTESIAN_POINT ( 'NONE',  ( -21.53943276465977519, -0.05219959533937600094, 28.75109039468567929 ) ) ;
#101070=CARTESIAN_POINT ( 'NONE',  ( -13.89961937509977652, 13.97604488694528158, 105.6239096053143527 ) ) ;
#101071=CARTESIAN_POINT ( 'NONE',  ( 16.55341960407618274, -4.379528057220086978, 101.0427570613523756 ) ) ;
#101072=CARTESIAN_POINT ( 'NONE',  ( -0.05219959533934338120, 16.53943276465976808, 97.50109039468567573 ) ) ;
#101073=CARTESIAN_POINT ( 'NONE',  ( 14.29746914071037800, 8.314922557961029526, 26.66775706135235424 ) ) ;
#101074=CARTESIAN_POINT ( 'NONE',  ( -9.474510206698964154, 16.51473224551069663, 50.41557627198102409 ) ) ;
#101075=CARTESIAN_POINT ( 'NONE',  ( 14.34966873604960469, 8.224510206698951720, 109.1655762719810383 ) ) ;
#101076=CARTESIAN_POINT ( 'NONE',  ( -10.72451020669898014, 18.67979575497178502, 115.4155762719810241 ) ) ;
#101077=CARTESIAN_POINT ( 'NONE',  ( 19.03943276465977164, -0.05219959533909143690, 28.74890960531435624 ) ) ;
#101078=CARTESIAN_POINT ( 'NONE',  ( 13.97604488694527802, 13.89961937509977652, 99.37390960531436690 ) ) ;
#101079=CARTESIAN_POINT ( 'NONE',  ( -9.474510206698964154, 16.51473224551069663, 30.41557627198102054 ) ) ;
#101080=CARTESIAN_POINT ( 'NONE',  ( -19.03943276465977164, 0.05219959533909376836, 101.2489096053143669 ) ) ;
#101081=CARTESIAN_POINT ( 'NONE',  ( 18.22780087662123805, -5.499999999999989342, 63.51763182126896368 ) ) ;
#101083=CARTESIAN_POINT ( 'NONE',  ( 9.564922557960805705, 16.46253265017160317, 104.5822429386476955 ) ) ;
#101084=CARTESIAN_POINT ( 'NONE',  ( 21.52544592524334988, 5.823673210054432836, 51.45942372801901854 ) ) ;
#101085=CARTESIAN_POINT ( 'NONE',  ( 14.34966873604960469, 8.224510206698951720, 89.16557627198102409 ) ) ;
#101086=CARTESIAN_POINT ( 'NONE',  ( -16.46253265017160317, 9.564922557960807481, 90.83224293864769550 ) ) ;
#101087=DIRECTION ( 'NONE',  ( 0.000000000000000000, 0.000000000000000000, -1.000000000000000000 ) ) ;
#101088=CARTESIAN_POINT ( 'NONE',  ( 0.05219959533934541429, -16.53943276465976808, 70.00109039468568994 ) ) ;
#101089=CARTESIAN_POINT ( 'NONE',  ( -15.72974639402176322, -15.80617190586768395, 79.37609039468567573 ) ) ;
#101090=CARTESIAN_POINT ( 'NONE',  ( 4.483927247898790824, -16.52544592524335698, 40.20942372801901854 ) ) ;
#101091=CARTESIAN_POINT ( 'NONE',  ( -5.049401038298153566, 19.05341960407611168, 80.20724293864769550 ) ) ;
#101092=CARTESIAN_POINT ( 'NONE',  ( 19.03943276465977164, 0.05219959533936151252, 111.2510903946856757 ) ) ;
#101093=CARTESIAN_POINT ( 'NONE',  ( -14.29746914071037622, -8.314922557961029526, 84.16775706135234714 ) ) ;
#101094=CARTESIAN_POINT ( 'NONE',  ( -16.51473224551082808, 9.474510206698731452, 88.33442372801900433 ) ) ;
#101095=CARTESIAN_POINT ( 'NONE',  ( -9.564922557960796823, -16.46253265017161027, 57.08224293864769550 ) ) ;
#101096=CARTESIAN_POINT ( 'NONE',  ( 18.67979575497178502, 10.72451020669898547, 104.1655762719810241 ) ) ;
#101097=CARTESIAN_POINT ( 'NONE',  ( -14.34966873604960291, -8.224510206698953496, 86.66557627198102409 ) ) ;
#101098=CARTESIAN_POINT ( 'NONE',  ( 13.89961937509957401, 13.97604488694547697, 96.87609039468566152 ) ) ;
#101099=CARTESIAN_POINT ( 'NONE',  ( -4.379528057220086978, -16.55341960407618274, 54.79275706135235424 ) ) ;
#101100=CARTESIAN_POINT ( 'NONE',  ( -19.25663599770060941, 5.499999999999452882, 78.99419308057203182 ) ) ;
#101101=CARTESIAN_POINT ( 'NONE',  ( -19.02544592524334988, -5.153800228976617603, 58.95942372801900433 ) ) ;
#101102=CARTESIAN_POINT ( 'NONE',  ( 12.06949235617757843, -12.14591786802309237, 33.12390960531435979 ) ) ;
#101103=CARTESIAN_POINT ( 'NONE',  ( -16.55341960407611168, -4.379528057220339221, 76.45724293864769550 ) ) ;
#101104=CARTESIAN_POINT ( 'NONE',  ( 13.89961937509957401, 13.97604488694547697, 21.87609039468566152 ) ) ;
#101105=CARTESIAN_POINT ( 'NONE',  ( 17.50000000000000000, -5.500000000000000888, 103.2969038253417153 ) ) ;
#101106=CARTESIAN_POINT ( 'NONE',  ( -18.62759615963255300, -10.81492255796106328, 29.16775706135234003 ) ) ;
#101107=CARTESIAN_POINT ( 'NONE',  ( 13.97604488694527802, 13.89961937509977652, 114.3739096053143669 ) ) ;
#101108=CARTESIAN_POINT ( 'NONE',  ( 19.02544592524343514, -5.153800228976328945, 73.54057627198103830 ) ) ;
#101109=CARTESIAN_POINT ( 'NONE',  ( 15.72974639402176855, 15.80617190586768217, 91.87609039468568994 ) ) ;
#101110=CARTESIAN_POINT ( 'NONE',  ( 16.46253265017160672, -9.564922557960803928, 78.33224293864769550 ) ) ;
#101111=CARTESIAN_POINT ( 'NONE',  ( 21.55341960407610458, 5.719274019375980345, 43.95724293864769550 ) ) ;
#101112=CARTESIAN_POINT ( 'NONE',  ( 12.06949235617757843, -12.14591786802309237, 83.12390960531436690 ) ) ;
#101113=CARTESIAN_POINT ( 'NONE',  ( -9.564922557960796823, -16.46253265017161027, 57.08224293864769550 ) ) ;
#101114=CARTESIAN_POINT ( 'NONE',  ( 8.224510206698953496, -14.34966873604960469, 107.9155762719810241 ) ) ;
#101115=CARTESIAN_POINT ( 'NONE',  ( -0.05219959533937732626, 21.53943276465977519, 22.50109039468567573 ) ) ;
#101116=CARTESIAN_POINT ( 'NONE',  ( -21.53943276465977519, -0.05219959533937600094, 68.75109039468568994 ) ) ;
#101117=CARTESIAN_POINT ( 'NONE',  ( 9.474510206698971260, -16.51473224551069308, 47.91557627198102409 ) ) ;
#101118=CARTESIAN_POINT ( 'NONE',  ( 0.05219959533934541429, -16.53943276465976808, 60.00109039468568284 ) ) ;
#101119=CARTESIAN_POINT ( 'NONE',  ( 15.72974639402199770, -15.80617190586745480, 113.1239096053143953 ) ) ;
#101120=CARTESIAN_POINT ( 'NONE',  ( 0.05219959533907565091, 21.53943276465977519, 114.9989096053143669 ) ) ;
#101121=CARTESIAN_POINT ( 'NONE',  ( -16.51473224551082808, 9.474510206698731452, 43.33442372801900433 ) ) ;
#101122=CARTESIAN_POINT ( 'NONE',  ( -19.02544592524342804, 5.153800228976336051, 61.04057627198103120 ) ) ;
#101124=CARTESIAN_POINT ( 'NONE',  ( -5.823673210054431948, 21.52544592524334988, 67.70942372801901854 ) ) ;
#101125=CARTESIAN_POINT ( 'NONE',  ( -21.53943276465977519, 0.05219959533907696930, 56.24890960531436690 ) ) ;
#101126=CARTESIAN_POINT ( 'NONE',  ( 16.52544592524342804, -4.483927247898539470, 43.54057627198103830 ) ) ;
#101127=CARTESIAN_POINT ( 'NONE',  ( 10.81492255796106328, -18.62759615963255655, 75.41775706135233293 ) ) ;
#101128=CARTESIAN_POINT ( 'NONE',  ( 18.67979575497194134, -10.72451020669871369, 105.8344237280190328 ) ) ;
#101129=CARTESIAN_POINT ( 'NONE',  ( -16.53943276465976808, 0.05219959533911058130, 61.24890960531435979 ) ) ;
#101130=CARTESIAN_POINT ( 'NONE',  ( -16.52544592524342804, 4.483927247898546575, 101.0405762719810383 ) ) ;
#101131=CARTESIAN_POINT ( 'NONE',  ( 5.049401038297881783, 19.05341960407617563, 62.29275706135234003 ) ) ;
#101132=CARTESIAN_POINT ( 'NONE',  ( 4.379528057220092307, 16.55341960407617563, 112.2927570613523471 ) ) ;
#101133=CARTESIAN_POINT ( 'NONE',  ( -21.55341960407619339, 5.719274019375674811, 63.54275706135234003 ) ) ;
#101134=CARTESIAN_POINT ( 'NONE',  ( -5.049401038298153566, 19.05341960407611168, 70.20724293864769550 ) ) ;
#101135=CARTESIAN_POINT ( 'NONE',  ( 16.51473224551083163, -9.474510206698727899, 40.83442372801900433 ) ) ;
#101136=CARTESIAN_POINT ( 'NONE',  ( 21.52544592524344225, -5.823673210054117533, 33.54057627198102409 ) ) ;
#101137=CARTESIAN_POINT ( 'NONE',  ( 15.80617190586769283, -15.72974639402175789, 50.62609039468568994 ) ) ;
#101138=CARTESIAN_POINT ( 'NONE',  ( -10.81492255796078084, -18.62759615963271287, 102.0822429386476955 ) ) ;
#101139=CARTESIAN_POINT ( 'NONE',  ( -19.02544592524334988, -5.153800228976617603, 103.9594237280190043 ) ) ;
#101140=CARTESIAN_POINT ( 'NONE',  ( -16.52544592524335698, -4.483927247898792601, 58.95942372801902565 ) ) ;
#101142=CARTESIAN_POINT ( 'NONE',  ( 21.53943276465977519, -0.05219959533907433946, 93.74890960531436690 ) ) ;
#101143=CARTESIAN_POINT ( 'NONE',  ( 16.55341960407611168, 4.379528057220329451, 83.95724293864770971 ) ) ;
#101145=CARTESIAN_POINT ( 'NONE',  ( 16.52544592524335698, 4.483927247898782831, 21.45942372801901499 ) ) ;
#101146=CARTESIAN_POINT ( 'NONE',  ( 15.80617190586746368, 15.72974639402197994, 49.37390960531436690 ) ) ;
#101147=CARTESIAN_POINT ( 'NONE',  ( 12.14591786802327356, -12.06949235617739191, 95.62609039468568994 ) ) ;
#101149=CARTESIAN_POINT ( 'NONE',  ( -14.29746914071037622, -8.314922557961029526, 59.16775706135234714 ) ) ;
#101150=CARTESIAN_POINT ( 'NONE',  ( -5.823673210054431948, 21.52544592524334988, 22.70942372801901499 ) ) ;
#101151=CARTESIAN_POINT ( 'NONE',  ( -15.80617190586745835, -15.72974639402198527, 46.87390960531435979 ) ) ;
#101152=CARTESIAN_POINT ( 'NONE',  ( -16.52544592524335698, -4.483927247898792601, 78.95942372801901854 ) ) ;
#101153=CARTESIAN_POINT ( 'NONE',  ( 19.02544592524343514, -5.153800228976328945, 103.5405762719809957 ) ) ;
#101154=CARTESIAN_POINT ( 'NONE',  ( 21.52544592524334988, 5.823673210054432836, 71.45942372801901854 ) ) ;
#101155=CARTESIAN_POINT ( 'NONE',  ( 18.67979575497178502, 10.72451020669898547, 44.16557627198103120 ) ) ;
#101156=CARTESIAN_POINT ( 'NONE',  ( 13.97604488694527802, 13.89961937509977652, 114.3739096053143669 ) ) ;
#101158=CARTESIAN_POINT ( 'NONE',  ( 19.05341960407617918, -5.049401038297876454, 46.04275706135233293 ) ) ;
#101159=CARTESIAN_POINT ( 'NONE',  ( -16.52544592524335698, -4.483927247898792601, 68.95942372801901854 ) ) ;
#101160=CARTESIAN_POINT ( 'NONE',  ( 21.52544592524344225, -5.823673210054117533, 33.54057627198102409 ) ) ;
#101162=CARTESIAN_POINT ( 'NONE',  ( -19.02544592524342804, 5.153800228976336051, 81.04057627198103830 ) ) ;
#101163=CARTESIAN_POINT ( 'NONE',  ( -16.55341960407617563, 4.379528057220093196, 113.5427570613523756 ) ) ;
#101165=CARTESIAN_POINT ( 'NONE',  ( 16.55341960407611168, 4.379528057220329451, 108.9572429386476955 ) ) ;
#101166=CARTESIAN_POINT ( 'NONE',  ( -10.81492255796078084, -18.62759615963271287, 52.08224293864768839 ) ) ;
#101167=CARTESIAN_POINT ( 'NONE',  ( -19.02544592524342804, 5.153800228976336051, 46.04057627198101699 ) ) ;
#101168=CARTESIAN_POINT ( 'NONE',  ( 4.379528057220092307, 16.55341960407617563, 72.29275706135236135 ) ) ;
#101169=CARTESIAN_POINT ( 'NONE',  ( -21.53943276465977519, -0.05219959533937600094, 33.75109039468568284 ) ) ;
#101170=CARTESIAN_POINT ( 'NONE',  ( -0.05219959533936034679, 19.03943276465977164, 87.50109039468567573 ) ) ;
#101171=CARTESIAN_POINT ( 'NONE',  ( 0.05219959533910956823, 16.53943276465976808, 84.99890960531436690 ) ) ;
#101172=CARTESIAN_POINT ( 'NONE',  ( -9.474510206698964154, 16.51473224551069663, 60.41557627198102409 ) ) ;
#101173=CARTESIAN_POINT ( 'NONE',  ( -13.89961937509977652, 13.97604488694528158, 25.62390960531434558 ) ) ;
#101174=CARTESIAN_POINT ( 'NONE',  ( 0.05219959533937995610, -21.53943276465977519, 100.0010903946857042 ) ) ;
#101175=CARTESIAN_POINT ( 'NONE',  ( -5.153800228976328057, -19.02544592524343514, 82.29057627198103830 ) ) ;
#101176=CARTESIAN_POINT ( 'NONE',  ( -16.53943276465976808, -0.05219959533934237506, 63.75109039468568284 ) ) ;
#101177=CARTESIAN_POINT ( 'NONE',  ( -10.72451020669870658, -18.67979575497194134, 89.58442372801901854 ) ) ;
#101178=CARTESIAN_POINT ( 'NONE',  ( 0.05219959533907565091, 21.53943276465977519, 49.99890960531437401 ) ) ;
#101179=CARTESIAN_POINT ( 'NONE',  ( 12.14591786802327356, -12.06949235617739191, 70.62609039468567573 ) ) ;
#101180=CARTESIAN_POINT ( 'NONE',  ( 13.89961937509957401, 13.97604488694547697, 56.87609039468564731 ) ) ;
#101181=CARTESIAN_POINT ( 'NONE',  ( -19.05341960407617563, 5.049401038297882671, 68.54275706135230450 ) ) ;
#101182=CARTESIAN_POINT ( 'NONE',  ( 21.52544592524334988, 5.823673210054432836, 66.45942372801903275 ) ) ;
#101183=CARTESIAN_POINT ( 'NONE',  ( -13.89961937509977652, 13.97604488694528158, 70.62390960531432427 ) ) ;
#101184=CARTESIAN_POINT ( 'NONE',  ( 18.22780087662119897, -5.500000000000096811, 58.51763182126894947 ) ) ;
#101185=CARTESIAN_POINT ( 'NONE',  ( 13.97604488694548053, -13.89961937509957401, 55.62609039468566863 ) ) ;
#101187=CARTESIAN_POINT ( 'NONE',  ( 16.46253265017160672, -9.564922557960803928, 98.33224293864769550 ) ) ;
#101188=CARTESIAN_POINT ( 'NONE',  ( 16.55341960407611168, 4.379528057220329451, 48.95724293864770971 ) ) ;
#101189=CARTESIAN_POINT ( 'NONE',  ( 18.67979575497178502, 10.72451020669898547, 44.16557627198103120 ) ) ;
#101190=CARTESIAN_POINT ( 'NONE',  ( 10.72451020669871369, 18.67979575497193778, 112.0844237280190185 ) ) ;
#101191=CARTESIAN_POINT ( 'NONE',  ( -19.02544592524342804, 5.153800228976336051, 46.04057627198101699 ) ) ;
#101192=CARTESIAN_POINT ( 'NONE',  ( -30.00000000000000000, -1.163414459189985801E-14, 97.50000000000000000 ) ) ;
#101195=CARTESIAN_POINT ( 'NONE',  ( 16.53943276465976808, 0.05219959533934440121, 61.25109039468567573 ) ) ;
#101196=CARTESIAN_POINT ( 'NONE',  ( 18.62759615963271287, -10.81492255796078972, 78.33224293864770971 ) ) ;
#101198=CARTESIAN_POINT ( 'NONE',  ( 12.06949235617757843, -12.14591786802309237, 58.12390960531435979 ) ) ;
#101199=CARTESIAN_POINT ( 'NONE',  ( -16.46253265017160317, 9.564922557960807481, 25.83224293864769194 ) ) ;
#101200=CARTESIAN_POINT ( 'NONE',  ( -22.00000000000000000, -5.510910596163089556E-15, 47.50000000000000000 ) ) ;
#101201=CARTESIAN_POINT ( 'NONE',  ( 5.719274019375673035, 21.55341960407619339, 47.29275706135234003 ) ) ;
#101202=CARTESIAN_POINT ( 'NONE',  ( 19.05341960407617918, -5.049401038297876454, 46.04275706135233293 ) ) ;
#101203=CARTESIAN_POINT ( 'NONE',  ( 5.153800228976335163, 19.02544592524342804, 29.79057627198102409 ) ) ;
#101204=CARTESIAN_POINT ( 'NONE',  ( 18.67979575497194134, -10.72451020669871369, 75.83442372801900433 ) ) ;
#101205=CARTESIAN_POINT ( 'NONE',  ( 16.62475595723699229, 7.163666690055317865, 96.97286648189530922 ) ) ;
#101206=ORIENTED_EDGE ( 'NONE', *, *, #181371, .T. ) ;
#101207=CARTESIAN_POINT ( 'NONE',  ( 8.224510206698953496, -14.34966873604960469, 42.91557627198103120 ) ) ;
#101208=CARTESIAN_POINT ( 'NONE',  ( 17.50000000000002842, 4.049696124445913981, 113.3196032933405775 ) ) ;
#101209=CARTESIAN_POINT ( 'NONE',  ( 0.05219959533907565091, 21.53943276465977519, 39.99890960531436690 ) ) ;
#101211=CARTESIAN_POINT ( 'NONE',  ( 13.97604488694527802, 13.89961937509977652, 89.37390960531436690 ) ) ;
#101212=CARTESIAN_POINT ( 'NONE',  ( 16.52544592524342804, -4.483927247898539470, 88.54057627198103830 ) ) ;
#101213=CARTESIAN_POINT ( 'NONE',  ( 4.483927247898790824, -16.52544592524335698, 25.20942372801901854 ) ) ;
#101214=CARTESIAN_POINT ( 'NONE',  ( 5.719274019375991003, -21.55341960407610458, 67.70724293864769550 ) ) ;
#101216=CARTESIAN_POINT ( 'NONE',  ( 9.474510206698971260, -16.51473224551069308, 27.91557627198103120 ) ) ;
#101217=CARTESIAN_POINT ( 'NONE',  ( 16.46253265017160672, -9.564922557960803928, 83.33224293864768129 ) ) ;
#101218=CARTESIAN_POINT ( 'NONE',  ( 21.55341960407610458, 5.719274019375980345, 83.95724293864770971 ) ) ;
#101220=CARTESIAN_POINT ( 'NONE',  ( -16.55341960407611168, -4.379528057220339221, 21.45724293864769550 ) ) ;
#101221=CARTESIAN_POINT ( 'NONE',  ( -5.049401038298153566, 19.05341960407611168, 100.2072429386476955 ) ) ;
#101222=CARTESIAN_POINT ( 'NONE',  ( 16.51473224551083163, -9.474510206698727899, 75.83442372801900433 ) ) ;
#101223=CARTESIAN_POINT ( 'NONE',  ( -21.55341960407619339, 5.719274019375674811, 113.5427570613523756 ) ) ;
#101224=CARTESIAN_POINT ( 'NONE',  ( -21.55341960407610458, -5.719274019375992779, 81.45724293864769550 ) ) ;
#101225=CARTESIAN_POINT ( 'NONE',  ( 10.81492255796078972, 18.62759615963270932, 39.58224293864769550 ) ) ;
#101226=CARTESIAN_POINT ( 'NONE',  ( -16.51473224551069308, -9.474510206698971260, 61.66557627198103120 ) ) ;
#101227=CARTESIAN_POINT ( 'NONE',  ( -16.52544592524335698, -4.483927247898792601, 108.9594237280190185 ) ) ;
#101228=CARTESIAN_POINT ( 'NONE',  ( -9.564922557960796823, -16.46253265017161027, 77.08224293864769550 ) ) ;
#101231=CARTESIAN_POINT ( 'NONE',  ( -19.02544592524334988, -5.153800228976617603, 23.95942372801900078 ) ) ;
#101232=CARTESIAN_POINT ( 'NONE',  ( -8.314922557960811034, -14.29746914071050412, 92.08224293864769550 ) ) ;
#101233=CARTESIAN_POINT ( 'NONE',  ( -15.80617190586768217, 15.72974639402176855, 23.12609039468567573 ) ) ;
#101235=CARTESIAN_POINT ( 'NONE',  ( -18.67979575497178146, -10.72451020669898902, 71.66557627198100988 ) ) ;
#101236=CARTESIAN_POINT ( 'NONE',  ( -16.55341960407617563, 4.379528057220093196, 88.54275706135236135 ) ) ;
#101237=CARTESIAN_POINT ( 'NONE',  ( 14.34966873604960469, 8.224510206698951720, 114.1655762719810383 ) ) ;
#101238=CARTESIAN_POINT ( 'NONE',  ( -19.05341960407611168, -5.049401038298163336, 76.45724293864769550 ) ) ;
#101240=CARTESIAN_POINT ( 'NONE',  ( -16.51473224551069308, -9.474510206698971260, 21.66557627198102765 ) ) ;
#101241=CARTESIAN_POINT ( 'NONE',  ( 12.14591786802309770, 12.06949235617756955, 24.37390960531435979 ) ) ;
#101242=CARTESIAN_POINT ( 'NONE',  ( 10.81492255796106328, -18.62759615963255655, 65.41775706135234714 ) ) ;
#101243=CARTESIAN_POINT ( 'NONE',  ( -9.564922557960796823, -16.46253265017161027, 112.0822429386476955 ) ) ;
#101244=CARTESIAN_POINT ( 'NONE',  ( -5.719274019375665041, -21.55341960407619695, 89.79275706135236135 ) ) ;
#101245=CARTESIAN_POINT ( 'NONE',  ( -19.02544592524342804, 5.153800228976336051, 46.04057627198101699 ) ) ;
#101246=CARTESIAN_POINT ( 'NONE',  ( 13.89961937509977652, -13.97604488694527269, 58.12390960531436690 ) ) ;
#101248=CARTESIAN_POINT ( 'NONE',  ( 18.67979575497194134, -10.72451020669871369, 90.83442372801901854 ) ) ;
#101249=CARTESIAN_POINT ( 'NONE',  ( 16.53943276465976808, 0.05219959533934440121, 56.25109039468568284 ) ) ;
#101250=CARTESIAN_POINT ( 'NONE',  ( 21.55341960407619695, -5.719274019375665929, 86.04275706135236135 ) ) ;
#101251=CARTESIAN_POINT ( 'NONE',  ( -18.62759615963270932, 10.81492255796079327, 25.83224293864769194 ) ) ;
#101252=CARTESIAN_POINT ( 'NONE',  ( 19.05341960407617918, -5.049401038297876454, 96.04275706135231871 ) ) ;
#101253=CARTESIAN_POINT ( 'NONE',  ( 0.05219959533937995610, -21.53943276465977519, 50.00109039468568994 ) ) ;
#101254=CARTESIAN_POINT ( 'NONE',  ( 12.14591786802327356, -12.06949235617739191, 40.62609039468567573 ) ) ;
#101255=CARTESIAN_POINT ( 'NONE',  ( -18.62759615963270932, 10.81492255796079327, 85.83224293864768129 ) ) ;
#101256=CARTESIAN_POINT ( 'NONE',  ( 19.05341960407617918, -5.049401038297876454, 86.04275706135233293 ) ) ;
#101257=CARTESIAN_POINT ( 'NONE',  ( 0.05219959533909260263, 19.03943276465977164, 69.99890960531435269 ) ) ;
#101258=CARTESIAN_POINT ( 'NONE',  ( 13.89961937509957401, 13.97604488694547697, 91.87609039468567573 ) ) ;
#101259=CARTESIAN_POINT ( 'NONE',  ( -5.153800228976607833, 19.02544592524334988, 102.7094237280189759 ) ) ;
#101260=CARTESIAN_POINT ( 'NONE',  ( -16.52544592524342804, 4.483927247898546575, 56.04057627198102409 ) ) ;
#101261=CARTESIAN_POINT ( 'NONE',  ( 16.51473224551083163, -9.474510206698727899, 80.83442372801899012 ) ) ;
#101262=CARTESIAN_POINT ( 'NONE',  ( 0.05219959533934541429, -16.53943276465976808, 60.00109039468568284 ) ) ;
#101263=CARTESIAN_POINT ( 'NONE',  ( 16.51473224551083163, -9.474510206698727899, 35.83442372801899722 ) ) ;
#101264=CARTESIAN_POINT ( 'NONE',  ( -0.05219959533909027116, -19.03943276465977164, 37.49890960531436690 ) ) ;
#101265=CARTESIAN_POINT ( 'NONE',  ( -0.05219959533909027116, -19.03943276465977164, 47.49890960531435979 ) ) ;
#101266=CARTESIAN_POINT ( 'NONE',  ( 16.55341960407618274, -4.379528057220086978, 61.04275706135234714 ) ) ;
#101269=CARTESIAN_POINT ( 'NONE',  ( 16.46253265017160672, -9.564922557960803928, 103.3322429386476955 ) ) ;
#101272=CARTESIAN_POINT ( 'NONE',  ( 9.474510206698729675, 16.51473224551082808, 97.08442372801900433 ) ) ;
#101273=CARTESIAN_POINT ( 'NONE',  ( 15.80617190586746368, 15.72974639402197994, 39.37390960531436690 ) ) ;
#101274=CARTESIAN_POINT ( 'NONE',  ( 13.97604488694548053, -13.89961937509957401, 35.62609039468567573 ) ) ;
#101275=CARTESIAN_POINT ( 'NONE',  ( 5.153800228976615827, -19.02544592524334988, 110.2094237280189901 ) ) ;
#101276=CARTESIAN_POINT ( 'NONE',  ( -19.03943276465977164, 0.05219959533909376836, 36.24890960531436690 ) ) ;
#101277=CARTESIAN_POINT ( 'NONE',  ( -16.46253265017160317, 9.564922557960807481, 50.83224293864770260 ) ) ;
#101278=CARTESIAN_POINT ( 'NONE',  ( -15.80617190586745835, -15.72974639402198527, 66.87390960531436690 ) ) ;
#101279=CARTESIAN_POINT ( 'NONE',  ( 16.51473224551069308, 9.474510206698969483, 104.1655762719810241 ) ) ;
#101281=CARTESIAN_POINT ( 'NONE',  ( -0.05219959533909027116, -19.03943276465977164, 32.49890960531435979 ) ) ;
#101283=CARTESIAN_POINT ( 'NONE',  ( -9.474510206698720793, -16.51473224551083518, 89.58442372801900433 ) ) ;
#101284=CARTESIAN_POINT ( 'NONE',  ( 8.314922557960818139, 14.29746914071049879, 49.58224293864769550 ) ) ;
#101285=CARTESIAN_POINT ( 'NONE',  ( 10.72451020669898902, -18.67979575497178502, 37.91557627198102409 ) ) ;
#101286=CARTESIAN_POINT ( 'NONE',  ( -0.05219959533937732626, 21.53943276465977519, 112.5010903946857042 ) ) ;
#101287=CARTESIAN_POINT ( 'NONE',  ( 15.72974639402199770, -15.80617190586745480, 93.12390960531436690 ) ) ;
#101288=CARTESIAN_POINT ( 'NONE',  ( 18.62759615963255655, 10.81492255796105972, 66.66775706135234714 ) ) ;
#101289=CARTESIAN_POINT ( 'NONE',  ( -5.823673210054431948, 21.52544592524334988, 82.70942372801900433 ) ) ;
#101290=CARTESIAN_POINT ( 'NONE',  ( -13.97604488694527625, -13.89961937509977652, 106.8739096053143669 ) ) ;
#101291=CARTESIAN_POINT ( 'NONE',  ( 12.06949235617739724, 12.14591786802326823, 106.8760903946856899 ) ) ;
#101292=CARTESIAN_POINT ( 'NONE',  ( -15.72974639402176322, -15.80617190586768395, 64.37609039468568994 ) ) ;
#101293=CARTESIAN_POINT ( 'NONE',  ( -9.564922557960796823, -16.46253265017161027, 67.08224293864769550 ) ) ;
#101295=CARTESIAN_POINT ( 'NONE',  ( 16.51473224551083163, -9.474510206698727899, 30.83442372801900433 ) ) ;
#101296=CARTESIAN_POINT ( 'NONE',  ( 10.81492255796106328, -18.62759615963255655, 35.41775706135234003 ) ) ;
#101297=CARTESIAN_POINT ( 'NONE',  ( 16.46253265017160672, -9.564922557960803928, 63.33224293864769550 ) ) ;
#101298=CARTESIAN_POINT ( 'NONE',  ( -8.314922557960811034, -14.29746914071050412, 87.08224293864769550 ) ) ;
#101299=CARTESIAN_POINT ( 'NONE',  ( -16.53943276465976808, 0.05219959533911058130, 46.24890960531435979 ) ) ;
#101300=CARTESIAN_POINT ( 'NONE',  ( 5.719274019375991003, -21.55341960407610458, 52.70724293864769550 ) ) ;
#101301=CARTESIAN_POINT ( 'NONE',  ( -9.474510206698964154, 16.51473224551069663, 65.41557627198102409 ) ) ;
#101302=CARTESIAN_POINT ( 'NONE',  ( -21.55341960407610458, -5.719274019375992779, 76.45724293864769550 ) ) ;
#101303=CARTESIAN_POINT ( 'NONE',  ( -13.97604488694547697, 13.89961937509957934, 53.12609039468565442 ) ) ;
#101304=CARTESIAN_POINT ( 'NONE',  ( 0.05219959533936267826, -19.03943276465977164, 25.00109039468566152 ) ) ;
#101305=CARTESIAN_POINT ( 'NONE',  ( -8.314922557960811034, -14.29746914071050412, 57.08224293864769550 ) ) ;
#101306=CARTESIAN_POINT ( 'NONE',  ( 21.55341960407610458, 5.719274019375980345, 38.95724293864768839 ) ) ;
#101309=CARTESIAN_POINT ( 'NONE',  ( 16.55341960407618274, -4.379528057220086978, 86.04275706135236135 ) ) ;
#101311=CARTESIAN_POINT ( 'NONE',  ( -5.049401038297874678, -19.05341960407617918, 94.79275706135230450 ) ) ;
#101312=CARTESIAN_POINT ( 'NONE',  ( -14.34966873604960291, -8.224510206698953496, 51.66557627198102409 ) ) ;
#101314=CARTESIAN_POINT ( 'NONE',  ( 5.049401038298161559, -19.05341960407611168, 47.70724293864770260 ) ) ;
#101315=CARTESIAN_POINT ( 'NONE',  ( -16.53943276465976808, 0.05219959533911058130, 36.24890960531435979 ) ) ;
#101316=CARTESIAN_POINT ( 'NONE',  ( 9.564922557960805705, 16.46253265017160317, 94.58224293864769550 ) ) ;
#101317=CARTESIAN_POINT ( 'NONE',  ( 13.89961937509977652, -13.97604488694527269, 58.12390960531436690 ) ) ;
#101318=CARTESIAN_POINT ( 'NONE',  ( 15.72974639402176855, 15.80617190586768217, 56.87609039468568994 ) ) ;
#101319=CARTESIAN_POINT ( 'NONE',  ( 13.89961937509977652, -13.97604488694527269, 73.12390960531436690 ) ) ;
#101321=CARTESIAN_POINT ( 'NONE',  ( -0.05219959533909027116, -19.03943276465977164, 77.49890960531435269 ) ) ;
#101322=CARTESIAN_POINT ( 'NONE',  ( 18.62759615963271287, -10.81492255796078972, 48.33224293864770260 ) ) ;
#101323=CARTESIAN_POINT ( 'NONE',  ( -16.46253265017160317, 9.564922557960807481, 30.83224293864769550 ) ) ;
#101324=CARTESIAN_POINT ( 'NONE',  ( -21.52544592524343514, 5.823673210054127303, 56.04057627198102409 ) ) ;
#101325=CARTESIAN_POINT ( 'NONE',  ( 14.29746914071037800, 8.314922557961029526, 101.6677570613523613 ) ) ;
#101326=EDGE_CURVE ( 'NONE', #62281, #52144, #104638, .T. ) ;
#101327=CARTESIAN_POINT ( 'NONE',  ( 0.05219959533936267826, -19.03943276465977164, 25.00109039468566152 ) ) ;
#101328=CARTESIAN_POINT ( 'NONE',  ( -12.14591786802326823, 12.06949235617739902, 48.12609039468568284 ) ) ;
#101329=CARTESIAN_POINT ( 'NONE',  ( -16.55341960407617563, 4.379528057220093196, 83.54275706135234714 ) ) ;
#101331=CARTESIAN_POINT ( 'NONE',  ( -16.55341960407617563, 4.379528057220093196, 73.54275706135234714 ) ) ;
#101332=CARTESIAN_POINT ( 'NONE',  ( -10.81492255796078084, -18.62759615963271287, 27.08224293864769550 ) ) ;
#101333=CARTESIAN_POINT ( 'NONE',  ( -0.05219959533909027116, -19.03943276465977164, 32.49890960531435979 ) ) ;
#101334=CARTESIAN_POINT ( 'NONE',  ( -0.05219959533934338120, 16.53943276465976808, 42.50109039468567573 ) ) ;
#101335=CARTESIAN_POINT ( 'NONE',  ( 13.89961937509977652, -13.97604488694527269, 48.12390960531435979 ) ) ;
#101336=CARTESIAN_POINT ( 'NONE',  ( -10.81492255796105439, 18.62759615963255655, 37.91775706135235424 ) ) ;
#101337=CARTESIAN_POINT ( 'NONE',  ( -4.483927247898782831, 16.52544592524335698, 32.70942372801900433 ) ) ;
#101338=CARTESIAN_POINT ( 'NONE',  ( 16.55341960407618274, -4.379528057220086978, 96.04275706135236135 ) ) ;
#101340=CARTESIAN_POINT ( 'NONE',  ( 18.62759615963255655, 10.81492255796105972, 96.66775706135234714 ) ) ;
#101341=CARTESIAN_POINT ( 'NONE',  ( -5.153800228976607833, 19.02544592524334988, 112.7094237280190043 ) ) ;
#101342=CARTESIAN_POINT ( 'NONE',  ( -13.89961937509957401, -13.97604488694547875, 64.37609039468567573 ) ) ;
#101343=CARTESIAN_POINT ( 'NONE',  ( 8.314922557960818139, 14.29746914071049879, 74.58224293864768129 ) ) ;
#101344=CARTESIAN_POINT ( 'NONE',  ( -19.02544592524342804, 5.153800228976336051, 31.04057627198102409 ) ) ;
#101345=CARTESIAN_POINT ( 'NONE',  ( 9.474510206698729675, 16.51473224551082808, 57.08442372801900433 ) ) ;
#101346=CARTESIAN_POINT ( 'NONE',  ( 16.52216118717207038, 7.221426719304519182, 78.57599021046991083 ) ) ;
#101347=CARTESIAN_POINT ( 'NONE',  ( -15.80617190586768217, 15.72974639402176855, 58.12609039468568994 ) ) ;
#101348=CARTESIAN_POINT ( 'NONE',  ( 8.224510206698742110, 14.34966873604972548, 27.08442372801901854 ) ) ;
#101349=CARTESIAN_POINT ( 'NONE',  ( 17.44270441346512968, 5.991230190323101112, 38.86335079264228654 ) ) ;
#101350=CARTESIAN_POINT ( 'NONE',  ( 18.62759615963271287, -10.81492255796078972, 28.33224293864769550 ) ) ;
#101351=CARTESIAN_POINT ( 'NONE',  ( -16.51473224551082808, 9.474510206698731452, 108.3344237280190043 ) ) ;
#101354=CARTESIAN_POINT ( 'NONE',  ( 9.564922557960805705, 16.46253265017160317, 29.58224293864769550 ) ) ;
#101355=CARTESIAN_POINT ( 'NONE',  ( 15.72974639402176855, 15.80617190586768217, 106.8760903946856899 ) ) ;
#101356=CARTESIAN_POINT ( 'NONE',  ( -13.89961937509977652, 13.97604488694528158, 60.62390960531436690 ) ) ;
#101357=CARTESIAN_POINT ( 'NONE',  ( -21.52544592524334988, -5.823673210054445271, 68.95942372801901854 ) ) ;
#101358=CARTESIAN_POINT ( 'NONE',  ( 21.53943276465977519, 0.05219959533937863772, 101.2510903946856757 ) ) ;
#101359=CARTESIAN_POINT ( 'NONE',  ( -16.52544592524342804, 4.483927247898546575, 31.04057627198102409 ) ) ;
#101360=CARTESIAN_POINT ( 'NONE',  ( -13.89961937509977652, 13.97604488694528158, 85.62390960531433848 ) ) ;
#101361=CARTESIAN_POINT ( 'NONE',  ( -15.80617190586768217, 15.72974639402176855, 63.12609039468568994 ) ) ;
#101363=CARTESIAN_POINT ( 'NONE',  ( 0.05219959533937995610, -21.53943276465977519, 50.00109039468568994 ) ) ;
#101364=CARTESIAN_POINT ( 'NONE',  ( -0.05219959533936034679, 19.03943276465977164, 77.50109039468566152 ) ) ;
#101365=CARTESIAN_POINT ( 'NONE',  ( -13.97604488694527625, -13.89961937509977652, 111.8739096053143243 ) ) ;
#101366=CARTESIAN_POINT ( 'NONE',  ( -13.97604488694527625, -13.89961937509977652, 26.87390960531434558 ) ) ;
#101367=CARTESIAN_POINT ( 'NONE',  ( -5.719274019375978568, 21.55341960407610458, 105.2072429386477097 ) ) ;
#101368=CARTESIAN_POINT ( 'NONE',  ( 19.05341960407617918, -5.049401038297876454, 36.04275706135234003 ) ) ;
#101369=CARTESIAN_POINT ( 'NONE',  ( 8.224510206698953496, -14.34966873604960469, 97.91557627198103830 ) ) ;
#101370=CARTESIAN_POINT ( 'NONE',  ( 16.46253265017160672, -9.564922557960803928, 43.33224293864769550 ) ) ;
#101371=CARTESIAN_POINT ( 'NONE',  ( -9.474510206698720793, -16.51473224551083518, 94.58442372801900433 ) ) ;
#101372=CARTESIAN_POINT ( 'NONE',  ( -16.52544592524342804, 4.483927247898546575, 66.04057627198103830 ) ) ;
#101373=CARTESIAN_POINT ( 'NONE',  ( -18.62759615963255300, -10.81492255796106328, 104.1677570613523471 ) ) ;
#101374=CARTESIAN_POINT ( 'NONE',  ( -0.05219959533909027116, -19.03943276465977164, 107.4989096053143527 ) ) ;
#101375=CARTESIAN_POINT ( 'NONE',  ( 19.03943276465977164, 0.05219959533936151252, 81.25109039468567573 ) ) ;
#101376=CARTESIAN_POINT ( 'NONE',  ( -15.80617190586745835, -15.72974639402198527, 91.87390960531436690 ) ) ;
#101377=CARTESIAN_POINT ( 'NONE',  ( -10.72451020669870658, -18.67979575497194134, 39.58442372801901143 ) ) ;
#101378=CARTESIAN_POINT ( 'NONE',  ( 16.52544592524335698, 4.483927247898782831, 46.45942372801901854 ) ) ;
#101379=CARTESIAN_POINT ( 'NONE',  ( -14.29746914071037622, -8.314922557961029526, 104.1677570613523471 ) ) ;
#101380=CARTESIAN_POINT ( 'NONE',  ( -12.06949235617739369, -12.14591786802326823, 39.37609039468567573 ) ) ;
#101381=CARTESIAN_POINT ( 'NONE',  ( -21.53943276465977519, -0.05219959533937600094, 33.75109039468568284 ) ) ;
#101382=CARTESIAN_POINT ( 'NONE',  ( -5.823673210054116645, -21.52544592524344225, 47.29057627198103120 ) ) ;
#101383=CARTESIAN_POINT ( 'NONE',  ( 19.03943276465977164, -0.05219959533909143690, 28.74890960531435624 ) ) ;
#101385=CARTESIAN_POINT ( 'NONE',  ( -16.53943276465976808, -0.05219959533934237506, 68.75109039468568994 ) ) ;
#101386=CARTESIAN_POINT ( 'NONE',  ( -15.72974639402197994, 15.80617190586746368, 90.62390960531436690 ) ) ;
#101387=CARTESIAN_POINT ( 'NONE',  ( 0.05219959533910956823, 16.53943276465976808, 34.99890960531435979 ) ) ;
#101388=CARTESIAN_POINT ( 'NONE',  ( 14.34966873604972726, -8.224510206698740333, 65.83442372801900433 ) ) ;
#101389=CARTESIAN_POINT ( 'NONE',  ( 16.51473224551069308, 9.474510206698969483, 54.16557627198103120 ) ) ;
#101390=CARTESIAN_POINT ( 'NONE',  ( -19.05341960407617563, 5.049401038297882671, 83.54275706135233293 ) ) ;
#101391=CARTESIAN_POINT ( 'NONE',  ( -21.52544592524343514, 5.823673210054127303, 86.04057627198102409 ) ) ;
#101392=CARTESIAN_POINT ( 'NONE',  ( 12.14591786802309770, 12.06949235617756955, 34.37390960531435979 ) ) ;
#101393=ORIENTED_EDGE ( 'NONE', *, *, #70314, .F. ) ;
#101395=CARTESIAN_POINT ( 'NONE',  ( -21.52544592524343514, 5.823673210054127303, 61.04057627198103120 ) ) ;
#101396=ORIENTED_EDGE ( 'NONE', *, *, #120600, .F. ) ;
#101397=CARTESIAN_POINT ( 'NONE',  ( -8.224510206698735004, -14.34966873604973081, 104.5844237280190185 ) ) ;
#101398=ORIENTED_EDGE ( 'NONE', *, *, #196572, .T. ) ;
#101400=CARTESIAN_POINT ( 'NONE',  ( 10.72451020669898902, -18.67979575497178502, 87.91557627198103830 ) ) ;
#101401=CARTESIAN_POINT ( 'NONE',  ( 21.55341960407610458, 5.719274019375980345, 108.9572429386476955 ) ) ;
#101402=CARTESIAN_POINT ( 'NONE',  ( -0.05219959533910754901, -16.53943276465976808, 22.49890960531436335 ) ) ;
#101403=CARTESIAN_POINT ( 'NONE',  ( -16.52544592524335698, -4.483927247898792601, 33.95942372801901143 ) ) ;
#101404=CARTESIAN_POINT ( 'NONE',  ( -13.89961937509977652, 13.97604488694528158, 40.62390960531435979 ) ) ;
#101405=CARTESIAN_POINT ( 'NONE',  ( 5.153800228976335163, 19.02544592524342804, 69.79057627198103830 ) ) ;
#101408=CARTESIAN_POINT ( 'NONE',  ( -5.153800228976328057, -19.02544592524343514, 112.2905762719810099 ) ) ;
#101410=CARTESIAN_POINT ( 'NONE',  ( 16.46253265017146816, 9.564922557961045513, 111.6677570613523329 ) ) ;
#101411=CARTESIAN_POINT ( 'NONE',  ( 5.153800228976615827, -19.02544592524334988, 35.20942372801899722 ) ) ;
#101412=CARTESIAN_POINT ( 'NONE',  ( 18.67979575497178502, 10.72451020669898547, 84.16557627198103830 ) ) ;
#101413=CARTESIAN_POINT ( 'NONE',  ( 4.379528057220339221, -16.55341960407611168, 22.70724293864769194 ) ) ;
#101414=CARTESIAN_POINT ( 'NONE',  ( 5.823673210054125526, 21.52544592524343514, 49.79057627198102409 ) ) ;
#101415=CARTESIAN_POINT ( 'NONE',  ( -5.823673210054116645, -21.52544592524344225, 82.29057627198103830 ) ) ;
#101416=CARTESIAN_POINT ( 'NONE',  ( -13.97604488694547697, 13.89961937509957934, 108.1260903946856331 ) ) ;
#101417=CARTESIAN_POINT ( 'NONE',  ( -13.97604488694527625, -13.89961937509977652, 101.8739096053143811 ) ) ;
#101419=CARTESIAN_POINT ( 'NONE',  ( 10.81492255796106328, -18.62759615963255655, 70.41775706135236135 ) ) ;
#101420=CARTESIAN_POINT ( 'NONE',  ( 16.51473224551069308, 9.474510206698969483, 64.16557627198102409 ) ) ;
#101421=CARTESIAN_POINT ( 'NONE',  ( -14.34966873604960291, -8.224510206698953496, 96.66557627198102409 ) ) ;
#101423=CARTESIAN_POINT ( 'NONE',  ( 19.03943276465977164, -0.05219959533909143690, 73.74890960531435269 ) ) ;
#101424=CARTESIAN_POINT ( 'NONE',  ( -0.05219959533910754901, -16.53943276465976808, 97.49890960531436690 ) ) ;
#101426=CARTESIAN_POINT ( 'NONE',  ( 0.05219959533936267826, -19.03943276465977164, 95.00109039468567573 ) ) ;
#101429=CARTESIAN_POINT ( 'NONE',  ( -5.153800228976328057, -19.02544592524343514, 62.29057627198100988 ) ) ;
#101430=CARTESIAN_POINT ( 'NONE',  ( -10.81492255796105439, 18.62759615963255655, 77.91775706135231871 ) ) ;
#101431=CARTESIAN_POINT ( 'NONE',  ( 13.89961937509977652, -13.97604488694527269, 98.12390960531433848 ) ) ;
#101432=CARTESIAN_POINT ( 'NONE',  ( 16.53943276465976808, 0.05219959533934440121, 76.25109039468568994 ) ) ;
#101433=CARTESIAN_POINT ( 'NONE',  ( -16.19135201231369692, -7.376712067591815192, 50.18680854052031037 ) ) ;
#101434=CARTESIAN_POINT ( 'NONE',  ( -16.51473224551082808, 9.474510206698731452, 38.33442372801899722 ) ) ;
#101435=CARTESIAN_POINT ( 'NONE',  ( 18.67979575497194134, -10.72451020669871369, 95.83442372801903275 ) ) ;
#101438=CARTESIAN_POINT ( 'NONE',  ( -16.52544592524335698, -4.483927247898792601, 103.9594237280190185 ) ) ;
#101440=CARTESIAN_POINT ( 'NONE',  ( 16.53943276465976808, 0.05219959533934440121, 91.25109039468568994 ) ) ;
#101442=CARTESIAN_POINT ( 'NONE',  ( -8.314922557961024197, 14.29746914071037800, 72.91775706135234714 ) ) ;
#101444=CARTESIAN_POINT ( 'NONE',  ( 21.55341960407619695, -5.719274019375665929, 76.04275706135237556 ) ) ;
#101445=CARTESIAN_POINT ( 'NONE',  ( -9.564922557961040184, 16.46253265017147172, 92.91775706135233293 ) ) ;
#101446=CARTESIAN_POINT ( 'NONE',  ( 5.153800228976615827, -19.02544592524334988, 45.20942372801901143 ) ) ;
#101447=CARTESIAN_POINT ( 'NONE',  ( -19.05341960407611168, -5.049401038298163336, 71.45724293864766707 ) ) ;
#101448=CARTESIAN_POINT ( 'NONE',  ( -19.05341960407611168, -5.049401038298163336, 61.45724293864769550 ) ) ;
#101449=CARTESIAN_POINT ( 'NONE',  ( -18.22780087662123094, -5.499999999999984901, 86.48459894673892734 ) ) ;
#101450=CARTESIAN_POINT ( 'NONE',  ( 5.823673210054125526, 21.52544592524343514, 84.79057627198102409 ) ) ;
#101452=CARTESIAN_POINT ( 'NONE',  ( -15.72974639402197994, 15.80617190586746368, 40.62390960531435269 ) ) ;
#101453=CARTESIAN_POINT ( 'NONE',  ( -5.049401038298153566, 19.05341960407611168, 30.20724293864768839 ) ) ;
#101454=CARTESIAN_POINT ( 'NONE',  ( -4.379528057220086978, -16.55341960407618274, 59.79275706135234714 ) ) ;
#101456=CARTESIAN_POINT ( 'NONE',  ( -21.55341960407619339, 5.719274019375674811, 28.54275706135234358 ) ) ;
#101457=CARTESIAN_POINT ( 'NONE',  ( 0.05219959533910956823, 16.53943276465976808, 69.99890960531435269 ) ) ;
#101459=CARTESIAN_POINT ( 'NONE',  ( 14.29746914071037800, 8.314922557961029526, 21.66775706135235069 ) ) ;
#101460=CARTESIAN_POINT ( 'NONE',  ( 9.564922557961047289, -16.46253265017146816, 50.41775706135233293 ) ) ;
#101461=CARTESIAN_POINT ( 'NONE',  ( -0.05219959533910754901, -16.53943276465976808, 57.49890960531435979 ) ) ;
#101462=CARTESIAN_POINT ( 'NONE',  ( 15.80617190586769283, -15.72974639402175789, 30.62609039468567929 ) ) ;
#101464=CARTESIAN_POINT ( 'NONE',  ( -10.81492255796078084, -18.62759615963271287, 82.08224293864768129 ) ) ;
#101465=CARTESIAN_POINT ( 'NONE',  ( 19.02544592524343514, -5.153800228976328945, 108.5405762719810383 ) ) ;
#101466=CARTESIAN_POINT ( 'NONE',  ( -4.379528057220328563, 16.55341960407611168, 55.20724293864770260 ) ) ;
#101467=CARTESIAN_POINT ( 'NONE',  ( -0.05219959533909027116, -19.03943276465977164, 112.4989096053143669 ) ) ;
#101470=CARTESIAN_POINT ( 'NONE',  ( 9.564922557961047289, -16.46253265017146816, 65.41775706135233293 ) ) ;
#101471=CARTESIAN_POINT ( 'NONE',  ( 21.55341960407610458, 5.719274019375980345, 108.9572429386476955 ) ) ;
#101472=CARTESIAN_POINT ( 'NONE',  ( -19.05341960407611168, -5.049401038298163336, 51.45724293864770260 ) ) ;
#101473=CARTESIAN_POINT ( 'NONE',  ( -16.46253265017146816, -9.564922557961047289, 44.16775706135232582 ) ) ;
#101474=CARTESIAN_POINT ( 'NONE',  ( -9.474510206698964154, 16.51473224551069663, 35.41557627198102409 ) ) ;
#101475=CARTESIAN_POINT ( 'NONE',  ( 18.62759615963255655, 10.81492255796105972, 61.66775706135235424 ) ) ;
#101476=CARTESIAN_POINT ( 'NONE',  ( -18.22780087662123805, 5.499999999999981348, 101.0176318212689495 ) ) ;
#101477=CARTESIAN_POINT ( 'NONE',  ( 16.53943276465976808, -0.05219959533910856209, 38.74890960531435979 ) ) ;
#101478=CARTESIAN_POINT ( 'NONE',  ( 19.05341960407611168, 5.049401038298154454, 63.95724293864769550 ) ) ;
#101480=CARTESIAN_POINT ( 'NONE',  ( 5.823673210054125526, 21.52544592524343514, 84.79057627198102409 ) ) ;
#101481=CARTESIAN_POINT ( 'NONE',  ( -19.05341960407611168, -5.049401038298163336, 56.45724293864768129 ) ) ;
#101483=CARTESIAN_POINT ( 'NONE',  ( 18.62759615963271287, -10.81492255796078972, 63.33224293864770260 ) ) ;
#101485=CARTESIAN_POINT ( 'NONE',  ( -21.52544592524334988, -5.823673210054445271, 98.95942372801903275 ) ) ;
#101486=CARTESIAN_POINT ( 'NONE',  ( 17.72662750342725602, 5.500000000000081712, 53.90179492283745333 ) ) ;
#101487=CARTESIAN_POINT ( 'NONE',  ( -0.05219959533934338120, 16.53943276465976808, 97.50109039468567573 ) ) ;
#101488=CARTESIAN_POINT ( 'NONE',  ( -14.34966873604960291, -8.224510206698953496, 86.66557627198102409 ) ) ;
#101489=CARTESIAN_POINT ( 'NONE',  ( 13.97604488694548053, -13.89961937509957401, 90.62609039468567573 ) ) ;
#101490=ORIENTED_EDGE ( 'NONE', *, *, #29212, .F. ) ;
#101491=CARTESIAN_POINT ( 'NONE',  ( -9.474510206698720793, -16.51473224551083518, 39.58442372801899722 ) ) ;
#101492=CARTESIAN_POINT ( 'NONE',  ( -8.314922557961024197, 14.29746914071037800, 107.9177570613523471 ) ) ;
#101493=CARTESIAN_POINT ( 'NONE',  ( 16.51473224551083163, -9.474510206698727899, 30.83442372801900433 ) ) ;
#101494=CARTESIAN_POINT ( 'NONE',  ( 19.02544592524343514, -5.153800228976328945, 93.54057627198102409 ) ) ;
#101495=CARTESIAN_POINT ( 'NONE',  ( 18.62759615963271287, -10.81492255796078972, 58.33224293864768839 ) ) ;
#101497=CARTESIAN_POINT ( 'NONE',  ( 5.153800228976335163, 19.02544592524342804, 24.79057627198102765 ) ) ;
#101498=CARTESIAN_POINT ( 'NONE',  ( -21.52544592524334988, -5.823673210054445271, 93.95942372801903275 ) ) ;
#101499=CARTESIAN_POINT ( 'NONE',  ( 4.379528057220092307, 16.55341960407617563, 72.29275706135236135 ) ) ;
#101500=CARTESIAN_POINT ( 'NONE',  ( 18.67979575497194134, -10.72451020669871369, 25.83442372801901499 ) ) ;
#101501=CARTESIAN_POINT ( 'NONE',  ( 12.06949235617739724, 12.14591786802326823, 36.87609039468568994 ) ) ;
#101502=CARTESIAN_POINT ( 'NONE',  ( -16.46253265017160317, 9.564922557960807481, 100.8322429386477097 ) ) ;
#101503=CARTESIAN_POINT ( 'NONE',  ( -13.97604488694527625, -13.89961937509977652, 36.87390960531436690 ) ) ;
#101504=CARTESIAN_POINT ( 'NONE',  ( 5.049401038298161559, -19.05341960407611168, 47.70724293864770260 ) ) ;
#101505=CARTESIAN_POINT ( 'NONE',  ( 12.06949235617739724, 12.14591786802326823, 41.87609039468568284 ) ) ;
#101506=CARTESIAN_POINT ( 'NONE',  ( -4.379528057220328563, 16.55341960407611168, 95.20724293864769550 ) ) ;
#101507=CARTESIAN_POINT ( 'NONE',  ( 4.483927247898790824, -16.52544592524335698, 105.2094237280190328 ) ) ;
#101508=CARTESIAN_POINT ( 'NONE',  ( -15.72974639402176322, -15.80617190586768395, 39.37609039468567573 ) ) ;
#101509=CARTESIAN_POINT ( 'NONE',  ( 0.05219959533909260263, 19.03943276465977164, 79.99890960531436690 ) ) ;
#101510=CARTESIAN_POINT ( 'NONE',  ( -19.03943276465977164, 0.05219959533909376836, 66.24890960531436690 ) ) ;
#101511=CARTESIAN_POINT ( 'NONE',  ( -0.05219959533909027116, -19.03943276465977164, 92.49890960531436690 ) ) ;
#101512=CARTESIAN_POINT ( 'NONE',  ( 4.483927247898545687, 16.52544592524342804, 29.79057627198102409 ) ) ;
#101513=CARTESIAN_POINT ( 'NONE',  ( -4.483927247898782831, 16.52544592524335698, 102.7094237280190185 ) ) ;
#101515=CARTESIAN_POINT ( 'NONE',  ( 9.564922557961047289, -16.46253265017146816, 50.41775706135233293 ) ) ;
#101516=CARTESIAN_POINT ( 'NONE',  ( 13.89961937509977652, -13.97604488694527269, 108.1239096053143669 ) ) ;
#101517=CARTESIAN_POINT ( 'NONE',  ( -5.153800228976328057, -19.02544592524343514, 57.29057627198103120 ) ) ;
#101518=CARTESIAN_POINT ( 'NONE',  ( 5.153800228976615827, -19.02544592524334988, 35.20942372801899722 ) ) ;
#101520=CARTESIAN_POINT ( 'NONE',  ( 19.26498983726236958, -5.499999999999790390, 73.05319577422000066 ) ) ;
#101521=CARTESIAN_POINT ( 'NONE',  ( -14.34966873604972548, 8.224510206698743886, 48.33442372801902565 ) ) ;
#101522=CARTESIAN_POINT ( 'NONE',  ( -9.564922557961040184, 16.46253265017147172, 77.91775706135234714 ) ) ;
#101523=CARTESIAN_POINT ( 'NONE',  ( 0.05219959533934541429, -16.53943276465976808, 55.00109039468568284 ) ) ;
#101524=SPHERICAL_SURFACE ( 'NONE', #178910, 2.000000000000000000 ) ;
#101525=CARTESIAN_POINT ( 'NONE',  ( 13.97604488694527802, 13.89961937509977652, 89.37390960531436690 ) ) ;
#101526=CARTESIAN_POINT ( 'NONE',  ( 0.05219959533907565091, 21.53943276465977519, 114.9989096053143669 ) ) ;
#101527=CARTESIAN_POINT ( 'NONE',  ( -9.474510206698720793, -16.51473224551083518, 79.58442372801899012 ) ) ;
#101528=CARTESIAN_POINT ( 'NONE',  ( 19.03943276465977164, -0.05219959533909143690, 98.74890960531436690 ) ) ;
#101529=CARTESIAN_POINT ( 'NONE',  ( 5.153800228976335163, 19.02544592524342804, 39.79057627198100988 ) ) ;
#101530=CARTESIAN_POINT ( 'NONE',  ( -13.97604488694527625, -13.89961937509977652, 71.87390960531433848 ) ) ;
#101531=CARTESIAN_POINT ( 'NONE',  ( 16.53943276465976808, -0.05219959533910856209, 33.74890960531436690 ) ) ;
#101532=CARTESIAN_POINT ( 'NONE',  ( -5.153800228976328057, -19.02544592524343514, 42.29057627198101699 ) ) ;
#101533=CARTESIAN_POINT ( 'NONE',  ( -5.049401038297874678, -19.05341960407617918, 54.79275706135234003 ) ) ;
#101534=CARTESIAN_POINT ( 'NONE',  ( 16.53943276465976808, -0.05219959533910856209, 93.74890960531436690 ) ) ;
#101535=CARTESIAN_POINT ( 'NONE',  ( -13.89961937509957401, -13.97604488694547875, 19.37609039468566507 ) ) ;
#101536=CARTESIAN_POINT ( 'NONE',  ( 9.474510206698971260, -16.51473224551069308, 47.91557627198102409 ) ) ;
#101538=CARTESIAN_POINT ( 'NONE',  ( -15.72974639402197994, 15.80617190586746368, 50.62390960531435979 ) ) ;
#101539=CARTESIAN_POINT ( 'NONE',  ( 8.224510206698953496, -14.34966873604960469, 57.91557627198103120 ) ) ;
#101540=CARTESIAN_POINT ( 'NONE',  ( 15.72974639402176855, 15.80617190586768217, 101.8760903946857042 ) ) ;
#101541=CARTESIAN_POINT ( 'NONE',  ( -16.51473224551069308, -9.474510206698971260, 111.6655762719810383 ) ) ;
#101542=CARTESIAN_POINT ( 'NONE',  ( -5.153800228976328057, -19.02544592524343514, 102.2905762719810383 ) ) ;
#101543=CARTESIAN_POINT ( 'NONE',  ( 19.05341960407611168, 5.049401038298154454, 43.95724293864769550 ) ) ;
#101544=CARTESIAN_POINT ( 'NONE',  ( -13.97604488694527625, -13.89961937509977652, 26.87390960531434558 ) ) ;
#101545=CARTESIAN_POINT ( 'NONE',  ( -12.14591786802309592, -12.06949235617757132, 81.87390960531435269 ) ) ;
#101546=CARTESIAN_POINT ( 'NONE',  ( -10.81492255796078084, -18.62759615963271287, 102.0822429386476955 ) ) ;
#101547=CARTESIAN_POINT ( 'NONE',  ( -5.153800228976328057, -19.02544592524343514, 97.29057627198099567 ) ) ;
#101548=CARTESIAN_POINT ( 'NONE',  ( -5.719274019375978568, 21.55341960407610458, 115.2072429386476955 ) ) ;
#101549=CARTESIAN_POINT ( 'NONE',  ( -19.03943276465977164, 0.05219959533909376836, 101.2489096053143669 ) ) ;
#101550=CARTESIAN_POINT ( 'NONE',  ( 17.59860650958994555, -7.585241751806880650, 65.92337014262493256 ) ) ;
#101551=CARTESIAN_POINT ( 'NONE',  ( 0.05219959533910956823, 16.53943276465976808, 104.9989096053143669 ) ) ;
#101552=CARTESIAN_POINT ( 'NONE',  ( -16.46253265017160317, 9.564922557960807481, 70.83224293864770971 ) ) ;
#101553=CARTESIAN_POINT ( 'NONE',  ( -18.67979575497178146, -10.72451020669898902, 76.66557627198103830 ) ) ;
#101556=CARTESIAN_POINT ( 'NONE',  ( 0.05219959533907565091, 21.53943276465977519, 24.99890960531435624 ) ) ;
#101557=CARTESIAN_POINT ( 'NONE',  ( 19.02130022317637881, -5.499999999999590550, 68.28188669246574705 ) ) ;
#101558=CARTESIAN_POINT ( 'NONE',  ( -8.224510206698735004, -14.34966873604973081, 39.58442372801901143 ) ) ;
#101559=CARTESIAN_POINT ( 'NONE',  ( 8.314922557960818139, 14.29746914071049879, 99.58224293864770971 ) ) ;
#101561=CARTESIAN_POINT ( 'NONE',  ( 19.49149378614662709, -5.499999999999593214, 51.93757513605365261 ) ) ;
#101562=CARTESIAN_POINT ( 'NONE',  ( 16.46253265017160672, -9.564922557960803928, 93.33224293864769550 ) ) ;
#101563=CARTESIAN_POINT ( 'NONE',  ( 9.564922557960805705, 16.46253265017160317, 59.58224293864769550 ) ) ;
#101564=CARTESIAN_POINT ( 'NONE',  ( -12.06949235617756955, 12.14591786802309770, 80.62390960531438111 ) ) ;
#101565=CARTESIAN_POINT ( 'NONE',  ( -18.62759615963270932, 10.81492255796079327, 35.83224293864768839 ) ) ;
#101566=CARTESIAN_POINT ( 'NONE',  ( 16.53943276465976808, -0.05219959533910856209, 53.74890960531437401 ) ) ;
#101567=CARTESIAN_POINT ( 'NONE',  ( 0.05219959533936267826, -19.03943276465977164, 110.0010903946856757 ) ) ;
#101568=CARTESIAN_POINT ( 'NONE',  ( 10.81492255796106328, -18.62759615963255655, 75.41775706135233293 ) ) ;
#101570=CARTESIAN_POINT ( 'NONE',  ( 17.50000000000000000, -5.499999999999992895, 76.21769037696435589 ) ) ;
#101571=CARTESIAN_POINT ( 'NONE',  ( 18.67979575497178502, 10.72451020669898547, 24.16557627198103120 ) ) ;
#101572=CARTESIAN_POINT ( 'NONE',  ( -16.52544592524335698, -4.483927247898792601, 88.95942372801901854 ) ) ;
#101573=CARTESIAN_POINT ( 'NONE',  ( -5.049401038298153566, 19.05341960407611168, 25.20724293864768484 ) ) ;
#101574=CARTESIAN_POINT ( 'NONE',  ( 5.049401038298161559, -19.05341960407611168, 87.70724293864769550 ) ) ;
#101575=CARTESIAN_POINT ( 'NONE',  ( -21.53943276465977519, 0.05219959533907696930, 91.24890960531436690 ) ) ;
#101577=CARTESIAN_POINT ( 'NONE',  ( -16.53943276465976808, -0.05219959533934237506, 28.75109039468567929 ) ) ;
#101578=CARTESIAN_POINT ( 'NONE',  ( -16.55341960407611168, -4.379528057220339221, 51.45724293864770260 ) ) ;
#101579=CARTESIAN_POINT ( 'NONE',  ( -21.55341960407619339, 5.719274019375674811, 73.54275706135234714 ) ) ;
#101581=CARTESIAN_POINT ( 'NONE',  ( -12.14591786802326823, 12.06949235617739902, 98.12609039468570415 ) ) ;
#101582=CARTESIAN_POINT ( 'NONE',  ( -18.62759615963270932, 10.81492255796079327, 30.83224293864770260 ) ) ;
#101583=CARTESIAN_POINT ( 'NONE',  ( -19.02544592524342804, 5.153800228976336939, 116.0405762719810383 ) ) ;
#101585=CARTESIAN_POINT ( 'NONE',  ( -0.05219959533934338120, 16.53943276465976808, 107.5010903946856899 ) ) ;
#101586=CARTESIAN_POINT ( 'NONE',  ( 8.314922557961029526, -14.29746914071037800, 60.41775706135235424 ) ) ;
#101587=CARTESIAN_POINT ( 'NONE',  ( 9.564922557960805705, 16.46253265017160317, 74.58224293864769550 ) ) ;
#101589=CARTESIAN_POINT ( 'NONE',  ( 19.02544592524343514, -5.153800228976328945, 88.54057627198102409 ) ) ;
#101590=CARTESIAN_POINT ( 'NONE',  ( 18.62759615963255655, 10.81492255796105972, 76.66775706135234714 ) ) ;
#101591=CARTESIAN_POINT ( 'NONE',  ( 4.483927247898790824, -16.52544592524335698, 75.20942372801901854 ) ) ;
#101592=CARTESIAN_POINT ( 'NONE',  ( -14.29746914071049879, 8.314922557960819915, 45.83224293864769550 ) ) ;
#101593=CARTESIAN_POINT ( 'NONE',  ( -13.89961937509977652, 13.97604488694528158, 55.62390960531434558 ) ) ;
#101595=CARTESIAN_POINT ( 'NONE',  ( -0.05219959533936034679, 19.03943276465977164, 112.5010903946856757 ) ) ;
#101596=CARTESIAN_POINT ( 'NONE',  ( 16.53943276465976808, -0.05219959533910856209, 113.7489096053143527 ) ) ;
#101597=CARTESIAN_POINT ( 'NONE',  ( 19.05341960407611168, 5.049401038298154454, 63.95724293864769550 ) ) ;
#101598=CARTESIAN_POINT ( 'NONE',  ( 13.97604488694548053, -13.89961937509957401, 100.6260903946856615 ) ) ;
#101600=CARTESIAN_POINT ( 'NONE',  ( -5.823673210054431948, 21.52544592524334988, 102.7094237280190185 ) ) ;
#101601=CARTESIAN_POINT ( 'NONE',  ( -12.14591786802326823, 12.06949235617739902, 83.12609039468568994 ) ) ;
#101602=CARTESIAN_POINT ( 'NONE',  ( -9.474510206698720793, -16.51473224551083518, 99.58442372801900433 ) ) ;
#101603=CARTESIAN_POINT ( 'NONE',  ( -5.823673210054116645, -21.52544592524344225, 62.29057627198102409 ) ) ;
#101604=CARTESIAN_POINT ( 'NONE',  ( -16.55341960407617563, 4.379528057220093196, 53.54275706135234714 ) ) ;
#101606=CARTESIAN_POINT ( 'NONE',  ( 13.89961937509957401, 13.97604488694547697, 56.87609039468564731 ) ) ;
#101607=CARTESIAN_POINT ( 'NONE',  ( 21.53943276465977519, 0.05219959533937863772, 91.25109039468568994 ) ) ;
#101608=CARTESIAN_POINT ( 'NONE',  ( -19.03943276465977164, 0.05219959533909376836, 31.24890960531435979 ) ) ;
#101609=CARTESIAN_POINT ( 'NONE',  ( 16.46253265017160672, -9.564922557960803928, 68.33224293864770971 ) ) ;
#101610=CARTESIAN_POINT ( 'NONE',  ( 16.55341960407611168, 4.379528057220329451, 58.95724293864770971 ) ) ;
#101612=CARTESIAN_POINT ( 'NONE',  ( -18.67979575497193778, 10.72451020669871902, 88.33442372801901854 ) ) ;
#101614=CARTESIAN_POINT ( 'NONE',  ( 5.049401038297881783, 19.05341960407617563, 47.29275706135231161 ) ) ;
#101615=CARTESIAN_POINT ( 'NONE',  ( 9.474510206698729675, 16.51473224551082808, 22.08442372801899722 ) ) ;
#101616=CARTESIAN_POINT ( 'NONE',  ( -13.89961937509977652, 13.97604488694528158, 115.6239096053143669 ) ) ;
#101617=CARTESIAN_POINT ( 'NONE',  ( 21.53943276465977519, 0.05219959533937863772, 91.25109039468568994 ) ) ;
#101618=CARTESIAN_POINT ( 'NONE',  ( -13.89961937509977652, 13.97604488694528158, 75.62390960531438111 ) ) ;
#101619=CARTESIAN_POINT ( 'NONE',  ( 5.719274019375673035, 21.55341960407619339, 87.29275706135236135 ) ) ;
#101620=CARTESIAN_POINT ( 'NONE',  ( 10.81492255796078972, 18.62759615963270932, 54.58224293864769550 ) ) ;
#101621=CARTESIAN_POINT ( 'NONE',  ( 16.51473224551069308, 9.474510206698969483, 79.16557627198103830 ) ) ;
#101622=CARTESIAN_POINT ( 'NONE',  ( -19.02544592524334988, -5.153800228976617603, 68.95942372801896170 ) ) ;
#101623=CARTESIAN_POINT ( 'NONE',  ( -19.02544592524342804, 5.153800228976336051, 46.04057627198101699 ) ) ;
#101624=CARTESIAN_POINT ( 'NONE',  ( -9.564922557960796823, -16.46253265017161027, 87.08224293864769550 ) ) ;
#101625=CARTESIAN_POINT ( 'NONE',  ( 19.02544592524334988, 5.153800228976608722, 96.45942372801897591 ) ) ;
#101626=CARTESIAN_POINT ( 'NONE',  ( 16.53943276465976808, 0.05219959533934440121, 46.25109039468567573 ) ) ;
#101627=CARTESIAN_POINT ( 'NONE',  ( 14.34966873604960469, 8.224510206698951720, 104.1655762719810241 ) ) ;
#101628=CARTESIAN_POINT ( 'NONE',  ( 16.46253265017160672, -9.564922557960803928, 68.33224293864770971 ) ) ;
#101629=CARTESIAN_POINT ( 'NONE',  ( -21.52544592524343514, 5.823673210054127303, 51.04057627198103120 ) ) ;
#101630=CARTESIAN_POINT ( 'NONE',  ( 4.483927247898790824, -16.52544592524335698, 35.20942372801901854 ) ) ;
#101631=CARTESIAN_POINT ( 'NONE',  ( 10.81492255796106328, -18.62759615963255655, 30.41775706135234358 ) ) ;
#101632=CARTESIAN_POINT ( 'NONE',  ( -5.719274019375665041, -21.55341960407619695, 89.79275706135236135 ) ) ;
#101633=CARTESIAN_POINT ( 'NONE',  ( 16.53943276465976808, 0.05219959533934440121, 86.25109039468568994 ) ) ;
#101634=CARTESIAN_POINT ( 'NONE',  ( 16.51473224551069308, 9.474510206698969483, 79.16557627198103830 ) ) ;
#101635=CARTESIAN_POINT ( 'NONE',  ( 14.29746914071037800, 8.314922557961029526, 101.6677570613523613 ) ) ;
#101636=CARTESIAN_POINT ( 'NONE',  ( 19.03943276465977164, 0.05219959533936151252, 56.25109039468566863 ) ) ;
#101637=CARTESIAN_POINT ( 'NONE',  ( -5.719274019375665041, -21.55341960407619695, 24.79275706135235779 ) ) ;
#101638=CARTESIAN_POINT ( 'NONE',  ( 4.379528057220339221, -16.55341960407611168, 77.70724293864770971 ) ) ;
#101639=CARTESIAN_POINT ( 'NONE',  ( -0.05219959533909027116, -19.03943276465977164, 97.49890960531436690 ) ) ;
#101640=CARTESIAN_POINT ( 'NONE',  ( -16.53943276465976808, -0.05219959533934237506, 103.7510903946857042 ) ) ;
#101641=CARTESIAN_POINT ( 'NONE',  ( -0.05219959533937732626, 21.53943276465977519, 67.50109039468568994 ) ) ;
#101642=CARTESIAN_POINT ( 'NONE',  ( 12.06949235617739724, 12.14591786802326823, 46.87609039468568994 ) ) ;
#101643=CARTESIAN_POINT ( 'NONE',  ( -5.823673210054431948, 21.52544592524334988, 32.70942372801900433 ) ) ;
#101644=CARTESIAN_POINT ( 'NONE',  ( 12.06949235617757843, -12.14591786802309237, 73.12390960531436690 ) ) ;
#101646=CARTESIAN_POINT ( 'NONE',  ( -10.81492255796105439, 18.62759615963255655, 22.91775706135235069 ) ) ;
#101647=CARTESIAN_POINT ( 'NONE',  ( 16.52544592524342804, -4.483927247898539470, 58.54057627198103120 ) ) ;
#101649=CARTESIAN_POINT ( 'NONE',  ( -21.52544592524343514, 5.823673210054127303, 31.04057627198102409 ) ) ;
#101650=CARTESIAN_POINT ( 'NONE',  ( 0.05219959533937995610, -21.53943276465977519, 45.00109039468568284 ) ) ;
#101651=CARTESIAN_POINT ( 'NONE',  ( 0.05219959533910956823, 16.53943276465976808, 59.99890960531436690 ) ) ;
#101652=CARTESIAN_POINT ( 'NONE',  ( 21.52544592524344225, -5.823673210054117533, 78.54057627198103830 ) ) ;
#101653=CARTESIAN_POINT ( 'NONE',  ( -19.05341960407611168, -5.049401038298163336, 71.45724293864766707 ) ) ;
#101654=CARTESIAN_POINT ( 'NONE',  ( 16.46253265017160672, -9.564922557960803928, 33.33224293864770260 ) ) ;
#101655=CARTESIAN_POINT ( 'NONE',  ( -5.153800228976607833, 19.02544592524334988, 82.70942372801897591 ) ) ;
#101657=CARTESIAN_POINT ( 'NONE',  ( 10.81492255796106328, -18.62759615963255655, 55.41775706135234714 ) ) ;
#101658=CARTESIAN_POINT ( 'NONE',  ( 21.53943276465977519, -0.05219959533907433946, 58.74890960531436690 ) ) ;
#101659=CARTESIAN_POINT ( 'NONE',  ( 13.97604488694527802, 13.89961937509977652, 44.37390960531435269 ) ) ;
#101660=CARTESIAN_POINT ( 'NONE',  ( -19.02544592524342804, 5.153800228976336051, 76.04057627198102409 ) ) ;
#101662=CARTESIAN_POINT ( 'NONE',  ( 4.379528057220092307, 16.55341960407617563, 47.29275706135234003 ) ) ;
#101663=CARTESIAN_POINT ( 'NONE',  ( 10.72451020669871369, 18.67979575497193778, 37.08442372801901143 ) ) ;
#101665=CARTESIAN_POINT ( 'NONE',  ( 0.05219959533937995610, -21.53943276465977519, 65.00109039468568994 ) ) ;
#101666=CARTESIAN_POINT ( 'NONE',  ( -5.153800228976328057, -19.02544592524343514, 102.2905762719810383 ) ) ;
#101667=CARTESIAN_POINT ( 'NONE',  ( -18.62759615963270932, 10.81492255796079327, 85.83224293864768129 ) ) ;
#101668=CARTESIAN_POINT ( 'NONE',  ( 10.81492255796106328, -18.62759615963255655, 20.41775706135234714 ) ) ;
#101669=CARTESIAN_POINT ( 'NONE',  ( -8.314922557961024197, 14.29746914071037800, 57.91775706135234714 ) ) ;
#101670=CARTESIAN_POINT ( 'NONE',  ( 18.67979575497178502, 10.72451020669898547, 44.16557627198103120 ) ) ;
#101671=CARTESIAN_POINT ( 'NONE',  ( -13.89961937509957401, -13.97604488694547875, 19.37609039468566507 ) ) ;
#101672=CARTESIAN_POINT ( 'NONE',  ( 19.05341960407611168, 5.049401038298154454, 53.95724293864770260 ) ) ;
#101673=CARTESIAN_POINT ( 'NONE',  ( 13.97604488694527802, 13.89961937509977652, 109.3739096053143669 ) ) ;
#101674=CARTESIAN_POINT ( 'NONE',  ( 0.05219959533909260263, 19.03943276465977164, 89.99890960531436690 ) ) ;
#101675=CARTESIAN_POINT ( 'NONE',  ( 5.049401038297881783, 19.05341960407617918, 52.29275706135233293 ) ) ;
#101676=CARTESIAN_POINT ( 'NONE',  ( -5.153800228976607833, 19.02544592524334988, 67.70942372801900433 ) ) ;
#101677=CARTESIAN_POINT ( 'NONE',  ( 10.81492255796078972, 18.62759615963270932, 49.58224293864769550 ) ) ;
#101678=CARTESIAN_POINT ( 'NONE',  ( 16.53943276465976808, -0.05219959533910856209, 28.74890960531435624 ) ) ;
#101679=CARTESIAN_POINT ( 'NONE',  ( -0.05219959533936034679, 19.03943276465977164, 92.50109039468566152 ) ) ;
#101681=AXIS2_PLACEMENT_3D ( 'NONE', #162018, #148860, #24525 ) ;
#101682=CARTESIAN_POINT ( 'NONE',  ( 10.81492255796106328, -18.62759615963255655, 110.4177570613523756 ) ) ;
#101683=CARTESIAN_POINT ( 'NONE',  ( -13.89961937509957401, -13.97604488694547875, 99.37609039468567573 ) ) ;
#101684=CARTESIAN_POINT ( 'NONE',  ( -9.474510206698720793, -16.51473224551083518, 49.58442372801899722 ) ) ;
#101686=CARTESIAN_POINT ( 'NONE',  ( -16.51473224551069308, -9.474510206698971260, 61.66557627198103120 ) ) ;
#101687=CARTESIAN_POINT ( 'NONE',  ( 8.224510206698953496, -14.34966873604960469, 47.91557627198102409 ) ) ;
#101688=CARTESIAN_POINT ( 'NONE',  ( 13.97604488694527802, 13.89961937509977652, 29.37390960531435979 ) ) ;
#101689=CARTESIAN_POINT ( 'NONE',  ( 16.53943276465976808, -0.05219959533910856209, 33.74890960531436690 ) ) ;
#101691=CARTESIAN_POINT ( 'NONE',  ( 14.29746914071037800, 8.314922557961029526, 101.6677570613523613 ) ) ;
#101692=CARTESIAN_POINT ( 'NONE',  ( -9.564922557960796823, -16.46253265017161027, 67.08224293864769550 ) ) ;
#101693=CARTESIAN_POINT ( 'NONE',  ( 19.03943276465977164, 0.05219959533936151252, 31.25109039468566863 ) ) ;
#101694=CARTESIAN_POINT ( 'NONE',  ( -12.06949235617739369, -12.14591786802326823, 34.37609039468568284 ) ) ;
#101695=CARTESIAN_POINT ( 'NONE',  ( -5.719274019375978568, 21.55341960407610458, 35.20724293864768839 ) ) ;
#101696=CARTESIAN_POINT ( 'NONE',  ( 18.62759615963255655, 10.81492255796105972, 101.6677570613523613 ) ) ;
#101697=CARTESIAN_POINT ( 'NONE',  ( -0.05219959533909027116, -19.03943276465977164, 62.49890960531435979 ) ) ;
#101698=CARTESIAN_POINT ( 'NONE',  ( -16.51473224551069308, -9.474510206698971260, 101.6655762719810241 ) ) ;
#101699=CARTESIAN_POINT ( 'NONE',  ( -13.97604488694527625, -13.89961937509977652, 101.8739096053143811 ) ) ;
#101701=CARTESIAN_POINT ( 'NONE',  ( 5.823673210054444382, -21.52544592524334988, 30.20942372801902565 ) ) ;
#101703=CARTESIAN_POINT ( 'NONE',  ( 12.14591786802309770, 12.06949235617756955, 89.37390960531435269 ) ) ;
#101704=CARTESIAN_POINT ( 'NONE',  ( 10.72451020669898902, -18.67979575497178502, 77.91557627198102409 ) ) ;
#101705=CARTESIAN_POINT ( 'NONE',  ( -13.97604488694527625, -13.89961937509977652, 71.87390960531433848 ) ) ;
#101706=CARTESIAN_POINT ( 'NONE',  ( 16.51473224551069308, 9.474510206698969483, 74.16557627198103830 ) ) ;
#101707=CARTESIAN_POINT ( 'NONE',  ( -15.80617190586745835, -15.72974639402198527, 106.8739096053143811 ) ) ;
#101709=CARTESIAN_POINT ( 'NONE',  ( 19.03943276465977164, -0.05219959533909143690, 78.74890960531436690 ) ) ;
#101711=CARTESIAN_POINT ( 'NONE',  ( -14.29746914071049879, 8.314922557960819915, 110.8322429386476955 ) ) ;
#101713=CARTESIAN_POINT ( 'NONE',  ( 13.89961937509977652, -13.97604488694527269, 63.12390960531435979 ) ) ;
#101714=CARTESIAN_POINT ( 'NONE',  ( 9.474510206698729675, 16.51473224551082808, 97.08442372801900433 ) ) ;
#101716=CARTESIAN_POINT ( 'NONE',  ( 4.379528057220339221, -16.55341960407611168, 97.70724293864772392 ) ) ;
#101717=CARTESIAN_POINT ( 'NONE',  ( 18.62759615963255655, 10.81492255796105972, 66.66775706135234714 ) ) ;
#101718=CARTESIAN_POINT ( 'NONE',  ( 19.02544592524343514, -5.153800228976328945, 53.54057627198102409 ) ) ;
#101719=CARTESIAN_POINT ( 'NONE',  ( -21.52544592524334988, -5.823673210054445271, 18.95942372801901143 ) ) ;
#101720=CARTESIAN_POINT ( 'NONE',  ( -10.72451020669898014, 18.67979575497178502, 115.4155762719810241 ) ) ;
#101722=CARTESIAN_POINT ( 'NONE',  ( -19.05341960407611168, -5.049401038298163336, 76.45724293864769550 ) ) ;
#101724=CARTESIAN_POINT ( 'NONE',  ( 16.38665767535055195, 7.295008042176099217, 112.2359913578545161 ) ) ;
#101725=CARTESIAN_POINT ( 'NONE',  ( 5.049401038297881783, 19.05341960407617563, 102.2927570613523045 ) ) ;
#101726=CARTESIAN_POINT ( 'NONE',  ( 15.80617190586746368, 15.72974639402197994, 34.37390960531435979 ) ) ;
#101727=CARTESIAN_POINT ( 'NONE',  ( -18.67979575497193778, 10.72451020669871902, 58.33442372801901143 ) ) ;
#101728=CARTESIAN_POINT ( 'NONE',  ( 0.05219959533910956823, 16.53943276465976808, 104.9989096053143669 ) ) ;
#101729=CARTESIAN_POINT ( 'NONE',  ( 19.03943276465977164, -0.05219959533909143690, 98.74890960531436690 ) ) ;
#101730=CARTESIAN_POINT ( 'NONE',  ( -5.049401038297874678, -19.05341960407617918, 79.79275706135233293 ) ) ;
#101731=CARTESIAN_POINT ( 'NONE',  ( 9.474510206698971260, -16.51473224551069308, 52.91557627198102409 ) ) ;
#101732=CARTESIAN_POINT ( 'NONE',  ( -19.02544592524342804, 5.153800228976336051, 66.04057627198103830 ) ) ;
#101733=CARTESIAN_POINT ( 'NONE',  ( -16.55341960407611168, -4.379528057220339221, 86.45724293864770971 ) ) ;
#101734=CARTESIAN_POINT ( 'NONE',  ( 19.05341960407611168, 5.049401038298154454, 103.9572429386476671 ) ) ;
#101735=CARTESIAN_POINT ( 'NONE',  ( 16.55341960407611168, 4.379528057220329451, 93.95724293864770971 ) ) ;
#101736=CARTESIAN_POINT ( 'NONE',  ( -9.474510206698964154, 16.51473224551069663, 95.41557627198102409 ) ) ;
#101737=CARTESIAN_POINT ( 'NONE',  ( -16.55341960407611168, -4.379528057220339221, 41.45724293864769550 ) ) ;
#101738=CARTESIAN_POINT ( 'NONE',  ( 0.05219959533909260263, 19.03943276465977164, 24.99890960531435269 ) ) ;
#101740=CARTESIAN_POINT ( 'NONE',  ( -5.719274019375665041, -21.55341960407619695, 54.79275706135235424 ) ) ;
#101741=CARTESIAN_POINT ( 'NONE',  ( -19.03943276465977164, -0.05219959533935918106, 73.75109039468566152 ) ) ;
#101742=CARTESIAN_POINT ( 'NONE',  ( -16.52544592524342804, 4.483927247898546575, 46.04057627198103830 ) ) ;
#101743=CARTESIAN_POINT ( 'NONE',  ( 5.719274019375991003, -21.55341960407610458, 102.7072429386476955 ) ) ;
#101744=CARTESIAN_POINT ( 'NONE',  ( -5.823673210054116645, -21.52544592524344225, 27.29057627198103120 ) ) ;
#101745=CARTESIAN_POINT ( 'NONE',  ( -16.53943276465976808, 0.05219959533911058130, 86.24890960531436690 ) ) ;
#101746=CARTESIAN_POINT ( 'NONE',  ( 16.46253265017160672, -9.564922557960803928, 53.33224293864768839 ) ) ;
#101747=CARTESIAN_POINT ( 'NONE',  ( -16.53943276465976808, 0.05219959533911058130, 26.24890960531435624 ) ) ;
#101749=CARTESIAN_POINT ( 'NONE',  ( -4.483927247898782831, 16.52544592524335698, 102.7094237280190185 ) ) ;
#101750=CARTESIAN_POINT ( 'NONE',  ( -16.52544592524335698, -4.483927247898792601, 68.95942372801901854 ) ) ;
#101751=CARTESIAN_POINT ( 'NONE',  ( -0.05219959533936034679, 19.03943276465977164, 27.50109039468566507 ) ) ;
#101752=CARTESIAN_POINT ( 'NONE',  ( 13.89961937509977652, -13.97604488694527269, 108.1239096053143669 ) ) ;
#101753=CARTESIAN_POINT ( 'NONE',  ( -19.03943276465977164, 0.05219959533909376836, 76.24890960531435269 ) ) ;
#101754=CARTESIAN_POINT ( 'NONE',  ( -16.51473224551069308, -9.474510206698971260, 36.66557627198102409 ) ) ;
#101755=CARTESIAN_POINT ( 'NONE',  ( 8.224510206698953496, -14.34966873604960469, 42.91557627198103120 ) ) ;
#101757=CARTESIAN_POINT ( 'NONE',  ( 5.153800228976335163, 19.02544592524342804, 99.79057627198102409 ) ) ;
#101758=CARTESIAN_POINT ( 'NONE',  ( -21.55341960407610458, -5.719274019375992779, 36.45724293864768839 ) ) ;
#101759=CARTESIAN_POINT ( 'NONE',  ( 12.14591786802309770, 12.06949235617756955, 69.37390960531436690 ) ) ;
#101760=CARTESIAN_POINT ( 'NONE',  ( 16.55341960407618274, -4.379528057220086978, 26.04275706135235779 ) ) ;
#101761=EDGE_CURVE ( 'NONE', #78133, #18983, #22596, .T. ) ;
#101762=CARTESIAN_POINT ( 'NONE',  ( 16.53943276465976808, -0.05219959533910856209, 68.74890960531435269 ) ) ;
#101764=CARTESIAN_POINT ( 'NONE',  ( 13.97604488694548053, -13.89961937509957401, 70.62609039468567573 ) ) ;
#101765=CARTESIAN_POINT ( 'NONE',  ( -19.05341960407611168, -5.049401038298163336, 101.4572429386476955 ) ) ;
#101766=CARTESIAN_POINT ( 'NONE',  ( -9.564922557961040184, 16.46253265017147172, 77.91775706135234714 ) ) ;
#101768=CARTESIAN_POINT ( 'NONE',  ( 13.89961937509957401, 13.97604488694547697, 106.8760903946856757 ) ) ;
#101769=CARTESIAN_POINT ( 'NONE',  ( -12.14591786802326823, 12.06949235617739902, 93.12609039468568994 ) ) ;
#101770=CARTESIAN_POINT ( 'NONE',  ( -13.97604488694527625, -13.89961937509977652, 36.87390960531436690 ) ) ;
#101771=CARTESIAN_POINT ( 'NONE',  ( 0.05219959533907565091, 21.53943276465977519, 29.99890960531435979 ) ) ;
#101772=CARTESIAN_POINT ( 'NONE',  ( 18.62759615963255655, 10.81492255796105972, 56.66775706135235424 ) ) ;
#101774=CARTESIAN_POINT ( 'NONE',  ( 8.314922557961029526, -14.29746914071037800, 20.41775706135234714 ) ) ;
#101776=CARTESIAN_POINT ( 'NONE',  ( 19.05341960407611168, 5.049401038298154454, 68.95724293864769550 ) ) ;
#101777=CARTESIAN_POINT ( 'NONE',  ( -19.03943276465977164, 0.05219959533909376836, 116.2489096053143669 ) ) ;
#101778=CARTESIAN_POINT ( 'NONE',  ( 14.34966873604960469, 8.224510206698951720, 89.16557627198102409 ) ) ;
#101779=CARTESIAN_POINT ( 'NONE',  ( -19.05341960407611168, -5.049401038298163336, 76.45724293864769550 ) ) ;
#101780=CARTESIAN_POINT ( 'NONE',  ( 13.89961937509977652, -13.97604488694527269, 93.12390960531436690 ) ) ;
#101782=CARTESIAN_POINT ( 'NONE',  ( 19.02544592524334988, 5.153800228976608722, 96.45942372801897591 ) ) ;
#101783=CARTESIAN_POINT ( 'NONE',  ( -21.52544592524343514, 5.823673210054127303, 61.04057627198103120 ) ) ;
#101784=CARTESIAN_POINT ( 'NONE',  ( 16.46253265017160672, -9.564922557960803928, 28.33224293864769550 ) ) ;
#101785=CARTESIAN_POINT ( 'NONE',  ( 19.03943276465977164, 0.05219959533936151252, 51.25109039468567573 ) ) ;
#101786=CARTESIAN_POINT ( 'NONE',  ( -9.564922557960796823, -16.46253265017161027, 57.08224293864769550 ) ) ;
#101787=CARTESIAN_POINT ( 'NONE',  ( 0.05219959533909260263, 19.03943276465977164, 94.99890960531436690 ) ) ;
#101789=CARTESIAN_POINT ( 'NONE',  ( 21.52544592524344225, -5.823673210054117533, 88.54057627198103830 ) ) ;
#101790=CARTESIAN_POINT ( 'NONE',  ( 14.29746914071049879, -8.314922557960816363, 98.33224293864769550 ) ) ;
#101791=CARTESIAN_POINT ( 'NONE',  ( 9.564922557961047289, -16.46253265017146816, 65.41775706135233293 ) ) ;
#101792=CARTESIAN_POINT ( 'NONE',  ( -5.719274019375978568, 21.55341960407610458, 95.20724293864769550 ) ) ;
#101793=CARTESIAN_POINT ( 'NONE',  ( 18.62759615963271287, -10.81492255796078972, 78.33224293864770971 ) ) ;
#101795=CARTESIAN_POINT ( 'NONE',  ( -4.483927247898539470, -16.52544592524342804, 27.29057627198103120 ) ) ;
#101796=CARTESIAN_POINT ( 'NONE',  ( 15.72974639402176855, 15.80617190586768217, 106.8760903946856899 ) ) ;
#101797=CARTESIAN_POINT ( 'NONE',  ( -0.05219959533934338120, 16.53943276465976808, 52.50109039468567573 ) ) ;
#101798=CARTESIAN_POINT ( 'NONE',  ( 16.46253265017160672, -9.564922557960803928, 83.33224293864768129 ) ) ;
#101799=CARTESIAN_POINT ( 'NONE',  ( -5.153800228976328057, -19.02544592524343514, 27.29057627198103120 ) ) ;
#101800=CARTESIAN_POINT ( 'NONE',  ( 5.823673210054444382, -21.52544592524334988, 40.20942372801901854 ) ) ;
#101801=CARTESIAN_POINT ( 'NONE',  ( 15.80617190586769283, -15.72974639402175789, 50.62609039468568994 ) ) ;
#101802=CARTESIAN_POINT ( 'NONE',  ( 19.05341960407611168, 5.049401038298154454, 43.95724293864769550 ) ) ;
#101803=CARTESIAN_POINT ( 'NONE',  ( -21.52544592524334988, -5.823673210054445271, 23.95942372801901143 ) ) ;
#101804=CARTESIAN_POINT ( 'NONE',  ( -0.05219959533936034679, 19.03943276465977164, 62.50109039468566863 ) ) ;
#101805=CARTESIAN_POINT ( 'NONE',  ( 9.474510206698729675, 16.51473224551082808, 72.08442372801900433 ) ) ;
#101806=CARTESIAN_POINT ( 'NONE',  ( 8.224510206698742110, 14.34966873604972548, 32.08442372801901854 ) ) ;
#101807=CARTESIAN_POINT ( 'NONE',  ( -9.564922557960796823, -16.46253265017161027, 22.08224293864768839 ) ) ;
#101808=CARTESIAN_POINT ( 'NONE',  ( -8.224510206698735004, -14.34966873604973081, 79.58442372801903275 ) ) ;
#101809=CARTESIAN_POINT ( 'NONE',  ( 5.049401038298161559, -19.05341960407611168, 42.70724293864767418 ) ) ;
#101811=CARTESIAN_POINT ( 'NONE',  ( -13.89961937509977652, 13.97604488694528158, 105.6239096053143527 ) ) ;
#101812=CARTESIAN_POINT ( 'NONE',  ( -5.153800228976328057, -19.02544592524343514, 27.29057627198103120 ) ) ;
#101813=CARTESIAN_POINT ( 'NONE',  ( 10.72451020669898902, -18.67979575497178502, 77.91557627198102409 ) ) ;
#101814=CARTESIAN_POINT ( 'NONE',  ( 16.52544592524335698, 4.483927247898782831, 61.45942372801901854 ) ) ;
#101815=CARTESIAN_POINT ( 'NONE',  ( 0.05219959533936267826, -19.03943276465977164, 20.00109039468567218 ) ) ;
#101816=CARTESIAN_POINT ( 'NONE',  ( 5.153800228976335163, 19.02544592524342804, 49.79057627198100988 ) ) ;
#101817=CARTESIAN_POINT ( 'NONE',  ( 4.379528057220339221, -16.55341960407611168, 37.70724293864769550 ) ) ;
#101818=CARTESIAN_POINT ( 'NONE',  ( 14.34966873604960469, 8.224510206698951720, 64.16557627198102409 ) ) ;
#101819=CARTESIAN_POINT ( 'NONE',  ( 5.153800228976335163, 19.02544592524342804, 84.79057627198099567 ) ) ;
#101820=CARTESIAN_POINT ( 'NONE',  ( -10.81492255796105439, 18.62759615963255655, 42.91775706135235424 ) ) ;
#101821=CARTESIAN_POINT ( 'NONE',  ( -19.02544592524342804, 5.153800228976336051, 86.04057627198103830 ) ) ;
#101822=CARTESIAN_POINT ( 'NONE',  ( 5.719274019375673035, 21.55341960407619339, 87.29275706135236135 ) ) ;
#101823=CARTESIAN_POINT ( 'NONE',  ( 8.314922557961029526, -14.29746914071037800, 70.41775706135236135 ) ) ;
#101824=CARTESIAN_POINT ( 'NONE',  ( -13.97604488694527625, -13.89961937509977652, 106.8739096053143669 ) ) ;
#101825=CARTESIAN_POINT ( 'NONE',  ( -18.67979575497178146, -10.72451020669898902, 91.66557627198103830 ) ) ;
#101826=CARTESIAN_POINT ( 'NONE',  ( -8.224510206698948167, 14.34966873604960824, 45.41557627198103830 ) ) ;
#101827=CARTESIAN_POINT ( 'NONE',  ( 9.474510206698971260, -16.51473224551069308, 22.91557627198102765 ) ) ;
#101828=CARTESIAN_POINT ( 'NONE',  ( -16.55341960407617563, 4.379528057220093196, 53.54275706135234714 ) ) ;
#101829=CARTESIAN_POINT ( 'NONE',  ( 12.14591786802309770, 12.06949235617756955, 54.37390960531435979 ) ) ;
#101830=CARTESIAN_POINT ( 'NONE',  ( 16.51473224551069308, 9.474510206698969483, 114.1655762719810241 ) ) ;
#101831=CARTESIAN_POINT ( 'NONE',  ( -0.05219959533907301413, -21.53943276465977519, 37.49890960531436690 ) ) ;
#101832=CARTESIAN_POINT ( 'NONE',  ( 18.67979575497194134, -10.72451020669871369, 110.8344237280190043 ) ) ;
#101833=CARTESIAN_POINT ( 'NONE',  ( -4.483927247898539470, -16.52544592524342804, 97.29057627198105251 ) ) ;
#101834=CARTESIAN_POINT ( 'NONE',  ( -5.153800228976328057, -19.02544592524343514, 92.29057627198099567 ) ) ;
#101836=CARTESIAN_POINT ( 'NONE',  ( -14.29746914071037622, -8.314922557961029526, 49.16775706135234003 ) ) ;
#101837=CARTESIAN_POINT ( 'NONE',  ( -9.474510206698964154, 16.51473224551069663, 60.41557627198102409 ) ) ;
#101838=CARTESIAN_POINT ( 'NONE',  ( 5.049401038297881783, 19.05341960407617563, 52.29275706135234003 ) ) ;
#101840=CARTESIAN_POINT ( 'NONE',  ( 16.52544592524335698, 4.483927247898782831, 91.45942372801901854 ) ) ;
#101841=CARTESIAN_POINT ( 'NONE',  ( 9.564922557961047289, -16.46253265017146816, 95.41775706135233293 ) ) ;
#101842=CARTESIAN_POINT ( 'NONE',  ( 15.80617190586769283, -15.72974639402175789, 70.62609039468567573 ) ) ;
#101843=CARTESIAN_POINT ( 'NONE',  ( -5.049401038298153566, 19.05341960407611168, 80.20724293864769550 ) ) ;
#101844=CARTESIAN_POINT ( 'NONE',  ( -15.72974639402197994, 15.80617190586746368, 95.62390960531436690 ) ) ;
#101845=CARTESIAN_POINT ( 'NONE',  ( -12.06949235617756955, 12.14591786802309770, 115.6239096053143669 ) ) ;
#101848=B_SPLINE_CURVE_WITH_KNOTS ( 'NONE', 3,
 ( #157019, #97304, #2334, #64015, #174188, #158011, #187382, #35656, #48851, #110506, #80164, #65001, #81147, #4308, #50837, #112494, #158990, #67984, #159999, #129638, #177192, #99317 ),
 .UNSPECIFIED., .F., .F.,
 ( 4, 2, 2, 2, 2, 2, 2, 2, 2, 2, 4 ),
 ( 1.127570259384924457E-17, 0.001309639967555342515, 0.001964459951333006292, 0.002291869943221834169, 0.002455574939166242036, 0.002619279935110649469, 0.002782984931055057336, 0.002946689926999464769, 0.003274099918888280069, 0.003928919902665910235, 0.005238559870221172303 ),
 .UNSPECIFIED. ) ;
#101849=CARTESIAN_POINT ( 'NONE',  ( 5.153800228976615827, -19.02544592524334988, 75.20942372801896170 ) ) ;
#101850=CARTESIAN_POINT ( 'NONE',  ( -18.62759615963270932, 10.81492255796079327, 75.83224293864769550 ) ) ;
#101851=CARTESIAN_POINT ( 'NONE',  ( 13.97604488694548053, -13.89961937509957401, 40.62609039468564731 ) ) ;
#101852=CARTESIAN_POINT ( 'NONE',  ( 19.49190055781011566, 5.500000000000002665, 98.06116087098784817 ) ) ;
#101853=CARTESIAN_POINT ( 'NONE',  ( 10.81492255796078972, 18.62759615963270932, 94.58224293864769550 ) ) ;
#101854=CARTESIAN_POINT ( 'NONE',  ( -17.26172910966778318, 6.454744622555849354, 85.80646908649221416 ) ) ;
#101855=CARTESIAN_POINT ( 'NONE',  ( -0.05219959533909027116, -19.03943276465977164, 62.49890960531435979 ) ) ;
#101856=CARTESIAN_POINT ( 'NONE',  ( -17.97058386085788939, -5.499999999999976019, 89.00390968646220813 ) ) ;
#101857=CARTESIAN_POINT ( 'NONE',  ( 16.52544592524335698, 4.483927247898782831, 26.45942372801901854 ) ) ;
#101858=DIRECTION ( 'NONE',  ( 0.000000000000000000, 0.000000000000000000, 1.000000000000000000 ) ) ;
#101859=CARTESIAN_POINT ( 'NONE',  ( -16.46253265017160317, 9.564922557960807481, 40.83224293864769550 ) ) ;
#101860=CARTESIAN_POINT ( 'NONE',  ( -5.049401038298153566, 19.05341960407611168, 115.2072429386477097 ) ) ;
#101861=CARTESIAN_POINT ( 'NONE',  ( -18.67979575497178146, -10.72451020669898902, 101.6655762719810383 ) ) ;
#101862=CARTESIAN_POINT ( 'NONE',  ( 8.314922557960818139, 14.29746914071049879, 44.58224293864769550 ) ) ;
#101863=CIRCLE ( 'NONE', #189054, 2.000000000000001776 ) ;
#101864=CARTESIAN_POINT ( 'NONE',  ( 21.52544592524334988, 5.823673210054432836, 71.45942372801901854 ) ) ;
#101865=CARTESIAN_POINT ( 'NONE',  ( 16.53943276465976808, 0.05219959533934440121, 21.25109039468567218 ) ) ;
#101866=CARTESIAN_POINT ( 'NONE',  ( -13.89961937509957401, -13.97604488694547875, 34.37609039468566863 ) ) ;
#101867=CARTESIAN_POINT ( 'NONE',  ( 16.55341960407611168, 4.379528057220329451, 33.95724293864769550 ) ) ;
#101868=CARTESIAN_POINT ( 'NONE',  ( -21.52544592524343514, 5.823673210054127303, 111.0405762719810525 ) ) ;
#101869=CARTESIAN_POINT ( 'NONE',  ( -14.34966873604960291, -8.224510206698953496, 46.66557627198102409 ) ) ;
#101870=CARTESIAN_POINT ( 'NONE',  ( 0.05219959533936267826, -19.03943276465977164, 90.00109039468567573 ) ) ;
#101871=CARTESIAN_POINT ( 'NONE',  ( 19.03943276465977164, 0.05219959533936151252, 66.25109039468567573 ) ) ;
#101873=CARTESIAN_POINT ( 'NONE',  ( 5.823673210054444382, -21.52544592524334988, 65.20942372801901854 ) ) ;
#101874=CARTESIAN_POINT ( 'NONE',  ( -9.564922557961040184, 16.46253265017147172, 47.91775706135233293 ) ) ;
#101875=CARTESIAN_POINT ( 'NONE',  ( 16.52544592524342804, -4.483927247898539470, 113.5405762719810383 ) ) ;
#101876=CARTESIAN_POINT ( 'NONE',  ( -21.53943276465977519, 0.05219959533907696930, 46.24890960531435979 ) ) ;
#101877=CARTESIAN_POINT ( 'NONE',  ( 14.29746914071049879, -8.314922557960816363, 43.33224293864769550 ) ) ;
#101878=CARTESIAN_POINT ( 'NONE',  ( -17.05116617787823685, -6.768360034955907878, 26.34324446740804859 ) ) ;
#101879=CARTESIAN_POINT ( 'NONE',  ( -5.823673210054431948, 21.52544592524334988, 112.7094237280190328 ) ) ;
#101880=CARTESIAN_POINT ( 'NONE',  ( -12.06949235617739369, -12.14591786802326823, 79.37609039468567573 ) ) ;
#101881=CARTESIAN_POINT ( 'NONE',  ( 0.05219959533910956823, 16.53943276465976808, 39.99890960531436690 ) ) ;
#101882=CARTESIAN_POINT ( 'NONE',  ( 18.67979575497194134, -10.72451020669871369, 80.83442372801901854 ) ) ;
#101883=CARTESIAN_POINT ( 'NONE',  ( -0.05219959533937732626, 21.53943276465977519, 72.50109039468568994 ) ) ;
#101884=CARTESIAN_POINT ( 'NONE',  ( -10.72451020669898014, 18.67979575497178502, 80.41557627198103830 ) ) ;
#101885=CARTESIAN_POINT ( 'NONE',  ( 19.05341960407611168, 5.049401038298154454, 43.95724293864769550 ) ) ;
#101886=CARTESIAN_POINT ( 'NONE',  ( 0.05219959533937995610, -21.53943276465977519, 55.00109039468568284 ) ) ;
#101887=CARTESIAN_POINT ( 'NONE',  ( 19.03943276465977164, -0.05219959533909143690, 38.74890960531436690 ) ) ;
#101888=CARTESIAN_POINT ( 'NONE',  ( 5.049401038298161559, -19.05341960407611168, 52.70724293864767418 ) ) ;
#101889=CARTESIAN_POINT ( 'NONE',  ( 16.53943276465976808, -0.05219959533910856209, 98.74890960531438111 ) ) ;
#101890=CARTESIAN_POINT ( 'NONE',  ( -5.049401038298153566, 19.05341960407611168, 100.2072429386476955 ) ) ;
#101891=CARTESIAN_POINT ( 'NONE',  ( 4.379528057220339221, -16.55341960407611168, 37.70724293864769550 ) ) ;
#101892=CARTESIAN_POINT ( 'NONE',  ( -12.14591786802309592, -12.06949235617757132, 101.8739096053143811 ) ) ;
#101893=CARTESIAN_POINT ( 'NONE',  ( 21.52544592524344225, -5.823673210054117533, 73.54057627198102409 ) ) ;
#101894=CARTESIAN_POINT ( 'NONE',  ( 18.67979575497194134, -10.72451020669871369, 20.83442372801901143 ) ) ;
#101895=CARTESIAN_POINT ( 'NONE',  ( -19.03943276465977164, 0.05219959533909376836, 116.2489096053143669 ) ) ;
#101896=CARTESIAN_POINT ( 'NONE',  ( -16.46253265017160317, 9.564922557960807481, 80.83224293864769550 ) ) ;
#101897=CARTESIAN_POINT ( 'NONE',  ( 12.06949235617739724, 12.14591786802326823, 21.87609039468567573 ) ) ;
#101898=CARTESIAN_POINT ( 'NONE',  ( 5.823673210054125526, 21.52544592524343514, 69.79057627198102409 ) ) ;
#101899=CARTESIAN_POINT ( 'NONE',  ( 18.62759615963255655, 10.81492255796105972, 96.66775706135234714 ) ) ;
#101900=CARTESIAN_POINT ( 'NONE',  ( -19.03943276465977164, 0.05219959533909376836, 76.24890960531435269 ) ) ;
#101901=CARTESIAN_POINT ( 'NONE',  ( 21.55341960407619695, -5.719274019375665929, 36.04275706135234714 ) ) ;
#101902=CARTESIAN_POINT ( 'NONE',  ( -5.823673210054116645, -21.52544592524344225, 22.29057627198102765 ) ) ;
#101903=CARTESIAN_POINT ( 'NONE',  ( 14.34966873604972726, -8.224510206698740333, 85.83442372801901854 ) ) ;
#101904=CARTESIAN_POINT ( 'NONE',  ( 5.719274019375673035, 21.55341960407619339, 67.29275706135234714 ) ) ;
#101905=CARTESIAN_POINT ( 'NONE',  ( -21.53943276465977519, -0.05219959533937600094, 103.7510903946857042 ) ) ;
#101906=CARTESIAN_POINT ( 'NONE',  ( -12.14591786802326823, 12.06949235617739902, 58.12609039468568994 ) ) ;
#101907=CARTESIAN_POINT ( 'NONE',  ( 21.55341960407619695, -5.719274019375665929, 26.04275706135235779 ) ) ;
#101908=CARTESIAN_POINT ( 'NONE',  ( 19.05341960407611168, 5.049401038298154454, 113.9572429386477097 ) ) ;
#101909=CARTESIAN_POINT ( 'NONE',  ( -5.719274019375665041, -21.55341960407619695, 94.79275706135234714 ) ) ;
#101910=CARTESIAN_POINT ( 'NONE',  ( 13.89961937509977652, -13.97604488694527269, 88.12390960531438111 ) ) ;
#101911=CARTESIAN_POINT ( 'NONE',  ( 21.55341960407610458, 5.719274019375980345, 83.95724293864770971 ) ) ;
#101912=CARTESIAN_POINT ( 'NONE',  ( 5.049401038297881783, 19.05341960407617563, 62.29275706135234003 ) ) ;
#101914=CARTESIAN_POINT ( 'NONE',  ( -10.81492255796078084, -18.62759615963271287, 47.08224293864770260 ) ) ;
#101915=CARTESIAN_POINT ( 'NONE',  ( 13.97604488694527802, 13.89961937509977652, 89.37390960531436690 ) ) ;
#101916=CARTESIAN_POINT ( 'NONE',  ( 0.05219959533910956823, 16.53943276465976808, 29.99890960531435979 ) ) ;
#101918=CARTESIAN_POINT ( 'NONE',  ( -5.153800228976607833, 19.02544592524334988, 72.70942372801900433 ) ) ;
#101920=CARTESIAN_POINT ( 'NONE',  ( -9.564922557961040184, 16.46253265017147172, 107.9177570613523471 ) ) ;
#101921=CARTESIAN_POINT ( 'NONE',  ( 0.05219959533907565091, 21.53943276465977519, 89.99890960531438111 ) ) ;
#101922=CARTESIAN_POINT ( 'NONE',  ( -12.06949235617756955, 12.14591786802309770, 60.62390960531437401 ) ) ;
#101923=CARTESIAN_POINT ( 'NONE',  ( -9.474510206698964154, 16.51473224551069663, 105.4155762719810383 ) ) ;
#101924=CARTESIAN_POINT ( 'NONE',  ( 0.05219959533934541429, -16.53943276465976808, 25.00109039468567218 ) ) ;
#101925=CARTESIAN_POINT ( 'NONE',  ( -5.049401038298153566, 19.05341960407611168, 60.20724293864768129 ) ) ;
#101926=CARTESIAN_POINT ( 'NONE',  ( 15.80617190586769283, -15.72974639402175789, 20.62609039468568639 ) ) ;
#101927=CARTESIAN_POINT ( 'NONE',  ( -13.89961937509957401, -13.97604488694547875, 79.37609039468567573 ) ) ;
#101928=CARTESIAN_POINT ( 'NONE',  ( 9.564922557960805705, 16.46253265017160317, 89.58224293864769550 ) ) ;
#101929=CARTESIAN_POINT ( 'NONE',  ( -16.46253265017160317, 9.564922557960807481, 80.83224293864769550 ) ) ;
#101930=CARTESIAN_POINT ( 'NONE',  ( -21.52544592524343514, 5.823673210054127303, 71.04057627198103830 ) ) ;
#101931=CARTESIAN_POINT ( 'NONE',  ( 9.474510206698971260, -16.51473224551069308, 47.91557627198102409 ) ) ;
#101933=CARTESIAN_POINT ( 'NONE',  ( -14.29746914071049879, 8.314922557960819915, 50.83224293864770971 ) ) ;
#101934=CARTESIAN_POINT ( 'NONE',  ( 13.89961937509977652, -13.97604488694527269, 108.1239096053143669 ) ) ;
#101936=CARTESIAN_POINT ( 'NONE',  ( -13.89961937509957401, -13.97604488694547875, 64.37609039468567573 ) ) ;
#101938=CARTESIAN_POINT ( 'NONE',  ( 5.823673210054125526, 21.52544592524343514, 94.79057627198105251 ) ) ;
#101939=CARTESIAN_POINT ( 'NONE',  ( -19.05341960407617563, 5.049401038297882671, 53.54275706135231871 ) ) ;
#101940=CARTESIAN_POINT ( 'NONE',  ( -0.05219959533909027116, -19.03943276465977164, 107.4989096053143527 ) ) ;
#101942=CARTESIAN_POINT ( 'NONE',  ( 18.67979575497178502, 10.72451020669898547, 39.16557627198102409 ) ) ;
#101943=CARTESIAN_POINT ( 'NONE',  ( -5.153800228976328057, -19.02544592524343514, 77.29057627198099567 ) ) ;
#101944=CARTESIAN_POINT ( 'NONE',  ( -10.81492255796105439, 18.62759615963255655, 62.91775706135236135 ) ) ;
#101945=CARTESIAN_POINT ( 'NONE',  ( 19.02544592524343514, -5.153800228976328945, 33.54057627198102409 ) ) ;
#101946=CARTESIAN_POINT ( 'NONE',  ( 14.34966873604960469, 8.224510206698951720, 74.16557627198102409 ) ) ;
#101948=CARTESIAN_POINT ( 'NONE',  ( -18.67979575497193778, 10.72451020669871902, 58.33442372801901143 ) ) ;
#101950=CARTESIAN_POINT ( 'NONE',  ( -5.049401038298153566, 19.05341960407611168, 110.2072429386476671 ) ) ;
#101951=CARTESIAN_POINT ( 'NONE',  ( 5.049401038297881783, 19.05341960407617563, 67.29275706135234714 ) ) ;
#101953=CARTESIAN_POINT ( 'NONE',  ( 18.62759615963255655, 10.81492255796105972, 26.66775706135235424 ) ) ;
#101954=CARTESIAN_POINT ( 'NONE',  ( 0.05219959533909260263, 19.03943276465977164, 64.99890960531436690 ) ) ;
#101955=CARTESIAN_POINT ( 'NONE',  ( -8.314922557961024197, 14.29746914071037800, 32.91775706135234714 ) ) ;
#101958=CARTESIAN_POINT ( 'NONE',  ( 5.153800228976615827, -19.02544592524334988, 20.20942372801899722 ) ) ;
#101959=CARTESIAN_POINT ( 'NONE',  ( 9.564922557960805705, 16.46253265017160317, 39.58224293864768839 ) ) ;
#101960=CARTESIAN_POINT ( 'NONE',  ( -10.72451020669870658, -18.67979575497194134, 109.5844237280190328 ) ) ;
#101961=CARTESIAN_POINT ( 'NONE',  ( -16.53943276465976808, -0.05219959533934237506, 88.75109039468567573 ) ) ;
#101962=CARTESIAN_POINT ( 'NONE',  ( 13.89961937509977652, -13.97604488694527269, 93.12390960531436690 ) ) ;
#101963=CARTESIAN_POINT ( 'NONE',  ( -10.81492255796105439, 18.62759615963255655, 72.91775706135234714 ) ) ;
#101965=CARTESIAN_POINT ( 'NONE',  ( -19.03943276465977164, 0.05219959533909376836, 106.2489096053143669 ) ) ;
#101966=CARTESIAN_POINT ( 'NONE',  ( 30.00000000000000000, 5.499999999999992895, 102.5000000000000142 ) ) ;
#101967=CARTESIAN_POINT ( 'NONE',  ( 4.483927247898790824, -16.52544592524335698, 50.20942372801901854 ) ) ;
#101968=CARTESIAN_POINT ( 'NONE',  ( 10.72451020669871369, 18.67979575497193778, 77.08442372801901854 ) ) ;
#101969=CARTESIAN_POINT ( 'NONE',  ( 21.52544592524334988, 5.823673210054432836, 96.45942372801901854 ) ) ;
#101971=CARTESIAN_POINT ( 'NONE',  ( -16.55341960407617563, 4.379528057220093196, 33.54275706135234714 ) ) ;
#101972=CARTESIAN_POINT ( 'NONE',  ( -13.89961937509977652, 13.97604488694528158, 90.62390960531432427 ) ) ;
#101973=CARTESIAN_POINT ( 'NONE',  ( -13.89961937509977652, 13.97604488694528158, 115.6239096053143669 ) ) ;
#101976=DIRECTION ( 'NONE',  ( -1.000000000000000000, -0.000000000000000000, -0.000000000000000000 ) ) ;
#101977=CARTESIAN_POINT ( 'NONE',  ( 13.97604488694527802, 13.89961937509977652, 29.37390960531435979 ) ) ;
#101978=CARTESIAN_POINT ( 'NONE',  ( -21.55341960407610458, -5.719274019375992779, 41.45724293864769550 ) ) ;
#101979=CARTESIAN_POINT ( 'NONE',  ( -0.05219959533934338120, 16.53943276465976808, 102.5010903946856899 ) ) ;
#101980=CARTESIAN_POINT ( 'NONE',  ( -16.55341960407611168, -4.379528057220339221, 86.45724293864770971 ) ) ;
#101981=CARTESIAN_POINT ( 'NONE',  ( 0.05219959533909260263, 19.03943276465977164, 69.99890960531435269 ) ) ;
#101982=CARTESIAN_POINT ( 'NONE',  ( -0.05219959533937732626, 21.53943276465977519, 107.5010903946856899 ) ) ;
#101983=CARTESIAN_POINT ( 'NONE',  ( 12.14591786802327356, -12.06949235617739191, 20.62609039468568639 ) ) ;
#101984=CARTESIAN_POINT ( 'NONE',  ( 4.379528057220339221, -16.55341960407611168, 82.70724293864770971 ) ) ;
#101985=CARTESIAN_POINT ( 'NONE',  ( -5.719274019375665041, -21.55341960407619695, 39.79275706135235424 ) ) ;
#101986=CARTESIAN_POINT ( 'NONE',  ( 5.823673210054125526, 21.52544592524343514, 79.79057627198102409 ) ) ;
#101987=CARTESIAN_POINT ( 'NONE',  ( -13.89961937509957401, -13.97604488694547875, 54.37609039468565442 ) ) ;
#101988=CARTESIAN_POINT ( 'NONE',  ( -13.89961937509977830, 13.97604488694528158, 45.62390960531435269 ) ) ;
#101989=CARTESIAN_POINT ( 'NONE',  ( -9.564922557960796823, -16.46253265017161027, 97.08224293864769550 ) ) ;
#101990=CARTESIAN_POINT ( 'NONE',  ( 14.29746914071049879, -8.314922557960816363, 68.33224293864769550 ) ) ;
#101991=CARTESIAN_POINT ( 'NONE',  ( -14.34966873604960291, -8.224510206698953496, 46.66557627198102409 ) ) ;
#101992=CARTESIAN_POINT ( 'NONE',  ( 14.34966873604960469, 8.224510206698951720, 24.16557627198103120 ) ) ;
#101993=CARTESIAN_POINT ( 'NONE',  ( -13.97604488694547697, 13.89961937509957934, 68.12609039468563310 ) ) ;
#101994=CARTESIAN_POINT ( 'NONE',  ( -19.03943276465977164, 0.05219959533909376836, 116.2489096053143669 ) ) ;
#101995=CARTESIAN_POINT ( 'NONE',  ( 14.34966873604960469, 8.224510206698951720, 84.16557627198103830 ) ) ;
#101997=CARTESIAN_POINT ( 'NONE',  ( -5.153800228976328057, -19.02544592524343514, 42.29057627198101699 ) ) ;
#101998=CARTESIAN_POINT ( 'NONE',  ( -10.72451020669898014, 18.67979575497178502, 50.41557627198103120 ) ) ;
#101999=CARTESIAN_POINT ( 'NONE',  ( -21.53943276465977519, 0.05219959533907696930, 76.24890960531435269 ) ) ;
#102000=CARTESIAN_POINT ( 'NONE',  ( 16.51473224551069308, 9.474510206698969483, 34.16557627198102409 ) ) ;
#102001=CARTESIAN_POINT ( 'NONE',  ( 4.483927247898790824, -16.52544592524335698, 60.20942372801902565 ) ) ;
#102002=CARTESIAN_POINT ( 'NONE',  ( -19.03943276465977164, 0.05219959533909376836, 66.24890960531436690 ) ) ;
#102003=CARTESIAN_POINT ( 'NONE',  ( 19.02544592524334988, 5.153800228976608722, 36.45942372801900433 ) ) ;
#102005=CARTESIAN_POINT ( 'NONE',  ( -21.53943276465977519, -0.05219959533937600094, 48.75109039468568284 ) ) ;
#102006=CARTESIAN_POINT ( 'NONE',  ( -8.314922557960811034, -14.29746914071050412, 107.0822429386476955 ) ) ;
#102007=CARTESIAN_POINT ( 'NONE',  ( -5.153800228976607833, 19.02544592524334988, 92.70942372801901854 ) ) ;
#102010=CARTESIAN_POINT ( 'NONE',  ( 15.80617190586746368, 15.72974639402197994, 44.37390960531435979 ) ) ;
#102011=CARTESIAN_POINT ( 'NONE',  ( 16.38665767535053064, -7.295008042176011287, 67.76400864214545550 ) ) ;
#102012=CARTESIAN_POINT ( 'NONE',  ( 5.719274019375673035, 21.55341960407619339, 87.29275706135236135 ) ) ;
#102013=CARTESIAN_POINT ( 'NONE',  ( -12.06949235617756955, 12.14591786802309770, 30.62390960531436335 ) ) ;
#102014=CARTESIAN_POINT ( 'NONE',  ( 14.29746914071037800, 8.314922557961029526, 56.66775706135235424 ) ) ;
#102015=CARTESIAN_POINT ( 'NONE',  ( -16.55341960407611168, -4.379528057220339221, 61.45724293864770260 ) ) ;
#102016=CARTESIAN_POINT ( 'NONE',  ( -5.823673210054116645, -21.52544592524344225, 82.29057627198103830 ) ) ;
#102017=CARTESIAN_POINT ( 'NONE',  ( 10.81492255796078972, 18.62759615963270932, 79.58224293864769550 ) ) ;
#102019=CARTESIAN_POINT ( 'NONE',  ( -9.564922557961040184, 16.46253265017147172, 82.91775706135233293 ) ) ;
#102020=CARTESIAN_POINT ( 'NONE',  ( -16.46253265017160317, 9.564922557960807481, 115.8322429386477097 ) ) ;
#102021=CARTESIAN_POINT ( 'NONE',  ( 16.51473224551069308, 9.474510206698969483, 64.16557627198102409 ) ) ;
#102022=CARTESIAN_POINT ( 'NONE',  ( 19.02544592524343514, -5.153800228976328945, 38.54057627198103120 ) ) ;
#102023=CARTESIAN_POINT ( 'NONE',  ( -17.60728821186568638, 5.500000000000037303, 75.86690927743003954 ) ) ;
#102024=ORIENTED_EDGE ( 'NONE', *, *, #107130, .F. ) ;
#102025=CARTESIAN_POINT ( 'NONE',  ( 12.06949235617739724, 12.14591786802326823, 81.87609039468568994 ) ) ;
#102026=B_SPLINE_CURVE_WITH_KNOTS ( 'NONE', 3,
 ( #166098, #90225, #138710, #42752, #89238, #181275, #31544, #149921, #150932, #105401, #11427, #134768, #104415, #197429, #61860, #183249, #182255, #73097, #29565, #151909 ),
 .UNSPECIFIED., .F., .F.,
 ( 4, 2, 2, 2, 2, 2, 2, 2, 2, 4 ),
 ( 0.004000878361811999878, 0.004499404418916020179, 0.004997930476020039613, 0.005496456533124059046, 0.005994982590228079347, 0.006244245618780067814, 0.006493508647332058015, 0.006992034704436035815, 0.007490560761540013615, 0.007989086818643992283 ),
 .UNSPECIFIED. ) ;
#102027=CARTESIAN_POINT ( 'NONE',  ( -15.72974639402197994, 15.80617190586746368, 105.6239096053143669 ) ) ;
#102028=CARTESIAN_POINT ( 'NONE',  ( -19.05341960407611168, -5.049401038298163336, 76.45724293864769550 ) ) ;
#102029=CARTESIAN_POINT ( 'NONE',  ( -21.53943276465977519, -0.05219959533937600094, 38.75109039468567573 ) ) ;
#102030=CARTESIAN_POINT ( 'NONE',  ( 5.153800228976335163, 19.02544592524342804, 94.79057627198103830 ) ) ;
#102033=CARTESIAN_POINT ( 'NONE',  ( -0.05219959533937732626, 21.53943276465977519, 27.50109039468567929 ) ) ;
#102035=CARTESIAN_POINT ( 'NONE',  ( -16.46253265017160317, 9.564922557960807481, 100.8322429386477097 ) ) ;
#102036=CARTESIAN_POINT ( 'NONE',  ( 5.049401038297881783, 19.05341960407617563, 57.29275706135231871 ) ) ;
#102037=CARTESIAN_POINT ( 'NONE',  ( 15.80617190586769283, -15.72974639402175789, 20.62609039468568639 ) ) ;
#102038=CARTESIAN_POINT ( 'NONE',  ( -13.97604488694547697, 13.89961937509957934, 43.12609039468566152 ) ) ;
#102039=CARTESIAN_POINT ( 'NONE',  ( 0.05219959533936267826, -19.03943276465977164, 45.00109039468566863 ) ) ;
#102040=CARTESIAN_POINT ( 'NONE',  ( 14.29746914071037800, 8.314922557961029526, 101.6677570613523613 ) ) ;
#102042=CARTESIAN_POINT ( 'NONE',  ( 9.564922557960805705, 16.46253265017160317, 69.58224293864770971 ) ) ;
#102044=CARTESIAN_POINT ( 'NONE',  ( -15.80617190586768217, 15.72974639402176855, 78.12609039468570415 ) ) ;
#102045=CARTESIAN_POINT ( 'NONE',  ( 0.05219959533937995610, -21.53943276465977519, 90.00109039468567573 ) ) ;
#102047=CARTESIAN_POINT ( 'NONE',  ( 13.97604488694527802, 13.89961937509977652, 94.37390960531436690 ) ) ;
#102048=CARTESIAN_POINT ( 'NONE',  ( 5.719274019375673035, 21.55341960407619339, 62.29275706135236845 ) ) ;
#102049=CARTESIAN_POINT ( 'NONE',  ( 8.314922557961029526, -14.29746914071037800, 20.41775706135234714 ) ) ;
#102050=CARTESIAN_POINT ( 'NONE',  ( 19.05341960407611168, 5.049401038298154454, 68.95724293864769550 ) ) ;
#102051=CARTESIAN_POINT ( 'NONE',  ( -15.80617190586745835, -15.72974639402198527, 21.87390960531436690 ) ) ;
#102052=CARTESIAN_POINT ( 'NONE',  ( -5.153800228976328057, -19.02544592524343514, 87.29057627198103830 ) ) ;
#102053=CARTESIAN_POINT ( 'NONE',  ( -5.153800228976607833, 19.02544592524335343, 87.70942372801897591 ) ) ;
#102054=CARTESIAN_POINT ( 'NONE',  ( -5.049401038298153566, 19.05341960407611168, 85.20724293864766707 ) ) ;
#102055=CARTESIAN_POINT ( 'NONE',  ( -5.153800228976328057, -19.02544592524343514, 57.29057627198103120 ) ) ;
#102056=CARTESIAN_POINT ( 'NONE',  ( 18.62759615963271287, -10.81492255796078972, 113.3322429386476955 ) ) ;
#102057=CARTESIAN_POINT ( 'NONE',  ( 16.52544592524335698, 4.483927247898782831, 106.4594237280190328 ) ) ;
#102058=CARTESIAN_POINT ( 'NONE',  ( -18.09867054820433907, -5.499999999999827693, 48.98393025253585620 ) ) ;
#102059=CARTESIAN_POINT ( 'NONE',  ( -16.46253265017146816, -9.564922557961047289, 64.16775706135233293 ) ) ;
#102060=CARTESIAN_POINT ( 'NONE',  ( 5.049401038298161559, -19.05341960407611168, 97.70724293864766707 ) ) ;
#102061=CARTESIAN_POINT ( 'NONE',  ( 14.34966873604960469, 8.224510206698951720, 69.16557627198102409 ) ) ;
#102062=CARTESIAN_POINT ( 'NONE',  ( 14.34966873604960469, 8.224510206698951720, 104.1655762719810241 ) ) ;
#102063=CARTESIAN_POINT ( 'NONE',  ( -21.52544592524343514, 5.823673210054127303, 31.04057627198102409 ) ) ;
#102064=CARTESIAN_POINT ( 'NONE',  ( -9.474510206698964154, 16.51473224551069663, 115.4155762719810241 ) ) ;
#102065=CARTESIAN_POINT ( 'NONE',  ( -16.52544592524342804, 4.483927247898546575, 96.04057627198102409 ) ) ;
#102067=CARTESIAN_POINT ( 'NONE',  ( -19.05341960407617563, 5.049401038297882671, 43.54275706135232582 ) ) ;
#102068=CARTESIAN_POINT ( 'NONE',  ( 16.55341960407618274, -4.379528057220086978, 101.0427570613523756 ) ) ;
#102069=CARTESIAN_POINT ( 'NONE',  ( -5.049401038298153566, 19.05341960407611168, 90.20724293864766707 ) ) ;
#102070=CARTESIAN_POINT ( 'NONE',  ( 21.52544592524334988, 5.823673210054432836, 56.45942372801902565 ) ) ;
#102071=CARTESIAN_POINT ( 'NONE',  ( 5.719274019375991003, -21.55341960407610458, 47.70724293864770260 ) ) ;
#102072=CARTESIAN_POINT ( 'NONE',  ( -0.05219959533937732626, 21.53943276465977519, 37.50109039468568284 ) ) ;
#102073=CARTESIAN_POINT ( 'NONE',  ( 0.05219959533907565091, 21.53943276465977519, 89.99890960531438111 ) ) ;
#102074=CARTESIAN_POINT ( 'NONE',  ( -0.05219959533910754901, -16.53943276465976808, 102.4989096053143811 ) ) ;
#102075=CARTESIAN_POINT ( 'NONE',  ( -9.564922557961040184, 16.46253265017147172, 72.91775706135233293 ) ) ;
#102076=CARTESIAN_POINT ( 'NONE',  ( 5.153800228976335163, 19.02544592524342804, 49.79057627198100988 ) ) ;
#102077=CARTESIAN_POINT ( 'NONE',  ( -19.03943276465977164, 0.05219959533909376836, 101.2489096053143669 ) ) ;
#102078=CARTESIAN_POINT ( 'NONE',  ( 0.05219959533909260263, 19.03943276465977164, 94.99890960531436690 ) ) ;
#102079=CARTESIAN_POINT ( 'NONE',  ( -16.53943276465976808, 0.05219959533911058130, 116.2489096053143669 ) ) ;
#102081=CARTESIAN_POINT ( 'NONE',  ( 16.52544592524342804, -4.483927247898539470, 38.54057627198103120 ) ) ;
#102082=CARTESIAN_POINT ( 'NONE',  ( 4.379528057220092307, 16.55341960407617563, 42.29275706135235424 ) ) ;
#102083=CARTESIAN_POINT ( 'NONE',  ( 5.719274019375673035, 21.55341960407619339, 107.2927570613523471 ) ) ;
#102085=CARTESIAN_POINT ( 'NONE',  ( 12.14591786802309770, 12.06949235617756955, 29.37390960531435269 ) ) ;
#102086=CARTESIAN_POINT ( 'NONE',  ( -15.80617190586768217, 15.72974639402176855, 28.12609039468568284 ) ) ;
#102087=CARTESIAN_POINT ( 'NONE',  ( 9.564922557960805705, 16.46253265017160317, 109.5822429386476955 ) ) ;
#102088=CARTESIAN_POINT ( 'NONE',  ( -12.06949235617739369, -12.14591786802326823, 104.3760903946856899 ) ) ;
#102089=CARTESIAN_POINT ( 'NONE',  ( -8.224510206698735004, -14.34966873604973081, 94.58442372801901854 ) ) ;
#102090=CARTESIAN_POINT ( 'NONE',  ( -14.34966873604972548, 8.224510206698743886, 23.33442372801901499 ) ) ;
#102091=CARTESIAN_POINT ( 'NONE',  ( 5.049401038298161559, -19.05341960407611168, 52.70724293864767418 ) ) ;
#102092=CARTESIAN_POINT ( 'NONE',  ( 8.224510206698953496, -14.34966873604960469, 107.9155762719810241 ) ) ;
#102093=CARTESIAN_POINT ( 'NONE',  ( 10.81492255796078972, 18.62759615963270932, 114.5822429386477097 ) ) ;
#102094=CARTESIAN_POINT ( 'NONE',  ( 9.474510206698971260, -16.51473224551069308, 37.91557627198102409 ) ) ;
#102095=CARTESIAN_POINT ( 'NONE',  ( 0.05219959533909260263, 19.03943276465977164, 109.9989096053143669 ) ) ;
#102096=CARTESIAN_POINT ( 'NONE',  ( -0.05219959533937732626, 21.53943276465977519, 32.50109039468568284 ) ) ;
#102098=CARTESIAN_POINT ( 'NONE',  ( 16.51473224551069308, 9.474510206698969483, 109.1655762719810383 ) ) ;
#102100=CARTESIAN_POINT ( 'NONE',  ( -9.564922557960796823, -16.46253265017161027, 97.08224293864769550 ) ) ;
#102101=CARTESIAN_POINT ( 'NONE',  ( 21.53943276465977519, 0.05219959533937863772, 46.25109039468567573 ) ) ;
#102102=CARTESIAN_POINT ( 'NONE',  ( -8.314922557960811034, -14.29746914071050412, 97.08224293864770971 ) ) ;
#102103=CARTESIAN_POINT ( 'NONE',  ( 0.05219959533909260263, 19.03943276465977164, 89.99890960531436690 ) ) ;
#102104=CARTESIAN_POINT ( 'NONE',  ( 18.22780087662122384, -5.500000000000022204, 71.01540105326107266 ) ) ;
#102105=CARTESIAN_POINT ( 'NONE',  ( -14.29746914071037622, -8.314922557961029526, 64.16775706135234714 ) ) ;
#102106=CARTESIAN_POINT ( 'NONE',  ( 10.81492255796106328, -18.62759615963255655, 75.41775706135233293 ) ) ;
#102107=CARTESIAN_POINT ( 'NONE',  ( 16.55341960407618274, -4.379528057220086978, 36.04275706135234714 ) ) ;
#102108=CARTESIAN_POINT ( 'NONE',  ( 13.89961937509977652, -13.97604488694527269, 78.12390960531433848 ) ) ;
#102109=CARTESIAN_POINT ( 'NONE',  ( 16.46253265017146816, 9.564922557961045513, 111.6677570613523329 ) ) ;
#102110=CARTESIAN_POINT ( 'NONE',  ( -16.53943276465976808, -0.05219959533934237506, 68.75109039468568994 ) ) ;
#102111=CARTESIAN_POINT ( 'NONE',  ( 18.62759615963255655, 10.81492255796105972, 111.6677570613523613 ) ) ;
#102112=CARTESIAN_POINT ( 'NONE',  ( -16.51473224551082808, 9.474510206698731452, 98.33442372801900433 ) ) ;
#102113=CARTESIAN_POINT ( 'NONE',  ( 5.049401038298161559, -19.05341960407611168, 62.70724293864769550 ) ) ;
#102114=CARTESIAN_POINT ( 'NONE',  ( 18.67979575497178502, 10.72451020669898547, 89.16557627198102409 ) ) ;
#102115=CARTESIAN_POINT ( 'NONE',  ( -16.53943276465976808, 0.05219959533911058130, 91.24890960531436690 ) ) ;
#102116=CARTESIAN_POINT ( 'NONE',  ( -13.89961937509957401, -13.97604488694547875, 94.37609039468566152 ) ) ;
#102117=CARTESIAN_POINT ( 'NONE',  ( -8.314922557961024197, 14.29746914071037800, 52.91775706135235424 ) ) ;
#102118=CARTESIAN_POINT ( 'NONE',  ( 16.81555441253556182, -7.025013491695411005, 63.13685445334259327 ) ) ;
#102119=CARTESIAN_POINT ( 'NONE',  ( -13.97604488694547697, 13.89961937509957934, 53.12609039468565442 ) ) ;
#102121=CARTESIAN_POINT ( 'NONE',  ( 14.34966873604960469, 8.224510206698951720, 34.16557627198102409 ) ) ;
#102122=CARTESIAN_POINT ( 'NONE',  ( -14.34966873604960291, -8.224510206698953496, 86.66557627198102409 ) ) ;
#102123=CARTESIAN_POINT ( 'NONE',  ( -16.51473224551082808, 9.474510206698731452, 23.33442372801900078 ) ) ;
#102124=CARTESIAN_POINT ( 'NONE',  ( -19.48894818550245134, 5.499999999999918288, 90.10307310435231898 ) ) ;
#102125=CARTESIAN_POINT ( 'NONE',  ( 0.05219959533937995610, -21.53943276465977519, 25.00109039468567218 ) ) ;
#102126=CARTESIAN_POINT ( 'NONE',  ( 0.05219959533909260263, 19.03943276465977164, 99.99890960531436690 ) ) ;
#102127=CARTESIAN_POINT ( 'NONE',  ( -16.46253265017160317, 9.564922557960807481, 80.83224293864769550 ) ) ;
#102128=CARTESIAN_POINT ( 'NONE',  ( 21.55341960407619695, -5.719274019375665929, 101.0427570613523756 ) ) ;
#102129=CARTESIAN_POINT ( 'NONE',  ( 16.51473224551069308, 9.474510206698969483, 79.16557627198103830 ) ) ;
#102130=CARTESIAN_POINT ( 'NONE',  ( -21.55341960407610458, -5.719274019375992779, 41.45724293864769550 ) ) ;
#102131=CARTESIAN_POINT ( 'NONE',  ( 0.05219959533910956823, 16.53943276465976808, 74.99890960531435269 ) ) ;
#102132=CARTESIAN_POINT ( 'NONE',  ( 19.03943276465977164, -0.05219959533909143690, 58.74890960531435979 ) ) ;
#102133=CARTESIAN_POINT ( 'NONE',  ( -16.55341960407611168, -4.379528057220339221, 101.4572429386476955 ) ) ;
#102134=CARTESIAN_POINT ( 'NONE',  ( -21.55341960407619339, 5.719274019375674811, 23.54275706135235424 ) ) ;
#102135=CARTESIAN_POINT ( 'NONE',  ( 5.823673210054444382, -21.52544592524334988, 60.20942372801902565 ) ) ;
#102136=CARTESIAN_POINT ( 'NONE',  ( 16.46253265017160672, -9.564922557960803928, 48.33224293864769550 ) ) ;
#102137=CARTESIAN_POINT ( 'NONE',  ( 4.379528057220092307, 16.55341960407617563, 62.29275706135236845 ) ) ;
#102138=CARTESIAN_POINT ( 'NONE',  ( 18.62759615963271287, -10.81492255796078972, 108.3322429386477097 ) ) ;
#102139=CARTESIAN_POINT ( 'NONE',  ( 21.53943276465977519, -0.05219959533907433946, 113.7489096053143527 ) ) ;
#102140=CARTESIAN_POINT ( 'NONE',  ( -13.89961937509957401, -13.97604488694547875, 44.37609039468566863 ) ) ;
#102141=CARTESIAN_POINT ( 'NONE',  ( 5.153800228976335163, 19.02544592524342804, 59.79057627198100988 ) ) ;
#102143=CARTESIAN_POINT ( 'NONE',  ( -5.719274019375665041, -21.55341960407619695, 69.79275706135234714 ) ) ;
#102144=CARTESIAN_POINT ( 'NONE',  ( 18.67979575497178502, 10.72451020669898547, 59.16557627198103120 ) ) ;
#102145=CARTESIAN_POINT ( 'NONE',  ( 8.314922557960818139, 14.29746914071049879, 34.58224293864770260 ) ) ;
#102146=CARTESIAN_POINT ( 'NONE',  ( 15.72974639402176855, 15.80617190586768217, 71.87609039468568994 ) ) ;
#102147=CARTESIAN_POINT ( 'NONE',  ( -10.81492255796105439, 18.62759615963255655, 112.9177570613523329 ) ) ;
#102148=CARTESIAN_POINT ( 'NONE',  ( 16.53943276465976808, -0.05219959533910856209, 58.74890960531436690 ) ) ;
#102149=CARTESIAN_POINT ( 'NONE',  ( 16.52544592524342804, -4.483927247898539470, 98.54057627198105251 ) ) ;
#102150=CARTESIAN_POINT ( 'NONE',  ( -13.89961937509957401, -13.97604488694547875, 49.37609039468567573 ) ) ;
#102151=CARTESIAN_POINT ( 'NONE',  ( 16.55341960407618274, -4.379528057220086978, 111.0427570613523613 ) ) ;
#102152=CARTESIAN_POINT ( 'NONE',  ( -15.72974639402176322, -15.80617190586768395, 74.37609039468568994 ) ) ;
#102153=CARTESIAN_POINT ( 'NONE',  ( 19.02544592524343514, -5.153800228976328945, 58.54057627198102409 ) ) ;
#102154=CARTESIAN_POINT ( 'NONE',  ( -13.89961937509957401, -13.97604488694547875, 29.37609039468565797 ) ) ;
#102155=CARTESIAN_POINT ( 'NONE',  ( -10.72451020669898014, 18.67979575497178502, 35.41557627198102409 ) ) ;
#102156=CARTESIAN_POINT ( 'NONE',  ( 18.62759615963255655, 10.81492255796105972, 36.66775706135234714 ) ) ;
#102157=CARTESIAN_POINT ( 'NONE',  ( -21.55341960407610458, -5.719274019375992779, 91.45724293864769550 ) ) ;
#102158=CARTESIAN_POINT ( 'NONE',  ( 19.02544592524334988, 5.153800228976608722, 81.45942372801897591 ) ) ;
#102159=CARTESIAN_POINT ( 'NONE',  ( 8.224510206698742110, 14.34966873604972548, 47.08442372801901854 ) ) ;
#102161=CARTESIAN_POINT ( 'NONE',  ( -5.719274019375978568, 21.55341960407610458, 90.20724293864770971 ) ) ;
#102162=CARTESIAN_POINT ( 'NONE',  ( -16.53943276465976808, 0.05219959533911058130, 86.24890960531436690 ) ) ;
#102164=CARTESIAN_POINT ( 'NONE',  ( -4.483927247898782831, 16.52544592524335698, 22.70942372801901499 ) ) ;
#102165=CARTESIAN_POINT ( 'NONE',  ( 21.52544592524344225, -5.823673210054117533, 53.54057627198103120 ) ) ;
#102166=CARTESIAN_POINT ( 'NONE',  ( -14.29746914071037622, -8.314922557961029526, 89.16775706135236135 ) ) ;
#102167=CARTESIAN_POINT ( 'NONE',  ( 17.50000000000000000, -5.499999999999992895, 56.21769037696436300 ) ) ;
#102168=CARTESIAN_POINT ( 'NONE',  ( -8.224510206698735004, -14.34966873604973081, 59.58442372801901854 ) ) ;
#102169=CARTESIAN_POINT ( 'NONE',  ( 18.62759615963255655, 10.81492255796105972, 31.66775706135234358 ) ) ;
#102170=CARTESIAN_POINT ( 'NONE',  ( -10.72451020669898014, 18.67979575497178502, 50.41557627198103120 ) ) ;
#102171=CARTESIAN_POINT ( 'NONE',  ( 12.06949235617739724, 12.14591786802326823, 81.87609039468568994 ) ) ;
#102172=CARTESIAN_POINT ( 'NONE',  ( 9.474510206698971260, -16.51473224551069308, 97.91557627198102409 ) ) ;
#102173=CARTESIAN_POINT ( 'NONE',  ( -0.05219959533937732626, 21.53943276465977519, 52.50109039468567573 ) ) ;
#102174=CARTESIAN_POINT ( 'NONE',  ( -13.89961937509977652, 13.97604488694528158, 30.62390960531435269 ) ) ;
#102175=CARTESIAN_POINT ( 'NONE',  ( 10.72451020669898902, -18.67979575497178502, 37.91557627198102409 ) ) ;
#102176=CARTESIAN_POINT ( 'NONE',  ( -0.05219959533909027116, -19.03943276465977164, 112.4989096053143669 ) ) ;
#102178=CARTESIAN_POINT ( 'NONE',  ( -9.564922557961040184, 16.46253265017147172, 42.91775706135234003 ) ) ;
#102179=CARTESIAN_POINT ( 'NONE',  ( -16.53943276465976808, -0.05219959533934237506, 63.75109039468568284 ) ) ;
#102180=CARTESIAN_POINT ( 'NONE',  ( -13.89961937509977652, 13.97604488694528158, 115.6239096053143669 ) ) ;
#102182=CARTESIAN_POINT ( 'NONE',  ( 16.46253265017160672, -9.564922557960803928, 88.33224293864769550 ) ) ;
#102183=CARTESIAN_POINT ( 'NONE',  ( 12.14591786802327356, -12.06949235617739191, 95.62609039468568994 ) ) ;
#102185=CARTESIAN_POINT ( 'NONE',  ( -4.379528057220328563, 16.55341960407611168, 100.2072429386476955 ) ) ;
#102186=CARTESIAN_POINT ( 'NONE',  ( -15.80617190586745835, -15.72974639402198527, 46.87390960531435979 ) ) ;
#102187=CARTESIAN_POINT ( 'NONE',  ( 19.05341960407611168, 5.049401038298154454, 28.95724293864769550 ) ) ;
#102188=CARTESIAN_POINT ( 'NONE',  ( -16.53943276465976808, -0.05219959533934237506, 78.75109039468568994 ) ) ;
#102189=CARTESIAN_POINT ( 'NONE',  ( 15.80617190586769283, -15.72974639402175789, 30.62609039468567929 ) ) ;
#102190=CARTESIAN_POINT ( 'NONE',  ( 16.46253265017146816, 9.564922557961045513, 96.66775706135233293 ) ) ;
#102191=CARTESIAN_POINT ( 'NONE',  ( -8.314922557960811034, -14.29746914071050412, 87.08224293864769550 ) ) ;
#102192=CARTESIAN_POINT ( 'NONE',  ( -19.05341960407611168, -5.049401038298163336, 36.45724293864766707 ) ) ;
#102193=AXIS2_PLACEMENT_3D ( 'NONE', #15082, #121258, #124237 ) ;
#102194=CARTESIAN_POINT ( 'NONE',  ( 13.89961937509977652, -13.97604488694527269, 108.1239096053143669 ) ) ;
#102195=CARTESIAN_POINT ( 'NONE',  ( 5.719274019375673035, 21.55341960407619339, 102.2927570613523613 ) ) ;
#102196=CARTESIAN_POINT ( 'NONE',  ( 13.89961937509977652, -13.97604488694527269, 73.12390960531436690 ) ) ;
#102197=CARTESIAN_POINT ( 'NONE',  ( 0.05219959533934541429, -16.53943276465976808, 60.00109039468568284 ) ) ;
#102198=CARTESIAN_POINT ( 'NONE',  ( 21.52544592524334988, 5.823673210054432836, 96.45942372801901854 ) ) ;
#102199=CARTESIAN_POINT ( 'NONE',  ( 0.05219959533934541429, -16.53943276465976808, 75.00109039468568994 ) ) ;
#102200=CARTESIAN_POINT ( 'NONE',  ( -5.153800228976607833, 19.02544592524334988, 52.70942372801900433 ) ) ;
#102201=CARTESIAN_POINT ( 'NONE',  ( 9.474510206698729675, 16.51473224551082808, 62.08442372801899722 ) ) ;
#102202=ORIENTED_EDGE ( 'NONE', *, *, #70410, .T. ) ;
#102203=CARTESIAN_POINT ( 'NONE',  ( 21.55341960407619695, -5.719274019375665929, 66.04275706135236135 ) ) ;
#102204=CARTESIAN_POINT ( 'NONE',  ( -16.46253265017160317, 9.564922557960807481, 65.83224293864769550 ) ) ;
#102205=CARTESIAN_POINT ( 'NONE',  ( -17.59860650958989936, -7.585241751807033417, 56.57662985737508166 ) ) ;
#102206=CARTESIAN_POINT ( 'NONE',  ( 16.46253265017146816, 9.564922557961045513, 61.66775706135234003 ) ) ;
#102208=CARTESIAN_POINT ( 'NONE',  ( -9.474510206698964154, 16.51473224551069663, 80.41557627198103830 ) ) ;
#102209=CARTESIAN_POINT ( 'NONE',  ( 16.53943276465976808, -0.05219959533910856209, 38.74890960531435979 ) ) ;
#102210=CARTESIAN_POINT ( 'NONE',  ( -10.81492255796078084, -18.62759615963271287, 42.08224293864769550 ) ) ;
#102212=CARTESIAN_POINT ( 'NONE',  ( -16.46253265017146816, -9.564922557961047289, 19.16775706135233293 ) ) ;
#102214=CARTESIAN_POINT ( 'NONE',  ( -16.51473224551069308, -9.474510206698971260, 41.66557627198103120 ) ) ;
#102216=CARTESIAN_POINT ( 'NONE',  ( -17.97161686093727795, 5.499999999999980460, 80.99637206859165417 ) ) ;
#102217=CARTESIAN_POINT ( 'NONE',  ( 18.67979575497194134, -10.72451020669871369, 70.83442372801901854 ) ) ;
#102219=CARTESIAN_POINT ( 'NONE',  ( 16.52544592524335698, 4.483927247898782831, 61.45942372801901854 ) ) ;
#102220=CARTESIAN_POINT ( 'NONE',  ( -5.823673210054116645, -21.52544592524344225, 87.29057627198103830 ) ) ;
#102221=CARTESIAN_POINT ( 'NONE',  ( 0.05219959533910956823, 16.53943276465976808, 54.99890960531435269 ) ) ;
#102222=CARTESIAN_POINT ( 'NONE',  ( 16.51473224551069308, 9.474510206698969483, 24.16557627198102765 ) ) ;
#102223=CARTESIAN_POINT ( 'NONE',  ( 13.89961937509977652, -13.97604488694527269, 103.1239096053143527 ) ) ;
#102224=CARTESIAN_POINT ( 'NONE',  ( -21.53943276465977519, -0.05219959533937600094, 43.75109039468568284 ) ) ;
#102225=CARTESIAN_POINT ( 'NONE',  ( -19.03943276465977164, -0.05219959533935918106, 43.75109039468566863 ) ) ;
#102226=CARTESIAN_POINT ( 'NONE',  ( -5.153800228976328057, -19.02544592524343514, 32.29057627198102409 ) ) ;
#102227=CARTESIAN_POINT ( 'NONE',  ( -21.53943276465977519, -0.05219959533937600094, 83.75109039468568994 ) ) ;
#102229=CARTESIAN_POINT ( 'NONE',  ( 14.29746914071049879, -8.314922557960816363, 28.33224293864769550 ) ) ;
#102231=CARTESIAN_POINT ( 'NONE',  ( 15.72974639402199770, -15.80617190586745480, 38.12390960531436690 ) ) ;
#102234=CARTESIAN_POINT ( 'NONE',  ( 16.51473224551069308, 9.474510206698969483, 89.16557627198103830 ) ) ;
#102235=CARTESIAN_POINT ( 'NONE',  ( -12.06949235617756955, 12.14591786802309770, 85.62390960531436690 ) ) ;
#102236=CARTESIAN_POINT ( 'NONE',  ( 9.474510206698729675, 16.51473224551082808, 102.0844237280190043 ) ) ;
#102237=CARTESIAN_POINT ( 'NONE',  ( -21.55341960407610458, -5.719274019375992779, 66.45724293864768129 ) ) ;
#102239=CARTESIAN_POINT ( 'NONE',  ( -16.51473224551069308, -9.474510206698971260, 36.66557627198102409 ) ) ;
#102240=CARTESIAN_POINT ( 'NONE',  ( -13.97604488694527625, -13.89961937509977652, 86.87390960531436690 ) ) ;
#102241=CARTESIAN_POINT ( 'NONE',  ( -10.81492255796078084, -18.62759615963271287, 92.08224293864769550 ) ) ;
#102242=CARTESIAN_POINT ( 'NONE',  ( -4.379528057220086978, -16.55341960407618274, 109.7927570613523613 ) ) ;
#102243=CARTESIAN_POINT ( 'NONE',  ( -5.049401038298153566, 19.05341960407611168, 105.2072429386476671 ) ) ;
#102244=CARTESIAN_POINT ( 'NONE',  ( 0.05219959533936267826, -19.03943276465977164, 80.00109039468567573 ) ) ;
#102245=CARTESIAN_POINT ( 'NONE',  ( 21.53943276465977519, 0.05219959533937863772, 96.25109039468568994 ) ) ;
#102246=CARTESIAN_POINT ( 'NONE',  ( 0.05219959533907565091, 21.53943276465977519, 74.99890960531435269 ) ) ;
#102247=CARTESIAN_POINT ( 'NONE',  ( -18.62759615963270932, 10.81492255796079327, 40.83224293864769550 ) ) ;
#102248=CARTESIAN_POINT ( 'NONE',  ( -13.89961937509977652, 13.97604488694528158, 45.62390960531433848 ) ) ;
#102249=CARTESIAN_POINT ( 'NONE',  ( 4.379528057220092307, 16.55341960407617563, 112.2927570613523471 ) ) ;
#102250=CARTESIAN_POINT ( 'NONE',  ( 13.89961937509977652, -13.97604488694527269, 63.12390960531435979 ) ) ;
#102253=CARTESIAN_POINT ( 'NONE',  ( 13.89961937509957401, 13.97604488694547697, 31.87609039468566863 ) ) ;
#102254=CARTESIAN_POINT ( 'NONE',  ( -4.379528057220328563, 16.55341960407611168, 85.20724293864770971 ) ) ;
#102255=( BOUNDED_SURFACE ( )  B_SPLINE_SURFACE ( 3, 2, ( 
 ( #42518, #104181, #165863, #197199, #120328, #182023, #130141, #40147, #193855, #160505, #68486, #179695, #21995, #191838, #55320, #149337, #83648, #56323, #53319, #116991, #26009, #42172, #39156, #70496, #6808, #176692, #192848, #54328, #25010, #114997, #147340, #180696, #177688, #132164, #164516, #195865, #161506, #8827, #41167, #72503, #145325, #38166, #178685, #100812, #115999, #101824, #10833, #163512, #99821, #148338, #69494, #22996, #86654, #133159, #85653, #9834, #71493, #87652, #84644, #146321, #119013, #194851, #102830, #118006, #134177, #57337, #7810, #131159, #162496, #23996, #199939, #61403, #170587, #32077, #92732, #197946, #91726, #138256, #60410, #123074, #184760, #107899, #44267, #46245, #198943, #74604, #93734, #75581, #166625, #47250, #14920, #181790, #169586, #137260, #43270, #155415, #185762, #77572, #104939, #63400, #122083, #31084, #62391, #140231, #16905, #154420, #78556, #28127, #719, #1724, #136271, #15914, #139244, #90744, #124061, #151452, #108907, #13915, #89767, #12939, #59416, #183774, #121090, #182784, #105925, #167610, #29106, #152427, #45260, #106914, #168587, #30085, #153422, #76580, #6689, #66380, #5695, #36035, #67371, #113862, #19880, #81521, #21878, #175558, #94726, #4688, #158391, #125077, #33071, #144210, #186774, #156404, #143207, #37034, #48245, #20870, #17908, #128041, #190731, #109899, #3705, #35048, #171583, #141231, #157408, #18901, #189742, #79564, #111890, #145206, #142221, #96702, #129030, #160389, #126068, #173579, #52204, #98695, #2722, #64399, #51215, #65383, #80547, #112876, #83528, #174569, #187764, #97684, #34063, #49234, #159374, #82528, #50235, #110892, #172577, #95722, #127043, #188750, #26891, #56206, #87540, #148224, #25895, #86540, #117889, #42054, #180580, #88534, #179579, #161386, #9718, #116875, #38046, #101705, #149227, #71382, #130018, #84524, #102714, #39041, #133046, #178566, #146201, #118895, #57222, #163395, #24892, #165398, #103718, #99702, #194736, #41050, #68367, #176572, #10718, #191717, #22877, #164403, #150231, #53201, #72381, #7687, #134056, #195748, #114878, #147221, #40031, #69371, #131041, #100698, #162379, #192731, #54213, #55206, #115884, #85533, #177574, #23881, #8712, #70381, #132049, #193738, #126557, #137759, #92241, #32578, #154919, #108415, #124579, #3222, #155912, #184275, #2226, #123569, #45758, #62899, #187276, #139732, #63908, #140737, #18413, #138749, #107410, #173084, #125578, #33568, #94231, #172081, #17407, #48746, #188257, #49731, #34563, #110399, #169083, #79064, #186275, #30589, #47754, #95230, #156916, #76083, #153927, #80062, #185264, #141732, #109408, #15421, #64896, #111399, #96219, #14419, #199443, #170090, #60911, #122587, #77080, #231, #61899, #46756, #31584, #93234, #16417, #78064, #1221, #171087, #66878, #68879, #127555, #145714, #190236, #176073, #85032, #69884, #51713, #114369, #19398, #189256, #157908, #131553, #39540, #21378, #50732, #177082, #112391, #38553, #116383, #81047, #99205, #100210, #130539, #161890, #174082, #37541, #191231, #142723, #65881, #23386, #4203, #35551, #52705, #146713, #97198, #53717, #158884, #160893, #8209, #20374, #36532, #67878, #82022, #143717, #113376, #175066, #22385, #5196, #144712, #178073, #98187, #129531, #193238, #54711, #128540, #6198, #159890, #83037, #84035, #7195, #192237, #115394, #195243, #11226, #90033, #42553, #70890, #89040, #10222, #132558, #149725, #73892, #26398, #150730, #27395, #105207, #25407, #194246, #59686, #12230, #120365, #181078, #58695, #119395, #135562, #74871, #13208, #121357, #197234, #55713, #104216, #72900, #117385, #134569, #182058, #165897, #162889, #179084, #43541, #71882, #166894, #196256, #40553, #151715, #28394, #136533, #101199, #183050, #56727, #198214, #24398, #86047, #147736, #9223, #102222, #163911, #87049, #148734, #133552, #118397, #180091, #41559, #103222, #164904, #88037, #57725, #62658, #171845, #156679 ),
 ( #126325, #186033, #125344, #155675, #187042, #33333, #139500, #983, #141500, #94993, #138512, #154683, #18173, #47515, #14178, #32341, #153686, #75848, #92997, #17170, #169852, #93994, #170850, #48512, #168845, #137524, #2984, #78824, #63670, #124337, #1991, #109171, #140502, #79830, #64663, #44534, #110166, #199206, #106189, #16178, #60673, #77833, #167873, #29372, #91003, #122348, #152689, #15182, #184037, #45520, #107174, #30350, #91992, #76841, #101728, #61663, #123332, #185025, #46512, #108171, #31346, #98958, #176838, #188022, #6951, #84788, #80809, #67635, #52466, #96966, #160648, #157672, #175826, #20138, #5957, #115145, #99964, #81783, #144473, #49494, #19161, #111156, #161648, #69642, #51476, #142488, #68631, #3966, #130287, #146467, #172845, #129294, #191981, #22140, #53468, #38309, #82791, #190990, #7959, #23144, #65646, #114124, #21136, #34326, #95987, #127308, #189019, #50493, #37299, #112157, #173846, #83790, #35312, #145470, #158646, #143470, #66639, #97948, #4954, #128302, #190002, #113138, #174828, #36292, #159640, #151481, #148491, #41315, #135325, #166656, #132316, #118154, #150493, #43301, #54475, #8982, #149482, #71642, #196997, #11990, #181822, #26155, #12972, #101980, #56476, #147491, #133309, #120131, #24154, #70650, #196011, #40304, #162648, #73653, #86805, #131308, #116145, #85805, #178836, #104969, #164660, #163660, #177836, #10978, #194998, #194008, #72651, #134326, #28157, #89799, #42315, #55471, #102975, #87797, #9982, #57486, #119156, #180838, #117141, #103976, #179844, #25163, #192998, #165655, #39304, #58464, #27153, #100963, #88800, #168615, #136302, #63432, #153450, #1754, #198971, #30115, #91756, #108937, #125108, #14948, #76608, #61432, #59447, #751, #138286, #29137, #45290, #199967, #123104, #184789, #15944, #60438, #186806, #48276, #62422, #109931, #92762, #156439, #154451, #46275, #77603, #107931, #170618, #169617, #124094, #167641, #139274, #171613, #31114, #33101, #106942, #94757, #74636, #197977, #13944, #185793, #47281, #121120, #182814, #90774, #152458, #44297, #32107, #93764, #105956, #155445, #16935, #78589, #75610, #140262, #137289, #122113, #183802, #34093, #53230, #68395, #172606, #159404, #65412, #130047, #143236, #98723, #3735, #21906, #187793, #190758, #79592, #95751, #52233, #188781, #20899, #66408, #157436, #191747, #83556, #113890, #17938, #99730, #111921, #82557, #160417, #176600, #114906, #129057, #6717, #141261, #37064, #38074, #110920, #97713, #144239, #127073, #175588, #49262, #5723, #50264, #36065, #145236, #2751, #173608, #174599, #64427, #18931, #126096, #80576, #142250, #81550, #35078, #96731, #158420, #19908, #4719, #128070, #67402, #189773, #51245, #112905, #150262, #56237, #117918, #58238, #11756, #131069, #41079, #194763, #161414, #69402, #180610, #22906, #192758, #179607, #73423, #84552, #57251, #54241, #102743, #26921, #43069, #40060, #71409, #7717, #177602, #193767, #55235, #25925, #115912, #148252, #181592, #178597, #133073, #165427, #196770, #162408, #9745, #42083, #135094, #146230, #39070, #164431, #101737, #116904, #87568, #119906, #149255, #100727, #10747, #70411, #23910, #72411, #134088, #86568, #195778, #118925, #88564, #85564, #147250, #8741, #103748, #132078, #163425, #24923, #122868, #154215, #78345, #16695, #124865, #92526, #197746, #184556, #153207, #74406, #138049, #123848, #46037, #28907, #60207, #198742, #139033, #31867, #45055, #121877, #91520, #89565, #30879, #183570, #59213, #75380, #106713, #168387, #14712, #107692, #90547, #93521, #140019, #15705, #155206, #169371, #186564, #77365, #29882, #512, #76372, #62184, #199730, #185546, #120882, #47040, #1508, #61196, #63185, #137052, #104736, #166427, #27922, #44064, #108697, #170376, #151251, #12740, #182581, #105724, #136072, #167411, #152229, #13714, #112666, #173367, #34837, #94512, #190519, #5480, #109693, #49023, #64189, #83317, #98480, #2509 ),
 ( #36814, #189533, #17694, #35828, #157194, #79351, #96492, #20655, #158182, #97474, #174358, #51993, #172358, #141022, #6475, #159160, #67163, #127827, #128820, #66165, #82309, #21663, #160173, #68155, #143999, #125856, #51005, #19672, #187556, #81314, #113652, #175346, #171375, #110678, #144994, #18688, #129807, #142997, #33848, #48037, #32862, #156194, #95508, #80335, #142007, #3496, #65172, #126831, #188537, #50015, #111680, #4475, #195532, #115675, #84314, #150009, #179369, #10505, #71171, #149017, #9505, #40831, #165184, #103508, #11515, #102504, #145993, #132835, #39821, #161170, #24680, #72167, #194522, #52982, #7476, #25686, #162171, #55994, #101487, #69160, #41840, #57006, #87331, #191506, #73185, #85317, #117672, #133842, #114661, #26679, #164188, #180371, #176357, #118679, #88319, #130827, #37830, #99490, #100492, #22667, #192518, #54001, #23669, #177363, #38834, #147009, #8494, #148016, #70171, #131839, #193522, #54997, #116666, #178357, #163176, #86329, #166182, #153969, #93276, #16457, #76126, #15466, #45800, #77123, #123610, #29642, #91274, #31626, #185305, #104501, #14464, #168145, #134856, #42836, #138792, #196534, #27683, #152965, #46796, #58004, #30632, #89324, #137804, #273, #119674, #13477, #44811, #181357, #151016, #167171, #28670, #199488, #12507, #121635, #154961, #151991, #106466, #61942, #170132, #135841, #183330, #108455, #74171, #197510, #58978, #60955, #75142, #90305, #122629, #120645, #184319, #182343, #107452, #43821, #105485, #169127, #92285, #59968, #136813, #198497, #1263, #157946, #18451, #109447, #96260, #19437, #69676, #131343, #189295, #94273, #188297, #34601, #156954, #81085, #142763, #4243, #140777, #65923, #95271, #171130, #193031, #172122, #62940, #143758, #111439, #78106, #127596, #33608, #139775, #54508, #80102, #5239, #2266, #141770, #3263, #112432, #116180, #64936, #126595, #49774, #124620, #50772, #173126, #32619, #48787, #174121, #35592, #97238, #158926, #63949, #177871, #39339, #20415, #100998, #82065, #162683, #186315, #47797, #155951, #17448, #79104, #125618, #187316, #110441, #42349, #151515, #180873, #13006, #56511, #59481, #136337, #74670, #163696, #57520, #165689, #121155, #9017, #178872, #117177, #182848, #104011, #73689, #132351, #88834, #149516, #11013, #70685, #166689, #181856, #85839, #25198, #40339, #44331, #198011, #102014, #27187, #71676, #105988, #72686, #105003, #10017, #28192, #194043, #197032, #89834, #43335, #24189, #119189, #147529, #195034, #134361, #86841, #164695, #55507, #148526, #133343, #150527, #118189, #179880, #41348, #103011, #26190, #87830, #196045, #12026, #135361, #58499, #120165, #171642, #2782, #168647, #154482, #186839, #79624, #90807, #45323, #185827, #107963, #61465, #77635, #156469, #108969, #137322, #155475, #76639, #199003, #15976, #140296, #92794, #16967, #93795, #33132, #91789, #60469, #126128, #78620, #48308, #47314, #125140, #170650, #1787, #141292, #64460, #187823, #63465, #122145, #32138, #139304, #183834, #783, #109963, #94789, #29171, #106973, #17970, #138317, #49292, #62454, #30146, #167674, #152490, #13977, #75644, #153483, #123136, #14979, #199999, #184822, #46307, #169650, #31146, #124128, #130080, #7747, #3764, #190788, #175619, #19939, #21936, #80607, #98753, #143265, #129088, #38106, #22937, #4749, #67431, #172635, #142284, #110950, #84583, #192789, #174629, #65441, #191778, #127102, #53261, #69433, #34123, #52262, #114938, #83587, #176631, #99761, #5755, #113920, #131101, #161446, #188810, #37094, #144268, #95782, #18961, #146263, #157468, #50294, #160446, #111951, #173640, #6748, #35109, #145267, #96761, #158450, #189803, #20929, #81580, #66438, #128099, #51275, #68427, #112936, #97746, #36094, #159433, #82587, #23940, #42115, #163455, #85594, #102773, #26953, #179639, #103777, #180640, #58267, #178627, #147281, #12772, #165456, #73452, #134119, #11788, #72443, #88595, #27954, #166457 ),
 ( #57280, #164460, #70440, #104769, #119936, #150292, #54271, #136103, #148283, #118954, #135125, #74436, #89595, #196799, #43101, #115944, #181621, #151282, #8771, #195808, #177634, #24953, #39101, #132106, #100757, #86600, #162439, #193798, #55265, #9777, #10777, #116934, #40090, #101768, #71439, #133104, #117949, #194793, #56266, #41109, #25954, #87597, #149283, #139068, #78379, #108733, #140055, #186600, #92560, #154248, #94550, #48072, #167442, #77398, #30912, #197779, #105756, #16731, #59245, #28939, #15739, #109728, #120914, #93555, #90580, #546, #63221, #79390, #76406, #107725, #44098, #13746, #29915, #91555, #62217, #152261, #184590, #17732, #14745, #169406, #1545, #32898, #198774, #46071, #124901, #171412, #182613, #75414, #123885, #138082, #153242, #185583, #156231, #47073, #155241, #137086, #60240, #121911, #183604, #45088, #106745, #170410, #168420, #199763, #122901, #61230, #31902, #145031, #110717, #113687, #6513, #160211, #191543, #35865, #161209, #111717, #66203, #157233, #81350, #129844, #33889, #80372, #5518, #50055, #172399, #83355, #96528, #22704, #125893, #95545, #188575, #53020, #174395, #173403, #64228, #20692, #143034, #18725, #159197, #82347, #114701, #176394, #52029, #142045, #51041, #97511, #19708, #144036, #67198, #128856, #3532, #190556, #158218, #65209, #37868, #34874, #187593, #68192, #175382, #141060, #36851, #4512, #2546, #99527, #127865, #49062, #126868, #189569, #112703, #98518, #21701, #24715, #101522, #71206, #69197, #10539, #163213, #38872, #55032, #39856, #86364, #132869, #25720, #70208, #11551, #196564, #72203, #73217, #102540, #166213, #164223, #148049, #87366, #194558, #180404, #56028, #133877, #177400, #149051, #134888, #40866, #58035, #116702, #119705, #181388, #42867, #23705, #117706, #195568, #104532, #130865, #100528, #162207, #84351, #57041, #118715, #192555, #41876, #9539, #179402, #54038, #26713, #85353, #103543, #165218, #193560, #88352, #115712, #150045, #178392, #146029, #7512, #147046, #8530, #131875, #89357, #59010, #27714, #139807, #109481, #91307, #197542, #46828, #120677, #108488, #186349, #151047, #169162, #170167, #138827, #31660, #16490, #122663, #184351, #124653, #78139, #182376, #107484, #60989, #12537, #135871, #93310, #74202, #43854, #45833, #1295, #105519, #123641, #167204, #30666, #154994, #28702, #106502, #137840, #90338, #152023, #60002, #121669, #92319, #13509, #14498, #47829, #44846, #199521, #62973, #75174, #136846, #76160, #198531, #183364, #168179, #29675, #154004, #152999, #15500, #77157, #307, #61975, #185338, #158956, #80131, #140808, #19468, #143789, #96289, #20446, #97268, #175137, #95300, #63980, #129603, #82097, #190308, #50802, #128615, #189325, #5272, #144788, #83111, #191299, #66953, #125650, #112460, #81113, #2298, #4273, #51784, #174152, #32651, #187347, #113444, #141801, #35623, #142793, #48817, #21450, #36604, #98261, #171164, #52775, #64966, #159963, #6271, #94305, #67949, #155983, #17480, #79137, #110470, #172152, #157976, #33638, #156984, #18482, #3294, #126625, #188326, #49805, #111470, #173155, #34630, #65954, #127625, #39615, #195320, #100284, #118473, #84106, #87123, #180163, #133628, #164977, #9297, #134643, #85105, #101274, #130614, #54786, #103298, #7267, #53790, #179157, #23458, #145785, #56800, #69962, #196329, #99277, #68951, #161962, #26472, #147811, #146791, #37615, #194319, #116461, #192310, #132631, #55787, #88114, #149798, #25481, #115465, #24470, #70963, #193312, #117458, #40625, #102295, #177154, #163984, #131628, #38627, #11304, #8284, #160964, #41633, #148808, #114444, #10298, #178150, #176145, #72974, #162964, #22458, #86120, #71955, #151787, #92073, #185099, #198285, #74942, #44607, #42626, #184114, #136605, #12300, #28468, #13278, #59763, #106262, #199282, #43614, #46588, #169929, #45596, #108249, #75924, #139574, #137599, #121431, #60749, #167946, #153762, #29444, #107249, #150804 ),
 ( #31421, #181151, #15257, #73966, #91076, #123406, #57797, #183124, #152763, #14253, #122422, #104290, #135635, #90103, #168920, #30426, #197305, #76915, #77907, #138586, #67, #61738, #93073, #58769, #154758, #16256, #119468, #165971, #120437, #27473, #89116, #182130, #105278, #166966, #172925, #109243, #157750, #125419, #170923, #141575, #142566, #18251, #19242, #80889, #112233, #2066, #32414, #143552, #4045, #127390, #111234, #189100, #49571, #65722, #20215, #158725, #5037, #50573, #94069, #34404, #3063, #155748, #126402, #173923, #96062, #62733, #17246, #35392, #187115, #97043, #64740, #78898, #81863, #66723, #1059, #124415, #186109, #156757, #47590, #140576, #63745, #48587, #110239, #171920, #33410, #95069, #79904, #188098, #139566, #157742, #170913, #47582, #17237, #15247, #156749, #109234, #185090, #1050, #186100, #32406, #78889, #171912, #16247, #19231, #142557, #18243, #80880, #48578, #112224, #110231, #94061, #33401, #140568, #126393, #2058, #79896, #123398, #95059, #4035, #187108, #65713, #62723, #127379, #189091, #50564, #169920, #63736, #141566, #30416, #76906, #46579, #108240, #92064, #3055, #64732, #138577, #188090, #153752, #31412, #49561, #124407, #111225, #125411, #93063, #57, #34396, #172917, #61730, #154750, #155740, #96054, #77899, #132385, #9047, #84858, #162717, #173914, #192055, #20205, #35383, #8028, #38378, #82865, #146535, #143540, #161720, #69710, #114194, #52533, #144543, #129365, #175898, #22210, #115214, #159709, #101032, #85873, #23215, #24223, #53537, #55541, #176907, #191061, #100034, #83859, #131377, #145540, #193065, #66712, #54541, #147562, #130356, #70717, #6028, #194078, #97034, #158715, #113209, #7019, #116214, #81851, #5027, #128373, #190069, #51545, #177905, #39373, #174897, #36363, #99028, #160718, #98015, #21208, #67707, #37370, #68701, #133377, #152523, #167709, #71709, #58533, #164729, #29205, #42381, #198046, #103047, #121189, #86874, #89867, #182882, #136369, #90839, #12060, #137356, #87863, #104044, #195067, #57552, #106022, #10049, #56547, #181889, #26223, #148558, #59512, #72722, #199035, #102048, #118224, #149551, #14011, #150561, #11046, #40374, #197065, #119221, #179915, #135395, #120199, #75677, #117213, #28227, #41381, #27220, #73722, #178906, #134395, #163732, #25233, #196081, #180906, #165724, #44365, #88868, #43367, #105039, #166723, #151549, #13039, #74705, #141330, #49328, #155510, #17005, #157505, #110989, #30182, #140332, #93830, #60505, #168682, #79661, #122180, #91825, #78657, #172674, #183872, #156505, #153518, #1822, #126164, #142321, #139339, #170685, #107009, #76676, #92831, #154516, #125178, #15015, #47350, #80644, #77670, #32174, #64497, #95820, #61502, #109006, #2818, #34159, #45357, #138352, #63503, #818, #16013, #186875, #18998, #48345, #200034, #109999, #169685, #123171, #171679, #33169, #185864, #94828, #18007, #187859, #184859, #46342, #107998, #31180, #62492, #124163, #161485, #21974, #53297, #177668, #115979, #23976, #191816, #96800, #83626, #52299, #173679, #37130, #22973, #145303, #65479, #19975, #38145, #174665, #6786, #113956, #81618, #54307, #7788, #99799, #3801, #85631, #97782, #68465, #84621, #162474, #39136, #114976, #192826, #127141, #130119, #50332, #188848, #146300, #176669, #112973, #69471, #35146, #131138, #67467, #158487, #111988, #100791, #36130, #20965, #190824, #143301, #4787, #144304, #82622, #159470, #5794, #129126, #175656, #66477, #189839, #128139, #51312, #98790, #160484, #165488, #28969, #26984, #102807, #88629, #57313, #43131, #118988, #196830, #40125, #150325, #74469, #103808, #136134, #179673, #182645, #59276, #197810, #86633, #180671, #11820, #44129, #132142, #101803, #163490, #105788, #73485, #58298, #55299, #135157, #72479, #134152, #193835, #89626, #104800, #8807, #148316, #24988, #167474, #120946, #9811, #119966, #194828, #147317, #195840, #27987, #133137, #151314, #116971 ),
 ( #181652, #56301, #178662, #12803, #164493, #70476, #71472, #117983, #41144, #25986, #42148, #87629, #149315, #166489, #10809, #121943, #108763, #170440, #79418, #141088, #1576, #106776, #574, #47102, #169439, #31931, #93585, #16760, #153276, #155271, #107756, #183636, #2574, #184619, #75444, #156259, #123914, #90611, #78408, #46101, #152292, #64255, #30943, #17762, #172428, #137119, #29947, #199795, #125922, #92590, #168451, #154279, #187620, #45118, #91585, #140084, #61262, #14777, #32926, #15769, #13776, #198805, #76437, #138114, #49090, #185613, #122932, #60270, #63251, #77429, #139100, #124930, #186628, #110747, #62245, #48099, #109755, #171439, #94581, #112731, #52061, #190585, #160242, #96558, #175414, #51070, #126898, #146058, #127894, #18755, #99557, #67227, #33917, #113717, #189597, #95574, #22733, #174424, #161239, #115742, #80401, #173433, #143062, #84381, #35893, #97540, #20722, #21731, #68222, #159227, #82379, #4540, #144067, #5548, #128885, #36882, #19736, #7542, #69227, #83384, #130895, #98548, #157260, #145061, #6542, #129874, #191572, #53051, #114731, #176425, #188604, #37899, #192585, #54068, #142074, #66234, #3560, #65238, #50085, #34903, #111745, #158245, #81377, #162236, #131906, #70238, #12566, #195599, #26742, #85385, #41907, #102570, #164255, #23736, #119735, #134917, #38900, #178422, #193590, #74232, #27744, #55061, #118746, #24746, #89387, #25750, #58064, #163245, #181418, #147078, #150075, #42896, #196594, #151075, #72233, #197572, #148079, #87396, #135900, #59039, #40898, #8563, #104561, #116733, #166243, #177429, #100557, #180434, #39886, #88381, #101553, #86395, #133908, #57072, #9570, #71236, #132899, #103573, #10569, #194588, #56058, #117737, #179432, #149081, #165248, #11580, #73247, #16520, #13539, #154034, #186380, #2328, #199549, #30697, #167234, #136876, #153029, #14529, #185366, #75205, #107514, #140839, #137870, #92348, #124683, #156013, #121699, #169190, #139836, #32682, #43884, #198562, #138855, #61019, #76190, #15528, #109511, #62003, #90369, #108518, #29706, #152054, #77185, #93339, #45861, #170197, #46858, #47858, #44876, #60032, #79168, #31690, #1325, #335, #78168, #123669, #155024, #94335, #17510, #120706, #63005, #183394, #171193, #182405, #106532, #105549, #28732, #168209, #91337, #122691, #184380, #34660, #66984, #112488, #80158, #114472, #67978, #159993, #64009, #145814, #158004, #128643, #144816, #22487, #99309, #175168, #52805, #125678, #82126, #110499, #187376, #98291, #190337, #173184, #36634, #33666, #21480, #127654, #18511, #172181, #176175, #96318, #20476, #48845, #95328, #157013, #189354, #50831, #141829, #6299, #83141, #3322, #64995, #126653, #160993, #37645, #188356, #5300, #111498, #84135, #174181, #129632, #49834, #191327, #19496, #81141, #142822, #4302, #65984, #158984, #35650, #97298, #143819, #51814, #113473, #196357, #100313, #146821, #71983, #116491, #38657, #149827, #162995, #89144, #192340, #161992, #54816, #119497, #40655, #39645, #130646, #87154, #147842, #23488, #25510, #148837, #57825, #181179, #118503, #85137, #117490, #164014, #86152, #10327, #133658, #195348, #69992, #56828, #24500, #8316, #42656, #101306, #53822, #73003, #102324, #7297, #180193, #9328, #68981, #104318, #70993, #134672, #115497, #177184, #131660, #178180, #166002, #132661, #194349, #55817, #41663, #103326, #179187, #165006, #26500, #88142, #11332, #27502, #193342, #136631, #77934, #62763, #138613, #139601, #168947, #32443, #30454, #106288, #92101, #60778, #46617, #122450, #95, #43642, #153789, #1087, #107276, #124443, #183151, #186139, #47618, #109272, #90129, #184142, #15285, #170951, #135663, #105305, #166993, #150833, #76944, #61765, #58798, #123433, #12329, #29472, #45624, #197335, #28495, #44636, #167973, #185126, #151813, #137627, #73994, #91105, #108278, #154785, #120466, #13304, #199312, #169956, #182158, #74969, #198313, #31448, #152793 ),
 ( #59791, #93101, #14285, #121459, #75953, #16282, #144335, #8838, #130149, #129156, #17274, #176700, #37160, #125447, #115006, #38174, #85663, #147350, #7818, #110267, #6816, #53327, #175685, #99830, #161514, #23006, #156785, #84652, #113987, #187143, #70506, #190853, #78928, #162506, #191846, #94097, #146329, #52330, #155776, #132174, #98819, #24007, #178696, #140604, #33437, #5823, #193865, #160513, #22004, #83656, #69502, #131168, #145334, #68494, #67499, #192858, #54337, #116008, #177698, #79932, #55331, #117001, #39165, #2094, #100823, #63775, #48615, #171948, #95096, #18278, #136170, #150359, #89663, #133170, #58332, #167509, #196866, #29004, #72513, #75478, #152326, #90644, #179704, #73521, #181686, #137151, #25020, #194860, #56333, #198840, #120000, #151349, #165523, #12838, #166524, #44163, #164525, #118015, #60304, #28021, #59311, #43167, #197845, #104834, #74504, #13812, #121979, #40158, #120980, #41176, #182678, #88664, #9843, #135192, #105822, #101834, #163521, #102839, #86663, #10844, #148347, #11856, #26018, #71502, #87662, #149347, #134188, #195875, #57348, #119023, #180706, #42182, #103842, #27019, #172464, #183670, #1610, #29983, #45155, #17796, #48133, #92622, #94616, #153310, #79452, #47138, #138149, #91622, #95609, #15802, #140119, #106811, #14811, #168485, #157294, #65272, #108796, #76472, #2612, #199830, #64289, #142109, #61297, #124966, #125956, #156295, #187654, #33951, #78445, #63286, #80436, #18791, #122967, #186663, #16795, #184654, #46136, #49125, #107789, #169474, #109790, #3594, #30975, #141122, #154313, #171473, #110783, #77463, #62280, #93620, #139133, #610, #123948, #185646, #32962, #170475, #31965, #155306, #144100, #36917, #130927, #162271, #127928, #113751, #146091, #38932, #50119, #4576, #145093, #67260, #20756, #98580, #115774, #68255, #96592, #114763, #35926, #158281, #175447, #99591, #81411, #34940, #100589, #159260, #83416, #188640, #19770, #126932, #23771, #8598, #190619, #143097, #7575, #66269, #69261, #85421, #111779, #129906, #192618, #37930, #54100, #177463, #21765, #6576, #147112, #173467, #189630, #191606, #160274, #51104, #112764, #174457, #97572, #82411, #53085, #5580, #128918, #22765, #52094, #176457, #161271, #84414, #149116, #180470, #116766, #86429, #102606, #164292, #134952, #24782, #57108, #90402, #87431, #41942, #74266, #105580, #71271, #118782, #89421, #182438, #193624, #148115, #88419, #10607, #25785, #103608, #59072, #11614, #39924, #58099, #179469, #101593, #165284, #42931, #195635, #119769, #196630, #135936, #194623, #163281, #28765, #181453, #151110, #150113, #27779, #73282, #104595, #43918, #167266, #152087, #166282, #9606, #12602, #26777, #132936, #197606, #120739, #70272, #131940, #56094, #55096, #40934, #178457, #117775, #72268, #133945, #17544, #109545, #13572, #95364, #107548, #78201, #94368, #172217, #48881, #124717, #2363, #75239, #31724, #60065, #136910, #47892, #139871, #122724, #186415, #183425, #171227, #77219, #32716, #44909, #156047, #138888, #168243, #121733, #125714, #45895, #170231, #198597, #106566, #29739, #187413, #91372, #368, #153063, #79205, #14565, #140874, #33701, #76223, #155059, #64044, #110536, #137902, #199584, #108552, #93372, #61052, #184414, #169224, #16554, #46892, #30733, #92380, #154066, #15561, #62039, #1360, #123703, #185401, #63039, #49868, #190375, #22521, #38692, #35685, #67019, #3356, #173219, #189388, #50865, #21515, #111534, #143856, #177219, #174217, #128678, #161027, #192374, #158039, #5335, #176210, #69014, #80193, #34695, #175204, #97333, #112523, #51850, #145848, #98328, #126687, #144850, #66020, #188391, #113509, #129665, #82160, #6333, #83176, #84168, #81175, #96352, #115531, #68013, #37679, #36669, #114508, #160028, #191361, #130680, #53857, #157049, #52839, #19530, #99344, #7330, #142857, #18546, #141865, #65031, #4336, #127688, #159019, #20512, #103361, #148870, #116525 ) ),
 .UNSPECIFIED., .T., .F., .F. ) 
 B_SPLINE_SURFACE_WITH_KNOTS ( ( 4, 3, 4 ),
 ( 3, 2, 2, 2, 2, 2, 2, 2, 2, 2, 2, 2, 2, 2, 2, 2, 2, 2, 2, 2, 2, 2, 2, 2, 2, 2, 2, 2, 2, 2, 2, 2, 2, 2, 2, 2, 2, 2, 2, 2, 2, 2, 2, 2, 2, 2, 2, 2, 2, 2, 2, 2, 2, 2, 2, 2, 2, 2, 2, 2, 2, 2, 2, 2, 2, 2, 2, 2, 2, 2, 2, 2, 2, 2, 2, 2, 2, 2, 2, 2, 2, 2, 2, 2, 2, 2, 2, 2, 2, 2, 2, 2, 2, 2, 2, 2, 2, 2, 2, 2, 2, 2, 2, 2, 2, 2, 2, 2, 2, 2, 2, 2, 2, 2, 2, 2, 2, 2, 2, 2, 2, 2, 2, 2, 2, 2, 2, 2, 2, 2, 2, 2, 2, 2, 2, 2, 2, 2, 2, 2, 2, 2, 2, 2, 2, 2, 2, 2, 2, 2, 2, 2, 2, 2, 2, 2, 2, 2, 2, 2, 2, 2, 2, 2, 2, 2, 2, 2, 2, 2, 2, 2, 2, 2, 2, 2, 2, 2, 2, 2, 2, 2, 2, 2, 2, 2, 2, 2, 2, 2, 2, 2, 2, 2, 2, 2, 2, 2, 2, 2, 2, 2, 2, 2, 2, 2, 2, 2, 2, 2, 2, 2, 2, 2, 2, 2, 2, 2, 2, 2, 2, 2, 2, 2, 2, 2, 2, 2, 3 ),
 ( 0.000000000000000000, 0.5000000000000000000, 1.000000000000000000 ),
 ( 0.000000000000000000, 0.004385964912280701511, 0.008771929824561403022, 0.01315789473684210453, 0.01754385964912280604, 0.02192982456140350755, 0.02631578947368420907, 0.03070175438596491058, 0.03508771929824561209, 0.03947368421052631360, 0.04385964912280701511, 0.04824561403508771662, 0.05263157894736841813, 0.05701754385964911964, 0.06140350877192982115, 0.06578947368421052266, 0.07017543859649122417, 0.07456140350877192569, 0.07894736842105262720, 0.08333333333333332871, 0.08771929824561403022, 0.09210526315789473173, 0.09649122807017543324, 0.1008771929824561348, 0.1052631578947368363, 0.1096491228070175378, 0.1140350877192982393, 0.1184210526315789408, 0.1228070175438596423, 0.1271929824561403577, 0.1315789473684210453, 0.1359649122807017607, 0.1403508771929824483, 0.1447368421052631637, 0.1491228070175438514, 0.1535087719298245668, 0.1578947368421052544, 0.1622807017543859698, 0.1666666666666666574, 0.1710526315789473728, 0.1754385964912280604, 0.1798245614035087758, 0.1842105263157894635, 0.1885964912280701788, 0.1929824561403508665, 0.1973684210526315819, 0.2017543859649122695, 0.2061403508771929849, 0.2105263157894736725, 0.2149122807017543879, 0.2192982456140350755, 0.2236842105263157909, 0.2280701754385964786, 0.2324561403508771940, 0.2368421052631578816, 0.2412280701754385970, 0.2456140350877192846, 0.2500000000000000000, 0.2543859649122807154, 0.2587719298245614308, 0.2631578947368420907, 0.2675438596491228060, 0.2719298245614035214, 0.2763157894736842368, 0.2807017543859648967, 0.2850877192982456121, 0.2894736842105263275, 0.2938596491228070429, 0.2982456140350877027, 0.3026315789473684181, 0.3070175438596491335, 0.3114035087719298489, 0.3157894736842105088, 0.3201754385964912242, 0.3245614035087719396, 0.3289473684210526550, 0.3333333333333333148, 0.3377192982456140302, 0.3421052631578947456, 0.3464912280701754610, 0.3508771929824561209, 0.3552631578947368363, 0.3596491228070175517, 0.3640350877192982670, 0.3684210526315789269, 0.3728070175438596423, 0.3771929824561403577, 0.3815789473684210731, 0.3859649122807017330, 0.3903508771929824483, 0.3947368421052631637, 0.3991228070175438791, 0.4035087719298245390, 0.4078947368421052544, 0.4122807017543859698, 0.4166666666666666852, 0.4210526315789473450, 0.4254385964912280604, 0.4298245614035087758, 0.4342105263157894912, 0.4385964912280701511, 0.4429824561403508665, 0.4473684210526315819, 0.4517543859649122973, 0.4561403508771929571, 0.4605263157894736725, 0.4649122807017543879, 0.4692982456140351033, 0.4736842105263157632, 0.4780701754385964786, 0.4824561403508771940, 0.4868421052631579093, 0.4912280701754385692, 0.4956140350877192846, 0.5000000000000000000, 0.5043859649122807154, 0.5087719298245614308, 0.5131578947368421462, 0.5175438596491228616, 0.5219298245614034659, 0.5263157894736841813, 0.5307017543859648967, 0.5350877192982456121, 0.5394736842105263275, 0.5438596491228070429, 0.5482456140350877583, 0.5526315789473684736, 0.5570175438596490780, 0.5614035087719297934, 0.5657894736842105088, 0.5701754385964912242, 0.5745614035087719396, 0.5789473684210526550, 0.5833333333333333703, 0.5877192982456140857, 0.5921052631578946901, 0.5964912280701754055, 0.6008771929824561209, 0.6052631578947368363, 0.6096491228070175517, 0.6140350877192982670, 0.6184210526315789824, 0.6228070175438596978, 0.6271929824561403022, 0.6315789473684210176, 0.6359649122807017330, 0.6403508771929824483, 0.6447368421052631637, 0.6491228070175438791, 0.6535087719298245945, 0.6578947368421053099, 0.6622807017543859143, 0.6666666666666666297, 0.6710526315789473450, 0.6754385964912280604, 0.6798245614035087758, 0.6842105263157894912, 0.6885964912280702066, 0.6929824561403509220, 0.6973684210526315264, 0.7017543859649122417, 0.7061403508771929571, 0.7105263157894736725, 0.7149122807017543879, 0.7192982456140351033, 0.7236842105263158187, 0.7280701754385965341, 0.7324561403508771384, 0.7368421052631578538, 0.7412280701754385692, 0.7456140350877192846, 0.7500000000000000000, 0.7543859649122807154, 0.7587719298245614308, 0.7631578947368421462, 0.7675438596491228616, 0.7719298245614034659, 0.7763157894736841813, 0.7807017543859648967, 0.7850877192982456121, 0.7894736842105263275, 0.7938596491228070429, 0.7982456140350877583, 0.8026315789473684736, 0.8070175438596490780, 0.8114035087719297934, 0.8157894736842105088, 0.8201754385964912242, 0.8245614035087719396, 0.8289473684210526550, 0.8333333333333333703, 0.8377192982456140857, 0.8421052631578946901, 0.8464912280701754055, 0.8508771929824561209, 0.8552631578947368363, 0.8596491228070175517, 0.8640350877192982670, 0.8684210526315789824, 0.8728070175438596978, 0.8771929824561403022, 0.8815789473684210176, 0.8859649122807017330, 0.8903508771929824483, 0.8947368421052631637, 0.8991228070175438791, 0.9035087719298245945, 0.9078947368421053099, 0.9122807017543859143, 0.9166666666666666297, 0.9210526315789473450, 0.9254385964912280604, 0.9298245614035087758, 0.9342105263157894912, 0.9385964912280702066, 0.9429824561403509220, 0.9473684210526315264, 0.9517543859649122417, 0.9561403508771929571, 0.9605263157894736725, 0.9649122807017543879, 0.9692982456140351033, 0.9736842105263158187, 0.9780701754385965341, 0.9824561403508771384, 0.9868421052631578538, 0.9912280701754385692, 0.9956140350877192846, 1.000000000000000000 ),
 .UNSPECIFIED. ) 
 GEOMETRIC_REPRESENTATION_ITEM ( )  RATIONAL_B_SPLINE_SURFACE ( (
 ( 1.000000000000000000, 0.9659258262890683122, 1.000000000000000000, 0.9659258262890683122, 1.000000000000000000, 0.9659258262890683122, 1.000000000000000000, 0.9659258262890683122, 1.000000000000000000, 0.9659258262890683122, 1.000000000000000000, 0.9659258262890683122, 1.000000000000000000, 0.9659258262890683122, 1.000000000000000000, 0.9659258262890683122, 1.000000000000000000, 0.9659258262890683122, 1.000000000000000000, 0.9659258262890683122, 1.000000000000000000, 0.9659258262890683122, 1.000000000000000000, 0.9659258262890683122, 1.000000000000000000, 0.9659258262890683122, 1.000000000000000000, 0.9659258262890683122, 1.000000000000000000, 0.9659258262890683122, 1.000000000000000000, 0.9659258262890683122, 1.000000000000000000, 0.9659258262890683122, 1.000000000000000000, 0.9659258262890683122, 1.000000000000000000, 0.9659258262890683122, 1.000000000000000000, 0.9659258262890683122, 1.000000000000000000, 0.9659258262890683122, 1.000000000000000000, 0.9659258262890683122, 1.000000000000000000, 0.9659258262890683122, 1.000000000000000000, 0.9659258262890683122, 1.000000000000000000, 0.9659258262890683122, 1.000000000000000000, 0.9659258262890683122, 1.000000000000000000, 0.9659258262890683122, 1.000000000000000000, 0.9659258262890683122, 1.000000000000000000, 0.9659258262890683122, 1.000000000000000000, 0.9659258262890683122, 1.000000000000000000, 0.9659258262890683122, 1.000000000000000000, 0.9659258262890683122, 1.000000000000000000, 0.9659258262890683122, 1.000000000000000000, 0.9659258262890683122, 1.000000000000000000, 0.9659258262890683122, 1.000000000000000000, 0.9659258262890683122, 1.000000000000000000, 0.9659258262890683122, 1.000000000000000000, 0.9659258262890683122, 1.000000000000000000, 0.9659258262890683122, 1.000000000000000000, 0.9659258262890683122, 1.000000000000000000, 0.9659258262890683122, 1.000000000000000000, 0.9659258262890683122, 1.000000000000000000, 0.9659258262890683122, 1.000000000000000000, 0.9659258262890683122, 1.000000000000000000, 0.9659258262890683122, 1.000000000000000000, 0.9659258262890683122, 1.000000000000000000, 0.9659258262890683122, 1.000000000000000000, 0.9659258262890683122, 1.000000000000000000, 0.9659258262890683122, 1.000000000000000000, 0.9659258262890683122, 1.000000000000000000, 0.9659258262890683122, 1.000000000000000000, 0.9659258262890683122, 1.000000000000000000, 0.9659258262890683122, 1.000000000000000000, 0.9659258262890683122, 1.000000000000000000, 0.9659258262890683122, 1.000000000000000000, 0.9659258262890683122, 1.000000000000000000, 0.9659258262890683122, 1.000000000000000000, 0.9659258262890683122, 1.000000000000000000, 0.9659258262890683122, 1.000000000000000000, 0.9659258262890683122, 1.000000000000000000, 0.9659258262890683122, 1.000000000000000000, 0.9659258262890683122, 1.000000000000000000, 0.9659258262890683122, 1.000000000000000000, 0.9659258262890683122, 1.000000000000000000, 0.9659258262890683122, 1.000000000000000000, 0.9659258262890683122, 1.000000000000000000, 0.9659258262890683122, 1.000000000000000000, 0.9659258262890683122, 1.000000000000000000, 0.9659258262890683122, 1.000000000000000000, 0.9659258262890683122, 1.000000000000000000, 0.9659258262890683122, 1.000000000000000000, 0.9659258262890683122, 1.000000000000000000, 0.9659258262890683122, 1.000000000000000000, 0.9659258262890683122, 1.000000000000000000, 0.9659258262890683122, 1.000000000000000000, 0.9659258262890683122, 1.000000000000000000, 0.9659258262890683122, 1.000000000000000000, 0.9659258262890683122, 1.000000000000000000, 0.9659258262890683122, 1.000000000000000000, 0.9659258262890683122, 1.000000000000000000, 0.9659258262890683122, 1.000000000000000000, 0.9659258262890683122, 1.000000000000000000, 0.9659258262890683122, 1.000000000000000000, 0.9659258262890683122, 1.000000000000000000, 0.9659258262890683122, 1.000000000000000000, 0.9659258262890683122, 1.000000000000000000, 0.9659258262890683122, 1.000000000000000000, 0.9659258262890683122, 1.000000000000000000, 0.9659258262890683122, 1.000000000000000000, 0.9659258262890683122, 1.000000000000000000, 0.9659258262890683122, 1.000000000000000000, 0.9659258262890683122, 1.000000000000000000, 0.9659258262890683122, 1.000000000000000000, 0.9659258262890683122, 1.000000000000000000, 0.9659258262890683122, 1.000000000000000000, 0.9659258262890683122, 1.000000000000000000, 0.9659258262890683122, 1.000000000000000000, 0.9659258262890683122, 1.000000000000000000, 0.9659258262890683122, 1.000000000000000000, 0.9659258262890683122, 1.000000000000000000, 0.9659258262890683122, 1.000000000000000000, 0.9659258262890683122, 1.000000000000000000, 0.9659258262890683122, 1.000000000000000000, 0.9659258262890683122, 1.000000000000000000, 0.9659258262890683122, 1.000000000000000000, 0.9659258262890683122, 1.000000000000000000, 0.9659258262890683122, 1.000000000000000000, 0.9659258262890683122, 1.000000000000000000, 0.9659258262890683122, 1.000000000000000000, 0.9659258262890683122, 1.000000000000000000, 0.9659258262890683122, 1.000000000000000000, 0.9659258262890683122, 1.000000000000000000, 0.9659258262890683122, 1.000000000000000000, 0.9659258262890683122, 1.000000000000000000, 0.9659258262890683122, 1.000000000000000000, 0.9659258262890683122, 1.000000000000000000, 0.9659258262890683122, 1.000000000000000000, 0.9659258262890683122, 1.000000000000000000, 0.9659258262890683122, 1.000000000000000000, 0.9659258262890683122, 1.000000000000000000, 0.9659258262890683122, 1.000000000000000000, 0.9659258262890683122, 1.000000000000000000, 0.9659258262890683122, 1.000000000000000000, 0.9659258262890683122, 1.000000000000000000, 0.9659258262890683122, 1.000000000000000000, 0.9659258262890683122, 1.000000000000000000, 0.9659258262890683122, 1.000000000000000000, 0.9659258262890683122, 1.000000000000000000, 0.9659258262890683122, 1.000000000000000000, 0.9659258262890683122, 1.000000000000000000, 0.9659258262890683122, 1.000000000000000000, 0.9659258262890683122, 1.000000000000000000, 0.9659258262890683122, 1.000000000000000000, 0.9659258262890683122, 1.000000000000000000, 0.9659258262890683122, 1.000000000000000000, 0.9659258262890683122, 1.000000000000000000, 0.9659258262890683122, 1.000000000000000000, 0.9659258262890683122, 1.000000000000000000, 0.9659258262890683122, 1.000000000000000000, 0.9659258262890683122, 1.000000000000000000, 0.9659258262890683122, 1.000000000000000000, 0.9659258262890683122, 1.000000000000000000, 0.9659258262890683122, 1.000000000000000000, 0.9659258262890683122, 1.000000000000000000, 0.9659258262890683122, 1.000000000000000000, 0.9659258262890683122, 1.000000000000000000, 0.9659258262890683122, 1.000000000000000000, 0.9659258262890683122, 1.000000000000000000, 0.9659258262890683122, 1.000000000000000000, 0.9659258262890683122, 1.000000000000000000, 0.9659258262890683122, 1.000000000000000000, 0.9659258262890683122, 1.000000000000000000, 0.9659258262890683122, 1.000000000000000000, 0.9659258262890683122, 1.000000000000000000, 0.9659258262890683122, 1.000000000000000000, 0.9659258262890683122, 1.000000000000000000, 0.9659258262890683122, 1.000000000000000000, 0.9659258262890683122, 1.000000000000000000, 0.9659258262890683122, 1.000000000000000000, 0.9659258262890683122, 1.000000000000000000, 0.9659258262890683122, 1.000000000000000000, 0.9659258262890683122, 1.000000000000000000, 0.9659258262890683122, 1.000000000000000000, 0.9659258262890683122, 1.000000000000000000, 0.9659258262890683122, 1.000000000000000000, 0.9659258262890683122, 1.000000000000000000, 0.9659258262890683122, 1.000000000000000000, 0.9659258262890683122, 1.000000000000000000, 0.9659258262890683122, 1.000000000000000000, 0.9659258262890683122, 1.000000000000000000, 0.9659258262890683122, 1.000000000000000000, 0.9659258262890683122, 1.000000000000000000, 0.9659258262890683122, 1.000000000000000000, 0.9659258262890683122, 1.000000000000000000, 0.9659258262890683122, 1.000000000000000000, 0.9659258262890683122, 1.000000000000000000, 0.9659258262890683122, 1.000000000000000000, 0.9659258262890683122, 1.000000000000000000, 0.9659258262890683122, 1.000000000000000000, 0.9659258262890683122, 1.000000000000000000, 0.9659258262890683122, 1.000000000000000000, 0.9659258262890683122, 1.000000000000000000, 0.9659258262890683122, 1.000000000000000000, 0.9659258262890683122, 1.000000000000000000, 0.9659258262890683122, 1.000000000000000000, 0.9659258262890683122, 1.000000000000000000, 0.9659258262890683122, 1.000000000000000000, 0.9659258262890683122, 1.000000000000000000, 0.9659258262890683122, 1.000000000000000000, 0.9659258262890683122, 1.000000000000000000, 0.9659258262890683122, 1.000000000000000000, 0.9659258262890683122, 1.000000000000000000, 0.9659258262890683122, 1.000000000000000000, 0.9659258262890683122, 1.000000000000000000, 0.9659258262890683122, 1.000000000000000000, 0.9659258262890683122, 1.000000000000000000, 0.9659258262890683122, 1.000000000000000000, 0.9659258262890683122, 1.000000000000000000, 0.9659258262890683122, 1.000000000000000000, 0.9659258262890683122, 1.000000000000000000, 0.9659258262890683122, 1.000000000000000000, 0.9659258262890683122, 1.000000000000000000, 0.9659258262890683122, 1.000000000000000000, 0.9659258262890683122, 1.000000000000000000, 0.9659258262890683122, 1.000000000000000000, 0.9659258262890683122, 1.000000000000000000, 0.9659258262890683122, 1.000000000000000000, 0.9659258262890683122, 1.000000000000000000, 0.9659258262890683122, 1.000000000000000000, 0.9659258262890683122, 1.000000000000000000, 0.9659258262890683122, 1.000000000000000000, 0.9659258262890683122, 1.000000000000000000, 0.9659258262890683122, 1.000000000000000000, 0.9659258262890683122, 1.000000000000000000, 0.9659258262890683122, 1.000000000000000000, 0.9659258262890683122, 1.000000000000000000, 0.9659258262890683122, 1.000000000000000000, 0.9659258262890683122, 1.000000000000000000, 0.9659258262890683122, 1.000000000000000000, 0.9659258262890683122, 1.000000000000000000, 0.9659258262890683122, 1.000000000000000000, 0.9659258262890683122, 1.000000000000000000, 0.9659258262890683122, 1.000000000000000000, 0.9659258262890683122, 1.000000000000000000, 0.9659258262890683122, 1.000000000000000000, 0.9659258262890683122, 1.000000000000000000, 0.9659258262890683122, 1.000000000000000000, 0.9659258262890683122, 1.000000000000000000),
 ( 0.3333333333333333703, 0.3219752754296894559, 0.3333333333333333703, 0.3219752754296894559, 0.3333333333333333703, 0.3219752754296894559, 0.3333333333333333703, 0.3219752754296894559, 0.3333333333333333703, 0.3219752754296894559, 0.3333333333333333703, 0.3219752754296894559, 0.3333333333333333703, 0.3219752754296894559, 0.3333333333333333703, 0.3219752754296894559, 0.3333333333333333703, 0.3219752754296894559, 0.3333333333333333703, 0.3219752754296894559, 0.3333333333333333703, 0.3219752754296894559, 0.3333333333333333703, 0.3219752754296894559, 0.3333333333333333703, 0.3219752754296894559, 0.3333333333333333703, 0.3219752754296894559, 0.3333333333333333703, 0.3219752754296894559, 0.3333333333333333703, 0.3219752754296894559, 0.3333333333333333703, 0.3219752754296894559, 0.3333333333333333703, 0.3219752754296894559, 0.3333333333333333703, 0.3219752754296894559, 0.3333333333333333703, 0.3219752754296894559, 0.3333333333333333703, 0.3219752754296894559, 0.3333333333333333703, 0.3219752754296894559, 0.3333333333333333703, 0.3219752754296894559, 0.3333333333333333703, 0.3219752754296894559, 0.3333333333333333703, 0.3219752754296894559, 0.3333333333333333703, 0.3219752754296894559, 0.3333333333333333703, 0.3219752754296894559, 0.3333333333333333703, 0.3219752754296894559, 0.3333333333333333703, 0.3219752754296894559, 0.3333333333333333703, 0.3219752754296894559, 0.3333333333333333703, 0.3219752754296894559, 0.3333333333333333703, 0.3219752754296894559, 0.3333333333333333703, 0.3219752754296894559, 0.3333333333333333703, 0.3219752754296894559, 0.3333333333333333703, 0.3219752754296894559, 0.3333333333333333703, 0.3219752754296894559, 0.3333333333333333703, 0.3219752754296894559, 0.3333333333333333703, 0.3219752754296894559, 0.3333333333333333703, 0.3219752754296894559, 0.3333333333333333703, 0.3219752754296894559, 0.3333333333333333703, 0.3219752754296894559, 0.3333333333333333703, 0.3219752754296894559, 0.3333333333333333703, 0.3219752754296894559, 0.3333333333333333703, 0.3219752754296894559, 0.3333333333333333703, 0.3219752754296894559, 0.3333333333333333703, 0.3219752754296894559, 0.3333333333333333703, 0.3219752754296894559, 0.3333333333333333703, 0.3219752754296894559, 0.3333333333333333703, 0.3219752754296894559, 0.3333333333333333703, 0.3219752754296894559, 0.3333333333333333703, 0.3219752754296894559, 0.3333333333333333703, 0.3219752754296894559, 0.3333333333333333703, 0.3219752754296894559, 0.3333333333333333703, 0.3219752754296894559, 0.3333333333333333703, 0.3219752754296894559, 0.3333333333333333703, 0.3219752754296894559, 0.3333333333333333703, 0.3219752754296894559, 0.3333333333333333703, 0.3219752754296894559, 0.3333333333333333703, 0.3219752754296894559, 0.3333333333333333703, 0.3219752754296894559, 0.3333333333333333703, 0.3219752754296894559, 0.3333333333333333703, 0.3219752754296894559, 0.3333333333333333703, 0.3219752754296894559, 0.3333333333333333703, 0.3219752754296894559, 0.3333333333333333703, 0.3219752754296894559, 0.3333333333333333703, 0.3219752754296894559, 0.3333333333333333703, 0.3219752754296894559, 0.3333333333333333703, 0.3219752754296894559, 0.3333333333333333703, 0.3219752754296894559, 0.3333333333333333703, 0.3219752754296894559, 0.3333333333333333703, 0.3219752754296894559, 0.3333333333333333703, 0.3219752754296894559, 0.3333333333333333703, 0.3219752754296894559, 0.3333333333333333703, 0.3219752754296894559, 0.3333333333333333703, 0.3219752754296894559, 0.3333333333333333703, 0.3219752754296894559, 0.3333333333333333703, 0.3219752754296894559, 0.3333333333333333703, 0.3219752754296894559, 0.3333333333333333703, 0.3219752754296894559, 0.3333333333333333703, 0.3219752754296894559, 0.3333333333333333703, 0.3219752754296894559, 0.3333333333333333703, 0.3219752754296894559, 0.3333333333333333703, 0.3219752754296894559, 0.3333333333333333703, 0.3219752754296894559, 0.3333333333333333703, 0.3219752754296894559, 0.3333333333333333703, 0.3219752754296894559, 0.3333333333333333703, 0.3219752754296894559, 0.3333333333333333703, 0.3219752754296894559, 0.3333333333333333703, 0.3219752754296894559, 0.3333333333333333703, 0.3219752754296894559, 0.3333333333333333703, 0.3219752754296894559, 0.3333333333333333703, 0.3219752754296894559, 0.3333333333333333703, 0.3219752754296894559, 0.3333333333333333703, 0.3219752754296894559, 0.3333333333333333703, 0.3219752754296894559, 0.3333333333333333703, 0.3219752754296894559, 0.3333333333333333703, 0.3219752754296894559, 0.3333333333333333703, 0.3219752754296894559, 0.3333333333333333703, 0.3219752754296894559, 0.3333333333333333703, 0.3219752754296894559, 0.3333333333333333703, 0.3219752754296894559, 0.3333333333333333703, 0.3219752754296894559, 0.3333333333333333703, 0.3219752754296894559, 0.3333333333333333703, 0.3219752754296894559, 0.3333333333333333703, 0.3219752754296894559, 0.3333333333333333703, 0.3219752754296894559, 0.3333333333333333703, 0.3219752754296894559, 0.3333333333333333703, 0.3219752754296894559, 0.3333333333333333703, 0.3219752754296894559, 0.3333333333333333703, 0.3219752754296894559, 0.3333333333333333703, 0.3219752754296894559, 0.3333333333333333703, 0.3219752754296894559, 0.3333333333333333703, 0.3219752754296894559, 0.3333333333333333703, 0.3219752754296894559, 0.3333333333333333703, 0.3219752754296894559, 0.3333333333333333703, 0.3219752754296894559, 0.3333333333333333703, 0.3219752754296894559, 0.3333333333333333703, 0.3219752754296894559, 0.3333333333333333703, 0.3219752754296894559, 0.3333333333333333703, 0.3219752754296894559, 0.3333333333333333703, 0.3219752754296894559, 0.3333333333333333703, 0.3219752754296894559, 0.3333333333333333703, 0.3219752754296894559, 0.3333333333333333703, 0.3219752754296894559, 0.3333333333333333703, 0.3219752754296894559, 0.3333333333333333703, 0.3219752754296894559, 0.3333333333333333703, 0.3219752754296894559, 0.3333333333333333703, 0.3219752754296894559, 0.3333333333333333703, 0.3219752754296894559, 0.3333333333333333703, 0.3219752754296894559, 0.3333333333333333703, 0.3219752754296894559, 0.3333333333333333703, 0.3219752754296894559, 0.3333333333333333703, 0.3219752754296894559, 0.3333333333333333703, 0.3219752754296894559, 0.3333333333333333703, 0.3219752754296894559, 0.3333333333333333703, 0.3219752754296894559, 0.3333333333333333703, 0.3219752754296894559, 0.3333333333333333703, 0.3219752754296894559, 0.3333333333333333703, 0.3219752754296894559, 0.3333333333333333703, 0.3219752754296894559, 0.3333333333333333703, 0.3219752754296894559, 0.3333333333333333703, 0.3219752754296894559, 0.3333333333333333703, 0.3219752754296894559, 0.3333333333333333703, 0.3219752754296894559, 0.3333333333333333703, 0.3219752754296894559, 0.3333333333333333703, 0.3219752754296894559, 0.3333333333333333703, 0.3219752754296894559, 0.3333333333333333703, 0.3219752754296894559, 0.3333333333333333703, 0.3219752754296894559, 0.3333333333333333703, 0.3219752754296894559, 0.3333333333333333703, 0.3219752754296894559, 0.3333333333333333703, 0.3219752754296894559, 0.3333333333333333703, 0.3219752754296894559, 0.3333333333333333703, 0.3219752754296894559, 0.3333333333333333703, 0.3219752754296894559, 0.3333333333333333703, 0.3219752754296894559, 0.3333333333333333703, 0.3219752754296894559, 0.3333333333333333703, 0.3219752754296894559, 0.3333333333333333703, 0.3219752754296894559, 0.3333333333333333703, 0.3219752754296894559, 0.3333333333333333703, 0.3219752754296894559, 0.3333333333333333703, 0.3219752754296894559, 0.3333333333333333703, 0.3219752754296894559, 0.3333333333333333703, 0.3219752754296894559, 0.3333333333333333703, 0.3219752754296894559, 0.3333333333333333703, 0.3219752754296894559, 0.3333333333333333703, 0.3219752754296894559, 0.3333333333333333703, 0.3219752754296894559, 0.3333333333333333703, 0.3219752754296894559, 0.3333333333333333703, 0.3219752754296894559, 0.3333333333333333703, 0.3219752754296894559, 0.3333333333333333703, 0.3219752754296894559, 0.3333333333333333703, 0.3219752754296894559, 0.3333333333333333703, 0.3219752754296894559, 0.3333333333333333703, 0.3219752754296894559, 0.3333333333333333703, 0.3219752754296894559, 0.3333333333333333703, 0.3219752754296894559, 0.3333333333333333703, 0.3219752754296894559, 0.3333333333333333703, 0.3219752754296894559, 0.3333333333333333703, 0.3219752754296894559, 0.3333333333333333703, 0.3219752754296894559, 0.3333333333333333703, 0.3219752754296894559, 0.3333333333333333703, 0.3219752754296894559, 0.3333333333333333703, 0.3219752754296894559, 0.3333333333333333703, 0.3219752754296894559, 0.3333333333333333703, 0.3219752754296894559, 0.3333333333333333703, 0.3219752754296894559, 0.3333333333333333703, 0.3219752754296894559, 0.3333333333333333703, 0.3219752754296894559, 0.3333333333333333703, 0.3219752754296894559, 0.3333333333333333703, 0.3219752754296894559, 0.3333333333333333703, 0.3219752754296894559, 0.3333333333333333703, 0.3219752754296894559, 0.3333333333333333703, 0.3219752754296894559, 0.3333333333333333703, 0.3219752754296894559, 0.3333333333333333703, 0.3219752754296894559, 0.3333333333333333703, 0.3219752754296894559, 0.3333333333333333703, 0.3219752754296894559, 0.3333333333333333703, 0.3219752754296894559, 0.3333333333333333703, 0.3219752754296894559, 0.3333333333333333703, 0.3219752754296894559, 0.3333333333333333703, 0.3219752754296894559, 0.3333333333333333703, 0.3219752754296894559, 0.3333333333333333703, 0.3219752754296894559, 0.3333333333333333703, 0.3219752754296894559, 0.3333333333333333703, 0.3219752754296894559, 0.3333333333333333703, 0.3219752754296894559, 0.3333333333333333703, 0.3219752754296894559, 0.3333333333333333703, 0.3219752754296894559, 0.3333333333333333703, 0.3219752754296894559, 0.3333333333333333703, 0.3219752754296894559, 0.3333333333333333703, 0.3219752754296894559, 0.3333333333333333703, 0.3219752754296894559, 0.3333333333333333703, 0.3219752754296894559, 0.3333333333333333703, 0.3219752754296894559, 0.3333333333333333703, 0.3219752754296894559, 0.3333333333333333703, 0.3219752754296894559, 0.3333333333333333703, 0.3219752754296894559, 0.3333333333333333703, 0.3219752754296894559, 0.3333333333333333703, 0.3219752754296894559, 0.3333333333333333703, 0.3219752754296894559, 0.3333333333333333703, 0.3219752754296894559, 0.3333333333333333703, 0.3219752754296894559, 0.3333333333333333703, 0.3219752754296894559, 0.3333333333333333703, 0.3219752754296894559, 0.3333333333333333703, 0.3219752754296894559, 0.3333333333333333703, 0.3219752754296894559, 0.3333333333333333703, 0.3219752754296894559, 0.3333333333333333703),
 ( 0.3333333333333333703, 0.3219752754296894559, 0.3333333333333333703, 0.3219752754296894559, 0.3333333333333333703, 0.3219752754296894559, 0.3333333333333333703, 0.3219752754296894559, 0.3333333333333333703, 0.3219752754296894559, 0.3333333333333333703, 0.3219752754296894559, 0.3333333333333333703, 0.3219752754296894559, 0.3333333333333333703, 0.3219752754296894559, 0.3333333333333333703, 0.3219752754296894559, 0.3333333333333333703, 0.3219752754296894559, 0.3333333333333333703, 0.3219752754296894559, 0.3333333333333333703, 0.3219752754296894559, 0.3333333333333333703, 0.3219752754296894559, 0.3333333333333333703, 0.3219752754296894559, 0.3333333333333333703, 0.3219752754296894559, 0.3333333333333333703, 0.3219752754296894559, 0.3333333333333333703, 0.3219752754296894559, 0.3333333333333333703, 0.3219752754296894559, 0.3333333333333333703, 0.3219752754296894559, 0.3333333333333333703, 0.3219752754296894559, 0.3333333333333333703, 0.3219752754296894559, 0.3333333333333333703, 0.3219752754296894559, 0.3333333333333333703, 0.3219752754296894559, 0.3333333333333333703, 0.3219752754296894559, 0.3333333333333333703, 0.3219752754296894559, 0.3333333333333333703, 0.3219752754296894559, 0.3333333333333333703, 0.3219752754296894559, 0.3333333333333333703, 0.3219752754296894559, 0.3333333333333333703, 0.3219752754296894559, 0.3333333333333333703, 0.3219752754296894559, 0.3333333333333333703, 0.3219752754296894559, 0.3333333333333333703, 0.3219752754296894559, 0.3333333333333333703, 0.3219752754296894559, 0.3333333333333333703, 0.3219752754296894559, 0.3333333333333333703, 0.3219752754296894559, 0.3333333333333333703, 0.3219752754296894559, 0.3333333333333333703, 0.3219752754296894559, 0.3333333333333333703, 0.3219752754296894559, 0.3333333333333333703, 0.3219752754296894559, 0.3333333333333333703, 0.3219752754296894559, 0.3333333333333333703, 0.3219752754296894559, 0.3333333333333333703, 0.3219752754296894559, 0.3333333333333333703, 0.3219752754296894559, 0.3333333333333333703, 0.3219752754296894559, 0.3333333333333333703, 0.3219752754296894559, 0.3333333333333333703, 0.3219752754296894559, 0.3333333333333333703, 0.3219752754296894559, 0.3333333333333333703, 0.3219752754296894559, 0.3333333333333333703, 0.3219752754296894559, 0.3333333333333333703, 0.3219752754296894559, 0.3333333333333333703, 0.3219752754296894559, 0.3333333333333333703, 0.3219752754296894559, 0.3333333333333333703, 0.3219752754296894559, 0.3333333333333333703, 0.3219752754296894559, 0.3333333333333333703, 0.3219752754296894559, 0.3333333333333333703, 0.3219752754296894559, 0.3333333333333333703, 0.3219752754296894559, 0.3333333333333333703, 0.3219752754296894559, 0.3333333333333333703, 0.3219752754296894559, 0.3333333333333333703, 0.3219752754296894559, 0.3333333333333333703, 0.3219752754296894559, 0.3333333333333333703, 0.3219752754296894559, 0.3333333333333333703, 0.3219752754296894559, 0.3333333333333333703, 0.3219752754296894559, 0.3333333333333333703, 0.3219752754296894559, 0.3333333333333333703, 0.3219752754296894559, 0.3333333333333333703, 0.3219752754296894559, 0.3333333333333333703, 0.3219752754296894559, 0.3333333333333333703, 0.3219752754296894559, 0.3333333333333333703, 0.3219752754296894559, 0.3333333333333333703, 0.3219752754296894559, 0.3333333333333333703, 0.3219752754296894559, 0.3333333333333333703, 0.3219752754296894559, 0.3333333333333333703, 0.3219752754296894559, 0.3333333333333333703, 0.3219752754296894559, 0.3333333333333333703, 0.3219752754296894559, 0.3333333333333333703, 0.3219752754296894559, 0.3333333333333333703, 0.3219752754296894559, 0.3333333333333333703, 0.3219752754296894559, 0.3333333333333333703, 0.3219752754296894559, 0.3333333333333333703, 0.3219752754296894559, 0.3333333333333333703, 0.3219752754296894559, 0.3333333333333333703, 0.3219752754296894559, 0.3333333333333333703, 0.3219752754296894559, 0.3333333333333333703, 0.3219752754296894559, 0.3333333333333333703, 0.3219752754296894559, 0.3333333333333333703, 0.3219752754296894559, 0.3333333333333333703, 0.3219752754296894559, 0.3333333333333333703, 0.3219752754296894559, 0.3333333333333333703, 0.3219752754296894559, 0.3333333333333333703, 0.3219752754296894559, 0.3333333333333333703, 0.3219752754296894559, 0.3333333333333333703, 0.3219752754296894559, 0.3333333333333333703, 0.3219752754296894559, 0.3333333333333333703, 0.3219752754296894559, 0.3333333333333333703, 0.3219752754296894559, 0.3333333333333333703, 0.3219752754296894559, 0.3333333333333333703, 0.3219752754296894559, 0.3333333333333333703, 0.3219752754296894559, 0.3333333333333333703, 0.3219752754296894559, 0.3333333333333333703, 0.3219752754296894559, 0.3333333333333333703, 0.3219752754296894559, 0.3333333333333333703, 0.3219752754296894559, 0.3333333333333333703, 0.3219752754296894559, 0.3333333333333333703, 0.3219752754296894559, 0.3333333333333333703, 0.3219752754296894559, 0.3333333333333333703, 0.3219752754296894559, 0.3333333333333333703, 0.3219752754296894559, 0.3333333333333333703, 0.3219752754296894559, 0.3333333333333333703, 0.3219752754296894559, 0.3333333333333333703, 0.3219752754296894559, 0.3333333333333333703, 0.3219752754296894559, 0.3333333333333333703, 0.3219752754296894559, 0.3333333333333333703, 0.3219752754296894559, 0.3333333333333333703, 0.3219752754296894559, 0.3333333333333333703, 0.3219752754296894559, 0.3333333333333333703, 0.3219752754296894559, 0.3333333333333333703, 0.3219752754296894559, 0.3333333333333333703, 0.3219752754296894559, 0.3333333333333333703, 0.3219752754296894559, 0.3333333333333333703, 0.3219752754296894559, 0.3333333333333333703, 0.3219752754296894559, 0.3333333333333333703, 0.3219752754296894559, 0.3333333333333333703, 0.3219752754296894559, 0.3333333333333333703, 0.3219752754296894559, 0.3333333333333333703, 0.3219752754296894559, 0.3333333333333333703, 0.3219752754296894559, 0.3333333333333333703, 0.3219752754296894559, 0.3333333333333333703, 0.3219752754296894559, 0.3333333333333333703, 0.3219752754296894559, 0.3333333333333333703, 0.3219752754296894559, 0.3333333333333333703, 0.3219752754296894559, 0.3333333333333333703, 0.3219752754296894559, 0.3333333333333333703, 0.3219752754296894559, 0.3333333333333333703, 0.3219752754296894559, 0.3333333333333333703, 0.3219752754296894559, 0.3333333333333333703, 0.3219752754296894559, 0.3333333333333333703, 0.3219752754296894559, 0.3333333333333333703, 0.3219752754296894559, 0.3333333333333333703, 0.3219752754296894559, 0.3333333333333333703, 0.3219752754296894559, 0.3333333333333333703, 0.3219752754296894559, 0.3333333333333333703, 0.3219752754296894559, 0.3333333333333333703, 0.3219752754296894559, 0.3333333333333333703, 0.3219752754296894559, 0.3333333333333333703, 0.3219752754296894559, 0.3333333333333333703, 0.3219752754296894559, 0.3333333333333333703, 0.3219752754296894559, 0.3333333333333333703, 0.3219752754296894559, 0.3333333333333333703, 0.3219752754296894559, 0.3333333333333333703, 0.3219752754296894559, 0.3333333333333333703, 0.3219752754296894559, 0.3333333333333333703, 0.3219752754296894559, 0.3333333333333333703, 0.3219752754296894559, 0.3333333333333333703, 0.3219752754296894559, 0.3333333333333333703, 0.3219752754296894559, 0.3333333333333333703, 0.3219752754296894559, 0.3333333333333333703, 0.3219752754296894559, 0.3333333333333333703, 0.3219752754296894559, 0.3333333333333333703, 0.3219752754296894559, 0.3333333333333333703, 0.3219752754296894559, 0.3333333333333333703, 0.3219752754296894559, 0.3333333333333333703, 0.3219752754296894559, 0.3333333333333333703, 0.3219752754296894559, 0.3333333333333333703, 0.3219752754296894559, 0.3333333333333333703, 0.3219752754296894559, 0.3333333333333333703, 0.3219752754296894559, 0.3333333333333333703, 0.3219752754296894559, 0.3333333333333333703, 0.3219752754296894559, 0.3333333333333333703, 0.3219752754296894559, 0.3333333333333333703, 0.3219752754296894559, 0.3333333333333333703, 0.3219752754296894559, 0.3333333333333333703, 0.3219752754296894559, 0.3333333333333333703, 0.3219752754296894559, 0.3333333333333333703, 0.3219752754296894559, 0.3333333333333333703, 0.3219752754296894559, 0.3333333333333333703, 0.3219752754296894559, 0.3333333333333333703, 0.3219752754296894559, 0.3333333333333333703, 0.3219752754296894559, 0.3333333333333333703, 0.3219752754296894559, 0.3333333333333333703, 0.3219752754296894559, 0.3333333333333333703, 0.3219752754296894559, 0.3333333333333333703, 0.3219752754296894559, 0.3333333333333333703, 0.3219752754296894559, 0.3333333333333333703, 0.3219752754296894559, 0.3333333333333333703, 0.3219752754296894559, 0.3333333333333333703, 0.3219752754296894559, 0.3333333333333333703, 0.3219752754296894559, 0.3333333333333333703, 0.3219752754296894559, 0.3333333333333333703, 0.3219752754296894559, 0.3333333333333333703, 0.3219752754296894559, 0.3333333333333333703, 0.3219752754296894559, 0.3333333333333333703, 0.3219752754296894559, 0.3333333333333333703, 0.3219752754296894559, 0.3333333333333333703, 0.3219752754296894559, 0.3333333333333333703, 0.3219752754296894559, 0.3333333333333333703, 0.3219752754296894559, 0.3333333333333333703, 0.3219752754296894559, 0.3333333333333333703, 0.3219752754296894559, 0.3333333333333333703, 0.3219752754296894559, 0.3333333333333333703, 0.3219752754296894559, 0.3333333333333333703, 0.3219752754296894559, 0.3333333333333333703, 0.3219752754296894559, 0.3333333333333333703, 0.3219752754296894559, 0.3333333333333333703, 0.3219752754296894559, 0.3333333333333333703, 0.3219752754296894559, 0.3333333333333333703, 0.3219752754296894559, 0.3333333333333333703, 0.3219752754296894559, 0.3333333333333333703, 0.3219752754296894559, 0.3333333333333333703, 0.3219752754296894559, 0.3333333333333333703, 0.3219752754296894559, 0.3333333333333333703, 0.3219752754296894559, 0.3333333333333333703, 0.3219752754296894559, 0.3333333333333333703, 0.3219752754296894559, 0.3333333333333333703, 0.3219752754296894559, 0.3333333333333333703, 0.3219752754296894559, 0.3333333333333333703, 0.3219752754296894559, 0.3333333333333333703, 0.3219752754296894559, 0.3333333333333333703, 0.3219752754296894559, 0.3333333333333333703, 0.3219752754296894559, 0.3333333333333333703, 0.3219752754296894559, 0.3333333333333333703, 0.3219752754296894559, 0.3333333333333333703, 0.3219752754296894559, 0.3333333333333333703, 0.3219752754296894559, 0.3333333333333333703, 0.3219752754296894559, 0.3333333333333333703, 0.3219752754296894559, 0.3333333333333333703, 0.3219752754296894559, 0.3333333333333333703, 0.3219752754296894559, 0.3333333333333333703),
 ( 1.000000000000000000, 0.9659258262890683122, 1.000000000000000000, 0.9659258262890683122, 1.000000000000000000, 0.9659258262890683122, 1.000000000000000000, 0.9659258262890683122, 1.000000000000000000, 0.9659258262890683122, 1.000000000000000000, 0.9659258262890683122, 1.000000000000000000, 0.9659258262890683122, 1.000000000000000000, 0.9659258262890683122, 1.000000000000000000, 0.9659258262890683122, 1.000000000000000000, 0.9659258262890683122, 1.000000000000000000, 0.9659258262890683122, 1.000000000000000000, 0.9659258262890683122, 1.000000000000000000, 0.9659258262890683122, 1.000000000000000000, 0.9659258262890683122, 1.000000000000000000, 0.9659258262890683122, 1.000000000000000000, 0.9659258262890683122, 1.000000000000000000, 0.9659258262890683122, 1.000000000000000000, 0.9659258262890683122, 1.000000000000000000, 0.9659258262890683122, 1.000000000000000000, 0.9659258262890683122, 1.000000000000000000, 0.9659258262890683122, 1.000000000000000000, 0.9659258262890683122, 1.000000000000000000, 0.9659258262890683122, 1.000000000000000000, 0.9659258262890683122, 1.000000000000000000, 0.9659258262890683122, 1.000000000000000000, 0.9659258262890683122, 1.000000000000000000, 0.9659258262890683122, 1.000000000000000000, 0.9659258262890683122, 1.000000000000000000, 0.9659258262890683122, 1.000000000000000000, 0.9659258262890683122, 1.000000000000000000, 0.9659258262890683122, 1.000000000000000000, 0.9659258262890683122, 1.000000000000000000, 0.9659258262890683122, 1.000000000000000000, 0.9659258262890683122, 1.000000000000000000, 0.9659258262890683122, 1.000000000000000000, 0.9659258262890683122, 1.000000000000000000, 0.9659258262890683122, 1.000000000000000000, 0.9659258262890683122, 1.000000000000000000, 0.9659258262890683122, 1.000000000000000000, 0.9659258262890683122, 1.000000000000000000, 0.9659258262890683122, 1.000000000000000000, 0.9659258262890683122, 1.000000000000000000, 0.9659258262890683122, 1.000000000000000000, 0.9659258262890683122, 1.000000000000000000, 0.9659258262890683122, 1.000000000000000000, 0.9659258262890683122, 1.000000000000000000, 0.9659258262890683122, 1.000000000000000000, 0.9659258262890683122, 1.000000000000000000, 0.9659258262890683122, 1.000000000000000000, 0.9659258262890683122, 1.000000000000000000, 0.9659258262890683122, 1.000000000000000000, 0.9659258262890683122, 1.000000000000000000, 0.9659258262890683122, 1.000000000000000000, 0.9659258262890683122, 1.000000000000000000, 0.9659258262890683122, 1.000000000000000000, 0.9659258262890683122, 1.000000000000000000, 0.9659258262890683122, 1.000000000000000000, 0.9659258262890683122, 1.000000000000000000, 0.9659258262890683122, 1.000000000000000000, 0.9659258262890683122, 1.000000000000000000, 0.9659258262890683122, 1.000000000000000000, 0.9659258262890683122, 1.000000000000000000, 0.9659258262890683122, 1.000000000000000000, 0.9659258262890683122, 1.000000000000000000, 0.9659258262890683122, 1.000000000000000000, 0.9659258262890683122, 1.000000000000000000, 0.9659258262890683122, 1.000000000000000000, 0.9659258262890683122, 1.000000000000000000, 0.9659258262890683122, 1.000000000000000000, 0.9659258262890683122, 1.000000000000000000, 0.9659258262890683122, 1.000000000000000000, 0.9659258262890683122, 1.000000000000000000, 0.9659258262890683122, 1.000000000000000000, 0.9659258262890683122, 1.000000000000000000, 0.9659258262890683122, 1.000000000000000000, 0.9659258262890683122, 1.000000000000000000, 0.9659258262890683122, 1.000000000000000000, 0.9659258262890683122, 1.000000000000000000, 0.9659258262890683122, 1.000000000000000000, 0.9659258262890683122, 1.000000000000000000, 0.9659258262890683122, 1.000000000000000000, 0.9659258262890683122, 1.000000000000000000, 0.9659258262890683122, 1.000000000000000000, 0.9659258262890683122, 1.000000000000000000, 0.9659258262890683122, 1.000000000000000000, 0.9659258262890683122, 1.000000000000000000, 0.9659258262890683122, 1.000000000000000000, 0.9659258262890683122, 1.000000000000000000, 0.9659258262890683122, 1.000000000000000000, 0.9659258262890683122, 1.000000000000000000, 0.9659258262890683122, 1.000000000000000000, 0.9659258262890683122, 1.000000000000000000, 0.9659258262890683122, 1.000000000000000000, 0.9659258262890683122, 1.000000000000000000, 0.9659258262890683122, 1.000000000000000000, 0.9659258262890683122, 1.000000000000000000, 0.9659258262890683122, 1.000000000000000000, 0.9659258262890683122, 1.000000000000000000, 0.9659258262890683122, 1.000000000000000000, 0.9659258262890683122, 1.000000000000000000, 0.9659258262890683122, 1.000000000000000000, 0.9659258262890683122, 1.000000000000000000, 0.9659258262890683122, 1.000000000000000000, 0.9659258262890683122, 1.000000000000000000, 0.9659258262890683122, 1.000000000000000000, 0.9659258262890683122, 1.000000000000000000, 0.9659258262890683122, 1.000000000000000000, 0.9659258262890683122, 1.000000000000000000, 0.9659258262890683122, 1.000000000000000000, 0.9659258262890683122, 1.000000000000000000, 0.9659258262890683122, 1.000000000000000000, 0.9659258262890683122, 1.000000000000000000, 0.9659258262890683122, 1.000000000000000000, 0.9659258262890683122, 1.000000000000000000, 0.9659258262890683122, 1.000000000000000000, 0.9659258262890683122, 1.000000000000000000, 0.9659258262890683122, 1.000000000000000000, 0.9659258262890683122, 1.000000000000000000, 0.9659258262890683122, 1.000000000000000000, 0.9659258262890683122, 1.000000000000000000, 0.9659258262890683122, 1.000000000000000000, 0.9659258262890683122, 1.000000000000000000, 0.9659258262890683122, 1.000000000000000000, 0.9659258262890683122, 1.000000000000000000, 0.9659258262890683122, 1.000000000000000000, 0.9659258262890683122, 1.000000000000000000, 0.9659258262890683122, 1.000000000000000000, 0.9659258262890683122, 1.000000000000000000, 0.9659258262890683122, 1.000000000000000000, 0.9659258262890683122, 1.000000000000000000, 0.9659258262890683122, 1.000000000000000000, 0.9659258262890683122, 1.000000000000000000, 0.9659258262890683122, 1.000000000000000000, 0.9659258262890683122, 1.000000000000000000, 0.9659258262890683122, 1.000000000000000000, 0.9659258262890683122, 1.000000000000000000, 0.9659258262890683122, 1.000000000000000000, 0.9659258262890683122, 1.000000000000000000, 0.9659258262890683122, 1.000000000000000000, 0.9659258262890683122, 1.000000000000000000, 0.9659258262890683122, 1.000000000000000000, 0.9659258262890683122, 1.000000000000000000, 0.9659258262890683122, 1.000000000000000000, 0.9659258262890683122, 1.000000000000000000, 0.9659258262890683122, 1.000000000000000000, 0.9659258262890683122, 1.000000000000000000, 0.9659258262890683122, 1.000000000000000000, 0.9659258262890683122, 1.000000000000000000, 0.9659258262890683122, 1.000000000000000000, 0.9659258262890683122, 1.000000000000000000, 0.9659258262890683122, 1.000000000000000000, 0.9659258262890683122, 1.000000000000000000, 0.9659258262890683122, 1.000000000000000000, 0.9659258262890683122, 1.000000000000000000, 0.9659258262890683122, 1.000000000000000000, 0.9659258262890683122, 1.000000000000000000, 0.9659258262890683122, 1.000000000000000000, 0.9659258262890683122, 1.000000000000000000, 0.9659258262890683122, 1.000000000000000000, 0.9659258262890683122, 1.000000000000000000, 0.9659258262890683122, 1.000000000000000000, 0.9659258262890683122, 1.000000000000000000, 0.9659258262890683122, 1.000000000000000000, 0.9659258262890683122, 1.000000000000000000, 0.9659258262890683122, 1.000000000000000000, 0.9659258262890683122, 1.000000000000000000, 0.9659258262890683122, 1.000000000000000000, 0.9659258262890683122, 1.000000000000000000, 0.9659258262890683122, 1.000000000000000000, 0.9659258262890683122, 1.000000000000000000, 0.9659258262890683122, 1.000000000000000000, 0.9659258262890683122, 1.000000000000000000, 0.9659258262890683122, 1.000000000000000000, 0.9659258262890683122, 1.000000000000000000, 0.9659258262890683122, 1.000000000000000000, 0.9659258262890683122, 1.000000000000000000, 0.9659258262890683122, 1.000000000000000000, 0.9659258262890683122, 1.000000000000000000, 0.9659258262890683122, 1.000000000000000000, 0.9659258262890683122, 1.000000000000000000, 0.9659258262890683122, 1.000000000000000000, 0.9659258262890683122, 1.000000000000000000, 0.9659258262890683122, 1.000000000000000000, 0.9659258262890683122, 1.000000000000000000, 0.9659258262890683122, 1.000000000000000000, 0.9659258262890683122, 1.000000000000000000, 0.9659258262890683122, 1.000000000000000000, 0.9659258262890683122, 1.000000000000000000, 0.9659258262890683122, 1.000000000000000000, 0.9659258262890683122, 1.000000000000000000, 0.9659258262890683122, 1.000000000000000000, 0.9659258262890683122, 1.000000000000000000, 0.9659258262890683122, 1.000000000000000000, 0.9659258262890683122, 1.000000000000000000, 0.9659258262890683122, 1.000000000000000000, 0.9659258262890683122, 1.000000000000000000, 0.9659258262890683122, 1.000000000000000000, 0.9659258262890683122, 1.000000000000000000, 0.9659258262890683122, 1.000000000000000000, 0.9659258262890683122, 1.000000000000000000, 0.9659258262890683122, 1.000000000000000000, 0.9659258262890683122, 1.000000000000000000, 0.9659258262890683122, 1.000000000000000000, 0.9659258262890683122, 1.000000000000000000, 0.9659258262890683122, 1.000000000000000000, 0.9659258262890683122, 1.000000000000000000, 0.9659258262890683122, 1.000000000000000000, 0.9659258262890683122, 1.000000000000000000, 0.9659258262890683122, 1.000000000000000000, 0.9659258262890683122, 1.000000000000000000, 0.9659258262890683122, 1.000000000000000000, 0.9659258262890683122, 1.000000000000000000, 0.9659258262890683122, 1.000000000000000000, 0.9659258262890683122, 1.000000000000000000, 0.9659258262890683122, 1.000000000000000000, 0.9659258262890683122, 1.000000000000000000, 0.9659258262890683122, 1.000000000000000000, 0.9659258262890683122, 1.000000000000000000, 0.9659258262890683122, 1.000000000000000000, 0.9659258262890683122, 1.000000000000000000, 0.9659258262890683122, 1.000000000000000000, 0.9659258262890683122, 1.000000000000000000, 0.9659258262890683122, 1.000000000000000000, 0.9659258262890683122, 1.000000000000000000, 0.9659258262890683122, 1.000000000000000000, 0.9659258262890683122, 1.000000000000000000, 0.9659258262890683122, 1.000000000000000000, 0.9659258262890683122, 1.000000000000000000),
 ( 0.3333333333333333703, 0.3219752754296894559, 0.3333333333333333703, 0.3219752754296894559, 0.3333333333333333703, 0.3219752754296894559, 0.3333333333333333703, 0.3219752754296894559, 0.3333333333333333703, 0.3219752754296894559, 0.3333333333333333703, 0.3219752754296894559, 0.3333333333333333703, 0.3219752754296894559, 0.3333333333333333703, 0.3219752754296894559, 0.3333333333333333703, 0.3219752754296894559, 0.3333333333333333703, 0.3219752754296894559, 0.3333333333333333703, 0.3219752754296894559, 0.3333333333333333703, 0.3219752754296894559, 0.3333333333333333703, 0.3219752754296894559, 0.3333333333333333703, 0.3219752754296894559, 0.3333333333333333703, 0.3219752754296894559, 0.3333333333333333703, 0.3219752754296894559, 0.3333333333333333703, 0.3219752754296894559, 0.3333333333333333703, 0.3219752754296894559, 0.3333333333333333703, 0.3219752754296894559, 0.3333333333333333703, 0.3219752754296894559, 0.3333333333333333703, 0.3219752754296894559, 0.3333333333333333703, 0.3219752754296894559, 0.3333333333333333703, 0.3219752754296894559, 0.3333333333333333703, 0.3219752754296894559, 0.3333333333333333703, 0.3219752754296894559, 0.3333333333333333703, 0.3219752754296894559, 0.3333333333333333703, 0.3219752754296894559, 0.3333333333333333703, 0.3219752754296894559, 0.3333333333333333703, 0.3219752754296894559, 0.3333333333333333703, 0.3219752754296894559, 0.3333333333333333703, 0.3219752754296894559, 0.3333333333333333703, 0.3219752754296894559, 0.3333333333333333703, 0.3219752754296894559, 0.3333333333333333703, 0.3219752754296894559, 0.3333333333333333703, 0.3219752754296894559, 0.3333333333333333703, 0.3219752754296894559, 0.3333333333333333703, 0.3219752754296894559, 0.3333333333333333703, 0.3219752754296894559, 0.3333333333333333703, 0.3219752754296894559, 0.3333333333333333703, 0.3219752754296894559, 0.3333333333333333703, 0.3219752754296894559, 0.3333333333333333703, 0.3219752754296894559, 0.3333333333333333703, 0.3219752754296894559, 0.3333333333333333703, 0.3219752754296894559, 0.3333333333333333703, 0.3219752754296894559, 0.3333333333333333703, 0.3219752754296894559, 0.3333333333333333703, 0.3219752754296894559, 0.3333333333333333703, 0.3219752754296894559, 0.3333333333333333703, 0.3219752754296894559, 0.3333333333333333703, 0.3219752754296894559, 0.3333333333333333703, 0.3219752754296894559, 0.3333333333333333703, 0.3219752754296894559, 0.3333333333333333703, 0.3219752754296894559, 0.3333333333333333703, 0.3219752754296894559, 0.3333333333333333703, 0.3219752754296894559, 0.3333333333333333703, 0.3219752754296894559, 0.3333333333333333703, 0.3219752754296894559, 0.3333333333333333703, 0.3219752754296894559, 0.3333333333333333703, 0.3219752754296894559, 0.3333333333333333703, 0.3219752754296894559, 0.3333333333333333703, 0.3219752754296894559, 0.3333333333333333703, 0.3219752754296894559, 0.3333333333333333703, 0.3219752754296894559, 0.3333333333333333703, 0.3219752754296894559, 0.3333333333333333703, 0.3219752754296894559, 0.3333333333333333703, 0.3219752754296894559, 0.3333333333333333703, 0.3219752754296894559, 0.3333333333333333703, 0.3219752754296894559, 0.3333333333333333703, 0.3219752754296894559, 0.3333333333333333703, 0.3219752754296894559, 0.3333333333333333703, 0.3219752754296894559, 0.3333333333333333703, 0.3219752754296894559, 0.3333333333333333703, 0.3219752754296894559, 0.3333333333333333703, 0.3219752754296894559, 0.3333333333333333703, 0.3219752754296894559, 0.3333333333333333703, 0.3219752754296894559, 0.3333333333333333703, 0.3219752754296894559, 0.3333333333333333703, 0.3219752754296894559, 0.3333333333333333703, 0.3219752754296894559, 0.3333333333333333703, 0.3219752754296894559, 0.3333333333333333703, 0.3219752754296894559, 0.3333333333333333703, 0.3219752754296894559, 0.3333333333333333703, 0.3219752754296894559, 0.3333333333333333703, 0.3219752754296894559, 0.3333333333333333703, 0.3219752754296894559, 0.3333333333333333703, 0.3219752754296894559, 0.3333333333333333703, 0.3219752754296894559, 0.3333333333333333703, 0.3219752754296894559, 0.3333333333333333703, 0.3219752754296894559, 0.3333333333333333703, 0.3219752754296894559, 0.3333333333333333703, 0.3219752754296894559, 0.3333333333333333703, 0.3219752754296894559, 0.3333333333333333703, 0.3219752754296894559, 0.3333333333333333703, 0.3219752754296894559, 0.3333333333333333703, 0.3219752754296894559, 0.3333333333333333703, 0.3219752754296894559, 0.3333333333333333703, 0.3219752754296894559, 0.3333333333333333703, 0.3219752754296894559, 0.3333333333333333703, 0.3219752754296894559, 0.3333333333333333703, 0.3219752754296894559, 0.3333333333333333703, 0.3219752754296894559, 0.3333333333333333703, 0.3219752754296894559, 0.3333333333333333703, 0.3219752754296894559, 0.3333333333333333703, 0.3219752754296894559, 0.3333333333333333703, 0.3219752754296894559, 0.3333333333333333703, 0.3219752754296894559, 0.3333333333333333703, 0.3219752754296894559, 0.3333333333333333703, 0.3219752754296894559, 0.3333333333333333703, 0.3219752754296894559, 0.3333333333333333703, 0.3219752754296894559, 0.3333333333333333703, 0.3219752754296894559, 0.3333333333333333703, 0.3219752754296894559, 0.3333333333333333703, 0.3219752754296894559, 0.3333333333333333703, 0.3219752754296894559, 0.3333333333333333703, 0.3219752754296894559, 0.3333333333333333703, 0.3219752754296894559, 0.3333333333333333703, 0.3219752754296894559, 0.3333333333333333703, 0.3219752754296894559, 0.3333333333333333703, 0.3219752754296894559, 0.3333333333333333703, 0.3219752754296894559, 0.3333333333333333703, 0.3219752754296894559, 0.3333333333333333703, 0.3219752754296894559, 0.3333333333333333703, 0.3219752754296894559, 0.3333333333333333703, 0.3219752754296894559, 0.3333333333333333703, 0.3219752754296894559, 0.3333333333333333703, 0.3219752754296894559, 0.3333333333333333703, 0.3219752754296894559, 0.3333333333333333703, 0.3219752754296894559, 0.3333333333333333703, 0.3219752754296894559, 0.3333333333333333703, 0.3219752754296894559, 0.3333333333333333703, 0.3219752754296894559, 0.3333333333333333703, 0.3219752754296894559, 0.3333333333333333703, 0.3219752754296894559, 0.3333333333333333703, 0.3219752754296894559, 0.3333333333333333703, 0.3219752754296894559, 0.3333333333333333703, 0.3219752754296894559, 0.3333333333333333703, 0.3219752754296894559, 0.3333333333333333703, 0.3219752754296894559, 0.3333333333333333703, 0.3219752754296894559, 0.3333333333333333703, 0.3219752754296894559, 0.3333333333333333703, 0.3219752754296894559, 0.3333333333333333703, 0.3219752754296894559, 0.3333333333333333703, 0.3219752754296894559, 0.3333333333333333703, 0.3219752754296894559, 0.3333333333333333703, 0.3219752754296894559, 0.3333333333333333703, 0.3219752754296894559, 0.3333333333333333703, 0.3219752754296894559, 0.3333333333333333703, 0.3219752754296894559, 0.3333333333333333703, 0.3219752754296894559, 0.3333333333333333703, 0.3219752754296894559, 0.3333333333333333703, 0.3219752754296894559, 0.3333333333333333703, 0.3219752754296894559, 0.3333333333333333703, 0.3219752754296894559, 0.3333333333333333703, 0.3219752754296894559, 0.3333333333333333703, 0.3219752754296894559, 0.3333333333333333703, 0.3219752754296894559, 0.3333333333333333703, 0.3219752754296894559, 0.3333333333333333703, 0.3219752754296894559, 0.3333333333333333703, 0.3219752754296894559, 0.3333333333333333703, 0.3219752754296894559, 0.3333333333333333703, 0.3219752754296894559, 0.3333333333333333703, 0.3219752754296894559, 0.3333333333333333703, 0.3219752754296894559, 0.3333333333333333703, 0.3219752754296894559, 0.3333333333333333703, 0.3219752754296894559, 0.3333333333333333703, 0.3219752754296894559, 0.3333333333333333703, 0.3219752754296894559, 0.3333333333333333703, 0.3219752754296894559, 0.3333333333333333703, 0.3219752754296894559, 0.3333333333333333703, 0.3219752754296894559, 0.3333333333333333703, 0.3219752754296894559, 0.3333333333333333703, 0.3219752754296894559, 0.3333333333333333703, 0.3219752754296894559, 0.3333333333333333703, 0.3219752754296894559, 0.3333333333333333703, 0.3219752754296894559, 0.3333333333333333703, 0.3219752754296894559, 0.3333333333333333703, 0.3219752754296894559, 0.3333333333333333703, 0.3219752754296894559, 0.3333333333333333703, 0.3219752754296894559, 0.3333333333333333703, 0.3219752754296894559, 0.3333333333333333703, 0.3219752754296894559, 0.3333333333333333703, 0.3219752754296894559, 0.3333333333333333703, 0.3219752754296894559, 0.3333333333333333703, 0.3219752754296894559, 0.3333333333333333703, 0.3219752754296894559, 0.3333333333333333703, 0.3219752754296894559, 0.3333333333333333703, 0.3219752754296894559, 0.3333333333333333703, 0.3219752754296894559, 0.3333333333333333703, 0.3219752754296894559, 0.3333333333333333703, 0.3219752754296894559, 0.3333333333333333703, 0.3219752754296894559, 0.3333333333333333703, 0.3219752754296894559, 0.3333333333333333703, 0.3219752754296894559, 0.3333333333333333703, 0.3219752754296894559, 0.3333333333333333703, 0.3219752754296894559, 0.3333333333333333703, 0.3219752754296894559, 0.3333333333333333703, 0.3219752754296894559, 0.3333333333333333703, 0.3219752754296894559, 0.3333333333333333703, 0.3219752754296894559, 0.3333333333333333703, 0.3219752754296894559, 0.3333333333333333703, 0.3219752754296894559, 0.3333333333333333703, 0.3219752754296894559, 0.3333333333333333703, 0.3219752754296894559, 0.3333333333333333703, 0.3219752754296894559, 0.3333333333333333703, 0.3219752754296894559, 0.3333333333333333703, 0.3219752754296894559, 0.3333333333333333703, 0.3219752754296894559, 0.3333333333333333703, 0.3219752754296894559, 0.3333333333333333703, 0.3219752754296894559, 0.3333333333333333703, 0.3219752754296894559, 0.3333333333333333703, 0.3219752754296894559, 0.3333333333333333703, 0.3219752754296894559, 0.3333333333333333703, 0.3219752754296894559, 0.3333333333333333703, 0.3219752754296894559, 0.3333333333333333703, 0.3219752754296894559, 0.3333333333333333703, 0.3219752754296894559, 0.3333333333333333703, 0.3219752754296894559, 0.3333333333333333703, 0.3219752754296894559, 0.3333333333333333703, 0.3219752754296894559, 0.3333333333333333703, 0.3219752754296894559, 0.3333333333333333703, 0.3219752754296894559, 0.3333333333333333703, 0.3219752754296894559, 0.3333333333333333703, 0.3219752754296894559, 0.3333333333333333703, 0.3219752754296894559, 0.3333333333333333703, 0.3219752754296894559, 0.3333333333333333703, 0.3219752754296894559, 0.3333333333333333703, 0.3219752754296894559, 0.3333333333333333703, 0.3219752754296894559, 0.3333333333333333703),
 ( 0.3333333333333333703, 0.3219752754296894559, 0.3333333333333333703, 0.3219752754296894559, 0.3333333333333333703, 0.3219752754296894559, 0.3333333333333333703, 0.3219752754296894559, 0.3333333333333333703, 0.3219752754296894559, 0.3333333333333333703, 0.3219752754296894559, 0.3333333333333333703, 0.3219752754296894559, 0.3333333333333333703, 0.3219752754296894559, 0.3333333333333333703, 0.3219752754296894559, 0.3333333333333333703, 0.3219752754296894559, 0.3333333333333333703, 0.3219752754296894559, 0.3333333333333333703, 0.3219752754296894559, 0.3333333333333333703, 0.3219752754296894559, 0.3333333333333333703, 0.3219752754296894559, 0.3333333333333333703, 0.3219752754296894559, 0.3333333333333333703, 0.3219752754296894559, 0.3333333333333333703, 0.3219752754296894559, 0.3333333333333333703, 0.3219752754296894559, 0.3333333333333333703, 0.3219752754296894559, 0.3333333333333333703, 0.3219752754296894559, 0.3333333333333333703, 0.3219752754296894559, 0.3333333333333333703, 0.3219752754296894559, 0.3333333333333333703, 0.3219752754296894559, 0.3333333333333333703, 0.3219752754296894559, 0.3333333333333333703, 0.3219752754296894559, 0.3333333333333333703, 0.3219752754296894559, 0.3333333333333333703, 0.3219752754296894559, 0.3333333333333333703, 0.3219752754296894559, 0.3333333333333333703, 0.3219752754296894559, 0.3333333333333333703, 0.3219752754296894559, 0.3333333333333333703, 0.3219752754296894559, 0.3333333333333333703, 0.3219752754296894559, 0.3333333333333333703, 0.3219752754296894559, 0.3333333333333333703, 0.3219752754296894559, 0.3333333333333333703, 0.3219752754296894559, 0.3333333333333333703, 0.3219752754296894559, 0.3333333333333333703, 0.3219752754296894559, 0.3333333333333333703, 0.3219752754296894559, 0.3333333333333333703, 0.3219752754296894559, 0.3333333333333333703, 0.3219752754296894559, 0.3333333333333333703, 0.3219752754296894559, 0.3333333333333333703, 0.3219752754296894559, 0.3333333333333333703, 0.3219752754296894559, 0.3333333333333333703, 0.3219752754296894559, 0.3333333333333333703, 0.3219752754296894559, 0.3333333333333333703, 0.3219752754296894559, 0.3333333333333333703, 0.3219752754296894559, 0.3333333333333333703, 0.3219752754296894559, 0.3333333333333333703, 0.3219752754296894559, 0.3333333333333333703, 0.3219752754296894559, 0.3333333333333333703, 0.3219752754296894559, 0.3333333333333333703, 0.3219752754296894559, 0.3333333333333333703, 0.3219752754296894559, 0.3333333333333333703, 0.3219752754296894559, 0.3333333333333333703, 0.3219752754296894559, 0.3333333333333333703, 0.3219752754296894559, 0.3333333333333333703, 0.3219752754296894559, 0.3333333333333333703, 0.3219752754296894559, 0.3333333333333333703, 0.3219752754296894559, 0.3333333333333333703, 0.3219752754296894559, 0.3333333333333333703, 0.3219752754296894559, 0.3333333333333333703, 0.3219752754296894559, 0.3333333333333333703, 0.3219752754296894559, 0.3333333333333333703, 0.3219752754296894559, 0.3333333333333333703, 0.3219752754296894559, 0.3333333333333333703, 0.3219752754296894559, 0.3333333333333333703, 0.3219752754296894559, 0.3333333333333333703, 0.3219752754296894559, 0.3333333333333333703, 0.3219752754296894559, 0.3333333333333333703, 0.3219752754296894559, 0.3333333333333333703, 0.3219752754296894559, 0.3333333333333333703, 0.3219752754296894559, 0.3333333333333333703, 0.3219752754296894559, 0.3333333333333333703, 0.3219752754296894559, 0.3333333333333333703, 0.3219752754296894559, 0.3333333333333333703, 0.3219752754296894559, 0.3333333333333333703, 0.3219752754296894559, 0.3333333333333333703, 0.3219752754296894559, 0.3333333333333333703, 0.3219752754296894559, 0.3333333333333333703, 0.3219752754296894559, 0.3333333333333333703, 0.3219752754296894559, 0.3333333333333333703, 0.3219752754296894559, 0.3333333333333333703, 0.3219752754296894559, 0.3333333333333333703, 0.3219752754296894559, 0.3333333333333333703, 0.3219752754296894559, 0.3333333333333333703, 0.3219752754296894559, 0.3333333333333333703, 0.3219752754296894559, 0.3333333333333333703, 0.3219752754296894559, 0.3333333333333333703, 0.3219752754296894559, 0.3333333333333333703, 0.3219752754296894559, 0.3333333333333333703, 0.3219752754296894559, 0.3333333333333333703, 0.3219752754296894559, 0.3333333333333333703, 0.3219752754296894559, 0.3333333333333333703, 0.3219752754296894559, 0.3333333333333333703, 0.3219752754296894559, 0.3333333333333333703, 0.3219752754296894559, 0.3333333333333333703, 0.3219752754296894559, 0.3333333333333333703, 0.3219752754296894559, 0.3333333333333333703, 0.3219752754296894559, 0.3333333333333333703, 0.3219752754296894559, 0.3333333333333333703, 0.3219752754296894559, 0.3333333333333333703, 0.3219752754296894559, 0.3333333333333333703, 0.3219752754296894559, 0.3333333333333333703, 0.3219752754296894559, 0.3333333333333333703, 0.3219752754296894559, 0.3333333333333333703, 0.3219752754296894559, 0.3333333333333333703, 0.3219752754296894559, 0.3333333333333333703, 0.3219752754296894559, 0.3333333333333333703, 0.3219752754296894559, 0.3333333333333333703, 0.3219752754296894559, 0.3333333333333333703, 0.3219752754296894559, 0.3333333333333333703, 0.3219752754296894559, 0.3333333333333333703, 0.3219752754296894559, 0.3333333333333333703, 0.3219752754296894559, 0.3333333333333333703, 0.3219752754296894559, 0.3333333333333333703, 0.3219752754296894559, 0.3333333333333333703, 0.3219752754296894559, 0.3333333333333333703, 0.3219752754296894559, 0.3333333333333333703, 0.3219752754296894559, 0.3333333333333333703, 0.3219752754296894559, 0.3333333333333333703, 0.3219752754296894559, 0.3333333333333333703, 0.3219752754296894559, 0.3333333333333333703, 0.3219752754296894559, 0.3333333333333333703, 0.3219752754296894559, 0.3333333333333333703, 0.3219752754296894559, 0.3333333333333333703, 0.3219752754296894559, 0.3333333333333333703, 0.3219752754296894559, 0.3333333333333333703, 0.3219752754296894559, 0.3333333333333333703, 0.3219752754296894559, 0.3333333333333333703, 0.3219752754296894559, 0.3333333333333333703, 0.3219752754296894559, 0.3333333333333333703, 0.3219752754296894559, 0.3333333333333333703, 0.3219752754296894559, 0.3333333333333333703, 0.3219752754296894559, 0.3333333333333333703, 0.3219752754296894559, 0.3333333333333333703, 0.3219752754296894559, 0.3333333333333333703, 0.3219752754296894559, 0.3333333333333333703, 0.3219752754296894559, 0.3333333333333333703, 0.3219752754296894559, 0.3333333333333333703, 0.3219752754296894559, 0.3333333333333333703, 0.3219752754296894559, 0.3333333333333333703, 0.3219752754296894559, 0.3333333333333333703, 0.3219752754296894559, 0.3333333333333333703, 0.3219752754296894559, 0.3333333333333333703, 0.3219752754296894559, 0.3333333333333333703, 0.3219752754296894559, 0.3333333333333333703, 0.3219752754296894559, 0.3333333333333333703, 0.3219752754296894559, 0.3333333333333333703, 0.3219752754296894559, 0.3333333333333333703, 0.3219752754296894559, 0.3333333333333333703, 0.3219752754296894559, 0.3333333333333333703, 0.3219752754296894559, 0.3333333333333333703, 0.3219752754296894559, 0.3333333333333333703, 0.3219752754296894559, 0.3333333333333333703, 0.3219752754296894559, 0.3333333333333333703, 0.3219752754296894559, 0.3333333333333333703, 0.3219752754296894559, 0.3333333333333333703, 0.3219752754296894559, 0.3333333333333333703, 0.3219752754296894559, 0.3333333333333333703, 0.3219752754296894559, 0.3333333333333333703, 0.3219752754296894559, 0.3333333333333333703, 0.3219752754296894559, 0.3333333333333333703, 0.3219752754296894559, 0.3333333333333333703, 0.3219752754296894559, 0.3333333333333333703, 0.3219752754296894559, 0.3333333333333333703, 0.3219752754296894559, 0.3333333333333333703, 0.3219752754296894559, 0.3333333333333333703, 0.3219752754296894559, 0.3333333333333333703, 0.3219752754296894559, 0.3333333333333333703, 0.3219752754296894559, 0.3333333333333333703, 0.3219752754296894559, 0.3333333333333333703, 0.3219752754296894559, 0.3333333333333333703, 0.3219752754296894559, 0.3333333333333333703, 0.3219752754296894559, 0.3333333333333333703, 0.3219752754296894559, 0.3333333333333333703, 0.3219752754296894559, 0.3333333333333333703, 0.3219752754296894559, 0.3333333333333333703, 0.3219752754296894559, 0.3333333333333333703, 0.3219752754296894559, 0.3333333333333333703, 0.3219752754296894559, 0.3333333333333333703, 0.3219752754296894559, 0.3333333333333333703, 0.3219752754296894559, 0.3333333333333333703, 0.3219752754296894559, 0.3333333333333333703, 0.3219752754296894559, 0.3333333333333333703, 0.3219752754296894559, 0.3333333333333333703, 0.3219752754296894559, 0.3333333333333333703, 0.3219752754296894559, 0.3333333333333333703, 0.3219752754296894559, 0.3333333333333333703, 0.3219752754296894559, 0.3333333333333333703, 0.3219752754296894559, 0.3333333333333333703, 0.3219752754296894559, 0.3333333333333333703, 0.3219752754296894559, 0.3333333333333333703, 0.3219752754296894559, 0.3333333333333333703, 0.3219752754296894559, 0.3333333333333333703, 0.3219752754296894559, 0.3333333333333333703, 0.3219752754296894559, 0.3333333333333333703, 0.3219752754296894559, 0.3333333333333333703, 0.3219752754296894559, 0.3333333333333333703, 0.3219752754296894559, 0.3333333333333333703, 0.3219752754296894559, 0.3333333333333333703, 0.3219752754296894559, 0.3333333333333333703, 0.3219752754296894559, 0.3333333333333333703, 0.3219752754296894559, 0.3333333333333333703, 0.3219752754296894559, 0.3333333333333333703, 0.3219752754296894559, 0.3333333333333333703, 0.3219752754296894559, 0.3333333333333333703, 0.3219752754296894559, 0.3333333333333333703, 0.3219752754296894559, 0.3333333333333333703, 0.3219752754296894559, 0.3333333333333333703, 0.3219752754296894559, 0.3333333333333333703, 0.3219752754296894559, 0.3333333333333333703, 0.3219752754296894559, 0.3333333333333333703, 0.3219752754296894559, 0.3333333333333333703, 0.3219752754296894559, 0.3333333333333333703, 0.3219752754296894559, 0.3333333333333333703, 0.3219752754296894559, 0.3333333333333333703, 0.3219752754296894559, 0.3333333333333333703, 0.3219752754296894559, 0.3333333333333333703, 0.3219752754296894559, 0.3333333333333333703, 0.3219752754296894559, 0.3333333333333333703, 0.3219752754296894559, 0.3333333333333333703, 0.3219752754296894559, 0.3333333333333333703, 0.3219752754296894559, 0.3333333333333333703, 0.3219752754296894559, 0.3333333333333333703, 0.3219752754296894559, 0.3333333333333333703, 0.3219752754296894559, 0.3333333333333333703, 0.3219752754296894559, 0.3333333333333333703, 0.3219752754296894559, 0.3333333333333333703),
 ( 1.000000000000000000, 0.9659258262890683122, 1.000000000000000000, 0.9659258262890683122, 1.000000000000000000, 0.9659258262890683122, 1.000000000000000000, 0.9659258262890683122, 1.000000000000000000, 0.9659258262890683122, 1.000000000000000000, 0.9659258262890683122, 1.000000000000000000, 0.9659258262890683122, 1.000000000000000000, 0.9659258262890683122, 1.000000000000000000, 0.9659258262890683122, 1.000000000000000000, 0.9659258262890683122, 1.000000000000000000, 0.9659258262890683122, 1.000000000000000000, 0.9659258262890683122, 1.000000000000000000, 0.9659258262890683122, 1.000000000000000000, 0.9659258262890683122, 1.000000000000000000, 0.9659258262890683122, 1.000000000000000000, 0.9659258262890683122, 1.000000000000000000, 0.9659258262890683122, 1.000000000000000000, 0.9659258262890683122, 1.000000000000000000, 0.9659258262890683122, 1.000000000000000000, 0.9659258262890683122, 1.000000000000000000, 0.9659258262890683122, 1.000000000000000000, 0.9659258262890683122, 1.000000000000000000, 0.9659258262890683122, 1.000000000000000000, 0.9659258262890683122, 1.000000000000000000, 0.9659258262890683122, 1.000000000000000000, 0.9659258262890683122, 1.000000000000000000, 0.9659258262890683122, 1.000000000000000000, 0.9659258262890683122, 1.000000000000000000, 0.9659258262890683122, 1.000000000000000000, 0.9659258262890683122, 1.000000000000000000, 0.9659258262890683122, 1.000000000000000000, 0.9659258262890683122, 1.000000000000000000, 0.9659258262890683122, 1.000000000000000000, 0.9659258262890683122, 1.000000000000000000, 0.9659258262890683122, 1.000000000000000000, 0.9659258262890683122, 1.000000000000000000, 0.9659258262890683122, 1.000000000000000000, 0.9659258262890683122, 1.000000000000000000, 0.9659258262890683122, 1.000000000000000000, 0.9659258262890683122, 1.000000000000000000, 0.9659258262890683122, 1.000000000000000000, 0.9659258262890683122, 1.000000000000000000, 0.9659258262890683122, 1.000000000000000000, 0.9659258262890683122, 1.000000000000000000, 0.9659258262890683122, 1.000000000000000000, 0.9659258262890683122, 1.000000000000000000, 0.9659258262890683122, 1.000000000000000000, 0.9659258262890683122, 1.000000000000000000, 0.9659258262890683122, 1.000000000000000000, 0.9659258262890683122, 1.000000000000000000, 0.9659258262890683122, 1.000000000000000000, 0.9659258262890683122, 1.000000000000000000, 0.9659258262890683122, 1.000000000000000000, 0.9659258262890683122, 1.000000000000000000, 0.9659258262890683122, 1.000000000000000000, 0.9659258262890683122, 1.000000000000000000, 0.9659258262890683122, 1.000000000000000000, 0.9659258262890683122, 1.000000000000000000, 0.9659258262890683122, 1.000000000000000000, 0.9659258262890683122, 1.000000000000000000, 0.9659258262890683122, 1.000000000000000000, 0.9659258262890683122, 1.000000000000000000, 0.9659258262890683122, 1.000000000000000000, 0.9659258262890683122, 1.000000000000000000, 0.9659258262890683122, 1.000000000000000000, 0.9659258262890683122, 1.000000000000000000, 0.9659258262890683122, 1.000000000000000000, 0.9659258262890683122, 1.000000000000000000, 0.9659258262890683122, 1.000000000000000000, 0.9659258262890683122, 1.000000000000000000, 0.9659258262890683122, 1.000000000000000000, 0.9659258262890683122, 1.000000000000000000, 0.9659258262890683122, 1.000000000000000000, 0.9659258262890683122, 1.000000000000000000, 0.9659258262890683122, 1.000000000000000000, 0.9659258262890683122, 1.000000000000000000, 0.9659258262890683122, 1.000000000000000000, 0.9659258262890683122, 1.000000000000000000, 0.9659258262890683122, 1.000000000000000000, 0.9659258262890683122, 1.000000000000000000, 0.9659258262890683122, 1.000000000000000000, 0.9659258262890683122, 1.000000000000000000, 0.9659258262890683122, 1.000000000000000000, 0.9659258262890683122, 1.000000000000000000, 0.9659258262890683122, 1.000000000000000000, 0.9659258262890683122, 1.000000000000000000, 0.9659258262890683122, 1.000000000000000000, 0.9659258262890683122, 1.000000000000000000, 0.9659258262890683122, 1.000000000000000000, 0.9659258262890683122, 1.000000000000000000, 0.9659258262890683122, 1.000000000000000000, 0.9659258262890683122, 1.000000000000000000, 0.9659258262890683122, 1.000000000000000000, 0.9659258262890683122, 1.000000000000000000, 0.9659258262890683122, 1.000000000000000000, 0.9659258262890683122, 1.000000000000000000, 0.9659258262890683122, 1.000000000000000000, 0.9659258262890683122, 1.000000000000000000, 0.9659258262890683122, 1.000000000000000000, 0.9659258262890683122, 1.000000000000000000, 0.9659258262890683122, 1.000000000000000000, 0.9659258262890683122, 1.000000000000000000, 0.9659258262890683122, 1.000000000000000000, 0.9659258262890683122, 1.000000000000000000, 0.9659258262890683122, 1.000000000000000000, 0.9659258262890683122, 1.000000000000000000, 0.9659258262890683122, 1.000000000000000000, 0.9659258262890683122, 1.000000000000000000, 0.9659258262890683122, 1.000000000000000000, 0.9659258262890683122, 1.000000000000000000, 0.9659258262890683122, 1.000000000000000000, 0.9659258262890683122, 1.000000000000000000, 0.9659258262890683122, 1.000000000000000000, 0.9659258262890683122, 1.000000000000000000, 0.9659258262890683122, 1.000000000000000000, 0.9659258262890683122, 1.000000000000000000, 0.9659258262890683122, 1.000000000000000000, 0.9659258262890683122, 1.000000000000000000, 0.9659258262890683122, 1.000000000000000000, 0.9659258262890683122, 1.000000000000000000, 0.9659258262890683122, 1.000000000000000000, 0.9659258262890683122, 1.000000000000000000, 0.9659258262890683122, 1.000000000000000000, 0.9659258262890683122, 1.000000000000000000, 0.9659258262890683122, 1.000000000000000000, 0.9659258262890683122, 1.000000000000000000, 0.9659258262890683122, 1.000000000000000000, 0.9659258262890683122, 1.000000000000000000, 0.9659258262890683122, 1.000000000000000000, 0.9659258262890683122, 1.000000000000000000, 0.9659258262890683122, 1.000000000000000000, 0.9659258262890683122, 1.000000000000000000, 0.9659258262890683122, 1.000000000000000000, 0.9659258262890683122, 1.000000000000000000, 0.9659258262890683122, 1.000000000000000000, 0.9659258262890683122, 1.000000000000000000, 0.9659258262890683122, 1.000000000000000000, 0.9659258262890683122, 1.000000000000000000, 0.9659258262890683122, 1.000000000000000000, 0.9659258262890683122, 1.000000000000000000, 0.9659258262890683122, 1.000000000000000000, 0.9659258262890683122, 1.000000000000000000, 0.9659258262890683122, 1.000000000000000000, 0.9659258262890683122, 1.000000000000000000, 0.9659258262890683122, 1.000000000000000000, 0.9659258262890683122, 1.000000000000000000, 0.9659258262890683122, 1.000000000000000000, 0.9659258262890683122, 1.000000000000000000, 0.9659258262890683122, 1.000000000000000000, 0.9659258262890683122, 1.000000000000000000, 0.9659258262890683122, 1.000000000000000000, 0.9659258262890683122, 1.000000000000000000, 0.9659258262890683122, 1.000000000000000000, 0.9659258262890683122, 1.000000000000000000, 0.9659258262890683122, 1.000000000000000000, 0.9659258262890683122, 1.000000000000000000, 0.9659258262890683122, 1.000000000000000000, 0.9659258262890683122, 1.000000000000000000, 0.9659258262890683122, 1.000000000000000000, 0.9659258262890683122, 1.000000000000000000, 0.9659258262890683122, 1.000000000000000000, 0.9659258262890683122, 1.000000000000000000, 0.9659258262890683122, 1.000000000000000000, 0.9659258262890683122, 1.000000000000000000, 0.9659258262890683122, 1.000000000000000000, 0.9659258262890683122, 1.000000000000000000, 0.9659258262890683122, 1.000000000000000000, 0.9659258262890683122, 1.000000000000000000, 0.9659258262890683122, 1.000000000000000000, 0.9659258262890683122, 1.000000000000000000, 0.9659258262890683122, 1.000000000000000000, 0.9659258262890683122, 1.000000000000000000, 0.9659258262890683122, 1.000000000000000000, 0.9659258262890683122, 1.000000000000000000, 0.9659258262890683122, 1.000000000000000000, 0.9659258262890683122, 1.000000000000000000, 0.9659258262890683122, 1.000000000000000000, 0.9659258262890683122, 1.000000000000000000, 0.9659258262890683122, 1.000000000000000000, 0.9659258262890683122, 1.000000000000000000, 0.9659258262890683122, 1.000000000000000000, 0.9659258262890683122, 1.000000000000000000, 0.9659258262890683122, 1.000000000000000000, 0.9659258262890683122, 1.000000000000000000, 0.9659258262890683122, 1.000000000000000000, 0.9659258262890683122, 1.000000000000000000, 0.9659258262890683122, 1.000000000000000000, 0.9659258262890683122, 1.000000000000000000, 0.9659258262890683122, 1.000000000000000000, 0.9659258262890683122, 1.000000000000000000, 0.9659258262890683122, 1.000000000000000000, 0.9659258262890683122, 1.000000000000000000, 0.9659258262890683122, 1.000000000000000000, 0.9659258262890683122, 1.000000000000000000, 0.9659258262890683122, 1.000000000000000000, 0.9659258262890683122, 1.000000000000000000, 0.9659258262890683122, 1.000000000000000000, 0.9659258262890683122, 1.000000000000000000, 0.9659258262890683122, 1.000000000000000000, 0.9659258262890683122, 1.000000000000000000, 0.9659258262890683122, 1.000000000000000000, 0.9659258262890683122, 1.000000000000000000, 0.9659258262890683122, 1.000000000000000000, 0.9659258262890683122, 1.000000000000000000, 0.9659258262890683122, 1.000000000000000000, 0.9659258262890683122, 1.000000000000000000, 0.9659258262890683122, 1.000000000000000000, 0.9659258262890683122, 1.000000000000000000, 0.9659258262890683122, 1.000000000000000000, 0.9659258262890683122, 1.000000000000000000, 0.9659258262890683122, 1.000000000000000000, 0.9659258262890683122, 1.000000000000000000, 0.9659258262890683122, 1.000000000000000000, 0.9659258262890683122, 1.000000000000000000, 0.9659258262890683122, 1.000000000000000000, 0.9659258262890683122, 1.000000000000000000, 0.9659258262890683122, 1.000000000000000000, 0.9659258262890683122, 1.000000000000000000, 0.9659258262890683122, 1.000000000000000000, 0.9659258262890683122, 1.000000000000000000, 0.9659258262890683122, 1.000000000000000000, 0.9659258262890683122, 1.000000000000000000, 0.9659258262890683122, 1.000000000000000000, 0.9659258262890683122, 1.000000000000000000, 0.9659258262890683122, 1.000000000000000000, 0.9659258262890683122, 1.000000000000000000, 0.9659258262890683122, 1.000000000000000000, 0.9659258262890683122, 1.000000000000000000) ) ) 
 REPRESENTATION_ITEM ( '' )  SURFACE ( )  );
#102256=CARTESIAN_POINT ( 'NONE',  ( -21.53943276465977519, -0.05219959533937600094, 18.75109039468568639 ) ) ;
#102258=CARTESIAN_POINT ( 'NONE',  ( 21.55341960407610458, 5.719274019375980345, 63.95724293864770260 ) ) ;
#102259=CARTESIAN_POINT ( 'NONE',  ( -16.55341960407617563, 4.379528057220093196, 98.54275706135234714 ) ) ;
#102260=CARTESIAN_POINT ( 'NONE',  ( -12.06949235617756955, 12.14591786802309770, 115.6239096053143669 ) ) ;
#102261=CARTESIAN_POINT ( 'NONE',  ( -16.46253265017160317, 9.564922557960807481, 70.83224293864770971 ) ) ;
#102263=CARTESIAN_POINT ( 'NONE',  ( 8.314922557960818139, 14.29746914071049879, 29.58224293864769905 ) ) ;
#102264=CARTESIAN_POINT ( 'NONE',  ( 18.67979575497194134, -10.72451020669871369, 60.83442372801901854 ) ) ;
#102265=CARTESIAN_POINT ( 'NONE',  ( 19.03943276465977164, -0.05219959533909143690, 108.7489096053143527 ) ) ;
#102266=CARTESIAN_POINT ( 'NONE',  ( 15.72974639402176855, 15.80617190586768217, 96.87609039468568994 ) ) ;
#102267=CARTESIAN_POINT ( 'NONE',  ( -16.51473224551069308, -9.474510206698971260, 36.66557627198102409 ) ) ;
#102268=CARTESIAN_POINT ( 'NONE',  ( 16.46253265017160672, -9.564922557960803928, 33.33224293864770260 ) ) ;
#102270=CARTESIAN_POINT ( 'NONE',  ( -0.05219959533937732626, 21.53943276465977519, 97.50109039468567573 ) ) ;
#102271=CARTESIAN_POINT ( 'NONE',  ( 0.05219959533934541429, -16.53943276465976808, 55.00109039468568284 ) ) ;
#102272=CARTESIAN_POINT ( 'NONE',  ( -18.62759615963255300, -10.81492255796106328, 84.16775706135234714 ) ) ;
#102273=CARTESIAN_POINT ( 'NONE',  ( 16.46253265017160672, -9.564922557960803928, 113.3322429386476955 ) ) ;
#102274=CARTESIAN_POINT ( 'NONE',  ( -13.89961937509957401, -13.97604488694547875, 89.37609039468563310 ) ) ;
#102275=CARTESIAN_POINT ( 'NONE',  ( 5.719274019375673035, 21.55341960407619339, 62.29275706135236845 ) ) ;
#102276=CARTESIAN_POINT ( 'NONE',  ( -13.97604488694547697, 13.89961937509957934, 113.1260903946856757 ) ) ;
#102277=CARTESIAN_POINT ( 'NONE',  ( 5.049401038297881783, 19.05341960407617563, 87.29275706135234714 ) ) ;
#102278=CARTESIAN_POINT ( 'NONE',  ( 19.02544592524343514, -5.153800228976328945, 53.54057627198102409 ) ) ;
#102279=CARTESIAN_POINT ( 'NONE',  ( 19.05341960407617918, -5.049401038297876454, 96.04275706135231871 ) ) ;
#102280=CARTESIAN_POINT ( 'NONE',  ( 16.51473224551083163, -9.474510206698727899, 85.83442372801900433 ) ) ;
#102281=CARTESIAN_POINT ( 'NONE',  ( 14.34966873604960469, 8.224510206698951720, 59.16557627198103120 ) ) ;
#102282=CARTESIAN_POINT ( 'NONE',  ( -13.97604488694547697, 13.89961937509957934, 78.12609039468567573 ) ) ;
#102283=CARTESIAN_POINT ( 'NONE',  ( 16.52544592524335698, 4.483927247898782831, 61.45942372801901854 ) ) ;
#102284=CARTESIAN_POINT ( 'NONE',  ( 19.02544592524334988, 5.153800228976608722, 21.45942372801899012 ) ) ;
#102285=CARTESIAN_POINT ( 'NONE',  ( 5.049401038298161559, -19.05341960407611168, 32.70724293864768129 ) ) ;
#102286=CARTESIAN_POINT ( 'NONE',  ( 13.89961937509977652, -13.97604488694527269, 43.12390960531434558 ) ) ;
#102287=CARTESIAN_POINT ( 'NONE',  ( 8.314922557961029526, -14.29746914071037800, 65.41775706135234714 ) ) ;
#102290=CARTESIAN_POINT ( 'NONE',  ( -19.03943276465977164, 0.05219959533909376836, 106.2489096053143669 ) ) ;
#102291=DIRECTION ( 'NONE',  ( 0.000000000000000000, 0.000000000000000000, -1.000000000000000000 ) ) ;
#102293=CARTESIAN_POINT ( 'NONE',  ( 19.02544592524334988, 5.153800228976608722, 91.45942372801900433 ) ) ;
#102294=CARTESIAN_POINT ( 'NONE',  ( 21.52544592524344225, -5.823673210054117533, 38.54057627198103120 ) ) ;
#102295=CARTESIAN_POINT ( 'NONE',  ( -19.03943276465977164, -0.05219959533935918106, 28.75109039468566507 ) ) ;
#102296=CARTESIAN_POINT ( 'NONE',  ( 13.97604488694548053, -13.89961937509957401, 110.6260903946856615 ) ) ;
#102297=CARTESIAN_POINT ( 'NONE',  ( 19.05341960407611168, 5.049401038298154454, 28.95724293864769550 ) ) ;
#102298=CARTESIAN_POINT ( 'NONE',  ( -13.89961937509977652, 13.97604488694528158, 35.62390960531435269 ) ) ;
#102299=CARTESIAN_POINT ( 'NONE',  ( -18.67979575497178146, -10.72451020669898902, 76.66557627198103830 ) ) ;
#102300=CARTESIAN_POINT ( 'NONE',  ( -19.03943276465977164, 0.05219959533909376836, 31.24890960531435979 ) ) ;
#102302=CARTESIAN_POINT ( 'NONE',  ( -9.564922557961040184, 16.46253265017147172, 87.91775706135233293 ) ) ;
#102303=CARTESIAN_POINT ( 'NONE',  ( 12.14591786802309770, 12.06949235617756955, 59.37390960531436690 ) ) ;
#102304=CARTESIAN_POINT ( 'NONE',  ( -21.55341960407610458, -5.719274019375992779, 36.45724293864768839 ) ) ;
#102305=CARTESIAN_POINT ( 'NONE',  ( 10.81492255796106328, -18.62759615963255655, 105.4177570613523613 ) ) ;
#102306=CARTESIAN_POINT ( 'NONE',  ( 21.55341960407610458, 5.719274019375980345, 78.95724293864769550 ) ) ;
#102307=CARTESIAN_POINT ( 'NONE',  ( 21.52544592524334988, 5.823673210054432836, 71.45942372801901854 ) ) ;
#102308=CARTESIAN_POINT ( 'NONE',  ( -18.67979575497193778, 10.72451020669871902, 63.33442372801900433 ) ) ;
#102309=CARTESIAN_POINT ( 'NONE',  ( -5.153800228976328057, -19.02544592524343514, 112.2905762719810099 ) ) ;
#102310=CARTESIAN_POINT ( 'NONE',  ( -12.06949235617739369, -12.14591786802326823, 104.3760903946856899 ) ) ;
#102311=CARTESIAN_POINT ( 'NONE',  ( -21.53943276465977519, -0.05219959533937600094, 58.75109039468568994 ) ) ;
#102312=CARTESIAN_POINT ( 'NONE',  ( -5.049401038298153566, 19.05341960407611168, 55.20724293864769550 ) ) ;
#102313=CARTESIAN_POINT ( 'NONE',  ( 5.049401038297881783, 19.05341960407617563, 32.29275706135233293 ) ) ;
#102314=CARTESIAN_POINT ( 'NONE',  ( 0.05219959533937995610, -21.53943276465977519, 35.00109039468568284 ) ) ;
#102315=CARTESIAN_POINT ( 'NONE',  ( 19.02544592524343514, -5.153800228976328945, 73.54057627198103830 ) ) ;
#102316=CARTESIAN_POINT ( 'NONE',  ( -16.55341960407611168, -4.379528057220339221, 76.45724293864769550 ) ) ;
#102317=CARTESIAN_POINT ( 'NONE',  ( 8.224510206698953496, -14.34966873604960469, 52.91557627198103830 ) ) ;
#102318=CARTESIAN_POINT ( 'NONE',  ( 5.719274019375991003, -21.55341960407610458, 62.70724293864769550 ) ) ;
#102319=CARTESIAN_POINT ( 'NONE',  ( -0.05219959533909027116, -19.03943276465977164, 47.49890960531435979 ) ) ;
#102320=CARTESIAN_POINT ( 'NONE',  ( 15.72974639402199770, -15.80617190586745480, 68.12390960531436690 ) ) ;
#102321=CARTESIAN_POINT ( 'NONE',  ( -5.153800228976607833, 19.02544592524334988, 57.70942372801899012 ) ) ;
#102323=CARTESIAN_POINT ( 'NONE',  ( 12.14591786802309770, 12.06949235617756955, 59.37390960531436690 ) ) ;
#102324=CARTESIAN_POINT ( 'NONE',  ( 18.62759615963271287, -10.81492255796078972, 38.33224293864768839 ) ) ;
#102326=CARTESIAN_POINT ( 'NONE',  ( 17.44270441346516520, 5.991230190323025617, 103.8633507926423079 ) ) ;
#102327=CARTESIAN_POINT ( 'NONE',  ( 4.483927247898790824, -16.52544592524335698, 90.20942372801903275 ) ) ;
#102329=CARTESIAN_POINT ( 'NONE',  ( 9.474510206698729675, 16.51473224551082808, 92.08442372801900433 ) ) ;
#102330=CARTESIAN_POINT ( 'NONE',  ( 12.06949235617757843, -12.14591786802309237, 48.12390960531436690 ) ) ;
#102332=CARTESIAN_POINT ( 'NONE',  ( 9.474510206698971260, -16.51473224551069308, 47.91557627198102409 ) ) ;
#102333=CARTESIAN_POINT ( 'NONE',  ( -12.06949235617756955, 12.14591786802309770, 35.62390960531437401 ) ) ;
#102334=CARTESIAN_POINT ( 'NONE',  ( 19.05341960407611168, 5.049401038298154454, 93.95724293864769550 ) ) ;
#102335=CARTESIAN_POINT ( 'NONE',  ( -16.51473224551069308, -9.474510206698971260, 51.66557627198102409 ) ) ;
#102336=CARTESIAN_POINT ( 'NONE',  ( 21.55341960407619695, -5.719274019375665929, 56.04275706135235424 ) ) ;
#102337=CARTESIAN_POINT ( 'NONE',  ( 13.89961937509977652, -13.97604488694527269, 68.12390960531436690 ) ) ;
#102338=CARTESIAN_POINT ( 'NONE',  ( 9.564922557960805705, 16.46253265017160317, 24.58224293864769194 ) ) ;
#102340=CARTESIAN_POINT ( 'NONE',  ( 19.02544592524343514, -5.153800228976328945, 73.54057627198103830 ) ) ;
#102341=CARTESIAN_POINT ( 'NONE',  ( 10.81492255796078972, 18.62759615963270932, 54.58224293864769550 ) ) ;
#102342=CARTESIAN_POINT ( 'NONE',  ( 19.03943276465977164, -0.05219959533909143690, 33.74890960531435979 ) ) ;
#102343=CARTESIAN_POINT ( 'NONE',  ( -21.53943276465977519, 0.05219959533907696930, 41.24890960531435269 ) ) ;
#102344=CARTESIAN_POINT ( 'NONE',  ( -8.224510206698735004, -14.34966873604973081, 104.5844237280190185 ) ) ;
#102345=CARTESIAN_POINT ( 'NONE',  ( 9.474510206698729675, 16.51473224551082808, 22.08442372801899722 ) ) ;
#102346=CARTESIAN_POINT ( 'NONE',  ( -0.05219959533934338120, 16.53943276465976808, 42.50109039468567573 ) ) ;
#102347=CARTESIAN_POINT ( 'NONE',  ( 14.29746914071037800, 8.314922557961029526, 86.66775706135234714 ) ) ;
#102349=CARTESIAN_POINT ( 'NONE',  ( -4.379528057220086978, -16.55341960407618274, 64.79275706135234714 ) ) ;
#102350=CARTESIAN_POINT ( 'NONE',  ( -19.02544592524342804, 5.153800228976336051, 106.0405762719810241 ) ) ;
#102351=CARTESIAN_POINT ( 'NONE',  ( 16.46253265017160672, -9.564922557960803928, 38.33224293864768839 ) ) ;
#102352=CARTESIAN_POINT ( 'NONE',  ( -16.52544592524335698, -4.483927247898792601, 38.95942372801901854 ) ) ;
#102353=CARTESIAN_POINT ( 'NONE',  ( -5.153800228976328057, -19.02544592524343514, 42.29057627198101699 ) ) ;
#102354=CARTESIAN_POINT ( 'NONE',  ( -5.719274019375665041, -21.55341960407619695, 24.79275706135235779 ) ) ;
#102355=CARTESIAN_POINT ( 'NONE',  ( -4.379528057220086978, -16.55341960407618274, 39.79275706135235424 ) ) ;
#102356=CARTESIAN_POINT ( 'NONE',  ( 8.224510206698742110, 14.34966873604972548, 97.08442372801904696 ) ) ;
#102357=CARTESIAN_POINT ( 'NONE',  ( -21.52544592524334988, -5.823673210054445271, 98.95942372801903275 ) ) ;
#102358=CARTESIAN_POINT ( 'NONE',  ( -13.97604488694547697, 13.89961937509957934, 93.12609039468566152 ) ) ;
#102360=CARTESIAN_POINT ( 'NONE',  ( 19.05341960407617918, -5.049401038297876454, 56.04275706135234714 ) ) ;
#102361=CARTESIAN_POINT ( 'NONE',  ( -14.34966873604960291, -8.224510206698953496, 56.66557627198103830 ) ) ;
#102362=CARTESIAN_POINT ( 'NONE',  ( 16.53943276465976808, -0.05219959533910856209, 113.7489096053143527 ) ) ;
#102363=CARTESIAN_POINT ( 'NONE',  ( 19.05341960407617918, -5.049401038297876454, 61.04275706135232582 ) ) ;
#102364=CARTESIAN_POINT ( 'NONE',  ( 17.40805194821983903, -6.112264579160781253, 58.33371272510607497 ) ) ;
#102365=CARTESIAN_POINT ( 'NONE',  ( -18.67979575497193778, 10.72451020669871902, 68.33442372801900433 ) ) ;
#102366=CARTESIAN_POINT ( 'NONE',  ( 14.29746914071037800, 8.314922557961029526, 26.66775706135235424 ) ) ;
#102367=CARTESIAN_POINT ( 'NONE',  ( 19.35633801406907395, -5.499999999999770850, 56.63373818172765795 ) ) ;
#102368=CARTESIAN_POINT ( 'NONE',  ( -0.05219959533907301413, -21.53943276465977519, 22.49890960531436335 ) ) ;
#102369=CARTESIAN_POINT ( 'NONE',  ( -16.46253265017146816, -9.564922557961047289, 109.1677570613523471 ) ) ;
#102370=CARTESIAN_POINT ( 'NONE',  ( 18.22780087662122384, -5.500000000000022204, 96.01540105326108687 ) ) ;
#102372=CARTESIAN_POINT ( 'NONE',  ( -19.05341960407611168, -5.049401038298163336, 21.45724293864768839 ) ) ;
#102373=CARTESIAN_POINT ( 'NONE',  ( 18.62759615963255655, 10.81492255796105972, 111.6677570613523613 ) ) ;
#102374=CARTESIAN_POINT ( 'NONE',  ( 0.05219959533909260263, 19.03943276465977164, 54.99890960531435979 ) ) ;
#102376=CARTESIAN_POINT ( 'NONE',  ( 10.81492255796106328, -18.62759615963255655, 65.41775706135234714 ) ) ;
#102377=CARTESIAN_POINT ( 'NONE',  ( -21.53943276465977519, -0.05219959533937600094, 98.75109039468568994 ) ) ;
#102378=CARTESIAN_POINT ( 'NONE',  ( 14.34966873604972726, -8.224510206698740333, 105.8344237280190328 ) ) ;
#102379=CARTESIAN_POINT ( 'NONE',  ( -13.89961937509977652, 13.97604488694528158, 80.62390960531436690 ) ) ;
#102380=CARTESIAN_POINT ( 'NONE',  ( 18.67979575497194134, -10.72451020669871369, 50.83442372801901143 ) ) ;
#102381=CARTESIAN_POINT ( 'NONE',  ( 15.80617190586769283, -15.72974639402175789, 50.62609039468568994 ) ) ;
#102382=CARTESIAN_POINT ( 'NONE',  ( -9.564922557961040184, 16.46253265017147172, 82.91775706135233293 ) ) ;
#102383=CARTESIAN_POINT ( 'NONE',  ( -19.03943276465977164, 0.05219959533909376836, 106.2489096053143669 ) ) ;
#102384=CARTESIAN_POINT ( 'NONE',  ( 19.03943276465977164, -0.05219959533909143690, 28.74890960531435624 ) ) ;
#102385=CARTESIAN_POINT ( 'NONE',  ( 5.823673210054125526, 21.52544592524343514, 94.79057627198105251 ) ) ;
#102386=CARTESIAN_POINT ( 'NONE',  ( 9.474510206698729675, 16.51473224551082808, 27.08442372801900433 ) ) ;
#102387=CARTESIAN_POINT ( 'NONE',  ( 12.14591786802309770, 12.06949235617756955, 94.37390960531436690 ) ) ;
#102388=CARTESIAN_POINT ( 'NONE',  ( -9.474510206698964154, 16.51473224551069663, 50.41557627198102409 ) ) ;
#102389=CARTESIAN_POINT ( 'NONE',  ( -16.51473224551082808, 9.474510206698731452, 93.33442372801900433 ) ) ;
#102390=CARTESIAN_POINT ( 'NONE',  ( -8.314922557960811034, -14.29746914071050412, 67.08224293864770971 ) ) ;
#102391=CARTESIAN_POINT ( 'NONE',  ( 15.80617190586769283, -15.72974639402175789, 110.6260903946857042 ) ) ;
#102392=CARTESIAN_POINT ( 'NONE',  ( 16.46253265017160672, -9.564922557960803928, 108.3322429386476955 ) ) ;
#102393=CARTESIAN_POINT ( 'NONE',  ( 5.153800228976615827, -19.02544592524334988, 75.20942372801896170 ) ) ;
#102394=CARTESIAN_POINT ( 'NONE',  ( -21.53943276465977519, 0.05219959533907696930, 81.24890960531436690 ) ) ;
#102395=CARTESIAN_POINT ( 'NONE',  ( 5.719274019375673035, 21.55341960407619339, 37.29275706135235424 ) ) ;
#102396=B_SPLINE_CURVE_WITH_KNOTS ( 'NONE', 3,
 ( #109274, #154786, #2096, #90132, #185127, #46618, #14287, #168949 ),
 .UNSPECIFIED., .F., .F.,
 ( 4, 2, 2, 4 ),
 ( 0.002324770996990997447, 0.005594641632894387095, 0.007229576950846082137, 0.008864512268797777178 ),
 .UNSPECIFIED. ) ;
#102397=CARTESIAN_POINT ( 'NONE',  ( -8.314922557961024197, 14.29746914071037800, 47.91775706135234714 ) ) ;
#102398=CARTESIAN_POINT ( 'NONE',  ( -0.05219959533934338120, 16.53943276465976808, 97.50109039468567573 ) ) ;
#102399=CARTESIAN_POINT ( 'NONE',  ( 4.379528057220092307, 16.55341960407617563, 47.29275706135234003 ) ) ;
#102400=CARTESIAN_POINT ( 'NONE',  ( -10.72451020669870658, -18.67979575497194134, 39.58442372801901143 ) ) ;
#102401=CARTESIAN_POINT ( 'NONE',  ( 21.53943276465977519, -0.05219959533907433946, 43.74890960531435979 ) ) ;
#102402=CARTESIAN_POINT ( 'NONE',  ( -9.564922557960796823, -16.46253265017161027, 32.08224293864769550 ) ) ;
#102404=CARTESIAN_POINT ( 'NONE',  ( 4.379528057220092307, 16.55341960407617563, 62.29275706135236845 ) ) ;
#102405=CARTESIAN_POINT ( 'NONE',  ( 21.53943276465977519, -0.05219959533907433946, 83.74890960531435269 ) ) ;
#102406=CARTESIAN_POINT ( 'NONE',  ( -4.483927247898539470, -16.52544592524342804, 37.29057627198102409 ) ) ;
#102407=CARTESIAN_POINT ( 'NONE',  ( 14.34966873604972726, -8.224510206698740333, 50.83442372801901143 ) ) ;
#102408=CARTESIAN_POINT ( 'NONE',  ( 13.89961937509977652, -13.97604488694527269, 58.12390960531436690 ) ) ;
#102409=CARTESIAN_POINT ( 'NONE',  ( 8.314922557961029526, -14.29746914071037800, 90.41775706135236135 ) ) ;
#102410=CARTESIAN_POINT ( 'NONE',  ( 19.03943276465977164, 0.05219959533936151252, 91.25109039468566152 ) ) ;
#102411=CARTESIAN_POINT ( 'NONE',  ( -18.67979575497178146, -10.72451020669898902, 86.66557627198102409 ) ) ;
#102412=CARTESIAN_POINT ( 'NONE',  ( 16.53943276465976808, -0.05219959533910856209, 28.74890960531435624 ) ) ;
#102413=VERTEX_POINT ( 'NONE', #104987 ) ;
#102414=CARTESIAN_POINT ( 'NONE',  ( 18.87580814761076553, -5.499999999999953815, 93.37172394265763842 ) ) ;
#102415=CARTESIAN_POINT ( 'NONE',  ( -10.72451020669898014, 18.67979575497178502, 55.41557627198102409 ) ) ;
#102416=CARTESIAN_POINT ( 'NONE',  ( 4.379528057220092307, 16.55341960407617563, 102.2927570613523613 ) ) ;
#102417=ORIENTED_EDGE ( 'NONE', *, *, #78315, .F. ) ;
#102418=CARTESIAN_POINT ( 'NONE',  ( 17.50000000000005684, -3.647616755424155865, 102.7966979427856273 ) ) ;
#102419=CARTESIAN_POINT ( 'NONE',  ( 15.72974639402199770, -15.80617190586745480, 93.12390960531436690 ) ) ;
#102420=CARTESIAN_POINT ( 'NONE',  ( -16.53943276465976808, -0.05219959533934237506, 113.7510903946856757 ) ) ;
#102421=CARTESIAN_POINT ( 'NONE',  ( 4.483927247898790824, -16.52544592524335698, 40.20942372801901854 ) ) ;
#102422=CARTESIAN_POINT ( 'NONE',  ( 5.153800228976335163, 19.02544592524342804, 29.79057627198102409 ) ) ;
#102423=B_SPLINE_CURVE_WITH_KNOTS ( 'NONE', 3,
 ( #65611, #131268, #22102, #35276, #21099, #128267 ),
 .UNSPECIFIED., .F., .F.,
 ( 4, 2, 4 ),
 ( 0.000000000000000000, 0.0003837532665635023064, 0.0007675065331270046129 ),
 .UNSPECIFIED. ) ;
#102424=CARTESIAN_POINT ( 'NONE',  ( -5.049401038298153566, 19.05341960407611168, 55.20724293864769550 ) ) ;
#102426=CARTESIAN_POINT ( 'NONE',  ( 10.72451020669898902, -18.67979575497178502, 27.91557627198103830 ) ) ;
#102428=CARTESIAN_POINT ( 'NONE',  ( 8.314922557961029526, -14.29746914071037800, 100.4177570613523471 ) ) ;
#102429=CARTESIAN_POINT ( 'NONE',  ( -13.97604488694547697, 13.89961937509957934, 108.1260903946856331 ) ) ;
#102430=CARTESIAN_POINT ( 'NONE',  ( 19.03943276465977164, 0.05219959533936151252, 41.25109039468566152 ) ) ;
#102431=CARTESIAN_POINT ( 'NONE',  ( -21.53943276465977519, 0.05219959533907696930, 91.24890960531436690 ) ) ;
#102432=CARTESIAN_POINT ( 'NONE',  ( -12.14591786802309592, -12.06949235617757132, 26.87390960531435979 ) ) ;
#102433=CARTESIAN_POINT ( 'NONE',  ( 10.81492255796078972, 18.62759615963270932, 29.58224293864769905 ) ) ;
#102434=CARTESIAN_POINT ( 'NONE',  ( -16.51473224551082808, 9.474510206698731452, 113.3344237280190043 ) ) ;
#102435=CARTESIAN_POINT ( 'NONE',  ( -16.51473224551069308, -9.474510206698971260, 111.6655762719810383 ) ) ;
#102436=CARTESIAN_POINT ( 'NONE',  ( -0.05219959533937732626, 21.53943276465977519, 67.50109039468568994 ) ) ;
#102437=CARTESIAN_POINT ( 'NONE',  ( 16.51473224551069308, 9.474510206698969483, 54.16557627198103120 ) ) ;
#102438=CARTESIAN_POINT ( 'NONE',  ( -8.224510206698948167, 14.34966873604960824, 100.4155762719810241 ) ) ;
#102440=CARTESIAN_POINT ( 'NONE',  ( -0.05219959533909027116, -19.03943276465977164, 67.49890960531436690 ) ) ;
#102441=CARTESIAN_POINT ( 'NONE',  ( 4.483927247898545687, 16.52544592524342804, 74.79057627198105251 ) ) ;
#102442=VERTEX_POINT ( 'NONE', #43320 ) ;
#102443=CARTESIAN_POINT ( 'NONE',  ( -19.03943276465977164, -0.05219959533935918106, 88.75109039468567573 ) ) ;
#102444=CARTESIAN_POINT ( 'NONE',  ( 19.49190055781010145, 5.500000000000001776, 93.06116087098783396 ) ) ;
#102445=CARTESIAN_POINT ( 'NONE',  ( -16.51473224551069308, -9.474510206698971260, 61.66557627198103120 ) ) ;
#102447=CARTESIAN_POINT ( 'NONE',  ( -16.51473224551069308, -9.474510206698971260, 71.66557627198102409 ) ) ;
#102448=CARTESIAN_POINT ( 'NONE',  ( 19.02544592524343514, -5.153800228976328945, 103.5405762719809957 ) ) ;
#102449=CARTESIAN_POINT ( 'NONE',  ( -4.379528057220086978, -16.55341960407618274, 59.79275706135234714 ) ) ;
#102450=CARTESIAN_POINT ( 'NONE',  ( -17.05116617787825106, -6.768360034955700044, 51.34324446740803438 ) ) ;
#102451=CARTESIAN_POINT ( 'NONE',  ( 9.474510206698729675, 16.51473224551082808, 47.08442372801900433 ) ) ;
#102452=CARTESIAN_POINT ( 'NONE',  ( 21.52544592524334988, 5.823673210054432836, 96.45942372801901854 ) ) ;
#102454=CARTESIAN_POINT ( 'NONE',  ( -5.153800228976328057, -19.02544592524343514, 112.2905762719810099 ) ) ;
#102455=CARTESIAN_POINT ( 'NONE',  ( -14.29746914071037622, -8.314922557961029526, 104.1677570613523471 ) ) ;
#102457=CARTESIAN_POINT ( 'NONE',  ( -16.53943276465976808, -0.05219959533934237506, 98.75109039468568994 ) ) ;
#102458=CARTESIAN_POINT ( 'NONE',  ( -16.61371651742605238, 7.165104196376023360, 28.85415069992995640 ) ) ;
#102459=CARTESIAN_POINT ( 'NONE',  ( -12.14591786802326823, 12.06949235617739902, 68.12609039468567573 ) ) ;
#102460=ORIENTED_EDGE ( 'NONE', *, *, #58823, .F. ) ;
#102461=CARTESIAN_POINT ( 'NONE',  ( 15.72974639402176855, 15.80617190586768217, 76.87609039468567573 ) ) ;
#102462=CARTESIAN_POINT ( 'NONE',  ( 5.153800228976615827, -19.02544592524334988, 90.20942372801900433 ) ) ;
#102463=CARTESIAN_POINT ( 'NONE',  ( -9.564922557961040184, 16.46253265017147172, 27.91775706135232582 ) ) ;
#102464=CARTESIAN_POINT ( 'NONE',  ( 5.153800228976335163, 19.02544592524342804, 69.79057627198103830 ) ) ;
#102465=CARTESIAN_POINT ( 'NONE',  ( -9.564922557960796823, -16.46253265017161027, 52.08224293864768839 ) ) ;
#102467=CARTESIAN_POINT ( 'NONE',  ( -10.81492255796078084, -18.62759615963271287, 82.08224293864768129 ) ) ;
#102469=CARTESIAN_POINT ( 'NONE',  ( -5.719274019375978568, 21.55341960407610458, 40.20724293864769550 ) ) ;
#102470=CARTESIAN_POINT ( 'NONE',  ( 13.97604488694527802, 13.89961937509977652, 39.37390960531435269 ) ) ;
#102471=CARTESIAN_POINT ( 'NONE',  ( -0.05219959533934338120, 16.53943276465976808, 62.50109039468568284 ) ) ;
#102472=ORIENTED_EDGE ( 'NONE', *, *, #139157, .T. ) ;
#102473=CARTESIAN_POINT ( 'NONE',  ( -21.55341960407619339, 5.719274019375674811, 33.54275706135234714 ) ) ;
#102474=CARTESIAN_POINT ( 'NONE',  ( -14.34966873604960291, -8.224510206698953496, 66.66557627198102409 ) ) ;
#102476=CARTESIAN_POINT ( 'NONE',  ( -12.06949235617739369, -12.14591786802326823, 29.37609039468568284 ) ) ;
#102477=CARTESIAN_POINT ( 'NONE',  ( -16.46253265017146816, -9.564922557961047289, 49.16775706135233293 ) ) ;
#102478=CARTESIAN_POINT ( 'NONE',  ( -16.55341960407611168, -4.379528057220339221, 51.45724293864770260 ) ) ;
#102479=CARTESIAN_POINT ( 'NONE',  ( -5.719274019375665041, -21.55341960407619695, 24.79275706135235779 ) ) ;
#102480=CARTESIAN_POINT ( 'NONE',  ( -5.049401038298153566, 19.05341960407611168, 100.2072429386476955 ) ) ;
#102481=CARTESIAN_POINT ( 'NONE',  ( -15.72974639402197994, 15.80617190586746368, 75.62390960531439532 ) ) ;
#102482=CARTESIAN_POINT ( 'NONE',  ( 13.97604488694527802, 13.89961937509977652, 84.37390960531433848 ) ) ;
#102483=CARTESIAN_POINT ( 'NONE',  ( -16.55341960407611168, -4.379528057220339221, 56.45724293864768839 ) ) ;
#102486=CARTESIAN_POINT ( 'NONE',  ( -16.46253265017146816, -9.564922557961047289, 69.16775706135233293 ) ) ;
#102487=CARTESIAN_POINT ( 'NONE',  ( -5.823673210054116645, -21.52544592524344225, 102.2905762719810383 ) ) ;
#102488=CARTESIAN_POINT ( 'NONE',  ( -16.46253265017160317, 9.564922557960807481, 50.83224293864770260 ) ) ;
#102489=CARTESIAN_POINT ( 'NONE',  ( -19.02544592524334988, -5.153800228976617603, 38.95942372801900433 ) ) ;
#102490=CARTESIAN_POINT ( 'NONE',  ( 5.153800228976335163, 19.02544592524342804, 29.79057627198102409 ) ) ;
#102492=CARTESIAN_POINT ( 'NONE',  ( 15.80617190586769283, -15.72974639402175789, 70.62609039468567573 ) ) ;
#102494=CARTESIAN_POINT ( 'NONE',  ( -18.56453257813365454, 5.499999999999960032, 100.9900042369068842 ) ) ;
#102495=CARTESIAN_POINT ( 'NONE',  ( -14.29746914071049879, 8.314922557960819915, 40.83224293864769550 ) ) ;
#102496=CARTESIAN_POINT ( 'NONE',  ( -9.474510206698964154, 16.51473224551069663, 65.41557627198102409 ) ) ;
#102497=CARTESIAN_POINT ( 'NONE',  ( -5.719274019375978568, 21.55341960407610458, 70.20724293864769550 ) ) ;
#102498=CARTESIAN_POINT ( 'NONE',  ( 9.564922557960805705, 16.46253265017160317, 54.58224293864769550 ) ) ;
#102500=CARTESIAN_POINT ( 'NONE',  ( -15.72974639402197994, 15.80617190586746368, 60.62390960531437401 ) ) ;
#102501=ORIENTED_EDGE ( 'NONE', *, *, #141568, .T. ) ;
#102502=CARTESIAN_POINT ( 'NONE',  ( 0.05219959533937995610, -21.53943276465977519, 105.0010903946856757 ) ) ;
#102504=CARTESIAN_POINT ( 'NONE',  ( 4.483927247898790824, -16.52544592524335698, 100.2094237280190043 ) ) ;
#102505=CARTESIAN_POINT ( 'NONE',  ( -16.53943276465976808, 0.05219959533911058130, 81.24890960531436690 ) ) ;
#102506=CARTESIAN_POINT ( 'NONE',  ( -9.564922557961040184, 16.46253265017147172, 87.91775706135233293 ) ) ;
#102507=ORIENTED_EDGE ( 'NONE', *, *, #26552, .F. ) ;
#102508=CARTESIAN_POINT ( 'NONE',  ( 9.474510206698729675, 16.51473224551082808, 42.08442372801900433 ) ) ;
#102509=CARTESIAN_POINT ( 'NONE',  ( -14.29746914071037622, -8.314922557961029526, 104.1677570613523471 ) ) ;
#102510=CARTESIAN_POINT ( 'NONE',  ( 19.03943276465977164, 0.05219959533936151252, 26.25109039468566507 ) ) ;
#102511=CARTESIAN_POINT ( 'NONE',  ( 13.97604488694527802, 13.89961937509977652, 94.37390960531436690 ) ) ;
#102512=CARTESIAN_POINT ( 'NONE',  ( -21.52544592524343514, 5.823673210054127303, 56.04057627198102409 ) ) ;
#102514=CARTESIAN_POINT ( 'NONE',  ( -4.379528057220328563, 16.55341960407611168, 115.2072429386476955 ) ) ;
#102516=CARTESIAN_POINT ( 'NONE',  ( 21.55341960407619695, -5.719274019375665929, 91.04275706135236135 ) ) ;
#102517=CARTESIAN_POINT ( 'NONE',  ( -12.14591786802326823, 12.06949235617739902, 78.12609039468570415 ) ) ;
#102518=CARTESIAN_POINT ( 'NONE',  ( -21.55341960407619339, 5.719274019375674811, 28.54275706135234358 ) ) ;
#102519=CARTESIAN_POINT ( 'NONE',  ( -14.29746914071037622, -8.314922557961029526, 24.16775706135235424 ) ) ;
#102520=CARTESIAN_POINT ( 'NONE',  ( -16.51473224551069308, -9.474510206698971260, 91.66557627198103830 ) ) ;
#102521=CARTESIAN_POINT ( 'NONE',  ( -13.97604488694527625, -13.89961937509977652, 46.87390960531435979 ) ) ;
#102522=CARTESIAN_POINT ( 'NONE',  ( -19.03943276465977164, 0.05219959533909376836, 56.24890960531435979 ) ) ;
#102524=CARTESIAN_POINT ( 'NONE',  ( 4.483927247898790824, -16.52544592524335698, 30.20942372801902565 ) ) ;
#102525=CARTESIAN_POINT ( 'NONE',  ( -8.224510206698948167, 14.34966873604960824, 90.41557627198103830 ) ) ;
#102526=CARTESIAN_POINT ( 'NONE',  ( 16.53943276465976808, 0.05219959533934440121, 106.2510903946856757 ) ) ;
#102527=CARTESIAN_POINT ( 'NONE',  ( 10.72451020669871369, 18.67979575497193778, 37.08442372801901143 ) ) ;
#102528=CARTESIAN_POINT ( 'NONE',  ( -19.05341960407611168, -5.049401038298163336, 81.45724293864769550 ) ) ;
#102529=CARTESIAN_POINT ( 'NONE',  ( -9.474510206698964154, 16.51473224551069663, 60.41557627198102409 ) ) ;
#102530=CARTESIAN_POINT ( 'NONE',  ( -19.05341960407611168, -5.049401038298163336, 81.45724293864769550 ) ) ;
#102531=CARTESIAN_POINT ( 'NONE',  ( 4.483927247898545687, 16.52544592524342804, 34.79057627198103120 ) ) ;
#102532=CARTESIAN_POINT ( 'NONE',  ( -12.06949235617739369, -12.14591786802326823, 99.37609039468568994 ) ) ;
#102534=CARTESIAN_POINT ( 'NONE',  ( -9.564922557961040184, 16.46253265017147172, 47.91775706135233293 ) ) ;
#102536=CARTESIAN_POINT ( 'NONE',  ( -9.564922557960796823, -16.46253265017161027, 52.08224293864768839 ) ) ;
#102537=CARTESIAN_POINT ( 'NONE',  ( -13.97604488694547697, 13.89961937509957934, 38.12609039468566152 ) ) ;
#102539=CARTESIAN_POINT ( 'NONE',  ( 14.29746914071037800, 8.314922557961029526, 46.66775706135234714 ) ) ;
#102540=CARTESIAN_POINT ( 'NONE',  ( -9.474510206698720793, -16.51473224551083518, 74.58442372801900433 ) ) ;
#102541=CARTESIAN_POINT ( 'NONE',  ( 12.06949235617739724, 12.14591786802326823, 61.87609039468568284 ) ) ;
#102542=CARTESIAN_POINT ( 'NONE',  ( 16.46253265017160672, -9.564922557960803928, 113.3322429386476955 ) ) ;
#102543=CARTESIAN_POINT ( 'NONE',  ( -19.03943276465977164, 0.05219959533909376836, 76.24890960531435269 ) ) ;
#102544=CARTESIAN_POINT ( 'NONE',  ( -21.53943276465977519, 0.05219959533907696930, 106.2489096053143811 ) ) ;
#102545=CARTESIAN_POINT ( 'NONE',  ( -13.89961937509957401, -13.97604488694547875, 74.37609039468566152 ) ) ;
#102546=CARTESIAN_POINT ( 'NONE',  ( -13.97604488694527625, -13.89961937509977652, 111.8739096053143243 ) ) ;
#102547=CARTESIAN_POINT ( 'NONE',  ( -19.03943276465977164, 0.05219959533909376836, 31.24890960531435979 ) ) ;
#102548=CARTESIAN_POINT ( 'NONE',  ( 9.564922557960805705, 16.46253265017160317, 79.58224293864769550 ) ) ;
#102549=CARTESIAN_POINT ( 'NONE',  ( -14.34966873604960291, -8.224510206698953496, 31.66557627198102054 ) ) ;
#102550=CARTESIAN_POINT ( 'NONE',  ( -9.474510206698964154, 16.51473224551069663, 40.41557627198103120 ) ) ;
#102551=CARTESIAN_POINT ( 'NONE',  ( -19.05341960407617563, 5.049401038297882671, 48.54275706135233293 ) ) ;
#102552=CARTESIAN_POINT ( 'NONE',  ( 8.224510206698953496, -14.34966873604960469, 92.91557627198103830 ) ) ;
#102553=CARTESIAN_POINT ( 'NONE',  ( 5.823673210054444382, -21.52544592524334988, 110.2094237280190185 ) ) ;
#102554=CARTESIAN_POINT ( 'NONE',  ( -19.03943276465977164, 0.05219959533909376836, 46.24890960531435979 ) ) ;
#102555=CARTESIAN_POINT ( 'NONE',  ( -18.62759615963270932, 10.81492255796079327, 45.83224293864769550 ) ) ;
#102556=CARTESIAN_POINT ( 'NONE',  ( -0.05219959533910754901, -16.53943276465976808, 52.49890960531435979 ) ) ;
#102557=CARTESIAN_POINT ( 'NONE',  ( -5.719274019375665041, -21.55341960407619695, 104.7927570613523898 ) ) ;
#102558=CARTESIAN_POINT ( 'NONE',  ( 5.153800228976335163, 19.02544592524342804, 94.79057627198103830 ) ) ;
#102559=CARTESIAN_POINT ( 'NONE',  ( -9.474510206698964154, 16.51473224551069663, 110.4155762719810383 ) ) ;
#102560=CARTESIAN_POINT ( 'NONE',  ( -13.97604488694527625, -13.89961937509977652, 41.87390960531435979 ) ) ;
#102561=CARTESIAN_POINT ( 'NONE',  ( -19.03943276465977164, 0.05219959533909376836, 21.24890960531436335 ) ) ;
#102562=CARTESIAN_POINT ( 'NONE',  ( 4.379528057220339221, -16.55341960407611168, 82.70724293864770971 ) ) ;
#102563=CARTESIAN_POINT ( 'NONE',  ( 10.81492255796078972, 18.62759615963270932, 99.58224293864770971 ) ) ;
#102564=CARTESIAN_POINT ( 'NONE',  ( 19.05341960407611168, 5.049401038298154454, 103.9572429386476671 ) ) ;
#102565=CARTESIAN_POINT ( 'NONE',  ( -10.72451020669898014, 18.67979575497178502, 115.4155762719810241 ) ) ;
#102566=CARTESIAN_POINT ( 'NONE',  ( -16.51473224551069308, -9.474510206698971260, 91.66557627198103830 ) ) ;
#102568=CARTESIAN_POINT ( 'NONE',  ( -14.34966873604960291, -8.224510206698953496, 101.6655762719810383 ) ) ;
#102569=CARTESIAN_POINT ( 'NONE',  ( -19.02544592524342804, 5.153800228976336051, 76.04057627198102409 ) ) ;
#102570=CARTESIAN_POINT ( 'NONE',  ( 5.823673210054125526, 21.52544592524343514, 84.79057627198102409 ) ) ;
#102572=CARTESIAN_POINT ( 'NONE',  ( -16.46253265017160317, 9.564922557960807481, 115.8322429386477097 ) ) ;
#102574=CARTESIAN_POINT ( 'NONE',  ( -5.719274019375978568, 21.55341960407610458, 25.20724293864769550 ) ) ;
#102576=CARTESIAN_POINT ( 'NONE',  ( -16.52544592524335698, -4.483927247898792601, 38.95942372801901854 ) ) ;
#102577=CARTESIAN_POINT ( 'NONE',  ( 4.483927247898545687, 16.52544592524342804, 99.79057627198103830 ) ) ;
#102579=CARTESIAN_POINT ( 'NONE',  ( 9.564922557960805705, 16.46253265017160317, 89.58224293864769550 ) ) ;
#102580=CARTESIAN_POINT ( 'NONE',  ( -16.51473224551069308, -9.474510206698971260, 51.66557627198102409 ) ) ;
#102581=CARTESIAN_POINT ( 'NONE',  ( 12.06949235617757843, -12.14591786802309237, 78.12390960531436690 ) ) ;
#102582=CARTESIAN_POINT ( 'NONE',  ( 5.719274019375991003, -21.55341960407610458, 32.70724293864770260 ) ) ;
#102583=CARTESIAN_POINT ( 'NONE',  ( 4.483927247898545687, 16.52544592524342804, 49.79057627198102409 ) ) ;
#102584=CARTESIAN_POINT ( 'NONE',  ( 19.05341960407617918, -5.049401038297876454, 106.0427570613523471 ) ) ;
#102585=CARTESIAN_POINT ( 'NONE',  ( -10.81492255796105439, 18.62759615963255655, 67.91775706135234714 ) ) ;
#102587=CARTESIAN_POINT ( 'NONE',  ( -19.02544592524342804, 5.153800228976336051, 111.0405762719810099 ) ) ;
#102588=CARTESIAN_POINT ( 'NONE',  ( 4.483927247898790824, -16.52544592524335698, 80.20942372801901854 ) ) ;
#102589=CARTESIAN_POINT ( 'NONE',  ( -13.97604488694527625, -13.89961937509977652, 21.87390960531435979 ) ) ;
#102590=CARTESIAN_POINT ( 'NONE',  ( -0.05219959533909027116, -19.03943276465977164, 82.49890960531436690 ) ) ;
#102591=CARTESIAN_POINT ( 'NONE',  ( -21.52544592524343514, 5.823673210054127303, 86.04057627198102409 ) ) ;
#102592=CARTESIAN_POINT ( 'NONE',  ( 8.224510206698742110, 14.34966873604972548, 27.08442372801901854 ) ) ;
#102593=CARTESIAN_POINT ( 'NONE',  ( 14.34966873604960469, 8.224510206698951720, 49.16557627198102409 ) ) ;
#102594=CARTESIAN_POINT ( 'NONE',  ( -18.62759615963255300, -10.81492255796106328, 79.16775706135234714 ) ) ;
#102595=CARTESIAN_POINT ( 'NONE',  ( -12.06949235617739369, -12.14591786802326823, 89.37609039468568994 ) ) ;
#102596=CARTESIAN_POINT ( 'NONE',  ( 0.05219959533907565091, 21.53943276465977519, 29.99890960531435979 ) ) ;
#102597=CARTESIAN_POINT ( 'NONE',  ( -19.02544592524342804, 5.153800228976336939, 111.0405762719810241 ) ) ;
#102599=CARTESIAN_POINT ( 'NONE',  ( 16.53943276465976808, 0.05219959533934440121, 101.2510903946856757 ) ) ;
#102600=CARTESIAN_POINT ( 'NONE',  ( -0.05219959533934338120, 16.53943276465976808, 62.50109039468568284 ) ) ;
#102601=CARTESIAN_POINT ( 'NONE',  ( -16.46253265017160317, 9.564922557960807481, 75.83224293864769550 ) ) ;
#102602=CARTESIAN_POINT ( 'NONE',  ( 5.049401038298161559, -19.05341960407611168, 92.70724293864769550 ) ) ;
#102603=CARTESIAN_POINT ( 'NONE',  ( 10.81492255796106328, -18.62759615963255655, 70.41775706135236135 ) ) ;
#102604=CARTESIAN_POINT ( 'NONE',  ( -8.314922557961024197, 14.29746914071037800, 72.91775706135234714 ) ) ;
#102605=CARTESIAN_POINT ( 'NONE',  ( -12.14591786802309592, -12.06949235617757132, 51.87390960531437401 ) ) ;
#102606=CARTESIAN_POINT ( 'NONE',  ( -16.46253265017160317, 9.564922557960807481, 60.83224293864769550 ) ) ;
#102607=CARTESIAN_POINT ( 'NONE',  ( 9.474510206698971260, -16.51473224551069308, 42.91557627198103120 ) ) ;
#102608=ORIENTED_EDGE ( 'NONE', *, *, #32278, .F. ) ;
#102609=CARTESIAN_POINT ( 'NONE',  ( 16.51473224551083163, -9.474510206698727899, 95.83442372801900433 ) ) ;
#102610=CARTESIAN_POINT ( 'NONE',  ( 8.224510206698953496, -14.34966873604960469, 107.9155762719810241 ) ) ;
#102611=CARTESIAN_POINT ( 'NONE',  ( 5.049401038298161559, -19.05341960407611168, 62.70724293864769550 ) ) ;
#102612=CARTESIAN_POINT ( 'NONE',  ( -9.564922557961040184, 16.46253265017147172, 102.9177570613523329 ) ) ;
#102614=CARTESIAN_POINT ( 'NONE',  ( -5.823673210054431948, 21.52544592524334988, 107.7094237280190328 ) ) ;
#102615=CARTESIAN_POINT ( 'NONE',  ( 8.224510206698742110, 14.34966873604972548, 62.08442372801901143 ) ) ;
#102616=CARTESIAN_POINT ( 'NONE',  ( -19.02544592524334988, -5.153800228976617603, 93.95942372801900433 ) ) ;
#102617=CARTESIAN_POINT ( 'NONE',  ( 18.62759615963271287, -10.81492255796078972, 63.33224293864770260 ) ) ;
#102618=CARTESIAN_POINT ( 'NONE',  ( -4.483927247898782831, 16.52544592524335698, 47.70942372801902565 ) ) ;
#102620=CARTESIAN_POINT ( 'NONE',  ( 13.97604488694548053, -13.89961937509957401, 60.62609039468564731 ) ) ;
#102621=CARTESIAN_POINT ( 'NONE',  ( -10.81492255796105439, 18.62759615963255655, 97.91775706135236135 ) ) ;
#102622=CARTESIAN_POINT ( 'NONE',  ( -13.89961937509977652, 13.97604488694528158, 25.62390960531434558 ) ) ;
#102623=CARTESIAN_POINT ( 'NONE',  ( 13.97604488694527802, 13.89961937509977652, 69.37390960531436690 ) ) ;
#102624=CARTESIAN_POINT ( 'NONE',  ( 8.314922557960818139, 14.29746914071049879, 64.58224293864769550 ) ) ;
#102626=CARTESIAN_POINT ( 'NONE',  ( -21.55341960407619339, 5.719274019375674811, 93.54275706135234714 ) ) ;
#102627=CARTESIAN_POINT ( 'NONE',  ( -19.03943276465977164, -0.05219959533935918106, 43.75109039468566863 ) ) ;
#102628=CARTESIAN_POINT ( 'NONE',  ( -19.02544592524334988, -5.153800228976617603, 23.95942372801900078 ) ) ;
#102629=CARTESIAN_POINT ( 'NONE',  ( 13.97604488694527802, 13.89961937509977652, 114.3739096053143669 ) ) ;
#102630=CARTESIAN_POINT ( 'NONE',  ( 0.05219959533937995610, -21.53943276465977519, 95.00109039468568994 ) ) ;
#102631=CARTESIAN_POINT ( 'NONE',  ( -5.153800228976328057, -19.02544592524343514, 72.29057627198102409 ) ) ;
#102632=CARTESIAN_POINT ( 'NONE',  ( 5.823673210054444382, -21.52544592524334988, 95.20942372801903275 ) ) ;
#102633=CARTESIAN_POINT ( 'NONE',  ( -10.72451020669898014, 18.67979575497178502, 50.41557627198103120 ) ) ;
#102634=CARTESIAN_POINT ( 'NONE',  ( -9.474510206698964154, 16.51473224551069663, 85.41557627198102409 ) ) ;
#102635=CARTESIAN_POINT ( 'NONE',  ( -19.03943276465977164, -0.05219959533935918106, 58.75109039468566863 ) ) ;
#102636=CARTESIAN_POINT ( 'NONE',  ( -16.51473224551069308, -9.474510206698971260, 36.66557627198102409 ) ) ;
#102637=CARTESIAN_POINT ( 'NONE',  ( -9.474510206698964154, 16.51473224551069663, 90.41557627198103830 ) ) ;
#102638=CARTESIAN_POINT ( 'NONE',  ( 5.049401038297881783, 19.05341960407617563, 87.29275706135234714 ) ) ;
#102639=CARTESIAN_POINT ( 'NONE',  ( -4.379528057220086978, -16.55341960407618274, 44.79275706135234714 ) ) ;
#102640=CARTESIAN_POINT ( 'NONE',  ( 4.379528057220339221, -16.55341960407611168, 107.7072429386476955 ) ) ;
#102641=CARTESIAN_POINT ( 'NONE',  ( -9.474510206698964154, 16.51473224551069663, 65.41557627198102409 ) ) ;
#102642=CARTESIAN_POINT ( 'NONE',  ( -18.67979575497178146, -10.72451020669898902, 51.66557627198102409 ) ) ;
#102643=CARTESIAN_POINT ( 'NONE',  ( 16.53943276465976808, 0.05219959533934440121, 21.25109039468567218 ) ) ;
#102644=CARTESIAN_POINT ( 'NONE',  ( 5.719274019375673035, 21.55341960407619339, 27.29275706135234358 ) ) ;
#102645=CARTESIAN_POINT ( 'NONE',  ( 5.719274019375673035, 21.55341960407619339, 82.29275706135234714 ) ) ;
#102646=CARTESIAN_POINT ( 'NONE',  ( -4.483927247898782831, 16.52544592524335698, 82.70942372801900433 ) ) ;
#102647=CARTESIAN_POINT ( 'NONE',  ( -0.05219959533909027116, -19.03943276465977164, 72.49890960531435269 ) ) ;
#102648=CARTESIAN_POINT ( 'NONE',  ( -16.53943276465976808, -0.05219959533934237506, 98.75109039468568994 ) ) ;
#102649=CARTESIAN_POINT ( 'NONE',  ( 5.049401038297881783, 19.05341960407617563, 62.29275706135234003 ) ) ;
#102650=CARTESIAN_POINT ( 'NONE',  ( 18.67979575497194134, -10.72451020669871369, 30.83442372801902209 ) ) ;
#102651=CARTESIAN_POINT ( 'NONE',  ( 14.34966873604960469, 8.224510206698951720, 74.16557627198102409 ) ) ;
#102652=CARTESIAN_POINT ( 'NONE',  ( 9.474510206698971260, -16.51473224551069308, 92.91557627198103830 ) ) ;
#102653=CARTESIAN_POINT ( 'NONE',  ( -4.379528057220086978, -16.55341960407618274, 84.79275706135234714 ) ) ;
#102654=CARTESIAN_POINT ( 'NONE',  ( -5.823673210054431948, 21.52544592524334988, 67.70942372801901854 ) ) ;
#102655=CARTESIAN_POINT ( 'NONE',  ( 12.14591786802327356, -12.06949235617739191, 35.62609039468568994 ) ) ;
#102656=CARTESIAN_POINT ( 'NONE',  ( 18.67979575497194134, -10.72451020669871369, 30.83442372801902209 ) ) ;
#102657=CARTESIAN_POINT ( 'NONE',  ( 16.55341960407611168, 4.379528057220329451, 68.95724293864769550 ) ) ;
#102658=ORIENTED_EDGE ( 'NONE', *, *, #86027, .F. ) ;
#102659=CARTESIAN_POINT ( 'NONE',  ( 21.55341960407610458, 5.719274019375980345, 98.95724293864770971 ) ) ;
#102660=CARTESIAN_POINT ( 'NONE',  ( 16.52544592524342804, -4.483927247898539470, 53.54057627198103120 ) ) ;
#102661=ORIENTED_EDGE ( 'NONE', *, *, #131087, .T. ) ;
#102662=CYLINDRICAL_SURFACE ( 'NONE', #17811, 2.500000000000002220 ) ;
#102663=CARTESIAN_POINT ( 'NONE',  ( 21.53943276465977519, -0.05219959533907433946, 23.74890960531435269 ) ) ;
#102664=CARTESIAN_POINT ( 'NONE',  ( -21.53943276465977519, -0.05219959533937600094, 43.75109039468568284 ) ) ;
#102665=CARTESIAN_POINT ( 'NONE',  ( 16.53943276465976808, -0.05219959533910856209, 58.74890960531436690 ) ) ;
#102666=CARTESIAN_POINT ( 'NONE',  ( -18.67979575497178146, -10.72451020669898902, 66.66557627198102409 ) ) ;
#102667=CARTESIAN_POINT ( 'NONE',  ( 19.03943276465977164, -0.05219959533909143690, 68.74890960531436690 ) ) ;
#102668=FACE_OUTER_BOUND ( 'NONE', #23198, .T. ) ;
#102669=CARTESIAN_POINT ( 'NONE',  ( 5.153800228976615827, -19.02544592524334988, 80.20942372801901854 ) ) ;
#102670=CARTESIAN_POINT ( 'NONE',  ( 10.72451020669898902, -18.67979575497178502, 67.91557627198102409 ) ) ;
#102671=CARTESIAN_POINT ( 'NONE',  ( -13.89961937509977652, 13.97604488694528158, 45.62390960531433848 ) ) ;
#102672=CARTESIAN_POINT ( 'NONE',  ( -19.05341960407611168, -5.049401038298163336, 76.45724293864769550 ) ) ;
#102674=CARTESIAN_POINT ( 'NONE',  ( -16.55341960407617563, 4.379528057220093196, 53.54275706135234714 ) ) ;
#102675=CARTESIAN_POINT ( 'NONE',  ( -5.823673210054431948, 21.52544592524334988, 32.70942372801900433 ) ) ;
#102676=CARTESIAN_POINT ( 'NONE',  ( -5.719274019375665041, -21.55341960407619695, 54.79275706135235424 ) ) ;
#102677=CARTESIAN_POINT ( 'NONE',  ( 5.153800228976335163, 19.02544592524342804, 99.79057627198102409 ) ) ;
#102678=CARTESIAN_POINT ( 'NONE',  ( 18.67979575497178502, 10.72451020669898547, 89.16557627198102409 ) ) ;
#102679=CARTESIAN_POINT ( 'NONE',  ( -0.05219959533907301413, -21.53943276465977519, 112.4989096053143669 ) ) ;
#102680=CARTESIAN_POINT ( 'NONE',  ( 14.29746914071037800, 8.314922557961029526, 51.66775706135234714 ) ) ;
#102681=CARTESIAN_POINT ( 'NONE',  ( -10.81492255796078084, -18.62759615963271287, 52.08224293864768839 ) ) ;
#102682=CARTESIAN_POINT ( 'NONE',  ( 18.62759615963255655, 10.81492255796105972, 106.6677570613523756 ) ) ;
#102683=CARTESIAN_POINT ( 'NONE',  ( 13.97604488694527802, 13.89961937509977652, 54.37390960531435979 ) ) ;
#102684=CARTESIAN_POINT ( 'NONE',  ( -16.51473224551069308, -9.474510206698971260, 106.6655762719810383 ) ) ;
#102685=CARTESIAN_POINT ( 'NONE',  ( 19.03943276465977164, -0.05219959533909143690, 93.74890960531435269 ) ) ;
#102687=CARTESIAN_POINT ( 'NONE',  ( 9.474510206698729675, 16.51473224551082808, 67.08442372801900433 ) ) ;
#102688=CARTESIAN_POINT ( 'NONE',  ( 15.80617190586746368, 15.72974639402197994, 49.37390960531436690 ) ) ;
#102689=CARTESIAN_POINT ( 'NONE',  ( -8.314922557961024197, 14.29746914071037800, 107.9177570613523471 ) ) ;
#102690=CARTESIAN_POINT ( 'NONE',  ( -16.46253265017146816, -9.564922557961047289, 89.16775706135234714 ) ) ;
#102692=CARTESIAN_POINT ( 'NONE',  ( -9.474510206698720793, -16.51473224551083518, 24.58442372801900078 ) ) ;
#102693=CARTESIAN_POINT ( 'NONE',  ( 19.02544592524334988, 5.153800228976608722, 81.45942372801897591 ) ) ;
#102694=CARTESIAN_POINT ( 'NONE',  ( -9.474510206698720793, -16.51473224551083518, 39.58442372801899722 ) ) ;
#102696=CARTESIAN_POINT ( 'NONE',  ( -16.46253265017160317, 9.564922557960807481, 55.83224293864769550 ) ) ;
#102697=CARTESIAN_POINT ( 'NONE',  ( 16.55341960407611168, 4.379528057220329451, 43.95724293864769550 ) ) ;
#102698=CARTESIAN_POINT ( 'NONE',  ( -0.05219959533909027116, -19.03943276465977164, 32.49890960531435979 ) ) ;
#102699=CARTESIAN_POINT ( 'NONE',  ( 16.52544592524342804, -4.483927247898539470, 43.54057627198103830 ) ) ;
#102701=CARTESIAN_POINT ( 'NONE',  ( -12.14591786802326823, 12.06949235617739902, 108.1260903946856757 ) ) ;
#102702=CARTESIAN_POINT ( 'NONE',  ( -13.97604488694527625, -13.89961937509977652, 56.87390960531434558 ) ) ;
#102703=CARTESIAN_POINT ( 'NONE',  ( -13.89961937509957401, -13.97604488694547875, 24.37609039468565442 ) ) ;
#102704=CARTESIAN_POINT ( 'NONE',  ( 12.06949235617739724, 12.14591786802326823, 36.87609039468568994 ) ) ;
#102705=CARTESIAN_POINT ( 'NONE',  ( 10.72451020669898902, -18.67979575497178502, 37.91557627198102409 ) ) ;
#102706=CARTESIAN_POINT ( 'NONE',  ( -21.53943276465977519, -0.05219959533937600094, 88.75109039468567573 ) ) ;
#102707=CARTESIAN_POINT ( 'NONE',  ( 9.474510206698971260, -16.51473224551069308, 57.91557627198103120 ) ) ;
#102708=CARTESIAN_POINT ( 'NONE',  ( -19.02544592524342804, 5.153800228976336051, 106.0405762719810241 ) ) ;
#102709=CARTESIAN_POINT ( 'NONE',  ( -13.97604488694527625, -13.89961937509977652, 96.87390960531433848 ) ) ;
#102711=CARTESIAN_POINT ( 'NONE',  ( 0.05219959533937995610, -21.53943276465977519, 20.00109039468568639 ) ) ;
#102712=CARTESIAN_POINT ( 'NONE',  ( 12.06949235617757843, -12.14591786802309237, 78.12390960531436690 ) ) ;
#102713=CARTESIAN_POINT ( 'NONE',  ( -21.53943276465977519, 0.05219959533907696930, 81.24890960531436690 ) ) ;
#102714=CARTESIAN_POINT ( 'NONE',  ( -16.46253265017160317, 9.564922557960807481, 70.83224293864770971 ) ) ;
#102715=CARTESIAN_POINT ( 'NONE',  ( -9.564922557960796823, -16.46253265017161027, 77.08224293864769550 ) ) ;
#102716=CARTESIAN_POINT ( 'NONE',  ( 10.72451020669898902, -18.67979575497178502, 112.9155762719810383 ) ) ;
#102718=CARTESIAN_POINT ( 'NONE',  ( -19.03943276465977164, 0.05219959533909376836, 56.24890960531435979 ) ) ;
#102719=CARTESIAN_POINT ( 'NONE',  ( 12.14591786802309770, 12.06949235617756955, 99.37390960531436690 ) ) ;
#102720=CARTESIAN_POINT ( 'NONE',  ( -5.049401038298153566, 19.05341960407611168, 25.20724293864768484 ) ) ;
#102721=CARTESIAN_POINT ( 'NONE',  ( -9.474510206698964154, 16.51473224551069663, 70.41557627198102409 ) ) ;
#102722=CARTESIAN_POINT ( 'NONE',  ( 5.049401038297881783, 19.05341960407617563, 87.29275706135234714 ) ) ;
#102723=CARTESIAN_POINT ( 'NONE',  ( 8.314922557960818139, 14.29746914071049879, 94.58224293864769550 ) ) ;
#102724=CARTESIAN_POINT ( 'NONE',  ( -15.72974639402176322, -15.80617190586768395, 54.37609039468568994 ) ) ;
#102725=CARTESIAN_POINT ( 'NONE',  ( -13.89961937509977652, 13.97604488694528158, 55.62390960531434558 ) ) ;
#102726=CARTESIAN_POINT ( 'NONE',  ( -18.67979575497193778, 10.72451020669871902, 23.33442372801901499 ) ) ;
#102727=CARTESIAN_POINT ( 'NONE',  ( 14.34966873604960469, 8.224510206698951720, 104.1655762719810241 ) ) ;
#102729=CARTESIAN_POINT ( 'NONE',  ( -16.46253265017160317, 9.564922557960807481, 70.83224293864770971 ) ) ;
#102730=CARTESIAN_POINT ( 'NONE',  ( -17.49999999999999645, -5.500000000000000888, 120.0000000000000142 ) ) ;
#102731=CARTESIAN_POINT ( 'NONE',  ( -13.89961937509957401, -13.97604488694547875, 109.3760903946856331 ) ) ;
#102732=CARTESIAN_POINT ( 'NONE',  ( -10.81492255796078084, -18.62759615963271287, 32.08224293864769550 ) ) ;
#102733=CARTESIAN_POINT ( 'NONE',  ( -18.67979575497193778, 10.72451020669871902, 48.33442372801902565 ) ) ;
#102734=CARTESIAN_POINT ( 'NONE',  ( 9.474510206698971260, -16.51473224551069308, 102.9155762719810241 ) ) ;
#102735=CARTESIAN_POINT ( 'NONE',  ( 5.049401038297881783, 19.05341960407617563, 87.29275706135234714 ) ) ;
#102736=CARTESIAN_POINT ( 'NONE',  ( -16.46253265017160317, 9.564922557960807481, 75.83224293864769550 ) ) ;
#102738=CARTESIAN_POINT ( 'NONE',  ( -16.52544592524342804, 4.483927247898546575, 76.04057627198102409 ) ) ;
#102739=CARTESIAN_POINT ( 'NONE',  ( -0.05219959533909027116, -19.03943276465977164, 97.49890960531436690 ) ) ;
#102740=CARTESIAN_POINT ( 'NONE',  ( -4.483927247898539470, -16.52544592524342804, 77.29057627198102409 ) ) ;
#102741=CARTESIAN_POINT ( 'NONE',  ( 16.46253265017160672, -9.564922557960803928, 93.33224293864769550 ) ) ;
#102742=CARTESIAN_POINT ( 'NONE',  ( 19.03943276465977164, -0.05219959533909143690, 48.74890960531435979 ) ) ;
#102743=CARTESIAN_POINT ( 'NONE',  ( -16.55341960407611168, -4.379528057220339221, 46.45724293864769550 ) ) ;
#102744=CARTESIAN_POINT ( 'NONE',  ( 19.05341960407611168, 5.049401038298154454, 28.95724293864769550 ) ) ;
#102746=CARTESIAN_POINT ( 'NONE',  ( 15.72974639402176855, 15.80617190586768217, 41.87609039468568284 ) ) ;
#102747=CARTESIAN_POINT ( 'NONE',  ( -9.474510206698720793, -16.51473224551083518, 79.58442372801899012 ) ) ;
#102748=CARTESIAN_POINT ( 'NONE',  ( -4.379528057220328563, 16.55341960407611168, 55.20724293864770260 ) ) ;
#102749=CARTESIAN_POINT ( 'NONE',  ( 21.53943276465977519, -0.05219959533907433946, 93.74890960531436690 ) ) ;
#102750=CARTESIAN_POINT ( 'NONE',  ( -5.823673210054116645, -21.52544592524344225, 32.29057627198102409 ) ) ;
#102751=CARTESIAN_POINT ( 'NONE',  ( -12.06949235617756955, 12.14591786802309770, 80.62390960531438111 ) ) ;
#102752=CARTESIAN_POINT ( 'NONE',  ( 9.564922557960805705, 16.46253265017160317, 49.58224293864770260 ) ) ;
#102753=CARTESIAN_POINT ( 'NONE',  ( -14.34966873604960291, -8.224510206698953496, 26.66557627198103475 ) ) ;
#102755=CARTESIAN_POINT ( 'NONE',  ( 4.379528057220092307, 16.55341960407617563, 87.29275706135236135 ) ) ;
#102756=CARTESIAN_POINT ( 'NONE',  ( -14.29746914071037622, -8.314922557961029526, 74.16775706135231871 ) ) ;
#102757=CARTESIAN_POINT ( 'NONE',  ( 5.049401038297881783, 19.05341960407617563, 32.29275706135233293 ) ) ;
#102758=CARTESIAN_POINT ( 'NONE',  ( -13.97604488694527625, -13.89961937509977652, 96.87390960531433848 ) ) ;
#102759=CARTESIAN_POINT ( 'NONE',  ( 13.97604488694527802, 13.89961937509977652, 79.37390960531435269 ) ) ;
#102760=CARTESIAN_POINT ( 'NONE',  ( -8.224510206698735004, -14.34966873604973081, 74.58442372801901854 ) ) ;
#102761=CARTESIAN_POINT ( 'NONE',  ( 5.153800228976335163, 19.02544592524342804, 39.79057627198100988 ) ) ;
#102762=CARTESIAN_POINT ( 'NONE',  ( -16.55341960407611168, -4.379528057220339221, 51.45724293864770260 ) ) ;
#102763=CARTESIAN_POINT ( 'NONE',  ( -9.474510206698964154, 16.51473224551069663, 115.4155762719810241 ) ) ;
#102764=CARTESIAN_POINT ( 'NONE',  ( 16.51473224551069308, 9.474510206698969483, 99.16557627198102409 ) ) ;
#102765=CARTESIAN_POINT ( 'NONE',  ( -5.823673210054116645, -21.52544592524344225, 32.29057627198102409 ) ) ;
#102766=CARTESIAN_POINT ( 'NONE',  ( -4.379528057220328563, 16.55341960407611168, 75.20724293864769550 ) ) ;
#102767=CARTESIAN_POINT ( 'NONE',  ( 4.483927247898545687, 16.52544592524342804, 69.79057627198102409 ) ) ;
#102769=CARTESIAN_POINT ( 'NONE',  ( 5.153800228976615827, -19.02544592524334988, 65.20942372801900433 ) ) ;
#102770=CARTESIAN_POINT ( 'NONE',  ( -9.474510206698964154, 16.51473224551069663, 100.4155762719810241 ) ) ;
#102771=CARTESIAN_POINT ( 'NONE',  ( 9.564922557961047289, -16.46253265017146816, 80.41775706135234714 ) ) ;
#102773=CARTESIAN_POINT ( 'NONE',  ( 8.224510206698742110, 14.34966873604972548, 22.08442372801901143 ) ) ;
#102774=CARTESIAN_POINT ( 'NONE',  ( -16.53943276465976808, -0.05219959533934237506, 93.75109039468567573 ) ) ;
#102775=CARTESIAN_POINT ( 'NONE',  ( 19.03943276465977164, -0.05219959533909143690, 33.74890960531435979 ) ) ;
#102776=CARTESIAN_POINT ( 'NONE',  ( 18.67979575497178502, 10.72451020669898547, 34.16557627198102409 ) ) ;
#102777=CARTESIAN_POINT ( 'NONE',  ( -15.80617190586768217, 15.72974639402176855, 53.12609039468568284 ) ) ;
#102778=CARTESIAN_POINT ( 'NONE',  ( -8.314922557961024197, 14.29746914071037800, 22.91775706135235069 ) ) ;
#102780=CARTESIAN_POINT ( 'NONE',  ( -13.97604488694527625, -13.89961937509977652, 71.87390960531433848 ) ) ;
#102782=CARTESIAN_POINT ( 'NONE',  ( 13.89961937509977652, -13.97604488694527269, 113.1239096053143527 ) ) ;
#102783=CARTESIAN_POINT ( 'NONE',  ( 4.483927247898545687, 16.52544592524342804, 69.79057627198102409 ) ) ;
#102784=CARTESIAN_POINT ( 'NONE',  ( 9.564922557960805705, 16.46253265017160317, 79.58224293864769550 ) ) ;
#102785=CARTESIAN_POINT ( 'NONE',  ( 13.89961937509977652, -13.97604488694527269, 88.12390960531438111 ) ) ;
#102787=CARTESIAN_POINT ( 'NONE',  ( 19.05341960407617918, -5.049401038297876454, 86.04275706135233293 ) ) ;
#102788=CARTESIAN_POINT ( 'NONE',  ( 21.53943276465977519, -0.05219959533907433946, 58.74890960531436690 ) ) ;
#102789=CARTESIAN_POINT ( 'NONE',  ( 5.153800228976335163, 19.02544592524342804, 29.79057627198102409 ) ) ;
#102790=CARTESIAN_POINT ( 'NONE',  ( 16.51473224551083163, -9.474510206698727899, 50.83442372801899722 ) ) ;
#102791=CARTESIAN_POINT ( 'NONE',  ( -5.049401038298153566, 19.05341960407611168, 55.20724293864769550 ) ) ;
#102792=CARTESIAN_POINT ( 'NONE',  ( 16.46253265017160672, -9.564922557960803928, 98.33224293864769550 ) ) ;
#102794=CARTESIAN_POINT ( 'NONE',  ( -21.52544592524343514, 5.823673210054127303, 86.04057627198102409 ) ) ;
#102795=CARTESIAN_POINT ( 'NONE',  ( 16.52544592524342804, -4.483927247898539470, 98.54057627198105251 ) ) ;
#102796=CARTESIAN_POINT ( 'NONE',  ( -16.46253265017146816, -9.564922557961047289, 54.16775706135234003 ) ) ;
#102797=CARTESIAN_POINT ( 'NONE',  ( -10.72451020669898014, 18.67979575497178502, 95.41557627198102409 ) ) ;
#102798=CARTESIAN_POINT ( 'NONE',  ( 21.52544592524344225, -5.823673210054117533, 78.54057627198103830 ) ) ;
#102799=CARTESIAN_POINT ( 'NONE',  ( -16.53943276465976808, 0.05219959533911058130, 26.24890960531435624 ) ) ;
#102800=CARTESIAN_POINT ( 'NONE',  ( -18.62759615963255300, -10.81492255796106328, 109.1677570613523613 ) ) ;
#102801=CARTESIAN_POINT ( 'NONE',  ( 0.05219959533934541429, -16.53943276465976808, 55.00109039468568284 ) ) ;
#102802=CARTESIAN_POINT ( 'NONE',  ( 13.97604488694527802, 13.89961937509977652, 74.37390960531436690 ) ) ;
#102803=CARTESIAN_POINT ( 'NONE',  ( 5.049401038298161559, -19.05341960407611168, 27.70724293864769550 ) ) ;
#102804=CARTESIAN_POINT ( 'NONE',  ( 21.55341960407619695, -5.719274019375665929, 36.04275706135234714 ) ) ;
#102805=CARTESIAN_POINT ( 'NONE',  ( -10.72451020669870658, -18.67979575497194134, 54.58442372801901143 ) ) ;
#102806=CARTESIAN_POINT ( 'NONE',  ( 19.03943276465977164, -0.05219959533909143690, 53.74890960531436690 ) ) ;
#102807=CARTESIAN_POINT ( 'NONE',  ( -15.80617190586768217, 15.72974639402176855, 28.12609039468568284 ) ) ;
#102809=CARTESIAN_POINT ( 'NONE',  ( 19.03943276465977164, 0.05219959533936151252, 66.25109039468567573 ) ) ;
#102810=CARTESIAN_POINT ( 'NONE',  ( 9.564922557960805705, 16.46253265017160317, 39.58224293864768839 ) ) ;
#102811=CARTESIAN_POINT ( 'NONE',  ( 4.483927247898790824, -16.52544592524335698, 25.20942372801901854 ) ) ;
#102812=CARTESIAN_POINT ( 'NONE',  ( -0.05219959533909027116, -19.03943276465977164, 32.49890960531435979 ) ) ;
#102813=CARTESIAN_POINT ( 'NONE',  ( 12.06949235617739724, 12.14591786802326823, 76.87609039468567573 ) ) ;
#102814=CARTESIAN_POINT ( 'NONE',  ( -13.89961937509977652, 13.97604488694528158, 45.62390960531433848 ) ) ;
#102816=CARTESIAN_POINT ( 'NONE',  ( -9.474510206698964154, 16.51473224551069663, 85.41557627198102409 ) ) ;
#102817=CARTESIAN_POINT ( 'NONE',  ( 19.02544592524343514, -5.153800228976328945, 23.54057627198102054 ) ) ;
#102818=CARTESIAN_POINT ( 'NONE',  ( 10.81492255796078972, 18.62759615963270932, 69.58224293864769550 ) ) ;
#102819=CARTESIAN_POINT ( 'NONE',  ( 12.06949235617739724, 12.14591786802326823, 56.87609039468568994 ) ) ;
#102820=CARTESIAN_POINT ( 'NONE',  ( 5.719274019375673035, 21.55341960407619339, 107.2927570613523471 ) ) ;
#102821=CARTESIAN_POINT ( 'NONE',  ( -5.153800228976328057, -19.02544592524343514, 37.29057627198102409 ) ) ;
#102822=CARTESIAN_POINT ( 'NONE',  ( -8.314922557960811034, -14.29746914071050412, 32.08224293864769550 ) ) ;
#102823=CARTESIAN_POINT ( 'NONE',  ( 16.55341960407611168, 4.379528057220329451, 73.95724293864769550 ) ) ;
#102824=CARTESIAN_POINT ( 'NONE',  ( -19.02544592524342804, 5.153800228976336051, 66.04057627198103830 ) ) ;
#102825=CARTESIAN_POINT ( 'NONE',  ( 21.53943276465977519, 0.05219959533937863772, 111.2510903946856899 ) ) ;
#102826=CARTESIAN_POINT ( 'NONE',  ( -21.52544592524334988, -5.823673210054445271, 18.95942372801901143 ) ) ;
#102827=CARTESIAN_POINT ( 'NONE',  ( 5.153800228976335163, 19.02544592524342804, 84.79057627198099567 ) ) ;
#102828=CARTESIAN_POINT ( 'NONE',  ( -10.72451020669870658, -18.67979575497194134, 84.58442372801903275 ) ) ;
#102829=CARTESIAN_POINT ( 'NONE',  ( 16.53943276465976808, 0.05219959533934440121, 61.25109039468567573 ) ) ;
#102830=CARTESIAN_POINT ( 'NONE',  ( 16.46253265017160672, -9.564922557960803928, 103.3322429386476955 ) ) ;
#102831=CARTESIAN_POINT ( 'NONE',  ( 4.483927247898545687, 16.52544592524342804, 29.79057627198102409 ) ) ;
#102832=CARTESIAN_POINT ( 'NONE',  ( -13.89961937509977652, 13.97604488694528158, 30.62390960531435269 ) ) ;
#102833=CARTESIAN_POINT ( 'NONE',  ( 16.55341960407618274, -4.379528057220086978, 56.04275706135235424 ) ) ;
#102834=CARTESIAN_POINT ( 'NONE',  ( -14.29746914071049879, 8.314922557960819915, 55.83224293864770260 ) ) ;
#102835=CARTESIAN_POINT ( 'NONE',  ( -19.03943276465977164, 0.05219959533909376836, 106.2489096053143669 ) ) ;
#102836=CARTESIAN_POINT ( 'NONE',  ( -10.81492255796078084, -18.62759615963271287, 37.08224293864768129 ) ) ;
#102837=CARTESIAN_POINT ( 'NONE',  ( 15.72974639402176855, 15.80617190586768217, 106.8760903946856899 ) ) ;
#102838=CARTESIAN_POINT ( 'NONE',  ( 12.06949235617757843, -12.14591786802309237, 88.12390960531436690 ) ) ;
#102839=CARTESIAN_POINT ( 'NONE',  ( -13.97604488694527625, -13.89961937509977652, 91.87390960531432427 ) ) ;
#102840=EDGE_LOOP ( 'NONE', ( #169664, #116393, #162459, #110941 ) ) ;
#102841=CARTESIAN_POINT ( 'NONE',  ( -12.06949235617739369, -12.14591786802326823, 54.37609039468568994 ) ) ;
#102842=CARTESIAN_POINT ( 'NONE',  ( -19.05341960407611168, -5.049401038298163336, 61.45724293864769550 ) ) ;
#102843=CARTESIAN_POINT ( 'NONE',  ( -17.29957754486504129, -5.500000000000000888, 21.12734848878977445 ) ) ;
#102844=CARTESIAN_POINT ( 'NONE',  ( -13.97604488694547697, 13.89961937509957934, 53.12609039468565442 ) ) ;
#102845=CARTESIAN_POINT ( 'NONE',  ( 9.564922557960805705, 16.46253265017160317, 44.58224293864769550 ) ) ;
#102846=CARTESIAN_POINT ( 'NONE',  ( -16.52544592524335698, -4.483927247898792601, 78.95942372801901854 ) ) ;
#102847=CARTESIAN_POINT ( 'NONE',  ( -19.02544592524334988, -5.153800228976617603, 93.95942372801900433 ) ) ;
#102848=CARTESIAN_POINT ( 'NONE',  ( -0.05219959533937732626, 21.53943276465977519, 67.50109039468568994 ) ) ;
#102849=CARTESIAN_POINT ( 'NONE',  ( 5.153800228976335163, 19.02544592524342804, 59.79057627198100988 ) ) ;
#102850=CARTESIAN_POINT ( 'NONE',  ( 10.81492255796078972, 18.62759615963270932, 94.58224293864769550 ) ) ;
#102851=CARTESIAN_POINT ( 'NONE',  ( 14.34966873604960469, 8.224510206698951720, 99.16557627198100988 ) ) ;
#102852=CARTESIAN_POINT ( 'NONE',  ( -13.97604488694547697, 13.89961937509957934, 68.12609039468563310 ) ) ;
#102853=CARTESIAN_POINT ( 'NONE',  ( 21.55341960407610458, 5.719274019375980345, 68.95724293864769550 ) ) ;
#102854=CARTESIAN_POINT ( 'NONE',  ( -0.05219959533936034679, 19.03943276465977164, 42.50109039468566152 ) ) ;
#102855=CARTESIAN_POINT ( 'NONE',  ( 18.89770734986047884, 5.499999999999944933, 96.60214472496645044 ) ) ;
#102856=CARTESIAN_POINT ( 'NONE',  ( 5.719274019375991003, -21.55341960407610458, 92.70724293864770971 ) ) ;
#102857=CARTESIAN_POINT ( 'NONE',  ( -19.01533133064925352, 5.499999999999451994, 53.76586590595741200 ) ) ;
#102858=CARTESIAN_POINT ( 'NONE',  ( 16.52544592524335698, 4.483927247898782831, 21.45942372801901499 ) ) ;
#102860=CARTESIAN_POINT ( 'NONE',  ( 14.29746914071037800, 8.314922557961029526, 26.66775706135235424 ) ) ;
#102861=CARTESIAN_POINT ( 'NONE',  ( -13.97604488694527625, -13.89961937509977652, 46.87390960531435979 ) ) ;
#102862=CARTESIAN_POINT ( 'NONE',  ( 0.05219959533909260263, 19.03943276465977164, 104.9989096053143669 ) ) ;
#102863=CARTESIAN_POINT ( 'NONE',  ( -21.53943276465977519, 0.05219959533907696930, 91.24890960531436690 ) ) ;
#102864=CARTESIAN_POINT ( 'NONE',  ( -5.719274019375665041, -21.55341960407619695, 69.79275706135234714 ) ) ;
#102865=CARTESIAN_POINT ( 'NONE',  ( -4.379528057220086978, -16.55341960407618274, 19.79275706135235069 ) ) ;
#102866=CARTESIAN_POINT ( 'NONE',  ( 16.46253265017146816, 9.564922557961045513, 31.66775706135232937 ) ) ;
#102867=CARTESIAN_POINT ( 'NONE',  ( -0.05219959533910754901, -16.53943276465976808, 32.49890960531435979 ) ) ;
#102868=CARTESIAN_POINT ( 'NONE',  ( 15.80617190586746368, 15.72974639402197994, 114.3739096053143527 ) ) ;
#102869=CARTESIAN_POINT ( 'NONE',  ( 16.52544592524342804, -4.483927247898539470, 53.54057627198103120 ) ) ;
#102870=CARTESIAN_POINT ( 'NONE',  ( 9.474510206698729675, 16.51473224551082808, 97.08442372801900433 ) ) ;
#102871=CARTESIAN_POINT ( 'NONE',  ( 9.564922557961047289, -16.46253265017146816, 55.41775706135234003 ) ) ;
#102872=CARTESIAN_POINT ( 'NONE',  ( -15.72974639402176322, -15.80617190586768395, 69.37609039468567573 ) ) ;
#102873=CARTESIAN_POINT ( 'NONE',  ( -5.153800228976607833, 19.02544592524334988, 57.70942372801899012 ) ) ;
#102874=CARTESIAN_POINT ( 'NONE',  ( -16.46253265017160317, 9.564922557960807481, 25.83224293864769194 ) ) ;
#102875=CARTESIAN_POINT ( 'NONE',  ( 15.72974639402199770, -15.80617190586745480, 38.12390960531436690 ) ) ;
#102876=CARTESIAN_POINT ( 'NONE',  ( 16.52544592524342804, -4.483927247898539470, 48.54057627198103120 ) ) ;
#102877=CARTESIAN_POINT ( 'NONE',  ( -17.60779699588839975, -5.500000000000025757, 51.34981316670105400 ) ) ;
#102878=CARTESIAN_POINT ( 'NONE',  ( -13.97604488694547697, 13.89961937509957934, 23.12609039468565442 ) ) ;
#102879=CARTESIAN_POINT ( 'NONE',  ( 4.483927247898790824, -16.52544592524335698, 65.20942372801901854 ) ) ;
#102880=CARTESIAN_POINT ( 'NONE',  ( -8.314922557960811034, -14.29746914071050412, 42.08224293864769550 ) ) ;
#102881=CARTESIAN_POINT ( 'NONE',  ( 15.72974639402176855, 15.80617190586768217, 81.87609039468568994 ) ) ;
#102882=CARTESIAN_POINT ( 'NONE',  ( 10.72451020669871369, 18.67979575497193778, 67.08442372801901854 ) ) ;
#102883=CARTESIAN_POINT ( 'NONE',  ( 21.52544592524344225, -5.823673210054117533, 83.54057627198102409 ) ) ;
#102884=CARTESIAN_POINT ( 'NONE',  ( 19.03943276465977164, -0.05219959533909143690, 43.74890960531435979 ) ) ;
#102885=CARTESIAN_POINT ( 'NONE',  ( 15.72974639402176855, 15.80617190586768217, 41.87609039468568284 ) ) ;
#102886=CARTESIAN_POINT ( 'NONE',  ( -9.564922557960796823, -16.46253265017161027, 27.08224293864769550 ) ) ;
#102887=CARTESIAN_POINT ( 'NONE',  ( 0.05219959533909260263, 19.03943276465977164, 34.99890960531435979 ) ) ;
#102888=CARTESIAN_POINT ( 'NONE',  ( -14.34966873604960291, -8.224510206698953496, 96.66557627198102409 ) ) ;
#102889=CARTESIAN_POINT ( 'NONE',  ( -19.03943276465977164, 0.05219959533909376836, 81.24890960531436690 ) ) ;
#102890=CARTESIAN_POINT ( 'NONE',  ( -16.53943276465976808, 0.05219959533911058130, 41.24890960531435269 ) ) ;
#102891=CARTESIAN_POINT ( 'NONE',  ( -4.483927247898539470, -16.52544592524342804, 97.29057627198105251 ) ) ;
#102892=CARTESIAN_POINT ( 'NONE',  ( -5.719274019375978568, 21.55341960407610458, 65.20724293864768129 ) ) ;
#102893=CARTESIAN_POINT ( 'NONE',  ( -5.823673210054431948, 21.52544592524334988, 22.70942372801901499 ) ) ;
#102894=CARTESIAN_POINT ( 'NONE',  ( 13.97604488694527802, 13.89961937509977652, 114.3739096053143669 ) ) ;
#102895=CARTESIAN_POINT ( 'NONE',  ( -13.89961937509977652, 13.97604488694528158, 60.62390960531436690 ) ) ;
#102896=CARTESIAN_POINT ( 'NONE',  ( -14.34966873604972548, 8.224510206698743886, 23.33442372801901499 ) ) ;
#102897=CARTESIAN_POINT ( 'NONE',  ( -18.62759615963270932, 10.81492255796079327, 75.83224293864769550 ) ) ;
#102898=CARTESIAN_POINT ( 'NONE',  ( 21.53943276465977519, 0.05219959533937863772, 91.25109039468568994 ) ) ;
#102899=CARTESIAN_POINT ( 'NONE',  ( 19.05341960407611168, 5.049401038298154454, 78.95724293864769550 ) ) ;
#102900=CARTESIAN_POINT ( 'NONE',  ( 15.72974639402199770, -15.80617190586745480, 113.1239096053143953 ) ) ;
#102901=EDGE_CURVE ( 'NONE', #7679, #65322, #73114, .T. ) ;
#102902=CARTESIAN_POINT ( 'NONE',  ( -16.46253265017160317, 9.564922557960807481, 115.8322429386477097 ) ) ;
#102903=CARTESIAN_POINT ( 'NONE',  ( 14.29746914071037800, 8.314922557961029526, 96.66775706135234714 ) ) ;
#102904=CARTESIAN_POINT ( 'NONE',  ( -5.719274019375665041, -21.55341960407619695, 74.79275706135234714 ) ) ;
#102905=CARTESIAN_POINT ( 'NONE',  ( -15.72974639402176322, -15.80617190586768395, 104.3760903946856899 ) ) ;
#102906=CARTESIAN_POINT ( 'NONE',  ( 14.34966873604972726, -8.224510206698740333, 55.83442372801901854 ) ) ;
#102907=CARTESIAN_POINT ( 'NONE',  ( -18.62759615963255300, -10.81492255796106328, 29.16775706135234003 ) ) ;
#102908=CARTESIAN_POINT ( 'NONE',  ( 19.02544592524343514, -5.153800228976328945, 113.5405762719810241 ) ) ;
#102909=CARTESIAN_POINT ( 'NONE',  ( -5.823673210054431948, 21.52544592524334988, 87.70942372801901854 ) ) ;
#102910=CARTESIAN_POINT ( 'NONE',  ( 19.05341960407611168, 5.049401038298154454, 93.95724293864769550 ) ) ;
#102911=CARTESIAN_POINT ( 'NONE',  ( -15.80617190586745835, -15.72974639402198527, 86.87390960531438111 ) ) ;
#102912=CARTESIAN_POINT ( 'NONE',  ( 13.97604488694548053, -13.89961937509957401, 55.62609039468566863 ) ) ;
#102913=CARTESIAN_POINT ( 'NONE',  ( -21.55341960407610458, -5.719274019375992779, 51.45724293864770260 ) ) ;
#102914=CARTESIAN_POINT ( 'NONE',  ( 16.46253265017160672, -9.564922557960803928, 93.33224293864769550 ) ) ;
#102915=CARTESIAN_POINT ( 'NONE',  ( -16.55341960407611168, -4.379528057220339221, 36.45724293864768839 ) ) ;
#102917=CARTESIAN_POINT ( 'NONE',  ( 19.05341960407617918, -5.049401038297876454, 71.04275706135234714 ) ) ;
#102919=CARTESIAN_POINT ( 'NONE',  ( 13.89961937509957401, 13.97604488694547697, 106.8760903946856757 ) ) ;
#102920=CARTESIAN_POINT ( 'NONE',  ( 5.823673210054125526, 21.52544592524343514, 79.79057627198102409 ) ) ;
#102921=CARTESIAN_POINT ( 'NONE',  ( 14.34966873604960469, 8.224510206698951720, 59.16557627198103120 ) ) ;
#102922=CARTESIAN_POINT ( 'NONE',  ( -12.14591786802326823, 12.06949235617739902, 33.12609039468569705 ) ) ;
#102923=CARTESIAN_POINT ( 'NONE',  ( 9.564922557960805705, 16.46253265017160317, 44.58224293864769550 ) ) ;
#102924=CARTESIAN_POINT ( 'NONE',  ( -21.52544592524334988, -5.823673210054445271, 18.95942372801901143 ) ) ;
#102925=CARTESIAN_POINT ( 'NONE',  ( 13.97604488694548053, -13.89961937509957401, 90.62609039468567573 ) ) ;
#102926=CARTESIAN_POINT ( 'NONE',  ( -16.51473224551069308, -9.474510206698971260, 91.66557627198103830 ) ) ;
#102927=CARTESIAN_POINT ( 'NONE',  ( 16.46253265017160672, -9.564922557960803928, 73.33224293864769550 ) ) ;
#102928=CARTESIAN_POINT ( 'NONE',  ( 5.823673210054125526, 21.52544592524343514, 79.79057627198102409 ) ) ;
#102929=CARTESIAN_POINT ( 'NONE',  ( 16.51473224551069308, 9.474510206698969483, 44.16557627198103120 ) ) ;
#102931=CARTESIAN_POINT ( 'NONE',  ( -4.379528057220328563, 16.55341960407611168, 55.20724293864770260 ) ) ;
#102932=CARTESIAN_POINT ( 'NONE',  ( -16.51473224551069308, -9.474510206698971260, 86.66557627198102409 ) ) ;
#102934=CARTESIAN_POINT ( 'NONE',  ( -19.02544592524334988, -5.153800228976617603, 68.95942372801896170 ) ) ;
#102935=CARTESIAN_POINT ( 'NONE',  ( 5.719274019375991003, -21.55341960407610458, 77.70724293864770971 ) ) ;
#102936=CARTESIAN_POINT ( 'NONE',  ( -9.474510206698720793, -16.51473224551083518, 34.58442372801899722 ) ) ;
#102937=CARTESIAN_POINT ( 'NONE',  ( -9.474510206698964154, 16.51473224551069663, 105.4155762719810383 ) ) ;
#102938=CARTESIAN_POINT ( 'NONE',  ( -17.50000000000146372, 3.202012800152269190, 114.9282241602726202 ) ) ;
#102939=CARTESIAN_POINT ( 'NONE',  ( 21.55341960407610458, 5.719274019375980345, 43.95724293864769550 ) ) ;
#102941=CARTESIAN_POINT ( 'NONE',  ( -19.05341960407611168, -5.049401038298163336, 66.45724293864769550 ) ) ;
#102942=CARTESIAN_POINT ( 'NONE',  ( -18.62759615963255300, -10.81492255796106328, 69.16775706135234714 ) ) ;
#102943=CARTESIAN_POINT ( 'NONE',  ( -13.97604488694527625, -13.89961937509977652, 26.87390960531434558 ) ) ;
#102944=CARTESIAN_POINT ( 'NONE',  ( 18.62759615963271287, -10.81492255796078972, 113.3322429386476955 ) ) ;
#102946=CARTESIAN_POINT ( 'NONE',  ( -15.80617190586768217, 15.72974639402176855, 48.12609039468568284 ) ) ;
#102947=ORIENTED_EDGE ( 'NONE', *, *, #142282, .T. ) ;
#102948=CARTESIAN_POINT ( 'NONE',  ( -5.049401038298153566, 19.05341960407611168, 115.2072429386477097 ) ) ;
#102949=CARTESIAN_POINT ( 'NONE',  ( 5.049401038297881783, 19.05341960407617563, 72.29275706135234714 ) ) ;
#102951=CARTESIAN_POINT ( 'NONE',  ( 15.72974639402199770, -15.80617190586745480, 108.1239096053143811 ) ) ;
#102952=CARTESIAN_POINT ( 'NONE',  ( 19.05341960407611168, 5.049401038298154454, 58.95724293864768129 ) ) ;
#102953=CARTESIAN_POINT ( 'NONE',  ( -16.55341960407617563, 4.379528057220093196, 38.54275706135234714 ) ) ;
#102955=CARTESIAN_POINT ( 'NONE',  ( -10.72451020669870658, -18.67979575497194134, 104.5844237280190185 ) ) ;
#102956=CARTESIAN_POINT ( 'NONE',  ( -19.05341960407611168, -5.049401038298163336, 36.45724293864766707 ) ) ;
#102957=CARTESIAN_POINT ( 'NONE',  ( -18.62759615963255300, -10.81492255796106328, 109.1677570613523613 ) ) ;
#102958=CARTESIAN_POINT ( 'NONE',  ( -9.474510206698964154, 16.51473224551069663, 85.41557627198102409 ) ) ;
#102959=CARTESIAN_POINT ( 'NONE',  ( -18.62759615963255300, -10.81492255796106328, 64.16775706135234714 ) ) ;
#102962=FACE_OUTER_BOUND ( 'NONE', #100128, .T. ) ;
#102963=CARTESIAN_POINT ( 'NONE',  ( -4.483927247898782831, 16.52544592524335698, 47.70942372801902565 ) ) ;
#102964=CARTESIAN_POINT ( 'NONE',  ( 5.719274019375673035, 21.55341960407619339, 72.29275706135236135 ) ) ;
#102965=CARTESIAN_POINT ( 'NONE',  ( 21.53943276465977519, 0.05219959533937863772, 91.25109039468568994 ) ) ;
#102967=CARTESIAN_POINT ( 'NONE',  ( -14.34966873604972548, 8.224510206698743886, 23.33442372801901499 ) ) ;
#102968=CARTESIAN_POINT ( 'NONE',  ( -16.51473224551069308, -9.474510206698971260, 91.66557627198103830 ) ) ;
#102969=CARTESIAN_POINT ( 'NONE',  ( -19.03943276465977164, 0.05219959533909376836, 21.24890960531436335 ) ) ;
#102972=CARTESIAN_POINT ( 'NONE',  ( -0.05219959533909027116, -19.03943276465977164, 22.49890960531436690 ) ) ;
#102973=CARTESIAN_POINT ( 'NONE',  ( -10.81492255796078084, -18.62759615963271287, 47.08224293864770260 ) ) ;
#102974=CARTESIAN_POINT ( 'NONE',  ( -0.05219959533934338120, 16.53943276465976808, 107.5010903946856899 ) ) ;
#102975=CARTESIAN_POINT ( 'NONE',  ( -8.224510206698948167, 14.34966873604960824, 80.41557627198103830 ) ) ;
#102976=CARTESIAN_POINT ( 'NONE',  ( -16.51473224551069308, -9.474510206698971260, 66.66557627198102409 ) ) ;
#102977=CARTESIAN_POINT ( 'NONE',  ( 15.72974639402176855, 15.80617190586768217, 91.87609039468568994 ) ) ;
#102978=CARTESIAN_POINT ( 'NONE',  ( 16.53943276465976808, 0.05219959533934440121, 21.25109039468567218 ) ) ;
#102979=CARTESIAN_POINT ( 'NONE',  ( 14.29746914071049879, -8.314922557960816363, 88.33224293864769550 ) ) ;
#102980=CARTESIAN_POINT ( 'NONE',  ( 0.05219959533937995610, -21.53943276465977519, 45.00109039468568284 ) ) ;
#102981=CARTESIAN_POINT ( 'NONE',  ( -5.823673210054116645, -21.52544592524344225, 77.29057627198102409 ) ) ;
#102982=CARTESIAN_POINT ( 'NONE',  ( -5.153800228976607833, 19.02544592524334988, 42.70942372801901143 ) ) ;
#102984=CARTESIAN_POINT ( 'NONE',  ( 13.89961937509977652, -13.97604488694527269, 98.12390960531433848 ) ) ;
#102985=CARTESIAN_POINT ( 'NONE',  ( -8.224510206698948167, 14.34966873604960824, 60.41557627198102409 ) ) ;
#102986=CARTESIAN_POINT ( 'NONE',  ( 14.34966873604960469, 8.224510206698951720, 34.16557627198102409 ) ) ;
#102987=CARTESIAN_POINT ( 'NONE',  ( -16.52544592524335698, -4.483927247898792601, 108.9594237280190185 ) ) ;
#102988=CARTESIAN_POINT ( 'NONE',  ( 5.049401038297881783, 19.05341960407617563, 72.29275706135234714 ) ) ;
#102990=CARTESIAN_POINT ( 'NONE',  ( -15.80617190586745835, -15.72974639402198527, 26.87390960531435979 ) ) ;
#102991=EDGE_CURVE ( 'NONE', #22958, #196449, #12944, .T. ) ;
#102992=CARTESIAN_POINT ( 'NONE',  ( 0.05219959533910956823, 16.53943276465976808, 89.99890960531438111 ) ) ;
#102994=CARTESIAN_POINT ( 'NONE',  ( 16.51473224551069308, 9.474510206698969483, 49.16557627198102409 ) ) ;
#102995=CARTESIAN_POINT ( 'NONE',  ( 15.72974639402199770, -15.80617190586745480, 48.12390960531436690 ) ) ;
#102996=CARTESIAN_POINT ( 'NONE',  ( -18.67979575497178146, -10.72451020669898902, 76.66557627198103830 ) ) ;
#102997=CARTESIAN_POINT ( 'NONE',  ( -12.06949235617756955, 12.14591786802309770, 110.6239096053143669 ) ) ;
#102998=CARTESIAN_POINT ( 'NONE',  ( 12.06949235617739724, 12.14591786802326823, 61.87609039468568284 ) ) ;
#102999=CARTESIAN_POINT ( 'NONE',  ( -13.97604488694527625, -13.89961937509977652, 41.87390960531435979 ) ) ;
#103000=CARTESIAN_POINT ( 'NONE',  ( -10.81492255796105439, 18.62759615963255655, 52.91775706135235424 ) ) ;
#103002=CARTESIAN_POINT ( 'NONE',  ( -16.52544592524342804, 4.483927247898546575, 101.0405762719810383 ) ) ;
#103003=CARTESIAN_POINT ( 'NONE',  ( -5.049401038297874678, -19.05341960407617918, 84.79275706135233293 ) ) ;
#103006=CARTESIAN_POINT ( 'NONE',  ( -21.53943276465977519, 0.05219959533907696930, 51.24890960531436690 ) ) ;
#103007=CARTESIAN_POINT ( 'NONE',  ( 17.05587630539787014, -6.762274262135690606, 68.24180309037316761 ) ) ;
#103008=CARTESIAN_POINT ( 'NONE',  ( -5.719274019375665041, -21.55341960407619695, 79.79275706135236135 ) ) ;
#103010=CARTESIAN_POINT ( 'NONE',  ( 4.379528057220339221, -16.55341960407611168, 27.70724293864769905 ) ) ;
#103011=CARTESIAN_POINT ( 'NONE',  ( 16.53943276465976808, 0.05219959533934440121, 51.25109039468568994 ) ) ;
#103012=CARTESIAN_POINT ( 'NONE',  ( 8.314922557960818139, 14.29746914071049879, 39.58224293864769550 ) ) ;
#103013=CARTESIAN_POINT ( 'NONE',  ( 21.55341960407610458, 5.719274019375980345, 63.95724293864770260 ) ) ;
#103015=CARTESIAN_POINT ( 'NONE',  ( -21.55341960407610458, -5.719274019375992779, 71.45724293864769550 ) ) ;
#103017=CARTESIAN_POINT ( 'NONE',  ( -19.03943276465977164, -0.05219959533935918106, 78.75109039468567573 ) ) ;
#103018=CARTESIAN_POINT ( 'NONE',  ( -21.52544592524343514, 5.823673210054127303, 26.04057627198103475 ) ) ;
#103019=CARTESIAN_POINT ( 'NONE',  ( -13.89961937509977652, 13.97604488694528158, 55.62390960531434558 ) ) ;
#103020=CARTESIAN_POINT ( 'NONE',  ( -8.314922557960811034, -14.29746914071050412, 112.0822429386477097 ) ) ;
#103023=ORIENTED_EDGE ( 'NONE', *, *, #188637, .F. ) ;
#103024=CARTESIAN_POINT ( 'NONE',  ( -14.34966873604972548, 8.224510206698743886, 83.33442372801903275 ) ) ;
#103026=CARTESIAN_POINT ( 'NONE',  ( -21.52544592524343514, 5.823673210054127303, 111.0405762719810525 ) ) ;
#103027=CARTESIAN_POINT ( 'NONE',  ( 19.02544592524343514, -5.153800228976328945, 68.54057627198103830 ) ) ;
#103028=CARTESIAN_POINT ( 'NONE',  ( 0.05219959533937995610, -21.53943276465977519, 35.00109039468568284 ) ) ;
#103029=CARTESIAN_POINT ( 'NONE',  ( 0.05219959533909260263, 19.03943276465977164, 94.99890960531436690 ) ) ;
#103032=CARTESIAN_POINT ( 'NONE',  ( 10.72451020669871369, 18.67979575497193778, 27.08442372801901854 ) ) ;
#103033=CARTESIAN_POINT ( 'NONE',  ( 19.02544592524343514, -5.153800228976328945, 28.54057627198102409 ) ) ;
#103034=CARTESIAN_POINT ( 'NONE',  ( 19.03943276465977164, 0.05219959533936151252, 91.25109039468566152 ) ) ;
#103035=CARTESIAN_POINT ( 'NONE',  ( -19.02544592524334988, -5.153800228976617603, 43.95942372801899012 ) ) ;
#103036=CARTESIAN_POINT ( 'NONE',  ( 0.05219959533907565091, 21.53943276465977519, 114.9989096053143669 ) ) ;
#103037=CARTESIAN_POINT ( 'NONE',  ( -16.51473224551082808, 9.474510206698731452, 43.33442372801900433 ) ) ;
#103038=CARTESIAN_POINT ( 'NONE',  ( 9.564922557961047289, -16.46253265017146816, 50.41775706135233293 ) ) ;
#103039=CARTESIAN_POINT ( 'NONE',  ( -16.53943276465976808, -0.05219959533934237506, 93.75109039468567573 ) ) ;
#103041=ORIENTED_EDGE ( 'NONE', *, *, #180229, .T. ) ;
#103042=CARTESIAN_POINT ( 'NONE',  ( -9.474510206698964154, 16.51473224551069663, 70.41557627198102409 ) ) ;
#103043=CARTESIAN_POINT ( 'NONE',  ( -18.62759615963255300, -10.81492255796106328, 79.16775706135234714 ) ) ;
#103044=CARTESIAN_POINT ( 'NONE',  ( 10.81492255796106328, -18.62759615963255655, 95.41775706135234714 ) ) ;
#103046=CARTESIAN_POINT ( 'NONE',  ( -5.049401038298153566, 19.05341960407611168, 90.20724293864766707 ) ) ;
#103047=CARTESIAN_POINT ( 'NONE',  ( 15.72974639402176855, 15.80617190586768217, 66.87609039468568994 ) ) ;
#103048=CARTESIAN_POINT ( 'NONE',  ( 19.02544592524334988, 5.153800228976608722, 106.4594237280190185 ) ) ;
#103049=CARTESIAN_POINT ( 'NONE',  ( -16.46253265017160317, 9.564922557960807481, 65.83224293864769550 ) ) ;
#103050=CARTESIAN_POINT ( 'NONE',  ( -13.89961937509977652, 13.97604488694528158, 105.6239096053143527 ) ) ;
#103051=CARTESIAN_POINT ( 'NONE',  ( -19.02544592524342804, 5.153800228976336051, 81.04057627198103830 ) ) ;
#103052=CARTESIAN_POINT ( 'NONE',  ( 13.89961937509957579, 13.97604488694547520, 86.87609039468566152 ) ) ;
#103053=CARTESIAN_POINT ( 'NONE',  ( 19.02544592524343514, -5.153800228976328945, 63.54057627198103830 ) ) ;
#103054=CARTESIAN_POINT ( 'NONE',  ( 16.51473224551069308, 9.474510206698969483, 49.16557627198102409 ) ) ;
#103055=CARTESIAN_POINT ( 'NONE',  ( 15.72974639402199770, -15.80617190586745480, 113.1239096053143953 ) ) ;
#103056=CARTESIAN_POINT ( 'NONE',  ( 4.483927247898790824, -16.52544592524335698, 100.2094237280190043 ) ) ;
#103059=CARTESIAN_POINT ( 'NONE',  ( 16.51473224551083163, -9.474510206698727899, 55.83442372801899722 ) ) ;
#103060=CARTESIAN_POINT ( 'NONE',  ( 9.474510206698971260, -16.51473224551069308, 82.91557627198103830 ) ) ;
#103061=CARTESIAN_POINT ( 'NONE',  ( -4.379528057220328563, 16.55341960407611168, 65.20724293864768129 ) ) ;
#103062=CARTESIAN_POINT ( 'NONE',  ( -8.314922557960811034, -14.29746914071050412, 112.0822429386477097 ) ) ;
#103063=CARTESIAN_POINT ( 'NONE',  ( 18.62759615963271287, -10.81492255796078972, 38.33224293864768839 ) ) ;
#103064=CARTESIAN_POINT ( 'NONE',  ( 13.97604488694527802, 13.89961937509977652, 99.37390960531436690 ) ) ;
#103065=CARTESIAN_POINT ( 'NONE',  ( 14.29746914071049879, -8.314922557960816363, 88.33224293864769550 ) ) ;
#103067=CARTESIAN_POINT ( 'NONE',  ( -0.05219959533936034679, 19.03943276465977164, 32.50109039468566863 ) ) ;
#103068=CARTESIAN_POINT ( 'NONE',  ( 4.379528057220092307, 16.55341960407617563, 107.2927570613523471 ) ) ;
#103069=CARTESIAN_POINT ( 'NONE',  ( 0.05219959533909260263, 19.03943276465977164, 94.99890960531436690 ) ) ;
#103070=CARTESIAN_POINT ( 'NONE',  ( -21.52544592524334988, -5.823673210054445271, 58.95942372801902565 ) ) ;
#103071=CARTESIAN_POINT ( 'NONE',  ( -15.72974639402197994, 15.80617190586746368, 50.62390960531435979 ) ) ;
#103072=CARTESIAN_POINT ( 'NONE',  ( 15.80617190586769283, -15.72974639402175789, 30.62609039468567929 ) ) ;
#103073=CARTESIAN_POINT ( 'NONE',  ( 21.53943276465977519, -0.05219959533907433946, 78.74890960531436690 ) ) ;
#103074=CARTESIAN_POINT ( 'NONE',  ( -16.53943276465976808, 0.05219959533911058130, 96.24890960531435269 ) ) ;
#103075=CARTESIAN_POINT ( 'NONE',  ( -13.89961937509957401, -13.97604488694547875, 59.37609039468566863 ) ) ;
#103076=CARTESIAN_POINT ( 'NONE',  ( 5.153800228976335163, 19.02544592524342804, 34.79057627198102409 ) ) ;
#103078=CARTESIAN_POINT ( 'NONE',  ( 16.46253265017160672, -9.564922557960803928, 98.33224293864769550 ) ) ;
#103079=CARTESIAN_POINT ( 'NONE',  ( -5.153800228976328057, -19.02544592524343514, 92.29057627198099567 ) ) ;
#103080=CARTESIAN_POINT ( 'NONE',  ( 0.05219959533910956823, 16.53943276465976808, 109.9989096053143527 ) ) ;
#103081=CARTESIAN_POINT ( 'NONE',  ( -16.55341960407611168, -4.379528057220339221, 21.45724293864769550 ) ) ;
#103082=CARTESIAN_POINT ( 'NONE',  ( 8.314922557961029526, -14.29746914071037800, 35.41775706135234003 ) ) ;
#103083=CARTESIAN_POINT ( 'NONE',  ( 21.55341960407619695, -5.719274019375665929, 111.0427570613523613 ) ) ;
#103084=CARTESIAN_POINT ( 'NONE',  ( 19.05341960407611168, 5.049401038298154454, 113.9572429386477097 ) ) ;
#103085=CARTESIAN_POINT ( 'NONE',  ( 0.05219959533910956823, 16.53943276465976808, 24.99890960531435624 ) ) ;
#103086=CARTESIAN_POINT ( 'NONE',  ( 0.05219959533937995610, -21.53943276465977519, 35.00109039468568284 ) ) ;
#103087=CARTESIAN_POINT ( 'NONE',  ( -19.05341960407611168, -5.049401038298163336, 46.45724293864768129 ) ) ;
#103088=CARTESIAN_POINT ( 'NONE',  ( -16.53943276465976808, -0.05219959533934237506, 43.75109039468568284 ) ) ;
#103089=CARTESIAN_POINT ( 'NONE',  ( -0.05219959533934338120, 16.53943276465976808, 107.5010903946856899 ) ) ;
#103090=CARTESIAN_POINT ( 'NONE',  ( 4.483927247898790824, -16.52544592524335698, 95.20942372801903275 ) ) ;
#103091=CARTESIAN_POINT ( 'NONE',  ( 16.46253265017146816, 9.564922557961045513, 106.6677570613523471 ) ) ;
#103092=CARTESIAN_POINT ( 'NONE',  ( 13.97604488694527802, 13.89961937509977652, 29.37390960531435979 ) ) ;
#103093=CARTESIAN_POINT ( 'NONE',  ( -0.05219959533910754901, -16.53943276465976808, 97.49890960531436690 ) ) ;
#103094=CARTESIAN_POINT ( 'NONE',  ( 10.72451020669898902, -18.67979575497178502, 97.91557627198103830 ) ) ;
#103095=CARTESIAN_POINT ( 'NONE',  ( 0.05219959533909260263, 19.03943276465977164, 29.99890960531435979 ) ) ;
#103096=CARTESIAN_POINT ( 'NONE',  ( 5.153800228976335163, 19.02544592524342804, 109.7905762719810099 ) ) ;
#103097=CARTESIAN_POINT ( 'NONE',  ( -18.62759615963255300, -10.81492255796106328, 34.16775706135234714 ) ) ;
#103098=CARTESIAN_POINT ( 'NONE',  ( 13.97604488694527802, 13.89961937509977652, 24.37390960531435624 ) ) ;
#103100=CARTESIAN_POINT ( 'NONE',  ( -19.05341960407611168, -5.049401038298163336, 111.4572429386476671 ) ) ;
#103101=CARTESIAN_POINT ( 'NONE',  ( 17.13100169013302221, -6.664070546373126902, 113.2678983569985292 ) ) ;
#103102=CARTESIAN_POINT ( 'NONE',  ( 19.05341960407611168, 5.049401038298154454, 83.95724293864766707 ) ) ;
#103103=CARTESIAN_POINT ( 'NONE',  ( 5.719274019375673035, 21.55341960407619339, 27.29275706135234358 ) ) ;
#103104=CARTESIAN_POINT ( 'NONE',  ( -16.55341960407611168, -4.379528057220339221, 91.45724293864769550 ) ) ;
#103105=CARTESIAN_POINT ( 'NONE',  ( -0.05219959533909027116, -19.03943276465977164, 92.49890960531436690 ) ) ;
#103107=CARTESIAN_POINT ( 'NONE',  ( 14.34966873604972726, -8.224510206698740333, 65.83442372801900433 ) ) ;
#103108=CARTESIAN_POINT ( 'NONE',  ( 15.80617190586769283, -15.72974639402175789, 75.62609039468567573 ) ) ;
#103109=CARTESIAN_POINT ( 'NONE',  ( -12.06949235617739369, -12.14591786802326823, 39.37609039468567573 ) ) ;
#103110=CARTESIAN_POINT ( 'NONE',  ( 19.03943276465977164, -0.05219959533909143690, 88.74890960531436690 ) ) ;
#103111=CARTESIAN_POINT ( 'NONE',  ( -13.97604488694547697, 13.89961937509957934, 103.1260903946856473 ) ) ;
#103112=CARTESIAN_POINT ( 'NONE',  ( 0.05219959533934541429, -16.53943276465976808, 65.00109039468568994 ) ) ;
#103113=CARTESIAN_POINT ( 'NONE',  ( 19.03943276465977164, 0.05219959533936151252, 21.25109039468565797 ) ) ;
#103114=CARTESIAN_POINT ( 'NONE',  ( 9.564922557961047289, -16.46253265017146816, 90.41775706135234714 ) ) ;
#103115=CARTESIAN_POINT ( 'NONE',  ( 0.05219959533909260263, 19.03943276465977164, 69.99890960531435269 ) ) ;
#103116=CARTESIAN_POINT ( 'NONE',  ( 21.55341960407610458, 5.719274019375980345, 88.95724293864769550 ) ) ;
#103117=CARTESIAN_POINT ( 'NONE',  ( 0.05219959533910956823, 16.53943276465976808, 89.99890960531438111 ) ) ;
#103118=CARTESIAN_POINT ( 'NONE',  ( -13.89961937509957401, -13.97604488694547875, 89.37609039468563310 ) ) ;
#103119=CARTESIAN_POINT ( 'NONE',  ( -14.34966873604972548, 8.224510206698743886, 63.33442372801900433 ) ) ;
#103120=CARTESIAN_POINT ( 'NONE',  ( -19.52217212775661181, 5.499999999999920064, 79.93993709005260939 ) ) ;
#103121=CARTESIAN_POINT ( 'NONE',  ( 19.02544592524334988, 5.153800228976608722, 51.45942372801900433 ) ) ;
#103122=CARTESIAN_POINT ( 'NONE',  ( -8.314922557960811034, -14.29746914071050412, 27.08224293864769550 ) ) ;
#103123=CARTESIAN_POINT ( 'NONE',  ( 4.483927247898545687, 16.52544592524342804, 79.79057627198102409 ) ) ;
#103124=CARTESIAN_POINT ( 'NONE',  ( -21.53943276465977519, -0.05219959533937600094, 113.7510903946856757 ) ) ;
#103125=CARTESIAN_POINT ( 'NONE',  ( -17.13100169013227259, 6.664070546374130544, 40.76789835699826625 ) ) ;
#103126=CARTESIAN_POINT ( 'NONE',  ( -5.719274019375665041, -21.55341960407619695, 29.79275706135234358 ) ) ;
#103127=CARTESIAN_POINT ( 'NONE',  ( -5.153800228976328057, -19.02544592524343514, 97.29057627198099567 ) ) ;
#103128=CARTESIAN_POINT ( 'NONE',  ( 13.89961937509977652, -13.97604488694527269, 78.12390960531433848 ) ) ;
#103129=CARTESIAN_POINT ( 'NONE',  ( 21.55341960407619695, -5.719274019375665929, 91.04275706135236135 ) ) ;
#103130=CARTESIAN_POINT ( 'NONE',  ( -9.564922557960796823, -16.46253265017161027, 82.08224293864768129 ) ) ;
#103131=CARTESIAN_POINT ( 'NONE',  ( -10.81492255796078084, -18.62759615963271287, 32.08224293864769550 ) ) ;
#103132=CARTESIAN_POINT ( 'NONE',  ( -14.34966873604960291, -8.224510206698953496, 86.66557627198102409 ) ) ;
#103133=CARTESIAN_POINT ( 'NONE',  ( 16.51473224551069308, 9.474510206698969483, 44.16557627198103120 ) ) ;
#103134=CARTESIAN_POINT ( 'NONE',  ( 0.05219959533910956823, 16.53943276465976808, 99.99890960531436690 ) ) ;
#103135=CARTESIAN_POINT ( 'NONE',  ( -18.62759615963270932, 10.81492255796079327, 110.8322429386476955 ) ) ;
#103136=CARTESIAN_POINT ( 'NONE',  ( 18.62759615963255655, 10.81492255796105972, 66.66775706135234714 ) ) ;
#103137=CARTESIAN_POINT ( 'NONE',  ( -19.03943276465977164, 0.05219959533909376836, 31.24890960531435979 ) ) ;
#103138=CARTESIAN_POINT ( 'NONE',  ( -16.53943276465976808, -0.05219959533934237506, 68.75109039468568994 ) ) ;
#103139=CARTESIAN_POINT ( 'NONE',  ( -21.55341960407610458, -5.719274019375992779, 101.4572429386476955 ) ) ;
#103140=CARTESIAN_POINT ( 'NONE',  ( 15.72974639402199770, -15.80617190586745480, 113.1239096053143953 ) ) ;
#103141=CARTESIAN_POINT ( 'NONE',  ( -13.89961937509957401, -13.97604488694547875, 39.37609039468566152 ) ) ;
#103142=CARTESIAN_POINT ( 'NONE',  ( -19.02544592524342804, 5.153800228976336051, 51.04057627198103120 ) ) ;
#103143=CARTESIAN_POINT ( 'NONE',  ( 19.05341960407611168, 5.049401038298154454, 113.9572429386477097 ) ) ;
#103144=CARTESIAN_POINT ( 'NONE',  ( -21.53943276465977519, -0.05219959533937600094, 63.75109039468568284 ) ) ;
#103145=EDGE_CURVE ( 'NONE', #16134, #133123, #88819, .T. ) ;
#103146=CARTESIAN_POINT ( 'NONE',  ( 10.81492255796078972, 18.62759615963270932, 59.58224293864770260 ) ) ;
#103147=CARTESIAN_POINT ( 'NONE',  ( -16.52544592524342804, 4.483927247898546575, 41.04057627198103120 ) ) ;
#103148=CARTESIAN_POINT ( 'NONE',  ( 21.52544592524334988, 5.823673210054432836, 71.45942372801901854 ) ) ;
#103149=CARTESIAN_POINT ( 'NONE',  ( 0.05219959533937995610, -21.53943276465977519, 105.0010903946856757 ) ) ;
#103150=CARTESIAN_POINT ( 'NONE',  ( 16.55341960407611168, 4.379528057220329451, 63.95724293864770260 ) ) ;
#103151=CARTESIAN_POINT ( 'NONE',  ( -14.34966873604960291, -8.224510206698953496, 106.6655762719810383 ) ) ;
#103152=CARTESIAN_POINT ( 'NONE',  ( 16.46253265017146816, 9.564922557961045513, 41.66775706135234003 ) ) ;
#103153=CARTESIAN_POINT ( 'NONE',  ( 14.29746914071037800, 8.314922557961029526, 101.6677570613523613 ) ) ;
#103154=CARTESIAN_POINT ( 'NONE',  ( 10.72451020669871369, 18.67979575497193778, 72.08442372801899012 ) ) ;
#103155=CARTESIAN_POINT ( 'NONE',  ( 5.049401038298161559, -19.05341960407611168, 57.70724293864769550 ) ) ;
#103156=CARTESIAN_POINT ( 'NONE',  ( -19.05341960407617563, 5.049401038297882671, 33.54275706135231871 ) ) ;
#103157=CARTESIAN_POINT ( 'NONE',  ( 18.62759615963271287, -10.81492255796078972, 38.33224293864768839 ) ) ;
#103158=CARTESIAN_POINT ( 'NONE',  ( -5.823673210054431948, 21.52544592524334988, 27.70942372801901854 ) ) ;
#103160=CARTESIAN_POINT ( 'NONE',  ( 15.80617190586746368, 15.72974639402197994, 84.37390960531438111 ) ) ;
#103161=CARTESIAN_POINT ( 'NONE',  ( 19.05341960407617918, -5.049401038297876454, 91.04275706135234714 ) ) ;
#103162=CARTESIAN_POINT ( 'NONE',  ( -8.314922557961024197, 14.29746914071037800, 52.91775706135235424 ) ) ;
#103163=CARTESIAN_POINT ( 'NONE',  ( 17.49999999999999289, -3.341627039121392695, 37.07768976001553085 ) ) ;
#103164=CARTESIAN_POINT ( 'NONE',  ( -21.53943276465977519, 0.05219959533907696930, 91.24890960531436690 ) ) ;
#103165=CARTESIAN_POINT ( 'NONE',  ( -4.379528057220328563, 16.55341960407611168, 80.20724293864769550 ) ) ;
#103166=CARTESIAN_POINT ( 'NONE',  ( -17.31747979337947285, -6.344076630961058783, 101.3794486806517909 ) ) ;
#103167=CARTESIAN_POINT ( 'NONE',  ( 16.55341960407618274, -4.379528057220086978, 26.04275706135235779 ) ) ;
#103168=CARTESIAN_POINT ( 'NONE',  ( -10.81492255796078084, -18.62759615963271287, 42.08224293864769550 ) ) ;
#103169=CARTESIAN_POINT ( 'NONE',  ( -16.55341960407617563, 4.379528057220093196, 73.54275706135234714 ) ) ;
#103170=CARTESIAN_POINT ( 'NONE',  ( 16.46253265017160672, -9.564922557960803928, 23.33224293864769194 ) ) ;
#103171=CARTESIAN_POINT ( 'NONE',  ( 4.379528057220092307, 16.55341960407617563, 57.29275706135234714 ) ) ;
#103172=CARTESIAN_POINT ( 'NONE',  ( 5.823673210054444382, -21.52544592524334988, 25.20942372801901854 ) ) ;
#103173=CARTESIAN_POINT ( 'NONE',  ( -18.62759615963270932, 10.81492255796079327, 45.83224293864769550 ) ) ;
#103174=CARTESIAN_POINT ( 'NONE',  ( 8.314922557961029526, -14.29746914071037800, 70.41775706135236135 ) ) ;
#103175=CARTESIAN_POINT ( 'NONE',  ( 13.97604488694527802, 13.89961937509977652, 84.37390960531433848 ) ) ;
#103176=CARTESIAN_POINT ( 'NONE',  ( 10.72451020669871369, 18.67979575497193778, 62.08442372801901143 ) ) ;
#103177=CARTESIAN_POINT ( 'NONE',  ( -0.05219959533909027116, -19.03943276465977164, 22.49890960531436690 ) ) ;
#103178=CARTESIAN_POINT ( 'NONE',  ( 21.53943276465977519, -0.05219959533907433946, 38.74890960531435979 ) ) ;
#103179=CARTESIAN_POINT ( 'NONE',  ( 19.03943276465977164, -0.05219959533909143690, 113.7489096053143669 ) ) ;
#103181=CARTESIAN_POINT ( 'NONE',  ( 19.05341960407617918, -5.049401038297876454, 36.04275706135234003 ) ) ;
#103182=CARTESIAN_POINT ( 'NONE',  ( 12.14591786802327356, -12.06949235617739191, 45.62609039468567573 ) ) ;
#103183=CARTESIAN_POINT ( 'NONE',  ( -0.05219959533907301413, -21.53943276465977519, 22.49890960531436335 ) ) ;
#103185=CARTESIAN_POINT ( 'NONE',  ( -16.51473224551069308, -9.474510206698971260, 91.66557627198103830 ) ) ;
#103186=CARTESIAN_POINT ( 'NONE',  ( -12.14591786802326823, 12.06949235617739902, 98.12609039468570415 ) ) ;
#103188=CARTESIAN_POINT ( 'NONE',  ( 12.14591786802309770, 12.06949235617756955, 89.37390960531435269 ) ) ;
#103189=CARTESIAN_POINT ( 'NONE',  ( 21.55341960407610458, 5.719274019375980345, 48.95724293864770971 ) ) ;
#103190=CARTESIAN_POINT ( 'NONE',  ( -0.05219959533909027116, -19.03943276465977164, 32.49890960531435979 ) ) ;
#103191=CARTESIAN_POINT ( 'NONE',  ( -4.483927247898782831, 16.52544592524335698, 72.70942372801901854 ) ) ;
#103192=CARTESIAN_POINT ( 'NONE',  ( -18.62759615963255300, -10.81492255796106328, 24.16775706135235424 ) ) ;
#103193=CARTESIAN_POINT ( 'NONE',  ( -9.474510206698720793, -16.51473224551083518, 94.58442372801900433 ) ) ;
#103194=CARTESIAN_POINT ( 'NONE',  ( -13.89961937509977652, 13.97604488694528158, 35.62390960531435269 ) ) ;
#103196=CARTESIAN_POINT ( 'NONE',  ( -19.02544592524342804, 5.153800228976336051, 111.0405762719810099 ) ) ;
#103197=CARTESIAN_POINT ( 'NONE',  ( -10.72451020669870658, -18.67979575497194134, 99.58442372801900433 ) ) ;
#103198=CARTESIAN_POINT ( 'NONE',  ( -19.05341960407611168, -5.049401038298163336, 71.45724293864766707 ) ) ;
#103199=CARTESIAN_POINT ( 'NONE',  ( 12.14591786802327356, -12.06949235617739191, 65.62609039468568994 ) ) ;
#103200=CARTESIAN_POINT ( 'NONE',  ( -18.62759615963255300, -10.81492255796106328, 89.16775706135236135 ) ) ;
#103201=CARTESIAN_POINT ( 'NONE',  ( -19.05341960407617563, 5.049401038297882671, 58.54275706135234003 ) ) ;
#103202=CARTESIAN_POINT ( 'NONE',  ( 16.51473224551083163, -9.474510206698727899, 55.83442372801899722 ) ) ;
#103204=CARTESIAN_POINT ( 'NONE',  ( 10.72451020669871369, 18.67979575497193778, 52.08442372801901854 ) ) ;
#103205=CARTESIAN_POINT ( 'NONE',  ( -18.22780087662121673, -5.500000000000062172, 56.48459894673892734 ) ) ;
#103206=CARTESIAN_POINT ( 'NONE',  ( 16.51473224551083163, -9.474510206698727899, 50.83442372801899722 ) ) ;
#103207=CARTESIAN_POINT ( 'NONE',  ( 19.03943276465977164, -0.05219959533909143690, 98.74890960531436690 ) ) ;
#103208=CARTESIAN_POINT ( 'NONE',  ( 16.46253265017160672, -9.564922557960803928, 88.33224293864769550 ) ) ;
#103209=CARTESIAN_POINT ( 'NONE',  ( -4.379528057220328563, 16.55341960407611168, 35.20724293864768839 ) ) ;
#103210=CARTESIAN_POINT ( 'NONE',  ( -21.53943276465977519, 0.05219959533907696930, 36.24890960531435979 ) ) ;
#103213=CARTESIAN_POINT ( 'NONE',  ( -5.719274019375665041, -21.55341960407619695, 109.7927570613523613 ) ) ;
#103215=CARTESIAN_POINT ( 'NONE',  ( -13.97604488694527625, -13.89961937509977652, 31.87390960531435979 ) ) ;
#103216=CARTESIAN_POINT ( 'NONE',  ( 19.03943276465977164, -0.05219959533909143690, 28.74890960531435624 ) ) ;
#103219=CARTESIAN_POINT ( 'NONE',  ( 12.14591786802327356, -12.06949235617739191, 65.62609039468568994 ) ) ;
#103220=CARTESIAN_POINT ( 'NONE',  ( -18.67979575497178146, -10.72451020669898902, 86.66557627198102409 ) ) ;
#103221=CARTESIAN_POINT ( 'NONE',  ( -14.29746914071049879, 8.314922557960819915, 55.83224293864770260 ) ) ;
#103222=CARTESIAN_POINT ( 'NONE',  ( -0.05219959533909027116, -19.03943276465977164, 22.49890960531436690 ) ) ;
#103223=CARTESIAN_POINT ( 'NONE',  ( -9.474510206698964154, 16.51473224551069663, 105.4155762719810383 ) ) ;
#103224=CARTESIAN_POINT ( 'NONE',  ( 15.80617190586769283, -15.72974639402175789, 25.62609039468567929 ) ) ;
#103225=CARTESIAN_POINT ( 'NONE',  ( 13.97604488694548053, -13.89961937509957401, 30.62609039468566863 ) ) ;
#103226=CARTESIAN_POINT ( 'NONE',  ( 16.46253265017160672, -9.564922557960803928, 28.33224293864769550 ) ) ;
#103227=CARTESIAN_POINT ( 'NONE',  ( -15.72974639402176322, -15.80617190586768395, 79.37609039468567573 ) ) ;
#103228=CARTESIAN_POINT ( 'NONE',  ( -17.49999999999999645, 5.499999999999992895, 48.71769037696437010 ) ) ;
#103229=CARTESIAN_POINT ( 'NONE',  ( 4.379528057220339221, -16.55341960407611168, 27.70724293864769905 ) ) ;
#103230=CARTESIAN_POINT ( 'NONE',  ( 17.49999999999999645, 3.805241302050201391, 112.1264752721741758 ) ) ;
#103231=CARTESIAN_POINT ( 'NONE',  ( -21.53943276465977519, 0.05219959533907696930, 46.24890960531435979 ) ) ;
#103232=CARTESIAN_POINT ( 'NONE',  ( -14.29746914071049879, 8.314922557960819915, 100.8322429386477097 ) ) ;
#103234=CARTESIAN_POINT ( 'NONE',  ( 13.89961937509977652, -13.97604488694527269, 93.12390960531436690 ) ) ;
#103235=CARTESIAN_POINT ( 'NONE',  ( -4.379528057220328563, 16.55341960407611168, 95.20724293864769550 ) ) ;
#103236=CARTESIAN_POINT ( 'NONE',  ( 5.049401038297881783, 19.05341960407617563, 102.2927570613523045 ) ) ;
#103237=CARTESIAN_POINT ( 'NONE',  ( -18.67979575497178146, -10.72451020669898902, 61.66557627198103120 ) ) ;
#103240=CARTESIAN_POINT ( 'NONE',  ( -19.05341960407611168, -5.049401038298163336, 26.45724293864769550 ) ) ;
#103241=CARTESIAN_POINT ( 'NONE',  ( 5.049401038298161559, -19.05341960407611168, 87.70724293864769550 ) ) ;
#103242=CARTESIAN_POINT ( 'NONE',  ( 5.823673210054125526, 21.52544592524343514, 89.79057627198103830 ) ) ;
#103243=CARTESIAN_POINT ( 'NONE',  ( 0.05219959533934541429, -16.53943276465976808, 105.0010903946856757 ) ) ;
#103244=CARTESIAN_POINT ( 'NONE',  ( 13.97604488694527802, 13.89961937509977652, 89.37390960531436690 ) ) ;
#103245=CARTESIAN_POINT ( 'NONE',  ( 19.05341960407617918, -5.049401038297876454, 81.04275706135231871 ) ) ;
#103246=CARTESIAN_POINT ( 'NONE',  ( 18.67979575497194134, -10.72451020669871369, 100.8344237280190185 ) ) ;
#103247=CARTESIAN_POINT ( 'NONE',  ( -10.81492255796078084, -18.62759615963271287, 72.08224293864769550 ) ) ;
#103248=CARTESIAN_POINT ( 'NONE',  ( -21.55341960407610458, -5.719274019375992779, 36.45724293864768839 ) ) ;
#103249=CARTESIAN_POINT ( 'NONE',  ( -13.89961937509977652, 13.97604488694528158, 55.62390960531434558 ) ) ;
#103250=CARTESIAN_POINT ( 'NONE',  ( -14.34966873604972548, 8.224510206698743886, 108.3344237280190185 ) ) ;
#103251=CARTESIAN_POINT ( 'NONE',  ( 16.51473224551069308, 9.474510206698969483, 64.16557627198102409 ) ) ;
#103254=CARTESIAN_POINT ( 'NONE',  ( -16.46253265017146816, -9.564922557961047289, 29.16775706135232937 ) ) ;
#103255=CARTESIAN_POINT ( 'NONE',  ( 12.06949235617757843, -12.14591786802309237, 68.12390960531436690 ) ) ;
#103256=CARTESIAN_POINT ( 'NONE',  ( -10.72451020669898014, 18.67979575497178502, 115.4155762719810241 ) ) ;
#103258=CARTESIAN_POINT ( 'NONE',  ( -21.52544592524343514, 5.823673210054127303, 66.04057627198103830 ) ) ;
#103259=CARTESIAN_POINT ( 'NONE',  ( -12.06949235617739369, -12.14591786802326823, 94.37609039468568994 ) ) ;
#103260=CARTESIAN_POINT ( 'NONE',  ( -14.34966873604960291, -8.224510206698953496, 106.6655762719810383 ) ) ;
#103261=CARTESIAN_POINT ( 'NONE',  ( -9.564922557960796823, -16.46253265017161027, 72.08224293864770971 ) ) ;
#103263=CARTESIAN_POINT ( 'NONE',  ( 8.314922557960818139, 14.29746914071049879, 24.58224293864768839 ) ) ;
#103265=CARTESIAN_POINT ( 'NONE',  ( -21.53943276465977519, -0.05219959533937600094, 43.75109039468568284 ) ) ;
#103266=CARTESIAN_POINT ( 'NONE',  ( -16.46253265017160317, 9.564922557960807481, 110.8322429386476955 ) ) ;
#103267=CARTESIAN_POINT ( 'NONE',  ( 21.53943276465977519, 0.05219959533937863772, 86.25109039468568994 ) ) ;
#103268=CARTESIAN_POINT ( 'NONE',  ( -5.153800228976328057, -19.02544592524343514, 32.29057627198102409 ) ) ;
#103269=CARTESIAN_POINT ( 'NONE',  ( -5.153800228976328057, -19.02544592524343514, 37.29057627198102409 ) ) ;
#103271=CARTESIAN_POINT ( 'NONE',  ( 21.55341960407619695, -5.719274019375665929, 101.0427570613523756 ) ) ;
#103272=CARTESIAN_POINT ( 'NONE',  ( -8.224510206698735004, -14.34966873604973081, 44.58442372801901854 ) ) ;
#103273=CARTESIAN_POINT ( 'NONE',  ( -5.719274019375665041, -21.55341960407619695, 74.79275706135234714 ) ) ;
#103274=CARTESIAN_POINT ( 'NONE',  ( 13.89961937509977652, -13.97604488694527269, 98.12390960531433848 ) ) ;
#103275=CARTESIAN_POINT ( 'NONE',  ( -9.474510206698720793, -16.51473224551083518, 84.58442372801900433 ) ) ;
#103276=CARTESIAN_POINT ( 'NONE',  ( -18.67979575497193778, 10.72451020669871902, 58.33442372801901143 ) ) ;
#103277=CARTESIAN_POINT ( 'NONE',  ( 9.474510206698729675, 16.51473224551082808, 112.0844237280190043 ) ) ;
#103278=CARTESIAN_POINT ( 'NONE',  ( -19.03943276465977164, -0.05219959533935918106, 88.75109039468567573 ) ) ;
#103279=CARTESIAN_POINT ( 'NONE',  ( -13.89961937509977652, 13.97604488694528158, 45.62390960531433848 ) ) ;
#103280=CARTESIAN_POINT ( 'NONE',  ( 16.51473224551083163, -9.474510206698727899, 90.83442372801900433 ) ) ;
#103281=CARTESIAN_POINT ( 'NONE',  ( -12.14591786802309592, -12.06949235617757132, 26.87390960531435979 ) ) ;
#103282=CARTESIAN_POINT ( 'NONE',  ( 13.89961937509957401, 13.97604488694547697, 86.87609039468567573 ) ) ;
#103283=CARTESIAN_POINT ( 'NONE',  ( -14.29746914071049879, 8.314922557960819915, 45.83224293864769550 ) ) ;
#103284=CARTESIAN_POINT ( 'NONE',  ( 13.89961937509957401, 13.97604488694547697, 66.87609039468567573 ) ) ;
#103285=CARTESIAN_POINT ( 'NONE',  ( 0.05219959533934541429, -16.53943276465976808, 50.00109039468568994 ) ) ;
#103286=CARTESIAN_POINT ( 'NONE',  ( -19.05341960407617563, 5.049401038297882671, 28.54275706135232937 ) ) ;
#103287=CARTESIAN_POINT ( 'NONE',  ( -5.153800228976328057, -19.02544592524343514, 27.29057627198103120 ) ) ;
#103288=CARTESIAN_POINT ( 'NONE',  ( -13.97604488694527625, -13.89961937509977652, 46.87390960531435979 ) ) ;
#103289=CARTESIAN_POINT ( 'NONE',  ( -14.34966873604972548, 8.224510206698743886, 43.33442372801901143 ) ) ;
#103292=CARTESIAN_POINT ( 'NONE',  ( -13.97604488694527625, -13.89961937509977652, 86.87390960531436690 ) ) ;
#103295=CARTESIAN_POINT ( 'NONE',  ( 13.97604488694548053, -13.89961937509957401, 100.6260903946856615 ) ) ;
#103296=VECTOR ( 'NONE', #108279, 1000.000000000000000 ) ;
#103297=CARTESIAN_POINT ( 'NONE',  ( 5.719274019375991003, -21.55341960407610458, 27.70724293864769905 ) ) ;
#103298=CARTESIAN_POINT ( 'NONE',  ( 0.05219959533936267826, -19.03943276465977164, 35.00109039468566863 ) ) ;
#103299=CARTESIAN_POINT ( 'NONE',  ( 19.03943276465977164, 0.05219959533936151252, 106.2510903946856615 ) ) ;
#103300=CARTESIAN_POINT ( 'NONE',  ( -16.52544592524342804, 4.483927247898546575, 111.0405762719810525 ) ) ;
#103301=CARTESIAN_POINT ( 'NONE',  ( 5.049401038298161559, -19.05341960407611168, 37.70724293864768839 ) ) ;
#103302=CARTESIAN_POINT ( 'NONE',  ( 5.719274019375991003, -21.55341960407610458, 77.70724293864770971 ) ) ;
#103303=CARTESIAN_POINT ( 'NONE',  ( 5.049401038298161559, -19.05341960407611168, 42.70724293864767418 ) ) ;
#103305=CARTESIAN_POINT ( 'NONE',  ( -13.97604488694547697, 13.89961937509957934, 68.12609039468563310 ) ) ;
#103306=CARTESIAN_POINT ( 'NONE',  ( -16.55341960407611168, -4.379528057220339221, 56.45724293864768839 ) ) ;
#103307=CARTESIAN_POINT ( 'NONE',  ( -18.67979575497178146, -10.72451020669898902, 36.66557627198103120 ) ) ;
#103308=CARTESIAN_POINT ( 'NONE',  ( 5.719274019375673035, 21.55341960407619339, 97.29275706135234714 ) ) ;
#103309=CARTESIAN_POINT ( 'NONE',  ( -0.05219959533907301413, -21.53943276465977519, 82.49890960531436690 ) ) ;
#103310=CARTESIAN_POINT ( 'NONE',  ( -15.72974639402176322, -15.80617190586768395, 69.37609039468567573 ) ) ;
#103311=CARTESIAN_POINT ( 'NONE',  ( 18.67979575497194134, -10.72451020669871369, 70.83442372801901854 ) ) ;
#103312=CARTESIAN_POINT ( 'NONE',  ( -13.89961937509977652, 13.97604488694528158, 90.62390960531432427 ) ) ;
#103313=CARTESIAN_POINT ( 'NONE',  ( -12.06949235617739369, -12.14591786802326823, 89.37609039468568994 ) ) ;
#103314=CARTESIAN_POINT ( 'NONE',  ( -18.62759615963255300, -10.81492255796106328, 69.16775706135234714 ) ) ;
#103315=CARTESIAN_POINT ( 'NONE',  ( 5.049401038298161559, -19.05341960407611168, 52.70724293864767418 ) ) ;
#103316=CARTESIAN_POINT ( 'NONE',  ( 10.72451020669871369, 18.67979575497193778, 27.08442372801901854 ) ) ;
#103317=CARTESIAN_POINT ( 'NONE',  ( 19.05341960407611168, 5.049401038298154454, 73.95724293864768129 ) ) ;
#103318=CARTESIAN_POINT ( 'NONE',  ( -14.29746914071049879, 8.314922557960819915, 75.83224293864769550 ) ) ;
#103319=CARTESIAN_POINT ( 'NONE',  ( 16.53943276465976808, -0.05219959533910856209, 43.74890960531435979 ) ) ;
#103320=CARTESIAN_POINT ( 'NONE',  ( -0.05219959533907301413, -21.53943276465977519, 57.49890960531435979 ) ) ;
#103321=CARTESIAN_POINT ( 'NONE',  ( -5.153800228976328057, -19.02544592524343514, 42.29057627198101699 ) ) ;
#103322=CARTESIAN_POINT ( 'NONE',  ( 15.72974639402199770, -15.80617190586745480, 63.12390960531435979 ) ) ;
#103323=CARTESIAN_POINT ( 'NONE',  ( 13.89961937509957401, 13.97604488694547697, 46.87609039468565442 ) ) ;
#103324=CARTESIAN_POINT ( 'NONE',  ( -19.03943276465977164, -0.05219959533935946555, 18.75109039468567218 ) ) ;
#103325=CARTESIAN_POINT ( 'NONE',  ( 16.52544592524342804, -4.483927247898539470, 68.54057627198103830 ) ) ;
#103326=CARTESIAN_POINT ( 'NONE',  ( 5.823673210054125526, 21.52544592524343514, 34.79057627198103120 ) ) ;
#103329=CARTESIAN_POINT ( 'NONE',  ( 17.50000000000000355, 5.499999999999989342, 103.7823096230356867 ) ) ;
#103330=CARTESIAN_POINT ( 'NONE',  ( 12.14591786802327356, -12.06949235617739191, 85.62609039468568994 ) ) ;
#103331=CARTESIAN_POINT ( 'NONE',  ( -5.153800228976607833, 19.02544592524334988, 92.70942372801901854 ) ) ;
#103332=CARTESIAN_POINT ( 'NONE',  ( -12.14591786802309592, -12.06949235617757132, 56.87390960531436690 ) ) ;
#103334=CARTESIAN_POINT ( 'NONE',  ( 9.474510206698971260, -16.51473224551069308, 52.91557627198102409 ) ) ;
#103335=CARTESIAN_POINT ( 'NONE',  ( 12.14591786802309770, 12.06949235617756955, 39.37390960531436690 ) ) ;
#103336=CARTESIAN_POINT ( 'NONE',  ( 19.02544592524343514, -5.153800228976328945, 73.54057627198103830 ) ) ;
#103337=CARTESIAN_POINT ( 'NONE',  ( -0.05219959533909027116, -19.03943276465977164, 47.49890960531435979 ) ) ;
#103338=CARTESIAN_POINT ( 'NONE',  ( -10.72451020669870658, -18.67979575497194134, 64.58442372801900433 ) ) ;
#103339=CARTESIAN_POINT ( 'NONE',  ( 19.02544592524343514, -5.153800228976328945, 68.54057627198103830 ) ) ;
#103340=CARTESIAN_POINT ( 'NONE',  ( 16.46253265017160672, -9.564922557960803928, 23.33224293864769194 ) ) ;
#103341=CARTESIAN_POINT ( 'NONE',  ( 5.049401038298161559, -19.05341960407611168, 62.70724293864769550 ) ) ;
#103343=CARTESIAN_POINT ( 'NONE',  ( -5.719274019375978568, 21.55341960407610458, 55.20724293864770260 ) ) ;
#103344=CARTESIAN_POINT ( 'NONE',  ( -0.05219959533909027116, -19.03943276465977164, 32.49890960531435979 ) ) ;
#103345=CARTESIAN_POINT ( 'NONE',  ( -5.823673210054116645, -21.52544592524344225, 42.29057627198103120 ) ) ;
#103346=CARTESIAN_POINT ( 'NONE',  ( 14.34966873604972726, -8.224510206698740333, 100.8344237280190185 ) ) ;
#103347=CARTESIAN_POINT ( 'NONE',  ( -10.81492255796105439, 18.62759615963255655, 112.9177570613523329 ) ) ;
#103348=CARTESIAN_POINT ( 'NONE',  ( 14.34966873604972726, -8.224510206698740333, 40.83442372801901854 ) ) ;
#103349=CARTESIAN_POINT ( 'NONE',  ( 16.55341960407618274, -4.379528057220086978, 76.04275706135237556 ) ) ;
#103352=CARTESIAN_POINT ( 'NONE',  ( 14.29746914071037800, 8.314922557961029526, 66.66775706135234714 ) ) ;
#103353=CARTESIAN_POINT ( 'NONE',  ( 4.483927247898790824, -16.52544592524335698, 60.20942372801902565 ) ) ;
#103354=CARTESIAN_POINT ( 'NONE',  ( 19.05341960407611168, 5.049401038298154454, 113.9572429386477097 ) ) ;
#103355=CARTESIAN_POINT ( 'NONE',  ( 19.03943276465977164, -0.05219959533909143690, 38.74890960531436690 ) ) ;
#103356=CARTESIAN_POINT ( 'NONE',  ( -4.483927247898782831, 16.52544592524335698, 42.70942372801901854 ) ) ;
#103357=CARTESIAN_POINT ( 'NONE',  ( 0.05219959533909260263, 19.03943276465977164, 49.99890960531435979 ) ) ;
#103358=CARTESIAN_POINT ( 'NONE',  ( 21.55341960407619695, -5.719274019375665929, 21.04275706135234714 ) ) ;
#103359=CARTESIAN_POINT ( 'NONE',  ( -14.34966873604972548, 8.224510206698743886, 33.33442372801900433 ) ) ;
#103360=CARTESIAN_POINT ( 'NONE',  ( -4.483927247898782831, 16.52544592524335698, 97.70942372801904696 ) ) ;
#103361=CARTESIAN_POINT ( 'NONE',  ( -16.51473224551069308, -9.474510206698971260, 21.66557627198102765 ) ) ;
#103362=CARTESIAN_POINT ( 'NONE',  ( 21.55341960407619695, -5.719274019375665929, 101.0427570613523756 ) ) ;
#103363=CARTESIAN_POINT ( 'NONE',  ( 19.02544592524334988, 5.153800228976608722, 101.4594237280189759 ) ) ;
#103364=CARTESIAN_POINT ( 'NONE',  ( -16.55341960407611168, -4.379528057220339221, 51.45724293864770260 ) ) ;
#103365=CARTESIAN_POINT ( 'NONE',  ( -5.049401038298153566, 19.05341960407611168, 30.20724293864768839 ) ) ;
#103366=CARTESIAN_POINT ( 'NONE',  ( 16.51473224551083163, -9.474510206698727899, 65.83442372801900433 ) ) ;
#103368=CARTESIAN_POINT ( 'NONE',  ( -15.72974639402176322, -15.80617190586768395, 69.37609039468567573 ) ) ;
#103369=CARTESIAN_POINT ( 'NONE',  ( 16.52544592524335698, 4.483927247898782831, 21.45942372801901499 ) ) ;
#103370=CARTESIAN_POINT ( 'NONE',  ( 16.52216118717206683, 7.221426719304520070, 83.57599021046989662 ) ) ;
#103371=CARTESIAN_POINT ( 'NONE',  ( 13.97604488694527802, 13.89961937509977652, 114.3739096053143669 ) ) ;
#103372=CARTESIAN_POINT ( 'NONE',  ( 0.05219959533936267826, -19.03943276465977164, 110.0010903946856757 ) ) ;
#103375=CARTESIAN_POINT ( 'NONE',  ( -0.05219959533909027116, -19.03943276465977164, 22.49890960531436690 ) ) ;
#103376=CARTESIAN_POINT ( 'NONE',  ( -5.823673210054431948, 21.52544592524334988, 112.7094237280190328 ) ) ;
#103377=CARTESIAN_POINT ( 'NONE',  ( -16.51473224551069308, -9.474510206698971260, 36.66557627198102409 ) ) ;
#103378=CARTESIAN_POINT ( 'NONE',  ( 21.55341960407619695, -5.719274019375665929, 46.04275706135234714 ) ) ;
#103379=CARTESIAN_POINT ( 'NONE',  ( -21.55341960407619339, 5.719274019375674811, 98.54275706135234714 ) ) ;
#103380=CARTESIAN_POINT ( 'NONE',  ( -14.29746914071037622, -8.314922557961029526, 104.1677570613523471 ) ) ;
#103381=CARTESIAN_POINT ( 'NONE',  ( -5.049401038298153566, 19.05341960407611168, 85.20724293864766707 ) ) ;
#103382=CARTESIAN_POINT ( 'NONE',  ( 5.823673210054444382, -21.52544592524334988, 60.20942372801902565 ) ) ;
#103383=CARTESIAN_POINT ( 'NONE',  ( -0.05219959533937732626, 21.53943276465977519, 47.50109039468568994 ) ) ;
#103384=CARTESIAN_POINT ( 'NONE',  ( 5.153800228976615827, -19.02544592524334988, 75.20942372801896170 ) ) ;
#103385=CARTESIAN_POINT ( 'NONE',  ( -19.05341960407611168, -5.049401038298163336, 91.45724293864766707 ) ) ;
#103386=CARTESIAN_POINT ( 'NONE',  ( 16.55341960407611168, 4.379528057220329451, 113.9572429386477239 ) ) ;
#103387=CARTESIAN_POINT ( 'NONE',  ( 21.52544592524344225, -5.823673210054117533, 98.54057627198105251 ) ) ;
#103388=CARTESIAN_POINT ( 'NONE',  ( 16.46253265017146816, 9.564922557961045513, 26.66775706135234003 ) ) ;
#103389=CARTESIAN_POINT ( 'NONE',  ( -12.14591786802309592, -12.06949235617757132, 101.8739096053143811 ) ) ;
#103390=CARTESIAN_POINT ( 'NONE',  ( 5.153800228976335163, 19.02544592524342804, 54.79057627198103120 ) ) ;
#103391=CARTESIAN_POINT ( 'NONE',  ( 13.89961937509957401, 13.97604488694547697, 81.87609039468564731 ) ) ;
#103392=CARTESIAN_POINT ( 'NONE',  ( 12.14591786802309770, 12.06949235617756955, 54.37390960531435979 ) ) ;
#103393=CARTESIAN_POINT ( 'NONE',  ( 21.55341960407619695, -5.719274019375665929, 106.0427570613523471 ) ) ;
#103394=CARTESIAN_POINT ( 'NONE',  ( 16.51473224551069308, 9.474510206698969483, 109.1655762719810383 ) ) ;
#103395=CARTESIAN_POINT ( 'NONE',  ( 5.049401038297881783, 19.05341960407617563, 72.29275706135234714 ) ) ;
#103396=CARTESIAN_POINT ( 'NONE',  ( 21.53943276465977519, -0.05219959533907433946, 73.74890960531433848 ) ) ;
#103397=CARTESIAN_POINT ( 'NONE',  ( -5.823673210054431948, 21.52544592524334988, 32.70942372801900433 ) ) ;
#103398=CARTESIAN_POINT ( 'NONE',  ( -12.14591786802326823, 12.06949235617739902, 28.12609039468568284 ) ) ;
#103399=CARTESIAN_POINT ( 'NONE',  ( -14.29746914071037622, -8.314922557961029526, 94.16775706135237556 ) ) ;
#103400=CARTESIAN_POINT ( 'NONE',  ( 19.05341960407611168, 5.049401038298154454, 28.95724293864769550 ) ) ;
#103401=CARTESIAN_POINT ( 'NONE',  ( 18.67979575497194134, -10.72451020669871369, 30.83442372801902209 ) ) ;
#103402=CARTESIAN_POINT ( 'NONE',  ( -15.80617190586745835, -15.72974639402198527, 46.87390960531435979 ) ) ;
#103403=CARTESIAN_POINT ( 'NONE',  ( 19.05341960407611168, 5.049401038298154454, 23.95724293864769194 ) ) ;
#103405=CARTESIAN_POINT ( 'NONE',  ( -0.05219959533934338120, 16.53943276465976808, 67.50109039468568994 ) ) ;
#103406=CARTESIAN_POINT ( 'NONE',  ( -8.314922557960811034, -14.29746914071050412, 92.08224293864769550 ) ) ;
#103407=CARTESIAN_POINT ( 'NONE',  ( -21.55341960407610458, -5.719274019375992779, 86.45724293864770971 ) ) ;
#103408=CARTESIAN_POINT ( 'NONE',  ( -8.314922557961024197, 14.29746914071037800, 112.9177570613523329 ) ) ;
#103409=CARTESIAN_POINT ( 'NONE',  ( 16.53943276465976808, 0.05219959533934440121, 51.25109039468568994 ) ) ;
#103410=CARTESIAN_POINT ( 'NONE',  ( 19.03943276465977164, -0.05219959533909143690, 63.74890960531435979 ) ) ;
#103411=CARTESIAN_POINT ( 'NONE',  ( -4.483927247898782831, 16.52544592524335698, 87.70942372801901854 ) ) ;
#103412=CARTESIAN_POINT ( 'NONE',  ( 5.049401038297881783, 19.05341960407617563, 92.29275706135234714 ) ) ;
#103413=CARTESIAN_POINT ( 'NONE',  ( 5.823673210054125526, 21.52544592524343514, 84.79057627198102409 ) ) ;
#103414=CARTESIAN_POINT ( 'NONE',  ( 16.53943276465976808, 0.05219959533934440121, 106.2510903946856757 ) ) ;
#103417=CARTESIAN_POINT ( 'NONE',  ( 21.52544592524344225, -5.823673210054117533, 63.54057627198103830 ) ) ;
#103418=CARTESIAN_POINT ( 'NONE',  ( -0.05219959533934338120, 16.53943276465976808, 92.50109039468567573 ) ) ;
#103420=CARTESIAN_POINT ( 'NONE',  ( -5.823673210054116645, -21.52544592524344225, 37.29057627198102409 ) ) ;
#103421=CARTESIAN_POINT ( 'NONE',  ( 18.22780087662121673, 5.500000000000056843, 88.98459894673892734 ) ) ;
#103422=CARTESIAN_POINT ( 'NONE',  ( -18.62759615963270932, 10.81492255796079327, 90.83224293864769550 ) ) ;
#103423=CARTESIAN_POINT ( 'NONE',  ( 16.52544592524335698, 4.483927247898782831, 111.4594237280190328 ) ) ;
#103424=CARTESIAN_POINT ( 'NONE',  ( -0.05219959533934338120, 16.53943276465976808, 32.50109039468568284 ) ) ;
#103425=CARTESIAN_POINT ( 'NONE',  ( 13.89961937509977652, -13.97604488694527269, 33.12390960531434558 ) ) ;
#103426=CARTESIAN_POINT ( 'NONE',  ( 16.52544592524335698, 4.483927247898782831, 26.45942372801901854 ) ) ;
#103427=CARTESIAN_POINT ( 'NONE',  ( -9.474510206698964154, 16.51473224551069663, 50.41557627198102409 ) ) ;
#103429=CARTESIAN_POINT ( 'NONE',  ( 0.05219959533909260263, 19.03943276465977164, 104.9989096053143669 ) ) ;
#103430=CARTESIAN_POINT ( 'NONE',  ( 13.89961937509977652, -13.97604488694527269, 113.1239096053143527 ) ) ;
#103431=CARTESIAN_POINT ( 'NONE',  ( -16.52544592524335698, -4.483927247898792601, 98.95942372801903275 ) ) ;
#103432=CARTESIAN_POINT ( 'NONE',  ( 5.153800228976615827, -19.02544592524334988, 95.20942372801897591 ) ) ;
#103433=CARTESIAN_POINT ( 'NONE',  ( -5.049401038297874678, -19.05341960407617918, 34.79275706135233293 ) ) ;
#103434=CARTESIAN_POINT ( 'NONE',  ( 10.72451020669898902, -18.67979575497178502, 72.91557627198103830 ) ) ;
#103435=CARTESIAN_POINT ( 'NONE',  ( 4.483927247898790824, -16.52544592524335698, 100.2094237280190043 ) ) ;
#103436=CARTESIAN_POINT ( 'NONE',  ( 21.52544592524344225, -5.823673210054117533, 33.54057627198102409 ) ) ;
#103437=CARTESIAN_POINT ( 'NONE',  ( 19.05341960407617918, -5.049401038297876454, 106.0427570613523471 ) ) ;
#103438=CARTESIAN_POINT ( 'NONE',  ( 5.153800228976335163, 19.02544592524342804, 104.7905762719809957 ) ) ;
#103439=CARTESIAN_POINT ( 'NONE',  ( -0.05219959533937732626, 21.53943276465977519, 62.50109039468568284 ) ) ;
#103440=CARTESIAN_POINT ( 'NONE',  ( -19.02544592524342804, 5.153800228976336051, 66.04057627198103830 ) ) ;
#103442=CARTESIAN_POINT ( 'NONE',  ( -8.314922557960811034, -14.29746914071050412, 97.08224293864770971 ) ) ;
#103444=CARTESIAN_POINT ( 'NONE',  ( -4.483927247898539470, -16.52544592524342804, 77.29057627198102409 ) ) ;
#103445=CARTESIAN_POINT ( 'NONE',  ( 18.62759615963271287, -10.81492255796078972, 73.33224293864769550 ) ) ;
#103447=CARTESIAN_POINT ( 'NONE',  ( 5.153800228976615827, -19.02544592524334988, 85.20942372801900433 ) ) ;
#103448=( BOUNDED_SURFACE ( )  B_SPLINE_SURFACE ( 3, 2, ( 
 ( #17824, #122991, #169498, #94643, #109818, #170500, #63315, #199854, #62304, #141151, #31990, #140146, #183692, #91644, #95636, #184677, #46160, #14834, #172492, #60328, #138173, #33980, #157324, #155333, #30997, #18819, #122002, #124995, #137173, #32990, #76497, #186690, #111807, #145122, #190647, #173495, #188668, #7604, #82439, #3621, #66296, #36947, #50147, #83444, #68285, #158309, #34968, #114793, #6606, #22796, #146120, #128946, #96620, #53115, #142137, #129936, #115802, #65300, #19797, #51132, #144127, #100618, #69290, #126959, #81438, #191635, #143124, #176486, #37962, #4604, #99620, #52123, #161300, #84442, #130956, #127955, #112792, #192646, #54129, #113779, #177492, #189659, #159287, #38961, #5608, #160303, #174486, #35953, #162300, #97599, #20784, #67288, #80463, #175475, #98609, #21793, #182471, #40965, #148145, #104627, #85450, #103640, #166316, #58132, #8628, #132966, #55125, #88451, #133977, #116794, #131969, #151143, #25815, #42964, #117807, #41973, #26811, #179500, #147140, #178486, #74299, #57139, #118815, #119801, #102637, #10638, #134985, #181486, #180501, #43952, #70300, #195668, #72298, #193653, #39953, #196663, #165318, #150146, #11648, #27813, #101624, #163313, #89454, #73314, #87461, #12634, #135968, #164322, #24811, #197639, #59105, #120770, #105614, #23800, #86460, #9636, #71303, #194655, #56125, #149148, #75273, #138919, #108586, #106600, #136943, #155092, #187446, #45927, #154099, #78234, #1394, #123737, #125746, #152123, #77251, #15593, #28798, #121766, #139905, #400, #185436, #170263, #109580, #90437, #198632, #47926, #62072, #169259, #46926, #93406, #61084, #44945, #31757, #16586, #64076, #63075, #124754, #168276, #186450, #48914, #171263, #13605, #30766, #60098, #32751, #94402, #29773, #183459, #156083, #167302, #137934, #17579, #79240, #140911, #91408, #2397, #153096, #14600, #76256, #184447, #199618, #122757, #107582, #92413, #176243, #190408, #126720, #37714, #82195, #21549, #189423, #127721, #144884, #175237, #66053, #141897, #7363, #4370, #159052, #67053, #128711, #142888, #192407, #51884, #3388, #50898, #112556, #174251, #35719, #161059, #157083, #98363, #99376, #160062, #188424, #69048, #22554, #97366, #130713, #20546, #191395, #110568, #113543, #143888, #5369, #34727, #172249, #84200, #33736, #36702, #83209, #6366, #68046, #49901, #129698, #52872, #114543, #145880, #96385, #65063, #19563, #95397, #18579, #80226, #111568, #173252, #158072, #81207, #9391, #177251, #8383, #104383, #87219, #148901, #88205, #103390, #131726, #149889, #74056, #118566, #38723, #117554, #162059, #25575, #195414, #193408, #23555, #41726, #135727, #24566, #180256, #165068, #11395, #100381, #10391, #40719, #102388, #85203, #71057, #166066, #27567, #164076, #89207, #119561, #133722, #70058, #181244, #72048, #26562, #132723, #194411, #73065, #134737, #55881, #146891, #150900, #147905, #56892, #196419, #57889, #86215, #53889, #42721, #54883, #179253, #12394, #115564, #116557, #178246, #39707, #101370, #163059, #46681, #75031, #155839, #62825, #14350, #17336, #184204, #77995, #78992, #158, #76015, #122514, #121522, #197398, #171017, #58864, #61827, #107337, #29533, #31511, #136697, #123497, #93164, #154849, #60839, #183217, #28557, #106352, #120530, #185190, #137690, #124508, #199375, #15350, #108340, #152855, #182223, #151877, #47685, #30514, #92166, #16346, #45686, #169010, #170021, #139662, #153852, #43707, #105369, #77006, #138678, #167056, #13367, #1150, #186203, #109335, #32508, #94160, #90194, #198378, #59855, #44698, #168036, #91166, #66808, #34494, #18341, #143643, #81951, #37475, #128471, #174998, #4134, #64829, #172010, #49661, #2158, #190167, #80980, #6129, #142655, #158815, #5126, #96152, #63836, #95158, #191166, #174011, #35482, #36463, #19332, #127482, #51643, #98120, #97131, #99136, #125509, #50660, #189187, #187206, #156846, #113307, #112321, #20303, #159817 ),
 ( #52639, #21312, #114304, #82969, #144646, #67812, #129467, #48677, #176006, #110329, #160826, #157841, #22314, #140666, #33499, #79996, #126491, #141664, #3156, #188189, #111325, #173015, #65813, #118326, #148664, #26328, #149656, #132487, #53644, #56653, #145645, #10152, #119322, #7125, #115321, #54638, #147664, #104146, #11154, #68807, #100139, #71812, #130466, #180019, #41486, #177013, #103151, #55640, #133480, #195172, #164832, #69812, #116313, #87968, #72828, #117313, #134497, #146641, #162816, #196184, #9151, #163834, #192164, #38482, #42483, #8134, #131479, #161820, #57656, #23315, #84959, #181009, #165828, #101130, #193166, #83965, #178002, #25336, #39469, #24325, #85974, #70818, #194176, #179009, #40477, #102149, #86977, #156354, #91675, #126017, #2671, #199888, #64348, #1671, #94675, #79511, #110842, #15862, #62337, #187712, #141181, #63349, #17855, #92680, #108854, #172526, #155365, #109847, #76529, #138206, #188698, #154368, #77520, #61352, #157355, #153366, #31030, #80495, #50179, #47194, #139192, #34011, #14868, #171532, #95668, #49184, #123023, #667, #184708, #18850, #140178, #46193, #107846, #142169, #32024, #3653, #185705, #169530, #65331, #170534, #93682, #124007, #16854, #78505, #125026, #33020, #186722, #48193, #126991, #111836, #27325, #159318, #51162, #112822, #34996, #7635, #175504, #191665, #20813, #161331, #69319, #68314, #96650, #177521, #52152, #130985, #190676, #127986, #160333, #158338, #113809, #83475, #146148, #100647, #23829, #53144, #147168, #192676, #54159, #115832, #114823, #19827, #38991, #81468, #131997, #36978, #162328, #37992, #84470, #143154, #82469, #129965, #4635, #176515, #22824, #174515, #66325, #85479, #99648, #8656, #70330, #21823, #189689, #193683, #35982, #55153, #173525, #97629, #144155, #5640, #145152, #67317, #128977, #98638, #6636, #136972, #87489, #42993, #27842, #74329, #163343, #73342, #103668, #165346, #24838, #134005, #167331, #90467, #26839, #28827, #182501, #196692, #132993, #43980, #88479, #89483, #195696, #57167, #151174, #181514, #72329, #148173, #13634, #10666, #150176, #135015, #58161, #149177, #198662, #119829, #9664, #118846, #180529, #42002, #11676, #152151, #86488, #104658, #105642, #166345, #194684, #75301, #116823, #12662, #178514, #135996, #197667, #39980, #59133, #120800, #101651, #40997, #71331, #56153, #117835, #179528, #102665, #164350, #25845, #137965, #186480, #156112, #94431, #123766, #184477, #91438, #169289, #121795, #47957, #429, #125774, #62103, #78262, #63104, #15623, #183489, #14629, #110596, #93435, #155121, #17609, #138949, #46956, #171292, #79269, #16615, #18607, #44973, #170292, #108615, #106631, #76286, #32779, #31786, #139935, #1424, #2427, #168305, #29802, #140940, #124782, #185465, #109608, #64107, #154129, #199648, #187474, #48943, #157111, #172278, #33767, #61114, #95427, #80255, #141925, #153125, #60128, #122787, #77280, #45956, #107611, #30795, #92443, #50927, #176276, #53921, #96414, #189450, #81235, #142916, #65091, #37747, #5398, #21579, #112585, #191426, #99407, #98394, #126750, #7396, #82226, #161090, #20574, #158100, #190437, #188452, #143917, #113572, #22585, #130746, #115595, #83237, #177284, #84233, #145911, #69080, #144913, #49932, #192439, #111597, #162093, #67081, #38755, #68075, #114577, #173282, #174279, #160093, #34755, #6396, #52902, #4398, #19592, #100412, #129729, #23588, #85236, #51913, #66082, #3416, #127749, #35748, #97394, #159080, #128741, #175266, #36732, #167089, #12427, #70089, #163095, #73100, #8417, #42754, #119594, #116588, #181277, #118600, #11429, #196453, #27602, #132754, #179286, #104417, #57923, #180290, #134770, #9422, #25606, #89241, #72082, #26595, #193440, #54916, #105404, #71087, #194441, #178277, #74090, #131758, #147936, #197431, #28590, #164107, #55912, #150934, #39740, #88238, #135760, #166100, #101402, #117586, #24599, #58897, #56925, #86246, #40752 ),
 ( #102420, #120563, #182257, #87250, #43742, #41758, #146926, #148934, #10424, #133756, #195450, #103423, #165102, #149923, #154884, #152888, #169046, #171051, #15385, #170056, #136730, #198412, #48710, #14383, #137725, #59889, #17371, #13400, #91198, #140701, #110363, #107374, #76049, #32541, #151911, #31547, #94194, #124543, #75064, #199409, #121555, #16382, #194, #183251, #44732, #79026, #92204, #109369, #45721, #29567, #186240, #30552, #153888, #106388, #184240, #77042, #168069, #93199, #60873, #122550, #62861, #2191, #138713, #61863, #123532, #185226, #46717, #47718, #108380, #78029, #139698, #1184, #155874, #63873, #125544, #187240, #172045, #90227, #50699, #188223, #20339, #18377, #112358, #143681, #6166, #160862, #84004, #113344, #7164, #67846, #191201, #129501, #175036, #95194, #52676, #156880, #192202, #174049, #114339, #98155, #144681, #80029, #19365, #190203, #141698, #36501, #21348, #111361, #3189, #176042, #159855, #37510, #99172, #81988, #64862, #22352, #126524, #83006, #68847, #49696, #173050, #4169, #97166, #35518, #157876, #145682, #34527, #130506, #53684, #115361, #96187, #142689, #81014, #33532, #5162, #65847, #127517, #189221, #158851, #66845, #128508, #51682, #72868, #117353, #40517, #146679, #70856, #55679, #193204, #180059, #116351, #24363, #149695, #27363, #69850, #162856, #54677, #178040, #38521, #11193, #179049, #195212, #86014, #164872, #134537, #71851, #100177, #181047, #102188, #196225, #194214, #131518, #163876, #161859, #25375, #87017, #57695, #104185, #89009, #56692, #150700, #119363, #42522, #165867, #118366, #23353, #12198, #84998, #135532, #148703, #73863, #41528, #88007, #8174, #147703, #133520, #39508, #103191, #26367, #101168, #9191, #197203, #58666, #177051, #132525, #10191, #28364, #200161, #182027, #15147, #948, #43510, #90002, #106158, #75814, #124301, #31310, #105176, #92963, #62623, #29341, #60639, #168812, #30316, #167840, #185998, #91959, #151684, #90970, #14147, #137492, #199172, #16144, #166862, #76809, #77799, #138480, #74839, #120332, #13176, #107142, #136502, #61631, #198182, #59652, #154649, #153652, #123299, #122313, #121326, #183018, #152657, #184004, #44502, #184991, #108135, #46475, #45487, #139468, #169819, #151342, #59304, #118009, #25014, #181679, #162500, #180699, #43160, #135185, #85657, #9837, #132168, #165516, #10836, #193859, #8832, #28014, #102833, #119993, #56327, #40152, #196859, #41170, #164519, #70500, #194854, #179698, #116995, #103835, #101828, #148341, #73514, #12831, #55324, #86657, #178690, #163515, #24001, #58325, #26012, #119016, #71496, #88656, #104827, #195868, #147344, #166516, #87655, #89656, #149340, #133162, #72506, #134181, #57341, #42175, #74497, #136163, #197838, #27012, #120973, #182671, #100817, #150352, #11849, #105815, #1602, #167502, #2603, #61289, #16787, #108788, #155297, #28997, #29975, #602, #152319, #47130, #31957, #121970, #13805, #78437, #170467, #186655, #109782, #92614, #75471, #140111, #90637, #93612, #79444, #137144, #198832, #14803, #107781, #64281, #63278, #44155, #125948, #76464, #60296, #124958, #48125, #183662, #171465, #15794, #32953, #94608, #156287, #91614, #138141, #17788, #141114, #77454, #45147, #106803, #122959, #168477, #169466, #123940, #153302, #154305, #199821, #184646, #46127, #30967, #139125, #62272, #185638, #130404, #192102, #98058, #129408, #25276, #8076, #69752, #9091, #53584, #161764, #85916, #70759, #131421, #133422, #159758, #84902, #23259, #36404, #191105, #147604, #146582, #193108, #116255, #117256, #21253, #144586, #55582, #54582, #176954, #177946, #101073, #68746, #52579, #39413, #162758, #71753, #24267, #132427, #114239, #194119, #195111, #178949, #82908, #38423, #6072, #40419, #102090, #175945, #67750, #163775, #56594, #145587, #86918, #148601, #10093, #37415, #174942, #99075, #160765, #22255, #115261, #83904, #7065, #100079, #168722, #183911, #198086, #134439, #45396 ),
 ( #90879, #89906, #182924, #167747, #199076, #104086, #150604, #75718, #29245, #151589, #44407, #180947, #197106, #60545, #43411, #59553, #164772, #26267, #76716, #42423, #165768, #87909, #107049, #41425, #119264, #30223, #138392, #135436, #27263, #122220, #179958, #121231, #91866, #152562, #103091, #88912, #149595, #106061, #57595, #12100, #14051, #153558, #11093, #73763, #196124, #58573, #72769, #137395, #120238, #136408, #181929, #15056, #200073, #13080, #105081, #118268, #166767, #28268, #74745, #16054, #48388, #46383, #140378, #171725, #34203, #188895, #112036, #141376, #35193, #95866, #19042, #157549, #2863, #123210, #80689, #184900, #20019, #78700, #142365, #126207, #172721, #108042, #47393, #18053, #169727, #64541, #49372, #139378, #31221, #3845, #187903, #65524, #127184, #110045, #92871, #50376, #154558, #111034, #96846, #77712, #860, #32217, #125220, #81662, #173724, #61541, #143345, #93874, #62534, #158531, #124209, #185907, #109047, #33213, #170725, #155552, #17046, #1865, #63546, #186917, #94872, #156553, #79707, #67513, #83669, #85675, #130162, #84664, #51356, #113017, #163533, #129170, #52344, #174709, #132187, #128183, #5837, #55343, #25033, #22017, #190868, #147362, #66520, #146343, #8851, #39178, #189881, #114000, #36173, #69516, #115020, #97825, #159514, #193878, #6829, #24021, #161526, #175698, #23018, #162518, #68508, #21010, #98833, #145347, #82666, #70518, #37174, #160528, #117013, #116021, #176713, #131181, #191859, #53341, #178708, #38186, #7830, #144350, #99842, #86676, #192871, #54349, #177710, #40170, #100835, #101849, #4833, #106826, #165536, #72525, #29019, #9855, #28035, #90659, #182693, #133182, #57364, #179719, #12853, #58345, #41190, #56345, #75492, #150374, #167523, #104847, #195889, #166537, #105836, #11870, #118028, #42194, #27033, #164538, #151362, #87675, #119037, #120994, #198854, #102852, #134201, #26030, #149360, #71514, #44178, #73534, #89676, #180719, #136183, #152341, #43179, #194872, #13826, #88678, #137165, #135207, #10856, #196879, #103855, #120013, #181698, #60320, #121995, #183685, #74518, #45171, #168501, #29999, #148360, #197858, #59325, #49144, #14827, #50139, #108814, #64308, #156315, #2632, #76489, #77480, #48152, #199847, #94635, #79474, #169490, #61313, #125976, #17816, #33971, #157315, #140138, #122983, #187674, #153325, #141142, #126951, #138166, #184670, #62297, #155325, #111798, #110802, #91637, #173487, #123967, #46153, #172484, #95628, #107808, #18811, #63307, #80455, #142129, #30990, #185664, #93640, #16813, #78463, #3613, #92639, #65292, #188660, #154329, #15819, #139149, #626, #170493, #47155, #1630, #31983, #124986, #186682, #109810, #171493, #32982, #116786, #8620, #193645, #99612, #145113, #67279, #69282, #112784, #161292, #130948, #192638, #98601, #159279, #66288, #144119, #96612, #22787, #175467, #176478, #34960, #158301, #190639, #52115, #19789, #189650, #85442, #68277, #129928, #54121, #113771, #21785, #146112, #115794, #191627, #55117, #81430, #6598, #83436, #143116, #51124, #7596, #53107, #114785, #37954, #177484, #4596, #127947, #38953, #84434, #36939, #100609, #162292, #128938, #174478, #23792, #147132, #131960, #70292, #35945, #97591, #20776, #82431, #5600, #160295, #41964, #86451, #150136, #119790, #117798, #148136, #166305, #198621, #149138, #104616, #89442, #135957, #24802, #134975, #165306, #26800, #9627, #195659, #28786, #152111, #88441, #90425, #43941, #58121, #194645, #105602, #11637, #151132, #57130, #118806, #73304, #181474, #72289, #167289, #75261, #133967, #196652, #42952, #27801, #10628, #60087, #12623, #180492, #56115, #74288, #179491, #25806, #197627, #13594, #71294, #164313, #40956, #102628, #39944, #59093, #103630, #120759, #87452, #182460, #136932, #178477, #101615, #163304, #132957, #156069, #138908, #76245, #108575, #106589, #388, #31746, #94390, #51621, #174977, #1382, #98096, #17567, #79228 ),
 ( #29762, #124742, #109568, #199607, #91396, #140899, #186438, #66786, #190146, #170252, #153085, #5105, #183448, #47914, #159794, #44932, #14589, #92402, #185424, #144624, #128450, #121755, #6107, #154088, #168265, #113286, #36441, #137923, #21289, #93394, #171250, #32738, #82946, #107570, #15582, #61073, #122745, #155081, #184436, #45916, #62061, #169247, #46915, #63063, #30755, #77240, #123726, #16575, #78222, #139893, #195150, #191144, #68784, #118305, #26305, #84938, #192140, #148640, #129445, #147641, #10130, #102128, #52618, #176990, #99112, #132464, #177981, #160804, #175983, #56631, #69789, #86956, #24304, #115297, #85953, #25314, #131457, #37451, #161799, #22292, #23294, #146619, #83943, #70796, #7102, #38460, #40454, #179997, #145623, #53621, #130441, #100116, #114280, #163812, #193144, #9130, #8111, #55619, #71791, #162795, #54616, #133460, #116291, #41464, #39448, #101109, #194155, #117292, #178987, #103129, #164810, #87945, #149633, #67788, #184934, #183945, #168755, #107083, #152598, #72806, #30258, #134476, #169761, #28304, #45430, #75755, #122255, #196161, #197142, #167783, #119301, #14089, #199112, #88950, #180984, #91901, #137432, #153593, #76751, #59592, #42460, #15091, #57635, #60579, #46419, #104124, #165806, #181967, #74782, #31256, #138426, #11131, #92906, #43450, #27303, #200106, #61574, #150641, #123243, #182960, #108077, #12137, #73801, #58609, #105118, #135474, #120275, #44443, #166804, #89944, #151625, #13118, #136444, #90913, #198125, #121266, #106097, #29282, #1900, #62569, #81695, #77746, #155586, #4870, #113051, #171759, #78735, #35226, #16088, #34237, #96879, #188932, #139412, #63580, #185941, #19075, #64576, #47426, #124246, #143378, #156590, #173758, #111068, #125254, #172757, #112070, #18085, #174743, #157582, #33248, #79740, #140411, #36206, #128218, #154592, #80723, #126241, #186953, #50410, #32250, #142401, #158563, #20052, #141409, #48423, #109082, #110079, #895, #3880, #94906, #95899, #170761, #93908, #2897, #187936, #17081, #49405, #66554, #65559, #127219, #189915, #51390, #84699, #8887, #132222, #54385, #56382, #82701, #7867, #146379, #159550, #52379, #70555, #69553, #116058, #39215, #40207, #21047, #67547, #178743, #131217, #99877, #177746, #24058, #191894, #175734, #100871, #162553, #194907, #85713, #147399, #37212, #193915, #118064, #55378, #144385, #161561, #5871, #192908, #117048, #98868, #129205, #101886, #179754, #68543, #163568, #25068, #86711, #190903, #148396, #9890, #71551, #114036, #115056, #133216, #97860, #160564, #22053, #83704, #145382, #6864, #130199, #53378, #176748, #38222, #23054, #12886, #182727, #135240, #106858, #138199, #196912, #89711, #197891, #59360, #73567, #123016, #121029, #134236, #58379, #43214, #10888, #152374, #74549, #105870, #103888, #120046, #122028, #166570, #44211, #87707, #149393, #199881, #165568, #136216, #75526, #181733, #28070, #13859, #137201, #167557, #61345, #26064, #151396, #29051, #102885, #195921, #198887, #90691, #60355, #183718, #45204, #164570, #72561, #168532, #30030, #104882, #91668, #153359, #14861, #119069, #76522, #41224, #57397, #180751, #42227, #27067, #88713, #150408, #11903, #169523, #48185, #92673, #156347, #126009, #124000, #154361, #172518, #4627, #155358, #110834, #95659, #142161, #31023, #141173, #171525, #33013, #15855, #1664, #34988, #158330, #94668, #96642, #50171, #64340, #660, #111828, #17847, #157347, #63342, #125019, #79504, #187704, #78498, #173516, #81460, #140171, #2663, #49176, #34003, #16847, #66317, #18842, #143146, #108847, #186715, #77513, #109840, #19819, #139185, #80487, #184701, #3645, #62330, #46186, #107839, #65323, #185698, #126983, #188690, #47187, #170527, #32017, #93675, #52145, #9659, #101646, #86483, #192670, #37986, #160326, #162323, #5633, #54153, #23824, #85474, #191658, #113802, #159311, #36970, #189681, #115827, #68307, #69313, #127978, #51153, #83468 ),
 ( #177516, #67310, #147163, #148168, #38986, #112814, #53137, #35974, #99642, #130979, #128969, #97621, #100642, #174507, #98631, #8651, #70325, #131992, #20806, #84464, #114816, #176508, #82462, #145145, #178510, #163338, #161325, #39976, #193678, #7629, #144148, #55148, #22818, #116819, #6628, #129958, #146142, #24833, #21816, #190669, #175497, #165340, #119823, #27836, #89477, #103662, #153118, #151168, #29795, #195690, #150170, #117829, #135009, #121789, #179522, #59127, #60122, #120794, #149171, #91431, #136966, #88473, #71326, #58155, #152145, #132988, #74323, #11670, #196686, #57161, #194679, #44967, #56148, #135990, #181508, #26833, #105636, #10660, #197661, #167325, #28821, #42986, #118840, #102659, #180523, #40991, #182494, #73336, #12656, #164344, #25839, #104652, #166338, #87483, #72323, #183483, #43974, #90461, #13628, #75295, #198655, #106625, #168299, #133999, #41996, #199641, #124775, #63096, #76279, #169282, #187467, #186473, #32772, #156104, #157104, #137958, #184470, #95419, #1417, #16608, #171285, #110589, #17602, #61107, #172270, #122780, #173274, #31779, #48936, #79261, #125767, #45949, #422, #94424, #107604, #140933, #2419, #92436, #30788, #33760, #64100, #18600, #80248, #47950, #154122, #141918, #15616, #3409, #49925, #77273, #138942, #185458, #78255, #34748, #65084, #14622, #96407, #46948, #62096, #126743, #188445, #123759, #111589, #109601, #108608, #170285, #93428, #155114, #139928, #127742, #69073, #129723, #22579, #20568, #36726, #38748, #83232, #37740, #4392, #66076, #116582, #82220, #5392, #189444, #85229, #81229, #159074, #8409, #178271, #175260, #143909, #100406, #19586, #99401, #162087, #192432, #142910, #67075, #50921, #84226, #68069, #112579, #174273, #146920, #160086, #177277, #114571, #128735, #176268, #115589, #21573, #35742, #51907, #98388, #97388, #161084, #190431, #113566, #130740, #70083, #144907, #6390, #191420, #52896, #145905, #53914, #7390, #23581, #131751, #193434, #54909, #39734, #158094, #105396, #180283, #135753, #118594, #55907, #88232, #86240, #41752, #11423, #74083, #28584, #151904, #181271, #75057, #197424, #58890, #183243, #119588, #59882, #25601, #103417, #147930, #165096, #13393, #9416, #89233, #90220, #150927, #179281, #121548, #167082, #26589, #101395, #149917, #182250, #163089, #104410, #73093, #134764, #87245, #24592, #136723, #71082, #166093, #196447, #133749, #120556, #40746, #27595, #43734, #198405, #57916, #148928, #132748, #10417, #194436, #12420, #42748, #117581, #102415, #164102, #56918, #72075, #195443, #199401, #95186, #78020, #139689, #79017, #123523, #31537, #155864, #140693, #1175, #3181, #29560, #154875, #93190, #106380, #60865, #17362, #16372, #62852, #186230, #187231, #168062, #14376, #125534, #124534, #46708, #47710, #171042, #138704, #122540, #109360, #32533, #141690, #94185, #2183, #184231, #63863, #64854, #48702, #91191, #108370, #152881, #110354, #172036, #45712, #76042, #33524, #126516, #15376, #156872, #18369, #80021, #137717, #44724, #107364, #169036, #30543, #61854, #92194, #153878, #77032, #185, #185217, #170047, #4159, #53671, #159844, #99161, #66835, #5153, #21337, #129493, #81978, #115349, #84986, #143672, #36489, #144671, #6156, #20329, #177039, #82995, #160851, #128499, #190194, #67836, #191190, #51670, #38509, #146667, #113333, #98145, #52666, #114328, #175026, #69838, #176031, #8162, #112347, #37499, #34519, #22340, #100165, #96178, #83991, #161847, #145670, #65838, #188214, #23341, #7152, #49686, #68835, #130494, #111351, #192190, #173041, #157867, #174038, #19357, #81006, #142680, #127508, #189212, #50690, #35508, #97158, #158841, #30055, #168558, #195200, #55667, #162844, #40505, #193192, #122053, #71839, #72856, #131505, #54665, #87004, #148691, #116339, #86002, #184729, #164859, #26355, #91697, #10179, #118354, #45231, #153390, #87995, #92700, #178028, #41516, #180047, #39496, #147691, #106885 ),
 ( #134526, #196213, #31051, #183745, #14889, #9178, #76550, #154388, #60381, #101156, #56680, #24351, #103179, #138226, #70845, #132513, #199908, #15883, #102176, #61372, #123043, #46213, #194202, #149683, #11181, #107867, #117341, #133508, #169555, #179037, #163864, #25363, #143177, #157378, #93702, #188720, #111859, #34032, #36004, #62359, #187733, #126037, #139213, #32045, #50204, #49204, #95690, #18871, #19849, #688, #47217, #158361, #64368, #79532, #80517, #3674, #171552, #155385, #142190, #65352, #174537, #127013, #173549, #16874, #35018, #97651, #96673, #124029, #141202, #185728, #110862, #81490, #78525, #108875, #4657, #159340, #48213, #66348, #128010, #189712, #170555, #51185, #172547, #112846, #140199, #94696, #77541, #1693, #63369, #125046, #186742, #109867, #33041, #156374, #17878, #2691, #99671, #38015, #192698, #162350, #114845, #86509, #117857, #176539, #69340, #177544, #39013, #53167, #102685, #100668, #179549, #145174, #161355, #67340, #84493, #71352, #129001, #8679, #9687, #70351, #98662, #41019, #148194, #22846, #20837, #7656, #101674, #82494, #23851, #146171, #131006, #6658, #144177, #194706, #5663, #85500, #54181, #115854, #55176, #160356, #147189, #116845, #178535, #132018, #68336, #52174, #129986, #190699, #193706, #40002, #163364, #113831, #175526, #24860, #133016, #37001, #21846, #56175, #83497, #191686, #198681, #43012, #151193, #42023, #90489, #60148, #121816, #27863, #88503, #195717, #73364, #25865, #152171, #104679, #105665, #164371, #87509, #119848, #181533, #149197, #118866, #14649, #197687, #59152, #183512, #166366, #12682, #75321, #44995, #120822, #122808, #10687, #74348, #136014, #72351, #180550, #136992, #182522, #44003, #167351, #106654, #134025, #57190, #168327, #28849, #89504, #13654, #29823, #58181, #103688, #91459, #153147, #61136, #76309, #137987, #165367, #199670, #184498, #45978, #26861, #150199, #11697, #135036, #196712, #123789, #15645, #125796, #111620, #93459, #2449, #187498, #172300, #92465, #94454, #186503, #47979, #154153, #78285, #3437, #126771, #109632, #65113, #18629, #17633, #451, #80276, #171315, #48964, #139958, #1448, #32802, #79293, #155145, #141947, #49956, #16638, #156134, #140962, #64131, #63126, #173305, #110618, #107632, #170315, #124805, #77304, #33789, #188475, #138973, #95449, #169310, #157134, #185488, #30816, #62126, #46978, #108637, #31808, #168955, #108285, #91112, #105315, #13312, #12338, #169963, #61773, #46625, #152802, #198322, #120475, #122458, #11341, #74002, #44645, #196367, #14294, #75961, #166012, #57835, #184151, #137635, #30461, #153797, #136640, #119508, #60787, #149837, #199322, #123441, #73012, #181189, #58807, #151823, #88152, #45632, #134681, #42666, #182167, #104328, #107284, #92109, #27512, #15292, #59799, #76952, #138622, #103, #89153, #150842, #135672, #185134, #121469, #197344, #43652, #167002, #28504, #74978, #167983, #90138, #183161, #106297, #29481, #78936, #139608, #158758, #154793, #32453, #81895, #190111, #48624, #155785, #112265, #93108, #111269, #173957, #65757, #16291, #140612, #62770, #96097, #141611, #124451, #1094, #20247, #33445, #50606, #188135, #2102, #49606, #189134, #95104, #186147, #125455, #110276, #47626, #34438, #170959, #63783, #4079, #143588, #109280, #17282, #94106, #187151, #77941, #127426, #156793, #172960, #171957, #19276, #35424, #126437, #18286, #97077, #79941, #5071, #3098, #64775, #157786, #80923, #142599, #66754, #128415, #51586, #113251, #31455, #169020, #88215, #90204, #44708, #165078, #43718, #149899, #151887, #121532, #119571, #11406, #168046, #137700, #103400, #138688, #197408, #152865, #106362, #150910, #153862, #76025, #91176, #199385, #26572, #136707, #167066, #28567, #73075, #58874, #30525, #15360, #13377, #92177, #45696, #59865, #196429, #107347, #75041, #14360, #120540, #182233, #198388, #183227, #74066, #77016, #169, #135737, #29543, #60849, #122524, #12404 ) ),
 .UNSPECIFIED., .T., .F., .F. ) 
 B_SPLINE_SURFACE_WITH_KNOTS ( ( 4, 3, 4 ),
 ( 3, 2, 2, 2, 2, 2, 2, 2, 2, 2, 2, 2, 2, 2, 2, 2, 2, 2, 2, 2, 2, 2, 2, 2, 2, 2, 2, 2, 2, 2, 2, 2, 2, 2, 2, 2, 2, 2, 2, 2, 2, 2, 2, 2, 2, 2, 2, 2, 2, 2, 2, 2, 2, 2, 2, 2, 2, 2, 2, 2, 2, 2, 2, 2, 2, 2, 2, 2, 2, 2, 2, 2, 2, 2, 2, 2, 2, 2, 2, 2, 2, 2, 2, 2, 2, 2, 2, 2, 2, 2, 2, 2, 2, 2, 2, 2, 2, 2, 2, 2, 2, 2, 2, 2, 2, 2, 2, 2, 2, 2, 2, 2, 2, 2, 2, 2, 2, 2, 2, 2, 2, 2, 2, 2, 2, 2, 2, 2, 2, 2, 2, 2, 2, 2, 2, 2, 2, 2, 2, 2, 2, 2, 2, 2, 2, 2, 2, 2, 2, 2, 2, 2, 2, 2, 2, 2, 2, 2, 2, 2, 2, 2, 2, 2, 2, 2, 2, 2, 2, 2, 2, 2, 2, 2, 2, 2, 2, 2, 2, 2, 2, 2, 2, 2, 2, 2, 2, 2, 2, 2, 2, 2, 2, 2, 2, 2, 2, 2, 2, 2, 2, 2, 2, 2, 2, 2, 2, 2, 2, 2, 2, 2, 2, 2, 2, 2, 2, 2, 2, 2, 2, 2, 2, 2, 2, 2, 2, 2, 3 ),
 ( 0.000000000000000000, 0.5000000000000000000, 1.000000000000000000 ),
 ( 0.000000000000000000, 0.004385964912280701511, 0.008771929824561403022, 0.01315789473684210453, 0.01754385964912280604, 0.02192982456140350755, 0.02631578947368420907, 0.03070175438596491058, 0.03508771929824561209, 0.03947368421052631360, 0.04385964912280701511, 0.04824561403508771662, 0.05263157894736841813, 0.05701754385964911964, 0.06140350877192982115, 0.06578947368421052266, 0.07017543859649122417, 0.07456140350877192569, 0.07894736842105262720, 0.08333333333333332871, 0.08771929824561403022, 0.09210526315789473173, 0.09649122807017543324, 0.1008771929824561348, 0.1052631578947368363, 0.1096491228070175378, 0.1140350877192982393, 0.1184210526315789408, 0.1228070175438596423, 0.1271929824561403577, 0.1315789473684210453, 0.1359649122807017607, 0.1403508771929824483, 0.1447368421052631637, 0.1491228070175438514, 0.1535087719298245668, 0.1578947368421052544, 0.1622807017543859698, 0.1666666666666666574, 0.1710526315789473728, 0.1754385964912280604, 0.1798245614035087758, 0.1842105263157894635, 0.1885964912280701788, 0.1929824561403508665, 0.1973684210526315819, 0.2017543859649122695, 0.2061403508771929849, 0.2105263157894736725, 0.2149122807017543879, 0.2192982456140350755, 0.2236842105263157909, 0.2280701754385964786, 0.2324561403508771940, 0.2368421052631578816, 0.2412280701754385970, 0.2456140350877192846, 0.2500000000000000000, 0.2543859649122807154, 0.2587719298245614308, 0.2631578947368420907, 0.2675438596491228060, 0.2719298245614035214, 0.2763157894736842368, 0.2807017543859648967, 0.2850877192982456121, 0.2894736842105263275, 0.2938596491228070429, 0.2982456140350877027, 0.3026315789473684181, 0.3070175438596491335, 0.3114035087719298489, 0.3157894736842105088, 0.3201754385964912242, 0.3245614035087719396, 0.3289473684210526550, 0.3333333333333333148, 0.3377192982456140302, 0.3421052631578947456, 0.3464912280701754610, 0.3508771929824561209, 0.3552631578947368363, 0.3596491228070175517, 0.3640350877192982670, 0.3684210526315789269, 0.3728070175438596423, 0.3771929824561403577, 0.3815789473684210731, 0.3859649122807017330, 0.3903508771929824483, 0.3947368421052631637, 0.3991228070175438791, 0.4035087719298245390, 0.4078947368421052544, 0.4122807017543859698, 0.4166666666666666852, 0.4210526315789473450, 0.4254385964912280604, 0.4298245614035087758, 0.4342105263157894912, 0.4385964912280701511, 0.4429824561403508665, 0.4473684210526315819, 0.4517543859649122973, 0.4561403508771929571, 0.4605263157894736725, 0.4649122807017543879, 0.4692982456140351033, 0.4736842105263157632, 0.4780701754385964786, 0.4824561403508771940, 0.4868421052631579093, 0.4912280701754385692, 0.4956140350877192846, 0.5000000000000000000, 0.5043859649122807154, 0.5087719298245614308, 0.5131578947368421462, 0.5175438596491228616, 0.5219298245614034659, 0.5263157894736841813, 0.5307017543859648967, 0.5350877192982456121, 0.5394736842105263275, 0.5438596491228070429, 0.5482456140350877583, 0.5526315789473684736, 0.5570175438596490780, 0.5614035087719297934, 0.5657894736842105088, 0.5701754385964912242, 0.5745614035087719396, 0.5789473684210526550, 0.5833333333333333703, 0.5877192982456140857, 0.5921052631578946901, 0.5964912280701754055, 0.6008771929824561209, 0.6052631578947368363, 0.6096491228070175517, 0.6140350877192982670, 0.6184210526315789824, 0.6228070175438596978, 0.6271929824561403022, 0.6315789473684210176, 0.6359649122807017330, 0.6403508771929824483, 0.6447368421052631637, 0.6491228070175438791, 0.6535087719298245945, 0.6578947368421053099, 0.6622807017543859143, 0.6666666666666666297, 0.6710526315789473450, 0.6754385964912280604, 0.6798245614035087758, 0.6842105263157894912, 0.6885964912280702066, 0.6929824561403509220, 0.6973684210526315264, 0.7017543859649122417, 0.7061403508771929571, 0.7105263157894736725, 0.7149122807017543879, 0.7192982456140351033, 0.7236842105263158187, 0.7280701754385965341, 0.7324561403508771384, 0.7368421052631578538, 0.7412280701754385692, 0.7456140350877192846, 0.7500000000000000000, 0.7543859649122807154, 0.7587719298245614308, 0.7631578947368421462, 0.7675438596491228616, 0.7719298245614034659, 0.7763157894736841813, 0.7807017543859648967, 0.7850877192982456121, 0.7894736842105263275, 0.7938596491228070429, 0.7982456140350877583, 0.8026315789473684736, 0.8070175438596490780, 0.8114035087719297934, 0.8157894736842105088, 0.8201754385964912242, 0.8245614035087719396, 0.8289473684210526550, 0.8333333333333333703, 0.8377192982456140857, 0.8421052631578946901, 0.8464912280701754055, 0.8508771929824561209, 0.8552631578947368363, 0.8596491228070175517, 0.8640350877192982670, 0.8684210526315789824, 0.8728070175438596978, 0.8771929824561403022, 0.8815789473684210176, 0.8859649122807017330, 0.8903508771929824483, 0.8947368421052631637, 0.8991228070175438791, 0.9035087719298245945, 0.9078947368421053099, 0.9122807017543859143, 0.9166666666666666297, 0.9210526315789473450, 0.9254385964912280604, 0.9298245614035087758, 0.9342105263157894912, 0.9385964912280702066, 0.9429824561403509220, 0.9473684210526315264, 0.9517543859649122417, 0.9561403508771929571, 0.9605263157894736725, 0.9649122807017543879, 0.9692982456140351033, 0.9736842105263158187, 0.9780701754385965341, 0.9824561403508771384, 0.9868421052631578538, 0.9912280701754385692, 0.9956140350877192846, 1.000000000000000000 ),
 .UNSPECIFIED. ) 
 GEOMETRIC_REPRESENTATION_ITEM ( )  RATIONAL_B_SPLINE_SURFACE ( (
 ( 1.000000000000000000, 0.9659258262890683122, 1.000000000000000000, 0.9659258262890683122, 1.000000000000000000, 0.9659258262890683122, 1.000000000000000000, 0.9659258262890683122, 1.000000000000000000, 0.9659258262890683122, 1.000000000000000000, 0.9659258262890683122, 1.000000000000000000, 0.9659258262890683122, 1.000000000000000000, 0.9659258262890683122, 1.000000000000000000, 0.9659258262890683122, 1.000000000000000000, 0.9659258262890683122, 1.000000000000000000, 0.9659258262890683122, 1.000000000000000000, 0.9659258262890683122, 1.000000000000000000, 0.9659258262890683122, 1.000000000000000000, 0.9659258262890683122, 1.000000000000000000, 0.9659258262890683122, 1.000000000000000000, 0.9659258262890683122, 1.000000000000000000, 0.9659258262890683122, 1.000000000000000000, 0.9659258262890683122, 1.000000000000000000, 0.9659258262890683122, 1.000000000000000000, 0.9659258262890683122, 1.000000000000000000, 0.9659258262890683122, 1.000000000000000000, 0.9659258262890683122, 1.000000000000000000, 0.9659258262890683122, 1.000000000000000000, 0.9659258262890683122, 1.000000000000000000, 0.9659258262890683122, 1.000000000000000000, 0.9659258262890683122, 1.000000000000000000, 0.9659258262890683122, 1.000000000000000000, 0.9659258262890683122, 1.000000000000000000, 0.9659258262890683122, 1.000000000000000000, 0.9659258262890683122, 1.000000000000000000, 0.9659258262890683122, 1.000000000000000000, 0.9659258262890683122, 1.000000000000000000, 0.9659258262890683122, 1.000000000000000000, 0.9659258262890683122, 1.000000000000000000, 0.9659258262890683122, 1.000000000000000000, 0.9659258262890683122, 1.000000000000000000, 0.9659258262890683122, 1.000000000000000000, 0.9659258262890683122, 1.000000000000000000, 0.9659258262890683122, 1.000000000000000000, 0.9659258262890683122, 1.000000000000000000, 0.9659258262890683122, 1.000000000000000000, 0.9659258262890683122, 1.000000000000000000, 0.9659258262890683122, 1.000000000000000000, 0.9659258262890683122, 1.000000000000000000, 0.9659258262890683122, 1.000000000000000000, 0.9659258262890683122, 1.000000000000000000, 0.9659258262890683122, 1.000000000000000000, 0.9659258262890683122, 1.000000000000000000, 0.9659258262890683122, 1.000000000000000000, 0.9659258262890683122, 1.000000000000000000, 0.9659258262890683122, 1.000000000000000000, 0.9659258262890683122, 1.000000000000000000, 0.9659258262890683122, 1.000000000000000000, 0.9659258262890683122, 1.000000000000000000, 0.9659258262890683122, 1.000000000000000000, 0.9659258262890683122, 1.000000000000000000, 0.9659258262890683122, 1.000000000000000000, 0.9659258262890683122, 1.000000000000000000, 0.9659258262890683122, 1.000000000000000000, 0.9659258262890683122, 1.000000000000000000, 0.9659258262890683122, 1.000000000000000000, 0.9659258262890683122, 1.000000000000000000, 0.9659258262890683122, 1.000000000000000000, 0.9659258262890683122, 1.000000000000000000, 0.9659258262890683122, 1.000000000000000000, 0.9659258262890683122, 1.000000000000000000, 0.9659258262890683122, 1.000000000000000000, 0.9659258262890683122, 1.000000000000000000, 0.9659258262890683122, 1.000000000000000000, 0.9659258262890683122, 1.000000000000000000, 0.9659258262890683122, 1.000000000000000000, 0.9659258262890683122, 1.000000000000000000, 0.9659258262890683122, 1.000000000000000000, 0.9659258262890683122, 1.000000000000000000, 0.9659258262890683122, 1.000000000000000000, 0.9659258262890683122, 1.000000000000000000, 0.9659258262890683122, 1.000000000000000000, 0.9659258262890683122, 1.000000000000000000, 0.9659258262890683122, 1.000000000000000000, 0.9659258262890683122, 1.000000000000000000, 0.9659258262890683122, 1.000000000000000000, 0.9659258262890683122, 1.000000000000000000, 0.9659258262890683122, 1.000000000000000000, 0.9659258262890683122, 1.000000000000000000, 0.9659258262890683122, 1.000000000000000000, 0.9659258262890683122, 1.000000000000000000, 0.9659258262890683122, 1.000000000000000000, 0.9659258262890683122, 1.000000000000000000, 0.9659258262890683122, 1.000000000000000000, 0.9659258262890683122, 1.000000000000000000, 0.9659258262890683122, 1.000000000000000000, 0.9659258262890683122, 1.000000000000000000, 0.9659258262890683122, 1.000000000000000000, 0.9659258262890683122, 1.000000000000000000, 0.9659258262890683122, 1.000000000000000000, 0.9659258262890683122, 1.000000000000000000, 0.9659258262890683122, 1.000000000000000000, 0.9659258262890683122, 1.000000000000000000, 0.9659258262890683122, 1.000000000000000000, 0.9659258262890683122, 1.000000000000000000, 0.9659258262890683122, 1.000000000000000000, 0.9659258262890683122, 1.000000000000000000, 0.9659258262890683122, 1.000000000000000000, 0.9659258262890683122, 1.000000000000000000, 0.9659258262890683122, 1.000000000000000000, 0.9659258262890683122, 1.000000000000000000, 0.9659258262890683122, 1.000000000000000000, 0.9659258262890683122, 1.000000000000000000, 0.9659258262890683122, 1.000000000000000000, 0.9659258262890683122, 1.000000000000000000, 0.9659258262890683122, 1.000000000000000000, 0.9659258262890683122, 1.000000000000000000, 0.9659258262890683122, 1.000000000000000000, 0.9659258262890683122, 1.000000000000000000, 0.9659258262890683122, 1.000000000000000000, 0.9659258262890683122, 1.000000000000000000, 0.9659258262890683122, 1.000000000000000000, 0.9659258262890683122, 1.000000000000000000, 0.9659258262890683122, 1.000000000000000000, 0.9659258262890683122, 1.000000000000000000, 0.9659258262890683122, 1.000000000000000000, 0.9659258262890683122, 1.000000000000000000, 0.9659258262890683122, 1.000000000000000000, 0.9659258262890683122, 1.000000000000000000, 0.9659258262890683122, 1.000000000000000000, 0.9659258262890683122, 1.000000000000000000, 0.9659258262890683122, 1.000000000000000000, 0.9659258262890683122, 1.000000000000000000, 0.9659258262890683122, 1.000000000000000000, 0.9659258262890683122, 1.000000000000000000, 0.9659258262890683122, 1.000000000000000000, 0.9659258262890683122, 1.000000000000000000, 0.9659258262890683122, 1.000000000000000000, 0.9659258262890683122, 1.000000000000000000, 0.9659258262890683122, 1.000000000000000000, 0.9659258262890683122, 1.000000000000000000, 0.9659258262890683122, 1.000000000000000000, 0.9659258262890683122, 1.000000000000000000, 0.9659258262890683122, 1.000000000000000000, 0.9659258262890683122, 1.000000000000000000, 0.9659258262890683122, 1.000000000000000000, 0.9659258262890683122, 1.000000000000000000, 0.9659258262890683122, 1.000000000000000000, 0.9659258262890683122, 1.000000000000000000, 0.9659258262890683122, 1.000000000000000000, 0.9659258262890683122, 1.000000000000000000, 0.9659258262890683122, 1.000000000000000000, 0.9659258262890683122, 1.000000000000000000, 0.9659258262890683122, 1.000000000000000000, 0.9659258262890683122, 1.000000000000000000, 0.9659258262890683122, 1.000000000000000000, 0.9659258262890683122, 1.000000000000000000, 0.9659258262890683122, 1.000000000000000000, 0.9659258262890683122, 1.000000000000000000, 0.9659258262890683122, 1.000000000000000000, 0.9659258262890683122, 1.000000000000000000, 0.9659258262890683122, 1.000000000000000000, 0.9659258262890683122, 1.000000000000000000, 0.9659258262890683122, 1.000000000000000000, 0.9659258262890683122, 1.000000000000000000, 0.9659258262890683122, 1.000000000000000000, 0.9659258262890683122, 1.000000000000000000, 0.9659258262890683122, 1.000000000000000000, 0.9659258262890683122, 1.000000000000000000, 0.9659258262890683122, 1.000000000000000000, 0.9659258262890683122, 1.000000000000000000, 0.9659258262890683122, 1.000000000000000000, 0.9659258262890683122, 1.000000000000000000, 0.9659258262890683122, 1.000000000000000000, 0.9659258262890683122, 1.000000000000000000, 0.9659258262890683122, 1.000000000000000000, 0.9659258262890683122, 1.000000000000000000, 0.9659258262890683122, 1.000000000000000000, 0.9659258262890683122, 1.000000000000000000, 0.9659258262890683122, 1.000000000000000000, 0.9659258262890683122, 1.000000000000000000, 0.9659258262890683122, 1.000000000000000000, 0.9659258262890683122, 1.000000000000000000, 0.9659258262890683122, 1.000000000000000000, 0.9659258262890683122, 1.000000000000000000, 0.9659258262890683122, 1.000000000000000000, 0.9659258262890683122, 1.000000000000000000, 0.9659258262890683122, 1.000000000000000000, 0.9659258262890683122, 1.000000000000000000, 0.9659258262890683122, 1.000000000000000000, 0.9659258262890683122, 1.000000000000000000, 0.9659258262890683122, 1.000000000000000000, 0.9659258262890683122, 1.000000000000000000, 0.9659258262890683122, 1.000000000000000000, 0.9659258262890683122, 1.000000000000000000, 0.9659258262890683122, 1.000000000000000000, 0.9659258262890683122, 1.000000000000000000, 0.9659258262890683122, 1.000000000000000000, 0.9659258262890683122, 1.000000000000000000, 0.9659258262890683122, 1.000000000000000000, 0.9659258262890683122, 1.000000000000000000, 0.9659258262890683122, 1.000000000000000000, 0.9659258262890683122, 1.000000000000000000, 0.9659258262890683122, 1.000000000000000000, 0.9659258262890683122, 1.000000000000000000, 0.9659258262890683122, 1.000000000000000000, 0.9659258262890683122, 1.000000000000000000, 0.9659258262890683122, 1.000000000000000000, 0.9659258262890683122, 1.000000000000000000, 0.9659258262890683122, 1.000000000000000000, 0.9659258262890683122, 1.000000000000000000, 0.9659258262890683122, 1.000000000000000000, 0.9659258262890683122, 1.000000000000000000, 0.9659258262890683122, 1.000000000000000000, 0.9659258262890683122, 1.000000000000000000, 0.9659258262890683122, 1.000000000000000000, 0.9659258262890683122, 1.000000000000000000, 0.9659258262890683122, 1.000000000000000000, 0.9659258262890683122, 1.000000000000000000, 0.9659258262890683122, 1.000000000000000000, 0.9659258262890683122, 1.000000000000000000, 0.9659258262890683122, 1.000000000000000000, 0.9659258262890683122, 1.000000000000000000, 0.9659258262890683122, 1.000000000000000000, 0.9659258262890683122, 1.000000000000000000, 0.9659258262890683122, 1.000000000000000000, 0.9659258262890683122, 1.000000000000000000, 0.9659258262890683122, 1.000000000000000000, 0.9659258262890683122, 1.000000000000000000, 0.9659258262890683122, 1.000000000000000000, 0.9659258262890683122, 1.000000000000000000, 0.9659258262890683122, 1.000000000000000000, 0.9659258262890683122, 1.000000000000000000),
 ( 0.3333333333333333703, 0.3219752754296894559, 0.3333333333333333703, 0.3219752754296894559, 0.3333333333333333703, 0.3219752754296894559, 0.3333333333333333703, 0.3219752754296894559, 0.3333333333333333703, 0.3219752754296894559, 0.3333333333333333703, 0.3219752754296894559, 0.3333333333333333703, 0.3219752754296894559, 0.3333333333333333703, 0.3219752754296894559, 0.3333333333333333703, 0.3219752754296894559, 0.3333333333333333703, 0.3219752754296894559, 0.3333333333333333703, 0.3219752754296894559, 0.3333333333333333703, 0.3219752754296894559, 0.3333333333333333703, 0.3219752754296894559, 0.3333333333333333703, 0.3219752754296894559, 0.3333333333333333703, 0.3219752754296894559, 0.3333333333333333703, 0.3219752754296894559, 0.3333333333333333703, 0.3219752754296894559, 0.3333333333333333703, 0.3219752754296894559, 0.3333333333333333703, 0.3219752754296894559, 0.3333333333333333703, 0.3219752754296894559, 0.3333333333333333703, 0.3219752754296894559, 0.3333333333333333703, 0.3219752754296894559, 0.3333333333333333703, 0.3219752754296894559, 0.3333333333333333703, 0.3219752754296894559, 0.3333333333333333703, 0.3219752754296894559, 0.3333333333333333703, 0.3219752754296894559, 0.3333333333333333703, 0.3219752754296894559, 0.3333333333333333703, 0.3219752754296894559, 0.3333333333333333703, 0.3219752754296894559, 0.3333333333333333703, 0.3219752754296894559, 0.3333333333333333703, 0.3219752754296894559, 0.3333333333333333703, 0.3219752754296894559, 0.3333333333333333703, 0.3219752754296894559, 0.3333333333333333703, 0.3219752754296894559, 0.3333333333333333703, 0.3219752754296894559, 0.3333333333333333703, 0.3219752754296894559, 0.3333333333333333703, 0.3219752754296894559, 0.3333333333333333703, 0.3219752754296894559, 0.3333333333333333703, 0.3219752754296894559, 0.3333333333333333703, 0.3219752754296894559, 0.3333333333333333703, 0.3219752754296894559, 0.3333333333333333703, 0.3219752754296894559, 0.3333333333333333703, 0.3219752754296894559, 0.3333333333333333703, 0.3219752754296894559, 0.3333333333333333703, 0.3219752754296894559, 0.3333333333333333703, 0.3219752754296894559, 0.3333333333333333703, 0.3219752754296894559, 0.3333333333333333703, 0.3219752754296894559, 0.3333333333333333703, 0.3219752754296894559, 0.3333333333333333703, 0.3219752754296894559, 0.3333333333333333703, 0.3219752754296894559, 0.3333333333333333703, 0.3219752754296894559, 0.3333333333333333703, 0.3219752754296894559, 0.3333333333333333703, 0.3219752754296894559, 0.3333333333333333703, 0.3219752754296894559, 0.3333333333333333703, 0.3219752754296894559, 0.3333333333333333703, 0.3219752754296894559, 0.3333333333333333703, 0.3219752754296894559, 0.3333333333333333703, 0.3219752754296894559, 0.3333333333333333703, 0.3219752754296894559, 0.3333333333333333703, 0.3219752754296894559, 0.3333333333333333703, 0.3219752754296894559, 0.3333333333333333703, 0.3219752754296894559, 0.3333333333333333703, 0.3219752754296894559, 0.3333333333333333703, 0.3219752754296894559, 0.3333333333333333703, 0.3219752754296894559, 0.3333333333333333703, 0.3219752754296894559, 0.3333333333333333703, 0.3219752754296894559, 0.3333333333333333703, 0.3219752754296894559, 0.3333333333333333703, 0.3219752754296894559, 0.3333333333333333703, 0.3219752754296894559, 0.3333333333333333703, 0.3219752754296894559, 0.3333333333333333703, 0.3219752754296894559, 0.3333333333333333703, 0.3219752754296894559, 0.3333333333333333703, 0.3219752754296894559, 0.3333333333333333703, 0.3219752754296894559, 0.3333333333333333703, 0.3219752754296894559, 0.3333333333333333703, 0.3219752754296894559, 0.3333333333333333703, 0.3219752754296894559, 0.3333333333333333703, 0.3219752754296894559, 0.3333333333333333703, 0.3219752754296894559, 0.3333333333333333703, 0.3219752754296894559, 0.3333333333333333703, 0.3219752754296894559, 0.3333333333333333703, 0.3219752754296894559, 0.3333333333333333703, 0.3219752754296894559, 0.3333333333333333703, 0.3219752754296894559, 0.3333333333333333703, 0.3219752754296894559, 0.3333333333333333703, 0.3219752754296894559, 0.3333333333333333703, 0.3219752754296894559, 0.3333333333333333703, 0.3219752754296894559, 0.3333333333333333703, 0.3219752754296894559, 0.3333333333333333703, 0.3219752754296894559, 0.3333333333333333703, 0.3219752754296894559, 0.3333333333333333703, 0.3219752754296894559, 0.3333333333333333703, 0.3219752754296894559, 0.3333333333333333703, 0.3219752754296894559, 0.3333333333333333703, 0.3219752754296894559, 0.3333333333333333703, 0.3219752754296894559, 0.3333333333333333703, 0.3219752754296894559, 0.3333333333333333703, 0.3219752754296894559, 0.3333333333333333703, 0.3219752754296894559, 0.3333333333333333703, 0.3219752754296894559, 0.3333333333333333703, 0.3219752754296894559, 0.3333333333333333703, 0.3219752754296894559, 0.3333333333333333703, 0.3219752754296894559, 0.3333333333333333703, 0.3219752754296894559, 0.3333333333333333703, 0.3219752754296894559, 0.3333333333333333703, 0.3219752754296894559, 0.3333333333333333703, 0.3219752754296894559, 0.3333333333333333703, 0.3219752754296894559, 0.3333333333333333703, 0.3219752754296894559, 0.3333333333333333703, 0.3219752754296894559, 0.3333333333333333703, 0.3219752754296894559, 0.3333333333333333703, 0.3219752754296894559, 0.3333333333333333703, 0.3219752754296894559, 0.3333333333333333703, 0.3219752754296894559, 0.3333333333333333703, 0.3219752754296894559, 0.3333333333333333703, 0.3219752754296894559, 0.3333333333333333703, 0.3219752754296894559, 0.3333333333333333703, 0.3219752754296894559, 0.3333333333333333703, 0.3219752754296894559, 0.3333333333333333703, 0.3219752754296894559, 0.3333333333333333703, 0.3219752754296894559, 0.3333333333333333703, 0.3219752754296894559, 0.3333333333333333703, 0.3219752754296894559, 0.3333333333333333703, 0.3219752754296894559, 0.3333333333333333703, 0.3219752754296894559, 0.3333333333333333703, 0.3219752754296894559, 0.3333333333333333703, 0.3219752754296894559, 0.3333333333333333703, 0.3219752754296894559, 0.3333333333333333703, 0.3219752754296894559, 0.3333333333333333703, 0.3219752754296894559, 0.3333333333333333703, 0.3219752754296894559, 0.3333333333333333703, 0.3219752754296894559, 0.3333333333333333703, 0.3219752754296894559, 0.3333333333333333703, 0.3219752754296894559, 0.3333333333333333703, 0.3219752754296894559, 0.3333333333333333703, 0.3219752754296894559, 0.3333333333333333703, 0.3219752754296894559, 0.3333333333333333703, 0.3219752754296894559, 0.3333333333333333703, 0.3219752754296894559, 0.3333333333333333703, 0.3219752754296894559, 0.3333333333333333703, 0.3219752754296894559, 0.3333333333333333703, 0.3219752754296894559, 0.3333333333333333703, 0.3219752754296894559, 0.3333333333333333703, 0.3219752754296894559, 0.3333333333333333703, 0.3219752754296894559, 0.3333333333333333703, 0.3219752754296894559, 0.3333333333333333703, 0.3219752754296894559, 0.3333333333333333703, 0.3219752754296894559, 0.3333333333333333703, 0.3219752754296894559, 0.3333333333333333703, 0.3219752754296894559, 0.3333333333333333703, 0.3219752754296894559, 0.3333333333333333703, 0.3219752754296894559, 0.3333333333333333703, 0.3219752754296894559, 0.3333333333333333703, 0.3219752754296894559, 0.3333333333333333703, 0.3219752754296894559, 0.3333333333333333703, 0.3219752754296894559, 0.3333333333333333703, 0.3219752754296894559, 0.3333333333333333703, 0.3219752754296894559, 0.3333333333333333703, 0.3219752754296894559, 0.3333333333333333703, 0.3219752754296894559, 0.3333333333333333703, 0.3219752754296894559, 0.3333333333333333703, 0.3219752754296894559, 0.3333333333333333703, 0.3219752754296894559, 0.3333333333333333703, 0.3219752754296894559, 0.3333333333333333703, 0.3219752754296894559, 0.3333333333333333703, 0.3219752754296894559, 0.3333333333333333703, 0.3219752754296894559, 0.3333333333333333703, 0.3219752754296894559, 0.3333333333333333703, 0.3219752754296894559, 0.3333333333333333703, 0.3219752754296894559, 0.3333333333333333703, 0.3219752754296894559, 0.3333333333333333703, 0.3219752754296894559, 0.3333333333333333703, 0.3219752754296894559, 0.3333333333333333703, 0.3219752754296894559, 0.3333333333333333703, 0.3219752754296894559, 0.3333333333333333703, 0.3219752754296894559, 0.3333333333333333703, 0.3219752754296894559, 0.3333333333333333703, 0.3219752754296894559, 0.3333333333333333703, 0.3219752754296894559, 0.3333333333333333703, 0.3219752754296894559, 0.3333333333333333703, 0.3219752754296894559, 0.3333333333333333703, 0.3219752754296894559, 0.3333333333333333703, 0.3219752754296894559, 0.3333333333333333703, 0.3219752754296894559, 0.3333333333333333703, 0.3219752754296894559, 0.3333333333333333703, 0.3219752754296894559, 0.3333333333333333703, 0.3219752754296894559, 0.3333333333333333703, 0.3219752754296894559, 0.3333333333333333703, 0.3219752754296894559, 0.3333333333333333703, 0.3219752754296894559, 0.3333333333333333703, 0.3219752754296894559, 0.3333333333333333703, 0.3219752754296894559, 0.3333333333333333703, 0.3219752754296894559, 0.3333333333333333703, 0.3219752754296894559, 0.3333333333333333703, 0.3219752754296894559, 0.3333333333333333703, 0.3219752754296894559, 0.3333333333333333703, 0.3219752754296894559, 0.3333333333333333703, 0.3219752754296894559, 0.3333333333333333703, 0.3219752754296894559, 0.3333333333333333703, 0.3219752754296894559, 0.3333333333333333703, 0.3219752754296894559, 0.3333333333333333703, 0.3219752754296894559, 0.3333333333333333703, 0.3219752754296894559, 0.3333333333333333703, 0.3219752754296894559, 0.3333333333333333703, 0.3219752754296894559, 0.3333333333333333703, 0.3219752754296894559, 0.3333333333333333703, 0.3219752754296894559, 0.3333333333333333703, 0.3219752754296894559, 0.3333333333333333703, 0.3219752754296894559, 0.3333333333333333703, 0.3219752754296894559, 0.3333333333333333703, 0.3219752754296894559, 0.3333333333333333703, 0.3219752754296894559, 0.3333333333333333703, 0.3219752754296894559, 0.3333333333333333703, 0.3219752754296894559, 0.3333333333333333703, 0.3219752754296894559, 0.3333333333333333703, 0.3219752754296894559, 0.3333333333333333703, 0.3219752754296894559, 0.3333333333333333703, 0.3219752754296894559, 0.3333333333333333703, 0.3219752754296894559, 0.3333333333333333703, 0.3219752754296894559, 0.3333333333333333703, 0.3219752754296894559, 0.3333333333333333703, 0.3219752754296894559, 0.3333333333333333703, 0.3219752754296894559, 0.3333333333333333703, 0.3219752754296894559, 0.3333333333333333703, 0.3219752754296894559, 0.3333333333333333703, 0.3219752754296894559, 0.3333333333333333703),
 ( 0.3333333333333333703, 0.3219752754296894559, 0.3333333333333333703, 0.3219752754296894559, 0.3333333333333333703, 0.3219752754296894559, 0.3333333333333333703, 0.3219752754296894559, 0.3333333333333333703, 0.3219752754296894559, 0.3333333333333333703, 0.3219752754296894559, 0.3333333333333333703, 0.3219752754296894559, 0.3333333333333333703, 0.3219752754296894559, 0.3333333333333333703, 0.3219752754296894559, 0.3333333333333333703, 0.3219752754296894559, 0.3333333333333333703, 0.3219752754296894559, 0.3333333333333333703, 0.3219752754296894559, 0.3333333333333333703, 0.3219752754296894559, 0.3333333333333333703, 0.3219752754296894559, 0.3333333333333333703, 0.3219752754296894559, 0.3333333333333333703, 0.3219752754296894559, 0.3333333333333333703, 0.3219752754296894559, 0.3333333333333333703, 0.3219752754296894559, 0.3333333333333333703, 0.3219752754296894559, 0.3333333333333333703, 0.3219752754296894559, 0.3333333333333333703, 0.3219752754296894559, 0.3333333333333333703, 0.3219752754296894559, 0.3333333333333333703, 0.3219752754296894559, 0.3333333333333333703, 0.3219752754296894559, 0.3333333333333333703, 0.3219752754296894559, 0.3333333333333333703, 0.3219752754296894559, 0.3333333333333333703, 0.3219752754296894559, 0.3333333333333333703, 0.3219752754296894559, 0.3333333333333333703, 0.3219752754296894559, 0.3333333333333333703, 0.3219752754296894559, 0.3333333333333333703, 0.3219752754296894559, 0.3333333333333333703, 0.3219752754296894559, 0.3333333333333333703, 0.3219752754296894559, 0.3333333333333333703, 0.3219752754296894559, 0.3333333333333333703, 0.3219752754296894559, 0.3333333333333333703, 0.3219752754296894559, 0.3333333333333333703, 0.3219752754296894559, 0.3333333333333333703, 0.3219752754296894559, 0.3333333333333333703, 0.3219752754296894559, 0.3333333333333333703, 0.3219752754296894559, 0.3333333333333333703, 0.3219752754296894559, 0.3333333333333333703, 0.3219752754296894559, 0.3333333333333333703, 0.3219752754296894559, 0.3333333333333333703, 0.3219752754296894559, 0.3333333333333333703, 0.3219752754296894559, 0.3333333333333333703, 0.3219752754296894559, 0.3333333333333333703, 0.3219752754296894559, 0.3333333333333333703, 0.3219752754296894559, 0.3333333333333333703, 0.3219752754296894559, 0.3333333333333333703, 0.3219752754296894559, 0.3333333333333333703, 0.3219752754296894559, 0.3333333333333333703, 0.3219752754296894559, 0.3333333333333333703, 0.3219752754296894559, 0.3333333333333333703, 0.3219752754296894559, 0.3333333333333333703, 0.3219752754296894559, 0.3333333333333333703, 0.3219752754296894559, 0.3333333333333333703, 0.3219752754296894559, 0.3333333333333333703, 0.3219752754296894559, 0.3333333333333333703, 0.3219752754296894559, 0.3333333333333333703, 0.3219752754296894559, 0.3333333333333333703, 0.3219752754296894559, 0.3333333333333333703, 0.3219752754296894559, 0.3333333333333333703, 0.3219752754296894559, 0.3333333333333333703, 0.3219752754296894559, 0.3333333333333333703, 0.3219752754296894559, 0.3333333333333333703, 0.3219752754296894559, 0.3333333333333333703, 0.3219752754296894559, 0.3333333333333333703, 0.3219752754296894559, 0.3333333333333333703, 0.3219752754296894559, 0.3333333333333333703, 0.3219752754296894559, 0.3333333333333333703, 0.3219752754296894559, 0.3333333333333333703, 0.3219752754296894559, 0.3333333333333333703, 0.3219752754296894559, 0.3333333333333333703, 0.3219752754296894559, 0.3333333333333333703, 0.3219752754296894559, 0.3333333333333333703, 0.3219752754296894559, 0.3333333333333333703, 0.3219752754296894559, 0.3333333333333333703, 0.3219752754296894559, 0.3333333333333333703, 0.3219752754296894559, 0.3333333333333333703, 0.3219752754296894559, 0.3333333333333333703, 0.3219752754296894559, 0.3333333333333333703, 0.3219752754296894559, 0.3333333333333333703, 0.3219752754296894559, 0.3333333333333333703, 0.3219752754296894559, 0.3333333333333333703, 0.3219752754296894559, 0.3333333333333333703, 0.3219752754296894559, 0.3333333333333333703, 0.3219752754296894559, 0.3333333333333333703, 0.3219752754296894559, 0.3333333333333333703, 0.3219752754296894559, 0.3333333333333333703, 0.3219752754296894559, 0.3333333333333333703, 0.3219752754296894559, 0.3333333333333333703, 0.3219752754296894559, 0.3333333333333333703, 0.3219752754296894559, 0.3333333333333333703, 0.3219752754296894559, 0.3333333333333333703, 0.3219752754296894559, 0.3333333333333333703, 0.3219752754296894559, 0.3333333333333333703, 0.3219752754296894559, 0.3333333333333333703, 0.3219752754296894559, 0.3333333333333333703, 0.3219752754296894559, 0.3333333333333333703, 0.3219752754296894559, 0.3333333333333333703, 0.3219752754296894559, 0.3333333333333333703, 0.3219752754296894559, 0.3333333333333333703, 0.3219752754296894559, 0.3333333333333333703, 0.3219752754296894559, 0.3333333333333333703, 0.3219752754296894559, 0.3333333333333333703, 0.3219752754296894559, 0.3333333333333333703, 0.3219752754296894559, 0.3333333333333333703, 0.3219752754296894559, 0.3333333333333333703, 0.3219752754296894559, 0.3333333333333333703, 0.3219752754296894559, 0.3333333333333333703, 0.3219752754296894559, 0.3333333333333333703, 0.3219752754296894559, 0.3333333333333333703, 0.3219752754296894559, 0.3333333333333333703, 0.3219752754296894559, 0.3333333333333333703, 0.3219752754296894559, 0.3333333333333333703, 0.3219752754296894559, 0.3333333333333333703, 0.3219752754296894559, 0.3333333333333333703, 0.3219752754296894559, 0.3333333333333333703, 0.3219752754296894559, 0.3333333333333333703, 0.3219752754296894559, 0.3333333333333333703, 0.3219752754296894559, 0.3333333333333333703, 0.3219752754296894559, 0.3333333333333333703, 0.3219752754296894559, 0.3333333333333333703, 0.3219752754296894559, 0.3333333333333333703, 0.3219752754296894559, 0.3333333333333333703, 0.3219752754296894559, 0.3333333333333333703, 0.3219752754296894559, 0.3333333333333333703, 0.3219752754296894559, 0.3333333333333333703, 0.3219752754296894559, 0.3333333333333333703, 0.3219752754296894559, 0.3333333333333333703, 0.3219752754296894559, 0.3333333333333333703, 0.3219752754296894559, 0.3333333333333333703, 0.3219752754296894559, 0.3333333333333333703, 0.3219752754296894559, 0.3333333333333333703, 0.3219752754296894559, 0.3333333333333333703, 0.3219752754296894559, 0.3333333333333333703, 0.3219752754296894559, 0.3333333333333333703, 0.3219752754296894559, 0.3333333333333333703, 0.3219752754296894559, 0.3333333333333333703, 0.3219752754296894559, 0.3333333333333333703, 0.3219752754296894559, 0.3333333333333333703, 0.3219752754296894559, 0.3333333333333333703, 0.3219752754296894559, 0.3333333333333333703, 0.3219752754296894559, 0.3333333333333333703, 0.3219752754296894559, 0.3333333333333333703, 0.3219752754296894559, 0.3333333333333333703, 0.3219752754296894559, 0.3333333333333333703, 0.3219752754296894559, 0.3333333333333333703, 0.3219752754296894559, 0.3333333333333333703, 0.3219752754296894559, 0.3333333333333333703, 0.3219752754296894559, 0.3333333333333333703, 0.3219752754296894559, 0.3333333333333333703, 0.3219752754296894559, 0.3333333333333333703, 0.3219752754296894559, 0.3333333333333333703, 0.3219752754296894559, 0.3333333333333333703, 0.3219752754296894559, 0.3333333333333333703, 0.3219752754296894559, 0.3333333333333333703, 0.3219752754296894559, 0.3333333333333333703, 0.3219752754296894559, 0.3333333333333333703, 0.3219752754296894559, 0.3333333333333333703, 0.3219752754296894559, 0.3333333333333333703, 0.3219752754296894559, 0.3333333333333333703, 0.3219752754296894559, 0.3333333333333333703, 0.3219752754296894559, 0.3333333333333333703, 0.3219752754296894559, 0.3333333333333333703, 0.3219752754296894559, 0.3333333333333333703, 0.3219752754296894559, 0.3333333333333333703, 0.3219752754296894559, 0.3333333333333333703, 0.3219752754296894559, 0.3333333333333333703, 0.3219752754296894559, 0.3333333333333333703, 0.3219752754296894559, 0.3333333333333333703, 0.3219752754296894559, 0.3333333333333333703, 0.3219752754296894559, 0.3333333333333333703, 0.3219752754296894559, 0.3333333333333333703, 0.3219752754296894559, 0.3333333333333333703, 0.3219752754296894559, 0.3333333333333333703, 0.3219752754296894559, 0.3333333333333333703, 0.3219752754296894559, 0.3333333333333333703, 0.3219752754296894559, 0.3333333333333333703, 0.3219752754296894559, 0.3333333333333333703, 0.3219752754296894559, 0.3333333333333333703, 0.3219752754296894559, 0.3333333333333333703, 0.3219752754296894559, 0.3333333333333333703, 0.3219752754296894559, 0.3333333333333333703, 0.3219752754296894559, 0.3333333333333333703, 0.3219752754296894559, 0.3333333333333333703, 0.3219752754296894559, 0.3333333333333333703, 0.3219752754296894559, 0.3333333333333333703, 0.3219752754296894559, 0.3333333333333333703, 0.3219752754296894559, 0.3333333333333333703, 0.3219752754296894559, 0.3333333333333333703, 0.3219752754296894559, 0.3333333333333333703, 0.3219752754296894559, 0.3333333333333333703, 0.3219752754296894559, 0.3333333333333333703, 0.3219752754296894559, 0.3333333333333333703, 0.3219752754296894559, 0.3333333333333333703, 0.3219752754296894559, 0.3333333333333333703, 0.3219752754296894559, 0.3333333333333333703, 0.3219752754296894559, 0.3333333333333333703, 0.3219752754296894559, 0.3333333333333333703, 0.3219752754296894559, 0.3333333333333333703, 0.3219752754296894559, 0.3333333333333333703, 0.3219752754296894559, 0.3333333333333333703, 0.3219752754296894559, 0.3333333333333333703, 0.3219752754296894559, 0.3333333333333333703, 0.3219752754296894559, 0.3333333333333333703, 0.3219752754296894559, 0.3333333333333333703, 0.3219752754296894559, 0.3333333333333333703, 0.3219752754296894559, 0.3333333333333333703, 0.3219752754296894559, 0.3333333333333333703, 0.3219752754296894559, 0.3333333333333333703, 0.3219752754296894559, 0.3333333333333333703, 0.3219752754296894559, 0.3333333333333333703, 0.3219752754296894559, 0.3333333333333333703, 0.3219752754296894559, 0.3333333333333333703, 0.3219752754296894559, 0.3333333333333333703, 0.3219752754296894559, 0.3333333333333333703, 0.3219752754296894559, 0.3333333333333333703, 0.3219752754296894559, 0.3333333333333333703, 0.3219752754296894559, 0.3333333333333333703, 0.3219752754296894559, 0.3333333333333333703, 0.3219752754296894559, 0.3333333333333333703, 0.3219752754296894559, 0.3333333333333333703, 0.3219752754296894559, 0.3333333333333333703, 0.3219752754296894559, 0.3333333333333333703, 0.3219752754296894559, 0.3333333333333333703, 0.3219752754296894559, 0.3333333333333333703, 0.3219752754296894559, 0.3333333333333333703),
 ( 1.000000000000000000, 0.9659258262890683122, 1.000000000000000000, 0.9659258262890683122, 1.000000000000000000, 0.9659258262890683122, 1.000000000000000000, 0.9659258262890683122, 1.000000000000000000, 0.9659258262890683122, 1.000000000000000000, 0.9659258262890683122, 1.000000000000000000, 0.9659258262890683122, 1.000000000000000000, 0.9659258262890683122, 1.000000000000000000, 0.9659258262890683122, 1.000000000000000000, 0.9659258262890683122, 1.000000000000000000, 0.9659258262890683122, 1.000000000000000000, 0.9659258262890683122, 1.000000000000000000, 0.9659258262890683122, 1.000000000000000000, 0.9659258262890683122, 1.000000000000000000, 0.9659258262890683122, 1.000000000000000000, 0.9659258262890683122, 1.000000000000000000, 0.9659258262890683122, 1.000000000000000000, 0.9659258262890683122, 1.000000000000000000, 0.9659258262890683122, 1.000000000000000000, 0.9659258262890683122, 1.000000000000000000, 0.9659258262890683122, 1.000000000000000000, 0.9659258262890683122, 1.000000000000000000, 0.9659258262890683122, 1.000000000000000000, 0.9659258262890683122, 1.000000000000000000, 0.9659258262890683122, 1.000000000000000000, 0.9659258262890683122, 1.000000000000000000, 0.9659258262890683122, 1.000000000000000000, 0.9659258262890683122, 1.000000000000000000, 0.9659258262890683122, 1.000000000000000000, 0.9659258262890683122, 1.000000000000000000, 0.9659258262890683122, 1.000000000000000000, 0.9659258262890683122, 1.000000000000000000, 0.9659258262890683122, 1.000000000000000000, 0.9659258262890683122, 1.000000000000000000, 0.9659258262890683122, 1.000000000000000000, 0.9659258262890683122, 1.000000000000000000, 0.9659258262890683122, 1.000000000000000000, 0.9659258262890683122, 1.000000000000000000, 0.9659258262890683122, 1.000000000000000000, 0.9659258262890683122, 1.000000000000000000, 0.9659258262890683122, 1.000000000000000000, 0.9659258262890683122, 1.000000000000000000, 0.9659258262890683122, 1.000000000000000000, 0.9659258262890683122, 1.000000000000000000, 0.9659258262890683122, 1.000000000000000000, 0.9659258262890683122, 1.000000000000000000, 0.9659258262890683122, 1.000000000000000000, 0.9659258262890683122, 1.000000000000000000, 0.9659258262890683122, 1.000000000000000000, 0.9659258262890683122, 1.000000000000000000, 0.9659258262890683122, 1.000000000000000000, 0.9659258262890683122, 1.000000000000000000, 0.9659258262890683122, 1.000000000000000000, 0.9659258262890683122, 1.000000000000000000, 0.9659258262890683122, 1.000000000000000000, 0.9659258262890683122, 1.000000000000000000, 0.9659258262890683122, 1.000000000000000000, 0.9659258262890683122, 1.000000000000000000, 0.9659258262890683122, 1.000000000000000000, 0.9659258262890683122, 1.000000000000000000, 0.9659258262890683122, 1.000000000000000000, 0.9659258262890683122, 1.000000000000000000, 0.9659258262890683122, 1.000000000000000000, 0.9659258262890683122, 1.000000000000000000, 0.9659258262890683122, 1.000000000000000000, 0.9659258262890683122, 1.000000000000000000, 0.9659258262890683122, 1.000000000000000000, 0.9659258262890683122, 1.000000000000000000, 0.9659258262890683122, 1.000000000000000000, 0.9659258262890683122, 1.000000000000000000, 0.9659258262890683122, 1.000000000000000000, 0.9659258262890683122, 1.000000000000000000, 0.9659258262890683122, 1.000000000000000000, 0.9659258262890683122, 1.000000000000000000, 0.9659258262890683122, 1.000000000000000000, 0.9659258262890683122, 1.000000000000000000, 0.9659258262890683122, 1.000000000000000000, 0.9659258262890683122, 1.000000000000000000, 0.9659258262890683122, 1.000000000000000000, 0.9659258262890683122, 1.000000000000000000, 0.9659258262890683122, 1.000000000000000000, 0.9659258262890683122, 1.000000000000000000, 0.9659258262890683122, 1.000000000000000000, 0.9659258262890683122, 1.000000000000000000, 0.9659258262890683122, 1.000000000000000000, 0.9659258262890683122, 1.000000000000000000, 0.9659258262890683122, 1.000000000000000000, 0.9659258262890683122, 1.000000000000000000, 0.9659258262890683122, 1.000000000000000000, 0.9659258262890683122, 1.000000000000000000, 0.9659258262890683122, 1.000000000000000000, 0.9659258262890683122, 1.000000000000000000, 0.9659258262890683122, 1.000000000000000000, 0.9659258262890683122, 1.000000000000000000, 0.9659258262890683122, 1.000000000000000000, 0.9659258262890683122, 1.000000000000000000, 0.9659258262890683122, 1.000000000000000000, 0.9659258262890683122, 1.000000000000000000, 0.9659258262890683122, 1.000000000000000000, 0.9659258262890683122, 1.000000000000000000, 0.9659258262890683122, 1.000000000000000000, 0.9659258262890683122, 1.000000000000000000, 0.9659258262890683122, 1.000000000000000000, 0.9659258262890683122, 1.000000000000000000, 0.9659258262890683122, 1.000000000000000000, 0.9659258262890683122, 1.000000000000000000, 0.9659258262890683122, 1.000000000000000000, 0.9659258262890683122, 1.000000000000000000, 0.9659258262890683122, 1.000000000000000000, 0.9659258262890683122, 1.000000000000000000, 0.9659258262890683122, 1.000000000000000000, 0.9659258262890683122, 1.000000000000000000, 0.9659258262890683122, 1.000000000000000000, 0.9659258262890683122, 1.000000000000000000, 0.9659258262890683122, 1.000000000000000000, 0.9659258262890683122, 1.000000000000000000, 0.9659258262890683122, 1.000000000000000000, 0.9659258262890683122, 1.000000000000000000, 0.9659258262890683122, 1.000000000000000000, 0.9659258262890683122, 1.000000000000000000, 0.9659258262890683122, 1.000000000000000000, 0.9659258262890683122, 1.000000000000000000, 0.9659258262890683122, 1.000000000000000000, 0.9659258262890683122, 1.000000000000000000, 0.9659258262890683122, 1.000000000000000000, 0.9659258262890683122, 1.000000000000000000, 0.9659258262890683122, 1.000000000000000000, 0.9659258262890683122, 1.000000000000000000, 0.9659258262890683122, 1.000000000000000000, 0.9659258262890683122, 1.000000000000000000, 0.9659258262890683122, 1.000000000000000000, 0.9659258262890683122, 1.000000000000000000, 0.9659258262890683122, 1.000000000000000000, 0.9659258262890683122, 1.000000000000000000, 0.9659258262890683122, 1.000000000000000000, 0.9659258262890683122, 1.000000000000000000, 0.9659258262890683122, 1.000000000000000000, 0.9659258262890683122, 1.000000000000000000, 0.9659258262890683122, 1.000000000000000000, 0.9659258262890683122, 1.000000000000000000, 0.9659258262890683122, 1.000000000000000000, 0.9659258262890683122, 1.000000000000000000, 0.9659258262890683122, 1.000000000000000000, 0.9659258262890683122, 1.000000000000000000, 0.9659258262890683122, 1.000000000000000000, 0.9659258262890683122, 1.000000000000000000, 0.9659258262890683122, 1.000000000000000000, 0.9659258262890683122, 1.000000000000000000, 0.9659258262890683122, 1.000000000000000000, 0.9659258262890683122, 1.000000000000000000, 0.9659258262890683122, 1.000000000000000000, 0.9659258262890683122, 1.000000000000000000, 0.9659258262890683122, 1.000000000000000000, 0.9659258262890683122, 1.000000000000000000, 0.9659258262890683122, 1.000000000000000000, 0.9659258262890683122, 1.000000000000000000, 0.9659258262890683122, 1.000000000000000000, 0.9659258262890683122, 1.000000000000000000, 0.9659258262890683122, 1.000000000000000000, 0.9659258262890683122, 1.000000000000000000, 0.9659258262890683122, 1.000000000000000000, 0.9659258262890683122, 1.000000000000000000, 0.9659258262890683122, 1.000000000000000000, 0.9659258262890683122, 1.000000000000000000, 0.9659258262890683122, 1.000000000000000000, 0.9659258262890683122, 1.000000000000000000, 0.9659258262890683122, 1.000000000000000000, 0.9659258262890683122, 1.000000000000000000, 0.9659258262890683122, 1.000000000000000000, 0.9659258262890683122, 1.000000000000000000, 0.9659258262890683122, 1.000000000000000000, 0.9659258262890683122, 1.000000000000000000, 0.9659258262890683122, 1.000000000000000000, 0.9659258262890683122, 1.000000000000000000, 0.9659258262890683122, 1.000000000000000000, 0.9659258262890683122, 1.000000000000000000, 0.9659258262890683122, 1.000000000000000000, 0.9659258262890683122, 1.000000000000000000, 0.9659258262890683122, 1.000000000000000000, 0.9659258262890683122, 1.000000000000000000, 0.9659258262890683122, 1.000000000000000000, 0.9659258262890683122, 1.000000000000000000, 0.9659258262890683122, 1.000000000000000000, 0.9659258262890683122, 1.000000000000000000, 0.9659258262890683122, 1.000000000000000000, 0.9659258262890683122, 1.000000000000000000, 0.9659258262890683122, 1.000000000000000000, 0.9659258262890683122, 1.000000000000000000, 0.9659258262890683122, 1.000000000000000000, 0.9659258262890683122, 1.000000000000000000, 0.9659258262890683122, 1.000000000000000000, 0.9659258262890683122, 1.000000000000000000, 0.9659258262890683122, 1.000000000000000000, 0.9659258262890683122, 1.000000000000000000, 0.9659258262890683122, 1.000000000000000000, 0.9659258262890683122, 1.000000000000000000, 0.9659258262890683122, 1.000000000000000000, 0.9659258262890683122, 1.000000000000000000, 0.9659258262890683122, 1.000000000000000000, 0.9659258262890683122, 1.000000000000000000, 0.9659258262890683122, 1.000000000000000000, 0.9659258262890683122, 1.000000000000000000, 0.9659258262890683122, 1.000000000000000000, 0.9659258262890683122, 1.000000000000000000, 0.9659258262890683122, 1.000000000000000000, 0.9659258262890683122, 1.000000000000000000, 0.9659258262890683122, 1.000000000000000000, 0.9659258262890683122, 1.000000000000000000, 0.9659258262890683122, 1.000000000000000000, 0.9659258262890683122, 1.000000000000000000, 0.9659258262890683122, 1.000000000000000000, 0.9659258262890683122, 1.000000000000000000, 0.9659258262890683122, 1.000000000000000000, 0.9659258262890683122, 1.000000000000000000, 0.9659258262890683122, 1.000000000000000000, 0.9659258262890683122, 1.000000000000000000, 0.9659258262890683122, 1.000000000000000000, 0.9659258262890683122, 1.000000000000000000, 0.9659258262890683122, 1.000000000000000000, 0.9659258262890683122, 1.000000000000000000, 0.9659258262890683122, 1.000000000000000000, 0.9659258262890683122, 1.000000000000000000, 0.9659258262890683122, 1.000000000000000000, 0.9659258262890683122, 1.000000000000000000, 0.9659258262890683122, 1.000000000000000000, 0.9659258262890683122, 1.000000000000000000, 0.9659258262890683122, 1.000000000000000000, 0.9659258262890683122, 1.000000000000000000),
 ( 0.3333333333333333703, 0.3219752754296894559, 0.3333333333333333703, 0.3219752754296894559, 0.3333333333333333703, 0.3219752754296894559, 0.3333333333333333703, 0.3219752754296894559, 0.3333333333333333703, 0.3219752754296894559, 0.3333333333333333703, 0.3219752754296894559, 0.3333333333333333703, 0.3219752754296894559, 0.3333333333333333703, 0.3219752754296894559, 0.3333333333333333703, 0.3219752754296894559, 0.3333333333333333703, 0.3219752754296894559, 0.3333333333333333703, 0.3219752754296894559, 0.3333333333333333703, 0.3219752754296894559, 0.3333333333333333703, 0.3219752754296894559, 0.3333333333333333703, 0.3219752754296894559, 0.3333333333333333703, 0.3219752754296894559, 0.3333333333333333703, 0.3219752754296894559, 0.3333333333333333703, 0.3219752754296894559, 0.3333333333333333703, 0.3219752754296894559, 0.3333333333333333703, 0.3219752754296894559, 0.3333333333333333703, 0.3219752754296894559, 0.3333333333333333703, 0.3219752754296894559, 0.3333333333333333703, 0.3219752754296894559, 0.3333333333333333703, 0.3219752754296894559, 0.3333333333333333703, 0.3219752754296894559, 0.3333333333333333703, 0.3219752754296894559, 0.3333333333333333703, 0.3219752754296894559, 0.3333333333333333703, 0.3219752754296894559, 0.3333333333333333703, 0.3219752754296894559, 0.3333333333333333703, 0.3219752754296894559, 0.3333333333333333703, 0.3219752754296894559, 0.3333333333333333703, 0.3219752754296894559, 0.3333333333333333703, 0.3219752754296894559, 0.3333333333333333703, 0.3219752754296894559, 0.3333333333333333703, 0.3219752754296894559, 0.3333333333333333703, 0.3219752754296894559, 0.3333333333333333703, 0.3219752754296894559, 0.3333333333333333703, 0.3219752754296894559, 0.3333333333333333703, 0.3219752754296894559, 0.3333333333333333703, 0.3219752754296894559, 0.3333333333333333703, 0.3219752754296894559, 0.3333333333333333703, 0.3219752754296894559, 0.3333333333333333703, 0.3219752754296894559, 0.3333333333333333703, 0.3219752754296894559, 0.3333333333333333703, 0.3219752754296894559, 0.3333333333333333703, 0.3219752754296894559, 0.3333333333333333703, 0.3219752754296894559, 0.3333333333333333703, 0.3219752754296894559, 0.3333333333333333703, 0.3219752754296894559, 0.3333333333333333703, 0.3219752754296894559, 0.3333333333333333703, 0.3219752754296894559, 0.3333333333333333703, 0.3219752754296894559, 0.3333333333333333703, 0.3219752754296894559, 0.3333333333333333703, 0.3219752754296894559, 0.3333333333333333703, 0.3219752754296894559, 0.3333333333333333703, 0.3219752754296894559, 0.3333333333333333703, 0.3219752754296894559, 0.3333333333333333703, 0.3219752754296894559, 0.3333333333333333703, 0.3219752754296894559, 0.3333333333333333703, 0.3219752754296894559, 0.3333333333333333703, 0.3219752754296894559, 0.3333333333333333703, 0.3219752754296894559, 0.3333333333333333703, 0.3219752754296894559, 0.3333333333333333703, 0.3219752754296894559, 0.3333333333333333703, 0.3219752754296894559, 0.3333333333333333703, 0.3219752754296894559, 0.3333333333333333703, 0.3219752754296894559, 0.3333333333333333703, 0.3219752754296894559, 0.3333333333333333703, 0.3219752754296894559, 0.3333333333333333703, 0.3219752754296894559, 0.3333333333333333703, 0.3219752754296894559, 0.3333333333333333703, 0.3219752754296894559, 0.3333333333333333703, 0.3219752754296894559, 0.3333333333333333703, 0.3219752754296894559, 0.3333333333333333703, 0.3219752754296894559, 0.3333333333333333703, 0.3219752754296894559, 0.3333333333333333703, 0.3219752754296894559, 0.3333333333333333703, 0.3219752754296894559, 0.3333333333333333703, 0.3219752754296894559, 0.3333333333333333703, 0.3219752754296894559, 0.3333333333333333703, 0.3219752754296894559, 0.3333333333333333703, 0.3219752754296894559, 0.3333333333333333703, 0.3219752754296894559, 0.3333333333333333703, 0.3219752754296894559, 0.3333333333333333703, 0.3219752754296894559, 0.3333333333333333703, 0.3219752754296894559, 0.3333333333333333703, 0.3219752754296894559, 0.3333333333333333703, 0.3219752754296894559, 0.3333333333333333703, 0.3219752754296894559, 0.3333333333333333703, 0.3219752754296894559, 0.3333333333333333703, 0.3219752754296894559, 0.3333333333333333703, 0.3219752754296894559, 0.3333333333333333703, 0.3219752754296894559, 0.3333333333333333703, 0.3219752754296894559, 0.3333333333333333703, 0.3219752754296894559, 0.3333333333333333703, 0.3219752754296894559, 0.3333333333333333703, 0.3219752754296894559, 0.3333333333333333703, 0.3219752754296894559, 0.3333333333333333703, 0.3219752754296894559, 0.3333333333333333703, 0.3219752754296894559, 0.3333333333333333703, 0.3219752754296894559, 0.3333333333333333703, 0.3219752754296894559, 0.3333333333333333703, 0.3219752754296894559, 0.3333333333333333703, 0.3219752754296894559, 0.3333333333333333703, 0.3219752754296894559, 0.3333333333333333703, 0.3219752754296894559, 0.3333333333333333703, 0.3219752754296894559, 0.3333333333333333703, 0.3219752754296894559, 0.3333333333333333703, 0.3219752754296894559, 0.3333333333333333703, 0.3219752754296894559, 0.3333333333333333703, 0.3219752754296894559, 0.3333333333333333703, 0.3219752754296894559, 0.3333333333333333703, 0.3219752754296894559, 0.3333333333333333703, 0.3219752754296894559, 0.3333333333333333703, 0.3219752754296894559, 0.3333333333333333703, 0.3219752754296894559, 0.3333333333333333703, 0.3219752754296894559, 0.3333333333333333703, 0.3219752754296894559, 0.3333333333333333703, 0.3219752754296894559, 0.3333333333333333703, 0.3219752754296894559, 0.3333333333333333703, 0.3219752754296894559, 0.3333333333333333703, 0.3219752754296894559, 0.3333333333333333703, 0.3219752754296894559, 0.3333333333333333703, 0.3219752754296894559, 0.3333333333333333703, 0.3219752754296894559, 0.3333333333333333703, 0.3219752754296894559, 0.3333333333333333703, 0.3219752754296894559, 0.3333333333333333703, 0.3219752754296894559, 0.3333333333333333703, 0.3219752754296894559, 0.3333333333333333703, 0.3219752754296894559, 0.3333333333333333703, 0.3219752754296894559, 0.3333333333333333703, 0.3219752754296894559, 0.3333333333333333703, 0.3219752754296894559, 0.3333333333333333703, 0.3219752754296894559, 0.3333333333333333703, 0.3219752754296894559, 0.3333333333333333703, 0.3219752754296894559, 0.3333333333333333703, 0.3219752754296894559, 0.3333333333333333703, 0.3219752754296894559, 0.3333333333333333703, 0.3219752754296894559, 0.3333333333333333703, 0.3219752754296894559, 0.3333333333333333703, 0.3219752754296894559, 0.3333333333333333703, 0.3219752754296894559, 0.3333333333333333703, 0.3219752754296894559, 0.3333333333333333703, 0.3219752754296894559, 0.3333333333333333703, 0.3219752754296894559, 0.3333333333333333703, 0.3219752754296894559, 0.3333333333333333703, 0.3219752754296894559, 0.3333333333333333703, 0.3219752754296894559, 0.3333333333333333703, 0.3219752754296894559, 0.3333333333333333703, 0.3219752754296894559, 0.3333333333333333703, 0.3219752754296894559, 0.3333333333333333703, 0.3219752754296894559, 0.3333333333333333703, 0.3219752754296894559, 0.3333333333333333703, 0.3219752754296894559, 0.3333333333333333703, 0.3219752754296894559, 0.3333333333333333703, 0.3219752754296894559, 0.3333333333333333703, 0.3219752754296894559, 0.3333333333333333703, 0.3219752754296894559, 0.3333333333333333703, 0.3219752754296894559, 0.3333333333333333703, 0.3219752754296894559, 0.3333333333333333703, 0.3219752754296894559, 0.3333333333333333703, 0.3219752754296894559, 0.3333333333333333703, 0.3219752754296894559, 0.3333333333333333703, 0.3219752754296894559, 0.3333333333333333703, 0.3219752754296894559, 0.3333333333333333703, 0.3219752754296894559, 0.3333333333333333703, 0.3219752754296894559, 0.3333333333333333703, 0.3219752754296894559, 0.3333333333333333703, 0.3219752754296894559, 0.3333333333333333703, 0.3219752754296894559, 0.3333333333333333703, 0.3219752754296894559, 0.3333333333333333703, 0.3219752754296894559, 0.3333333333333333703, 0.3219752754296894559, 0.3333333333333333703, 0.3219752754296894559, 0.3333333333333333703, 0.3219752754296894559, 0.3333333333333333703, 0.3219752754296894559, 0.3333333333333333703, 0.3219752754296894559, 0.3333333333333333703, 0.3219752754296894559, 0.3333333333333333703, 0.3219752754296894559, 0.3333333333333333703, 0.3219752754296894559, 0.3333333333333333703, 0.3219752754296894559, 0.3333333333333333703, 0.3219752754296894559, 0.3333333333333333703, 0.3219752754296894559, 0.3333333333333333703, 0.3219752754296894559, 0.3333333333333333703, 0.3219752754296894559, 0.3333333333333333703, 0.3219752754296894559, 0.3333333333333333703, 0.3219752754296894559, 0.3333333333333333703, 0.3219752754296894559, 0.3333333333333333703, 0.3219752754296894559, 0.3333333333333333703, 0.3219752754296894559, 0.3333333333333333703, 0.3219752754296894559, 0.3333333333333333703, 0.3219752754296894559, 0.3333333333333333703, 0.3219752754296894559, 0.3333333333333333703, 0.3219752754296894559, 0.3333333333333333703, 0.3219752754296894559, 0.3333333333333333703, 0.3219752754296894559, 0.3333333333333333703, 0.3219752754296894559, 0.3333333333333333703, 0.3219752754296894559, 0.3333333333333333703, 0.3219752754296894559, 0.3333333333333333703, 0.3219752754296894559, 0.3333333333333333703, 0.3219752754296894559, 0.3333333333333333703, 0.3219752754296894559, 0.3333333333333333703, 0.3219752754296894559, 0.3333333333333333703, 0.3219752754296894559, 0.3333333333333333703, 0.3219752754296894559, 0.3333333333333333703, 0.3219752754296894559, 0.3333333333333333703, 0.3219752754296894559, 0.3333333333333333703, 0.3219752754296894559, 0.3333333333333333703, 0.3219752754296894559, 0.3333333333333333703, 0.3219752754296894559, 0.3333333333333333703, 0.3219752754296894559, 0.3333333333333333703, 0.3219752754296894559, 0.3333333333333333703, 0.3219752754296894559, 0.3333333333333333703, 0.3219752754296894559, 0.3333333333333333703, 0.3219752754296894559, 0.3333333333333333703, 0.3219752754296894559, 0.3333333333333333703, 0.3219752754296894559, 0.3333333333333333703, 0.3219752754296894559, 0.3333333333333333703, 0.3219752754296894559, 0.3333333333333333703, 0.3219752754296894559, 0.3333333333333333703, 0.3219752754296894559, 0.3333333333333333703, 0.3219752754296894559, 0.3333333333333333703, 0.3219752754296894559, 0.3333333333333333703, 0.3219752754296894559, 0.3333333333333333703, 0.3219752754296894559, 0.3333333333333333703, 0.3219752754296894559, 0.3333333333333333703, 0.3219752754296894559, 0.3333333333333333703, 0.3219752754296894559, 0.3333333333333333703, 0.3219752754296894559, 0.3333333333333333703),
 ( 0.3333333333333333703, 0.3219752754296894559, 0.3333333333333333703, 0.3219752754296894559, 0.3333333333333333703, 0.3219752754296894559, 0.3333333333333333703, 0.3219752754296894559, 0.3333333333333333703, 0.3219752754296894559, 0.3333333333333333703, 0.3219752754296894559, 0.3333333333333333703, 0.3219752754296894559, 0.3333333333333333703, 0.3219752754296894559, 0.3333333333333333703, 0.3219752754296894559, 0.3333333333333333703, 0.3219752754296894559, 0.3333333333333333703, 0.3219752754296894559, 0.3333333333333333703, 0.3219752754296894559, 0.3333333333333333703, 0.3219752754296894559, 0.3333333333333333703, 0.3219752754296894559, 0.3333333333333333703, 0.3219752754296894559, 0.3333333333333333703, 0.3219752754296894559, 0.3333333333333333703, 0.3219752754296894559, 0.3333333333333333703, 0.3219752754296894559, 0.3333333333333333703, 0.3219752754296894559, 0.3333333333333333703, 0.3219752754296894559, 0.3333333333333333703, 0.3219752754296894559, 0.3333333333333333703, 0.3219752754296894559, 0.3333333333333333703, 0.3219752754296894559, 0.3333333333333333703, 0.3219752754296894559, 0.3333333333333333703, 0.3219752754296894559, 0.3333333333333333703, 0.3219752754296894559, 0.3333333333333333703, 0.3219752754296894559, 0.3333333333333333703, 0.3219752754296894559, 0.3333333333333333703, 0.3219752754296894559, 0.3333333333333333703, 0.3219752754296894559, 0.3333333333333333703, 0.3219752754296894559, 0.3333333333333333703, 0.3219752754296894559, 0.3333333333333333703, 0.3219752754296894559, 0.3333333333333333703, 0.3219752754296894559, 0.3333333333333333703, 0.3219752754296894559, 0.3333333333333333703, 0.3219752754296894559, 0.3333333333333333703, 0.3219752754296894559, 0.3333333333333333703, 0.3219752754296894559, 0.3333333333333333703, 0.3219752754296894559, 0.3333333333333333703, 0.3219752754296894559, 0.3333333333333333703, 0.3219752754296894559, 0.3333333333333333703, 0.3219752754296894559, 0.3333333333333333703, 0.3219752754296894559, 0.3333333333333333703, 0.3219752754296894559, 0.3333333333333333703, 0.3219752754296894559, 0.3333333333333333703, 0.3219752754296894559, 0.3333333333333333703, 0.3219752754296894559, 0.3333333333333333703, 0.3219752754296894559, 0.3333333333333333703, 0.3219752754296894559, 0.3333333333333333703, 0.3219752754296894559, 0.3333333333333333703, 0.3219752754296894559, 0.3333333333333333703, 0.3219752754296894559, 0.3333333333333333703, 0.3219752754296894559, 0.3333333333333333703, 0.3219752754296894559, 0.3333333333333333703, 0.3219752754296894559, 0.3333333333333333703, 0.3219752754296894559, 0.3333333333333333703, 0.3219752754296894559, 0.3333333333333333703, 0.3219752754296894559, 0.3333333333333333703, 0.3219752754296894559, 0.3333333333333333703, 0.3219752754296894559, 0.3333333333333333703, 0.3219752754296894559, 0.3333333333333333703, 0.3219752754296894559, 0.3333333333333333703, 0.3219752754296894559, 0.3333333333333333703, 0.3219752754296894559, 0.3333333333333333703, 0.3219752754296894559, 0.3333333333333333703, 0.3219752754296894559, 0.3333333333333333703, 0.3219752754296894559, 0.3333333333333333703, 0.3219752754296894559, 0.3333333333333333703, 0.3219752754296894559, 0.3333333333333333703, 0.3219752754296894559, 0.3333333333333333703, 0.3219752754296894559, 0.3333333333333333703, 0.3219752754296894559, 0.3333333333333333703, 0.3219752754296894559, 0.3333333333333333703, 0.3219752754296894559, 0.3333333333333333703, 0.3219752754296894559, 0.3333333333333333703, 0.3219752754296894559, 0.3333333333333333703, 0.3219752754296894559, 0.3333333333333333703, 0.3219752754296894559, 0.3333333333333333703, 0.3219752754296894559, 0.3333333333333333703, 0.3219752754296894559, 0.3333333333333333703, 0.3219752754296894559, 0.3333333333333333703, 0.3219752754296894559, 0.3333333333333333703, 0.3219752754296894559, 0.3333333333333333703, 0.3219752754296894559, 0.3333333333333333703, 0.3219752754296894559, 0.3333333333333333703, 0.3219752754296894559, 0.3333333333333333703, 0.3219752754296894559, 0.3333333333333333703, 0.3219752754296894559, 0.3333333333333333703, 0.3219752754296894559, 0.3333333333333333703, 0.3219752754296894559, 0.3333333333333333703, 0.3219752754296894559, 0.3333333333333333703, 0.3219752754296894559, 0.3333333333333333703, 0.3219752754296894559, 0.3333333333333333703, 0.3219752754296894559, 0.3333333333333333703, 0.3219752754296894559, 0.3333333333333333703, 0.3219752754296894559, 0.3333333333333333703, 0.3219752754296894559, 0.3333333333333333703, 0.3219752754296894559, 0.3333333333333333703, 0.3219752754296894559, 0.3333333333333333703, 0.3219752754296894559, 0.3333333333333333703, 0.3219752754296894559, 0.3333333333333333703, 0.3219752754296894559, 0.3333333333333333703, 0.3219752754296894559, 0.3333333333333333703, 0.3219752754296894559, 0.3333333333333333703, 0.3219752754296894559, 0.3333333333333333703, 0.3219752754296894559, 0.3333333333333333703, 0.3219752754296894559, 0.3333333333333333703, 0.3219752754296894559, 0.3333333333333333703, 0.3219752754296894559, 0.3333333333333333703, 0.3219752754296894559, 0.3333333333333333703, 0.3219752754296894559, 0.3333333333333333703, 0.3219752754296894559, 0.3333333333333333703, 0.3219752754296894559, 0.3333333333333333703, 0.3219752754296894559, 0.3333333333333333703, 0.3219752754296894559, 0.3333333333333333703, 0.3219752754296894559, 0.3333333333333333703, 0.3219752754296894559, 0.3333333333333333703, 0.3219752754296894559, 0.3333333333333333703, 0.3219752754296894559, 0.3333333333333333703, 0.3219752754296894559, 0.3333333333333333703, 0.3219752754296894559, 0.3333333333333333703, 0.3219752754296894559, 0.3333333333333333703, 0.3219752754296894559, 0.3333333333333333703, 0.3219752754296894559, 0.3333333333333333703, 0.3219752754296894559, 0.3333333333333333703, 0.3219752754296894559, 0.3333333333333333703, 0.3219752754296894559, 0.3333333333333333703, 0.3219752754296894559, 0.3333333333333333703, 0.3219752754296894559, 0.3333333333333333703, 0.3219752754296894559, 0.3333333333333333703, 0.3219752754296894559, 0.3333333333333333703, 0.3219752754296894559, 0.3333333333333333703, 0.3219752754296894559, 0.3333333333333333703, 0.3219752754296894559, 0.3333333333333333703, 0.3219752754296894559, 0.3333333333333333703, 0.3219752754296894559, 0.3333333333333333703, 0.3219752754296894559, 0.3333333333333333703, 0.3219752754296894559, 0.3333333333333333703, 0.3219752754296894559, 0.3333333333333333703, 0.3219752754296894559, 0.3333333333333333703, 0.3219752754296894559, 0.3333333333333333703, 0.3219752754296894559, 0.3333333333333333703, 0.3219752754296894559, 0.3333333333333333703, 0.3219752754296894559, 0.3333333333333333703, 0.3219752754296894559, 0.3333333333333333703, 0.3219752754296894559, 0.3333333333333333703, 0.3219752754296894559, 0.3333333333333333703, 0.3219752754296894559, 0.3333333333333333703, 0.3219752754296894559, 0.3333333333333333703, 0.3219752754296894559, 0.3333333333333333703, 0.3219752754296894559, 0.3333333333333333703, 0.3219752754296894559, 0.3333333333333333703, 0.3219752754296894559, 0.3333333333333333703, 0.3219752754296894559, 0.3333333333333333703, 0.3219752754296894559, 0.3333333333333333703, 0.3219752754296894559, 0.3333333333333333703, 0.3219752754296894559, 0.3333333333333333703, 0.3219752754296894559, 0.3333333333333333703, 0.3219752754296894559, 0.3333333333333333703, 0.3219752754296894559, 0.3333333333333333703, 0.3219752754296894559, 0.3333333333333333703, 0.3219752754296894559, 0.3333333333333333703, 0.3219752754296894559, 0.3333333333333333703, 0.3219752754296894559, 0.3333333333333333703, 0.3219752754296894559, 0.3333333333333333703, 0.3219752754296894559, 0.3333333333333333703, 0.3219752754296894559, 0.3333333333333333703, 0.3219752754296894559, 0.3333333333333333703, 0.3219752754296894559, 0.3333333333333333703, 0.3219752754296894559, 0.3333333333333333703, 0.3219752754296894559, 0.3333333333333333703, 0.3219752754296894559, 0.3333333333333333703, 0.3219752754296894559, 0.3333333333333333703, 0.3219752754296894559, 0.3333333333333333703, 0.3219752754296894559, 0.3333333333333333703, 0.3219752754296894559, 0.3333333333333333703, 0.3219752754296894559, 0.3333333333333333703, 0.3219752754296894559, 0.3333333333333333703, 0.3219752754296894559, 0.3333333333333333703, 0.3219752754296894559, 0.3333333333333333703, 0.3219752754296894559, 0.3333333333333333703, 0.3219752754296894559, 0.3333333333333333703, 0.3219752754296894559, 0.3333333333333333703, 0.3219752754296894559, 0.3333333333333333703, 0.3219752754296894559, 0.3333333333333333703, 0.3219752754296894559, 0.3333333333333333703, 0.3219752754296894559, 0.3333333333333333703, 0.3219752754296894559, 0.3333333333333333703, 0.3219752754296894559, 0.3333333333333333703, 0.3219752754296894559, 0.3333333333333333703, 0.3219752754296894559, 0.3333333333333333703, 0.3219752754296894559, 0.3333333333333333703, 0.3219752754296894559, 0.3333333333333333703, 0.3219752754296894559, 0.3333333333333333703, 0.3219752754296894559, 0.3333333333333333703, 0.3219752754296894559, 0.3333333333333333703, 0.3219752754296894559, 0.3333333333333333703, 0.3219752754296894559, 0.3333333333333333703, 0.3219752754296894559, 0.3333333333333333703, 0.3219752754296894559, 0.3333333333333333703, 0.3219752754296894559, 0.3333333333333333703, 0.3219752754296894559, 0.3333333333333333703, 0.3219752754296894559, 0.3333333333333333703, 0.3219752754296894559, 0.3333333333333333703, 0.3219752754296894559, 0.3333333333333333703, 0.3219752754296894559, 0.3333333333333333703, 0.3219752754296894559, 0.3333333333333333703, 0.3219752754296894559, 0.3333333333333333703, 0.3219752754296894559, 0.3333333333333333703, 0.3219752754296894559, 0.3333333333333333703, 0.3219752754296894559, 0.3333333333333333703, 0.3219752754296894559, 0.3333333333333333703, 0.3219752754296894559, 0.3333333333333333703, 0.3219752754296894559, 0.3333333333333333703, 0.3219752754296894559, 0.3333333333333333703, 0.3219752754296894559, 0.3333333333333333703, 0.3219752754296894559, 0.3333333333333333703, 0.3219752754296894559, 0.3333333333333333703, 0.3219752754296894559, 0.3333333333333333703, 0.3219752754296894559, 0.3333333333333333703, 0.3219752754296894559, 0.3333333333333333703, 0.3219752754296894559, 0.3333333333333333703, 0.3219752754296894559, 0.3333333333333333703, 0.3219752754296894559, 0.3333333333333333703, 0.3219752754296894559, 0.3333333333333333703, 0.3219752754296894559, 0.3333333333333333703, 0.3219752754296894559, 0.3333333333333333703, 0.3219752754296894559, 0.3333333333333333703),
 ( 1.000000000000000000, 0.9659258262890683122, 1.000000000000000000, 0.9659258262890683122, 1.000000000000000000, 0.9659258262890683122, 1.000000000000000000, 0.9659258262890683122, 1.000000000000000000, 0.9659258262890683122, 1.000000000000000000, 0.9659258262890683122, 1.000000000000000000, 0.9659258262890683122, 1.000000000000000000, 0.9659258262890683122, 1.000000000000000000, 0.9659258262890683122, 1.000000000000000000, 0.9659258262890683122, 1.000000000000000000, 0.9659258262890683122, 1.000000000000000000, 0.9659258262890683122, 1.000000000000000000, 0.9659258262890683122, 1.000000000000000000, 0.9659258262890683122, 1.000000000000000000, 0.9659258262890683122, 1.000000000000000000, 0.9659258262890683122, 1.000000000000000000, 0.9659258262890683122, 1.000000000000000000, 0.9659258262890683122, 1.000000000000000000, 0.9659258262890683122, 1.000000000000000000, 0.9659258262890683122, 1.000000000000000000, 0.9659258262890683122, 1.000000000000000000, 0.9659258262890683122, 1.000000000000000000, 0.9659258262890683122, 1.000000000000000000, 0.9659258262890683122, 1.000000000000000000, 0.9659258262890683122, 1.000000000000000000, 0.9659258262890683122, 1.000000000000000000, 0.9659258262890683122, 1.000000000000000000, 0.9659258262890683122, 1.000000000000000000, 0.9659258262890683122, 1.000000000000000000, 0.9659258262890683122, 1.000000000000000000, 0.9659258262890683122, 1.000000000000000000, 0.9659258262890683122, 1.000000000000000000, 0.9659258262890683122, 1.000000000000000000, 0.9659258262890683122, 1.000000000000000000, 0.9659258262890683122, 1.000000000000000000, 0.9659258262890683122, 1.000000000000000000, 0.9659258262890683122, 1.000000000000000000, 0.9659258262890683122, 1.000000000000000000, 0.9659258262890683122, 1.000000000000000000, 0.9659258262890683122, 1.000000000000000000, 0.9659258262890683122, 1.000000000000000000, 0.9659258262890683122, 1.000000000000000000, 0.9659258262890683122, 1.000000000000000000, 0.9659258262890683122, 1.000000000000000000, 0.9659258262890683122, 1.000000000000000000, 0.9659258262890683122, 1.000000000000000000, 0.9659258262890683122, 1.000000000000000000, 0.9659258262890683122, 1.000000000000000000, 0.9659258262890683122, 1.000000000000000000, 0.9659258262890683122, 1.000000000000000000, 0.9659258262890683122, 1.000000000000000000, 0.9659258262890683122, 1.000000000000000000, 0.9659258262890683122, 1.000000000000000000, 0.9659258262890683122, 1.000000000000000000, 0.9659258262890683122, 1.000000000000000000, 0.9659258262890683122, 1.000000000000000000, 0.9659258262890683122, 1.000000000000000000, 0.9659258262890683122, 1.000000000000000000, 0.9659258262890683122, 1.000000000000000000, 0.9659258262890683122, 1.000000000000000000, 0.9659258262890683122, 1.000000000000000000, 0.9659258262890683122, 1.000000000000000000, 0.9659258262890683122, 1.000000000000000000, 0.9659258262890683122, 1.000000000000000000, 0.9659258262890683122, 1.000000000000000000, 0.9659258262890683122, 1.000000000000000000, 0.9659258262890683122, 1.000000000000000000, 0.9659258262890683122, 1.000000000000000000, 0.9659258262890683122, 1.000000000000000000, 0.9659258262890683122, 1.000000000000000000, 0.9659258262890683122, 1.000000000000000000, 0.9659258262890683122, 1.000000000000000000, 0.9659258262890683122, 1.000000000000000000, 0.9659258262890683122, 1.000000000000000000, 0.9659258262890683122, 1.000000000000000000, 0.9659258262890683122, 1.000000000000000000, 0.9659258262890683122, 1.000000000000000000, 0.9659258262890683122, 1.000000000000000000, 0.9659258262890683122, 1.000000000000000000, 0.9659258262890683122, 1.000000000000000000, 0.9659258262890683122, 1.000000000000000000, 0.9659258262890683122, 1.000000000000000000, 0.9659258262890683122, 1.000000000000000000, 0.9659258262890683122, 1.000000000000000000, 0.9659258262890683122, 1.000000000000000000, 0.9659258262890683122, 1.000000000000000000, 0.9659258262890683122, 1.000000000000000000, 0.9659258262890683122, 1.000000000000000000, 0.9659258262890683122, 1.000000000000000000, 0.9659258262890683122, 1.000000000000000000, 0.9659258262890683122, 1.000000000000000000, 0.9659258262890683122, 1.000000000000000000, 0.9659258262890683122, 1.000000000000000000, 0.9659258262890683122, 1.000000000000000000, 0.9659258262890683122, 1.000000000000000000, 0.9659258262890683122, 1.000000000000000000, 0.9659258262890683122, 1.000000000000000000, 0.9659258262890683122, 1.000000000000000000, 0.9659258262890683122, 1.000000000000000000, 0.9659258262890683122, 1.000000000000000000, 0.9659258262890683122, 1.000000000000000000, 0.9659258262890683122, 1.000000000000000000, 0.9659258262890683122, 1.000000000000000000, 0.9659258262890683122, 1.000000000000000000, 0.9659258262890683122, 1.000000000000000000, 0.9659258262890683122, 1.000000000000000000, 0.9659258262890683122, 1.000000000000000000, 0.9659258262890683122, 1.000000000000000000, 0.9659258262890683122, 1.000000000000000000, 0.9659258262890683122, 1.000000000000000000, 0.9659258262890683122, 1.000000000000000000, 0.9659258262890683122, 1.000000000000000000, 0.9659258262890683122, 1.000000000000000000, 0.9659258262890683122, 1.000000000000000000, 0.9659258262890683122, 1.000000000000000000, 0.9659258262890683122, 1.000000000000000000, 0.9659258262890683122, 1.000000000000000000, 0.9659258262890683122, 1.000000000000000000, 0.9659258262890683122, 1.000000000000000000, 0.9659258262890683122, 1.000000000000000000, 0.9659258262890683122, 1.000000000000000000, 0.9659258262890683122, 1.000000000000000000, 0.9659258262890683122, 1.000000000000000000, 0.9659258262890683122, 1.000000000000000000, 0.9659258262890683122, 1.000000000000000000, 0.9659258262890683122, 1.000000000000000000, 0.9659258262890683122, 1.000000000000000000, 0.9659258262890683122, 1.000000000000000000, 0.9659258262890683122, 1.000000000000000000, 0.9659258262890683122, 1.000000000000000000, 0.9659258262890683122, 1.000000000000000000, 0.9659258262890683122, 1.000000000000000000, 0.9659258262890683122, 1.000000000000000000, 0.9659258262890683122, 1.000000000000000000, 0.9659258262890683122, 1.000000000000000000, 0.9659258262890683122, 1.000000000000000000, 0.9659258262890683122, 1.000000000000000000, 0.9659258262890683122, 1.000000000000000000, 0.9659258262890683122, 1.000000000000000000, 0.9659258262890683122, 1.000000000000000000, 0.9659258262890683122, 1.000000000000000000, 0.9659258262890683122, 1.000000000000000000, 0.9659258262890683122, 1.000000000000000000, 0.9659258262890683122, 1.000000000000000000, 0.9659258262890683122, 1.000000000000000000, 0.9659258262890683122, 1.000000000000000000, 0.9659258262890683122, 1.000000000000000000, 0.9659258262890683122, 1.000000000000000000, 0.9659258262890683122, 1.000000000000000000, 0.9659258262890683122, 1.000000000000000000, 0.9659258262890683122, 1.000000000000000000, 0.9659258262890683122, 1.000000000000000000, 0.9659258262890683122, 1.000000000000000000, 0.9659258262890683122, 1.000000000000000000, 0.9659258262890683122, 1.000000000000000000, 0.9659258262890683122, 1.000000000000000000, 0.9659258262890683122, 1.000000000000000000, 0.9659258262890683122, 1.000000000000000000, 0.9659258262890683122, 1.000000000000000000, 0.9659258262890683122, 1.000000000000000000, 0.9659258262890683122, 1.000000000000000000, 0.9659258262890683122, 1.000000000000000000, 0.9659258262890683122, 1.000000000000000000, 0.9659258262890683122, 1.000000000000000000, 0.9659258262890683122, 1.000000000000000000, 0.9659258262890683122, 1.000000000000000000, 0.9659258262890683122, 1.000000000000000000, 0.9659258262890683122, 1.000000000000000000, 0.9659258262890683122, 1.000000000000000000, 0.9659258262890683122, 1.000000000000000000, 0.9659258262890683122, 1.000000000000000000, 0.9659258262890683122, 1.000000000000000000, 0.9659258262890683122, 1.000000000000000000, 0.9659258262890683122, 1.000000000000000000, 0.9659258262890683122, 1.000000000000000000, 0.9659258262890683122, 1.000000000000000000, 0.9659258262890683122, 1.000000000000000000, 0.9659258262890683122, 1.000000000000000000, 0.9659258262890683122, 1.000000000000000000, 0.9659258262890683122, 1.000000000000000000, 0.9659258262890683122, 1.000000000000000000, 0.9659258262890683122, 1.000000000000000000, 0.9659258262890683122, 1.000000000000000000, 0.9659258262890683122, 1.000000000000000000, 0.9659258262890683122, 1.000000000000000000, 0.9659258262890683122, 1.000000000000000000, 0.9659258262890683122, 1.000000000000000000, 0.9659258262890683122, 1.000000000000000000, 0.9659258262890683122, 1.000000000000000000, 0.9659258262890683122, 1.000000000000000000, 0.9659258262890683122, 1.000000000000000000, 0.9659258262890683122, 1.000000000000000000, 0.9659258262890683122, 1.000000000000000000, 0.9659258262890683122, 1.000000000000000000, 0.9659258262890683122, 1.000000000000000000, 0.9659258262890683122, 1.000000000000000000, 0.9659258262890683122, 1.000000000000000000, 0.9659258262890683122, 1.000000000000000000, 0.9659258262890683122, 1.000000000000000000, 0.9659258262890683122, 1.000000000000000000, 0.9659258262890683122, 1.000000000000000000, 0.9659258262890683122, 1.000000000000000000, 0.9659258262890683122, 1.000000000000000000, 0.9659258262890683122, 1.000000000000000000, 0.9659258262890683122, 1.000000000000000000, 0.9659258262890683122, 1.000000000000000000, 0.9659258262890683122, 1.000000000000000000, 0.9659258262890683122, 1.000000000000000000, 0.9659258262890683122, 1.000000000000000000, 0.9659258262890683122, 1.000000000000000000, 0.9659258262890683122, 1.000000000000000000, 0.9659258262890683122, 1.000000000000000000, 0.9659258262890683122, 1.000000000000000000, 0.9659258262890683122, 1.000000000000000000, 0.9659258262890683122, 1.000000000000000000, 0.9659258262890683122, 1.000000000000000000, 0.9659258262890683122, 1.000000000000000000, 0.9659258262890683122, 1.000000000000000000, 0.9659258262890683122, 1.000000000000000000, 0.9659258262890683122, 1.000000000000000000, 0.9659258262890683122, 1.000000000000000000, 0.9659258262890683122, 1.000000000000000000, 0.9659258262890683122, 1.000000000000000000, 0.9659258262890683122, 1.000000000000000000, 0.9659258262890683122, 1.000000000000000000, 0.9659258262890683122, 1.000000000000000000, 0.9659258262890683122, 1.000000000000000000, 0.9659258262890683122, 1.000000000000000000) ) ) 
 REPRESENTATION_ITEM ( '' )  SURFACE ( )  );
#103449=CARTESIAN_POINT ( 'NONE',  ( 18.22780087662123805, 5.499999999999960032, 91.48236817873106475 ) ) ;
#103450=CARTESIAN_POINT ( 'NONE',  ( 5.153800228976335163, 19.02544592524342804, 64.79057627198100988 ) ) ;
#103452=CARTESIAN_POINT ( 'NONE',  ( -0.05219959533909027116, -19.03943276465977164, 77.49890960531435269 ) ) ;
#103453=CARTESIAN_POINT ( 'NONE',  ( 19.03943276465977164, -0.05219959533909143690, 83.74890960531436690 ) ) ;
#103454=CARTESIAN_POINT ( 'NONE',  ( 4.483927247898790824, -16.52544592524335698, 65.20942372801901854 ) ) ;
#103456=CARTESIAN_POINT ( 'NONE',  ( -13.89961937509957401, -13.97604488694547875, 44.37609039468566863 ) ) ;
#103458=CARTESIAN_POINT ( 'NONE',  ( 16.51473224551069308, 9.474510206698969483, 109.1655762719810383 ) ) ;
#103459=CARTESIAN_POINT ( 'NONE',  ( -16.55341960407617563, 4.379528057220093196, 103.5427570613523613 ) ) ;
#103461=CARTESIAN_POINT ( 'NONE',  ( -12.14591786802326823, 12.06949235617739902, 93.12609039468568994 ) ) ;
#103462=CARTESIAN_POINT ( 'NONE',  ( -16.62475595723696387, 7.163666690055231712, 30.52713351810466591 ) ) ;
#103463=CARTESIAN_POINT ( 'NONE',  ( -12.06949235617739369, -12.14591786802326823, 69.37609039468567573 ) ) ;
#103465=CARTESIAN_POINT ( 'NONE',  ( -21.52544592524334988, -5.823673210054445271, 68.95942372801901854 ) ) ;
#103466=CARTESIAN_POINT ( 'NONE',  ( -0.05219959533936034679, 19.03943276465977164, 82.50109039468567573 ) ) ;
#103467=CARTESIAN_POINT ( 'NONE',  ( -13.97604488694547697, 13.89961937509957934, 33.12609039468566863 ) ) ;
#103468=CARTESIAN_POINT ( 'NONE',  ( -16.46253265017160317, 9.564922557960807481, 65.83224293864769550 ) ) ;
#103469=CARTESIAN_POINT ( 'NONE',  ( -13.97604488694527625, -13.89961937509977652, 41.87390960531435979 ) ) ;
#103470=CARTESIAN_POINT ( 'NONE',  ( 17.00313601523450302, -6.825168380507106392, 23.22137502641442808 ) ) ;
#103471=CARTESIAN_POINT ( 'NONE',  ( -10.72451020669898014, 18.67979575497178502, 80.41557627198103830 ) ) ;
#103473=CARTESIAN_POINT ( 'NONE',  ( 18.62759615963271287, -10.81492255796078972, 28.33224293864769550 ) ) ;
#103474=CARTESIAN_POINT ( 'NONE',  ( 5.049401038298161559, -19.05341960407611168, 32.70724293864768129 ) ) ;
#103475=CARTESIAN_POINT ( 'NONE',  ( -12.06949235617739369, -12.14591786802326823, 54.37609039468568994 ) ) ;
#103476=ORIENTED_EDGE ( 'NONE', *, *, #15340, .F. ) ;
#103477=CARTESIAN_POINT ( 'NONE',  ( -10.81492255796105439, 18.62759615963255655, 32.91775706135234714 ) ) ;
#103478=CARTESIAN_POINT ( 'NONE',  ( 12.06949235617757843, -12.14591786802309237, 53.12390960531436690 ) ) ;
#103480=CARTESIAN_POINT ( 'NONE',  ( -14.29746914071037622, -8.314922557961029526, 24.16775706135235424 ) ) ;
#103481=CARTESIAN_POINT ( 'NONE',  ( -19.02544592524334988, -5.153800228976617603, 33.95942372801897591 ) ) ;
#103482=CARTESIAN_POINT ( 'NONE',  ( 4.379528057220339221, -16.55341960407611168, 52.70724293864769550 ) ) ;
#103483=CARTESIAN_POINT ( 'NONE',  ( 21.55341960407610458, 5.719274019375980345, 113.9572429386477239 ) ) ;
#103485=CARTESIAN_POINT ( 'NONE',  ( 5.823673210054125526, 21.52544592524343514, 74.79057627198105251 ) ) ;
#103486=CARTESIAN_POINT ( 'NONE',  ( -19.02544592524342804, 5.153800228976336051, 86.04057627198103830 ) ) ;
#103487=CARTESIAN_POINT ( 'NONE',  ( 0.05219959533910956823, 16.53943276465976808, 54.99890960531435269 ) ) ;
#103488=CARTESIAN_POINT ( 'NONE',  ( -19.05341960407611168, -5.049401038298163336, 101.4572429386476955 ) ) ;
#103490=CARTESIAN_POINT ( 'NONE',  ( -16.51473224551082808, 9.474510206698731452, 68.33442372801900433 ) ) ;
#103491=CARTESIAN_POINT ( 'NONE',  ( -21.52544592524343514, 5.823673210054127303, 106.0405762719810525 ) ) ;
#103492=CARTESIAN_POINT ( 'NONE',  ( -0.05219959533909027116, -19.03943276465977164, 52.49890960531436690 ) ) ;
#103493=CARTESIAN_POINT ( 'NONE',  ( 5.153800228976615827, -19.02544592524334988, 45.20942372801901143 ) ) ;
#103494=CARTESIAN_POINT ( 'NONE',  ( -4.483927247898539470, -16.52544592524342804, 107.2905762719810525 ) ) ;
#103495=CARTESIAN_POINT ( 'NONE',  ( 0.05219959533937995610, -21.53943276465977519, 65.00109039468568994 ) ) ;
#103497=CARTESIAN_POINT ( 'NONE',  ( -12.06949235617756955, 12.14591786802309770, 35.62390960531437401 ) ) ;
#103498=CARTESIAN_POINT ( 'NONE',  ( 9.474510206698971260, -16.51473224551069308, 52.91557627198102409 ) ) ;
#103499=CARTESIAN_POINT ( 'NONE',  ( 18.56399227203341695, 5.500000000000001776, 71.47830131249902763 ) ) ;
#103500=CARTESIAN_POINT ( 'NONE',  ( 10.72451020669898902, -18.67979575497178502, 72.91557627198103830 ) ) ;
#103502=CARTESIAN_POINT ( 'NONE',  ( 16.51473224551069308, 9.474510206698969483, 39.16557627198103120 ) ) ;
#103504=CARTESIAN_POINT ( 'NONE',  ( -5.823673210054116645, -21.52544592524344225, 67.29057627198103830 ) ) ;
#103506=CARTESIAN_POINT ( 'NONE',  ( -21.52544592524334988, -5.823673210054445271, 83.95942372801900433 ) ) ;
#103508=CARTESIAN_POINT ( 'NONE',  ( 12.14591786802327356, -12.06949235617739191, 100.6260903946857184 ) ) ;
#103509=CARTESIAN_POINT ( 'NONE',  ( -16.55341960407611168, -4.379528057220339221, 86.45724293864770971 ) ) ;
#103510=CARTESIAN_POINT ( 'NONE',  ( -5.049401038298153566, 19.05341960407611168, 70.20724293864769550 ) ) ;
#103512=CARTESIAN_POINT ( 'NONE',  ( -16.51473224551082808, 9.474510206698731452, 43.33442372801900433 ) ) ;
#103513=CARTESIAN_POINT ( 'NONE',  ( -0.05219959533934338120, 16.53943276465976808, 82.50109039468568994 ) ) ;
#103514=CARTESIAN_POINT ( 'NONE',  ( -5.153800228976607833, 19.02544592524334988, 22.70942372801899012 ) ) ;
#103515=CARTESIAN_POINT ( 'NONE',  ( -5.153800228976328057, -19.02544592524343514, 87.29057627198103830 ) ) ;
#103516=CARTESIAN_POINT ( 'NONE',  ( 5.823673210054125526, 21.52544592524343514, 49.79057627198102409 ) ) ;
#103518=CARTESIAN_POINT ( 'NONE',  ( 0.05219959533937995610, -21.53943276465977519, 100.0010903946857042 ) ) ;
#103519=CARTESIAN_POINT ( 'NONE',  ( 14.34966873604972726, -8.224510206698740333, 65.83442372801900433 ) ) ;
#103520=CARTESIAN_POINT ( 'NONE',  ( -21.53943276465977519, 0.05219959533907696930, 116.2489096053143669 ) ) ;
#103521=CARTESIAN_POINT ( 'NONE',  ( -16.52544592524335698, -4.483927247898792601, 28.95942372801902209 ) ) ;
#103522=CARTESIAN_POINT ( 'NONE',  ( 16.46253265017160672, -9.564922557960803928, 98.33224293864769550 ) ) ;
#103524=CARTESIAN_POINT ( 'NONE',  ( 5.049401038298161559, -19.05341960407611168, 37.70724293864768839 ) ) ;
#103525=CARTESIAN_POINT ( 'NONE',  ( 19.02544592524343514, -5.153800228976328945, 53.54057627198102409 ) ) ;
#103526=CARTESIAN_POINT ( 'NONE',  ( -14.29746914071037622, -8.314922557961029526, 29.16775706135234003 ) ) ;
#103527=CARTESIAN_POINT ( 'NONE',  ( 4.379528057220339221, -16.55341960407611168, 87.70724293864769550 ) ) ;
#103528=CARTESIAN_POINT ( 'NONE',  ( 12.06949235617739724, 12.14591786802326823, 96.87609039468568994 ) ) ;
#103529=CARTESIAN_POINT ( 'NONE',  ( 0.05219959533937995610, -21.53943276465977519, 50.00109039468568994 ) ) ;
#103530=CARTESIAN_POINT ( 'NONE',  ( -9.474510206698964154, 16.51473224551069663, 70.41557627198102409 ) ) ;
#103531=CARTESIAN_POINT ( 'NONE',  ( -19.03943276465977164, 0.05219959533909376836, 51.24890960531436690 ) ) ;
#103532=CARTESIAN_POINT ( 'NONE',  ( 19.02544592524343514, -5.153800228976328945, 78.54057627198099567 ) ) ;
#103533=CARTESIAN_POINT ( 'NONE',  ( 12.14591786802309770, 12.06949235617756955, 34.37390960531435979 ) ) ;
#103534=CARTESIAN_POINT ( 'NONE',  ( -4.379528057220086978, -16.55341960407618274, 104.7927570613523898 ) ) ;
#103535=VERTEX_POINT ( 'NONE', #86789 ) ;
#103536=CARTESIAN_POINT ( 'NONE',  ( 9.474510206698729675, 16.51473224551082808, 37.08442372801899722 ) ) ;
#103537=CARTESIAN_POINT ( 'NONE',  ( -5.153800228976328057, -19.02544592524343514, 107.2905762719810383 ) ) ;
#103539=CARTESIAN_POINT ( 'NONE',  ( -16.46253265017160317, 9.564922557960807481, 50.83224293864770260 ) ) ;
#103540=CARTESIAN_POINT ( 'NONE',  ( -16.51473224551082808, 9.474510206698731452, 28.33442372801900433 ) ) ;
#103542=CARTESIAN_POINT ( 'NONE',  ( 12.06949235617739724, 12.14591786802326823, 46.87609039468568994 ) ) ;
#103543=CARTESIAN_POINT ( 'NONE',  ( 5.049401038297881783, 19.05341960407617563, 67.29275706135234714 ) ) ;
#103544=CARTESIAN_POINT ( 'NONE',  ( -4.379528057220086978, -16.55341960407618274, 49.79275706135234714 ) ) ;
#103546=CARTESIAN_POINT ( 'NONE',  ( 16.46253265017160672, -9.564922557960803928, 78.33224293864769550 ) ) ;
#103547=CARTESIAN_POINT ( 'NONE',  ( 21.55341960407610458, 5.719274019375980345, 113.9572429386477239 ) ) ;
#103548=CARTESIAN_POINT ( 'NONE',  ( 13.97604488694548053, -13.89961937509957401, 65.62609039468567573 ) ) ;
#103549=CARTESIAN_POINT ( 'NONE',  ( 16.46253265017160672, -9.564922557960803928, 103.3322429386476955 ) ) ;
#103550=CARTESIAN_POINT ( 'NONE',  ( -16.46253265017160317, 9.564922557960807481, 35.83224293864768839 ) ) ;
#103551=CARTESIAN_POINT ( 'NONE',  ( 13.89961937509977652, -13.97604488694527269, 73.12390960531436690 ) ) ;
#103552=CARTESIAN_POINT ( 'NONE',  ( 4.379528057220339221, -16.55341960407611168, 37.70724293864769550 ) ) ;
#103553=CARTESIAN_POINT ( 'NONE',  ( 9.564922557960805705, 16.46253265017160317, 39.58224293864768839 ) ) ;
#103554=CARTESIAN_POINT ( 'NONE',  ( 9.564922557961047289, -16.46253265017146816, 35.41775706135233293 ) ) ;
#103555=CARTESIAN_POINT ( 'NONE',  ( -4.483927247898539470, -16.52544592524342804, 77.29057627198102409 ) ) ;
#103556=CARTESIAN_POINT ( 'NONE',  ( 10.72451020669871369, 18.67979575497193778, 112.0844237280190185 ) ) ;
#103557=CARTESIAN_POINT ( 'NONE',  ( -0.05219959533909027116, -19.03943276465977164, 57.49890960531435979 ) ) ;
#103558=CARTESIAN_POINT ( 'NONE',  ( -18.67979575497178146, -10.72451020669898902, 51.66557627198102409 ) ) ;
#103559=CARTESIAN_POINT ( 'NONE',  ( 4.483927247898545687, 16.52544592524342804, 54.79057627198104541 ) ) ;
#103560=CARTESIAN_POINT ( 'NONE',  ( -15.72974639402176322, -15.80617190586768395, 99.37609039468568994 ) ) ;
#103561=CARTESIAN_POINT ( 'NONE',  ( 5.153800228976335163, 19.02544592524342804, 89.79057627198102409 ) ) ;
#103562=CARTESIAN_POINT ( 'NONE',  ( 13.97604488694527802, 13.89961937509977652, 104.3739096053143385 ) ) ;
#103563=CARTESIAN_POINT ( 'NONE',  ( -16.51473224551069308, -9.474510206698971260, 41.66557627198103120 ) ) ;
#103564=CARTESIAN_POINT ( 'NONE',  ( 19.05341960407611168, 5.049401038298154454, 28.95724293864769550 ) ) ;
#103565=CARTESIAN_POINT ( 'NONE',  ( 4.379528057220339221, -16.55341960407611168, 87.70724293864769550 ) ) ;
#103566=CARTESIAN_POINT ( 'NONE',  ( -5.823673210054116645, -21.52544592524344225, 97.29057627198105251 ) ) ;
#103567=CARTESIAN_POINT ( 'NONE',  ( -13.97604488694527625, -13.89961937509977652, 81.87390960531436690 ) ) ;
#103568=CARTESIAN_POINT ( 'NONE',  ( -5.719274019375978568, 21.55341960407610458, 105.2072429386477097 ) ) ;
#103569=CARTESIAN_POINT ( 'NONE',  ( 13.97604488694527802, 13.89961937509977652, 94.37390960531436690 ) ) ;
#103570=LINE ( 'NONE', #117734, #165629 ) ;
#103571=CARTESIAN_POINT ( 'NONE',  ( 14.34966873604960469, 8.224510206698951720, 109.1655762719810383 ) ) ;
#103572=CARTESIAN_POINT ( 'NONE',  ( 9.474510206698971260, -16.51473224551069308, 67.91557627198102409 ) ) ;
#103573=CARTESIAN_POINT ( 'NONE',  ( -5.719274019375978568, 21.55341960407610458, 75.20724293864769550 ) ) ;
#103576=CARTESIAN_POINT ( 'NONE',  ( -5.719274019375978568, 21.55341960407610458, 35.20724293864768839 ) ) ;
#103577=DIRECTION ( 'NONE',  ( 0.000000000000000000, 0.000000000000000000, -1.000000000000000000 ) ) ;
#103578=CARTESIAN_POINT ( 'NONE',  ( 8.314922557961029526, -14.29746914071037800, 30.41775706135234358 ) ) ;
#103579=CARTESIAN_POINT ( 'NONE',  ( -4.483927247898539470, -16.52544592524342804, 92.29057627198103830 ) ) ;
#103580=CARTESIAN_POINT ( 'NONE',  ( 18.56453257813367941, -5.499999999999872102, 53.49000423690684158 ) ) ;
#103581=CARTESIAN_POINT ( 'NONE',  ( -13.97604488694527625, -13.89961937509977652, 91.87390960531432427 ) ) ;
#103582=CARTESIAN_POINT ( 'NONE',  ( -16.51473224551069308, -9.474510206698971260, 41.66557627198103120 ) ) ;
#103583=CARTESIAN_POINT ( 'NONE',  ( -16.53943276465976808, 0.05219959533911058130, 81.24890960531436690 ) ) ;
#103584=CARTESIAN_POINT ( 'NONE',  ( -21.55341960407610458, -5.719274019375992779, 31.45724293864769550 ) ) ;
#103585=CARTESIAN_POINT ( 'NONE',  ( 14.29746914071049879, -8.314922557960816363, 48.33224293864770260 ) ) ;
#103586=CARTESIAN_POINT ( 'NONE',  ( -5.153800228976607833, 19.02544592524334988, 97.70942372801900433 ) ) ;
#103587=CARTESIAN_POINT ( 'NONE',  ( 18.62759615963255655, 10.81492255796105972, 61.66775706135235424 ) ) ;
#103589=CARTESIAN_POINT ( 'NONE',  ( -5.049401038298153566, 19.05341960407611168, 100.2072429386476955 ) ) ;
#103590=CARTESIAN_POINT ( 'NONE',  ( 12.14591786802327356, -12.06949235617739191, 90.62609039468567573 ) ) ;
#103591=CARTESIAN_POINT ( 'NONE',  ( -19.03943276465977164, 0.05219959533909376836, 21.24890960531436335 ) ) ;
#103592=CARTESIAN_POINT ( 'NONE',  ( -5.049401038298153566, 19.05341960407611168, 70.20724293864769550 ) ) ;
#103593=CARTESIAN_POINT ( 'NONE',  ( -5.719274019375978568, 21.55341960407610458, 75.20724293864769550 ) ) ;
#103594=CARTESIAN_POINT ( 'NONE',  ( -9.564922557961040184, 16.46253265017147172, 107.9177570613523471 ) ) ;
#103595=CARTESIAN_POINT ( 'NONE',  ( -4.379528057220328563, 16.55341960407611168, 50.20724293864769550 ) ) ;
#103596=CARTESIAN_POINT ( 'NONE',  ( 21.53943276465977519, 0.05219959533937863772, 56.25109039468568284 ) ) ;
#103597=CARTESIAN_POINT ( 'NONE',  ( 16.52544592524335698, 4.483927247898782831, 81.45942372801900433 ) ) ;
#103598=CARTESIAN_POINT ( 'NONE',  ( 21.55341960407610458, 5.719274019375980345, 28.95724293864769905 ) ) ;
#103599=CARTESIAN_POINT ( 'NONE',  ( 17.49999999999999645, 5.500000000000000888, 28.78230962303566542 ) ) ;
#103600=CARTESIAN_POINT ( 'NONE',  ( -16.81555441253552274, 7.025013491695482948, 80.63685445334257906 ) ) ;
#103601=CARTESIAN_POINT ( 'NONE',  ( -8.224510206698735004, -14.34966873604973081, 104.5844237280190185 ) ) ;
#103602=CARTESIAN_POINT ( 'NONE',  ( 0.05219959533934541429, -16.53943276465976808, 60.00109039468568284 ) ) ;
#103603=CARTESIAN_POINT ( 'NONE',  ( 13.97604488694527802, 13.89961937509977652, 74.37390960531436690 ) ) ;
#103604=CARTESIAN_POINT ( 'NONE',  ( 5.153800228976335163, 19.02544592524342804, 89.79057627198102409 ) ) ;
#103605=CARTESIAN_POINT ( 'NONE',  ( 21.55341960407619695, -5.719274019375665929, 71.04275706135234714 ) ) ;
#103606=CARTESIAN_POINT ( 'NONE',  ( 0.05219959533934541429, -16.53943276465976808, 75.00109039468568994 ) ) ;
#103607=CARTESIAN_POINT ( 'NONE',  ( -16.52544592524342804, 4.483927247898546575, 41.04057627198103120 ) ) ;
#103608=CARTESIAN_POINT ( 'NONE',  ( -13.97604488694527625, -13.89961937509977652, 56.87390960531434558 ) ) ;
#103609=CARTESIAN_POINT ( 'NONE',  ( -5.153800228976328057, -19.02544592524343514, 52.29057627198100988 ) ) ;
#103610=CARTESIAN_POINT ( 'NONE',  ( 16.53943276465976808, 0.05219959533934440121, 36.25109039468567573 ) ) ;
#103612=CARTESIAN_POINT ( 'NONE',  ( -19.03943276465977164, -0.05219959533935918106, 93.75109039468566152 ) ) ;
#103613=CARTESIAN_POINT ( 'NONE',  ( -4.483927247898539470, -16.52544592524342804, 92.29057627198103830 ) ) ;
#103614=CARTESIAN_POINT ( 'NONE',  ( -9.474510206698964154, 16.51473224551069663, 60.41557627198102409 ) ) ;
#103615=CARTESIAN_POINT ( 'NONE',  ( 16.51473224551083163, -9.474510206698727899, 100.8344237280190043 ) ) ;
#103617=CARTESIAN_POINT ( 'NONE',  ( 15.72974639402176855, 15.80617190586768217, 106.8760903946856899 ) ) ;
#103618=CARTESIAN_POINT ( 'NONE',  ( -16.55341960407617563, 4.379528057220093196, 63.54275706135234003 ) ) ;
#103620=CARTESIAN_POINT ( 'NONE',  ( 18.67979575497178502, 10.72451020669898547, 59.16557627198103120 ) ) ;
#103621=CARTESIAN_POINT ( 'NONE',  ( -4.379528057220086978, -16.55341960407618274, 59.79275706135234714 ) ) ;
#103623=CARTESIAN_POINT ( 'NONE',  ( 19.05341960407617918, -5.049401038297876454, 61.04275706135232582 ) ) ;
#103624=CARTESIAN_POINT ( 'NONE',  ( 5.049401038298161559, -19.05341960407611168, 87.70724293864769550 ) ) ;
#103625=CARTESIAN_POINT ( 'NONE',  ( -0.05219959533909027116, -19.03943276465977164, 22.49890960531436690 ) ) ;
#103626=CARTESIAN_POINT ( 'NONE',  ( 19.03943276465977164, -0.05219959533909143690, 68.74890960531436690 ) ) ;
#103627=CARTESIAN_POINT ( 'NONE',  ( 16.53943276465976808, -0.05219959533910856209, 63.74890960531435979 ) ) ;
#103628=CARTESIAN_POINT ( 'NONE',  ( -21.52544592524334988, -5.823673210054445271, 78.95942372801901854 ) ) ;
#103629=CARTESIAN_POINT ( 'NONE',  ( -19.05341960407617563, 5.049401038297882671, 43.54275706135232582 ) ) ;
#103630=CARTESIAN_POINT ( 'NONE',  ( -16.51473224551082808, 9.474510206698731452, 23.33442372801900078 ) ) ;
#103631=CARTESIAN_POINT ( 'NONE',  ( -16.51473224551069308, -9.474510206698971260, 56.66557627198103120 ) ) ;
#103632=CARTESIAN_POINT ( 'NONE',  ( 15.80617190586746368, 15.72974639402197994, 24.37390960531435979 ) ) ;
#103633=CARTESIAN_POINT ( 'NONE',  ( 5.719274019375673035, 21.55341960407619339, 102.2927570613523613 ) ) ;
#103634=CARTESIAN_POINT ( 'NONE',  ( 5.153800228976335163, 19.02544592524342804, 59.79057627198100988 ) ) ;
#103635=CARTESIAN_POINT ( 'NONE',  ( -15.72974639402176322, -15.80617190586768395, 99.37609039468568994 ) ) ;
#103636=CARTESIAN_POINT ( 'NONE',  ( -15.80617190586745835, -15.72974639402198527, 56.87390960531436690 ) ) ;
#103637=CARTESIAN_POINT ( 'NONE',  ( 0.05219959533909260263, 19.03943276465977164, 79.99890960531436690 ) ) ;
#103638=CARTESIAN_POINT ( 'NONE',  ( 5.049401038297881783, 19.05341960407617563, 57.29275706135231871 ) ) ;
#103639=CARTESIAN_POINT ( 'NONE',  ( -19.03943276465977164, 0.05219959533909376836, 36.24890960531436690 ) ) ;
#103640=CARTESIAN_POINT ( 'NONE',  ( -5.049401038298153566, 19.05341960407611168, 95.20724293864770971 ) ) ;
#103641=CARTESIAN_POINT ( 'NONE',  ( -19.03943276465977164, -0.05219959533935918106, 88.75109039468567573 ) ) ;
#103642=CARTESIAN_POINT ( 'NONE',  ( 4.379528057220092307, 16.55341960407617563, 32.29275706135235424 ) ) ;
#103643=CARTESIAN_POINT ( 'NONE',  ( -12.14591786802309592, -12.06949235617757132, 106.8739096053143811 ) ) ;
#103644=CARTESIAN_POINT ( 'NONE',  ( -13.97604488694527625, -13.89961937509977652, 71.87390960531433848 ) ) ;
#103645=CARTESIAN_POINT ( 'NONE',  ( 10.81492255796078972, 18.62759615963270932, 44.58224293864769550 ) ) ;
#103646=CARTESIAN_POINT ( 'NONE',  ( -9.474510206698720793, -16.51473224551083518, 109.5844237280190043 ) ) ;
#103647=CARTESIAN_POINT ( 'NONE',  ( -21.55341960407619339, 5.719274019375674811, 23.54275706135235424 ) ) ;
#103648=CARTESIAN_POINT ( 'NONE',  ( 21.55341960407619695, -5.719274019375665929, 66.04275706135236135 ) ) ;
#103649=CARTESIAN_POINT ( 'NONE',  ( 14.34966873604972726, -8.224510206698740333, 65.83442372801900433 ) ) ;
#103650=CARTESIAN_POINT ( 'NONE',  ( -19.02544592524342804, 5.153800228976336051, 76.04057627198102409 ) ) ;
#103651=CARTESIAN_POINT ( 'NONE',  ( -16.55341960407617563, 4.379528057220093196, 98.54275706135234714 ) ) ;
#103652=CARTESIAN_POINT ( 'NONE',  ( -5.153800228976607833, 19.02544592524334988, 42.70942372801901143 ) ) ;
#103653=CARTESIAN_POINT ( 'NONE',  ( -10.72451020669870658, -18.67979575497194134, 29.58442372801901854 ) ) ;
#103654=CARTESIAN_POINT ( 'NONE',  ( 14.34966873604960469, 8.224510206698951720, 84.16557627198103830 ) ) ;
#103655=CARTESIAN_POINT ( 'NONE',  ( 19.02544592524343514, -5.153800228976328945, 103.5405762719809957 ) ) ;
#103656=CARTESIAN_POINT ( 'NONE',  ( 12.14591786802327356, -12.06949235617739191, 85.62609039468568994 ) ) ;
#103657=CARTESIAN_POINT ( 'NONE',  ( 10.72451020669871369, 18.67979575497193778, 67.08442372801901854 ) ) ;
#103658=CARTESIAN_POINT ( 'NONE',  ( -0.05219959533934338120, 16.53943276465976808, 27.50109039468567929 ) ) ;
#103659=CARTESIAN_POINT ( 'NONE',  ( -15.72974639402176322, -15.80617190586768395, 24.37609039468567573 ) ) ;
#103660=CARTESIAN_POINT ( 'NONE',  ( -4.379528057220328563, 16.55341960407611168, 75.20724293864769550 ) ) ;
#103661=ORIENTED_EDGE ( 'NONE', *, *, #136149, .T. ) ;
#103662=CARTESIAN_POINT ( 'NONE',  ( -15.80617190586745835, -15.72974639402198527, 106.8739096053143811 ) ) ;
#103663=CARTESIAN_POINT ( 'NONE',  ( 14.34966873604960469, 8.224510206698951720, 49.16557627198102409 ) ) ;
#103664=ORIENTED_EDGE ( 'NONE', *, *, #10693, .F. ) ;
#103665=CARTESIAN_POINT ( 'NONE',  ( 19.05341960407611168, 5.049401038298154454, 23.95724293864769194 ) ) ;
#103666=CARTESIAN_POINT ( 'NONE',  ( 10.72451020669898902, -18.67979575497178502, 27.91557627198103830 ) ) ;
#103667=CARTESIAN_POINT ( 'NONE',  ( -21.53943276465977519, -0.05219959533937600094, 33.75109039468568284 ) ) ;
#103668=CARTESIAN_POINT ( 'NONE',  ( 0.05219959533910956823, 16.53943276465976808, 69.99890960531435269 ) ) ;
#103669=CARTESIAN_POINT ( 'NONE',  ( -5.719274019375978568, 21.55341960407610458, 65.20724293864768129 ) ) ;
#103670=CARTESIAN_POINT ( 'NONE',  ( -19.02544592524342804, 5.153800228976336051, 76.04057627198102409 ) ) ;
#103671=CARTESIAN_POINT ( 'NONE',  ( 19.02544592524343514, -5.153800228976328945, 28.54057627198102409 ) ) ;
#103672=CARTESIAN_POINT ( 'NONE',  ( -16.46253265017146816, -9.564922557961047289, 84.16775706135233293 ) ) ;
#103673=CARTESIAN_POINT ( 'NONE',  ( 21.53943276465977519, -0.05219959533907433946, 53.74890960531437401 ) ) ;
#103674=CARTESIAN_POINT ( 'NONE',  ( -19.05341960407611168, -5.049401038298163336, 46.45724293864768129 ) ) ;
#103675=CARTESIAN_POINT ( 'NONE',  ( 5.049401038298161559, -19.05341960407611168, 72.70724293864768129 ) ) ;
#103676=CARTESIAN_POINT ( 'NONE',  ( 16.53943276465976808, 0.05219959533934440121, 31.25109039468568639 ) ) ;
#103677=CARTESIAN_POINT ( 'NONE',  ( 21.53943276465977519, 0.05219959533937863772, 26.25109039468567573 ) ) ;
#103678=CARTESIAN_POINT ( 'NONE',  ( -12.14591786802309592, -12.06949235617757132, 46.87390960531435979 ) ) ;
#103679=CARTESIAN_POINT ( 'NONE',  ( 10.81492255796106328, -18.62759615963255655, 55.41775706135234714 ) ) ;
#103680=CARTESIAN_POINT ( 'NONE',  ( -16.51473224551069308, -9.474510206698971260, 106.6655762719810383 ) ) ;
#103681=CARTESIAN_POINT ( 'NONE',  ( 21.55341960407610458, 5.719274019375980345, 68.95724293864769550 ) ) ;
#103682=CARTESIAN_POINT ( 'NONE',  ( -5.823673210054116645, -21.52544592524344225, 107.2905762719810525 ) ) ;
#103683=CARTESIAN_POINT ( 'NONE',  ( -12.14591786802326823, 12.06949235617739902, 58.12609039468568994 ) ) ;
#103684=CARTESIAN_POINT ( 'NONE',  ( 18.67979575497178502, 10.72451020669898547, 54.16557627198103120 ) ) ;
#103685=CARTESIAN_POINT ( 'NONE',  ( 10.81492255796106328, -18.62759615963255655, 100.4177570613523471 ) ) ;
#103686=CARTESIAN_POINT ( 'NONE',  ( -16.51473224551069308, -9.474510206698971260, 56.66557627198103120 ) ) ;
#103687=CARTESIAN_POINT ( 'NONE',  ( -5.153800228976328057, -19.02544592524343514, 107.2905762719810383 ) ) ;
#103688=CARTESIAN_POINT ( 'NONE',  ( 5.049401038298161559, -19.05341960407611168, 72.70724293864768129 ) ) ;
#103689=CARTESIAN_POINT ( 'NONE',  ( 17.05116617787848554, -6.768360034955522408, 86.15675553259193009 ) ) ;
#103690=CARTESIAN_POINT ( 'NONE',  ( 13.97604488694548053, -13.89961937509957401, 70.62609039468567573 ) ) ;
#103691=CARTESIAN_POINT ( 'NONE',  ( -16.46253265017146816, -9.564922557961047289, 19.16775706135233293 ) ) ;
#103692=CARTESIAN_POINT ( 'NONE',  ( 21.55341960407610458, 5.719274019375980345, 28.95724293864769905 ) ) ;
#103693=CARTESIAN_POINT ( 'NONE',  ( -14.34966873604972548, 8.224510206698743886, 103.3344237280190043 ) ) ;
#103694=CARTESIAN_POINT ( 'NONE',  ( 13.89961937509957401, 13.97604488694547697, 81.87609039468564731 ) ) ;
#103696=CARTESIAN_POINT ( 'NONE',  ( 16.46253265017146816, 9.564922557961045513, 21.66775706135233648 ) ) ;
#103697=CARTESIAN_POINT ( 'NONE',  ( -13.89961937509957401, -13.97604488694547875, 89.37609039468563310 ) ) ;
#103698=CARTESIAN_POINT ( 'NONE',  ( 19.03943276465977164, 0.05219959533936151252, 51.25109039468567573 ) ) ;
#103699=CARTESIAN_POINT ( 'NONE',  ( -17.26172910966777962, -6.454744622555871558, 44.19353091350777163 ) ) ;
#103700=CARTESIAN_POINT ( 'NONE',  ( -5.153800228976328057, -19.02544592524343514, 37.29057627198102409 ) ) ;
#103701=CARTESIAN_POINT ( 'NONE',  ( -12.06949235617756955, 12.14591786802309770, 45.62390960531436690 ) ) ;
#103702=CARTESIAN_POINT ( 'NONE',  ( 9.474510206698971260, -16.51473224551069308, 32.91557627198102409 ) ) ;
#103703=CARTESIAN_POINT ( 'NONE',  ( 12.06949235617757843, -12.14591786802309237, 38.12390960531436690 ) ) ;
#103705=CARTESIAN_POINT ( 'NONE',  ( 12.06949235617739724, 12.14591786802326823, 111.8760903946856615 ) ) ;
#103706=CARTESIAN_POINT ( 'NONE',  ( -19.02544592524342804, 5.153800228976336051, 56.04057627198100988 ) ) ;
#103707=CARTESIAN_POINT ( 'NONE',  ( -0.05219959533936034679, 19.03943276465977164, 27.50109039468566507 ) ) ;
#103708=CARTESIAN_POINT ( 'NONE',  ( -4.379528057220086978, -16.55341960407618274, 29.79275706135234358 ) ) ;
#103709=CARTESIAN_POINT ( 'NONE',  ( 18.62759615963271287, -10.81492255796078972, 38.33224293864768839 ) ) ;
#103710=CARTESIAN_POINT ( 'NONE',  ( 10.81492255796106328, -18.62759615963255655, 90.41775706135236135 ) ) ;
#103712=CARTESIAN_POINT ( 'NONE',  ( -0.05219959533909027116, -19.03943276465977164, 102.4989096053143669 ) ) ;
#103713=CARTESIAN_POINT ( 'NONE',  ( -5.049401038298153566, 19.05341960407611168, 90.20724293864766707 ) ) ;
#103715=CARTESIAN_POINT ( 'NONE',  ( -10.72451020669898014, 18.67979575497178502, 115.4155762719810241 ) ) ;
#103716=CARTESIAN_POINT ( 'NONE',  ( -16.52544592524342804, 4.483927247898546575, 76.04057627198102409 ) ) ;
#103717=CARTESIAN_POINT ( 'NONE',  ( -5.719274019375978568, 21.55341960407610458, 75.20724293864769550 ) ) ;
#103718=CARTESIAN_POINT ( 'NONE',  ( 19.03943276465977164, -0.05219959533909143690, 68.74890960531436690 ) ) ;
#103719=CARTESIAN_POINT ( 'NONE',  ( -9.474510206698964154, 16.51473224551069663, 70.41557627198102409 ) ) ;
#103720=CARTESIAN_POINT ( 'NONE',  ( -21.55341960407610458, -5.719274019375992779, 91.45724293864769550 ) ) ;
#103722=CARTESIAN_POINT ( 'NONE',  ( 9.564922557960805705, 16.46253265017160317, 54.58224293864769550 ) ) ;
#103723=CARTESIAN_POINT ( 'NONE',  ( 16.55341960407611168, 4.379528057220329451, 98.95724293864770971 ) ) ;
#103725=CARTESIAN_POINT ( 'NONE',  ( -16.51473224551069308, -9.474510206698971260, 66.66557627198102409 ) ) ;
#103726=CARTESIAN_POINT ( 'NONE',  ( 16.46253265017146816, 9.564922557961045513, 81.66775706135233293 ) ) ;
#103727=CARTESIAN_POINT ( 'NONE',  ( 16.53943276465976808, -0.05219959533910856209, 103.7489096053143669 ) ) ;
#103728=CARTESIAN_POINT ( 'NONE',  ( 21.55341960407619695, -5.719274019375665929, 56.04275706135235424 ) ) ;
#103729=CARTESIAN_POINT ( 'NONE',  ( 5.153800228976335163, 19.02544592524342804, 54.79057627198103120 ) ) ;
#103730=CARTESIAN_POINT ( 'NONE',  ( 21.55341960407619695, -5.719274019375665929, 26.04275706135235779 ) ) ;
#103731=CARTESIAN_POINT ( 'NONE',  ( -4.379528057220328563, 16.55341960407611168, 105.2072429386477097 ) ) ;
#103733=CARTESIAN_POINT ( 'NONE',  ( 16.51473224551069308, 9.474510206698969483, 74.16557627198103830 ) ) ;
#103735=CARTESIAN_POINT ( 'NONE',  ( 5.049401038297881783, 19.05341960407617563, 107.2927570613523187 ) ) ;
#103736=CARTESIAN_POINT ( 'NONE',  ( 10.72451020669898902, -18.67979575497178502, 22.91557627198102765 ) ) ;
#103737=CARTESIAN_POINT ( 'NONE',  ( -18.62759615963255300, -10.81492255796106328, 44.16775706135234714 ) ) ;
#103738=CARTESIAN_POINT ( 'NONE',  ( 9.564922557960805705, 16.46253265017160317, 99.58224293864770971 ) ) ;
#103739=CARTESIAN_POINT ( 'NONE',  ( 19.02544592524334988, 5.153800228976608722, 86.45942372801900433 ) ) ;
#103740=CARTESIAN_POINT ( 'NONE',  ( -19.05341960407611168, -5.049401038298163336, 51.45724293864770260 ) ) ;
#103741=CARTESIAN_POINT ( 'NONE',  ( -0.05219959533910754901, -16.53943276465976808, 82.49890960531436690 ) ) ;
#103742=CARTESIAN_POINT ( 'NONE',  ( -19.05341960407611168, -5.049401038298163336, 106.4572429386476955 ) ) ;
#103743=CARTESIAN_POINT ( 'NONE',  ( 12.14591786802309770, 12.06949235617756955, 74.37390960531436690 ) ) ;
#103744=CARTESIAN_POINT ( 'NONE',  ( 16.51473224551069308, 9.474510206698969483, 99.16557627198102409 ) ) ;
#103746=CARTESIAN_POINT ( 'NONE',  ( 9.564922557961047289, -16.46253265017146816, 50.41775706135233293 ) ) ;
#103747=CARTESIAN_POINT ( 'NONE',  ( -5.049401038298153566, 19.05341960407611168, 55.20724293864769550 ) ) ;
#103748=CARTESIAN_POINT ( 'NONE',  ( 4.379528057220339221, -16.55341960407611168, 37.70724293864769550 ) ) ;
#103749=CARTESIAN_POINT ( 'NONE',  ( 13.97604488694527802, 13.89961937509977652, 24.37390960531435624 ) ) ;
#103751=CARTESIAN_POINT ( 'NONE',  ( 21.55341960407619695, -5.719274019375665929, 51.04275706135234714 ) ) ;
#103752=CARTESIAN_POINT ( 'NONE',  ( -13.97604488694547697, 13.89961937509957934, 78.12609039468567573 ) ) ;
#103753=CARTESIAN_POINT ( 'NONE',  ( -14.29746914071049879, 8.314922557960819915, 30.83224293864770260 ) ) ;
#103754=CARTESIAN_POINT ( 'NONE',  ( 15.80617190586746368, 15.72974639402197994, 104.3739096053143669 ) ) ;
#103755=CARTESIAN_POINT ( 'NONE',  ( 18.67979575497178502, 10.72451020669898547, 34.16557627198102409 ) ) ;
#103756=CARTESIAN_POINT ( 'NONE',  ( 16.52544592524342804, -4.483927247898539470, 88.54057627198103830 ) ) ;
#103757=CARTESIAN_POINT ( 'NONE',  ( -19.03943276465977164, 0.05219959533909376836, 41.24890960531435269 ) ) ;
#103758=CARTESIAN_POINT ( 'NONE',  ( 14.29746914071037800, 8.314922557961029526, 106.6677570613523756 ) ) ;
#103759=CARTESIAN_POINT ( 'NONE',  ( -4.483927247898782831, 16.52544592524335698, 72.70942372801901854 ) ) ;
#103760=CARTESIAN_POINT ( 'NONE',  ( -16.46253265017146816, -9.564922557961047289, 24.16775706135233648 ) ) ;
#103761=CARTESIAN_POINT ( 'NONE',  ( 16.46253265017160672, -9.564922557960803928, 98.33224293864769550 ) ) ;
#103762=CARTESIAN_POINT ( 'NONE',  ( -13.89961937509977652, 13.97604488694528158, 80.62390960531436690 ) ) ;
#103763=CARTESIAN_POINT ( 'NONE',  ( 8.314922557961029526, -14.29746914071037800, 70.41775706135236135 ) ) ;
#103764=CARTESIAN_POINT ( 'NONE',  ( -9.564922557960796823, -16.46253265017161027, 32.08224293864769550 ) ) ;
#103765=CARTESIAN_POINT ( 'NONE',  ( -8.224510206698948167, 14.34966873604960824, 45.41557627198103830 ) ) ;
#103766=CARTESIAN_POINT ( 'NONE',  ( 13.89961937509977652, -13.97604488694527269, 113.1239096053143527 ) ) ;
#103767=CARTESIAN_POINT ( 'NONE',  ( 0.05219959533909260263, 19.03943276465977164, 84.99890960531436690 ) ) ;
#103768=CARTESIAN_POINT ( 'NONE',  ( 21.53943276465977519, -0.05219959533907433946, 23.74890960531435269 ) ) ;
#103769=CARTESIAN_POINT ( 'NONE',  ( 16.55341960407611168, 4.379528057220329451, 73.95724293864769550 ) ) ;
#103770=CARTESIAN_POINT ( 'NONE',  ( 14.29746914071049879, -8.314922557960816363, 68.33224293864769550 ) ) ;
#103771=CARTESIAN_POINT ( 'NONE',  ( -12.06949235617739369, -12.14591786802326823, 49.37609039468569705 ) ) ;
#103772=CARTESIAN_POINT ( 'NONE',  ( 17.49999999999999645, -3.805241302050391461, 32.87352472782595214 ) ) ;
#103773=CARTESIAN_POINT ( 'NONE',  ( -19.02544592524334988, -5.153800228976617603, 63.95942372801899012 ) ) ;
#103774=CARTESIAN_POINT ( 'NONE',  ( -19.03943276465977164, 0.05219959533909376836, 86.24890960531436690 ) ) ;
#103775=CARTESIAN_POINT ( 'NONE',  ( 13.97604488694548053, -13.89961937509957401, 65.62609039468567573 ) ) ;
#103777=CARTESIAN_POINT ( 'NONE',  ( 16.52544592524335698, 4.483927247898782831, 21.45942372801901499 ) ) ;
#103778=CARTESIAN_POINT ( 'NONE',  ( 12.14591786802327356, -12.06949235617739191, 95.62609039468568994 ) ) ;
#103779=CARTESIAN_POINT ( 'NONE',  ( -19.02544592524342804, 5.153800228976336051, 41.04057627198103120 ) ) ;
#103780=CARTESIAN_POINT ( 'NONE',  ( -18.67979575497178146, -10.72451020669898902, 21.66557627198102409 ) ) ;
#103781=CARTESIAN_POINT ( 'NONE',  ( -15.72974639402176322, -15.80617190586768395, 59.37609039468568284 ) ) ;
#103782=CARTESIAN_POINT ( 'NONE',  ( 4.483927247898790824, -16.52544592524335698, 25.20942372801901854 ) ) ;
#103783=CARTESIAN_POINT ( 'NONE',  ( -5.049401038297874678, -19.05341960407618274, 54.79275706135234003 ) ) ;
#103784=CARTESIAN_POINT ( 'NONE',  ( 16.51473224551069308, 9.474510206698969483, 74.16557627198103830 ) ) ;
#103785=CARTESIAN_POINT ( 'NONE',  ( -13.97604488694527625, -13.89961937509977652, 111.8739096053143243 ) ) ;
#103786=CARTESIAN_POINT ( 'NONE',  ( 14.34966873604960469, 8.224510206698951720, 79.16557627198103830 ) ) ;
#103787=CARTESIAN_POINT ( 'NONE',  ( 5.049401038298161559, -19.05341960407611168, 82.70724293864770971 ) ) ;
#103788=CARTESIAN_POINT ( 'NONE',  ( -5.049401038298153566, 19.05341960407611168, 80.20724293864769550 ) ) ;
#103789=CARTESIAN_POINT ( 'NONE',  ( -9.564922557961040184, 16.46253265017147172, 97.91775706135233293 ) ) ;
#103790=CARTESIAN_POINT ( 'NONE',  ( 5.719274019375991003, -21.55341960407610458, 67.70724293864769550 ) ) ;
#103791=CARTESIAN_POINT ( 'NONE',  ( -5.049401038298153566, 19.05341960407611168, 25.20724293864768484 ) ) ;
#103792=CARTESIAN_POINT ( 'NONE',  ( 9.474510206698729675, 16.51473224551082808, 57.08442372801900433 ) ) ;
#103793=CARTESIAN_POINT ( 'NONE',  ( -13.89961937509977652, 13.97604488694528158, 55.62390960531434558 ) ) ;
#103794=CARTESIAN_POINT ( 'NONE',  ( 9.474510206698971260, -16.51473224551069308, 97.91557627198102409 ) ) ;
#103796=CARTESIAN_POINT ( 'NONE',  ( 21.55341960407610458, 5.719274019375980345, 83.95724293864770971 ) ) ;
#103797=CARTESIAN_POINT ( 'NONE',  ( -16.53943276465976808, 0.05219959533911058130, 91.24890960531436690 ) ) ;
#103798=CARTESIAN_POINT ( 'NONE',  ( -19.02544592524334988, -5.153800228976617603, 43.95942372801899012 ) ) ;
#103799=CARTESIAN_POINT ( 'NONE',  ( 5.823673210054125526, 21.52544592524343514, 69.79057627198102409 ) ) ;
#103800=CARTESIAN_POINT ( 'NONE',  ( 18.62759615963271287, -10.81492255796078972, 73.33224293864769550 ) ) ;
#103801=CARTESIAN_POINT ( 'NONE',  ( -16.53943276465976808, 0.05219959533911058130, 31.24890960531435979 ) ) ;
#103802=CARTESIAN_POINT ( 'NONE',  ( 5.823673210054444382, -21.52544592524334988, 105.2094237280190328 ) ) ;
#103803=CARTESIAN_POINT ( 'NONE',  ( -13.89961937509977652, 13.97604488694528158, 85.62390960531433848 ) ) ;
#103804=CARTESIAN_POINT ( 'NONE',  ( -5.153800228976328057, -19.02544592524343514, 37.29057627198102409 ) ) ;
#103805=CARTESIAN_POINT ( 'NONE',  ( 21.55341960407619695, -5.719274019375665929, 41.04275706135236135 ) ) ;
#103806=CARTESIAN_POINT ( 'NONE',  ( 0.05219959533937995610, -21.53943276465977519, 55.00109039468568284 ) ) ;
#103807=CARTESIAN_POINT ( 'NONE',  ( 13.89961937509977652, -13.97604488694527269, 48.12390960531435979 ) ) ;
#103808=CARTESIAN_POINT ( 'NONE',  ( 21.53943276465977519, 0.05219959533937863772, 26.25109039468567573 ) ) ;
#103809=CARTESIAN_POINT ( 'NONE',  ( -5.153800228976607833, 19.02544592524334988, 62.70942372801899722 ) ) ;
#103810=CARTESIAN_POINT ( 'NONE',  ( 9.474510206698971260, -16.51473224551069308, 32.91557627198102409 ) ) ;
#103811=CARTESIAN_POINT ( 'NONE',  ( 14.34966873604972726, -8.224510206698740333, 30.83442372801902209 ) ) ;
#103812=CARTESIAN_POINT ( 'NONE',  ( -19.03943276465977164, 0.05219959533909376836, 21.24890960531436335 ) ) ;
#103813=CARTESIAN_POINT ( 'NONE',  ( 14.29746914071037800, 8.314922557961029526, 71.66775706135234714 ) ) ;
#103814=CARTESIAN_POINT ( 'NONE',  ( -9.564922557960796823, -16.46253265017161027, 37.08224293864768839 ) ) ;
#103816=CARTESIAN_POINT ( 'NONE',  ( -13.97604488694527625, -13.89961937509977652, 86.87390960531436690 ) ) ;
#103817=CARTESIAN_POINT ( 'NONE',  ( 16.46253265017160672, -9.564922557960803928, 28.33224293864769550 ) ) ;
#103818=CARTESIAN_POINT ( 'NONE',  ( 21.53943276465977519, -0.05219959533907433946, 73.74890960531433848 ) ) ;
#103819=CARTESIAN_POINT ( 'NONE',  ( 14.29746914071037800, 8.314922557961029526, 51.66775706135234714 ) ) ;
#103820=CARTESIAN_POINT ( 'NONE',  ( -18.67979575497193778, 10.72451020669871902, 103.3344237280190043 ) ) ;
#103821=CARTESIAN_POINT ( 'NONE',  ( 19.03943276465977164, -0.05219959533909143690, 38.74890960531436690 ) ) ;
#103822=CARTESIAN_POINT ( 'NONE',  ( -14.29746914071049879, 8.314922557960819915, 30.83224293864770260 ) ) ;
#103823=CARTESIAN_POINT ( 'NONE',  ( -12.14591786802309592, -12.06949235617757132, 71.87390960531438111 ) ) ;
#103824=CARTESIAN_POINT ( 'NONE',  ( -19.03943276465977164, 0.05219959533909376836, 66.24890960531436690 ) ) ;
#103825=CARTESIAN_POINT ( 'NONE',  ( -21.55341960407619339, 5.719274019375674811, 103.5427570613523613 ) ) ;
#103826=CARTESIAN_POINT ( 'NONE',  ( 21.55341960407619695, -5.719274019375665929, 26.04275706135235779 ) ) ;
#103827=CARTESIAN_POINT ( 'NONE',  ( 13.89961937509977652, -13.97604488694527269, 73.12390960531436690 ) ) ;
#103828=CARTESIAN_POINT ( 'NONE',  ( 18.67979575497194134, -10.72451020669871369, 85.83442372801901854 ) ) ;
#103829=CARTESIAN_POINT ( 'NONE',  ( -14.29746914071037622, -8.314922557961029526, 64.16775706135234714 ) ) ;
#103830=CARTESIAN_POINT ( 'NONE',  ( -0.05219959533934338120, 16.53943276465976808, 32.50109039468568284 ) ) ;
#103831=CARTESIAN_POINT ( 'NONE',  ( 14.29746914071049879, -8.314922557960816363, 93.33224293864769550 ) ) ;
#103832=CARTESIAN_POINT ( 'NONE',  ( 10.81492255796106328, -18.62759615963255655, 100.4177570613523471 ) ) ;
#103833=CARTESIAN_POINT ( 'NONE',  ( 14.29746914071049879, -8.314922557960816363, 33.33224293864769550 ) ) ;
#103834=CARTESIAN_POINT ( 'NONE',  ( -5.049401038298153566, 19.05341960407611168, 30.20724293864768839 ) ) ;
#103835=CARTESIAN_POINT ( 'NONE',  ( -16.53943276465976808, -0.05219959533934237506, 53.75109039468568994 ) ) ;
#103836=CARTESIAN_POINT ( 'NONE',  ( -14.34966873604960291, -8.224510206698953496, 56.66557627198103830 ) ) ;
#103837=CARTESIAN_POINT ( 'NONE',  ( 14.34966873604972726, -8.224510206698740333, 95.83442372801903275 ) ) ;
#103838=CARTESIAN_POINT ( 'NONE',  ( 9.564922557960805705, 16.46253265017160317, 109.5822429386476955 ) ) ;
#103839=CARTESIAN_POINT ( 'NONE',  ( 15.72974639402199770, -15.80617190586745480, 38.12390960531436690 ) ) ;
#103840=CARTESIAN_POINT ( 'NONE',  ( -5.049401038297874678, -19.05341960407617918, 19.79275706135233293 ) ) ;
#103841=CARTESIAN_POINT ( 'NONE',  ( -14.29746914071049879, 8.314922557960819915, 80.83224293864769550 ) ) ;
#103842=CARTESIAN_POINT ( 'NONE',  ( 19.03943276465977164, -0.05219959533909143690, 88.74890960531436690 ) ) ;
#103844=CARTESIAN_POINT ( 'NONE',  ( -16.52544592524335698, -4.483927247898792601, 33.95942372801901143 ) ) ;
#103845=CARTESIAN_POINT ( 'NONE',  ( 16.46253265017160672, -9.564922557960803928, 38.33224293864768839 ) ) ;
#103846=CARTESIAN_POINT ( 'NONE',  ( -12.06949235617739369, -12.14591786802326823, 39.37609039468567573 ) ) ;
#103848=CARTESIAN_POINT ( 'NONE',  ( 0.05219959533936267826, -19.03943276465977164, 50.00109039468566863 ) ) ;
#103849=CARTESIAN_POINT ( 'NONE',  ( 0.05219959533909260263, 19.03943276465977164, 39.99890960531436690 ) ) ;
#103850=CARTESIAN_POINT ( 'NONE',  ( -16.53943276465976808, -0.05219959533934237506, 73.75109039468567573 ) ) ;
#103851=CARTESIAN_POINT ( 'NONE',  ( -13.97604488694547697, 13.89961937509957934, 98.12609039468566152 ) ) ;
#103852=CARTESIAN_POINT ( 'NONE',  ( -13.89961937509957401, -13.97604488694547875, 29.37609039468565797 ) ) ;
#103853=CARTESIAN_POINT ( 'NONE',  ( -9.564922557960796823, -16.46253265017161027, 62.08224293864769550 ) ) ;
#103854=CARTESIAN_POINT ( 'NONE',  ( 12.14591786802309770, 12.06949235617756955, 94.37390960531436690 ) ) ;
#103855=CARTESIAN_POINT ( 'NONE',  ( -16.46253265017146816, -9.564922557961047289, 64.16775706135233293 ) ) ;
#103856=CARTESIAN_POINT ( 'NONE',  ( 10.81492255796078972, 18.62759615963270932, 59.58224293864770260 ) ) ;
#103857=CARTESIAN_POINT ( 'NONE',  ( -16.46253265017146816, -9.564922557961047289, 39.16775706135234003 ) ) ;
#103858=CARTESIAN_POINT ( 'NONE',  ( 19.39056639909673763, 5.500000000000001776, 98.28948781074342378 ) ) ;
#103859=CARTESIAN_POINT ( 'NONE',  ( -5.719274019375978568, 21.55341960407610458, 85.20724293864770971 ) ) ;
#103860=CARTESIAN_POINT ( 'NONE',  ( -17.50000000000001776, 5.622605283950872668, 83.68792689403892382 ) ) ;
#103861=CARTESIAN_POINT ( 'NONE',  ( -16.51473224551082808, 9.474510206698731452, 108.3344237280190043 ) ) ;
#103862=CARTESIAN_POINT ( 'NONE',  ( -18.56197773271731677, 5.499999999999904965, 58.55066217314453780 ) ) ;
#103863=CARTESIAN_POINT ( 'NONE',  ( 4.483927247898790824, -16.52544592524335698, 30.20942372801902565 ) ) ;
#103864=CARTESIAN_POINT ( 'NONE',  ( 19.02544592524343514, -5.153800228976328945, 48.54057627198103120 ) ) ;
#103865=CARTESIAN_POINT ( 'NONE',  ( 0.05219959533909260263, 19.03943276465977164, 114.9989096053143669 ) ) ;
#103866=CARTESIAN_POINT ( 'NONE',  ( 21.55341960407610458, 5.719274019375980345, 93.95724293864770971 ) ) ;
#103867=CARTESIAN_POINT ( 'NONE',  ( -18.62759615963255300, -10.81492255796106328, 64.16775706135234714 ) ) ;
#103868=CARTESIAN_POINT ( 'NONE',  ( 9.474510206698729675, 16.51473224551082808, 102.0844237280190043 ) ) ;
#103869=CARTESIAN_POINT ( 'NONE',  ( 0.05219959533936267826, -19.03943276465977164, 20.00109039468567218 ) ) ;
#103870=CARTESIAN_POINT ( 'NONE',  ( 0.05219959533910956823, 16.53943276465976808, 29.99890960531435979 ) ) ;
#103871=CARTESIAN_POINT ( 'NONE',  ( -5.823673210054116645, -21.52544592524344225, 102.2905762719810383 ) ) ;
#103872=CARTESIAN_POINT ( 'NONE',  ( -16.53943276465976808, 0.05219959533911058130, 46.24890960531435979 ) ) ;
#103873=CARTESIAN_POINT ( 'NONE',  ( -5.153800228976607833, 19.02544592524334988, 87.70942372801897591 ) ) ;
#103875=CARTESIAN_POINT ( 'NONE',  ( -16.51473224551082808, 9.474510206698731452, 53.33442372801900433 ) ) ;
#103876=CARTESIAN_POINT ( 'NONE',  ( 21.53943276465977519, 0.05219959533937863772, 76.25109039468568994 ) ) ;
#103877=CARTESIAN_POINT ( 'NONE',  ( -9.564922557961040184, 16.46253265017147172, 37.91775706135233293 ) ) ;
#103878=CARTESIAN_POINT ( 'NONE',  ( -5.049401038298153566, 19.05341960407611168, 25.20724293864768484 ) ) ;
#103879=CARTESIAN_POINT ( 'NONE',  ( -5.823673210054116645, -21.52544592524344225, 47.29057627198103120 ) ) ;
#103880=CARTESIAN_POINT ( 'NONE',  ( -16.55341960407611168, -4.379528057220339221, 36.45724293864768839 ) ) ;
#103881=CARTESIAN_POINT ( 'NONE',  ( -13.89961937509957401, -13.97604488694547875, 19.37609039468566507 ) ) ;
#103882=CARTESIAN_POINT ( 'NONE',  ( -14.29746914071037622, -8.314922557961029526, 69.16775706135234714 ) ) ;
#103883=CARTESIAN_POINT ( 'NONE',  ( 4.379528057220339221, -16.55341960407611168, 42.70724293864770260 ) ) ;
#103884=CARTESIAN_POINT ( 'NONE',  ( 10.72451020669871369, 18.67979575497193778, 72.08442372801899012 ) ) ;
#103885=CARTESIAN_POINT ( 'NONE',  ( 18.67979575497194134, -10.72451020669871369, 70.83442372801901854 ) ) ;
#103886=CARTESIAN_POINT ( 'NONE',  ( -15.80617190586745835, -15.72974639402198527, 61.87390960531436690 ) ) ;
#103887=CARTESIAN_POINT ( 'NONE',  ( -5.153800228976328057, -19.02544592524343514, 42.29057627198101699 ) ) ;
#103888=CARTESIAN_POINT ( 'NONE',  ( 21.55341960407619695, -5.719274019375665929, 46.04275706135234714 ) ) ;
#103889=CARTESIAN_POINT ( 'NONE',  ( -4.483927247898539470, -16.52544592524342804, 112.2905762719810241 ) ) ;
#103890=CARTESIAN_POINT ( 'NONE',  ( 13.97604488694527802, 13.89961937509977652, 39.37390960531435269 ) ) ;
#103891=CARTESIAN_POINT ( 'NONE',  ( 4.379528057220339221, -16.55341960407611168, 87.70724293864769550 ) ) ;
#103892=CARTESIAN_POINT ( 'NONE',  ( 19.03943276465977164, -0.05219959533909143690, 83.74890960531436690 ) ) ;
#103893=CARTESIAN_POINT ( 'NONE',  ( 12.14591786802309770, 12.06949235617756955, 44.37390960531435979 ) ) ;
#103894=CARTESIAN_POINT ( 'NONE',  ( 8.224510206698953496, -14.34966873604960469, 102.9155762719810383 ) ) ;
#103895=CARTESIAN_POINT ( 'NONE',  ( 15.72974639402199770, -15.80617190586745480, 63.12390960531435979 ) ) ;
#103896=CARTESIAN_POINT ( 'NONE',  ( 18.62759615963271287, -10.81492255796078972, 108.3322429386477097 ) ) ;
#103897=CARTESIAN_POINT ( 'NONE',  ( -16.46253265017160317, 9.564922557960807481, 115.8322429386477097 ) ) ;
#103898=CARTESIAN_POINT ( 'NONE',  ( 5.153800228976335163, 19.02544592524342804, 59.79057627198100988 ) ) ;
#103899=CARTESIAN_POINT ( 'NONE',  ( 0.05219959533934541429, -16.53943276465976808, 30.00109039468568284 ) ) ;
#103900=CARTESIAN_POINT ( 'NONE',  ( -15.80617190586745835, -15.72974639402198527, 56.87390960531436690 ) ) ;
#103901=CARTESIAN_POINT ( 'NONE',  ( -15.72974639402176322, -15.80617190586768395, 89.37609039468568994 ) ) ;
#103902=CARTESIAN_POINT ( 'NONE',  ( 19.02544592524343514, -5.153800228976328945, 73.54057627198103830 ) ) ;
#103903=CARTESIAN_POINT ( 'NONE',  ( 5.823673210054125526, 21.52544592524343514, 114.7905762719810383 ) ) ;
#103904=CARTESIAN_POINT ( 'NONE',  ( -16.51473224551069308, -9.474510206698971260, 106.6655762719810383 ) ) ;
#103905=CARTESIAN_POINT ( 'NONE',  ( 4.483927247898790824, -16.52544592524335698, 90.20942372801903275 ) ) ;
#103906=CARTESIAN_POINT ( 'NONE',  ( 0.05219959533937995610, -21.53943276465977519, 70.00109039468568994 ) ) ;
#103907=CARTESIAN_POINT ( 'NONE',  ( -0.05219959533937732626, 21.53943276465977519, 102.5010903946856899 ) ) ;
#103908=CARTESIAN_POINT ( 'NONE',  ( 4.483927247898790824, -16.52544592524335698, 55.20942372801902565 ) ) ;
#103909=CARTESIAN_POINT ( 'NONE',  ( -21.55341960407610458, -5.719274019375992779, 111.4572429386476813 ) ) ;
#103910=CARTESIAN_POINT ( 'NONE',  ( -13.97604488694527625, -13.89961937509977652, 21.87390960531435979 ) ) ;
#103911=CARTESIAN_POINT ( 'NONE',  ( 5.823673210054444382, -21.52544592524334988, 95.20942372801903275 ) ) ;
#103913=CARTESIAN_POINT ( 'NONE',  ( 18.62759615963271287, -10.81492255796078972, 88.33224293864769550 ) ) ;
#103914=CARTESIAN_POINT ( 'NONE',  ( -16.51473224551082808, 9.474510206698731452, 48.33442372801900433 ) ) ;
#103915=CARTESIAN_POINT ( 'NONE',  ( 15.72974639402199770, -15.80617190586745480, 53.12390960531436690 ) ) ;
#103916=CARTESIAN_POINT ( 'NONE',  ( -19.05341960407611168, -5.049401038298163336, 101.4572429386476955 ) ) ;
#103917=CARTESIAN_POINT ( 'NONE',  ( -4.379528057220328563, 16.55341960407611168, 40.20724293864769550 ) ) ;
#103920=CARTESIAN_POINT ( 'NONE',  ( 19.02544592524334988, 5.153800228976608722, 106.4594237280190185 ) ) ;
#103921=CARTESIAN_POINT ( 'NONE',  ( 5.719274019375991003, -21.55341960407610458, 87.70724293864769550 ) ) ;
#103922=CARTESIAN_POINT ( 'NONE',  ( -16.53943276465976808, 0.05219959533911058130, 46.24890960531435979 ) ) ;
#103923=CARTESIAN_POINT ( 'NONE',  ( -16.52544592524335698, -4.483927247898792601, 28.95942372801902209 ) ) ;
#103924=CARTESIAN_POINT ( 'NONE',  ( 19.05341960407611168, 5.049401038298154454, 38.95724293864767418 ) ) ;
#103925=CARTESIAN_POINT ( 'NONE',  ( -10.72451020669870658, -18.67979575497194134, 19.58442372801901143 ) ) ;
#103926=CARTESIAN_POINT ( 'NONE',  ( 9.474510206698729675, 16.51473224551082808, 82.08442372801899012 ) ) ;
#103927=CARTESIAN_POINT ( 'NONE',  ( 19.03943276465977164, -0.05219959533909143690, 83.74890960531436690 ) ) ;
#103928=CARTESIAN_POINT ( 'NONE',  ( 9.564922557960805705, 16.46253265017160317, 74.58224293864769550 ) ) ;
#103929=CARTESIAN_POINT ( 'NONE',  ( 5.719274019375991003, -21.55341960407610458, 77.70724293864770971 ) ) ;
#103930=CARTESIAN_POINT ( 'NONE',  ( 13.89961937509977652, -13.97604488694527269, 38.12390960531436690 ) ) ;
#103932=CARTESIAN_POINT ( 'NONE',  ( -16.53943276465976808, 0.05219959533911058130, 61.24890960531435979 ) ) ;
#103933=CARTESIAN_POINT ( 'NONE',  ( 0.05219959533909260263, 19.03943276465977164, 84.99890960531436690 ) ) ;
#103935=CARTESIAN_POINT ( 'NONE',  ( 13.97604488694548053, -13.89961937509957401, 60.62609039468564731 ) ) ;
#103936=CARTESIAN_POINT ( 'NONE',  ( -18.67979575497178146, -10.72451020669898902, 81.66557627198103830 ) ) ;
#103937=CARTESIAN_POINT ( 'NONE',  ( 19.05341960407617918, -5.049401038297876454, 31.04275706135232227 ) ) ;
#103938=CARTESIAN_POINT ( 'NONE',  ( -13.89961937509977652, 13.97604488694528158, 105.6239096053143527 ) ) ;
#103940=CARTESIAN_POINT ( 'NONE',  ( 0.05219959533907565091, 21.53943276465977519, 39.99890960531436690 ) ) ;
#103941=CARTESIAN_POINT ( 'NONE',  ( 0.05219959533909260263, 19.03943276465977164, 74.99890960531435269 ) ) ;
#103942=CARTESIAN_POINT ( 'NONE',  ( -10.72451020669870658, -18.67979575497194134, 54.58442372801901143 ) ) ;
#103943=CARTESIAN_POINT ( 'NONE',  ( -19.03943276465977164, 0.05219959533909376836, 31.24890960531435979 ) ) ;
#103945=CARTESIAN_POINT ( 'NONE',  ( -5.823673210054431948, 21.52544592524334988, 22.70942372801901499 ) ) ;
#103947=CARTESIAN_POINT ( 'NONE',  ( 18.62759615963255655, 10.81492255796105972, 36.66775706135234714 ) ) ;
#103949=CARTESIAN_POINT ( 'NONE',  ( 19.05341960407611168, 5.049401038298154454, 103.9572429386476671 ) ) ;
#103950=AXIS2_PLACEMENT_3D ( 'NONE', #177150, #21446, #83107 ) ;
#103951=CARTESIAN_POINT ( 'NONE',  ( 5.153800228976335163, 19.02544592524342804, 89.79057627198102409 ) ) ;
#103952=CARTESIAN_POINT ( 'NONE',  ( -10.81492255796078084, -18.62759615963271287, 102.0822429386476955 ) ) ;
#103953=CARTESIAN_POINT ( 'NONE',  ( -16.51473224551069308, -9.474510206698971260, 56.66557627198103120 ) ) ;
#103954=CARTESIAN_POINT ( 'NONE',  ( 8.224510206698742110, 14.34966873604972548, 22.08442372801901143 ) ) ;
#103956=CARTESIAN_POINT ( 'NONE',  ( -15.80617190586768217, 15.72974639402176855, 103.1260903946856757 ) ) ;
#103957=CARTESIAN_POINT ( 'NONE',  ( 5.049401038298161559, -19.05341960407611168, 47.70724293864770260 ) ) ;
#103958=CARTESIAN_POINT ( 'NONE',  ( 15.72974639402176855, 15.80617190586768217, 101.8760903946857042 ) ) ;
#103960=CARTESIAN_POINT ( 'NONE',  ( 19.02544592524343514, -5.153800228976328945, 93.54057627198102409 ) ) ;
#103961=CARTESIAN_POINT ( 'NONE',  ( -18.62759615963255300, -10.81492255796106328, 59.16775706135234714 ) ) ;
#103963=CARTESIAN_POINT ( 'NONE',  ( 16.46253265017160672, -9.564922557960803928, 108.3322429386476955 ) ) ;
#103964=CARTESIAN_POINT ( 'NONE',  ( 17.50000000000000000, 5.499999999999992895, 46.70309617465829888 ) ) ;
#103965=CARTESIAN_POINT ( 'NONE',  ( 16.53943276465976808, 0.05219959533934440121, 56.25109039468568284 ) ) ;
#103966=CARTESIAN_POINT ( 'NONE',  ( 0.05219959533937995610, -21.53943276465977519, 60.00109039468568284 ) ) ;
#103967=CARTESIAN_POINT ( 'NONE',  ( -10.72451020669870658, -18.67979575497194134, 84.58442372801903275 ) ) ;
#103969=CARTESIAN_POINT ( 'NONE',  ( 12.06949235617739724, 12.14591786802326823, 21.87609039468567573 ) ) ;
#103970=CARTESIAN_POINT ( 'NONE',  ( -9.564922557960796823, -16.46253265017161027, 67.08224293864769550 ) ) ;
#103971=CARTESIAN_POINT ( 'NONE',  ( -19.05341960407611168, -5.049401038298163336, 21.45724293864768839 ) ) ;
#103972=DIRECTION ( 'NONE',  ( 0.000000000000000000, 0.000000000000000000, 1.000000000000000000 ) ) ;
#103973=CARTESIAN_POINT ( 'NONE',  ( 19.03943276465977164, -0.05219959533909143690, 28.74890960531435624 ) ) ;
#103974=CARTESIAN_POINT ( 'NONE',  ( 15.80617190586746368, 15.72974639402197994, 39.37390960531436690 ) ) ;
#103975=CARTESIAN_POINT ( 'NONE',  ( -14.34966873604972548, 8.224510206698743886, 98.33442372801901854 ) ) ;
#103976=CARTESIAN_POINT ( 'NONE',  ( 16.55341960407611168, 4.379528057220329451, 78.95724293864769550 ) ) ;
#103977=CARTESIAN_POINT ( 'NONE',  ( -9.564922557960796823, -16.46253265017161027, 72.08224293864770971 ) ) ;
#103978=CARTESIAN_POINT ( 'NONE',  ( -10.72451020669870658, -18.67979575497194134, 84.58442372801903275 ) ) ;
#103980=CARTESIAN_POINT ( 'NONE',  ( 8.224510206698742110, 14.34966873604972548, 27.08442372801901854 ) ) ;
#103981=CARTESIAN_POINT ( 'NONE',  ( -4.483927247898539470, -16.52544592524342804, 92.29057627198103830 ) ) ;
#103982=CARTESIAN_POINT ( 'NONE',  ( 15.72974639402176855, 15.80617190586768217, 36.87609039468568994 ) ) ;
#103983=CARTESIAN_POINT ( 'NONE',  ( 18.62759615963271287, -10.81492255796078972, 73.33224293864769550 ) ) ;
#103984=CARTESIAN_POINT ( 'NONE',  ( -16.46253265017146816, -9.564922557961047289, 34.16775706135233293 ) ) ;
#103986=CARTESIAN_POINT ( 'NONE',  ( 13.97604488694527802, 13.89961937509977652, 84.37390960531433848 ) ) ;
#103987=CARTESIAN_POINT ( 'NONE',  ( 16.52544592524342804, -4.483927247898539470, 58.54057627198103120 ) ) ;
#103988=CARTESIAN_POINT ( 'NONE',  ( -8.224510206698948167, 14.34966873604960824, 35.41557627198102409 ) ) ;
#103989=CARTESIAN_POINT ( 'NONE',  ( -4.379528057220086978, -16.55341960407618274, 104.7927570613523898 ) ) ;
#103990=CARTESIAN_POINT ( 'NONE',  ( 16.46253265017146816, 9.564922557961045513, 66.66775706135233293 ) ) ;
#103991=CARTESIAN_POINT ( 'NONE',  ( 19.25918095147782338, 5.499999999999580780, 51.95284276293935477 ) ) ;
#103992=CARTESIAN_POINT ( 'NONE',  ( 5.823673210054125526, 21.52544592524343514, 24.79057627198103120 ) ) ;
#103993=CARTESIAN_POINT ( 'NONE',  ( -16.55341960407611168, -4.379528057220339221, 86.45724293864770971 ) ) ;
#103994=B_SPLINE_CURVE_WITH_KNOTS ( 'NONE', 3,
 ( #27096, #89737, #139212, #182754, #151423, #168557, #29076, #140198, #61371, #59386, #43243, #12910, #154387, #62358, #123042, #47216, #166598, #169552, #44238, #184728, #198912, #14888, #60380, #122052, #78524, #92699, #31050, #138225, #687, #76549, #120073, #74574 ),
 .UNSPECIFIED., .F., .F.,
 ( 4, 2, 2, 2, 2, 2, 2, 2, 2, 2, 2, 2, 2, 2, 2, 4 ),
 ( 2.539163526713095107E-17, 0.0003712461730036932289, 0.0007424923460073610875, 0.001113738519011029000, 0.001484984692014696805, 0.002227477038022051496, 0.002598723211025728407, 0.002969969384029405319, 0.003341215557033082231, 0.003712461730036759576, 0.004083707903040436488, 0.004454954076044113399, 0.004826200249047790311, 0.005197446422051468090, 0.005568692595055144134, 0.005939938768058821913 ),
 .UNSPECIFIED. ) ;
#103996=CARTESIAN_POINT ( 'NONE',  ( 19.05341960407611168, 5.049401038298154454, 48.95724293864768129 ) ) ;
#103997=CARTESIAN_POINT ( 'NONE',  ( -18.67979575497178146, -10.72451020669898902, 46.66557627198102409 ) ) ;
#103998=CARTESIAN_POINT ( 'NONE',  ( -5.719274019375978568, 21.55341960407610458, 65.20724293864768129 ) ) ;
#103999=CARTESIAN_POINT ( 'NONE',  ( -8.314922557960811034, -14.29746914071050412, 107.0822429386476955 ) ) ;
#104000=CARTESIAN_POINT ( 'NONE',  ( 14.34966873604972726, -8.224510206698740333, 65.83442372801900433 ) ) ;
#104001=CARTESIAN_POINT ( 'NONE',  ( -16.46253265017160317, 9.564922557960807481, 45.83224293864769550 ) ) ;
#104002=CARTESIAN_POINT ( 'NONE',  ( 21.52544592524334988, 5.823673210054432836, 56.45942372801902565 ) ) ;
#104003=ORIENTED_EDGE ( 'NONE', *, *, #186989, .T. ) ;
#104004=CARTESIAN_POINT ( 'NONE',  ( -16.52544592524342804, 4.483927247898546575, 106.0405762719810525 ) ) ;
#104005=CARTESIAN_POINT ( 'NONE',  ( 0.05219959533936267826, -19.03943276465977164, 95.00109039468567573 ) ) ;
#104008=CARTESIAN_POINT ( 'NONE',  ( 21.53943276465977519, -0.05219959533907433946, 38.74890960531435979 ) ) ;
#104009=CARTESIAN_POINT ( 'NONE',  ( -9.564922557960796823, -16.46253265017161027, 22.08224293864768839 ) ) ;
#104010=CARTESIAN_POINT ( 'NONE',  ( 21.53943276465977519, 0.05219959533937863772, 66.25109039468567573 ) ) ;
#104011=CARTESIAN_POINT ( 'NONE',  ( -8.224510206698735004, -14.34966873604973081, 59.58442372801901854 ) ) ;
#104012=CARTESIAN_POINT ( 'NONE',  ( 16.53943276465976808, -0.05219959533910856209, 43.74890960531435979 ) ) ;
#104013=CARTESIAN_POINT ( 'NONE',  ( 15.72974639402199770, -15.80617190586745480, 63.12390960531435979 ) ) ;
#104014=CARTESIAN_POINT ( 'NONE',  ( 5.719274019375991003, -21.55341960407610458, 67.70724293864769550 ) ) ;
#104016=CARTESIAN_POINT ( 'NONE',  ( -5.153800228976607833, 19.02544592524334988, 87.70942372801897591 ) ) ;
#104017=CARTESIAN_POINT ( 'NONE',  ( -16.51473224551069308, -9.474510206698971260, 111.6655762719810383 ) ) ;
#104018=CARTESIAN_POINT ( 'NONE',  ( 19.02544592524343514, -5.153800228976328945, 53.54057627198102409 ) ) ;
#104019=CARTESIAN_POINT ( 'NONE',  ( 13.97604488694527802, 13.89961937509977652, 24.37390960531435624 ) ) ;
#104021=CARTESIAN_POINT ( 'NONE',  ( -5.049401038298153566, 19.05341960407611168, 110.2072429386476671 ) ) ;
#104023=CARTESIAN_POINT ( 'NONE',  ( -8.224510206698735004, -14.34966873604973081, 64.58442372801900433 ) ) ;
#104024=CARTESIAN_POINT ( 'NONE',  ( 18.67979575497178502, 10.72451020669898547, 99.16557627198100988 ) ) ;
#104025=CARTESIAN_POINT ( 'NONE',  ( -16.46253265017160317, 9.564922557960807481, 75.83224293864769550 ) ) ;
#104026=CARTESIAN_POINT ( 'NONE',  ( 5.719274019375673035, 21.55341960407619339, 42.29275706135235424 ) ) ;
#104027=CARTESIAN_POINT ( 'NONE',  ( 13.97604488694527802, 13.89961937509977652, 99.37390960531436690 ) ) ;
#104030=CARTESIAN_POINT ( 'NONE',  ( 18.67979575497194134, -10.72451020669871369, 35.83442372801901143 ) ) ;
#104031=CARTESIAN_POINT ( 'NONE',  ( -5.153800228976328057, -19.02544592524343514, 27.29057627198103120 ) ) ;
#104032=CARTESIAN_POINT ( 'NONE',  ( 5.153800228976615827, -19.02544592524334988, 85.20942372801900433 ) ) ;
#104033=CARTESIAN_POINT ( 'NONE',  ( -13.89961937509957401, -13.97604488694547875, 39.37609039468566152 ) ) ;
#104034=CARTESIAN_POINT ( 'NONE',  ( -15.72974639402197994, 15.80617190586746368, 110.6239096053143669 ) ) ;
#104035=CARTESIAN_POINT ( 'NONE',  ( -16.46253265017146816, -9.564922557961047289, 34.16775706135233293 ) ) ;
#104036=CARTESIAN_POINT ( 'NONE',  ( 5.049401038297881783, 19.05341960407617563, 52.29275706135234003 ) ) ;
#104037=CARTESIAN_POINT ( 'NONE',  ( -12.14591786802326823, 12.06949235617739902, 88.12609039468570415 ) ) ;
#104039=CARTESIAN_POINT ( 'NONE',  ( -5.049401038298153566, 19.05341960407611168, 75.20724293864769550 ) ) ;
#104040=CARTESIAN_POINT ( 'NONE',  ( 5.823673210054444382, -21.52544592524334988, 85.20942372801901854 ) ) ;
#104041=CARTESIAN_POINT ( 'NONE',  ( -10.72451020669870658, -18.67979575497194134, 99.58442372801900433 ) ) ;
#104043=CARTESIAN_POINT ( 'NONE',  ( -19.03943276465977164, 0.05219959533909376836, 91.24890960531436690 ) ) ;
#104044=CARTESIAN_POINT ( 'NONE',  ( -5.719274019375665041, -21.55341960407619695, 64.79275706135234714 ) ) ;
#104045=CARTESIAN_POINT ( 'NONE',  ( -9.474510206698720793, -16.51473224551083518, 94.58442372801900433 ) ) ;
#104046=CARTESIAN_POINT ( 'NONE',  ( -16.51473224551069308, -9.474510206698971260, 71.66557627198102409 ) ) ;
#104047=CARTESIAN_POINT ( 'NONE',  ( -9.564922557960796823, -16.46253265017161027, 112.0822429386476955 ) ) ;
#104048=CARTESIAN_POINT ( 'NONE',  ( 5.049401038298161559, -19.05341960407611168, 77.70724293864765286 ) ) ;
#104049=CARTESIAN_POINT ( 'NONE',  ( 17.49999999999996803, -4.264887584952425037, 23.02877294406987474 ) ) ;
#104050=CARTESIAN_POINT ( 'NONE',  ( -16.46253265017160317, 9.564922557960807481, 70.83224293864770971 ) ) ;
#104051=CARTESIAN_POINT ( 'NONE',  ( -13.97604488694527625, -13.89961937509977652, 51.87390960531436690 ) ) ;
#104052=CARTESIAN_POINT ( 'NONE',  ( -21.53943276465977519, -0.05219959533937600094, 18.75109039468568639 ) ) ;
#104053=CARTESIAN_POINT ( 'NONE',  ( -8.224510206698735004, -14.34966873604973081, 89.58442372801901854 ) ) ;
#104056=CARTESIAN_POINT ( 'NONE',  ( -5.153800228976607833, 19.02544592524334988, 57.70942372801899012 ) ) ;
#104057=CARTESIAN_POINT ( 'NONE',  ( 13.97604488694527802, 13.89961937509977652, 74.37390960531436690 ) ) ;
#104058=CARTESIAN_POINT ( 'NONE',  ( -16.53943276465976808, 0.05219959533911058130, 66.24890960531436690 ) ) ;
#104059=CARTESIAN_POINT ( 'NONE',  ( -8.314922557960811034, -14.29746914071050412, 102.0822429386476955 ) ) ;
#104060=CARTESIAN_POINT ( 'NONE',  ( 19.03943276465977164, -0.05219959533909143690, 108.7489096053143527 ) ) ;
#104061=CARTESIAN_POINT ( 'NONE',  ( 16.46253265017160672, -9.564922557960803928, 108.3322429386476955 ) ) ;
#104062=CARTESIAN_POINT ( 'NONE',  ( -16.53943276465976808, 0.05219959533911058130, 96.24890960531435269 ) ) ;
#104063=CARTESIAN_POINT ( 'NONE',  ( -19.02544592524342804, 5.153800228976336051, 116.0405762719810383 ) ) ;
#104064=CARTESIAN_POINT ( 'NONE',  ( 16.51473224551083163, -9.474510206698727899, 35.83442372801899722 ) ) ;
#104065=CARTESIAN_POINT ( 'NONE',  ( 16.52544592524335698, 4.483927247898782831, 106.4594237280190328 ) ) ;
#104066=CARTESIAN_POINT ( 'NONE',  ( 5.049401038298161559, -19.05341960407611168, 92.70724293864769550 ) ) ;
#104067=CARTESIAN_POINT ( 'NONE',  ( -10.72451020669870658, -18.67979575497194134, 54.58442372801901143 ) ) ;
#104068=CARTESIAN_POINT ( 'NONE',  ( 15.72974639402199770, -15.80617190586745480, 48.12390960531436690 ) ) ;
#104069=CARTESIAN_POINT ( 'NONE',  ( -18.62759615963255300, -10.81492255796106328, 19.16775706135234714 ) ) ;
#104070=CARTESIAN_POINT ( 'NONE',  ( 15.72974639402199770, -15.80617190586745480, 68.12390960531436690 ) ) ;
#104071=CARTESIAN_POINT ( 'NONE',  ( 16.55341960407611168, 4.379528057220329451, 88.95724293864769550 ) ) ;
#104072=CARTESIAN_POINT ( 'NONE',  ( 0.05219959533936267826, -19.03943276465977164, 60.00109039468566863 ) ) ;
#104073=CARTESIAN_POINT ( 'NONE',  ( -9.564922557960796823, -16.46253265017161027, 27.08224293864769550 ) ) ;
#104074=CARTESIAN_POINT ( 'NONE',  ( 0.05219959533909260263, 19.03943276465977164, 84.99890960531436690 ) ) ;
#104075=CARTESIAN_POINT ( 'NONE',  ( 16.46253265017160672, -9.564922557960803928, 83.33224293864768129 ) ) ;
#104076=CARTESIAN_POINT ( 'NONE',  ( 0.05219959533910956823, 16.53943276465976808, 104.9989096053143669 ) ) ;
#104078=CARTESIAN_POINT ( 'NONE',  ( 12.06949235617757843, -12.14591786802309237, 33.12390960531435979 ) ) ;
#104079=CARTESIAN_POINT ( 'NONE',  ( -4.379528057220086978, -16.55341960407618274, 39.79275706135235424 ) ) ;
#104080=CARTESIAN_POINT ( 'NONE',  ( -10.72451020669870658, -18.67979575497194134, 109.5844237280190328 ) ) ;
#104081=CARTESIAN_POINT ( 'NONE',  ( -0.05219959533909027116, -19.03943276465977164, 107.4989096053143527 ) ) ;
#104082=CARTESIAN_POINT ( 'NONE',  ( 15.72974639402176855, 15.80617190586768217, 36.87609039468568994 ) ) ;
#104083=CARTESIAN_POINT ( 'NONE',  ( 5.153800228976335163, 19.02544592524342804, 44.79057627198103830 ) ) ;
#104084=CARTESIAN_POINT ( 'NONE',  ( 0.05219959533934541429, -16.53943276465976808, 45.00109039468568284 ) ) ;
#104085=CARTESIAN_POINT ( 'NONE',  ( -16.53943276465976808, -0.05219959533934237506, 88.75109039468567573 ) ) ;
#104086=CARTESIAN_POINT ( 'NONE',  ( -5.153800228976607833, 19.02544592524334988, 112.7094237280190043 ) ) ;
#104087=CARTESIAN_POINT ( 'NONE',  ( -16.51473224551069308, -9.474510206698971260, 31.66557627198102054 ) ) ;
#104088=CARTESIAN_POINT ( 'NONE',  ( -4.483927247898539470, -16.52544592524342804, 92.29057627198103830 ) ) ;
#104089=CARTESIAN_POINT ( 'NONE',  ( -18.67979575497178146, -10.72451020669898902, 106.6655762719810383 ) ) ;
#104090=CARTESIAN_POINT ( 'NONE',  ( 13.97604488694548053, -13.89961937509957401, 85.62609039468568994 ) ) ;
#104091=CARTESIAN_POINT ( 'NONE',  ( -5.153800228976328057, -19.02544592524343514, 27.29057627198103120 ) ) ;
#104092=CARTESIAN_POINT ( 'NONE',  ( -13.89961937509977652, 13.97604488694528158, 90.62390960531432427 ) ) ;
#104093=CARTESIAN_POINT ( 'NONE',  ( -0.05219959533937732626, 21.53943276465977519, 37.50109039468568284 ) ) ;
#104095=CARTESIAN_POINT ( 'NONE',  ( -9.474510206698964154, 16.51473224551069663, 90.41557627198103830 ) ) ;
#104097=CARTESIAN_POINT ( 'NONE',  ( -5.049401038298153566, 19.05341960407611168, 80.20724293864769550 ) ) ;
#104098=CARTESIAN_POINT ( 'NONE',  ( 21.55341960407619695, -5.719274019375665929, 26.04275706135235779 ) ) ;
#104099=CARTESIAN_POINT ( 'NONE',  ( -0.05219959533910754901, -16.53943276465976808, 87.49890960531436690 ) ) ;
#104100=CARTESIAN_POINT ( 'NONE',  ( -19.05341960407611168, -5.049401038298163336, 91.45724293864766707 ) ) ;
#104101=CARTESIAN_POINT ( 'NONE',  ( -13.89961937509957401, -13.97604488694547875, 19.37609039468566507 ) ) ;
#104102=CARTESIAN_POINT ( 'NONE',  ( -16.53943276465976808, -0.05219959533934237506, 53.75109039468568994 ) ) ;
#104103=CARTESIAN_POINT ( 'NONE',  ( -21.53943276465977519, -0.05219959533937600094, 78.75109039468568994 ) ) ;
#104104=CARTESIAN_POINT ( 'NONE',  ( 8.314922557961029526, -14.29746914071037800, 40.41775706135234714 ) ) ;
#104105=CARTESIAN_POINT ( 'NONE',  ( 16.46253265017160672, -9.564922557960803928, 83.33224293864768129 ) ) ;
#104107=CARTESIAN_POINT ( 'NONE',  ( 9.564922557961047289, -16.46253265017146816, 100.4177570613523329 ) ) ;
#104108=CARTESIAN_POINT ( 'NONE',  ( -4.379528057220086978, -16.55341960407618274, 64.79275706135234714 ) ) ;
#104109=CARTESIAN_POINT ( 'NONE',  ( 21.52544592524334988, 5.823673210054432836, 111.4594237280190328 ) ) ;
#104110=CARTESIAN_POINT ( 'NONE',  ( 5.049401038297881783, 19.05341960407617563, 77.29275706135231871 ) ) ;
#104111=CARTESIAN_POINT ( 'NONE',  ( -13.89961937509977652, 13.97604488694528158, 65.62390960531436690 ) ) ;
#104112=CARTESIAN_POINT ( 'NONE',  ( 10.72451020669898902, -18.67979575497178502, 77.91557627198102409 ) ) ;
#104113=CARTESIAN_POINT ( 'NONE',  ( -0.05219959533910754901, -16.53943276465976808, 77.49890960531433848 ) ) ;
#104114=CARTESIAN_POINT ( 'NONE',  ( 16.51473224551083163, -9.474510206698727899, 95.83442372801900433 ) ) ;
#104116=CARTESIAN_POINT ( 'NONE',  ( 0.05219959533936267826, -19.03943276465977164, 60.00109039468566863 ) ) ;
#104117=CARTESIAN_POINT ( 'NONE',  ( 16.52544592524335698, 4.483927247898782831, 106.4594237280190328 ) ) ;
#104118=CARTESIAN_POINT ( 'NONE',  ( -14.29746914071049879, 8.314922557960819915, 75.83224293864769550 ) ) ;
#104119=CARTESIAN_POINT ( 'NONE',  ( -15.72974639402176322, -15.80617190586768395, 109.3760903946857042 ) ) ;
#104120=CARTESIAN_POINT ( 'NONE',  ( -19.53037848336981597, 5.499999999999898748, 89.85532783611444074 ) ) ;
#104121=CARTESIAN_POINT ( 'NONE',  ( 21.55341960407610458, 5.719274019375980345, 108.9572429386476955 ) ) ;
#104122=CARTESIAN_POINT ( 'NONE',  ( -13.97604488694527625, -13.89961937509977652, 106.8739096053143669 ) ) ;
#104123=CARTESIAN_POINT ( 'NONE',  ( -9.474510206698964154, 16.51473224551069663, 75.41557627198103830 ) ) ;
#104124=CARTESIAN_POINT ( 'NONE',  ( -21.55341960407619339, 5.719274019375674811, 83.54275706135234714 ) ) ;
#104125=CARTESIAN_POINT ( 'NONE',  ( 13.97604488694527802, 13.89961937509977652, 69.37390960531436690 ) ) ;
#104126=CARTESIAN_POINT ( 'NONE',  ( -5.153800228976328057, -19.02544592524343514, 42.29057627198101699 ) ) ;
#104127=CARTESIAN_POINT ( 'NONE',  ( -21.55341960407610458, -5.719274019375992779, 26.45724293864768839 ) ) ;
#104128=CARTESIAN_POINT ( 'NONE',  ( -8.314922557960811034, -14.29746914071050412, 82.08224293864768129 ) ) ;
#104129=CARTESIAN_POINT ( 'NONE',  ( -0.05219959533909027116, -19.03943276465977164, 47.49890960531435979 ) ) ;
#104130=CARTESIAN_POINT ( 'NONE',  ( -4.379528057220328563, 16.55341960407611168, 100.2072429386476955 ) ) ;
#104131=CARTESIAN_POINT ( 'NONE',  ( 18.67979575497178502, 10.72451020669898547, 104.1655762719810241 ) ) ;
#104132=CARTESIAN_POINT ( 'NONE',  ( -15.80617190586768217, 15.72974639402176855, 53.12609039468568284 ) ) ;
#104133=CARTESIAN_POINT ( 'NONE',  ( -16.46253265017160317, 9.564922557960807481, 25.83224293864769194 ) ) ;
#104134=CARTESIAN_POINT ( 'NONE',  ( -14.29746914071037622, -8.314922557961029526, 59.16775706135234714 ) ) ;
#104135=ADVANCED_FACE ( 'NONE', ( #166411 ), #11741, .T. ) ;
#104136=CARTESIAN_POINT ( 'NONE',  ( 5.719274019375991003, -21.55341960407610458, 97.70724293864772392 ) ) ;
#104137=CARTESIAN_POINT ( 'NONE',  ( -0.05219959533907301413, -21.53943276465977519, 97.49890960531436690 ) ) ;
#104138=CARTESIAN_POINT ( 'NONE',  ( 16.46253265017146816, 9.564922557961045513, 36.66775706135233293 ) ) ;
#104139=CARTESIAN_POINT ( 'NONE',  ( 9.564922557960805705, 16.46253265017160317, 54.58224293864769550 ) ) ;
#104141=CARTESIAN_POINT ( 'NONE',  ( 21.53943276465977519, 0.05219959533937863772, 61.25109039468567573 ) ) ;
#104142=CARTESIAN_POINT ( 'NONE',  ( -15.72974639402197994, 15.80617190586746368, 55.62390960531436690 ) ) ;
#104143=CARTESIAN_POINT ( 'NONE',  ( -14.34966873604960291, -8.224510206698953496, 36.66557627198103120 ) ) ;
#104144=CARTESIAN_POINT ( 'NONE',  ( 5.719274019375673035, 21.55341960407619339, 82.29275706135234714 ) ) ;
#104145=CARTESIAN_POINT ( 'NONE',  ( 5.049401038297881783, 19.05341960407617563, 22.29275706135233648 ) ) ;
#104146=CARTESIAN_POINT ( 'NONE',  ( 16.52544592524342804, -4.483927247898539470, 108.5405762719810241 ) ) ;
#104147=CARTESIAN_POINT ( 'NONE',  ( 19.03943276465977164, 0.05219959533936151252, 41.25109039468566152 ) ) ;
#104148=CARTESIAN_POINT ( 'NONE',  ( 16.52544592524335698, 4.483927247898782831, 106.4594237280190328 ) ) ;
#104149=CARTESIAN_POINT ( 'NONE',  ( -18.62759615963255300, -10.81492255796106328, 74.16775706135231871 ) ) ;
#104150=CARTESIAN_POINT ( 'NONE',  ( 13.89961937509977652, -13.97604488694527269, 58.12390960531436690 ) ) ;
#104151=CARTESIAN_POINT ( 'NONE',  ( -9.474510206698720793, -16.51473224551083518, 29.58442372801900433 ) ) ;
#104152=CARTESIAN_POINT ( 'NONE',  ( -21.53943276465977519, 0.05219959533907696930, 41.24890960531435269 ) ) ;
#104153=B_SPLINE_CURVE_WITH_KNOTS ( 'NONE', 3,
 ( #33476, #79973, #141641, #64806, #189162, #173986, #143616, #5100, #11127, #104120, #85948, #102124, #118301, #194151, #161795, #115293, #149629, #180980, #177977, #178983 ),
 .UNSPECIFIED., .F., .F.,
 ( 4, 2, 2, 2, 2, 2, 2, 2, 2, 4 ),
 ( 0.004000878361811981664, 0.004499404418915974209, 0.004997930476019966754, 0.005496456533123960167, 0.005994982590227952712, 0.006244245618779948985, 0.006493508647331945258, 0.006992034704435934334, 0.007490560761539921675, 0.007989086818643910751 ),
 .UNSPECIFIED. ) ;
#104154=CARTESIAN_POINT ( 'NONE',  ( 10.81492255796106328, -18.62759615963255655, 35.41775706135234003 ) ) ;
#104155=CARTESIAN_POINT ( 'NONE',  ( -0.05219959533907301413, -21.53943276465977519, 87.49890960531436690 ) ) ;
#104156=CARTESIAN_POINT ( 'NONE',  ( 13.97604488694548053, -13.89961937509957401, 85.62609039468568994 ) ) ;
#104157=CARTESIAN_POINT ( 'NONE',  ( -16.53943276465976808, -0.05219959533934237506, 48.75109039468568284 ) ) ;
#104159=CARTESIAN_POINT ( 'NONE',  ( 21.55341960407610458, 5.719274019375980345, 88.95724293864769550 ) ) ;
#104160=CARTESIAN_POINT ( 'NONE',  ( 4.483927247898790824, -16.52544592524335698, 85.20942372801901854 ) ) ;
#104161=CARTESIAN_POINT ( 'NONE',  ( 4.379528057220339221, -16.55341960407611168, 82.70724293864770971 ) ) ;
#104163=CARTESIAN_POINT ( 'NONE',  ( -19.02544592524334988, -5.153800228976617603, 108.9594237280189759 ) ) ;
#104164=CARTESIAN_POINT ( 'NONE',  ( -10.81492255796078084, -18.62759615963271287, 32.08224293864769550 ) ) ;
#104166=CARTESIAN_POINT ( 'NONE',  ( 8.314922557961029526, -14.29746914071037800, 50.41775706135235424 ) ) ;
#104167=CARTESIAN_POINT ( 'NONE',  ( -21.53943276465977519, -0.05219959533937600094, 23.75109039468567929 ) ) ;
#104168=CARTESIAN_POINT ( 'NONE',  ( -21.52544592524343514, 5.823673210054127303, 41.04057627198103120 ) ) ;
#104169=CARTESIAN_POINT ( 'NONE',  ( 16.52544592524335698, 4.483927247898782831, 76.45942372801901854 ) ) ;
#104170=CARTESIAN_POINT ( 'NONE',  ( -9.474510206698964154, 16.51473224551069663, 80.41557627198103830 ) ) ;
#104171=CARTESIAN_POINT ( 'NONE',  ( 10.72451020669871369, 18.67979575497193778, 57.08442372801901854 ) ) ;
#104172=CARTESIAN_POINT ( 'NONE',  ( -19.03943276465977164, 0.05219959533909376836, 31.24890960531435979 ) ) ;
#104173=CARTESIAN_POINT ( 'NONE',  ( -21.55341960407610458, -5.719274019375992779, 41.45724293864769550 ) ) ;
#104175=CARTESIAN_POINT ( 'NONE',  ( -19.05341960407617563, 5.049401038297882671, 43.54275706135232582 ) ) ;
#104176=CARTESIAN_POINT ( 'NONE',  ( 14.29746914071037800, 8.314922557961029526, 51.66775706135234714 ) ) ;
#104177=CARTESIAN_POINT ( 'NONE',  ( -9.474510206698964154, 16.51473224551069663, 115.4155762719810241 ) ) ;
#104179=CARTESIAN_POINT ( 'NONE',  ( -13.97604488694527625, -13.89961937509977652, 91.87390960531432427 ) ) ;
#104180=CARTESIAN_POINT ( 'NONE',  ( 16.52544592524335698, 4.483927247898782831, 101.4594237280190185 ) ) ;
#104181=CARTESIAN_POINT ( 'NONE',  ( -19.02544592524342804, 5.153800228976336051, 116.0405762719810383 ) ) ;
#104182=CARTESIAN_POINT ( 'NONE',  ( 8.314922557960818139, 14.29746914071049879, 94.58224293864769550 ) ) ;
#104183=CARTESIAN_POINT ( 'NONE',  ( 15.72974639402199770, -15.80617190586745480, 33.12390960531435979 ) ) ;
#104184=CARTESIAN_POINT ( 'NONE',  ( 16.46253265017160672, -9.564922557960803928, 38.33224293864768839 ) ) ;
#104185=CARTESIAN_POINT ( 'NONE',  ( 12.06949235617739724, 12.14591786802326823, 76.87609039468567573 ) ) ;
#104186=CARTESIAN_POINT ( 'NONE',  ( 5.823673210054444382, -21.52544592524334988, 20.20942372801900788 ) ) ;
#104187=CARTESIAN_POINT ( 'NONE',  ( 19.05341960407617918, -5.049401038297876454, 71.04275706135234714 ) ) ;
#104188=CARTESIAN_POINT ( 'NONE',  ( -19.03943276465977164, 0.05219959533909376836, 41.24890960531435269 ) ) ;
#104189=CARTESIAN_POINT ( 'NONE',  ( -19.05341960407611168, -5.049401038298163336, 111.4572429386476671 ) ) ;
#104190=CARTESIAN_POINT ( 'NONE',  ( 0.05219959533937995610, -21.53943276465977519, 105.0010903946856757 ) ) ;
#104191=CARTESIAN_POINT ( 'NONE',  ( -5.049401038298153566, 19.05341960407611168, 60.20724293864768129 ) ) ;
#104192=EDGE_CURVE ( 'NONE', #56021, #102442, #196322, .T. ) ;
#104193=CARTESIAN_POINT ( 'NONE',  ( 16.55341960407618274, -4.379528057220086978, 51.04275706135234714 ) ) ;
#104194=CARTESIAN_POINT ( 'NONE',  ( -15.80617190586768217, 15.72974639402176855, 93.12609039468568994 ) ) ;
#104195=CARTESIAN_POINT ( 'NONE',  ( -19.03943276465977164, -0.05219959533935918106, 38.75109039468566152 ) ) ;
#104196=CARTESIAN_POINT ( 'NONE',  ( -0.05219959533936034679, 19.03943276465977164, 47.50109039468566863 ) ) ;
#104197=ORIENTED_EDGE ( 'NONE', *, *, #294, .F. ) ;
#104198=CARTESIAN_POINT ( 'NONE',  ( 10.81492255796106328, -18.62759615963255655, 45.41775706135234003 ) ) ;
#104199=CARTESIAN_POINT ( 'NONE',  ( -9.474510206698964154, 16.51473224551069663, 25.41557627198103120 ) ) ;
#104200=CARTESIAN_POINT ( 'NONE',  ( 9.474510206698729675, 16.51473224551082808, 52.08442372801900433 ) ) ;
#104201=CARTESIAN_POINT ( 'NONE',  ( 19.05341960407611168, 5.049401038298154454, 93.95724293864769550 ) ) ;
#104202=CARTESIAN_POINT ( 'NONE',  ( 9.474510206698971260, -16.51473224551069308, 82.91557627198103830 ) ) ;
#104203=CARTESIAN_POINT ( 'NONE',  ( -8.314922557960811034, -14.29746914071050412, 32.08224293864769550 ) ) ;
#104204=CARTESIAN_POINT ( 'NONE',  ( 15.72974639402199770, -15.80617190586745480, 33.12390960531435979 ) ) ;
#104207=CARTESIAN_POINT ( 'NONE',  ( 18.62759615963255655, 10.81492255796105972, 106.6677570613523756 ) ) ;
#104209=CARTESIAN_POINT ( 'NONE',  ( -5.049401038298153566, 19.05341960407611168, 35.20724293864768839 ) ) ;
#104210=CARTESIAN_POINT ( 'NONE',  ( -19.05341960407611168, -5.049401038298163336, 111.4572429386476671 ) ) ;
#104213=CARTESIAN_POINT ( 'NONE',  ( -4.379528057220086978, -16.55341960407618274, 59.79275706135234714 ) ) ;
#104214=CARTESIAN_POINT ( 'NONE',  ( 21.55341960407610458, 5.719274019375980345, 88.95724293864769550 ) ) ;
#104215=CARTESIAN_POINT ( 'NONE',  ( 4.483927247898545687, 16.52544592524342804, 39.79057627198103830 ) ) ;
#104216=CARTESIAN_POINT ( 'NONE',  ( 16.51473224551069308, 9.474510206698969483, 29.16557627198103475 ) ) ;
#104217=CARTESIAN_POINT ( 'NONE',  ( -13.97604488694527625, -13.89961937509977652, 111.8739096053143243 ) ) ;
#104218=CARTESIAN_POINT ( 'NONE',  ( 21.53943276465977519, 0.05219959533937863772, 26.25109039468567573 ) ) ;
#104219=CARTESIAN_POINT ( 'NONE',  ( 0.05219959533936267826, -19.03943276465977164, 30.00109039468566863 ) ) ;
#104220=CARTESIAN_POINT ( 'NONE',  ( -0.05219959533909027116, -19.03943276465977164, 32.49890960531435979 ) ) ;
#104221=CARTESIAN_POINT ( 'NONE',  ( 5.719274019375673035, 21.55341960407619339, 77.29275706135234714 ) ) ;
#104223=CARTESIAN_POINT ( 'NONE',  ( -12.14591786802309592, -12.06949235617757132, 31.87390960531435979 ) ) ;
#104225=CARTESIAN_POINT ( 'NONE',  ( -21.52544592524343514, 5.823673210054127303, 26.04057627198103475 ) ) ;
#104226=CARTESIAN_POINT ( 'NONE',  ( 12.14591786802309770, 12.06949235617756955, 99.37390960531436690 ) ) ;
#104227=LINE ( 'NONE', #151726, #65859 ) ;
#104228=CARTESIAN_POINT ( 'NONE',  ( 16.51473224551069308, 9.474510206698969483, 94.16557627198103830 ) ) ;
#104229=CARTESIAN_POINT ( 'NONE',  ( 0.05219959533910956823, 16.53943276465976808, 74.99890960531435269 ) ) ;
#104230=CARTESIAN_POINT ( 'NONE',  ( 0.05219959533936267826, -19.03943276465977164, 100.0010903946856757 ) ) ;
#104231=CARTESIAN_POINT ( 'NONE',  ( 18.67979575497178502, 10.72451020669898547, 69.16557627198102409 ) ) ;
#104233=CARTESIAN_POINT ( 'NONE',  ( -9.564922557960796823, -16.46253265017161027, 32.08224293864769550 ) ) ;
#104234=CARTESIAN_POINT ( 'NONE',  ( -9.474510206698964154, 16.51473224551069663, 90.41557627198103830 ) ) ;
#104235=CARTESIAN_POINT ( 'NONE',  ( -15.72974639402197994, 15.80617190586746368, 90.62390960531436690 ) ) ;
#104236=CARTESIAN_POINT ( 'NONE',  ( -8.224510206698735004, -14.34966873604973081, 104.5844237280190185 ) ) ;
#104237=CARTESIAN_POINT ( 'NONE',  ( 9.474510206698971260, -16.51473224551069308, 82.91557627198103830 ) ) ;
#104238=CARTESIAN_POINT ( 'NONE',  ( 16.46253265017146816, 9.564922557961045513, 76.66775706135234714 ) ) ;
#104239=CARTESIAN_POINT ( 'NONE',  ( 18.62759615963255655, 10.81492255796105972, 91.66775706135234714 ) ) ;
#104240=CARTESIAN_POINT ( 'NONE',  ( 5.719274019375991003, -21.55341960407610458, 82.70724293864770971 ) ) ;
#104241=CARTESIAN_POINT ( 'NONE',  ( -10.81492255796078084, -18.62759615963271287, 32.08224293864769550 ) ) ;
#104242=CARTESIAN_POINT ( 'NONE',  ( -19.02544592524342804, 5.153800228976336051, 51.04057627198103120 ) ) ;
#104243=CARTESIAN_POINT ( 'NONE',  ( 4.379528057220339221, -16.55341960407611168, 22.70724293864769194 ) ) ;
#104244=CARTESIAN_POINT ( 'NONE',  ( -13.89961937509977652, 13.97604488694528158, 70.62390960531432427 ) ) ;
#104246=CARTESIAN_POINT ( 'NONE',  ( -21.55341960407619339, 5.719274019375674811, 108.5427570613523756 ) ) ;
#104247=CARTESIAN_POINT ( 'NONE',  ( 8.224510206698953496, -14.34966873604960469, 72.91557627198103830 ) ) ;
#104248=CARTESIAN_POINT ( 'NONE',  ( 21.52544592524344225, -5.823673210054117533, 108.5405762719810241 ) ) ;
#104249=CARTESIAN_POINT ( 'NONE',  ( -10.81492255796078084, -18.62759615963271287, 112.0822429386477097 ) ) ;
#104251=CARTESIAN_POINT ( 'NONE',  ( 18.67979575497178502, 10.72451020669898547, 59.16557627198103120 ) ) ;
#104252=CARTESIAN_POINT ( 'NONE',  ( 12.14591786802327356, -12.06949235617739191, 90.62609039468567573 ) ) ;
#104253=CARTESIAN_POINT ( 'NONE',  ( 16.55341960407611168, 4.379528057220329451, 98.95724293864770971 ) ) ;
#104254=CARTESIAN_POINT ( 'NONE',  ( -9.474510206698964154, 16.51473224551069663, 60.41557627198102409 ) ) ;
#104256=CARTESIAN_POINT ( 'NONE',  ( 0.05219959533910956823, 16.53943276465976808, 34.99890960531435979 ) ) ;
#104257=CARTESIAN_POINT ( 'NONE',  ( -10.72451020669870658, -18.67979575497194134, 44.58442372801901854 ) ) ;
#104258=CARTESIAN_POINT ( 'NONE',  ( -16.46253265017160317, 9.564922557960807481, 105.8322429386476955 ) ) ;
#104259=CARTESIAN_POINT ( 'NONE',  ( 10.72451020669871369, 18.67979575497193778, 87.08442372801901854 ) ) ;
#104260=CARTESIAN_POINT ( 'NONE',  ( -13.89961937509977652, 13.97604488694528158, 30.62390960531435269 ) ) ;
#104261=CARTESIAN_POINT ( 'NONE',  ( -0.05219959533909027116, -19.03943276465977164, 37.49890960531436690 ) ) ;
#104262=( BOUNDED_CURVE ( )  B_SPLINE_CURVE ( 2, ( #46749, #171080, #63902, #187270, #16410, #48739, #185256, #124572, #93227, #199436, #152916, #30581, #140731 ),
 .UNSPECIFIED., .F., .T. ) 
 B_SPLINE_CURVE_WITH_KNOTS ( ( 3, 2, 2, 2, 2, 2, 3 ),
 ( 0.3445813794070300973, 0.3464912280701754610, 0.3508771929824561209, 0.3552631578947368363, 0.3596491228070175517, 0.3640350877192982670, 0.3659906162045339362 ),
 .UNSPECIFIED. ) 
 CURVE ( )  GEOMETRIC_REPRESENTATION_ITEM ( )  RATIONAL_B_SPLINE_CURVE ( ( 0.9832469066685285419, 0.9851625545550100060, 1.000000000000000000, 0.9659258262890683122, 1.000000000000000000, 0.9659258262890683122, 1.000000000000000000, 0.9659258262890683122, 1.000000000000000000, 0.9659258262890683122, 1.000000000000000000, 0.9848076720550081875, 0.9831626618144004848 ) ) 
 REPRESENTATION_ITEM ( '' )  );
#104264=CARTESIAN_POINT ( 'NONE',  ( 5.823673210054444382, -21.52544592524334988, 85.20942372801901854 ) ) ;
#104265=CARTESIAN_POINT ( 'NONE',  ( -14.29746914071037622, -8.314922557961029526, 44.16775706135234714 ) ) ;
#104266=CARTESIAN_POINT ( 'NONE',  ( -18.62759615963255300, -10.81492255796106328, 69.16775706135234714 ) ) ;
#104267=CARTESIAN_POINT ( 'NONE',  ( 5.049401038298161559, -19.05341960407611168, 102.7072429386476955 ) ) ;
#104268=CARTESIAN_POINT ( 'NONE',  ( 19.03943276465977164, 0.05219959533936151252, 76.25109039468566152 ) ) ;
#104269=CARTESIAN_POINT ( 'NONE',  ( 21.52544592524334988, 5.823673210054432836, 56.45942372801902565 ) ) ;
#104270=CARTESIAN_POINT ( 'NONE',  ( -12.06949235617739369, -12.14591786802326823, 29.37609039468568284 ) ) ;
#104271=CARTESIAN_POINT ( 'NONE',  ( 19.03943276465977164, 0.05219959533936151252, 76.25109039468566152 ) ) ;
#104272=CARTESIAN_POINT ( 'NONE',  ( -19.03943276465977164, 0.05219959533909376836, 56.24890960531435979 ) ) ;
#104273=CARTESIAN_POINT ( 'NONE',  ( 9.474510206698729675, 16.51473224551082808, 87.08442372801900433 ) ) ;
#104274=CARTESIAN_POINT ( 'NONE',  ( -12.14591786802326823, 12.06949235617739902, 113.1260903946856899 ) ) ;
#104275=CARTESIAN_POINT ( 'NONE',  ( -16.46253265017146816, -9.564922557961047289, 84.16775706135233293 ) ) ;
#104276=CARTESIAN_POINT ( 'NONE',  ( -8.224510206698948167, 14.34966873604960824, 45.41557627198103830 ) ) ;
#104277=CARTESIAN_POINT ( 'NONE',  ( -9.474510206698720793, -16.51473224551083518, 64.58442372801900433 ) ) ;
#104278=CARTESIAN_POINT ( 'NONE',  ( 8.314922557961029526, -14.29746914071037800, 45.41775706135234003 ) ) ;
#104279=CARTESIAN_POINT ( 'NONE',  ( -5.049401038297874678, -19.05341960407617918, 29.79275706135232227 ) ) ;
#104280=CARTESIAN_POINT ( 'NONE',  ( -16.51473224551069308, -9.474510206698971260, 41.66557627198103120 ) ) ;
#104281=CARTESIAN_POINT ( 'NONE',  ( -12.14591786802326823, 12.06949235617739902, 43.12609039468568284 ) ) ;
#104286=CARTESIAN_POINT ( 'NONE',  ( -9.474510206698964154, 16.51473224551069663, 90.41557627198103830 ) ) ;
#104288=CARTESIAN_POINT ( 'NONE',  ( -9.474510206698720793, -16.51473224551083518, 99.58442372801900433 ) ) ;
#104289=CARTESIAN_POINT ( 'NONE',  ( 16.46253265017160672, -9.564922557960803928, 113.3322429386476955 ) ) ;
#104290=CARTESIAN_POINT ( 'NONE',  ( 21.52544592524334988, 5.823673210054432836, 111.4594237280190328 ) ) ;
#104291=CARTESIAN_POINT ( 'NONE',  ( -14.29746914071037622, -8.314922557961029526, 19.16775706135234714 ) ) ;
#104292=CARTESIAN_POINT ( 'NONE',  ( 14.29746914071049879, -8.314922557960816363, 113.3322429386476955 ) ) ;
#104293=CARTESIAN_POINT ( 'NONE',  ( 5.153800228976335163, 19.02544592524342804, 39.79057627198100988 ) ) ;
#104294=CARTESIAN_POINT ( 'NONE',  ( -21.53943276465977519, 0.05219959533907696930, 71.24890960531435269 ) ) ;
#104295=CARTESIAN_POINT ( 'NONE',  ( 13.89961937509977652, -13.97604488694527269, 43.12390960531434558 ) ) ;
#104296=CARTESIAN_POINT ( 'NONE',  ( -0.05219959533936034679, 19.03943276465977164, 47.50109039468566863 ) ) ;
#104297=CARTESIAN_POINT ( 'NONE',  ( -9.474510206698720793, -16.51473224551083518, 64.58442372801900433 ) ) ;
#104298=CARTESIAN_POINT ( 'NONE',  ( -16.52544592524342804, 4.483927247898546575, 51.04057627198103120 ) ) ;
#104299=CARTESIAN_POINT ( 'NONE',  ( -15.72974639402197994, 15.80617190586746368, 30.62390960531436335 ) ) ;
#104300=CARTESIAN_POINT ( 'NONE',  ( -10.81492255796105439, 18.62759615963255655, 87.91775706135234714 ) ) ;
#104301=CARTESIAN_POINT ( 'NONE',  ( -21.52544592524343514, 5.823673210054127303, 86.04057627198102409 ) ) ;
#104302=CARTESIAN_POINT ( 'NONE',  ( -5.719274019375665041, -21.55341960407619695, 59.79275706135234714 ) ) ;
#104303=CARTESIAN_POINT ( 'NONE',  ( -15.72974639402176322, -15.80617190586768395, 59.37609039468568284 ) ) ;
#104304=CARTESIAN_POINT ( 'NONE',  ( 19.02544592524343514, -5.153800228976328945, 98.54057627198100988 ) ) ;
#104305=CARTESIAN_POINT ( 'NONE',  ( -4.483927247898782831, 16.52544592524335698, 87.70942372801901854 ) ) ;
#104306=CARTESIAN_POINT ( 'NONE',  ( 21.53943276465977519, 0.05219959533937863772, 61.25109039468567573 ) ) ;
#104307=CARTESIAN_POINT ( 'NONE',  ( -5.153800228976328057, -19.02544592524343514, 57.29057627198103120 ) ) ;
#104308=CARTESIAN_POINT ( 'NONE',  ( 9.564922557960805705, 16.46253265017160317, 29.58224293864769550 ) ) ;
#104309=CARTESIAN_POINT ( 'NONE',  ( -9.564922557960796823, -16.46253265017161027, 52.08224293864768839 ) ) ;
#104310=CARTESIAN_POINT ( 'NONE',  ( 8.314922557960818139, 14.29746914071049879, 64.58224293864769550 ) ) ;
#104311=CARTESIAN_POINT ( 'NONE',  ( 16.55341960407611168, 4.379528057220329451, 38.95724293864768839 ) ) ;
#104312=CARTESIAN_POINT ( 'NONE',  ( -21.55341960407610458, -5.719274019375992779, 46.45724293864769550 ) ) ;
#104313=CARTESIAN_POINT ( 'NONE',  ( -16.46253265017160317, 9.564922557960807481, 50.83224293864770260 ) ) ;
#104314=CARTESIAN_POINT ( 'NONE',  ( -0.05219959533907301413, -21.53943276465977519, 57.49890960531435979 ) ) ;
#104315=CARTESIAN_POINT ( 'NONE',  ( -9.564922557961040184, 16.46253265017147172, 57.91775706135233293 ) ) ;
#104316=CARTESIAN_POINT ( 'NONE',  ( -17.13100169013299379, -6.664070546373170423, 39.23210164300152059 ) ) ;
#104317=CARTESIAN_POINT ( 'NONE',  ( 4.483927247898545687, 16.52544592524342804, 69.79057627198102409 ) ) ;
#104318=CARTESIAN_POINT ( 'NONE',  ( -5.823673210054116645, -21.52544592524344225, 37.29057627198102409 ) ) ;
#104319=ORIENTED_EDGE ( 'NONE', *, *, #143971, .F. ) ;
#104321=CARTESIAN_POINT ( 'NONE',  ( 17.40861289039003523, 6.110651285853316850, 103.8723247082743200 ) ) ;
#104322=CARTESIAN_POINT ( 'NONE',  ( 14.29746914071037800, 8.314922557961029526, 81.66775706135236135 ) ) ;
#104323=CARTESIAN_POINT ( 'NONE',  ( -19.03943276465977164, -0.05219959533935918106, 78.75109039468567573 ) ) ;
#104324=CARTESIAN_POINT ( 'NONE',  ( 12.14591786802309770, 12.06949235617756955, 49.37390960531436690 ) ) ;
#104326=CARTESIAN_POINT ( 'NONE',  ( -13.97604488694527625, -13.89961937509977652, 51.87390960531436690 ) ) ;
#104327=CARTESIAN_POINT ( 'NONE',  ( 16.52544592524342804, -4.483927247898539470, 43.54057627198103830 ) ) ;
#104328=CARTESIAN_POINT ( 'NONE',  ( 0.05219959533909260263, 19.03943276465977164, 49.99890960531435979 ) ) ;
#104329=CARTESIAN_POINT ( 'NONE',  ( 16.51473224551069308, 9.474510206698969483, 69.16557627198102409 ) ) ;
#104330=CARTESIAN_POINT ( 'NONE',  ( -19.03943276465977164, 0.05219959533909376836, 36.24890960531436690 ) ) ;
#104331=CARTESIAN_POINT ( 'NONE',  ( 10.81492255796106328, -18.62759615963255655, 40.41775706135234714 ) ) ;
#104332=CARTESIAN_POINT ( 'NONE',  ( 19.05341960407611168, 5.049401038298154454, 73.95724293864768129 ) ) ;
#104333=CARTESIAN_POINT ( 'NONE',  ( -16.46253265017160317, 9.564922557960807481, 30.83224293864769550 ) ) ;
#104334=CARTESIAN_POINT ( 'NONE',  ( -16.51473224551069308, -9.474510206698971260, 61.66557627198103120 ) ) ;
#104335=CARTESIAN_POINT ( 'NONE',  ( 21.53943276465977519, -0.05219959533907433946, 53.74890960531437401 ) ) ;
#104336=CARTESIAN_POINT ( 'NONE',  ( 5.153800228976335163, 19.02544592524342804, 34.79057627198102409 ) ) ;
#104337=CARTESIAN_POINT ( 'NONE',  ( -15.72974639402197994, 15.80617190586746368, 40.62390960531435269 ) ) ;
#104338=CARTESIAN_POINT ( 'NONE',  ( -12.14591786802326823, 12.06949235617739902, 98.12609039468570415 ) ) ;
#104339=CARTESIAN_POINT ( 'NONE',  ( -5.049401038297874678, -19.05341960407617918, 19.79275706135233293 ) ) ;
#104340=CARTESIAN_POINT ( 'NONE',  ( -8.314922557961024197, 14.29746914071037800, 42.91775706135235424 ) ) ;
#104341=CARTESIAN_POINT ( 'NONE',  ( -4.483927247898782831, 16.52544592524335698, 82.70942372801900433 ) ) ;
#104343=CARTESIAN_POINT ( 'NONE',  ( 4.483927247898790824, -16.52544592524335698, 70.20942372801904696 ) ) ;
#104344=CARTESIAN_POINT ( 'NONE',  ( 14.29746914071037800, 8.314922557961029526, 36.66775706135234714 ) ) ;
#104345=CARTESIAN_POINT ( 'NONE',  ( -9.564922557960796823, -16.46253265017161027, 102.0822429386477097 ) ) ;
#104346=CARTESIAN_POINT ( 'NONE',  ( -14.29746914071037622, -8.314922557961029526, 39.16775706135235424 ) ) ;
#104347=CARTESIAN_POINT ( 'NONE',  ( 0.05219959533909260263, 19.03943276465977164, 29.99890960531435979 ) ) ;
#104348=CARTESIAN_POINT ( 'NONE',  ( 21.55341960407619695, -5.719274019375665929, 31.04275706135234714 ) ) ;
#104349=CARTESIAN_POINT ( 'NONE',  ( -4.483927247898782831, 16.52544592524335698, 37.70942372801900433 ) ) ;
#104350=CARTESIAN_POINT ( 'NONE',  ( 4.483927247898790824, -16.52544592524335698, 105.2094237280190328 ) ) ;
#104352=CARTESIAN_POINT ( 'NONE',  ( 18.67979575497194134, -10.72451020669871369, 100.8344237280190185 ) ) ;
#104353=CARTESIAN_POINT ( 'NONE',  ( 19.02544592524334988, 5.153800228976608722, 96.45942372801897591 ) ) ;
#104354=CARTESIAN_POINT ( 'NONE',  ( 12.06949235617757843, -12.14591786802309237, 58.12390960531435979 ) ) ;
#104355=CARTESIAN_POINT ( 'NONE',  ( 19.05341960407611168, 5.049401038298154454, 28.95724293864769550 ) ) ;
#104356=CARTESIAN_POINT ( 'NONE',  ( 5.049401038297881783, 19.05341960407617563, 57.29275706135231871 ) ) ;
#104357=CARTESIAN_POINT ( 'NONE',  ( 17.50000000000000355, 5.500000000000011546, 78.78230962303567253 ) ) ;
#104358=CARTESIAN_POINT ( 'NONE',  ( 10.72451020669871369, 18.67979575497193778, 62.08442372801901143 ) ) ;
#104359=CARTESIAN_POINT ( 'NONE',  ( -4.483927247898782831, 16.52544592524335698, 27.70942372801901854 ) ) ;
#104360=CARTESIAN_POINT ( 'NONE',  ( 17.49999999999999645, 5.622605283950889543, 83.81207310596114723 ) ) ;
#104361=CARTESIAN_POINT ( 'NONE',  ( 16.46253265017160672, -9.564922557960803928, 113.3322429386476955 ) ) ;
#104362=CARTESIAN_POINT ( 'NONE',  ( 18.62759615963271287, -10.81492255796078972, 78.33224293864770971 ) ) ;
#104363=CARTESIAN_POINT ( 'NONE',  ( 9.564922557961047289, -16.46253265017146816, 110.4177570613523471 ) ) ;
#104364=CARTESIAN_POINT ( 'NONE',  ( 9.474510206698971260, -16.51473224551069308, 97.91557627198102409 ) ) ;
#104366=CARTESIAN_POINT ( 'NONE',  ( 8.314922557960818139, 14.29746914071049879, 114.5822429386477097 ) ) ;
#104367=CARTESIAN_POINT ( 'NONE',  ( 21.53943276465977519, 0.05219959533937863772, 111.2510903946856899 ) ) ;
#104368=CARTESIAN_POINT ( 'NONE',  ( 9.564922557960805705, 16.46253265017160317, 49.58224293864770260 ) ) ;
#104369=CARTESIAN_POINT ( 'NONE',  ( 5.823673210054444382, -21.52544592524334988, 50.20942372801901854 ) ) ;
#104370=CARTESIAN_POINT ( 'NONE',  ( 18.67979575497194134, -10.72451020669871369, 95.83442372801903275 ) ) ;
#104371=CARTESIAN_POINT ( 'NONE',  ( -12.14591786802326823, 12.06949235617739902, 108.1260903946856757 ) ) ;
#104373=CARTESIAN_POINT ( 'NONE',  ( -16.46253265017160317, 9.564922557960807481, 75.83224293864769550 ) ) ;
#104374=CARTESIAN_POINT ( 'NONE',  ( -5.823673210054431948, 21.52544592524334988, 42.70942372801901854 ) ) ;
#104375=CARTESIAN_POINT ( 'NONE',  ( -5.719274019375665041, -21.55341960407619695, 54.79275706135235424 ) ) ;
#104376=CARTESIAN_POINT ( 'NONE',  ( -16.51473224551082808, 9.474510206698731452, 83.33442372801899012 ) ) ;
#104377=CARTESIAN_POINT ( 'NONE',  ( -13.97604488694527625, -13.89961937509977652, 86.87390960531436690 ) ) ;
#104378=CARTESIAN_POINT ( 'NONE',  ( 12.06949235617757843, -12.14591786802309237, 98.12390960531436690 ) ) ;
#104379=CARTESIAN_POINT ( 'NONE',  ( 10.72451020669898902, -18.67979575497178502, 97.91557627198103830 ) ) ;
#104380=CARTESIAN_POINT ( 'NONE',  ( -12.06949235617756955, 12.14591786802309770, 75.62390960531439532 ) ) ;
#104381=CARTESIAN_POINT ( 'NONE',  ( 15.80617190586769283, -15.72974639402175789, 110.6260903946857042 ) ) ;
#104382=CARTESIAN_POINT ( 'NONE',  ( -8.224510206698948167, 14.34966873604960824, 95.41557627198102409 ) ) ;
#104383=CARTESIAN_POINT ( 'NONE',  ( -13.89961937509977652, 13.97604488694528158, 55.62390960531434558 ) ) ;
#104384=CARTESIAN_POINT ( 'NONE',  ( -16.46253265017146816, -9.564922557961047289, 79.16775706135234714 ) ) ;
#104385=CARTESIAN_POINT ( 'NONE',  ( 12.06949235617757843, -12.14591786802309237, 53.12390960531436690 ) ) ;
#104386=CARTESIAN_POINT ( 'NONE',  ( 10.72451020669871369, 18.67979575497193778, 112.0844237280190185 ) ) ;
#104387=CARTESIAN_POINT ( 'NONE',  ( 9.564922557960805705, 16.46253265017160317, 109.5822429386476955 ) ) ;
#104388=CARTESIAN_POINT ( 'NONE',  ( -9.474510206698720793, -16.51473224551083518, 79.58442372801899012 ) ) ;
#104389=CARTESIAN_POINT ( 'NONE',  ( 21.55341960407610458, 5.719274019375980345, 78.95724293864769550 ) ) ;
#104390=CARTESIAN_POINT ( 'NONE',  ( -10.72451020669870658, -18.67979575497194134, 29.58442372801901854 ) ) ;
#104391=CARTESIAN_POINT ( 'NONE',  ( -16.52544592524335698, -4.483927247898792601, 28.95942372801902209 ) ) ;
#104392=CARTESIAN_POINT ( 'NONE',  ( 8.224510206698742110, 14.34966873604972548, 97.08442372801904696 ) ) ;
#104393=CARTESIAN_POINT ( 'NONE',  ( 17.31728774477272736, 6.344390552232406222, 61.68093348310681279 ) ) ;
#104394=CARTESIAN_POINT ( 'NONE',  ( -15.72974639402176322, -15.80617190586768395, 34.37609039468568284 ) ) ;
#104395=CARTESIAN_POINT ( 'NONE',  ( 5.719274019375991003, -21.55341960407610458, 47.70724293864770260 ) ) ;
#104396=CARTESIAN_POINT ( 'NONE',  ( 4.483927247898545687, 16.52544592524342804, 114.7905762719810383 ) ) ;
#104398=CARTESIAN_POINT ( 'NONE',  ( 12.14591786802327356, -12.06949235617739191, 65.62609039468568994 ) ) ;
#104399=CARTESIAN_POINT ( 'NONE',  ( 14.29746914071049879, -8.314922557960816363, 93.33224293864769550 ) ) ;
#104400=CARTESIAN_POINT ( 'NONE',  ( -15.72974639402197994, 15.80617190586746368, 75.62390960531439532 ) ) ;
#104401=CARTESIAN_POINT ( 'NONE',  ( 16.55341960407611168, 4.379528057220329451, 28.95724293864769905 ) ) ;
#104402=CARTESIAN_POINT ( 'NONE',  ( 12.06949235617739724, 12.14591786802326823, 51.87609039468568284 ) ) ;
#104403=CARTESIAN_POINT ( 'NONE',  ( -5.153800228976328057, -19.02544592524343514, 42.29057627198101699 ) ) ;
#104404=CARTESIAN_POINT ( 'NONE',  ( 8.224510206698742110, 14.34966873604972548, 97.08442372801904696 ) ) ;
#104405=CARTESIAN_POINT ( 'NONE',  ( -16.51473224551082808, 9.474510206698731452, 83.33442372801899012 ) ) ;
#104406=CARTESIAN_POINT ( 'NONE',  ( -5.823673210054116645, -21.52544592524344225, 82.29057627198103830 ) ) ;
#104407=CARTESIAN_POINT ( 'NONE',  ( -8.224510206698735004, -14.34966873604973081, 104.5844237280190185 ) ) ;
#104409=CARTESIAN_POINT ( 'NONE',  ( 19.02544592524343514, -5.153800228976328945, 113.5405762719810241 ) ) ;
#104410=CARTESIAN_POINT ( 'NONE',  ( -5.719274019375978568, 21.55341960407610458, 60.20724293864768839 ) ) ;
#104412=CARTESIAN_POINT ( 'NONE',  ( 8.224510206698742110, 14.34966873604972548, 97.08442372801904696 ) ) ;
#104414=CARTESIAN_POINT ( 'NONE',  ( 0.05219959533907565091, 21.53943276465977519, 34.99890960531435979 ) ) ;
#104415=CARTESIAN_POINT ( 'NONE',  ( -19.46398650005391673, 5.499999999999954703, 75.18269651486372140 ) ) ;
#104416=CARTESIAN_POINT ( 'NONE',  ( -10.72451020669898014, 18.67979575497178502, 80.41557627198103830 ) ) ;
#104417=CARTESIAN_POINT ( 'NONE',  ( 12.06949235617757843, -12.14591786802309237, 28.12390960531435979 ) ) ;
#104418=CARTESIAN_POINT ( 'NONE',  ( 14.34966873604972726, -8.224510206698740333, 25.83442372801901499 ) ) ;
#104419=CARTESIAN_POINT ( 'NONE',  ( -13.97604488694527625, -13.89961937509977652, 31.87390960531435979 ) ) ;
#104420=CARTESIAN_POINT ( 'NONE',  ( -14.29746914071037622, -8.314922557961029526, 34.16775706135234714 ) ) ;
#104421=CARTESIAN_POINT ( 'NONE',  ( 13.89961937509977652, -13.97604488694527269, 53.12390960531434558 ) ) ;
#104423=CARTESIAN_POINT ( 'NONE',  ( 16.51473224551069308, 9.474510206698969483, 104.1655762719810241 ) ) ;
#104424=CARTESIAN_POINT ( 'NONE',  ( -5.049401038298153566, 19.05341960407611168, 105.2072429386476671 ) ) ;
#104425=CARTESIAN_POINT ( 'NONE',  ( 0.05219959533934541429, -16.53943276465976808, 90.00109039468567573 ) ) ;
#104426=CARTESIAN_POINT ( 'NONE',  ( 19.05341960407617918, -5.049401038297876454, 91.04275706135234714 ) ) ;
#104427=CARTESIAN_POINT ( 'NONE',  ( -9.564922557961040184, 16.46253265017147172, 32.91775706135233293 ) ) ;
#104428=CARTESIAN_POINT ( 'NONE',  ( -18.62759615963270932, 10.81492255796079327, 70.83224293864770971 ) ) ;
#104429=CARTESIAN_POINT ( 'NONE',  ( 16.53943276465976808, 0.05219959533934440121, 96.25109039468568994 ) ) ;
#104430=CARTESIAN_POINT ( 'NONE',  ( -5.719274019375978568, 21.55341960407610458, 35.20724293864768839 ) ) ;
#104431=CARTESIAN_POINT ( 'NONE',  ( 13.97604488694548053, -13.89961937509957401, 90.62609039468567573 ) ) ;
#104432=CARTESIAN_POINT ( 'NONE',  ( -9.564922557960796823, -16.46253265017161027, 47.08224293864769550 ) ) ;
#104433=CARTESIAN_POINT ( 'NONE',  ( 5.153800228976335163, 19.02544592524342804, 89.79057627198102409 ) ) ;
#104434=CARTESIAN_POINT ( 'NONE',  ( 21.53943276465977519, 0.05219959533937863772, 56.25109039468568284 ) ) ;
#104435=CARTESIAN_POINT ( 'NONE',  ( 5.049401038298161559, -19.05341960407611168, 57.70724293864769550 ) ) ;
#104436=CARTESIAN_POINT ( 'NONE',  ( 4.483927247898545687, 16.52544592524342804, 104.7905762719810241 ) ) ;
#104438=CARTESIAN_POINT ( 'NONE',  ( -16.52544592524342804, 4.483927247898546575, 81.04057627198102409 ) ) ;
#104439=CARTESIAN_POINT ( 'NONE',  ( 10.72451020669898902, -18.67979575497178502, 67.91557627198102409 ) ) ;
#104440=CARTESIAN_POINT ( 'NONE',  ( -5.049401038297874678, -19.05341960407617918, 84.79275706135233293 ) ) ;
#104441=CARTESIAN_POINT ( 'NONE',  ( 18.39639308325437739, 5.500000000000010658, 93.98252246182197212 ) ) ;
#104442=CARTESIAN_POINT ( 'NONE',  ( -19.02544592524342804, 5.153800228976336051, 56.04057627198100988 ) ) ;
#104444=CARTESIAN_POINT ( 'NONE',  ( 19.05341960407611168, 5.049401038298154454, 83.95724293864766707 ) ) ;
#104445=CARTESIAN_POINT ( 'NONE',  ( 9.564922557960805705, 16.46253265017160317, 89.58224293864769550 ) ) ;
#104447=CARTESIAN_POINT ( 'NONE',  ( -14.34966873604972548, 8.224510206698743886, 63.33442372801900433 ) ) ;
#104448=CARTESIAN_POINT ( 'NONE',  ( -16.20579543436680225, -7.371946100354968223, 50.56520834171872991 ) ) ;
#104449=CARTESIAN_POINT ( 'NONE',  ( -0.05219959533936034679, 19.03943276465977164, 42.50109039468566152 ) ) ;
#104451=CARTESIAN_POINT ( 'NONE',  ( -19.05341960407611168, -5.049401038298163336, 111.4572429386476671 ) ) ;
#104452=CARTESIAN_POINT ( 'NONE',  ( -16.53943276465976808, -0.05219959533934237506, 103.7510903946857042 ) ) ;
#104454=CARTESIAN_POINT ( 'NONE',  ( 16.53943276465976808, 0.05219959533934440121, 76.25109039468568994 ) ) ;
#104455=CARTESIAN_POINT ( 'NONE',  ( -17.40861289039003523, 6.110651285853254677, 28.62767529172569070 ) ) ;
#104456=CARTESIAN_POINT ( 'NONE',  ( 8.314922557961029526, -14.29746914071037800, 55.41775706135234714 ) ) ;
#104458=CARTESIAN_POINT ( 'NONE',  ( -15.80617190586768217, 15.72974639402176855, 63.12609039468568994 ) ) ;
#104459=CARTESIAN_POINT ( 'NONE',  ( 0.05219959533936267826, -19.03943276465977164, 75.00109039468566152 ) ) ;
#104460=CARTESIAN_POINT ( 'NONE',  ( 19.02544592524334988, 5.153800228976608722, 31.45942372801900433 ) ) ;
#104461=CARTESIAN_POINT ( 'NONE',  ( -16.46253265017160317, 9.564922557960807481, 60.83224293864769550 ) ) ;
#104462=CARTESIAN_POINT ( 'NONE',  ( -19.05341960407611168, -5.049401038298163336, 46.45724293864768129 ) ) ;
#104463=CARTESIAN_POINT ( 'NONE',  ( 16.24969088024964492, -7.354500926750625389, 22.52456153141350370 ) ) ;
#104464=CARTESIAN_POINT ( 'NONE',  ( 10.72451020669898902, -18.67979575497178502, 72.91557627198103830 ) ) ;
#104465=CARTESIAN_POINT ( 'NONE',  ( -10.72451020669898014, 18.67979575497178502, 40.41557627198103120 ) ) ;
#104466=CARTESIAN_POINT ( 'NONE',  ( 14.34966873604960469, 8.224510206698951720, 109.1655762719810383 ) ) ;
#104467=CARTESIAN_POINT ( 'NONE',  ( 16.52544592524335698, 4.483927247898782831, 56.45942372801902565 ) ) ;
#104468=EDGE_LOOP ( 'NONE', ( #153357, #40656 ) ) ;
#104469=CARTESIAN_POINT ( 'NONE',  ( -5.719274019375665041, -21.55341960407619695, 29.79275706135234358 ) ) ;
#104470=CARTESIAN_POINT ( 'NONE',  ( -4.379528057220328563, 16.55341960407611168, 55.20724293864770260 ) ) ;
#104472=CARTESIAN_POINT ( 'NONE',  ( 8.224510206698742110, 14.34966873604972548, 27.08442372801901854 ) ) ;
#104473=CARTESIAN_POINT ( 'NONE',  ( -13.89961937509957401, -13.97604488694547875, 34.37609039468566863 ) ) ;
#104474=CARTESIAN_POINT ( 'NONE',  ( -16.55341960407611168, -4.379528057220339221, 46.45724293864769550 ) ) ;
#104475=CARTESIAN_POINT ( 'NONE',  ( 5.719274019375991003, -21.55341960407610458, 112.7072429386476955 ) ) ;
#104476=ADVANCED_FACE ( 'NONE', ( #10487 ), #63271, .T. ) ;
#104478=CARTESIAN_POINT ( 'NONE',  ( 5.719274019375991003, -21.55341960407610458, 82.70724293864770971 ) ) ;
#104479=CARTESIAN_POINT ( 'NONE',  ( -0.05219959533909027116, -19.03943276465977164, 92.49890960531436690 ) ) ;
#104480=CARTESIAN_POINT ( 'NONE',  ( 14.29746914071049879, -8.314922557960816363, 63.33224293864770260 ) ) ;
#104481=CARTESIAN_POINT ( 'NONE',  ( 19.03943276465977164, -0.05219959533909143690, 108.7489096053143527 ) ) ;
#104483=CARTESIAN_POINT ( 'NONE',  ( 0.05219959533936267826, -19.03943276465977164, 65.00109039468567573 ) ) ;
#104484=CARTESIAN_POINT ( 'NONE',  ( -18.62759615963270932, 10.81492255796079327, 105.8322429386476955 ) ) ;
#104485=CARTESIAN_POINT ( 'NONE',  ( 16.51473224551069308, 9.474510206698969483, 59.16557627198102409 ) ) ;
#104486=CARTESIAN_POINT ( 'NONE',  ( 9.474510206698971260, -16.51473224551069308, 22.91557627198102765 ) ) ;
#104488=CARTESIAN_POINT ( 'NONE',  ( -15.72974639402176322, -15.80617190586768395, 54.37609039468568994 ) ) ;
#104491=CARTESIAN_POINT ( 'NONE',  ( -14.34966873604960291, -8.224510206698953496, 46.66557627198102409 ) ) ;
#104492=CARTESIAN_POINT ( 'NONE',  ( 13.89961937509977652, -13.97604488694527269, 48.12390960531435979 ) ) ;
#104493=CARTESIAN_POINT ( 'NONE',  ( -16.51473224551069308, -9.474510206698971260, 101.6655762719810241 ) ) ;
#104494=CARTESIAN_POINT ( 'NONE',  ( -5.823673210054116645, -21.52544592524344225, 77.29057627198102409 ) ) ;
#104496=CARTESIAN_POINT ( 'NONE',  ( 19.03943276465977164, -0.05219959533909143690, 38.74890960531436690 ) ) ;
#104497=ORIENTED_EDGE ( 'NONE', *, *, #175152, .T. ) ;
#104498=CARTESIAN_POINT ( 'NONE',  ( -5.823673210054116645, -21.52544592524344225, 62.29057627198102409 ) ) ;
#104499=CARTESIAN_POINT ( 'NONE',  ( 15.80617190586769283, -15.72974639402175789, 80.62609039468567573 ) ) ;
#104501=CARTESIAN_POINT ( 'NONE',  ( 12.06949235617739724, 12.14591786802326823, 86.87609039468568994 ) ) ;
#104502=CARTESIAN_POINT ( 'NONE',  ( -14.34966873604960291, -8.224510206698953496, 81.66557627198103830 ) ) ;
#104503=CARTESIAN_POINT ( 'NONE',  ( 9.474510206698971260, -16.51473224551069308, 67.91557627198102409 ) ) ;
#104505=CARTESIAN_POINT ( 'NONE',  ( 19.03943276465977164, 0.05219959533936151252, 36.25109039468567573 ) ) ;
#104506=CARTESIAN_POINT ( 'NONE',  ( -14.29746914071037622, -8.314922557961029526, 94.16775706135237556 ) ) ;
#104507=CARTESIAN_POINT ( 'NONE',  ( -0.05219959533937732626, 21.53943276465977519, 112.5010903946857042 ) ) ;
#104508=CARTESIAN_POINT ( 'NONE',  ( 19.05341960407611168, 5.049401038298154454, 93.95724293864769550 ) ) ;
#104509=CARTESIAN_POINT ( 'NONE',  ( 10.72451020669898902, -18.67979575497178502, 42.91557627198103120 ) ) ;
#104510=CARTESIAN_POINT ( 'NONE',  ( 15.72974639402176855, 15.80617190586768217, 91.87609039468568994 ) ) ;
#104511=CARTESIAN_POINT ( 'NONE',  ( -0.05219959533934338120, 16.53943276465976808, 57.50109039468568994 ) ) ;
#104512=CARTESIAN_POINT ( 'NONE',  ( 5.719274019375991003, -21.55341960407610458, 112.7072429386476955 ) ) ;
#104513=CARTESIAN_POINT ( 'NONE',  ( 16.55341960407618274, -4.379528057220086978, 36.04275706135234714 ) ) ;
#104514=CARTESIAN_POINT ( 'NONE',  ( -9.564922557960796823, -16.46253265017161027, 87.08224293864769550 ) ) ;
#104515=CARTESIAN_POINT ( 'NONE',  ( 8.314922557961029526, -14.29746914071037800, 25.41775706135235779 ) ) ;
#104516=CARTESIAN_POINT ( 'NONE',  ( -13.97604488694527625, -13.89961937509977652, 51.87390960531436690 ) ) ;
#104517=CARTESIAN_POINT ( 'NONE',  ( 8.314922557961029526, -14.29746914071037800, 35.41775706135234003 ) ) ;
#104518=CARTESIAN_POINT ( 'NONE',  ( 14.34966873604960469, 8.224510206698951720, 79.16557627198103830 ) ) ;
#104519=CARTESIAN_POINT ( 'NONE',  ( 8.224510206698742110, 14.34966873604972548, 87.08442372801901854 ) ) ;
#104520=CARTESIAN_POINT ( 'NONE',  ( -21.52544592524334988, -5.823673210054445271, 38.95942372801901854 ) ) ;
#104521=CARTESIAN_POINT ( 'NONE',  ( -19.03943276465977164, 0.05219959533909376836, 71.24890960531435269 ) ) ;
#104522=CARTESIAN_POINT ( 'NONE',  ( -13.97604488694527625, -13.89961937509977652, 81.87390960531436690 ) ) ;
#104523=CARTESIAN_POINT ( 'NONE',  ( 8.314922557960818139, 14.29746914071049879, 29.58224293864769905 ) ) ;
#104524=CARTESIAN_POINT ( 'NONE',  ( 16.52544592524335698, 4.483927247898782831, 91.45942372801901854 ) ) ;
#104527=CARTESIAN_POINT ( 'NONE',  ( -5.049401038297874678, -19.05341960407617918, 24.79275706135233648 ) ) ;
#104528=CARTESIAN_POINT ( 'NONE',  ( 13.97604488694527802, 13.89961937509977652, 94.37390960531436690 ) ) ;
#104529=CARTESIAN_POINT ( 'NONE',  ( -19.02544592524342804, 5.153800228976336051, 56.04057627198100988 ) ) ;
#104530=CARTESIAN_POINT ( 'NONE',  ( 16.46253265017160672, -9.564922557960803928, 113.3322429386476955 ) ) ;
#104531=CARTESIAN_POINT ( 'NONE',  ( 4.483927247898790824, -16.52544592524335698, 45.20942372801901854 ) ) ;
#104532=CARTESIAN_POINT ( 'NONE',  ( 5.153800228976615827, -19.02544592524334988, 70.20942372801899012 ) ) ;
#104533=CARTESIAN_POINT ( 'NONE',  ( 14.34966873604972726, -8.224510206698740333, 55.83442372801901854 ) ) ;
#104534=CARTESIAN_POINT ( 'NONE',  ( 15.50000000000000178, 5.499999999999998224, 22.00000000000000000 ) ) ;
#104535=CARTESIAN_POINT ( 'NONE',  ( 16.51473224551069308, 9.474510206698969483, 79.16557627198103830 ) ) ;
#104536=CARTESIAN_POINT ( 'NONE',  ( 18.62759615963255655, 10.81492255796105972, 21.66775706135235069 ) ) ;
#104537=CARTESIAN_POINT ( 'NONE',  ( 0.05219959533936267826, -19.03943276465977164, 65.00109039468567573 ) ) ;
#104538=CARTESIAN_POINT ( 'NONE',  ( -16.51473224551069308, -9.474510206698971260, 101.6655762719810241 ) ) ;
#104539=CARTESIAN_POINT ( 'NONE',  ( 30.00000000000000000, -1.163414459189985801E-14, 95.00000000000000000 ) ) ;
#104540=CARTESIAN_POINT ( 'NONE',  ( -16.46253265017160317, 9.564922557960807481, 70.83224293864770971 ) ) ;
#104541=CARTESIAN_POINT ( 'NONE',  ( 8.314922557960818139, 14.29746914071049879, 34.58224293864770260 ) ) ;
#104542=CARTESIAN_POINT ( 'NONE',  ( 0.05219959533909260263, 19.03943276465977164, 29.99890960531435979 ) ) ;
#104543=CARTESIAN_POINT ( 'NONE',  ( 13.89961937509957401, 13.97604488694547697, 31.87609039468566863 ) ) ;
#104544=CARTESIAN_POINT ( 'NONE',  ( -4.379528057220328563, 16.55341960407611168, 75.20724293864769550 ) ) ;
#104545=CARTESIAN_POINT ( 'NONE',  ( -0.05219959533937732626, 21.53943276465977519, 107.5010903946856899 ) ) ;
#104546=CARTESIAN_POINT ( 'NONE',  ( 19.02544592524343514, -5.153800228976328945, 58.54057627198102409 ) ) ;
#104547=CARTESIAN_POINT ( 'NONE',  ( -16.53943276465976808, 0.05219959533911058130, 36.24890960531435979 ) ) ;
#104548=CARTESIAN_POINT ( 'NONE',  ( 21.55341960407619695, -5.719274019375665929, 106.0427570613523471 ) ) ;
#104549=CARTESIAN_POINT ( 'NONE',  ( 13.89961937509977652, -13.97604488694527269, 88.12390960531438111 ) ) ;
#104550=CARTESIAN_POINT ( 'NONE',  ( -16.51473224551069308, -9.474510206698971260, 106.6655762719810383 ) ) ;
#104551=CARTESIAN_POINT ( 'NONE',  ( -13.89961937509977652, 13.97604488694528158, 45.62390960531433848 ) ) ;
#104552=CARTESIAN_POINT ( 'NONE',  ( 4.379528057220339221, -16.55341960407611168, 112.7072429386476955 ) ) ;
#104553=CARTESIAN_POINT ( 'NONE',  ( 8.224510206698953496, -14.34966873604960469, 72.91557627198103830 ) ) ;
#104554=CARTESIAN_POINT ( 'NONE',  ( -5.719274019375978568, 21.55341960407610458, 90.20724293864770971 ) ) ;
#104555=CARTESIAN_POINT ( 'NONE',  ( 5.049401038298161559, -19.05341960407611168, 92.70724293864769550 ) ) ;
#104556=CARTESIAN_POINT ( 'NONE',  ( 10.81492255796078972, 18.62759615963270932, 99.58224293864770971 ) ) ;
#104557=CARTESIAN_POINT ( 'NONE',  ( 13.89961937509977652, -13.97604488694527269, 88.12390960531438111 ) ) ;
#104559=CARTESIAN_POINT ( 'NONE',  ( 8.224510206698953496, -14.34966873604960469, 102.9155762719810383 ) ) ;
#104560=CARTESIAN_POINT ( 'NONE',  ( -19.02544592524342804, 5.153800228976336051, 71.04057627198099567 ) ) ;
#104561=CARTESIAN_POINT ( 'NONE',  ( 18.62759615963271287, -10.81492255796078972, 78.33224293864770971 ) ) ;
#104563=CARTESIAN_POINT ( 'NONE',  ( 21.55341960407610458, 5.719274019375980345, 33.95724293864769550 ) ) ;
#104564=CARTESIAN_POINT ( 'NONE',  ( 19.53037848336980176, -5.499999999999891642, 67.35532783611444074 ) ) ;
#104565=CARTESIAN_POINT ( 'NONE',  ( 16.55341960407618274, -4.379528057220086978, 36.04275706135234714 ) ) ;
#104566=CARTESIAN_POINT ( 'NONE',  ( -4.379528057220328563, 16.55341960407611168, 100.2072429386476955 ) ) ;
#104567=CARTESIAN_POINT ( 'NONE',  ( -18.22780087662121673, -5.500000000000063061, 46.48459894673893444 ) ) ;
#104568=CARTESIAN_POINT ( 'NONE',  ( 9.474510206698971260, -16.51473224551069308, 87.91557627198102409 ) ) ;
#104569=CARTESIAN_POINT ( 'NONE',  ( -9.474510206698964154, 16.51473224551069663, 45.41557627198103120 ) ) ;
#104570=CARTESIAN_POINT ( 'NONE',  ( -16.55341960407611168, -4.379528057220339221, 81.45724293864769550 ) ) ;
#104572=CARTESIAN_POINT ( 'NONE',  ( 19.03943276465977164, -0.05219959533909143690, 113.7489096053143669 ) ) ;
#104573=CARTESIAN_POINT ( 'NONE',  ( 4.379528057220339221, -16.55341960407611168, 52.70724293864769550 ) ) ;
#104574=CARTESIAN_POINT ( 'NONE',  ( -13.97604488694547697, 13.89961937509957934, 103.1260903946856473 ) ) ;
#104575=CARTESIAN_POINT ( 'NONE',  ( -21.55341960407619339, 5.719274019375674811, 63.54275706135234003 ) ) ;
#104577=CARTESIAN_POINT ( 'NONE',  ( -13.97604488694527625, -13.89961937509977652, 96.87390960531433848 ) ) ;
#104578=CARTESIAN_POINT ( 'NONE',  ( -12.06949235617739369, -12.14591786802326823, 84.37609039468570415 ) ) ;
#104579=CARTESIAN_POINT ( 'NONE',  ( -9.474510206698964154, 16.51473224551069663, 25.41557627198103120 ) ) ;
#104580=CARTESIAN_POINT ( 'NONE',  ( -19.05341960407611168, -5.049401038298163336, 71.45724293864766707 ) ) ;
#104581=CARTESIAN_POINT ( 'NONE',  ( -0.05219959533907301413, -21.53943276465977519, 87.49890960531436690 ) ) ;
#104582=CARTESIAN_POINT ( 'NONE',  ( 9.564922557961047289, -16.46253265017146816, 110.4177570613523471 ) ) ;
#104583=CARTESIAN_POINT ( 'NONE',  ( -14.34966873604960291, -8.224510206698953496, 46.66557627198102409 ) ) ;
#104584=CARTESIAN_POINT ( 'NONE',  ( 10.72451020669871369, 18.67979575497193778, 57.08442372801901854 ) ) ;
#104585=CARTESIAN_POINT ( 'NONE',  ( -0.05219959533934338120, 16.53943276465976808, 87.50109039468568994 ) ) ;
#104586=CARTESIAN_POINT ( 'NONE',  ( 9.564922557960805705, 16.46253265017160317, 114.5822429386476955 ) ) ;
#104587=CARTESIAN_POINT ( 'NONE',  ( -16.46253265017160317, 9.564922557960807481, 110.8322429386476955 ) ) ;
#104588=CARTESIAN_POINT ( 'NONE',  ( -16.53943276465976808, -0.05219959533934237506, 108.7510903946857042 ) ) ;
#104589=CARTESIAN_POINT ( 'NONE',  ( -0.05219959533934338120, 16.53943276465976808, 57.50109039468568994 ) ) ;
#104590=CARTESIAN_POINT ( 'NONE',  ( -5.153800228976328057, -19.02544592524343514, 72.29057627198102409 ) ) ;
#104591=CARTESIAN_POINT ( 'NONE',  ( 9.564922557960805705, 16.46253265017160317, 74.58224293864769550 ) ) ;
#104592=CARTESIAN_POINT ( 'NONE',  ( 21.53943276465977519, 0.05219959533937863772, 71.25109039468568994 ) ) ;
#104593=CARTESIAN_POINT ( 'NONE',  ( 12.14591786802327356, -12.06949235617739191, 80.62609039468567573 ) ) ;
#104594=CARTESIAN_POINT ( 'NONE',  ( -0.05219959533910754901, -16.53943276465976808, 47.49890960531435979 ) ) ;
#104595=CARTESIAN_POINT ( 'NONE',  ( -0.05219959533909027116, -19.03943276465977164, 52.49890960531436690 ) ) ;
#104596=CARTESIAN_POINT ( 'NONE',  ( 0.05219959533909260263, 19.03943276465977164, 44.99890960531435979 ) ) ;
#104597=CARTESIAN_POINT ( 'NONE',  ( -14.29746914071037622, -8.314922557961029526, 44.16775706135234714 ) ) ;
#104599=CARTESIAN_POINT ( 'NONE',  ( -19.03943276465977164, -0.05219959533935918106, 98.75109039468567573 ) ) ;
#104600=CARTESIAN_POINT ( 'NONE',  ( -16.52544592524342804, 4.483927247898546575, 91.04057627198103830 ) ) ;
#104601=CARTESIAN_POINT ( 'NONE',  ( 5.153800228976335163, 19.02544592524342804, 64.79057627198100988 ) ) ;
#104602=CARTESIAN_POINT ( 'NONE',  ( -9.564922557961040184, 16.46253265017147172, 97.91775706135233293 ) ) ;
#104604=CARTESIAN_POINT ( 'NONE',  ( 0.05219959533937995610, -21.53943276465977519, 100.0010903946857042 ) ) ;
#104605=CARTESIAN_POINT ( 'NONE',  ( -0.05219959533934338120, 16.53943276465976808, 72.50109039468568994 ) ) ;
#104606=DIRECTION ( 'NONE',  ( 0.000000000000000000, -0.000000000000000000, 1.000000000000000000 ) ) ;
#104607=CARTESIAN_POINT ( 'NONE',  ( 10.72451020669898902, -18.67979575497178502, 62.91557627198102409 ) ) ;
#104608=CARTESIAN_POINT ( 'NONE',  ( -14.34966873604972548, 8.224510206698743886, 53.33442372801901854 ) ) ;
#104610=CARTESIAN_POINT ( 'NONE',  ( 0.05219959533936267826, -19.03943276465977164, 40.00109039468566152 ) ) ;
#104611=CARTESIAN_POINT ( 'NONE',  ( -19.05341960407611168, -5.049401038298163336, 96.45724293864769550 ) ) ;
#104612=CARTESIAN_POINT ( 'NONE',  ( -13.97604488694527625, -13.89961937509977652, 26.87390960531434558 ) ) ;
#104613=CARTESIAN_POINT ( 'NONE',  ( -5.049401038298153566, 19.05341960407611168, 60.20724293864768129 ) ) ;
#104614=CARTESIAN_POINT ( 'NONE',  ( 10.81492255796106328, -18.62759615963255655, 70.41775706135236135 ) ) ;
#104615=CARTESIAN_POINT ( 'NONE',  ( 19.05341960407617918, -5.049401038297876454, 51.04275706135231871 ) ) ;
#104616=CARTESIAN_POINT ( 'NONE',  ( -9.564922557961040184, 16.46253265017147172, 32.91775706135233293 ) ) ;
#104617=CARTESIAN_POINT ( 'NONE',  ( 9.564922557960805705, 16.46253265017160317, 54.58224293864769550 ) ) ;
#104618=CARTESIAN_POINT ( 'NONE',  ( 0.05219959533907565091, 21.53943276465977519, 29.99890960531435979 ) ) ;
#104619=CARTESIAN_POINT ( 'NONE',  ( -21.53943276465977519, -0.05219959533937600094, 88.75109039468567573 ) ) ;
#104620=CARTESIAN_POINT ( 'NONE',  ( 19.05341960407611168, 5.049401038298154454, 68.95724293864769550 ) ) ;
#104621=CARTESIAN_POINT ( 'NONE',  ( -10.81492255796105439, 18.62759615963255655, 97.91775706135236135 ) ) ;
#104622=CARTESIAN_POINT ( 'NONE',  ( 15.80617190586746368, 15.72974639402197994, 34.37390960531435979 ) ) ;
#104623=CARTESIAN_POINT ( 'NONE',  ( 5.049401038298161559, -19.05341960407611168, 82.70724293864770971 ) ) ;
#104624=CARTESIAN_POINT ( 'NONE',  ( 10.72451020669871369, 18.67979575497193778, 42.08442372801901854 ) ) ;
#104625=CARTESIAN_POINT ( 'NONE',  ( -13.97604488694547697, 13.89961937509957934, 63.12609039468566152 ) ) ;
#104626=CARTESIAN_POINT ( 'NONE',  ( 5.153800228976335163, 19.02544592524342804, 39.79057627198100988 ) ) ;
#104627=CARTESIAN_POINT ( 'NONE',  ( -13.89961937509977652, 13.97604488694528158, 95.62390960531436690 ) ) ;
#104628=CARTESIAN_POINT ( 'NONE',  ( 0.05219959533934541429, -16.53943276465976808, 25.00109039468567218 ) ) ;
#104629=CARTESIAN_POINT ( 'NONE',  ( 4.483927247898545687, 16.52544592524342804, 84.79057627198102409 ) ) ;
#104630=CARTESIAN_POINT ( 'NONE',  ( 19.03943276465977164, -0.05219959533909143690, 73.74890960531435269 ) ) ;
#104631=CARTESIAN_POINT ( 'NONE',  ( 21.53943276465977519, -0.05219959533907433946, 53.74890960531437401 ) ) ;
#104632=CARTESIAN_POINT ( 'NONE',  ( -9.564922557961040184, 16.46253265017147172, 112.9177570613523329 ) ) ;
#104633=CARTESIAN_POINT ( 'NONE',  ( -15.72974639402176322, -15.80617190586768395, 24.37609039468567573 ) ) ;
#104634=CARTESIAN_POINT ( 'NONE',  ( -15.72974639402176322, -15.80617190586768395, 74.37609039468568994 ) ) ;
#104635=CARTESIAN_POINT ( 'NONE',  ( -4.379528057220086978, -16.55341960407618274, 69.79275706135234714 ) ) ;
#104636=CARTESIAN_POINT ( 'NONE',  ( -16.52544592524335698, -4.483927247898792601, 63.95942372801901854 ) ) ;
#104638=( BOUNDED_CURVE ( )  B_SPLINE_CURVE ( 2, ( #78842, #93015, #154701, #140520, #77851, #33351, #139518, #95010, #1001, #126343, #45537, #34344, #80829 ),
 .UNSPECIFIED., .F., .F. ) 
 B_SPLINE_CURVE_WITH_KNOTS ( ( 3, 2, 2, 2, 2, 2, 3 ),
 ( 0.1340550636175563970, 0.1359649122807017607, 0.1403508771929824483, 0.1447368421052631637, 0.1491228070175438514, 0.1535087719298245668, 0.1554643004150602359 ),
 .UNSPECIFIED. ) 
 CURVE ( )  GEOMETRIC_REPRESENTATION_ITEM ( )  RATIONAL_B_SPLINE_CURVE ( ( 0.9832469066685285419, 0.9851625545550100060, 1.000000000000000000, 0.9659258262890683122, 1.000000000000000000, 0.9659258262890683122, 1.000000000000000000, 0.9659258262890683122, 1.000000000000000000, 0.9659258262890683122, 1.000000000000000000, 0.9848076720550082985, 0.9831626618144004848 ) ) 
 REPRESENTATION_ITEM ( '' )  );
#104639=CARTESIAN_POINT ( 'NONE',  ( -16.51473224551069308, -9.474510206698971260, 61.66557627198103120 ) ) ;
#104640=CARTESIAN_POINT ( 'NONE',  ( -12.06949235617739369, -12.14591786802326823, 104.3760903946856899 ) ) ;
#104641=CARTESIAN_POINT ( 'NONE',  ( 9.474510206698729675, 16.51473224551082808, 47.08442372801900433 ) ) ;
#104642=CARTESIAN_POINT ( 'NONE',  ( -10.72451020669898014, 18.67979575497178502, 110.4155762719810383 ) ) ;
#104643=CARTESIAN_POINT ( 'NONE',  ( -12.06949235617756955, 12.14591786802309770, 65.62390960531436690 ) ) ;
#104644=CARTESIAN_POINT ( 'NONE',  ( 9.564922557960805705, 16.46253265017160317, 94.58224293864769550 ) ) ;
#104645=CARTESIAN_POINT ( 'NONE',  ( 4.483927247898790824, -16.52544592524335698, 95.20942372801903275 ) ) ;
#104646=CARTESIAN_POINT ( 'NONE',  ( -10.72451020669870658, -18.67979575497194134, 54.58442372801901143 ) ) ;
#104647=CARTESIAN_POINT ( 'NONE',  ( 16.55341960407618274, -4.379528057220086978, 26.04275706135235779 ) ) ;
#104648=CARTESIAN_POINT ( 'NONE',  ( 15.72974639402176855, 15.80617190586768217, 21.87609039468567573 ) ) ;
#104649=CARTESIAN_POINT ( 'NONE',  ( -16.53943276465976808, 0.05219959533911058130, 56.24890960531436690 ) ) ;
#104651=ORIENTED_EDGE ( 'NONE', *, *, #196038, .T. ) ;
#104652=CARTESIAN_POINT ( 'NONE',  ( -5.823673210054116645, -21.52544592524344225, 97.29057627198105251 ) ) ;
#104653=CARTESIAN_POINT ( 'NONE',  ( -4.483927247898539470, -16.52544592524342804, 42.29057627198103120 ) ) ;
#104654=VERTEX_POINT ( 'NONE', #66206 ) ;
#104656=CARTESIAN_POINT ( 'NONE',  ( 18.62759615963271287, -10.81492255796078972, 28.33224293864769550 ) ) ;
#104657=CARTESIAN_POINT ( 'NONE',  ( -5.823673210054431948, 21.52544592524334988, 37.70942372801900433 ) ) ;
#104658=CARTESIAN_POINT ( 'NONE',  ( 4.379528057220339221, -16.55341960407611168, 62.70724293864769550 ) ) ;
#104660=VECTOR ( 'NONE', #37536, 1000.000000000000000 ) ;
#104661=CARTESIAN_POINT ( 'NONE',  ( 10.81492255796078972, 18.62759615963270932, 69.58224293864769550 ) ) ;
#104662=CARTESIAN_POINT ( 'NONE',  ( -0.05219959533909027116, -19.03943276465977164, 77.49890960531435269 ) ) ;
#104663=CARTESIAN_POINT ( 'NONE',  ( 16.51473224551069308, 9.474510206698969483, 29.16557627198103475 ) ) ;
#104664=CARTESIAN_POINT ( 'NONE',  ( 13.89961937509957401, 13.97604488694547697, 66.87609039468567573 ) ) ;
#104665=CARTESIAN_POINT ( 'NONE',  ( 5.823673210054125526, 21.52544592524343514, 54.79057627198104541 ) ) ;
#104666=CARTESIAN_POINT ( 'NONE',  ( 16.46253265017160672, -9.564922557960803928, 58.33224293864769550 ) ) ;
#104668=CARTESIAN_POINT ( 'NONE',  ( -14.29746914071037622, -8.314922557961029526, 39.16775706135235424 ) ) ;
#104669=CARTESIAN_POINT ( 'NONE',  ( 18.62759615963255655, 10.81492255796105972, 21.66775706135235069 ) ) ;
#104670=CARTESIAN_POINT ( 'NONE',  ( 4.379528057220339221, -16.55341960407611168, 42.70724293864770260 ) ) ;
#104671=CARTESIAN_POINT ( 'NONE',  ( -13.89961937509977652, 13.97604488694528158, 100.6239096053143669 ) ) ;
#104672=CARTESIAN_POINT ( 'NONE',  ( -18.62759615963270932, 10.81492255796079327, 70.83224293864770971 ) ) ;
#104673=CARTESIAN_POINT ( 'NONE',  ( -5.823673210054116645, -21.52544592524344225, 102.2905762719810383 ) ) ;
#104674=CARTESIAN_POINT ( 'NONE',  ( -4.483927247898782831, 16.52544592524335698, 32.70942372801900433 ) ) ;
#104675=CARTESIAN_POINT ( 'NONE',  ( 15.72974639402199770, -15.80617190586745480, 53.12390960531436690 ) ) ;
#104676=CARTESIAN_POINT ( 'NONE',  ( 15.72974639402176855, 15.80617190586768217, 96.87609039468568994 ) ) ;
#104677=CARTESIAN_POINT ( 'NONE',  ( -13.97604488694527625, -13.89961937509977652, 41.87390960531435979 ) ) ;
#104678=CARTESIAN_POINT ( 'NONE',  ( -13.89961937509977652, 13.97604488694528158, 100.6239096053143669 ) ) ;
#104679=CARTESIAN_POINT ( 'NONE',  ( -5.049401038298153566, 19.05341960407611168, 80.20724293864769550 ) ) ;
#104680=CARTESIAN_POINT ( 'NONE',  ( 16.31925111598412315, -7.325300261831691806, 87.66424538967174840 ) ) ;
#104681=CARTESIAN_POINT ( 'NONE',  ( -13.97604488694547697, 13.89961937509957934, 58.12609039468566863 ) ) ;
#104682=CARTESIAN_POINT ( 'NONE',  ( 10.72451020669871369, 18.67979575497193778, 107.0844237280190043 ) ) ;
#104683=CARTESIAN_POINT ( 'NONE',  ( -5.823673210054116645, -21.52544592524344225, 27.29057627198103120 ) ) ;
#104684=CARTESIAN_POINT ( 'NONE',  ( -12.14591786802326823, 12.06949235617739902, 98.12609039468570415 ) ) ;
#104685=CARTESIAN_POINT ( 'NONE',  ( 13.97604488694548053, -13.89961937509957401, 85.62609039468568994 ) ) ;
#104687=CARTESIAN_POINT ( 'NONE',  ( 5.049401038297881783, 19.05341960407617563, 87.29275706135234714 ) ) ;
#104688=CARTESIAN_POINT ( 'NONE',  ( 16.51473224551083163, -9.474510206698727899, 50.83442372801899722 ) ) ;
#104689=CARTESIAN_POINT ( 'NONE',  ( 17.05116617787822975, 6.768360034955819948, 108.8432444674080415 ) ) ;
#104690=CARTESIAN_POINT ( 'NONE',  ( -0.05219959533909027116, -19.03943276465977164, 42.49890960531435269 ) ) ;
#104691=CARTESIAN_POINT ( 'NONE',  ( 12.14591786802309770, 12.06949235617756955, 49.37390960531436690 ) ) ;
#104692=CARTESIAN_POINT ( 'NONE',  ( -16.46253265017160317, 9.564922557960807481, 40.83224293864769550 ) ) ;
#104693=CARTESIAN_POINT ( 'NONE',  ( -14.34966873604960291, -8.224510206698953496, 46.66557627198102409 ) ) ;
#104694=DIRECTION ( 'NONE',  ( -0.000000000000000000, -1.000000000000000000, -0.000000000000000000 ) ) ;
#104695=CARTESIAN_POINT ( 'NONE',  ( 12.06949235617739724, 12.14591786802326823, 106.8760903946856899 ) ) ;
#104696=CARTESIAN_POINT ( 'NONE',  ( -9.564922557960796823, -16.46253265017161027, 52.08224293864768839 ) ) ;
#104697=CARTESIAN_POINT ( 'NONE',  ( -10.72451020669870658, -18.67979575497194134, 104.5844237280190185 ) ) ;
#104698=CARTESIAN_POINT ( 'NONE',  ( -16.53943276465976808, -0.05219959533934237506, 23.75109039468567929 ) ) ;
#104699=CARTESIAN_POINT ( 'NONE',  ( -18.67979575497178146, -10.72451020669898902, 36.66557627198103120 ) ) ;
#104700=CARTESIAN_POINT ( 'NONE',  ( 10.81492255796106328, -18.62759615963255655, 95.41775706135234714 ) ) ;
#104701=CARTESIAN_POINT ( 'NONE',  ( 9.564922557960805705, 16.46253265017160317, 109.5822429386476955 ) ) ;
#104702=CARTESIAN_POINT ( 'NONE',  ( 19.05341960407611168, 5.049401038298154454, 78.95724293864769550 ) ) ;
#104704=CARTESIAN_POINT ( 'NONE',  ( 5.719274019375991003, -21.55341960407610458, 112.7072429386476955 ) ) ;
#104705=CARTESIAN_POINT ( 'NONE',  ( -16.55341960407611168, -4.379528057220339221, 86.45724293864770971 ) ) ;
#104706=CARTESIAN_POINT ( 'NONE',  ( 5.719274019375991003, -21.55341960407610458, 72.70724293864769550 ) ) ;
#104707=CARTESIAN_POINT ( 'NONE',  ( 19.05341960407611168, 5.049401038298154454, 68.95724293864769550 ) ) ;
#104708=CARTESIAN_POINT ( 'NONE',  ( -5.823673210054116645, -21.52544592524344225, 102.2905762719810383 ) ) ;
#104710=CARTESIAN_POINT ( 'NONE',  ( 13.97604488694527802, 13.89961937509977652, 64.37390960531436690 ) ) ;
#104711=CARTESIAN_POINT ( 'NONE',  ( -4.379528057220328563, 16.55341960407611168, 90.20724293864770971 ) ) ;
#104713=CARTESIAN_POINT ( 'NONE',  ( -19.05341960407611168, -5.049401038298163336, 61.45724293864769550 ) ) ;
#104714=CARTESIAN_POINT ( 'NONE',  ( -5.153800228976607833, 19.02544592524334988, 82.70942372801897591 ) ) ;
#104715=CARTESIAN_POINT ( 'NONE',  ( 4.379528057220339221, -16.55341960407611168, 102.7072429386476955 ) ) ;
#104716=CARTESIAN_POINT ( 'NONE',  ( -5.719274019375665041, -21.55341960407619695, 54.79275706135235424 ) ) ;
#104717=CARTESIAN_POINT ( 'NONE',  ( -16.46253265017160317, 9.564922557960807481, 45.83224293864769550 ) ) ;
#104718=CARTESIAN_POINT ( 'NONE',  ( -15.72974639402176322, -15.80617190586768395, 19.37609039468568639 ) ) ;
#104719=CARTESIAN_POINT ( 'NONE',  ( -16.52544592524342804, 4.483927247898546575, 101.0405762719810383 ) ) ;
#104721=CARTESIAN_POINT ( 'NONE',  ( 0.05219959533909260263, 19.03943276465977164, 59.99890960531436690 ) ) ;
#104723=CARTESIAN_POINT ( 'NONE',  ( -16.51473224551082808, 9.474510206698731452, 103.3344237280190043 ) ) ;
#104724=CARTESIAN_POINT ( 'NONE',  ( 13.89961937509977652, -13.97604488694527269, 108.1239096053143669 ) ) ;
#104725=CARTESIAN_POINT ( 'NONE',  ( -18.67979575497193778, 10.72451020669871902, 53.33442372801901854 ) ) ;
#104726=CARTESIAN_POINT ( 'NONE',  ( 16.51473224551069308, 9.474510206698969483, 99.16557627198102409 ) ) ;
#104727=CARTESIAN_POINT ( 'NONE',  ( 9.564922557961047289, -16.46253265017146816, 80.41775706135234714 ) ) ;
#104728=CARTESIAN_POINT ( 'NONE',  ( 13.89961937509977652, -13.97604488694527269, 53.12390960531434558 ) ) ;
#104729=CARTESIAN_POINT ( 'NONE',  ( 8.314922557960818139, 14.29746914071049879, 79.58224293864769550 ) ) ;
#104730=CARTESIAN_POINT ( 'NONE',  ( 9.564922557960805705, 16.46253265017160317, 94.58224293864769550 ) ) ;
#104731=CARTESIAN_POINT ( 'NONE',  ( -12.06949235617756955, 12.14591786802309770, 80.62390960531438111 ) ) ;
#104732=CARTESIAN_POINT ( 'NONE',  ( 0.05219959533909260263, 19.03943276465977164, 89.99890960531436690 ) ) ;
#104734=CARTESIAN_POINT ( 'NONE',  ( 13.89961937509957401, 13.97604488694547697, 26.87609039468566507 ) ) ;
#104735=CARTESIAN_POINT ( 'NONE',  ( -5.153800228976328057, -19.02544592524343514, 47.29057627198102409 ) ) ;
#104736=CARTESIAN_POINT ( 'NONE',  ( -16.55341960407611168, -4.379528057220339221, 26.45724293864768839 ) ) ;
#104737=CARTESIAN_POINT ( 'NONE',  ( -13.97604488694527625, -13.89961937509977652, 31.87390960531435979 ) ) ;
#104739=CARTESIAN_POINT ( 'NONE',  ( 0.05219959533937995610, -21.53943276465977519, 40.00109039468567573 ) ) ;
#104740=CARTESIAN_POINT ( 'NONE',  ( -13.89961937509957401, -13.97604488694547875, 79.37609039468567573 ) ) ;
#104741=CARTESIAN_POINT ( 'NONE',  ( -16.53943276465976808, 0.05219959533911058130, 41.24890960531435269 ) ) ;
#104742=CARTESIAN_POINT ( 'NONE',  ( -21.55341960407610458, -5.719274019375992779, 86.45724293864770971 ) ) ;
#104743=CARTESIAN_POINT ( 'NONE',  ( 15.80617190586746368, 15.72974639402197994, 29.37390960531435269 ) ) ;
#104744=CARTESIAN_POINT ( 'NONE',  ( 14.34966873604960469, 8.224510206698951720, 64.16557627198102409 ) ) ;
#104745=CARTESIAN_POINT ( 'NONE',  ( 5.153800228976335163, 19.02544592524342804, 44.79057627198103830 ) ) ;
#104746=CARTESIAN_POINT ( 'NONE',  ( -16.53943276465976808, -0.05219959533934237506, 103.7510903946857042 ) ) ;
#104747=CARTESIAN_POINT ( 'NONE',  ( -4.379528057220086978, -16.55341960407618274, 69.79275706135234714 ) ) ;
#104748=CARTESIAN_POINT ( 'NONE',  ( 18.67979575497178502, 10.72451020669898547, 34.16557627198102409 ) ) ;
#104749=CARTESIAN_POINT ( 'NONE',  ( -0.05219959533936034679, 19.03943276465977164, 22.50109039468566152 ) ) ;
#104750=CARTESIAN_POINT ( 'NONE',  ( 19.05341960407611168, 5.049401038298154454, 93.95724293864769550 ) ) ;
#104751=CARTESIAN_POINT ( 'NONE',  ( -19.02544592524342804, 5.153800228976336051, 61.04057627198103120 ) ) ;
#104752=CARTESIAN_POINT ( 'NONE',  ( -12.14591786802326823, 12.06949235617739902, 78.12609039468570415 ) ) ;
#104753=CARTESIAN_POINT ( 'NONE',  ( 19.05341960407611168, 5.049401038298154454, 28.95724293864769550 ) ) ;
#104754=CARTESIAN_POINT ( 'NONE',  ( -16.52544592524342804, 4.483927247898546575, 36.04057627198102409 ) ) ;
#104755=CARTESIAN_POINT ( 'NONE',  ( 0.05219959533909260263, 19.03943276465977164, 104.9989096053143669 ) ) ;
#104756=CARTESIAN_POINT ( 'NONE',  ( 19.02544592524343514, -5.153800228976328945, 88.54057627198102409 ) ) ;
#104757=CARTESIAN_POINT ( 'NONE',  ( 21.55341960407610458, 5.719274019375980345, 23.95724293864769550 ) ) ;
#104759=CARTESIAN_POINT ( 'NONE',  ( -16.53943276465976808, 0.05219959533911058130, 71.24890960531435269 ) ) ;
#104761=CARTESIAN_POINT ( 'NONE',  ( -4.379528057220328563, 16.55341960407611168, 70.20724293864769550 ) ) ;
#104762=CARTESIAN_POINT ( 'NONE',  ( 8.314922557961029526, -14.29746914071037800, 55.41775706135234714 ) ) ;
#104765=CARTESIAN_POINT ( 'NONE',  ( -0.05219959533936034679, 19.03943276465977164, 57.50109039468566863 ) ) ;
#104766=CARTESIAN_POINT ( 'NONE',  ( 19.02544592524343514, -5.153800228976328945, 88.54057627198102409 ) ) ;
#104767=CARTESIAN_POINT ( 'NONE',  ( -16.46253265017146816, -9.564922557961047289, 59.16775706135233293 ) ) ;
#104769=CARTESIAN_POINT ( 'NONE',  ( -13.97604488694547697, 13.89961937509957934, 113.1260903946856757 ) ) ;
#104770=CARTESIAN_POINT ( 'NONE',  ( -0.05219959533934338120, 16.53943276465976808, 92.50109039468567573 ) ) ;
#104771=CARTESIAN_POINT ( 'NONE',  ( -13.89961937509977652, 13.97604488694528158, 35.62390960531435269 ) ) ;
#104772=CARTESIAN_POINT ( 'NONE',  ( 10.81492255796078972, 18.62759615963270932, 24.58224293864768839 ) ) ;
#104773=CARTESIAN_POINT ( 'NONE',  ( -0.05219959533937732626, 21.53943276465977519, 52.50109039468567573 ) ) ;
#104774=CARTESIAN_POINT ( 'NONE',  ( -13.97604488694547697, 13.89961937509957934, 108.1260903946856331 ) ) ;
#104776=CARTESIAN_POINT ( 'NONE',  ( -5.153800228976328057, -19.02544592524343514, 72.29057627198102409 ) ) ;
#104778=CARTESIAN_POINT ( 'NONE',  ( -14.29746914071049879, 8.314922557960819915, 70.83224293864770971 ) ) ;
#104779=CARTESIAN_POINT ( 'NONE',  ( -19.03943276465977164, 0.05219959533909376836, 66.24890960531436690 ) ) ;
#104780=CARTESIAN_POINT ( 'NONE',  ( -16.51473224551069308, -9.474510206698971260, 76.66557627198103830 ) ) ;
#104781=CARTESIAN_POINT ( 'NONE',  ( 5.153800228976615827, -19.02544592524334988, 75.20942372801896170 ) ) ;
#104782=CARTESIAN_POINT ( 'NONE',  ( -10.72451020669898014, 18.67979575497178502, 60.41557627198102409 ) ) ;
#104783=CARTESIAN_POINT ( 'NONE',  ( 8.314922557960818139, 14.29746914071049879, 114.5822429386477097 ) ) ;
#104784=CARTESIAN_POINT ( 'NONE',  ( -13.97604488694547697, 13.89961937509957934, 53.12609039468565442 ) ) ;
#104785=CARTESIAN_POINT ( 'NONE',  ( -9.474510206698964154, 16.51473224551069663, 55.41557627198103120 ) ) ;
#104786=CARTESIAN_POINT ( 'NONE',  ( 0.05219959533909260263, 19.03943276465977164, 89.99890960531436690 ) ) ;
#104787=CARTESIAN_POINT ( 'NONE',  ( -5.719274019375978568, 21.55341960407610458, 85.20724293864770971 ) ) ;
#104788=CARTESIAN_POINT ( 'NONE',  ( 16.53943276465976808, -0.05219959533910856209, 78.74890960531436690 ) ) ;
#104789=CARTESIAN_POINT ( 'NONE',  ( 16.51473224551083163, -9.474510206698727899, 45.83442372801900433 ) ) ;
#104790=CARTESIAN_POINT ( 'NONE',  ( -0.05219959533907301413, -21.53943276465977519, 82.49890960531436690 ) ) ;
#104791=CARTESIAN_POINT ( 'NONE',  ( 5.719274019375991003, -21.55341960407610458, 62.70724293864769550 ) ) ;
#104792=CARTESIAN_POINT ( 'NONE',  ( 12.06949235617757843, -12.14591786802309237, 33.12390960531435979 ) ) ;
#104793=CARTESIAN_POINT ( 'NONE',  ( 18.62759615963255655, 10.81492255796105972, 106.6677570613523756 ) ) ;
#104794=CARTESIAN_POINT ( 'NONE',  ( 0.05219959533909260263, 19.03943276465977164, 79.99890960531436690 ) ) ;
#104795=CARTESIAN_POINT ( 'NONE',  ( 9.564922557960805705, 16.46253265017160317, 29.58224293864769550 ) ) ;
#104797=CARTESIAN_POINT ( 'NONE',  ( 10.81492255796106328, -18.62759615963255655, 40.41775706135234714 ) ) ;
#104798=CARTESIAN_POINT ( 'NONE',  ( -18.62759615963255300, -10.81492255796106328, 39.16775706135235424 ) ) ;
#104799=CARTESIAN_POINT ( 'NONE',  ( -19.02544592524342804, 5.153800228976336051, 46.04057627198101699 ) ) ;
#104800=CARTESIAN_POINT ( 'NONE',  ( 18.62759615963255655, 10.81492255796105972, 21.66775706135235069 ) ) ;
#104801=CARTESIAN_POINT ( 'NONE',  ( -9.474510206698720793, -16.51473224551083518, 64.58442372801900433 ) ) ;
#104802=CARTESIAN_POINT ( 'NONE',  ( -5.049401038298153566, 19.05341960407611168, 30.20724293864768839 ) ) ;
#104803=CARTESIAN_POINT ( 'NONE',  ( 8.314922557961029526, -14.29746914071037800, 25.41775706135235779 ) ) ;
#104805=CARTESIAN_POINT ( 'NONE',  ( 8.314922557961029526, -14.29746914071037800, 70.41775706135236135 ) ) ;
#104806=CARTESIAN_POINT ( 'NONE',  ( -16.46253265017160317, 9.564922557960807481, 45.83224293864769550 ) ) ;
#104808=CARTESIAN_POINT ( 'NONE',  ( -13.97604488694527625, -13.89961937509977652, 91.87390960531432427 ) ) ;
#104809=CARTESIAN_POINT ( 'NONE',  ( -16.53943276465976808, 0.05219959533911058130, 116.2489096053143669 ) ) ;
#104810=CARTESIAN_POINT ( 'NONE',  ( -10.81492255796078084, -18.62759615963271287, 62.08224293864769550 ) ) ;
#104811=CARTESIAN_POINT ( 'NONE',  ( -16.55341960407617563, 4.379528057220093196, 43.54275706135235424 ) ) ;
#104812=CARTESIAN_POINT ( 'NONE',  ( 15.80617190586769283, -15.72974639402175789, 95.62609039468568994 ) ) ;
#104813=CARTESIAN_POINT ( 'NONE',  ( -13.89961937509977652, 13.97604488694528158, 35.62390960531435269 ) ) ;
#104814=CARTESIAN_POINT ( 'NONE',  ( -4.483927247898539470, -16.52544592524342804, 32.29057627198102409 ) ) ;
#104815=CARTESIAN_POINT ( 'NONE',  ( 4.379528057220339221, -16.55341960407611168, 72.70724293864769550 ) ) ;
#104816=CARTESIAN_POINT ( 'NONE',  ( 16.51473224551069308, 9.474510206698969483, 64.16557627198102409 ) ) ;
#104817=CARTESIAN_POINT ( 'NONE',  ( -10.72451020669870658, -18.67979575497194134, 109.5844237280190328 ) ) ;
#104818=CARTESIAN_POINT ( 'NONE',  ( 21.55341960407619695, -5.719274019375665929, 21.04275706135234714 ) ) ;
#104819=CARTESIAN_POINT ( 'NONE',  ( 9.564922557960805705, 16.46253265017160317, 79.58224293864769550 ) ) ;
#104820=CARTESIAN_POINT ( 'NONE',  ( 21.55341960407619695, -5.719274019375665929, 86.04275706135236135 ) ) ;
#104821=CARTESIAN_POINT ( 'NONE',  ( 16.52544592524335698, 4.483927247898782831, 56.45942372801902565 ) ) ;
#104822=CARTESIAN_POINT ( 'NONE',  ( -8.314922557961024197, 14.29746914071037800, 32.91775706135234714 ) ) ;
#104823=CARTESIAN_POINT ( 'NONE',  ( 16.55341960407611168, 4.379528057220329451, 93.95724293864770971 ) ) ;
#104824=CARTESIAN_POINT ( 'NONE',  ( -0.05219959533937732626, 21.53943276465977519, 102.5010903946856899 ) ) ;
#104825=CARTESIAN_POINT ( 'NONE',  ( -12.14591786802309592, -12.06949235617757132, 36.87390960531435979 ) ) ;
#104826=CARTESIAN_POINT ( 'NONE',  ( 5.153800228976335163, 19.02544592524342804, 34.79057627198102409 ) ) ;
#104827=CARTESIAN_POINT ( 'NONE',  ( 12.14591786802327356, -12.06949235617739191, 50.62609039468568994 ) ) ;
#104828=CARTESIAN_POINT ( 'NONE',  ( 16.52544592524342804, -4.483927247898539470, 58.54057627198103120 ) ) ;
#104829=CARTESIAN_POINT ( 'NONE',  ( 14.29746914071037800, 8.314922557961029526, 101.6677570613523613 ) ) ;
#104830=CARTESIAN_POINT ( 'NONE',  ( 21.53943276465977519, -0.05219959533907433946, 23.74890960531435269 ) ) ;
#104831=CARTESIAN_POINT ( 'NONE',  ( -16.46253265017160317, 9.564922557960807481, 110.8322429386476955 ) ) ;
#104832=CARTESIAN_POINT ( 'NONE',  ( 5.153800228976615827, -19.02544592524334988, 20.20942372801899722 ) ) ;
#104833=CARTESIAN_POINT ( 'NONE',  ( -16.55341960407611168, -4.379528057220339221, 91.45724293864769550 ) ) ;
#104834=CARTESIAN_POINT ( 'NONE',  ( 5.153800228976335163, 19.02544592524342804, 94.79057627198103830 ) ) ;
#104836=CARTESIAN_POINT ( 'NONE',  ( -4.483927247898782831, 16.52544592524335698, 37.70942372801900433 ) ) ;
#104837=CARTESIAN_POINT ( 'NONE',  ( -19.05341960407611168, -5.049401038298163336, 41.45724293864769550 ) ) ;
#104838=CARTESIAN_POINT ( 'NONE',  ( -0.05219959533934338120, 16.53943276465976808, 47.50109039468568994 ) ) ;
#104839=CARTESIAN_POINT ( 'NONE',  ( 13.97604488694548053, -13.89961937509957401, 45.62609039468566863 ) ) ;
#104840=CARTESIAN_POINT ( 'NONE',  ( -5.153800228976328057, -19.02544592524343514, 52.29057627198100988 ) ) ;
#104841=CARTESIAN_POINT ( 'NONE',  ( 16.53943276465976808, 0.05219959533934440121, 86.25109039468568994 ) ) ;
#104842=CARTESIAN_POINT ( 'NONE',  ( 13.89961937509957401, 13.97604488694547697, 86.87609039468567573 ) ) ;
#104843=CARTESIAN_POINT ( 'NONE',  ( -16.51473224551082808, 9.474510206698731452, 33.33442372801899722 ) ) ;
#104844=CARTESIAN_POINT ( 'NONE',  ( -5.049401038298153566, 19.05341960407611168, 60.20724293864768129 ) ) ;
#104845=CARTESIAN_POINT ( 'NONE',  ( -16.55341960407611168, -4.379528057220339221, 101.4572429386476955 ) ) ;
#104847=CARTESIAN_POINT ( 'NONE',  ( 19.05341960407617918, -5.049401038297876454, 71.04275706135234714 ) ) ;
#104848=CARTESIAN_POINT ( 'NONE',  ( 5.823673210054125526, 21.52544592524343514, 69.79057627198102409 ) ) ;
#104849=CARTESIAN_POINT ( 'NONE',  ( -5.153800228976607833, 19.02544592524334988, 47.70942372801900433 ) ) ;
#104850=CARTESIAN_POINT ( 'NONE',  ( 16.51473224551069308, 9.474510206698969483, 109.1655762719810383 ) ) ;
#104852=CARTESIAN_POINT ( 'NONE',  ( 15.72974639402199770, -15.80617190586745480, 73.12390960531436690 ) ) ;
#104853=CARTESIAN_POINT ( 'NONE',  ( -17.05116617787824396, 6.768360034955813731, 83.65675553259198693 ) ) ;
#104854=CARTESIAN_POINT ( 'NONE',  ( 16.46253265017146816, 9.564922557961045513, 106.6677570613523471 ) ) ;
#104855=CARTESIAN_POINT ( 'NONE',  ( -18.22780087662123805, -5.499999999999968026, 98.98236817873106475 ) ) ;
#104856=CARTESIAN_POINT ( 'NONE',  ( -4.483927247898782831, 16.52544592524335698, 22.70942372801901499 ) ) ;
#104857=CARTESIAN_POINT ( 'NONE',  ( 13.97604488694527802, 13.89961937509977652, 34.37390960531436690 ) ) ;
#104858=CARTESIAN_POINT ( 'NONE',  ( 0.05219959533909260263, 19.03943276465977164, 109.9989096053143669 ) ) ;
#104859=CARTESIAN_POINT ( 'NONE',  ( 18.67979575497178502, 10.72451020669898547, 94.16557627198103830 ) ) ;
#104860=CARTESIAN_POINT ( 'NONE',  ( 5.823673210054444382, -21.52544592524334988, 55.20942372801902565 ) ) ;
#104861=CARTESIAN_POINT ( 'NONE',  ( 19.03943276465977164, 0.05219959533936151252, 101.2510903946856757 ) ) ;
#104862=CARTESIAN_POINT ( 'NONE',  ( 19.05341960407617918, -5.049401038297876454, 21.04275706135232582 ) ) ;
#104863=CARTESIAN_POINT ( 'NONE',  ( -12.06949235617739369, -12.14591786802326823, 104.3760903946856899 ) ) ;
#104864=CARTESIAN_POINT ( 'NONE',  ( -21.55341960407610458, -5.719274019375992779, 101.4572429386476955 ) ) ;
#104865=CARTESIAN_POINT ( 'NONE',  ( 4.483927247898545687, 16.52544592524342804, 44.79057627198103120 ) ) ;
#104866=CARTESIAN_POINT ( 'NONE',  ( -16.51473224551082808, 9.474510206698731452, 88.33442372801900433 ) ) ;
#104867=CARTESIAN_POINT ( 'NONE',  ( 19.05341960407617918, -5.049401038297876454, 51.04275706135231871 ) ) ;
#104868=CARTESIAN_POINT ( 'NONE',  ( 21.53943276465977519, 0.05219959533937863772, 71.25109039468568994 ) ) ;
#104869=CARTESIAN_POINT ( 'NONE',  ( 19.02544592524334988, 5.153800228976608722, 36.45942372801900433 ) ) ;
#104870=CARTESIAN_POINT ( 'NONE',  ( -14.34966873604960291, -8.224510206698953496, 111.6655762719810525 ) ) ;
#104871=CARTESIAN_POINT ( 'NONE',  ( 18.67979575497178502, 10.72451020669898547, 49.16557627198102409 ) ) ;
#104872=CARTESIAN_POINT ( 'NONE',  ( 0.05219959533910956823, 16.53943276465976808, 29.99890960531435979 ) ) ;
#104873=CARTESIAN_POINT ( 'NONE',  ( -18.62759615963255300, -10.81492255796106328, 109.1677570613523613 ) ) ;
#104874=CARTESIAN_POINT ( 'NONE',  ( 8.224510206698742110, 14.34966873604972548, 72.08442372801899012 ) ) ;
#104875=CARTESIAN_POINT ( 'NONE',  ( 14.34966873604960469, 8.224510206698951720, 29.16557627198103120 ) ) ;
#104876=CARTESIAN_POINT ( 'NONE',  ( -10.72451020669870658, -18.67979575497194134, 59.58442372801901854 ) ) ;
#104877=CARTESIAN_POINT ( 'NONE',  ( -21.53943276465977519, -0.05219959533937600094, 63.75109039468568284 ) ) ;
#104878=CARTESIAN_POINT ( 'NONE',  ( -10.81492255796078084, -18.62759615963271287, 67.08224293864770971 ) ) ;
#104879=ADVANCED_FACE ( 'NONE', ( #145033 ), #97513, .T. ) ;
#104880=VECTOR ( 'NONE', #174714, 1000.000000000000000 ) ;
#104881=CARTESIAN_POINT ( 'NONE',  ( -16.46253265017160317, 9.564922557960807481, 25.83224293864769194 ) ) ;
#104882=CARTESIAN_POINT ( 'NONE',  ( -10.72451020669870658, -18.67979575497194134, 39.58442372801901143 ) ) ;
#104883=CARTESIAN_POINT ( 'NONE',  ( 5.049401038298161559, -19.05341960407611168, 22.70724293864769194 ) ) ;
#104884=CARTESIAN_POINT ( 'NONE',  ( -5.153800228976328057, -19.02544592524343514, 42.29057627198101699 ) ) ;
#104885=CARTESIAN_POINT ( 'NONE',  ( -4.379528057220328563, 16.55341960407611168, 75.20724293864769550 ) ) ;
#104886=CARTESIAN_POINT ( 'NONE',  ( -16.46253265017160317, 9.564922557960807481, 90.83224293864769550 ) ) ;
#104887=CARTESIAN_POINT ( 'NONE',  ( -4.483927247898539470, -16.52544592524342804, 32.29057627198102409 ) ) ;
#104888=CARTESIAN_POINT ( 'NONE',  ( -14.29746914071049879, 8.314922557960819915, 100.8322429386477097 ) ) ;
#104889=CARTESIAN_POINT ( 'NONE',  ( 21.52544592524344225, -5.823673210054117533, 68.54057627198103830 ) ) ;
#104890=CARTESIAN_POINT ( 'NONE',  ( -18.67979575497178146, -10.72451020669898902, 106.6655762719810383 ) ) ;
#104891=CARTESIAN_POINT ( 'NONE',  ( 16.46253265017160672, -9.564922557960803928, 108.3322429386476955 ) ) ;
#104892=CARTESIAN_POINT ( 'NONE',  ( 19.05341960407611168, 5.049401038298154454, 68.95724293864769550 ) ) ;
#104893=CARTESIAN_POINT ( 'NONE',  ( -8.224510206698735004, -14.34966873604973081, 19.58442372801901143 ) ) ;
#104894=CARTESIAN_POINT ( 'NONE',  ( -18.67979575497178146, -10.72451020669898902, 51.66557627198102409 ) ) ;
#104895=CARTESIAN_POINT ( 'NONE',  ( -18.67979575497193778, 10.72451020669871902, 78.33442372801901854 ) ) ;
#104896=CARTESIAN_POINT ( 'NONE',  ( -9.564922557960796823, -16.46253265017161027, 82.08224293864768129 ) ) ;
#104897=CARTESIAN_POINT ( 'NONE',  ( -16.46253265017160317, 9.564922557960807481, 105.8322429386476955 ) ) ;
#104898=CARTESIAN_POINT ( 'NONE',  ( 14.34966873604972726, -8.224510206698740333, 80.83442372801901854 ) ) ;
#104899=CARTESIAN_POINT ( 'NONE',  ( 10.72451020669871369, 18.67979575497193778, 52.08442372801901854 ) ) ;
#104900=CARTESIAN_POINT ( 'NONE',  ( 10.81492255796106328, -18.62759615963255655, 105.4177570613523613 ) ) ;
#104901=CARTESIAN_POINT ( 'NONE',  ( 0.05219959533934541429, -16.53943276465976808, 60.00109039468568284 ) ) ;
#104902=CARTESIAN_POINT ( 'NONE',  ( 15.72974639402199770, -15.80617190586745480, 108.1239096053143811 ) ) ;
#104904=CARTESIAN_POINT ( 'NONE',  ( 9.564922557960805705, 16.46253265017160317, 114.5822429386476955 ) ) ;
#104905=CARTESIAN_POINT ( 'NONE',  ( -10.81492255796078084, -18.62759615963271287, 87.08224293864769550 ) ) ;
#104906=CARTESIAN_POINT ( 'NONE',  ( 19.02544592524334988, 5.153800228976608722, 46.45942372801899012 ) ) ;
#104907=CARTESIAN_POINT ( 'NONE',  ( 5.719274019375991003, -21.55341960407610458, 42.70724293864770260 ) ) ;
#104908=CARTESIAN_POINT ( 'NONE',  ( -16.51473224551069308, -9.474510206698971260, 81.66557627198103830 ) ) ;
#104909=CARTESIAN_POINT ( 'NONE',  ( -16.52544592524342804, 4.483927247898546575, 41.04057627198103120 ) ) ;
#104910=B_SPLINE_CURVE_WITH_KNOTS ( 'NONE', 3,
 ( #189126, #95094, #17272, #35416, #97068, #139599 ),
 .UNSPECIFIED., .F., .F.,
 ( 4, 2, 4 ),
 ( 0.007228050697041489385, 0.007608510107494970143, 0.007988969517948450033 ),
 .UNSPECIFIED. ) ;
#104913=CARTESIAN_POINT ( 'NONE',  ( -0.05219959533936034679, 19.03943276465977164, 97.50109039468567573 ) ) ;
#104914=CARTESIAN_POINT ( 'NONE',  ( 21.52544592524344225, -5.823673210054117533, 68.54057627198103830 ) ) ;
#104915=CARTESIAN_POINT ( 'NONE',  ( 8.314922557960818139, 14.29746914071049879, 49.58224293864769550 ) ) ;
#104916=CARTESIAN_POINT ( 'NONE',  ( -0.05219959533934338120, 16.53943276465976808, 37.50109039468568284 ) ) ;
#104917=CARTESIAN_POINT ( 'NONE',  ( -13.97604488694527625, -13.89961937509977652, 41.87390960531435979 ) ) ;
#104918=CARTESIAN_POINT ( 'NONE',  ( 21.52544592524334988, 5.823673210054432836, 21.45942372801901499 ) ) ;
#104919=CARTESIAN_POINT ( 'NONE',  ( -19.02544592524334988, -5.153800228976617603, 78.95942372801900433 ) ) ;
#104920=CARTESIAN_POINT ( 'NONE',  ( -9.564922557960796823, -16.46253265017161027, 77.08224293864769550 ) ) ;
#104921=CARTESIAN_POINT ( 'NONE',  ( 9.474510206698971260, -16.51473224551069308, 77.91557627198103830 ) ) ;
#104922=CARTESIAN_POINT ( 'NONE',  ( 15.72974639402199770, -15.80617190586745480, 83.12390960531436690 ) ) ;
#104923=CARTESIAN_POINT ( 'NONE',  ( 9.474510206698971260, -16.51473224551069308, 32.91557627198102409 ) ) ;
#104925=CARTESIAN_POINT ( 'NONE',  ( -0.05219959533910754901, -16.53943276465976808, 57.49890960531435979 ) ) ;
#104926=CARTESIAN_POINT ( 'NONE',  ( -9.564922557960796823, -16.46253265017161027, 92.08224293864769550 ) ) ;
#104928=CARTESIAN_POINT ( 'NONE',  ( 16.46253265017146816, 9.564922557961045513, 56.66775706135233293 ) ) ;
#104929=CARTESIAN_POINT ( 'NONE',  ( 15.72974639402199770, -15.80617190586745480, 73.12390960531436690 ) ) ;
#104930=CARTESIAN_POINT ( 'NONE',  ( 5.153800228976615827, -19.02544592524334988, 30.20942372801900433 ) ) ;
#104931=CARTESIAN_POINT ( 'NONE',  ( -5.049401038298153566, 19.05341960407611168, 85.20724293864766707 ) ) ;
#104932=CARTESIAN_POINT ( 'NONE',  ( -18.09867054820431775, -5.499999999999926281, 73.98393025253585620 ) ) ;
#104933=CARTESIAN_POINT ( 'NONE',  ( 21.55341960407610458, 5.719274019375980345, 23.95724293864769550 ) ) ;
#104935=CARTESIAN_POINT ( 'NONE',  ( -9.564922557960796823, -16.46253265017161027, 77.08224293864769550 ) ) ;
#104936=CARTESIAN_POINT ( 'NONE',  ( 21.52544592524334988, 5.823673210054432836, 46.45942372801901854 ) ) ;
#104937=CARTESIAN_POINT ( 'NONE',  ( -5.153800228976328057, -19.02544592524343514, 27.29057627198103120 ) ) ;
#104938=CARTESIAN_POINT ( 'NONE',  ( 10.81492255796078972, 18.62759615963270932, 114.5822429386477097 ) ) ;
#104939=CARTESIAN_POINT ( 'NONE',  ( -16.46253265017160317, 9.564922557960807481, 95.83224293864769550 ) ) ;
#104941=CARTESIAN_POINT ( 'NONE',  ( -15.72974639402176322, -15.80617190586768395, 34.37609039468568284 ) ) ;
#104943=CARTESIAN_POINT ( 'NONE',  ( -16.51473224551069308, -9.474510206698971260, 101.6655762719810241 ) ) ;
#104945=CARTESIAN_POINT ( 'NONE',  ( 18.62759615963271287, -10.81492255796078972, 103.3322429386476955 ) ) ;
#104946=CARTESIAN_POINT ( 'NONE',  ( 13.97604488694527802, 13.89961937509977652, 59.37390960531434558 ) ) ;
#104947=CARTESIAN_POINT ( 'NONE',  ( 0.05219959533934541429, -16.53943276465976808, 25.00109039468567218 ) ) ;
#104949=CARTESIAN_POINT ( 'NONE',  ( 10.81492255796106328, -18.62759615963255655, 100.4177570613523471 ) ) ;
#104950=CARTESIAN_POINT ( 'NONE',  ( 16.46253265017160672, -9.564922557960803928, 38.33224293864768839 ) ) ;
#104951=CARTESIAN_POINT ( 'NONE',  ( -18.62759615963255300, -10.81492255796106328, 99.16775706135234714 ) ) ;
#104952=CARTESIAN_POINT ( 'NONE',  ( -16.51473224551069308, -9.474510206698971260, 91.66557627198103830 ) ) ;
#104953=CARTESIAN_POINT ( 'NONE',  ( -15.80617190586768217, 15.72974639402176855, 58.12609039468568994 ) ) ;
#104955=CARTESIAN_POINT ( 'NONE',  ( -19.03943276465977164, 0.05219959533909376836, 101.2489096053143669 ) ) ;
#104956=CARTESIAN_POINT ( 'NONE',  ( -17.50000000000000000, 4.013004640162651349, 30.44605720994411513 ) ) ;
#104957=CARTESIAN_POINT ( 'NONE',  ( -14.29746914071037622, -8.314922557961029526, 54.16775706135235424 ) ) ;
#104958=CARTESIAN_POINT ( 'NONE',  ( 12.06949235617739724, 12.14591786802326823, 66.87609039468568994 ) ) ;
#104959=CARTESIAN_POINT ( 'NONE',  ( -5.823673210054431948, 21.52544592524334988, 52.70942372801902565 ) ) ;
#104960=CARTESIAN_POINT ( 'NONE',  ( -15.80617190586768217, 15.72974639402176855, 88.12609039468570415 ) ) ;
#104962=CARTESIAN_POINT ( 'NONE',  ( -16.52544592524335698, -4.483927247898792601, 28.95942372801902209 ) ) ;
#104963=CARTESIAN_POINT ( 'NONE',  ( 13.97604488694527802, 13.89961937509977652, 69.37390960531436690 ) ) ;
#104964=CARTESIAN_POINT ( 'NONE',  ( -19.02544592524342804, 5.153800228976336051, 101.0405762719810241 ) ) ;
#104966=CARTESIAN_POINT ( 'NONE',  ( 0.05219959533909260263, 19.03943276465977164, 24.99890960531435269 ) ) ;
#104967=CARTESIAN_POINT ( 'NONE',  ( 21.55341960407610458, 5.719274019375980345, 33.95724293864769550 ) ) ;
#104968=CARTESIAN_POINT ( 'NONE',  ( 12.14591786802327356, -12.06949235617739191, 90.62609039468567573 ) ) ;
#104969=CARTESIAN_POINT ( 'NONE',  ( 12.06949235617757843, -12.14591786802309237, 83.12390960531436690 ) ) ;
#104970=CARTESIAN_POINT ( 'NONE',  ( -13.97604488694527625, -13.89961937509977652, 71.87390960531433848 ) ) ;
#104971=CARTESIAN_POINT ( 'NONE',  ( -5.719274019375665041, -21.55341960407619695, 94.79275706135234714 ) ) ;
#104973=CARTESIAN_POINT ( 'NONE',  ( 16.53943276465976808, 0.05219959533934440121, 26.25109039468567573 ) ) ;
#104974=CARTESIAN_POINT ( 'NONE',  ( 12.14591786802309770, 12.06949235617756955, 74.37390960531436690 ) ) ;
#104975=CARTESIAN_POINT ( 'NONE',  ( 18.67979575497194134, -10.72451020669871369, 40.83442372801901854 ) ) ;
#104976=CARTESIAN_POINT ( 'NONE',  ( 5.823673210054125526, 21.52544592524343514, 74.79057627198105251 ) ) ;
#104977=CARTESIAN_POINT ( 'NONE',  ( 16.46253265017146816, 9.564922557961045513, 41.66775706135234003 ) ) ;
#104978=CARTESIAN_POINT ( 'NONE',  ( 15.50000000000000178, 5.499999999999998224, 120.0000000000000142 ) ) ;
#104979=CARTESIAN_POINT ( 'NONE',  ( -5.153800228976328057, -19.02544592524343514, 87.29057627198103830 ) ) ;
#104980=CARTESIAN_POINT ( 'NONE',  ( 4.483927247898545687, 16.52544592524342804, 44.79057627198103120 ) ) ;
#104981=CARTESIAN_POINT ( 'NONE',  ( 12.14591786802309770, 12.06949235617756955, 34.37390960531435979 ) ) ;
#104982=CARTESIAN_POINT ( 'NONE',  ( 4.379528057220092307, 16.55341960407617563, 107.2927570613523471 ) ) ;
#104983=CARTESIAN_POINT ( 'NONE',  ( 19.03943276465977164, 0.05219959533936151252, 61.25109039468566863 ) ) ;
#104985=CARTESIAN_POINT ( 'NONE',  ( -15.80617190586745835, -15.72974639402198527, 21.87390960531436690 ) ) ;
#104986=CARTESIAN_POINT ( 'NONE',  ( -12.14591786802309592, -12.06949235617757132, 91.87390960531436690 ) ) ;
#104987=CARTESIAN_POINT ( 'NONE',  ( -22.00000000000000000, -5.204748896376250896E-15, 42.49999999999999289 ) ) ;
#104988=CARTESIAN_POINT ( 'NONE',  ( 13.89961937509977652, -13.97604488694527269, 33.12390960531434558 ) ) ;
#104989=CARTESIAN_POINT ( 'NONE',  ( -10.72451020669898014, 18.67979575497178502, 30.41557627198101699 ) ) ;
#104990=CARTESIAN_POINT ( 'NONE',  ( -21.52544592524343514, 5.823673210054127303, 71.04057627198103830 ) ) ;
#104991=CARTESIAN_POINT ( 'NONE',  ( -12.14591786802309592, -12.06949235617757132, 111.8739096053143669 ) ) ;
#104992=CARTESIAN_POINT ( 'NONE',  ( -14.34966873604972548, 8.224510206698743886, 68.33442372801900433 ) ) ;
#104993=CARTESIAN_POINT ( 'NONE',  ( -16.51473224551069308, -9.474510206698971260, 46.66557627198102409 ) ) ;
#104994=CARTESIAN_POINT ( 'NONE',  ( 5.823673210054444382, -21.52544592524334988, 50.20942372801901854 ) ) ;
#104995=CARTESIAN_POINT ( 'NONE',  ( -12.06949235617756955, 12.14591786802309770, 110.6239096053143669 ) ) ;
#104996=B_SPLINE_CURVE_WITH_KNOTS ( 'NONE', 3,
 ( #120373, #151723, #59694, #74879, #103230, #198222, #149733, #166902, #133560, #181086, #178081, #39549, #132565, #42561, #71890, #11234, #163919, #164912, #101208, #87057, #86055, #182066 ),
 .UNSPECIFIED., .F., .F.,
 ( 4, 2, 2, 2, 2, 2, 2, 2, 2, 2, 4 ),
 ( 8.673617379884035472E-19, 0.001309639967555473270, 0.001964459951333209688, 0.002291869943222077897, 0.002455574939166497474, 0.002619279935110917917, 0.002782984931055337927, 0.002946689926999758371, 0.003274099918888572370, 0.003928919902666201669, 0.005238559870221456798 ),
 .UNSPECIFIED. ) ;
#104997=CARTESIAN_POINT ( 'NONE',  ( -19.03943276465977164, -0.05219959533935918106, 93.75109039468566152 ) ) ;
#105000=CARTESIAN_POINT ( 'NONE',  ( -18.67979575497178146, -10.72451020669898902, 31.66557627198102054 ) ) ;
#105001=DIRECTION ( 'NONE',  ( -0.000000000000000000, -0.000000000000000000, 1.000000000000000000 ) ) ;
#105002=CARTESIAN_POINT ( 'NONE',  ( -18.62759615963255300, -10.81492255796106328, 64.16775706135234714 ) ) ;
#105003=CARTESIAN_POINT ( 'NONE',  ( 12.14591786802327356, -12.06949235617739191, 55.62609039468568284 ) ) ;
#105004=CARTESIAN_POINT ( 'NONE',  ( -14.29746914071049879, 8.314922557960819915, 40.83224293864769550 ) ) ;
#105005=CARTESIAN_POINT ( 'NONE',  ( 10.72451020669898902, -18.67979575497178502, 72.91557627198103830 ) ) ;
#105006=CARTESIAN_POINT ( 'NONE',  ( 0.05219959533907565091, 21.53943276465977519, 64.99890960531435269 ) ) ;
#105008=CARTESIAN_POINT ( 'NONE',  ( -16.46253265017146816, -9.564922557961047289, 84.16775706135233293 ) ) ;
#105009=CARTESIAN_POINT ( 'NONE',  ( -5.049401038298153566, 19.05341960407611168, 110.2072429386476671 ) ) ;
#105012=CARTESIAN_POINT ( 'NONE',  ( 19.05341960407611168, 5.049401038298154454, 48.95724293864768129 ) ) ;
#105013=CARTESIAN_POINT ( 'NONE',  ( 14.34966873604960469, 8.224510206698951720, 114.1655762719810383 ) ) ;
#105015=CARTESIAN_POINT ( 'NONE',  ( -9.474510206698964154, 16.51473224551069663, 110.4155762719810383 ) ) ;
#105017=CARTESIAN_POINT ( 'NONE',  ( 4.379528057220092307, 16.55341960407617563, 67.29275706135234714 ) ) ;
#105018=CARTESIAN_POINT ( 'NONE',  ( 21.53943276465977519, -0.05219959533907433946, 108.7489096053143669 ) ) ;
#105019=CARTESIAN_POINT ( 'NONE',  ( 19.03943276465977164, -0.05219959533909143690, 53.74890960531436690 ) ) ;
#105020=CARTESIAN_POINT ( 'NONE',  ( 10.81492255796106328, -18.62759615963255655, 40.41775706135234714 ) ) ;
#105021=CARTESIAN_POINT ( 'NONE',  ( 5.049401038298161559, -19.05341960407611168, 97.70724293864766707 ) ) ;
#105024=CARTESIAN_POINT ( 'NONE',  ( -5.719274019375665041, -21.55341960407619695, 34.79275706135235424 ) ) ;
#105025=CARTESIAN_POINT ( 'NONE',  ( 5.049401038298161559, -19.05341960407611168, 112.7072429386476813 ) ) ;
#105026=CARTESIAN_POINT ( 'NONE',  ( -19.02544592524334988, -5.153800228976617603, 83.95942372801901854 ) ) ;
#105027=CARTESIAN_POINT ( 'NONE',  ( 19.02544592524334988, 5.153800228976608722, 36.45942372801900433 ) ) ;
#105028=CARTESIAN_POINT ( 'NONE',  ( 15.72974639402199770, -15.80617190586745480, 103.1239096053143811 ) ) ;
#105029=CARTESIAN_POINT ( 'NONE',  ( -19.03943276465977164, -0.05219959533935918106, 28.75109039468566507 ) ) ;
#105030=CARTESIAN_POINT ( 'NONE',  ( 9.474510206698729675, 16.51473224551082808, 47.08442372801900433 ) ) ;
#105031=CARTESIAN_POINT ( 'NONE',  ( 14.29746914071037800, 8.314922557961029526, 86.66775706135234714 ) ) ;
#105033=CARTESIAN_POINT ( 'NONE',  ( 19.03943276465977164, -0.05219959533909143690, 73.74890960531435269 ) ) ;
#105035=CARTESIAN_POINT ( 'NONE',  ( -0.05219959533937732626, 21.53943276465977519, 77.50109039468567573 ) ) ;
#105036=CARTESIAN_POINT ( 'NONE',  ( -10.81492255796105439, 18.62759615963255655, 82.91775706135234714 ) ) ;
#105038=CARTESIAN_POINT ( 'NONE',  ( -19.02544592524342804, 5.153800228976336051, 91.04057627198100988 ) ) ;
#105039=CARTESIAN_POINT ( 'NONE',  ( 21.52544592524334988, 5.823673210054432836, 56.45942372801902565 ) ) ;
#105040=CARTESIAN_POINT ( 'NONE',  ( 13.97604488694548053, -13.89961937509957401, 100.6260903946856615 ) ) ;
#105041=CARTESIAN_POINT ( 'NONE',  ( -19.02544592524342804, 5.153800228976336051, 66.04057627198103830 ) ) ;
#105042=CARTESIAN_POINT ( 'NONE',  ( 19.02544592524343514, -5.153800228976328945, 108.5405762719810383 ) ) ;
#105043=CARTESIAN_POINT ( 'NONE',  ( 19.05341960407611168, 5.049401038298154454, 78.95724293864769550 ) ) ;
#105044=CARTESIAN_POINT ( 'NONE',  ( -17.40861289039006010, -6.110651285853244907, 91.37232470827437680 ) ) ;
#105045=CARTESIAN_POINT ( 'NONE',  ( -13.97604488694527625, -13.89961937509977652, 66.87390960531436690 ) ) ;
#105046=CARTESIAN_POINT ( 'NONE',  ( -19.02544592524342804, 5.153800228976336051, 51.04057627198103120 ) ) ;
#105047=CARTESIAN_POINT ( 'NONE',  ( 18.67979575497178502, 10.72451020669898547, 114.1655762719810383 ) ) ;
#105048=CARTESIAN_POINT ( 'NONE',  ( -8.224510206698735004, -14.34966873604973081, 84.58442372801903275 ) ) ;
#105050=CARTESIAN_POINT ( 'NONE',  ( 16.51473224551083163, -9.474510206698727899, 45.83442372801900433 ) ) ;
#105051=CARTESIAN_POINT ( 'NONE',  ( 16.46253265017160672, -9.564922557960803928, 83.33224293864768129 ) ) ;
#105052=CARTESIAN_POINT ( 'NONE',  ( -16.52544592524342804, 4.483927247898546575, 76.04057627198102409 ) ) ;
#105053=CARTESIAN_POINT ( 'NONE',  ( -12.06949235617756955, 12.14591786802309770, 105.6239096053143669 ) ) ;
#105055=CARTESIAN_POINT ( 'NONE',  ( 0.05219959533909260263, 19.03943276465977164, 114.9989096053143669 ) ) ;
#105056=CARTESIAN_POINT ( 'NONE',  ( 9.474510206698971260, -16.51473224551069308, 102.9155762719810241 ) ) ;
#105057=CARTESIAN_POINT ( 'NONE',  ( 14.29746914071049879, -8.314922557960816363, 83.33224293864769550 ) ) ;
#105059=CARTESIAN_POINT ( 'NONE',  ( 16.46253265017146816, 9.564922557961045513, 26.66775706135234003 ) ) ;
#105060=CARTESIAN_POINT ( 'NONE',  ( 4.379528057220092307, 16.55341960407617563, 87.29275706135236135 ) ) ;
#105061=CARTESIAN_POINT ( 'NONE',  ( -13.89961937509977652, 13.97604488694528158, 85.62390960531433848 ) ) ;
#105062=CARTESIAN_POINT ( 'NONE',  ( -0.05219959533937732626, 21.53943276465977519, 52.50109039468567573 ) ) ;
#105063=CARTESIAN_POINT ( 'NONE',  ( -10.81492255796078084, -18.62759615963271287, 47.08224293864770260 ) ) ;
#105064=CARTESIAN_POINT ( 'NONE',  ( 0.05219959533937995610, -21.53943276465977519, 25.00109039468567218 ) ) ;
#105065=CARTESIAN_POINT ( 'NONE',  ( 21.53943276465977519, -0.05219959533907433946, 68.74890960531435269 ) ) ;
#105066=CARTESIAN_POINT ( 'NONE',  ( -16.52544592524342804, 4.483927247898546575, 96.04057627198102409 ) ) ;
#105067=CARTESIAN_POINT ( 'NONE',  ( -19.03943276465977164, -0.05219959533935918106, 53.75109039468566863 ) ) ;
#105068=CARTESIAN_POINT ( 'NONE',  ( -13.97604488694527625, -13.89961937509977652, 36.87390960531436690 ) ) ;
#105069=CARTESIAN_POINT ( 'NONE',  ( 16.46253265017160672, -9.564922557960803928, 88.33224293864769550 ) ) ;
#105070=CARTESIAN_POINT ( 'NONE',  ( -9.564922557960796823, -16.46253265017161027, 77.08224293864769550 ) ) ;
#105071=CARTESIAN_POINT ( 'NONE',  ( -16.53943276465976808, 0.05219959533911058130, 96.24890960531435269 ) ) ;
#105073=CARTESIAN_POINT ( 'NONE',  ( -8.314922557960811034, -14.29746914071050412, 27.08224293864769550 ) ) ;
#105074=CARTESIAN_POINT ( 'NONE',  ( 12.14591786802327356, -12.06949235617739191, 35.62609039468568994 ) ) ;
#105075=CARTESIAN_POINT ( 'NONE',  ( -18.62759615963255300, -10.81492255796106328, 109.1677570613523613 ) ) ;
#105076=CARTESIAN_POINT ( 'NONE',  ( 5.153800228976335163, 19.02544592524342804, 94.79057627198103830 ) ) ;
#105077=CARTESIAN_POINT ( 'NONE',  ( 10.81492255796106328, -18.62759615963255655, 30.41775706135234358 ) ) ;
#105078=CARTESIAN_POINT ( 'NONE',  ( 13.97604488694527802, 13.89961937509977652, 39.37390960531435269 ) ) ;
#105079=EDGE_CURVE ( 'NONE', #137808, #56021, #78077, .T. ) ;
#105080=CARTESIAN_POINT ( 'NONE',  ( 12.06949235617739724, 12.14591786802326823, 46.87609039468568994 ) ) ;
#105081=CARTESIAN_POINT ( 'NONE',  ( -0.05219959533936034679, 19.03943276465977164, 102.5010903946856757 ) ) ;
#105082=CARTESIAN_POINT ( 'NONE',  ( 9.474510206698971260, -16.51473224551069308, 32.91557627198102409 ) ) ;
#105083=CARTESIAN_POINT ( 'NONE',  ( 16.52544592524342804, -4.483927247898539470, 98.54057627198105251 ) ) ;
#105084=CARTESIAN_POINT ( 'NONE',  ( 21.55341960407610458, 5.719274019375980345, 103.9572429386476813 ) ) ;
#105085=CARTESIAN_POINT ( 'NONE',  ( -9.564922557961040184, 16.46253265017147172, 82.91775706135233293 ) ) ;
#105087=CARTESIAN_POINT ( 'NONE',  ( -19.03943276465977164, 0.05219959533909376836, 86.24890960531436690 ) ) ;
#105088=CARTESIAN_POINT ( 'NONE',  ( -15.72974639402176322, -15.80617190586768395, 39.37609039468567573 ) ) ;
#105090=CARTESIAN_POINT ( 'NONE',  ( 16.51473224551069308, 9.474510206698969483, 89.16557627198103830 ) ) ;
#105091=CARTESIAN_POINT ( 'NONE',  ( 17.26172910966780805, -6.454744622555828037, 113.3064690864922568 ) ) ;
#105092=CARTESIAN_POINT ( 'NONE',  ( -13.89961937509977652, 13.97604488694528158, 90.62390960531432427 ) ) ;
#105093=CARTESIAN_POINT ( 'NONE',  ( 10.72451020669871369, 18.67979575497193778, 37.08442372801901143 ) ) ;
#105094=CARTESIAN_POINT ( 'NONE',  ( -16.53943276465976808, 0.05219959533911058130, 91.24890960531436690 ) ) ;
#105095=CARTESIAN_POINT ( 'NONE',  ( -5.153800228976328057, -19.02544592524343514, 97.29057627198099567 ) ) ;
#105096=CARTESIAN_POINT ( 'NONE',  ( 16.51473224551083163, -9.474510206698727899, 20.83442372801899722 ) ) ;
#105097=CARTESIAN_POINT ( 'NONE',  ( 4.379528057220092307, 16.55341960407617563, 47.29275706135234003 ) ) ;
#105098=CARTESIAN_POINT ( 'NONE',  ( -21.52544592524334988, -5.823673210054445271, 63.95942372801901854 ) ) ;
#105099=CARTESIAN_POINT ( 'NONE',  ( 16.55341960407618274, -4.379528057220086978, 26.04275706135235779 ) ) ;
#105100=CARTESIAN_POINT ( 'NONE',  ( -0.05219959533909027116, -19.03943276465977164, 72.49890960531435269 ) ) ;
#105101=CARTESIAN_POINT ( 'NONE',  ( -19.02544592524334988, -5.153800228976617603, 98.95942372801900433 ) ) ;
#105102=CARTESIAN_POINT ( 'NONE',  ( 14.34966873604972726, -8.224510206698740333, 70.83442372801901854 ) ) ;
#105103=CARTESIAN_POINT ( 'NONE',  ( 21.55341960407619695, -5.719274019375665929, 111.0427570613523613 ) ) ;
#105104=CARTESIAN_POINT ( 'NONE',  ( -16.46253265017146816, -9.564922557961047289, 74.16775706135234714 ) ) ;
#105105=CARTESIAN_POINT ( 'NONE',  ( 16.51473224551069308, 9.474510206698969483, 59.16557627198102409 ) ) ;
#105106=CARTESIAN_POINT ( 'NONE',  ( -18.62759615963270932, 10.81492255796079327, 80.83224293864769550 ) ) ;
#105107=CARTESIAN_POINT ( 'NONE',  ( -4.379528057220328563, 16.55341960407611168, 80.20724293864769550 ) ) ;
#105108=CARTESIAN_POINT ( 'NONE',  ( 13.89961937509957401, 13.97604488694547697, 76.87609039468566152 ) ) ;
#105110=CARTESIAN_POINT ( 'NONE',  ( -5.049401038297874678, -19.05341960407617918, 59.79275706135231871 ) ) ;
#105111=CARTESIAN_POINT ( 'NONE',  ( 14.34966873604972726, -8.224510206698740333, 105.8344237280190328 ) ) ;
#105112=CARTESIAN_POINT ( 'NONE',  ( 14.29746914071049879, -8.314922557960816363, 73.33224293864769550 ) ) ;
#105113=CARTESIAN_POINT ( 'NONE',  ( 21.55341960407619695, -5.719274019375665929, 106.0427570613523471 ) ) ;
#105115=CARTESIAN_POINT ( 'NONE',  ( -5.823673210054116645, -21.52544592524344225, 102.2905762719810383 ) ) ;
#105116=CARTESIAN_POINT ( 'NONE',  ( -0.05219959533909027116, -19.03943276465977164, 97.49890960531436690 ) ) ;
#105117=CARTESIAN_POINT ( 'NONE',  ( -0.05219959533909027116, -19.03943276465977164, 67.49890960531436690 ) ) ;
#105118=CARTESIAN_POINT ( 'NONE',  ( -10.72451020669870658, -18.67979575497194134, 79.58442372801903275 ) ) ;
#105119=CARTESIAN_POINT ( 'NONE',  ( 5.153800228976335163, 19.02544592524342804, 59.79057627198100988 ) ) ;
#105120=CARTESIAN_POINT ( 'NONE',  ( -19.05341960407611168, -5.049401038298163336, 41.45724293864769550 ) ) ;
#105121=CARTESIAN_POINT ( 'NONE',  ( 15.80617190586746368, 15.72974639402197994, 24.37390960531435979 ) ) ;
#105123=CARTESIAN_POINT ( 'NONE',  ( 8.224510206698953496, -14.34966873604960469, 67.91557627198102409 ) ) ;
#105124=CARTESIAN_POINT ( 'NONE',  ( 19.02544592524343514, -5.153800228976328945, 43.54057627198103120 ) ) ;
#105125=CARTESIAN_POINT ( 'NONE',  ( -0.05219959533910754901, -16.53943276465976808, 97.49890960531436690 ) ) ;
#105126=CARTESIAN_POINT ( 'NONE',  ( -15.72974639402197994, 15.80617190586746368, 110.6239096053143669 ) ) ;
#105127=CARTESIAN_POINT ( 'NONE',  ( -15.80617190586768217, 15.72974639402176855, 43.12609039468568284 ) ) ;
#105128=CARTESIAN_POINT ( 'NONE',  ( 19.02544592524343514, -5.153800228976328945, 33.54057627198102409 ) ) ;
#105129=CARTESIAN_POINT ( 'NONE',  ( 14.29746914071037800, 8.314922557961029526, 61.66775706135235424 ) ) ;
#105130=CARTESIAN_POINT ( 'NONE',  ( 10.81492255796078972, 18.62759615963270932, 104.5822429386477097 ) ) ;
#105131=CARTESIAN_POINT ( 'NONE',  ( -15.72974639402197994, 15.80617190586746368, 95.62390960531436690 ) ) ;
#105132=CARTESIAN_POINT ( 'NONE',  ( 19.02544592524334988, 5.153800228976608722, 31.45942372801900433 ) ) ;
#105133=CARTESIAN_POINT ( 'NONE',  ( -16.46253265017160317, 9.564922557960807481, 55.83224293864769550 ) ) ;
#105134=CARTESIAN_POINT ( 'NONE',  ( -17.49999999999999645, 5.499999999999992895, 83.71769037696435589 ) ) ;
#105135=CARTESIAN_POINT ( 'NONE',  ( -5.823673210054431948, 21.52544592524334988, 62.70942372801902565 ) ) ;
#105136=CARTESIAN_POINT ( 'NONE',  ( 21.53943276465977519, -0.05219959533907433946, 58.74890960531436690 ) ) ;
#105137=CARTESIAN_POINT ( 'NONE',  ( -12.14591786802309592, -12.06949235617757132, 26.87390960531435979 ) ) ;
#105138=CARTESIAN_POINT ( 'NONE',  ( 10.81492255796106328, -18.62759615963255655, 80.41775706135234714 ) ) ;
#105139=CARTESIAN_POINT ( 'NONE',  ( -21.53943276465977519, -0.05219959533937600094, 103.7510903946857042 ) ) ;
#105140=CARTESIAN_POINT ( 'NONE',  ( -19.05341960407617563, 5.049401038297882671, 48.54275706135233293 ) ) ;
#105141=CARTESIAN_POINT ( 'NONE',  ( 4.483927247898790824, -16.52544592524335698, 100.2094237280190043 ) ) ;
#105142=CARTESIAN_POINT ( 'NONE',  ( 21.55341960407619695, -5.719274019375665929, 61.04275706135234714 ) ) ;
#105143=CARTESIAN_POINT ( 'NONE',  ( 5.153800228976335163, 19.02544592524342804, 59.79057627198100988 ) ) ;
#105144=CARTESIAN_POINT ( 'NONE',  ( -19.02544592524334988, -5.153800228976617603, 38.95942372801900433 ) ) ;
#105145=CARTESIAN_POINT ( 'NONE',  ( 21.53943276465977519, -0.05219959533907433946, 43.74890960531435979 ) ) ;
#105146=CARTESIAN_POINT ( 'NONE',  ( -15.80617190586768217, 15.72974639402176855, 38.12609039468567573 ) ) ;
#105147=CARTESIAN_POINT ( 'NONE',  ( 21.53943276465977519, -0.05219959533907433946, 88.74890960531436690 ) ) ;
#105148=CARTESIAN_POINT ( 'NONE',  ( -13.89961937509957401, -13.97604488694547875, 89.37609039468563310 ) ) ;
#105149=CARTESIAN_POINT ( 'NONE',  ( -4.483927247898782831, 16.52544592524335698, 57.70942372801901143 ) ) ;
#105151=CARTESIAN_POINT ( 'NONE',  ( -10.72451020669898014, 18.67979575497178502, 95.41557627198102409 ) ) ;
#105152=CARTESIAN_POINT ( 'NONE',  ( -12.06949235617739369, -12.14591786802326823, 79.37609039468567573 ) ) ;
#105153=CARTESIAN_POINT ( 'NONE',  ( 16.55341960407611168, 4.379528057220329451, 78.95724293864769550 ) ) ;
#105155=CARTESIAN_POINT ( 'NONE',  ( 19.03943276465977164, 0.05219959533936151252, 101.2510903946856757 ) ) ;
#105156=CARTESIAN_POINT ( 'NONE',  ( -10.72451020669898014, 18.67979575497178502, 30.41557627198101699 ) ) ;
#105158=CARTESIAN_POINT ( 'NONE',  ( 8.224510206698742110, 14.34966873604972548, 57.08442372801901854 ) ) ;
#105159=CARTESIAN_POINT ( 'NONE',  ( 5.823673210054125526, 21.52544592524343514, 109.7905762719810383 ) ) ;
#105160=CARTESIAN_POINT ( 'NONE',  ( 15.72974639402199770, -15.80617190586745480, 33.12390960531435979 ) ) ;
#105161=CARTESIAN_POINT ( 'NONE',  ( -0.05219959533934338120, 16.53943276465976808, 67.50109039468568994 ) ) ;
#105162=CARTESIAN_POINT ( 'NONE',  ( 19.05341960407611168, 5.049401038298154454, 78.95724293864769550 ) ) ;
#105163=CARTESIAN_POINT ( 'NONE',  ( 0.05219959533937995610, -21.53943276465977519, 55.00109039468568284 ) ) ;
#105164=CARTESIAN_POINT ( 'NONE',  ( 0.05219959533909260263, 19.03943276465977164, 24.99890960531435269 ) ) ;
#105165=CARTESIAN_POINT ( 'NONE',  ( 15.80617190586746368, 15.72974639402197994, 24.37390960531435979 ) ) ;
#105166=EDGE_LOOP ( 'NONE', ( #67500, #41945 ) ) ;
#105167=CARTESIAN_POINT ( 'NONE',  ( 9.564922557961047289, -16.46253265017146816, 45.41775706135232582 ) ) ;
#105168=CARTESIAN_POINT ( 'NONE',  ( 12.06949235617739724, 12.14591786802326823, 56.87609039468568994 ) ) ;
#105169=CARTESIAN_POINT ( 'NONE',  ( 13.89961937509977652, -13.97604488694527269, 113.1239096053143527 ) ) ;
#105170=CARTESIAN_POINT ( 'NONE',  ( 19.03943276465977164, -0.05219959533909143690, 78.74890960531436690 ) ) ;
#105171=CARTESIAN_POINT ( 'NONE',  ( -16.52544592524335698, -4.483927247898792601, 103.9594237280190185 ) ) ;
#105173=CARTESIAN_POINT ( 'NONE',  ( -14.29746914071049879, 8.314922557960819915, 100.8322429386477097 ) ) ;
#105174=CARTESIAN_POINT ( 'NONE',  ( -0.05219959533907301413, -21.53943276465977519, 32.49890960531435979 ) ) ;
#105175=CARTESIAN_POINT ( 'NONE',  ( -19.02544592524342804, 5.153800228976336051, 31.04057627198102409 ) ) ;
#105176=CARTESIAN_POINT ( 'NONE',  ( -16.55341960407617563, 4.379528057220093196, 68.54275706135234714 ) ) ;
#105177=CARTESIAN_POINT ( 'NONE',  ( -10.72451020669898014, 18.67979575497178502, 115.4155762719810241 ) ) ;
#105178=CARTESIAN_POINT ( 'NONE',  ( -0.05219959533936034679, 19.03943276465977164, 72.50109039468566152 ) ) ;
#105179=CARTESIAN_POINT ( 'NONE',  ( -5.049401038298153566, 19.05341960407611168, 40.20724293864768839 ) ) ;
#105180=CARTESIAN_POINT ( 'NONE',  ( 10.72451020669898902, -18.67979575497178502, 72.91557627198103830 ) ) ;
#105182=CARTESIAN_POINT ( 'NONE',  ( 10.81492255796106328, -18.62759615963255655, 85.41775706135236135 ) ) ;
#105183=CARTESIAN_POINT ( 'NONE',  ( -5.153800228976328057, -19.02544592524343514, 67.29057627198102409 ) ) ;
#105184=CARTESIAN_POINT ( 'NONE',  ( 12.06949235617739724, 12.14591786802326823, 51.87609039468568284 ) ) ;
#105185=CARTESIAN_POINT ( 'NONE',  ( 5.823673210054444382, -21.52544592524334988, 75.20942372801901854 ) ) ;
#105186=CARTESIAN_POINT ( 'NONE',  ( 5.049401038297881783, 19.05341960407617563, 42.29275706135234003 ) ) ;
#105187=CARTESIAN_POINT ( 'NONE',  ( 13.97604488694548053, -13.89961937509957401, 50.62609039468566152 ) ) ;
#105188=ORIENTED_EDGE ( 'NONE', *, *, #65989, .T. ) ;
#105189=CARTESIAN_POINT ( 'NONE',  ( 0.05219959533937995610, -21.53943276465977519, 50.00109039468568994 ) ) ;
#105190=CARTESIAN_POINT ( 'NONE',  ( -16.51473224551069308, -9.474510206698971260, 21.66557627198102765 ) ) ;
#105191=CARTESIAN_POINT ( 'NONE',  ( -5.153800228976607833, 19.02544592524334988, 47.70942372801900433 ) ) ;
#105192=CARTESIAN_POINT ( 'NONE',  ( 9.564922557960805705, 16.46253265017160317, 94.58224293864769550 ) ) ;
#105193=CARTESIAN_POINT ( 'NONE',  ( -5.153800228976328057, -19.02544592524343514, 77.29057627198099567 ) ) ;
#105194=CARTESIAN_POINT ( 'NONE',  ( 12.14591786802309770, 12.06949235617756955, 39.37390960531436690 ) ) ;
#105195=CARTESIAN_POINT ( 'NONE',  ( 18.67979575497178502, 10.72451020669898547, 39.16557627198102409 ) ) ;
#105197=CARTESIAN_POINT ( 'NONE',  ( 17.26058549869089731, 6.457015423128627418, 58.87745837476068544 ) ) ;
#105198=CARTESIAN_POINT ( 'NONE',  ( 10.72451020669871369, 18.67979575497193778, 102.0844237280190185 ) ) ;
#105200=CARTESIAN_POINT ( 'NONE',  ( -16.51473224551069308, -9.474510206698971260, 36.66557627198102409 ) ) ;
#105201=CARTESIAN_POINT ( 'NONE',  ( -9.474510206698964154, 16.51473224551069663, 115.4155762719810241 ) ) ;
#105204=CARTESIAN_POINT ( 'NONE',  ( -8.314922557961024197, 14.29746914071037800, 47.91775706135234714 ) ) ;
#105205=CARTESIAN_POINT ( 'NONE',  ( -0.05219959533907301413, -21.53943276465977519, 77.49890960531433848 ) ) ;
#105206=CARTESIAN_POINT ( 'NONE',  ( 12.14591786802309770, 12.06949235617756955, 34.37390960531435979 ) ) ;
#105207=CARTESIAN_POINT ( 'NONE',  ( -5.153800228976328057, -19.02544592524343514, 32.29057627198102409 ) ) ;
#105208=CARTESIAN_POINT ( 'NONE',  ( -5.153800228976328057, -19.02544592524343514, 112.2905762719810099 ) ) ;
#105209=CARTESIAN_POINT ( 'NONE',  ( 15.72974639402176855, 15.80617190586768217, 31.87609039468567929 ) ) ;
#105210=CARTESIAN_POINT ( 'NONE',  ( -13.89961937509957401, -13.97604488694547875, 34.37609039468566863 ) ) ;
#105211=CARTESIAN_POINT ( 'NONE',  ( -13.89961937509977652, 13.97604488694528158, 25.62390960531434558 ) ) ;
#105212=CARTESIAN_POINT ( 'NONE',  ( 0.05219959533937995610, -21.53943276465977519, 80.00109039468568994 ) ) ;
#105214=CARTESIAN_POINT ( 'NONE',  ( 16.53943276465976808, -0.05219959533910856209, 33.74890960531436690 ) ) ;
#105216=CARTESIAN_POINT ( 'NONE',  ( -10.81492255796078084, -18.62759615963271287, 32.08224293864769550 ) ) ;
#105217=CARTESIAN_POINT ( 'NONE',  ( -4.379528057220328563, 16.55341960407611168, 85.20724293864770971 ) ) ;
#105219=CARTESIAN_POINT ( 'NONE',  ( 13.89961937509977652, -13.97604488694527269, 73.12390960531436690 ) ) ;
#105220=CARTESIAN_POINT ( 'NONE',  ( -4.379528057220328563, 16.55341960407611168, 70.20724293864769550 ) ) ;
#105221=CARTESIAN_POINT ( 'NONE',  ( 19.05341960407617918, -5.049401038297876454, 111.0427570613523329 ) ) ;
#105222=CARTESIAN_POINT ( 'NONE',  ( 21.52544592524344225, -5.823673210054117533, 63.54057627198103830 ) ) ;
#105224=CARTESIAN_POINT ( 'NONE',  ( 5.153800228976335163, 19.02544592524342804, 29.79057627198102409 ) ) ;
#105225=CARTESIAN_POINT ( 'NONE',  ( -0.05219959533909027116, -19.03943276465977164, 82.49890960531436690 ) ) ;
#105226=CARTESIAN_POINT ( 'NONE',  ( -5.823673210054116645, -21.52544592524344225, 72.29057627198102409 ) ) ;
#105227=CARTESIAN_POINT ( 'NONE',  ( -4.483927247898782831, 16.52544592524335698, 102.7094237280190185 ) ) ;
#105228=CARTESIAN_POINT ( 'NONE',  ( -0.05219959533909027116, -19.03943276465977164, 82.49890960531436690 ) ) ;
#105229=CARTESIAN_POINT ( 'NONE',  ( 9.474510206698729675, 16.51473224551082808, 72.08442372801900433 ) ) ;
#105230=CARTESIAN_POINT ( 'NONE',  ( 0.05219959533937995610, -21.53943276465977519, 100.0010903946857042 ) ) ;
#105231=CARTESIAN_POINT ( 'NONE',  ( -0.05219959533907301413, -21.53943276465977519, 72.49890960531435269 ) ) ;
#105232=CARTESIAN_POINT ( 'NONE',  ( 5.153800228976335163, 19.02544592524342804, 114.7905762719810241 ) ) ;
#105233=CARTESIAN_POINT ( 'NONE',  ( 0.05219959533909260263, 19.03943276465977164, 44.99890960531435979 ) ) ;
#105234=CARTESIAN_POINT ( 'NONE',  ( -0.05219959533934338120, 16.53943276465976808, 112.5010903946857042 ) ) ;
#105235=CARTESIAN_POINT ( 'NONE',  ( -5.153800228976328057, -19.02544592524343514, 67.29057627198102409 ) ) ;
#105237=CARTESIAN_POINT ( 'NONE',  ( -15.72974639402176322, -15.80617190586768395, 104.3760903946856899 ) ) ;
#105238=CARTESIAN_POINT ( 'NONE',  ( -8.224510206698948167, 14.34966873604960824, 70.41557627198102409 ) ) ;
#105239=CARTESIAN_POINT ( 'NONE',  ( -15.72974639402197994, 15.80617190586746368, 110.6239096053143669 ) ) ;
#105240=CARTESIAN_POINT ( 'NONE',  ( -5.719274019375978568, 21.55341960407610458, 105.2072429386477097 ) ) ;
#105242=CARTESIAN_POINT ( 'NONE',  ( 15.72974639402199770, -15.80617190586745480, 58.12390960531435979 ) ) ;
#105244=CARTESIAN_POINT ( 'NONE',  ( 14.29746914071037800, 8.314922557961029526, 86.66775706135234714 ) ) ;
#105245=CARTESIAN_POINT ( 'NONE',  ( -4.483927247898539470, -16.52544592524342804, 107.2905762719810525 ) ) ;
#105246=CARTESIAN_POINT ( 'NONE',  ( 19.05341960407611168, 5.049401038298154454, 63.95724293864769550 ) ) ;
#105248=CARTESIAN_POINT ( 'NONE',  ( 16.55341960407618274, -4.379528057220086978, 106.0427570613523471 ) ) ;
#105249=CARTESIAN_POINT ( 'NONE',  ( -21.55341960407619339, 5.719274019375674811, 43.54275706135235424 ) ) ;
#105250=CARTESIAN_POINT ( 'NONE',  ( -19.03943276465977164, 0.05219959533909376836, 111.2489096053143669 ) ) ;
#105251=CARTESIAN_POINT ( 'NONE',  ( 5.719274019375673035, 21.55341960407619339, 87.29275706135236135 ) ) ;
#105252=CARTESIAN_POINT ( 'NONE',  ( 5.153800228976335163, 19.02544592524342804, 34.79057627198102409 ) ) ;
#105253=CARTESIAN_POINT ( 'NONE',  ( -9.474510206698964154, 16.51473224551069663, 35.41557627198102409 ) ) ;
#105255=CARTESIAN_POINT ( 'NONE',  ( -21.52544592524334988, -5.823673210054445271, 68.95942372801901854 ) ) ;
#105256=CARTESIAN_POINT ( 'NONE',  ( -5.049401038298153566, 19.05341960407611168, 105.2072429386476671 ) ) ;
#105257=CARTESIAN_POINT ( 'NONE',  ( 19.02544592524334988, 5.153800228976608722, 81.45942372801897591 ) ) ;
#105258=CARTESIAN_POINT ( 'NONE',  ( -21.52544592524334988, -5.823673210054445271, 43.95942372801902565 ) ) ;
#105259=CARTESIAN_POINT ( 'NONE',  ( 14.29746914071037800, 8.314922557961029526, 21.66775706135235069 ) ) ;
#105260=CARTESIAN_POINT ( 'NONE',  ( 19.02544592524334988, 5.153800228976608722, 71.45942372801900433 ) ) ;
#105261=CARTESIAN_POINT ( 'NONE',  ( -19.05341960407611168, -5.049401038298163336, 51.45724293864770260 ) ) ;
#105262=CARTESIAN_POINT ( 'NONE',  ( 19.03943276465977164, 0.05219959533936151252, 81.25109039468567573 ) ) ;
#105263=CARTESIAN_POINT ( 'NONE',  ( -16.53943276465976808, 0.05219959533911058130, 31.24890960531435979 ) ) ;
#105264=CARTESIAN_POINT ( 'NONE',  ( 19.05341960407617918, -5.049401038297876454, 86.04275706135233293 ) ) ;
#105265=CARTESIAN_POINT ( 'NONE',  ( 12.06949235617757843, -12.14591786802309237, 33.12390960531435979 ) ) ;
#105266=CARTESIAN_POINT ( 'NONE',  ( -16.46253265017146816, -9.564922557961047289, 64.16775706135233293 ) ) ;
#105267=CARTESIAN_POINT ( 'NONE',  ( -12.06949235617739369, -12.14591786802326823, 49.37609039468569705 ) ) ;
#105268=CARTESIAN_POINT ( 'NONE',  ( 9.474510206698729675, 16.51473224551082808, 22.08442372801899722 ) ) ;
#105269=CARTESIAN_POINT ( 'NONE',  ( 19.03943276465977164, -0.05219959533909143690, 43.74890960531435979 ) ) ;
#105270=CARTESIAN_POINT ( 'NONE',  ( -17.44279575226823908, -5.990770900252488040, 64.16442432485685288 ) ) ;
#105271=CARTESIAN_POINT ( 'NONE',  ( -12.06949235617739369, -12.14591786802326823, 44.37609039468567573 ) ) ;
#105274=CARTESIAN_POINT ( 'NONE',  ( -19.02544592524342804, 5.153800228976336051, 91.04057627198100988 ) ) ;
#105276=CARTESIAN_POINT ( 'NONE',  ( 13.89961937509957401, 13.97604488694547697, 86.87609039468567573 ) ) ;
#105277=CARTESIAN_POINT ( 'NONE',  ( 13.89961937509977652, -13.97604488694527269, 113.1239096053143527 ) ) ;
#105278=CARTESIAN_POINT ( 'NONE',  ( 10.72451020669871369, 18.67979575497193778, 107.0844237280190043 ) ) ;
#105279=CARTESIAN_POINT ( 'NONE',  ( 16.51473224551083163, -9.474510206698727899, 100.8344237280190043 ) ) ;
#105280=CARTESIAN_POINT ( 'NONE',  ( -19.03943276465977164, 0.05219959533909376836, 21.24890960531436335 ) ) ;
#105281=CARTESIAN_POINT ( 'NONE',  ( 9.474510206698971260, -16.51473224551069308, 42.91557627198103120 ) ) ;
#105282=CARTESIAN_POINT ( 'NONE',  ( 18.67979575497178502, 10.72451020669898547, 64.16557627198102409 ) ) ;
#105283=CARTESIAN_POINT ( 'NONE',  ( 13.97604488694527802, 13.89961937509977652, 29.37390960531435979 ) ) ;
#105285=CARTESIAN_POINT ( 'NONE',  ( 9.474510206698729675, 16.51473224551082808, 72.08442372801900433 ) ) ;
#105286=CARTESIAN_POINT ( 'NONE',  ( 12.14591786802309770, 12.06949235617756955, 54.37390960531435979 ) ) ;
#105287=CARTESIAN_POINT ( 'NONE',  ( 5.823673210054125526, 21.52544592524343514, 39.79057627198103830 ) ) ;
#105288=CARTESIAN_POINT ( 'NONE',  ( -21.53943276465977519, -0.05219959533937600094, 98.75109039468568994 ) ) ;
#105289=CARTESIAN_POINT ( 'NONE',  ( -5.823673210054116645, -21.52544592524344225, 87.29057627198103830 ) ) ;
#105290=CARTESIAN_POINT ( 'NONE',  ( 21.53943276465977519, 0.05219959533937863772, 61.25109039468567573 ) ) ;
#105291=CARTESIAN_POINT ( 'NONE',  ( -10.81492255796105439, 18.62759615963255655, 62.91775706135236135 ) ) ;
#105292=CARTESIAN_POINT ( 'NONE',  ( 9.474510206698971260, -16.51473224551069308, 97.91557627198102409 ) ) ;
#105293=CARTESIAN_POINT ( 'NONE',  ( -16.55341960407617563, 4.379528057220093196, 88.54275706135236135 ) ) ;
#105294=CARTESIAN_POINT ( 'NONE',  ( -21.53943276465977519, -0.05219959533937600094, 68.75109039468568994 ) ) ;
#105295=CARTESIAN_POINT ( 'NONE',  ( -19.03943276465977164, 0.05219959533909376836, 21.24890960531436335 ) ) ;
#105296=CARTESIAN_POINT ( 'NONE',  ( -8.314922557960811034, -14.29746914071050412, 62.08224293864769550 ) ) ;
#105297=CARTESIAN_POINT ( 'NONE',  ( -12.14591786802309592, -12.06949235617757132, 31.87390960531435979 ) ) ;
#105298=CARTESIAN_POINT ( 'NONE',  ( -10.72451020669898014, 18.67979575497178502, 45.41557627198103830 ) ) ;
#105300=CARTESIAN_POINT ( 'NONE',  ( 16.51473224551069308, 9.474510206698969483, 49.16557627198102409 ) ) ;
#105301=CARTESIAN_POINT ( 'NONE',  ( 0.05219959533907565091, 21.53943276465977519, 54.99890960531435269 ) ) ;
#105302=CARTESIAN_POINT ( 'NONE',  ( 13.97604488694548053, -13.89961937509957401, 45.62609039468566863 ) ) ;
#105303=CARTESIAN_POINT ( 'NONE',  ( -16.19135201231369336, -7.376712067591814304, 40.18680854052033169 ) ) ;
#105304=CARTESIAN_POINT ( 'NONE',  ( 14.34966873604960469, 8.224510206698951720, 44.16557627198103120 ) ) ;
#105305=CARTESIAN_POINT ( 'NONE',  ( -5.823673210054116645, -21.52544592524344225, 27.29057627198103120 ) ) ;
#105307=ORIENTED_EDGE ( 'NONE', *, *, #20087, .F. ) ;
#105309=CARTESIAN_POINT ( 'NONE',  ( 16.55341960407618274, -4.379528057220086978, 76.04275706135237556 ) ) ;
#105311=CARTESIAN_POINT ( 'NONE',  ( 5.049401038297881783, 19.05341960407617563, 77.29275706135231871 ) ) ;
#105312=CARTESIAN_POINT ( 'NONE',  ( -4.483927247898539470, -16.52544592524342804, 37.29057627198102409 ) ) ;
#105314=CARTESIAN_POINT ( 'NONE',  ( -16.52544592524342804, 4.483927247898546575, 31.04057627198102409 ) ) ;
#105315=CARTESIAN_POINT ( 'NONE',  ( 5.049401038298161559, -19.05341960407611168, 57.70724293864769550 ) ) ;
#105316=CARTESIAN_POINT ( 'NONE',  ( -19.05341960407611168, -5.049401038298163336, 71.45724293864766707 ) ) ;
#105317=CARTESIAN_POINT ( 'NONE',  ( 16.51473224551069308, 9.474510206698969483, 39.16557627198103120 ) ) ;
#105318=CARTESIAN_POINT ( 'NONE',  ( -5.823673210054431948, 21.52544592524334988, 52.70942372801902565 ) ) ;
#105319=CARTESIAN_POINT ( 'NONE',  ( 16.46253265017160672, -9.564922557960803928, 53.33224293864768839 ) ) ;
#105321=CARTESIAN_POINT ( 'NONE',  ( 19.02544592524343514, -5.153800228976328945, 63.54057627198103830 ) ) ;
#105322=CARTESIAN_POINT ( 'NONE',  ( -10.81492255796078084, -18.62759615963271287, 42.08224293864769550 ) ) ;
#105323=CARTESIAN_POINT ( 'NONE',  ( -0.05219959533909027116, -19.03943276465977164, 42.49890960531435269 ) ) ;
#105324=CARTESIAN_POINT ( 'NONE',  ( 21.52544592524344225, -5.823673210054117533, 43.54057627198103830 ) ) ;
#105325=CARTESIAN_POINT ( 'NONE',  ( 12.14591786802327356, -12.06949235617739191, 90.62609039468567573 ) ) ;
#105326=CARTESIAN_POINT ( 'NONE',  ( 0.05219959533936267826, -19.03943276465977164, 20.00109039468567218 ) ) ;
#105327=CARTESIAN_POINT ( 'NONE',  ( 16.52544592524335698, 4.483927247898782831, 71.45942372801901854 ) ) ;
#105328=CARTESIAN_POINT ( 'NONE',  ( 9.474510206698971260, -16.51473224551069308, 102.9155762719810241 ) ) ;
#105329=CARTESIAN_POINT ( 'NONE',  ( 4.483927247898790824, -16.52544592524335698, 50.20942372801901854 ) ) ;
#105330=CARTESIAN_POINT ( 'NONE',  ( 16.52544592524335698, 4.483927247898782831, 46.45942372801901854 ) ) ;
#105331=CARTESIAN_POINT ( 'NONE',  ( -9.474510206698964154, 16.51473224551069663, 105.4155762719810383 ) ) ;
#105332=CARTESIAN_POINT ( 'NONE',  ( -12.14591786802326823, 12.06949235617739902, 28.12609039468568284 ) ) ;
#105333=CARTESIAN_POINT ( 'NONE',  ( -0.05219959533909027116, -19.03943276465977164, 37.49890960531436690 ) ) ;
#105334=CARTESIAN_POINT ( 'NONE',  ( -5.823673210054431948, 21.52544592524334988, 32.70942372801900433 ) ) ;
#105335=CARTESIAN_POINT ( 'NONE',  ( 16.46253265017146816, 9.564922557961045513, 111.6677570613523329 ) ) ;
#105336=CARTESIAN_POINT ( 'NONE',  ( 16.55341960407618274, -4.379528057220086978, 101.0427570613523756 ) ) ;
#105338=CARTESIAN_POINT ( 'NONE',  ( -15.80617190586768217, 15.72974639402176855, 103.1260903946856757 ) ) ;
#105339=CARTESIAN_POINT ( 'NONE',  ( 16.46253265017146816, 9.564922557961045513, 91.66775706135234714 ) ) ;
#105340=CARTESIAN_POINT ( 'NONE',  ( 16.53943276465976808, -0.05219959533910856209, 58.74890960531436690 ) ) ;
#105341=CARTESIAN_POINT ( 'NONE',  ( 5.153800228976335163, 19.02544592524342804, 24.79057627198102765 ) ) ;
#105342=CARTESIAN_POINT ( 'NONE',  ( -9.564922557961040184, 16.46253265017147172, 57.91775706135233293 ) ) ;
#105344=CARTESIAN_POINT ( 'NONE',  ( 0.05219959533937995610, -21.53943276465977519, 55.00109039468568284 ) ) ;
#105345=CARTESIAN_POINT ( 'NONE',  ( -8.314922557961024197, 14.29746914071037800, 22.91775706135235069 ) ) ;
#105346=CARTESIAN_POINT ( 'NONE',  ( -17.97182807773875624, 5.499999999999873879, 63.53038844047289047 ) ) ;
#105347=CARTESIAN_POINT ( 'NONE',  ( -9.474510206698964154, 16.51473224551069663, 105.4155762719810383 ) ) ;
#105348=CARTESIAN_POINT ( 'NONE',  ( 15.72974639402199770, -15.80617190586745480, 68.12390960531436690 ) ) ;
#105349=CARTESIAN_POINT ( 'NONE',  ( -8.224510206698735004, -14.34966873604973081, 19.58442372801901143 ) ) ;
#105350=CARTESIAN_POINT ( 'NONE',  ( 13.89961937509977652, -13.97604488694527269, 108.1239096053143669 ) ) ;
#105352=CARTESIAN_POINT ( 'NONE',  ( -5.049401038298153566, 19.05341960407611168, 30.20724293864768839 ) ) ;
#105353=CARTESIAN_POINT ( 'NONE',  ( 21.55341960407619695, -5.719274019375665929, 96.04275706135236135 ) ) ;
#105354=CARTESIAN_POINT ( 'NONE',  ( 19.03943276465977164, -0.05219959533909143690, 43.74890960531435979 ) ) ;
#105356=CARTESIAN_POINT ( 'NONE',  ( 10.81492255796106328, -18.62759615963255655, 45.41775706135234003 ) ) ;
#105357=CARTESIAN_POINT ( 'NONE',  ( 18.62759615963255655, 10.81492255796105972, 91.66775706135234714 ) ) ;
#105358=CARTESIAN_POINT ( 'NONE',  ( 16.53943276465976808, 0.05219959533934440121, 106.2510903946856757 ) ) ;
#105359=CARTESIAN_POINT ( 'NONE',  ( 5.153800228976335163, 19.02544592524342804, 79.79057627198102409 ) ) ;
#105360=CARTESIAN_POINT ( 'NONE',  ( 5.823673210054444382, -21.52544592524334988, 45.20942372801901854 ) ) ;
#105361=CARTESIAN_POINT ( 'NONE',  ( 5.823673210054444382, -21.52544592524334988, 45.20942372801901854 ) ) ;
#105362=CARTESIAN_POINT ( 'NONE',  ( 19.05341960407617918, -5.049401038297876454, 66.04275706135233293 ) ) ;
#105363=CARTESIAN_POINT ( 'NONE',  ( 19.02544592524343514, -5.153800228976328945, 98.54057627198100988 ) ) ;
#105364=CARTESIAN_POINT ( 'NONE',  ( -16.52544592524342804, 4.483927247898546575, 106.0405762719810525 ) ) ;
#105365=CARTESIAN_POINT ( 'NONE',  ( 18.62759615963271287, -10.81492255796078972, 98.33224293864769550 ) ) ;
#105366=CARTESIAN_POINT ( 'NONE',  ( -14.29746914071049879, 8.314922557960819915, 60.83224293864769550 ) ) ;
#105367=CARTESIAN_POINT ( 'NONE',  ( 13.89961937509957401, 13.97604488694547697, 26.87609039468566507 ) ) ;
#105368=CARTESIAN_POINT ( 'NONE',  ( -0.05219959533910754901, -16.53943276465976808, 97.49890960531436690 ) ) ;
#105369=CARTESIAN_POINT ( 'NONE',  ( 9.474510206698971260, -16.51473224551069308, 32.91557627198102409 ) ) ;
#105370=CARTESIAN_POINT ( 'NONE',  ( 13.97604488694548053, -13.89961937509957401, 90.62609039468567573 ) ) ;
#105371=CARTESIAN_POINT ( 'NONE',  ( -0.05219959533910754901, -16.53943276465976808, 42.49890960531435979 ) ) ;
#105372=CARTESIAN_POINT ( 'NONE',  ( 10.81492255796106328, -18.62759615963255655, 95.41775706135234714 ) ) ;
#105373=CARTESIAN_POINT ( 'NONE',  ( -16.51473224551069308, -9.474510206698971260, 101.6655762719810241 ) ) ;
#105374=CARTESIAN_POINT ( 'NONE',  ( -19.03943276465977164, -0.05219959533935918106, 73.75109039468566152 ) ) ;
#105375=CARTESIAN_POINT ( 'NONE',  ( 10.72451020669898902, -18.67979575497178502, 77.91557627198102409 ) ) ;
#105376=CARTESIAN_POINT ( 'NONE',  ( -15.72974639402176322, -15.80617190586768395, 29.37609039468568284 ) ) ;
#105377=CARTESIAN_POINT ( 'NONE',  ( 0.05219959533934541429, -16.53943276465976808, 35.00109039468568284 ) ) ;
#105378=CARTESIAN_POINT ( 'NONE',  ( 12.06949235617739724, 12.14591786802326823, 96.87609039468568994 ) ) ;
#105379=DIRECTION ( 'NONE',  ( -0.000000000000000000, 1.000000000000000000, 0.000000000000000000 ) ) ;
#105380=CARTESIAN_POINT ( 'NONE',  ( -10.81492255796105439, 18.62759615963255655, 37.91775706135235424 ) ) ;
#105381=CARTESIAN_POINT ( 'NONE',  ( 5.049401038298161559, -19.05341960407611168, 22.70724293864769194 ) ) ;
#105383=CARTESIAN_POINT ( 'NONE',  ( -0.05219959533934338120, 16.53943276465976808, 47.50109039468568994 ) ) ;
#105384=CARTESIAN_POINT ( 'NONE',  ( 16.55341960407611168, 4.379528057220329451, 78.95724293864769550 ) ) ;
#105385=CARTESIAN_POINT ( 'NONE',  ( 10.72451020669898902, -18.67979575497178502, 72.91557627198103830 ) ) ;
#105386=CARTESIAN_POINT ( 'NONE',  ( -0.05219959533910754901, -16.53943276465976808, 27.49890960531435269 ) ) ;
#105387=CARTESIAN_POINT ( 'NONE',  ( 14.29746914071037800, 8.314922557961029526, 51.66775706135234714 ) ) ;
#105388=CARTESIAN_POINT ( 'NONE',  ( -16.51473224551069308, -9.474510206698971260, 41.66557627198103120 ) ) ;
#105389=B_SPLINE_CURVE_WITH_KNOTS ( 'NONE', 3,
 ( #122418, #16252, #2063, #186106, #138582, #185096 ),
 .UNSPECIFIED., .F., .F.,
 ( 4, 2, 4 ),
 ( 3.469446951953614189E-18, 0.0003837532665554453833, 0.0007675065331108872971 ),
 .UNSPECIFIED. ) ;
#105390=CARTESIAN_POINT ( 'NONE',  ( 16.55341960407618274, -4.379528057220086978, 91.04275706135236135 ) ) ;
#105391=CARTESIAN_POINT ( 'NONE',  ( 16.51473224551083163, -9.474510206698727899, 85.83442372801900433 ) ) ;
#105392=CARTESIAN_POINT ( 'NONE',  ( -10.72451020669898014, 18.67979575497178502, 70.41557627198102409 ) ) ;
#105393=CARTESIAN_POINT ( 'NONE',  ( -14.34966873604972548, 8.224510206698743886, 113.3344237280190328 ) ) ;
#105394=ORIENTED_EDGE ( 'NONE', *, *, #20087, .T. ) ;
#105396=CARTESIAN_POINT ( 'NONE',  ( 5.719274019375991003, -21.55341960407610458, 67.70724293864769550 ) ) ;
#105398=CARTESIAN_POINT ( 'NONE',  ( -16.53943276465976808, -0.05219959533934237506, 98.75109039468568994 ) ) ;
#105400=CARTESIAN_POINT ( 'NONE',  ( -19.03943276465977164, 0.05219959533909376836, 111.2489096053143669 ) ) ;
#105401=CARTESIAN_POINT ( 'NONE',  ( -19.53037848336980886, 5.499999999999896971, 74.85532783611441232 ) ) ;
#105402=CARTESIAN_POINT ( 'NONE',  ( -21.52544592524343514, 5.823673210054127303, 71.04057627198103830 ) ) ;
#105403=VECTOR ( 'NONE', #159418, 1000.000000000000000 ) ;
#105404=CARTESIAN_POINT ( 'NONE',  ( -14.29746914071049879, 8.314922557960819915, 25.83224293864769194 ) ) ;
#105405=CARTESIAN_POINT ( 'NONE',  ( 8.314922557961029526, -14.29746914071037800, 25.41775706135235779 ) ) ;
#105406=CARTESIAN_POINT ( 'NONE',  ( -19.03943276465977164, 0.05219959533909376836, 21.24890960531436335 ) ) ;
#105407=CARTESIAN_POINT ( 'NONE',  ( -16.53943276465976808, -0.05219959533934237506, 28.75109039468567929 ) ) ;
#105409=CARTESIAN_POINT ( 'NONE',  ( 9.474510206698971260, -16.51473224551069308, 52.91557627198102409 ) ) ;
#105411=CARTESIAN_POINT ( 'NONE',  ( -0.05219959533909027116, -19.03943276465977164, 102.4989096053143669 ) ) ;
#105412=CARTESIAN_POINT ( 'NONE',  ( 4.483927247898790824, -16.52544592524335698, 90.20942372801903275 ) ) ;
#105413=CARTESIAN_POINT ( 'NONE',  ( 19.03943276465977164, 0.05219959533936151252, 91.25109039468566152 ) ) ;
#105414=CARTESIAN_POINT ( 'NONE',  ( 5.153800228976615827, -19.02544592524334988, 30.20942372801900433 ) ) ;
#105415=CARTESIAN_POINT ( 'NONE',  ( -0.05219959533907301413, -21.53943276465977519, 72.49890960531435269 ) ) ;
#105417=CARTESIAN_POINT ( 'NONE',  ( 12.06949235617739724, 12.14591786802326823, 106.8760903946856899 ) ) ;
#105418=CARTESIAN_POINT ( 'NONE',  ( 0.05219959533936267826, -19.03943276465977164, 95.00109039468567573 ) ) ;
#105419=CARTESIAN_POINT ( 'NONE',  ( -5.049401038298153566, 19.05341960407611168, 55.20724293864769550 ) ) ;
#105420=CARTESIAN_POINT ( 'NONE',  ( -13.97604488694527625, -13.89961937509977652, 86.87390960531436690 ) ) ;
#105421=CARTESIAN_POINT ( 'NONE',  ( -5.823673210054431948, 21.52544592524334988, 57.70942372801901143 ) ) ;
#105422=CARTESIAN_POINT ( 'NONE',  ( -13.89961937509977652, 13.97604488694528158, 60.62390960531436690 ) ) ;
#105423=CARTESIAN_POINT ( 'NONE',  ( -12.06949235617756955, 12.14591786802309770, 80.62390960531438111 ) ) ;
#105425=CARTESIAN_POINT ( 'NONE',  ( 16.52544592524342804, -4.483927247898539470, 78.54057627198103830 ) ) ;
#105426=CARTESIAN_POINT ( 'NONE',  ( -10.81492255796078084, -18.62759615963271287, 77.08224293864769550 ) ) ;
#105427=CARTESIAN_POINT ( 'NONE',  ( -19.05341960407617563, 5.049401038297882671, 88.54275706135230450 ) ) ;
#105429=CARTESIAN_POINT ( 'NONE',  ( 19.05341960407617918, -5.049401038297876454, 41.04275706135233293 ) ) ;
#105431=CARTESIAN_POINT ( 'NONE',  ( 19.02544592524343514, -5.153800228976328945, 83.54057627198100988 ) ) ;
#105432=CARTESIAN_POINT ( 'NONE',  ( 16.51473224551069308, 9.474510206698969483, 89.16557627198103830 ) ) ;
#105433=CARTESIAN_POINT ( 'NONE',  ( -8.314922557961024197, 14.29746914071037800, 62.91775706135236135 ) ) ;
#105435=CARTESIAN_POINT ( 'NONE',  ( -13.89961937509957401, -13.97604488694547875, 39.37609039468566152 ) ) ;
#105437=CARTESIAN_POINT ( 'NONE',  ( 9.564922557960805705, 16.46253265017160317, 114.5822429386476955 ) ) ;
#105438=CARTESIAN_POINT ( 'NONE',  ( 16.52544592524335698, 4.483927247898782831, 101.4594237280190185 ) ) ;
#105439=CARTESIAN_POINT ( 'NONE',  ( -17.49999999999999645, -5.499999999999992895, 89.20309617465829888 ) ) ;
#105440=CARTESIAN_POINT ( 'NONE',  ( 0.05219959533934541429, -16.53943276465976808, 75.00109039468568994 ) ) ;
#105441=CARTESIAN_POINT ( 'NONE',  ( 17.49999999999999645, 5.500000000000010658, 53.78230962303567964 ) ) ;
#105443=CARTESIAN_POINT ( 'NONE',  ( -8.314922557961024197, 14.29746914071037800, 57.91775706135234714 ) ) ;
#105445=CARTESIAN_POINT ( 'NONE',  ( 21.55341960407619695, -5.719274019375665929, 71.04275706135234714 ) ) ;
#105446=CARTESIAN_POINT ( 'NONE',  ( -9.564922557961040184, 16.46253265017147172, 72.91775706135233293 ) ) ;
#105447=CARTESIAN_POINT ( 'NONE',  ( -5.153800228976607833, 19.02544592524334988, 27.70942372801899722 ) ) ;
#105448=CARTESIAN_POINT ( 'NONE',  ( -5.153800228976328057, -19.02544592524343514, 57.29057627198103120 ) ) ;
#105449=CARTESIAN_POINT ( 'NONE',  ( 19.05341960407611168, 5.049401038298154454, 48.95724293864768129 ) ) ;
#105450=CARTESIAN_POINT ( 'NONE',  ( 16.18474525874326631, -7.379450460607309026, 22.26924095202841514 ) ) ;
#105451=CARTESIAN_POINT ( 'NONE',  ( -5.823673210054116645, -21.52544592524344225, 72.29057627198102409 ) ) ;
#105452=CARTESIAN_POINT ( 'NONE',  ( -0.05219959533907301413, -21.53943276465977519, 37.49890960531436690 ) ) ;
#105453=CARTESIAN_POINT ( 'NONE',  ( -19.05341960407611168, -5.049401038298163336, 21.45724293864768839 ) ) ;
#105454=CARTESIAN_POINT ( 'NONE',  ( -12.14591786802326823, 12.06949235617739902, 48.12609039468568284 ) ) ;
#105456=CARTESIAN_POINT ( 'NONE',  ( -5.823673210054431948, 21.52544592524334988, 27.70942372801901854 ) ) ;
#105457=CARTESIAN_POINT ( 'NONE',  ( -12.14591786802309592, -12.06949235617757132, 46.87390960531435979 ) ) ;
#105459=CARTESIAN_POINT ( 'NONE',  ( 13.97604488694548053, -13.89961937509957401, 100.6260903946856615 ) ) ;
#105460=CARTESIAN_POINT ( 'NONE',  ( -5.153800228976607833, 19.02544592524334988, 37.70942372801899722 ) ) ;
#105461=CARTESIAN_POINT ( 'NONE',  ( -0.05219959533910754901, -16.53943276465976808, 42.49890960531435979 ) ) ;
#105462=CARTESIAN_POINT ( 'NONE',  ( -10.72451020669898014, 18.67979575497178502, 115.4155762719810241 ) ) ;
#105464=CARTESIAN_POINT ( 'NONE',  ( -0.05219959533907301413, -21.53943276465977519, 72.49890960531435269 ) ) ;
#105465=CARTESIAN_POINT ( 'NONE',  ( 16.51473224551069308, 9.474510206698969483, 89.16557627198103830 ) ) ;
#105466=CARTESIAN_POINT ( 'NONE',  ( 12.14591786802309770, 12.06949235617756955, 64.37390960531435269 ) ) ;
#105467=CARTESIAN_POINT ( 'NONE',  ( -9.474510206698964154, 16.51473224551069663, 110.4155762719810383 ) ) ;
#105468=CARTESIAN_POINT ( 'NONE',  ( -17.58332526062529411, 7.635886036038502134, 80.92334959558466778 ) ) ;
#105469=CARTESIAN_POINT ( 'NONE',  ( -5.049401038297874678, -19.05341960407617918, 49.79275706135231871 ) ) ;
#105470=CARTESIAN_POINT ( 'NONE',  ( -21.53943276465977519, 0.05219959533907696930, 106.2489096053143811 ) ) ;
#105471=CARTESIAN_POINT ( 'NONE',  ( -13.97604488694527625, -13.89961937509977652, 46.87390960531435979 ) ) ;
#105472=CARTESIAN_POINT ( 'NONE',  ( -4.483927247898539470, -16.52544592524342804, 112.2905762719810241 ) ) ;
#105473=CARTESIAN_POINT ( 'NONE',  ( -21.55341960407619339, 5.719274019375674811, 48.54275706135234714 ) ) ;
#105475=CARTESIAN_POINT ( 'NONE',  ( 16.55341960407611168, 4.379528057220329451, 28.95724293864769905 ) ) ;
#105476=CARTESIAN_POINT ( 'NONE',  ( 5.153800228976335163, 19.02544592524342804, 44.79057627198103830 ) ) ;
#105477=CARTESIAN_POINT ( 'NONE',  ( 5.153800228976335163, 19.02544592524342804, 94.79057627198103830 ) ) ;
#105478=CARTESIAN_POINT ( 'NONE',  ( 18.67979575497178502, 10.72451020669898547, 79.16557627198103830 ) ) ;
#105480=CARTESIAN_POINT ( 'NONE',  ( -9.564922557960796823, -16.46253265017161027, 47.08224293864769550 ) ) ;
#105482=CARTESIAN_POINT ( 'NONE',  ( 15.72974639402199770, -15.80617190586745480, 58.12390960531435979 ) ) ;
#105483=CARTESIAN_POINT ( 'NONE',  ( -18.62759615963255300, -10.81492255796106328, 84.16775706135234714 ) ) ;
#105485=CARTESIAN_POINT ( 'NONE',  ( -0.05219959533934338120, 16.53943276465976808, 77.50109039468567573 ) ) ;
#105486=CARTESIAN_POINT ( 'NONE',  ( -16.52544592524342804, 4.483927247898546575, 66.04057627198103830 ) ) ;
#105487=CARTESIAN_POINT ( 'NONE',  ( 0.05219959533909260263, 19.03943276465977164, 69.99890960531435269 ) ) ;
#105489=CARTESIAN_POINT ( 'NONE',  ( 5.049401038297881783, 19.05341960407617563, 22.29275706135233648 ) ) ;
#105490=CARTESIAN_POINT ( 'NONE',  ( 16.55341960407618274, -4.379528057220086978, 91.04275706135236135 ) ) ;
#105491=CARTESIAN_POINT ( 'NONE',  ( 5.823673210054444382, -21.52544592524334988, 110.2094237280190185 ) ) ;
#105492=CARTESIAN_POINT ( 'NONE',  ( 19.03943276465977164, -0.05219959533909143690, 73.74890960531435269 ) ) ;
#105493=CARTESIAN_POINT ( 'NONE',  ( 5.719274019375991003, -21.55341960407610458, 47.70724293864770260 ) ) ;
#105494=CARTESIAN_POINT ( 'NONE',  ( 12.06949235617739724, 12.14591786802326823, 26.87609039468567218 ) ) ;
#105495=CARTESIAN_POINT ( 'NONE',  ( -5.719274019375665041, -21.55341960407619695, 94.79275706135234714 ) ) ;
#105496=CARTESIAN_POINT ( 'NONE',  ( -16.53943276465976808, -0.05219959533934237506, 68.75109039468568994 ) ) ;
#105497=CARTESIAN_POINT ( 'NONE',  ( 5.823673210054125526, 21.52544592524343514, 109.7905762719810383 ) ) ;
#105498=CARTESIAN_POINT ( 'NONE',  ( 16.53943276465976808, 0.05219959533934440121, 21.25109039468567218 ) ) ;
#105499=CARTESIAN_POINT ( 'NONE',  ( -13.89961937509977652, 13.97604488694528158, 85.62390960531433848 ) ) ;
#105500=CARTESIAN_POINT ( 'NONE',  ( -0.05219959533934338120, 16.53943276465976808, 32.50109039468568284 ) ) ;
#105501=CARTESIAN_POINT ( 'NONE',  ( -5.049401038298153566, 19.05341960407611168, 50.20724293864770260 ) ) ;
#105502=VECTOR ( 'NONE', #19707, 1000.000000000000000 ) ;
#105503=CARTESIAN_POINT ( 'NONE',  ( -16.53943276465976808, -0.05219959533934237506, 33.75109039468568284 ) ) ;
#105504=CARTESIAN_POINT ( 'NONE',  ( 8.224510206698953496, -14.34966873604960469, 72.91557627198103830 ) ) ;
#105505=CARTESIAN_POINT ( 'NONE',  ( -12.06949235617739369, -12.14591786802326823, 84.37609039468570415 ) ) ;
#105506=CARTESIAN_POINT ( 'NONE',  ( -15.80617190586768217, 15.72974639402176855, 38.12609039468567573 ) ) ;
#105507=CARTESIAN_POINT ( 'NONE',  ( 9.474510206698971260, -16.51473224551069308, 62.91557627198102409 ) ) ;
#105508=CARTESIAN_POINT ( 'NONE',  ( 5.049401038298161559, -19.05341960407611168, 87.70724293864769550 ) ) ;
#105509=ADVANCED_FACE ( 'NONE', ( #58037 ), #101524, .T. ) ;
#105510=CARTESIAN_POINT ( 'NONE',  ( -8.224510206698735004, -14.34966873604973081, 84.58442372801903275 ) ) ;
#105512=VERTEX_POINT ( 'NONE', #87368 ) ;
#105514=CARTESIAN_POINT ( 'NONE',  ( -16.46253265017146816, -9.564922557961047289, 34.16775706135233293 ) ) ;
#105515=CARTESIAN_POINT ( 'NONE',  ( -5.049401038298153566, 19.05341960407611168, 100.2072429386476955 ) ) ;
#105516=CARTESIAN_POINT ( 'NONE',  ( -13.89961937509977652, 13.97604488694528158, 50.62390960531435979 ) ) ;
#105518=CARTESIAN_POINT ( 'NONE',  ( 12.06949235617739724, 12.14591786802326823, 36.87609039468568994 ) ) ;
#105519=CARTESIAN_POINT ( 'NONE',  ( -16.51473224551082808, 9.474510206698731452, 58.33442372801900433 ) ) ;
#105520=CARTESIAN_POINT ( 'NONE',  ( 16.53943276465976808, 0.05219959533934440121, 56.25109039468568284 ) ) ;
#105521=CARTESIAN_POINT ( 'NONE',  ( -19.03943276465977164, 0.05219959533909376836, 111.2489096053143669 ) ) ;
#105522=CARTESIAN_POINT ( 'NONE',  ( 13.89961937509977652, -13.97604488694527269, 83.12390960531436690 ) ) ;
#105523=CARTESIAN_POINT ( 'NONE',  ( -21.55341960407610458, -5.719274019375992779, 101.4572429386476955 ) ) ;
#105524=CARTESIAN_POINT ( 'NONE',  ( 5.153800228976615827, -19.02544592524334988, 60.20942372801899012 ) ) ;
#105525=CARTESIAN_POINT ( 'NONE',  ( 19.03943276465977164, -0.05219959533909143690, 93.74890960531435269 ) ) ;
#105527=CARTESIAN_POINT ( 'NONE',  ( -9.564922557960796823, -16.46253265017161027, 77.08224293864769550 ) ) ;
#105528=CARTESIAN_POINT ( 'NONE',  ( 12.06949235617757843, -12.14591786802309237, 38.12390960531436690 ) ) ;
#105529=CARTESIAN_POINT ( 'NONE',  ( 19.02544592524343514, -5.153800228976328945, 23.54057627198102054 ) ) ;
#105530=CARTESIAN_POINT ( 'NONE',  ( 19.03943276465977164, 0.05219959533936151252, 41.25109039468566152 ) ) ;
#105531=CARTESIAN_POINT ( 'NONE',  ( 16.52544592524342804, -4.483927247898539470, 68.54057627198103830 ) ) ;
#105532=CARTESIAN_POINT ( 'NONE',  ( -18.62759615963255300, -10.81492255796106328, 104.1677570613523471 ) ) ;
#105533=CARTESIAN_POINT ( 'NONE',  ( -19.05341960407611168, -5.049401038298163336, 41.45724293864769550 ) ) ;
#105534=CARTESIAN_POINT ( 'NONE',  ( 16.55341960407611168, 4.379528057220329451, 33.95724293864769550 ) ) ;
#105535=CARTESIAN_POINT ( 'NONE',  ( -15.72974639402176322, -15.80617190586768395, 104.3760903946856899 ) ) ;
#105536=CARTESIAN_POINT ( 'NONE',  ( -9.474510206698964154, 16.51473224551069663, 90.41557627198103830 ) ) ;
#105537=CARTESIAN_POINT ( 'NONE',  ( 19.05341960407611168, 5.049401038298154454, 88.95724293864769550 ) ) ;
#105538=CARTESIAN_POINT ( 'NONE',  ( -9.474510206698964154, 16.51473224551069663, 30.41557627198102054 ) ) ;
#105539=CARTESIAN_POINT ( 'NONE',  ( 14.34966873604960469, 8.224510206698951720, 109.1655762719810383 ) ) ;
#105540=CARTESIAN_POINT ( 'NONE',  ( 8.314922557960818139, 14.29746914071049879, 69.58224293864769550 ) ) ;
#105541=CARTESIAN_POINT ( 'NONE',  ( 5.823673210054125526, 21.52544592524343514, 79.79057627198102409 ) ) ;
#105542=CARTESIAN_POINT ( 'NONE',  ( -19.03943276465977164, 0.05219959533909376836, 86.24890960531436690 ) ) ;
#105543=CARTESIAN_POINT ( 'NONE',  ( -5.823673210054116645, -21.52544592524344225, 102.2905762719810383 ) ) ;
#105544=CARTESIAN_POINT ( 'NONE',  ( -0.05219959533909027116, -19.03943276465977164, 87.49890960531436690 ) ) ;
#105545=CARTESIAN_POINT ( 'NONE',  ( 0.05219959533936267826, -19.03943276465977164, 65.00109039468567573 ) ) ;
#105546=CARTESIAN_POINT ( 'NONE',  ( -4.379528057220328563, 16.55341960407611168, 95.20724293864769550 ) ) ;
#105548=CARTESIAN_POINT ( 'NONE',  ( 9.474510206698971260, -16.51473224551069308, 72.91557627198102409 ) ) ;
#105549=CARTESIAN_POINT ( 'NONE',  ( -21.52544592524343514, 5.823673210054127303, 61.04057627198103120 ) ) ;
#105551=CARTESIAN_POINT ( 'NONE',  ( -8.224510206698735004, -14.34966873604973081, 109.5844237280190328 ) ) ;
#105552=CARTESIAN_POINT ( 'NONE',  ( -12.06949235617739369, -12.14591786802326823, 24.37609039468567573 ) ) ;
#105553=CARTESIAN_POINT ( 'NONE',  ( 16.52544592524342804, -4.483927247898539470, 93.54057627198103830 ) ) ;
#105554=CARTESIAN_POINT ( 'NONE',  ( -17.40861289039001392, -6.110651285853318626, 96.37232470827430575 ) ) ;
#105555=CARTESIAN_POINT ( 'NONE',  ( -16.51473224551069308, -9.474510206698971260, 86.66557627198102409 ) ) ;
#105556=CARTESIAN_POINT ( 'NONE',  ( -13.89961937509977652, 13.97604488694528158, 45.62390960531433848 ) ) ;
#105557=CARTESIAN_POINT ( 'NONE',  ( 4.483927247898545687, 16.52544592524342804, 79.79057627198102409 ) ) ;
#105558=CARTESIAN_POINT ( 'NONE',  ( -13.97604488694527625, -13.89961937509977652, 111.8739096053143243 ) ) ;
#105559=CARTESIAN_POINT ( 'NONE',  ( -19.03943276465977164, -0.05219959533935918106, 103.7510903946856757 ) ) ;
#105560=CARTESIAN_POINT ( 'NONE',  ( -10.72451020669870658, -18.67979575497194134, 64.58442372801900433 ) ) ;
#105561=CARTESIAN_POINT ( 'NONE',  ( 16.46253265017160672, -9.564922557960803928, 93.33224293864769550 ) ) ;
#105562=CARTESIAN_POINT ( 'NONE',  ( -0.05219959533907301413, -21.53943276465977519, 82.49890960531436690 ) ) ;
#105563=CARTESIAN_POINT ( 'NONE',  ( 16.55341960407618274, -4.379528057220086978, 76.04275706135237556 ) ) ;
#105564=CARTESIAN_POINT ( 'NONE',  ( -19.05341960407611168, -5.049401038298163336, 21.45724293864768839 ) ) ;
#105565=CARTESIAN_POINT ( 'NONE',  ( -19.05341960407611168, -5.049401038298163336, 76.45724293864769550 ) ) ;
#105566=CARTESIAN_POINT ( 'NONE',  ( -0.05219959533907301413, -21.53943276465977519, 77.49890960531433848 ) ) ;
#105567=CARTESIAN_POINT ( 'NONE',  ( 5.153800228976615827, -19.02544592524334988, 110.2094237280189901 ) ) ;
#105568=CARTESIAN_POINT ( 'NONE',  ( 0.05219959533910956823, 16.53943276465976808, 44.99890960531435979 ) ) ;
#105569=CARTESIAN_POINT ( 'NONE',  ( -21.52544592524334988, -5.823673210054445271, 53.95942372801900433 ) ) ;
#105570=CARTESIAN_POINT ( 'NONE',  ( -4.483927247898782831, 16.52544592524335698, 87.70942372801901854 ) ) ;
#105571=CARTESIAN_POINT ( 'NONE',  ( 15.80617190586746368, 15.72974639402197994, 29.37390960531435269 ) ) ;
#105572=CARTESIAN_POINT ( 'NONE',  ( -16.51473224551069308, -9.474510206698971260, 101.6655762719810241 ) ) ;
#105573=CARTESIAN_POINT ( 'NONE',  ( -17.12812012977028431, 6.668231424565929544, 78.64051240676859322 ) ) ;
#105574=CARTESIAN_POINT ( 'NONE',  ( -14.34966873604972548, 8.224510206698743886, 113.3344237280190328 ) ) ;
#105575=CARTESIAN_POINT ( 'NONE',  ( -16.52544592524335698, -4.483927247898792601, 48.95942372801902565 ) ) ;
#105576=CARTESIAN_POINT ( 'NONE',  ( -16.51473224551069308, -9.474510206698971260, 61.66557627198103120 ) ) ;
#105577=CARTESIAN_POINT ( 'NONE',  ( 13.89961937509977652, -13.97604488694527269, 68.12390960531436690 ) ) ;
#105578=CARTESIAN_POINT ( 'NONE',  ( 14.34966873604972726, -8.224510206698740333, 70.83442372801901854 ) ) ;
#105579=CARTESIAN_POINT ( 'NONE',  ( 12.14591786802309770, 12.06949235617756955, 49.37390960531436690 ) ) ;
#105580=CARTESIAN_POINT ( 'NONE',  ( 19.05341960407611168, 5.049401038298154454, 58.95724293864768129 ) ) ;
#105581=CARTESIAN_POINT ( 'NONE',  ( -16.46253265017160317, 9.564922557960807481, 45.83224293864769550 ) ) ;
#105582=CARTESIAN_POINT ( 'NONE',  ( 8.224510206698742110, 14.34966873604972548, 42.08442372801901854 ) ) ;
#105583=CARTESIAN_POINT ( 'NONE',  ( 0.05219959533936267826, -19.03943276465977164, 90.00109039468567573 ) ) ;
#105584=CARTESIAN_POINT ( 'NONE',  ( 12.14591786802309770, 12.06949235617756955, 99.37390960531436690 ) ) ;
#105585=CARTESIAN_POINT ( 'NONE',  ( 16.51473224551069308, 9.474510206698969483, 59.16557627198102409 ) ) ;
#105586=CARTESIAN_POINT ( 'NONE',  ( -9.474510206698720793, -16.51473224551083518, 99.58442372801900433 ) ) ;
#105588=CARTESIAN_POINT ( 'NONE',  ( 21.55341960407619695, -5.719274019375665929, 91.04275706135236135 ) ) ;
#105589=CARTESIAN_POINT ( 'NONE',  ( -8.224510206698735004, -14.34966873604973081, 64.58442372801900433 ) ) ;
#105591=CARTESIAN_POINT ( 'NONE',  ( -5.719274019375978568, 21.55341960407610458, 60.20724293864768839 ) ) ;
#105592=CARTESIAN_POINT ( 'NONE',  ( -12.06949235617739369, -12.14591786802326823, 54.37609039468568994 ) ) ;
#105593=CARTESIAN_POINT ( 'NONE',  ( 0.05219959533909260263, 19.03943276465977164, 34.99890960531435979 ) ) ;
#105594=CARTESIAN_POINT ( 'NONE',  ( 19.02544592524334988, 5.153800228976608722, 36.45942372801900433 ) ) ;
#105595=CARTESIAN_POINT ( 'NONE',  ( 16.46253265017160672, -9.564922557960803928, 93.33224293864769550 ) ) ;
#105596=CARTESIAN_POINT ( 'NONE',  ( 8.224510206698953496, -14.34966873604960469, 112.9155762719810383 ) ) ;
#105597=CARTESIAN_POINT ( 'NONE',  ( -13.97604488694527625, -13.89961937509977652, 66.87390960531436690 ) ) ;
#105599=CARTESIAN_POINT ( 'NONE',  ( -0.05219959533937732626, 21.53943276465977519, 82.50109039468568994 ) ) ;
#105600=CARTESIAN_POINT ( 'NONE',  ( -9.564922557960796823, -16.46253265017161027, 92.08224293864769550 ) ) ;
#105601=CARTESIAN_POINT ( 'NONE',  ( 16.51473224551083163, -9.474510206698727899, 30.83442372801900433 ) ) ;
#105602=CARTESIAN_POINT ( 'NONE',  ( -9.474510206698720793, -16.51473224551083518, 29.58442372801900433 ) ) ;
#105603=CARTESIAN_POINT ( 'NONE',  ( -14.29746914071049879, 8.314922557960819915, 50.83224293864770971 ) ) ;
#105604=CARTESIAN_POINT ( 'NONE',  ( -9.474510206698964154, 16.51473224551069663, 55.41557627198103120 ) ) ;
#105605=CARTESIAN_POINT ( 'NONE',  ( -5.719274019375978568, 21.55341960407610458, 30.20724293864769550 ) ) ;
#105606=CARTESIAN_POINT ( 'NONE',  ( 15.80617190586769283, -15.72974639402175789, 80.62609039468567573 ) ) ;
#105607=CARTESIAN_POINT ( 'NONE',  ( -13.89961937509977652, 13.97604488694528158, 70.62390960531432427 ) ) ;
#105608=CARTESIAN_POINT ( 'NONE',  ( 21.53943276465977519, 0.05219959533937863772, 81.25109039468568994 ) ) ;
#105609=CARTESIAN_POINT ( 'NONE',  ( -10.81492255796078084, -18.62759615963271287, 32.08224293864769550 ) ) ;
#105610=CARTESIAN_POINT ( 'NONE',  ( -19.02544592524342804, 5.153800228976336051, 66.04057627198103830 ) ) ;
#105611=CARTESIAN_POINT ( 'NONE',  ( -21.55341960407619339, 5.719274019375674811, 38.54275706135234714 ) ) ;
#105612=CARTESIAN_POINT ( 'NONE',  ( 5.153800228976615827, -19.02544592524334988, 65.20942372801900433 ) ) ;
#105613=CARTESIAN_POINT ( 'NONE',  ( 19.05341960407611168, 5.049401038298154454, 38.95724293864767418 ) ) ;
#105614=CARTESIAN_POINT ( 'NONE',  ( 9.564922557960805705, 16.46253265017160317, 84.58224293864769550 ) ) ;
#105615=CARTESIAN_POINT ( 'NONE',  ( -16.55341960407617563, 4.379528057220093196, 23.54275706135235424 ) ) ;
#105616=CARTESIAN_POINT ( 'NONE',  ( 8.224510206698953496, -14.34966873604960469, 82.91557627198103830 ) ) ;
#105617=CARTESIAN_POINT ( 'NONE',  ( 19.02544592524343514, -5.153800228976328945, 63.54057627198103830 ) ) ;
#105618=CARTESIAN_POINT ( 'NONE',  ( -18.62759615963270932, 10.81492255796079327, 55.83224293864770260 ) ) ;
#105619=CARTESIAN_POINT ( 'NONE',  ( -14.29746914071037622, -8.314922557961029526, 24.16775706135235424 ) ) ;
#105620=CARTESIAN_POINT ( 'NONE',  ( -21.52544592524334988, -5.823673210054445271, 23.95942372801901143 ) ) ;
#105621=CARTESIAN_POINT ( 'NONE',  ( 21.55341960407619695, -5.719274019375665929, 71.04275706135234714 ) ) ;
#105622=CARTESIAN_POINT ( 'NONE',  ( -14.29746914071037622, -8.314922557961029526, 74.16775706135231871 ) ) ;
#105623=CARTESIAN_POINT ( 'NONE',  ( 4.483927247898790824, -16.52544592524335698, 70.20942372801904696 ) ) ;
#105624=CARTESIAN_POINT ( 'NONE',  ( -16.51473224551069308, -9.474510206698971260, 56.66557627198103120 ) ) ;
#105625=CARTESIAN_POINT ( 'NONE',  ( -16.53943276465976808, -0.05219959533934237506, 93.75109039468567573 ) ) ;
#105626=CARTESIAN_POINT ( 'NONE',  ( -19.02544592524334988, -5.153800228976617603, 43.95942372801899012 ) ) ;
#105627=CARTESIAN_POINT ( 'NONE',  ( -21.52544592524334988, -5.823673210054445271, 23.95942372801901143 ) ) ;
#105628=CARTESIAN_POINT ( 'NONE',  ( -16.52544592524342804, 4.483927247898546575, 61.04057627198103120 ) ) ;
#105629=CARTESIAN_POINT ( 'NONE',  ( -19.02544592524342804, 5.153800228976336051, 91.04057627198100988 ) ) ;
#105630=CARTESIAN_POINT ( 'NONE',  ( -16.53943276465976808, -0.05219959533934237506, 93.75109039468567573 ) ) ;
#105631=CARTESIAN_POINT ( 'NONE',  ( 21.55341960407619695, -5.719274019375665929, 56.04275706135235424 ) ) ;
#105632=CARTESIAN_POINT ( 'NONE',  ( -8.224510206698735004, -14.34966873604973081, 34.58442372801900433 ) ) ;
#105633=CARTESIAN_POINT ( 'NONE',  ( -21.53943276465977519, -0.05219959533937600094, 23.75109039468567929 ) ) ;
#105634=CARTESIAN_POINT ( 'NONE',  ( 8.314922557960818139, 14.29746914071049879, 64.58224293864769550 ) ) ;
#105636=CARTESIAN_POINT ( 'NONE',  ( -10.72451020669898014, 18.67979575497178502, 100.4155762719810241 ) ) ;
#105637=CARTESIAN_POINT ( 'NONE',  ( -16.52544592524342804, 4.483927247898546575, 36.04057627198102409 ) ) ;
#105640=CARTESIAN_POINT ( 'NONE',  ( 15.80617190586746368, 15.72974639402197994, 29.37390960531435269 ) ) ;
#105641=CARTESIAN_POINT ( 'NONE',  ( 18.62759615963255655, 10.81492255796105972, 31.66775706135234358 ) ) ;
#105642=CARTESIAN_POINT ( 'NONE',  ( -0.05219959533910754901, -16.53943276465976808, 62.49890960531436690 ) ) ;
#105643=CARTESIAN_POINT ( 'NONE',  ( -19.05341960407611168, -5.049401038298163336, 76.45724293864769550 ) ) ;
#105644=CARTESIAN_POINT ( 'NONE',  ( -19.03943276465977164, 0.05219959533909376836, 31.24890960531435979 ) ) ;
#105645=CARTESIAN_POINT ( 'NONE',  ( -5.153800228976607833, 19.02544592524334988, 67.70942372801900433 ) ) ;
#105646=CARTESIAN_POINT ( 'NONE',  ( 15.80617190586746368, 15.72974639402197994, 49.37390960531436690 ) ) ;
#105648=CARTESIAN_POINT ( 'NONE',  ( 19.02544592524343514, -5.153800228976328945, 58.54057627198102409 ) ) ;
#105649=CARTESIAN_POINT ( 'NONE',  ( 8.314922557961029526, -14.29746914071037800, 30.41775706135234358 ) ) ;
#105650=CARTESIAN_POINT ( 'NONE',  ( -18.62759615963270932, 10.81492255796079327, 115.8322429386477097 ) ) ;
#105652=CARTESIAN_POINT ( 'NONE',  ( 14.34966873604960469, 8.224510206698951720, 54.16557627198103120 ) ) ;
#105654=CARTESIAN_POINT ( 'NONE',  ( 16.51473224551069308, 9.474510206698969483, 94.16557627198103830 ) ) ;
#105655=CARTESIAN_POINT ( 'NONE',  ( 18.62759615963271287, -10.81492255796078972, 68.33224293864769550 ) ) ;
#105656=CARTESIAN_POINT ( 'NONE',  ( -0.05219959533907301413, -21.53943276465977519, 107.4989096053143669 ) ) ;
#105657=CARTESIAN_POINT ( 'NONE',  ( 0.05219959533934541429, -16.53943276465976808, 40.00109039468567573 ) ) ;
#105659=CARTESIAN_POINT ( 'NONE',  ( 15.72974639402199770, -15.80617190586745480, 33.12390960531435979 ) ) ;
#105660=CARTESIAN_POINT ( 'NONE',  ( 10.72451020669871369, 18.67979575497193778, 102.0844237280190185 ) ) ;
#105661=CARTESIAN_POINT ( 'NONE',  ( 16.51473224551069308, 9.474510206698969483, 94.16557627198103830 ) ) ;
#105662=CARTESIAN_POINT ( 'NONE',  ( -13.97604488694527625, -13.89961937509977652, 46.87390960531435979 ) ) ;
#105663=CARTESIAN_POINT ( 'NONE',  ( 19.02544592524343514, -5.153800228976328945, 103.5405762719809957 ) ) ;
#105664=B_SPLINE_CURVE_WITH_KNOTS ( 'NONE', 3,
 ( #68309, #98633, #37988, #161327, #51156, #22820, #189683, #147164, #128972, #146144, #7631, #21818, #69315, #190671, #52147, #8652, #112816, #174509, #160328, #76233 ),
 .UNSPECIFIED., .F., .F.,
 ( 4, 2, 2, 2, 2, 2, 2, 2, 2, 4 ),
 ( 0.000000000000000000, 0.0004987090165372536207, 0.0009974180330745072414, 0.001246772541343133889, 0.001496127049611760971, 0.001994836066149014483, 0.002493545082686267778, 0.002742899590954906135, 0.002992254099223544492, 0.003989672132298113100 ),
 .UNSPECIFIED. ) ;
#105665=CARTESIAN_POINT ( 'NONE',  ( 0.05219959533909260263, 19.03943276465977164, 79.99890960531436690 ) ) ;
#105666=CARTESIAN_POINT ( 'NONE',  ( 17.05587630539710275, -6.762274262136627634, 88.24180309037284076 ) ) ;
#105667=CARTESIAN_POINT ( 'NONE',  ( -13.89961937509957401, -13.97604488694547875, 59.37609039468566863 ) ) ;
#105668=CARTESIAN_POINT ( 'NONE',  ( -5.823673210054431948, 21.52544592524334988, 112.7094237280190328 ) ) ;
#105669=CARTESIAN_POINT ( 'NONE',  ( 21.55341960407610458, 5.719274019375980345, 33.95724293864769550 ) ) ;
#105670=CARTESIAN_POINT ( 'NONE',  ( 14.29746914071037800, 8.314922557961029526, 106.6677570613523756 ) ) ;
#105671=CARTESIAN_POINT ( 'NONE',  ( -19.05341960407617563, 5.049401038297882671, 83.54275706135233293 ) ) ;
#105673=CARTESIAN_POINT ( 'NONE',  ( -16.46253265017146816, -9.564922557961047289, 79.16775706135234714 ) ) ;
#105674=CARTESIAN_POINT ( 'NONE',  ( 13.89961937509957401, 13.97604488694547697, 31.87609039468566863 ) ) ;
#105675=CARTESIAN_POINT ( 'NONE',  ( 18.09867054820430710, 5.500000000000000000, 71.48393025253585620 ) ) ;
#105676=CARTESIAN_POINT ( 'NONE',  ( -5.049401038298153566, 19.05341960407611168, 45.20724293864769550 ) ) ;
#105677=CARTESIAN_POINT ( 'NONE',  ( 12.14591786802309770, 12.06949235617756955, 54.37390960531435979 ) ) ;
#105678=CARTESIAN_POINT ( 'NONE',  ( -17.49999999999999645, -5.624438216177585659, 109.1832965508535551 ) ) ;
#105679=CARTESIAN_POINT ( 'NONE',  ( -8.224510206698948167, 14.34966873604960824, 30.41557627198101699 ) ) ;
#105680=LINE ( 'NONE', #88520, #3246 ) ;
#105681=CARTESIAN_POINT ( 'NONE',  ( 16.52544592524335698, 4.483927247898782831, 96.45942372801901854 ) ) ;
#105682=CARTESIAN_POINT ( 'NONE',  ( 19.02544592524343514, -5.153800228976328945, 53.54057627198102409 ) ) ;
#105683=CARTESIAN_POINT ( 'NONE',  ( -5.719274019375665041, -21.55341960407619695, 109.7927570613523613 ) ) ;
#105684=CARTESIAN_POINT ( 'NONE',  ( 13.97604488694548053, -13.89961937509957401, 110.6260903946856615 ) ) ;
#105685=CARTESIAN_POINT ( 'NONE',  ( -18.67979575497193778, 10.72451020669871902, 93.33442372801901854 ) ) ;
#105687=CARTESIAN_POINT ( 'NONE',  ( 19.05341960407611168, 5.049401038298154454, 88.95724293864769550 ) ) ;
#105688=CARTESIAN_POINT ( 'NONE',  ( 19.02544592524343514, -5.153800228976328945, 78.54057627198099567 ) ) ;
#105690=CARTESIAN_POINT ( 'NONE',  ( -5.719274019375978568, 21.55341960407610458, 110.2072429386477239 ) ) ;
#105692=CARTESIAN_POINT ( 'NONE',  ( 16.55341960407611168, 4.379528057220329451, 78.95724293864769550 ) ) ;
#105693=CARTESIAN_POINT ( 'NONE',  ( 21.53943276465977519, -0.05219959533907433946, 73.74890960531433848 ) ) ;
#105694=CARTESIAN_POINT ( 'NONE',  ( -19.02544592524342804, 5.153800228976336051, 56.04057627198100988 ) ) ;
#105695=CARTESIAN_POINT ( 'NONE',  ( 18.67979575497178502, 10.72451020669898547, 99.16557627198100988 ) ) ;
#105696=CARTESIAN_POINT ( 'NONE',  ( 0.05219959533934541429, -16.53943276465976808, 85.00109039468568994 ) ) ;
#105698=CARTESIAN_POINT ( 'NONE',  ( -16.46253265017160317, 9.564922557960807481, 65.83224293864769550 ) ) ;
#105699=CARTESIAN_POINT ( 'NONE',  ( -0.05219959533910754901, -16.53943276465976808, 87.49890960531436690 ) ) ;
#105701=CARTESIAN_POINT ( 'NONE',  ( -9.564922557960796823, -16.46253265017161027, 67.08224293864769550 ) ) ;
#105702=CARTESIAN_POINT ( 'NONE',  ( 13.89961937509957401, 13.97604488694547697, 81.87609039468564731 ) ) ;
#105703=CARTESIAN_POINT ( 'NONE',  ( -12.06949235617756955, 12.14591786802309770, 80.62390960531438111 ) ) ;
#105704=CARTESIAN_POINT ( 'NONE',  ( 5.719274019375673035, 21.55341960407619339, 62.29275706135236845 ) ) ;
#105705=CARTESIAN_POINT ( 'NONE',  ( 9.474510206698971260, -16.51473224551069308, 47.91557627198102409 ) ) ;
#105706=CARTESIAN_POINT ( 'NONE',  ( -10.72451020669870658, -18.67979575497194134, 19.58442372801901143 ) ) ;
#105707=CARTESIAN_POINT ( 'NONE',  ( 16.55341960407611168, 4.379528057220329451, 98.95724293864770971 ) ) ;
#105708=CARTESIAN_POINT ( 'NONE',  ( 17.97214573761834799, 5.499999999999959144, 93.96970049038657180 ) ) ;
#105709=CARTESIAN_POINT ( 'NONE',  ( 16.51473224551069308, 9.474510206698969483, 54.16557627198103120 ) ) ;
#105711=CARTESIAN_POINT ( 'NONE',  ( -16.51473224551082808, 9.474510206698731452, 93.33442372801900433 ) ) ;
#105712=CARTESIAN_POINT ( 'NONE',  ( 13.97604488694527802, 13.89961937509977652, 109.3739096053143669 ) ) ;
#105713=CARTESIAN_POINT ( 'NONE',  ( 5.823673210054444382, -21.52544592524334988, 45.20942372801901854 ) ) ;
#105714=CARTESIAN_POINT ( 'NONE',  ( 19.02544592524343514, -5.153800228976328945, 88.54057627198102409 ) ) ;
#105715=CARTESIAN_POINT ( 'NONE',  ( 19.05341960407617918, -5.049401038297876454, 76.04275706135230450 ) ) ;
#105716=CARTESIAN_POINT ( 'NONE',  ( 16.51473224551069308, 9.474510206698969483, 64.16557627198102409 ) ) ;
#105717=CARTESIAN_POINT ( 'NONE',  ( 12.14591786802309770, 12.06949235617756955, 79.37390960531436690 ) ) ;
#105718=CARTESIAN_POINT ( 'NONE',  ( 4.483927247898545687, 16.52544592524342804, 74.79057627198105251 ) ) ;
#105719=CARTESIAN_POINT ( 'NONE',  ( -5.049401038298153566, 19.05341960407611168, 90.20724293864766707 ) ) ;
#105720=CARTESIAN_POINT ( 'NONE',  ( 16.55341960407611168, 4.379528057220329451, 78.95724293864769550 ) ) ;
#105721=CARTESIAN_POINT ( 'NONE',  ( 9.564922557960805705, 16.46253265017160317, 89.58224293864769550 ) ) ;
#105722=CARTESIAN_POINT ( 'NONE',  ( -19.02544592524334988, -5.153800228976617603, 33.95942372801897591 ) ) ;
#105723=CARTESIAN_POINT ( 'NONE',  ( -0.05219959533909027116, -19.03943276465977164, 47.49890960531435979 ) ) ;
#105724=CARTESIAN_POINT ( 'NONE',  ( 8.314922557960818139, 14.29746914071049879, 24.58224293864768839 ) ) ;
#105725=CARTESIAN_POINT ( 'NONE',  ( 4.379528057220339221, -16.55341960407611168, 112.7072429386476955 ) ) ;
#105727=CARTESIAN_POINT ( 'NONE',  ( -10.72451020669870658, -18.67979575497194134, 44.58442372801901854 ) ) ;
#105728=CARTESIAN_POINT ( 'NONE',  ( 5.153800228976615827, -19.02544592524334988, 70.20942372801899012 ) ) ;
#105729=CARTESIAN_POINT ( 'NONE',  ( -4.483927247898539470, -16.52544592524342804, 42.29057627198103120 ) ) ;
#105730=CARTESIAN_POINT ( 'NONE',  ( -18.67979575497178146, -10.72451020669898902, 81.66557627198103830 ) ) ;
#105731=CARTESIAN_POINT ( 'NONE',  ( -16.51473224551069308, -9.474510206698971260, 111.6655762719810383 ) ) ;
#105732=CARTESIAN_POINT ( 'NONE',  ( -4.483927247898539470, -16.52544592524342804, 67.29057627198103830 ) ) ;
#105733=CARTESIAN_POINT ( 'NONE',  ( -5.049401038298153566, 19.05341960407611168, 40.20724293864768839 ) ) ;
#105734=CARTESIAN_POINT ( 'NONE',  ( 16.46253265017146816, 9.564922557961045513, 46.66775706135233293 ) ) ;
#105735=CARTESIAN_POINT ( 'NONE',  ( 12.06949235617739724, 12.14591786802326823, 106.8760903946856899 ) ) ;
#105736=CARTESIAN_POINT ( 'NONE',  ( 8.224510206698742110, 14.34966873604972548, 52.08442372801901854 ) ) ;
#105737=CARTESIAN_POINT ( 'NONE',  ( 10.81492255796078972, 18.62759615963270932, 39.58224293864769550 ) ) ;
#105738=CARTESIAN_POINT ( 'NONE',  ( -10.72451020669870658, -18.67979575497194134, 109.5844237280190328 ) ) ;
#105739=CARTESIAN_POINT ( 'NONE',  ( -13.97604488694527625, -13.89961937509977652, 91.87390960531432427 ) ) ;
#105740=CARTESIAN_POINT ( 'NONE',  ( -16.52544592524335698, -4.483927247898792601, 78.95942372801901854 ) ) ;
#105741=CARTESIAN_POINT ( 'NONE',  ( 16.52544592524342804, -4.483927247898539470, 113.5405762719810383 ) ) ;
#105742=CARTESIAN_POINT ( 'NONE',  ( -16.52544592524342804, 4.483927247898546575, 41.04057627198103120 ) ) ;
#105743=CARTESIAN_POINT ( 'NONE',  ( -19.02544592524342804, 5.153800228976336051, 101.0405762719810241 ) ) ;
#105744=CARTESIAN_POINT ( 'NONE',  ( -16.46253265017160317, 9.564922557960807481, 95.83224293864769550 ) ) ;
#105745=CARTESIAN_POINT ( 'NONE',  ( 5.823673210054125526, 21.52544592524343514, 29.79057627198102409 ) ) ;
#105747=CARTESIAN_POINT ( 'NONE',  ( -16.55341960407611168, -4.379528057220339221, 71.45724293864769550 ) ) ;
#105748=CARTESIAN_POINT ( 'NONE',  ( -16.53943276465976808, 0.05219959533911058130, 56.24890960531436690 ) ) ;
#105749=CARTESIAN_POINT ( 'NONE',  ( -14.34966873604972548, 8.224510206698743886, 58.33442372801901143 ) ) ;
#105751=CARTESIAN_POINT ( 'NONE',  ( 13.89961937509957401, 13.97604488694547697, 56.87609039468564731 ) ) ;
#105752=CARTESIAN_POINT ( 'NONE',  ( 19.05341960407611168, 5.049401038298154454, 93.95724293864769550 ) ) ;
#105753=CARTESIAN_POINT ( 'NONE',  ( 0.05219959533936267826, -19.03943276465977164, 70.00109039468566152 ) ) ;
#105755=CARTESIAN_POINT ( 'NONE',  ( -0.05219959533936034679, 19.03943276465977164, 52.50109039468566863 ) ) ;
#105756=CARTESIAN_POINT ( 'NONE',  ( 9.474510206698729675, 16.51473224551082808, 102.0844237280190043 ) ) ;
#105757=CARTESIAN_POINT ( 'NONE',  ( 8.224510206698742110, 14.34966873604972548, 97.08442372801904696 ) ) ;
#105759=CARTESIAN_POINT ( 'NONE',  ( 5.153800228976335163, 19.02544592524342804, 39.79057627198100988 ) ) ;
#105760=CARTESIAN_POINT ( 'NONE',  ( 0.05219959533909260263, 19.03943276465977164, 114.9989096053143669 ) ) ;
#105761=CARTESIAN_POINT ( 'NONE',  ( -21.55341960407619339, 5.719274019375674811, 53.54275706135234714 ) ) ;
#105762=CARTESIAN_POINT ( 'NONE',  ( -9.474510206698720793, -16.51473224551083518, 109.5844237280190043 ) ) ;
#105763=CARTESIAN_POINT ( 'NONE',  ( 17.50000000000001421, 3.817821230385223696, 23.21443863932539742 ) ) ;
#105764=CARTESIAN_POINT ( 'NONE',  ( 16.46253265017160672, -9.564922557960803928, 58.33224293864769550 ) ) ;
#105766=CARTESIAN_POINT ( 'NONE',  ( 16.52544592524342804, -4.483927247898539470, 73.54057627198102409 ) ) ;
#105767=CARTESIAN_POINT ( 'NONE',  ( 5.153800228976335163, 19.02544592524342804, 64.79057627198100988 ) ) ;
#105768=CARTESIAN_POINT ( 'NONE',  ( -5.153800228976328057, -19.02544592524343514, 72.29057627198102409 ) ) ;
#105769=CARTESIAN_POINT ( 'NONE',  ( -19.02544592524334988, -5.153800228976617603, 78.95942372801900433 ) ) ;
#105770=CARTESIAN_POINT ( 'NONE',  ( 10.81492255796078972, 18.62759615963270932, 69.58224293864769550 ) ) ;
#105771=CARTESIAN_POINT ( 'NONE',  ( 4.379528057220339221, -16.55341960407611168, 112.7072429386476955 ) ) ;
#105772=CARTESIAN_POINT ( 'NONE',  ( 16.51473224551083163, -9.474510206698727899, 40.83442372801900433 ) ) ;
#105773=CARTESIAN_POINT ( 'NONE',  ( 19.03943276465977164, -0.05219959533909143690, 73.74890960531435269 ) ) ;
#105774=ADVANCED_FACE ( 'NONE', ( #147048 ), #88899, .T. ) ;
#105775=CARTESIAN_POINT ( 'NONE',  ( 10.81492255796078972, 18.62759615963270932, 89.58224293864768129 ) ) ;
#105776=CARTESIAN_POINT ( 'NONE',  ( -8.224510206698948167, 14.34966873604960824, 75.41557627198102409 ) ) ;
#105777=CARTESIAN_POINT ( 'NONE',  ( -13.89961937509957401, -13.97604488694547875, 44.37609039468566863 ) ) ;
#105778=CARTESIAN_POINT ( 'NONE',  ( -0.05219959533907301413, -21.53943276465977519, 77.49890960531433848 ) ) ;
#105779=CARTESIAN_POINT ( 'NONE',  ( -18.67979575497178146, -10.72451020669898902, 61.66557627198103120 ) ) ;
#105780=CARTESIAN_POINT ( 'NONE',  ( 15.80617190586746368, 15.72974639402197994, 34.37390960531435979 ) ) ;
#105781=CARTESIAN_POINT ( 'NONE',  ( 15.72974639402176855, 15.80617190586768217, 96.87609039468568994 ) ) ;
#105782=CARTESIAN_POINT ( 'NONE',  ( -16.51473224551069308, -9.474510206698971260, 81.66557627198103830 ) ) ;
#105783=CARTESIAN_POINT ( 'NONE',  ( 8.314922557960818139, 14.29746914071049879, 114.5822429386477097 ) ) ;
#105785=CARTESIAN_POINT ( 'NONE',  ( -18.62759615963255300, -10.81492255796106328, 29.16775706135234003 ) ) ;
#105786=CARTESIAN_POINT ( 'NONE',  ( -0.05219959533937732626, 21.53943276465977519, 37.50109039468568284 ) ) ;
#105787=CARTESIAN_POINT ( 'NONE',  ( 5.049401038298161559, -19.05341960407611168, 32.70724293864768129 ) ) ;
#105788=CARTESIAN_POINT ( 'NONE',  ( -21.55341960407619339, 5.719274019375674811, 23.54275706135235424 ) ) ;
#105789=CARTESIAN_POINT ( 'NONE',  ( -19.05341960407617563, 5.049401038297882671, 58.54275706135234003 ) ) ;
#105790=CARTESIAN_POINT ( 'NONE',  ( 19.02544592524343514, -5.153800228976328945, 38.54057627198103120 ) ) ;
#105791=CARTESIAN_POINT ( 'NONE',  ( -14.29746914071037622, -8.314922557961029526, 34.16775706135234714 ) ) ;
#105792=CARTESIAN_POINT ( 'NONE',  ( 5.153800228976335163, 19.02544592524342804, 24.79057627198102765 ) ) ;
#105793=CARTESIAN_POINT ( 'NONE',  ( 16.52544592524335698, 4.483927247898782831, 66.45942372801903275 ) ) ;
#105794=CARTESIAN_POINT ( 'NONE',  ( 5.153800228976335163, 19.02544592524342804, 34.79057627198102409 ) ) ;
#105796=CARTESIAN_POINT ( 'NONE',  ( 19.05341960407611168, 5.049401038298154454, 88.95724293864769550 ) ) ;
#105797=CARTESIAN_POINT ( 'NONE',  ( 0.05219959533909260263, 19.03943276465977164, 29.99890960531435979 ) ) ;
#105798=CARTESIAN_POINT ( 'NONE',  ( -21.53943276465977519, 0.05219959533907696930, 56.24890960531436690 ) ) ;
#105799=CARTESIAN_POINT ( 'NONE',  ( -14.34966873604972548, 8.224510206698743886, 48.33442372801902565 ) ) ;
#105800=CARTESIAN_POINT ( 'NONE',  ( -18.67979575497193778, 10.72451020669871902, 93.33442372801901854 ) ) ;
#105801=CARTESIAN_POINT ( 'NONE',  ( 13.89961937509977652, -13.97604488694527269, 38.12390960531436690 ) ) ;
#105802=CARTESIAN_POINT ( 'NONE',  ( 12.06949235617757843, -12.14591786802309237, 38.12390960531436690 ) ) ;
#105803=CARTESIAN_POINT ( 'NONE',  ( 14.34966873604960469, 8.224510206698951720, 74.16557627198102409 ) ) ;
#105804=CARTESIAN_POINT ( 'NONE',  ( -5.049401038298153566, 19.05341960407611168, 70.20724293864769550 ) ) ;
#105805=CARTESIAN_POINT ( 'NONE',  ( 19.05341960407617918, -5.049401038297876454, 21.04275706135232582 ) ) ;
#105806=CARTESIAN_POINT ( 'NONE',  ( 21.52544592524334988, 5.823673210054432836, 26.45942372801901854 ) ) ;
#105807=CARTESIAN_POINT ( 'NONE',  ( 10.72451020669871369, 18.67979575497193778, 82.08442372801901854 ) ) ;
#105808=CARTESIAN_POINT ( 'NONE',  ( -16.55341960407617563, 4.379528057220093196, 48.54275706135234714 ) ) ;
#105809=CARTESIAN_POINT ( 'NONE',  ( -16.52544592524335698, -4.483927247898792601, 33.95942372801901143 ) ) ;
#105810=CARTESIAN_POINT ( 'NONE',  ( 12.14591786802309770, 12.06949235617756955, 89.37390960531435269 ) ) ;
#105811=CARTESIAN_POINT ( 'NONE',  ( -5.719274019375665041, -21.55341960407619695, 94.79275706135234714 ) ) ;
#105813=CARTESIAN_POINT ( 'NONE',  ( -4.483927247898539470, -16.52544592524342804, 32.29057627198102409 ) ) ;
#105814=CARTESIAN_POINT ( 'NONE',  ( 9.474510206698971260, -16.51473224551069308, 27.91557627198103120 ) ) ;
#105815=CARTESIAN_POINT ( 'NONE',  ( 16.53943276465976808, 0.05219959533934440121, 46.25109039468567573 ) ) ;
#105816=CARTESIAN_POINT ( 'NONE',  ( -8.224510206698948167, 14.34966873604960824, 55.41557627198102409 ) ) ;
#105817=CARTESIAN_POINT ( 'NONE',  ( 14.29746914071037800, 8.314922557961029526, 81.66775706135236135 ) ) ;
#105818=CARTESIAN_POINT ( 'NONE',  ( 19.02544592524343514, -5.153800228976328945, 98.54057627198100988 ) ) ;
#105819=CARTESIAN_POINT ( 'NONE',  ( 15.80617190586746368, 15.72974639402197994, 24.37390960531435979 ) ) ;
#105820=CARTESIAN_POINT ( 'NONE',  ( -0.05219959533936034679, 19.03943276465977164, 22.50109039468566152 ) ) ;
#105821=CARTESIAN_POINT ( 'NONE',  ( 12.14591786802309770, 12.06949235617756955, 84.37390960531438111 ) ) ;
#105822=CARTESIAN_POINT ( 'NONE',  ( -0.05219959533909027116, -19.03943276465977164, 92.49890960531436690 ) ) ;
#105824=CARTESIAN_POINT ( 'NONE',  ( 4.379528057220092307, 16.55341960407617563, 37.29275706135235424 ) ) ;
#105825=CARTESIAN_POINT ( 'NONE',  ( -19.05341960407611168, -5.049401038298163336, 46.45724293864768129 ) ) ;
#105826=CARTESIAN_POINT ( 'NONE',  ( 16.51473224551069308, 9.474510206698969483, 109.1655762719810383 ) ) ;
#105827=CARTESIAN_POINT ( 'NONE',  ( 12.06949235617739724, 12.14591786802326823, 46.87609039468568994 ) ) ;
#105828=CARTESIAN_POINT ( 'NONE',  ( -17.49999999999999645, -5.499999999999992895, 79.20309617465829888 ) ) ;
#105829=CARTESIAN_POINT ( 'NONE',  ( -19.05341960407617563, 5.049401038297882671, 43.54275706135232582 ) ) ;
#105830=CARTESIAN_POINT ( 'NONE',  ( 5.153800228976335163, 19.02544592524342804, 49.79057627198100988 ) ) ;
#105831=CARTESIAN_POINT ( 'NONE',  ( -0.05219959533934338120, 16.53943276465976808, 77.50109039468567573 ) ) ;
#105832=CARTESIAN_POINT ( 'NONE',  ( -19.05341960407617563, 5.049401038297882671, 83.54275706135233293 ) ) ;
#105833=CARTESIAN_POINT ( 'NONE',  ( -9.474510206698720793, -16.51473224551083518, 24.58442372801900078 ) ) ;
#105834=CARTESIAN_POINT ( 'NONE',  ( -16.46253265017160317, 9.564922557960807481, 55.83224293864769550 ) ) ;
#105835=CARTESIAN_POINT ( 'NONE',  ( 16.55341960407611168, 4.379528057220329451, 98.95724293864770971 ) ) ;
#105836=CARTESIAN_POINT ( 'NONE',  ( 9.564922557961047289, -16.46253265017146816, 70.41775706135233293 ) ) ;
#105837=CARTESIAN_POINT ( 'NONE',  ( -5.719274019375978568, 21.55341960407610458, 70.20724293864769550 ) ) ;
#105838=CARTESIAN_POINT ( 'NONE',  ( -9.564922557961040184, 16.46253265017147172, 27.91775706135232582 ) ) ;
#105839=CARTESIAN_POINT ( 'NONE',  ( 19.05341960407611168, 5.049401038298154454, 103.9572429386476671 ) ) ;
#105840=CARTESIAN_POINT ( 'NONE',  ( 10.72451020669898902, -18.67979575497178502, 82.91557627198103830 ) ) ;
#105842=CARTESIAN_POINT ( 'NONE',  ( 9.564922557961047289, -16.46253265017146816, 100.4177570613523329 ) ) ;
#105843=DIRECTION ( 'NONE',  ( -1.000000000000000000, -0.000000000000000000, -0.000000000000000000 ) ) ;
#105845=CARTESIAN_POINT ( 'NONE',  ( -14.34966873604972548, 8.224510206698743886, 28.33442372801902209 ) ) ;
#105846=CARTESIAN_POINT ( 'NONE',  ( -9.564922557960796823, -16.46253265017161027, 37.08224293864768839 ) ) ;
#105847=CARTESIAN_POINT ( 'NONE',  ( -13.89961937509977652, 13.97604488694528158, 115.6239096053143669 ) ) ;
#105848=CARTESIAN_POINT ( 'NONE',  ( 5.823673210054125526, 21.52544592524343514, 94.79057627198105251 ) ) ;
#105849=CARTESIAN_POINT ( 'NONE',  ( 21.52544592524334988, 5.823673210054432836, 66.45942372801903275 ) ) ;
#105850=CARTESIAN_POINT ( 'NONE',  ( 19.03943276465977164, 0.05219959533936151252, 111.2510903946856757 ) ) ;
#105851=CARTESIAN_POINT ( 'NONE',  ( 21.55341960407619695, -5.719274019375665929, 111.0427570613523613 ) ) ;
#105852=CARTESIAN_POINT ( 'NONE',  ( -16.52544592524335698, -4.483927247898792601, 103.9594237280190185 ) ) ;
#105853=CARTESIAN_POINT ( 'NONE',  ( 10.81492255796078972, 18.62759615963270932, 99.58224293864770971 ) ) ;
#105854=CARTESIAN_POINT ( 'NONE',  ( -8.224510206698948167, 14.34966873604960824, 55.41557627198102409 ) ) ;
#105855=CARTESIAN_POINT ( 'NONE',  ( -16.51473224551082808, 9.474510206698731452, 83.33442372801899012 ) ) ;
#105856=CARTESIAN_POINT ( 'NONE',  ( -5.153800228976607833, 19.02544592524334988, 52.70942372801900433 ) ) ;
#105857=CARTESIAN_POINT ( 'NONE',  ( 21.52544592524334988, 5.823673210054432836, 61.45942372801901854 ) ) ;
#105858=CARTESIAN_POINT ( 'NONE',  ( 16.51473224551083163, -9.474510206698727899, 35.83442372801899722 ) ) ;
#105859=CARTESIAN_POINT ( 'NONE',  ( 8.314922557960818139, 14.29746914071049879, 99.58224293864770971 ) ) ;
#105860=CARTESIAN_POINT ( 'NONE',  ( -5.719274019375978568, 21.55341960407610458, 35.20724293864768839 ) ) ;
#105861=CARTESIAN_POINT ( 'NONE',  ( -0.05219959533910754901, -16.53943276465976808, 32.49890960531435979 ) ) ;
#105862=CARTESIAN_POINT ( 'NONE',  ( -21.53943276465977519, -0.05219959533937600094, 93.75109039468567573 ) ) ;
#105863=CARTESIAN_POINT ( 'NONE',  ( -4.483927247898782831, 16.52544592524335698, 72.70942372801901854 ) ) ;
#105864=CARTESIAN_POINT ( 'NONE',  ( 12.06949235617757843, -12.14591786802309237, 33.12390960531435979 ) ) ;
#105865=CARTESIAN_POINT ( 'NONE',  ( 21.52544592524334988, 5.823673210054432836, 56.45942372801902565 ) ) ;
#105866=CARTESIAN_POINT ( 'NONE',  ( -5.823673210054431948, 21.52544592524334988, 72.70942372801901854 ) ) ;
#105867=CARTESIAN_POINT ( 'NONE',  ( 10.81492255796078972, 18.62759615963270932, 64.58224293864769550 ) ) ;
#105869=CARTESIAN_POINT ( 'NONE',  ( -13.97604488694527625, -13.89961937509977652, 26.87390960531434558 ) ) ;
#105870=CARTESIAN_POINT ( 'NONE',  ( 21.53943276465977519, 0.05219959533937863772, 46.25109039468567573 ) ) ;
#105871=CARTESIAN_POINT ( 'NONE',  ( -9.564922557960796823, -16.46253265017161027, 22.08224293864768839 ) ) ;
#105872=CARTESIAN_POINT ( 'NONE',  ( -9.474510206698964154, 16.51473224551069663, 35.41557627198102409 ) ) ;
#105873=CARTESIAN_POINT ( 'NONE',  ( 16.53943276465976808, -0.05219959533910856209, 83.74890960531435269 ) ) ;
#105874=CARTESIAN_POINT ( 'NONE',  ( 19.02544592524343514, -5.153800228976328945, 83.54057627198100988 ) ) ;
#105875=CARTESIAN_POINT ( 'NONE',  ( 14.34966873604960469, 8.224510206698951720, 24.16557627198103120 ) ) ;
#105876=CARTESIAN_POINT ( 'NONE',  ( 14.34966873604960469, 8.224510206698951720, 99.16557627198100988 ) ) ;
#105877=CARTESIAN_POINT ( 'NONE',  ( -15.72974639402197994, 15.80617190586746368, 65.62390960531436690 ) ) ;
#105878=CARTESIAN_POINT ( 'NONE',  ( 15.72974639402199770, -15.80617190586745480, 103.1239096053143811 ) ) ;
#105879=CARTESIAN_POINT ( 'NONE',  ( -16.46253265017160317, 9.564922557960807481, 110.8322429386476955 ) ) ;
#105880=CARTESIAN_POINT ( 'NONE',  ( -13.89961937509977652, 13.97604488694528158, 65.62390960531436690 ) ) ;
#105881=CARTESIAN_POINT ( 'NONE',  ( 5.049401038297881783, 19.05341960407617563, 107.2927570613523187 ) ) ;
#105882=CARTESIAN_POINT ( 'NONE',  ( -10.81492255796078084, -18.62759615963271287, 57.08224293864769550 ) ) ;
#105883=CARTESIAN_POINT ( 'NONE',  ( 10.81492255796106328, -18.62759615963255655, 85.41775706135236135 ) ) ;
#105884=CARTESIAN_POINT ( 'NONE',  ( 5.049401038298161559, -19.05341960407611168, 72.70724293864768129 ) ) ;
#105885=CARTESIAN_POINT ( 'NONE',  ( 13.97604488694527802, 13.89961937509977652, 94.37390960531436690 ) ) ;
#105886=CARTESIAN_POINT ( 'NONE',  ( -8.314922557961024197, 14.29746914071037800, 72.91775706135234714 ) ) ;
#105887=CARTESIAN_POINT ( 'NONE',  ( 15.80617190586769283, -15.72974639402175789, 60.62609039468567573 ) ) ;
#105888=CARTESIAN_POINT ( 'NONE',  ( -5.823673210054431948, 21.52544592524334988, 102.7094237280190185 ) ) ;
#105889=CARTESIAN_POINT ( 'NONE',  ( 0.05219959533907565091, 21.53943276465977519, 109.9989096053143527 ) ) ;
#105890=CARTESIAN_POINT ( 'NONE',  ( 5.719274019375991003, -21.55341960407610458, 77.70724293864770971 ) ) ;
#105891=CARTESIAN_POINT ( 'NONE',  ( 19.03943276465977164, 0.05219959533936151252, 51.25109039468567573 ) ) ;
#105892=CARTESIAN_POINT ( 'NONE',  ( -5.823673210054116645, -21.52544592524344225, 37.29057627198102409 ) ) ;
#105893=CARTESIAN_POINT ( 'NONE',  ( 16.51473224551069308, 9.474510206698969483, 79.16557627198103830 ) ) ;
#105894=CARTESIAN_POINT ( 'NONE',  ( 0.05219959533910956823, 16.53943276465976808, 34.99890960531435979 ) ) ;
#105897=CARTESIAN_POINT ( 'NONE',  ( 13.89961937509957401, 13.97604488694547697, 91.87609039468567573 ) ) ;
#105898=CARTESIAN_POINT ( 'NONE',  ( 10.81492255796078972, 18.62759615963270932, 69.58224293864769550 ) ) ;
#105899=CARTESIAN_POINT ( 'NONE',  ( -4.483927247898539470, -16.52544592524342804, 52.29057627198102409 ) ) ;
#105900=CARTESIAN_POINT ( 'NONE',  ( 8.314922557961029526, -14.29746914071037800, 35.41775706135234003 ) ) ;
#105901=CARTESIAN_POINT ( 'NONE',  ( 19.03943276465977164, -0.05219959533909143690, 43.74890960531435979 ) ) ;
#105902=CARTESIAN_POINT ( 'NONE',  ( -21.52544592524343514, 5.823673210054127303, 116.0405762719810383 ) ) ;
#105903=CARTESIAN_POINT ( 'NONE',  ( -9.474510206698720793, -16.51473224551083518, 79.58442372801899012 ) ) ;
#105904=CARTESIAN_POINT ( 'NONE',  ( -16.46253265017160317, 9.564922557960807481, 85.83224293864769550 ) ) ;
#105905=CARTESIAN_POINT ( 'NONE',  ( -12.06949235617756955, 12.14591786802309770, 85.62390960531436690 ) ) ;
#105906=CARTESIAN_POINT ( 'NONE',  ( -16.46253265017160317, 9.564922557960807481, 65.83224293864769550 ) ) ;
#105907=CARTESIAN_POINT ( 'NONE',  ( 14.34966873604960469, 8.224510206698951720, 69.16557627198102409 ) ) ;
#105908=CARTESIAN_POINT ( 'NONE',  ( 19.03943276465977164, -0.05219959533909143690, 38.74890960531436690 ) ) ;
#105910=CARTESIAN_POINT ( 'NONE',  ( 12.06949235617757843, -12.14591786802309237, 43.12390960531435269 ) ) ;
#105911=CARTESIAN_POINT ( 'NONE',  ( -16.51473224551069308, -9.474510206698971260, 91.66557627198103830 ) ) ;
#105913=CARTESIAN_POINT ( 'NONE',  ( 16.46253265017146816, 9.564922557961045513, 46.66775706135233293 ) ) ;
#105914=CARTESIAN_POINT ( 'NONE',  ( 8.314922557961029526, -14.29746914071037800, 55.41775706135234714 ) ) ;
#105915=CARTESIAN_POINT ( 'NONE',  ( 18.62759615963271287, -10.81492255796078972, 73.33224293864769550 ) ) ;
#105916=CARTESIAN_POINT ( 'NONE',  ( -16.51473224551082808, 9.474510206698731452, 43.33442372801900433 ) ) ;
#105917=CARTESIAN_POINT ( 'NONE',  ( 13.97604488694527802, 13.89961937509977652, 94.37390960531436690 ) ) ;
#105918=CARTESIAN_POINT ( 'NONE',  ( -17.50000000000000355, 5.068104630630384300, 115.7281840534003408 ) ) ;
#105919=CARTESIAN_POINT ( 'NONE',  ( 0.05219959533907565091, 21.53943276465977519, 29.99890960531435979 ) ) ;
#105921=CARTESIAN_POINT ( 'NONE',  ( 13.89961937509977652, -13.97604488694527269, 63.12390960531435979 ) ) ;
#105922=CARTESIAN_POINT ( 'NONE',  ( -18.67979575497193778, 10.72451020669871902, 48.33442372801902565 ) ) ;
#105923=CARTESIAN_POINT ( 'NONE',  ( 19.02544592524343514, -5.153800228976328945, 23.54057627198102054 ) ) ;
#105924=CARTESIAN_POINT ( 'NONE',  ( -15.72974639402176322, -15.80617190586768395, 19.37609039468568639 ) ) ;
#105925=CARTESIAN_POINT ( 'NONE',  ( -9.474510206698964154, 16.51473224551069663, 90.41557627198103830 ) ) ;
#105927=CARTESIAN_POINT ( 'NONE',  ( -18.67979575497193778, 10.72451020669871902, 33.33442372801900433 ) ) ;
#105928=ORIENTED_EDGE ( 'NONE', *, *, #134324, .T. ) ;
#105929=CARTESIAN_POINT ( 'NONE',  ( -13.89961937509977652, 13.97604488694528158, 105.6239096053143527 ) ) ;
#105931=CARTESIAN_POINT ( 'NONE',  ( 5.823673210054125526, 21.52544592524343514, 109.7905762719810383 ) ) ;
#105932=CARTESIAN_POINT ( 'NONE',  ( -13.97604488694527625, -13.89961937509977652, 51.87390960531436690 ) ) ;
#105933=CARTESIAN_POINT ( 'NONE',  ( 16.53943276465976808, 0.05219959533934440121, 31.25109039468568639 ) ) ;
#105935=CARTESIAN_POINT ( 'NONE',  ( -21.53943276465977519, -0.05219959533937600094, 98.75109039468568994 ) ) ;
#105936=CARTESIAN_POINT ( 'NONE',  ( -16.46253265017160317, 9.564922557960807481, 35.83224293864768839 ) ) ;
#105937=CARTESIAN_POINT ( 'NONE',  ( 15.80617190586769283, -15.72974639402175789, 100.6260903946857184 ) ) ;
#105938=CARTESIAN_POINT ( 'NONE',  ( 0.05219959533909260263, 19.03943276465977164, 94.99890960531436690 ) ) ;
#105939=CARTESIAN_POINT ( 'NONE',  ( -5.719274019375665041, -21.55341960407619695, 59.79275706135234714 ) ) ;
#105941=CARTESIAN_POINT ( 'NONE',  ( 5.153800228976335163, 19.02544592524342804, 104.7905762719809957 ) ) ;
#105942=CARTESIAN_POINT ( 'NONE',  ( -22.00000000000000000, -1.163414459189985801E-14, 95.00000000000000000 ) ) ;
#105943=CARTESIAN_POINT ( 'NONE',  ( 14.29746914071037800, 8.314922557961029526, 56.66775706135235424 ) ) ;
#105944=CARTESIAN_POINT ( 'NONE',  ( 12.14591786802327356, -12.06949235617739191, 70.62609039468567573 ) ) ;
#105945=CARTESIAN_POINT ( 'NONE',  ( -21.53943276465977519, -0.05219959533937600094, 53.75109039468568994 ) ) ;
#105946=CARTESIAN_POINT ( 'NONE',  ( -21.53943276465977519, -0.05219959533937600094, 88.75109039468567573 ) ) ;
#105948=CARTESIAN_POINT ( 'NONE',  ( 16.53943276465976808, 0.05219959533934440121, 31.25109039468568639 ) ) ;
#105949=CARTESIAN_POINT ( 'NONE',  ( 5.153800228976335163, 19.02544592524342804, 79.79057627198102409 ) ) ;
#105950=CARTESIAN_POINT ( 'NONE',  ( 13.89961937509977652, -13.97604488694527269, 103.1239096053143527 ) ) ;
#105952=CARTESIAN_POINT ( 'NONE',  ( -13.89961937509977652, 13.97604488694528158, 110.6239096053143243 ) ) ;
#105953=CARTESIAN_POINT ( 'NONE',  ( 16.51473224551069308, 9.474510206698969483, 24.16557627198102765 ) ) ;
#105954=CARTESIAN_POINT ( 'NONE',  ( -0.05219959533907301413, -21.53943276465977519, 32.49890960531435979 ) ) ;
#105955=CARTESIAN_POINT ( 'NONE',  ( 0.05219959533934541429, -16.53943276465976808, 90.00109039468567573 ) ) ;
#105956=CARTESIAN_POINT ( 'NONE',  ( -8.224510206698948167, 14.34966873604960824, 65.41557627198102409 ) ) ;
#105957=CARTESIAN_POINT ( 'NONE',  ( -13.97604488694527625, -13.89961937509977652, 66.87390960531436690 ) ) ;
#105958=CARTESIAN_POINT ( 'NONE',  ( 15.72974639402176855, 15.80617190586768217, 96.87609039468568994 ) ) ;
#105959=CARTESIAN_POINT ( 'NONE',  ( 17.47980958864297918, 5.499999999999998224, 21.71653220162190934 ) ) ;
#105960=CARTESIAN_POINT ( 'NONE',  ( 5.153800228976615827, -19.02544592524334988, 105.2094237280190185 ) ) ;
#105961=CARTESIAN_POINT ( 'NONE',  ( -16.52544592524342804, 4.483927247898546575, 81.04057627198102409 ) ) ;
#105962=CARTESIAN_POINT ( 'NONE',  ( -0.05219959533937732626, 21.53943276465977519, 32.50109039468568284 ) ) ;
#105963=CARTESIAN_POINT ( 'NONE',  ( -5.719274019375978568, 21.55341960407610458, 70.20724293864769550 ) ) ;
#105964=CARTESIAN_POINT ( 'NONE',  ( 16.46253265017146816, 9.564922557961045513, 36.66775706135233293 ) ) ;
#105966=CARTESIAN_POINT ( 'NONE',  ( -13.89961937509977652, 13.97604488694528158, 80.62390960531436690 ) ) ;
#105967=CARTESIAN_POINT ( 'NONE',  ( -8.224510206698948167, 14.34966873604960824, 55.41557627198102409 ) ) ;
#105968=CARTESIAN_POINT ( 'NONE',  ( -14.29746914071049879, 8.314922557960819915, 40.83224293864769550 ) ) ;
#105969=CARTESIAN_POINT ( 'NONE',  ( -8.224510206698735004, -14.34966873604973081, 104.5844237280190185 ) ) ;
#105970=CARTESIAN_POINT ( 'NONE',  ( -19.02544592524334988, -5.153800228976617603, 68.95942372801896170 ) ) ;
#105971=CARTESIAN_POINT ( 'NONE',  ( -18.22780087662122028, 5.500000000000031086, 78.51540105326107266 ) ) ;
#105972=CARTESIAN_POINT ( 'NONE',  ( 16.51473224551069308, 9.474510206698969483, 109.1655762719810383 ) ) ;
#105973=CARTESIAN_POINT ( 'NONE',  ( -12.06949235617756955, 12.14591786802309770, 75.62390960531439532 ) ) ;
#105974=CARTESIAN_POINT ( 'NONE',  ( -17.49999999999999645, 5.499999999999992895, 58.71769037696435589 ) ) ;
#105975=CARTESIAN_POINT ( 'NONE',  ( -19.02544592524342804, 5.153800228976336051, 26.04057627198103120 ) ) ;
#105976=CARTESIAN_POINT ( 'NONE',  ( -21.53943276465977519, 0.05219959533907696930, 31.24890960531435979 ) ) ;
#105977=CARTESIAN_POINT ( 'NONE',  ( -0.05219959533907301413, -21.53943276465977519, 72.49890960531435269 ) ) ;
#105978=CARTESIAN_POINT ( 'NONE',  ( 8.314922557960818139, 14.29746914071049879, 109.5822429386476955 ) ) ;
#105979=CARTESIAN_POINT ( 'NONE',  ( 14.29746914071037800, 8.314922557961029526, 71.66775706135234714 ) ) ;
#105980=CARTESIAN_POINT ( 'NONE',  ( -13.89961937509977652, 13.97604488694528158, 45.62390960531433848 ) ) ;
#105981=CARTESIAN_POINT ( 'NONE',  ( 15.72974639402176855, 15.80617190586768217, 56.87609039468568994 ) ) ;
#105982=CARTESIAN_POINT ( 'NONE',  ( -16.53943276465976808, 0.05219959533911058130, 91.24890960531436690 ) ) ;
#105986=CARTESIAN_POINT ( 'NONE',  ( -10.81492255796078084, -18.62759615963271287, 32.08224293864769550 ) ) ;
#105987=CARTESIAN_POINT ( 'NONE',  ( 19.50973618000807619, -5.499999999999992895, 37.50000000000000000 ) ) ;
#105988=CARTESIAN_POINT ( 'NONE',  ( 16.55341960407618274, -4.379528057220086978, 56.04275706135235424 ) ) ;
#105989=CARTESIAN_POINT ( 'NONE',  ( 16.52544592524342804, -4.483927247898539470, 38.54057627198103120 ) ) ;
#105990=CARTESIAN_POINT ( 'NONE',  ( -15.80617190586745835, -15.72974639402198527, 71.87390960531438111 ) ) ;
#105991=CARTESIAN_POINT ( 'NONE',  ( 10.81492255796078972, 18.62759615963270932, 64.58224293864769550 ) ) ;
#105993=CARTESIAN_POINT ( 'NONE',  ( -13.97604488694547697, 13.89961937509957934, 78.12609039468567573 ) ) ;
#105994=CARTESIAN_POINT ( 'NONE',  ( -19.05341960407611168, -5.049401038298163336, 106.4572429386476955 ) ) ;
#105995=CARTESIAN_POINT ( 'NONE',  ( -16.46253265017160317, 9.564922557960807481, 45.83224293864769550 ) ) ;
#105996=CARTESIAN_POINT ( 'NONE',  ( 9.564922557960805705, 16.46253265017160317, 24.58224293864769194 ) ) ;
#106000=CARTESIAN_POINT ( 'NONE',  ( 8.314922557961029526, -14.29746914071037800, 75.41775706135233293 ) ) ;
#106001=CARTESIAN_POINT ( 'NONE',  ( 0.05219959533907565091, 21.53943276465977519, 99.99890960531436690 ) ) ;
#106002=CARTESIAN_POINT ( 'NONE',  ( -19.03943276465977164, 0.05219959533909376836, 51.24890960531436690 ) ) ;
#106003=CARTESIAN_POINT ( 'NONE',  ( -0.05219959533937732626, 21.53943276465977519, 42.50109039468567573 ) ) ;
#106004=CARTESIAN_POINT ( 'NONE',  ( 5.049401038298161559, -19.05341960407611168, 102.7072429386476955 ) ) ;
#106005=CARTESIAN_POINT ( 'NONE',  ( 9.564922557960805705, 16.46253265017160317, 114.5822429386476955 ) ) ;
#106006=EDGE_CURVE ( 'NONE', #190052, #106384, #152451, .T. ) ;
#106008=CARTESIAN_POINT ( 'NONE',  ( -21.52544592524334988, -5.823673210054445271, 33.95942372801901143 ) ) ;
#106009=CARTESIAN_POINT ( 'NONE',  ( 16.46253265017160672, -9.564922557960803928, 113.3322429386476955 ) ) ;
#106010=CARTESIAN_POINT ( 'NONE',  ( 19.02544592524334988, 5.153800228976608722, 91.45942372801900433 ) ) ;
#106011=CARTESIAN_POINT ( 'NONE',  ( -5.049401038297874678, -19.05341960407617918, 34.79275706135233293 ) ) ;
#106012=CARTESIAN_POINT ( 'NONE',  ( 21.53943276465977519, -0.05219959533907433946, 103.7489096053143669 ) ) ;
#106013=CARTESIAN_POINT ( 'NONE',  ( -16.51473224551082808, 9.474510206698731452, 33.33442372801899722 ) ) ;
#106014=CARTESIAN_POINT ( 'NONE',  ( 9.474510206698729675, 16.51473224551082808, 42.08442372801900433 ) ) ;
#106015=CARTESIAN_POINT ( 'NONE',  ( 14.34966873604972726, -8.224510206698740333, 85.83442372801901854 ) ) ;
#106016=DIRECTION ( 'NONE',  ( 0.000000000000000000, -0.000000000000000000, -1.000000000000000000 ) ) ;
#106017=CARTESIAN_POINT ( 'NONE',  ( 19.02544592524343514, -5.153800228976328945, 58.54057627198102409 ) ) ;
#106018=CARTESIAN_POINT ( 'NONE',  ( 21.53943276465977519, 0.05219959533937863772, 66.25109039468567573 ) ) ;
#106019=CARTESIAN_POINT ( 'NONE',  ( -21.55341960407619339, 5.719274019375674811, 83.54275706135234714 ) ) ;
#106020=CARTESIAN_POINT ( 'NONE',  ( -18.22780087662126647, -5.499999999999827693, 53.98236817873107185 ) ) ;
#106021=CARTESIAN_POINT ( 'NONE',  ( -9.474510206698964154, 16.51473224551069663, 85.41557627198102409 ) ) ;
#106022=CARTESIAN_POINT ( 'NONE',  ( -18.62759615963255300, -10.81492255796106328, 64.16775706135234714 ) ) ;
#106023=CARTESIAN_POINT ( 'NONE',  ( -19.05341960407617563, 5.049401038297882671, 103.5427570613523329 ) ) ;
#106024=CARTESIAN_POINT ( 'NONE',  ( 5.049401038298161559, -19.05341960407611168, 67.70724293864769550 ) ) ;
#106025=CARTESIAN_POINT ( 'NONE',  ( -9.474510206698964154, 16.51473224551069663, 95.41557627198102409 ) ) ;
#106026=CARTESIAN_POINT ( 'NONE',  ( -13.97604488694527625, -13.89961937509977652, 76.87390960531433848 ) ) ;
#106028=CARTESIAN_POINT ( 'NONE',  ( 0.05219959533909260263, 19.03943276465977164, 64.99890960531436690 ) ) ;
#106029=CARTESIAN_POINT ( 'NONE',  ( 5.719274019375991003, -21.55341960407610458, 102.7072429386476955 ) ) ;
#106030=CARTESIAN_POINT ( 'NONE',  ( -14.34966873604972548, 8.224510206698743886, 93.33442372801901854 ) ) ;
#106032=CARTESIAN_POINT ( 'NONE',  ( -5.153800228976607833, 19.02544592524334988, 47.70942372801900433 ) ) ;
#106033=CARTESIAN_POINT ( 'NONE',  ( 19.02544592524343514, -5.153800228976328945, 83.54057627198100988 ) ) ;
#106034=CARTESIAN_POINT ( 'NONE',  ( -14.29746914071049879, 8.314922557960819915, 75.83224293864769550 ) ) ;
#106035=CARTESIAN_POINT ( 'NONE',  ( 16.52544592524342804, -4.483927247898539470, 113.5405762719810383 ) ) ;
#106036=CARTESIAN_POINT ( 'NONE',  ( 0.05219959533909260263, 19.03943276465977164, 109.9989096053143669 ) ) ;
#106037=CARTESIAN_POINT ( 'NONE',  ( 5.153800228976335163, 19.02544592524342804, 104.7905762719809957 ) ) ;
#106038=CARTESIAN_POINT ( 'NONE',  ( 13.89961937509978007, -13.97604488694527269, 83.12390960531438111 ) ) ;
#106039=CARTESIAN_POINT ( 'NONE',  ( 19.02544592524334988, 5.153800228976608722, 31.45942372801900433 ) ) ;
#106040=CARTESIAN_POINT ( 'NONE',  ( -8.314922557961024197, 14.29746914071037800, 92.91775706135236135 ) ) ;
#106041=CARTESIAN_POINT ( 'NONE',  ( 9.564922557960805705, 16.46253265017160317, 79.58224293864769550 ) ) ;
#106042=CARTESIAN_POINT ( 'NONE',  ( -10.72451020669870658, -18.67979575497194134, 49.58442372801901143 ) ) ;
#106043=CARTESIAN_POINT ( 'NONE',  ( 10.81492255796078972, 18.62759615963270932, 44.58224293864769550 ) ) ;
#106044=CARTESIAN_POINT ( 'NONE',  ( -10.72451020669898014, 18.67979575497178502, 115.4155762719810241 ) ) ;
#106045=CARTESIAN_POINT ( 'NONE',  ( 18.62759615963271287, -10.81492255796078972, 68.33224293864769550 ) ) ;
#106046=CARTESIAN_POINT ( 'NONE',  ( 4.379528057220339221, -16.55341960407611168, 92.70724293864770971 ) ) ;
#106047=CARTESIAN_POINT ( 'NONE',  ( -19.05341960407617563, 5.049401038297882671, 58.54275706135234003 ) ) ;
#106048=CARTESIAN_POINT ( 'NONE',  ( -19.02544592524342804, 5.153800228976336051, 31.04057627198102409 ) ) ;
#106049=CARTESIAN_POINT ( 'NONE',  ( 16.51473224551069308, 9.474510206698969483, 79.16557627198103830 ) ) ;
#106050=CARTESIAN_POINT ( 'NONE',  ( -9.474510206698964154, 16.51473224551069663, 85.41557627198102409 ) ) ;
#106052=CARTESIAN_POINT ( 'NONE',  ( 12.14591786802309770, 12.06949235617756955, 99.37390960531436690 ) ) ;
#106053=ORIENTED_EDGE ( 'NONE', *, *, #156075, .T. ) ;
#106054=CARTESIAN_POINT ( 'NONE',  ( -0.05219959533910754901, -16.53943276465976808, 32.49890960531435979 ) ) ;
#106055=CARTESIAN_POINT ( 'NONE',  ( -16.53943276465976808, -0.05219959533934237506, 28.75109039468567929 ) ) ;
#106056=CARTESIAN_POINT ( 'NONE',  ( -0.05219959533937732626, 21.53943276465977519, 97.50109039468567573 ) ) ;
#106057=CARTESIAN_POINT ( 'NONE',  ( 19.03943276465977164, -0.05219959533909143690, 98.74890960531436690 ) ) ;
#106058=CARTESIAN_POINT ( 'NONE',  ( 21.55341960407619695, -5.719274019375665929, 21.04275706135234714 ) ) ;
#106059=CARTESIAN_POINT ( 'NONE',  ( 5.049401038298161559, -19.05341960407611168, 42.70724293864767418 ) ) ;
#106060=CARTESIAN_POINT ( 'NONE',  ( 14.34966873604972726, -8.224510206698740333, 45.83442372801901854 ) ) ;
#106061=CARTESIAN_POINT ( 'NONE',  ( 19.05341960407617918, -5.049401038297876454, 106.0427570613523471 ) ) ;
#106062=CARTESIAN_POINT ( 'NONE',  ( -0.05219959533909027116, -19.03943276465977164, 32.49890960531435979 ) ) ;
#106063=CARTESIAN_POINT ( 'NONE',  ( 16.55341960407611168, 4.379528057220329451, 93.95724293864770971 ) ) ;
#106064=CARTESIAN_POINT ( 'NONE',  ( 10.72451020669898902, -18.67979575497178502, 102.9155762719810383 ) ) ;
#106065=CARTESIAN_POINT ( 'NONE',  ( -5.153800228976607833, 19.02544592524334988, 62.70942372801899722 ) ) ;
#106067=CARTESIAN_POINT ( 'NONE',  ( 10.81492255796106328, -18.62759615963255655, 25.41775706135235779 ) ) ;
#106068=CARTESIAN_POINT ( 'NONE',  ( -0.05219959533909027116, -19.03943276465977164, 22.49890960531436690 ) ) ;
#106069=CARTESIAN_POINT ( 'NONE',  ( -19.03943276465977164, 0.05219959533909376836, 91.24890960531436690 ) ) ;
#106070=CARTESIAN_POINT ( 'NONE',  ( -19.03943276465977164, 0.05219959533909376836, 91.24890960531436690 ) ) ;
#106071=CARTESIAN_POINT ( 'NONE',  ( -10.72451020669870658, -18.67979575497194134, 29.58442372801901854 ) ) ;
#106072=CARTESIAN_POINT ( 'NONE',  ( 14.29746914071049879, -8.314922557960816363, 78.33224293864770971 ) ) ;
#106073=CARTESIAN_POINT ( 'NONE',  ( 16.51473224551069308, 9.474510206698969483, 79.16557627198103830 ) ) ;
#106074=CARTESIAN_POINT ( 'NONE',  ( -0.05219959533936034679, 19.03943276465977164, 22.50109039468566152 ) ) ;
#106075=CARTESIAN_POINT ( 'NONE',  ( 8.314922557961029526, -14.29746914071037800, 55.41775706135234714 ) ) ;
#106076=CARTESIAN_POINT ( 'NONE',  ( -9.564922557961040184, 16.46253265017147172, 52.91775706135233293 ) ) ;
#106077=CARTESIAN_POINT ( 'NONE',  ( 10.81492255796106328, -18.62759615963255655, 60.41775706135235424 ) ) ;
#106078=AXIS2_PLACEMENT_3D ( 'NONE', #109962, #78619, #136336 ) ;
#106079=CARTESIAN_POINT ( 'NONE',  ( -14.34966873604972548, 8.224510206698743886, 23.33442372801901499 ) ) ;
#106080=CARTESIAN_POINT ( 'NONE',  ( 13.89961937509977652, -13.97604488694527269, 63.12390960531435979 ) ) ;
#106081=CARTESIAN_POINT ( 'NONE',  ( 13.89961937509957401, 13.97604488694547697, 96.87609039468566152 ) ) ;
#106082=CARTESIAN_POINT ( 'NONE',  ( 16.53943276465976808, 0.05219959533934440121, 66.25109039468567573 ) ) ;
#106083=CARTESIAN_POINT ( 'NONE',  ( -21.55341960407619339, 5.719274019375674811, 103.5427570613523613 ) ) ;
#106084=CARTESIAN_POINT ( 'NONE',  ( 5.049401038297881783, 19.05341960407617563, 82.29275706135229029 ) ) ;
#106085=CARTESIAN_POINT ( 'NONE',  ( 5.153800228976335163, 19.02544592524342804, 49.79057627198100988 ) ) ;
#106086=CARTESIAN_POINT ( 'NONE',  ( -15.72974639402197994, 15.80617190586746368, 65.62390960531436690 ) ) ;
#106087=CARTESIAN_POINT ( 'NONE',  ( -4.379528057220328563, 16.55341960407611168, 75.20724293864769550 ) ) ;
#106088=CARTESIAN_POINT ( 'NONE',  ( 13.89961937509957401, 13.97604488694547697, 71.87609039468567573 ) ) ;
#106089=CARTESIAN_POINT ( 'NONE',  ( 17.50000000000000000, -5.500000000000000888, 120.0000000000000142 ) ) ;
#106090=CARTESIAN_POINT ( 'NONE',  ( -5.153800228976607833, 19.02544592524334988, 42.70942372801901143 ) ) ;
#106091=CARTESIAN_POINT ( 'NONE',  ( -12.06949235617739369, -12.14591786802326823, 109.3760903946857042 ) ) ;
#106092=CARTESIAN_POINT ( 'NONE',  ( 4.483927247898545687, 16.52544592524342804, 69.79057627198102409 ) ) ;
#106093=CARTESIAN_POINT ( 'NONE',  ( -21.55341960407619339, 5.719274019375674811, 103.5427570613523613 ) ) ;
#106095=CARTESIAN_POINT ( 'NONE',  ( -18.67979575497178146, -10.72451020669898902, 101.6655762719810383 ) ) ;
#106096=CARTESIAN_POINT ( 'NONE',  ( 19.03943276465977164, -0.05219959533909143690, 68.74890960531436690 ) ) ;
#106097=CARTESIAN_POINT ( 'NONE',  ( 10.72451020669871369, 18.67979575497193778, 77.08442372801901854 ) ) ;
#106098=CARTESIAN_POINT ( 'NONE',  ( 19.03943276465977164, -0.05219959533909143690, 63.74890960531435979 ) ) ;
#106100=CARTESIAN_POINT ( 'NONE',  ( 16.53943276465976808, -0.05219959533910856209, 113.7489096053143527 ) ) ;
#106101=CARTESIAN_POINT ( 'NONE',  ( -0.05219959533907301413, -21.53943276465977519, 27.49890960531435269 ) ) ;
#106102=CARTESIAN_POINT ( 'NONE',  ( -8.314922557960811034, -14.29746914071050412, 62.08224293864769550 ) ) ;
#106103=CARTESIAN_POINT ( 'NONE',  ( -19.02544592524342804, 5.153800228976336051, 46.04057627198101699 ) ) ;
#106104=CARTESIAN_POINT ( 'NONE',  ( -8.224510206698948167, 14.34966873604960824, 95.41557627198102409 ) ) ;
#106105=CARTESIAN_POINT ( 'NONE',  ( -21.53943276465977519, 0.05219959533907696930, 111.2489096053143669 ) ) ;
#106106=CARTESIAN_POINT ( 'NONE',  ( 18.62759615963255655, 10.81492255796105972, 46.66775706135234714 ) ) ;
#106107=CARTESIAN_POINT ( 'NONE',  ( 0.05219959533909260263, 19.03943276465977164, 24.99890960531435269 ) ) ;
#106108=CARTESIAN_POINT ( 'NONE',  ( -16.55341960407617563, 4.379528057220093196, 53.54275706135234714 ) ) ;
#106110=CARTESIAN_POINT ( 'NONE',  ( -5.823673210054116645, -21.52544592524344225, 102.2905762719810383 ) ) ;
#106111=CARTESIAN_POINT ( 'NONE',  ( -15.80617190586745835, -15.72974639402198527, 96.87390960531436690 ) ) ;
#106112=CARTESIAN_POINT ( 'NONE',  ( 0.05219959533936267826, -19.03943276465977164, 20.00109039468567218 ) ) ;
#106113=CARTESIAN_POINT ( 'NONE',  ( -19.05341960407611168, -5.049401038298163336, 56.45724293864768129 ) ) ;
#106114=CARTESIAN_POINT ( 'NONE',  ( -5.049401038298153566, 19.05341960407611168, 110.2072429386476671 ) ) ;
#106115=CARTESIAN_POINT ( 'NONE',  ( -21.53943276465977519, -0.05219959533937600094, 53.75109039468568994 ) ) ;
#106116=CARTESIAN_POINT ( 'NONE',  ( 21.55341960407610458, 5.719274019375980345, 43.95724293864769550 ) ) ;
#106117=CARTESIAN_POINT ( 'NONE',  ( -8.224510206698948167, 14.34966873604960824, 25.41557627198103120 ) ) ;
#106118=CARTESIAN_POINT ( 'NONE',  ( -21.55341960407619339, 5.719274019375674811, 63.54275706135234003 ) ) ;
#106119=CARTESIAN_POINT ( 'NONE',  ( -18.62759615963255300, -10.81492255796106328, 99.16775706135234714 ) ) ;
#106120=CARTESIAN_POINT ( 'NONE',  ( 19.02544592524334988, 5.153800228976608722, 46.45942372801899012 ) ) ;
#106121=CARTESIAN_POINT ( 'NONE',  ( 8.224510206698742110, 14.34966873604972548, 102.0844237280190185 ) ) ;
#106122=CARTESIAN_POINT ( 'NONE',  ( -21.52544592524334988, -5.823673210054445271, 48.95942372801902565 ) ) ;
#106123=CARTESIAN_POINT ( 'NONE',  ( -5.153800228976328057, -19.02544592524343514, 57.29057627198103120 ) ) ;
#106124=CARTESIAN_POINT ( 'NONE',  ( -13.89961937509957401, -13.97604488694547875, 24.37609039468565442 ) ) ;
#106125=CARTESIAN_POINT ( 'NONE',  ( 21.55341960407610458, 5.719274019375980345, 23.95724293864769550 ) ) ;
#106127=CARTESIAN_POINT ( 'NONE',  ( 21.55341960407619695, -5.719274019375665929, 26.04275706135235779 ) ) ;
#106128=CARTESIAN_POINT ( 'NONE',  ( 18.62759615963271287, -10.81492255796078972, 83.33224293864769550 ) ) ;
#106129=CARTESIAN_POINT ( 'NONE',  ( -12.14591786802326823, 12.06949235617739902, 38.12609039468567573 ) ) ;
#106130=CARTESIAN_POINT ( 'NONE',  ( 17.49999999999999289, -4.601506711240598513, 36.47308481467552355 ) ) ;
#106131=CARTESIAN_POINT ( 'NONE',  ( -5.719274019375978568, 21.55341960407610458, 85.20724293864770971 ) ) ;
#106132=CARTESIAN_POINT ( 'NONE',  ( 14.34966873604972726, -8.224510206698740333, 60.83442372801901854 ) ) ;
#106133=CARTESIAN_POINT ( 'NONE',  ( -14.34966873604960291, -8.224510206698953496, 71.66557627198100988 ) ) ;
#106135=CARTESIAN_POINT ( 'NONE',  ( -16.51473224551082808, 9.474510206698731452, 108.3344237280190043 ) ) ;
#106137=CARTESIAN_POINT ( 'NONE',  ( 10.81492255796078972, 18.62759615963270932, 34.58224293864770260 ) ) ;
#106139=CARTESIAN_POINT ( 'NONE',  ( 14.34966873604972726, -8.224510206698740333, 45.83442372801901854 ) ) ;
#106140=CARTESIAN_POINT ( 'NONE',  ( -5.719274019375665041, -21.55341960407619695, 19.79275706135235069 ) ) ;
#106142=CARTESIAN_POINT ( 'NONE',  ( 0.05219959533907565091, 21.53943276465977519, 29.99890960531435979 ) ) ;
#106143=CARTESIAN_POINT ( 'NONE',  ( -16.52544592524335698, -4.483927247898792601, 68.95942372801901854 ) ) ;
#106144=CARTESIAN_POINT ( 'NONE',  ( -19.02544592524342804, 5.153800228976336051, 91.04057627198100988 ) ) ;
#106145=CARTESIAN_POINT ( 'NONE',  ( 10.81492255796106328, -18.62759615963255655, 50.41775706135235424 ) ) ;
#106146=CARTESIAN_POINT ( 'NONE',  ( 5.049401038298161559, -19.05341960407611168, 27.70724293864769550 ) ) ;
#106147=CARTESIAN_POINT ( 'NONE',  ( -9.474510206698964154, 16.51473224551069663, 115.4155762719810241 ) ) ;
#106149=CARTESIAN_POINT ( 'NONE',  ( -19.02544592524334988, -5.153800228976617603, 38.95942372801900433 ) ) ;
#106150=CARTESIAN_POINT ( 'NONE',  ( 14.29746914071037800, 8.314922557961029526, 46.66775706135234714 ) ) ;
#106151=CARTESIAN_POINT ( 'NONE',  ( -18.67979575497178146, -10.72451020669898902, 21.66557627198102409 ) ) ;
#106152=CARTESIAN_POINT ( 'NONE',  ( 16.51473224551069308, 9.474510206698969483, 79.16557627198103830 ) ) ;
#106153=CARTESIAN_POINT ( 'NONE',  ( -14.29746914071037622, -8.314922557961029526, 94.16775706135237556 ) ) ;
#106155=CARTESIAN_POINT ( 'NONE',  ( -12.14591786802309592, -12.06949235617757132, 96.87390960531436690 ) ) ;
#106156=CARTESIAN_POINT ( 'NONE',  ( 21.55341960407610458, 5.719274019375980345, 38.95724293864768839 ) ) ;
#106157=CARTESIAN_POINT ( 'NONE',  ( -19.03943276465977164, 0.05219959533909376836, 31.24890960531435979 ) ) ;
#106158=CARTESIAN_POINT ( 'NONE',  ( -12.06949235617739369, -12.14591786802326823, 69.37609039468567573 ) ) ;
#106159=CARTESIAN_POINT ( 'NONE',  ( 15.80617190586746368, 15.72974639402197994, 114.3739096053143527 ) ) ;
#106160=CARTESIAN_POINT ( 'NONE',  ( -9.474510206698720793, -16.51473224551083518, 79.58442372801899012 ) ) ;
#106161=CARTESIAN_POINT ( 'NONE',  ( 9.564922557960805705, 16.46253265017160317, 44.58224293864769550 ) ) ;
#106162=CARTESIAN_POINT ( 'NONE',  ( -15.80617190586745835, -15.72974639402198527, 66.87390960531436690 ) ) ;
#106163=CARTESIAN_POINT ( 'NONE',  ( -16.46253265017160317, 9.564922557960807481, 115.8322429386477097 ) ) ;
#106164=CARTESIAN_POINT ( 'NONE',  ( -5.719274019375665041, -21.55341960407619695, 89.79275706135236135 ) ) ;
#106165=CARTESIAN_POINT ( 'NONE',  ( -9.564922557960796823, -16.46253265017161027, 62.08224293864769550 ) ) ;
#106166=CARTESIAN_POINT ( 'NONE',  ( -16.52544592524335698, -4.483927247898792601, 48.95942372801902565 ) ) ;
#106167=CARTESIAN_POINT ( 'NONE',  ( -9.474510206698964154, 16.51473224551069663, 60.41557627198102409 ) ) ;
#106168=CARTESIAN_POINT ( 'NONE',  ( -10.81492255796105439, 18.62759615963255655, 77.91775706135231871 ) ) ;
#106169=CARTESIAN_POINT ( 'NONE',  ( 9.474510206698729675, 16.51473224551082808, 42.08442372801900433 ) ) ;
#106170=CARTESIAN_POINT ( 'NONE',  ( -5.049401038297874678, -19.05341960407617918, 49.79275706135231871 ) ) ;
#106171=CARTESIAN_POINT ( 'NONE',  ( -10.72451020669870658, -18.67979575497194134, 54.58442372801901143 ) ) ;
#106172=CARTESIAN_POINT ( 'NONE',  ( -17.49999999999999645, -5.500000000000000888, 120.0000000000000142 ) ) ;
#106173=CARTESIAN_POINT ( 'NONE',  ( 9.474510206698729675, 16.51473224551082808, 47.08442372801900433 ) ) ;
#106174=CARTESIAN_POINT ( 'NONE',  ( -16.51473224551069308, -9.474510206698971260, 101.6655762719810241 ) ) ;
#106175=CARTESIAN_POINT ( 'NONE',  ( -13.97604488694527625, -13.89961937509977652, 71.87390960531433848 ) ) ;
#106176=CARTESIAN_POINT ( 'NONE',  ( 14.29746914071049879, -8.314922557960816363, 23.33224293864769194 ) ) ;
#106177=CARTESIAN_POINT ( 'NONE',  ( 10.81492255796078972, 18.62759615963270932, 29.58224293864769905 ) ) ;
#106178=CARTESIAN_POINT ( 'NONE',  ( 15.72974639402176855, 15.80617190586768217, 96.87609039468568994 ) ) ;
#106180=CARTESIAN_POINT ( 'NONE',  ( -18.22780087662122028, 5.500000000000031086, 38.51540105326107266 ) ) ;
#106181=CARTESIAN_POINT ( 'NONE',  ( 15.80617190586769283, -15.72974639402175789, 95.62609039468568994 ) ) ;
#106183=CARTESIAN_POINT ( 'NONE',  ( -13.89961937509977652, 13.97604488694528158, 40.62390960531435979 ) ) ;
#106186=CARTESIAN_POINT ( 'NONE',  ( -4.379528057220086978, -16.55341960407618274, 44.79275706135234714 ) ) ;
#106187=CARTESIAN_POINT ( 'NONE',  ( 5.823673210054125526, 21.52544592524343514, 64.79057627198103830 ) ) ;
#106188=CARTESIAN_POINT ( 'NONE',  ( 4.483927247898545687, 16.52544592524342804, 44.79057627198103120 ) ) ;
#106189=CARTESIAN_POINT ( 'NONE',  ( 14.29746914071049879, -8.314922557960816363, 108.3322429386477097 ) ) ;
#106190=CARTESIAN_POINT ( 'NONE',  ( 9.564922557960805705, 16.46253265017160317, 109.5822429386476955 ) ) ;
#106191=CARTESIAN_POINT ( 'NONE',  ( 15.80617190586769283, -15.72974639402175789, 30.62609039468567929 ) ) ;
#106192=CARTESIAN_POINT ( 'NONE',  ( 9.474510206698729675, 16.51473224551082808, 42.08442372801900433 ) ) ;
#106193=CARTESIAN_POINT ( 'NONE',  ( -16.55341960407611168, -4.379528057220339221, 111.4572429386476813 ) ) ;
#106194=CARTESIAN_POINT ( 'NONE',  ( -18.62759615963255300, -10.81492255796106328, 69.16775706135234714 ) ) ;
#106195=CARTESIAN_POINT ( 'NONE',  ( 17.40805194822031865, -6.112264579159335298, 33.33371272510612471 ) ) ;
#106196=CARTESIAN_POINT ( 'NONE',  ( 12.06949235617757843, -12.14591786802309237, 23.12390960531436335 ) ) ;
#106198=CARTESIAN_POINT ( 'NONE',  ( -10.81492255796078084, -18.62759615963271287, 22.08224293864769194 ) ) ;
#106199=CARTESIAN_POINT ( 'NONE',  ( 14.34966873604960469, 8.224510206698951720, 89.16557627198102409 ) ) ;
#106200=CARTESIAN_POINT ( 'NONE',  ( -17.60691670004650433, -5.500000000000071054, 39.13333313366439370 ) ) ;
#106201=CARTESIAN_POINT ( 'NONE',  ( -5.049401038298153566, 19.05341960407611168, 80.20724293864769550 ) ) ;
#106202=CARTESIAN_POINT ( 'NONE',  ( 8.224510206698953496, -14.34966873604960469, 77.91557627198102409 ) ) ;
#106203=CARTESIAN_POINT ( 'NONE',  ( 16.46253265017146816, 9.564922557961045513, 106.6677570613523471 ) ) ;
#106204=CARTESIAN_POINT ( 'NONE',  ( -10.81492255796078084, -18.62759615963271287, 52.08224293864768839 ) ) ;
#106206=CARTESIAN_POINT ( 'NONE',  ( -12.06949235617756955, 12.14591786802309770, 115.6239096053143669 ) ) ;
#106207=CARTESIAN_POINT ( 'NONE',  ( 19.03943276465977164, -0.05219959533909143690, 78.74890960531436690 ) ) ;
#106208=CARTESIAN_POINT ( 'NONE',  ( 18.62759615963271287, -10.81492255796078972, 73.33224293864769550 ) ) ;
#106209=CARTESIAN_POINT ( 'NONE',  ( 14.29746914071037800, 8.314922557961029526, 106.6677570613523756 ) ) ;
#106210=CARTESIAN_POINT ( 'NONE',  ( -5.049401038298153566, 19.05341960407611168, 90.20724293864766707 ) ) ;
#106211=CARTESIAN_POINT ( 'NONE',  ( -13.97604488694547697, 13.89961937509957934, 73.12609039468568994 ) ) ;
#106212=CARTESIAN_POINT ( 'NONE',  ( -21.53943276465977519, -0.05219959533937600094, 93.75109039468567573 ) ) ;
#106213=CARTESIAN_POINT ( 'NONE',  ( 18.62759615963271287, -10.81492255796078972, 68.33224293864769550 ) ) ;
#106214=CARTESIAN_POINT ( 'NONE',  ( 13.89961937509977652, -13.97604488694527269, 113.1239096053143527 ) ) ;
#106215=CARTESIAN_POINT ( 'NONE',  ( -19.05341960407611168, -5.049401038298163336, 36.45724293864766707 ) ) ;
#106216=CARTESIAN_POINT ( 'NONE',  ( 16.53943276465976808, 0.05219959533934440121, 106.2510903946856757 ) ) ;
#106217=CARTESIAN_POINT ( 'NONE',  ( -19.03943276465977164, 0.05219959533909376836, 61.24890960531436690 ) ) ;
#106218=CARTESIAN_POINT ( 'NONE',  ( 4.379528057220092307, 16.55341960407617563, 22.29275706135235069 ) ) ;
#106219=CARTESIAN_POINT ( 'NONE',  ( 16.62475595723695676, 7.163666690055253028, 51.97286648189534475 ) ) ;
#106220=CARTESIAN_POINT ( 'NONE',  ( 21.52544592524334988, 5.823673210054432836, 111.4594237280190328 ) ) ;
#106221=CARTESIAN_POINT ( 'NONE',  ( 4.379528057220339221, -16.55341960407611168, 77.70724293864770971 ) ) ;
#106222=CARTESIAN_POINT ( 'NONE',  ( 10.81492255796078972, 18.62759615963270932, 114.5822429386477097 ) ) ;
#106223=CARTESIAN_POINT ( 'NONE',  ( -5.823673210054116645, -21.52544592524344225, 97.29057627198105251 ) ) ;
#106225=CARTESIAN_POINT ( 'NONE',  ( 18.62759615963271287, -10.81492255796078972, 58.33224293864768839 ) ) ;
#106226=CARTESIAN_POINT ( 'NONE',  ( 12.14591786802327356, -12.06949235617739191, 75.62609039468567573 ) ) ;
#106227=CARTESIAN_POINT ( 'NONE',  ( -14.34966873604960291, -8.224510206698953496, 101.6655762719810383 ) ) ;
#106228=CARTESIAN_POINT ( 'NONE',  ( 16.46253265017160672, -9.564922557960803928, 58.33224293864769550 ) ) ;
#106230=CARTESIAN_POINT ( 'NONE',  ( 4.483927247898790824, -16.52544592524335698, 110.2094237280190185 ) ) ;
#106231=CARTESIAN_POINT ( 'NONE',  ( -21.52544592524334988, -5.823673210054445271, 48.95942372801902565 ) ) ;
#106232=CARTESIAN_POINT ( 'NONE',  ( -5.153800228976328057, -19.02544592524343514, 102.2905762719810383 ) ) ;
#106233=CARTESIAN_POINT ( 'NONE',  ( 0.05219959533937995610, -21.53943276465977519, 85.00109039468568994 ) ) ;
#106234=CARTESIAN_POINT ( 'NONE',  ( 19.03943276465977164, -0.05219959533909143690, 23.74890960531435269 ) ) ;
#106235=CARTESIAN_POINT ( 'NONE',  ( -9.564922557960796823, -16.46253265017161027, 42.08224293864769550 ) ) ;
#106238=CARTESIAN_POINT ( 'NONE',  ( 18.67979575497194134, -10.72451020669871369, 75.83442372801900433 ) ) ;
#106239=CARTESIAN_POINT ( 'NONE',  ( -9.564922557960796823, -16.46253265017161027, 102.0822429386477097 ) ) ;
#106240=CARTESIAN_POINT ( 'NONE',  ( -13.89961937509957401, -13.97604488694547875, 74.37609039468566152 ) ) ;
#106241=CARTESIAN_POINT ( 'NONE',  ( -18.62759615963255300, -10.81492255796106328, 44.16775706135234714 ) ) ;
#106242=CARTESIAN_POINT ( 'NONE',  ( 16.55341960407618274, -4.379528057220086978, 21.04275706135234714 ) ) ;
#106243=CARTESIAN_POINT ( 'NONE',  ( -19.03943276465977164, -0.05219959533935918106, 68.75109039468566152 ) ) ;
#106244=CARTESIAN_POINT ( 'NONE',  ( -19.02544592524342804, 5.153800228976336051, 56.04057627198100988 ) ) ;
#106245=CARTESIAN_POINT ( 'NONE',  ( 5.049401038297881783, 19.05341960407617563, 82.29275706135229029 ) ) ;
#106246=CARTESIAN_POINT ( 'NONE',  ( -14.34966873604960291, -8.224510206698953496, 31.66557627198102054 ) ) ;
#106247=CARTESIAN_POINT ( 'NONE',  ( -16.51473224551082808, 9.474510206698731452, 73.33442372801900433 ) ) ;
#106248=CARTESIAN_POINT ( 'NONE',  ( 4.483927247898545687, 16.52544592524342804, 44.79057627198103120 ) ) ;
#106249=CARTESIAN_POINT ( 'NONE',  ( -16.46253265017146816, -9.564922557961047289, 59.16775706135233293 ) ) ;
#106250=CARTESIAN_POINT ( 'NONE',  ( 4.379528057220092307, 16.55341960407617563, 52.29275706135236135 ) ) ;
#106251=CARTESIAN_POINT ( 'NONE',  ( 19.02544592524334988, 5.153800228976608722, 26.45942372801899722 ) ) ;
#106252=CARTESIAN_POINT ( 'NONE',  ( 16.46253265017160672, -9.564922557960803928, 33.33224293864770260 ) ) ;
#106253=CARTESIAN_POINT ( 'NONE',  ( -16.61371651742603106, -7.165104196376047341, 66.14584930007005426 ) ) ;
#106254=CARTESIAN_POINT ( 'NONE',  ( 4.379528057220092307, 16.55341960407617563, 42.29275706135235424 ) ) ;
#106255=CARTESIAN_POINT ( 'NONE',  ( 15.50000000000000355, 7.499999999999998224, 118.0000000000000142 ) ) ;
#106257=CARTESIAN_POINT ( 'NONE',  ( 13.89961937509977652, -13.97604488694527269, 98.12390960531433848 ) ) ;
#106260=CARTESIAN_POINT ( 'NONE',  ( 19.03943276465977164, 0.05219959533936151252, 91.25109039468566152 ) ) ;
#106261=CARTESIAN_POINT ( 'NONE',  ( 5.719274019375991003, -21.55341960407610458, 22.70724293864769194 ) ) ;
#106262=CARTESIAN_POINT ( 'NONE',  ( 9.474510206698729675, 16.51473224551082808, 22.08442372801899722 ) ) ;
#106263=CARTESIAN_POINT ( 'NONE',  ( -9.564922557961040184, 16.46253265017147172, 102.9177570613523329 ) ) ;
#106264=CARTESIAN_POINT ( 'NONE',  ( 16.52544592524342804, -4.483927247898539470, 108.5405762719810241 ) ) ;
#106265=CARTESIAN_POINT ( 'NONE',  ( -9.474510206698964154, 16.51473224551069663, 40.41557627198103120 ) ) ;
#106266=CARTESIAN_POINT ( 'NONE',  ( -18.67979575497178146, -10.72451020669898902, 56.66557627198103830 ) ) ;
#106267=CARTESIAN_POINT ( 'NONE',  ( -4.483927247898539470, -16.52544592524342804, 112.2905762719810241 ) ) ;
#106268=CARTESIAN_POINT ( 'NONE',  ( -19.03943276465977164, -0.05219959533935918106, 73.75109039468566152 ) ) ;
#106269=CARTESIAN_POINT ( 'NONE',  ( 8.314922557960818139, 14.29746914071049879, 39.58224293864769550 ) ) ;
#106270=CARTESIAN_POINT ( 'NONE',  ( 16.51473224551069308, 9.474510206698969483, 109.1655762719810383 ) ) ;
#106271=CARTESIAN_POINT ( 'NONE',  ( -5.719274019375665041, -21.55341960407619695, 89.79275706135236135 ) ) ;
#106272=CARTESIAN_POINT ( 'NONE',  ( 21.52544592524344225, -5.823673210054117533, 83.54057627198102409 ) ) ;
#106273=CARTESIAN_POINT ( 'NONE',  ( 18.62759615963255655, 10.81492255796105972, 61.66775706135235424 ) ) ;
#106274=CARTESIAN_POINT ( 'NONE',  ( -21.53943276465977519, -0.05219959533937600094, 63.75109039468568284 ) ) ;
#106275=CARTESIAN_POINT ( 'NONE',  ( -19.03943276465977164, 0.05219959533909376836, 96.24890960531436690 ) ) ;
#106276=CARTESIAN_POINT ( 'NONE',  ( 4.483927247898790824, -16.52544592524335698, 95.20942372801903275 ) ) ;
#106277=CARTESIAN_POINT ( 'NONE',  ( 18.67979575497194134, -10.72451020669871369, 55.83442372801901854 ) ) ;
#106278=CARTESIAN_POINT ( 'NONE',  ( 4.379528057220339221, -16.55341960407611168, 112.7072429386476955 ) ) ;
#106279=CARTESIAN_POINT ( 'NONE',  ( -14.34966873604960291, -8.224510206698953496, 71.66557627198100988 ) ) ;
#106280=CARTESIAN_POINT ( 'NONE',  ( -16.53943276465976808, 0.05219959533911058130, 31.24890960531435979 ) ) ;
#106281=CARTESIAN_POINT ( 'NONE',  ( -21.55341960407610458, -5.719274019375992779, 41.45724293864769550 ) ) ;
#106282=CARTESIAN_POINT ( 'NONE',  ( 16.51473224551069308, 9.474510206698969483, 64.16557627198102409 ) ) ;
#106283=CARTESIAN_POINT ( 'NONE',  ( -13.97604488694527625, -13.89961937509977652, 51.87390960531436690 ) ) ;
#106284=CARTESIAN_POINT ( 'NONE',  ( -15.80617190586745835, -15.72974639402198527, 56.87390960531436690 ) ) ;
#106285=CARTESIAN_POINT ( 'NONE',  ( 13.89961937509957401, 13.97604488694547697, 41.87609039468566152 ) ) ;
#106286=CARTESIAN_POINT ( 'NONE',  ( -16.36317988757057051, -7.306389748694945396, 40.90210391636773579 ) ) ;
#106287=CARTESIAN_POINT ( 'NONE',  ( -16.55341960407611168, -4.379528057220339221, 51.45724293864770260 ) ) ;
#106288=CARTESIAN_POINT ( 'NONE',  ( -21.55341960407610458, -5.719274019375992779, 31.45724293864769550 ) ) ;
#106291=DIRECTION ( 'NONE',  ( -1.000000000000000000, -0.000000000000000000, -0.000000000000000000 ) ) ;
#106292=CARTESIAN_POINT ( 'NONE',  ( 16.52544592524335698, 4.483927247898782831, 76.45942372801901854 ) ) ;
#106293=CARTESIAN_POINT ( 'NONE',  ( -0.05219959533936034679, 19.03943276465977164, 77.50109039468566152 ) ) ;
#106294=CARTESIAN_POINT ( 'NONE',  ( 12.06949235617757843, -12.14591786802309237, 43.12390960531435269 ) ) ;
#106295=CARTESIAN_POINT ( 'NONE',  ( -30.00000000000000000, -5.204748896376250896E-15, 42.49999999999999289 ) ) ;
#106296=CARTESIAN_POINT ( 'NONE',  ( -8.224510206698948167, 14.34966873604960824, 30.41557627198101699 ) ) ;
#106297=CARTESIAN_POINT ( 'NONE',  ( -9.474510206698964154, 16.51473224551069663, 45.41557627198103120 ) ) ;
#106298=CARTESIAN_POINT ( 'NONE',  ( -13.97604488694527625, -13.89961937509977652, 76.87390960531433848 ) ) ;
#106299=CARTESIAN_POINT ( 'NONE',  ( -5.153800228976328057, -19.02544592524343514, 37.29057627198102409 ) ) ;
#106300=CARTESIAN_POINT ( 'NONE',  ( 5.719274019375673035, 21.55341960407619339, 47.29275706135234003 ) ) ;
#106301=CARTESIAN_POINT ( 'NONE',  ( 16.51473224551069308, 9.474510206698969483, 59.16557627198102409 ) ) ;
#106302=CARTESIAN_POINT ( 'NONE',  ( 18.10062525802553424, -5.500000000000022204, 81.01383468041919400 ) ) ;
#106303=CARTESIAN_POINT ( 'NONE',  ( 19.05341960407611168, 5.049401038298154454, 63.95724293864769550 ) ) ;
#106304=CARTESIAN_POINT ( 'NONE',  ( -18.62759615963270932, 10.81492255796079327, 30.83224293864770260 ) ) ;
#106306=CARTESIAN_POINT ( 'NONE',  ( 14.29746914071049879, -8.314922557960816363, 113.3322429386476955 ) ) ;
#106307=CARTESIAN_POINT ( 'NONE',  ( 5.823673210054125526, 21.52544592524343514, 24.79057627198103120 ) ) ;
#106308=CARTESIAN_POINT ( 'NONE',  ( -4.483927247898782831, 16.52544592524335698, 97.70942372801904696 ) ) ;
#106309=CARTESIAN_POINT ( 'NONE',  ( 5.719274019375673035, 21.55341960407619339, 112.2927570613523471 ) ) ;
#106310=CARTESIAN_POINT ( 'NONE',  ( -0.05219959533934338120, 16.53943276465976808, 67.50109039468568994 ) ) ;
#106311=CARTESIAN_POINT ( 'NONE',  ( 13.97604488694527802, 13.89961937509977652, 114.3739096053143669 ) ) ;
#106312=CARTESIAN_POINT ( 'NONE',  ( -16.53943276465976808, -0.05219959533934237506, 53.75109039468568994 ) ) ;
#106313=CARTESIAN_POINT ( 'NONE',  ( -16.52544592524335698, -4.483927247898792601, 33.95942372801901143 ) ) ;
#106314=CARTESIAN_POINT ( 'NONE',  ( -9.474510206698964154, 16.51473224551069663, 110.4155762719810383 ) ) ;
#106315=CARTESIAN_POINT ( 'NONE',  ( 14.34966873604972726, -8.224510206698740333, 30.83442372801902209 ) ) ;
#106316=CARTESIAN_POINT ( 'NONE',  ( -9.474510206698964154, 16.51473224551069663, 35.41557627198102409 ) ) ;
#106317=CARTESIAN_POINT ( 'NONE',  ( 18.67979575497194134, -10.72451020669871369, 20.83442372801901143 ) ) ;
#106318=CARTESIAN_POINT ( 'NONE',  ( -12.06949235617739369, -12.14591786802326823, 24.37609039468567573 ) ) ;
#106319=CARTESIAN_POINT ( 'NONE',  ( -8.224510206698735004, -14.34966873604973081, 79.58442372801903275 ) ) ;
#106321=CARTESIAN_POINT ( 'NONE',  ( 21.53943276465977519, 0.05219959533937863772, 91.25109039468568994 ) ) ;
#106322=CARTESIAN_POINT ( 'NONE',  ( 19.02544592524334988, 5.153800228976608722, 86.45942372801900433 ) ) ;
#106323=CARTESIAN_POINT ( 'NONE',  ( -14.34966873604960291, -8.224510206698953496, 61.66557627198103120 ) ) ;
#106324=CARTESIAN_POINT ( 'NONE',  ( 4.483927247898545687, 16.52544592524342804, 109.7905762719810383 ) ) ;
#106325=CARTESIAN_POINT ( 'NONE',  ( -16.51473224551082808, 9.474510206698731452, 43.33442372801900433 ) ) ;
#106327=CARTESIAN_POINT ( 'NONE',  ( 18.67979575497194134, -10.72451020669871369, 55.83442372801901854 ) ) ;
#106328=CARTESIAN_POINT ( 'NONE',  ( -19.05341960407617563, 5.049401038297882671, 103.5427570613523329 ) ) ;
#106330=CARTESIAN_POINT ( 'NONE',  ( 5.049401038298161559, -19.05341960407611168, 102.7072429386476955 ) ) ;
#106331=CARTESIAN_POINT ( 'NONE',  ( 5.719274019375991003, -21.55341960407610458, 77.70724293864770971 ) ) ;
#106332=CARTESIAN_POINT ( 'NONE',  ( 19.05341960407617918, -5.049401038297876454, 91.04275706135234714 ) ) ;
#106333=CARTESIAN_POINT ( 'NONE',  ( 16.51473224551069308, 9.474510206698969483, 109.1655762719810383 ) ) ;
#106335=CARTESIAN_POINT ( 'NONE',  ( -8.314922557960811034, -14.29746914071050412, 102.0822429386476955 ) ) ;
#106336=CARTESIAN_POINT ( 'NONE',  ( 21.52544592524334988, 5.823673210054432836, 96.45942372801901854 ) ) ;
#106337=CARTESIAN_POINT ( 'NONE',  ( 13.97604488694527802, 13.89961937509977652, 39.37390960531435269 ) ) ;
#106338=CARTESIAN_POINT ( 'NONE',  ( 18.62759615963255655, 10.81492255796105972, 51.66775706135234714 ) ) ;
#106340=CARTESIAN_POINT ( 'NONE',  ( -10.81492255796105439, 18.62759615963255655, 82.91775706135234714 ) ) ;
#106341=CARTESIAN_POINT ( 'NONE',  ( -14.34966873604972548, 8.224510206698743886, 103.3344237280190043 ) ) ;
#106342=CARTESIAN_POINT ( 'NONE',  ( 9.474510206698971260, -16.51473224551069308, 67.91557627198102409 ) ) ;
#106343=CARTESIAN_POINT ( 'NONE',  ( 5.719274019375673035, 21.55341960407619339, 42.29275706135235424 ) ) ;
#106344=CARTESIAN_POINT ( 'NONE',  ( -10.72451020669870658, -18.67979575497194134, 34.58442372801900433 ) ) ;
#106345=CARTESIAN_POINT ( 'NONE',  ( -16.46253265017146816, -9.564922557961047289, 64.16775706135233293 ) ) ;
#106346=CARTESIAN_POINT ( 'NONE',  ( 19.02544592524343514, -5.153800228976328945, 88.54057627198102409 ) ) ;
#106347=CARTESIAN_POINT ( 'NONE',  ( 16.53943276465976808, -0.05219959533910856209, 103.7489096053143669 ) ) ;
#106348=CARTESIAN_POINT ( 'NONE',  ( -10.72451020669898014, 18.67979575497178502, 90.41557627198103830 ) ) ;
#106349=CARTESIAN_POINT ( 'NONE',  ( 4.379528057220339221, -16.55341960407611168, 67.70724293864769550 ) ) ;
#106350=CARTESIAN_POINT ( 'NONE',  ( -19.02544592524334988, -5.153800228976617603, 23.95942372801900078 ) ) ;
#106351=CARTESIAN_POINT ( 'NONE',  ( -16.55341960407611168, -4.379528057220339221, 86.45724293864770971 ) ) ;
#106352=CARTESIAN_POINT ( 'NONE',  ( -5.153800228976328057, -19.02544592524343514, 37.29057627198102409 ) ) ;
#106353=CARTESIAN_POINT ( 'NONE',  ( -16.46253265017146816, -9.564922557961047289, 84.16775706135233293 ) ) ;
#106354=CARTESIAN_POINT ( 'NONE',  ( -8.314922557960811034, -14.29746914071050412, 47.08224293864770260 ) ) ;
#106355=CARTESIAN_POINT ( 'NONE',  ( -21.55341960407619339, 5.719274019375674811, 93.54275706135234714 ) ) ;
#106356=CARTESIAN_POINT ( 'NONE',  ( 9.474510206698971260, -16.51473224551069308, 97.91557627198102409 ) ) ;
#106357=CARTESIAN_POINT ( 'NONE',  ( -16.51473224551082808, 9.474510206698731452, 63.33442372801900433 ) ) ;
#106358=CARTESIAN_POINT ( 'NONE',  ( 21.52544592524344225, -5.823673210054117533, 78.54057627198103830 ) ) ;
#106359=CARTESIAN_POINT ( 'NONE',  ( 21.55341960407619695, -5.719274019375665929, 31.04275706135234714 ) ) ;
#106360=CARTESIAN_POINT ( 'NONE',  ( -14.29746914071037622, -8.314922557961029526, 34.16775706135234714 ) ) ;
#106361=CARTESIAN_POINT ( 'NONE',  ( -12.14591786802326823, 12.06949235617739902, 88.12609039468570415 ) ) ;
#106362=CARTESIAN_POINT ( 'NONE',  ( 13.89961937509977652, -13.97604488694527269, 28.12390960531435624 ) ) ;
#106363=CARTESIAN_POINT ( 'NONE',  ( -21.53943276465977519, 0.05219959533907696930, 116.2489096053143669 ) ) ;
#106365=CARTESIAN_POINT ( 'NONE',  ( -16.46253265017160317, 9.564922557960807481, 25.83224293864769194 ) ) ;
#106367=CARTESIAN_POINT ( 'NONE',  ( 12.14591786802327356, -12.06949235617739191, 55.62609039468568284 ) ) ;
#106369=CARTESIAN_POINT ( 'NONE',  ( -8.224510206698948167, 14.34966873604960824, 75.41557627198102409 ) ) ;
#106370=CARTESIAN_POINT ( 'NONE',  ( -21.55341960407610458, -5.719274019375992779, 71.45724293864769550 ) ) ;
#106371=CARTESIAN_POINT ( 'NONE',  ( -16.52544592524342804, 4.483927247898546575, 26.04057627198103475 ) ) ;
#106372=CARTESIAN_POINT ( 'NONE',  ( 14.34966873604972726, -8.224510206698740333, 45.83442372801901854 ) ) ;
#106373=CARTESIAN_POINT ( 'NONE',  ( -0.05219959533909027116, -19.03943276465977164, 47.49890960531435979 ) ) ;
#106374=CARTESIAN_POINT ( 'NONE',  ( 16.55341960407618274, -4.379528057220086978, 81.04275706135236135 ) ) ;
#106375=CARTESIAN_POINT ( 'NONE',  ( 5.153800228976615827, -19.02544592524334988, 75.20942372801896170 ) ) ;
#106376=CARTESIAN_POINT ( 'NONE',  ( -21.52544592524343514, 5.823673210054127303, 71.04057627198103830 ) ) ;
#106377=CARTESIAN_POINT ( 'NONE',  ( 12.14591786802309770, 12.06949235617756955, 24.37390960531435979 ) ) ;
#106380=CARTESIAN_POINT ( 'NONE',  ( -21.55341960407610458, -5.719274019375992779, 51.45724293864770260 ) ) ;
#106381=VERTEX_POINT ( 'NONE', #191587 ) ;
#106383=CARTESIAN_POINT ( 'NONE',  ( 16.52544592524335698, 4.483927247898782831, 91.45942372801901854 ) ) ;
#106384=VERTEX_POINT ( 'NONE', #38913 ) ;
#106385=CARTESIAN_POINT ( 'NONE',  ( 0.05219959533909260263, 19.03943276465977164, 109.9989096053143669 ) ) ;
#106386=CARTESIAN_POINT ( 'NONE',  ( 18.22780087662121673, 5.500000000000056843, 48.98459894673892734 ) ) ;
#106387=CARTESIAN_POINT ( 'NONE',  ( 21.52544592524344225, -5.823673210054117533, 68.54057627198103830 ) ) ;
#106388=CARTESIAN_POINT ( 'NONE',  ( -4.483927247898782831, 16.52544592524335698, 102.7094237280190185 ) ) ;
#106389=CARTESIAN_POINT ( 'NONE',  ( 16.52544592524335698, 4.483927247898782831, 26.45942372801901854 ) ) ;
#106390=CARTESIAN_POINT ( 'NONE',  ( -16.53943276465976808, 0.05219959533911058130, 111.2489096053143669 ) ) ;
#106391=CARTESIAN_POINT ( 'NONE',  ( -12.06949235617739369, -12.14591786802326823, 24.37609039468567573 ) ) ;
#106392=CARTESIAN_POINT ( 'NONE',  ( 5.153800228976335163, 19.02544592524342804, 59.79057627198100988 ) ) ;
#106394=CARTESIAN_POINT ( 'NONE',  ( 9.564922557960805705, 16.46253265017160317, 99.58224293864770971 ) ) ;
#106395=CARTESIAN_POINT ( 'NONE',  ( 14.29746914071037800, 8.314922557961029526, 86.66775706135234714 ) ) ;
#106396=CARTESIAN_POINT ( 'NONE',  ( -0.05219959533936034679, 19.03943276465977164, 92.50109039468566152 ) ) ;
#106397=CARTESIAN_POINT ( 'NONE',  ( 9.474510206698729675, 16.51473224551082808, 22.08442372801899722 ) ) ;
#106398=CARTESIAN_POINT ( 'NONE',  ( 18.67979575497178502, 10.72451020669898547, 74.16557627198102409 ) ) ;
#106399=CARTESIAN_POINT ( 'NONE',  ( 16.55341960407618274, -4.379528057220086978, 101.0427570613523756 ) ) ;
#106400=CARTESIAN_POINT ( 'NONE',  ( -16.46253265017146816, -9.564922557961047289, 94.16775706135233293 ) ) ;
#106401=CARTESIAN_POINT ( 'NONE',  ( -5.153800228976328057, -19.02544592524343514, 47.29057627198102409 ) ) ;
#106402=CARTESIAN_POINT ( 'NONE',  ( 13.97604488694527802, 13.89961937509977652, 89.37390960531436690 ) ) ;
#106403=CARTESIAN_POINT ( 'NONE',  ( -21.55341960407619339, 5.719274019375674811, 63.54275706135234003 ) ) ;
#106404=CARTESIAN_POINT ( 'NONE',  ( -5.049401038298153566, 19.05341960407611168, 45.20724293864769550 ) ) ;
#106406=CARTESIAN_POINT ( 'NONE',  ( 14.34966873604960469, 8.224510206698951720, 79.16557627198103830 ) ) ;
#106407=CARTESIAN_POINT ( 'NONE',  ( -5.823673210054116645, -21.52544592524344225, 72.29057627198102409 ) ) ;
#106408=CARTESIAN_POINT ( 'NONE',  ( 19.50973618000807264, -5.499999999999992895, 102.5000000000000142 ) ) ;
#106410=CARTESIAN_POINT ( 'NONE',  ( 9.474510206698729675, 16.51473224551082808, 47.08442372801900433 ) ) ;
#106411=CARTESIAN_POINT ( 'NONE',  ( 17.05587630539709920, -6.762274262136624969, 73.24180309037285497 ) ) ;
#106412=CARTESIAN_POINT ( 'NONE',  ( 13.89961937509977652, -13.97604488694527269, 78.12390960531433848 ) ) ;
#106413=CARTESIAN_POINT ( 'NONE',  ( 16.51473224551069308, 9.474510206698969483, 84.16557627198102409 ) ) ;
#106414=CARTESIAN_POINT ( 'NONE',  ( -12.06949235617739369, -12.14591786802326823, 64.37609039468568994 ) ) ;
#106416=CARTESIAN_POINT ( 'NONE',  ( -13.97604488694547697, 13.89961937509957934, 28.12609039468565797 ) ) ;
#106418=CARTESIAN_POINT ( 'NONE',  ( 4.483927247898790824, -16.52544592524335698, 85.20942372801901854 ) ) ;
#106420=CARTESIAN_POINT ( 'NONE',  ( -12.14591786802326823, 12.06949235617739902, 83.12609039468568994 ) ) ;
#106421=CARTESIAN_POINT ( 'NONE',  ( -17.31728774477273802, 6.344390552232388458, 30.81906651689318721 ) ) ;
#106422=CARTESIAN_POINT ( 'NONE',  ( 0.05219959533934541429, -16.53943276465976808, 55.00109039468568284 ) ) ;
#106423=CARTESIAN_POINT ( 'NONE',  ( 18.22780087662121673, 5.500000000000056843, 73.98459894673894155 ) ) ;
#106424=CARTESIAN_POINT ( 'NONE',  ( -10.81492255796105439, 18.62759615963255655, 67.91775706135234714 ) ) ;
#106425=CARTESIAN_POINT ( 'NONE',  ( -19.03943276465977164, -0.05219959533935918106, 78.75109039468567573 ) ) ;
#106426=CARTESIAN_POINT ( 'NONE',  ( -19.05341960407617563, 5.049401038297882671, 23.54275706135233648 ) ) ;
#106427=CARTESIAN_POINT ( 'NONE',  ( 5.049401038298161559, -19.05341960407611168, 47.70724293864770260 ) ) ;
#106428=CARTESIAN_POINT ( 'NONE',  ( 13.97604488694527802, 13.89961937509977652, 39.37390960531435269 ) ) ;
#106429=CARTESIAN_POINT ( 'NONE',  ( -17.49999999999999645, -5.499999999999992895, 64.20309617465829888 ) ) ;
#106430=CARTESIAN_POINT ( 'NONE',  ( -15.72974639402197994, 15.80617190586746368, 65.62390960531436690 ) ) ;
#106431=CARTESIAN_POINT ( 'NONE',  ( -5.049401038298153566, 19.05341960407611168, 115.2072429386477097 ) ) ;
#106432=CARTESIAN_POINT ( 'NONE',  ( 12.14591786802309770, 12.06949235617756955, 109.3739096053143811 ) ) ;
#106433=CARTESIAN_POINT ( 'NONE',  ( 12.06949235617739724, 12.14591786802326823, 46.87609039468568994 ) ) ;
#106436=CARTESIAN_POINT ( 'NONE',  ( 5.823673210054125526, 21.52544592524343514, 114.7905762719810383 ) ) ;
#106437=CARTESIAN_POINT ( 'NONE',  ( 4.483927247898545687, 16.52544592524342804, 49.79057627198102409 ) ) ;
#106439=CARTESIAN_POINT ( 'NONE',  ( 19.05341960407617918, -5.049401038297876454, 106.0427570613523471 ) ) ;
#106440=CARTESIAN_POINT ( 'NONE',  ( -19.05341960407617563, 5.049401038297882671, 43.54275706135232582 ) ) ;
#106441=CARTESIAN_POINT ( 'NONE',  ( 16.55341960407611168, 4.379528057220329451, 38.95724293864768839 ) ) ;
#106442=CARTESIAN_POINT ( 'NONE',  ( 5.823673210054444382, -21.52544592524334988, 20.20942372801900788 ) ) ;
#106443=CARTESIAN_POINT ( 'NONE',  ( 17.26172910966779384, 6.454744622555870670, 31.69353091350778229 ) ) ;
#106444=CARTESIAN_POINT ( 'NONE',  ( 21.53943276465977519, -0.05219959533907433946, 63.74890960531435979 ) ) ;
#106445=CARTESIAN_POINT ( 'NONE',  ( -9.474510206698964154, 16.51473224551069663, 90.41557627198103830 ) ) ;
#106446=CARTESIAN_POINT ( 'NONE',  ( -16.55341960407611168, -4.379528057220339221, 51.45724293864770260 ) ) ;
#106447=CARTESIAN_POINT ( 'NONE',  ( 0.05219959533909260263, 19.03943276465977164, 109.9989096053143669 ) ) ;
#106448=EDGE_CURVE ( 'NONE', #5512, #49306, #123924, .T. ) ;
#106449=VECTOR ( 'NONE', #157266, 1000.000000000000000 ) ;
#106451=CARTESIAN_POINT ( 'NONE',  ( -5.049401038297874678, -19.05341960407617918, 59.79275706135231871 ) ) ;
#106452=CARTESIAN_POINT ( 'NONE',  ( -10.72451020669898014, 18.67979575497178502, 95.41557627198102409 ) ) ;
#106453=CARTESIAN_POINT ( 'NONE',  ( -5.049401038298153566, 19.05341960407611168, 40.20724293864768839 ) ) ;
#106454=CARTESIAN_POINT ( 'NONE',  ( 19.05341960407611168, 5.049401038298154454, 23.95724293864769194 ) ) ;
#106455=CARTESIAN_POINT ( 'NONE',  ( -18.62759615963255300, -10.81492255796106328, 44.16775706135234714 ) ) ;
#106457=CARTESIAN_POINT ( 'NONE',  ( -0.05219959533910754901, -16.53943276465976808, 22.49890960531436335 ) ) ;
#106458=CARTESIAN_POINT ( 'NONE',  ( -13.97604488694527625, -13.89961937509977652, 51.87390960531436690 ) ) ;
#106459=CARTESIAN_POINT ( 'NONE',  ( -9.474510206698964154, 16.51473224551069663, 100.4155762719810241 ) ) ;
#106460=CARTESIAN_POINT ( 'NONE',  ( 15.72974639402199770, -15.80617190586745480, 68.12390960531436690 ) ) ;
#106462=CARTESIAN_POINT ( 'NONE',  ( 13.97604488694527802, 13.89961937509977652, 44.37390960531435269 ) ) ;
#106463=CARTESIAN_POINT ( 'NONE',  ( 0.05219959533907565091, 21.53943276465977519, 54.99890960531435269 ) ) ;
#106464=CARTESIAN_POINT ( 'NONE',  ( 21.55341960407619695, -5.719274019375665929, 86.04275706135236135 ) ) ;
#106466=CARTESIAN_POINT ( 'NONE',  ( 16.53943276465976808, 0.05219959533934440121, 81.25109039468568994 ) ) ;
#106467=CARTESIAN_POINT ( 'NONE',  ( -12.14591786802309592, -12.06949235617757132, 71.87390960531438111 ) ) ;
#106468=CARTESIAN_POINT ( 'NONE',  ( 8.314922557961029526, -14.29746914071037800, 90.41775706135236135 ) ) ;
#106469=CARTESIAN_POINT ( 'NONE',  ( -13.89961937509977652, 13.97604488694528158, 75.62390960531438111 ) ) ;
#106470=ORIENTED_EDGE ( 'NONE', *, *, #137592, .F. ) ;
#106471=CARTESIAN_POINT ( 'NONE',  ( 16.51473224551083163, -9.474510206698727899, 25.83442372801900078 ) ) ;
#106472=CARTESIAN_POINT ( 'NONE',  ( 8.224510206698742110, 14.34966873604972548, 92.08442372801901854 ) ) ;
#106473=CARTESIAN_POINT ( 'NONE',  ( -16.51473224551082808, 9.474510206698731452, 23.33442372801900078 ) ) ;
#106474=CARTESIAN_POINT ( 'NONE',  ( 13.89961937509977652, -13.97604488694527269, 78.12390960531433848 ) ) ;
#106475=CARTESIAN_POINT ( 'NONE',  ( 21.55341960407610458, 5.719274019375980345, 48.95724293864770971 ) ) ;
#106476=CARTESIAN_POINT ( 'NONE',  ( 14.34966873604972726, -8.224510206698740333, 30.83442372801902209 ) ) ;
#106477=CARTESIAN_POINT ( 'NONE',  ( 15.80617190586769283, -15.72974639402175789, 80.62609039468567573 ) ) ;
#106478=CARTESIAN_POINT ( 'NONE',  ( -12.06949235617739369, -12.14591786802326823, 69.37609039468567573 ) ) ;
#106479=CARTESIAN_POINT ( 'NONE',  ( -18.62759615963255300, -10.81492255796106328, 19.16775706135234714 ) ) ;
#106480=CARTESIAN_POINT ( 'NONE',  ( 5.049401038297881783, 19.05341960407617563, 107.2927570613523187 ) ) ;
#106481=CARTESIAN_POINT ( 'NONE',  ( 5.153800228976335163, 19.02544592524342804, 89.79057627198102409 ) ) ;
#106482=CARTESIAN_POINT ( 'NONE',  ( -8.224510206698735004, -14.34966873604973081, 24.58442372801901499 ) ) ;
#106483=CARTESIAN_POINT ( 'NONE',  ( -13.97604488694527625, -13.89961937509977652, 41.87390960531435979 ) ) ;
#106484=AXIS2_PLACEMENT_3D ( 'NONE', #38760, #114584, #179294 ) ;
#106485=CARTESIAN_POINT ( 'NONE',  ( 0.05219959533934541429, -16.53943276465976808, 30.00109039468568284 ) ) ;
#106486=CARTESIAN_POINT ( 'NONE',  ( -0.05219959533910754901, -16.53943276465976808, 77.49890960531433848 ) ) ;
#106487=CARTESIAN_POINT ( 'NONE',  ( 14.29746914071037800, 8.314922557961029526, 86.66775706135234714 ) ) ;
#106488=CARTESIAN_POINT ( 'NONE',  ( 5.823673210054444382, -21.52544592524334988, 35.20942372801901854 ) ) ;
#106489=CARTESIAN_POINT ( 'NONE',  ( 5.153800228976335163, 19.02544592524342804, 69.79057627198103830 ) ) ;
#106490=CARTESIAN_POINT ( 'NONE',  ( -16.46253265017160317, 9.564922557960807481, 85.83224293864769550 ) ) ;
#106491=B_SPLINE_CURVE_WITH_KNOTS ( 'NONE', 3,
 ( #137292, #61435, #183805, #28160, #167644, #105959 ),
 .UNSPECIFIED., .F., .F.,
 ( 4, 2, 4 ),
 ( 0.000000000000000000, 0.0006703399052047476865, 0.001340679810409495373 ),
 .UNSPECIFIED. ) ;
#106492=CARTESIAN_POINT ( 'NONE',  ( 12.14591786802327356, -12.06949235617739191, 85.62609039468568994 ) ) ;
#106494=VERTEX_POINT ( 'NONE', #119749 ) ;
#106496=CARTESIAN_POINT ( 'NONE',  ( 13.97604488694548053, -13.89961937509957401, 30.62609039468566863 ) ) ;
#106497=CARTESIAN_POINT ( 'NONE',  ( 5.049401038298161559, -19.05341960407611168, 92.70724293864769550 ) ) ;
#106498=CARTESIAN_POINT ( 'NONE',  ( -5.049401038298153566, 19.05341960407611168, 45.20724293864769550 ) ) ;
#106499=CARTESIAN_POINT ( 'NONE',  ( 13.97604488694527802, 13.89961937509977652, 114.3739096053143669 ) ) ;
#106500=ORIENTED_EDGE ( 'NONE', *, *, #158923, .T. ) ;
#106501=CARTESIAN_POINT ( 'NONE',  ( 0.05219959533934541429, -16.53943276465976808, 35.00109039468568284 ) ) ;
#106502=CARTESIAN_POINT ( 'NONE',  ( 9.474510206698729675, 16.51473224551082808, 57.08442372801900433 ) ) ;
#106503=CARTESIAN_POINT ( 'NONE',  ( 16.53943276465976808, 0.05219959533934440121, 36.25109039468567573 ) ) ;
#106504=CARTESIAN_POINT ( 'NONE',  ( -16.46253265017160317, 9.564922557960807481, 100.8322429386477097 ) ) ;
#106505=CARTESIAN_POINT ( 'NONE',  ( -16.46253265017160317, 9.564922557960807481, 70.83224293864770971 ) ) ;
#106506=CARTESIAN_POINT ( 'NONE',  ( 18.67979575497178502, 10.72451020669898547, 94.16557627198103830 ) ) ;
#106507=CARTESIAN_POINT ( 'NONE',  ( -9.474510206698720793, -16.51473224551083518, 59.58442372801900433 ) ) ;
#106508=CARTESIAN_POINT ( 'NONE',  ( -16.46253265017160317, 9.564922557960807481, 85.83224293864769550 ) ) ;
#106510=CARTESIAN_POINT ( 'NONE',  ( -5.049401038298153566, 19.05341960407611168, 60.20724293864768129 ) ) ;
#106511=CARTESIAN_POINT ( 'NONE',  ( -8.314922557960811034, -14.29746914071050412, 27.08224293864769550 ) ) ;
#106512=CARTESIAN_POINT ( 'NONE',  ( -5.049401038298153566, 19.05341960407611168, 25.20724293864768484 ) ) ;
#106513=CARTESIAN_POINT ( 'NONE',  ( 13.89961937509957401, 13.97604488694547697, 41.87609039468566152 ) ) ;
#106514=CARTESIAN_POINT ( 'NONE',  ( -8.314922557960811034, -14.29746914071050412, 72.08224293864769550 ) ) ;
#106515=CARTESIAN_POINT ( 'NONE',  ( -21.53943276465977519, -0.05219959533937600094, 93.75109039468567573 ) ) ;
#106516=CARTESIAN_POINT ( 'NONE',  ( -9.474510206698964154, 16.51473224551069663, 45.41557627198103120 ) ) ;
#106517=CARTESIAN_POINT ( 'NONE',  ( -16.52544592524335698, -4.483927247898792601, 53.95942372801900433 ) ) ;
#106518=CARTESIAN_POINT ( 'NONE',  ( 4.379528057220339221, -16.55341960407611168, 42.70724293864770260 ) ) ;
#106519=CARTESIAN_POINT ( 'NONE',  ( -0.05219959533937732626, 21.53943276465977519, 92.50109039468567573 ) ) ;
#106520=CARTESIAN_POINT ( 'NONE',  ( -9.564922557960796823, -16.46253265017161027, 87.08224293864769550 ) ) ;
#106521=ORIENTED_EDGE ( 'NONE', *, *, #116955, .T. ) ;
#106522=CARTESIAN_POINT ( 'NONE',  ( 19.03943276465977164, -0.05219959533909143690, 98.74890960531436690 ) ) ;
#106523=CARTESIAN_POINT ( 'NONE',  ( -16.53943276465976808, 0.05219959533911058130, 101.2489096053143669 ) ) ;
#106524=CARTESIAN_POINT ( 'NONE',  ( 14.34966873604960469, 8.224510206698951720, 79.16557627198103830 ) ) ;
#106525=CARTESIAN_POINT ( 'NONE',  ( -18.62759615963270932, 10.81492255796079327, 80.83224293864769550 ) ) ;
#106526=CARTESIAN_POINT ( 'NONE',  ( 16.46253265017160672, -9.564922557960803928, 83.33224293864768129 ) ) ;
#106527=CARTESIAN_POINT ( 'NONE',  ( 18.67979575497178502, 10.72451020669898547, 104.1655762719810241 ) ) ;
#106528=CARTESIAN_POINT ( 'NONE',  ( 16.51473224551069308, 9.474510206698969483, 94.16557627198103830 ) ) ;
#106529=CARTESIAN_POINT ( 'NONE',  ( -19.49190055781011210, -5.499999999999966249, 90.56116087098783396 ) ) ;
#106530=CARTESIAN_POINT ( 'NONE',  ( 4.483927247898545687, 16.52544592524342804, 94.79057627198105251 ) ) ;
#106531=CARTESIAN_POINT ( 'NONE',  ( -13.89961937509977652, 13.97604488694528158, 55.62390960531434558 ) ) ;
#106532=CARTESIAN_POINT ( 'NONE',  ( -21.53943276465977519, 0.05219959533907696930, 61.24890960531435979 ) ) ;
#106533=CARTESIAN_POINT ( 'NONE',  ( 17.26058549869091152, -6.457015423128605214, 26.12254162523933232 ) ) ;
#106534=CARTESIAN_POINT ( 'NONE',  ( 14.29746914071037800, 8.314922557961029526, 111.6677570613523613 ) ) ;
#106536=CARTESIAN_POINT ( 'NONE',  ( -19.05341960407617563, 5.049401038297882671, 113.5427570613523471 ) ) ;
#106537=CARTESIAN_POINT ( 'NONE',  ( -8.314922557960811034, -14.29746914071050412, 87.08224293864769550 ) ) ;
#106538=CARTESIAN_POINT ( 'NONE',  ( 18.39635199886970440, -5.499999999999988454, 53.51967076360000419 ) ) ;
#106539=CARTESIAN_POINT ( 'NONE',  ( -5.153800228976328057, -19.02544592524343514, 72.29057627198102409 ) ) ;
#106540=CARTESIAN_POINT ( 'NONE',  ( 9.564922557960805705, 16.46253265017160317, 39.58224293864768839 ) ) ;
#106541=CARTESIAN_POINT ( 'NONE',  ( 8.224510206698953496, -14.34966873604960469, 72.91557627198103830 ) ) ;
#106543=CARTESIAN_POINT ( 'NONE',  ( -9.564922557960796823, -16.46253265017161027, 112.0822429386476955 ) ) ;
#106544=CARTESIAN_POINT ( 'NONE',  ( -13.89961937509957401, -13.97604488694547875, 99.37609039468567573 ) ) ;
#106545=CARTESIAN_POINT ( 'NONE',  ( -13.89961937509977652, 13.97604488694528158, 105.6239096053143527 ) ) ;
#106546=CARTESIAN_POINT ( 'NONE',  ( -5.823673210054116645, -21.52544592524344225, 72.29057627198102409 ) ) ;
#106547=CARTESIAN_POINT ( 'NONE',  ( -4.379528057220086978, -16.55341960407618274, 74.79275706135234714 ) ) ;
#106548=CARTESIAN_POINT ( 'NONE',  ( -16.18388926212247725, 7.379444403734498614, 94.56046848633769741 ) ) ;
#106549=CARTESIAN_POINT ( 'NONE',  ( -19.03943276465977164, 0.05219959533909376836, 76.24890960531435269 ) ) ;
#106550=CARTESIAN_POINT ( 'NONE',  ( 21.53943276465977519, -0.05219959533907433946, 78.74890960531436690 ) ) ;
#106551=CARTESIAN_POINT ( 'NONE',  ( 13.97604488694548053, -13.89961937509957401, 110.6260903946856615 ) ) ;
#106552=CARTESIAN_POINT ( 'NONE',  ( -4.379528057220328563, 16.55341960407611168, 35.20724293864768839 ) ) ;
#106553=CARTESIAN_POINT ( 'NONE',  ( 0.05219959533937995610, -21.53943276465977519, 65.00109039468568994 ) ) ;
#106554=CARTESIAN_POINT ( 'NONE',  ( 17.58332526062524437, 7.635886036038643354, 71.57665040441537485 ) ) ;
#106555=CARTESIAN_POINT ( 'NONE',  ( 16.53943276465976808, 0.05219959533934440121, 91.25109039468568994 ) ) ;
#106556=CARTESIAN_POINT ( 'NONE',  ( -19.05341960407611168, -5.049401038298163336, 106.4572429386476955 ) ) ;
#106558=CARTESIAN_POINT ( 'NONE',  ( -17.50000000000000355, 5.622605283950870891, 78.68792689403892382 ) ) ;
#106559=CARTESIAN_POINT ( 'NONE',  ( 4.483927247898790824, -16.52544592524335698, 100.2094237280190043 ) ) ;
#106560=CARTESIAN_POINT ( 'NONE',  ( 14.34966873604972726, -8.224510206698740333, 40.83442372801901854 ) ) ;
#106561=CARTESIAN_POINT ( 'NONE',  ( -13.97604488694527625, -13.89961937509977652, 56.87390960531434558 ) ) ;
#106562=CARTESIAN_POINT ( 'NONE',  ( -13.89961937509977652, 13.97604488694528158, 75.62390960531438111 ) ) ;
#106563=CARTESIAN_POINT ( 'NONE',  ( 21.55341960407619695, -5.719274019375665929, 71.04275706135234714 ) ) ;
#106564=CARTESIAN_POINT ( 'NONE',  ( 8.224510206698742110, 14.34966873604972548, 67.08442372801901854 ) ) ;
#106565=CARTESIAN_POINT ( 'NONE',  ( 16.53943276465976808, -0.05219959533910856209, 38.74890960531435979 ) ) ;
#106566=CARTESIAN_POINT ( 'NONE',  ( -16.51473224551069308, -9.474510206698971260, 41.66557627198103120 ) ) ;
#106567=CARTESIAN_POINT ( 'NONE',  ( 19.03943276465977164, -0.05219959533909143690, 48.74890960531435979 ) ) ;
#106568=CARTESIAN_POINT ( 'NONE',  ( 8.314922557961029526, -14.29746914071037800, 35.41775706135234003 ) ) ;
#106569=CARTESIAN_POINT ( 'NONE',  ( 16.46253265017146816, 9.564922557961045513, 101.6677570613523329 ) ) ;
#106570=CARTESIAN_POINT ( 'NONE',  ( -8.224510206698948167, 14.34966873604960824, 90.41557627198103830 ) ) ;
#106571=CARTESIAN_POINT ( 'NONE',  ( 19.03943276465977164, -0.05219959533909143690, 53.74890960531436690 ) ) ;
#106572=CARTESIAN_POINT ( 'NONE',  ( 5.153800228976615827, -19.02544592524334988, 85.20942372801900433 ) ) ;
#106574=CARTESIAN_POINT ( 'NONE',  ( 18.62759615963255655, 10.81492255796105972, 86.66775706135234714 ) ) ;
#106575=CARTESIAN_POINT ( 'NONE',  ( 0.05219959533934541429, -16.53943276465976808, 50.00109039468568994 ) ) ;
#106577=CARTESIAN_POINT ( 'NONE',  ( 18.67979575497178502, 10.72451020669898547, 49.16557627198102409 ) ) ;
#106578=CARTESIAN_POINT ( 'NONE',  ( -8.224510206698735004, -14.34966873604973081, 34.58442372801900433 ) ) ;
#106579=CARTESIAN_POINT ( 'NONE',  ( -18.56197773271725993, 5.500000000000080824, 68.55066217314451649 ) ) ;
#106580=CARTESIAN_POINT ( 'NONE',  ( 5.049401038297881783, 19.05341960407617563, 47.29275706135231161 ) ) ;
#106581=CARTESIAN_POINT ( 'NONE',  ( -5.049401038298153566, 19.05341960407611168, 85.20724293864766707 ) ) ;
#106582=CARTESIAN_POINT ( 'NONE',  ( -19.05341960407611168, -5.049401038298163336, 21.45724293864768839 ) ) ;
#106583=CARTESIAN_POINT ( 'NONE',  ( -9.564922557960796823, -16.46253265017161027, 57.08224293864769550 ) ) ;
#106585=CARTESIAN_POINT ( 'NONE',  ( 18.62759615963255655, 10.81492255796105972, 76.66775706135234714 ) ) ;
#106586=DIRECTION ( 'NONE',  ( 0.000000000000000000, -1.000000000000000000, 0.000000000000000000 ) ) ;
#106588=CARTESIAN_POINT ( 'NONE',  ( -13.89961937509957401, -13.97604488694547875, 29.37609039468565797 ) ) ;
#106589=CARTESIAN_POINT ( 'NONE',  ( 13.97604488694548053, -13.89961937509957401, 20.62609039468567573 ) ) ;
#106590=CARTESIAN_POINT ( 'NONE',  ( 4.379528057220339221, -16.55341960407611168, 47.70724293864770260 ) ) ;
#106591=CARTESIAN_POINT ( 'NONE',  ( 19.02544592524343514, -5.153800228976328945, 58.54057627198102409 ) ) ;
#106592=CARTESIAN_POINT ( 'NONE',  ( 5.049401038298161559, -19.05341960407611168, 107.7072429386476955 ) ) ;
#106593=CARTESIAN_POINT ( 'NONE',  ( -21.52544592524334988, -5.823673210054445271, 83.95942372801900433 ) ) ;
#106594=CARTESIAN_POINT ( 'NONE',  ( 0.05219959533909260263, 19.03943276465977164, 69.99890960531435269 ) ) ;
#106595=CARTESIAN_POINT ( 'NONE',  ( 10.81492255796106328, -18.62759615963255655, 80.41775706135234714 ) ) ;
#106596=CARTESIAN_POINT ( 'NONE',  ( -5.823673210054116645, -21.52544592524344225, 42.29057627198103120 ) ) ;
#106597=CARTESIAN_POINT ( 'NONE',  ( -5.719274019375665041, -21.55341960407619695, 39.79275706135235424 ) ) ;
#106598=CARTESIAN_POINT ( 'NONE',  ( 13.97604488694548053, -13.89961937509957401, 60.62609039468564731 ) ) ;
#106599=CARTESIAN_POINT ( 'NONE',  ( -5.049401038298153566, 19.05341960407611168, 30.20724293864768839 ) ) ;
#106600=CARTESIAN_POINT ( 'NONE',  ( -5.153800228976328057, -19.02544592524343514, 82.29057627198103830 ) ) ;
#106601=CARTESIAN_POINT ( 'NONE',  ( 16.55341960407618274, -4.379528057220086978, 26.04275706135235779 ) ) ;
#106602=CARTESIAN_POINT ( 'NONE',  ( 0.05219959533910956823, 16.53943276465976808, 89.99890960531438111 ) ) ;
#106603=CARTESIAN_POINT ( 'NONE',  ( -5.153800228976328057, -19.02544592524343514, 57.29057627198103120 ) ) ;
#106604=CARTESIAN_POINT ( 'NONE',  ( -10.72451020669898014, 18.67979575497178502, 35.41557627198102409 ) ) ;
#106605=AXIS2_PLACEMENT_3D ( 'NONE', #34795, #172315, #157150 ) ;
#106606=CARTESIAN_POINT ( 'NONE',  ( -14.34966873604972548, 8.224510206698743886, 23.33442372801901499 ) ) ;
#106607=CARTESIAN_POINT ( 'NONE',  ( -21.53943276465977519, 0.05219959533907696930, 116.2489096053143669 ) ) ;
#106608=CARTESIAN_POINT ( 'NONE',  ( -5.823673210054431948, 21.52544592524334988, 67.70942372801901854 ) ) ;
#106609=CARTESIAN_POINT ( 'NONE',  ( 8.314922557961029526, -14.29746914071037800, 75.41775706135233293 ) ) ;
#106610=CARTESIAN_POINT ( 'NONE',  ( -4.379528057220086978, -16.55341960407618274, 74.79275706135234714 ) ) ;
#106611=ORIENTED_EDGE ( 'NONE', *, *, #119374, .F. ) ;
#106612=CARTESIAN_POINT ( 'NONE',  ( 19.05341960407611168, 5.049401038298154454, 58.95724293864768129 ) ) ;
#106613=CARTESIAN_POINT ( 'NONE',  ( -8.224510206698735004, -14.34966873604973081, 84.58442372801903275 ) ) ;
#106614=CARTESIAN_POINT ( 'NONE',  ( -19.05341960407617563, 5.049401038297882671, 43.54275706135232582 ) ) ;
#106616=CARTESIAN_POINT ( 'NONE',  ( 10.81492255796106328, -18.62759615963255655, 20.41775706135234714 ) ) ;
#106617=CARTESIAN_POINT ( 'NONE',  ( 12.14591786802309770, 12.06949235617756955, 64.37390960531435269 ) ) ;
#106618=CARTESIAN_POINT ( 'NONE',  ( -16.46253265017160317, 9.564922557960807481, 90.83224293864769550 ) ) ;
#106619=CARTESIAN_POINT ( 'NONE',  ( 14.29746914071037800, 8.314922557961029526, 86.66775706135234714 ) ) ;
#106620=CARTESIAN_POINT ( 'NONE',  ( -18.67979575497193778, 10.72451020669871902, 58.33442372801901143 ) ) ;
#106621=CARTESIAN_POINT ( 'NONE',  ( -16.55341960407617563, 4.379528057220093196, 28.54275706135234358 ) ) ;
#106622=CARTESIAN_POINT ( 'NONE',  ( 15.72974639402199770, -15.80617190586745480, 113.1239096053143953 ) ) ;
#106623=CARTESIAN_POINT ( 'NONE',  ( 12.14591786802309770, 12.06949235617756955, 64.37390960531435269 ) ) ;
#106624=EDGE_LOOP ( 'NONE', ( #85232, #43643, #169587, #102460, #60958, #28696, #68256, #99010, #41575, #91623, #24426, #101026, #106470, #143912, #100702, #124647, #25689, #127740, #43352, #120345, #69156, #53734, #11333, #50317, #9183, #169341, #27065, #182103, #193730, #147553, #97812, #171524, #180281, #13224, #53941, #72374, #42085, #154594, #186049, #26307, #67134, #181521 ) ) ;
#106625=CARTESIAN_POINT ( 'NONE',  ( -5.719274019375978568, 21.55341960407610458, 95.20724293864769550 ) ) ;
#106626=CARTESIAN_POINT ( 'NONE',  ( -8.314922557960811034, -14.29746914071050412, 37.08224293864768129 ) ) ;
#106629=CARTESIAN_POINT ( 'NONE',  ( -16.46253265017160317, 9.564922557960807481, 110.8322429386476955 ) ) ;
#106630=CARTESIAN_POINT ( 'NONE',  ( -15.80617190586768217, 15.72974639402176855, 33.12609039468569705 ) ) ;
#106631=CARTESIAN_POINT ( 'NONE',  ( -14.34966873604960291, -8.224510206698953496, 51.66557627198102409 ) ) ;
#106633=CARTESIAN_POINT ( 'NONE',  ( 16.46253265017160672, -9.564922557960803928, 58.33224293864769550 ) ) ;
#106634=CARTESIAN_POINT ( 'NONE',  ( 9.474510206698729675, 16.51473224551082808, 67.08442372801900433 ) ) ;
#106635=CARTESIAN_POINT ( 'NONE',  ( 5.049401038298161559, -19.05341960407611168, 97.70724293864766707 ) ) ;
#106637=CARTESIAN_POINT ( 'NONE',  ( -21.53943276465977519, 0.05219959533907696930, 51.24890960531436690 ) ) ;
#106639=CARTESIAN_POINT ( 'NONE',  ( -5.153800228976328057, -19.02544592524343514, 57.29057627198103120 ) ) ;
#106640=CARTESIAN_POINT ( 'NONE',  ( -4.483927247898782831, 16.52544592524335698, 42.70942372801901854 ) ) ;
#106641=CARTESIAN_POINT ( 'NONE',  ( -13.89961937509957401, -13.97604488694547875, 64.37609039468567573 ) ) ;
#106642=CARTESIAN_POINT ( 'NONE',  ( -10.72451020669898014, 18.67979575497178502, 115.4155762719810241 ) ) ;
#106643=CARTESIAN_POINT ( 'NONE',  ( -8.224510206698948167, 14.34966873604960824, 45.41557627198103830 ) ) ;
#106644=ORIENTED_EDGE ( 'NONE', *, *, #46491, .T. ) ;
#106645=CARTESIAN_POINT ( 'NONE',  ( -19.03943276465977164, 0.05219959533909376836, 96.24890960531436690 ) ) ;
#106646=CARTESIAN_POINT ( 'NONE',  ( 0.05219959533907565091, 21.53943276465977519, 74.99890960531435269 ) ) ;
#106647=CARTESIAN_POINT ( 'NONE',  ( -18.67979575497178146, -10.72451020669898902, 106.6655762719810383 ) ) ;
#106648=CARTESIAN_POINT ( 'NONE',  ( 16.52544592524335698, 4.483927247898782831, 41.45942372801901143 ) ) ;
#106649=CARTESIAN_POINT ( 'NONE',  ( 18.62759615963271287, -10.81492255796078972, 33.33224293864769550 ) ) ;
#106650=CARTESIAN_POINT ( 'NONE',  ( 15.80617190586769283, -15.72974639402175789, 105.6260903946856899 ) ) ;
#106651=CARTESIAN_POINT ( 'NONE',  ( -13.97604488694527625, -13.89961937509977652, 106.8739096053143669 ) ) ;
#106652=CARTESIAN_POINT ( 'NONE',  ( -5.153800228976328057, -19.02544592524343514, 42.29057627198101699 ) ) ;
#106653=CARTESIAN_POINT ( 'NONE',  ( -19.02544592524342804, 5.153800228976336051, 101.0405762719810241 ) ) ;
#106654=CARTESIAN_POINT ( 'NONE',  ( 9.564922557960805705, 16.46253265017160317, 74.58224293864769550 ) ) ;
#106655=CARTESIAN_POINT ( 'NONE',  ( -16.52544592524335698, -4.483927247898792601, 23.95942372801901143 ) ) ;
#106656=CARTESIAN_POINT ( 'NONE',  ( 16.29526858892907626, -7.335722546920038667, 86.70329402199736535 ) ) ;
#106657=CARTESIAN_POINT ( 'NONE',  ( -19.03943276465977164, -0.05219959533935918106, 58.75109039468566863 ) ) ;
#106658=CARTESIAN_POINT ( 'NONE',  ( -5.823673210054431948, 21.52544592524334988, 107.7094237280190328 ) ) ;
#106659=CARTESIAN_POINT ( 'NONE',  ( 5.719274019375991003, -21.55341960407610458, 37.70724293864769550 ) ) ;
#106660=CARTESIAN_POINT ( 'NONE',  ( 16.53943276465976808, 0.05219959533934440121, 101.2510903946856757 ) ) ;
#106662=CARTESIAN_POINT ( 'NONE',  ( 0.05219959533936267826, -19.03943276465977164, 80.00109039468567573 ) ) ;
#106663=CARTESIAN_POINT ( 'NONE',  ( 13.89961937509957401, 13.97604488694547697, 26.87609039468566507 ) ) ;
#106664=DIRECTION ( 'NONE',  ( -1.000000000000000000, -0.000000000000000000, -0.000000000000000000 ) ) ;
#106665=CARTESIAN_POINT ( 'NONE',  ( -16.51473224551069308, -9.474510206698971260, 46.66557627198102409 ) ) ;
#106666=CARTESIAN_POINT ( 'NONE',  ( -16.53943276465976808, 0.05219959533911058130, 36.24890960531435979 ) ) ;
#106667=CARTESIAN_POINT ( 'NONE',  ( -0.05219959533909027116, -19.03943276465977164, 27.49890960531435624 ) ) ;
#106668=CARTESIAN_POINT ( 'NONE',  ( 16.52544592524342804, -4.483927247898539470, 23.54057627198102765 ) ) ;
#106669=CARTESIAN_POINT ( 'NONE',  ( 17.50000000000000000, -5.499999999999992895, 46.21769037696434168 ) ) ;
#106670=CARTESIAN_POINT ( 'NONE',  ( -4.379528057220086978, -16.55341960407618274, 94.79275706135234714 ) ) ;
#106671=CARTESIAN_POINT ( 'NONE',  ( -13.97604488694527625, -13.89961937509977652, 46.87390960531435979 ) ) ;
#106672=CARTESIAN_POINT ( 'NONE',  ( 15.72974639402176855, 15.80617190586768217, 101.8760903946857042 ) ) ;
#106673=CARTESIAN_POINT ( 'NONE',  ( -9.474510206698720793, -16.51473224551083518, 109.5844237280190043 ) ) ;
#106674=CARTESIAN_POINT ( 'NONE',  ( -0.05219959533937732626, 21.53943276465977519, 87.50109039468568994 ) ) ;
#106676=CARTESIAN_POINT ( 'NONE',  ( -19.02544592524334988, -5.153800228976617603, 68.95942372801896170 ) ) ;
#106677=CARTESIAN_POINT ( 'NONE',  ( -0.05219959533909027116, -19.03943276465977164, 97.49890960531436690 ) ) ;
#106678=CARTESIAN_POINT ( 'NONE',  ( 19.02544592524343514, -5.153800228976328945, 83.54057627198100988 ) ) ;
#106680=CARTESIAN_POINT ( 'NONE',  ( -18.62759615963270932, 10.81492255796079327, 110.8322429386476955 ) ) ;
#106681=CARTESIAN_POINT ( 'NONE',  ( -4.483927247898539470, -16.52544592524342804, 62.29057627198102409 ) ) ;
#106682=CARTESIAN_POINT ( 'NONE',  ( -10.81492255796078084, -18.62759615963271287, 57.08224293864769550 ) ) ;
#106683=CARTESIAN_POINT ( 'NONE',  ( 16.51473224551069308, 9.474510206698969483, 54.16557627198103120 ) ) ;
#106684=CARTESIAN_POINT ( 'NONE',  ( 21.52544592524344225, -5.823673210054117533, 93.54057627198103830 ) ) ;
#106685=CARTESIAN_POINT ( 'NONE',  ( 14.34966873604972726, -8.224510206698740333, 85.83442372801901854 ) ) ;
#106687=CARTESIAN_POINT ( 'NONE',  ( -19.05341960407611168, -5.049401038298163336, 61.45724293864769550 ) ) ;
#106688=CARTESIAN_POINT ( 'NONE',  ( 8.314922557960818139, 14.29746914071049879, 89.58224293864768129 ) ) ;
#106690=CARTESIAN_POINT ( 'NONE',  ( 0.05219959533909260263, 19.03943276465977164, 54.99890960531435979 ) ) ;
#106691=CARTESIAN_POINT ( 'NONE',  ( 9.474510206698729675, 16.51473224551082808, 82.08442372801899012 ) ) ;
#106692=CARTESIAN_POINT ( 'NONE',  ( -12.14591786802309592, -12.06949235617757132, 81.87390960531435269 ) ) ;
#106693=CARTESIAN_POINT ( 'NONE',  ( 10.72451020669871369, 18.67979575497193778, 62.08442372801901143 ) ) ;
#106694=CARTESIAN_POINT ( 'NONE',  ( -5.049401038298153566, 19.05341960407611168, 35.20724293864768839 ) ) ;
#106695=CARTESIAN_POINT ( 'NONE',  ( 10.72451020669898902, -18.67979575497178502, 97.91557627198103830 ) ) ;
#106696=CARTESIAN_POINT ( 'NONE',  ( 12.14591786802309770, 12.06949235617756955, 104.3739096053143669 ) ) ;
#106698=CARTESIAN_POINT ( 'NONE',  ( -19.02544592524342804, 5.153800228976336051, 56.04057627198100988 ) ) ;
#106700=CARTESIAN_POINT ( 'NONE',  ( 5.049401038297881783, 19.05341960407617563, 97.29275706135233293 ) ) ;
#106701=CARTESIAN_POINT ( 'NONE',  ( -19.02544592524342804, 5.153800228976336051, 111.0405762719810099 ) ) ;
#106702=CARTESIAN_POINT ( 'NONE',  ( 18.67979575497194134, -10.72451020669871369, 35.83442372801901143 ) ) ;
#106703=CARTESIAN_POINT ( 'NONE',  ( 13.97604488694527802, 13.89961937509977652, 89.37390960531436690 ) ) ;
#106704=CARTESIAN_POINT ( 'NONE',  ( 13.89961937509957401, 13.97604488694547697, 66.87609039468567573 ) ) ;
#106705=CARTESIAN_POINT ( 'NONE',  ( 19.03943276465977164, -0.05219959533909143690, 53.74890960531436690 ) ) ;
#106706=CARTESIAN_POINT ( 'NONE',  ( -16.52544592524342804, 4.483927247898546575, 81.04057627198102409 ) ) ;
#106707=CARTESIAN_POINT ( 'NONE',  ( -16.53943276465976808, 0.05219959533911058130, 71.24890960531435269 ) ) ;
#106708=CARTESIAN_POINT ( 'NONE',  ( -16.46253265017160317, 9.564922557960807481, 90.83224293864769550 ) ) ;
#106709=CARTESIAN_POINT ( 'NONE',  ( 0.05219959533910956823, 16.53943276465976808, 74.99890960531435269 ) ) ;
#106710=CARTESIAN_POINT ( 'NONE',  ( 9.564922557960805705, 16.46253265017160317, 79.58224293864769550 ) ) ;
#106711=CARTESIAN_POINT ( 'NONE',  ( 13.89961937509957401, 13.97604488694547697, 36.87609039468565442 ) ) ;
#106712=CARTESIAN_POINT ( 'NONE',  ( 5.049401038298161559, -19.05341960407611168, 52.70724293864767418 ) ) ;
#106713=CARTESIAN_POINT ( 'NONE',  ( -16.55341960407611168, -4.379528057220339221, 31.45724293864769550 ) ) ;
#106714=CARTESIAN_POINT ( 'NONE',  ( -14.29746914071049879, 8.314922557960819915, 105.8322429386476955 ) ) ;
#106716=CARTESIAN_POINT ( 'NONE',  ( 21.55341960407619695, -5.719274019375665929, 46.04275706135234714 ) ) ;
#106717=CARTESIAN_POINT ( 'NONE',  ( 0.05219959533936267826, -19.03943276465977164, 70.00109039468566152 ) ) ;
#106718=CARTESIAN_POINT ( 'NONE',  ( -4.379528057220328563, 16.55341960407611168, 35.20724293864768839 ) ) ;
#106719=CARTESIAN_POINT ( 'NONE',  ( -15.80617190586745835, -15.72974639402198527, 86.87390960531438111 ) ) ;
#106720=CARTESIAN_POINT ( 'NONE',  ( -9.564922557960796823, -16.46253265017161027, 112.0822429386476955 ) ) ;
#106721=CARTESIAN_POINT ( 'NONE',  ( -14.34966873604960291, -8.224510206698953496, 71.66557627198100988 ) ) ;
#106722=CARTESIAN_POINT ( 'NONE',  ( 19.03943276465977164, -0.05219959533909143690, 38.74890960531436690 ) ) ;
#106723=CARTESIAN_POINT ( 'NONE',  ( -16.51473224551082808, 9.474510206698731452, 33.33442372801899722 ) ) ;
#106724=CARTESIAN_POINT ( 'NONE',  ( -16.52544592524335698, -4.483927247898792601, 98.95942372801903275 ) ) ;
#106725=CARTESIAN_POINT ( 'NONE',  ( -4.379528057220086978, -16.55341960407618274, 59.79275706135234714 ) ) ;
#106726=CARTESIAN_POINT ( 'NONE',  ( -18.62759615963270932, 10.81492255796079327, 30.83224293864770260 ) ) ;
#106727=CARTESIAN_POINT ( 'NONE',  ( -10.81492255796105439, 18.62759615963255655, 107.9177570613523471 ) ) ;
#106728=CARTESIAN_POINT ( 'NONE',  ( -16.46253265017160317, 9.564922557960807481, 90.83224293864769550 ) ) ;
#106729=CARTESIAN_POINT ( 'NONE',  ( -4.379528057220086978, -16.55341960407618274, 69.79275706135234714 ) ) ;
#106730=CARTESIAN_POINT ( 'NONE',  ( -16.51473224551069308, -9.474510206698971260, 26.66557627198103120 ) ) ;
#106731=CARTESIAN_POINT ( 'NONE',  ( 16.53943276465976808, -0.05219959533910856209, 28.74890960531435624 ) ) ;
#106732=CARTESIAN_POINT ( 'NONE',  ( 9.474510206698971260, -16.51473224551069308, 102.9155762719810241 ) ) ;
#106733=CARTESIAN_POINT ( 'NONE',  ( 5.153800228976335163, 19.02544592524342804, 89.79057627198102409 ) ) ;
#106734=CARTESIAN_POINT ( 'NONE',  ( 18.62759615963271287, -10.81492255796078972, 23.33224293864769194 ) ) ;
#106735=CARTESIAN_POINT ( 'NONE',  ( 8.314922557960818139, 14.29746914071049879, 64.58224293864769550 ) ) ;
#106736=CARTESIAN_POINT ( 'NONE',  ( 14.29746914071049879, -8.314922557960816363, 38.33224293864768839 ) ) ;
#106737=CARTESIAN_POINT ( 'NONE',  ( 14.34966873604960469, 8.224510206698951720, 54.16557627198103120 ) ) ;
#106738=CARTESIAN_POINT ( 'NONE',  ( -16.52544592524335698, -4.483927247898792601, 48.95942372801902565 ) ) ;
#106740=CARTESIAN_POINT ( 'NONE',  ( -13.97604488694547697, 13.89961937509957934, 48.12609039468566863 ) ) ;
#106741=CARTESIAN_POINT ( 'NONE',  ( -16.46253265017160317, 9.564922557960807481, 90.83224293864769550 ) ) ;
#106742=CARTESIAN_POINT ( 'NONE',  ( -5.049401038297874678, -19.05341960407617918, 64.79275706135233293 ) ) ;
#106744=CARTESIAN_POINT ( 'NONE',  ( -16.51473224551082808, 9.474510206698731452, 53.33442372801900433 ) ) ;
#106745=CARTESIAN_POINT ( 'NONE',  ( -9.564922557961040184, 16.46253265017147172, 92.91775706135233293 ) ) ;
#106746=CARTESIAN_POINT ( 'NONE',  ( 4.379528057220092307, 16.55341960407617563, 77.29275706135234714 ) ) ;
#106748=CARTESIAN_POINT ( 'NONE',  ( -19.02544592524342804, 5.153800228976336051, 26.04057627198103120 ) ) ;
#106749=CARTESIAN_POINT ( 'NONE',  ( 15.72974639402199770, -15.80617190586745480, 28.12390960531435979 ) ) ;
#106750=CARTESIAN_POINT ( 'NONE',  ( 5.823673210054444382, -21.52544592524334988, 40.20942372801901854 ) ) ;
#106751=CARTESIAN_POINT ( 'NONE',  ( 19.02544592524334988, 5.153800228976608722, 101.4594237280189759 ) ) ;
#106753=CARTESIAN_POINT ( 'NONE',  ( 5.049401038298161559, -19.05341960407611168, 62.70724293864769550 ) ) ;
#106754=CARTESIAN_POINT ( 'NONE',  ( 19.02544592524343514, -5.153800228976328945, 108.5405762719810383 ) ) ;
#106755=CARTESIAN_POINT ( 'NONE',  ( 12.06949235617757843, -12.14591786802309237, 78.12390960531436690 ) ) ;
#106756=CARTESIAN_POINT ( 'NONE',  ( 9.564922557960805705, 16.46253265017160317, 64.58224293864769550 ) ) ;
#106757=CARTESIAN_POINT ( 'NONE',  ( 9.564922557960805705, 16.46253265017160317, 69.58224293864770971 ) ) ;
#106758=CARTESIAN_POINT ( 'NONE',  ( -19.05341960407617563, 5.049401038297882671, 78.54275706135233293 ) ) ;
#106759=CARTESIAN_POINT ( 'NONE',  ( -21.52544592524343514, 5.823673210054127303, 56.04057627198102409 ) ) ;
#106760=CARTESIAN_POINT ( 'NONE',  ( 8.224510206698953496, -14.34966873604960469, 107.9155762719810241 ) ) ;
#106761=CARTESIAN_POINT ( 'NONE',  ( -16.51473224551082808, 9.474510206698731452, 38.33442372801899722 ) ) ;
#106762=CARTESIAN_POINT ( 'NONE',  ( -13.89961937509977652, 13.97604488694528158, 85.62390960531433848 ) ) ;
#106763=CARTESIAN_POINT ( 'NONE',  ( -18.67979575497178146, -10.72451020669898902, 76.66557627198103830 ) ) ;
#106764=CARTESIAN_POINT ( 'NONE',  ( -12.06949235617756955, 12.14591786802309770, 80.62390960531438111 ) ) ;
#106765=CARTESIAN_POINT ( 'NONE',  ( 19.02544592524334988, 5.153800228976608722, 46.45942372801899012 ) ) ;
#106766=CARTESIAN_POINT ( 'NONE',  ( -15.72974639402197994, 15.80617190586746368, 80.62390960531438111 ) ) ;
#106767=CARTESIAN_POINT ( 'NONE',  ( 0.05219959533907565091, 21.53943276465977519, 64.99890960531435269 ) ) ;
#106768=CARTESIAN_POINT ( 'NONE',  ( 21.52544592524344225, -5.823673210054117533, 33.54057627198102409 ) ) ;
#106769=CARTESIAN_POINT ( 'NONE',  ( 18.62759615963255655, 10.81492255796105972, 96.66775706135234714 ) ) ;
#106770=CARTESIAN_POINT ( 'NONE',  ( -0.05219959533909027116, -19.03943276465977164, 72.49890960531435269 ) ) ;
#106771=CARTESIAN_POINT ( 'NONE',  ( -12.06949235617756955, 12.14591786802309770, 110.6239096053143669 ) ) ;
#106773=CARTESIAN_POINT ( 'NONE',  ( -10.72451020669870658, -18.67979575497194134, 29.58442372801901854 ) ) ;
#106774=CARTESIAN_POINT ( 'NONE',  ( 5.719274019375673035, 21.55341960407619339, 47.29275706135234003 ) ) ;
#106775=CARTESIAN_POINT ( 'NONE',  ( 9.564922557960805705, 16.46253265017160317, 34.58224293864770260 ) ) ;
#106776=CARTESIAN_POINT ( 'NONE',  ( -15.80617190586745835, -15.72974639402198527, 111.8739096053143669 ) ) ;
#106777=CARTESIAN_POINT ( 'NONE',  ( -19.05341960407617563, 5.049401038297882671, 48.54275706135233293 ) ) ;
#106778=CARTESIAN_POINT ( 'NONE',  ( -19.03943276465977164, 0.05219959533909376836, 36.24890960531436690 ) ) ;
#106779=CARTESIAN_POINT ( 'NONE',  ( 19.03943276465977164, -0.05219959533909143690, 23.74890960531435269 ) ) ;
#106781=CARTESIAN_POINT ( 'NONE',  ( -8.224510206698735004, -14.34966873604973081, 54.58442372801901143 ) ) ;
#106782=CARTESIAN_POINT ( 'NONE',  ( 16.46253265017160672, -9.564922557960803928, 23.33224293864769194 ) ) ;
#106784=CARTESIAN_POINT ( 'NONE',  ( -19.03943276465977164, 0.05219959533909376836, 81.24890960531436690 ) ) ;
#106785=CARTESIAN_POINT ( 'NONE',  ( -8.314922557960811034, -14.29746914071050412, 102.0822429386476955 ) ) ;
#106787=CARTESIAN_POINT ( 'NONE',  ( 18.62759615963271287, -10.81492255796078972, 63.33224293864770260 ) ) ;
#106788=CARTESIAN_POINT ( 'NONE',  ( -4.483927247898782831, 16.52544592524335698, 42.70942372801901854 ) ) ;
#106789=CARTESIAN_POINT ( 'NONE',  ( 10.81492255796106328, -18.62759615963255655, 100.4177570613523471 ) ) ;
#106790=CARTESIAN_POINT ( 'NONE',  ( 5.153800228976335163, 19.02544592524342804, 24.79057627198102765 ) ) ;
#106791=CARTESIAN_POINT ( 'NONE',  ( -0.05219959533934338120, 16.53943276465976808, 107.5010903946856899 ) ) ;
#106792=CARTESIAN_POINT ( 'NONE',  ( 14.29746914071049879, -8.314922557960816363, 53.33224293864769550 ) ) ;
#106793=CARTESIAN_POINT ( 'NONE',  ( -0.05219959533909027116, -19.03943276465977164, 62.49890960531435979 ) ) ;
#106794=CARTESIAN_POINT ( 'NONE',  ( -21.55341960407619339, 5.719274019375674811, 113.5427570613523756 ) ) ;
#106795=CARTESIAN_POINT ( 'NONE',  ( -10.72451020669870658, -18.67979575497194134, 19.58442372801901143 ) ) ;
#106796=CARTESIAN_POINT ( 'NONE',  ( -18.67979575497193778, 10.72451020669871902, 73.33442372801901854 ) ) ;
#106797=CARTESIAN_POINT ( 'NONE',  ( -12.06949235617739369, -12.14591786802326823, 59.37609039468568284 ) ) ;
#106798=CARTESIAN_POINT ( 'NONE',  ( -14.29746914071037622, -8.314922557961029526, 34.16775706135234714 ) ) ;
#106799=CARTESIAN_POINT ( 'NONE',  ( -16.53943276465976808, 0.05219959533911058130, 81.24890960531436690 ) ) ;
#106800=CARTESIAN_POINT ( 'NONE',  ( 21.52544592524334988, 5.823673210054432836, 101.4594237280190185 ) ) ;
#106801=CARTESIAN_POINT ( 'NONE',  ( 8.314922557960818139, 14.29746914071049879, 29.58224293864769905 ) ) ;
#106802=CARTESIAN_POINT ( 'NONE',  ( -16.88567814943160528, 6.947325034625694506, 113.7099887734741799 ) ) ;
#106803=CARTESIAN_POINT ( 'NONE',  ( 14.34966873604972726, -8.224510206698740333, 35.83442372801901143 ) ) ;
#106804=CARTESIAN_POINT ( 'NONE',  ( 0.05219959533910956823, 16.53943276465976808, 44.99890960531435979 ) ) ;
#106805=CARTESIAN_POINT ( 'NONE',  ( 4.379528057220092307, 16.55341960407617563, 82.29275706135234714 ) ) ;
#106806=CARTESIAN_POINT ( 'NONE',  ( 16.46253265017160672, -9.564922557960803928, 93.33224293864769550 ) ) ;
#106807=CARTESIAN_POINT ( 'NONE',  ( 19.02544592524343514, -5.153800228976328945, 113.5405762719810241 ) ) ;
#106808=CARTESIAN_POINT ( 'NONE',  ( 18.62759615963255655, 10.81492255796105972, 101.6677570613523613 ) ) ;
#106809=CARTESIAN_POINT ( 'NONE',  ( 14.34966873604972726, -8.224510206698740333, 100.8344237280190185 ) ) ;
#106810=CARTESIAN_POINT ( 'NONE',  ( -12.06949235617756955, 12.14591786802309770, 85.62390960531436690 ) ) ;
#106811=CARTESIAN_POINT ( 'NONE',  ( 5.153800228976335163, 19.02544592524342804, 84.79057627198099567 ) ) ;
#106813=CARTESIAN_POINT ( 'NONE',  ( 8.314922557961029526, -14.29746914071037800, 40.41775706135234714 ) ) ;
#106814=CARTESIAN_POINT ( 'NONE',  ( -16.51473224551069308, -9.474510206698971260, 46.66557627198102409 ) ) ;
#106815=CARTESIAN_POINT ( 'NONE',  ( -16.46253265017160317, 9.564922557960807481, 105.8322429386476955 ) ) ;
#106816=CARTESIAN_POINT ( 'NONE',  ( 0.05219959533934541429, -16.53943276465976808, 45.00109039468568284 ) ) ;
#106818=CARTESIAN_POINT ( 'NONE',  ( 13.97604488694548053, -13.89961937509957401, 30.62609039468566863 ) ) ;
#106819=CARTESIAN_POINT ( 'NONE',  ( -12.14591786802326823, 12.06949235617739902, 103.1260903946856757 ) ) ;
#106820=CARTESIAN_POINT ( 'NONE',  ( -16.46253265017160317, 9.564922557960807481, 30.83224293864769550 ) ) ;
#106821=CARTESIAN_POINT ( 'NONE',  ( 16.55341960407618274, -4.379528057220086978, 76.04275706135237556 ) ) ;
#106822=CARTESIAN_POINT ( 'NONE',  ( -19.03943276465977164, -0.05219959533935918106, 83.75109039468567573 ) ) ;
#106823=CARTESIAN_POINT ( 'NONE',  ( -19.02544592524334988, -5.153800228976617603, 33.95942372801897591 ) ) ;
#106824=CARTESIAN_POINT ( 'NONE',  ( 5.153800228976335163, 19.02544592524342804, 64.79057627198100988 ) ) ;
#106825=CARTESIAN_POINT ( 'NONE',  ( 8.224510206698953496, -14.34966873604960469, 97.91557627198103830 ) ) ;
#106826=CARTESIAN_POINT ( 'NONE',  ( -5.049401038297874678, -19.05341960407617918, 74.79275706135231871 ) ) ;
#106827=CARTESIAN_POINT ( 'NONE',  ( -5.823673210054116645, -21.52544592524344225, 62.29057627198102409 ) ) ;
#106828=CARTESIAN_POINT ( 'NONE',  ( 16.51473224551083163, -9.474510206698727899, 30.83442372801900433 ) ) ;
#106829=CARTESIAN_POINT ( 'NONE',  ( 13.89961937509977652, -13.97604488694527269, 103.1239096053143527 ) ) ;
#106830=CARTESIAN_POINT ( 'NONE',  ( -21.52544592524343514, 5.823673210054127303, 76.04057627198102409 ) ) ;
#106831=CARTESIAN_POINT ( 'NONE',  ( -19.05341960407611168, -5.049401038298163336, 111.4572429386476671 ) ) ;
#106832=CARTESIAN_POINT ( 'NONE',  ( 16.46253265017146816, 9.564922557961045513, 101.6677570613523329 ) ) ;
#106834=CARTESIAN_POINT ( 'NONE',  ( 16.53943276465976808, 0.05219959533934440121, 21.25109039468567218 ) ) ;
#106835=CARTESIAN_POINT ( 'NONE',  ( -9.564922557960796823, -16.46253265017161027, 27.08224293864769550 ) ) ;
#106836=CARTESIAN_POINT ( 'NONE',  ( 19.03943276465977164, -0.05219959533909143690, 93.74890960531435269 ) ) ;
#106837=CARTESIAN_POINT ( 'NONE',  ( 18.62759615963271287, -10.81492255796078972, 88.33224293864769550 ) ) ;
#106838=CARTESIAN_POINT ( 'NONE',  ( 16.55341960407618274, -4.379528057220086978, 61.04275706135234714 ) ) ;
#106839=CARTESIAN_POINT ( 'NONE',  ( -10.81492255796105439, 18.62759615963255655, 57.91775706135234714 ) ) ;
#106840=CARTESIAN_POINT ( 'NONE',  ( -5.153800228976607833, 19.02544592524334988, 107.7094237280189759 ) ) ;
#106841=CARTESIAN_POINT ( 'NONE',  ( -5.719274019375665041, -21.55341960407619695, 109.7927570613523613 ) ) ;
#106842=CARTESIAN_POINT ( 'NONE',  ( -0.05219959533934338120, 16.53943276465976808, 107.5010903946856899 ) ) ;
#106843=CARTESIAN_POINT ( 'NONE',  ( 15.72974639402199770, -15.80617190586745480, 103.1239096053143811 ) ) ;
#106844=CARTESIAN_POINT ( 'NONE',  ( 16.52544592524342804, -4.483927247898539470, 38.54057627198103120 ) ) ;
#106845=CARTESIAN_POINT ( 'NONE',  ( -16.46253265017146816, -9.564922557961047289, 84.16775706135233293 ) ) ;
#106846=CARTESIAN_POINT ( 'NONE',  ( -10.72451020669870658, -18.67979575497194134, 54.58442372801901143 ) ) ;
#106847=CARTESIAN_POINT ( 'NONE',  ( -16.46253265017146816, -9.564922557961047289, 34.16775706135233293 ) ) ;
#106848=CARTESIAN_POINT ( 'NONE',  ( -12.14591786802309592, -12.06949235617757132, 106.8739096053143811 ) ) ;
#106849=CARTESIAN_POINT ( 'NONE',  ( 21.53943276465977519, -0.05219959533907433946, 28.74890960531435624 ) ) ;
#106850=CARTESIAN_POINT ( 'NONE',  ( 12.14591786802309770, 12.06949235617756955, 34.37390960531435979 ) ) ;
#106851=CARTESIAN_POINT ( 'NONE',  ( 21.55341960407619695, -5.719274019375665929, 96.04275706135236135 ) ) ;
#106852=CARTESIAN_POINT ( 'NONE',  ( 12.06949235617739724, 12.14591786802326823, 66.87609039468568994 ) ) ;
#106853=CARTESIAN_POINT ( 'NONE',  ( -12.14591786802309592, -12.06949235617757132, 31.87390960531435979 ) ) ;
#106854=CARTESIAN_POINT ( 'NONE',  ( -15.80617190586768217, 15.72974639402176855, 68.12609039468567573 ) ) ;
#106855=CARTESIAN_POINT ( 'NONE',  ( -18.62759615963255300, -10.81492255796106328, 54.16775706135235424 ) ) ;
#106857=CARTESIAN_POINT ( 'NONE',  ( -9.564922557960796823, -16.46253265017161027, 62.08224293864769550 ) ) ;
#106858=CARTESIAN_POINT ( 'NONE',  ( -15.72974639402176322, -15.80617190586768395, 49.37609039468569705 ) ) ;
#106859=CARTESIAN_POINT ( 'NONE',  ( 16.52544592524342804, -4.483927247898539470, 113.5405762719810383 ) ) ;
#106860=CARTESIAN_POINT ( 'NONE',  ( 9.564922557960805705, 16.46253265017160317, 44.58224293864769550 ) ) ;
#106861=CARTESIAN_POINT ( 'NONE',  ( -12.06949235617756955, 12.14591786802309770, 80.62390960531438111 ) ) ;
#106862=CARTESIAN_POINT ( 'NONE',  ( -5.153800228976328057, -19.02544592524343514, 87.29057627198103830 ) ) ;
#106863=CARTESIAN_POINT ( 'NONE',  ( -14.29746914071049879, 8.314922557960819915, 25.83224293864769194 ) ) ;
#106864=CARTESIAN_POINT ( 'NONE',  ( 5.719274019375991003, -21.55341960407610458, 62.70724293864769550 ) ) ;
#106865=CARTESIAN_POINT ( 'NONE',  ( -15.80617190586745835, -15.72974639402198527, 106.8739096053143811 ) ) ;
#106866=CARTESIAN_POINT ( 'NONE',  ( -13.97604488694527625, -13.89961937509977652, 106.8739096053143669 ) ) ;
#106867=CARTESIAN_POINT ( 'NONE',  ( 9.564922557960805705, 16.46253265017160317, 64.58224293864769550 ) ) ;
#106868=CARTESIAN_POINT ( 'NONE',  ( 13.97604488694548053, -13.89961937509957401, 105.6260903946856757 ) ) ;
#106870=CARTESIAN_POINT ( 'NONE',  ( 5.719274019375991003, -21.55341960407610458, 52.70724293864769550 ) ) ;
#106871=CARTESIAN_POINT ( 'NONE',  ( 5.823673210054444382, -21.52544592524334988, 75.20942372801901854 ) ) ;
#106872=CARTESIAN_POINT ( 'NONE',  ( -16.46253265017160317, 9.564922557960807481, 70.83224293864770971 ) ) ;
#106873=CARTESIAN_POINT ( 'NONE',  ( 19.02544592524343514, -5.153800228976328945, 103.5405762719809957 ) ) ;
#106874=CARTESIAN_POINT ( 'NONE',  ( 8.314922557961029526, -14.29746914071037800, 70.41775706135236135 ) ) ;
#106875=CARTESIAN_POINT ( 'NONE',  ( -0.05219959533937732626, 21.53943276465977519, 57.50109039468568994 ) ) ;
#106876=CARTESIAN_POINT ( 'NONE',  ( 21.53943276465977519, 0.05219959533937863772, 91.25109039468568994 ) ) ;
#106877=CARTESIAN_POINT ( 'NONE',  ( -10.72451020669898014, 18.67979575497178502, 110.4155762719810383 ) ) ;
#106878=CARTESIAN_POINT ( 'NONE',  ( 16.52544592524335698, 4.483927247898782831, 81.45942372801900433 ) ) ;
#106879=CARTESIAN_POINT ( 'NONE',  ( -18.62759615963270932, 10.81492255796079327, 70.83224293864770971 ) ) ;
#106880=CARTESIAN_POINT ( 'NONE',  ( -19.05341960407617563, 5.049401038297882671, 53.54275706135231871 ) ) ;
#106881=CARTESIAN_POINT ( 'NONE',  ( -0.05219959533907301413, -21.53943276465977519, 42.49890960531435979 ) ) ;
#106882=CARTESIAN_POINT ( 'NONE',  ( -19.05341960407611168, -5.049401038298163336, 81.45724293864769550 ) ) ;
#106883=CARTESIAN_POINT ( 'NONE',  ( 16.53943276465976808, -0.05219959533910856209, 28.74890960531435624 ) ) ;
#106885=CARTESIAN_POINT ( 'NONE',  ( -21.53943276465977519, 0.05219959533907696930, 21.24890960531436690 ) ) ;
#106887=CARTESIAN_POINT ( 'NONE',  ( -13.89961937509957401, -13.97604488694547875, 89.37609039468563310 ) ) ;
#106888=CARTESIAN_POINT ( 'NONE',  ( 21.53943276465977519, -0.05219959533907433946, 68.74890960531435269 ) ) ;
#106889=CARTESIAN_POINT ( 'NONE',  ( -16.55341960407611168, -4.379528057220339221, 51.45724293864770260 ) ) ;
#106890=CARTESIAN_POINT ( 'NONE',  ( -19.03943276465977164, -0.05219959533935918106, 108.7510903946856615 ) ) ;
#106891=CARTESIAN_POINT ( 'NONE',  ( 9.564922557960805705, 16.46253265017160317, 39.58224293864768839 ) ) ;
#106892=CARTESIAN_POINT ( 'NONE',  ( 10.81492255796078972, 18.62759615963270932, 99.58224293864770971 ) ) ;
#106893=CARTESIAN_POINT ( 'NONE',  ( -5.153800228976607833, 19.02544592524334988, 77.70942372801900433 ) ) ;
#106894=CARTESIAN_POINT ( 'NONE',  ( -13.89961937509977652, 13.97604488694528158, 80.62390960531436690 ) ) ;
#106895=CARTESIAN_POINT ( 'NONE',  ( -4.379528057220328563, 16.55341960407611168, 90.20724293864770971 ) ) ;
#106896=CARTESIAN_POINT ( 'NONE',  ( 5.049401038298161559, -19.05341960407611168, 57.70724293864769550 ) ) ;
#106897=CARTESIAN_POINT ( 'NONE',  ( -16.53943276465976808, 0.05219959533911058130, 61.24890960531435979 ) ) ;
#106898=CARTESIAN_POINT ( 'NONE',  ( 0.05219959533909260263, 19.03943276465977164, 34.99890960531435979 ) ) ;
#106899=CARTESIAN_POINT ( 'NONE',  ( -16.99472585857189699, -5.499999999999960032, 20.67116795353343051 ) ) ;
#106900=CARTESIAN_POINT ( 'NONE',  ( -16.53943276465976808, 0.05219959533911058130, 41.24890960531435269 ) ) ;
#106901=CARTESIAN_POINT ( 'NONE',  ( -16.46253265017160317, 9.564922557960807481, 95.83224293864769550 ) ) ;
#106903=CARTESIAN_POINT ( 'NONE',  ( -19.02544592524334988, -5.153800228976617603, 48.95942372801900433 ) ) ;
#106904=CARTESIAN_POINT ( 'NONE',  ( 14.29746914071037800, 8.314922557961029526, 61.66775706135235424 ) ) ;
#106905=CARTESIAN_POINT ( 'NONE',  ( 21.52544592524344225, -5.823673210054117533, 68.54057627198103830 ) ) ;
#106906=CARTESIAN_POINT ( 'NONE',  ( 13.97604488694548053, -13.89961937509957401, 35.62609039468567573 ) ) ;
#106907=CARTESIAN_POINT ( 'NONE',  ( 16.46253265017160672, -9.564922557960803928, 88.33224293864769550 ) ) ;
#106909=CARTESIAN_POINT ( 'NONE',  ( -21.53943276465977519, 0.05219959533907696930, 26.24890960531435624 ) ) ;
#106910=CARTESIAN_POINT ( 'NONE',  ( -9.474510206698964154, 16.51473224551069663, 65.41557627198102409 ) ) ;
#106911=CARTESIAN_POINT ( 'NONE',  ( -10.81492255796105439, 18.62759615963255655, 47.91775706135234714 ) ) ;
#106912=CARTESIAN_POINT ( 'NONE',  ( -16.53943276465976808, 0.05219959533911058130, 116.2489096053143669 ) ) ;
#106913=CARTESIAN_POINT ( 'NONE',  ( 15.72974639402199770, -15.80617190586745480, 113.1239096053143953 ) ) ;
#106914=CARTESIAN_POINT ( 'NONE',  ( 13.97604488694527802, 13.89961937509977652, 89.37390960531436690 ) ) ;
#106916=CARTESIAN_POINT ( 'NONE',  ( 10.81492255796106328, -18.62759615963255655, 35.41775706135234003 ) ) ;
#106918=CARTESIAN_POINT ( 'NONE',  ( 16.51473224551069308, 9.474510206698969483, 99.16557627198102409 ) ) ;
#106920=CARTESIAN_POINT ( 'NONE',  ( -5.823673210054116645, -21.52544592524344225, 112.2905762719810241 ) ) ;
#106921=CARTESIAN_POINT ( 'NONE',  ( -5.049401038298153566, 19.05341960407611168, 45.20724293864769550 ) ) ;
#106922=CARTESIAN_POINT ( 'NONE',  ( 14.34966873604972726, -8.224510206698740333, 25.83442372801901499 ) ) ;
#106924=CARTESIAN_POINT ( 'NONE',  ( 5.153800228976335163, 19.02544592524342804, 24.79057627198102765 ) ) ;
#106925=CARTESIAN_POINT ( 'NONE',  ( -15.72974639402176322, -15.80617190586768395, 99.37609039468568994 ) ) ;
#106926=CARTESIAN_POINT ( 'NONE',  ( 0.05219959533909260263, 19.03943276465977164, 69.99890960531435269 ) ) ;
#106927=CARTESIAN_POINT ( 'NONE',  ( 21.55341960407619695, -5.719274019375665929, 46.04275706135234714 ) ) ;
#106929=CARTESIAN_POINT ( 'NONE',  ( -13.97604488694527625, -13.89961937509977652, 96.87390960531433848 ) ) ;
#106931=CARTESIAN_POINT ( 'NONE',  ( 4.483927247898790824, -16.52544592524335698, 40.20942372801901854 ) ) ;
#106932=CARTESIAN_POINT ( 'NONE',  ( 12.14591786802327356, -12.06949235617739191, 65.62609039468568994 ) ) ;
#106933=CARTESIAN_POINT ( 'NONE',  ( -5.823673210054431948, 21.52544592524334988, 57.70942372801901143 ) ) ;
#106934=CARTESIAN_POINT ( 'NONE',  ( 21.53943276465977519, 0.05219959533937863772, 86.25109039468568994 ) ) ;
#106936=CARTESIAN_POINT ( 'NONE',  ( 0.05219959533936267826, -19.03943276465977164, 105.0010903946856615 ) ) ;
#106937=CARTESIAN_POINT ( 'NONE',  ( 13.89961937509977652, -13.97604488694527269, 73.12390960531436690 ) ) ;
#106938=CARTESIAN_POINT ( 'NONE',  ( -13.89961937509977652, 13.97604488694528158, 100.6239096053143669 ) ) ;
#106939=CARTESIAN_POINT ( 'NONE',  ( 14.34966873604960469, 8.224510206698951720, 109.1655762719810383 ) ) ;
#106940=CARTESIAN_POINT ( 'NONE',  ( -21.55341960407610458, -5.719274019375992779, 31.45724293864769550 ) ) ;
#106941=CARTESIAN_POINT ( 'NONE',  ( -12.14591786802326823, 12.06949235617739902, 93.12609039468568994 ) ) ;
#106942=CARTESIAN_POINT ( 'NONE',  ( 14.29746914071049879, -8.314922557960816363, 68.33224293864769550 ) ) ;
#106943=CARTESIAN_POINT ( 'NONE',  ( -16.46253265017160317, 9.564922557960807481, 60.83224293864769550 ) ) ;
#106944=CARTESIAN_POINT ( 'NONE',  ( 10.72451020669871369, 18.67979575497193778, 87.08442372801901854 ) ) ;
#106946=CARTESIAN_POINT ( 'NONE',  ( -5.153800228976607833, 19.02544592524334988, 102.7094237280189759 ) ) ;
#106947=CARTESIAN_POINT ( 'NONE',  ( -14.34966873604960291, -8.224510206698953496, 76.66557627198103830 ) ) ;
#106948=CARTESIAN_POINT ( 'NONE',  ( -18.62759615963255300, -10.81492255796106328, 29.16775706135234003 ) ) ;
#106949=CARTESIAN_POINT ( 'NONE',  ( -18.62759615963270932, 10.81492255796079327, 60.83224293864769550 ) ) ;
#106950=CARTESIAN_POINT ( 'NONE',  ( 0.05219959533936267826, -19.03943276465977164, 35.00109039468566863 ) ) ;
#106952=CARTESIAN_POINT ( 'NONE',  ( 19.05341960407611168, 5.049401038298154454, 78.95724293864769550 ) ) ;
#106953=CARTESIAN_POINT ( 'NONE',  ( -14.34966873604960291, -8.224510206698953496, 51.66557627198102409 ) ) ;
#106954=CARTESIAN_POINT ( 'NONE',  ( -0.05219959533910754901, -16.53943276465976808, 37.49890960531436690 ) ) ;
#106955=CARTESIAN_POINT ( 'NONE',  ( -12.06949235617739369, -12.14591786802326823, 99.37609039468568994 ) ) ;
#106956=CARTESIAN_POINT ( 'NONE',  ( -9.564922557961040184, 16.46253265017147172, 47.91775706135233293 ) ) ;
#106957=CARTESIAN_POINT ( 'NONE',  ( 9.564922557960805705, 16.46253265017160317, 99.58224293864770971 ) ) ;
#106958=CARTESIAN_POINT ( 'NONE',  ( -8.314922557960811034, -14.29746914071050412, 72.08224293864769550 ) ) ;
#106959=CARTESIAN_POINT ( 'NONE',  ( 13.97604488694548053, -13.89961937509957401, 45.62609039468566863 ) ) ;
#106960=CARTESIAN_POINT ( 'NONE',  ( 19.02544592524343514, -5.153800228976328945, 38.54057627198103120 ) ) ;
#106961=CARTESIAN_POINT ( 'NONE',  ( 15.72974639402199770, -15.80617190586745480, 38.12390960531436690 ) ) ;
#106962=CARTESIAN_POINT ( 'NONE',  ( 21.55341960407610458, 5.719274019375980345, 63.95724293864770260 ) ) ;
#106963=CARTESIAN_POINT ( 'NONE',  ( 0.05219959533910956823, 16.53943276465976808, 99.99890960531436690 ) ) ;
#106964=CARTESIAN_POINT ( 'NONE',  ( 14.29746914071037800, 8.314922557961029526, 56.66775706135235424 ) ) ;
#106965=CARTESIAN_POINT ( 'NONE',  ( 0.05219959533937995610, -21.53943276465977519, 45.00109039468568284 ) ) ;
#106966=CARTESIAN_POINT ( 'NONE',  ( 14.34966873604960469, 8.224510206698951720, 94.16557627198103830 ) ) ;
#106969=CARTESIAN_POINT ( 'NONE',  ( -16.38665767535054130, 7.295008042176025498, 50.26400864214546260 ) ) ;
#106970=CARTESIAN_POINT ( 'NONE',  ( -15.72974639402197994, 15.80617190586746368, 40.62390960531435269 ) ) ;
#106973=CARTESIAN_POINT ( 'NONE',  ( 4.483927247898790824, -16.52544592524335698, 40.20942372801901854 ) ) ;
#106974=CARTESIAN_POINT ( 'NONE',  ( -16.55341960407611168, -4.379528057220339221, 46.45724293864769550 ) ) ;
#106975=CARTESIAN_POINT ( 'NONE',  ( -21.52544592524343514, 5.823673210054127303, 66.04057627198103830 ) ) ;
#106976=CARTESIAN_POINT ( 'NONE',  ( 19.02544592524334988, 5.153800228976608722, 91.45942372801900433 ) ) ;
#106977=CARTESIAN_POINT ( 'NONE',  ( -5.823673210054116645, -21.52544592524344225, 62.29057627198102409 ) ) ;
#106979=CARTESIAN_POINT ( 'NONE',  ( -13.97604488694527625, -13.89961937509977652, 36.87390960531436690 ) ) ;
#106980=CARTESIAN_POINT ( 'NONE',  ( 19.02544592524343514, -5.153800228976328945, 98.54057627198100988 ) ) ;
#106981=CARTESIAN_POINT ( 'NONE',  ( 0.05219959533909260263, 19.03943276465977164, 34.99890960531435979 ) ) ;
#106982=CARTESIAN_POINT ( 'NONE',  ( 14.29746914071049879, -8.314922557960816363, 108.3322429386477097 ) ) ;
#106985=CARTESIAN_POINT ( 'NONE',  ( -5.153800228976328057, -19.02544592524343514, 112.2905762719810099 ) ) ;
#106987=CARTESIAN_POINT ( 'NONE',  ( -8.224510206698735004, -14.34966873604973081, 74.58442372801901854 ) ) ;
#106988=CARTESIAN_POINT ( 'NONE',  ( 18.62759615963271287, -10.81492255796078972, 88.33224293864769550 ) ) ;
#106989=CARTESIAN_POINT ( 'NONE',  ( 19.02544592524343514, -5.153800228976328945, 58.54057627198102409 ) ) ;
#106990=CARTESIAN_POINT ( 'NONE',  ( 10.72451020669871369, 18.67979575497193778, 32.08442372801901854 ) ) ;
#106991=CARTESIAN_POINT ( 'NONE',  ( 19.03943276465977164, -0.05219959533909143690, 78.74890960531436690 ) ) ;
#106993=ORIENTED_EDGE ( 'NONE', *, *, #169362, .T. ) ;
#106994=CARTESIAN_POINT ( 'NONE',  ( 15.72974639402199770, -15.80617190586745480, 113.1239096053143953 ) ) ;
#106995=CARTESIAN_POINT ( 'NONE',  ( 13.97604488694527802, 13.89961937509977652, 24.37390960531435624 ) ) ;
#106996=CARTESIAN_POINT ( 'NONE',  ( -19.02544592524342804, 5.153800228976336051, 106.0405762719810241 ) ) ;
#106997=CARTESIAN_POINT ( 'NONE',  ( 13.89961937509957401, 13.97604488694547697, 81.87609039468564731 ) ) ;
#106998=CARTESIAN_POINT ( 'NONE',  ( 0.05219959533936267826, -19.03943276465977164, 30.00109039468566863 ) ) ;
#106999=CARTESIAN_POINT ( 'NONE',  ( -21.53943276465977519, 0.05219959533907696930, 96.24890960531435269 ) ) ;
#107000=CARTESIAN_POINT ( 'NONE',  ( -0.05219959533936034679, 19.03943276465977164, 32.50109039468566863 ) ) ;
#107001=CARTESIAN_POINT ( 'NONE',  ( 16.46253265017146816, 9.564922557961045513, 36.66775706135233293 ) ) ;
#107002=CARTESIAN_POINT ( 'NONE',  ( 16.55341960407618274, -4.379528057220086978, 86.04275706135236135 ) ) ;
#107003=CARTESIAN_POINT ( 'NONE',  ( 19.03943276465977164, -0.05219959533909143690, 103.7489096053143669 ) ) ;
#107004=CARTESIAN_POINT ( 'NONE',  ( 19.03943276465977164, -0.05219959533909143690, 53.74890960531436690 ) ) ;
#107005=CARTESIAN_POINT ( 'NONE',  ( 21.53943276465977519, 0.05219959533937863772, 71.25109039468568994 ) ) ;
#107006=CARTESIAN_POINT ( 'NONE',  ( 0.05219959533937995610, -21.53943276465977519, 80.00109039468568994 ) ) ;
#107007=CARTESIAN_POINT ( 'NONE',  ( 13.97604488694527802, 13.89961937509977652, 114.3739096053143669 ) ) ;
#107008=CARTESIAN_POINT ( 'NONE',  ( -13.89961937509977652, 13.97604488694528158, 75.62390960531438111 ) ) ;
#107009=CARTESIAN_POINT ( 'NONE',  ( 10.81492255796106328, -18.62759615963255655, 50.41775706135235424 ) ) ;
#107010=CARTESIAN_POINT ( 'NONE',  ( 5.049401038297881783, 19.05341960407617563, 97.29275706135233293 ) ) ;
#107011=CARTESIAN_POINT ( 'NONE',  ( 13.89961937509977652, -13.97604488694527269, 48.12390960531435979 ) ) ;
#107012=CARTESIAN_POINT ( 'NONE',  ( 13.97604488694527802, 13.89961937509977652, 94.37390960531436690 ) ) ;
#107013=CARTESIAN_POINT ( 'NONE',  ( -19.02544592524342804, 5.153800228976336051, 86.04057627198103830 ) ) ;
#107015=CARTESIAN_POINT ( 'NONE',  ( 13.97604488694527802, 13.89961937509977652, 54.37390960531435979 ) ) ;
#107017=CARTESIAN_POINT ( 'NONE',  ( 21.52544592524344225, -5.823673210054117533, 93.54057627198103830 ) ) ;
#107018=CARTESIAN_POINT ( 'NONE',  ( -4.483927247898782831, 16.52544592524335698, 82.70942372801900433 ) ) ;
#107020=CARTESIAN_POINT ( 'NONE',  ( -0.05219959533936034679, 19.03943276465977164, 47.50109039468566863 ) ) ;
#107021=CARTESIAN_POINT ( 'NONE',  ( -9.564922557960796823, -16.46253265017161027, 82.08224293864768129 ) ) ;
#107022=CARTESIAN_POINT ( 'NONE',  ( -14.29746914071049879, 8.314922557960819915, 55.83224293864770260 ) ) ;
#107023=CARTESIAN_POINT ( 'NONE',  ( 4.379528057220339221, -16.55341960407611168, 97.70724293864772392 ) ) ;
#107024=CARTESIAN_POINT ( 'NONE',  ( -10.72451020669898014, 18.67979575497178502, 25.41557627198103120 ) ) ;
#107025=CARTESIAN_POINT ( 'NONE',  ( -5.153800228976328057, -19.02544592524343514, 107.2905762719810383 ) ) ;
#107026=CARTESIAN_POINT ( 'NONE',  ( 9.564922557960805705, 16.46253265017160317, 114.5822429386476955 ) ) ;
#107027=CARTESIAN_POINT ( 'NONE',  ( -16.51473224551082808, 9.474510206698731452, 28.33442372801900433 ) ) ;
#107028=CARTESIAN_POINT ( 'NONE',  ( -16.52544592524335698, -4.483927247898792601, 93.95942372801903275 ) ) ;
#107029=CARTESIAN_POINT ( 'NONE',  ( -19.05341960407611168, -5.049401038298163336, 76.45724293864769550 ) ) ;
#107030=CARTESIAN_POINT ( 'NONE',  ( -15.72974639402176322, -15.80617190586768395, 34.37609039468568284 ) ) ;
#107031=CARTESIAN_POINT ( 'NONE',  ( -5.823673210054116645, -21.52544592524344225, 32.29057627198102409 ) ) ;
#107032=CARTESIAN_POINT ( 'NONE',  ( 15.80617190586769283, -15.72974639402175789, 20.62609039468568639 ) ) ;
#107033=CARTESIAN_POINT ( 'NONE',  ( -21.53943276465977519, 0.05219959533907696930, 66.24890960531436690 ) ) ;
#107034=CARTESIAN_POINT ( 'NONE',  ( 14.34966873604960469, 8.224510206698951720, 94.16557627198103830 ) ) ;
#107035=CARTESIAN_POINT ( 'NONE',  ( -19.03943276465977164, -0.05219959533935918106, 43.75109039468566863 ) ) ;
#107036=CARTESIAN_POINT ( 'NONE',  ( -5.049401038298153566, 19.05341960407611168, 30.20724293864768839 ) ) ;
#107037=CARTESIAN_POINT ( 'NONE',  ( -5.153800228976328057, -19.02544592524343514, 87.29057627198103830 ) ) ;
#107038=CARTESIAN_POINT ( 'NONE',  ( 9.564922557960805705, 16.46253265017160317, 84.58224293864769550 ) ) ;
#107040=CARTESIAN_POINT ( 'NONE',  ( 16.52544592524342804, -4.483927247898539470, 103.5405762719810383 ) ) ;
#107042=CARTESIAN_POINT ( 'NONE',  ( -12.06949235617756955, 12.14591786802309770, 30.62390960531436335 ) ) ;
#107043=CARTESIAN_POINT ( 'NONE',  ( -14.34966873604972548, 8.224510206698743886, 33.33442372801900433 ) ) ;
#107044=CARTESIAN_POINT ( 'NONE',  ( -10.81492255796105439, 18.62759615963255655, 87.91775706135234714 ) ) ;
#107045=CARTESIAN_POINT ( 'NONE',  ( 9.474510206698971260, -16.51473224551069308, 97.91557627198102409 ) ) ;
#107046=CARTESIAN_POINT ( 'NONE',  ( -21.55341960407610458, -5.719274019375992779, 111.4572429386476813 ) ) ;
#107047=CARTESIAN_POINT ( 'NONE',  ( -0.05219959533909027116, -19.03943276465977164, 42.49890960531435269 ) ) ;
#107048=CARTESIAN_POINT ( 'NONE',  ( 8.224510206698742110, 14.34966873604972548, 47.08442372801901854 ) ) ;
#107049=CARTESIAN_POINT ( 'NONE',  ( -16.46253265017146816, -9.564922557961047289, 109.1677570613523471 ) ) ;
#107050=CARTESIAN_POINT ( 'NONE',  ( 0.05219959533910956823, 16.53943276465976808, 94.99890960531436690 ) ) ;
#107051=CARTESIAN_POINT ( 'NONE',  ( 5.719274019375991003, -21.55341960407610458, 102.7072429386476955 ) ) ;
#107052=CARTESIAN_POINT ( 'NONE',  ( -16.46253265017146816, -9.564922557961047289, 69.16775706135233293 ) ) ;
#107054=CARTESIAN_POINT ( 'NONE',  ( -18.62759615963270932, 10.81492255796079327, 115.8322429386477097 ) ) ;
#107056=CARTESIAN_POINT ( 'NONE',  ( 0.05219959533909260263, 19.03943276465977164, 89.99890960531436690 ) ) ;
#107058=CARTESIAN_POINT ( 'NONE',  ( -9.474510206698964154, 16.51473224551069663, 90.41557627198103830 ) ) ;
#107059=CARTESIAN_POINT ( 'NONE',  ( -21.53943276465977519, -0.05219959533937600094, 38.75109039468567573 ) ) ;
#107060=CARTESIAN_POINT ( 'NONE',  ( -14.29746914071049879, 8.314922557960819915, 75.83224293864769550 ) ) ;
#107061=CARTESIAN_POINT ( 'NONE',  ( -9.564922557960796823, -16.46253265017161027, 87.08224293864769550 ) ) ;
#107062=CARTESIAN_POINT ( 'NONE',  ( -12.14591786802326823, 12.06949235617739902, 48.12609039468568284 ) ) ;
#107063=CARTESIAN_POINT ( 'NONE',  ( 16.51473224551083163, -9.474510206698727899, 55.83442372801899722 ) ) ;
#107064=CARTESIAN_POINT ( 'NONE',  ( -18.62759615963255300, -10.81492255796106328, 59.16775706135234714 ) ) ;
#107065=CARTESIAN_POINT ( 'NONE',  ( 8.314922557961029526, -14.29746914071037800, 25.41775706135235779 ) ) ;
#107066=CARTESIAN_POINT ( 'NONE',  ( 0.05219959533909260263, 19.03943276465977164, 69.99890960531435269 ) ) ;
#107067=CARTESIAN_POINT ( 'NONE',  ( -13.89961937509957401, -13.97604488694547875, 94.37609039468566152 ) ) ;
#107068=CARTESIAN_POINT ( 'NONE',  ( -4.483927247898782831, 16.52544592524335698, 52.70942372801902565 ) ) ;
#107069=CARTESIAN_POINT ( 'NONE',  ( -5.823673210054431948, 21.52544592524334988, 102.7094237280190185 ) ) ;
#107070=CARTESIAN_POINT ( 'NONE',  ( -19.02544592524334988, -5.153800228976617603, 78.95942372801900433 ) ) ;
#107071=CARTESIAN_POINT ( 'NONE',  ( -16.51473224551069308, -9.474510206698971260, 46.66557627198102409 ) ) ;
#107072=CARTESIAN_POINT ( 'NONE',  ( -15.80617190586745835, -15.72974639402198527, 76.87390960531439532 ) ) ;
#107073=CARTESIAN_POINT ( 'NONE',  ( 14.34966873604960469, 8.224510206698951720, 79.16557627198103830 ) ) ;
#107074=CARTESIAN_POINT ( 'NONE',  ( 19.02544592524334988, 5.153800228976608722, 81.45942372801897591 ) ) ;
#107075=CARTESIAN_POINT ( 'NONE',  ( -19.53091890409952924, -5.499999999999944933, 70.06097431831416600 ) ) ;
#107076=CARTESIAN_POINT ( 'NONE',  ( 16.51473224551083163, -9.474510206698727899, 45.83442372801900433 ) ) ;
#107077=CARTESIAN_POINT ( 'NONE',  ( 16.55341960407618274, -4.379528057220086978, 111.0427570613523613 ) ) ;
#107078=CARTESIAN_POINT ( 'NONE',  ( -0.05219959533910754901, -16.53943276465976808, 67.49890960531436690 ) ) ;
#107079=CARTESIAN_POINT ( 'NONE',  ( 10.81492255796106328, -18.62759615963255655, 105.4177570613523613 ) ) ;
#107081=CARTESIAN_POINT ( 'NONE',  ( -21.55341960407610458, -5.719274019375992779, 106.4572429386477097 ) ) ;
#107082=CARTESIAN_POINT ( 'NONE',  ( 9.474510206698971260, -16.51473224551069308, 67.91557627198102409 ) ) ;
#107083=CARTESIAN_POINT ( 'NONE',  ( -15.72974639402176322, -15.80617190586768395, 89.37609039468568994 ) ) ;
#107084=CARTESIAN_POINT ( 'NONE',  ( 16.51473224551069308, 9.474510206698969483, 64.16557627198102409 ) ) ;
#107085=VERTEX_POINT ( 'NONE', #59697 ) ;
#107086=CARTESIAN_POINT ( 'NONE',  ( 16.51473224551069308, 9.474510206698969483, 29.16557627198103475 ) ) ;
#107087=CARTESIAN_POINT ( 'NONE',  ( -15.72974639402197994, 15.80617190586746368, 30.62390960531436335 ) ) ;
#107088=CARTESIAN_POINT ( 'NONE',  ( -4.483927247898539470, -16.52544592524342804, 72.29057627198102409 ) ) ;
#107089=CARTESIAN_POINT ( 'NONE',  ( 5.049401038298161559, -19.05341960407611168, 47.70724293864770260 ) ) ;
#107090=CARTESIAN_POINT ( 'NONE',  ( -16.55341960407611168, -4.379528057220339221, 81.45724293864769550 ) ) ;
#107091=CARTESIAN_POINT ( 'NONE',  ( -21.52544592524343514, 5.823673210054127303, 111.0405762719810525 ) ) ;
#107093=CARTESIAN_POINT ( 'NONE',  ( -5.823673210054431948, 21.52544592524334988, 52.70942372801902565 ) ) ;
#107094=CARTESIAN_POINT ( 'NONE',  ( -19.05341960407611168, -5.049401038298163336, 36.45724293864766707 ) ) ;
#107095=CARTESIAN_POINT ( 'NONE',  ( -8.314922557961024197, 14.29746914071037800, 47.91775706135234714 ) ) ;
#107096=CARTESIAN_POINT ( 'NONE',  ( 5.823673210054125526, 21.52544592524343514, 99.79057627198103830 ) ) ;
#107097=CARTESIAN_POINT ( 'NONE',  ( -5.049401038297874678, -19.05341960407617918, 24.79275706135233648 ) ) ;
#107098=CARTESIAN_POINT ( 'NONE',  ( 0.05219959533909260263, 19.03943276465977164, 54.99890960531435979 ) ) ;
#107099=CARTESIAN_POINT ( 'NONE',  ( 13.89961937509977652, -13.97604488694527269, 108.1239096053143669 ) ) ;
#107100=CARTESIAN_POINT ( 'NONE',  ( -21.55341960407619339, 5.719274019375674811, 53.54275706135234714 ) ) ;
#107101=B_SPLINE_CURVE_WITH_KNOTS ( 'NONE', 3,
 ( #96005, #155693, #62675, #187060, #107191, #123350, #169872, #142506, #18192, #47535, #30367, #79849, #184054, #17188, #156698, #7, #48530, #141518, #3005, #109189, #46530, #153704, #92011, #49510, #124356, #64681, #63689, #15200, #125364, #111173, #170868, #76858 ),
 .UNSPECIFIED., .F., .F.,
 ( 4, 2, 2, 2, 2, 2, 2, 2, 2, 2, 2, 2, 2, 2, 2, 4 ),
 ( 2.195984522899319407E-17, 0.0003712461730036906811, 0.0007424923460073594612, 0.001113738519011028133, 0.001484984692014696805, 0.002227477038022034582, 0.002598723211025703254, 0.002969969384029371925, 0.003341215557033051006, 0.003712461730036730519, 0.004083707903040409599, 0.004454954076044089113, 0.004826200249047772096, 0.005197446422051455080, 0.005568692595055138063, 0.005939938768058821913 ),
 .UNSPECIFIED. ) ;
#107102=CARTESIAN_POINT ( 'NONE',  ( -18.67979575497178146, -10.72451020669898902, 46.66557627198102409 ) ) ;
#107103=CARTESIAN_POINT ( 'NONE',  ( -12.06949235617756955, 12.14591786802309770, 25.62390960531435624 ) ) ;
#107104=CARTESIAN_POINT ( 'NONE',  ( 5.719274019375673035, 21.55341960407619339, 57.29275706135234714 ) ) ;
#107105=CARTESIAN_POINT ( 'NONE',  ( -18.67979575497193778, 10.72451020669871902, 93.33442372801901854 ) ) ;
#107106=CARTESIAN_POINT ( 'NONE',  ( -9.474510206698720793, -16.51473224551083518, 29.58442372801900433 ) ) ;
#107107=CARTESIAN_POINT ( 'NONE',  ( -16.55341960407617563, 4.379528057220093196, 103.5427570613523613 ) ) ;
#107108=CARTESIAN_POINT ( 'NONE',  ( -5.823673210054431948, 21.52544592524334988, 57.70942372801901143 ) ) ;
#107109=CARTESIAN_POINT ( 'NONE',  ( -19.03943276465977164, 0.05219959533909376836, 51.24890960531436690 ) ) ;
#107110=CARTESIAN_POINT ( 'NONE',  ( -9.474510206698720793, -16.51473224551083518, 24.58442372801900078 ) ) ;
#107111=CARTESIAN_POINT ( 'NONE',  ( 9.564922557960805705, 16.46253265017160317, 114.5822429386476955 ) ) ;
#107112=CARTESIAN_POINT ( 'NONE',  ( -18.62759615963255300, -10.81492255796106328, 19.16775706135234714 ) ) ;
#107113=CARTESIAN_POINT ( 'NONE',  ( -21.55341960407610458, -5.719274019375992779, 81.45724293864769550 ) ) ;
#107114=CARTESIAN_POINT ( 'NONE',  ( -14.34966873604972548, 8.224510206698743886, 43.33442372801901143 ) ) ;
#107116=CARTESIAN_POINT ( 'NONE',  ( 21.52544592524344225, -5.823673210054117533, 83.54057627198102409 ) ) ;
#107117=CARTESIAN_POINT ( 'NONE',  ( 0.05219959533934541429, -16.53943276465976808, 60.00109039468568284 ) ) ;
#107118=CARTESIAN_POINT ( 'NONE',  ( -14.29746914071049879, 8.314922557960819915, 70.83224293864770971 ) ) ;
#107120=CARTESIAN_POINT ( 'NONE',  ( 5.049401038297881783, 19.05341960407617563, 102.2927570613523045 ) ) ;
#107121=CARTESIAN_POINT ( 'NONE',  ( 18.67979575497178502, 10.72451020669898547, 29.16557627198103120 ) ) ;
#107123=CARTESIAN_POINT ( 'NONE',  ( -4.379528057220086978, -16.55341960407618274, 44.79275706135234714 ) ) ;
#107124=CARTESIAN_POINT ( 'NONE',  ( 10.72451020669898902, -18.67979575497178502, 107.9155762719810241 ) ) ;
#107125=CARTESIAN_POINT ( 'NONE',  ( 10.72451020669898902, -18.67979575497178502, 27.91557627198103830 ) ) ;
#107126=CARTESIAN_POINT ( 'NONE',  ( 4.483927247898790824, -16.52544592524335698, 75.20942372801901854 ) ) ;
#107127=CARTESIAN_POINT ( 'NONE',  ( -13.89961937509977652, 13.97604488694528158, 85.62390960531433848 ) ) ;
#107128=CARTESIAN_POINT ( 'NONE',  ( -18.62759615963255300, -10.81492255796106328, 39.16775706135235424 ) ) ;
#107129=CARTESIAN_POINT ( 'NONE',  ( 4.483927247898790824, -16.52544592524335698, 20.20942372801900788 ) ) ;
#107130=EDGE_CURVE ( 'NONE', #16989, #63341, #104227, .T. ) ;
#107131=CARTESIAN_POINT ( 'NONE',  ( -15.80617190586745835, -15.72974639402198527, 31.87390960531435979 ) ) ;
#107133=CARTESIAN_POINT ( 'NONE',  ( -9.474510206698720793, -16.51473224551083518, 29.58442372801900433 ) ) ;
#107134=CARTESIAN_POINT ( 'NONE',  ( -16.52544592524335698, -4.483927247898792601, 48.95942372801902565 ) ) ;
#107135=CARTESIAN_POINT ( 'NONE',  ( -19.05341960407611168, -5.049401038298163336, 96.45724293864769550 ) ) ;
#107136=CARTESIAN_POINT ( 'NONE',  ( -5.719274019375978568, 21.55341960407610458, 100.2072429386476955 ) ) ;
#107137=CARTESIAN_POINT ( 'NONE',  ( -19.03943276465977164, 0.05219959533909376836, 71.24890960531435269 ) ) ;
#107138=CARTESIAN_POINT ( 'NONE',  ( -17.31728774477272736, 6.344390552232388458, 25.81906651689319432 ) ) ;
#107139=CARTESIAN_POINT ( 'NONE',  ( -4.379528057220328563, 16.55341960407611168, 85.20724293864770971 ) ) ;
#107140=CARTESIAN_POINT ( 'NONE',  ( -18.62759615963270932, 10.81492255796079327, 35.83224293864768839 ) ) ;
#107141=CARTESIAN_POINT ( 'NONE',  ( -17.26172910966779739, 6.454744622555853795, 35.80646908649224969 ) ) ;
#107142=CARTESIAN_POINT ( 'NONE',  ( -16.53943276465976808, -0.05219959533934237506, 63.75109039468568284 ) ) ;
#107143=CARTESIAN_POINT ( 'NONE',  ( -5.823673210054116645, -21.52544592524344225, 112.2905762719810241 ) ) ;
#107144=CARTESIAN_POINT ( 'NONE',  ( 9.474510206698729675, 16.51473224551082808, 82.08442372801899012 ) ) ;
#107145=CARTESIAN_POINT ( 'NONE',  ( 13.89961937509977652, -13.97604488694527269, 28.12390960531435624 ) ) ;
#107146=CARTESIAN_POINT ( 'NONE',  ( -0.05219959533907301413, -21.53943276465977519, 62.49890960531436690 ) ) ;
#107147=CARTESIAN_POINT ( 'NONE',  ( -16.51473224551069308, -9.474510206698971260, 96.66557627198102409 ) ) ;
#107148=CARTESIAN_POINT ( 'NONE',  ( -0.05219959533937732626, 21.53943276465977519, 87.50109039468568994 ) ) ;
#107149=CARTESIAN_POINT ( 'NONE',  ( 9.474510206698971260, -16.51473224551069308, 67.91557627198102409 ) ) ;
#107150=CARTESIAN_POINT ( 'NONE',  ( 0.05219959533934541429, -16.53943276465976808, 45.00109039468568284 ) ) ;
#107151=CARTESIAN_POINT ( 'NONE',  ( -19.03943276465977164, 0.05219959533909376836, 61.24890960531436690 ) ) ;
#107152=CARTESIAN_POINT ( 'NONE',  ( 5.823673210054444382, -21.52544592524334988, 85.20942372801901854 ) ) ;
#107154=CARTESIAN_POINT ( 'NONE',  ( -16.51473224551082808, 9.474510206698731452, 38.33442372801899722 ) ) ;
#107155=CARTESIAN_POINT ( 'NONE',  ( 5.049401038297881783, 19.05341960407617563, 52.29275706135234003 ) ) ;
#107156=CARTESIAN_POINT ( 'NONE',  ( -18.62759615963255300, -10.81492255796106328, 49.16775706135234003 ) ) ;
#107158=CARTESIAN_POINT ( 'NONE',  ( 9.564922557961047289, -16.46253265017146816, 40.41775706135234003 ) ) ;
#107159=CARTESIAN_POINT ( 'NONE',  ( -5.153800228976328057, -19.02544592524343514, 97.29057627198099567 ) ) ;
#107160=CARTESIAN_POINT ( 'NONE',  ( -9.474510206698964154, 16.51473224551069663, 70.41557627198102409 ) ) ;
#107161=CARTESIAN_POINT ( 'NONE',  ( 8.224510206698742110, 14.34966873604972548, 112.0844237280190185 ) ) ;
#107162=CARTESIAN_POINT ( 'NONE',  ( 15.80617190586746368, 15.72974639402197994, 34.37390960531435979 ) ) ;
#107163=CARTESIAN_POINT ( 'NONE',  ( 15.80617190586769283, -15.72974639402175789, 100.6260903946857184 ) ) ;
#107165=CARTESIAN_POINT ( 'NONE',  ( 16.79531203550650886, 7.028104445595491079, 58.75244988220443787 ) ) ;
#107166=CARTESIAN_POINT ( 'NONE',  ( 21.52544592524334988, 5.823673210054432836, 101.4594237280190185 ) ) ;
#107167=CARTESIAN_POINT ( 'NONE',  ( 16.18388926212234935, -7.379444403734657598, 42.06046848633847191 ) ) ;
#107168=CARTESIAN_POINT ( 'NONE',  ( -13.97604488694527625, -13.89961937509977652, 21.87390960531435979 ) ) ;
#107169=CARTESIAN_POINT ( 'NONE',  ( -9.564922557960796823, -16.46253265017161027, 107.0822429386476955 ) ) ;
#107170=LINE ( 'NONE', #152685, #27575 ) ;
#107171=CARTESIAN_POINT ( 'NONE',  ( 14.34966873604972726, -8.224510206698740333, 55.83442372801901854 ) ) ;
#107172=CARTESIAN_POINT ( 'NONE',  ( -10.72451020669898014, 18.67979575497178502, 65.41557627198102409 ) ) ;
#107173=CARTESIAN_POINT ( 'NONE',  ( -14.29746914071049879, 8.314922557960819915, 45.83224293864769550 ) ) ;
#107174=CARTESIAN_POINT ( 'NONE',  ( -14.29746914071049879, 8.314922557960819915, 105.8322429386476955 ) ) ;
#107175=CARTESIAN_POINT ( 'NONE',  ( -19.02544592524342804, 5.153800228976336051, 101.0405762719810241 ) ) ;
#107176=CARTESIAN_POINT ( 'NONE',  ( -16.46253265017146816, -9.564922557961047289, 34.16775706135233293 ) ) ;
#107177=CARTESIAN_POINT ( 'NONE',  ( -19.05341960407611168, -5.049401038298163336, 21.45724293864768839 ) ) ;
#107178=CARTESIAN_POINT ( 'NONE',  ( -21.53943276465977519, -0.05219959533937600094, 73.75109039468567573 ) ) ;
#107180=CARTESIAN_POINT ( 'NONE',  ( -4.483927247898782831, 16.52544592524335698, 107.7094237280190328 ) ) ;
#107182=CARTESIAN_POINT ( 'NONE',  ( 18.62759615963271287, -10.81492255796078972, 23.33224293864769194 ) ) ;
#107183=CARTESIAN_POINT ( 'NONE',  ( 16.53943276465976808, -0.05219959533910856209, 88.74890960531436690 ) ) ;
#107184=CARTESIAN_POINT ( 'NONE',  ( -16.51473224551082808, 9.474510206698731452, 63.33442372801900433 ) ) ;
#107185=CARTESIAN_POINT ( 'NONE',  ( -16.51473224551069308, -9.474510206698971260, 71.66557627198102409 ) ) ;
#107186=CARTESIAN_POINT ( 'NONE',  ( 16.52544592524342804, -4.483927247898539470, 78.54057627198103830 ) ) ;
#107187=CARTESIAN_POINT ( 'NONE',  ( -19.03943276465977164, -0.05219959533935918106, 98.75109039468567573 ) ) ;
#107188=CARTESIAN_POINT ( 'NONE',  ( 18.67979575497178502, 10.72451020669898547, 54.16557627198103120 ) ) ;
#107189=ORIENTED_EDGE ( 'NONE', *, *, #190681, .F. ) ;
#107190=CARTESIAN_POINT ( 'NONE',  ( 19.02544592524343514, -5.153800228976328945, 23.54057627198102054 ) ) ;
#107191=CARTESIAN_POINT ( 'NONE',  ( -17.40805194822029378, -6.112264579159358391, 29.16628727489389661 ) ) ;
#107192=CARTESIAN_POINT ( 'NONE',  ( 13.89961937509977652, -13.97604488694527269, 78.12390960531433848 ) ) ;
#107193=CARTESIAN_POINT ( 'NONE',  ( -18.62759615963270932, 10.81492255796079327, 75.83224293864769550 ) ) ;
#107194=CARTESIAN_POINT ( 'NONE',  ( 12.14591786802327356, -12.06949235617739191, 85.62609039468568994 ) ) ;
#107195=CARTESIAN_POINT ( 'NONE',  ( -9.474510206698964154, 16.51473224551069663, 85.41557627198102409 ) ) ;
#107196=CARTESIAN_POINT ( 'NONE',  ( 16.46253265017146816, 9.564922557961045513, 66.66775706135233293 ) ) ;
#107197=CARTESIAN_POINT ( 'NONE',  ( -15.72974639402176322, -15.80617190586768395, 79.37609039468567573 ) ) ;
#107199=CARTESIAN_POINT ( 'NONE',  ( 10.81492255796078972, 18.62759615963270932, 59.58224293864770260 ) ) ;
#107200=CARTESIAN_POINT ( 'NONE',  ( -21.53943276465977519, 0.05219959533907696930, 21.24890960531436690 ) ) ;
#107201=CARTESIAN_POINT ( 'NONE',  ( 9.564922557960805705, 16.46253265017160317, 39.58224293864768839 ) ) ;
#107202=CARTESIAN_POINT ( 'NONE',  ( 4.483927247898790824, -16.52544592524335698, 105.2094237280190328 ) ) ;
#107203=CARTESIAN_POINT ( 'NONE',  ( 19.02544592524343514, -5.153800228976328945, 48.54057627198103120 ) ) ;
#107204=CARTESIAN_POINT ( 'NONE',  ( 13.89961937509957401, 13.97604488694547697, 111.8760903946856757 ) ) ;
#107205=CARTESIAN_POINT ( 'NONE',  ( 17.44279575226822487, 5.990770900252483600, 51.66442432485681735 ) ) ;
#107206=CARTESIAN_POINT ( 'NONE',  ( -0.05219959533937732626, 21.53943276465977519, 107.5010903946856899 ) ) ;
#107207=CARTESIAN_POINT ( 'NONE',  ( -4.379528057220328563, 16.55341960407611168, 60.20724293864768839 ) ) ;
#107208=CARTESIAN_POINT ( 'NONE',  ( 21.55341960407610458, 5.719274019375980345, 103.9572429386476813 ) ) ;
#107209=CARTESIAN_POINT ( 'NONE',  ( -21.52544592524343514, 5.823673210054127303, 106.0405762719810525 ) ) ;
#107211=CARTESIAN_POINT ( 'NONE',  ( -10.81492255796078084, -18.62759615963271287, 47.08224293864770260 ) ) ;
#107212=CARTESIAN_POINT ( 'NONE',  ( -8.224510206698735004, -14.34966873604973081, 79.58442372801903275 ) ) ;
#107213=CARTESIAN_POINT ( 'NONE',  ( -16.55341960407611168, -4.379528057220339221, 106.4572429386477097 ) ) ;
#107214=CARTESIAN_POINT ( 'NONE',  ( 13.97604488694527802, 13.89961937509977652, 54.37390960531435979 ) ) ;
#107215=CARTESIAN_POINT ( 'NONE',  ( -19.02130022317638947, 5.499999999999605649, 50.78188669246576126 ) ) ;
#107216=CARTESIAN_POINT ( 'NONE',  ( 8.314922557961029526, -14.29746914071037800, 110.4177570613523756 ) ) ;
#107217=CARTESIAN_POINT ( 'NONE',  ( 15.72974639402176855, 15.80617190586768217, 51.87609039468568284 ) ) ;
#107218=CARTESIAN_POINT ( 'NONE',  ( 9.474510206698971260, -16.51473224551069308, 102.9155762719810241 ) ) ;
#107219=CARTESIAN_POINT ( 'NONE',  ( -21.52544592524334988, -5.823673210054445271, 83.95942372801900433 ) ) ;
#107223=CARTESIAN_POINT ( 'NONE',  ( -21.52544592524334988, -5.823673210054445271, 73.95942372801901854 ) ) ;
#107224=CARTESIAN_POINT ( 'NONE',  ( -13.97604488694527625, -13.89961937509977652, 46.87390960531435979 ) ) ;
#107225=CARTESIAN_POINT ( 'NONE',  ( 9.564922557960805705, 16.46253265017160317, 99.58224293864770971 ) ) ;
#107226=CARTESIAN_POINT ( 'NONE',  ( -9.474510206698720793, -16.51473224551083518, 79.58442372801899012 ) ) ;
#107227=CARTESIAN_POINT ( 'NONE',  ( 18.62759615963255655, 10.81492255796105972, 36.66775706135234714 ) ) ;
#107228=CARTESIAN_POINT ( 'NONE',  ( 9.474510206698729675, 16.51473224551082808, 107.0844237280190043 ) ) ;
#107229=CARTESIAN_POINT ( 'NONE',  ( 5.153800228976615827, -19.02544592524334988, 75.20942372801896170 ) ) ;
#107230=CARTESIAN_POINT ( 'NONE',  ( 5.049401038298161559, -19.05341960407611168, 42.70724293864767418 ) ) ;
#107231=CARTESIAN_POINT ( 'NONE',  ( 9.564922557961047289, -16.46253265017146816, 85.41775706135233293 ) ) ;
#107232=CARTESIAN_POINT ( 'NONE',  ( 12.14591786802327356, -12.06949235617739191, 105.6260903946856899 ) ) ;
#107233=CARTESIAN_POINT ( 'NONE',  ( -13.97604488694547697, 13.89961937509957934, 73.12609039468568994 ) ) ;
#107234=CARTESIAN_POINT ( 'NONE',  ( -14.34966873604960291, -8.224510206698953496, 41.66557627198103120 ) ) ;
#107235=CARTESIAN_POINT ( 'NONE',  ( 16.51473224551083163, -9.474510206698727899, 60.83442372801900433 ) ) ;
#107236=CARTESIAN_POINT ( 'NONE',  ( -21.53943276465977519, -0.05219959533937600094, 103.7510903946857042 ) ) ;
#107237=CARTESIAN_POINT ( 'NONE',  ( 16.46253265017146816, 9.564922557961045513, 26.66775706135234003 ) ) ;
#107238=CARTESIAN_POINT ( 'NONE',  ( -19.05341960407611168, -5.049401038298163336, 26.45724293864769550 ) ) ;
#107240=CARTESIAN_POINT ( 'NONE',  ( -4.483927247898782831, 16.52544592524335698, 42.70942372801901854 ) ) ;
#107242=CARTESIAN_POINT ( 'NONE',  ( -5.049401038298153566, 19.05341960407611168, 95.20724293864770971 ) ) ;
#107244=CARTESIAN_POINT ( 'NONE',  ( -13.97604488694527625, -13.89961937509977652, 91.87390960531432427 ) ) ;
#107245=CARTESIAN_POINT ( 'NONE',  ( -17.40805194821983193, 6.112264579160852307, 100.8337127251061247 ) ) ;
#107247=CARTESIAN_POINT ( 'NONE',  ( -9.564922557961040184, 16.46253265017147172, 82.91775706135233293 ) ) ;
#107248=CARTESIAN_POINT ( 'NONE',  ( -21.53943276465977519, 0.05219959533907696930, 26.24890960531435624 ) ) ;
#107249=CARTESIAN_POINT ( 'NONE',  ( -19.02544592524334988, -5.153800228976617603, 18.95942372801899722 ) ) ;
#107250=CARTESIAN_POINT ( 'NONE',  ( -19.03943276465977164, -0.05219959533935918106, 103.7510903946856757 ) ) ;
#107251=CARTESIAN_POINT ( 'NONE',  ( -0.05219959533910754901, -16.53943276465976808, 112.4989096053143669 ) ) ;
#107252=CARTESIAN_POINT ( 'NONE',  ( -13.89961937509977652, 13.97604488694528158, 25.62390960531434558 ) ) ;
#107253=CARTESIAN_POINT ( 'NONE',  ( -18.67979575497178146, -10.72451020669898902, 61.66557627198103120 ) ) ;
#107254=CARTESIAN_POINT ( 'NONE',  ( 18.67979575497178502, 10.72451020669898547, 44.16557627198103120 ) ) ;
#107255=CARTESIAN_POINT ( 'NONE',  ( 9.564922557960805705, 16.46253265017160317, 24.58224293864769194 ) ) ;
#107257=CARTESIAN_POINT ( 'NONE',  ( 13.89961937509957401, 13.97604488694547697, 71.87609039468567573 ) ) ;
#107258=CARTESIAN_POINT ( 'NONE',  ( -12.06949235617756955, 12.14591786802309770, 40.62390960531435269 ) ) ;
#107259=CARTESIAN_POINT ( 'NONE',  ( -21.52544592524343514, 5.823673210054127303, 26.04057627198103475 ) ) ;
#107260=CARTESIAN_POINT ( 'NONE',  ( 21.55341960407619695, -5.719274019375665929, 96.04275706135236135 ) ) ;
#107261=CARTESIAN_POINT ( 'NONE',  ( -15.72974639402197994, 15.80617190586746368, 65.62390960531436690 ) ) ;
#107262=CARTESIAN_POINT ( 'NONE',  ( -0.05219959533937732626, 21.53943276465977519, 62.50109039468568284 ) ) ;
#107263=CARTESIAN_POINT ( 'NONE',  ( 15.72974639402176855, 15.80617190586768217, 46.87609039468568994 ) ) ;
#107264=CARTESIAN_POINT ( 'NONE',  ( -16.51473224551069308, -9.474510206698971260, 91.66557627198103830 ) ) ;
#107265=CARTESIAN_POINT ( 'NONE',  ( 8.224510206698742110, 14.34966873604972548, 92.08442372801901854 ) ) ;
#107266=CARTESIAN_POINT ( 'NONE',  ( 9.474510206698971260, -16.51473224551069308, 22.91557627198102765 ) ) ;
#107268=CARTESIAN_POINT ( 'NONE',  ( -4.483927247898539470, -16.52544592524342804, 67.29057627198103830 ) ) ;
#107269=CARTESIAN_POINT ( 'NONE',  ( 8.314922557960818139, 14.29746914071049879, 39.58224293864769550 ) ) ;
#107270=CARTESIAN_POINT ( 'NONE',  ( 19.03943276465977164, -0.05219959533909143690, 68.74890960531436690 ) ) ;
#107271=CARTESIAN_POINT ( 'NONE',  ( 13.89961937509977652, -13.97604488694527269, 28.12390960531435624 ) ) ;
#107272=CARTESIAN_POINT ( 'NONE',  ( -18.67979575497178146, -10.72451020669898902, 56.66557627198103830 ) ) ;
#107273=CARTESIAN_POINT ( 'NONE',  ( -0.05219959533936034679, 19.03943276465977164, 37.50109039468567573 ) ) ;
#107275=CARTESIAN_POINT ( 'NONE',  ( 12.06949235617757843, -12.14591786802309237, 53.12390960531436690 ) ) ;
#107276=CARTESIAN_POINT ( 'NONE',  ( 10.81492255796078972, 18.62759615963270932, 29.58224293864769905 ) ) ;
#107279=CARTESIAN_POINT ( 'NONE',  ( -16.53943276465976808, -0.05219959533934237506, 73.75109039468567573 ) ) ;
#107280=CARTESIAN_POINT ( 'NONE',  ( 13.89961937509957401, 13.97604488694547697, 71.87609039468567573 ) ) ;
#107281=CARTESIAN_POINT ( 'NONE',  ( 16.53943276465976808, -0.05219959533910856209, 38.74890960531435979 ) ) ;
#107283=CARTESIAN_POINT ( 'NONE',  ( 12.06949235617757843, -12.14591786802309237, 33.12390960531435979 ) ) ;
#107284=CARTESIAN_POINT ( 'NONE',  ( 5.153800228976335163, 19.02544592524342804, 49.79057627198100988 ) ) ;
#107285=CARTESIAN_POINT ( 'NONE',  ( 16.46253265017160672, -9.564922557960803928, 73.33224293864769550 ) ) ;
#107286=CARTESIAN_POINT ( 'NONE',  ( 9.474510206698971260, -16.51473224551069308, 37.91557627198102409 ) ) ;
#107287=CARTESIAN_POINT ( 'NONE',  ( 5.719274019375673035, 21.55341960407619339, 42.29275706135235424 ) ) ;
#107288=CARTESIAN_POINT ( 'NONE',  ( -5.049401038298153566, 19.05341960407611168, 65.20724293864765286 ) ) ;
#107290=CARTESIAN_POINT ( 'NONE',  ( -9.564922557960796823, -16.46253265017161027, 62.08224293864769550 ) ) ;
#107291=CARTESIAN_POINT ( 'NONE',  ( -5.719274019375978568, 21.55341960407610458, 30.20724293864769550 ) ) ;
#107292=CARTESIAN_POINT ( 'NONE',  ( -12.06949235617756955, 12.14591786802309770, 115.6239096053143669 ) ) ;
#107293=CARTESIAN_POINT ( 'NONE',  ( 21.52544592524344225, -5.823673210054117533, 23.54057627198102765 ) ) ;
#107294=CARTESIAN_POINT ( 'NONE',  ( -4.379528057220086978, -16.55341960407618274, 89.79275706135236135 ) ) ;
#107295=CARTESIAN_POINT ( 'NONE',  ( 21.55341960407619695, -5.719274019375665929, 111.0427570613523613 ) ) ;
#107296=CARTESIAN_POINT ( 'NONE',  ( -0.05219959533934338120, 16.53943276465976808, 62.50109039468568284 ) ) ;
#107297=CARTESIAN_POINT ( 'NONE',  ( 16.51473224551069308, 9.474510206698969483, 114.1655762719810241 ) ) ;
#107298=CARTESIAN_POINT ( 'NONE',  ( 8.314922557961029526, -14.29746914071037800, 50.41775706135235424 ) ) ;
#107299=CARTESIAN_POINT ( 'NONE',  ( -0.05219959533934338120, 16.53943276465976808, 37.50109039468568284 ) ) ;
#107300=CARTESIAN_POINT ( 'NONE',  ( -4.483927247898782831, 16.52544592524335698, 92.70942372801901854 ) ) ;
#107301=CARTESIAN_POINT ( 'NONE',  ( 12.14591786802327356, -12.06949235617739191, 30.62609039468567929 ) ) ;
#107302=CARTESIAN_POINT ( 'NONE',  ( 16.51473224551069308, 9.474510206698969483, 34.16557627198102409 ) ) ;
#107303=CARTESIAN_POINT ( 'NONE',  ( 15.72974639402199770, -15.80617190586745480, 113.1239096053143953 ) ) ;
#107304=CARTESIAN_POINT ( 'NONE',  ( 13.89961937509957401, 13.97604488694547697, 111.8760903946856757 ) ) ;
#107305=CARTESIAN_POINT ( 'NONE',  ( 16.55341960407618274, -4.379528057220086978, 86.04275706135236135 ) ) ;
#107307=CARTESIAN_POINT ( 'NONE',  ( -18.62759615963255300, -10.81492255796106328, 89.16775706135236135 ) ) ;
#107308=CARTESIAN_POINT ( 'NONE',  ( -19.02544592524334988, -5.153800228976617603, 88.95942372801897591 ) ) ;
#107309=CARTESIAN_POINT ( 'NONE',  ( -8.314922557960811034, -14.29746914071050412, 57.08224293864769550 ) ) ;
#107310=CARTESIAN_POINT ( 'NONE',  ( 8.224510206698953496, -14.34966873604960469, 42.91557627198103120 ) ) ;
#107311=CARTESIAN_POINT ( 'NONE',  ( -14.29746914071049879, 8.314922557960819915, 110.8322429386476955 ) ) ;
#107312=CARTESIAN_POINT ( 'NONE',  ( 19.03943276465977164, 0.05219959533936151252, 41.25109039468566152 ) ) ;
#107314=CARTESIAN_POINT ( 'NONE',  ( -15.80617190586768217, 15.72974639402176855, 48.12609039468568284 ) ) ;
#107315=CARTESIAN_POINT ( 'NONE',  ( -5.153800228976607833, 19.02544592524334988, 102.7094237280189759 ) ) ;
#107316=DIRECTION ( 'NONE',  ( 0.000000000000000000, 0.000000000000000000, -1.000000000000000000 ) ) ;
#107317=CARTESIAN_POINT ( 'NONE',  ( 13.97604488694527802, 13.89961937509977652, 109.3739096053143669 ) ) ;
#107318=CARTESIAN_POINT ( 'NONE',  ( -10.72451020669898014, 18.67979575497178502, 70.41557627198102409 ) ) ;
#107319=CARTESIAN_POINT ( 'NONE',  ( 13.97604488694548053, -13.89961937509957401, 95.62609039468563310 ) ) ;
#107320=CARTESIAN_POINT ( 'NONE',  ( 5.153800228976335163, 19.02544592524342804, 104.7905762719809957 ) ) ;
#107321=CARTESIAN_POINT ( 'NONE',  ( 17.59860650958997397, -7.585241751806833577, 50.92337014262493256 ) ) ;
#107322=CARTESIAN_POINT ( 'NONE',  ( 14.29746914071049879, -8.314922557960816363, 108.3322429386477097 ) ) ;
#107323=CARTESIAN_POINT ( 'NONE',  ( -5.719274019375665041, -21.55341960407619695, 99.79275706135234714 ) ) ;
#107324=CARTESIAN_POINT ( 'NONE',  ( 16.51473224551069308, 9.474510206698969483, 49.16557627198102409 ) ) ;
#107325=CARTESIAN_POINT ( 'NONE',  ( 21.53943276465977519, 0.05219959533937863772, 56.25109039468568284 ) ) ;
#107326=CARTESIAN_POINT ( 'NONE',  ( -18.67979575497193778, 10.72451020669871902, 93.33442372801901854 ) ) ;
#107327=CARTESIAN_POINT ( 'NONE',  ( -4.379528057220086978, -16.55341960407618274, 89.79275706135236135 ) ) ;
#107328=CARTESIAN_POINT ( 'NONE',  ( 10.81492255796106328, -18.62759615963255655, 40.41775706135234714 ) ) ;
#107329=CARTESIAN_POINT ( 'NONE',  ( -10.72451020669870658, -18.67979575497194134, 39.58442372801901143 ) ) ;
#107330=CARTESIAN_POINT ( 'NONE',  ( 9.564922557961047289, -16.46253265017146816, 65.41775706135233293 ) ) ;
#107331=CARTESIAN_POINT ( 'NONE',  ( 13.89961937509977652, -13.97604488694527269, 98.12390960531433848 ) ) ;
#107332=CARTESIAN_POINT ( 'NONE',  ( -4.379528057220328563, 16.55341960407611168, 100.2072429386476955 ) ) ;
#107333=CARTESIAN_POINT ( 'NONE',  ( 18.62759615963271287, -10.81492255796078972, 88.33224293864769550 ) ) ;
#107334=CARTESIAN_POINT ( 'NONE',  ( -16.53943276465976808, 0.05219959533911058130, 66.24890960531436690 ) ) ;
#107335=CARTESIAN_POINT ( 'NONE',  ( 10.81492255796106328, -18.62759615963255655, 100.4177570613523471 ) ) ;
#107336=CARTESIAN_POINT ( 'NONE',  ( 12.06949235617757843, -12.14591786802309237, 78.12390960531436690 ) ) ;
#107337=CARTESIAN_POINT ( 'NONE',  ( 13.97604488694527802, 13.89961937509977652, 39.37390960531435269 ) ) ;
#107338=CARTESIAN_POINT ( 'NONE',  ( -9.474510206698720793, -16.51473224551083518, 79.58442372801899012 ) ) ;
#107339=CARTESIAN_POINT ( 'NONE',  ( 4.483927247898545687, 16.52544592524342804, 49.79057627198102409 ) ) ;
#107340=CARTESIAN_POINT ( 'NONE',  ( -21.52544592524334988, -5.823673210054445271, 88.95942372801901854 ) ) ;
#107341=CARTESIAN_POINT ( 'NONE',  ( -19.02544592524342804, 5.153800228976336051, 96.04057627198103830 ) ) ;
#107342=CARTESIAN_POINT ( 'NONE',  ( 13.89961937509957401, 13.97604488694547697, 56.87609039468564731 ) ) ;
#107343=CARTESIAN_POINT ( 'NONE',  ( 5.719274019375991003, -21.55341960407610458, 67.70724293864769550 ) ) ;
#107344=CARTESIAN_POINT ( 'NONE',  ( -21.52544592524343514, 5.823673210054127303, 116.0405762719810383 ) ) ;
#107345=CARTESIAN_POINT ( 'NONE',  ( -0.05219959533934338120, 16.53943276465976808, 32.50109039468568284 ) ) ;
#107346=CARTESIAN_POINT ( 'NONE',  ( -4.379528057220086978, -16.55341960407618274, 79.79275706135236135 ) ) ;
#107347=CARTESIAN_POINT ( 'NONE',  ( 16.51473224551069308, 9.474510206698969483, 24.16557627198102765 ) ) ;
#107348=CARTESIAN_POINT ( 'NONE',  ( 10.81492255796106328, -18.62759615963255655, 25.41775706135235779 ) ) ;
#107349=CARTESIAN_POINT ( 'NONE',  ( -0.05219959533909027116, -19.03943276465977164, 27.49890960531435624 ) ) ;
#107351=CARTESIAN_POINT ( 'NONE',  ( -4.483927247898782831, 16.52544592524335698, 52.70942372801902565 ) ) ;
#107352=CARTESIAN_POINT ( 'NONE',  ( 14.34966873604960469, 8.224510206698951720, 79.16557627198103830 ) ) ;
#107353=CARTESIAN_POINT ( 'NONE',  ( -10.72451020669898014, 18.67979575497178502, 75.41557627198102409 ) ) ;
#107354=CARTESIAN_POINT ( 'NONE',  ( -4.379528057220328563, 16.55341960407611168, 30.20724293864769550 ) ) ;
#107355=CARTESIAN_POINT ( 'NONE',  ( 16.53943276465976808, 0.05219959533934440121, 41.25109039468568284 ) ) ;
#107356=CARTESIAN_POINT ( 'NONE',  ( 0.05219959533909260263, 19.03943276465977164, 39.99890960531436690 ) ) ;
#107357=CARTESIAN_POINT ( 'NONE',  ( 0.05219959533934541429, -16.53943276465976808, 75.00109039468568994 ) ) ;
#107358=CARTESIAN_POINT ( 'NONE',  ( -5.049401038297874678, -19.05341960407617918, 74.79275706135231871 ) ) ;
#107359=CARTESIAN_POINT ( 'NONE',  ( -21.55341960407610458, -5.719274019375992779, 71.45724293864769550 ) ) ;
#107360=CARTESIAN_POINT ( 'NONE',  ( -4.483927247898782831, 16.52544592524335698, 107.7094237280190328 ) ) ;
#107362=CARTESIAN_POINT ( 'NONE',  ( -21.53943276465977519, -0.05219959533937600094, 78.75109039468568994 ) ) ;
#107363=EDGE_CURVE ( 'NONE', #60866, #78316, #126727, .T. ) ;
#107364=CARTESIAN_POINT ( 'NONE',  ( 15.72974639402199770, -15.80617190586745480, 43.12390960531435269 ) ) ;
#107365=ORIENTED_EDGE ( 'NONE', *, *, #29998, .F. ) ;
#107367=CARTESIAN_POINT ( 'NONE',  ( -4.483927247898782831, 16.52544592524335698, 87.70942372801901854 ) ) ;
#107368=CARTESIAN_POINT ( 'NONE',  ( -5.823673210054116645, -21.52544592524344225, 47.29057627198103120 ) ) ;
#107370=CARTESIAN_POINT ( 'NONE',  ( -13.89961937509977652, 13.97604488694528158, 110.6239096053143243 ) ) ;
#107372=CARTESIAN_POINT ( 'NONE',  ( -19.02544592524342804, 5.153800228976336051, 26.04057627198103120 ) ) ;
#107373=CARTESIAN_POINT ( 'NONE',  ( -18.67979575497178146, -10.72451020669898902, 71.66557627198100988 ) ) ;
#107374=CARTESIAN_POINT ( 'NONE',  ( 4.379528057220092307, 16.55341960407617563, 107.2927570613523471 ) ) ;
#107375=CARTESIAN_POINT ( 'NONE',  ( -18.62759615963255300, -10.81492255796106328, 64.16775706135234714 ) ) ;
#107376=CARTESIAN_POINT ( 'NONE',  ( 16.53943276465976808, 0.05219959533934440121, 26.25109039468567573 ) ) ;
#107377=CARTESIAN_POINT ( 'NONE',  ( 14.34966873604960469, 8.224510206698951720, 114.1655762719810383 ) ) ;
#107378=CARTESIAN_POINT ( 'NONE',  ( -8.224510206698735004, -14.34966873604973081, 34.58442372801900433 ) ) ;
#107379=CARTESIAN_POINT ( 'NONE',  ( -16.46253265017160317, 9.564922557960807481, 45.83224293864769550 ) ) ;
#107381=CARTESIAN_POINT ( 'NONE',  ( 19.02544592524343514, -5.153800228976328945, 108.5405762719810383 ) ) ;
#107382=CARTESIAN_POINT ( 'NONE',  ( -8.224510206698735004, -14.34966873604973081, 89.58442372801901854 ) ) ;
#107383=CARTESIAN_POINT ( 'NONE',  ( 16.51473224551083163, -9.474510206698727899, 90.83442372801900433 ) ) ;
#107384=CARTESIAN_POINT ( 'NONE',  ( -10.81492255796105439, 18.62759615963255655, 112.9177570613523329 ) ) ;
#107385=CARTESIAN_POINT ( 'NONE',  ( 10.72451020669898902, -18.67979575497178502, 77.91557627198102409 ) ) ;
#107386=CARTESIAN_POINT ( 'NONE',  ( 16.55341960407618274, -4.379528057220086978, 96.04275706135236135 ) ) ;
#107387=CARTESIAN_POINT ( 'NONE',  ( 0.05219959533936267826, -19.03943276465977164, 90.00109039468567573 ) ) ;
#107388=CARTESIAN_POINT ( 'NONE',  ( -0.05219959533909027116, -19.03943276465977164, 47.49890960531435979 ) ) ;
#107389=CARTESIAN_POINT ( 'NONE',  ( 9.564922557960805705, 16.46253265017160317, 89.58224293864769550 ) ) ;
#107390=CARTESIAN_POINT ( 'NONE',  ( 15.72974639402176855, 15.80617190586768217, 51.87609039468568284 ) ) ;
#107391=CARTESIAN_POINT ( 'NONE',  ( 9.474510206698971260, -16.51473224551069308, 42.91557627198103120 ) ) ;
#107393=CARTESIAN_POINT ( 'NONE',  ( 13.89961937509977652, -13.97604488694527269, 113.1239096053143527 ) ) ;
#107394=CARTESIAN_POINT ( 'NONE',  ( 12.14591786802309770, 12.06949235617756955, 64.37390960531435269 ) ) ;
#107395=CARTESIAN_POINT ( 'NONE',  ( 21.53943276465977519, -0.05219959533907433946, 68.74890960531435269 ) ) ;
#107397=CARTESIAN_POINT ( 'NONE',  ( 19.03943276465977164, 0.05219959533936151252, 46.25109039468566863 ) ) ;
#107399=CARTESIAN_POINT ( 'NONE',  ( 13.97604488694527802, 13.89961937509977652, 69.37390960531436690 ) ) ;
#107400=CARTESIAN_POINT ( 'NONE',  ( -13.97604488694527625, -13.89961937509977652, 86.87390960531436690 ) ) ;
#107401=CARTESIAN_POINT ( 'NONE',  ( -16.52544592524335698, -4.483927247898792601, 48.95942372801902565 ) ) ;
#107403=CARTESIAN_POINT ( 'NONE',  ( 13.97604488694548053, -13.89961937509957401, 35.62609039468567573 ) ) ;
#107405=CARTESIAN_POINT ( 'NONE',  ( -16.52544592524335698, -4.483927247898792601, 93.95942372801903275 ) ) ;
#107407=CARTESIAN_POINT ( 'NONE',  ( -4.483927247898782831, 16.52544592524335698, 82.70942372801900433 ) ) ;
#107408=CARTESIAN_POINT ( 'NONE',  ( 14.34966873604972726, -8.224510206698740333, 55.83442372801901854 ) ) ;
#107409=CARTESIAN_POINT ( 'NONE',  ( 19.03943276465977164, 0.05219959533936151252, 26.25109039468566507 ) ) ;
#107410=CARTESIAN_POINT ( 'NONE',  ( -0.05219959533909027116, -19.03943276465977164, 57.49890960531435979 ) ) ;
#107412=CARTESIAN_POINT ( 'NONE',  ( 10.72451020669871369, 18.67979575497193778, 67.08442372801901854 ) ) ;
#107413=CARTESIAN_POINT ( 'NONE',  ( 13.89961937509957401, 13.97604488694547697, 81.87609039468564731 ) ) ;
#107414=CARTESIAN_POINT ( 'NONE',  ( -19.03943276465977164, -0.05219959533935918106, 18.75109039468567218 ) ) ;
#107415=CARTESIAN_POINT ( 'NONE',  ( -19.02544592524342804, 5.153800228976336051, 46.04057627198101699 ) ) ;
#107417=CARTESIAN_POINT ( 'NONE',  ( 15.80617190586746368, 15.72974639402197994, 69.37390960531436690 ) ) ;
#107418=CARTESIAN_POINT ( 'NONE',  ( -19.02544592524342804, 5.153800228976336051, 116.0405762719810383 ) ) ;
#107419=CARTESIAN_POINT ( 'NONE',  ( -0.05219959533910754901, -16.53943276465976808, 112.4989096053143669 ) ) ;
#107420=CARTESIAN_POINT ( 'NONE',  ( -14.29746914071037622, -8.314922557961029526, 44.16775706135234714 ) ) ;
#107421=CARTESIAN_POINT ( 'NONE',  ( -0.05219959533910754901, -16.53943276465976808, 27.49890960531435269 ) ) ;
#107423=CARTESIAN_POINT ( 'NONE',  ( -10.72451020669898014, 18.67979575497178502, 115.4155762719810241 ) ) ;
#107425=CARTESIAN_POINT ( 'NONE',  ( -16.53943276465976808, 0.05219959533911058130, 46.24890960531435979 ) ) ;
#107427=CARTESIAN_POINT ( 'NONE',  ( 16.46253265017146816, 9.564922557961045513, 111.6677570613523329 ) ) ;
#107428=CARTESIAN_POINT ( 'NONE',  ( -16.46253265017146816, -9.564922557961047289, 29.16775706135232937 ) ) ;
#107429=CARTESIAN_POINT ( 'NONE',  ( 4.483927247898545687, 16.52544592524342804, 49.79057627198102409 ) ) ;
#107430=CARTESIAN_POINT ( 'NONE',  ( -10.72451020669898014, 18.67979575497178502, 100.4155762719810241 ) ) ;
#107431=CARTESIAN_POINT ( 'NONE',  ( 17.50000000000000000, 5.500000000000001776, 33.78230962303567253 ) ) ;
#107432=CARTESIAN_POINT ( 'NONE',  ( 15.72974639402199770, -15.80617190586745480, 63.12390960531435979 ) ) ;
#107433=CARTESIAN_POINT ( 'NONE',  ( -5.153800228976328057, -19.02544592524343514, 77.29057627198099567 ) ) ;
#107434=CARTESIAN_POINT ( 'NONE',  ( -12.06949235617756955, 12.14591786802309770, 50.62390960531435979 ) ) ;
#107435=CARTESIAN_POINT ( 'NONE',  ( 19.05341960407611168, 5.049401038298154454, 98.95724293864766707 ) ) ;
#107437=CARTESIAN_POINT ( 'NONE',  ( -13.97604488694547697, 13.89961937509957934, 58.12609039468566863 ) ) ;
#107438=CARTESIAN_POINT ( 'NONE',  ( -15.80617190586745835, -15.72974639402198527, 96.87390960531436690 ) ) ;
#107439=CARTESIAN_POINT ( 'NONE',  ( 9.474510206698971260, -16.51473224551069308, 42.91557627198103120 ) ) ;
#107440=CARTESIAN_POINT ( 'NONE',  ( 16.51473224551069308, 9.474510206698969483, 24.16557627198102765 ) ) ;
#107441=CARTESIAN_POINT ( 'NONE',  ( -15.72974639402176322, -15.80617190586768395, 49.37609039468569705 ) ) ;
#107443=CARTESIAN_POINT ( 'NONE',  ( 16.55341960407611168, 4.379528057220329451, 33.95724293864769550 ) ) ;
#107444=CARTESIAN_POINT ( 'NONE',  ( -19.02544592524342804, 5.153800228976336051, 56.04057627198100988 ) ) ;
#107445=CARTESIAN_POINT ( 'NONE',  ( -16.51473224551069308, -9.474510206698971260, 96.66557627198102409 ) ) ;
#107446=CARTESIAN_POINT ( 'NONE',  ( 21.55341960407610458, 5.719274019375980345, 58.95724293864770971 ) ) ;
#107447=CARTESIAN_POINT ( 'NONE',  ( -19.52837319214027900, 5.499999999999900524, 44.60471352585542348 ) ) ;
#107448=CARTESIAN_POINT ( 'NONE',  ( -19.03943276465977164, 0.05219959533909376836, 41.24890960531435269 ) ) ;
#107449=CARTESIAN_POINT ( 'NONE',  ( -21.55341960407610458, -5.719274019375992779, 56.45724293864768839 ) ) ;
#107450=CARTESIAN_POINT ( 'NONE',  ( 21.52544592524334988, 5.823673210054432836, 86.45942372801901854 ) ) ;
#107452=CARTESIAN_POINT ( 'NONE',  ( -8.314922557961024197, 14.29746914071037800, 77.91775706135231871 ) ) ;
#107453=CARTESIAN_POINT ( 'NONE',  ( -0.05219959533934338120, 16.53943276465976808, 87.50109039468568994 ) ) ;
#107454=CARTESIAN_POINT ( 'NONE',  ( -19.03943276465977164, 0.05219959533909376836, 66.24890960531436690 ) ) ;
#107456=CARTESIAN_POINT ( 'NONE',  ( -13.97604488694547697, 13.89961937509957934, 28.12609039468565797 ) ) ;
#107457=CARTESIAN_POINT ( 'NONE',  ( 16.52544592524335698, 4.483927247898782831, 86.45942372801901854 ) ) ;
#107458=CARTESIAN_POINT ( 'NONE',  ( 15.72974639402176855, 15.80617190586768217, 111.8760903946856615 ) ) ;
#107459=CARTESIAN_POINT ( 'NONE',  ( 0.05219959533909260263, 19.03943276465977164, 74.99890960531435269 ) ) ;
#107460=CARTESIAN_POINT ( 'NONE',  ( 21.55341960407610458, 5.719274019375980345, 53.95724293864770260 ) ) ;
#107461=CARTESIAN_POINT ( 'NONE',  ( 16.52544592524335698, 4.483927247898782831, 21.45942372801901499 ) ) ;
#107462=CARTESIAN_POINT ( 'NONE',  ( 21.55341960407619695, -5.719274019375665929, 76.04275706135237556 ) ) ;
#107463=CARTESIAN_POINT ( 'NONE',  ( -8.314922557961024197, 14.29746914071037800, 67.91775706135234714 ) ) ;
#107464=CARTESIAN_POINT ( 'NONE',  ( -10.81492255796078084, -18.62759615963271287, 112.0822429386477097 ) ) ;
#107465=CARTESIAN_POINT ( 'NONE',  ( -19.03943276465977164, -0.05219959533935918106, 108.7510903946856615 ) ) ;
#107466=CARTESIAN_POINT ( 'NONE',  ( 19.03943276465977164, -0.05219959533909143690, 73.74890960531435269 ) ) ;
#107467=CARTESIAN_POINT ( 'NONE',  ( -14.29746914071037622, -8.314922557961029526, 24.16775706135235424 ) ) ;
#107468=CARTESIAN_POINT ( 'NONE',  ( 5.049401038298161559, -19.05341960407611168, 37.70724293864768839 ) ) ;
#107469=CARTESIAN_POINT ( 'NONE',  ( 5.049401038297881783, 19.05341960407617563, 112.2927570613523471 ) ) ;
#107470=CARTESIAN_POINT ( 'NONE',  ( 8.224510206698953496, -14.34966873604960469, 82.91557627198103830 ) ) ;
#107471=CARTESIAN_POINT ( 'NONE',  ( -16.55341960407617563, 4.379528057220093196, 93.54275706135234714 ) ) ;
#107472=CARTESIAN_POINT ( 'NONE',  ( 21.55341960407619695, -5.719274019375665929, 36.04275706135234714 ) ) ;
#107473=CARTESIAN_POINT ( 'NONE',  ( 9.564922557960805705, 16.46253265017160317, 69.58224293864770971 ) ) ;
#107474=CARTESIAN_POINT ( 'NONE',  ( 5.049401038298161559, -19.05341960407611168, 62.70724293864769550 ) ) ;
#107475=CARTESIAN_POINT ( 'NONE',  ( -8.224510206698735004, -14.34966873604973081, 89.58442372801901854 ) ) ;
#107479=CARTESIAN_POINT ( 'NONE',  ( 19.05341960407617918, -5.049401038297876454, 26.04275706135233293 ) ) ;
#107480=CARTESIAN_POINT ( 'NONE',  ( 9.474510206698971260, -16.51473224551069308, 32.91557627198102409 ) ) ;
#107482=VERTEX_POINT ( 'NONE', #89052 ) ;
#107483=CARTESIAN_POINT ( 'NONE',  ( 4.379528057220092307, 16.55341960407617563, 27.29275706135234358 ) ) ;
#107484=CARTESIAN_POINT ( 'NONE',  ( 5.153800228976615827, -19.02544592524334988, 60.20942372801899012 ) ) ;
#107485=CARTESIAN_POINT ( 'NONE',  ( -4.483927247898782831, 16.52544592524335698, 47.70942372801902565 ) ) ;
#107486=CARTESIAN_POINT ( 'NONE',  ( -19.05341960407611168, -5.049401038298163336, 111.4572429386476671 ) ) ;
#107487=CARTESIAN_POINT ( 'NONE',  ( 16.51473224551069308, 9.474510206698969483, 69.16557627198102409 ) ) ;
#107488=CARTESIAN_POINT ( 'NONE',  ( -15.80617190586745835, -15.72974639402198527, 96.87390960531436690 ) ) ;
#107489=CARTESIAN_POINT ( 'NONE',  ( 0.05219959533909260263, 19.03943276465977164, 94.99890960531436690 ) ) ;
#107490=CARTESIAN_POINT ( 'NONE',  ( -5.153800228976328057, -19.02544592524343514, 27.29057627198103120 ) ) ;
#107492=CARTESIAN_POINT ( 'NONE',  ( -19.03943276465977164, 0.05219959533909376836, 66.24890960531436690 ) ) ;
#107493=CARTESIAN_POINT ( 'NONE',  ( 16.55341960407611168, 4.379528057220329451, 23.95724293864769550 ) ) ;
#107494=CARTESIAN_POINT ( 'NONE',  ( 9.474510206698971260, -16.51473224551069308, 22.91557627198102765 ) ) ;
#107495=CARTESIAN_POINT ( 'NONE',  ( -19.03943276465977164, -0.05219959533935918106, 43.75109039468566863 ) ) ;
#107497=CARTESIAN_POINT ( 'NONE',  ( 16.52544592524342804, -4.483927247898539470, 73.54057627198102409 ) ) ;
#107498=CARTESIAN_POINT ( 'NONE',  ( 5.719274019375673035, 21.55341960407619339, 92.29275706135236135 ) ) ;
#107499=CARTESIAN_POINT ( 'NONE',  ( -13.97604488694527625, -13.89961937509977652, 36.87390960531436690 ) ) ;
#107500=CARTESIAN_POINT ( 'NONE',  ( -12.14591786802326823, 12.06949235617739902, 48.12609039468568284 ) ) ;
#107501=CARTESIAN_POINT ( 'NONE',  ( -16.52544592524342804, 4.483927247898546575, 46.04057627198103830 ) ) ;
#107502=CARTESIAN_POINT ( 'NONE',  ( -5.719274019375665041, -21.55341960407619695, 94.79275706135234714 ) ) ;
#107503=CARTESIAN_POINT ( 'NONE',  ( -9.474510206698964154, 16.51473224551069663, 85.41557627198102409 ) ) ;
#107504=CARTESIAN_POINT ( 'NONE',  ( -19.03943276465977164, 0.05219959533909376836, 91.24890960531436690 ) ) ;
#107505=CARTESIAN_POINT ( 'NONE',  ( 16.52544592524342804, -4.483927247898539470, 108.5405762719810241 ) ) ;
#107506=CARTESIAN_POINT ( 'NONE',  ( -16.55341960407611168, -4.379528057220339221, 76.45724293864769550 ) ) ;
#107507=CARTESIAN_POINT ( 'NONE',  ( -15.80617190586745835, -15.72974639402198527, 86.87390960531438111 ) ) ;
#107508=CARTESIAN_POINT ( 'NONE',  ( -13.97604488694527625, -13.89961937509977652, 91.87390960531432427 ) ) ;
#107509=CARTESIAN_POINT ( 'NONE',  ( 0.05219959533907565091, 21.53943276465977519, 94.99890960531436690 ) ) ;
#107510=CARTESIAN_POINT ( 'NONE',  ( 9.474510206698729675, 16.51473224551082808, 72.08442372801900433 ) ) ;
#107512=CARTESIAN_POINT ( 'NONE',  ( -14.29746914071049879, 8.314922557960819915, 95.83224293864770971 ) ) ;
#107513=CARTESIAN_POINT ( 'NONE',  ( -13.97604488694527625, -13.89961937509977652, 51.87390960531436690 ) ) ;
#107514=CARTESIAN_POINT ( 'NONE',  ( -10.72451020669898014, 18.67979575497178502, 70.41557627198102409 ) ) ;
#107515=CARTESIAN_POINT ( 'NONE',  ( 17.44270441346514033, -5.991230190323081573, 26.13664920735773478 ) ) ;
#107516=CARTESIAN_POINT ( 'NONE',  ( 14.34966873604972726, -8.224510206698740333, 105.8344237280190328 ) ) ;
#107518=CARTESIAN_POINT ( 'NONE',  ( 16.51473224551083163, -9.474510206698727899, 110.8344237280190043 ) ) ;
#107519=CARTESIAN_POINT ( 'NONE',  ( 8.314922557960818139, 14.29746914071049879, 79.58224293864769550 ) ) ;
#107521=CARTESIAN_POINT ( 'NONE',  ( 19.03943276465977164, -0.05219959533909143690, 68.74890960531436690 ) ) ;
#107522=CARTESIAN_POINT ( 'NONE',  ( 9.474510206698971260, -16.51473224551069308, 37.91557627198102409 ) ) ;
#107523=CARTESIAN_POINT ( 'NONE',  ( -12.14591786802309592, -12.06949235617757132, 71.87390960531438111 ) ) ;
#107524=CARTESIAN_POINT ( 'NONE',  ( -21.53943276465977519, 0.05219959533907696930, 26.24890960531435624 ) ) ;
#107525=CARTESIAN_POINT ( 'NONE',  ( 16.51473224551083163, -9.474510206698727899, 90.83442372801900433 ) ) ;
#107526=CARTESIAN_POINT ( 'NONE',  ( -16.46253265017160317, 9.564922557960807481, 100.8322429386477097 ) ) ;
#107527=CARTESIAN_POINT ( 'NONE',  ( -15.80617190586745835, -15.72974639402198527, 81.87390960531435269 ) ) ;
#107528=CARTESIAN_POINT ( 'NONE',  ( 8.314922557961029526, -14.29746914071037800, 70.41775706135236135 ) ) ;
#107529=CARTESIAN_POINT ( 'NONE',  ( -16.62475595723611832, 7.163666690055876529, 95.52713351810403708 ) ) ;
#107530=CARTESIAN_POINT ( 'NONE',  ( 13.97604488694527802, 13.89961937509977652, 64.37390960531436690 ) ) ;
#107531=CARTESIAN_POINT ( 'NONE',  ( 5.719274019375991003, -21.55341960407610458, 62.70724293864769550 ) ) ;
#107533=CARTESIAN_POINT ( 'NONE',  ( 13.89961937509957401, 13.97604488694547697, 101.8760903946856331 ) ) ;
#107534=CARTESIAN_POINT ( 'NONE',  ( 12.06949235617757843, -12.14591786802309237, 33.12390960531435979 ) ) ;
#107535=CARTESIAN_POINT ( 'NONE',  ( -15.80617190586768217, 15.72974639402176855, 58.12609039468568994 ) ) ;
#107536=CARTESIAN_POINT ( 'NONE',  ( 17.72662750342724536, 5.500000000000079048, 83.90179492283742491 ) ) ;
#107537=CARTESIAN_POINT ( 'NONE',  ( -8.224510206698735004, -14.34966873604973081, 69.58442372801900433 ) ) ;
#107538=CARTESIAN_POINT ( 'NONE',  ( 16.51473224551069308, 9.474510206698969483, 109.1655762719810383 ) ) ;
#107539=CARTESIAN_POINT ( 'NONE',  ( 5.153800228976335163, 19.02544592524342804, 104.7905762719810241 ) ) ;
#107541=CARTESIAN_POINT ( 'NONE',  ( -14.29746914071037622, -8.314922557961029526, 99.16775706135234714 ) ) ;
#107542=CARTESIAN_POINT ( 'NONE',  ( -8.224510206698735004, -14.34966873604973081, 49.58442372801901143 ) ) ;
#107543=CARTESIAN_POINT ( 'NONE',  ( -19.02544592524342804, 5.153800228976336051, 56.04057627198100988 ) ) ;
#107544=CARTESIAN_POINT ( 'NONE',  ( -5.049401038298153566, 19.05341960407611168, 70.20724293864769550 ) ) ;
#107545=CARTESIAN_POINT ( 'NONE',  ( -10.81492255796105439, 18.62759615963255655, 52.91775706135235424 ) ) ;
#107546=CARTESIAN_POINT ( 'NONE',  ( 16.52544592524335698, 4.483927247898782831, 56.45942372801902565 ) ) ;
#107547=CARTESIAN_POINT ( 'NONE',  ( 8.314922557960818139, 14.29746914071049879, 34.58224293864770260 ) ) ;
#107548=CARTESIAN_POINT ( 'NONE',  ( -0.05219959533909027116, -19.03943276465977164, 47.49890960531435979 ) ) ;
#107549=CARTESIAN_POINT ( 'NONE',  ( 16.46253265017160672, -9.564922557960803928, 33.33224293864770260 ) ) ;
#107550=CARTESIAN_POINT ( 'NONE',  ( -4.483927247898782831, 16.52544592524335698, 27.70942372801901854 ) ) ;
#107551=CARTESIAN_POINT ( 'NONE',  ( 16.46253265017146816, 9.564922557961045513, 76.66775706135234714 ) ) ;
#107552=CARTESIAN_POINT ( 'NONE',  ( 8.314922557960818139, 14.29746914071049879, 89.58224293864768129 ) ) ;
#107553=CARTESIAN_POINT ( 'NONE',  ( 19.02544592524343514, -5.153800228976328945, 48.54057627198103120 ) ) ;
#107554=CARTESIAN_POINT ( 'NONE',  ( 16.46253265017146816, 9.564922557961045513, 81.66775706135233293 ) ) ;
#107556=CARTESIAN_POINT ( 'NONE',  ( -5.719274019375665041, -21.55341960407619695, 84.79275706135234714 ) ) ;
#107557=CARTESIAN_POINT ( 'NONE',  ( -8.224510206698735004, -14.34966873604973081, 49.58442372801901143 ) ) ;
#107559=CARTESIAN_POINT ( 'NONE',  ( -18.62759615963270932, 10.81492255796079327, 50.83224293864770971 ) ) ;
#107560=CARTESIAN_POINT ( 'NONE',  ( -16.52544592524335698, -4.483927247898792601, 38.95942372801901854 ) ) ;
#107561=CARTESIAN_POINT ( 'NONE',  ( -19.36337904590693171, 5.499999999999952927, 70.41494137495622851 ) ) ;
#107562=CARTESIAN_POINT ( 'NONE',  ( 13.89961937509957401, 13.97604488694547697, 46.87609039468565442 ) ) ;
#107563=CARTESIAN_POINT ( 'NONE',  ( 19.03943276465977164, -0.05219959533909143690, 93.74890960531435269 ) ) ;
#107564=CARTESIAN_POINT ( 'NONE',  ( -16.51473224551069308, -9.474510206698971260, 56.66557627198103120 ) ) ;
#107565=CARTESIAN_POINT ( 'NONE',  ( 17.50000000000000000, 5.499999999999992895, 86.70309617465828467 ) ) ;
#107566=CARTESIAN_POINT ( 'NONE',  ( 5.719274019375673035, 21.55341960407619339, 72.29275706135236135 ) ) ;
#107569=CARTESIAN_POINT ( 'NONE',  ( -13.89961937509957401, -13.97604488694547875, 34.37609039468566863 ) ) ;
#107570=CARTESIAN_POINT ( 'NONE',  ( 15.72974639402176855, 15.80617190586768217, 106.8760903946856899 ) ) ;
#107571=CARTESIAN_POINT ( 'NONE',  ( -16.53943276465976808, 0.05219959533911058130, 31.24890960531435979 ) ) ;
#107572=CARTESIAN_POINT ( 'NONE',  ( 13.89961937509977652, -13.97604488694527269, 58.12390960531436690 ) ) ;
#107573=CARTESIAN_POINT ( 'NONE',  ( 13.97604488694527802, 13.89961937509977652, 104.3739096053143385 ) ) ;
#107574=CARTESIAN_POINT ( 'NONE',  ( 21.55341960407619695, -5.719274019375665929, 86.04275706135236135 ) ) ;
#107575=CARTESIAN_POINT ( 'NONE',  ( 13.97604488694527802, 13.89961937509977652, 64.37390960531436690 ) ) ;
#107576=CARTESIAN_POINT ( 'NONE',  ( -0.05219959533937732626, 21.53943276465977519, 82.50109039468568994 ) ) ;
#107577=CARTESIAN_POINT ( 'NONE',  ( 18.62759615963271287, -10.81492255796078972, 38.33224293864768839 ) ) ;
#107579=CARTESIAN_POINT ( 'NONE',  ( 18.67979575497194134, -10.72451020669871369, 30.83442372801902209 ) ) ;
#107580=CARTESIAN_POINT ( 'NONE',  ( -5.049401038297874678, -19.05341960407617918, 54.79275706135234003 ) ) ;
#107581=CARTESIAN_POINT ( 'NONE',  ( 19.05341960407611168, 5.049401038298154454, 23.95724293864769194 ) ) ;
#107582=CARTESIAN_POINT ( 'NONE',  ( 0.05219959533909260263, 19.03943276465977164, 69.99890960531435269 ) ) ;
#107583=CARTESIAN_POINT ( 'NONE',  ( -14.34966873604972548, 8.224510206698743886, 23.33442372801901499 ) ) ;
#107584=CARTESIAN_POINT ( 'NONE',  ( 4.483927247898545687, 16.52544592524342804, 89.79057627198103830 ) ) ;
#107585=CARTESIAN_POINT ( 'NONE',  ( -5.049401038298153566, 19.05341960407611168, 55.20724293864769550 ) ) ;
#107586=CARTESIAN_POINT ( 'NONE',  ( -10.81492255796078084, -18.62759615963271287, 42.08224293864769550 ) ) ;
#107587=CARTESIAN_POINT ( 'NONE',  ( 9.564922557961047289, -16.46253265017146816, 105.4177570613523471 ) ) ;
#107588=CARTESIAN_POINT ( 'NONE',  ( 0.05219959533907565091, 21.53943276465977519, 104.9989096053143669 ) ) ;
#107589=CARTESIAN_POINT ( 'NONE',  ( -5.719274019375665041, -21.55341960407619695, 69.79275706135234714 ) ) ;
#107590=CARTESIAN_POINT ( 'NONE',  ( 8.224510206698742110, 14.34966873604972548, 72.08442372801899012 ) ) ;
#107591=CARTESIAN_POINT ( 'NONE',  ( -14.34966873604972548, 8.224510206698743886, 63.33442372801900433 ) ) ;
#107592=CARTESIAN_POINT ( 'NONE',  ( -5.153800228976328057, -19.02544592524343514, 67.29057627198102409 ) ) ;
#107593=CARTESIAN_POINT ( 'NONE',  ( 14.29746914071037800, 8.314922557961029526, 91.66775706135234714 ) ) ;
#107594=CARTESIAN_POINT ( 'NONE',  ( -19.02544592524334988, -5.153800228976617603, 38.95942372801900433 ) ) ;
#107595=CARTESIAN_POINT ( 'NONE',  ( -0.05219959533937732626, 21.53943276465977519, 22.50109039468567573 ) ) ;
#107596=CARTESIAN_POINT ( 'NONE',  ( 4.379528057220339221, -16.55341960407611168, 62.70724293864769550 ) ) ;
#107597=CARTESIAN_POINT ( 'NONE',  ( 5.153800228976335163, 19.02544592524342804, 79.79057627198102409 ) ) ;
#107598=CARTESIAN_POINT ( 'NONE',  ( 4.379528057220092307, 16.55341960407617563, 82.29275706135234714 ) ) ;
#107599=CARTESIAN_POINT ( 'NONE',  ( -18.67979575497193778, 10.72451020669871902, 63.33442372801900433 ) ) ;
#107600=CARTESIAN_POINT ( 'NONE',  ( -16.52544592524335698, -4.483927247898792601, 23.95942372801901143 ) ) ;
#107601=CARTESIAN_POINT ( 'NONE',  ( -18.62759615963270932, 10.81492255796079327, 110.8322429386476955 ) ) ;
#107602=CARTESIAN_POINT ( 'NONE',  ( 16.53943276465976808, -0.05219959533910856209, 53.74890960531437401 ) ) ;
#107604=CARTESIAN_POINT ( 'NONE',  ( 18.62759615963271287, -10.81492255796078972, 88.33224293864769550 ) ) ;
#107605=CARTESIAN_POINT ( 'NONE',  ( 8.314922557960818139, 14.29746914071049879, 39.58224293864769550 ) ) ;
#107608=CARTESIAN_POINT ( 'NONE',  ( 0.05219959533907565091, 21.53943276465977519, 114.9989096053143669 ) ) ;
#107609=CARTESIAN_POINT ( 'NONE',  ( 13.97604488694527802, 13.89961937509977652, 109.3739096053143669 ) ) ;
#107610=CARTESIAN_POINT ( 'NONE',  ( 10.72451020669871369, 18.67979575497193778, 42.08442372801901854 ) ) ;
#107611=CARTESIAN_POINT ( 'NONE',  ( -8.224510206698948167, 14.34966873604960824, 45.41557627198103830 ) ) ;
#107612=CARTESIAN_POINT ( 'NONE',  ( -5.153800228976328057, -19.02544592524343514, 62.29057627198100988 ) ) ;
#107613=CARTESIAN_POINT ( 'NONE',  ( 13.97604488694548053, -13.89961937509957401, 60.62609039468564731 ) ) ;
#107614=CARTESIAN_POINT ( 'NONE',  ( -5.049401038298153566, 19.05341960407611168, 95.20724293864770971 ) ) ;
#107615=CARTESIAN_POINT ( 'NONE',  ( 21.55341960407610458, 5.719274019375980345, 53.95724293864770260 ) ) ;
#107617=CARTESIAN_POINT ( 'NONE',  ( 16.51473224551069308, 9.474510206698969483, 54.16557627198103120 ) ) ;
#107618=CARTESIAN_POINT ( 'NONE',  ( -14.29746914071037622, -8.314922557961029526, 34.16775706135234714 ) ) ;
#107619=CARTESIAN_POINT ( 'NONE',  ( -9.564922557961040184, 16.46253265017147172, 62.91775706135233293 ) ) ;
#107620=CARTESIAN_POINT ( 'NONE',  ( -10.72451020669870658, -18.67979575497194134, 19.58442372801901143 ) ) ;
#107621=CARTESIAN_POINT ( 'NONE',  ( -16.53943276465976808, 0.05219959533911058130, 46.24890960531435979 ) ) ;
#107622=CARTESIAN_POINT ( 'NONE',  ( -16.51473224551069308, -9.474510206698971260, 91.66557627198103830 ) ) ;
#107623=CARTESIAN_POINT ( 'NONE',  ( -5.719274019375978568, 21.55341960407610458, 75.20724293864769550 ) ) ;
#107624=CARTESIAN_POINT ( 'NONE',  ( -0.05219959533907301413, -21.53943276465977519, 97.49890960531436690 ) ) ;
#107625=CARTESIAN_POINT ( 'NONE',  ( 4.379528057220092307, 16.55341960407617563, 37.29275706135235424 ) ) ;
#107626=CARTESIAN_POINT ( 'NONE',  ( 21.55341960407610458, 5.719274019375980345, 38.95724293864768839 ) ) ;
#107627=CARTESIAN_POINT ( 'NONE',  ( -10.81492255796105439, 18.62759615963255655, 82.91775706135234714 ) ) ;
#107628=CARTESIAN_POINT ( 'NONE',  ( -5.153800228976328057, -19.02544592524343514, 87.29057627198103830 ) ) ;
#107629=CARTESIAN_POINT ( 'NONE',  ( 9.564922557960805705, 16.46253265017160317, 44.58224293864769550 ) ) ;
#107630=CARTESIAN_POINT ( 'NONE',  ( 0.05219959533909260263, 19.03943276465977164, 99.99890960531436690 ) ) ;
#107631=CARTESIAN_POINT ( 'NONE',  ( 14.29746914071049879, -8.314922557960816363, 98.33224293864769550 ) ) ;
#107632=CARTESIAN_POINT ( 'NONE',  ( -16.51473224551069308, -9.474510206698971260, 61.66557627198103120 ) ) ;
#107633=CARTESIAN_POINT ( 'NONE',  ( 8.224510206698742110, 14.34966873604972548, 27.08442372801901854 ) ) ;
#107634=VECTOR ( 'NONE', #87769, 1000.000000000000000 ) ;
#107635=CARTESIAN_POINT ( 'NONE',  ( 17.49999999999999645, 4.640572885337623354, 31.86211835451160113 ) ) ;
#107636=CARTESIAN_POINT ( 'NONE',  ( 16.46253265017146816, 9.564922557961045513, 51.66775706135233293 ) ) ;
#107637=CARTESIAN_POINT ( 'NONE',  ( 9.564922557961047289, -16.46253265017146816, 20.41775706135233293 ) ) ;
#107638=CARTESIAN_POINT ( 'NONE',  ( -21.52544592524343514, 5.823673210054127303, 36.04057627198102409 ) ) ;
#107639=CARTESIAN_POINT ( 'NONE',  ( 4.483927247898790824, -16.52544592524335698, 95.20942372801903275 ) ) ;
#107641=CARTESIAN_POINT ( 'NONE',  ( -16.51473224551082808, 9.474510206698731452, 73.33442372801900433 ) ) ;
#107642=CARTESIAN_POINT ( 'NONE',  ( -5.153800228976607833, 19.02544592524334988, 37.70942372801899722 ) ) ;
#107643=CARTESIAN_POINT ( 'NONE',  ( -17.31747979337948351, -6.344076630961018815, 46.37944868065184068 ) ) ;
#107644=CARTESIAN_POINT ( 'NONE',  ( -13.97604488694527625, -13.89961937509977652, 46.87390960531435979 ) ) ;
#107645=CARTESIAN_POINT ( 'NONE',  ( 12.06949235617757843, -12.14591786802309237, 43.12390960531435269 ) ) ;
#107646=CARTESIAN_POINT ( 'NONE',  ( 19.02544592524343514, -5.153800228976328945, 23.54057627198102054 ) ) ;
#107647=CARTESIAN_POINT ( 'NONE',  ( -8.314922557960811034, -14.29746914071050412, 27.08224293864769550 ) ) ;
#107649=CARTESIAN_POINT ( 'NONE',  ( -16.55341960407617563, 4.379528057220093196, 93.54275706135234714 ) ) ;
#107650=CARTESIAN_POINT ( 'NONE',  ( 16.51473224551069308, 9.474510206698969483, 34.16557627198102409 ) ) ;
#107651=CARTESIAN_POINT ( 'NONE',  ( 18.62759615963255655, 10.81492255796105972, 101.6677570613523613 ) ) ;
#107652=CARTESIAN_POINT ( 'NONE',  ( -16.55341960407617563, 4.379528057220093196, 23.54275706135235424 ) ) ;
#107653=CARTESIAN_POINT ( 'NONE',  ( 10.81492255796106328, -18.62759615963255655, 80.41775706135234714 ) ) ;
#107654=CARTESIAN_POINT ( 'NONE',  ( 16.51473224551083163, -9.474510206698727899, 50.83442372801899722 ) ) ;
#107655=CARTESIAN_POINT ( 'NONE',  ( 13.89961937509977652, -13.97604488694527269, 93.12390960531436690 ) ) ;
#107656=CARTESIAN_POINT ( 'NONE',  ( 9.564922557960805705, 16.46253265017160317, 84.58224293864769550 ) ) ;
#107657=CARTESIAN_POINT ( 'NONE',  ( -19.01533133064924996, 5.499999999999452882, 38.76586590595740489 ) ) ;
#107658=CARTESIAN_POINT ( 'NONE',  ( 18.62759615963271287, -10.81492255796078972, 103.3322429386476955 ) ) ;
#107659=CARTESIAN_POINT ( 'NONE',  ( 8.224510206698953496, -14.34966873604960469, 62.91557627198102409 ) ) ;
#107660=CARTESIAN_POINT ( 'NONE',  ( -10.72451020669898014, 18.67979575497178502, 55.41557627198102409 ) ) ;
#107661=CARTESIAN_POINT ( 'NONE',  ( -13.97604488694527625, -13.89961937509977652, 56.87390960531434558 ) ) ;
#107662=CARTESIAN_POINT ( 'NONE',  ( -21.53943276465977519, 0.05219959533907696930, 91.24890960531436690 ) ) ;
#107663=CARTESIAN_POINT ( 'NONE',  ( -8.224510206698735004, -14.34966873604973081, 89.58442372801901854 ) ) ;
#107665=CARTESIAN_POINT ( 'NONE',  ( -13.97604488694527625, -13.89961937509977652, 41.87390960531435979 ) ) ;
#107666=CARTESIAN_POINT ( 'NONE',  ( -16.52544592524342804, 4.483927247898546575, 96.04057627198102409 ) ) ;
#107668=CARTESIAN_POINT ( 'NONE',  ( -5.049401038298153566, 19.05341960407611168, 50.20724293864770260 ) ) ;
#107669=CARTESIAN_POINT ( 'NONE',  ( -9.564922557960796823, -16.46253265017161027, 22.08224293864768839 ) ) ;
#107670=CARTESIAN_POINT ( 'NONE',  ( 13.97604488694548053, -13.89961937509957401, 75.62609039468564731 ) ) ;
#107671=CARTESIAN_POINT ( 'NONE',  ( 16.52544592524342804, -4.483927247898539470, 88.54057627198103830 ) ) ;
#107672=CARTESIAN_POINT ( 'NONE',  ( 21.55341960407619695, -5.719274019375665929, 51.04275706135234714 ) ) ;
#107673=CARTESIAN_POINT ( 'NONE',  ( 19.03943276465977164, -0.05219959533909143690, 33.74890960531435979 ) ) ;
#107674=CARTESIAN_POINT ( 'NONE',  ( -18.62759615963270932, 10.81492255796079327, 100.8322429386477097 ) ) ;
#107675=CARTESIAN_POINT ( 'NONE',  ( 16.52544592524342804, -4.483927247898539470, 93.54057627198103830 ) ) ;
#107676=CARTESIAN_POINT ( 'NONE',  ( 17.60779699588841041, 5.499999999999981348, 93.84981316670106821 ) ) ;
#107677=CARTESIAN_POINT ( 'NONE',  ( 19.02544592524343514, -5.153800228976328945, 53.54057627198102409 ) ) ;
#107678=CARTESIAN_POINT ( 'NONE',  ( 18.56399227203345603, 5.499999999999817923, 46.47830131249904895 ) ) ;
#107679=CARTESIAN_POINT ( 'NONE',  ( 5.049401038297881783, 19.05341960407617563, 92.29275706135234714 ) ) ;
#107680=CARTESIAN_POINT ( 'NONE',  ( 21.53943276465977519, -0.05219959533907433946, 23.74890960531435269 ) ) ;
#107681=CARTESIAN_POINT ( 'NONE',  ( 21.55341960407619695, -5.719274019375665929, 31.04275706135234714 ) ) ;
#107682=CARTESIAN_POINT ( 'NONE',  ( -19.02544592524342804, 5.153800228976336051, 86.04057627198103830 ) ) ;
#107683=CARTESIAN_POINT ( 'NONE',  ( -19.03943276465977164, -0.05219959533935918106, 63.75109039468566863 ) ) ;
#107684=CARTESIAN_POINT ( 'NONE',  ( -5.049401038298153566, 19.05341960407611168, 55.20724293864769550 ) ) ;
#107685=CARTESIAN_POINT ( 'NONE',  ( 12.06949235617757843, -12.14591786802309237, 73.12390960531436690 ) ) ;
#107686=CARTESIAN_POINT ( 'NONE',  ( 4.379528057220339221, -16.55341960407611168, 72.70724293864769550 ) ) ;
#107687=CARTESIAN_POINT ( 'NONE',  ( 13.89961937509977652, -13.97604488694527269, 88.12390960531438111 ) ) ;
#107688=CARTESIAN_POINT ( 'NONE',  ( -18.62759615963270932, 10.81492255796079327, 95.83224293864770971 ) ) ;
#107689=CARTESIAN_POINT ( 'NONE',  ( -19.03943276465977164, 0.05219959533909376836, 91.24890960531436690 ) ) ;
#107690=CARTESIAN_POINT ( 'NONE',  ( -16.46253265017146816, -9.564922557961047289, 29.16775706135232937 ) ) ;
#107691=CARTESIAN_POINT ( 'NONE',  ( -13.89961937509977652, 13.97604488694528158, 40.62390960531435979 ) ) ;
#107692=CARTESIAN_POINT ( 'NONE',  ( -14.29746914071049879, 8.314922557960819915, 30.83224293864770260 ) ) ;
#107693=CARTESIAN_POINT ( 'NONE',  ( 12.14591786802309770, 12.06949235617756955, 109.3739096053143811 ) ) ;
#107695=CARTESIAN_POINT ( 'NONE',  ( -10.81492255796105439, 18.62759615963255655, 32.91775706135234714 ) ) ;
#107696=CARTESIAN_POINT ( 'NONE',  ( 16.51473224551083163, -9.474510206698727899, 65.83442372801900433 ) ) ;
#107697=CARTESIAN_POINT ( 'NONE',  ( -14.34966873604960291, -8.224510206698953496, 31.66557627198102054 ) ) ;
#107698=CARTESIAN_POINT ( 'NONE',  ( 15.80617190586746368, 15.72974639402197994, 89.37390960531435269 ) ) ;
#107699=CARTESIAN_POINT ( 'NONE',  ( -21.55341960407610458, -5.719274019375992779, 21.45724293864769550 ) ) ;
#107700=CARTESIAN_POINT ( 'NONE',  ( 16.52544592524342804, -4.483927247898539470, 73.54057627198102409 ) ) ;
#107701=CARTESIAN_POINT ( 'NONE',  ( -13.97604488694527625, -13.89961937509977652, 26.87390960531434558 ) ) ;
#107702=CARTESIAN_POINT ( 'NONE',  ( -5.153800228976607833, 19.02544592524334988, 22.70942372801899012 ) ) ;
#107703=CARTESIAN_POINT ( 'NONE',  ( 4.483927247898790824, -16.52544592524335698, 105.2094237280190328 ) ) ;
#107704=CARTESIAN_POINT ( 'NONE',  ( 16.52544592524335698, 4.483927247898782831, 56.45942372801902565 ) ) ;
#107705=CARTESIAN_POINT ( 'NONE',  ( -10.81492255796078084, -18.62759615963271287, 37.08224293864768129 ) ) ;
#107706=CARTESIAN_POINT ( 'NONE',  ( 5.823673210054444382, -21.52544592524334988, 105.2094237280190328 ) ) ;
#107707=CARTESIAN_POINT ( 'NONE',  ( -16.46253265017160317, 9.564922557960807481, 85.83224293864769550 ) ) ;
#107708=CARTESIAN_POINT ( 'NONE',  ( 4.483927247898790824, -16.52544592524335698, 55.20942372801902565 ) ) ;
#107709=CARTESIAN_POINT ( 'NONE',  ( -19.05341960407611168, -5.049401038298163336, 26.45724293864769550 ) ) ;
#107710=CARTESIAN_POINT ( 'NONE',  ( -16.52544592524342804, 4.483927247898546575, 31.04057627198102409 ) ) ;
#107711=CARTESIAN_POINT ( 'NONE',  ( -9.474510206698964154, 16.51473224551069663, 110.4155762719810383 ) ) ;
#107712=CARTESIAN_POINT ( 'NONE',  ( 19.03943276465977164, -0.05219959533909143690, 93.74890960531435269 ) ) ;
#107713=CARTESIAN_POINT ( 'NONE',  ( -0.05219959533909027116, -19.03943276465977164, 112.4989096053143669 ) ) ;
#107714=CARTESIAN_POINT ( 'NONE',  ( 8.224510206698953496, -14.34966873604960469, 52.91557627198103830 ) ) ;
#107715=CARTESIAN_POINT ( 'NONE',  ( 14.29746914071049879, -8.314922557960816363, 28.33224293864769550 ) ) ;
#107717=CARTESIAN_POINT ( 'NONE',  ( 8.314922557960818139, 14.29746914071049879, 49.58224293864769550 ) ) ;
#107718=CARTESIAN_POINT ( 'NONE',  ( -16.53943276465976808, -0.05219959533934237506, 38.75109039468567573 ) ) ;
#107719=CARTESIAN_POINT ( 'NONE',  ( 17.49999999999998579, -3.471454075611618784, 31.98332581144368447 ) ) ;
#107720=CARTESIAN_POINT ( 'NONE',  ( 19.05341960407617918, -5.049401038297876454, 46.04275706135233293 ) ) ;
#107721=CARTESIAN_POINT ( 'NONE',  ( 0.05219959533909260263, 19.03943276465977164, 84.99890960531436690 ) ) ;
#107722=CARTESIAN_POINT ( 'NONE',  ( 13.97604488694548053, -13.89961937509957401, 70.62609039468567573 ) ) ;
#107724=CARTESIAN_POINT ( 'NONE',  ( 9.564922557961047289, -16.46253265017146816, 50.41775706135233293 ) ) ;
#107725=CARTESIAN_POINT ( 'NONE',  ( -13.89961937509957401, -13.97604488694547875, 99.37609039468567573 ) ) ;
#107726=CARTESIAN_POINT ( 'NONE',  ( -4.483927247898782831, 16.52544592524335698, 82.70942372801900433 ) ) ;
#107728=CARTESIAN_POINT ( 'NONE',  ( -19.03943276465977164, 0.05219959533909376836, 21.24890960531436335 ) ) ;
#107729=CARTESIAN_POINT ( 'NONE',  ( 5.823673210054125526, 21.52544592524343514, 24.79057627198103120 ) ) ;
#107730=CARTESIAN_POINT ( 'NONE',  ( -15.80617190586768217, 15.72974639402176855, 43.12609039468568284 ) ) ;
#107731=CARTESIAN_POINT ( 'NONE',  ( -16.51473224551082808, 9.474510206698731452, 108.3344237280190043 ) ) ;
#107733=CARTESIAN_POINT ( 'NONE',  ( 9.564922557960805705, 16.46253265017160317, 64.58224293864769550 ) ) ;
#107735=CARTESIAN_POINT ( 'NONE',  ( -9.564922557960796823, -16.46253265017161027, 107.0822429386476955 ) ) ;
#107736=CARTESIAN_POINT ( 'NONE',  ( -14.34966873604960291, -8.224510206698953496, 61.66557627198103120 ) ) ;
#107737=CARTESIAN_POINT ( 'NONE',  ( -5.049401038298153566, 19.05341960407611168, 60.20724293864768129 ) ) ;
#107738=CARTESIAN_POINT ( 'NONE',  ( -16.46253265017160317, 9.564922557960807481, 70.83224293864770971 ) ) ;
#107739=CARTESIAN_POINT ( 'NONE',  ( 19.03943276465977164, 0.05219959533936151252, 81.25109039468567573 ) ) ;
#107740=CARTESIAN_POINT ( 'NONE',  ( -18.62759615963270932, 10.81492255796079327, 50.83224293864770971 ) ) ;
#107741=CARTESIAN_POINT ( 'NONE',  ( -4.483927247898539470, -16.52544592524342804, 112.2905762719810241 ) ) ;
#107742=CARTESIAN_POINT ( 'NONE',  ( 13.97604488694548053, -13.89961937509957401, 45.62609039468566863 ) ) ;
#107743=CARTESIAN_POINT ( 'NONE',  ( -19.02544592524342804, 5.153800228976336051, 81.04057627198103830 ) ) ;
#107744=CARTESIAN_POINT ( 'NONE',  ( -15.80617190586745835, -15.72974639402198527, 71.87390960531438111 ) ) ;
#107745=CARTESIAN_POINT ( 'NONE',  ( -12.06949235617756955, 12.14591786802309770, 75.62390960531439532 ) ) ;
#107746=CARTESIAN_POINT ( 'NONE',  ( -19.02544592524334988, -5.153800228976617603, 28.95942372801900433 ) ) ;
#107747=CARTESIAN_POINT ( 'NONE',  ( -15.80617190586745835, -15.72974639402198527, 56.87390960531436690 ) ) ;
#107748=CARTESIAN_POINT ( 'NONE',  ( 10.81492255796078972, 18.62759615963270932, 44.58224293864769550 ) ) ;
#107749=CARTESIAN_POINT ( 'NONE',  ( 15.80617190586769283, -15.72974639402175789, 90.62609039468567573 ) ) ;
#107750=CARTESIAN_POINT ( 'NONE',  ( -13.89961937509977652, 13.97604488694528158, 60.62390960531436690 ) ) ;
#107751=CARTESIAN_POINT ( 'NONE',  ( 8.314922557960818139, 14.29746914071049879, 109.5822429386476955 ) ) ;
#107752=CARTESIAN_POINT ( 'NONE',  ( 5.719274019375673035, 21.55341960407619339, 27.29275706135234358 ) ) ;
#107754=CARTESIAN_POINT ( 'NONE',  ( 5.719274019375673035, 21.55341960407619339, 42.29275706135235424 ) ) ;
#107755=CARTESIAN_POINT ( 'NONE',  ( -19.02544592524342804, 5.153800228976336051, 41.04057627198103120 ) ) ;
#107756=CARTESIAN_POINT ( 'NONE',  ( 0.05219959533907565091, 21.53943276465977519, 109.9989096053143527 ) ) ;
#107757=CARTESIAN_POINT ( 'NONE',  ( -5.153800228976607833, 19.02544592524334988, 47.70942372801900433 ) ) ;
#107758=CARTESIAN_POINT ( 'NONE',  ( -16.51473224551069308, -9.474510206698971260, 26.66557627198103120 ) ) ;
#107759=CARTESIAN_POINT ( 'NONE',  ( 13.89961937509977652, -13.97604488694527269, 28.12390960531435624 ) ) ;
#107760=CARTESIAN_POINT ( 'NONE',  ( -4.379528057220086978, -16.55341960407618274, 54.79275706135235424 ) ) ;
#107761=CARTESIAN_POINT ( 'NONE',  ( -19.03943276465977164, 0.05219959533909376836, 26.24890960531435624 ) ) ;
#107763=CARTESIAN_POINT ( 'NONE',  ( 19.02544592524343514, -5.153800228976328945, 68.54057627198103830 ) ) ;
#107764=CARTESIAN_POINT ( 'NONE',  ( -14.29746914071049879, 8.314922557960819915, 100.8322429386477097 ) ) ;
#107765=CARTESIAN_POINT ( 'NONE',  ( 15.80617190586746368, 15.72974639402197994, 64.37390960531435269 ) ) ;
#107766=CARTESIAN_POINT ( 'NONE',  ( -16.55341960407617563, 4.379528057220093196, 38.54275706135234714 ) ) ;
#107767=CARTESIAN_POINT ( 'NONE',  ( 18.67979575497194134, -10.72451020669871369, 100.8344237280190185 ) ) ;
#107768=CARTESIAN_POINT ( 'NONE',  ( 9.474510206698971260, -16.51473224551069308, 22.91557627198102765 ) ) ;
#107769=CARTESIAN_POINT ( 'NONE',  ( 8.314922557961029526, -14.29746914071037800, 110.4177570613523756 ) ) ;
#107770=CARTESIAN_POINT ( 'NONE',  ( 0.05219959533910956823, 16.53943276465976808, 49.99890960531437401 ) ) ;
#107771=CARTESIAN_POINT ( 'NONE',  ( -13.89961937509977652, 13.97604488694528158, 55.62390960531434558 ) ) ;
#107772=CARTESIAN_POINT ( 'NONE',  ( -5.823673210054431948, 21.52544592524334988, 92.70942372801901854 ) ) ;
#107773=CARTESIAN_POINT ( 'NONE',  ( -18.67979575497178146, -10.72451020669898902, 111.6655762719810525 ) ) ;
#107775=CARTESIAN_POINT ( 'NONE',  ( -10.81492255796105439, 18.62759615963255655, 67.91775706135234714 ) ) ;
#107776=CARTESIAN_POINT ( 'NONE',  ( -14.29746914071037622, -8.314922557961029526, 54.16775706135235424 ) ) ;
#107777=CARTESIAN_POINT ( 'NONE',  ( -8.314922557960811034, -14.29746914071050412, 82.08224293864768129 ) ) ;
#107778=CARTESIAN_POINT ( 'NONE',  ( 0.05219959533937995610, -21.53943276465977519, 100.0010903946857042 ) ) ;
#107779=CARTESIAN_POINT ( 'NONE',  ( -8.314922557960811034, -14.29746914071050412, 27.08224293864769550 ) ) ;
#107780=CARTESIAN_POINT ( 'NONE',  ( -16.36317988757057051, 7.306389748694942732, 114.0978960836323068 ) ) ;
#107781=CARTESIAN_POINT ( 'NONE',  ( 4.483927247898790824, -16.52544592524335698, 40.20942372801901854 ) ) ;
#107782=CARTESIAN_POINT ( 'NONE',  ( -14.29746914071049879, 8.314922557960819915, 40.83224293864769550 ) ) ;
#107783=CARTESIAN_POINT ( 'NONE',  ( 8.224510206698742110, 14.34966873604972548, 82.08442372801901854 ) ) ;
#107784=CARTESIAN_POINT ( 'NONE',  ( -9.474510206698964154, 16.51473224551069663, 105.4155762719810383 ) ) ;
#107785=CARTESIAN_POINT ( 'NONE',  ( 19.05341960407611168, 5.049401038298154454, 113.9572429386477097 ) ) ;
#107786=CARTESIAN_POINT ( 'NONE',  ( -18.62759615963255300, -10.81492255796106328, 104.1677570613523471 ) ) ;
#107787=CARTESIAN_POINT ( 'NONE',  ( 8.224510206698742110, 14.34966873604972548, 97.08442372801904696 ) ) ;
#107788=CARTESIAN_POINT ( 'NONE',  ( 16.55341960407611168, 4.379528057220329451, 78.95724293864769550 ) ) ;
#107789=CARTESIAN_POINT ( 'NONE',  ( 16.51473224551069308, 9.474510206698969483, 79.16557627198103830 ) ) ;
#107791=CARTESIAN_POINT ( 'NONE',  ( 12.14591786802327356, -12.06949235617739191, 45.62609039468567573 ) ) ;
#107793=CARTESIAN_POINT ( 'NONE',  ( -16.51473224551069308, -9.474510206698971260, 36.66557627198102409 ) ) ;
#107794=CARTESIAN_POINT ( 'NONE',  ( -9.564922557960796823, -16.46253265017161027, 97.08224293864769550 ) ) ;
#107795=CARTESIAN_POINT ( 'NONE',  ( 16.52544592524335698, 4.483927247898782831, 31.45942372801901854 ) ) ;
#107797=CARTESIAN_POINT ( 'NONE',  ( -13.89961937509957401, -13.97604488694547875, 34.37609039468566863 ) ) ;
#107798=CARTESIAN_POINT ( 'NONE',  ( 16.53943276465976808, 0.05219959533934440121, 96.25109039468568994 ) ) ;
#107799=CARTESIAN_POINT ( 'NONE',  ( 19.02544592524343514, -5.153800228976328945, 33.54057627198102409 ) ) ;
#107800=CARTESIAN_POINT ( 'NONE',  ( -0.05219959533934338120, 16.53943276465976808, 77.50109039468567573 ) ) ;
#107801=CARTESIAN_POINT ( 'NONE',  ( -8.314922557961024197, 14.29746914071037800, 62.91775706135236135 ) ) ;
#107802=CARTESIAN_POINT ( 'NONE',  ( 9.564922557961047289, -16.46253265017146816, 80.41775706135234714 ) ) ;
#107803=CARTESIAN_POINT ( 'NONE',  ( -5.153800228976607833, 19.02544592524334988, 27.70942372801899722 ) ) ;
#107804=CARTESIAN_POINT ( 'NONE',  ( 5.153800228976335163, 19.02544592524342804, 49.79057627198100988 ) ) ;
#107805=CARTESIAN_POINT ( 'NONE',  ( -12.06949235617756955, 12.14591786802309770, 85.62390960531436690 ) ) ;
#107808=CARTESIAN_POINT ( 'NONE',  ( -19.03943276465977164, -0.05219959533935918106, 53.75109039468566863 ) ) ;
#107809=CARTESIAN_POINT ( 'NONE',  ( -21.53943276465977519, 0.05219959533907696930, 56.24890960531436690 ) ) ;
#107810=CARTESIAN_POINT ( 'NONE',  ( 13.97604488694548053, -13.89961937509957401, 30.62609039468566863 ) ) ;
#107811=CARTESIAN_POINT ( 'NONE',  ( -19.02544592524342804, 5.153800228976336051, 101.0405762719810241 ) ) ;
#107812=CARTESIAN_POINT ( 'NONE',  ( 10.81492255796078972, 18.62759615963270932, 79.58224293864769550 ) ) ;
#107813=CARTESIAN_POINT ( 'NONE',  ( 19.02544592524343514, -5.153800228976328945, 113.5405762719810241 ) ) ;
#107814=CARTESIAN_POINT ( 'NONE',  ( 16.51473224551083163, -9.474510206698727899, 100.8344237280190043 ) ) ;
#107815=CARTESIAN_POINT ( 'NONE',  ( -19.05341960407617563, 5.049401038297882671, 113.5427570613523471 ) ) ;
#107816=CARTESIAN_POINT ( 'NONE',  ( 19.05341960407611168, 5.049401038298154454, 33.95724293864769550 ) ) ;
#107817=CARTESIAN_POINT ( 'NONE',  ( 19.05341960407611168, 5.049401038298154454, 93.95724293864769550 ) ) ;
#107818=CARTESIAN_POINT ( 'NONE',  ( 15.72974639402199770, -15.80617190586745480, 78.12390960531436690 ) ) ;
#107819=CARTESIAN_POINT ( 'NONE',  ( 16.52544592524335698, 4.483927247898782831, 41.45942372801901143 ) ) ;
#107820=CARTESIAN_POINT ( 'NONE',  ( 21.55341960407619695, -5.719274019375665929, 61.04275706135234714 ) ) ;
#107821=CARTESIAN_POINT ( 'NONE',  ( 13.97604488694548053, -13.89961937509957401, 100.6260903946856615 ) ) ;
#107822=CARTESIAN_POINT ( 'NONE',  ( -18.67979575497193778, 10.72451020669871902, 108.3344237280190185 ) ) ;
#107823=CARTESIAN_POINT ( 'NONE',  ( -16.53943276465976808, -0.05219959533934237506, 108.7510903946857042 ) ) ;
#107824=CARTESIAN_POINT ( 'NONE',  ( -15.80617190586745835, -15.72974639402198527, 96.87390960531436690 ) ) ;
#107825=CARTESIAN_POINT ( 'NONE',  ( -14.29746914071049879, 8.314922557960819915, 35.83224293864768839 ) ) ;
#107826=CARTESIAN_POINT ( 'NONE',  ( -13.89961937509957401, -13.97604488694547875, 79.37609039468567573 ) ) ;
#107827=CARTESIAN_POINT ( 'NONE',  ( -15.72974639402176322, -15.80617190586768395, 54.37609039468568994 ) ) ;
#107828=CARTESIAN_POINT ( 'NONE',  ( -19.05341960407617563, 5.049401038297882671, 33.54275706135231871 ) ) ;
#107829=CARTESIAN_POINT ( 'NONE',  ( 12.14591786802309770, 12.06949235617756955, 99.37390960531436690 ) ) ;
#107830=CARTESIAN_POINT ( 'NONE',  ( -18.62759615963270932, 10.81492255796079327, 30.83224293864770260 ) ) ;
#107831=CARTESIAN_POINT ( 'NONE',  ( -8.224510206698948167, 14.34966873604960824, 40.41557627198103120 ) ) ;
#107832=CARTESIAN_POINT ( 'NONE',  ( 15.80617190586769283, -15.72974639402175789, 100.6260903946857184 ) ) ;
#107833=CARTESIAN_POINT ( 'NONE',  ( 16.52544592524335698, 4.483927247898782831, 56.45942372801902565 ) ) ;
#107834=CARTESIAN_POINT ( 'NONE',  ( -8.314922557960811034, -14.29746914071050412, 27.08224293864769550 ) ) ;
#107835=CARTESIAN_POINT ( 'NONE',  ( -10.81492255796105439, 18.62759615963255655, 57.91775706135234714 ) ) ;
#107836=CARTESIAN_POINT ( 'NONE',  ( 21.55341960407619695, -5.719274019375665929, 51.04275706135234714 ) ) ;
#107838=CARTESIAN_POINT ( 'NONE',  ( 9.474510206698971260, -16.51473224551069308, 62.91557627198102409 ) ) ;
#107839=CARTESIAN_POINT ( 'NONE',  ( 5.823673210054444382, -21.52544592524334988, 25.20942372801901854 ) ) ;
#107840=CARTESIAN_POINT ( 'NONE',  ( 16.53943276465976808, -0.05219959533910856209, 108.7489096053143669 ) ) ;
#107841=CARTESIAN_POINT ( 'NONE',  ( 16.46253265017160672, -9.564922557960803928, 28.33224293864769550 ) ) ;
#107842=CARTESIAN_POINT ( 'NONE',  ( -16.55341960407611168, -4.379528057220339221, 76.45724293864769550 ) ) ;
#107843=CARTESIAN_POINT ( 'NONE',  ( -19.03943276465977164, 0.05219959533909376836, 71.24890960531435269 ) ) ;
#107844=CARTESIAN_POINT ( 'NONE',  ( 16.52544592524342804, -4.483927247898539470, 33.54057627198102409 ) ) ;
#107845=CARTESIAN_POINT ( 'NONE',  ( 15.72974639402199770, -15.80617190586745480, 53.12390960531436690 ) ) ;
#107846=CARTESIAN_POINT ( 'NONE',  ( 16.53943276465976808, -0.05219959533910856209, 88.74890960531436690 ) ) ;
#107847=CARTESIAN_POINT ( 'NONE',  ( 5.823673210054125526, 21.52544592524343514, 109.7905762719810383 ) ) ;
#107848=CARTESIAN_POINT ( 'NONE',  ( -19.05341960407611168, -5.049401038298163336, 106.4572429386476955 ) ) ;
#107849=CARTESIAN_POINT ( 'NONE',  ( 9.474510206698971260, -16.51473224551069308, 47.91557627198102409 ) ) ;
#107850=CARTESIAN_POINT ( 'NONE',  ( -9.474510206698720793, -16.51473224551083518, 109.5844237280190043 ) ) ;
#107851=CARTESIAN_POINT ( 'NONE',  ( -15.72974639402197994, 15.80617190586746368, 60.62390960531437401 ) ) ;
#107852=CARTESIAN_POINT ( 'NONE',  ( -10.81492255796105439, 18.62759615963255655, 82.91775706135234714 ) ) ;
#107853=CARTESIAN_POINT ( 'NONE',  ( -13.97604488694527625, -13.89961937509977652, 71.87390960531433848 ) ) ;
#107855=CARTESIAN_POINT ( 'NONE',  ( -0.05219959533909027116, -19.03943276465977164, 102.4989096053143669 ) ) ;
#107856=CARTESIAN_POINT ( 'NONE',  ( 4.379528057220092307, 16.55341960407617563, 82.29275706135234714 ) ) ;
#107857=CARTESIAN_POINT ( 'NONE',  ( 21.55341960407619695, -5.719274019375665929, 61.04275706135234714 ) ) ;
#107858=CARTESIAN_POINT ( 'NONE',  ( -15.80617190586768217, 15.72974639402176855, 83.12609039468568994 ) ) ;
#107859=CARTESIAN_POINT ( 'NONE',  ( 0.05219959533907565091, 21.53943276465977519, 114.9989096053143669 ) ) ;
#107860=CARTESIAN_POINT ( 'NONE',  ( -12.14591786802326823, 12.06949235617739902, 73.12609039468567573 ) ) ;
#107861=CARTESIAN_POINT ( 'NONE',  ( -5.719274019375978568, 21.55341960407610458, 80.20724293864769550 ) ) ;
#107862=CARTESIAN_POINT ( 'NONE',  ( 5.153800228976615827, -19.02544592524334988, 50.20942372801897591 ) ) ;
#107863=CARTESIAN_POINT ( 'NONE',  ( -5.719274019375978568, 21.55341960407610458, 45.20724293864769550 ) ) ;
#107864=CARTESIAN_POINT ( 'NONE',  ( 19.02544592524343514, -5.153800228976328945, 78.54057627198099567 ) ) ;
#107865=CARTESIAN_POINT ( 'NONE',  ( -16.55341960407617563, 4.379528057220093196, 113.5427570613523756 ) ) ;
#107867=CARTESIAN_POINT ( 'NONE',  ( -19.02544592524342804, 5.153800228976336051, 111.0405762719810099 ) ) ;
#107869=CARTESIAN_POINT ( 'NONE',  ( 19.03943276465977164, 0.05219959533936151252, 96.25109039468567573 ) ) ;
#107870=CARTESIAN_POINT ( 'NONE',  ( 21.55341960407610458, 5.719274019375980345, 68.95724293864769550 ) ) ;
#107871=CARTESIAN_POINT ( 'NONE',  ( -4.483927247898539470, -16.52544592524342804, 47.29057627198103120 ) ) ;
#107872=CARTESIAN_POINT ( 'NONE',  ( -13.89961937509957401, -13.97604488694547875, 109.3760903946856331 ) ) ;
#107873=CARTESIAN_POINT ( 'NONE',  ( -16.46253265017160317, 9.564922557960807481, 25.83224293864769194 ) ) ;
#107874=CARTESIAN_POINT ( 'NONE',  ( 0.05219959533936267826, -19.03943276465977164, 105.0010903946856615 ) ) ;
#107875=CARTESIAN_POINT ( 'NONE',  ( 18.67979575497178502, 10.72451020669898547, 94.16557627198103830 ) ) ;
#107876=CARTESIAN_POINT ( 'NONE',  ( 5.049401038297881783, 19.05341960407617563, 72.29275706135234714 ) ) ;
#107877=CARTESIAN_POINT ( 'NONE',  ( 12.14591786802327356, -12.06949235617739191, 85.62609039468568994 ) ) ;
#107878=CARTESIAN_POINT ( 'NONE',  ( -0.05219959533909027116, -19.03943276465977164, 77.49890960531435269 ) ) ;
#107879=CARTESIAN_POINT ( 'NONE',  ( -0.05219959533910754901, -16.53943276465976808, 82.49890960531436690 ) ) ;
#107881=CARTESIAN_POINT ( 'NONE',  ( 13.89961937509977652, -13.97604488694527269, 63.12390960531435979 ) ) ;
#107882=CARTESIAN_POINT ( 'NONE',  ( -8.224510206698948167, 14.34966873604960824, 60.41557627198102409 ) ) ;
#107883=CARTESIAN_POINT ( 'NONE',  ( 5.049401038298161559, -19.05341960407611168, 32.70724293864768129 ) ) ;
#107885=CARTESIAN_POINT ( 'NONE',  ( -12.14591786802309592, -12.06949235617757132, 46.87390960531435979 ) ) ;
#107886=CARTESIAN_POINT ( 'NONE',  ( -9.474510206698964154, 16.51473224551069663, 75.41557627198103830 ) ) ;
#107888=CARTESIAN_POINT ( 'NONE',  ( 19.05341960407617918, -5.049401038297876454, 56.04275706135234714 ) ) ;
#107889=CARTESIAN_POINT ( 'NONE',  ( 12.14591786802327356, -12.06949235617739191, 60.62609039468567573 ) ) ;
#107890=CARTESIAN_POINT ( 'NONE',  ( -18.62759615963270932, 10.81492255796079327, 65.83224293864769550 ) ) ;
#107891=CARTESIAN_POINT ( 'NONE',  ( -19.02544592524334988, -5.153800228976617603, 23.95942372801900078 ) ) ;
#107892=CARTESIAN_POINT ( 'NONE',  ( -13.97604488694527625, -13.89961937509977652, 91.87390960531432427 ) ) ;
#107894=CARTESIAN_POINT ( 'NONE',  ( 21.53943276465977519, -0.05219959533907433946, 28.74890960531435624 ) ) ;
#107895=CARTESIAN_POINT ( 'NONE',  ( 19.03943276465977164, -0.05219959533909143690, 58.74890960531435979 ) ) ;
#107896=CARTESIAN_POINT ( 'NONE',  ( 5.823673210054444382, -21.52544592524334988, 55.20942372801902565 ) ) ;
#107897=CARTESIAN_POINT ( 'NONE',  ( -8.224510206698948167, 14.34966873604960824, 105.4155762719810383 ) ) ;
#107898=CARTESIAN_POINT ( 'NONE',  ( -5.719274019375978568, 21.55341960407610458, 100.2072429386476955 ) ) ;
#107899=CARTESIAN_POINT ( 'NONE',  ( 13.97604488694527802, 13.89961937509977652, 99.37390960531436690 ) ) ;
#107901=CARTESIAN_POINT ( 'NONE',  ( 18.67979575497194134, -10.72451020669871369, 40.83442372801901854 ) ) ;
#107903=CARTESIAN_POINT ( 'NONE',  ( -9.564922557960796823, -16.46253265017161027, 97.08224293864769550 ) ) ;
#107904=ADVANCED_FACE ( 'NONE', ( #74716 ), #26235, .T. ) ;
#107905=CARTESIAN_POINT ( 'NONE',  ( -18.22780087662123805, 5.499999999999981348, 91.01763182126894947 ) ) ;
#107906=CARTESIAN_POINT ( 'NONE',  ( -15.72974639402197994, 15.80617190586746368, 90.62390960531436690 ) ) ;
#107907=CARTESIAN_POINT ( 'NONE',  ( -19.05341960407611168, -5.049401038298163336, 41.45724293864769550 ) ) ;
#107908=CARTESIAN_POINT ( 'NONE',  ( 16.55341960407618274, -4.379528057220086978, 31.04275706135234714 ) ) ;
#107911=CARTESIAN_POINT ( 'NONE',  ( -19.03943276465977164, 0.05219959533909376836, 26.24890960531435624 ) ) ;
#107912=CARTESIAN_POINT ( 'NONE',  ( -15.80617190586768217, 15.72974639402176855, 98.12609039468570415 ) ) ;
#107913=CARTESIAN_POINT ( 'NONE',  ( 19.05341960407611168, 5.049401038298154454, 73.95724293864768129 ) ) ;
#107914=CARTESIAN_POINT ( 'NONE',  ( -10.72451020669870658, -18.67979575497194134, 49.58442372801901143 ) ) ;
#107915=CARTESIAN_POINT ( 'NONE',  ( -15.80617190586768217, 15.72974639402176855, 28.12609039468568284 ) ) ;
#107917=CARTESIAN_POINT ( 'NONE',  ( 0.05219959533909260263, 19.03943276465977164, 104.9989096053143669 ) ) ;
#107918=CARTESIAN_POINT ( 'NONE',  ( 19.39056639909673763, 5.500000000000046185, 63.28948781074346641 ) ) ;
#107919=CARTESIAN_POINT ( 'NONE',  ( 0.05219959533934541429, -16.53943276465976808, 35.00109039468568284 ) ) ;
#107920=CARTESIAN_POINT ( 'NONE',  ( -14.29746914071037622, -8.314922557961029526, 69.16775706135234714 ) ) ;
#107921=CARTESIAN_POINT ( 'NONE',  ( -15.80617190586768217, 15.72974639402176855, 63.12609039468568994 ) ) ;
#107922=CARTESIAN_POINT ( 'NONE',  ( 10.72451020669871369, 18.67979575497193778, 77.08442372801901854 ) ) ;
#107924=CARTESIAN_POINT ( 'NONE',  ( -16.51473224551082808, 9.474510206698731452, 103.3344237280190043 ) ) ;
#107925=CARTESIAN_POINT ( 'NONE',  ( -19.05341960407611168, -5.049401038298163336, 71.45724293864766707 ) ) ;
#107926=CARTESIAN_POINT ( 'NONE',  ( -0.05219959533909027116, -19.03943276465977164, 102.4989096053143669 ) ) ;
#107927=CARTESIAN_POINT ( 'NONE',  ( -14.29746914071049879, 8.314922557960819915, 105.8322429386476955 ) ) ;
#107928=CARTESIAN_POINT ( 'NONE',  ( -16.53943276465976808, 0.05219959533911058130, 101.2489096053143669 ) ) ;
#107929=CARTESIAN_POINT ( 'NONE',  ( -15.72974639402197994, 15.80617190586746368, 25.62390960531435624 ) ) ;
#107930=CARTESIAN_POINT ( 'NONE',  ( -12.06949235617739369, -12.14591786802326823, 94.37609039468568994 ) ) ;
#107931=CARTESIAN_POINT ( 'NONE',  ( -4.379528057220328563, 16.55341960407611168, 70.20724293864769550 ) ) ;
#107932=CARTESIAN_POINT ( 'NONE',  ( 9.564922557960805705, 16.46253265017160317, 54.58224293864769550 ) ) ;
#107933=CARTESIAN_POINT ( 'NONE',  ( -21.55341960407619339, 5.719274019375674811, 73.54275706135234714 ) ) ;
#107935=CARTESIAN_POINT ( 'NONE',  ( 0.05219959533936267826, -19.03943276465977164, 100.0010903946856757 ) ) ;
#107936=CARTESIAN_POINT ( 'NONE',  ( 16.52544592524342804, -4.483927247898539470, 73.54057627198102409 ) ) ;
#107937=CARTESIAN_POINT ( 'NONE',  ( -10.72451020669870658, -18.67979575497194134, 34.58442372801900433 ) ) ;
#107938=CARTESIAN_POINT ( 'NONE',  ( 0.05219959533907565091, 21.53943276465977519, 59.99890960531436690 ) ) ;
#107939=CARTESIAN_POINT ( 'NONE',  ( -17.40805194822030799, -6.112264579159321087, 104.1662872748939179 ) ) ;
#107941=CARTESIAN_POINT ( 'NONE',  ( -16.51473224551069308, -9.474510206698971260, 71.66557627198102409 ) ) ;
#107942=CARTESIAN_POINT ( 'NONE',  ( 12.06949235617757843, -12.14591786802309237, 48.12390960531436690 ) ) ;
#107944=CARTESIAN_POINT ( 'NONE',  ( 12.06949235617757843, -12.14591786802309237, 28.12390960531435979 ) ) ;
#107945=CARTESIAN_POINT ( 'NONE',  ( 8.224510206698742110, 14.34966873604972548, 92.08442372801901854 ) ) ;
#107946=CARTESIAN_POINT ( 'NONE',  ( 19.03943276465977164, 0.05219959533936151252, 46.25109039468566863 ) ) ;
#107947=CARTESIAN_POINT ( 'NONE',  ( 16.29526858892879204, 7.335722546919999587, 48.29670597800208043 ) ) ;
#107948=CARTESIAN_POINT ( 'NONE',  ( 19.03943276465977164, -0.05219959533909143690, 103.7489096053143669 ) ) ;
#107949=CARTESIAN_POINT ( 'NONE',  ( 12.06949235617757843, -12.14591786802309237, 73.12390960531436690 ) ) ;
#107950=CARTESIAN_POINT ( 'NONE',  ( 19.05341960407617918, -5.049401038297876454, 46.04275706135233293 ) ) ;
#107951=CARTESIAN_POINT ( 'NONE',  ( 5.049401038298161559, -19.05341960407611168, 32.70724293864768129 ) ) ;
#107952=CARTESIAN_POINT ( 'NONE',  ( 5.719274019375991003, -21.55341960407610458, 37.70724293864769550 ) ) ;
#107953=CARTESIAN_POINT ( 'NONE',  ( -15.72974639402197994, 15.80617190586746368, 70.62390960531436690 ) ) ;
#107955=CARTESIAN_POINT ( 'NONE',  ( 16.53943276465976808, -0.05219959533910856209, 93.74890960531436690 ) ) ;
#107956=CARTESIAN_POINT ( 'NONE',  ( 8.224510206698742110, 14.34966873604972548, 47.08442372801901854 ) ) ;
#107957=CARTESIAN_POINT ( 'NONE',  ( -14.34966873604960291, -8.224510206698953496, 96.66557627198102409 ) ) ;
#107958=CARTESIAN_POINT ( 'NONE',  ( 17.48853670773243252, -5.747243402303151782, 36.16671299749992130 ) ) ;
#107959=CARTESIAN_POINT ( 'NONE',  ( -16.61371651742604882, 7.165104196376025136, 48.85415069992998127 ) ) ;
#107960=CARTESIAN_POINT ( 'NONE',  ( 0.05219959533907565091, 21.53943276465977519, 34.99890960531435979 ) ) ;
#107963=CARTESIAN_POINT ( 'NONE',  ( -4.483927247898782831, 16.52544592524335698, 47.70942372801902565 ) ) ;
#107964=CARTESIAN_POINT ( 'NONE',  ( 16.55341960407611168, 4.379528057220329451, 33.95724293864769550 ) ) ;
#107965=CARTESIAN_POINT ( 'NONE',  ( 18.62759615963271287, -10.81492255796078972, 53.33224293864769550 ) ) ;
#107966=CARTESIAN_POINT ( 'NONE',  ( -5.049401038297874678, -19.05341960407617918, 79.79275706135233293 ) ) ;
#107967=CARTESIAN_POINT ( 'NONE',  ( 0.05219959533907565091, 21.53943276465977519, 59.99890960531436690 ) ) ;
#107968=CARTESIAN_POINT ( 'NONE',  ( 18.62759615963255655, 10.81492255796105972, 76.66775706135234714 ) ) ;
#107970=CARTESIAN_POINT ( 'NONE',  ( -14.34966873604972548, 8.224510206698743886, 43.33442372801901143 ) ) ;
#107971=CARTESIAN_POINT ( 'NONE',  ( -5.153800228976328057, -19.02544592524343514, 32.29057627198102409 ) ) ;
#107972=CARTESIAN_POINT ( 'NONE',  ( -9.564922557960796823, -16.46253265017161027, 97.08224293864769550 ) ) ;
#107973=CARTESIAN_POINT ( 'NONE',  ( 19.02544592524343514, -5.153800228976328945, 33.54057627198102409 ) ) ;
#107974=CARTESIAN_POINT ( 'NONE',  ( 4.379528057220339221, -16.55341960407611168, 97.70724293864772392 ) ) ;
#107976=FACE_BOUND ( 'NONE', #73425, .T. ) ;
#107977=CARTESIAN_POINT ( 'NONE',  ( -14.29746914071037622, -8.314922557961029526, 74.16775706135231871 ) ) ;
#107978=CARTESIAN_POINT ( 'NONE',  ( -18.67979575497178146, -10.72451020669898902, 86.66557627198102409 ) ) ;
#107979=CARTESIAN_POINT ( 'NONE',  ( -5.153800228976328057, -19.02544592524343514, 62.29057627198100988 ) ) ;
#107980=CARTESIAN_POINT ( 'NONE',  ( -21.52544592524334988, -5.823673210054445271, 28.95942372801902209 ) ) ;
#107981=CARTESIAN_POINT ( 'NONE',  ( -19.03943276465977164, 0.05219959533909376836, 86.24890960531436690 ) ) ;
#107984=CARTESIAN_POINT ( 'NONE',  ( 5.823673210054125526, 21.52544592524343514, 114.7905762719810383 ) ) ;
#107985=CARTESIAN_POINT ( 'NONE',  ( -19.05341960407611168, -5.049401038298163336, 31.45724293864769550 ) ) ;
#107986=CARTESIAN_POINT ( 'NONE',  ( -5.049401038298153566, 19.05341960407611168, 105.2072429386476671 ) ) ;
#107987=CARTESIAN_POINT ( 'NONE',  ( -19.05341960407617563, 5.049401038297882671, 73.54275706135233293 ) ) ;
#107989=CARTESIAN_POINT ( 'NONE',  ( 9.564922557961047289, -16.46253265017146816, 25.41775706135234003 ) ) ;
#107990=CARTESIAN_POINT ( 'NONE',  ( 0.05219959533907565091, 21.53943276465977519, 94.99890960531436690 ) ) ;
#107991=CARTESIAN_POINT ( 'NONE',  ( 16.51473224551083163, -9.474510206698727899, 35.83442372801899722 ) ) ;
#107992=CARTESIAN_POINT ( 'NONE',  ( -8.314922557961024197, 14.29746914071037800, 82.91775706135234714 ) ) ;
#107993=CARTESIAN_POINT ( 'NONE',  ( 0.05219959533909260263, 19.03943276465977164, 109.9989096053143669 ) ) ;
#107994=CARTESIAN_POINT ( 'NONE',  ( 0.05219959533909260263, 19.03943276465977164, 59.99890960531436690 ) ) ;
#107995=CARTESIAN_POINT ( 'NONE',  ( 15.80617190586769283, -15.72974639402175789, 60.62609039468567573 ) ) ;
#107996=CARTESIAN_POINT ( 'NONE',  ( -15.72974639402176322, -15.80617190586768395, 79.37609039468567573 ) ) ;
#107997=CARTESIAN_POINT ( 'NONE',  ( -0.05219959533909027116, -19.03943276465977164, 77.49890960531435269 ) ) ;
#107998=CARTESIAN_POINT ( 'NONE',  ( -10.81492255796105439, 18.62759615963255655, 42.91775706135235424 ) ) ;
#107999=CARTESIAN_POINT ( 'NONE',  ( -19.02544592524334988, -5.153800228976617603, 83.95942372801901854 ) ) ;
#108001=CARTESIAN_POINT ( 'NONE',  ( 19.05341960407611168, 5.049401038298154454, 58.95724293864768129 ) ) ;
#108002=CARTESIAN_POINT ( 'NONE',  ( -0.05219959533909027116, -19.03943276465977164, 92.49890960531436690 ) ) ;
#108003=CARTESIAN_POINT ( 'NONE',  ( 19.05341960407611168, 5.049401038298154454, 63.95724293864769550 ) ) ;
#108004=CARTESIAN_POINT ( 'NONE',  ( -5.153800228976328057, -19.02544592524343514, 77.29057627198100988 ) ) ;
#108005=CARTESIAN_POINT ( 'NONE',  ( 9.474510206698971260, -16.51473224551069308, 57.91557627198103120 ) ) ;
#108007=CARTESIAN_POINT ( 'NONE',  ( 18.62759615963271287, -10.81492255796078972, 98.33224293864769550 ) ) ;
#108008=CARTESIAN_POINT ( 'NONE',  ( -16.52544592524335698, -4.483927247898792601, 83.95942372801900433 ) ) ;
#108010=CARTESIAN_POINT ( 'NONE',  ( 16.46253265017146816, 9.564922557961045513, 41.66775706135234003 ) ) ;
#108011=CARTESIAN_POINT ( 'NONE',  ( 0.05219959533909260263, 19.03943276465977164, 69.99890960531435269 ) ) ;
#108012=CARTESIAN_POINT ( 'NONE',  ( -16.52544592524342804, 4.483927247898546575, 56.04057627198102409 ) ) ;
#108013=CARTESIAN_POINT ( 'NONE',  ( 16.55341960407611168, 4.379528057220329451, 98.95724293864770971 ) ) ;
#108014=CARTESIAN_POINT ( 'NONE',  ( -5.153800228976328057, -19.02544592524343514, 112.2905762719810099 ) ) ;
#108015=CARTESIAN_POINT ( 'NONE',  ( -13.97604488694527625, -13.89961937509977652, 96.87390960531433848 ) ) ;
#108016=CARTESIAN_POINT ( 'NONE',  ( -16.46253265017160317, 9.564922557960807481, 110.8322429386476955 ) ) ;
#108017=CARTESIAN_POINT ( 'NONE',  ( -5.153800228976607833, 19.02544592524334988, 22.70942372801899012 ) ) ;
#108018=CARTESIAN_POINT ( 'NONE',  ( -16.55341960407617563, 4.379528057220093196, 93.54275706135234714 ) ) ;
#108019=CARTESIAN_POINT ( 'NONE',  ( -19.05341960407611168, -5.049401038298163336, 71.45724293864766707 ) ) ;
#108020=CARTESIAN_POINT ( 'NONE',  ( -21.52544592524334988, -5.823673210054445271, 33.95942372801901143 ) ) ;
#108021=CARTESIAN_POINT ( 'NONE',  ( -5.719274019375978568, 21.55341960407610458, 30.20724293864769550 ) ) ;
#108022=CARTESIAN_POINT ( 'NONE',  ( -18.62759615963255300, -10.81492255796106328, 24.16775706135235424 ) ) ;
#108023=CARTESIAN_POINT ( 'NONE',  ( -14.29746914071049879, 8.314922557960819915, 65.83224293864769550 ) ) ;
#108024=CARTESIAN_POINT ( 'NONE',  ( -16.46253265017160317, 9.564922557960807481, 60.83224293864769550 ) ) ;
#108025=CARTESIAN_POINT ( 'NONE',  ( 4.379528057220339221, -16.55341960407611168, 77.70724293864770971 ) ) ;
#108026=CARTESIAN_POINT ( 'NONE',  ( -19.03943276465977164, -0.05219959533935918106, 48.75109039468566863 ) ) ;
#108028=CARTESIAN_POINT ( 'NONE',  ( 13.89961937509977652, -13.97604488694527269, 23.12390960531436335 ) ) ;
#108029=CARTESIAN_POINT ( 'NONE',  ( -19.05341960407611168, -5.049401038298163336, 81.45724293864769550 ) ) ;
#108030=CARTESIAN_POINT ( 'NONE',  ( 5.153800228976335163, 19.02544592524342804, 79.79057627198102409 ) ) ;
#108032=CARTESIAN_POINT ( 'NONE',  ( -16.53943276465976808, 0.05219959533911058130, 106.2489096053143811 ) ) ;
#108033=ORIENTED_EDGE ( 'NONE', *, *, #60120, .T. ) ;
#108034=CARTESIAN_POINT ( 'NONE',  ( 8.224510206698742110, 14.34966873604972548, 102.0844237280190185 ) ) ;
#108035=CARTESIAN_POINT ( 'NONE',  ( 8.314922557961029526, -14.29746914071037800, 25.41775706135235779 ) ) ;
#108036=CARTESIAN_POINT ( 'NONE',  ( -18.67979575497193778, 10.72451020669871902, 98.33442372801901854 ) ) ;
#108037=CARTESIAN_POINT ( 'NONE',  ( 0.05219959533909260263, 19.03943276465977164, 99.99890960531436690 ) ) ;
#108038=CARTESIAN_POINT ( 'NONE',  ( 10.81492255796106328, -18.62759615963255655, 25.41775706135235779 ) ) ;
#108039=CARTESIAN_POINT ( 'NONE',  ( -13.97604488694527625, -13.89961937509977652, 26.87390960531434558 ) ) ;
#108040=CARTESIAN_POINT ( 'NONE',  ( -0.05219959533934338120, 16.53943276465976808, 32.50109039468568284 ) ) ;
#108042=CARTESIAN_POINT ( 'NONE',  ( 13.89961937509957401, 13.97604488694547697, 96.87609039468566152 ) ) ;
#108043=CARTESIAN_POINT ( 'NONE',  ( -18.62759615963270932, 10.81492255796079327, 90.83224293864769550 ) ) ;
#108044=CARTESIAN_POINT ( 'NONE',  ( -13.97604488694547697, 13.89961937509957934, 63.12609039468566152 ) ) ;
#108045=CARTESIAN_POINT ( 'NONE',  ( -17.49999999999999645, -5.499999999999992895, 64.20309617465829888 ) ) ;
#108046=CARTESIAN_POINT ( 'NONE',  ( 21.55341960407619695, -5.719274019375665929, 21.04275706135234714 ) ) ;
#108048=CARTESIAN_POINT ( 'NONE',  ( -16.46253265017160317, 9.564922557960807481, 95.83224293864769550 ) ) ;
#108049=CARTESIAN_POINT ( 'NONE',  ( 14.29746914071037800, 8.314922557961029526, 46.66775706135234714 ) ) ;
#108051=CARTESIAN_POINT ( 'NONE',  ( 19.03943276465977164, 0.05219959533936151252, 56.25109039468566863 ) ) ;
#108052=CARTESIAN_POINT ( 'NONE',  ( -18.62759615963270932, 10.81492255796079327, 110.8322429386476955 ) ) ;
#108053=CARTESIAN_POINT ( 'NONE',  ( 4.483927247898545687, 16.52544592524342804, 79.79057627198102409 ) ) ;
#108054=CARTESIAN_POINT ( 'NONE',  ( -19.05341960407611168, -5.049401038298163336, 86.45724293864769550 ) ) ;
#108056=CARTESIAN_POINT ( 'NONE',  ( -16.53943276465976808, -0.05219959533934237506, 48.75109039468568284 ) ) ;
#108057=CARTESIAN_POINT ( 'NONE',  ( 19.02544592524334988, 5.153800228976608722, 61.45942372801900433 ) ) ;
#108058=CARTESIAN_POINT ( 'NONE',  ( -5.823673210054431948, 21.52544592524334988, 62.70942372801902565 ) ) ;
#108059=CARTESIAN_POINT ( 'NONE',  ( 4.379528057220092307, 16.55341960407617563, 27.29275706135234358 ) ) ;
#108060=CARTESIAN_POINT ( 'NONE',  ( 19.05341960407611168, 5.049401038298154454, 68.95724293864769550 ) ) ;
#108061=CARTESIAN_POINT ( 'NONE',  ( -16.46253265017146816, -9.564922557961047289, 99.16775706135233293 ) ) ;
#108062=CARTESIAN_POINT ( 'NONE',  ( -16.55341960407617563, 4.379528057220093196, 58.54275706135235424 ) ) ;
#108063=CARTESIAN_POINT ( 'NONE',  ( -10.81492255796105439, 18.62759615963255655, 97.91775706135236135 ) ) ;
#108064=CARTESIAN_POINT ( 'NONE',  ( 13.89961937509957401, 13.97604488694547697, 76.87609039468566152 ) ) ;
#108065=CARTESIAN_POINT ( 'NONE',  ( -5.049401038298153566, 19.05341960407611168, 55.20724293864769550 ) ) ;
#108066=CARTESIAN_POINT ( 'NONE',  ( -10.81492255796078084, -18.62759615963271287, 67.08224293864770971 ) ) ;
#108067=CARTESIAN_POINT ( 'NONE',  ( 12.14591786802309770, 12.06949235617756955, 79.37390960531436690 ) ) ;
#108068=CARTESIAN_POINT ( 'NONE',  ( 19.05341960407617918, -5.049401038297876454, 76.04275706135230450 ) ) ;
#108069=CARTESIAN_POINT ( 'NONE',  ( 17.40861289038999971, -6.110651285853406556, 61.12767529172568715 ) ) ;
#108070=CARTESIAN_POINT ( 'NONE',  ( 9.564922557961047289, -16.46253265017146816, 40.41775706135234003 ) ) ;
#108071=CARTESIAN_POINT ( 'NONE',  ( 4.379528057220092307, 16.55341960407617563, 107.2927570613523471 ) ) ;
#108072=CARTESIAN_POINT ( 'NONE',  ( 8.224510206698953496, -14.34966873604960469, 72.91557627198103830 ) ) ;
#108073=CARTESIAN_POINT ( 'NONE',  ( -15.72974639402176322, -15.80617190586768395, 99.37609039468568994 ) ) ;
#108075=CARTESIAN_POINT ( 'NONE',  ( 5.823673210054125526, 21.52544592524343514, 104.7905762719810241 ) ) ;
#108076=CARTESIAN_POINT ( 'NONE',  ( 9.564922557960805705, 16.46253265017160317, 59.58224293864769550 ) ) ;
#108077=CARTESIAN_POINT ( 'NONE',  ( 10.81492255796106328, -18.62759615963255655, 80.41775706135234714 ) ) ;
#108078=CARTESIAN_POINT ( 'NONE',  ( 13.97604488694527802, 13.89961937509977652, 64.37390960531436690 ) ) ;
#108080=CARTESIAN_POINT ( 'NONE',  ( 13.89961937509977652, -13.97604488694527269, 28.12390960531435624 ) ) ;
#108081=CARTESIAN_POINT ( 'NONE',  ( 19.05341960407611168, 5.049401038298154454, 113.9572429386477097 ) ) ;
#108082=CARTESIAN_POINT ( 'NONE',  ( -14.34966873604960291, -8.224510206698953496, 66.66557627198102409 ) ) ;
#108083=CARTESIAN_POINT ( 'NONE',  ( -16.51473224551069308, -9.474510206698971260, 31.66557627198102054 ) ) ;
#108084=CARTESIAN_POINT ( 'NONE',  ( 8.314922557960818139, 14.29746914071049879, 89.58224293864768129 ) ) ;
#108086=CARTESIAN_POINT ( 'NONE',  ( -5.823673210054116645, -21.52544592524344225, 92.29057627198103830 ) ) ;
#108087=CARTESIAN_POINT ( 'NONE',  ( -21.55341960407619339, 5.719274019375674811, 43.54275706135235424 ) ) ;
#108089=CARTESIAN_POINT ( 'NONE',  ( 4.379528057220092307, 16.55341960407617563, 52.29275706135236135 ) ) ;
#108090=CARTESIAN_POINT ( 'NONE',  ( -21.53943276465977519, 0.05219959533907696930, 96.24890960531435269 ) ) ;
#108091=CARTESIAN_POINT ( 'NONE',  ( -13.97604488694547697, 13.89961937509957934, 23.12609039468565442 ) ) ;
#108092=CARTESIAN_POINT ( 'NONE',  ( 5.049401038298161559, -19.05341960407611168, 107.7072429386476955 ) ) ;
#108093=CARTESIAN_POINT ( 'NONE',  ( 10.72451020669871369, 18.67979575497193778, 42.08442372801901854 ) ) ;
#108094=CARTESIAN_POINT ( 'NONE',  ( 18.62759615963271287, -10.81492255796078972, 48.33224293864770260 ) ) ;
#108095=CARTESIAN_POINT ( 'NONE',  ( -14.29746914071049879, 8.314922557960819915, 30.83224293864770260 ) ) ;
#108096=CARTESIAN_POINT ( 'NONE',  ( -5.719274019375665041, -21.55341960407619695, 64.79275706135234714 ) ) ;
#108097=CARTESIAN_POINT ( 'NONE',  ( -0.05219959533937732626, 21.53943276465977519, 102.5010903946856899 ) ) ;
#108098=CARTESIAN_POINT ( 'NONE',  ( -5.049401038297874678, -19.05341960407617918, 29.79275706135232227 ) ) ;
#108099=CARTESIAN_POINT ( 'NONE',  ( -8.314922557961024197, 14.29746914071037800, 82.91775706135234714 ) ) ;
#108100=CARTESIAN_POINT ( 'NONE',  ( 21.53943276465977519, 0.05219959533937863772, 56.25109039468568284 ) ) ;
#108102=CARTESIAN_POINT ( 'NONE',  ( -16.51473224551069308, -9.474510206698971260, 41.66557627198103120 ) ) ;
#108103=CARTESIAN_POINT ( 'NONE',  ( 19.05341960407617918, -5.049401038297876454, 21.04275706135232582 ) ) ;
#108104=CARTESIAN_POINT ( 'NONE',  ( 18.67979575497178502, 10.72451020669898547, 29.16557627198103120 ) ) ;
#108105=CARTESIAN_POINT ( 'NONE',  ( 15.80617190586746368, 15.72974639402197994, 114.3739096053143527 ) ) ;
#108106=CARTESIAN_POINT ( 'NONE',  ( 5.719274019375991003, -21.55341960407610458, 77.70724293864770971 ) ) ;
#108107=CARTESIAN_POINT ( 'NONE',  ( -14.29746914071037622, -8.314922557961029526, 39.16775706135235424 ) ) ;
#108109=CARTESIAN_POINT ( 'NONE',  ( 15.80617190586746368, 15.72974639402197994, 74.37390960531436690 ) ) ;
#108110=CARTESIAN_POINT ( 'NONE',  ( 16.53943276465976808, 0.05219959533934440121, 71.25109039468568994 ) ) ;
#108111=CARTESIAN_POINT ( 'NONE',  ( 8.314922557960818139, 14.29746914071049879, 64.58224293864769550 ) ) ;
#108113=CARTESIAN_POINT ( 'NONE',  ( -19.05341960407617563, 5.049401038297882671, 103.5427570613523329 ) ) ;
#108114=CARTESIAN_POINT ( 'NONE',  ( -0.05219959533909027116, -19.03943276465977164, 112.4989096053143669 ) ) ;
#108115=CARTESIAN_POINT ( 'NONE',  ( 18.22780087662122384, 5.500000000000018652, 93.98459894673892734 ) ) ;
#108117=CARTESIAN_POINT ( 'NONE',  ( -8.314922557961024197, 14.29746914071037800, 42.91775706135235424 ) ) ;
#108118=CARTESIAN_POINT ( 'NONE',  ( -5.719274019375978568, 21.55341960407610458, 110.2072429386477239 ) ) ;
#108119=CARTESIAN_POINT ( 'NONE',  ( -21.53943276465977519, 0.05219959533907696930, 26.24890960531435624 ) ) ;
#108120=CARTESIAN_POINT ( 'NONE',  ( -14.34966873604972548, 8.224510206698743886, 58.33442372801901143 ) ) ;
#108121=CARTESIAN_POINT ( 'NONE',  ( 9.474510206698971260, -16.51473224551069308, 67.91557627198102409 ) ) ;
#108122=CARTESIAN_POINT ( 'NONE',  ( -0.05219959533937732626, 21.53943276465977519, 47.50109039468568994 ) ) ;
#108123=CARTESIAN_POINT ( 'NONE',  ( 4.379528057220092307, 16.55341960407617563, 22.29275706135235069 ) ) ;
#108124=CARTESIAN_POINT ( 'NONE',  ( 10.81492255796078972, 18.62759615963270932, 24.58224293864768839 ) ) ;
#108126=CARTESIAN_POINT ( 'NONE',  ( 16.46253265017146816, 9.564922557961045513, 21.66775706135233648 ) ) ;
#108127=CARTESIAN_POINT ( 'NONE',  ( 14.29746914071037800, 8.314922557961029526, 36.66775706135234714 ) ) ;
#108128=CARTESIAN_POINT ( 'NONE',  ( -5.153800228976328057, -19.02544592524343514, 107.2905762719810383 ) ) ;
#108129=CARTESIAN_POINT ( 'NONE',  ( -0.05219959533907301413, -21.53943276465977519, 97.49890960531436690 ) ) ;
#108130=CARTESIAN_POINT ( 'NONE',  ( 19.03943276465977164, -0.05219959533909143690, 68.74890960531436690 ) ) ;
#108132=CARTESIAN_POINT ( 'NONE',  ( 14.29746914071049879, -8.314922557960816363, 88.33224293864769550 ) ) ;
#108133=CARTESIAN_POINT ( 'NONE',  ( -21.52544592524343514, 5.823673210054127303, 41.04057627198103120 ) ) ;
#108134=CARTESIAN_POINT ( 'NONE',  ( 5.049401038298161559, -19.05341960407611168, 22.70724293864769194 ) ) ;
#108135=CARTESIAN_POINT ( 'NONE',  ( 12.14591786802327356, -12.06949235617739191, 60.62609039468567573 ) ) ;
#108136=CARTESIAN_POINT ( 'NONE',  ( -5.719274019375978568, 21.55341960407610458, 105.2072429386477097 ) ) ;
#108137=CARTESIAN_POINT ( 'NONE',  ( 19.03943276465977164, 0.05219959533936151252, 66.25109039468567573 ) ) ;
#108138=CARTESIAN_POINT ( 'NONE',  ( -15.80617190586745835, -15.72974639402198527, 31.87390960531435979 ) ) ;
#108139=CARTESIAN_POINT ( 'NONE',  ( -9.474510206698964154, 16.51473224551069663, 25.41557627198103120 ) ) ;
#108140=CARTESIAN_POINT ( 'NONE',  ( -18.62759615963270932, 10.81492255796079327, 70.83224293864770971 ) ) ;
#108141=CARTESIAN_POINT ( 'NONE',  ( 13.97604488694527802, 13.89961937509977652, 94.37390960531436690 ) ) ;
#108142=CARTESIAN_POINT ( 'NONE',  ( 10.72451020669871369, 18.67979575497193778, 97.08442372801904696 ) ) ;
#108143=CARTESIAN_POINT ( 'NONE',  ( -13.97604488694527625, -13.89961937509977652, 56.87390960531434558 ) ) ;
#108144=CARTESIAN_POINT ( 'NONE',  ( 8.314922557961029526, -14.29746914071037800, 35.41775706135234003 ) ) ;
#108145=CARTESIAN_POINT ( 'NONE',  ( -9.564922557960796823, -16.46253265017161027, 62.08224293864769550 ) ) ;
#108146=CARTESIAN_POINT ( 'NONE',  ( -21.53943276465977519, -0.05219959533937600094, 83.75109039468568994 ) ) ;
#108148=CARTESIAN_POINT ( 'NONE',  ( -16.51473224551082808, 9.474510206698731452, 33.33442372801899722 ) ) ;
#108150=VECTOR ( 'NONE', #80894, 1000.000000000000000 ) ;
#108151=CARTESIAN_POINT ( 'NONE',  ( -0.05219959533936034679, 19.03943276465977164, 37.50109039468567573 ) ) ;
#108152=CARTESIAN_POINT ( 'NONE',  ( -10.81492255796105439, 18.62759615963255655, 32.91775706135234714 ) ) ;
#108154=CARTESIAN_POINT ( 'NONE',  ( 16.46253265017146816, 9.564922557961045513, 26.66775706135234003 ) ) ;
#108155=CARTESIAN_POINT ( 'NONE',  ( -9.564922557960796823, -16.46253265017161027, 92.08224293864769550 ) ) ;
#108156=CARTESIAN_POINT ( 'NONE',  ( 0.05219959533909260263, 19.03943276465977164, 64.99890960531436690 ) ) ;
#108157=CARTESIAN_POINT ( 'NONE',  ( 16.52544592524335698, 4.483927247898782831, 111.4594237280190328 ) ) ;
#108158=CARTESIAN_POINT ( 'NONE',  ( -18.67979575497178146, -10.72451020669898902, 21.66557627198102409 ) ) ;
#108159=CARTESIAN_POINT ( 'NONE',  ( 18.62759615963255655, 10.81492255796105972, 86.66775706135234714 ) ) ;
#108162=CARTESIAN_POINT ( 'NONE',  ( -15.80617190586768217, 15.72974639402176855, 103.1260903946856757 ) ) ;
#108164=CARTESIAN_POINT ( 'NONE',  ( 14.29746914071049879, -8.314922557960816363, 113.3322429386476955 ) ) ;
#108165=CARTESIAN_POINT ( 'NONE',  ( 9.564922557960805705, 16.46253265017160317, 114.5822429386476955 ) ) ;
#108168=CARTESIAN_POINT ( 'NONE',  ( -4.379528057220086978, -16.55341960407618274, 49.79275706135234714 ) ) ;
#108169=CARTESIAN_POINT ( 'NONE',  ( -10.81492255796078084, -18.62759615963271287, 67.08224293864770971 ) ) ;
#108170=CARTESIAN_POINT ( 'NONE',  ( -14.34966873604960291, -8.224510206698953496, 36.66557627198103120 ) ) ;
#108171=CARTESIAN_POINT ( 'NONE',  ( 16.55341960407611168, 4.379528057220329451, 103.9572429386476813 ) ) ;
#108172=CARTESIAN_POINT ( 'NONE',  ( -19.02544592524342804, 5.153800228976336051, 91.04057627198100988 ) ) ;
#108173=CARTESIAN_POINT ( 'NONE',  ( -5.049401038297874678, -19.05341960407617918, 24.79275706135233648 ) ) ;
#108174=CARTESIAN_POINT ( 'NONE',  ( -4.379528057220328563, 16.55341960407611168, 115.2072429386476955 ) ) ;
#108175=CARTESIAN_POINT ( 'NONE',  ( -5.719274019375665041, -21.55341960407619695, 74.79275706135234714 ) ) ;
#108176=CARTESIAN_POINT ( 'NONE',  ( -19.05341960407611168, -5.049401038298163336, 111.4572429386476671 ) ) ;
#108177=CARTESIAN_POINT ( 'NONE',  ( 16.55341960407618274, -4.379528057220086978, 101.0427570613523756 ) ) ;
#108178=CARTESIAN_POINT ( 'NONE',  ( -13.97604488694547697, 13.89961937509957934, 68.12609039468563310 ) ) ;
#108180=CARTESIAN_POINT ( 'NONE',  ( -21.53943276465977519, 0.05219959533907696930, 21.24890960531436690 ) ) ;
#108181=CARTESIAN_POINT ( 'NONE',  ( -8.314922557960811034, -14.29746914071050412, 92.08224293864769550 ) ) ;
#108182=( GEOMETRIC_REPRESENTATION_CONTEXT ( 3 ) GLOBAL_UNCERTAINTY_ASSIGNED_CONTEXT ( ( #21632 ) ) GLOBAL_UNIT_ASSIGNED_CONTEXT ( ( #176802, #130253, #112123 ) ) REPRESENTATION_CONTEXT ( 'NONE', 'WORKASPACE' ) );
#108183=CARTESIAN_POINT ( 'NONE',  ( -19.05341960407617563, 5.049401038297882671, 63.54275706135234003 ) ) ;
#108184=CARTESIAN_POINT ( 'NONE',  ( -19.02544592524342804, 5.153800228976336051, 71.04057627198099567 ) ) ;
#108185=CARTESIAN_POINT ( 'NONE',  ( -14.34966873604960291, -8.224510206698953496, 81.66557627198103830 ) ) ;
#108186=CARTESIAN_POINT ( 'NONE',  ( 5.049401038297881783, 19.05341960407617563, 92.29275706135234714 ) ) ;
#108187=CARTESIAN_POINT ( 'NONE',  ( 0.05219959533907565091, 21.53943276465977519, 49.99890960531437401 ) ) ;
#108189=CARTESIAN_POINT ( 'NONE',  ( 4.379528057220339221, -16.55341960407611168, 112.7072429386476955 ) ) ;
#108191=CARTESIAN_POINT ( 'NONE',  ( -13.89961937509977652, 13.97604488694528158, 75.62390960531438111 ) ) ;
#108192=CARTESIAN_POINT ( 'NONE',  ( 18.67979575497178502, 10.72451020669898547, 74.16557627198102409 ) ) ;
#108193=CARTESIAN_POINT ( 'NONE',  ( -8.224510206698735004, -14.34966873604973081, 89.58442372801901854 ) ) ;
#108194=CARTESIAN_POINT ( 'NONE',  ( 13.97604488694527802, 13.89961937509977652, 69.37390960531436690 ) ) ;
#108195=CARTESIAN_POINT ( 'NONE',  ( 0.05219959533936267826, -19.03943276465977164, 65.00109039468567573 ) ) ;
#108196=CARTESIAN_POINT ( 'NONE',  ( -10.81492255796105439, 18.62759615963255655, 77.91775706135231871 ) ) ;
#108197=CARTESIAN_POINT ( 'NONE',  ( -10.81492255796078084, -18.62759615963271287, 67.08224293864770971 ) ) ;
#108198=CARTESIAN_POINT ( 'NONE',  ( 10.81492255796078972, 18.62759615963270932, 29.58224293864769905 ) ) ;
#108200=CARTESIAN_POINT ( 'NONE',  ( -13.97604488694527625, -13.89961937509977652, 36.87390960531436690 ) ) ;
#108201=CARTESIAN_POINT ( 'NONE',  ( -12.14591786802326823, 12.06949235617739902, 103.1260903946856757 ) ) ;
#108202=CARTESIAN_POINT ( 'NONE',  ( -5.049401038298153566, 19.05341960407611168, 55.20724293864769550 ) ) ;
#108203=CARTESIAN_POINT ( 'NONE',  ( -0.05219959533934338120, 16.53943276465976808, 22.50109039468567573 ) ) ;
#108204=CARTESIAN_POINT ( 'NONE',  ( 16.18388926212240975, 7.379444403734405356, 52.93953151366151388 ) ) ;
#108205=CARTESIAN_POINT ( 'NONE',  ( 15.80617190586769283, -15.72974639402175789, 105.6260903946856899 ) ) ;
#108207=CARTESIAN_POINT ( 'NONE',  ( 4.483927247898545687, 16.52544592524342804, 64.79057627198103830 ) ) ;
#108209=CARTESIAN_POINT ( 'NONE',  ( -0.05219959533907301413, -21.53943276465977519, 112.4989096053143669 ) ) ;
#108210=CARTESIAN_POINT ( 'NONE',  ( -10.72451020669898014, 18.67979575497178502, 105.4155762719810383 ) ) ;
#108212=CARTESIAN_POINT ( 'NONE',  ( 5.719274019375991003, -21.55341960407610458, 42.70724293864770260 ) ) ;
#108213=CARTESIAN_POINT ( 'NONE',  ( 12.14591786802327356, -12.06949235617739191, 80.62609039468567573 ) ) ;
#108214=CARTESIAN_POINT ( 'NONE',  ( -16.55341960407611168, -4.379528057220339221, 86.45724293864770971 ) ) ;
#108215=CARTESIAN_POINT ( 'NONE',  ( -5.049401038298153566, 19.05341960407611168, 55.20724293864769550 ) ) ;
#108217=CARTESIAN_POINT ( 'NONE',  ( -8.224510206698735004, -14.34966873604973081, 104.5844237280190185 ) ) ;
#108218=CARTESIAN_POINT ( 'NONE',  ( -21.52544592524334988, -5.823673210054445271, 28.95942372801902209 ) ) ;
#108219=CARTESIAN_POINT ( 'NONE',  ( 13.97604488694527802, 13.89961937509977652, 94.37390960531436690 ) ) ;
#108220=CARTESIAN_POINT ( 'NONE',  ( -21.55341960407619339, 5.719274019375674811, 63.54275706135234003 ) ) ;
#108222=CARTESIAN_POINT ( 'NONE',  ( -19.05341960407611168, -5.049401038298163336, 26.45724293864769550 ) ) ;
#108224=CARTESIAN_POINT ( 'NONE',  ( 0.05219959533937995610, -21.53943276465977519, 65.00109039468568994 ) ) ;
#108225=CARTESIAN_POINT ( 'NONE',  ( -16.51473224551069308, -9.474510206698971260, 46.66557627198102409 ) ) ;
#108226=CARTESIAN_POINT ( 'NONE',  ( 19.05341960407611168, 5.049401038298154454, 83.95724293864766707 ) ) ;
#108227=CARTESIAN_POINT ( 'NONE',  ( -16.51473224551082808, 9.474510206698731452, 68.33442372801900433 ) ) ;
#108228=CARTESIAN_POINT ( 'NONE',  ( 15.72974639402176855, 15.80617190586768217, 46.87609039468568994 ) ) ;
#108229=CARTESIAN_POINT ( 'NONE',  ( -13.89961937509957401, -13.97604488694547875, 99.37609039468567573 ) ) ;
#108230=CARTESIAN_POINT ( 'NONE',  ( 5.049401038297881783, 19.05341960407617563, 67.29275706135234714 ) ) ;
#108231=CARTESIAN_POINT ( 'NONE',  ( -9.474510206698964154, 16.51473224551069663, 35.41557627198102409 ) ) ;
#108233=CARTESIAN_POINT ( 'NONE',  ( 12.14591786802327356, -12.06949235617739191, 110.6260903946857042 ) ) ;
#108234=CARTESIAN_POINT ( 'NONE',  ( 19.03943276465977164, 0.05219959533936151252, 71.25109039468566152 ) ) ;
#108235=CARTESIAN_POINT ( 'NONE',  ( 12.14591786802309770, 12.06949235617756955, 24.37390960531435979 ) ) ;
#108236=CARTESIAN_POINT ( 'NONE',  ( 16.51473224551083163, -9.474510206698727899, 55.83442372801899722 ) ) ;
#108237=CARTESIAN_POINT ( 'NONE',  ( 5.823673210054444382, -21.52544592524334988, 105.2094237280190328 ) ) ;
#108238=CARTESIAN_POINT ( 'NONE',  ( 9.474510206698729675, 16.51473224551082808, 27.08442372801900433 ) ) ;
#108239=CARTESIAN_POINT ( 'NONE',  ( 19.02544592524343514, -5.153800228976328945, 23.54057627198102054 ) ) ;
#108240=CARTESIAN_POINT ( 'NONE',  ( 21.52544592524334988, 5.823673210054432836, 86.45942372801901854 ) ) ;
#108241=CARTESIAN_POINT ( 'NONE',  ( -14.34966873604972548, 8.224510206698743886, 38.33442372801900433 ) ) ;
#108243=CARTESIAN_POINT ( 'NONE',  ( -9.564922557960796823, -16.46253265017161027, 87.08224293864769550 ) ) ;
#108245=CARTESIAN_POINT ( 'NONE',  ( -16.51473224551069308, -9.474510206698971260, 81.66557627198103830 ) ) ;
#108247=CARTESIAN_POINT ( 'NONE',  ( -19.05341960407617563, 5.049401038297882671, 88.54275706135230450 ) ) ;
#108248=CARTESIAN_POINT ( 'NONE',  ( 0.05219959533909260263, 19.03943276465977164, 109.9989096053143669 ) ) ;
#108249=CARTESIAN_POINT ( 'NONE',  ( 16.51473224551083163, -9.474510206698727899, 20.83442372801899722 ) ) ;
#108250=CARTESIAN_POINT ( 'NONE',  ( -5.153800228976607833, 19.02544592524334988, 97.70942372801900433 ) ) ;
#108251=CARTESIAN_POINT ( 'NONE',  ( 12.06949235617757843, -12.14591786802309237, 93.12390960531436690 ) ) ;
#108253=CARTESIAN_POINT ( 'NONE',  ( 10.81492255796078972, 18.62759615963270932, 54.58224293864769550 ) ) ;
#108254=CARTESIAN_POINT ( 'NONE',  ( -5.719274019375978568, 21.55341960407610458, 35.20724293864768839 ) ) ;
#108255=CARTESIAN_POINT ( 'NONE',  ( 0.05219959533909260263, 19.03943276465977164, 29.99890960531435979 ) ) ;
#108257=CARTESIAN_POINT ( 'NONE',  ( 16.46253265017146816, 9.564922557961045513, 51.66775706135233293 ) ) ;
#108258=CARTESIAN_POINT ( 'NONE',  ( -16.55341960407611168, -4.379528057220339221, 36.45724293864768839 ) ) ;
#108259=CARTESIAN_POINT ( 'NONE',  ( -18.67979575497178146, -10.72451020669898902, 21.66557627198102409 ) ) ;
#108260=CARTESIAN_POINT ( 'NONE',  ( 5.823673210054444382, -21.52544592524334988, 75.20942372801901854 ) ) ;
#108261=CARTESIAN_POINT ( 'NONE',  ( 15.80617190586746368, 15.72974639402197994, 64.37390960531435269 ) ) ;
#108262=CARTESIAN_POINT ( 'NONE',  ( 0.05219959533937995610, -21.53943276465977519, 60.00109039468568284 ) ) ;
#108263=CARTESIAN_POINT ( 'NONE',  ( 21.52544592524334988, 5.823673210054432836, 56.45942372801902565 ) ) ;
#108265=CARTESIAN_POINT ( 'NONE',  ( -16.51473224551069308, -9.474510206698971260, 81.66557627198103830 ) ) ;
#108266=CARTESIAN_POINT ( 'NONE',  ( 12.06949235617739724, 12.14591786802326823, 81.87609039468568994 ) ) ;
#108267=CARTESIAN_POINT ( 'NONE',  ( -19.05341960407611168, -5.049401038298163336, 21.45724293864768839 ) ) ;
#108270=CARTESIAN_POINT ( 'NONE',  ( -16.53943276465976808, 0.05219959533911058130, 51.24890960531436690 ) ) ;
#108271=CARTESIAN_POINT ( 'NONE',  ( 16.55341960407611168, 4.379528057220329451, 28.95724293864769905 ) ) ;
#108272=CARTESIAN_POINT ( 'NONE',  ( -13.97604488694527625, -13.89961937509977652, 66.87390960531436690 ) ) ;
#108273=CARTESIAN_POINT ( 'NONE',  ( 16.51473224551069308, 9.474510206698969483, 39.16557627198103120 ) ) ;
#108274=CARTESIAN_POINT ( 'NONE',  ( 5.823673210054125526, 21.52544592524343514, 39.79057627198103830 ) ) ;
#108275=CARTESIAN_POINT ( 'NONE',  ( 13.89961937509957401, 13.97604488694547697, 31.87609039468566863 ) ) ;
#108277=CARTESIAN_POINT ( 'NONE',  ( -12.06949235617756955, 12.14591786802309770, 55.62390960531436690 ) ) ;
#108278=CARTESIAN_POINT ( 'NONE',  ( 18.62759615963271287, -10.81492255796078972, 23.33224293864769194 ) ) ;
#108279=DIRECTION ( 'NONE',  ( 0.000000000000000000, 0.000000000000000000, -1.000000000000000000 ) ) ;
#108280=CARTESIAN_POINT ( 'NONE',  ( 12.14591786802327356, -12.06949235617739191, 70.62609039468567573 ) ) ;
#108281=CARTESIAN_POINT ( 'NONE',  ( -9.564922557961040184, 16.46253265017147172, 72.91775706135233293 ) ) ;
#108282=CARTESIAN_POINT ( 'NONE',  ( 8.224510206698953496, -14.34966873604960469, 42.91557627198103120 ) ) ;
#108283=CARTESIAN_POINT ( 'NONE',  ( 17.26058549869091507, -6.457015423128522613, 51.12254162523935008 ) ) ;
#108284=CARTESIAN_POINT ( 'NONE',  ( -16.55341960407611168, -4.379528057220339221, 26.45724293864768839 ) ) ;
#108285=CARTESIAN_POINT ( 'NONE',  ( 13.89961937509977652, -13.97604488694527269, 58.12390960531436690 ) ) ;
#108286=CARTESIAN_POINT ( 'NONE',  ( -9.564922557960796823, -16.46253265017161027, 57.08224293864769550 ) ) ;
#108287=CARTESIAN_POINT ( 'NONE',  ( 9.564922557960805705, 16.46253265017160317, 39.58224293864768839 ) ) ;
#108288=CARTESIAN_POINT ( 'NONE',  ( 21.55341960407619695, -5.719274019375665929, 46.04275706135234714 ) ) ;
#108289=CARTESIAN_POINT ( 'NONE',  ( -0.05219959533909027116, -19.03943276465977164, 57.49890960531435979 ) ) ;
#108291=CARTESIAN_POINT ( 'NONE',  ( -19.02544592524342804, 5.153800228976336051, 51.04057627198103120 ) ) ;
#108292=CARTESIAN_POINT ( 'NONE',  ( 18.67979575497178502, 10.72451020669898547, 39.16557627198102409 ) ) ;
#108293=CARTESIAN_POINT ( 'NONE',  ( -15.72974639402176322, -15.80617190586768395, 74.37609039468568994 ) ) ;
#108294=CARTESIAN_POINT ( 'NONE',  ( 5.153800228976335163, 19.02544592524342804, 24.79057627198102765 ) ) ;
#108295=CARTESIAN_POINT ( 'NONE',  ( 5.719274019375991003, -21.55341960407610458, 22.70724293864769194 ) ) ;
#108296=CARTESIAN_POINT ( 'NONE',  ( 0.05219959533934541429, -16.53943276465976808, 90.00109039468567573 ) ) ;
#108297=CARTESIAN_POINT ( 'NONE',  ( 15.72974639402176855, 15.80617190586768217, 111.8760903946856615 ) ) ;
#108298=CARTESIAN_POINT ( 'NONE',  ( -4.379528057220086978, -16.55341960407618274, 69.79275706135234714 ) ) ;
#108299=CARTESIAN_POINT ( 'NONE',  ( 19.03943276465977164, -0.05219959533909143690, 113.7489096053143669 ) ) ;
#108300=CARTESIAN_POINT ( 'NONE',  ( -8.314922557961024197, 14.29746914071037800, 57.91775706135234714 ) ) ;
#108301=CARTESIAN_POINT ( 'NONE',  ( 12.06949235617739724, 12.14591786802326823, 36.87609039468568994 ) ) ;
#108302=CARTESIAN_POINT ( 'NONE',  ( 8.224510206698742110, 14.34966873604972548, 97.08442372801904696 ) ) ;
#108303=CARTESIAN_POINT ( 'NONE',  ( -18.62759615963255300, -10.81492255796106328, 59.16775706135234714 ) ) ;
#108304=CARTESIAN_POINT ( 'NONE',  ( -16.53943276465976808, -0.05219959533934237506, 18.75109039468568639 ) ) ;
#108305=CARTESIAN_POINT ( 'NONE',  ( 15.80617190586746368, 15.72974639402197994, 109.3739096053143811 ) ) ;
#108306=CARTESIAN_POINT ( 'NONE',  ( -16.53943276465976808, -0.05219959533934237506, 28.75109039468567929 ) ) ;
#108307=CARTESIAN_POINT ( 'NONE',  ( 4.379528057220092307, 16.55341960407617563, 92.29275706135236135 ) ) ;
#108309=CARTESIAN_POINT ( 'NONE',  ( -21.53943276465977519, -0.05219959533937600094, 88.75109039468567573 ) ) ;
#108310=CARTESIAN_POINT ( 'NONE',  ( 5.153800228976615827, -19.02544592524334988, 85.20942372801900433 ) ) ;
#108311=CARTESIAN_POINT ( 'NONE',  ( 0.05219959533910956823, 16.53943276465976808, 54.99890960531435269 ) ) ;
#108312=CARTESIAN_POINT ( 'NONE',  ( -4.379528057220328563, 16.55341960407611168, 50.20724293864769550 ) ) ;
#108313=CARTESIAN_POINT ( 'NONE',  ( 14.29746914071049879, -8.314922557960816363, 108.3322429386477097 ) ) ;
#108314=CARTESIAN_POINT ( 'NONE',  ( -13.97604488694547697, 13.89961937509957934, 48.12609039468566863 ) ) ;
#108315=CARTESIAN_POINT ( 'NONE',  ( 16.88567814943194634, -6.947325034625403184, 56.20998877347405909 ) ) ;
#108316=CARTESIAN_POINT ( 'NONE',  ( -15.72974639402176322, -15.80617190586768395, 44.37609039468567573 ) ) ;
#108317=CARTESIAN_POINT ( 'NONE',  ( -13.89961937509957401, -13.97604488694547875, 109.3760903946856331 ) ) ;
#108319=CARTESIAN_POINT ( 'NONE',  ( 5.153800228976335163, 19.02544592524342804, 109.7905762719810099 ) ) ;
#108320=CARTESIAN_POINT ( 'NONE',  ( -21.52544592524343514, 5.823673210054127303, 71.04057627198103830 ) ) ;
#108321=CARTESIAN_POINT ( 'NONE',  ( 16.51473224551083163, -9.474510206698727899, 95.83442372801900433 ) ) ;
#108322=CARTESIAN_POINT ( 'NONE',  ( 5.153800228976335163, 19.02544592524342804, 99.79057627198102409 ) ) ;
#108324=CARTESIAN_POINT ( 'NONE',  ( -12.14591786802309592, -12.06949235617757132, 101.8739096053143811 ) ) ;
#108325=CARTESIAN_POINT ( 'NONE',  ( 21.53943276465977519, 0.05219959533937863772, 91.25109039468568994 ) ) ;
#108326=CARTESIAN_POINT ( 'NONE',  ( 19.03943276465977164, -0.05219959533909143690, 28.74890960531435624 ) ) ;
#108328=CARTESIAN_POINT ( 'NONE',  ( -21.53943276465977519, -0.05219959533937600094, 38.75109039468567573 ) ) ;
#108329=CARTESIAN_POINT ( 'NONE',  ( 21.53943276465977519, 0.05219959533937863772, 86.25109039468568994 ) ) ;
#108330=CARTESIAN_POINT ( 'NONE',  ( -8.224510206698735004, -14.34966873604973081, 84.58442372801903275 ) ) ;
#108331=CARTESIAN_POINT ( 'NONE',  ( -21.55341960407619339, 5.719274019375674811, 48.54275706135234714 ) ) ;
#108332=CARTESIAN_POINT ( 'NONE',  ( 5.719274019375673035, 21.55341960407619339, 42.29275706135235424 ) ) ;
#108333=CARTESIAN_POINT ( 'NONE',  ( -5.153800228976607833, 19.02544592524334988, 62.70942372801899722 ) ) ;
#108334=CARTESIAN_POINT ( 'NONE',  ( -16.46253265017160317, 9.564922557960807481, 75.83224293864769550 ) ) ;
#108335=CARTESIAN_POINT ( 'NONE',  ( -4.379528057220328563, 16.55341960407611168, 110.2072429386477239 ) ) ;
#108336=CARTESIAN_POINT ( 'NONE',  ( -5.823673210054116645, -21.52544592524344225, 77.29057627198102409 ) ) ;
#108337=CARTESIAN_POINT ( 'NONE',  ( -4.483927247898539470, -16.52544592524342804, 67.29057627198103830 ) ) ;
#108338=CARTESIAN_POINT ( 'NONE',  ( -10.81492255796105439, 18.62759615963255655, 107.9177570613523471 ) ) ;
#108339=CARTESIAN_POINT ( 'NONE',  ( -8.314922557960811034, -14.29746914071050412, 82.08224293864768129 ) ) ;
#108340=CARTESIAN_POINT ( 'NONE',  ( -16.46253265017160317, 9.564922557960807481, 35.83224293864768839 ) ) ;
#108341=CARTESIAN_POINT ( 'NONE',  ( 5.153800228976615827, -19.02544592524334988, 65.20942372801900433 ) ) ;
#108342=CARTESIAN_POINT ( 'NONE',  ( 14.34966873604960469, 8.224510206698951720, 29.16557627198103120 ) ) ;
#108343=CARTESIAN_POINT ( 'NONE',  ( 21.55341960407619695, -5.719274019375665929, 96.04275706135236135 ) ) ;
#108344=EDGE_CURVE ( 'NONE', #122302, #44638, #195596, .T. ) ;
#108345=CARTESIAN_POINT ( 'NONE',  ( 16.46253265017160672, -9.564922557960803928, 98.33224293864769550 ) ) ;
#108346=CARTESIAN_POINT ( 'NONE',  ( -5.049401038297874678, -19.05341960407617918, 54.79275706135234003 ) ) ;
#108347=CARTESIAN_POINT ( 'NONE',  ( 5.823673210054125526, 21.52544592524343514, 59.79057627198103120 ) ) ;
#108349=CARTESIAN_POINT ( 'NONE',  ( 5.719274019375673035, 21.55341960407619339, 22.29275706135235069 ) ) ;
#108350=CARTESIAN_POINT ( 'NONE',  ( -16.51473224551082808, 9.474510206698731452, 113.3344237280190043 ) ) ;
#108351=CARTESIAN_POINT ( 'NONE',  ( -12.06949235617739369, -12.14591786802326823, 74.37609039468568994 ) ) ;
#108353=CARTESIAN_POINT ( 'NONE',  ( -21.53943276465977519, -0.05219959533937600094, 28.75109039468567929 ) ) ;
#108354=CARTESIAN_POINT ( 'NONE',  ( -14.34966873604960291, -8.224510206698953496, 101.6655762719810383 ) ) ;
#108356=CARTESIAN_POINT ( 'NONE',  ( 4.483927247898790824, -16.52544592524335698, 45.20942372801901854 ) ) ;
#108357=CARTESIAN_POINT ( 'NONE',  ( -4.379528057220328563, 16.55341960407611168, 75.20724293864769550 ) ) ;
#108358=CARTESIAN_POINT ( 'NONE',  ( -5.823673210054116645, -21.52544592524344225, 72.29057627198102409 ) ) ;
#108360=CARTESIAN_POINT ( 'NONE',  ( -8.224510206698735004, -14.34966873604973081, 99.58442372801900433 ) ) ;
#108361=CARTESIAN_POINT ( 'NONE',  ( 4.379528057220092307, 16.55341960407617563, 32.29275706135235424 ) ) ;
#108362=CARTESIAN_POINT ( 'NONE',  ( -13.89961937509977652, 13.97604488694528158, 50.62390960531435979 ) ) ;
#108363=CARTESIAN_POINT ( 'NONE',  ( 4.483927247898790824, -16.52544592524335698, 85.20942372801901854 ) ) ;
#108364=CARTESIAN_POINT ( 'NONE',  ( -9.564922557961040184, 16.46253265017147172, 67.91775706135233293 ) ) ;
#108365=CARTESIAN_POINT ( 'NONE',  ( 10.72451020669898902, -18.67979575497178502, 77.91557627198102409 ) ) ;
#108366=CARTESIAN_POINT ( 'NONE',  ( -12.06949235617739369, -12.14591786802326823, 99.37609039468568994 ) ) ;
#108368=CARTESIAN_POINT ( 'NONE',  ( -21.53943276465977519, -0.05219959533937600094, 83.75109039468568994 ) ) ;
#108369=CARTESIAN_POINT ( 'NONE',  ( -18.62759615963270932, 10.81492255796079327, 70.83224293864770971 ) ) ;
#108370=CARTESIAN_POINT ( 'NONE',  ( -21.52544592524343514, 5.823673210054127303, 46.04057627198103830 ) ) ;
#108371=ORIENTED_EDGE ( 'NONE', *, *, #10693, .T. ) ;
#108373=CARTESIAN_POINT ( 'NONE',  ( -12.06949235617739369, -12.14591786802326823, 79.37609039468567573 ) ) ;
#108374=CARTESIAN_POINT ( 'NONE',  ( -0.05219959533907301413, -21.53943276465977519, 52.49890960531435979 ) ) ;
#108376=CARTESIAN_POINT ( 'NONE',  ( -21.53943276465977519, 0.05219959533907696930, 21.24890960531436690 ) ) ;
#108378=CARTESIAN_POINT ( 'NONE',  ( -13.89961937509977652, 13.97604488694528158, 30.62390960531435269 ) ) ;
#108379=CARTESIAN_POINT ( 'NONE',  ( -18.67979575497178146, -10.72451020669898902, 81.66557627198103830 ) ) ;
#108380=CARTESIAN_POINT ( 'NONE',  ( -8.224510206698735004, -14.34966873604973081, 99.58442372801900433 ) ) ;
#108381=CARTESIAN_POINT ( 'NONE',  ( 21.52544592524334988, 5.823673210054432836, 46.45942372801901854 ) ) ;
#108382=CARTESIAN_POINT ( 'NONE',  ( -16.51473224551082808, 9.474510206698731452, 113.3344237280190043 ) ) ;
#108383=CARTESIAN_POINT ( 'NONE',  ( -4.483927247898539470, -16.52544592524342804, 112.2905762719810241 ) ) ;
#108384=CARTESIAN_POINT ( 'NONE',  ( -19.05341960407617563, 5.049401038297882671, 108.5427570613523187 ) ) ;
#108385=CARTESIAN_POINT ( 'NONE',  ( 16.51473224551069308, 9.474510206698969483, 34.16557627198102409 ) ) ;
#108387=CARTESIAN_POINT ( 'NONE',  ( 13.97604488694527802, 13.89961937509977652, 104.3739096053143385 ) ) ;
#108388=CARTESIAN_POINT ( 'NONE',  ( -4.483927247898782831, 16.52544592524335698, 82.70942372801900433 ) ) ;
#108389=CARTESIAN_POINT ( 'NONE',  ( 5.049401038297881783, 19.05341960407617563, 77.29275706135231871 ) ) ;
#108390=CARTESIAN_POINT ( 'NONE',  ( -5.153800228976607833, 19.02544592524334988, 22.70942372801899012 ) ) ;
#108391=CARTESIAN_POINT ( 'NONE',  ( -21.55341960407610458, -5.719274019375992779, 56.45724293864768839 ) ) ;
#108392=CARTESIAN_POINT ( 'NONE',  ( -12.14591786802326823, 12.06949235617739902, 83.12609039468568994 ) ) ;
#108393=CARTESIAN_POINT ( 'NONE',  ( -19.03943276465977164, -0.05219959533935918106, 88.75109039468567573 ) ) ;
#108394=CARTESIAN_POINT ( 'NONE',  ( 5.049401038298161559, -19.05341960407611168, 52.70724293864767418 ) ) ;
#108395=CARTESIAN_POINT ( 'NONE',  ( 13.89961937509977652, -13.97604488694527269, 98.12390960531433848 ) ) ;
#108396=CARTESIAN_POINT ( 'NONE',  ( 21.55341960407619695, -5.719274019375665929, 46.04275706135234714 ) ) ;
#108397=CARTESIAN_POINT ( 'NONE',  ( 9.474510206698971260, -16.51473224551069308, 52.91557627198102409 ) ) ;
#108399=CARTESIAN_POINT ( 'NONE',  ( -5.049401038298153566, 19.05341960407611168, 110.2072429386476671 ) ) ;
#108400=CARTESIAN_POINT ( 'NONE',  ( 14.34966873604960469, 8.224510206698951720, 69.16557627198102409 ) ) ;
#108401=CARTESIAN_POINT ( 'NONE',  ( 0.05219959533907565091, 21.53943276465977519, 54.99890960531435269 ) ) ;
#108402=CARTESIAN_POINT ( 'NONE',  ( 19.76836671444428006, -4.606730274327726526, 102.5000000000000284 ) ) ;
#108403=CARTESIAN_POINT ( 'NONE',  ( 19.02544592524334988, 5.153800228976608722, 46.45942372801899012 ) ) ;
#108405=CARTESIAN_POINT ( 'NONE',  ( 13.89961937509977652, -13.97604488694527269, 63.12390960531435979 ) ) ;
#108406=CARTESIAN_POINT ( 'NONE',  ( 19.03943276465977164, -0.05219959533909143690, 78.74890960531436690 ) ) ;
#108407=CARTESIAN_POINT ( 'NONE',  ( -16.52544592524335698, -4.483927247898792601, 53.95942372801900433 ) ) ;
#108408=CARTESIAN_POINT ( 'NONE',  ( -18.22780087662121673, -5.500000000000063061, 66.48459894673892734 ) ) ;
#108409=CARTESIAN_POINT ( 'NONE',  ( 17.97161686093727795, -5.499999999999969802, 93.49637206859166838 ) ) ;
#108410=CARTESIAN_POINT ( 'NONE',  ( -14.29746914071037622, -8.314922557961029526, 84.16775706135234714 ) ) ;
#108412=CARTESIAN_POINT ( 'NONE',  ( -16.55341960407617563, 4.379528057220093196, 78.54275706135236135 ) ) ;
#108413=CARTESIAN_POINT ( 'NONE',  ( 8.314922557961029526, -14.29746914071037800, 50.41775706135235424 ) ) ;
#108414=CARTESIAN_POINT ( 'NONE',  ( 19.05341960407617918, -5.049401038297876454, 21.04275706135232582 ) ) ;
#108415=CARTESIAN_POINT ( 'NONE',  ( -13.89961937509977652, 13.97604488694528158, 60.62390960531436690 ) ) ;
#108416=CARTESIAN_POINT ( 'NONE',  ( -21.55341960407619339, 5.719274019375674811, 48.54275706135234714 ) ) ;
#108417=CARTESIAN_POINT ( 'NONE',  ( -9.564922557961040184, 16.46253265017147172, 77.91775706135234714 ) ) ;
#108418=CARTESIAN_POINT ( 'NONE',  ( -9.474510206698720793, -16.51473224551083518, 19.58442372801899722 ) ) ;
#108420=CARTESIAN_POINT ( 'NONE',  ( -16.46253265017160317, 9.564922557960807481, 30.83224293864769550 ) ) ;
#108422=CARTESIAN_POINT ( 'NONE',  ( 10.72451020669898902, -18.67979575497178502, 67.91557627198102409 ) ) ;
#108423=CARTESIAN_POINT ( 'NONE',  ( 5.823673210054125526, 21.52544592524343514, 24.79057627198103120 ) ) ;
#108424=CARTESIAN_POINT ( 'NONE',  ( -0.05219959533909027116, -19.03943276465977164, 22.49890960531436690 ) ) ;
#108425=CARTESIAN_POINT ( 'NONE',  ( 12.06949235617739724, 12.14591786802326823, 31.87609039468567929 ) ) ;
#108426=CARTESIAN_POINT ( 'NONE',  ( 16.53943276465976808, -0.05219959533910856209, 23.74890960531435269 ) ) ;
#108428=CARTESIAN_POINT ( 'NONE',  ( -18.67979575497178146, -10.72451020669898902, 111.6655762719810525 ) ) ;
#108429=CARTESIAN_POINT ( 'NONE',  ( 12.14591786802309770, 12.06949235617756955, 39.37390960531436690 ) ) ;
#108431=CARTESIAN_POINT ( 'NONE',  ( 19.03943276465977164, 0.05219959533936151252, 111.2510903946856757 ) ) ;
#108432=CARTESIAN_POINT ( 'NONE',  ( 13.97604488694548053, -13.89961937509957401, 20.62609039468567573 ) ) ;
#108433=CARTESIAN_POINT ( 'NONE',  ( -16.53943276465976808, 0.05219959533911058130, 41.24890960531435269 ) ) ;
#108434=CARTESIAN_POINT ( 'NONE',  ( 5.719274019375991003, -21.55341960407610458, 102.7072429386476955 ) ) ;
#108435=CARTESIAN_POINT ( 'NONE',  ( 17.50000000000000000, 5.499999999999997335, 31.70309617465830243 ) ) ;
#108436=CARTESIAN_POINT ( 'NONE',  ( -10.72451020669898014, 18.67979575497178502, 65.41557627198102409 ) ) ;
#108437=CARTESIAN_POINT ( 'NONE',  ( 19.02544592524343514, -5.153800228976328945, 78.54057627198099567 ) ) ;
#108438=CARTESIAN_POINT ( 'NONE',  ( 8.224510206698953496, -14.34966873604960469, 42.91557627198103120 ) ) ;
#108439=CARTESIAN_POINT ( 'NONE',  ( -9.564922557960796823, -16.46253265017161027, 87.08224293864769550 ) ) ;
#108440=CARTESIAN_POINT ( 'NONE',  ( -18.22780087662123094, -5.499999999999984901, 86.48459894673892734 ) ) ;
#108441=CARTESIAN_POINT ( 'NONE',  ( -9.474510206698720793, -16.51473224551083518, 54.58442372801899722 ) ) ;
#108442=CARTESIAN_POINT ( 'NONE',  ( 10.72451020669898902, -18.67979575497178502, 87.91557627198103830 ) ) ;
#108443=CARTESIAN_POINT ( 'NONE',  ( 16.55341960407611168, 4.379528057220329451, 98.95724293864770971 ) ) ;
#108444=CARTESIAN_POINT ( 'NONE',  ( -18.67979575497193778, 10.72451020669871902, 53.33442372801901854 ) ) ;
#108446=CARTESIAN_POINT ( 'NONE',  ( 14.29746914071049879, -8.314922557960816363, 28.33224293864769550 ) ) ;
#108447=CARTESIAN_POINT ( 'NONE',  ( 19.05341960407611168, 5.049401038298154454, 38.95724293864767418 ) ) ;
#108448=CARTESIAN_POINT ( 'NONE',  ( -16.46253265017160317, 9.564922557960807481, 95.83224293864769550 ) ) ;
#108449=CARTESIAN_POINT ( 'NONE',  ( -18.62759615963270932, 10.81492255796079327, 65.83224293864769550 ) ) ;
#108450=CARTESIAN_POINT ( 'NONE',  ( 9.474510206698729675, 16.51473224551082808, 92.08442372801900433 ) ) ;
#108451=CARTESIAN_POINT ( 'NONE',  ( -13.97604488694527625, -13.89961937509977652, 31.87390960531435979 ) ) ;
#108452=CARTESIAN_POINT ( 'NONE',  ( 21.52544592524344225, -5.823673210054117533, 53.54057627198103120 ) ) ;
#108453=CARTESIAN_POINT ( 'NONE',  ( -21.52544592524334988, -5.823673210054445271, 78.95942372801901854 ) ) ;
#108455=CARTESIAN_POINT ( 'NONE',  ( 4.483927247898790824, -16.52544592524335698, 80.20942372801901854 ) ) ;
#108456=CARTESIAN_POINT ( 'NONE',  ( -13.97604488694527625, -13.89961937509977652, 51.87390960531436690 ) ) ;
#108457=CARTESIAN_POINT ( 'NONE',  ( 9.564922557960805705, 16.46253265017160317, 59.58224293864769550 ) ) ;
#108459=CARTESIAN_POINT ( 'NONE',  ( 9.474510206698729675, 16.51473224551082808, 32.08442372801900433 ) ) ;
#108460=CARTESIAN_POINT ( 'NONE',  ( 4.379528057220092307, 16.55341960407617563, 77.29275706135234714 ) ) ;
#108461=CARTESIAN_POINT ( 'NONE',  ( -10.72451020669870658, -18.67979575497194134, 94.58442372801901854 ) ) ;
#108462=CARTESIAN_POINT ( 'NONE',  ( 9.564922557960805705, 16.46253265017160317, 74.58224293864769550 ) ) ;
#108463=CARTESIAN_POINT ( 'NONE',  ( -10.81492255796078084, -18.62759615963271287, 37.08224293864768129 ) ) ;
#108464=CARTESIAN_POINT ( 'NONE',  ( 9.564922557961047289, -16.46253265017146816, 110.4177570613523471 ) ) ;
#108465=CARTESIAN_POINT ( 'NONE',  ( -18.62759615963255300, -10.81492255796106328, 79.16775706135234714 ) ) ;
#108466=CARTESIAN_POINT ( 'NONE',  ( 12.14591786802327356, -12.06949235617739191, 45.62609039468567573 ) ) ;
#108467=CARTESIAN_POINT ( 'NONE',  ( 15.72974639402199770, -15.80617190586745480, 103.1239096053143811 ) ) ;
#108468=CARTESIAN_POINT ( 'NONE',  ( 19.03943276465977164, 0.05219959533936151252, 106.2510903946856615 ) ) ;
#108469=CARTESIAN_POINT ( 'NONE',  ( 19.02544592524343514, -5.153800228976328945, 78.54057627198099567 ) ) ;
#108470=CARTESIAN_POINT ( 'NONE',  ( 8.224510206698742110, 14.34966873604972548, 32.08442372801901854 ) ) ;
#108471=CARTESIAN_POINT ( 'NONE',  ( -5.153800228976328057, -19.02544592524343514, 37.29057627198102409 ) ) ;
#108472=CARTESIAN_POINT ( 'NONE',  ( 12.14591786802327356, -12.06949235617739191, 20.62609039468568639 ) ) ;
#108473=CARTESIAN_POINT ( 'NONE',  ( -16.52544592524342804, 4.483927247898546575, 71.04057627198103830 ) ) ;
#108475=CARTESIAN_POINT ( 'NONE',  ( -14.34966873604972548, 8.224510206698743886, 83.33442372801903275 ) ) ;
#108476=CARTESIAN_POINT ( 'NONE',  ( -21.55341960407619339, 5.719274019375674811, 33.54275706135234714 ) ) ;
#108477=CARTESIAN_POINT ( 'NONE',  ( 0.05219959533909260263, 19.03943276465977164, 49.99890960531435979 ) ) ;
#108478=CARTESIAN_POINT ( 'NONE',  ( -9.474510206698964154, 16.51473224551069663, 75.41557627198103830 ) ) ;
#108479=CARTESIAN_POINT ( 'NONE',  ( 12.14591786802327356, -12.06949235617739191, 90.62609039468567573 ) ) ;
#108480=CARTESIAN_POINT ( 'NONE',  ( -17.97214573761834089, -5.500000000000018652, 81.46970049038658601 ) ) ;
#108482=ORIENTED_EDGE ( 'NONE', *, *, #125633, .T. ) ;
#108483=CARTESIAN_POINT ( 'NONE',  ( 21.52544592524334988, 5.823673210054432836, 111.4594237280190328 ) ) ;
#108484=CARTESIAN_POINT ( 'NONE',  ( 5.153800228976335163, 19.02544592524342804, 29.79057627198102409 ) ) ;
#108487=CARTESIAN_POINT ( 'NONE',  ( -4.379528057220086978, -16.55341960407618274, 34.79275706135235424 ) ) ;
#108488=CARTESIAN_POINT ( 'NONE',  ( -9.564922557961040184, 16.46253265017147172, 62.91775706135233293 ) ) ;
#108489=CARTESIAN_POINT ( 'NONE',  ( -0.05219959533934338120, 16.53943276465976808, 42.50109039468567573 ) ) ;
#108490=CARTESIAN_POINT ( 'NONE',  ( -0.05219959533909027116, -19.03943276465977164, 47.49890960531435979 ) ) ;
#108491=CARTESIAN_POINT ( 'NONE',  ( 9.564922557960805705, 16.46253265017160317, 109.5822429386476955 ) ) ;
#108492=CARTESIAN_POINT ( 'NONE',  ( -19.05341960407611168, -5.049401038298163336, 66.45724293864769550 ) ) ;
#108493=CARTESIAN_POINT ( 'NONE',  ( 21.52544592524344225, -5.823673210054117533, 93.54057627198103830 ) ) ;
#108494=CARTESIAN_POINT ( 'NONE',  ( 13.89961937509977652, -13.97604488694527269, 88.12390960531438111 ) ) ;
#108495=CARTESIAN_POINT ( 'NONE',  ( 5.049401038298161559, -19.05341960407611168, 27.70724293864769550 ) ) ;
#108496=CARTESIAN_POINT ( 'NONE',  ( 5.153800228976335163, 19.02544592524342804, 64.79057627198100988 ) ) ;
#108497=CARTESIAN_POINT ( 'NONE',  ( -4.483927247898782831, 16.52544592524335698, 107.7094237280190328 ) ) ;
#108498=CARTESIAN_POINT ( 'NONE',  ( -16.51473224551069308, -9.474510206698971260, 26.66557627198103120 ) ) ;
#108499=CARTESIAN_POINT ( 'NONE',  ( -19.03943276465977164, -0.05219959533935918106, 18.75109039468567218 ) ) ;
#108500=CARTESIAN_POINT ( 'NONE',  ( -16.55341960407611168, -4.379528057220339221, 61.45724293864770260 ) ) ;
#108501=CARTESIAN_POINT ( 'NONE',  ( -10.72451020669870658, -18.67979575497194134, 99.58442372801900433 ) ) ;
#108502=CARTESIAN_POINT ( 'NONE',  ( 5.153800228976335163, 19.02544592524342804, 34.79057627198102409 ) ) ;
#108504=CARTESIAN_POINT ( 'NONE',  ( -14.29746914071049879, 8.314922557960819915, 35.83224293864768839 ) ) ;
#108505=CARTESIAN_POINT ( 'NONE',  ( 10.81492255796106328, -18.62759615963255655, 85.41775706135236135 ) ) ;
#108506=CARTESIAN_POINT ( 'NONE',  ( -0.05219959533909027116, -19.03943276465977164, 82.49890960531436690 ) ) ;
#108507=CARTESIAN_POINT ( 'NONE',  ( 16.46253265017160672, -9.564922557960803928, 98.33224293864769550 ) ) ;
#108508=CARTESIAN_POINT ( 'NONE',  ( -8.224510206698948167, 14.34966873604960824, 110.4155762719810383 ) ) ;
#108509=CARTESIAN_POINT ( 'NONE',  ( 8.224510206698953496, -14.34966873604960469, 77.91557627198102409 ) ) ;
#108510=CARTESIAN_POINT ( 'NONE',  ( 15.72974639402199770, -15.80617190586745480, 83.12390960531436690 ) ) ;
#108511=CARTESIAN_POINT ( 'NONE',  ( 16.51473224551069308, 9.474510206698969483, 69.16557627198102409 ) ) ;
#108512=CARTESIAN_POINT ( 'NONE',  ( -21.55341960407610458, -5.719274019375992779, 91.45724293864769550 ) ) ;
#108513=CARTESIAN_POINT ( 'NONE',  ( -16.51473224551082808, 9.474510206698731452, 78.33442372801900433 ) ) ;
#108515=CARTESIAN_POINT ( 'NONE',  ( 18.22780087662119897, -5.500000000000096811, 48.51763182126894236 ) ) ;
#108516=CARTESIAN_POINT ( 'NONE',  ( -12.06949235617756955, 12.14591786802309770, 95.62390960531436690 ) ) ;
#108517=CARTESIAN_POINT ( 'NONE',  ( -19.05341960407611168, -5.049401038298163336, 61.45724293864769550 ) ) ;
#108518=CARTESIAN_POINT ( 'NONE',  ( -21.55341960407610458, -5.719274019375992779, 66.45724293864768129 ) ) ;
#108520=CARTESIAN_POINT ( 'NONE',  ( -14.34966873604972548, 8.224510206698743886, 108.3344237280190185 ) ) ;
#108522=CARTESIAN_POINT ( 'NONE',  ( -16.52544592524335698, -4.483927247898792601, 23.95942372801901143 ) ) ;
#108523=CARTESIAN_POINT ( 'NONE',  ( 4.483927247898545687, 16.52544592524342804, 74.79057627198105251 ) ) ;
#108525=CARTESIAN_POINT ( 'NONE',  ( -9.564922557960796823, -16.46253265017161027, 77.08224293864769550 ) ) ;
#108526=CARTESIAN_POINT ( 'NONE',  ( 9.474510206698971260, -16.51473224551069308, 32.91557627198102409 ) ) ;
#108527=CARTESIAN_POINT ( 'NONE',  ( -12.06949235617756955, 12.14591786802309770, 70.62390960531436690 ) ) ;
#108528=CARTESIAN_POINT ( 'NONE',  ( 19.05341960407611168, 5.049401038298154454, 108.9572429386477097 ) ) ;
#108529=CARTESIAN_POINT ( 'NONE',  ( -19.05341960407617563, 5.049401038297882671, 93.54275706135234714 ) ) ;
#108530=CARTESIAN_POINT ( 'NONE',  ( -19.05341960407611168, -5.049401038298163336, 76.45724293864769550 ) ) ;
#108531=CARTESIAN_POINT ( 'NONE',  ( 19.05341960407611168, 5.049401038298154454, 83.95724293864766707 ) ) ;
#108532=CARTESIAN_POINT ( 'NONE',  ( 15.80617190586746368, 15.72974639402197994, 79.37390960531436690 ) ) ;
#108533=CARTESIAN_POINT ( 'NONE',  ( -14.29746914071037622, -8.314922557961029526, 69.16775706135234714 ) ) ;
#108534=CARTESIAN_POINT ( 'NONE',  ( -16.21995358207276894, 7.366697692864291547, 94.93551001512068410 ) ) ;
#108535=CARTESIAN_POINT ( 'NONE',  ( -9.564922557960796823, -16.46253265017161027, 62.08224293864769550 ) ) ;
#108536=CARTESIAN_POINT ( 'NONE',  ( 21.52544592524344225, -5.823673210054117533, 73.54057627198102409 ) ) ;
#108537=CARTESIAN_POINT ( 'NONE',  ( 16.51473224551083163, -9.474510206698727899, 100.8344237280190043 ) ) ;
#108538=CARTESIAN_POINT ( 'NONE',  ( -14.34966873604960291, -8.224510206698953496, 36.66557627198103120 ) ) ;
#108539=CARTESIAN_POINT ( 'NONE',  ( -0.05219959533937732626, 21.53943276465977519, 52.50109039468567573 ) ) ;
#108540=CARTESIAN_POINT ( 'NONE',  ( 17.60779699588839620, 5.500000000000007105, 83.84981316670105400 ) ) ;
#108541=CARTESIAN_POINT ( 'NONE',  ( 16.55341960407618274, -4.379528057220086978, 76.04275706135237556 ) ) ;
#108542=CARTESIAN_POINT ( 'NONE',  ( -9.474510206698964154, 16.51473224551069663, 105.4155762719810383 ) ) ;
#108544=CARTESIAN_POINT ( 'NONE',  ( -16.79531203550647689, 7.028104445595609207, 78.74755011779562608 ) ) ;
#108545=CARTESIAN_POINT ( 'NONE',  ( -12.06949235617739369, -12.14591786802326823, 89.37609039468568994 ) ) ;
#108546=CARTESIAN_POINT ( 'NONE',  ( -8.314922557961024197, 14.29746914071037800, 47.91775706135234714 ) ) ;
#108547=CARTESIAN_POINT ( 'NONE',  ( 16.46253265017160672, -9.564922557960803928, 58.33224293864769550 ) ) ;
#108548=CARTESIAN_POINT ( 'NONE',  ( -19.03943276465977164, 0.05219959533909376836, 71.24890960531435269 ) ) ;
#108549=CARTESIAN_POINT ( 'NONE',  ( -0.05219959533937732626, 21.53943276465977519, 52.50109039468567573 ) ) ;
#108550=CARTESIAN_POINT ( 'NONE',  ( 16.53943276465976808, 0.05219959533934440121, 66.25109039468567573 ) ) ;
#108551=CARTESIAN_POINT ( 'NONE',  ( 8.224510206698953496, -14.34966873604960469, 32.91557627198102409 ) ) ;
#108552=CARTESIAN_POINT ( 'NONE',  ( 16.46253265017160672, -9.564922557960803928, 38.33224293864768839 ) ) ;
#108553=CARTESIAN_POINT ( 'NONE',  ( 9.564922557960805705, 16.46253265017160317, 29.58224293864769550 ) ) ;
#108554=CARTESIAN_POINT ( 'NONE',  ( 12.14591786802327356, -12.06949235617739191, 30.62609039468567929 ) ) ;
#108556=CARTESIAN_POINT ( 'NONE',  ( 9.564922557961047289, -16.46253265017146816, 80.41775706135234714 ) ) ;
#108557=CARTESIAN_POINT ( 'NONE',  ( -0.05219959533910754901, -16.53943276465976808, 77.49890960531433848 ) ) ;
#108558=CARTESIAN_POINT ( 'NONE',  ( 16.51473224551069308, 9.474510206698969483, 54.16557627198103120 ) ) ;
#108559=CARTESIAN_POINT ( 'NONE',  ( -5.153800228976607833, 19.02544592524334988, 92.70942372801901854 ) ) ;
#108561=CARTESIAN_POINT ( 'NONE',  ( -0.05219959533937732626, 21.53943276465977519, 92.50109039468567573 ) ) ;
#108562=CARTESIAN_POINT ( 'NONE',  ( 4.379528057220092307, 16.55341960407617563, 52.29275706135236135 ) ) ;
#108563=CARTESIAN_POINT ( 'NONE',  ( 16.18388926212240619, 7.379444403734400915, 37.93953151366152809 ) ) ;
#108564=CARTESIAN_POINT ( 'NONE',  ( 5.823673210054125526, 21.52544592524343514, 49.79057627198102409 ) ) ;
#108565=CARTESIAN_POINT ( 'NONE',  ( -16.53943276465976808, -0.05219959533934237506, 38.75109039468567573 ) ) ;
#108566=CARTESIAN_POINT ( 'NONE',  ( 13.89961937509978007, -13.97604488694527269, 38.12390960531436690 ) ) ;
#108567=CARTESIAN_POINT ( 'NONE',  ( 9.474510206698729675, 16.51473224551082808, 42.08442372801900433 ) ) ;
#108569=CARTESIAN_POINT ( 'NONE',  ( -9.564922557960796823, -16.46253265017161027, 77.08224293864769550 ) ) ;
#108570=CARTESIAN_POINT ( 'NONE',  ( 5.049401038298161559, -19.05341960407611168, 57.70724293864769550 ) ) ;
#108571=LINE ( 'NONE', #63057, #65639 ) ;
#108572=CARTESIAN_POINT ( 'NONE',  ( 19.03943276465977164, -0.05219959533909143690, 63.74890960531435979 ) ) ;
#108574=CARTESIAN_POINT ( 'NONE',  ( -9.474510206698720793, -16.51473224551083518, 34.58442372801899722 ) ) ;
#108575=CARTESIAN_POINT ( 'NONE',  ( 16.51473224551083163, -9.474510206698727899, 20.83442372801899722 ) ) ;
#108576=CARTESIAN_POINT ( 'NONE',  ( -16.55341960407611168, -4.379528057220339221, 41.45724293864769550 ) ) ;
#108577=CARTESIAN_POINT ( 'NONE',  ( 5.049401038298161559, -19.05341960407611168, 37.70724293864768839 ) ) ;
#108578=CARTESIAN_POINT ( 'NONE',  ( 16.51473224551069308, 9.474510206698969483, 104.1655762719810241 ) ) ;
#108579=CARTESIAN_POINT ( 'NONE',  ( -18.62759615963255300, -10.81492255796106328, 79.16775706135234714 ) ) ;
#108580=CARTESIAN_POINT ( 'NONE',  ( 16.46253265017160672, -9.564922557960803928, 53.33224293864768839 ) ) ;
#108581=CARTESIAN_POINT ( 'NONE',  ( 21.52544592524334988, 5.823673210054432836, 81.45942372801900433 ) ) ;
#108582=CARTESIAN_POINT ( 'NONE',  ( 21.55341960407610458, 5.719274019375980345, 38.95724293864768839 ) ) ;
#108583=CARTESIAN_POINT ( 'NONE',  ( 10.81492255796106328, -18.62759615963255655, 20.41775706135234714 ) ) ;
#108584=CARTESIAN_POINT ( 'NONE',  ( 19.03943276465977164, 0.05219959533936151252, 46.25109039468566863 ) ) ;
#108585=CARTESIAN_POINT ( 'NONE',  ( 19.03943276465977164, -0.05219959533909143690, 33.74890960531435979 ) ) ;
#108586=CARTESIAN_POINT ( 'NONE',  ( -0.05219959533909027116, -19.03943276465977164, 82.49890960531436690 ) ) ;
#108587=CARTESIAN_POINT ( 'NONE',  ( -0.05219959533934338120, 16.53943276465976808, 22.50109039468567573 ) ) ;
#108588=CARTESIAN_POINT ( 'NONE',  ( -14.34966873604960291, -8.224510206698953496, 86.66557627198102409 ) ) ;
#108589=CARTESIAN_POINT ( 'NONE',  ( -5.719274019375978568, 21.55341960407610458, 30.20724293864769550 ) ) ;
#108590=CARTESIAN_POINT ( 'NONE',  ( 16.51473224551083163, -9.474510206698727899, 95.83442372801900433 ) ) ;
#108591=CARTESIAN_POINT ( 'NONE',  ( 21.55341960407610458, 5.719274019375980345, 103.9572429386476813 ) ) ;
#108592=CARTESIAN_POINT ( 'NONE',  ( 15.72974639402176855, 15.80617190586768217, 51.87609039468568284 ) ) ;
#108593=CARTESIAN_POINT ( 'NONE',  ( 4.379528057220092307, 16.55341960407617563, 52.29275706135236135 ) ) ;
#108594=CARTESIAN_POINT ( 'NONE',  ( -4.483927247898782831, 16.52544592524335698, 67.70942372801901854 ) ) ;
#108596=CARTESIAN_POINT ( 'NONE',  ( -13.97604488694527625, -13.89961937509977652, 56.87390960531434558 ) ) ;
#108597=CARTESIAN_POINT ( 'NONE',  ( 8.314922557961029526, -14.29746914071037800, 90.41775706135236135 ) ) ;
#108598=CARTESIAN_POINT ( 'NONE',  ( 10.72451020669871369, 18.67979575497193778, 22.08442372801901143 ) ) ;
#108599=CARTESIAN_POINT ( 'NONE',  ( -8.224510206698948167, 14.34966873604960824, 65.41557627198102409 ) ) ;
#108600=CARTESIAN_POINT ( 'NONE',  ( 5.049401038298161559, -19.05341960407611168, 82.70724293864770971 ) ) ;
#108601=CARTESIAN_POINT ( 'NONE',  ( 8.314922557961029526, -14.29746914071037800, 70.41775706135236135 ) ) ;
#108602=CARTESIAN_POINT ( 'NONE',  ( 0.05219959533937995610, -21.53943276465977519, 60.00109039468568284 ) ) ;
#108603=CARTESIAN_POINT ( 'NONE',  ( 12.14591786802327356, -12.06949235617739191, 20.62609039468568639 ) ) ;
#108604=CARTESIAN_POINT ( 'NONE',  ( 5.823673210054125526, 21.52544592524343514, 114.7905762719810383 ) ) ;
#108605=CARTESIAN_POINT ( 'NONE',  ( 14.29746914071049879, -8.314922557960816363, 53.33224293864769550 ) ) ;
#108607=CARTESIAN_POINT ( 'NONE',  ( -16.20579543436678094, 7.371946100355086351, 74.43479165828127009 ) ) ;
#108608=CARTESIAN_POINT ( 'NONE',  ( -10.81492255796078084, -18.62759615963271287, 82.08224293864768129 ) ) ;
#108609=CARTESIAN_POINT ( 'NONE',  ( 16.55341960407611168, 4.379528057220329451, 43.95724293864769550 ) ) ;
#108612=CARTESIAN_POINT ( 'NONE',  ( 5.823673210054125526, 21.52544592524343514, 109.7905762719810383 ) ) ;
#108613=CARTESIAN_POINT ( 'NONE',  ( -19.05341960407611168, -5.049401038298163336, 111.4572429386476671 ) ) ;
#108614=CARTESIAN_POINT ( 'NONE',  ( 5.719274019375673035, 21.55341960407619339, 22.29275706135235069 ) ) ;
#108615=CARTESIAN_POINT ( 'NONE',  ( -12.14591786802309592, -12.06949235617757132, 51.87390960531437401 ) ) ;
#108616=CARTESIAN_POINT ( 'NONE',  ( -14.34966873604972548, 8.224510206698743886, 58.33442372801901143 ) ) ;
#108617=CARTESIAN_POINT ( 'NONE',  ( 16.51473224551069308, 9.474510206698969483, 64.16557627198102409 ) ) ;
#108618=CARTESIAN_POINT ( 'NONE',  ( -19.05341960407617563, 5.049401038297882671, 68.54275706135230450 ) ) ;
#108619=CARTESIAN_POINT ( 'NONE',  ( -19.05341960407611168, -5.049401038298163336, 86.45724293864769550 ) ) ;
#108620=CARTESIAN_POINT ( 'NONE',  ( 21.52544592524344225, -5.823673210054117533, 38.54057627198103120 ) ) ;
#108622=CARTESIAN_POINT ( 'NONE',  ( 9.474510206698971260, -16.51473224551069308, 57.91557627198103120 ) ) ;
#108623=CARTESIAN_POINT ( 'NONE',  ( 16.53943276465976808, 0.05219959533934440121, 26.25109039468567573 ) ) ;
#108624=CARTESIAN_POINT ( 'NONE',  ( 13.97604488694548053, -13.89961937509957401, 70.62609039468567573 ) ) ;
#108625=CARTESIAN_POINT ( 'NONE',  ( -21.52544592524343514, 5.823673210054127303, 101.0405762719810383 ) ) ;
#108626=CARTESIAN_POINT ( 'NONE',  ( 4.483927247898545687, 16.52544592524342804, 29.79057627198102409 ) ) ;
#108627=CARTESIAN_POINT ( 'NONE',  ( -5.049401038298153566, 19.05341960407611168, 90.20724293864766707 ) ) ;
#108628=CARTESIAN_POINT ( 'NONE',  ( -21.53943276465977519, 0.05219959533907696930, 56.24890960531436690 ) ) ;
#108629=CARTESIAN_POINT ( 'NONE',  ( 5.719274019375991003, -21.55341960407610458, 92.70724293864770971 ) ) ;
#108630=CARTESIAN_POINT ( 'NONE',  ( -16.53943276465976808, -0.05219959533934237506, 33.75109039468568284 ) ) ;
#108631=CARTESIAN_POINT ( 'NONE',  ( -15.72974639402197994, 15.80617190586746368, 35.62390960531437401 ) ) ;
#108632=CARTESIAN_POINT ( 'NONE',  ( 21.53943276465977519, 0.05219959533937863772, 86.25109039468568994 ) ) ;
#108633=CARTESIAN_POINT ( 'NONE',  ( 9.474510206698971260, -16.51473224551069308, 92.91557627198103830 ) ) ;
#108634=CARTESIAN_POINT ( 'NONE',  ( 5.049401038298161559, -19.05341960407611168, 42.70724293864767418 ) ) ;
#108635=CARTESIAN_POINT ( 'NONE',  ( -16.51473224551069308, -9.474510206698971260, 96.66557627198102409 ) ) ;
#108636=CARTESIAN_POINT ( 'NONE',  ( 14.34966873604960469, 8.224510206698951720, 99.16557627198100988 ) ) ;
#108637=CARTESIAN_POINT ( 'NONE',  ( 19.03943276465977164, -0.05219959533909143690, 58.74890960531435979 ) ) ;
#108638=CARTESIAN_POINT ( 'NONE',  ( 13.89961937509957401, 13.97604488694547697, 111.8760903946856757 ) ) ;
#108640=EDGE_CURVE ( 'NONE', #53672, #71844, #103570, .T. ) ;
#108641=CARTESIAN_POINT ( 'NONE',  ( -21.55341960407619339, 5.719274019375674811, 103.5427570613523613 ) ) ;
#108642=CARTESIAN_POINT ( 'NONE',  ( 13.97604488694527802, 13.89961937509977652, 109.3739096053143669 ) ) ;
#108643=CARTESIAN_POINT ( 'NONE',  ( 16.53943276465976808, 0.05219959533934440121, 86.25109039468568994 ) ) ;
#108645=CARTESIAN_POINT ( 'NONE',  ( 0.05219959533936267826, -19.03943276465977164, 70.00109039468566152 ) ) ;
#108646=CARTESIAN_POINT ( 'NONE',  ( -13.97604488694547697, 13.89961937509957934, 33.12609039468566863 ) ) ;
#108648=CARTESIAN_POINT ( 'NONE',  ( -5.153800228976328057, -19.02544592524343514, 32.29057627198102409 ) ) ;
#108649=CARTESIAN_POINT ( 'NONE',  ( -8.314922557960811034, -14.29746914071050412, 32.08224293864769550 ) ) ;
#108650=CARTESIAN_POINT ( 'NONE',  ( -16.46253265017160317, 9.564922557960807481, 25.83224293864769194 ) ) ;
#108651=CARTESIAN_POINT ( 'NONE',  ( -4.483927247898539470, -16.52544592524342804, 22.29057627198102765 ) ) ;
#108652=CARTESIAN_POINT ( 'NONE',  ( 17.31728774477273092, 6.344390552232405334, 66.68093348310682700 ) ) ;
#108653=CARTESIAN_POINT ( 'NONE',  ( 14.34966873604972726, -8.224510206698740333, 90.83442372801901854 ) ) ;
#108654=CARTESIAN_POINT ( 'NONE',  ( -19.03943276465977164, 0.05219959533909376836, 31.24890960531435979 ) ) ;
#108655=CARTESIAN_POINT ( 'NONE',  ( -0.05219959533937732626, 21.53943276465977519, 112.5010903946857042 ) ) ;
#108656=CARTESIAN_POINT ( 'NONE',  ( -12.06949235617739369, -12.14591786802326823, 19.37609039468568639 ) ) ;
#108657=CARTESIAN_POINT ( 'NONE',  ( -21.52544592524334988, -5.823673210054445271, 83.95942372801900433 ) ) ;
#108658=CARTESIAN_POINT ( 'NONE',  ( -19.02544592524334988, -5.153800228976617603, 48.95942372801900433 ) ) ;
#108659=CARTESIAN_POINT ( 'NONE',  ( 16.51473224551069308, 9.474510206698969483, 89.16557627198103830 ) ) ;
#108660=CARTESIAN_POINT ( 'NONE',  ( -16.46253265017160317, 9.564922557960807481, 75.83224293864769550 ) ) ;
#108661=CARTESIAN_POINT ( 'NONE',  ( -19.52217212775656563, 5.500000000000114575, 39.93993709005260939 ) ) ;
#108662=CARTESIAN_POINT ( 'NONE',  ( -5.823673210054116645, -21.52544592524344225, 92.29057627198103830 ) ) ;
#108664=CARTESIAN_POINT ( 'NONE',  ( 12.14591786802309770, 12.06949235617756955, 69.37390960531436690 ) ) ;
#108665=CARTESIAN_POINT ( 'NONE',  ( -15.72974639402197994, 15.80617190586746368, 65.62390960531436690 ) ) ;
#108666=CARTESIAN_POINT ( 'NONE',  ( 19.05341960407611168, 5.049401038298154454, 53.95724293864770260 ) ) ;
#108667=CARTESIAN_POINT ( 'NONE',  ( -18.62759615963270932, 10.81492255796079327, 85.83224293864768129 ) ) ;
#108668=CARTESIAN_POINT ( 'NONE',  ( -8.314922557961024197, 14.29746914071037800, 72.91775706135234714 ) ) ;
#108670=CARTESIAN_POINT ( 'NONE',  ( 0.05219959533909260263, 19.03943276465977164, 49.99890960531435979 ) ) ;
#108671=CARTESIAN_POINT ( 'NONE',  ( 16.52544592524342804, -4.483927247898539470, 83.54057627198102409 ) ) ;
#108673=CARTESIAN_POINT ( 'NONE',  ( -19.03943276465977164, 0.05219959533909376836, 51.24890960531436690 ) ) ;
#108674=CARTESIAN_POINT ( 'NONE',  ( 12.06949235617757843, -12.14591786802309237, 113.1239096053143953 ) ) ;
#108675=CARTESIAN_POINT ( 'NONE',  ( 16.51473224551083163, -9.474510206698727899, 60.83442372801900433 ) ) ;
#108676=CARTESIAN_POINT ( 'NONE',  ( 0.05219959533910956823, 16.53943276465976808, 79.99890960531435269 ) ) ;
#108677=CARTESIAN_POINT ( 'NONE',  ( -18.67979575497193778, 10.72451020669871902, 43.33442372801901143 ) ) ;
#108678=CARTESIAN_POINT ( 'NONE',  ( 13.89961937509977652, -13.97604488694527269, 38.12390960531436690 ) ) ;
#108679=CARTESIAN_POINT ( 'NONE',  ( -5.719274019375978568, 21.55341960407610458, 100.2072429386476955 ) ) ;
#108680=CARTESIAN_POINT ( 'NONE',  ( -0.05219959533910754901, -16.53943276465976808, 92.49890960531436690 ) ) ;
#108682=CARTESIAN_POINT ( 'NONE',  ( 9.564922557960805705, 16.46253265017160317, 49.58224293864770260 ) ) ;
#108684=CARTESIAN_POINT ( 'NONE',  ( 19.05341960407617918, -5.049401038297876454, 101.0427570613523045 ) ) ;
#108685=CARTESIAN_POINT ( 'NONE',  ( 9.564922557960805705, 16.46253265017160317, 94.58224293864769550 ) ) ;
#108686=CARTESIAN_POINT ( 'NONE',  ( 18.62759615963255655, 10.81492255796105972, 36.66775706135234714 ) ) ;
#108687=CARTESIAN_POINT ( 'NONE',  ( -0.05219959533909027116, -19.03943276465977164, 87.49890960531436690 ) ) ;
#108688=CARTESIAN_POINT ( 'NONE',  ( -9.564922557961040184, 16.46253265017147172, 67.91775706135233293 ) ) ;
#108689=CARTESIAN_POINT ( 'NONE',  ( 0.05219959533909260263, 19.03943276465977164, 44.99890960531435979 ) ) ;
#108690=CARTESIAN_POINT ( 'NONE',  ( -4.483927247898539470, -16.52544592524342804, 72.29057627198102409 ) ) ;
#108691=CARTESIAN_POINT ( 'NONE',  ( 14.29746914071049879, -8.314922557960816363, 73.33224293864769550 ) ) ;
#108692=CARTESIAN_POINT ( 'NONE',  ( 5.153800228976335163, 19.02544592524342804, 89.79057627198102409 ) ) ;
#108693=CARTESIAN_POINT ( 'NONE',  ( 15.72974639402199770, -15.80617190586745480, 98.12390960531436690 ) ) ;
#108694=CARTESIAN_POINT ( 'NONE',  ( 19.03943276465977164, -0.05219959533909143690, 78.74890960531436690 ) ) ;
#108695=CARTESIAN_POINT ( 'NONE',  ( 9.564922557961047289, -16.46253265017146816, 30.41775706135232937 ) ) ;
#108696=CARTESIAN_POINT ( 'NONE',  ( 5.153800228976335163, 19.02544592524342804, 39.79057627198100988 ) ) ;
#108697=CARTESIAN_POINT ( 'NONE',  ( -12.06949235617756955, 12.14591786802309770, 25.62390960531435624 ) ) ;
#108698=CARTESIAN_POINT ( 'NONE',  ( 16.53943276465976808, -0.05219959533910856209, 113.7489096053143527 ) ) ;
#108699=CARTESIAN_POINT ( 'NONE',  ( 13.97604488694548053, -13.89961937509957401, 105.6260903946856757 ) ) ;
#108701=CARTESIAN_POINT ( 'NONE',  ( -5.719274019375665041, -21.55341960407619695, 29.79275706135234358 ) ) ;
#108702=CARTESIAN_POINT ( 'NONE',  ( -13.89961937509957401, -13.97604488694547875, 69.37609039468564731 ) ) ;
#108703=CARTESIAN_POINT ( 'NONE',  ( 8.224510206698953496, -14.34966873604960469, 22.91557627198102765 ) ) ;
#108704=CARTESIAN_POINT ( 'NONE',  ( 18.62759615963271287, -10.81492255796078972, 88.33224293864769550 ) ) ;
#108705=CARTESIAN_POINT ( 'NONE',  ( 16.46253265017160672, -9.564922557960803928, 113.3322429386476955 ) ) ;
#108706=CARTESIAN_POINT ( 'NONE',  ( 16.53943276465976808, -0.05219959533910856209, 63.74890960531435979 ) ) ;
#108707=CARTESIAN_POINT ( 'NONE',  ( 9.474510206698971260, -16.51473224551069308, 32.91557627198102409 ) ) ;
#108708=CARTESIAN_POINT ( 'NONE',  ( 5.049401038297881783, 19.05341960407617563, 27.29275706135232937 ) ) ;
#108709=CARTESIAN_POINT ( 'NONE',  ( 0.05219959533934541429, -16.53943276465976808, 85.00109039468568994 ) ) ;
#108710=CARTESIAN_POINT ( 'NONE',  ( -12.06949235617739369, -12.14591786802326823, 59.37609039468568284 ) ) ;
#108711=CARTESIAN_POINT ( 'NONE',  ( 19.02544592524343514, -5.153800228976328945, 113.5405762719810241 ) ) ;
#108712=CARTESIAN_POINT ( 'NONE',  ( 5.823673210054444382, -21.52544592524334988, 110.2094237280190185 ) ) ;
#108713=CARTESIAN_POINT ( 'NONE',  ( -9.564922557960796823, -16.46253265017161027, 82.08224293864768129 ) ) ;
#108715=CARTESIAN_POINT ( 'NONE',  ( 8.224510206698742110, 14.34966873604972548, 62.08442372801901143 ) ) ;
#108716=CARTESIAN_POINT ( 'NONE',  ( 13.89961937509977652, -13.97604488694527269, 28.12390960531435624 ) ) ;
#108718=CARTESIAN_POINT ( 'NONE',  ( 4.483927247898545687, 16.52544592524342804, 34.79057627198103120 ) ) ;
#108720=CARTESIAN_POINT ( 'NONE',  ( -21.53943276465977519, -0.05219959533937600094, 63.75109039468568284 ) ) ;
#108721=CARTESIAN_POINT ( 'NONE',  ( 9.564922557960805705, 16.46253265017160317, 109.5822429386476955 ) ) ;
#108722=CARTESIAN_POINT ( 'NONE',  ( 19.03943276465977164, -0.05219959533909143690, 73.74890960531435269 ) ) ;
#108723=CARTESIAN_POINT ( 'NONE',  ( -9.474510206698964154, 16.51473224551069663, 110.4155762719810383 ) ) ;
#108724=CARTESIAN_POINT ( 'NONE',  ( 0.05219959533910956823, 16.53943276465976808, 54.99890960531435269 ) ) ;
#108725=CARTESIAN_POINT ( 'NONE',  ( 4.379528057220339221, -16.55341960407611168, 32.70724293864770260 ) ) ;
#108726=CARTESIAN_POINT ( 'NONE',  ( -12.14591786802309592, -12.06949235617757132, 56.87390960531436690 ) ) ;
#108727=CARTESIAN_POINT ( 'NONE',  ( -0.05219959533934338120, 16.53943276465976808, 42.50109039468567573 ) ) ;
#108729=CARTESIAN_POINT ( 'NONE',  ( 19.02544592524334988, 5.153800228976608722, 51.45942372801900433 ) ) ;
#108730=CARTESIAN_POINT ( 'NONE',  ( -13.89961937509977652, 13.97604488694528158, 70.62390960531432427 ) ) ;
#108731=CARTESIAN_POINT ( 'NONE',  ( -9.564922557961040184, 16.46253265017147172, 47.91775706135233293 ) ) ;
#108732=CARTESIAN_POINT ( 'NONE',  ( -0.05219959533936034679, 19.03943276465977164, 62.50109039468566863 ) ) ;
#108733=CARTESIAN_POINT ( 'NONE',  ( -13.89961937509957401, -13.97604488694547875, 104.3760903946856757 ) ) ;
#108734=CARTESIAN_POINT ( 'NONE',  ( 8.224510206698742110, 14.34966873604972548, 87.08442372801901854 ) ) ;
#108736=CARTESIAN_POINT ( 'NONE',  ( -13.89961937509977652, 13.97604488694528158, 30.62390960531435269 ) ) ;
#108738=CARTESIAN_POINT ( 'NONE',  ( -13.97604488694527625, -13.89961937509977652, 106.8739096053143669 ) ) ;
#108739=CARTESIAN_POINT ( 'NONE',  ( 10.72451020669871369, 18.67979575497193778, 42.08442372801901854 ) ) ;
#108740=CARTESIAN_POINT ( 'NONE',  ( -9.474510206698720793, -16.51473224551083518, 104.5844237280190043 ) ) ;
#108741=CARTESIAN_POINT ( 'NONE',  ( 17.50000000000000000, -5.068104630630386964, 108.2281840534002697 ) ) ;
#108742=CARTESIAN_POINT ( 'NONE',  ( -19.05341960407611168, -5.049401038298163336, 66.45724293864769550 ) ) ;
#108743=CARTESIAN_POINT ( 'NONE',  ( 9.564922557960805705, 16.46253265017160317, 109.5822429386476955 ) ) ;
#108744=CARTESIAN_POINT ( 'NONE',  ( 16.52544592524342804, -4.483927247898539470, 58.54057627198103120 ) ) ;
#108745=CARTESIAN_POINT ( 'NONE',  ( 19.05341960407611168, 5.049401038298154454, 58.95724293864768129 ) ) ;
#108746=CARTESIAN_POINT ( 'NONE',  ( -0.05219959533909027116, -19.03943276465977164, 57.49890960531435979 ) ) ;
#108747=CARTESIAN_POINT ( 'NONE',  ( -5.153800228976607833, 19.02544592524334988, 77.70942372801900433 ) ) ;
#108748=CARTESIAN_POINT ( 'NONE',  ( 21.55341960407610458, 5.719274019375980345, 48.95724293864770971 ) ) ;
#108749=CARTESIAN_POINT ( 'NONE',  ( -16.46253265017146816, -9.564922557961047289, 44.16775706135232582 ) ) ;
#108750=CARTESIAN_POINT ( 'NONE',  ( 16.46253265017160672, -9.564922557960803928, 83.33224293864768129 ) ) ;
#108751=CARTESIAN_POINT ( 'NONE',  ( -10.81492255796078084, -18.62759615963271287, 77.08224293864769550 ) ) ;
#108752=CARTESIAN_POINT ( 'NONE',  ( -16.52544592524342804, 4.483927247898546575, 86.04057627198102409 ) ) ;
#108753=CARTESIAN_POINT ( 'NONE',  ( 0.05219959533936267826, -19.03943276465977164, 40.00109039468566152 ) ) ;
#108754=CARTESIAN_POINT ( 'NONE',  ( -5.823673210054116645, -21.52544592524344225, 47.29057627198103120 ) ) ;
#108755=CARTESIAN_POINT ( 'NONE',  ( 21.55341960407610458, 5.719274019375980345, 38.95724293864768839 ) ) ;
#108756=CARTESIAN_POINT ( 'NONE',  ( 5.049401038298161559, -19.05341960407611168, 62.70724293864769550 ) ) ;
#108757=CARTESIAN_POINT ( 'NONE',  ( 13.89961937509977652, -13.97604488694527269, 48.12390960531435979 ) ) ;
#108758=CARTESIAN_POINT ( 'NONE',  ( -16.51473224551069308, -9.474510206698971260, 21.66557627198102765 ) ) ;
#108759=CARTESIAN_POINT ( 'NONE',  ( -18.67979575497193778, 10.72451020669871902, 28.33442372801902209 ) ) ;
#108760=CARTESIAN_POINT ( 'NONE',  ( -19.02544592524342804, 5.153800228976336051, 111.0405762719810099 ) ) ;
#108761=CARTESIAN_POINT ( 'NONE',  ( -15.80617190586768217, 15.72974639402176855, 38.12609039468567573 ) ) ;
#108762=CARTESIAN_POINT ( 'NONE',  ( -19.03943276465977164, 0.05219959533909376836, 36.24890960531436690 ) ) ;
#108763=CARTESIAN_POINT ( 'NONE',  ( 10.72451020669898902, -18.67979575497178502, 112.9155762719810383 ) ) ;
#108764=CARTESIAN_POINT ( 'NONE',  ( 19.02544592524334988, 5.153800228976608722, 41.45942372801900433 ) ) ;
#108766=CARTESIAN_POINT ( 'NONE',  ( 13.89961937509977652, -13.97604488694527269, 23.12390960531436335 ) ) ;
#108767=CARTESIAN_POINT ( 'NONE',  ( 4.483927247898790824, -16.52544592524335698, 55.20942372801902565 ) ) ;
#108768=CARTESIAN_POINT ( 'NONE',  ( 19.05341960407611168, 5.049401038298154454, 28.95724293864769550 ) ) ;
#108770=CARTESIAN_POINT ( 'NONE',  ( 5.049401038298161559, -19.05341960407611168, 77.70724293864765286 ) ) ;
#108771=CARTESIAN_POINT ( 'NONE',  ( 16.52544592524342804, -4.483927247898539470, 113.5405762719810383 ) ) ;
#108772=CARTESIAN_POINT ( 'NONE',  ( -21.52544592524343514, 5.823673210054127303, 61.04057627198103120 ) ) ;
#108773=CARTESIAN_POINT ( 'NONE',  ( -12.14591786802309592, -12.06949235617757132, 76.87390960531439532 ) ) ;
#108774=CARTESIAN_POINT ( 'NONE',  ( 16.52544592524335698, 4.483927247898782831, 36.45942372801901143 ) ) ;
#108775=CARTESIAN_POINT ( 'NONE',  ( -5.823673210054431948, 21.52544592524334988, 92.70942372801901854 ) ) ;
#108777=CARTESIAN_POINT ( 'NONE',  ( 12.14591786802327356, -12.06949235617739191, 105.6260903946856899 ) ) ;
#108778=CARTESIAN_POINT ( 'NONE',  ( 12.06949235617757843, -12.14591786802309237, 48.12390960531436690 ) ) ;
#108779=CARTESIAN_POINT ( 'NONE',  ( -13.89961937509977652, 13.97604488694528158, 50.62390960531435979 ) ) ;
#108780=CARTESIAN_POINT ( 'NONE',  ( -5.719274019375665041, -21.55341960407619695, 89.79275706135236135 ) ) ;
#108781=CARTESIAN_POINT ( 'NONE',  ( 10.81492255796078972, 18.62759615963270932, 104.5822429386477097 ) ) ;
#108782=CARTESIAN_POINT ( 'NONE',  ( 18.67979575497194134, -10.72451020669871369, 75.83442372801900433 ) ) ;
#108783=CARTESIAN_POINT ( 'NONE',  ( -14.34966873604972548, 8.224510206698743886, 58.33442372801901143 ) ) ;
#108784=CARTESIAN_POINT ( 'NONE',  ( 8.224510206698953496, -14.34966873604960469, 82.91557627198103830 ) ) ;
#108785=CARTESIAN_POINT ( 'NONE',  ( 18.67979575497194134, -10.72451020669871369, 90.83442372801901854 ) ) ;
#108786=CARTESIAN_POINT ( 'NONE',  ( -8.314922557961024197, 14.29746914071037800, 107.9177570613523471 ) ) ;
#108787=CARTESIAN_POINT ( 'NONE',  ( -16.38665767535054840, 7.295008042176092111, 115.2640086421455408 ) ) ;
#108788=CARTESIAN_POINT ( 'NONE',  ( 0.05219959533934541429, -16.53943276465976808, 45.00109039468568284 ) ) ;
#108789=CARTESIAN_POINT ( 'NONE',  ( -14.34966873604960291, -8.224510206698953496, 36.66557627198103120 ) ) ;
#108790=CARTESIAN_POINT ( 'NONE',  ( 8.314922557961029526, -14.29746914071037800, 80.41775706135234714 ) ) ;
#108791=CARTESIAN_POINT ( 'NONE',  ( -19.02544592524342804, 5.153800228976336051, 101.0405762719810241 ) ) ;
#108792=CARTESIAN_POINT ( 'NONE',  ( -5.719274019375978568, 21.55341960407610458, 25.20724293864769550 ) ) ;
#108793=CARTESIAN_POINT ( 'NONE',  ( 0.05219959533937995610, -21.53943276465977519, 95.00109039468568994 ) ) ;
#108794=CARTESIAN_POINT ( 'NONE',  ( 16.55341960407618274, -4.379528057220086978, 96.04275706135236135 ) ) ;
#108795=CARTESIAN_POINT ( 'NONE',  ( 12.14591786802309770, 12.06949235617756955, 69.37390960531436690 ) ) ;
#108796=CARTESIAN_POINT ( 'NONE',  ( 19.03943276465977164, -0.05219959533909143690, 83.74890960531436690 ) ) ;
#108798=CARTESIAN_POINT ( 'NONE',  ( -16.53943276465976808, -0.05219959533934237506, 23.75109039468567929 ) ) ;
#108799=CARTESIAN_POINT ( 'NONE',  ( 19.05341960407611168, 5.049401038298154454, 28.95724293864769550 ) ) ;
#108800=CARTESIAN_POINT ( 'NONE',  ( -16.46253265017160317, 9.564922557960807481, 85.83224293864769550 ) ) ;
#108801=CARTESIAN_POINT ( 'NONE',  ( -14.34966873604972548, 8.224510206698743886, 28.33442372801902209 ) ) ;
#108803=CARTESIAN_POINT ( 'NONE',  ( -19.03943276465977164, -0.05219959533935918106, 33.75109039468566863 ) ) ;
#108804=CARTESIAN_POINT ( 'NONE',  ( -16.52544592524335698, -4.483927247898792601, 98.95942372801903275 ) ) ;
#108805=CARTESIAN_POINT ( 'NONE',  ( 5.153800228976335163, 19.02544592524342804, 29.79057627198102409 ) ) ;
#108806=CARTESIAN_POINT ( 'NONE',  ( -14.34966873604972548, 8.224510206698743886, 73.33442372801901854 ) ) ;
#108807=CARTESIAN_POINT ( 'NONE',  ( 14.34966873604972726, -8.224510206698740333, 70.83442372801901854 ) ) ;
#108808=CARTESIAN_POINT ( 'NONE',  ( -16.51473224551082808, 9.474510206698731452, 78.33442372801900433 ) ) ;
#108809=CARTESIAN_POINT ( 'NONE',  ( -18.67979575497193778, 10.72451020669871902, 108.3344237280190185 ) ) ;
#108810=CARTESIAN_POINT ( 'NONE',  ( -0.05219959533909027116, -19.03943276465977164, 47.49890960531435979 ) ) ;
#108811=CARTESIAN_POINT ( 'NONE',  ( -19.02544592524342804, 5.153800228976336051, 86.04057627198103830 ) ) ;
#108812=CARTESIAN_POINT ( 'NONE',  ( -16.52544592524342804, 4.483927247898546575, 91.04057627198103830 ) ) ;
#108814=CARTESIAN_POINT ( 'NONE',  ( 16.51473224551083163, -9.474510206698727899, 60.83442372801900433 ) ) ;
#108815=CARTESIAN_POINT ( 'NONE',  ( 5.823673210054125526, 21.52544592524343514, 44.79057627198103120 ) ) ;
#108816=CARTESIAN_POINT ( 'NONE',  ( -19.02544592524334988, -5.153800228976617603, 28.95942372801900433 ) ) ;
#108817=CARTESIAN_POINT ( 'NONE',  ( -13.89961937509977652, 13.97604488694528158, 85.62390960531433848 ) ) ;
#108818=CARTESIAN_POINT ( 'NONE',  ( 18.67979575497178502, 10.72451020669898547, 79.16557627198103830 ) ) ;
#108819=CARTESIAN_POINT ( 'NONE',  ( -5.049401038298153566, 19.05341960407611168, 115.2072429386477097 ) ) ;
#108820=CARTESIAN_POINT ( 'NONE',  ( -0.05219959533936034679, 19.03943276465977164, 92.50109039468566152 ) ) ;
#108821=CARTESIAN_POINT ( 'NONE',  ( -17.49999999999999645, 3.305555262949665618, 109.6251715215659317 ) ) ;
#108822=CARTESIAN_POINT ( 'NONE',  ( -5.153800228976607833, 19.02544592524334988, 107.7094237280189759 ) ) ;
#108823=CARTESIAN_POINT ( 'NONE',  ( 9.564922557960805705, 16.46253265017160317, 29.58224293864769550 ) ) ;
#108824=CARTESIAN_POINT ( 'NONE',  ( 19.05341960407611168, 5.049401038298154454, 103.9572429386476671 ) ) ;
#108825=CARTESIAN_POINT ( 'NONE',  ( -15.72974639402197994, 15.80617190586746368, 70.62390960531436690 ) ) ;
#108826=CARTESIAN_POINT ( 'NONE',  ( 14.34966873604972726, -8.224510206698740333, 45.83442372801901854 ) ) ;
#108827=CARTESIAN_POINT ( 'NONE',  ( -21.53943276465977519, -0.05219959533937600094, 48.75109039468568284 ) ) ;
#108828=CARTESIAN_POINT ( 'NONE',  ( 5.049401038297881783, 19.05341960407617563, 87.29275706135234714 ) ) ;
#108829=CARTESIAN_POINT ( 'NONE',  ( 21.55341960407619695, -5.719274019375665929, 101.0427570613523756 ) ) ;
#108830=CARTESIAN_POINT ( 'NONE',  ( 8.314922557961029526, -14.29746914071037800, 110.4177570613523756 ) ) ;
#108831=CARTESIAN_POINT ( 'NONE',  ( -5.153800228976328057, -19.02544592524343514, 107.2905762719810383 ) ) ;
#108832=CARTESIAN_POINT ( 'NONE',  ( -8.224510206698948167, 14.34966873604960824, 90.41557627198103830 ) ) ;
#108833=CARTESIAN_POINT ( 'NONE',  ( 12.14591786802309770, 12.06949235617756955, 34.37390960531435979 ) ) ;
#108834=CARTESIAN_POINT ( 'NONE',  ( -13.89961937509957401, -13.97604488694547875, 69.37609039468564731 ) ) ;
#108835=CARTESIAN_POINT ( 'NONE',  ( -21.55341960407619339, 5.719274019375674811, 58.54275706135235424 ) ) ;
#108836=CARTESIAN_POINT ( 'NONE',  ( -13.89961937509957401, -13.97604488694547875, 29.37609039468565797 ) ) ;
#108837=CARTESIAN_POINT ( 'NONE',  ( -16.52544592524342804, 4.483927247898546575, 106.0405762719810525 ) ) ;
#108838=CARTESIAN_POINT ( 'NONE',  ( 21.55341960407610458, 5.719274019375980345, 33.95724293864769550 ) ) ;
#108839=CARTESIAN_POINT ( 'NONE',  ( 8.224510206698953496, -14.34966873604960469, 27.91557627198103830 ) ) ;
#108840=CARTESIAN_POINT ( 'NONE',  ( 18.62759615963255655, 10.81492255796105972, 101.6677570613523613 ) ) ;
#108841=CARTESIAN_POINT ( 'NONE',  ( 8.224510206698742110, 14.34966873604972548, 57.08442372801901854 ) ) ;
#108842=CARTESIAN_POINT ( 'NONE',  ( -14.34966873604960291, -8.224510206698953496, 31.66557627198102054 ) ) ;
#108843=CARTESIAN_POINT ( 'NONE',  ( -21.53943276465977519, -0.05219959533937600094, 63.75109039468568284 ) ) ;
#108844=CARTESIAN_POINT ( 'NONE',  ( -21.52544592524334988, -5.823673210054445271, 58.95942372801902565 ) ) ;
#108847=CARTESIAN_POINT ( 'NONE',  ( -0.05219959533937732626, 21.53943276465977519, 27.50109039468567929 ) ) ;
#108848=CARTESIAN_POINT ( 'NONE',  ( 0.05219959533910956823, 16.53943276465976808, 109.9989096053143527 ) ) ;
#108849=CARTESIAN_POINT ( 'NONE',  ( -13.89961937509977652, 13.97604488694528158, 25.62390960531434558 ) ) ;
#108850=CARTESIAN_POINT ( 'NONE',  ( -14.29746914071049879, 8.314922557960819915, 80.83224293864769550 ) ) ;
#108851=CARTESIAN_POINT ( 'NONE',  ( -9.564922557960796823, -16.46253265017161027, 67.08224293864769550 ) ) ;
#108852=CARTESIAN_POINT ( 'NONE',  ( 4.379528057220339221, -16.55341960407611168, 22.70724293864769194 ) ) ;
#108853=CARTESIAN_POINT ( 'NONE',  ( 5.823673210054125526, 21.52544592524343514, 49.79057627198102409 ) ) ;
#108854=CARTESIAN_POINT ( 'NONE',  ( 8.314922557960818139, 14.29746914071049879, 94.58224293864769550 ) ) ;
#108856=CARTESIAN_POINT ( 'NONE',  ( 15.80617190586746368, 15.72974639402197994, 99.37390960531436690 ) ) ;
#108857=CARTESIAN_POINT ( 'NONE',  ( -9.564922557960796823, -16.46253265017161027, 107.0822429386476955 ) ) ;
#108858=CARTESIAN_POINT ( 'NONE',  ( 9.474510206698971260, -16.51473224551069308, 52.91557627198102409 ) ) ;
#108859=CARTESIAN_POINT ( 'NONE',  ( -5.153800228976607833, 19.02544592524334988, 107.7094237280189759 ) ) ;
#108860=CARTESIAN_POINT ( 'NONE',  ( -10.72451020669898014, 18.67979575497178502, 50.41557627198103120 ) ) ;
#108861=CARTESIAN_POINT ( 'NONE',  ( 10.72451020669871369, 18.67979575497193778, 67.08442372801901854 ) ) ;
#108862=CARTESIAN_POINT ( 'NONE',  ( 13.89961937509977652, -13.97604488694527269, 63.12390960531435979 ) ) ;
#108863=CARTESIAN_POINT ( 'NONE',  ( -13.89961937509977652, 13.97604488694528158, 95.62390960531436690 ) ) ;
#108864=CARTESIAN_POINT ( 'NONE',  ( 16.53943276465976808, 0.05219959533934440121, 61.25109039468567573 ) ) ;
#108865=CARTESIAN_POINT ( 'NONE',  ( 15.72974639402176855, 15.80617190586768217, 56.87609039468568994 ) ) ;
#108866=CARTESIAN_POINT ( 'NONE',  ( -21.53943276465977519, -0.05219959533937600094, 88.75109039468567573 ) ) ;
#108867=CARTESIAN_POINT ( 'NONE',  ( -15.80617190586745835, -15.72974639402198527, 96.87390960531436690 ) ) ;
#108868=CARTESIAN_POINT ( 'NONE',  ( -18.67979575497193778, 10.72451020669871902, 38.33442372801900433 ) ) ;
#108869=CARTESIAN_POINT ( 'NONE',  ( -12.06949235617739369, -12.14591786802326823, 74.37609039468568994 ) ) ;
#108870=CARTESIAN_POINT ( 'NONE',  ( 5.719274019375991003, -21.55341960407610458, 82.70724293864770971 ) ) ;
#108871=CARTESIAN_POINT ( 'NONE',  ( 19.03943276465977164, 0.05219959533936151252, 31.25109039468566863 ) ) ;
#108872=CARTESIAN_POINT ( 'NONE',  ( 19.03943276465977164, -0.05219959533909143690, 83.74890960531436690 ) ) ;
#108873=CARTESIAN_POINT ( 'NONE',  ( -4.483927247898539470, -16.52544592524342804, 27.29057627198103120 ) ) ;
#108875=CARTESIAN_POINT ( 'NONE',  ( -19.02544592524342804, 5.153800228976336051, 101.0405762719810241 ) ) ;
#108877=ADVANCED_FACE ( 'NONE', ( #81627 ), #11577, .F. ) ;
#108878=CARTESIAN_POINT ( 'NONE',  ( -19.03943276465977164, -0.05219959533935918106, 93.75109039468566152 ) ) ;
#108879=CARTESIAN_POINT ( 'NONE',  ( 10.72451020669898902, -18.67979575497178502, 72.91557627198103830 ) ) ;
#108880=CARTESIAN_POINT ( 'NONE',  ( -16.53943276465976808, 0.05219959533911058130, 41.24890960531435269 ) ) ;
#108881=CARTESIAN_POINT ( 'NONE',  ( -5.153800228976607833, 19.02544592524334988, 107.7094237280189759 ) ) ;
#108882=CARTESIAN_POINT ( 'NONE',  ( 16.46253265017160672, -9.564922557960803928, 33.33224293864770260 ) ) ;
#108883=CARTESIAN_POINT ( 'NONE',  ( -9.474510206698720793, -16.51473224551083518, 104.5844237280190043 ) ) ;
#108884=CARTESIAN_POINT ( 'NONE',  ( -21.55341960407610458, -5.719274019375992779, 101.4572429386476955 ) ) ;
#108885=CARTESIAN_POINT ( 'NONE',  ( 16.51473224551083163, -9.474510206698727899, 70.83442372801900433 ) ) ;
#108886=CARTESIAN_POINT ( 'NONE',  ( 16.53943276465976808, 0.05219959533934440121, 81.25109039468568994 ) ) ;
#108887=CARTESIAN_POINT ( 'NONE',  ( -5.153800228976328057, -19.02544592524343514, 67.29057627198102409 ) ) ;
#108888=CARTESIAN_POINT ( 'NONE',  ( 12.06949235617757843, -12.14591786802309237, 83.12390960531436690 ) ) ;
#108889=CARTESIAN_POINT ( 'NONE',  ( 9.474510206698971260, -16.51473224551069308, 62.91557627198102409 ) ) ;
#108890=CARTESIAN_POINT ( 'NONE',  ( 4.379528057220339221, -16.55341960407611168, 62.70724293864769550 ) ) ;
#108891=CARTESIAN_POINT ( 'NONE',  ( -15.49999999999999822, -7.500000000000000888, 118.0000000000000142 ) ) ;
#108893=CARTESIAN_POINT ( 'NONE',  ( 0.05219959533910956823, 16.53943276465976808, 39.99890960531436690 ) ) ;
#108894=CARTESIAN_POINT ( 'NONE',  ( -9.564922557960796823, -16.46253265017161027, 72.08224293864770971 ) ) ;
#108895=LINE ( 'NONE', #184748, #189690 ) ;
#108896=CARTESIAN_POINT ( 'NONE',  ( -19.05341960407617563, 5.049401038297882671, 58.54275706135234003 ) ) ;
#108897=CARTESIAN_POINT ( 'NONE',  ( 8.314922557961029526, -14.29746914071037800, 60.41775706135235424 ) ) ;
#108898=CARTESIAN_POINT ( 'NONE',  ( 5.823673210054125526, 21.52544592524343514, 64.79057627198103830 ) ) ;
#108899=CARTESIAN_POINT ( 'NONE',  ( -13.97604488694547697, 13.89961937509957934, 28.12609039468565797 ) ) ;
#108900=CARTESIAN_POINT ( 'NONE',  ( -9.564922557960796823, -16.46253265017161027, 82.08224293864768129 ) ) ;
#108902=CARTESIAN_POINT ( 'NONE',  ( -5.153800228976328057, -19.02544592524343514, 107.2905762719810383 ) ) ;
#108903=CARTESIAN_POINT ( 'NONE',  ( 9.474510206698971260, -16.51473224551069308, 57.91557627198103120 ) ) ;
#108904=CARTESIAN_POINT ( 'NONE',  ( 21.55341960407619695, -5.719274019375665929, 41.04275706135236135 ) ) ;
#108905=CARTESIAN_POINT ( 'NONE',  ( -8.224510206698948167, 14.34966873604960824, 100.4155762719810241 ) ) ;
#108906=CARTESIAN_POINT ( 'NONE',  ( -21.55341960407610458, -5.719274019375992779, 101.4572429386476955 ) ) ;
#108907=CARTESIAN_POINT ( 'NONE',  ( -9.564922557960796823, -16.46253265017161027, 92.08224293864769550 ) ) ;
#108909=CARTESIAN_POINT ( 'NONE',  ( -5.719274019375665041, -21.55341960407619695, 29.79275706135234358 ) ) ;
#108910=ORIENTED_EDGE ( 'NONE', *, *, #96536, .F. ) ;
#108911=CARTESIAN_POINT ( 'NONE',  ( 13.97604488694527802, 13.89961937509977652, 84.37390960531433848 ) ) ;
#108913=CARTESIAN_POINT ( 'NONE',  ( 21.55341960407610458, 5.719274019375980345, 98.95724293864770971 ) ) ;
#108914=CARTESIAN_POINT ( 'NONE',  ( -0.05219959533909027116, -19.03943276465977164, 52.49890960531436690 ) ) ;
#108915=CARTESIAN_POINT ( 'NONE',  ( 13.89961937509957401, 13.97604488694547697, 106.8760903946856757 ) ) ;
#108917=CARTESIAN_POINT ( 'NONE',  ( 5.153800228976335163, 19.02544592524342804, 29.79057627198102409 ) ) ;
#108918=CARTESIAN_POINT ( 'NONE',  ( -21.55341960407619339, 5.719274019375674811, 83.54275706135234714 ) ) ;
#108919=CARTESIAN_POINT ( 'NONE',  ( 19.05341960407611168, 5.049401038298154454, 78.95724293864769550 ) ) ;
#108920=CARTESIAN_POINT ( 'NONE',  ( 0.05219959533937995610, -21.53943276465977519, 45.00109039468568284 ) ) ;
#108921=CARTESIAN_POINT ( 'NONE',  ( 5.823673210054444382, -21.52544592524334988, 25.20942372801901854 ) ) ;
#108923=CARTESIAN_POINT ( 'NONE',  ( 16.46253265017160672, -9.564922557960803928, 98.33224293864769550 ) ) ;
#108924=CARTESIAN_POINT ( 'NONE',  ( 19.01529144963331674, 5.500000000000158096, 63.73431955728439391 ) ) ;
#108925=CARTESIAN_POINT ( 'NONE',  ( -16.53943276465976808, -0.05219959533934237506, 43.75109039468568284 ) ) ;
#108926=CARTESIAN_POINT ( 'NONE',  ( 21.52544592524344225, -5.823673210054117533, 43.54057627198103830 ) ) ;
#108927=CARTESIAN_POINT ( 'NONE',  ( -18.62759615963255300, -10.81492255796106328, 49.16775706135234003 ) ) ;
#108928=CARTESIAN_POINT ( 'NONE',  ( 5.823673210054444382, -21.52544592524334988, 75.20942372801901854 ) ) ;
#108930=CARTESIAN_POINT ( 'NONE',  ( -16.51473224551082808, 9.474510206698731452, 113.3344237280190043 ) ) ;
#108931=CARTESIAN_POINT ( 'NONE',  ( 19.05341960407611168, 5.049401038298154454, 63.95724293864769550 ) ) ;
#108932=CARTESIAN_POINT ( 'NONE',  ( 16.46253265017160672, -9.564922557960803928, 103.3322429386476955 ) ) ;
#108933=CARTESIAN_POINT ( 'NONE',  ( 14.29746914071049879, -8.314922557960816363, 113.3322429386476955 ) ) ;
#108934=CARTESIAN_POINT ( 'NONE',  ( -8.314922557960811034, -14.29746914071050412, 107.0822429386476955 ) ) ;
#108935=CARTESIAN_POINT ( 'NONE',  ( -15.80617190586745835, -15.72974639402198527, 31.87390960531435979 ) ) ;
#108936=CARTESIAN_POINT ( 'NONE',  ( 8.314922557961029526, -14.29746914071037800, 80.41775706135234714 ) ) ;
#108937=CARTESIAN_POINT ( 'NONE',  ( -4.379528057220328563, 16.55341960407611168, 75.20724293864769550 ) ) ;
#108938=CARTESIAN_POINT ( 'NONE',  ( 16.51473224551069308, 9.474510206698969483, 54.16557627198103120 ) ) ;
#108939=CARTESIAN_POINT ( 'NONE',  ( 18.62759615963255655, 10.81492255796105972, 76.66775706135234714 ) ) ;
#108940=CARTESIAN_POINT ( 'NONE',  ( -0.05219959533937732626, 21.53943276465977519, 77.50109039468567573 ) ) ;
#108941=CARTESIAN_POINT ( 'NONE',  ( -13.97604488694547697, 13.89961937509957934, 103.1260903946856473 ) ) ;
#108942=CARTESIAN_POINT ( 'NONE',  ( 4.483927247898545687, 16.52544592524342804, 59.79057627198103120 ) ) ;
#108943=CARTESIAN_POINT ( 'NONE',  ( -21.55341960407619339, 5.719274019375674811, 28.54275706135234358 ) ) ;
#108944=CARTESIAN_POINT ( 'NONE',  ( 21.55341960407610458, 5.719274019375980345, 58.95724293864770971 ) ) ;
#108947=CARTESIAN_POINT ( 'NONE',  ( -5.153800228976328057, -19.02544592524343514, 67.29057627198102409 ) ) ;
#108948=CARTESIAN_POINT ( 'NONE',  ( -14.34966873604960291, -8.224510206698953496, 56.66557627198103830 ) ) ;
#108950=CARTESIAN_POINT ( 'NONE',  ( 16.53943276465976808, 0.05219959533934440121, 111.2510903946856899 ) ) ;
#108951=CARTESIAN_POINT ( 'NONE',  ( -16.53943276465976808, -0.05219959533934237506, 98.75109039468568994 ) ) ;
#108952=CARTESIAN_POINT ( 'NONE',  ( 9.474510206698729675, 16.51473224551082808, 52.08442372801900433 ) ) ;
#108953=CARTESIAN_POINT ( 'NONE',  ( 17.44270441346512968, 5.991230190323099336, 48.86335079264230075 ) ) ;
#108954=CARTESIAN_POINT ( 'NONE',  ( -16.51473224551069308, -9.474510206698971260, 101.6655762719810241 ) ) ;
#108956=CARTESIAN_POINT ( 'NONE',  ( 12.06949235617757843, -12.14591786802309237, 78.12390960531436690 ) ) ;
#108957=CARTESIAN_POINT ( 'NONE',  ( 0.05219959533936267826, -19.03943276465977164, 45.00109039468566863 ) ) ;
#108958=CARTESIAN_POINT ( 'NONE',  ( 9.474510206698971260, -16.51473224551069308, 37.91557627198102409 ) ) ;
#108959=CARTESIAN_POINT ( 'NONE',  ( -0.05219959533907301413, -21.53943276465977519, 32.49890960531435979 ) ) ;
#108960=CARTESIAN_POINT ( 'NONE',  ( 18.62759615963271287, -10.81492255796078972, 58.33224293864768839 ) ) ;
#108961=CARTESIAN_POINT ( 'NONE',  ( -4.483927247898539470, -16.52544592524342804, 102.2905762719810383 ) ) ;
#108962=CARTESIAN_POINT ( 'NONE',  ( -14.29746914071037622, -8.314922557961029526, 54.16775706135235424 ) ) ;
#108963=CARTESIAN_POINT ( 'NONE',  ( 8.314922557960818139, 14.29746914071049879, 94.58224293864769550 ) ) ;
#108965=CARTESIAN_POINT ( 'NONE',  ( -13.89961937509977652, 13.97604488694528158, 110.6239096053143243 ) ) ;
#108969=CARTESIAN_POINT ( 'NONE',  ( 12.06949235617739724, 12.14591786802326823, 46.87609039468568994 ) ) ;
#108970=CARTESIAN_POINT ( 'NONE',  ( -14.29746914071049879, 8.314922557960819915, 30.83224293864770260 ) ) ;
#108971=CARTESIAN_POINT ( 'NONE',  ( 18.67979575497178502, 10.72451020669898547, 59.16557627198103120 ) ) ;
#108972=CARTESIAN_POINT ( 'NONE',  ( -19.02544592524334988, -5.153800228976617603, 83.95942372801901854 ) ) ;
#108973=CARTESIAN_POINT ( 'NONE',  ( 5.719274019375991003, -21.55341960407610458, 42.70724293864770260 ) ) ;
#108974=CARTESIAN_POINT ( 'NONE',  ( 10.81492255796106328, -18.62759615963255655, 75.41775706135233293 ) ) ;
#108975=DIRECTION ( 'NONE',  ( -1.000000000000000000, 0.000000000000000000, 0.000000000000000000 ) ) ;
#108976=CARTESIAN_POINT ( 'NONE',  ( 16.52544592524335698, 4.483927247898782831, 51.45942372801901854 ) ) ;
#108977=CARTESIAN_POINT ( 'NONE',  ( -9.474510206698964154, 16.51473224551069663, 40.41557627198103120 ) ) ;
#108978=CARTESIAN_POINT ( 'NONE',  ( -19.03943276465977164, 0.05219959533909376836, 106.2489096053143669 ) ) ;
#108980=CARTESIAN_POINT ( 'NONE',  ( 5.153800228976335163, 19.02544592524342804, 29.79057627198102409 ) ) ;
#108981=CARTESIAN_POINT ( 'NONE',  ( 12.14591786802309770, 12.06949235617756955, 99.37390960531436690 ) ) ;
#108983=CARTESIAN_POINT ( 'NONE',  ( -16.51473224551069308, -9.474510206698971260, 101.6655762719810241 ) ) ;
#108984=CARTESIAN_POINT ( 'NONE',  ( 4.379528057220092307, 16.55341960407617563, 57.29275706135234714 ) ) ;
#108985=CARTESIAN_POINT ( 'NONE',  ( -21.52544592524343514, 5.823673210054127303, 96.04057627198102409 ) ) ;
#108986=CARTESIAN_POINT ( 'NONE',  ( 5.049401038298161559, -19.05341960407611168, 62.70724293864769550 ) ) ;
#108987=CARTESIAN_POINT ( 'NONE',  ( 10.81492255796106328, -18.62759615963255655, 30.41775706135234358 ) ) ;
#108988=CARTESIAN_POINT ( 'NONE',  ( 19.05341960407611168, 5.049401038298154454, 83.95724293864766707 ) ) ;
#108989=FACE_OUTER_BOUND ( 'NONE', #179609, .T. ) ;
#108991=CARTESIAN_POINT ( 'NONE',  ( -15.80617190586768217, 15.72974639402176855, 23.12609039468567573 ) ) ;
#108992=CARTESIAN_POINT ( 'NONE',  ( -0.05219959533909027116, -19.03943276465977164, 22.49890960531436690 ) ) ;
#108993=CARTESIAN_POINT ( 'NONE',  ( -9.564922557960796823, -16.46253265017161027, 107.0822429386476955 ) ) ;
#108994=CARTESIAN_POINT ( 'NONE',  ( 19.05341960407617918, -5.049401038297876454, 76.04275706135230450 ) ) ;
#108995=CARTESIAN_POINT ( 'NONE',  ( -19.03943276465977164, -0.05219959533935918106, 23.75109039468566152 ) ) ;
#108996=CARTESIAN_POINT ( 'NONE',  ( -10.72451020669898014, 18.67979575497178502, 95.41557627198102409 ) ) ;
#108997=CARTESIAN_POINT ( 'NONE',  ( 16.51473224551083163, -9.474510206698727899, 40.83442372801900433 ) ) ;
#108998=CARTESIAN_POINT ( 'NONE',  ( -0.05219959533934338120, 16.53943276465976808, 72.50109039468568994 ) ) ;
#108999=CARTESIAN_POINT ( 'NONE',  ( 5.049401038298161559, -19.05341960407611168, 102.7072429386476955 ) ) ;
#109001=CARTESIAN_POINT ( 'NONE',  ( 19.05341960407611168, 5.049401038298154454, 58.95724293864768129 ) ) ;
#109003=CARTESIAN_POINT ( 'NONE',  ( -21.52544592524334988, -5.823673210054445271, 68.95942372801901854 ) ) ;
#109004=CARTESIAN_POINT ( 'NONE',  ( 15.72974639402176855, 15.80617190586768217, 81.87609039468568994 ) ) ;
#109005=CARTESIAN_POINT ( 'NONE',  ( -13.97604488694527625, -13.89961937509977652, 76.87390960531433848 ) ) ;
#109006=CARTESIAN_POINT ( 'NONE',  ( -5.823673210054431948, 21.52544592524334988, 47.70942372801902565 ) ) ;
#109007=CARTESIAN_POINT ( 'NONE',  ( 19.03943276465977164, 0.05219959533936151252, 91.25109039468566152 ) ) ;
#109008=CARTESIAN_POINT ( 'NONE',  ( 5.049401038298161559, -19.05341960407611168, 52.70724293864767418 ) ) ;
#109009=CARTESIAN_POINT ( 'NONE',  ( 0.05219959533909260263, 19.03943276465977164, 104.9989096053143669 ) ) ;
#109010=CARTESIAN_POINT ( 'NONE',  ( 5.153800228976335163, 19.02544592524342804, 64.79057627198100988 ) ) ;
#109011=CARTESIAN_POINT ( 'NONE',  ( -16.46253265017160317, 9.564922557960807481, 105.8322429386476955 ) ) ;
#109012=CARTESIAN_POINT ( 'NONE',  ( -9.564922557960796823, -16.46253265017161027, 57.08224293864769550 ) ) ;
#109013=CARTESIAN_POINT ( 'NONE',  ( 18.62759615963271287, -10.81492255796078972, 103.3322429386476955 ) ) ;
#109014=CARTESIAN_POINT ( 'NONE',  ( -12.14591786802326823, 12.06949235617739902, 78.12609039468570415 ) ) ;
#109016=CARTESIAN_POINT ( 'NONE',  ( -16.46253265017146816, -9.564922557961047289, 44.16775706135232582 ) ) ;
#109017=CARTESIAN_POINT ( 'NONE',  ( -13.97604488694527625, -13.89961937509977652, 71.87390960531433848 ) ) ;
#109018=CARTESIAN_POINT ( 'NONE',  ( 14.34966873604960469, 8.224510206698951720, 64.16557627198102409 ) ) ;
#109019=CARTESIAN_POINT ( 'NONE',  ( 16.53943276465976808, -0.05219959533910856209, 88.74890960531436690 ) ) ;
#109020=CARTESIAN_POINT ( 'NONE',  ( -0.05219959533909027116, -19.03943276465977164, 102.4989096053143669 ) ) ;
#109021=CARTESIAN_POINT ( 'NONE',  ( -19.05341960407611168, -5.049401038298163336, 96.45724293864769550 ) ) ;
#109022=CARTESIAN_POINT ( 'NONE',  ( 16.51473224551069308, 9.474510206698969483, 104.1655762719810241 ) ) ;
#109023=CARTESIAN_POINT ( 'NONE',  ( 21.53943276465977519, 0.05219959533937863772, 106.2510903946856757 ) ) ;
#109024=CARTESIAN_POINT ( 'NONE',  ( -8.224510206698735004, -14.34966873604973081, 89.58442372801901854 ) ) ;
#109025=CARTESIAN_POINT ( 'NONE',  ( 13.89961937509977652, -13.97604488694527269, 73.12390960531436690 ) ) ;
#109026=CARTESIAN_POINT ( 'NONE',  ( 10.81492255796106328, -18.62759615963255655, 45.41775706135234003 ) ) ;
#109027=CARTESIAN_POINT ( 'NONE',  ( -0.05219959533907301413, -21.53943276465977519, 27.49890960531435269 ) ) ;
#109028=CARTESIAN_POINT ( 'NONE',  ( 21.55341960407610458, 5.719274019375980345, 98.95724293864770971 ) ) ;
#109029=CARTESIAN_POINT ( 'NONE',  ( -4.379528057220328563, 16.55341960407611168, 65.20724293864768129 ) ) ;
#109030=CARTESIAN_POINT ( 'NONE',  ( -19.05341960407611168, -5.049401038298163336, 56.45724293864768129 ) ) ;
#109031=CARTESIAN_POINT ( 'NONE',  ( -8.224510206698948167, 14.34966873604960824, 75.41557627198102409 ) ) ;
#109032=CARTESIAN_POINT ( 'NONE',  ( -5.153800228976607833, 19.02544592524334988, 47.70942372801900433 ) ) ;
#109033=CARTESIAN_POINT ( 'NONE',  ( -8.314922557960811034, -14.29746914071050412, 107.0822429386476955 ) ) ;
#109034=CARTESIAN_POINT ( 'NONE',  ( -16.52544592524335698, -4.483927247898792601, 63.95942372801901854 ) ) ;
#109035=CARTESIAN_POINT ( 'NONE',  ( 5.049401038298161559, -19.05341960407611168, 67.70724293864769550 ) ) ;
#109037=CARTESIAN_POINT ( 'NONE',  ( -8.314922557960811034, -14.29746914071050412, 92.08224293864769550 ) ) ;
#109038=CARTESIAN_POINT ( 'NONE',  ( -15.80617190586745835, -15.72974639402198527, 36.87390960531435979 ) ) ;
#109040=CARTESIAN_POINT ( 'NONE',  ( -16.52544592524335698, -4.483927247898792601, 103.9594237280190185 ) ) ;
#109041=CARTESIAN_POINT ( 'NONE',  ( 14.29746914071037800, 8.314922557961029526, 26.66775706135235424 ) ) ;
#109042=CARTESIAN_POINT ( 'NONE',  ( -5.823673210054431948, 21.52544592524334988, 97.70942372801904696 ) ) ;
#109043=CARTESIAN_POINT ( 'NONE',  ( -16.51473224551069308, -9.474510206698971260, 81.66557627198103830 ) ) ;
#109044=CARTESIAN_POINT ( 'NONE',  ( -10.72451020669898014, 18.67979575497178502, 115.4155762719810241 ) ) ;
#109045=CARTESIAN_POINT ( 'NONE',  ( 16.51473224551069308, 9.474510206698969483, 24.16557627198102765 ) ) ;
#109046=CARTESIAN_POINT ( 'NONE',  ( 12.06949235617739724, 12.14591786802326823, 26.87609039468567218 ) ) ;
#109047=CARTESIAN_POINT ( 'NONE',  ( 9.564922557961047289, -16.46253265017146816, 90.41775706135234714 ) ) ;
#109049=CARTESIAN_POINT ( 'NONE',  ( 10.81492255796078972, 18.62759615963270932, 84.58224293864769550 ) ) ;
#109050=CARTESIAN_POINT ( 'NONE',  ( 13.97604488694548053, -13.89961937509957401, 70.62609039468567573 ) ) ;
#109051=CARTESIAN_POINT ( 'NONE',  ( 16.46253265017160672, -9.564922557960803928, 23.33224293864769194 ) ) ;
#109052=CARTESIAN_POINT ( 'NONE',  ( 10.81492255796106328, -18.62759615963255655, 20.41775706135234714 ) ) ;
#109054=CARTESIAN_POINT ( 'NONE',  ( 5.153800228976335163, 19.02544592524342804, 84.79057627198099567 ) ) ;
#109055=CARTESIAN_POINT ( 'NONE',  ( -12.14591786802326823, 12.06949235617739902, 33.12609039468569705 ) ) ;
#109057=CARTESIAN_POINT ( 'NONE',  ( -0.05219959533936034679, 19.03943276465977164, 62.50109039468566863 ) ) ;
#109058=CARTESIAN_POINT ( 'NONE',  ( 15.80617190586769283, -15.72974639402175789, 25.62609039468567929 ) ) ;
#109059=CARTESIAN_POINT ( 'NONE',  ( -14.34966873604960291, -8.224510206698953496, 81.66557627198103830 ) ) ;
#109060=CARTESIAN_POINT ( 'NONE',  ( 16.46253265017160672, -9.564922557960803928, 83.33224293864768129 ) ) ;
#109061=CARTESIAN_POINT ( 'NONE',  ( 14.34966873604972726, -8.224510206698740333, 40.83442372801901854 ) ) ;
#109062=CARTESIAN_POINT ( 'NONE',  ( 16.51473224551083163, -9.474510206698727899, 50.83442372801899722 ) ) ;
#109063=CARTESIAN_POINT ( 'NONE',  ( 5.823673210054444382, -21.52544592524334988, 65.20942372801901854 ) ) ;
#109064=CARTESIAN_POINT ( 'NONE',  ( 4.379528057220092307, 16.55341960407617563, 22.29275706135235069 ) ) ;
#109065=CARTESIAN_POINT ( 'NONE',  ( -13.97604488694527625, -13.89961937509977652, 51.87390960531436690 ) ) ;
#109066=CARTESIAN_POINT ( 'NONE',  ( 9.564922557961047289, -16.46253265017146816, 80.41775706135234714 ) ) ;
#109067=CARTESIAN_POINT ( 'NONE',  ( 16.52544592524335698, 4.483927247898782831, 56.45942372801902565 ) ) ;
#109068=CARTESIAN_POINT ( 'NONE',  ( -21.55341960407619339, 5.719274019375674811, 98.54275706135234714 ) ) ;
#109069=CARTESIAN_POINT ( 'NONE',  ( -16.46253265017146816, -9.564922557961047289, 64.16775706135233293 ) ) ;
#109070=CARTESIAN_POINT ( 'NONE',  ( -19.03943276465977164, 0.05219959533909376836, 51.24890960531436690 ) ) ;
#109071=CARTESIAN_POINT ( 'NONE',  ( -15.80617190586745835, -15.72974639402198527, 66.87390960531436690 ) ) ;
#109072=CARTESIAN_POINT ( 'NONE',  ( 14.34966873604960469, 8.224510206698951720, 64.16557627198102409 ) ) ;
#109073=CARTESIAN_POINT ( 'NONE',  ( 19.05341960407617918, -5.049401038297876454, 81.04275706135231871 ) ) ;
#109074=CARTESIAN_POINT ( 'NONE',  ( 16.19135201231364718, -7.376712067592015920, 62.31319145947974647 ) ) ;
#109075=CARTESIAN_POINT ( 'NONE',  ( -19.03943276465977164, -0.05219959533935918106, 48.75109039468566863 ) ) ;
#109076=CARTESIAN_POINT ( 'NONE',  ( -16.53943276465976808, -0.05219959533934237506, 98.75109039468568994 ) ) ;
#109077=CARTESIAN_POINT ( 'NONE',  ( 8.314922557960818139, 14.29746914071049879, 69.58224293864769550 ) ) ;
#109078=CARTESIAN_POINT ( 'NONE',  ( -21.55341960407619339, 5.719274019375674811, 98.54275706135234714 ) ) ;
#109080=CARTESIAN_POINT ( 'NONE',  ( -15.80617190586745835, -15.72974639402198527, 91.87390960531436690 ) ) ;
#109081=CARTESIAN_POINT ( 'NONE',  ( 19.03943276465977164, -0.05219959533909143690, 58.74890960531435979 ) ) ;
#109082=CARTESIAN_POINT ( 'NONE',  ( 15.72974639402176855, 15.80617190586768217, 66.87609039468568994 ) ) ;
#109083=CARTESIAN_POINT ( 'NONE',  ( -5.049401038298153566, 19.05341960407611168, 50.20724293864770260 ) ) ;
#109085=CARTESIAN_POINT ( 'NONE',  ( -19.03943276465977164, 0.05219959533909376836, 21.24890960531436335 ) ) ;
#109086=CARTESIAN_POINT ( 'NONE',  ( 9.474510206698971260, -16.51473224551069308, 107.9155762719810383 ) ) ;
#109087=CARTESIAN_POINT ( 'NONE',  ( -16.53943276465976808, 0.05219959533911058130, 71.24890960531435269 ) ) ;
#109088=CARTESIAN_POINT ( 'NONE',  ( 5.049401038298161559, -19.05341960407611168, 32.70724293864768129 ) ) ;
#109089=CARTESIAN_POINT ( 'NONE',  ( 16.55341960407611168, 4.379528057220329451, 78.95724293864769550 ) ) ;
#109091=CARTESIAN_POINT ( 'NONE',  ( -21.53943276465977519, 0.05219959533907696930, 101.2489096053143669 ) ) ;
#109092=CARTESIAN_POINT ( 'NONE',  ( -18.62759615963255300, -10.81492255796106328, 34.16775706135234714 ) ) ;
#109093=CARTESIAN_POINT ( 'NONE',  ( 19.05341960407611168, 5.049401038298154454, 23.95724293864769194 ) ) ;
#109094=CARTESIAN_POINT ( 'NONE',  ( 8.314922557961029526, -14.29746914071037800, 55.41775706135234714 ) ) ;
#109095=CARTESIAN_POINT ( 'NONE',  ( -10.72451020669898014, 18.67979575497178502, 80.41557627198103830 ) ) ;
#109096=CARTESIAN_POINT ( 'NONE',  ( 19.03943276465977164, 0.05219959533936151252, 21.25109039468565797 ) ) ;
#109097=CARTESIAN_POINT ( 'NONE',  ( -19.03943276465977164, 0.05219959533909376836, 111.2489096053143669 ) ) ;
#109098=CARTESIAN_POINT ( 'NONE',  ( -21.53943276465977519, -0.05219959533937600094, 38.75109039468567573 ) ) ;
#109099=CARTESIAN_POINT ( 'NONE',  ( 15.72974639402199770, -15.80617190586745480, 38.12390960531436690 ) ) ;
#109100=CARTESIAN_POINT ( 'NONE',  ( -16.53943276465976808, 0.05219959533911058130, 26.24890960531435624 ) ) ;
#109101=CARTESIAN_POINT ( 'NONE',  ( 18.62759615963255655, 10.81492255796105972, 61.66775706135235424 ) ) ;
#109102=CARTESIAN_POINT ( 'NONE',  ( -18.62759615963255300, -10.81492255796106328, 94.16775706135237556 ) ) ;
#109103=CARTESIAN_POINT ( 'NONE',  ( -9.564922557961040184, 16.46253265017147172, 32.91775706135233293 ) ) ;
#109104=CARTESIAN_POINT ( 'NONE',  ( 12.06949235617739724, 12.14591786802326823, 81.87609039468568994 ) ) ;
#109105=CARTESIAN_POINT ( 'NONE',  ( -21.53943276465977519, -0.05219959533937600094, 53.75109039468568994 ) ) ;
#109106=CARTESIAN_POINT ( 'NONE',  ( 5.153800228976335163, 19.02544592524342804, 39.79057627198100988 ) ) ;
#109107=CARTESIAN_POINT ( 'NONE',  ( -16.46253265017146816, -9.564922557961047289, 24.16775706135233648 ) ) ;
#109108=CARTESIAN_POINT ( 'NONE',  ( -10.72451020669898014, 18.67979575497178502, 30.41557627198101699 ) ) ;
#109109=CARTESIAN_POINT ( 'NONE',  ( -10.72451020669898014, 18.67979575497178502, 115.4155762719810241 ) ) ;
#109110=CARTESIAN_POINT ( 'NONE',  ( -21.52544592524343514, 5.823673210054127303, 71.04057627198103830 ) ) ;
#109111=CARTESIAN_POINT ( 'NONE',  ( -16.52544592524335698, -4.483927247898792601, 43.95942372801902565 ) ) ;
#109113=CARTESIAN_POINT ( 'NONE',  ( 15.72974639402199770, -15.80617190586745480, 78.12390960531436690 ) ) ;
#109114=CARTESIAN_POINT ( 'NONE',  ( -4.483927247898782831, 16.52544592524335698, 67.70942372801901854 ) ) ;
#109115=CARTESIAN_POINT ( 'NONE',  ( 16.55341960407611168, 4.379528057220329451, 68.95724293864769550 ) ) ;
#109117=CARTESIAN_POINT ( 'NONE',  ( -19.02544592524334988, -5.153800228976617603, 93.95942372801900433 ) ) ;
#109118=VECTOR ( 'NONE', #37177, 1000.000000000000000 ) ;
#109120=CARTESIAN_POINT ( 'NONE',  ( 0.05219959533934541429, -16.53943276465976808, 35.00109039468568284 ) ) ;
#109121=CARTESIAN_POINT ( 'NONE',  ( -18.62759615963270932, 10.81492255796079327, 115.8322429386477097 ) ) ;
#109122=CARTESIAN_POINT ( 'NONE',  ( -21.52544592524343514, 5.823673210054127303, 81.04057627198102409 ) ) ;
#109123=CARTESIAN_POINT ( 'NONE',  ( -10.81492255796078084, -18.62759615963271287, 37.08224293864768129 ) ) ;
#109124=CARTESIAN_POINT ( 'NONE',  ( 16.55341960407618274, -4.379528057220086978, 61.04275706135234714 ) ) ;
#109125=CARTESIAN_POINT ( 'NONE',  ( -19.03943276465977164, 0.05219959533909376836, 76.24890960531435269 ) ) ;
#109126=CARTESIAN_POINT ( 'NONE',  ( 10.81492255796106328, -18.62759615963255655, 40.41775706135234714 ) ) ;
#109127=CARTESIAN_POINT ( 'NONE',  ( 19.05341960407617918, -5.049401038297876454, 106.0427570613523471 ) ) ;
#109128=CARTESIAN_POINT ( 'NONE',  ( -21.52544592524343514, 5.823673210054127303, 26.04057627198103475 ) ) ;
#109129=CARTESIAN_POINT ( 'NONE',  ( -19.03943276465977164, -0.05219959533935918106, 28.75109039468566507 ) ) ;
#109130=CARTESIAN_POINT ( 'NONE',  ( 16.53943276465976808, 0.05219959533934440121, 41.25109039468568284 ) ) ;
#109131=CARTESIAN_POINT ( 'NONE',  ( -16.46253265017160317, 9.564922557960807481, 100.8322429386477097 ) ) ;
#109132=CARTESIAN_POINT ( 'NONE',  ( 10.81492255796078972, 18.62759615963270932, 104.5822429386477097 ) ) ;
#109133=CARTESIAN_POINT ( 'NONE',  ( -9.474510206698964154, 16.51473224551069663, 75.41557627198103830 ) ) ;
#109135=CARTESIAN_POINT ( 'NONE',  ( 12.14591786802309770, 12.06949235617756955, 84.37390960531438111 ) ) ;
#109136=CARTESIAN_POINT ( 'NONE',  ( 5.719274019375991003, -21.55341960407610458, 27.70724293864769905 ) ) ;
#109137=CARTESIAN_POINT ( 'NONE',  ( -17.49999999999999645, 5.624438216177594541, 35.81670344914645199 ) ) ;
#109138=CARTESIAN_POINT ( 'NONE',  ( 5.823673210054125526, 21.52544592524343514, 109.7905762719810383 ) ) ;
#109139=CARTESIAN_POINT ( 'NONE',  ( 13.89961937509957401, 13.97604488694547697, 61.87609039468566863 ) ) ;
#109140=CARTESIAN_POINT ( 'NONE',  ( 15.80617190586746368, 15.72974639402197994, 29.37390960531435269 ) ) ;
#109141=CARTESIAN_POINT ( 'NONE',  ( 13.97604488694527802, 13.89961937509977652, 24.37390960531435624 ) ) ;
#109142=CARTESIAN_POINT ( 'NONE',  ( 5.823673210054125526, 21.52544592524343514, 69.79057627198102409 ) ) ;
#109143=CARTESIAN_POINT ( 'NONE',  ( 0.05219959533909260263, 19.03943276465977164, 104.9989096053143669 ) ) ;
#109144=CARTESIAN_POINT ( 'NONE',  ( -21.55341960407619339, 5.719274019375674811, 88.54275706135236135 ) ) ;
#109145=CARTESIAN_POINT ( 'NONE',  ( 19.03943276465977164, -0.05219959533909143690, 53.74890960531436690 ) ) ;
#109147=CARTESIAN_POINT ( 'NONE',  ( -8.314922557960811034, -14.29746914071050412, 82.08224293864768129 ) ) ;
#109148=CARTESIAN_POINT ( 'NONE',  ( 16.55341960407618274, -4.379528057220086978, 36.04275706135234714 ) ) ;
#109149=CARTESIAN_POINT ( 'NONE',  ( -13.97604488694527625, -13.89961937509977652, 56.87390960531434558 ) ) ;
#109150=CARTESIAN_POINT ( 'NONE',  ( -21.52544592524334988, -5.823673210054445271, 73.95942372801901854 ) ) ;
#109151=ORIENTED_EDGE ( 'NONE', *, *, #108344, .F. ) ;
#109152=CARTESIAN_POINT ( 'NONE',  ( 9.564922557961047289, -16.46253265017146816, 25.41775706135234003 ) ) ;
#109153=CARTESIAN_POINT ( 'NONE',  ( 0.05219959533936267826, -19.03943276465977164, 45.00109039468566863 ) ) ;
#109154=CARTESIAN_POINT ( 'NONE',  ( 15.80617190586769283, -15.72974639402175789, 30.62609039468567929 ) ) ;
#109156=CARTESIAN_POINT ( 'NONE',  ( 9.564922557961047289, -16.46253265017146816, 30.41775706135232937 ) ) ;
#109157=CARTESIAN_POINT ( 'NONE',  ( -9.564922557960796823, -16.46253265017161027, 82.08224293864768129 ) ) ;
#109158=CARTESIAN_POINT ( 'NONE',  ( -5.049401038298153566, 19.05341960407611168, 70.20724293864769550 ) ) ;
#109159=CARTESIAN_POINT ( 'NONE',  ( 16.52544592524342804, -4.483927247898539470, 28.54057627198103120 ) ) ;
#109160=CARTESIAN_POINT ( 'NONE',  ( -16.51473224551069308, -9.474510206698971260, 111.6655762719810383 ) ) ;
#109161=CARTESIAN_POINT ( 'NONE',  ( 5.823673210054444382, -21.52544592524334988, 85.20942372801901854 ) ) ;
#109164=CARTESIAN_POINT ( 'NONE',  ( -21.53943276465977519, -0.05219959533937600094, 88.75109039468567573 ) ) ;
#109165=CARTESIAN_POINT ( 'NONE',  ( 16.31925111598458500, -7.325300261831445781, 42.66424538967253000 ) ) ;
#109166=CARTESIAN_POINT ( 'NONE',  ( -5.153800228976328057, -19.02544592524343514, 97.29057627198099567 ) ) ;
#109168=CARTESIAN_POINT ( 'NONE',  ( -14.29746914071037622, -8.314922557961029526, 49.16775706135234003 ) ) ;
#109169=CARTESIAN_POINT ( 'NONE',  ( 18.62759615963271287, -10.81492255796078972, 73.33224293864769550 ) ) ;
#109170=CARTESIAN_POINT ( 'NONE',  ( -4.483927247898539470, -16.52544592524342804, 32.29057627198102409 ) ) ;
#109171=CARTESIAN_POINT ( 'NONE',  ( 4.483927247898545687, 16.52544592524342804, 109.7905762719810383 ) ) ;
#109172=CARTESIAN_POINT ( 'NONE',  ( 19.05341960407611168, 5.049401038298154454, 98.95724293864766707 ) ) ;
#109173=CARTESIAN_POINT ( 'NONE',  ( -10.81492255796105439, 18.62759615963255655, 112.9177570613523329 ) ) ;
#109174=CARTESIAN_POINT ( 'NONE',  ( 4.483927247898545687, 16.52544592524342804, 109.7905762719810383 ) ) ;
#109175=CARTESIAN_POINT ( 'NONE',  ( 18.62759615963255655, 10.81492255796105972, 66.66775706135234714 ) ) ;
#109176=CARTESIAN_POINT ( 'NONE',  ( 0.05219959533909260263, 19.03943276465977164, 109.9989096053143669 ) ) ;
#109177=CARTESIAN_POINT ( 'NONE',  ( 12.06949235617739724, 12.14591786802326823, 106.8760903946856899 ) ) ;
#109178=CARTESIAN_POINT ( 'NONE',  ( -16.51473224551082808, 9.474510206698731452, 58.33442372801900433 ) ) ;
#109179=CARTESIAN_POINT ( 'NONE',  ( 5.049401038297881783, 19.05341960407617918, 67.29275706135233293 ) ) ;
#109180=CARTESIAN_POINT ( 'NONE',  ( -5.049401038298153566, 19.05341960407611168, 105.2072429386476671 ) ) ;
#109181=CARTESIAN_POINT ( 'NONE',  ( 4.379528057220339221, -16.55341960407611168, 87.70724293864769550 ) ) ;
#109182=CARTESIAN_POINT ( 'NONE',  ( -16.46253265017146816, -9.564922557961047289, 64.16775706135233293 ) ) ;
#109183=CARTESIAN_POINT ( 'NONE',  ( -9.564922557960796823, -16.46253265017161027, 82.08224293864768129 ) ) ;
#109184=CARTESIAN_POINT ( 'NONE',  ( -8.314922557960811034, -14.29746914071050412, 67.08224293864770971 ) ) ;
#109185=CARTESIAN_POINT ( 'NONE',  ( 9.564922557961047289, -16.46253265017146816, 90.41775706135234714 ) ) ;
#109186=CARTESIAN_POINT ( 'NONE',  ( 21.55341960407610458, 5.719274019375980345, 48.95724293864770971 ) ) ;
#109188=CARTESIAN_POINT ( 'NONE',  ( 9.564922557960805705, 16.46253265017160317, 24.58224293864769194 ) ) ;
#109189=CARTESIAN_POINT ( 'NONE',  ( -16.52216118717207394, -7.221426719304521846, 31.07599021046992505 ) ) ;
#109190=CARTESIAN_POINT ( 'NONE',  ( 19.02544592524343514, -5.153800228976328945, 78.54057627198099567 ) ) ;
#109191=CARTESIAN_POINT ( 'NONE',  ( 21.53943276465977519, -0.05219959533907433946, 78.74890960531436690 ) ) ;
#109192=CARTESIAN_POINT ( 'NONE',  ( -4.379528057220086978, -16.55341960407618274, 89.79275706135236135 ) ) ;
#109193=CARTESIAN_POINT ( 'NONE',  ( 5.153800228976335163, 19.02544592524342804, 69.79057627198103830 ) ) ;
#109194=CARTESIAN_POINT ( 'NONE',  ( -0.05219959533936034679, 19.03943276465977164, 62.50109039468566863 ) ) ;
#109195=CARTESIAN_POINT ( 'NONE',  ( 10.81492255796106328, -18.62759615963255655, 80.41775706135234714 ) ) ;
#109196=CARTESIAN_POINT ( 'NONE',  ( 18.62759615963271287, -10.81492255796078972, 63.33224293864770260 ) ) ;
#109197=CARTESIAN_POINT ( 'NONE',  ( -5.823673210054116645, -21.52544592524344225, 22.29057627198102765 ) ) ;
#109198=CARTESIAN_POINT ( 'NONE',  ( -9.474510206698964154, 16.51473224551069663, 35.41557627198102409 ) ) ;
#109199=CARTESIAN_POINT ( 'NONE',  ( 0.05219959533934541429, -16.53943276465976808, 100.0010903946857042 ) ) ;
#109200=CARTESIAN_POINT ( 'NONE',  ( -8.224510206698735004, -14.34966873604973081, 19.58442372801901143 ) ) ;
#109201=CARTESIAN_POINT ( 'NONE',  ( 16.36317988757059183, 7.306389748694952502, 53.40210391636777842 ) ) ;
#109202=CARTESIAN_POINT ( 'NONE',  ( 21.53943276465977519, 0.05219959533937863772, 91.25109039468568994 ) ) ;
#109203=CARTESIAN_POINT ( 'NONE',  ( 16.53943276465976808, -0.05219959533910856209, 53.74890960531437401 ) ) ;
#109204=CARTESIAN_POINT ( 'NONE',  ( -10.81492255796078084, -18.62759615963271287, 92.08224293864769550 ) ) ;
#109205=CARTESIAN_POINT ( 'NONE',  ( -5.823673210054116645, -21.52544592524344225, 102.2905762719810383 ) ) ;
#109206=CARTESIAN_POINT ( 'NONE',  ( 16.61371651742602396, -7.165104196376141488, 96.35415069992994574 ) ) ;
#109207=CARTESIAN_POINT ( 'NONE',  ( -10.81492255796078084, -18.62759615963271287, 42.08224293864769550 ) ) ;
#109208=CARTESIAN_POINT ( 'NONE',  ( -14.29746914071037622, -8.314922557961029526, 74.16775706135231871 ) ) ;
#109209=CARTESIAN_POINT ( 'NONE',  ( -4.379528057220328563, 16.55341960407611168, 90.20724293864770971 ) ) ;
#109210=CARTESIAN_POINT ( 'NONE',  ( -19.03943276465977164, 0.05219959533909376836, 41.24890960531435269 ) ) ;
#109212=CARTESIAN_POINT ( 'NONE',  ( -16.52544592524335698, -4.483927247898792601, 108.9594237280190185 ) ) ;
#109213=CARTESIAN_POINT ( 'NONE',  ( 5.719274019375673035, 21.55341960407619339, 27.29275706135234358 ) ) ;
#109214=CARTESIAN_POINT ( 'NONE',  ( -16.46253265017160317, 9.564922557960807481, 90.83224293864769550 ) ) ;
#109215=CARTESIAN_POINT ( 'NONE',  ( 0.05219959533937995610, -21.53943276465977519, 70.00109039468568994 ) ) ;
#109217=CARTESIAN_POINT ( 'NONE',  ( -19.03943276465977164, 0.05219959533909376836, 31.24890960531435979 ) ) ;
#109219=CARTESIAN_POINT ( 'NONE',  ( -5.823673210054431948, 21.52544592524334988, 62.70942372801902565 ) ) ;
#109220=CARTESIAN_POINT ( 'NONE',  ( -13.89961937509977652, 13.97604488694528158, 50.62390960531435979 ) ) ;
#109221=CARTESIAN_POINT ( 'NONE',  ( 13.97604488694527802, 13.89961937509977652, 114.3739096053143669 ) ) ;
#109222=CARTESIAN_POINT ( 'NONE',  ( -5.049401038298153566, 19.05341960407611168, 85.20724293864766707 ) ) ;
#109223=CARTESIAN_POINT ( 'NONE',  ( 9.564922557961047289, -16.46253265017146816, 65.41775706135233293 ) ) ;
#109224=CARTESIAN_POINT ( 'NONE',  ( 10.81492255796106328, -18.62759615963255655, 45.41775706135234003 ) ) ;
#109225=CARTESIAN_POINT ( 'NONE',  ( -13.89961937509957401, -13.97604488694547875, 64.37609039468567573 ) ) ;
#109226=CARTESIAN_POINT ( 'NONE',  ( -5.153800228976328057, -19.02544592524343514, 37.29057627198102409 ) ) ;
#109227=CARTESIAN_POINT ( 'NONE',  ( 14.29746914071037800, 8.314922557961029526, 101.6677570613523613 ) ) ;
#109228=CARTESIAN_POINT ( 'NONE',  ( 19.02544592524334988, 5.153800228976608722, 81.45942372801897591 ) ) ;
#109229=CARTESIAN_POINT ( 'NONE',  ( -16.53943276465976808, 0.05219959533911058130, 26.24890960531435624 ) ) ;
#109230=CARTESIAN_POINT ( 'NONE',  ( -16.46253265017146816, -9.564922557961047289, 44.16775706135232582 ) ) ;
#109231=CARTESIAN_POINT ( 'NONE',  ( 21.55341960407619695, -5.719274019375665929, 106.0427570613523471 ) ) ;
#109232=CARTESIAN_POINT ( 'NONE',  ( -13.89961937509957401, -13.97604488694547875, 29.37609039468565797 ) ) ;
#109233=CARTESIAN_POINT ( 'NONE',  ( -16.51473224551069308, -9.474510206698971260, 31.66557627198102054 ) ) ;
#109234=CARTESIAN_POINT ( 'NONE',  ( -21.52544592524334988, -5.823673210054445271, 93.95942372801903275 ) ) ;
#109235=CARTESIAN_POINT ( 'NONE',  ( 12.06949235617739724, 12.14591786802326823, 36.87609039468568994 ) ) ;
#109236=CARTESIAN_POINT ( 'NONE',  ( -16.51473224551069308, -9.474510206698971260, 86.66557627198102409 ) ) ;
#109237=B_SPLINE_CURVE_WITH_KNOTS ( 'NONE', 3,
 ( #23081, #132251, #158591, #66580, #67576, #160590, #117075, #131245, #96908, #178771, #129234, #20080, #192934, #54411, #128245, #116083, #130226, #161587, #146404, #84726 ),
 .UNSPECIFIED., .F., .F.,
 ( 4, 2, 2, 2, 2, 2, 2, 2, 2, 4 ),
 ( 0.000000000000000000, 0.0004987090165372625112, 0.0009974180330745250223, 0.001246772541343159910, 0.001496127049611795014, 0.001994836066149060453, 0.002493545082686326325, 0.002742899590954956876, 0.002992254099223587861, 0.003989672132298188560 ),
 .UNSPECIFIED. ) ;
#109239=CARTESIAN_POINT ( 'NONE',  ( -9.474510206698964154, 16.51473224551069663, 85.41557627198102409 ) ) ;
#109241=CARTESIAN_POINT ( 'NONE',  ( 19.02544592524334988, 5.153800228976608722, 81.45942372801897591 ) ) ;
#109242=CARTESIAN_POINT ( 'NONE',  ( 9.474510206698971260, -16.51473224551069308, 112.9155762719810383 ) ) ;
#109243=CARTESIAN_POINT ( 'NONE',  ( 21.52544592524334988, 5.823673210054432836, 106.4594237280190328 ) ) ;
#109244=CARTESIAN_POINT ( 'NONE',  ( 0.05219959533910956823, 16.53943276465976808, 104.9989096053143669 ) ) ;
#109246=CARTESIAN_POINT ( 'NONE',  ( -15.72974639402197994, 15.80617190586746368, 55.62390960531436690 ) ) ;
#109247=CARTESIAN_POINT ( 'NONE',  ( 21.55341960407610458, 5.719274019375980345, 33.95724293864769550 ) ) ;
#109248=CARTESIAN_POINT ( 'NONE',  ( 19.03943276465977164, -0.05219959533909143690, 23.74890960531435269 ) ) ;
#109250=CARTESIAN_POINT ( 'NONE',  ( 5.153800228976615827, -19.02544592524334988, 55.20942372801899722 ) ) ;
#109251=CARTESIAN_POINT ( 'NONE',  ( 16.53943276465976808, -0.05219959533910856209, 43.74890960531435979 ) ) ;
#109253=CARTESIAN_POINT ( 'NONE',  ( -10.81492255796078084, -18.62759615963271287, 22.08224293864769194 ) ) ;
#109254=CARTESIAN_POINT ( 'NONE',  ( -10.72451020669870658, -18.67979575497194134, 74.58442372801901854 ) ) ;
#109255=CARTESIAN_POINT ( 'NONE',  ( -21.53943276465977519, 0.05219959533907696930, 71.24890960531435269 ) ) ;
#109256=CARTESIAN_POINT ( 'NONE',  ( 18.67979575497194134, -10.72451020669871369, 45.83442372801901854 ) ) ;
#109257=CARTESIAN_POINT ( 'NONE',  ( 15.72974639402199770, -15.80617190586745480, 103.1239096053143811 ) ) ;
#109258=CARTESIAN_POINT ( 'NONE',  ( 5.823673210054444382, -21.52544592524334988, 45.20942372801901854 ) ) ;
#109259=CARTESIAN_POINT ( 'NONE',  ( 16.51473224551069308, 9.474510206698969483, 29.16557627198103475 ) ) ;
#109260=CARTESIAN_POINT ( 'NONE',  ( -19.05341960407611168, -5.049401038298163336, 76.45724293864769550 ) ) ;
#109261=CARTESIAN_POINT ( 'NONE',  ( 4.379528057220092307, 16.55341960407617563, 77.29275706135234714 ) ) ;
#109262=CARTESIAN_POINT ( 'NONE',  ( -12.14591786802309592, -12.06949235617757132, 106.8739096053143811 ) ) ;
#109264=CARTESIAN_POINT ( 'NONE',  ( -12.14591786802309592, -12.06949235617757132, 56.87390960531436690 ) ) ;
#109265=CARTESIAN_POINT ( 'NONE',  ( 4.483927247898545687, 16.52544592524342804, 24.79057627198103120 ) ) ;
#109266=CARTESIAN_POINT ( 'NONE',  ( 5.049401038298161559, -19.05341960407611168, 62.70724293864769550 ) ) ;
#109267=CARTESIAN_POINT ( 'NONE',  ( -9.474510206698964154, 16.51473224551069663, 30.41557627198102054 ) ) ;
#109268=CARTESIAN_POINT ( 'NONE',  ( -0.05219959533907301413, -21.53943276465977519, 47.49890960531435979 ) ) ;
#109269=CARTESIAN_POINT ( 'NONE',  ( 16.51473224551083163, -9.474510206698727899, 35.83442372801899722 ) ) ;
#109270=CARTESIAN_POINT ( 'NONE',  ( -17.31747979337948351, -6.344076630961017926, 41.37944868065184778 ) ) ;
#109271=CARTESIAN_POINT ( 'NONE',  ( 16.52544592524342804, -4.483927247898539470, 38.54057627198103120 ) ) ;
#109272=CARTESIAN_POINT ( 'NONE',  ( 21.52544592524344225, -5.823673210054117533, 28.54057627198103120 ) ) ;
#109273=CARTESIAN_POINT ( 'NONE',  ( -15.80617190586768217, 15.72974639402176855, 63.12609039468568994 ) ) ;
#109274=CARTESIAN_POINT ( 'NONE',  ( 17.50000000000001776, -3.242565516147306592, 37.50000000000000000 ) ) ;
#109275=CARTESIAN_POINT ( 'NONE',  ( 16.53943276465976808, 0.05219959533934440121, 66.25109039468567573 ) ) ;
#109276=CARTESIAN_POINT ( 'NONE',  ( 16.46253265017146816, 9.564922557961045513, 56.66775706135233293 ) ) ;
#109277=CARTESIAN_POINT ( 'NONE',  ( -0.05219959533910754901, -16.53943276465976808, 42.49890960531435979 ) ) ;
#109278=CARTESIAN_POINT ( 'NONE',  ( 17.12812012977027720, -6.668231424565973953, 51.14051240676860743 ) ) ;
#109279=CARTESIAN_POINT ( 'NONE',  ( -14.29746914071049879, 8.314922557960819915, 25.83224293864769194 ) ) ;
#109280=CARTESIAN_POINT ( 'NONE',  ( -9.564922557960796823, -16.46253265017161027, 37.08224293864768839 ) ) ;
#109281=EDGE_CURVE ( 'NONE', #122538, #128850, #26922, .T. ) ;
#109282=CARTESIAN_POINT ( 'NONE',  ( -19.03943276465977164, 0.05219959533909376836, 56.24890960531435979 ) ) ;
#109283=CARTESIAN_POINT ( 'NONE',  ( -4.379528057220328563, 16.55341960407611168, 115.2072429386476955 ) ) ;
#109284=CARTESIAN_POINT ( 'NONE',  ( 5.719274019375673035, 21.55341960407619339, 32.29275706135235424 ) ) ;
#109285=CARTESIAN_POINT ( 'NONE',  ( -13.89961937509977652, 13.97604488694528158, 55.62390960531434558 ) ) ;
#109287=CARTESIAN_POINT ( 'NONE',  ( 19.05341960407611168, 5.049401038298154454, 43.95724293864769550 ) ) ;
#109288=CARTESIAN_POINT ( 'NONE',  ( 18.62759615963271287, -10.81492255796078972, 38.33224293864768839 ) ) ;
#109289=CARTESIAN_POINT ( 'NONE',  ( 0.05219959533937995610, -21.53943276465977519, 55.00109039468568284 ) ) ;
#109290=CARTESIAN_POINT ( 'NONE',  ( -12.14591786802309592, -12.06949235617757132, 111.8739096053143669 ) ) ;
#109291=CARTESIAN_POINT ( 'NONE',  ( -21.55341960407610458, -5.719274019375992779, 21.45724293864769550 ) ) ;
#109292=CARTESIAN_POINT ( 'NONE',  ( 4.483927247898790824, -16.52544592524335698, 95.20942372801903275 ) ) ;
#109293=CARTESIAN_POINT ( 'NONE',  ( 15.80617190586769283, -15.72974639402175789, 110.6260903946857042 ) ) ;
#109294=CARTESIAN_POINT ( 'NONE',  ( 14.34966873604972726, -8.224510206698740333, 60.83442372801901854 ) ) ;
#109295=CARTESIAN_POINT ( 'NONE',  ( 9.564922557960805705, 16.46253265017160317, 114.5822429386476955 ) ) ;
#109296=CARTESIAN_POINT ( 'NONE',  ( -16.52544592524335698, -4.483927247898792601, 48.95942372801902565 ) ) ;
#109297=CARTESIAN_POINT ( 'NONE',  ( 0.05219959533934541429, -16.53943276465976808, 25.00109039468567218 ) ) ;
#109298=CARTESIAN_POINT ( 'NONE',  ( 4.379528057220092307, 16.55341960407617563, 92.29275706135236135 ) ) ;
#109299=CARTESIAN_POINT ( 'NONE',  ( -10.81492255796105439, 18.62759615963255655, 47.91775706135234714 ) ) ;
#109300=CARTESIAN_POINT ( 'NONE',  ( 0.05219959533936267826, -19.03943276465977164, 110.0010903946856757 ) ) ;
#109301=CARTESIAN_POINT ( 'NONE',  ( -21.52544592524334988, -5.823673210054445271, 18.95942372801901143 ) ) ;
#109302=CARTESIAN_POINT ( 'NONE',  ( -14.29746914071037622, -8.314922557961029526, 29.16775706135234003 ) ) ;
#109303=CARTESIAN_POINT ( 'NONE',  ( 0.05219959533934541429, -16.53943276465976808, 85.00109039468568994 ) ) ;
#109305=CARTESIAN_POINT ( 'NONE',  ( 5.719274019375673035, 21.55341960407619339, 92.29275706135236135 ) ) ;
#109306=CARTESIAN_POINT ( 'NONE',  ( -13.89961937509957401, -13.97604488694547875, 84.37609039468567573 ) ) ;
#109307=CARTESIAN_POINT ( 'NONE',  ( 0.05219959533910956823, 16.53943276465976808, 44.99890960531435979 ) ) ;
#109308=CARTESIAN_POINT ( 'NONE',  ( -16.55341960407611168, -4.379528057220339221, 41.45724293864769550 ) ) ;
#109309=CARTESIAN_POINT ( 'NONE',  ( -12.06949235617756955, 12.14591786802309770, 105.6239096053143669 ) ) ;
#109310=CARTESIAN_POINT ( 'NONE',  ( -13.97604488694547697, 13.89961937509957934, 53.12609039468565442 ) ) ;
#109311=CARTESIAN_POINT ( 'NONE',  ( 17.50000000000002487, -5.499999999999880984, 53.29690382534172244 ) ) ;
#109312=CARTESIAN_POINT ( 'NONE',  ( 21.55341960407619695, -5.719274019375665929, 46.04275706135234714 ) ) ;
#109313=CARTESIAN_POINT ( 'NONE',  ( 19.05341960407617918, -5.049401038297876454, 111.0427570613523329 ) ) ;
#109315=CARTESIAN_POINT ( 'NONE',  ( 9.564922557960805705, 16.46253265017160317, 99.58224293864770971 ) ) ;
#109316=CARTESIAN_POINT ( 'NONE',  ( -21.52544592524343514, 5.823673210054127303, 56.04057627198102409 ) ) ;
#109317=CARTESIAN_POINT ( 'NONE',  ( 5.049401038297881783, 19.05341960407617563, 97.29275706135233293 ) ) ;
#109318=CARTESIAN_POINT ( 'NONE',  ( 16.51473224551069308, 9.474510206698969483, 89.16557627198103830 ) ) ;
#109319=CARTESIAN_POINT ( 'NONE',  ( -21.53943276465977519, 0.05219959533907696930, 56.24890960531436690 ) ) ;
#109320=CARTESIAN_POINT ( 'NONE',  ( -16.52544592524342804, 4.483927247898546575, 106.0405762719810525 ) ) ;
#109321=CARTESIAN_POINT ( 'NONE',  ( 13.97604488694527802, 13.89961937509977652, 64.37390960531436690 ) ) ;
#109322=CARTESIAN_POINT ( 'NONE',  ( 13.97604488694527802, 13.89961937509977652, 29.37390960531435979 ) ) ;
#109323=CARTESIAN_POINT ( 'NONE',  ( -18.67979575497193778, 10.72451020669871902, 43.33442372801901143 ) ) ;
#109324=CARTESIAN_POINT ( 'NONE',  ( -15.72974639402176322, -15.80617190586768395, 74.37609039468568994 ) ) ;
#109325=CARTESIAN_POINT ( 'NONE',  ( 16.53943276465976808, 0.05219959533934440121, 91.25109039468568994 ) ) ;
#109326=CARTESIAN_POINT ( 'NONE',  ( -10.81492255796105439, 18.62759615963255655, 27.91775706135234358 ) ) ;
#109327=CARTESIAN_POINT ( 'NONE',  ( 18.67979575497194134, -10.72451020669871369, 35.83442372801901143 ) ) ;
#109328=CARTESIAN_POINT ( 'NONE',  ( -5.049401038297874678, -19.05341960407617918, 69.79275706135233293 ) ) ;
#109329=CARTESIAN_POINT ( 'NONE',  ( 9.564922557960805705, 16.46253265017160317, 74.58224293864769550 ) ) ;
#109330=CARTESIAN_POINT ( 'NONE',  ( 21.55341960407619695, -5.719274019375665929, 81.04275706135236135 ) ) ;
#109331=CARTESIAN_POINT ( 'NONE',  ( 21.53943276465977519, -0.05219959533907433946, 83.74890960531435269 ) ) ;
#109332=CARTESIAN_POINT ( 'NONE',  ( 16.52544592524342804, -4.483927247898539470, 68.54057627198103830 ) ) ;
#109333=CARTESIAN_POINT ( 'NONE',  ( 18.67979575497194134, -10.72451020669871369, 105.8344237280190328 ) ) ;
#109334=CARTESIAN_POINT ( 'NONE',  ( -12.06949235617756955, 12.14591786802309770, 80.62390960531438111 ) ) ;
#109335=CARTESIAN_POINT ( 'NONE',  ( -19.05341960407611168, -5.049401038298163336, 31.45724293864769550 ) ) ;
#109336=CARTESIAN_POINT ( 'NONE',  ( -9.474510206698720793, -16.51473224551083518, 69.58442372801901854 ) ) ;
#109337=CARTESIAN_POINT ( 'NONE',  ( 16.53943276465976808, -0.05219959533910856209, 38.74890960531435979 ) ) ;
#109338=CARTESIAN_POINT ( 'NONE',  ( -10.81492255796105439, 18.62759615963255655, 97.91775706135236135 ) ) ;
#109339=CARTESIAN_POINT ( 'NONE',  ( 19.02544592524343514, -5.153800228976328945, 98.54057627198100988 ) ) ;
#109340=CARTESIAN_POINT ( 'NONE',  ( 5.049401038297881783, 19.05341960407617563, 62.29275706135234003 ) ) ;
#109341=CARTESIAN_POINT ( 'NONE',  ( -15.80617190586745835, -15.72974639402198527, 66.87390960531436690 ) ) ;
#109342=CARTESIAN_POINT ( 'NONE',  ( -21.53943276465977519, -0.05219959533937600094, 23.75109039468567929 ) ) ;
#109343=CARTESIAN_POINT ( 'NONE',  ( -5.153800228976607833, 19.02544592524334988, 112.7094237280190043 ) ) ;
#109344=CARTESIAN_POINT ( 'NONE',  ( 16.52544592524335698, 4.483927247898782831, 81.45942372801900433 ) ) ;
#109346=CARTESIAN_POINT ( 'NONE',  ( -15.80617190586768217, 15.72974639402176855, 28.12609039468568284 ) ) ;
#109347=CARTESIAN_POINT ( 'NONE',  ( 16.55341960407611168, 4.379528057220329451, 108.9572429386476955 ) ) ;
#109349=CARTESIAN_POINT ( 'NONE',  ( 8.224510206698742110, 14.34966873604972548, 52.08442372801901854 ) ) ;
#109350=CARTESIAN_POINT ( 'NONE',  ( -10.81492255796078084, -18.62759615963271287, 67.08224293864770971 ) ) ;
#109351=CARTESIAN_POINT ( 'NONE',  ( 4.483927247898790824, -16.52544592524335698, 100.2094237280190043 ) ) ;
#109352=CARTESIAN_POINT ( 'NONE',  ( 12.06949235617739724, 12.14591786802326823, 31.87609039468567929 ) ) ;
#109353=CARTESIAN_POINT ( 'NONE',  ( -9.564922557960796823, -16.46253265017161027, 27.08224293864769550 ) ) ;
#109354=CARTESIAN_POINT ( 'NONE',  ( -16.53943276465976808, -0.05219959533934237506, 78.75109039468568994 ) ) ;
#109355=CARTESIAN_POINT ( 'NONE',  ( -9.564922557961040184, 16.46253265017147172, 77.91775706135234714 ) ) ;
#109356=CARTESIAN_POINT ( 'NONE',  ( -5.719274019375978568, 21.55341960407610458, 70.20724293864769550 ) ) ;
#109357=CARTESIAN_POINT ( 'NONE',  ( -8.224510206698735004, -14.34966873604973081, 94.58442372801901854 ) ) ;
#109358=CARTESIAN_POINT ( 'NONE',  ( -15.72974639402176322, -15.80617190586768395, 84.37609039468570415 ) ) ;
#109359=CARTESIAN_POINT ( 'NONE',  ( -0.05219959533907301413, -21.53943276465977519, 67.49890960531436690 ) ) ;
#109360=CARTESIAN_POINT ( 'NONE',  ( 15.72974639402199770, -15.80617190586745480, 48.12390960531436690 ) ) ;
#109362=CARTESIAN_POINT ( 'NONE',  ( 0.05219959533934541429, -16.53943276465976808, 85.00109039468568994 ) ) ;
#109363=CARTESIAN_POINT ( 'NONE',  ( -0.05219959533907301413, -21.53943276465977519, 47.49890960531435979 ) ) ;
#109365=CARTESIAN_POINT ( 'NONE',  ( -13.97604488694527625, -13.89961937509977652, 111.8739096053143243 ) ) ;
#109367=CARTESIAN_POINT ( 'NONE',  ( 19.02544592524343514, -5.153800228976328945, 28.54057627198102409 ) ) ;
#109368=CARTESIAN_POINT ( 'NONE',  ( -5.823673210054116645, -21.52544592524344225, 57.29057627198103120 ) ) ;
#109369=CARTESIAN_POINT ( 'NONE',  ( -16.52544592524335698, -4.483927247898792601, 103.9594237280190185 ) ) ;
#109370=CARTESIAN_POINT ( 'NONE',  ( 21.53943276465977519, 0.05219959533937863772, 41.25109039468568284 ) ) ;
#109371=CARTESIAN_POINT ( 'NONE',  ( 0.05219959533936267826, -19.03943276465977164, 100.0010903946856757 ) ) ;
#109372=CARTESIAN_POINT ( 'NONE',  ( -19.05341960407611168, -5.049401038298163336, 26.45724293864769550 ) ) ;
#109373=CARTESIAN_POINT ( 'NONE',  ( -9.474510206698720793, -16.51473224551083518, 109.5844237280190043 ) ) ;
#109374=CARTESIAN_POINT ( 'NONE',  ( 9.474510206698971260, -16.51473224551069308, 42.91557627198103120 ) ) ;
#109376=CARTESIAN_POINT ( 'NONE',  ( 9.474510206698971260, -16.51473224551069308, 97.91557627198102409 ) ) ;
#109378=CARTESIAN_POINT ( 'NONE',  ( 16.53943276465976808, 0.05219959533934440121, 76.25109039468568994 ) ) ;
#109379=B_SPLINE_CURVE_WITH_KNOTS ( 'NONE', 3,
 ( #96958, #175816, #6940, #20129, #68619, #33324 ),
 .UNSPECIFIED., .F., .F.,
 ( 4, 2, 4 ),
 ( 0.003239945802372283350, 0.003620412082092137277, 0.004000878361811991205 ),
 .UNSPECIFIED. ) ;
#109380=CARTESIAN_POINT ( 'NONE',  ( 0.05219959533936267826, -19.03943276465977164, 85.00109039468567573 ) ) ;
#109381=CARTESIAN_POINT ( 'NONE',  ( -19.02544592524334988, -5.153800228976617603, 18.95942372801899722 ) ) ;
#109382=CARTESIAN_POINT ( 'NONE',  ( -18.67979575497178146, -10.72451020669898902, 66.66557627198102409 ) ) ;
#109383=CARTESIAN_POINT ( 'NONE',  ( 14.34966873604972726, -8.224510206698740333, 90.83442372801901854 ) ) ;
#109384=CARTESIAN_POINT ( 'NONE',  ( -19.02544592524334988, -5.153800228976617603, 83.95942372801901854 ) ) ;
#109385=CARTESIAN_POINT ( 'NONE',  ( -9.564922557960796823, -16.46253265017161027, 42.08224293864769550 ) ) ;
#109386=CARTESIAN_POINT ( 'NONE',  ( -9.474510206698964154, 16.51473224551069663, 75.41557627198103830 ) ) ;
#109387=CARTESIAN_POINT ( 'NONE',  ( -10.81492255796105439, 18.62759615963255655, 52.91775706135235424 ) ) ;
#109388=CARTESIAN_POINT ( 'NONE',  ( 9.564922557960805705, 16.46253265017160317, 44.58224293864769550 ) ) ;
#109389=CARTESIAN_POINT ( 'NONE',  ( 0.05219959533936267826, -19.03943276465977164, 75.00109039468566152 ) ) ;
#109391=CARTESIAN_POINT ( 'NONE',  ( 5.049401038298161559, -19.05341960407611168, 107.7072429386476955 ) ) ;
#109392=CARTESIAN_POINT ( 'NONE',  ( 8.224510206698953496, -14.34966873604960469, 62.91557627198102409 ) ) ;
#109393=CARTESIAN_POINT ( 'NONE',  ( 10.81492255796078972, 18.62759615963270932, 59.58224293864770260 ) ) ;
#109395=CARTESIAN_POINT ( 'NONE',  ( -19.03943276465977164, -0.05219959533935918106, 38.75109039468566152 ) ) ;
#109396=CARTESIAN_POINT ( 'NONE',  ( -17.72696623605160582, 5.500000000000055955, 88.59811031808420978 ) ) ;
#109397=CARTESIAN_POINT ( 'NONE',  ( -19.02544592524342804, 5.153800228976336051, 61.04057627198103120 ) ) ;
#109398=CARTESIAN_POINT ( 'NONE',  ( -16.51473224551069308, -9.474510206698971260, 71.66557627198102409 ) ) ;
#109399=CARTESIAN_POINT ( 'NONE',  ( 0.05219959533934541429, -16.53943276465976808, 45.00109039468568284 ) ) ;
#109402=CARTESIAN_POINT ( 'NONE',  ( -16.55341960407617563, 4.379528057220093196, 93.54275706135234714 ) ) ;
#109403=EDGE_CURVE ( 'NONE', #184582, #154217, #143554, .T. ) ;
#109404=CARTESIAN_POINT ( 'NONE',  ( 17.97058386085787163, 5.500000000000006217, 96.50390968646217971 ) ) ;
#109405=CARTESIAN_POINT ( 'NONE',  ( 4.483927247898790824, -16.52544592524335698, 65.20942372801901854 ) ) ;
#109406=CARTESIAN_POINT ( 'NONE',  ( 16.52544592524335698, 4.483927247898782831, 46.45942372801901854 ) ) ;
#109407=CARTESIAN_POINT ( 'NONE',  ( -13.89961937509957401, -13.97604488694547875, 24.37609039468565442 ) ) ;
#109408=CARTESIAN_POINT ( 'NONE',  ( -0.05219959533909027116, -19.03943276465977164, 52.49890960531436690 ) ) ;
#109410=CARTESIAN_POINT ( 'NONE',  ( -10.72451020669870658, -18.67979575497194134, 54.58442372801901143 ) ) ;
#109411=CARTESIAN_POINT ( 'NONE',  ( -16.51473224551082808, 9.474510206698731452, 63.33442372801900433 ) ) ;
#109412=CARTESIAN_POINT ( 'NONE',  ( 21.53943276465977519, 0.05219959533937863772, 106.2510903946856757 ) ) ;
#109413=CARTESIAN_POINT ( 'NONE',  ( -16.46253265017160317, 9.564922557960807481, 35.83224293864768839 ) ) ;
#109415=CARTESIAN_POINT ( 'NONE',  ( 21.55341960407610458, 5.719274019375980345, 53.95724293864770260 ) ) ;
#109416=CARTESIAN_POINT ( 'NONE',  ( 10.72451020669898902, -18.67979575497178502, 27.91557627198103830 ) ) ;
#109417=CARTESIAN_POINT ( 'NONE',  ( -4.483927247898539470, -16.52544592524342804, 97.29057627198105251 ) ) ;
#109418=CARTESIAN_POINT ( 'NONE',  ( 14.34966873604972726, -8.224510206698740333, 30.83442372801902209 ) ) ;
#109419=CARTESIAN_POINT ( 'NONE',  ( 14.29746914071049879, -8.314922557960816363, 28.33224293864769550 ) ) ;
#109421=CARTESIAN_POINT ( 'NONE',  ( -15.72974639402197994, 15.80617190586746368, 110.6239096053143669 ) ) ;
#109422=CARTESIAN_POINT ( 'NONE',  ( -8.224510206698948167, 14.34966873604960824, 35.41557627198102409 ) ) ;
#109423=CARTESIAN_POINT ( 'NONE',  ( 9.564922557960805705, 16.46253265017160317, 114.5822429386476955 ) ) ;
#109424=CARTESIAN_POINT ( 'NONE',  ( 16.46253265017146816, 9.564922557961045513, 106.6677570613523471 ) ) ;
#109425=CARTESIAN_POINT ( 'NONE',  ( -16.46253265017146816, -9.564922557961047289, 24.16775706135233648 ) ) ;
#109426=CARTESIAN_POINT ( 'NONE',  ( -16.55341960407611168, -4.379528057220339221, 31.45724293864769550 ) ) ;
#109427=CARTESIAN_POINT ( 'NONE',  ( 10.81492255796078972, 18.62759615963270932, 109.5822429386476955 ) ) ;
#109428=CARTESIAN_POINT ( 'NONE',  ( 16.20579543436681647, 7.371946100354974440, 33.06520834171879386 ) ) ;
#109429=CARTESIAN_POINT ( 'NONE',  ( 0.05219959533907565091, 21.53943276465977519, 64.99890960531435269 ) ) ;
#109430=CARTESIAN_POINT ( 'NONE',  ( -19.02544592524342804, 5.153800228976336051, 76.04057627198102409 ) ) ;
#109431=CARTESIAN_POINT ( 'NONE',  ( 14.34966873604960469, 8.224510206698951720, 54.16557627198103120 ) ) ;
#109432=CARTESIAN_POINT ( 'NONE',  ( -16.46253265017160317, 9.564922557960807481, 95.83224293864769550 ) ) ;
#109433=CARTESIAN_POINT ( 'NONE',  ( 16.46253265017146816, 9.564922557961045513, 56.66775706135233293 ) ) ;
#109434=CARTESIAN_POINT ( 'NONE',  ( 18.62759615963271287, -10.81492255796078972, 98.33224293864769550 ) ) ;
#109435=CARTESIAN_POINT ( 'NONE',  ( 14.34966873604960469, 8.224510206698951720, 94.16557627198103830 ) ) ;
#109436=CARTESIAN_POINT ( 'NONE',  ( 5.719274019375673035, 21.55341960407619339, 42.29275706135235424 ) ) ;
#109438=CARTESIAN_POINT ( 'NONE',  ( -14.34966873604960291, -8.224510206698953496, 26.66557627198103475 ) ) ;
#109439=CARTESIAN_POINT ( 'NONE',  ( -0.05219959533909027116, -19.03943276465977164, 32.49890960531435979 ) ) ;
#109440=CARTESIAN_POINT ( 'NONE',  ( 0.05219959533909260263, 19.03943276465977164, 79.99890960531436690 ) ) ;
#109441=CARTESIAN_POINT ( 'NONE',  ( 21.53943276465977519, -0.05219959533907433946, 63.74890960531435979 ) ) ;
#109442=CARTESIAN_POINT ( 'NONE',  ( -19.01533133064926062, 5.499999999999455547, 43.76586590595741200 ) ) ;
#109443=CARTESIAN_POINT ( 'NONE',  ( -9.564922557960796823, -16.46253265017161027, 32.08224293864769550 ) ) ;
#109444=CARTESIAN_POINT ( 'NONE',  ( 18.62759615963271287, -10.81492255796078972, 48.33224293864770260 ) ) ;
#109445=CARTESIAN_POINT ( 'NONE',  ( -15.72974639402176322, -15.80617190586768395, 74.37609039468568994 ) ) ;
#109447=CARTESIAN_POINT ( 'NONE',  ( 12.14591786802327356, -12.06949235617739191, 75.62609039468567573 ) ) ;
#109448=CARTESIAN_POINT ( 'NONE',  ( -9.564922557960796823, -16.46253265017161027, 62.08224293864769550 ) ) ;
#109449=CARTESIAN_POINT ( 'NONE',  ( 9.564922557960805705, 16.46253265017160317, 69.58224293864770971 ) ) ;
#109451=CARTESIAN_POINT ( 'NONE',  ( -18.62759615963255300, -10.81492255796106328, 109.1677570613523613 ) ) ;
#109452=CARTESIAN_POINT ( 'NONE',  ( -8.314922557961024197, 14.29746914071037800, 77.91775706135231871 ) ) ;
#109453=CARTESIAN_POINT ( 'NONE',  ( -15.72974639402176322, -15.80617190586768395, 94.37609039468568994 ) ) ;
#109454=CARTESIAN_POINT ( 'NONE',  ( -19.03943276465977164, 0.05219959533909376836, 71.24890960531435269 ) ) ;
#109455=CARTESIAN_POINT ( 'NONE',  ( 5.719274019375991003, -21.55341960407610458, 37.70724293864769550 ) ) ;
#109456=CARTESIAN_POINT ( 'NONE',  ( -19.02544592524334988, -5.153800228976617603, 108.9594237280189759 ) ) ;
#109457=CARTESIAN_POINT ( 'NONE',  ( 5.823673210054444382, -21.52544592524334988, 80.20942372801901854 ) ) ;
#109458=CARTESIAN_POINT ( 'NONE',  ( -8.224510206698735004, -14.34966873604973081, 44.58442372801901854 ) ) ;
#109459=CARTESIAN_POINT ( 'NONE',  ( 21.53943276465977519, -0.05219959533907433946, 93.74890960531436690 ) ) ;
#109460=CARTESIAN_POINT ( 'NONE',  ( -12.14591786802326823, 12.06949235617739902, 23.12609039468567573 ) ) ;
#109461=CARTESIAN_POINT ( 'NONE',  ( -9.564922557960796823, -16.46253265017161027, 77.08224293864769550 ) ) ;
#109462=CARTESIAN_POINT ( 'NONE',  ( 16.46253265017146816, 9.564922557961045513, 111.6677570613523329 ) ) ;
#109463=CARTESIAN_POINT ( 'NONE',  ( -13.89961937509977652, 13.97604488694528158, 40.62390960531435979 ) ) ;
#109464=CARTESIAN_POINT ( 'NONE',  ( -0.05219959533936034679, 19.03943276465977164, 112.5010903946856757 ) ) ;
#109465=CARTESIAN_POINT ( 'NONE',  ( -14.29746914071049879, 8.314922557960819915, 65.83224293864769550 ) ) ;
#109466=CARTESIAN_POINT ( 'NONE',  ( 12.06949235617739724, 12.14591786802326823, 71.87609039468568994 ) ) ;
#109467=CARTESIAN_POINT ( 'NONE',  ( 21.52544592524334988, 5.823673210054432836, 26.45942372801901854 ) ) ;
#109468=CARTESIAN_POINT ( 'NONE',  ( -16.46253265017160317, 9.564922557960807481, 45.83224293864769550 ) ) ;
#109469=CARTESIAN_POINT ( 'NONE',  ( 5.153800228976335163, 19.02544592524342804, 64.79057627198100988 ) ) ;
#109470=CARTESIAN_POINT ( 'NONE',  ( 16.52544592524335698, 4.483927247898782831, 76.45942372801901854 ) ) ;
#109472=VERTEX_POINT ( 'NONE', #135897 ) ;
#109474=CARTESIAN_POINT ( 'NONE',  ( 5.823673210054444382, -21.52544592524334988, 110.2094237280190185 ) ) ;
#109475=EDGE_CURVE ( 'NONE', #104654, #111651, #59036, .T. ) ;
#109476=CARTESIAN_POINT ( 'NONE',  ( 13.89961937509977652, -13.97604488694527269, 33.12390960531434558 ) ) ;
#109477=CARTESIAN_POINT ( 'NONE',  ( -19.05341960407611168, -5.049401038298163336, 101.4572429386476955 ) ) ;
#109478=ORIENTED_EDGE ( 'NONE', *, *, #61610, .F. ) ;
#109479=CARTESIAN_POINT ( 'NONE',  ( 14.29746914071037800, 8.314922557961029526, 31.66775706135234358 ) ) ;
#109481=CARTESIAN_POINT ( 'NONE',  ( -19.02544592524334988, -5.153800228976617603, 63.95942372801899012 ) ) ;
#109482=CARTESIAN_POINT ( 'NONE',  ( 8.224510206698742110, 14.34966873604972548, 37.08442372801901143 ) ) ;
#109483=CARTESIAN_POINT ( 'NONE',  ( -19.02544592524342804, 5.153800228976336051, 41.04057627198103120 ) ) ;
#109484=CARTESIAN_POINT ( 'NONE',  ( 9.474510206698971260, -16.51473224551069308, 107.9155762719810383 ) ) ;
#109485=CARTESIAN_POINT ( 'NONE',  ( -19.02544592524342804, 5.153800228976336051, 66.04057627198103830 ) ) ;
#109486=CARTESIAN_POINT ( 'NONE',  ( -15.72974639402197994, 15.80617190586746368, 105.6239096053143669 ) ) ;
#109487=CARTESIAN_POINT ( 'NONE',  ( 9.564922557960805705, 16.46253265017160317, 94.58224293864769550 ) ) ;
#109488=FACE_OUTER_BOUND ( 'NONE', #133513, .T. ) ;
#109489=CARTESIAN_POINT ( 'NONE',  ( 13.97604488694527802, 13.89961937509977652, 69.37390960531436690 ) ) ;
#109490=CARTESIAN_POINT ( 'NONE',  ( 14.34966873604960469, 8.224510206698951720, 24.16557627198103120 ) ) ;
#109492=CARTESIAN_POINT ( 'NONE',  ( -19.03943276465977164, -0.05219959533935918106, 98.75109039468567573 ) ) ;
#109493=CARTESIAN_POINT ( 'NONE',  ( -5.049401038297874678, -19.05341960407617918, 29.79275706135232227 ) ) ;
#109495=CARTESIAN_POINT ( 'NONE',  ( 8.314922557960818139, 14.29746914071049879, 54.58224293864769550 ) ) ;
#109496=CARTESIAN_POINT ( 'NONE',  ( -5.823673210054431948, 21.52544592524334988, 92.70942372801901854 ) ) ;
#109497=CARTESIAN_POINT ( 'NONE',  ( -19.05341960407611168, -5.049401038298163336, 31.45724293864769550 ) ) ;
#109498=CARTESIAN_POINT ( 'NONE',  ( -4.483927247898539470, -16.52544592524342804, 27.29057627198103120 ) ) ;
#109499=CARTESIAN_POINT ( 'NONE',  ( -21.52544592524334988, -5.823673210054445271, 83.95942372801900433 ) ) ;
#109500=CARTESIAN_POINT ( 'NONE',  ( -0.05219959533909027116, -19.03943276465977164, 77.49890960531435269 ) ) ;
#109501=CARTESIAN_POINT ( 'NONE',  ( 19.05341960407611168, 5.049401038298154454, 98.95724293864766707 ) ) ;
#109502=CARTESIAN_POINT ( 'NONE',  ( -4.379528057220328563, 16.55341960407611168, 100.2072429386476955 ) ) ;
#109503=CARTESIAN_POINT ( 'NONE',  ( 4.483927247898545687, 16.52544592524342804, 64.79057627198103830 ) ) ;
#109504=CARTESIAN_POINT ( 'NONE',  ( -18.67979575497178146, -10.72451020669898902, 76.66557627198103830 ) ) ;
#109505=CARTESIAN_POINT ( 'NONE',  ( 13.89961937509977652, -13.97604488694527269, 73.12390960531436690 ) ) ;
#109506=CARTESIAN_POINT ( 'NONE',  ( -15.80617190586745835, -15.72974639402198527, 86.87390960531438111 ) ) ;
#109507=CARTESIAN_POINT ( 'NONE',  ( 9.474510206698729675, 16.51473224551082808, 82.08442372801899012 ) ) ;
#109508=CARTESIAN_POINT ( 'NONE',  ( -0.05219959533936034679, 19.03943276465977164, 32.50109039468566863 ) ) ;
#109509=CARTESIAN_POINT ( 'NONE',  ( -16.55341960407611168, -4.379528057220339221, 86.45724293864770971 ) ) ;
#109510=CARTESIAN_POINT ( 'NONE',  ( -19.02544592524342804, 5.153800228976336051, 61.04057627198103120 ) ) ;
#109511=CARTESIAN_POINT ( 'NONE',  ( -10.81492255796078084, -18.62759615963271287, 67.08224293864770971 ) ) ;
#109512=CARTESIAN_POINT ( 'NONE',  ( 16.20579543436675252, -7.371946100355229348, 26.93479165828123811 ) ) ;
#109513=CARTESIAN_POINT ( 'NONE',  ( 8.224510206698953496, -14.34966873604960469, 22.91557627198102765 ) ) ;
#109515=CARTESIAN_POINT ( 'NONE',  ( 19.02544592524334988, 5.153800228976608722, 101.4594237280189759 ) ) ;
#109516=CARTESIAN_POINT ( 'NONE',  ( 16.52544592524342804, -4.483927247898539470, 78.54057627198103830 ) ) ;
#109518=CARTESIAN_POINT ( 'NONE',  ( 13.89961937509977652, -13.97604488694527269, 78.12390960531433848 ) ) ;
#109519=CARTESIAN_POINT ( 'NONE',  ( -16.51473224551069308, -9.474510206698971260, 31.66557627198102054 ) ) ;
#109520=CARTESIAN_POINT ( 'NONE',  ( -8.314922557960811034, -14.29746914071050412, 67.08224293864770971 ) ) ;
#109521=CARTESIAN_POINT ( 'NONE',  ( 5.049401038298161559, -19.05341960407611168, 107.7072429386476955 ) ) ;
#109522=CARTESIAN_POINT ( 'NONE',  ( 13.97604488694548053, -13.89961937509957401, 95.62609039468563310 ) ) ;
#109523=CARTESIAN_POINT ( 'NONE',  ( 13.89961937509977652, -13.97604488694527269, 68.12390960531436690 ) ) ;
#109524=CARTESIAN_POINT ( 'NONE',  ( 19.03943276465977164, -0.05219959533909143690, 88.74890960531436690 ) ) ;
#109525=CARTESIAN_POINT ( 'NONE',  ( 5.823673210054125526, 21.52544592524343514, 74.79057627198105251 ) ) ;
#109526=CARTESIAN_POINT ( 'NONE',  ( -14.29746914071037622, -8.314922557961029526, 74.16775706135231871 ) ) ;
#109527=CARTESIAN_POINT ( 'NONE',  ( -17.49999999999999645, 5.499999999999992895, 93.71769037696437010 ) ) ;
#109528=CARTESIAN_POINT ( 'NONE',  ( 16.51473224551069308, 9.474510206698969483, 64.16557627198102409 ) ) ;
#109529=CARTESIAN_POINT ( 'NONE',  ( 21.52544592524344225, -5.823673210054117533, 68.54057627198103830 ) ) ;
#109530=CARTESIAN_POINT ( 'NONE',  ( 0.05219959533936267826, -19.03943276465977164, 90.00109039468567573 ) ) ;
#109531=CARTESIAN_POINT ( 'NONE',  ( 16.52544592524342804, -4.483927247898539470, 38.54057627198103120 ) ) ;
#109532=CARTESIAN_POINT ( 'NONE',  ( 21.52544592524334988, 5.823673210054432836, 41.45942372801901143 ) ) ;
#109534=CARTESIAN_POINT ( 'NONE',  ( 12.14591786802327356, -12.06949235617739191, 75.62609039468567573 ) ) ;
#109535=CARTESIAN_POINT ( 'NONE',  ( -5.153800228976328057, -19.02544592524343514, 102.2905762719810383 ) ) ;
#109536=CARTESIAN_POINT ( 'NONE',  ( 9.474510206698971260, -16.51473224551069308, 102.9155762719810241 ) ) ;
#109538=CARTESIAN_POINT ( 'NONE',  ( -4.483927247898782831, 16.52544592524335698, 87.70942372801901854 ) ) ;
#109539=CARTESIAN_POINT ( 'NONE',  ( 16.55341960407618274, -4.379528057220086978, 46.04275706135234714 ) ) ;
#109540=CARTESIAN_POINT ( 'NONE',  ( -16.46253265017160317, 9.564922557960807481, 60.83224293864769550 ) ) ;
#109541=CARTESIAN_POINT ( 'NONE',  ( -16.46253265017160317, 9.564922557960807481, 55.83224293864769550 ) ) ;
#109542=CARTESIAN_POINT ( 'NONE',  ( 5.823673210054444382, -21.52544592524334988, 50.20942372801901854 ) ) ;
#109543=CARTESIAN_POINT ( 'NONE',  ( 12.06949235617739724, 12.14591786802326823, 61.87609039468568284 ) ) ;
#109544=CARTESIAN_POINT ( 'NONE',  ( -14.29746914071049879, 8.314922557960819915, 30.83224293864770260 ) ) ;
#109545=CARTESIAN_POINT ( 'NONE',  ( 13.89961937509977652, -13.97604488694527269, 48.12390960531435979 ) ) ;
#109546=CARTESIAN_POINT ( 'NONE',  ( 19.05341960407611168, 5.049401038298154454, 28.95724293864769550 ) ) ;
#109547=CARTESIAN_POINT ( 'NONE',  ( 4.379528057220092307, 16.55341960407617563, 32.29275706135235424 ) ) ;
#109548=( BOUNDED_SURFACE ( )  B_SPLINE_SURFACE ( 3, 2, ( 
 ( #95109, #126442, #140617, #174948, #50611, #37420, #129413, #156798, #112270, #173962, #2107, #18291, #17287, #98064, #159763, #21258, #82913, #63788, #79946, #3103, #64781, #119269, #145592, #70764, #9097, #23264, #25281, #177951, #26272, #178954, #102095, #103096, #195116, #117262, #180952, #7071, #132432, #194124, #84908, #86924, #39419, #87914, #40424, #163780, #164778, #22260, #130409, #41430, #147609, #162763, #148606, #10098, #54587, #38428, #71758, #133428, #57600, #56599, #149601, #24272, #85921, #83909, #118273, #68752, #55587, #192107, #179964, #11098, #100084, #53590, #72774, #131427, #134444, #196129, #42430, #160770, #115266, #176959, #161769, #146587, #8081, #101078, #69757, #193113, #116260, #157311, #172481, #186680, #120244, #33969, #78461, #17814, #185661, #123963, #140135, #48150, #198094, #95626, #3611, #59559, #155323, #63304, #124983, #136414, #188657, #109807, #93637, #142126, #150610, #12106, #170490, #18808, #73769, #94633, #65290, #171490, #181935, #32979, #79471, #80453, #126949, #1627, #187672, #104092, #156312, #47153, #31981, #28274, #165775, #27269, #135442, #64306, #88918, #141139, #2629, #43417, #125973, #49142, #110800, #16811, #89913, #197111, #13086, #58578, #105087, #108811, #166773, #151595, #74751, #144117, #5597, #173484, #4593, #100605, #83433, #145110, #84430, #128935, #36935, #161288, #66286, #191623, #158298, #53102, #37948, #127945, #19787, #146107, #114781, #192634, #115790, #98598, #81428, #22782, #111796, #176474, #85437, #34957, #143114, #20773, #113768, #70288, #7591, #50137, #131956, #82429, #96609, #69277, #130944, #189647, #54116, #21782, #99608, #177479, #51122, #23787, #112781, #174474, #38948, #6593, #162287, #35943, #147128, #97589, #8615, #68272, #159277, #67277, #160291, #190636, #52111, #175464, #129923, #116782, #194641, #43936, #152105, #10624, #42949, #39940, #182455, #13589, #74284, #27798, #178473, #102623, #24798, #58117, #103626, #86446, #101609, #120756, #195654, #12620, #134970, #163299, #196647, #105597, #57126, #148132, #87448, #72285, #9623, #119787, #132953, #40951, #166301, #167283, #71288, #179487, #56111, #117792, #55112, #89439, #41960, #28781, #164309, #90420, #151127, #75256, #133962, #25802, #135954, #180488, #118800, #150131, #181471, #149133, #165302, #104613, #197624, #193640, #59089, #26795, #88437, #11633, #73300, #1377, #121750, #384, #44927, #108570, #78217, #76240, #106583, #185418, #107564, #110552, #32733, #109563, #168260, #171244, #170247, #63056, #186433, #29756, #172233, #91391, #18562, #47909, #31741, #124736, #199601, #94385, #183442, #79222, #93389, #61068, #153080, #46909, #169242, #184431, #14582, #64060, #60082, #137918, #187429, #95380, #154083, #156064, #122740, #125730, #157066, #17562, #140892, #45911, #30748, #92397, #2381, #155075, #15577, #77235, #48897, #138904, #33718, #139888, #62056, #136927, #198614, #123721, #16570, #174233, #159035, #96368, #83192, #19546, #127704, #52854, #130695, #173235, #66037, #158056, #81191, #141881, #114525, #128694, #69030, #3372, #115546, #191378, #177234, #37695, #190391, #20528, #176226, #97349, #34711, #67035, #65047, #82176, #51866, #99359, #7345, #192389, #160044, #53872, #68029, #142872, #143872, #21531, #126703, #161042, #188407, #38706, #5351, #22536, #144866, #100363, #162042, #4352, #6349, #49885, #129680, #84183, #189404, #111550, #145863, #80210, #50881, #112539, #113526, #35702, #175220, #36685, #98345, #58847, #85184, #193390, #194396, #87204, #43690, #196404, #23538, #105352, #55864, #146873, #101354, #26546, #165053, #120514, #11379, #27550, #25560, #148885, #8365, #88190, #70040, #10376, #131709, #195398, #149874, #163043, #54866, #72033, #117538, #197382, #119546, #134721, #181229, #116540, #180241, #133706, #56876, #178228, #40702, #74040, #182206, #118550, #135711, #89190, #103375, #39692, #150883, #41710, #57874, #102372, #164061 ),
 ( #24550, #86200, #147890, #73049, #9376, #71041, #42705, #132708, #104366, #179236, #166050, #12378, #140651, #2141, #143, #47668, #187190, #170004, #184189, #92150, #91151, #48661, #63820, #75015, #124491, #28541, #61812, #1135, #44682, #93148, #62809, #186187, #30499, #152840, #198362, #75999, #90177, #154832, #107322, #125493, #17321, #183200, #60824, #122498, #151860, #121506, #78976, #123482, #185174, #109320, #45671, #153836, #77980, #171000, #46665, #167039, #13351, #76991, #15333, #29517, #31495, #168995, #32492, #94145, #155824, #136680, #138662, #59837, #106335, #108324, #16330, #139647, #168021, #14334, #137673, #199359, #99115, #33483, #145626, #21292, #7106, #67792, #158796, #189169, #144627, #127463, #64813, #97113, #95141, #50641, #20285, #82949, #37454, #160807, #190149, #22295, #98099, #3138, #173993, #51624, #171995, #129448, #156830, #68787, #112303, #6110, #174980, #130445, #192144, #126474, #113289, #18323, #36444, #159797, #188172, #79980, #191147, #52621, #114283, #175986, #81931, #141648, #83946, #49645, #110313, #111308, #172997, #34475, #80961, #35462, #96134, #157823, #19313, #142637, #4115, #65794, #143623, #5108, #66789, #128453, #25317, #118308, #103132, #146622, #27307, #23297, #135478, #164813, #86959, #180000, #116294, #26309, #38463, #196164, #10133, #177984, #8115, #163815, #24307, #101112, #161802, #180988, #176993, #54619, #104128, #12142, #70799, #87949, #100119, #42465, #73806, #134479, #149637, #84941, #162798, #69792, #41467, #148644, #131460, #193147, #165810, #55622, #72810, #195153, #39451, #56635, #88955, #117295, #85956, #147644, #132467, #9133, #11135, #194158, #178990, #57638, #150645, #40458, #102131, #71794, #133463, #115300, #119304, #53624, #75760, #31260, #14093, #151629, #183949, #181972, #137438, #107088, #169767, #124251, #47431, #76755, #109087, #184939, #89949, #60584, #138430, #58613, #154597, #120280, #155592, #199117, #92911, #61579, #17087, #78740, #13123, #200111, #105123, #123248, #46424, #74786, #166809, #16093, #108082, #139417, #62573, #45435, #28309, #77751, #43454, #899, #32256, #136448, #198129, #167787, #122260, #197147, #185947, #59597, #121271, #29286, #182965, #170767, #93914, #44448, #106102, #168759, #90917, #152603, #30262, #91906, #153599, #15096, #51396, #112075, #4876, #2903, #113056, #125260, #82708, #96885, #64581, #33253, #50416, #111074, #187942, #48429, #67553, #63586, #141415, #190908, #98873, #157588, #189921, #186958, #129210, #160569, #21052, #174748, #110085, #49411, #171764, #66559, #173764, #94911, #156596, #52385, #142407, #159555, #81701, #18091, #143384, #114042, #3885, #79746, #34244, #19080, #126246, #128224, #172763, #95904, #36212, #175740, #80728, #65564, #127224, #188938, #1907, #97865, #35231, #37217, #158568, #22058, #144391, #140416, #20057, #5876, #147404, #134241, #130204, #71556, #119074, #25073, #99882, #86716, #194912, #57402, #180756, #117053, #164575, #103893, #148401, #100876, #8892, #7872, #165573, #42232, #191899, #41229, #145387, #178748, #118069, #161567, #9895, #179759, #102890, #70560, #69558, #115062, #192913, #6869, #133221, #24063, #83709, #195926, #23060, #177751, #39220, #68548, #38227, #53384, #40212, #101891, #26069, #162558, #132227, #56387, #87712, #163573, #176754, #84705, #193920, #55383, #146384, #149398, #85718, #10893, #72566, #131223, #54390, #116063, #196917, #107844, #13864, #29056, #183723, #153364, #121034, #104887, #30035, #168537, #124005, #14866, #31028, #90696, #152379, #150413, #91673, #11908, #75531, #135245, #198892, #76527, #166575, #58384, #137206, #197896, #665, #123021, #138204, #184706, #73572, #45209, #60360, #122033, #120051, #44216, #77518, #62335, #106863, #139190, #92678, #199886, #43219, #154366, #61350, #46191, #105875, #167562, #169528, #15860, #182732, #185703, #47192, #108852, #27072, #88718, #181738, #59365, #28075, #89716, #151401 ),
 ( #12891, #74554, #136221, #20810, #128974, #187709, #19824, #16852, #159315, #190673, #51159, #4632, #155363, #79509, #1669, #34993, #80492, #63347, #78503, #97626, #172523, #189686, #111833, #140176, #173522, #82466, #34008, #125024, #64345, #49181, #186720, #96647, #109845, #17853, #143151, #144152, #48190, #156352, #171530, #33018, #32022, #66322, #18847, #5637, #93680, #67314, #81465, #52149, #127983, #142166, #110839, #112819, #95665, #94673, #157352, #141178, #3650, #65328, #174512, #170532, #2668, #50176, #126014, #158335, #126988, #188695, #35979, #175501, #74076, #36974, #75051, #133742, #89227, #181265, #136717, #198398, #68311, #57910, #21820, #119582, #104404, #191662, #83472, #150921, #42742, #58884, #182243, #165089, #145149, #12414, #98635, #166086, #151897, #160330, #6633, #87239, #180277, #113806, #135747, #129962, #53141, #148922, #114820, #197418, #120550, #176512, #43728, #88226, #27589, #105390, #40739, #90214, #102409, #164096, #167076, #149910, #10411, #195437, #25595, #28578, #72069, #56912, #13387, #118587, #41747, #103411, #26583, #11417, #73087, #134758, #196440, #48696, #183237, #95178, #171036, #156865, #17356, #108363, #138698, #94179, #77026, #14370, #46701, #44718, #180, #170041, #32527, #187225, #110348, #139682, #172030, #47704, #152875, #123517, #1169, #121542, #79011, #106374, #18361, #61848, #155858, #124528, #80014, #141683, #76036, #62844, #168056, #186223, #109354, #137711, #29553, #140685, #2177, #63857, #125528, #31531, #91186, #33518, #199395, #59876, #60859, #122534, #184225, #30536, #185210, #45706, #107357, #169030, #92188, #153872, #15370, #93184, #154869, #16366, #78014, #175019, #67830, #52660, #96170, #177032, #173034, #84978, #114322, #36483, #129486, #65831, #176024, #188207, #145663, #159837, #127500, #157860, #113326, #174030, #50682, #111343, #130487, #126509, #4152, #53664, #161840, #20322, #37493, #49679, #192183, #23334, #83984, #99155, #34512, #112340, #19350, #191184, #98139, #80999, #142673, #115342, #5146, #22333, #144665, #189205, #6150, #38502, #66828, #35501, #160844, #97151, #7144, #68828, #100158, #128492, #158834, #81971, #143664, #64847, #3174, #190187, #51662, #21331, #82989, #40496, #102168, #69831, #101149, #197185, #180039, #41508, #181028, #25355, #133500, #57676, #42502, #103171, #105158, #131498, #56672, #195192, #9171, #11173, #163856, #12179, #165848, #88990, #28346, #86996, #116332, #27344, #118345, #148683, #164851, #72848, #10171, #24344, #149675, #87987, #43491, #134518, #150681, #71831, #26347, #193185, #196204, #54658, #119344, #178021, #104166, #73843, #85995, #39489, #135514, #117334, #120315, #58649, #182009, #166844, #162835, #146660, #8155, #147684, #70838, #132506, #194195, #55660, #179028, #140448, #155624, #169800, #106139, #17120, #61613, #931, #168794, #107123, #123281, #31293, #183984, #78772, #186990, #45469, #138462, #46457, #108117, #122294, #171795, #92945, #76791, #125294, #136484, #198164, #153634, #1938, #59634, #77781, #48460, #154631, #167822, #16126, #62605, #63618, #110117, #184972, #170798, #89984, #139450, #121308, #90951, #151665, #13159, #30298, #124283, #183000, #74823, #44484, #29321, #152638, #14128, #47463, #75795, #185980, #109120, #137473, #32290, #93945, #199153, #15129, #60620, #91941, #200143, #94943, #21083, #173795, #6898, #83737, #49442, #127256, #188969, #156627, #187973, #145416, #66588, #128252, #67583, #112104, #20088, #144420, #129241, #189950, #191929, #18122, #143418, #81732, #95934, #97895, #50445, #98903, #52414, #175773, #115090, #35261, #2934, #114072, #4905, #96916, #51424, #159586, #158598, #111105, #36242, #174776, #130233, #82740, #37247, #113084, #5906, #79777, #190937, #141449, #160597, #64614, #22087, #68577, #172794, #126276, #53413, #3916, #33283, #34275, #157620, #19110, #80760, #142438, #65596, #163602, #84733, #193949, #27099, #150438, #25103 ),
 ( #73597, #70590, #86747, #133250, #194942, #8922, #58409, #56418, #148430, #11934, #23088, #146411, #40246, #88745, #7902, #164604, #135269, #118098, #192941, #179788, #87741, #196941, #176782, #9925, #117083, #41257, #161594, #177778, #101920, #100904, #71584, #69586, #55412, #102919, #149426, #103920, #38255, #26098, #99909, #10922, #131253, #72595, #134269, #54420, #195956, #116090, #39248, #178778, #57429, #119102, #162588, #24093, #85747, #180783, #147434, #42260, #165600, #132258, #89739, #154390, #184731, #62362, #185730, #168560, #151425, #92702, #181764, #46216, #155386, #43245, #12912, #90717, #183747, #140201, #15885, #120076, #1695, #152400, #104913, #77543, #139215, #74576, #690, #91699, #107869, #169557, #136244, #93704, #197920, #166600, #31054, #153393, #124031, #182756, #47219, #28100, #108878, #76552, #44240, #59388, #30058, #13887, #14891, #121062, #170557, #105897, #167583, #32047, #78527, #137230, #16876, #29078, #75554, #198914, #60383, #122055, #45233, #106887, #138228, #199910, #61374, #123045, #171553, #190702, #65354, #82497, #4659, #33043, #66350, #52175, #127015, #94698, #157380, #142193, #79534, #128012, #2694, #110864, #36006, #113833, #156375, #49206, #141204, #64371, #125048, #97655, #111861, #175529, #186745, #98664, #174539, #160358, #20840, #173551, #3676, #159344, #80519, #17880, #126039, #189714, #144180, #5666, #188722, #187735, #172549, #34034, #48215, #51187, #50206, #37003, #21848, #95692, #18873, #35020, #109869, #96675, #83499, #158363, #19852, #67342, #81492, #143179, #129003, #145176, #112848, #63371, #191688, #116847, #55178, #69342, #71354, #23853, #72353, #25868, #149199, #88505, #147192, #176541, #87511, #193709, #8682, #163366, #133018, #100670, #84495, #9689, #148196, #103690, #194708, #10689, #70353, #132020, #129988, #56177, #53170, #178538, #114847, #40004, #117860, #146173, #38017, #101676, #177546, #180552, #102687, #179551, #164375, #99673, #24862, #86512, #41021, #161357, #85503, #57193, #42026, #134027, #118868, #195720, #165369, #22848, #26863, #6660, #68338, #7658, #131009, #192700, #54183, #162352, #115856, #39015, #59155, #90491, #198683, #60150, #197690, #15648, #121818, #28851, #30820, #135038, #196714, #105667, #45981, #58183, #106657, #169313, #183514, #104681, #44997, #29826, #92468, #154156, #75324, #44005, #168330, #119851, #27865, #152173, #151196, #150201, #11699, #181535, #137989, #43014, #91463, #14652, #153150, #136994, #76312, #12684, #199673, #166368, #122811, #61139, #74350, #89506, #184501, #120824, #107636, #136016, #73366, #13656, #182524, #167353, #77622, #60457, #109950, #13963, #47300, #186825, #30133, #78607, #48294, #174365, #15962, #76626, #183819, #61452, #75630, #140281, #92781, #128827, #5487, #168633, #46293, #107950, #137308, #106959, #67170, #185813, #108957, #35835, #31133, #139292, #63451, #97481, #170636, #113659, #198989, #62439, #769, #14966, #16953, #169637, #20662, #159167, #82316, #36821, #154470, #122132, #144006, #124113, #32125, #93782, #1773, #155463, #91776, #125128, #190526, #52000, #175353, #152476, #45309, #153470, #138304, #199985, #123122, #184807, #6482, #70178, #39827, #37837, #68162, #147016, #69167, #72174, #194529, #9511, #56000, #145001, #55003, #85324, #8501, #129814, #115682, #149023, #133848, #131846, #10511, #164194, #178363, #114668, #25692, #193529, #71177, #177370, #38842, #116673, #101493, #192525, #87337, #195538, #54008, #163182, #24686, #86335, #130834, #180377, #148022, #132841, #57012, #191513, #52990, #117678, #179375, #40837, #176364, #118685, #99497, #98487, #102510, #160180, #21670, #161178, #83324, #22674, #84321, #146000, #7483, #100499, #162178, #23676, #75148, #73191, #106473, #134862, #28676, #103514, #11521, #41847, #91281, #88325, #30639, #61949, #122635, #76133, #26685, #151022, #196540, #168152, #151997, #58010, #150016, #169134, #43827, #60961, #183336 ),
 ( #137811, #198503, #280, #119680, #13483, #90311, #104507, #29649, #58984, #107458, #184325, #45807, #123616, #182349, #181363, #92292, #136819, #105491, #59974, #152972, #135847, #42842, #44818, #14471, #138799, #199495, #153976, #167177, #121641, #165190, #15473, #166188, #77130, #27689, #89330, #12513, #74177, #197516, #120651, #155957, #158932, #81091, #96266, #142769, #31633, #141776, #172128, #33614, #93282, #2272, #35598, #20421, #95277, #97244, #50778, #64942, #1269, #112438, #156960, #157952, #63955, #125624, #18457, #126601, #79110, #174127, #82071, #140783, #80108, #3270, #188303, #17454, #187322, #46802, #4250, #19443, #154967, #65929, #49780, #111445, #34607, #78112, #143764, #16463, #66926, #127602, #173132, #189301, #47803, #5245, #170138, #185311, #108461, #109453, #139781, #62946, #48793, #124626, #186321, #171136, #32625, #94279, #110447, #98235, #128589, #178123, #175112, #117435, #148783, #9272, #162939, #113420, #37591, #159938, #193287, #38602, #21425, #36580, #55761, #130590, #147786, #69938, #83085, #131602, #179133, #192286, #144761, #22432, #7243, #6246, #54761, #67925, #176120, #101250, #40601, #129578, #114419, #191275, #52750, #190283, #24446, #177131, #102272, #51759, #163960, #39591, #25458, #86095, #100258, #68928, #70938, #145761, #99253, #115440, #160940, #53766, #161939, #132606, #87098, #10272, #8258, #84082, #116435, #23434, #85081, #194295, #146765, #29420, #195293, #30400, #89089, #44581, #136581, #92046, #153735, #26446, #13255, #180139, #74918, #59737, #149774, #41608, #106238, #198261, #14228, #137573, #120413, #103273, #167920, #133601, #121406, #107223, #56774, #164953, #42602, #135610, #71931, #91051, #118447, #88088, #45570, #11276, #72949, #183100, #43589, #152738, #134619, #75899, #196303, #199256, #28444, #57773, #119443, #182104, #104266, #105255, #181128, #60723, #165948, #58744, #27448, #150781, #12276, #122397, #73941, #184087, #197281, #168894, #166941, #90080, #151762, #46563, #79881, #125395, #108224, #123382, #142540, #17221, #34378, #156732, #185074, #18225, #4019, #78873, #169904, #109219, #94045, #31397, #141550, #154734, #62707, #188074, #65697, #93047, #1034, #16230, #77882, #76890, #49545, #63720, #127363, #138561, #50548, #126377, #112208, #172900, #187092, #155723, #111208, #32390, #139550, #2040, #39, #140552, #48562, #96038, #189075, #173898, #95043, #35367, #3039, #124389, #110215, #64715, #61714, #157725, #186084, #97019, #171896, #19214, #80864, #15231, #47567, #170898, #33384, #66693, #161703, #146521, #36347, #128357, #193050, #23199, #101017, #24207, #7003, #190053, #131361, #20189, #84842, #194063, #81835, #51529, #129349, #22193, #178890, #54527, #158700, #40358, #191044, #143523, #116200, #177889, #113192, #39359, #130340, #8011, #69694, #174881, #162702, #5011, #53520, #85856, #98000, #147545, #9033, #70702, #83842, #82847, #159694, #67691, #21191, #132370, #99011, #55524, #117198, #144526, #52517, #114178, #6012, #175882, #37353, #192039, #115198, #160702, #145524, #68685, #176890, #38361, #100016, #60490, #86860, #12044, #150545, #164714, #166708, #119207, #167694, #121174, #44349, #183855, #42367, #71695, #182868, #88852, #104030, #58518, #28212, #196065, #179900, #105024, #43353, #199021, #89852, #106008, #165709, #27206, #25218, #151535, #148544, #73708, #10035, #135380, #13024, #41366, #133362, #197050, #72707, #75664, #198031, #74689, #59499, #195053, #120184, #181874, #136355, #56531, #180892, #152508, #137341, #29191, #13997, #90825, #122165, #118209, #102033, #163716, #103032, #26209, #87848, #149536, #11031, #57538, #134379, #142308, #139326, #93817, #1809, #63487, #77657, #127128, #125163, #32160, #80631, #91811, #153503, #108991, #95806, #15000, #33155, #3788, #186862, #61487, #48331, #156492, #18985, #65465, #78644, #185849, #109986, #30167, #46329, #92817, #45342, #141316, #170672, #76660, #138339 ),
 ( #184845, #154503, #17994, #157492, #200019, #31167, #123157, #107984, #47336, #169671, #171666, #62478, #110975, #64483, #187846, #106994, #155497, #15999, #126150, #16990, #140319, #94814, #79647, #805, #124150, #2805, #49315, #168667, #172660, #34147, #190811, #52286, #111974, #53282, #173666, #113943, #96785, #160469, #130105, #128124, #158474, #37116, #159456, #162460, #84607, #99784, #146286, #35133, #145289, #175642, #98775, #19962, #5780, #39122, #23961, #21960, #100777, #54293, #68451, #4774, #115965, #83611, #161470, #67454, #129112, #6772, #191801, #82609, #177653, #85616, #144290, #114961, #176654, #38131, #20952, #70462, #22959, #7773, #147303, #81604, #143288, #69456, #8792, #66462, #131123, #188834, #192811, #189826, #50319, #51298, #112959, #174652, #36117, #97769, #196818, #116957, #133124, #179660, #152280, #27974, #57299, #40111, #89613, #193820, #26972, #166475, #9797, #58285, #151302, #12791, #195828, #56287, #163477, #74456, #55285, #88615, #136122, #71459, #119954, #197798, #59264, #118976, #117969, #24974, #41130, #178648, #181640, #72466, #105775, #182632, #148303, #25974, #87617, #101789, #86620, #44116, #165476, #150312, #120933, #10797, #180659, #43119, #167462, #11808, #194814, #102794, #132127, #134139, #164480, #104787, #149303, #28957, #90598, #13764, #42135, #103796, #73472, #135145, #62234, #77416, #31919, #1563, #169425, #153262, #78396, #16748, #172415, #63238, #79405, #139088, #563, #198792, #140072, #60258, #123902, #183624, #47090, #124918, #14763, #45106, #185601, #46089, #49077, #171427, #186615, #32914, #121929, #93573, #108751, #170427, #106763, #92578, #125910, #110734, #155258, #187608, #141076, #48087, #91573, #2561, #109743, #94569, #154266, #15757, #156247, #17749, #30930, #64243, #33903, #95560, #157247, #75432, #137106, #107744, #168438, #29934, #76424, #138100, #199781, #61249, #122920, #184608, #65224, #6528, #54054, #160226, #34889, #21717, #129860, #192570, #115728, #52047, #159213, #83370, #3546, #19723, #66219, #38886, #114717, #144052, #126884, #96545, #188590, #53037, #145047, #161225, #84367, #67213, #50071, #191558, #80388, #68208, #177415, #142060, #111732, #189583, #82364, #100543, #176409, #18741, #173419, #51055, #158232, #37885, #99543, #81364, #22719, #190571, #146044, #7528, #143048, #4527, #127879, #112717, #69213, #113703, #130881, #174410, #35879, #97526, #20708, #175400, #5534, #128871, #36868, #98533, #195584, #193575, #29449, #55047, #149066, #23721, #131891, #162222, #14260, #8546, #153767, #185104, #45601, #199287, #147063, #71221, #116718, #91081, #72218, #178407, #70223, #92078, #164240, #184119, #103558, #39871, #165233, #15262, #25735, #101538, #56043, #40882, #163230, #152768, #24730, #9555, #137604, #76920, #86380, #148064, #138591, #41892, #73, #10554, #133893, #61743, #85370, #123411, #75929, #46594, #122427, #57056, #102555, #60754, #179417, #132884, #118731, #194573, #87381, #180419, #107254, #117722, #168925, #30431, #158728, #96065, #1063, #171924, #49574, #169934, #65725, #31425, #66726, #125423, #80892, #172928, #128386, #190082, #62738, #111237, #16260, #34407, #157754, #77911, #2070, #187119, #124418, #19245, #47594, #155752, #142569, #20218, #186114, #94073, #81866, #188101, #143557, #156760, #18254, #97046, #93078, #5040, #4048, #108254, #127394, #79907, #48591, #189103, #110242, #109247, #95072, #154762, #33413, #141578, #50576, #35395, #139578, #112236, #170927, #173926, #32418, #3066, #17250, #78903, #140580, #63749, #64743, #126405, #24241, #116229, #71725, #133394, #6043, #193081, #159727, #54556, #39388, #129379, #21223, #85890, #177920, #194094, #117229, #100048, #82879, #147578, #113222, #101048, #86891, #174912, #144557, #22224, #115230, #51558, #9064, #36376, #98030, #83873, #67721, #70734, #132401, #191075, #55556, #23229, #162733, #178923, #52548, #25249, #114209, #175914, #40393 ),
 ( #37385, #99042, #160732, #145555, #102064, #176921, #7033, #163749, #68715, #146550, #148575, #130372, #10065, #192070, #53551, #38392, #161734, #84872, #8046, #69725, #131393, #135411, #168697, #45372, #11064, #88885, #150577, #118241, #56567, #89883, #29221, #72742, #121206, #90854, #152539, #58549, #119239, #26241, #104061, #179932, #182897, #197082, #30199, #107025, #134413, #12076, #73739, #41399, #149568, #91840, #28243, #151566, #14027, #120215, #181905, #106037, #75692, #13055, #87880, #164746, #195085, #43384, #57569, #59528, #105056, #60521, #137372, #199050, #76691, #166740, #196099, #122195, #74722, #136385, #198062, #44382, #167723, #180923, #183887, #153534, #15031, #103064, #42398, #165741, #27236, #61517, #2834, #123186, #1837, #46357, #110014, #79676, #77686, #108015, #186890, #109021, #112006, #34175, #49342, #95836, #184875, #94843, #125194, #48360, #169701, #155525, #188864, #173695, #171695, #50347, #3816, #18023, #154531, #65494, #33184, #111004, #17020, #78673, #156524, #141347, #32189, #127156, #35163, #93847, #64512, #126179, #187874, #170700, #19990, #172690, #157520, #96818, #31195, #92846, #63519, #158503, #16028, #19014, #138367, #80660, #139354, #142336, #200048, #835, #62508, #124179, #140349, #185881, #47366, #82638, #129143, #101819, #177683, #6802, #189855, #39151, #146315, #163507, #81633, #36147, #22990, #51329, #84638, #69488, #159488, #112989, #115994, #7804, #23991, #147335, #130135, #174682, #54322, #143316, #131153, #116986, #4803, #97799, #52316, #145319, #66492, #100807, #128155, #20981, #113974, #144321, #162490, #85648, #5810, #8822, #53313, #192842, #70491, #67485, #55315, #190840, #175672, #132158, #114991, #193850, #37146, #178679, #98805, #40142, #38160, #160499, #21989, #191832, #83642, #176685, #68480, #99815, #161500, #11837, #86649, #194845, #25005, #74486, #71488, #13795, #45136, #105804, #59293, #9828, #134169, #56318, #89643, #135174, #118000, #133154, #152309, #27000, #44145, #166505, #179689, #28003, #75460, #88645, #41161, #119005, #103824, #102824, #151331, #164510, #72495, #197827, #137134, #26003, #10825, #198821, #104816, #60286, #73502, #196848, #121959, #148333, #183652, #136152, #106793, #182661, #58314, #165504, #120962, #42164, #87645, #119982, #149331, #150341, #181668, #167491, #195857, #57329, #12820, #180688, #28987, #43147, #90627, #109773, #29965, #125939, #91603, #126915, #185629, #141105, #153292, #32944, #14793, #31948, #76453, #140102, #171456, #107771, #138130, #16778, #139116, #142092, #64272, #79434, #187637, #199811, #124949, #155288, #78427, #61279, #47121, #18772, #3577, #1593, #80419, #33934, #48116, #184637, #95592, #63268, #2593, #108779, #170457, #186645, #94599, #62263, #157276, #65255, #123931, #156278, #17779, #49107, #592, #50102, #110765, #172446, #188621, #122949, #46118, #93603, #168467, #169457, #30958, #92605, #154295, #15785, #77445, #22749, #85404, #147096, #145077, #52078, #176441, #96575, #112747, #159244, #131923, #7559, #36900, #19753, #69245, #173451, #6559, #146074, #189613, #37914, #130911, #192601, #175431, #35910, #143080, #20739, #34919, #99573, #113734, #8581, #162255, #127911, #5564, #67243, #158264, #66251, #23754, #68237, #129890, #54084, #190602, #98564, #84398, #115758, #191590, #4559, #81394, #111762, #160258, #174441, #161255, #128902, #177446, #38916, #100573, #193607, #21748, #51087, #70255, #83399, #53069, #114747, #97556, #82395, #144083, #58082, #196612, #152070, #42913, #59056, #57090, #118764, #148097, #28749, #24765, #136893, #166263, #26760, #119752, #117758, #27762, #39907, #197590, #11597, #179450, #9589, #165266, #25768, #88400, #86412, #181435, #71254, #41925, #116749, #132918, #55079, #104579, #101573, #43901, #75221, #135919, #89405, #163263, #164273, #194605, #151094, #150094, #56077, #40916, #182423, #180453, #74250, #12585, #102589, #120723, #105564, #103591 ) ),
 .UNSPECIFIED., .T., .F., .F. ) 
 B_SPLINE_SURFACE_WITH_KNOTS ( ( 4, 3, 4 ),
 ( 3, 2, 2, 2, 2, 2, 2, 2, 2, 2, 2, 2, 2, 2, 2, 2, 2, 2, 2, 2, 2, 2, 2, 2, 2, 2, 2, 2, 2, 2, 2, 2, 2, 2, 2, 2, 2, 2, 2, 2, 2, 2, 2, 2, 2, 2, 2, 2, 2, 2, 2, 2, 2, 2, 2, 2, 2, 2, 2, 2, 2, 2, 2, 2, 2, 2, 2, 2, 2, 2, 2, 2, 2, 2, 2, 2, 2, 2, 2, 2, 2, 2, 2, 2, 2, 2, 2, 2, 2, 2, 2, 2, 2, 2, 2, 2, 2, 2, 2, 2, 2, 2, 2, 2, 2, 2, 2, 2, 2, 2, 2, 2, 2, 2, 2, 2, 2, 2, 2, 2, 2, 2, 2, 2, 2, 2, 2, 2, 2, 2, 2, 2, 2, 2, 2, 2, 2, 2, 2, 2, 2, 2, 2, 2, 2, 2, 2, 2, 2, 2, 2, 2, 2, 2, 2, 2, 2, 2, 2, 2, 2, 2, 2, 2, 2, 2, 2, 2, 2, 2, 2, 2, 2, 2, 2, 2, 2, 2, 2, 2, 2, 2, 2, 2, 2, 2, 2, 2, 2, 2, 2, 2, 2, 2, 2, 2, 2, 2, 2, 2, 2, 2, 2, 2, 2, 2, 2, 2, 2, 2, 2, 2, 2, 2, 2, 2, 2, 2, 2, 2, 2, 2, 2, 2, 2, 2, 2, 2, 3 ),
 ( 0.000000000000000000, 0.5000000000000000000, 1.000000000000000000 ),
 ( 0.000000000000000000, 0.004385964912280701511, 0.008771929824561403022, 0.01315789473684210453, 0.01754385964912280604, 0.02192982456140350755, 0.02631578947368420907, 0.03070175438596491058, 0.03508771929824561209, 0.03947368421052631360, 0.04385964912280701511, 0.04824561403508771662, 0.05263157894736841813, 0.05701754385964911964, 0.06140350877192982115, 0.06578947368421052266, 0.07017543859649122417, 0.07456140350877192569, 0.07894736842105262720, 0.08333333333333332871, 0.08771929824561403022, 0.09210526315789473173, 0.09649122807017543324, 0.1008771929824561348, 0.1052631578947368363, 0.1096491228070175378, 0.1140350877192982393, 0.1184210526315789408, 0.1228070175438596423, 0.1271929824561403577, 0.1315789473684210453, 0.1359649122807017607, 0.1403508771929824483, 0.1447368421052631637, 0.1491228070175438514, 0.1535087719298245668, 0.1578947368421052544, 0.1622807017543859698, 0.1666666666666666574, 0.1710526315789473728, 0.1754385964912280604, 0.1798245614035087758, 0.1842105263157894635, 0.1885964912280701788, 0.1929824561403508665, 0.1973684210526315819, 0.2017543859649122695, 0.2061403508771929849, 0.2105263157894736725, 0.2149122807017543879, 0.2192982456140350755, 0.2236842105263157909, 0.2280701754385964786, 0.2324561403508771940, 0.2368421052631578816, 0.2412280701754385970, 0.2456140350877192846, 0.2500000000000000000, 0.2543859649122807154, 0.2587719298245614308, 0.2631578947368420907, 0.2675438596491228060, 0.2719298245614035214, 0.2763157894736842368, 0.2807017543859648967, 0.2850877192982456121, 0.2894736842105263275, 0.2938596491228070429, 0.2982456140350877027, 0.3026315789473684181, 0.3070175438596491335, 0.3114035087719298489, 0.3157894736842105088, 0.3201754385964912242, 0.3245614035087719396, 0.3289473684210526550, 0.3333333333333333148, 0.3377192982456140302, 0.3421052631578947456, 0.3464912280701754610, 0.3508771929824561209, 0.3552631578947368363, 0.3596491228070175517, 0.3640350877192982670, 0.3684210526315789269, 0.3728070175438596423, 0.3771929824561403577, 0.3815789473684210731, 0.3859649122807017330, 0.3903508771929824483, 0.3947368421052631637, 0.3991228070175438791, 0.4035087719298245390, 0.4078947368421052544, 0.4122807017543859698, 0.4166666666666666852, 0.4210526315789473450, 0.4254385964912280604, 0.4298245614035087758, 0.4342105263157894912, 0.4385964912280701511, 0.4429824561403508665, 0.4473684210526315819, 0.4517543859649122973, 0.4561403508771929571, 0.4605263157894736725, 0.4649122807017543879, 0.4692982456140351033, 0.4736842105263157632, 0.4780701754385964786, 0.4824561403508771940, 0.4868421052631579093, 0.4912280701754385692, 0.4956140350877192846, 0.5000000000000000000, 0.5043859649122807154, 0.5087719298245614308, 0.5131578947368421462, 0.5175438596491228616, 0.5219298245614034659, 0.5263157894736841813, 0.5307017543859648967, 0.5350877192982456121, 0.5394736842105263275, 0.5438596491228070429, 0.5482456140350877583, 0.5526315789473684736, 0.5570175438596490780, 0.5614035087719297934, 0.5657894736842105088, 0.5701754385964912242, 0.5745614035087719396, 0.5789473684210526550, 0.5833333333333333703, 0.5877192982456140857, 0.5921052631578946901, 0.5964912280701754055, 0.6008771929824561209, 0.6052631578947368363, 0.6096491228070175517, 0.6140350877192982670, 0.6184210526315789824, 0.6228070175438596978, 0.6271929824561403022, 0.6315789473684210176, 0.6359649122807017330, 0.6403508771929824483, 0.6447368421052631637, 0.6491228070175438791, 0.6535087719298245945, 0.6578947368421053099, 0.6622807017543859143, 0.6666666666666666297, 0.6710526315789473450, 0.6754385964912280604, 0.6798245614035087758, 0.6842105263157894912, 0.6885964912280702066, 0.6929824561403509220, 0.6973684210526315264, 0.7017543859649122417, 0.7061403508771929571, 0.7105263157894736725, 0.7149122807017543879, 0.7192982456140351033, 0.7236842105263158187, 0.7280701754385965341, 0.7324561403508771384, 0.7368421052631578538, 0.7412280701754385692, 0.7456140350877192846, 0.7500000000000000000, 0.7543859649122807154, 0.7587719298245614308, 0.7631578947368421462, 0.7675438596491228616, 0.7719298245614034659, 0.7763157894736841813, 0.7807017543859648967, 0.7850877192982456121, 0.7894736842105263275, 0.7938596491228070429, 0.7982456140350877583, 0.8026315789473684736, 0.8070175438596490780, 0.8114035087719297934, 0.8157894736842105088, 0.8201754385964912242, 0.8245614035087719396, 0.8289473684210526550, 0.8333333333333333703, 0.8377192982456140857, 0.8421052631578946901, 0.8464912280701754055, 0.8508771929824561209, 0.8552631578947368363, 0.8596491228070175517, 0.8640350877192982670, 0.8684210526315789824, 0.8728070175438596978, 0.8771929824561403022, 0.8815789473684210176, 0.8859649122807017330, 0.8903508771929824483, 0.8947368421052631637, 0.8991228070175438791, 0.9035087719298245945, 0.9078947368421053099, 0.9122807017543859143, 0.9166666666666666297, 0.9210526315789473450, 0.9254385964912280604, 0.9298245614035087758, 0.9342105263157894912, 0.9385964912280702066, 0.9429824561403509220, 0.9473684210526315264, 0.9517543859649122417, 0.9561403508771929571, 0.9605263157894736725, 0.9649122807017543879, 0.9692982456140351033, 0.9736842105263158187, 0.9780701754385965341, 0.9824561403508771384, 0.9868421052631578538, 0.9912280701754385692, 0.9956140350877192846, 1.000000000000000000 ),
 .UNSPECIFIED. ) 
 GEOMETRIC_REPRESENTATION_ITEM ( )  RATIONAL_B_SPLINE_SURFACE ( (
 ( 1.000000000000000000, 0.9659258262890683122, 1.000000000000000000, 0.9659258262890683122, 1.000000000000000000, 0.9659258262890683122, 1.000000000000000000, 0.9659258262890683122, 1.000000000000000000, 0.9659258262890683122, 1.000000000000000000, 0.9659258262890683122, 1.000000000000000000, 0.9659258262890683122, 1.000000000000000000, 0.9659258262890683122, 1.000000000000000000, 0.9659258262890683122, 1.000000000000000000, 0.9659258262890683122, 1.000000000000000000, 0.9659258262890683122, 1.000000000000000000, 0.9659258262890683122, 1.000000000000000000, 0.9659258262890683122, 1.000000000000000000, 0.9659258262890683122, 1.000000000000000000, 0.9659258262890683122, 1.000000000000000000, 0.9659258262890683122, 1.000000000000000000, 0.9659258262890683122, 1.000000000000000000, 0.9659258262890683122, 1.000000000000000000, 0.9659258262890683122, 1.000000000000000000, 0.9659258262890683122, 1.000000000000000000, 0.9659258262890683122, 1.000000000000000000, 0.9659258262890683122, 1.000000000000000000, 0.9659258262890683122, 1.000000000000000000, 0.9659258262890683122, 1.000000000000000000, 0.9659258262890683122, 1.000000000000000000, 0.9659258262890683122, 1.000000000000000000, 0.9659258262890683122, 1.000000000000000000, 0.9659258262890683122, 1.000000000000000000, 0.9659258262890683122, 1.000000000000000000, 0.9659258262890683122, 1.000000000000000000, 0.9659258262890683122, 1.000000000000000000, 0.9659258262890683122, 1.000000000000000000, 0.9659258262890683122, 1.000000000000000000, 0.9659258262890683122, 1.000000000000000000, 0.9659258262890683122, 1.000000000000000000, 0.9659258262890683122, 1.000000000000000000, 0.9659258262890683122, 1.000000000000000000, 0.9659258262890683122, 1.000000000000000000, 0.9659258262890683122, 1.000000000000000000, 0.9659258262890683122, 1.000000000000000000, 0.9659258262890683122, 1.000000000000000000, 0.9659258262890683122, 1.000000000000000000, 0.9659258262890683122, 1.000000000000000000, 0.9659258262890683122, 1.000000000000000000, 0.9659258262890683122, 1.000000000000000000, 0.9659258262890683122, 1.000000000000000000, 0.9659258262890683122, 1.000000000000000000, 0.9659258262890683122, 1.000000000000000000, 0.9659258262890683122, 1.000000000000000000, 0.9659258262890683122, 1.000000000000000000, 0.9659258262890683122, 1.000000000000000000, 0.9659258262890683122, 1.000000000000000000, 0.9659258262890683122, 1.000000000000000000, 0.9659258262890683122, 1.000000000000000000, 0.9659258262890683122, 1.000000000000000000, 0.9659258262890683122, 1.000000000000000000, 0.9659258262890683122, 1.000000000000000000, 0.9659258262890683122, 1.000000000000000000, 0.9659258262890683122, 1.000000000000000000, 0.9659258262890683122, 1.000000000000000000, 0.9659258262890683122, 1.000000000000000000, 0.9659258262890683122, 1.000000000000000000, 0.9659258262890683122, 1.000000000000000000, 0.9659258262890683122, 1.000000000000000000, 0.9659258262890683122, 1.000000000000000000, 0.9659258262890683122, 1.000000000000000000, 0.9659258262890683122, 1.000000000000000000, 0.9659258262890683122, 1.000000000000000000, 0.9659258262890683122, 1.000000000000000000, 0.9659258262890683122, 1.000000000000000000, 0.9659258262890683122, 1.000000000000000000, 0.9659258262890683122, 1.000000000000000000, 0.9659258262890683122, 1.000000000000000000, 0.9659258262890683122, 1.000000000000000000, 0.9659258262890683122, 1.000000000000000000, 0.9659258262890683122, 1.000000000000000000, 0.9659258262890683122, 1.000000000000000000, 0.9659258262890683122, 1.000000000000000000, 0.9659258262890683122, 1.000000000000000000, 0.9659258262890683122, 1.000000000000000000, 0.9659258262890683122, 1.000000000000000000, 0.9659258262890683122, 1.000000000000000000, 0.9659258262890683122, 1.000000000000000000, 0.9659258262890683122, 1.000000000000000000, 0.9659258262890683122, 1.000000000000000000, 0.9659258262890683122, 1.000000000000000000, 0.9659258262890683122, 1.000000000000000000, 0.9659258262890683122, 1.000000000000000000, 0.9659258262890683122, 1.000000000000000000, 0.9659258262890683122, 1.000000000000000000, 0.9659258262890683122, 1.000000000000000000, 0.9659258262890683122, 1.000000000000000000, 0.9659258262890683122, 1.000000000000000000, 0.9659258262890683122, 1.000000000000000000, 0.9659258262890683122, 1.000000000000000000, 0.9659258262890683122, 1.000000000000000000, 0.9659258262890683122, 1.000000000000000000, 0.9659258262890683122, 1.000000000000000000, 0.9659258262890683122, 1.000000000000000000, 0.9659258262890683122, 1.000000000000000000, 0.9659258262890683122, 1.000000000000000000, 0.9659258262890683122, 1.000000000000000000, 0.9659258262890683122, 1.000000000000000000, 0.9659258262890683122, 1.000000000000000000, 0.9659258262890683122, 1.000000000000000000, 0.9659258262890683122, 1.000000000000000000, 0.9659258262890683122, 1.000000000000000000, 0.9659258262890683122, 1.000000000000000000, 0.9659258262890683122, 1.000000000000000000, 0.9659258262890683122, 1.000000000000000000, 0.9659258262890683122, 1.000000000000000000, 0.9659258262890683122, 1.000000000000000000, 0.9659258262890683122, 1.000000000000000000, 0.9659258262890683122, 1.000000000000000000, 0.9659258262890683122, 1.000000000000000000, 0.9659258262890683122, 1.000000000000000000, 0.9659258262890683122, 1.000000000000000000, 0.9659258262890683122, 1.000000000000000000, 0.9659258262890683122, 1.000000000000000000, 0.9659258262890683122, 1.000000000000000000, 0.9659258262890683122, 1.000000000000000000, 0.9659258262890683122, 1.000000000000000000, 0.9659258262890683122, 1.000000000000000000, 0.9659258262890683122, 1.000000000000000000, 0.9659258262890683122, 1.000000000000000000, 0.9659258262890683122, 1.000000000000000000, 0.9659258262890683122, 1.000000000000000000, 0.9659258262890683122, 1.000000000000000000, 0.9659258262890683122, 1.000000000000000000, 0.9659258262890683122, 1.000000000000000000, 0.9659258262890683122, 1.000000000000000000, 0.9659258262890683122, 1.000000000000000000, 0.9659258262890683122, 1.000000000000000000, 0.9659258262890683122, 1.000000000000000000, 0.9659258262890683122, 1.000000000000000000, 0.9659258262890683122, 1.000000000000000000, 0.9659258262890683122, 1.000000000000000000, 0.9659258262890683122, 1.000000000000000000, 0.9659258262890683122, 1.000000000000000000, 0.9659258262890683122, 1.000000000000000000, 0.9659258262890683122, 1.000000000000000000, 0.9659258262890683122, 1.000000000000000000, 0.9659258262890683122, 1.000000000000000000, 0.9659258262890683122, 1.000000000000000000, 0.9659258262890683122, 1.000000000000000000, 0.9659258262890683122, 1.000000000000000000, 0.9659258262890683122, 1.000000000000000000, 0.9659258262890683122, 1.000000000000000000, 0.9659258262890683122, 1.000000000000000000, 0.9659258262890683122, 1.000000000000000000, 0.9659258262890683122, 1.000000000000000000, 0.9659258262890683122, 1.000000000000000000, 0.9659258262890683122, 1.000000000000000000, 0.9659258262890683122, 1.000000000000000000, 0.9659258262890683122, 1.000000000000000000, 0.9659258262890683122, 1.000000000000000000, 0.9659258262890683122, 1.000000000000000000, 0.9659258262890683122, 1.000000000000000000, 0.9659258262890683122, 1.000000000000000000, 0.9659258262890683122, 1.000000000000000000, 0.9659258262890683122, 1.000000000000000000, 0.9659258262890683122, 1.000000000000000000, 0.9659258262890683122, 1.000000000000000000, 0.9659258262890683122, 1.000000000000000000, 0.9659258262890683122, 1.000000000000000000, 0.9659258262890683122, 1.000000000000000000, 0.9659258262890683122, 1.000000000000000000, 0.9659258262890683122, 1.000000000000000000, 0.9659258262890683122, 1.000000000000000000, 0.9659258262890683122, 1.000000000000000000, 0.9659258262890683122, 1.000000000000000000, 0.9659258262890683122, 1.000000000000000000, 0.9659258262890683122, 1.000000000000000000, 0.9659258262890683122, 1.000000000000000000, 0.9659258262890683122, 1.000000000000000000, 0.9659258262890683122, 1.000000000000000000, 0.9659258262890683122, 1.000000000000000000, 0.9659258262890683122, 1.000000000000000000, 0.9659258262890683122, 1.000000000000000000, 0.9659258262890683122, 1.000000000000000000, 0.9659258262890683122, 1.000000000000000000, 0.9659258262890683122, 1.000000000000000000, 0.9659258262890683122, 1.000000000000000000, 0.9659258262890683122, 1.000000000000000000, 0.9659258262890683122, 1.000000000000000000, 0.9659258262890683122, 1.000000000000000000, 0.9659258262890683122, 1.000000000000000000, 0.9659258262890683122, 1.000000000000000000, 0.9659258262890683122, 1.000000000000000000, 0.9659258262890683122, 1.000000000000000000, 0.9659258262890683122, 1.000000000000000000, 0.9659258262890683122, 1.000000000000000000, 0.9659258262890683122, 1.000000000000000000, 0.9659258262890683122, 1.000000000000000000, 0.9659258262890683122, 1.000000000000000000, 0.9659258262890683122, 1.000000000000000000, 0.9659258262890683122, 1.000000000000000000, 0.9659258262890683122, 1.000000000000000000, 0.9659258262890683122, 1.000000000000000000, 0.9659258262890683122, 1.000000000000000000, 0.9659258262890683122, 1.000000000000000000, 0.9659258262890683122, 1.000000000000000000, 0.9659258262890683122, 1.000000000000000000, 0.9659258262890683122, 1.000000000000000000, 0.9659258262890683122, 1.000000000000000000, 0.9659258262890683122, 1.000000000000000000, 0.9659258262890683122, 1.000000000000000000, 0.9659258262890683122, 1.000000000000000000, 0.9659258262890683122, 1.000000000000000000, 0.9659258262890683122, 1.000000000000000000, 0.9659258262890683122, 1.000000000000000000, 0.9659258262890683122, 1.000000000000000000, 0.9659258262890683122, 1.000000000000000000, 0.9659258262890683122, 1.000000000000000000, 0.9659258262890683122, 1.000000000000000000, 0.9659258262890683122, 1.000000000000000000, 0.9659258262890683122, 1.000000000000000000, 0.9659258262890683122, 1.000000000000000000, 0.9659258262890683122, 1.000000000000000000, 0.9659258262890683122, 1.000000000000000000, 0.9659258262890683122, 1.000000000000000000, 0.9659258262890683122, 1.000000000000000000, 0.9659258262890683122, 1.000000000000000000, 0.9659258262890683122, 1.000000000000000000, 0.9659258262890683122, 1.000000000000000000, 0.9659258262890683122, 1.000000000000000000, 0.9659258262890683122, 1.000000000000000000, 0.9659258262890683122, 1.000000000000000000),
 ( 0.3333333333333333703, 0.3219752754296894559, 0.3333333333333333703, 0.3219752754296894559, 0.3333333333333333703, 0.3219752754296894559, 0.3333333333333333703, 0.3219752754296894559, 0.3333333333333333703, 0.3219752754296894559, 0.3333333333333333703, 0.3219752754296894559, 0.3333333333333333703, 0.3219752754296894559, 0.3333333333333333703, 0.3219752754296894559, 0.3333333333333333703, 0.3219752754296894559, 0.3333333333333333703, 0.3219752754296894559, 0.3333333333333333703, 0.3219752754296894559, 0.3333333333333333703, 0.3219752754296894559, 0.3333333333333333703, 0.3219752754296894559, 0.3333333333333333703, 0.3219752754296894559, 0.3333333333333333703, 0.3219752754296894559, 0.3333333333333333703, 0.3219752754296894559, 0.3333333333333333703, 0.3219752754296894559, 0.3333333333333333703, 0.3219752754296894559, 0.3333333333333333703, 0.3219752754296894559, 0.3333333333333333703, 0.3219752754296894559, 0.3333333333333333703, 0.3219752754296894559, 0.3333333333333333703, 0.3219752754296894559, 0.3333333333333333703, 0.3219752754296894559, 0.3333333333333333703, 0.3219752754296894559, 0.3333333333333333703, 0.3219752754296894559, 0.3333333333333333703, 0.3219752754296894559, 0.3333333333333333703, 0.3219752754296894559, 0.3333333333333333703, 0.3219752754296894559, 0.3333333333333333703, 0.3219752754296894559, 0.3333333333333333703, 0.3219752754296894559, 0.3333333333333333703, 0.3219752754296894559, 0.3333333333333333703, 0.3219752754296894559, 0.3333333333333333703, 0.3219752754296894559, 0.3333333333333333703, 0.3219752754296894559, 0.3333333333333333703, 0.3219752754296894559, 0.3333333333333333703, 0.3219752754296894559, 0.3333333333333333703, 0.3219752754296894559, 0.3333333333333333703, 0.3219752754296894559, 0.3333333333333333703, 0.3219752754296894559, 0.3333333333333333703, 0.3219752754296894559, 0.3333333333333333703, 0.3219752754296894559, 0.3333333333333333703, 0.3219752754296894559, 0.3333333333333333703, 0.3219752754296894559, 0.3333333333333333703, 0.3219752754296894559, 0.3333333333333333703, 0.3219752754296894559, 0.3333333333333333703, 0.3219752754296894559, 0.3333333333333333703, 0.3219752754296894559, 0.3333333333333333703, 0.3219752754296894559, 0.3333333333333333703, 0.3219752754296894559, 0.3333333333333333703, 0.3219752754296894559, 0.3333333333333333703, 0.3219752754296894559, 0.3333333333333333703, 0.3219752754296894559, 0.3333333333333333703, 0.3219752754296894559, 0.3333333333333333703, 0.3219752754296894559, 0.3333333333333333703, 0.3219752754296894559, 0.3333333333333333703, 0.3219752754296894559, 0.3333333333333333703, 0.3219752754296894559, 0.3333333333333333703, 0.3219752754296894559, 0.3333333333333333703, 0.3219752754296894559, 0.3333333333333333703, 0.3219752754296894559, 0.3333333333333333703, 0.3219752754296894559, 0.3333333333333333703, 0.3219752754296894559, 0.3333333333333333703, 0.3219752754296894559, 0.3333333333333333703, 0.3219752754296894559, 0.3333333333333333703, 0.3219752754296894559, 0.3333333333333333703, 0.3219752754296894559, 0.3333333333333333703, 0.3219752754296894559, 0.3333333333333333703, 0.3219752754296894559, 0.3333333333333333703, 0.3219752754296894559, 0.3333333333333333703, 0.3219752754296894559, 0.3333333333333333703, 0.3219752754296894559, 0.3333333333333333703, 0.3219752754296894559, 0.3333333333333333703, 0.3219752754296894559, 0.3333333333333333703, 0.3219752754296894559, 0.3333333333333333703, 0.3219752754296894559, 0.3333333333333333703, 0.3219752754296894559, 0.3333333333333333703, 0.3219752754296894559, 0.3333333333333333703, 0.3219752754296894559, 0.3333333333333333703, 0.3219752754296894559, 0.3333333333333333703, 0.3219752754296894559, 0.3333333333333333703, 0.3219752754296894559, 0.3333333333333333703, 0.3219752754296894559, 0.3333333333333333703, 0.3219752754296894559, 0.3333333333333333703, 0.3219752754296894559, 0.3333333333333333703, 0.3219752754296894559, 0.3333333333333333703, 0.3219752754296894559, 0.3333333333333333703, 0.3219752754296894559, 0.3333333333333333703, 0.3219752754296894559, 0.3333333333333333703, 0.3219752754296894559, 0.3333333333333333703, 0.3219752754296894559, 0.3333333333333333703, 0.3219752754296894559, 0.3333333333333333703, 0.3219752754296894559, 0.3333333333333333703, 0.3219752754296894559, 0.3333333333333333703, 0.3219752754296894559, 0.3333333333333333703, 0.3219752754296894559, 0.3333333333333333703, 0.3219752754296894559, 0.3333333333333333703, 0.3219752754296894559, 0.3333333333333333703, 0.3219752754296894559, 0.3333333333333333703, 0.3219752754296894559, 0.3333333333333333703, 0.3219752754296894559, 0.3333333333333333703, 0.3219752754296894559, 0.3333333333333333703, 0.3219752754296894559, 0.3333333333333333703, 0.3219752754296894559, 0.3333333333333333703, 0.3219752754296894559, 0.3333333333333333703, 0.3219752754296894559, 0.3333333333333333703, 0.3219752754296894559, 0.3333333333333333703, 0.3219752754296894559, 0.3333333333333333703, 0.3219752754296894559, 0.3333333333333333703, 0.3219752754296894559, 0.3333333333333333703, 0.3219752754296894559, 0.3333333333333333703, 0.3219752754296894559, 0.3333333333333333703, 0.3219752754296894559, 0.3333333333333333703, 0.3219752754296894559, 0.3333333333333333703, 0.3219752754296894559, 0.3333333333333333703, 0.3219752754296894559, 0.3333333333333333703, 0.3219752754296894559, 0.3333333333333333703, 0.3219752754296894559, 0.3333333333333333703, 0.3219752754296894559, 0.3333333333333333703, 0.3219752754296894559, 0.3333333333333333703, 0.3219752754296894559, 0.3333333333333333703, 0.3219752754296894559, 0.3333333333333333703, 0.3219752754296894559, 0.3333333333333333703, 0.3219752754296894559, 0.3333333333333333703, 0.3219752754296894559, 0.3333333333333333703, 0.3219752754296894559, 0.3333333333333333703, 0.3219752754296894559, 0.3333333333333333703, 0.3219752754296894559, 0.3333333333333333703, 0.3219752754296894559, 0.3333333333333333703, 0.3219752754296894559, 0.3333333333333333703, 0.3219752754296894559, 0.3333333333333333703, 0.3219752754296894559, 0.3333333333333333703, 0.3219752754296894559, 0.3333333333333333703, 0.3219752754296894559, 0.3333333333333333703, 0.3219752754296894559, 0.3333333333333333703, 0.3219752754296894559, 0.3333333333333333703, 0.3219752754296894559, 0.3333333333333333703, 0.3219752754296894559, 0.3333333333333333703, 0.3219752754296894559, 0.3333333333333333703, 0.3219752754296894559, 0.3333333333333333703, 0.3219752754296894559, 0.3333333333333333703, 0.3219752754296894559, 0.3333333333333333703, 0.3219752754296894559, 0.3333333333333333703, 0.3219752754296894559, 0.3333333333333333703, 0.3219752754296894559, 0.3333333333333333703, 0.3219752754296894559, 0.3333333333333333703, 0.3219752754296894559, 0.3333333333333333703, 0.3219752754296894559, 0.3333333333333333703, 0.3219752754296894559, 0.3333333333333333703, 0.3219752754296894559, 0.3333333333333333703, 0.3219752754296894559, 0.3333333333333333703, 0.3219752754296894559, 0.3333333333333333703, 0.3219752754296894559, 0.3333333333333333703, 0.3219752754296894559, 0.3333333333333333703, 0.3219752754296894559, 0.3333333333333333703, 0.3219752754296894559, 0.3333333333333333703, 0.3219752754296894559, 0.3333333333333333703, 0.3219752754296894559, 0.3333333333333333703, 0.3219752754296894559, 0.3333333333333333703, 0.3219752754296894559, 0.3333333333333333703, 0.3219752754296894559, 0.3333333333333333703, 0.3219752754296894559, 0.3333333333333333703, 0.3219752754296894559, 0.3333333333333333703, 0.3219752754296894559, 0.3333333333333333703, 0.3219752754296894559, 0.3333333333333333703, 0.3219752754296894559, 0.3333333333333333703, 0.3219752754296894559, 0.3333333333333333703, 0.3219752754296894559, 0.3333333333333333703, 0.3219752754296894559, 0.3333333333333333703, 0.3219752754296894559, 0.3333333333333333703, 0.3219752754296894559, 0.3333333333333333703, 0.3219752754296894559, 0.3333333333333333703, 0.3219752754296894559, 0.3333333333333333703, 0.3219752754296894559, 0.3333333333333333703, 0.3219752754296894559, 0.3333333333333333703, 0.3219752754296894559, 0.3333333333333333703, 0.3219752754296894559, 0.3333333333333333703, 0.3219752754296894559, 0.3333333333333333703, 0.3219752754296894559, 0.3333333333333333703, 0.3219752754296894559, 0.3333333333333333703, 0.3219752754296894559, 0.3333333333333333703, 0.3219752754296894559, 0.3333333333333333703, 0.3219752754296894559, 0.3333333333333333703, 0.3219752754296894559, 0.3333333333333333703, 0.3219752754296894559, 0.3333333333333333703, 0.3219752754296894559, 0.3333333333333333703, 0.3219752754296894559, 0.3333333333333333703, 0.3219752754296894559, 0.3333333333333333703, 0.3219752754296894559, 0.3333333333333333703, 0.3219752754296894559, 0.3333333333333333703, 0.3219752754296894559, 0.3333333333333333703, 0.3219752754296894559, 0.3333333333333333703, 0.3219752754296894559, 0.3333333333333333703, 0.3219752754296894559, 0.3333333333333333703, 0.3219752754296894559, 0.3333333333333333703, 0.3219752754296894559, 0.3333333333333333703, 0.3219752754296894559, 0.3333333333333333703, 0.3219752754296894559, 0.3333333333333333703, 0.3219752754296894559, 0.3333333333333333703, 0.3219752754296894559, 0.3333333333333333703, 0.3219752754296894559, 0.3333333333333333703, 0.3219752754296894559, 0.3333333333333333703, 0.3219752754296894559, 0.3333333333333333703, 0.3219752754296894559, 0.3333333333333333703, 0.3219752754296894559, 0.3333333333333333703, 0.3219752754296894559, 0.3333333333333333703, 0.3219752754296894559, 0.3333333333333333703, 0.3219752754296894559, 0.3333333333333333703, 0.3219752754296894559, 0.3333333333333333703, 0.3219752754296894559, 0.3333333333333333703, 0.3219752754296894559, 0.3333333333333333703, 0.3219752754296894559, 0.3333333333333333703, 0.3219752754296894559, 0.3333333333333333703, 0.3219752754296894559, 0.3333333333333333703, 0.3219752754296894559, 0.3333333333333333703, 0.3219752754296894559, 0.3333333333333333703, 0.3219752754296894559, 0.3333333333333333703, 0.3219752754296894559, 0.3333333333333333703, 0.3219752754296894559, 0.3333333333333333703, 0.3219752754296894559, 0.3333333333333333703, 0.3219752754296894559, 0.3333333333333333703, 0.3219752754296894559, 0.3333333333333333703, 0.3219752754296894559, 0.3333333333333333703, 0.3219752754296894559, 0.3333333333333333703, 0.3219752754296894559, 0.3333333333333333703, 0.3219752754296894559, 0.3333333333333333703, 0.3219752754296894559, 0.3333333333333333703, 0.3219752754296894559, 0.3333333333333333703, 0.3219752754296894559, 0.3333333333333333703),
 ( 0.3333333333333333703, 0.3219752754296894559, 0.3333333333333333703, 0.3219752754296894559, 0.3333333333333333703, 0.3219752754296894559, 0.3333333333333333703, 0.3219752754296894559, 0.3333333333333333703, 0.3219752754296894559, 0.3333333333333333703, 0.3219752754296894559, 0.3333333333333333703, 0.3219752754296894559, 0.3333333333333333703, 0.3219752754296894559, 0.3333333333333333703, 0.3219752754296894559, 0.3333333333333333703, 0.3219752754296894559, 0.3333333333333333703, 0.3219752754296894559, 0.3333333333333333703, 0.3219752754296894559, 0.3333333333333333703, 0.3219752754296894559, 0.3333333333333333703, 0.3219752754296894559, 0.3333333333333333703, 0.3219752754296894559, 0.3333333333333333703, 0.3219752754296894559, 0.3333333333333333703, 0.3219752754296894559, 0.3333333333333333703, 0.3219752754296894559, 0.3333333333333333703, 0.3219752754296894559, 0.3333333333333333703, 0.3219752754296894559, 0.3333333333333333703, 0.3219752754296894559, 0.3333333333333333703, 0.3219752754296894559, 0.3333333333333333703, 0.3219752754296894559, 0.3333333333333333703, 0.3219752754296894559, 0.3333333333333333703, 0.3219752754296894559, 0.3333333333333333703, 0.3219752754296894559, 0.3333333333333333703, 0.3219752754296894559, 0.3333333333333333703, 0.3219752754296894559, 0.3333333333333333703, 0.3219752754296894559, 0.3333333333333333703, 0.3219752754296894559, 0.3333333333333333703, 0.3219752754296894559, 0.3333333333333333703, 0.3219752754296894559, 0.3333333333333333703, 0.3219752754296894559, 0.3333333333333333703, 0.3219752754296894559, 0.3333333333333333703, 0.3219752754296894559, 0.3333333333333333703, 0.3219752754296894559, 0.3333333333333333703, 0.3219752754296894559, 0.3333333333333333703, 0.3219752754296894559, 0.3333333333333333703, 0.3219752754296894559, 0.3333333333333333703, 0.3219752754296894559, 0.3333333333333333703, 0.3219752754296894559, 0.3333333333333333703, 0.3219752754296894559, 0.3333333333333333703, 0.3219752754296894559, 0.3333333333333333703, 0.3219752754296894559, 0.3333333333333333703, 0.3219752754296894559, 0.3333333333333333703, 0.3219752754296894559, 0.3333333333333333703, 0.3219752754296894559, 0.3333333333333333703, 0.3219752754296894559, 0.3333333333333333703, 0.3219752754296894559, 0.3333333333333333703, 0.3219752754296894559, 0.3333333333333333703, 0.3219752754296894559, 0.3333333333333333703, 0.3219752754296894559, 0.3333333333333333703, 0.3219752754296894559, 0.3333333333333333703, 0.3219752754296894559, 0.3333333333333333703, 0.3219752754296894559, 0.3333333333333333703, 0.3219752754296894559, 0.3333333333333333703, 0.3219752754296894559, 0.3333333333333333703, 0.3219752754296894559, 0.3333333333333333703, 0.3219752754296894559, 0.3333333333333333703, 0.3219752754296894559, 0.3333333333333333703, 0.3219752754296894559, 0.3333333333333333703, 0.3219752754296894559, 0.3333333333333333703, 0.3219752754296894559, 0.3333333333333333703, 0.3219752754296894559, 0.3333333333333333703, 0.3219752754296894559, 0.3333333333333333703, 0.3219752754296894559, 0.3333333333333333703, 0.3219752754296894559, 0.3333333333333333703, 0.3219752754296894559, 0.3333333333333333703, 0.3219752754296894559, 0.3333333333333333703, 0.3219752754296894559, 0.3333333333333333703, 0.3219752754296894559, 0.3333333333333333703, 0.3219752754296894559, 0.3333333333333333703, 0.3219752754296894559, 0.3333333333333333703, 0.3219752754296894559, 0.3333333333333333703, 0.3219752754296894559, 0.3333333333333333703, 0.3219752754296894559, 0.3333333333333333703, 0.3219752754296894559, 0.3333333333333333703, 0.3219752754296894559, 0.3333333333333333703, 0.3219752754296894559, 0.3333333333333333703, 0.3219752754296894559, 0.3333333333333333703, 0.3219752754296894559, 0.3333333333333333703, 0.3219752754296894559, 0.3333333333333333703, 0.3219752754296894559, 0.3333333333333333703, 0.3219752754296894559, 0.3333333333333333703, 0.3219752754296894559, 0.3333333333333333703, 0.3219752754296894559, 0.3333333333333333703, 0.3219752754296894559, 0.3333333333333333703, 0.3219752754296894559, 0.3333333333333333703, 0.3219752754296894559, 0.3333333333333333703, 0.3219752754296894559, 0.3333333333333333703, 0.3219752754296894559, 0.3333333333333333703, 0.3219752754296894559, 0.3333333333333333703, 0.3219752754296894559, 0.3333333333333333703, 0.3219752754296894559, 0.3333333333333333703, 0.3219752754296894559, 0.3333333333333333703, 0.3219752754296894559, 0.3333333333333333703, 0.3219752754296894559, 0.3333333333333333703, 0.3219752754296894559, 0.3333333333333333703, 0.3219752754296894559, 0.3333333333333333703, 0.3219752754296894559, 0.3333333333333333703, 0.3219752754296894559, 0.3333333333333333703, 0.3219752754296894559, 0.3333333333333333703, 0.3219752754296894559, 0.3333333333333333703, 0.3219752754296894559, 0.3333333333333333703, 0.3219752754296894559, 0.3333333333333333703, 0.3219752754296894559, 0.3333333333333333703, 0.3219752754296894559, 0.3333333333333333703, 0.3219752754296894559, 0.3333333333333333703, 0.3219752754296894559, 0.3333333333333333703, 0.3219752754296894559, 0.3333333333333333703, 0.3219752754296894559, 0.3333333333333333703, 0.3219752754296894559, 0.3333333333333333703, 0.3219752754296894559, 0.3333333333333333703, 0.3219752754296894559, 0.3333333333333333703, 0.3219752754296894559, 0.3333333333333333703, 0.3219752754296894559, 0.3333333333333333703, 0.3219752754296894559, 0.3333333333333333703, 0.3219752754296894559, 0.3333333333333333703, 0.3219752754296894559, 0.3333333333333333703, 0.3219752754296894559, 0.3333333333333333703, 0.3219752754296894559, 0.3333333333333333703, 0.3219752754296894559, 0.3333333333333333703, 0.3219752754296894559, 0.3333333333333333703, 0.3219752754296894559, 0.3333333333333333703, 0.3219752754296894559, 0.3333333333333333703, 0.3219752754296894559, 0.3333333333333333703, 0.3219752754296894559, 0.3333333333333333703, 0.3219752754296894559, 0.3333333333333333703, 0.3219752754296894559, 0.3333333333333333703, 0.3219752754296894559, 0.3333333333333333703, 0.3219752754296894559, 0.3333333333333333703, 0.3219752754296894559, 0.3333333333333333703, 0.3219752754296894559, 0.3333333333333333703, 0.3219752754296894559, 0.3333333333333333703, 0.3219752754296894559, 0.3333333333333333703, 0.3219752754296894559, 0.3333333333333333703, 0.3219752754296894559, 0.3333333333333333703, 0.3219752754296894559, 0.3333333333333333703, 0.3219752754296894559, 0.3333333333333333703, 0.3219752754296894559, 0.3333333333333333703, 0.3219752754296894559, 0.3333333333333333703, 0.3219752754296894559, 0.3333333333333333703, 0.3219752754296894559, 0.3333333333333333703, 0.3219752754296894559, 0.3333333333333333703, 0.3219752754296894559, 0.3333333333333333703, 0.3219752754296894559, 0.3333333333333333703, 0.3219752754296894559, 0.3333333333333333703, 0.3219752754296894559, 0.3333333333333333703, 0.3219752754296894559, 0.3333333333333333703, 0.3219752754296894559, 0.3333333333333333703, 0.3219752754296894559, 0.3333333333333333703, 0.3219752754296894559, 0.3333333333333333703, 0.3219752754296894559, 0.3333333333333333703, 0.3219752754296894559, 0.3333333333333333703, 0.3219752754296894559, 0.3333333333333333703, 0.3219752754296894559, 0.3333333333333333703, 0.3219752754296894559, 0.3333333333333333703, 0.3219752754296894559, 0.3333333333333333703, 0.3219752754296894559, 0.3333333333333333703, 0.3219752754296894559, 0.3333333333333333703, 0.3219752754296894559, 0.3333333333333333703, 0.3219752754296894559, 0.3333333333333333703, 0.3219752754296894559, 0.3333333333333333703, 0.3219752754296894559, 0.3333333333333333703, 0.3219752754296894559, 0.3333333333333333703, 0.3219752754296894559, 0.3333333333333333703, 0.3219752754296894559, 0.3333333333333333703, 0.3219752754296894559, 0.3333333333333333703, 0.3219752754296894559, 0.3333333333333333703, 0.3219752754296894559, 0.3333333333333333703, 0.3219752754296894559, 0.3333333333333333703, 0.3219752754296894559, 0.3333333333333333703, 0.3219752754296894559, 0.3333333333333333703, 0.3219752754296894559, 0.3333333333333333703, 0.3219752754296894559, 0.3333333333333333703, 0.3219752754296894559, 0.3333333333333333703, 0.3219752754296894559, 0.3333333333333333703, 0.3219752754296894559, 0.3333333333333333703, 0.3219752754296894559, 0.3333333333333333703, 0.3219752754296894559, 0.3333333333333333703, 0.3219752754296894559, 0.3333333333333333703, 0.3219752754296894559, 0.3333333333333333703, 0.3219752754296894559, 0.3333333333333333703, 0.3219752754296894559, 0.3333333333333333703, 0.3219752754296894559, 0.3333333333333333703, 0.3219752754296894559, 0.3333333333333333703, 0.3219752754296894559, 0.3333333333333333703, 0.3219752754296894559, 0.3333333333333333703, 0.3219752754296894559, 0.3333333333333333703, 0.3219752754296894559, 0.3333333333333333703, 0.3219752754296894559, 0.3333333333333333703, 0.3219752754296894559, 0.3333333333333333703, 0.3219752754296894559, 0.3333333333333333703, 0.3219752754296894559, 0.3333333333333333703, 0.3219752754296894559, 0.3333333333333333703, 0.3219752754296894559, 0.3333333333333333703, 0.3219752754296894559, 0.3333333333333333703, 0.3219752754296894559, 0.3333333333333333703, 0.3219752754296894559, 0.3333333333333333703, 0.3219752754296894559, 0.3333333333333333703, 0.3219752754296894559, 0.3333333333333333703, 0.3219752754296894559, 0.3333333333333333703, 0.3219752754296894559, 0.3333333333333333703, 0.3219752754296894559, 0.3333333333333333703, 0.3219752754296894559, 0.3333333333333333703, 0.3219752754296894559, 0.3333333333333333703, 0.3219752754296894559, 0.3333333333333333703, 0.3219752754296894559, 0.3333333333333333703, 0.3219752754296894559, 0.3333333333333333703, 0.3219752754296894559, 0.3333333333333333703, 0.3219752754296894559, 0.3333333333333333703, 0.3219752754296894559, 0.3333333333333333703, 0.3219752754296894559, 0.3333333333333333703, 0.3219752754296894559, 0.3333333333333333703, 0.3219752754296894559, 0.3333333333333333703, 0.3219752754296894559, 0.3333333333333333703, 0.3219752754296894559, 0.3333333333333333703, 0.3219752754296894559, 0.3333333333333333703, 0.3219752754296894559, 0.3333333333333333703, 0.3219752754296894559, 0.3333333333333333703, 0.3219752754296894559, 0.3333333333333333703, 0.3219752754296894559, 0.3333333333333333703, 0.3219752754296894559, 0.3333333333333333703, 0.3219752754296894559, 0.3333333333333333703, 0.3219752754296894559, 0.3333333333333333703, 0.3219752754296894559, 0.3333333333333333703, 0.3219752754296894559, 0.3333333333333333703, 0.3219752754296894559, 0.3333333333333333703),
 ( 1.000000000000000000, 0.9659258262890683122, 1.000000000000000000, 0.9659258262890683122, 1.000000000000000000, 0.9659258262890683122, 1.000000000000000000, 0.9659258262890683122, 1.000000000000000000, 0.9659258262890683122, 1.000000000000000000, 0.9659258262890683122, 1.000000000000000000, 0.9659258262890683122, 1.000000000000000000, 0.9659258262890683122, 1.000000000000000000, 0.9659258262890683122, 1.000000000000000000, 0.9659258262890683122, 1.000000000000000000, 0.9659258262890683122, 1.000000000000000000, 0.9659258262890683122, 1.000000000000000000, 0.9659258262890683122, 1.000000000000000000, 0.9659258262890683122, 1.000000000000000000, 0.9659258262890683122, 1.000000000000000000, 0.9659258262890683122, 1.000000000000000000, 0.9659258262890683122, 1.000000000000000000, 0.9659258262890683122, 1.000000000000000000, 0.9659258262890683122, 1.000000000000000000, 0.9659258262890683122, 1.000000000000000000, 0.9659258262890683122, 1.000000000000000000, 0.9659258262890683122, 1.000000000000000000, 0.9659258262890683122, 1.000000000000000000, 0.9659258262890683122, 1.000000000000000000, 0.9659258262890683122, 1.000000000000000000, 0.9659258262890683122, 1.000000000000000000, 0.9659258262890683122, 1.000000000000000000, 0.9659258262890683122, 1.000000000000000000, 0.9659258262890683122, 1.000000000000000000, 0.9659258262890683122, 1.000000000000000000, 0.9659258262890683122, 1.000000000000000000, 0.9659258262890683122, 1.000000000000000000, 0.9659258262890683122, 1.000000000000000000, 0.9659258262890683122, 1.000000000000000000, 0.9659258262890683122, 1.000000000000000000, 0.9659258262890683122, 1.000000000000000000, 0.9659258262890683122, 1.000000000000000000, 0.9659258262890683122, 1.000000000000000000, 0.9659258262890683122, 1.000000000000000000, 0.9659258262890683122, 1.000000000000000000, 0.9659258262890683122, 1.000000000000000000, 0.9659258262890683122, 1.000000000000000000, 0.9659258262890683122, 1.000000000000000000, 0.9659258262890683122, 1.000000000000000000, 0.9659258262890683122, 1.000000000000000000, 0.9659258262890683122, 1.000000000000000000, 0.9659258262890683122, 1.000000000000000000, 0.9659258262890683122, 1.000000000000000000, 0.9659258262890683122, 1.000000000000000000, 0.9659258262890683122, 1.000000000000000000, 0.9659258262890683122, 1.000000000000000000, 0.9659258262890683122, 1.000000000000000000, 0.9659258262890683122, 1.000000000000000000, 0.9659258262890683122, 1.000000000000000000, 0.9659258262890683122, 1.000000000000000000, 0.9659258262890683122, 1.000000000000000000, 0.9659258262890683122, 1.000000000000000000, 0.9659258262890683122, 1.000000000000000000, 0.9659258262890683122, 1.000000000000000000, 0.9659258262890683122, 1.000000000000000000, 0.9659258262890683122, 1.000000000000000000, 0.9659258262890683122, 1.000000000000000000, 0.9659258262890683122, 1.000000000000000000, 0.9659258262890683122, 1.000000000000000000, 0.9659258262890683122, 1.000000000000000000, 0.9659258262890683122, 1.000000000000000000, 0.9659258262890683122, 1.000000000000000000, 0.9659258262890683122, 1.000000000000000000, 0.9659258262890683122, 1.000000000000000000, 0.9659258262890683122, 1.000000000000000000, 0.9659258262890683122, 1.000000000000000000, 0.9659258262890683122, 1.000000000000000000, 0.9659258262890683122, 1.000000000000000000, 0.9659258262890683122, 1.000000000000000000, 0.9659258262890683122, 1.000000000000000000, 0.9659258262890683122, 1.000000000000000000, 0.9659258262890683122, 1.000000000000000000, 0.9659258262890683122, 1.000000000000000000, 0.9659258262890683122, 1.000000000000000000, 0.9659258262890683122, 1.000000000000000000, 0.9659258262890683122, 1.000000000000000000, 0.9659258262890683122, 1.000000000000000000, 0.9659258262890683122, 1.000000000000000000, 0.9659258262890683122, 1.000000000000000000, 0.9659258262890683122, 1.000000000000000000, 0.9659258262890683122, 1.000000000000000000, 0.9659258262890683122, 1.000000000000000000, 0.9659258262890683122, 1.000000000000000000, 0.9659258262890683122, 1.000000000000000000, 0.9659258262890683122, 1.000000000000000000, 0.9659258262890683122, 1.000000000000000000, 0.9659258262890683122, 1.000000000000000000, 0.9659258262890683122, 1.000000000000000000, 0.9659258262890683122, 1.000000000000000000, 0.9659258262890683122, 1.000000000000000000, 0.9659258262890683122, 1.000000000000000000, 0.9659258262890683122, 1.000000000000000000, 0.9659258262890683122, 1.000000000000000000, 0.9659258262890683122, 1.000000000000000000, 0.9659258262890683122, 1.000000000000000000, 0.9659258262890683122, 1.000000000000000000, 0.9659258262890683122, 1.000000000000000000, 0.9659258262890683122, 1.000000000000000000, 0.9659258262890683122, 1.000000000000000000, 0.9659258262890683122, 1.000000000000000000, 0.9659258262890683122, 1.000000000000000000, 0.9659258262890683122, 1.000000000000000000, 0.9659258262890683122, 1.000000000000000000, 0.9659258262890683122, 1.000000000000000000, 0.9659258262890683122, 1.000000000000000000, 0.9659258262890683122, 1.000000000000000000, 0.9659258262890683122, 1.000000000000000000, 0.9659258262890683122, 1.000000000000000000, 0.9659258262890683122, 1.000000000000000000, 0.9659258262890683122, 1.000000000000000000, 0.9659258262890683122, 1.000000000000000000, 0.9659258262890683122, 1.000000000000000000, 0.9659258262890683122, 1.000000000000000000, 0.9659258262890683122, 1.000000000000000000, 0.9659258262890683122, 1.000000000000000000, 0.9659258262890683122, 1.000000000000000000, 0.9659258262890683122, 1.000000000000000000, 0.9659258262890683122, 1.000000000000000000, 0.9659258262890683122, 1.000000000000000000, 0.9659258262890683122, 1.000000000000000000, 0.9659258262890683122, 1.000000000000000000, 0.9659258262890683122, 1.000000000000000000, 0.9659258262890683122, 1.000000000000000000, 0.9659258262890683122, 1.000000000000000000, 0.9659258262890683122, 1.000000000000000000, 0.9659258262890683122, 1.000000000000000000, 0.9659258262890683122, 1.000000000000000000, 0.9659258262890683122, 1.000000000000000000, 0.9659258262890683122, 1.000000000000000000, 0.9659258262890683122, 1.000000000000000000, 0.9659258262890683122, 1.000000000000000000, 0.9659258262890683122, 1.000000000000000000, 0.9659258262890683122, 1.000000000000000000, 0.9659258262890683122, 1.000000000000000000, 0.9659258262890683122, 1.000000000000000000, 0.9659258262890683122, 1.000000000000000000, 0.9659258262890683122, 1.000000000000000000, 0.9659258262890683122, 1.000000000000000000, 0.9659258262890683122, 1.000000000000000000, 0.9659258262890683122, 1.000000000000000000, 0.9659258262890683122, 1.000000000000000000, 0.9659258262890683122, 1.000000000000000000, 0.9659258262890683122, 1.000000000000000000, 0.9659258262890683122, 1.000000000000000000, 0.9659258262890683122, 1.000000000000000000, 0.9659258262890683122, 1.000000000000000000, 0.9659258262890683122, 1.000000000000000000, 0.9659258262890683122, 1.000000000000000000, 0.9659258262890683122, 1.000000000000000000, 0.9659258262890683122, 1.000000000000000000, 0.9659258262890683122, 1.000000000000000000, 0.9659258262890683122, 1.000000000000000000, 0.9659258262890683122, 1.000000000000000000, 0.9659258262890683122, 1.000000000000000000, 0.9659258262890683122, 1.000000000000000000, 0.9659258262890683122, 1.000000000000000000, 0.9659258262890683122, 1.000000000000000000, 0.9659258262890683122, 1.000000000000000000, 0.9659258262890683122, 1.000000000000000000, 0.9659258262890683122, 1.000000000000000000, 0.9659258262890683122, 1.000000000000000000, 0.9659258262890683122, 1.000000000000000000, 0.9659258262890683122, 1.000000000000000000, 0.9659258262890683122, 1.000000000000000000, 0.9659258262890683122, 1.000000000000000000, 0.9659258262890683122, 1.000000000000000000, 0.9659258262890683122, 1.000000000000000000, 0.9659258262890683122, 1.000000000000000000, 0.9659258262890683122, 1.000000000000000000, 0.9659258262890683122, 1.000000000000000000, 0.9659258262890683122, 1.000000000000000000, 0.9659258262890683122, 1.000000000000000000, 0.9659258262890683122, 1.000000000000000000, 0.9659258262890683122, 1.000000000000000000, 0.9659258262890683122, 1.000000000000000000, 0.9659258262890683122, 1.000000000000000000, 0.9659258262890683122, 1.000000000000000000, 0.9659258262890683122, 1.000000000000000000, 0.9659258262890683122, 1.000000000000000000, 0.9659258262890683122, 1.000000000000000000, 0.9659258262890683122, 1.000000000000000000, 0.9659258262890683122, 1.000000000000000000, 0.9659258262890683122, 1.000000000000000000, 0.9659258262890683122, 1.000000000000000000, 0.9659258262890683122, 1.000000000000000000, 0.9659258262890683122, 1.000000000000000000, 0.9659258262890683122, 1.000000000000000000, 0.9659258262890683122, 1.000000000000000000, 0.9659258262890683122, 1.000000000000000000, 0.9659258262890683122, 1.000000000000000000, 0.9659258262890683122, 1.000000000000000000, 0.9659258262890683122, 1.000000000000000000, 0.9659258262890683122, 1.000000000000000000, 0.9659258262890683122, 1.000000000000000000, 0.9659258262890683122, 1.000000000000000000, 0.9659258262890683122, 1.000000000000000000, 0.9659258262890683122, 1.000000000000000000, 0.9659258262890683122, 1.000000000000000000, 0.9659258262890683122, 1.000000000000000000, 0.9659258262890683122, 1.000000000000000000, 0.9659258262890683122, 1.000000000000000000, 0.9659258262890683122, 1.000000000000000000, 0.9659258262890683122, 1.000000000000000000, 0.9659258262890683122, 1.000000000000000000, 0.9659258262890683122, 1.000000000000000000, 0.9659258262890683122, 1.000000000000000000, 0.9659258262890683122, 1.000000000000000000, 0.9659258262890683122, 1.000000000000000000, 0.9659258262890683122, 1.000000000000000000, 0.9659258262890683122, 1.000000000000000000, 0.9659258262890683122, 1.000000000000000000, 0.9659258262890683122, 1.000000000000000000, 0.9659258262890683122, 1.000000000000000000, 0.9659258262890683122, 1.000000000000000000, 0.9659258262890683122, 1.000000000000000000, 0.9659258262890683122, 1.000000000000000000, 0.9659258262890683122, 1.000000000000000000, 0.9659258262890683122, 1.000000000000000000, 0.9659258262890683122, 1.000000000000000000, 0.9659258262890683122, 1.000000000000000000, 0.9659258262890683122, 1.000000000000000000, 0.9659258262890683122, 1.000000000000000000, 0.9659258262890683122, 1.000000000000000000),
 ( 0.3333333333333333703, 0.3219752754296894559, 0.3333333333333333703, 0.3219752754296894559, 0.3333333333333333703, 0.3219752754296894559, 0.3333333333333333703, 0.3219752754296894559, 0.3333333333333333703, 0.3219752754296894559, 0.3333333333333333703, 0.3219752754296894559, 0.3333333333333333703, 0.3219752754296894559, 0.3333333333333333703, 0.3219752754296894559, 0.3333333333333333703, 0.3219752754296894559, 0.3333333333333333703, 0.3219752754296894559, 0.3333333333333333703, 0.3219752754296894559, 0.3333333333333333703, 0.3219752754296894559, 0.3333333333333333703, 0.3219752754296894559, 0.3333333333333333703, 0.3219752754296894559, 0.3333333333333333703, 0.3219752754296894559, 0.3333333333333333703, 0.3219752754296894559, 0.3333333333333333703, 0.3219752754296894559, 0.3333333333333333703, 0.3219752754296894559, 0.3333333333333333703, 0.3219752754296894559, 0.3333333333333333703, 0.3219752754296894559, 0.3333333333333333703, 0.3219752754296894559, 0.3333333333333333703, 0.3219752754296894559, 0.3333333333333333703, 0.3219752754296894559, 0.3333333333333333703, 0.3219752754296894559, 0.3333333333333333703, 0.3219752754296894559, 0.3333333333333333703, 0.3219752754296894559, 0.3333333333333333703, 0.3219752754296894559, 0.3333333333333333703, 0.3219752754296894559, 0.3333333333333333703, 0.3219752754296894559, 0.3333333333333333703, 0.3219752754296894559, 0.3333333333333333703, 0.3219752754296894559, 0.3333333333333333703, 0.3219752754296894559, 0.3333333333333333703, 0.3219752754296894559, 0.3333333333333333703, 0.3219752754296894559, 0.3333333333333333703, 0.3219752754296894559, 0.3333333333333333703, 0.3219752754296894559, 0.3333333333333333703, 0.3219752754296894559, 0.3333333333333333703, 0.3219752754296894559, 0.3333333333333333703, 0.3219752754296894559, 0.3333333333333333703, 0.3219752754296894559, 0.3333333333333333703, 0.3219752754296894559, 0.3333333333333333703, 0.3219752754296894559, 0.3333333333333333703, 0.3219752754296894559, 0.3333333333333333703, 0.3219752754296894559, 0.3333333333333333703, 0.3219752754296894559, 0.3333333333333333703, 0.3219752754296894559, 0.3333333333333333703, 0.3219752754296894559, 0.3333333333333333703, 0.3219752754296894559, 0.3333333333333333703, 0.3219752754296894559, 0.3333333333333333703, 0.3219752754296894559, 0.3333333333333333703, 0.3219752754296894559, 0.3333333333333333703, 0.3219752754296894559, 0.3333333333333333703, 0.3219752754296894559, 0.3333333333333333703, 0.3219752754296894559, 0.3333333333333333703, 0.3219752754296894559, 0.3333333333333333703, 0.3219752754296894559, 0.3333333333333333703, 0.3219752754296894559, 0.3333333333333333703, 0.3219752754296894559, 0.3333333333333333703, 0.3219752754296894559, 0.3333333333333333703, 0.3219752754296894559, 0.3333333333333333703, 0.3219752754296894559, 0.3333333333333333703, 0.3219752754296894559, 0.3333333333333333703, 0.3219752754296894559, 0.3333333333333333703, 0.3219752754296894559, 0.3333333333333333703, 0.3219752754296894559, 0.3333333333333333703, 0.3219752754296894559, 0.3333333333333333703, 0.3219752754296894559, 0.3333333333333333703, 0.3219752754296894559, 0.3333333333333333703, 0.3219752754296894559, 0.3333333333333333703, 0.3219752754296894559, 0.3333333333333333703, 0.3219752754296894559, 0.3333333333333333703, 0.3219752754296894559, 0.3333333333333333703, 0.3219752754296894559, 0.3333333333333333703, 0.3219752754296894559, 0.3333333333333333703, 0.3219752754296894559, 0.3333333333333333703, 0.3219752754296894559, 0.3333333333333333703, 0.3219752754296894559, 0.3333333333333333703, 0.3219752754296894559, 0.3333333333333333703, 0.3219752754296894559, 0.3333333333333333703, 0.3219752754296894559, 0.3333333333333333703, 0.3219752754296894559, 0.3333333333333333703, 0.3219752754296894559, 0.3333333333333333703, 0.3219752754296894559, 0.3333333333333333703, 0.3219752754296894559, 0.3333333333333333703, 0.3219752754296894559, 0.3333333333333333703, 0.3219752754296894559, 0.3333333333333333703, 0.3219752754296894559, 0.3333333333333333703, 0.3219752754296894559, 0.3333333333333333703, 0.3219752754296894559, 0.3333333333333333703, 0.3219752754296894559, 0.3333333333333333703, 0.3219752754296894559, 0.3333333333333333703, 0.3219752754296894559, 0.3333333333333333703, 0.3219752754296894559, 0.3333333333333333703, 0.3219752754296894559, 0.3333333333333333703, 0.3219752754296894559, 0.3333333333333333703, 0.3219752754296894559, 0.3333333333333333703, 0.3219752754296894559, 0.3333333333333333703, 0.3219752754296894559, 0.3333333333333333703, 0.3219752754296894559, 0.3333333333333333703, 0.3219752754296894559, 0.3333333333333333703, 0.3219752754296894559, 0.3333333333333333703, 0.3219752754296894559, 0.3333333333333333703, 0.3219752754296894559, 0.3333333333333333703, 0.3219752754296894559, 0.3333333333333333703, 0.3219752754296894559, 0.3333333333333333703, 0.3219752754296894559, 0.3333333333333333703, 0.3219752754296894559, 0.3333333333333333703, 0.3219752754296894559, 0.3333333333333333703, 0.3219752754296894559, 0.3333333333333333703, 0.3219752754296894559, 0.3333333333333333703, 0.3219752754296894559, 0.3333333333333333703, 0.3219752754296894559, 0.3333333333333333703, 0.3219752754296894559, 0.3333333333333333703, 0.3219752754296894559, 0.3333333333333333703, 0.3219752754296894559, 0.3333333333333333703, 0.3219752754296894559, 0.3333333333333333703, 0.3219752754296894559, 0.3333333333333333703, 0.3219752754296894559, 0.3333333333333333703, 0.3219752754296894559, 0.3333333333333333703, 0.3219752754296894559, 0.3333333333333333703, 0.3219752754296894559, 0.3333333333333333703, 0.3219752754296894559, 0.3333333333333333703, 0.3219752754296894559, 0.3333333333333333703, 0.3219752754296894559, 0.3333333333333333703, 0.3219752754296894559, 0.3333333333333333703, 0.3219752754296894559, 0.3333333333333333703, 0.3219752754296894559, 0.3333333333333333703, 0.3219752754296894559, 0.3333333333333333703, 0.3219752754296894559, 0.3333333333333333703, 0.3219752754296894559, 0.3333333333333333703, 0.3219752754296894559, 0.3333333333333333703, 0.3219752754296894559, 0.3333333333333333703, 0.3219752754296894559, 0.3333333333333333703, 0.3219752754296894559, 0.3333333333333333703, 0.3219752754296894559, 0.3333333333333333703, 0.3219752754296894559, 0.3333333333333333703, 0.3219752754296894559, 0.3333333333333333703, 0.3219752754296894559, 0.3333333333333333703, 0.3219752754296894559, 0.3333333333333333703, 0.3219752754296894559, 0.3333333333333333703, 0.3219752754296894559, 0.3333333333333333703, 0.3219752754296894559, 0.3333333333333333703, 0.3219752754296894559, 0.3333333333333333703, 0.3219752754296894559, 0.3333333333333333703, 0.3219752754296894559, 0.3333333333333333703, 0.3219752754296894559, 0.3333333333333333703, 0.3219752754296894559, 0.3333333333333333703, 0.3219752754296894559, 0.3333333333333333703, 0.3219752754296894559, 0.3333333333333333703, 0.3219752754296894559, 0.3333333333333333703, 0.3219752754296894559, 0.3333333333333333703, 0.3219752754296894559, 0.3333333333333333703, 0.3219752754296894559, 0.3333333333333333703, 0.3219752754296894559, 0.3333333333333333703, 0.3219752754296894559, 0.3333333333333333703, 0.3219752754296894559, 0.3333333333333333703, 0.3219752754296894559, 0.3333333333333333703, 0.3219752754296894559, 0.3333333333333333703, 0.3219752754296894559, 0.3333333333333333703, 0.3219752754296894559, 0.3333333333333333703, 0.3219752754296894559, 0.3333333333333333703, 0.3219752754296894559, 0.3333333333333333703, 0.3219752754296894559, 0.3333333333333333703, 0.3219752754296894559, 0.3333333333333333703, 0.3219752754296894559, 0.3333333333333333703, 0.3219752754296894559, 0.3333333333333333703, 0.3219752754296894559, 0.3333333333333333703, 0.3219752754296894559, 0.3333333333333333703, 0.3219752754296894559, 0.3333333333333333703, 0.3219752754296894559, 0.3333333333333333703, 0.3219752754296894559, 0.3333333333333333703, 0.3219752754296894559, 0.3333333333333333703, 0.3219752754296894559, 0.3333333333333333703, 0.3219752754296894559, 0.3333333333333333703, 0.3219752754296894559, 0.3333333333333333703, 0.3219752754296894559, 0.3333333333333333703, 0.3219752754296894559, 0.3333333333333333703, 0.3219752754296894559, 0.3333333333333333703, 0.3219752754296894559, 0.3333333333333333703, 0.3219752754296894559, 0.3333333333333333703, 0.3219752754296894559, 0.3333333333333333703, 0.3219752754296894559, 0.3333333333333333703, 0.3219752754296894559, 0.3333333333333333703, 0.3219752754296894559, 0.3333333333333333703, 0.3219752754296894559, 0.3333333333333333703, 0.3219752754296894559, 0.3333333333333333703, 0.3219752754296894559, 0.3333333333333333703, 0.3219752754296894559, 0.3333333333333333703, 0.3219752754296894559, 0.3333333333333333703, 0.3219752754296894559, 0.3333333333333333703, 0.3219752754296894559, 0.3333333333333333703, 0.3219752754296894559, 0.3333333333333333703, 0.3219752754296894559, 0.3333333333333333703, 0.3219752754296894559, 0.3333333333333333703, 0.3219752754296894559, 0.3333333333333333703, 0.3219752754296894559, 0.3333333333333333703, 0.3219752754296894559, 0.3333333333333333703, 0.3219752754296894559, 0.3333333333333333703, 0.3219752754296894559, 0.3333333333333333703, 0.3219752754296894559, 0.3333333333333333703, 0.3219752754296894559, 0.3333333333333333703, 0.3219752754296894559, 0.3333333333333333703, 0.3219752754296894559, 0.3333333333333333703, 0.3219752754296894559, 0.3333333333333333703, 0.3219752754296894559, 0.3333333333333333703, 0.3219752754296894559, 0.3333333333333333703, 0.3219752754296894559, 0.3333333333333333703, 0.3219752754296894559, 0.3333333333333333703, 0.3219752754296894559, 0.3333333333333333703, 0.3219752754296894559, 0.3333333333333333703, 0.3219752754296894559, 0.3333333333333333703, 0.3219752754296894559, 0.3333333333333333703, 0.3219752754296894559, 0.3333333333333333703, 0.3219752754296894559, 0.3333333333333333703, 0.3219752754296894559, 0.3333333333333333703, 0.3219752754296894559, 0.3333333333333333703, 0.3219752754296894559, 0.3333333333333333703, 0.3219752754296894559, 0.3333333333333333703, 0.3219752754296894559, 0.3333333333333333703, 0.3219752754296894559, 0.3333333333333333703, 0.3219752754296894559, 0.3333333333333333703, 0.3219752754296894559, 0.3333333333333333703, 0.3219752754296894559, 0.3333333333333333703, 0.3219752754296894559, 0.3333333333333333703, 0.3219752754296894559, 0.3333333333333333703, 0.3219752754296894559, 0.3333333333333333703, 0.3219752754296894559, 0.3333333333333333703, 0.3219752754296894559, 0.3333333333333333703),
 ( 0.3333333333333333703, 0.3219752754296894559, 0.3333333333333333703, 0.3219752754296894559, 0.3333333333333333703, 0.3219752754296894559, 0.3333333333333333703, 0.3219752754296894559, 0.3333333333333333703, 0.3219752754296894559, 0.3333333333333333703, 0.3219752754296894559, 0.3333333333333333703, 0.3219752754296894559, 0.3333333333333333703, 0.3219752754296894559, 0.3333333333333333703, 0.3219752754296894559, 0.3333333333333333703, 0.3219752754296894559, 0.3333333333333333703, 0.3219752754296894559, 0.3333333333333333703, 0.3219752754296894559, 0.3333333333333333703, 0.3219752754296894559, 0.3333333333333333703, 0.3219752754296894559, 0.3333333333333333703, 0.3219752754296894559, 0.3333333333333333703, 0.3219752754296894559, 0.3333333333333333703, 0.3219752754296894559, 0.3333333333333333703, 0.3219752754296894559, 0.3333333333333333703, 0.3219752754296894559, 0.3333333333333333703, 0.3219752754296894559, 0.3333333333333333703, 0.3219752754296894559, 0.3333333333333333703, 0.3219752754296894559, 0.3333333333333333703, 0.3219752754296894559, 0.3333333333333333703, 0.3219752754296894559, 0.3333333333333333703, 0.3219752754296894559, 0.3333333333333333703, 0.3219752754296894559, 0.3333333333333333703, 0.3219752754296894559, 0.3333333333333333703, 0.3219752754296894559, 0.3333333333333333703, 0.3219752754296894559, 0.3333333333333333703, 0.3219752754296894559, 0.3333333333333333703, 0.3219752754296894559, 0.3333333333333333703, 0.3219752754296894559, 0.3333333333333333703, 0.3219752754296894559, 0.3333333333333333703, 0.3219752754296894559, 0.3333333333333333703, 0.3219752754296894559, 0.3333333333333333703, 0.3219752754296894559, 0.3333333333333333703, 0.3219752754296894559, 0.3333333333333333703, 0.3219752754296894559, 0.3333333333333333703, 0.3219752754296894559, 0.3333333333333333703, 0.3219752754296894559, 0.3333333333333333703, 0.3219752754296894559, 0.3333333333333333703, 0.3219752754296894559, 0.3333333333333333703, 0.3219752754296894559, 0.3333333333333333703, 0.3219752754296894559, 0.3333333333333333703, 0.3219752754296894559, 0.3333333333333333703, 0.3219752754296894559, 0.3333333333333333703, 0.3219752754296894559, 0.3333333333333333703, 0.3219752754296894559, 0.3333333333333333703, 0.3219752754296894559, 0.3333333333333333703, 0.3219752754296894559, 0.3333333333333333703, 0.3219752754296894559, 0.3333333333333333703, 0.3219752754296894559, 0.3333333333333333703, 0.3219752754296894559, 0.3333333333333333703, 0.3219752754296894559, 0.3333333333333333703, 0.3219752754296894559, 0.3333333333333333703, 0.3219752754296894559, 0.3333333333333333703, 0.3219752754296894559, 0.3333333333333333703, 0.3219752754296894559, 0.3333333333333333703, 0.3219752754296894559, 0.3333333333333333703, 0.3219752754296894559, 0.3333333333333333703, 0.3219752754296894559, 0.3333333333333333703, 0.3219752754296894559, 0.3333333333333333703, 0.3219752754296894559, 0.3333333333333333703, 0.3219752754296894559, 0.3333333333333333703, 0.3219752754296894559, 0.3333333333333333703, 0.3219752754296894559, 0.3333333333333333703, 0.3219752754296894559, 0.3333333333333333703, 0.3219752754296894559, 0.3333333333333333703, 0.3219752754296894559, 0.3333333333333333703, 0.3219752754296894559, 0.3333333333333333703, 0.3219752754296894559, 0.3333333333333333703, 0.3219752754296894559, 0.3333333333333333703, 0.3219752754296894559, 0.3333333333333333703, 0.3219752754296894559, 0.3333333333333333703, 0.3219752754296894559, 0.3333333333333333703, 0.3219752754296894559, 0.3333333333333333703, 0.3219752754296894559, 0.3333333333333333703, 0.3219752754296894559, 0.3333333333333333703, 0.3219752754296894559, 0.3333333333333333703, 0.3219752754296894559, 0.3333333333333333703, 0.3219752754296894559, 0.3333333333333333703, 0.3219752754296894559, 0.3333333333333333703, 0.3219752754296894559, 0.3333333333333333703, 0.3219752754296894559, 0.3333333333333333703, 0.3219752754296894559, 0.3333333333333333703, 0.3219752754296894559, 0.3333333333333333703, 0.3219752754296894559, 0.3333333333333333703, 0.3219752754296894559, 0.3333333333333333703, 0.3219752754296894559, 0.3333333333333333703, 0.3219752754296894559, 0.3333333333333333703, 0.3219752754296894559, 0.3333333333333333703, 0.3219752754296894559, 0.3333333333333333703, 0.3219752754296894559, 0.3333333333333333703, 0.3219752754296894559, 0.3333333333333333703, 0.3219752754296894559, 0.3333333333333333703, 0.3219752754296894559, 0.3333333333333333703, 0.3219752754296894559, 0.3333333333333333703, 0.3219752754296894559, 0.3333333333333333703, 0.3219752754296894559, 0.3333333333333333703, 0.3219752754296894559, 0.3333333333333333703, 0.3219752754296894559, 0.3333333333333333703, 0.3219752754296894559, 0.3333333333333333703, 0.3219752754296894559, 0.3333333333333333703, 0.3219752754296894559, 0.3333333333333333703, 0.3219752754296894559, 0.3333333333333333703, 0.3219752754296894559, 0.3333333333333333703, 0.3219752754296894559, 0.3333333333333333703, 0.3219752754296894559, 0.3333333333333333703, 0.3219752754296894559, 0.3333333333333333703, 0.3219752754296894559, 0.3333333333333333703, 0.3219752754296894559, 0.3333333333333333703, 0.3219752754296894559, 0.3333333333333333703, 0.3219752754296894559, 0.3333333333333333703, 0.3219752754296894559, 0.3333333333333333703, 0.3219752754296894559, 0.3333333333333333703, 0.3219752754296894559, 0.3333333333333333703, 0.3219752754296894559, 0.3333333333333333703, 0.3219752754296894559, 0.3333333333333333703, 0.3219752754296894559, 0.3333333333333333703, 0.3219752754296894559, 0.3333333333333333703, 0.3219752754296894559, 0.3333333333333333703, 0.3219752754296894559, 0.3333333333333333703, 0.3219752754296894559, 0.3333333333333333703, 0.3219752754296894559, 0.3333333333333333703, 0.3219752754296894559, 0.3333333333333333703, 0.3219752754296894559, 0.3333333333333333703, 0.3219752754296894559, 0.3333333333333333703, 0.3219752754296894559, 0.3333333333333333703, 0.3219752754296894559, 0.3333333333333333703, 0.3219752754296894559, 0.3333333333333333703, 0.3219752754296894559, 0.3333333333333333703, 0.3219752754296894559, 0.3333333333333333703, 0.3219752754296894559, 0.3333333333333333703, 0.3219752754296894559, 0.3333333333333333703, 0.3219752754296894559, 0.3333333333333333703, 0.3219752754296894559, 0.3333333333333333703, 0.3219752754296894559, 0.3333333333333333703, 0.3219752754296894559, 0.3333333333333333703, 0.3219752754296894559, 0.3333333333333333703, 0.3219752754296894559, 0.3333333333333333703, 0.3219752754296894559, 0.3333333333333333703, 0.3219752754296894559, 0.3333333333333333703, 0.3219752754296894559, 0.3333333333333333703, 0.3219752754296894559, 0.3333333333333333703, 0.3219752754296894559, 0.3333333333333333703, 0.3219752754296894559, 0.3333333333333333703, 0.3219752754296894559, 0.3333333333333333703, 0.3219752754296894559, 0.3333333333333333703, 0.3219752754296894559, 0.3333333333333333703, 0.3219752754296894559, 0.3333333333333333703, 0.3219752754296894559, 0.3333333333333333703, 0.3219752754296894559, 0.3333333333333333703, 0.3219752754296894559, 0.3333333333333333703, 0.3219752754296894559, 0.3333333333333333703, 0.3219752754296894559, 0.3333333333333333703, 0.3219752754296894559, 0.3333333333333333703, 0.3219752754296894559, 0.3333333333333333703, 0.3219752754296894559, 0.3333333333333333703, 0.3219752754296894559, 0.3333333333333333703, 0.3219752754296894559, 0.3333333333333333703, 0.3219752754296894559, 0.3333333333333333703, 0.3219752754296894559, 0.3333333333333333703, 0.3219752754296894559, 0.3333333333333333703, 0.3219752754296894559, 0.3333333333333333703, 0.3219752754296894559, 0.3333333333333333703, 0.3219752754296894559, 0.3333333333333333703, 0.3219752754296894559, 0.3333333333333333703, 0.3219752754296894559, 0.3333333333333333703, 0.3219752754296894559, 0.3333333333333333703, 0.3219752754296894559, 0.3333333333333333703, 0.3219752754296894559, 0.3333333333333333703, 0.3219752754296894559, 0.3333333333333333703, 0.3219752754296894559, 0.3333333333333333703, 0.3219752754296894559, 0.3333333333333333703, 0.3219752754296894559, 0.3333333333333333703, 0.3219752754296894559, 0.3333333333333333703, 0.3219752754296894559, 0.3333333333333333703, 0.3219752754296894559, 0.3333333333333333703, 0.3219752754296894559, 0.3333333333333333703, 0.3219752754296894559, 0.3333333333333333703, 0.3219752754296894559, 0.3333333333333333703, 0.3219752754296894559, 0.3333333333333333703, 0.3219752754296894559, 0.3333333333333333703, 0.3219752754296894559, 0.3333333333333333703, 0.3219752754296894559, 0.3333333333333333703, 0.3219752754296894559, 0.3333333333333333703, 0.3219752754296894559, 0.3333333333333333703, 0.3219752754296894559, 0.3333333333333333703, 0.3219752754296894559, 0.3333333333333333703, 0.3219752754296894559, 0.3333333333333333703, 0.3219752754296894559, 0.3333333333333333703, 0.3219752754296894559, 0.3333333333333333703, 0.3219752754296894559, 0.3333333333333333703, 0.3219752754296894559, 0.3333333333333333703, 0.3219752754296894559, 0.3333333333333333703, 0.3219752754296894559, 0.3333333333333333703, 0.3219752754296894559, 0.3333333333333333703, 0.3219752754296894559, 0.3333333333333333703, 0.3219752754296894559, 0.3333333333333333703, 0.3219752754296894559, 0.3333333333333333703, 0.3219752754296894559, 0.3333333333333333703, 0.3219752754296894559, 0.3333333333333333703, 0.3219752754296894559, 0.3333333333333333703, 0.3219752754296894559, 0.3333333333333333703, 0.3219752754296894559, 0.3333333333333333703, 0.3219752754296894559, 0.3333333333333333703, 0.3219752754296894559, 0.3333333333333333703, 0.3219752754296894559, 0.3333333333333333703, 0.3219752754296894559, 0.3333333333333333703, 0.3219752754296894559, 0.3333333333333333703, 0.3219752754296894559, 0.3333333333333333703, 0.3219752754296894559, 0.3333333333333333703, 0.3219752754296894559, 0.3333333333333333703, 0.3219752754296894559, 0.3333333333333333703, 0.3219752754296894559, 0.3333333333333333703, 0.3219752754296894559, 0.3333333333333333703, 0.3219752754296894559, 0.3333333333333333703, 0.3219752754296894559, 0.3333333333333333703, 0.3219752754296894559, 0.3333333333333333703, 0.3219752754296894559, 0.3333333333333333703, 0.3219752754296894559, 0.3333333333333333703, 0.3219752754296894559, 0.3333333333333333703, 0.3219752754296894559, 0.3333333333333333703, 0.3219752754296894559, 0.3333333333333333703, 0.3219752754296894559, 0.3333333333333333703, 0.3219752754296894559, 0.3333333333333333703, 0.3219752754296894559, 0.3333333333333333703, 0.3219752754296894559, 0.3333333333333333703),
 ( 1.000000000000000000, 0.9659258262890683122, 1.000000000000000000, 0.9659258262890683122, 1.000000000000000000, 0.9659258262890683122, 1.000000000000000000, 0.9659258262890683122, 1.000000000000000000, 0.9659258262890683122, 1.000000000000000000, 0.9659258262890683122, 1.000000000000000000, 0.9659258262890683122, 1.000000000000000000, 0.9659258262890683122, 1.000000000000000000, 0.9659258262890683122, 1.000000000000000000, 0.9659258262890683122, 1.000000000000000000, 0.9659258262890683122, 1.000000000000000000, 0.9659258262890683122, 1.000000000000000000, 0.9659258262890683122, 1.000000000000000000, 0.9659258262890683122, 1.000000000000000000, 0.9659258262890683122, 1.000000000000000000, 0.9659258262890683122, 1.000000000000000000, 0.9659258262890683122, 1.000000000000000000, 0.9659258262890683122, 1.000000000000000000, 0.9659258262890683122, 1.000000000000000000, 0.9659258262890683122, 1.000000000000000000, 0.9659258262890683122, 1.000000000000000000, 0.9659258262890683122, 1.000000000000000000, 0.9659258262890683122, 1.000000000000000000, 0.9659258262890683122, 1.000000000000000000, 0.9659258262890683122, 1.000000000000000000, 0.9659258262890683122, 1.000000000000000000, 0.9659258262890683122, 1.000000000000000000, 0.9659258262890683122, 1.000000000000000000, 0.9659258262890683122, 1.000000000000000000, 0.9659258262890683122, 1.000000000000000000, 0.9659258262890683122, 1.000000000000000000, 0.9659258262890683122, 1.000000000000000000, 0.9659258262890683122, 1.000000000000000000, 0.9659258262890683122, 1.000000000000000000, 0.9659258262890683122, 1.000000000000000000, 0.9659258262890683122, 1.000000000000000000, 0.9659258262890683122, 1.000000000000000000, 0.9659258262890683122, 1.000000000000000000, 0.9659258262890683122, 1.000000000000000000, 0.9659258262890683122, 1.000000000000000000, 0.9659258262890683122, 1.000000000000000000, 0.9659258262890683122, 1.000000000000000000, 0.9659258262890683122, 1.000000000000000000, 0.9659258262890683122, 1.000000000000000000, 0.9659258262890683122, 1.000000000000000000, 0.9659258262890683122, 1.000000000000000000, 0.9659258262890683122, 1.000000000000000000, 0.9659258262890683122, 1.000000000000000000, 0.9659258262890683122, 1.000000000000000000, 0.9659258262890683122, 1.000000000000000000, 0.9659258262890683122, 1.000000000000000000, 0.9659258262890683122, 1.000000000000000000, 0.9659258262890683122, 1.000000000000000000, 0.9659258262890683122, 1.000000000000000000, 0.9659258262890683122, 1.000000000000000000, 0.9659258262890683122, 1.000000000000000000, 0.9659258262890683122, 1.000000000000000000, 0.9659258262890683122, 1.000000000000000000, 0.9659258262890683122, 1.000000000000000000, 0.9659258262890683122, 1.000000000000000000, 0.9659258262890683122, 1.000000000000000000, 0.9659258262890683122, 1.000000000000000000, 0.9659258262890683122, 1.000000000000000000, 0.9659258262890683122, 1.000000000000000000, 0.9659258262890683122, 1.000000000000000000, 0.9659258262890683122, 1.000000000000000000, 0.9659258262890683122, 1.000000000000000000, 0.9659258262890683122, 1.000000000000000000, 0.9659258262890683122, 1.000000000000000000, 0.9659258262890683122, 1.000000000000000000, 0.9659258262890683122, 1.000000000000000000, 0.9659258262890683122, 1.000000000000000000, 0.9659258262890683122, 1.000000000000000000, 0.9659258262890683122, 1.000000000000000000, 0.9659258262890683122, 1.000000000000000000, 0.9659258262890683122, 1.000000000000000000, 0.9659258262890683122, 1.000000000000000000, 0.9659258262890683122, 1.000000000000000000, 0.9659258262890683122, 1.000000000000000000, 0.9659258262890683122, 1.000000000000000000, 0.9659258262890683122, 1.000000000000000000, 0.9659258262890683122, 1.000000000000000000, 0.9659258262890683122, 1.000000000000000000, 0.9659258262890683122, 1.000000000000000000, 0.9659258262890683122, 1.000000000000000000, 0.9659258262890683122, 1.000000000000000000, 0.9659258262890683122, 1.000000000000000000, 0.9659258262890683122, 1.000000000000000000, 0.9659258262890683122, 1.000000000000000000, 0.9659258262890683122, 1.000000000000000000, 0.9659258262890683122, 1.000000000000000000, 0.9659258262890683122, 1.000000000000000000, 0.9659258262890683122, 1.000000000000000000, 0.9659258262890683122, 1.000000000000000000, 0.9659258262890683122, 1.000000000000000000, 0.9659258262890683122, 1.000000000000000000, 0.9659258262890683122, 1.000000000000000000, 0.9659258262890683122, 1.000000000000000000, 0.9659258262890683122, 1.000000000000000000, 0.9659258262890683122, 1.000000000000000000, 0.9659258262890683122, 1.000000000000000000, 0.9659258262890683122, 1.000000000000000000, 0.9659258262890683122, 1.000000000000000000, 0.9659258262890683122, 1.000000000000000000, 0.9659258262890683122, 1.000000000000000000, 0.9659258262890683122, 1.000000000000000000, 0.9659258262890683122, 1.000000000000000000, 0.9659258262890683122, 1.000000000000000000, 0.9659258262890683122, 1.000000000000000000, 0.9659258262890683122, 1.000000000000000000, 0.9659258262890683122, 1.000000000000000000, 0.9659258262890683122, 1.000000000000000000, 0.9659258262890683122, 1.000000000000000000, 0.9659258262890683122, 1.000000000000000000, 0.9659258262890683122, 1.000000000000000000, 0.9659258262890683122, 1.000000000000000000, 0.9659258262890683122, 1.000000000000000000, 0.9659258262890683122, 1.000000000000000000, 0.9659258262890683122, 1.000000000000000000, 0.9659258262890683122, 1.000000000000000000, 0.9659258262890683122, 1.000000000000000000, 0.9659258262890683122, 1.000000000000000000, 0.9659258262890683122, 1.000000000000000000, 0.9659258262890683122, 1.000000000000000000, 0.9659258262890683122, 1.000000000000000000, 0.9659258262890683122, 1.000000000000000000, 0.9659258262890683122, 1.000000000000000000, 0.9659258262890683122, 1.000000000000000000, 0.9659258262890683122, 1.000000000000000000, 0.9659258262890683122, 1.000000000000000000, 0.9659258262890683122, 1.000000000000000000, 0.9659258262890683122, 1.000000000000000000, 0.9659258262890683122, 1.000000000000000000, 0.9659258262890683122, 1.000000000000000000, 0.9659258262890683122, 1.000000000000000000, 0.9659258262890683122, 1.000000000000000000, 0.9659258262890683122, 1.000000000000000000, 0.9659258262890683122, 1.000000000000000000, 0.9659258262890683122, 1.000000000000000000, 0.9659258262890683122, 1.000000000000000000, 0.9659258262890683122, 1.000000000000000000, 0.9659258262890683122, 1.000000000000000000, 0.9659258262890683122, 1.000000000000000000, 0.9659258262890683122, 1.000000000000000000, 0.9659258262890683122, 1.000000000000000000, 0.9659258262890683122, 1.000000000000000000, 0.9659258262890683122, 1.000000000000000000, 0.9659258262890683122, 1.000000000000000000, 0.9659258262890683122, 1.000000000000000000, 0.9659258262890683122, 1.000000000000000000, 0.9659258262890683122, 1.000000000000000000, 0.9659258262890683122, 1.000000000000000000, 0.9659258262890683122, 1.000000000000000000, 0.9659258262890683122, 1.000000000000000000, 0.9659258262890683122, 1.000000000000000000, 0.9659258262890683122, 1.000000000000000000, 0.9659258262890683122, 1.000000000000000000, 0.9659258262890683122, 1.000000000000000000, 0.9659258262890683122, 1.000000000000000000, 0.9659258262890683122, 1.000000000000000000, 0.9659258262890683122, 1.000000000000000000, 0.9659258262890683122, 1.000000000000000000, 0.9659258262890683122, 1.000000000000000000, 0.9659258262890683122, 1.000000000000000000, 0.9659258262890683122, 1.000000000000000000, 0.9659258262890683122, 1.000000000000000000, 0.9659258262890683122, 1.000000000000000000, 0.9659258262890683122, 1.000000000000000000, 0.9659258262890683122, 1.000000000000000000, 0.9659258262890683122, 1.000000000000000000, 0.9659258262890683122, 1.000000000000000000, 0.9659258262890683122, 1.000000000000000000, 0.9659258262890683122, 1.000000000000000000, 0.9659258262890683122, 1.000000000000000000, 0.9659258262890683122, 1.000000000000000000, 0.9659258262890683122, 1.000000000000000000, 0.9659258262890683122, 1.000000000000000000, 0.9659258262890683122, 1.000000000000000000, 0.9659258262890683122, 1.000000000000000000, 0.9659258262890683122, 1.000000000000000000, 0.9659258262890683122, 1.000000000000000000, 0.9659258262890683122, 1.000000000000000000, 0.9659258262890683122, 1.000000000000000000, 0.9659258262890683122, 1.000000000000000000, 0.9659258262890683122, 1.000000000000000000, 0.9659258262890683122, 1.000000000000000000, 0.9659258262890683122, 1.000000000000000000, 0.9659258262890683122, 1.000000000000000000, 0.9659258262890683122, 1.000000000000000000, 0.9659258262890683122, 1.000000000000000000, 0.9659258262890683122, 1.000000000000000000, 0.9659258262890683122, 1.000000000000000000, 0.9659258262890683122, 1.000000000000000000, 0.9659258262890683122, 1.000000000000000000, 0.9659258262890683122, 1.000000000000000000, 0.9659258262890683122, 1.000000000000000000, 0.9659258262890683122, 1.000000000000000000, 0.9659258262890683122, 1.000000000000000000, 0.9659258262890683122, 1.000000000000000000, 0.9659258262890683122, 1.000000000000000000, 0.9659258262890683122, 1.000000000000000000, 0.9659258262890683122, 1.000000000000000000, 0.9659258262890683122, 1.000000000000000000, 0.9659258262890683122, 1.000000000000000000, 0.9659258262890683122, 1.000000000000000000, 0.9659258262890683122, 1.000000000000000000, 0.9659258262890683122, 1.000000000000000000, 0.9659258262890683122, 1.000000000000000000, 0.9659258262890683122, 1.000000000000000000, 0.9659258262890683122, 1.000000000000000000, 0.9659258262890683122, 1.000000000000000000, 0.9659258262890683122, 1.000000000000000000, 0.9659258262890683122, 1.000000000000000000, 0.9659258262890683122, 1.000000000000000000, 0.9659258262890683122, 1.000000000000000000, 0.9659258262890683122, 1.000000000000000000, 0.9659258262890683122, 1.000000000000000000, 0.9659258262890683122, 1.000000000000000000, 0.9659258262890683122, 1.000000000000000000, 0.9659258262890683122, 1.000000000000000000, 0.9659258262890683122, 1.000000000000000000, 0.9659258262890683122, 1.000000000000000000, 0.9659258262890683122, 1.000000000000000000, 0.9659258262890683122, 1.000000000000000000, 0.9659258262890683122, 1.000000000000000000, 0.9659258262890683122, 1.000000000000000000, 0.9659258262890683122, 1.000000000000000000, 0.9659258262890683122, 1.000000000000000000) ) ) 
 REPRESENTATION_ITEM ( '' )  SURFACE ( )  );
#109549=CARTESIAN_POINT ( 'NONE',  ( -19.05341960407617563, 5.049401038297882671, 83.54275706135233293 ) ) ;
#109550=CARTESIAN_POINT ( 'NONE',  ( 8.224510206698953496, -14.34966873604960469, 87.91557627198103830 ) ) ;
#109551=CARTESIAN_POINT ( 'NONE',  ( 19.05341960407611168, 5.049401038298154454, 48.95724293864768129 ) ) ;
#109552=CARTESIAN_POINT ( 'NONE',  ( -16.51473224551082808, 9.474510206698731452, 93.33442372801900433 ) ) ;
#109553=CARTESIAN_POINT ( 'NONE',  ( 17.49999999999999645, -5.500000000000031974, 93.29690382534172954 ) ) ;
#109554=CARTESIAN_POINT ( 'NONE',  ( 5.823673210054444382, -21.52544592524334988, 85.20942372801901854 ) ) ;
#109555=CARTESIAN_POINT ( 'NONE',  ( -8.314922557961024197, 14.29746914071037800, 57.91775706135234714 ) ) ;
#109556=CARTESIAN_POINT ( 'NONE',  ( 16.88567814943165857, 6.947325034625600360, 38.79001122652587696 ) ) ;
#109557=CARTESIAN_POINT ( 'NONE',  ( 5.823673210054125526, 21.52544592524343514, 44.79057627198103120 ) ) ;
#109558=CARTESIAN_POINT ( 'NONE',  ( 8.314922557961029526, -14.29746914071037800, 40.41775706135234714 ) ) ;
#109559=CARTESIAN_POINT ( 'NONE',  ( -19.02544592524342804, 5.153800228976336939, 26.04057627198103120 ) ) ;
#109560=CARTESIAN_POINT ( 'NONE',  ( 9.474510206698729675, 16.51473224551082808, 32.08442372801900433 ) ) ;
#109561=CARTESIAN_POINT ( 'NONE',  ( -19.02544592524342804, 5.153800228976336051, 71.04057627198099567 ) ) ;
#109563=CARTESIAN_POINT ( 'NONE',  ( -19.02544592524342804, 5.153800228976336051, 56.04057627198100988 ) ) ;
#109565=CARTESIAN_POINT ( 'NONE',  ( -9.474510206698964154, 16.51473224551069663, 65.41557627198102409 ) ) ;
#109566=CARTESIAN_POINT ( 'NONE',  ( -18.22780087662126647, -5.499999999999827693, 53.98236817873107185 ) ) ;
#109567=CARTESIAN_POINT ( 'NONE',  ( -13.97604488694547697, 13.89961937509957934, 28.12609039468565797 ) ) ;
#109568=CARTESIAN_POINT ( 'NONE',  ( -18.67979575497193778, 10.72451020669871902, 113.3344237280190328 ) ) ;
#109569=CARTESIAN_POINT ( 'NONE',  ( 8.224510206698953496, -14.34966873604960469, 32.91557627198102409 ) ) ;
#109570=CARTESIAN_POINT ( 'NONE',  ( -13.97604488694527625, -13.89961937509977652, 41.87390960531435979 ) ) ;
#109571=CARTESIAN_POINT ( 'NONE',  ( -5.153800228976328057, -19.02544592524343514, 102.2905762719810383 ) ) ;
#109572=CARTESIAN_POINT ( 'NONE',  ( 21.53943276465977519, 0.05219959533937863772, 76.25109039468568994 ) ) ;
#109573=CARTESIAN_POINT ( 'NONE',  ( -13.97604488694527625, -13.89961937509977652, 51.87390960531436690 ) ) ;
#109574=CARTESIAN_POINT ( 'NONE',  ( 0.05219959533937995610, -21.53943276465977519, 80.00109039468568994 ) ) ;
#109575=CARTESIAN_POINT ( 'NONE',  ( -19.02544592524342804, 5.153800228976336051, 116.0405762719810383 ) ) ;
#109576=CARTESIAN_POINT ( 'NONE',  ( 5.049401038298161559, -19.05341960407611168, 32.70724293864768129 ) ) ;
#109577=CARTESIAN_POINT ( 'NONE',  ( 18.62759615963255655, 10.81492255796105972, 31.66775706135234358 ) ) ;
#109578=CARTESIAN_POINT ( 'NONE',  ( 13.89961937509957401, 13.97604488694547697, 46.87609039468565442 ) ) ;
#109579=CARTESIAN_POINT ( 'NONE',  ( -9.474510206698964154, 16.51473224551069663, 30.41557627198102054 ) ) ;
#109580=CARTESIAN_POINT ( 'NONE',  ( 16.46253265017160672, -9.564922557960803928, 78.33224293864769550 ) ) ;
#109581=CARTESIAN_POINT ( 'NONE',  ( -13.97604488694547697, 13.89961937509957934, 108.1260903946856331 ) ) ;
#109582=CARTESIAN_POINT ( 'NONE',  ( -16.53943276465976808, 0.05219959533911058130, 76.24890960531435269 ) ) ;
#109583=CARTESIAN_POINT ( 'NONE',  ( 21.53943276465977519, -0.05219959533907433946, 33.74890960531436690 ) ) ;
#109584=CARTESIAN_POINT ( 'NONE',  ( 16.46253265017146816, 9.564922557961045513, 101.6677570613523329 ) ) ;
#109585=CARTESIAN_POINT ( 'NONE',  ( 15.72974639402199770, -15.80617190586745480, 108.1239096053143811 ) ) ;
#109586=CARTESIAN_POINT ( 'NONE',  ( -21.52544592524334988, -5.823673210054445271, 58.95942372801902565 ) ) ;
#109587=CARTESIAN_POINT ( 'NONE',  ( 16.53943276465976808, 0.05219959533934440121, 51.25109039468568994 ) ) ;
#109588=CARTESIAN_POINT ( 'NONE',  ( 16.55341960407618274, -4.379528057220086978, 56.04275706135235424 ) ) ;
#109589=CARTESIAN_POINT ( 'NONE',  ( -15.72974639402197994, 15.80617190586746368, 65.62390960531436690 ) ) ;
#109590=CARTESIAN_POINT ( 'NONE',  ( -16.51473224551069308, -9.474510206698971260, 46.66557627198102409 ) ) ;
#109591=CARTESIAN_POINT ( 'NONE',  ( -12.14591786802326823, 12.06949235617739902, 83.12609039468568994 ) ) ;
#109592=CARTESIAN_POINT ( 'NONE',  ( -0.05219959533907301413, -21.53943276465977519, 97.49890960531436690 ) ) ;
#109593=CARTESIAN_POINT ( 'NONE',  ( -14.34966873604960291, -8.224510206698953496, 46.66557627198102409 ) ) ;
#109594=CARTESIAN_POINT ( 'NONE',  ( -19.05341960407611168, -5.049401038298163336, 71.45724293864766707 ) ) ;
#109595=CARTESIAN_POINT ( 'NONE',  ( -16.55341960407617563, 4.379528057220093196, 78.54275706135236135 ) ) ;
#109596=CARTESIAN_POINT ( 'NONE',  ( 16.53943276465976808, 0.05219959533934440121, 21.25109039468567218 ) ) ;
#109597=CARTESIAN_POINT ( 'NONE',  ( 21.53943276465977519, -0.05219959533907433946, 113.7489096053143527 ) ) ;
#109598=CARTESIAN_POINT ( 'NONE',  ( 12.06949235617757843, -12.14591786802309237, 43.12390960531435269 ) ) ;
#109600=CARTESIAN_POINT ( 'NONE',  ( -17.31728774477273447, 6.344390552232393787, 75.81906651689320142 ) ) ;
#109601=CARTESIAN_POINT ( 'NONE',  ( -5.823673210054116645, -21.52544592524344225, 82.29057627198103830 ) ) ;
#109602=CARTESIAN_POINT ( 'NONE',  ( 16.52544592524342804, -4.483927247898539470, 28.54057627198103120 ) ) ;
#109604=CARTESIAN_POINT ( 'NONE',  ( -16.29526858892878849, -7.335722546920003140, 55.79670597800208753 ) ) ;
#109605=CARTESIAN_POINT ( 'NONE',  ( -21.53943276465977519, 0.05219959533907696930, 111.2489096053143669 ) ) ;
#109606=CARTESIAN_POINT ( 'NONE',  ( 13.89961937509977652, -13.97604488694527269, 108.1239096053143669 ) ) ;
#109607=CARTESIAN_POINT ( 'NONE',  ( -21.53943276465977519, -0.05219959533937600094, 23.75109039468567929 ) ) ;
#109608=CARTESIAN_POINT ( 'NONE',  ( 14.34966873604960469, 8.224510206698951720, 49.16557627198102409 ) ) ;
#109609=CARTESIAN_POINT ( 'NONE',  ( -16.55341960407617563, 4.379528057220093196, 48.54275706135234714 ) ) ;
#109610=CARTESIAN_POINT ( 'NONE',  ( 19.02544592524343514, -5.153800228976328945, 58.54057627198102409 ) ) ;
#109612=CARTESIAN_POINT ( 'NONE',  ( 13.97604488694548053, -13.89961937509957401, 50.62609039468566152 ) ) ;
#109613=CARTESIAN_POINT ( 'NONE',  ( -5.153800228976328057, -19.02544592524343514, 82.29057627198103830 ) ) ;
#109614=CARTESIAN_POINT ( 'NONE',  ( 21.55341960407610458, 5.719274019375980345, 33.95724293864769550 ) ) ;
#109616=CARTESIAN_POINT ( 'NONE',  ( -5.153800228976328057, -19.02544592524343514, 42.29057627198101699 ) ) ;
#109617=CARTESIAN_POINT ( 'NONE',  ( -4.379528057220086978, -16.55341960407618274, 24.79275706135235779 ) ) ;
#109618=CARTESIAN_POINT ( 'NONE',  ( -16.46253265017146816, -9.564922557961047289, 64.16775706135233293 ) ) ;
#109619=CARTESIAN_POINT ( 'NONE',  ( 10.72451020669898902, -18.67979575497178502, 97.91557627198103830 ) ) ;
#109620=CARTESIAN_POINT ( 'NONE',  ( -14.29746914071049879, 8.314922557960819915, 30.83224293864770260 ) ) ;
#109621=CARTESIAN_POINT ( 'NONE',  ( -19.05341960407611168, -5.049401038298163336, 91.45724293864766707 ) ) ;
#109622=CARTESIAN_POINT ( 'NONE',  ( 15.72974639402199770, -15.80617190586745480, 53.12390960531436690 ) ) ;
#109623=CARTESIAN_POINT ( 'NONE',  ( 18.62759615963271287, -10.81492255796078972, 98.33224293864769550 ) ) ;
#109624=CARTESIAN_POINT ( 'NONE',  ( -12.06949235617739369, -12.14591786802326823, 24.37609039468567573 ) ) ;
#109625=CARTESIAN_POINT ( 'NONE',  ( 15.80617190586746368, 15.72974639402197994, 39.37390960531436690 ) ) ;
#109626=CARTESIAN_POINT ( 'NONE',  ( -21.53943276465977519, -0.05219959533937600094, 83.75109039468568994 ) ) ;
#109627=CARTESIAN_POINT ( 'NONE',  ( -13.89961937509977652, 13.97604488694528158, 85.62390960531433848 ) ) ;
#109629=CARTESIAN_POINT ( 'NONE',  ( 16.46253265017160672, -9.564922557960803928, 33.33224293864770260 ) ) ;
#109630=CARTESIAN_POINT ( 'NONE',  ( -9.474510206698964154, 16.51473224551069663, 90.41557627198103830 ) ) ;
#109631=CARTESIAN_POINT ( 'NONE',  ( 12.06949235617757843, -12.14591786802309237, 98.12390960531436690 ) ) ;
#109632=CARTESIAN_POINT ( 'NONE',  ( -19.03943276465977164, 0.05219959533909376836, 66.24890960531436690 ) ) ;
#109633=CARTESIAN_POINT ( 'NONE',  ( 14.29746914071037800, 8.314922557961029526, 21.66775706135235069 ) ) ;
#109634=CARTESIAN_POINT ( 'NONE',  ( -18.22780087662122028, 5.500000000000031086, 43.51540105326107977 ) ) ;
#109635=CARTESIAN_POINT ( 'NONE',  ( -15.72974639402176322, -15.80617190586768395, 99.37609039468568994 ) ) ;
#109636=CARTESIAN_POINT ( 'NONE',  ( 10.72451020669898902, -18.67979575497178502, 22.91557627198102765 ) ) ;
#109637=CARTESIAN_POINT ( 'NONE',  ( 16.53943276465976808, 0.05219959533934440121, 91.25109039468568994 ) ) ;
#109639=CARTESIAN_POINT ( 'NONE',  ( -9.564922557961040184, 16.46253265017147172, 72.91775706135233293 ) ) ;
#109640=CARTESIAN_POINT ( 'NONE',  ( -9.564922557961040184, 16.46253265017147172, 32.91775706135233293 ) ) ;
#109642=CARTESIAN_POINT ( 'NONE',  ( 16.46253265017160672, -9.564922557960803928, 23.33224293864769194 ) ) ;
#109643=CARTESIAN_POINT ( 'NONE',  ( -12.06949235617756955, 12.14591786802309770, 35.62390960531437401 ) ) ;
#109645=CARTESIAN_POINT ( 'NONE',  ( 5.049401038298161559, -19.05341960407611168, 27.70724293864769550 ) ) ;
#109646=CARTESIAN_POINT ( 'NONE',  ( -0.05219959533910754901, -16.53943276465976808, 27.49890960531435269 ) ) ;
#109647=CARTESIAN_POINT ( 'NONE',  ( -18.56399227203343472, -5.499999999999928946, 83.97830131249904184 ) ) ;
#109648=CARTESIAN_POINT ( 'NONE',  ( 12.14591786802327356, -12.06949235617739191, 95.62609039468568994 ) ) ;
#109649=CARTESIAN_POINT ( 'NONE',  ( 9.564922557960805705, 16.46253265017160317, 34.58224293864770260 ) ) ;
#109650=CARTESIAN_POINT ( 'NONE',  ( -21.53943276465977519, -0.05219959533937600094, 88.75109039468567573 ) ) ;
#109651=CARTESIAN_POINT ( 'NONE',  ( -19.02544592524334988, -5.153800228976617603, 103.9594237280190043 ) ) ;
#109652=CARTESIAN_POINT ( 'NONE',  ( 10.72451020669871369, 18.67979575497193778, 82.08442372801901854 ) ) ;
#109653=CARTESIAN_POINT ( 'NONE',  ( 19.05341960407617918, -5.049401038297876454, 56.04275706135234714 ) ) ;
#109654=CARTESIAN_POINT ( 'NONE',  ( 19.02544592524343514, -5.153800228976328945, 93.54057627198102409 ) ) ;
#109655=CARTESIAN_POINT ( 'NONE',  ( -16.46253265017160317, 9.564922557960807481, 70.83224293864770971 ) ) ;
#109656=EDGE_CURVE ( 'NONE', #63455, #132514, #131391, .T. ) ;
#109657=CARTESIAN_POINT ( 'NONE',  ( 16.79531203550646623, 7.028104445595625194, 73.75244988220441655 ) ) ;
#109659=CARTESIAN_POINT ( 'NONE',  ( 14.29746914071049879, -8.314922557960816363, 68.33224293864769550 ) ) ;
#109660=CARTESIAN_POINT ( 'NONE',  ( -21.52544592524343514, 5.823673210054127303, 61.04057627198103120 ) ) ;
#109661=CARTESIAN_POINT ( 'NONE',  ( -5.153800228976328057, -19.02544592524343514, 57.29057627198103120 ) ) ;
#109662=CARTESIAN_POINT ( 'NONE',  ( -15.72974639402197994, 15.80617190586746368, 85.62390960531436690 ) ) ;
#109663=CARTESIAN_POINT ( 'NONE',  ( 14.34966873604972726, -8.224510206698740333, 80.83442372801901854 ) ) ;
#109664=VERTEX_POINT ( 'NONE', #5298 ) ;
#109665=CARTESIAN_POINT ( 'NONE',  ( -13.97604488694527625, -13.89961937509977652, 46.87390960531435979 ) ) ;
#109666=CARTESIAN_POINT ( 'NONE',  ( 14.34966873604960469, 8.224510206698951720, 74.16557627198102409 ) ) ;
#109668=CARTESIAN_POINT ( 'NONE',  ( -19.05341960407611168, -5.049401038298163336, 46.45724293864768129 ) ) ;
#109669=CARTESIAN_POINT ( 'NONE',  ( -4.379528057220328563, 16.55341960407611168, 110.2072429386477239 ) ) ;
#109670=CARTESIAN_POINT ( 'NONE',  ( -13.97604488694547697, 13.89961937509957934, 68.12609039468563310 ) ) ;
#109671=CARTESIAN_POINT ( 'NONE',  ( -16.52544592524342804, 4.483927247898546575, 66.04057627198103830 ) ) ;
#109672=CARTESIAN_POINT ( 'NONE',  ( -18.62759615963255300, -10.81492255796106328, 39.16775706135235424 ) ) ;
#109673=CARTESIAN_POINT ( 'NONE',  ( -19.02544592524342804, 5.153800228976336051, 31.04057627198102409 ) ) ;
#109674=CARTESIAN_POINT ( 'NONE',  ( -15.80617190586745835, -15.72974639402198527, 101.8739096053143811 ) ) ;
#109676=CARTESIAN_POINT ( 'NONE',  ( 14.34966873604960469, 8.224510206698951720, 84.16557627198103830 ) ) ;
#109678=CARTESIAN_POINT ( 'NONE',  ( -13.89961937509977652, 13.97604488694528158, 45.62390960531433848 ) ) ;
#109679=CARTESIAN_POINT ( 'NONE',  ( 17.50000000000000000, 5.499999999999995559, 113.7823096230356583 ) ) ;
#109680=CARTESIAN_POINT ( 'NONE',  ( -19.02544592524334988, -5.153800228976617603, 88.95942372801897591 ) ) ;
#109681=CARTESIAN_POINT ( 'NONE',  ( 5.049401038298161559, -19.05341960407611168, 97.70724293864766707 ) ) ;
#109682=CARTESIAN_POINT ( 'NONE',  ( 15.80617190586769283, -15.72974639402175789, 40.62609039468567573 ) ) ;
#109683=CARTESIAN_POINT ( 'NONE',  ( -16.46253265017160317, 9.564922557960807481, 80.83224293864769550 ) ) ;
#109684=CARTESIAN_POINT ( 'NONE',  ( 0.05219959533936267826, -19.03943276465977164, 70.00109039468566152 ) ) ;
#109685=CARTESIAN_POINT ( 'NONE',  ( -5.153800228976328057, -19.02544592524343514, 47.29057627198102409 ) ) ;
#109686=CARTESIAN_POINT ( 'NONE',  ( 0.05219959533910956823, 16.53943276465976808, 69.99890960531435269 ) ) ;
#109687=CARTESIAN_POINT ( 'NONE',  ( -14.29746914071049879, 8.314922557960819915, 65.83224293864769550 ) ) ;
#109688=CARTESIAN_POINT ( 'NONE',  ( -19.02544592524342804, 5.153800228976336051, 76.04057627198102409 ) ) ;
#109689=CARTESIAN_POINT ( 'NONE',  ( 5.719274019375991003, -21.55341960407610458, 102.7072429386476955 ) ) ;
#109690=CARTESIAN_POINT ( 'NONE',  ( 9.474510206698971260, -16.51473224551069308, 67.91557627198102409 ) ) ;
#109691=CARTESIAN_POINT ( 'NONE',  ( 13.97604488694548053, -13.89961937509957401, 20.62609039468567573 ) ) ;
#109692=CARTESIAN_POINT ( 'NONE',  ( -5.049401038298153566, 19.05341960407611168, 35.20724293864768839 ) ) ;
#109693=CARTESIAN_POINT ( 'NONE',  ( -4.483927247898539470, -16.52544592524342804, 22.29057627198102765 ) ) ;
#109694=CARTESIAN_POINT ( 'NONE',  ( 16.55341960407611168, 4.379528057220329451, 113.9572429386477239 ) ) ;
#109695=CARTESIAN_POINT ( 'NONE',  ( 5.153800228976615827, -19.02544592524334988, 110.2094237280189901 ) ) ;
#109697=CARTESIAN_POINT ( 'NONE',  ( -21.53943276465977519, -0.05219959533937600094, 28.75109039468567929 ) ) ;
#109698=CARTESIAN_POINT ( 'NONE',  ( 5.049401038297881783, 19.05341960407617563, 72.29275706135234714 ) ) ;
#109699=CARTESIAN_POINT ( 'NONE',  ( 12.14591786802327356, -12.06949235617739191, 110.6260903946857042 ) ) ;
#109700=CARTESIAN_POINT ( 'NONE',  ( -0.05219959533907301413, -21.53943276465977519, 77.49890960531433848 ) ) ;
#109701=CARTESIAN_POINT ( 'NONE',  ( -5.719274019375978568, 21.55341960407610458, 25.20724293864769550 ) ) ;
#109702=CARTESIAN_POINT ( 'NONE',  ( -16.55341960407611168, -4.379528057220339221, 51.45724293864770260 ) ) ;
#109703=CARTESIAN_POINT ( 'NONE',  ( 5.153800228976335163, 19.02544592524342804, 24.79057627198102765 ) ) ;
#109704=CARTESIAN_POINT ( 'NONE',  ( 19.02544592524343514, -5.153800228976328945, 43.54057627198103120 ) ) ;
#109705=CARTESIAN_POINT ( 'NONE',  ( 13.97604488694548053, -13.89961937509957401, 30.62609039468566863 ) ) ;
#109706=CARTESIAN_POINT ( 'NONE',  ( -12.14591786802326823, 12.06949235617739902, 83.12609039468568994 ) ) ;
#109707=CARTESIAN_POINT ( 'NONE',  ( -14.29746914071037622, -8.314922557961029526, 59.16775706135234714 ) ) ;
#109708=CARTESIAN_POINT ( 'NONE',  ( 15.72974639402199770, -15.80617190586745480, 23.12390960531436335 ) ) ;
#109709=CARTESIAN_POINT ( 'NONE',  ( 10.72451020669871369, 18.67979575497193778, 112.0844237280190185 ) ) ;
#109710=CARTESIAN_POINT ( 'NONE',  ( -19.02544592524342804, 5.153800228976336051, 81.04057627198103830 ) ) ;
#109711=CARTESIAN_POINT ( 'NONE',  ( 14.34966873604972726, -8.224510206698740333, 60.83442372801901854 ) ) ;
#109712=CARTESIAN_POINT ( 'NONE',  ( -8.314922557960811034, -14.29746914071050412, 107.0822429386476955 ) ) ;
#109713=CARTESIAN_POINT ( 'NONE',  ( 16.52544592524342804, -4.483927247898539470, 23.54057627198102765 ) ) ;
#109715=CARTESIAN_POINT ( 'NONE',  ( 18.67979575497194134, -10.72451020669871369, 65.83442372801900433 ) ) ;
#109716=CARTESIAN_POINT ( 'NONE',  ( 19.03943276465977164, -0.05219959533909143690, 93.74890960531435269 ) ) ;
#109717=CARTESIAN_POINT ( 'NONE',  ( -5.049401038298153566, 19.05341960407611168, 80.20724293864769550 ) ) ;
#109718=CARTESIAN_POINT ( 'NONE',  ( 5.153800228976335163, 19.02544592524342804, 114.7905762719810241 ) ) ;
#109719=CARTESIAN_POINT ( 'NONE',  ( 4.379528057220339221, -16.55341960407611168, 52.70724293864769550 ) ) ;
#109720=CARTESIAN_POINT ( 'NONE',  ( 16.55341960407618274, -4.379528057220086978, 106.0427570613523471 ) ) ;
#109721=CARTESIAN_POINT ( 'NONE',  ( -8.224510206698948167, 14.34966873604960824, 35.41557627198102409 ) ) ;
#109722=CARTESIAN_POINT ( 'NONE',  ( 12.14591786802327356, -12.06949235617739191, 45.62609039468567573 ) ) ;
#109724=CARTESIAN_POINT ( 'NONE',  ( 5.153800228976615827, -19.02544592524334988, 40.20942372801898301 ) ) ;
#109725=CARTESIAN_POINT ( 'NONE',  ( -13.97604488694527625, -13.89961937509977652, 71.87390960531433848 ) ) ;
#109726=CARTESIAN_POINT ( 'NONE',  ( -16.51473224551082808, 9.474510206698731452, 48.33442372801900433 ) ) ;
#109727=CARTESIAN_POINT ( 'NONE',  ( -13.89961937509957401, -13.97604488694547875, 54.37609039468565442 ) ) ;
#109728=CARTESIAN_POINT ( 'NONE',  ( 19.05341960407617918, -5.049401038297876454, 101.0427570613523045 ) ) ;
#109729=CARTESIAN_POINT ( 'NONE',  ( 4.379528057220092307, 16.55341960407617563, 82.29275706135234714 ) ) ;
#109730=CARTESIAN_POINT ( 'NONE',  ( 5.049401038298161559, -19.05341960407611168, 32.70724293864768129 ) ) ;
#109731=CARTESIAN_POINT ( 'NONE',  ( 5.049401038298161559, -19.05341960407611168, 102.7072429386476955 ) ) ;
#109732=CARTESIAN_POINT ( 'NONE',  ( 21.52544592524334988, 5.823673210054432836, 46.45942372801901854 ) ) ;
#109733=CARTESIAN_POINT ( 'NONE',  ( 19.03943276465977164, 0.05219959533936151252, 86.25109039468567573 ) ) ;
#109734=CARTESIAN_POINT ( 'NONE',  ( 17.50000000000013500, -3.292511757969739605, 107.5652027021053527 ) ) ;
#109735=CARTESIAN_POINT ( 'NONE',  ( -9.474510206698964154, 16.51473224551069663, 55.41557627198103120 ) ) ;
#109736=CARTESIAN_POINT ( 'NONE',  ( -5.153800228976328057, -19.02544592524343514, 97.29057627198099567 ) ) ;
#109737=CARTESIAN_POINT ( 'NONE',  ( 8.314922557960818139, 14.29746914071049879, 59.58224293864770260 ) ) ;
#109738=CARTESIAN_POINT ( 'NONE',  ( 9.564922557960805705, 16.46253265017160317, 54.58224293864769550 ) ) ;
#109739=CARTESIAN_POINT ( 'NONE',  ( 5.049401038298161559, -19.05341960407611168, 67.70724293864769550 ) ) ;
#109740=CARTESIAN_POINT ( 'NONE',  ( 5.049401038297881783, 19.05341960407617563, 67.29275706135234714 ) ) ;
#109741=CARTESIAN_POINT ( 'NONE',  ( -0.05219959533936034679, 19.03943276465977164, 47.50109039468566863 ) ) ;
#109742=CARTESIAN_POINT ( 'NONE',  ( -19.05341960407611168, -5.049401038298163336, 81.45724293864769550 ) ) ;
#109743=CARTESIAN_POINT ( 'NONE',  ( 10.81492255796078972, 18.62759615963270932, 74.58224293864768129 ) ) ;
#109744=CARTESIAN_POINT ( 'NONE',  ( 16.52544592524342804, -4.483927247898539470, 73.54057627198102409 ) ) ;
#109745=CARTESIAN_POINT ( 'NONE',  ( -0.05219959533936034679, 19.03943276465977164, 37.50109039468567573 ) ) ;
#109746=CARTESIAN_POINT ( 'NONE',  ( -15.80617190586745835, -15.72974639402198527, 41.87390960531435979 ) ) ;
#109747=CARTESIAN_POINT ( 'NONE',  ( 21.55341960407610458, 5.719274019375980345, 43.95724293864769550 ) ) ;
#109748=CARTESIAN_POINT ( 'NONE',  ( -13.97604488694527625, -13.89961937509977652, 61.87390960531435979 ) ) ;
#109749=CARTESIAN_POINT ( 'NONE',  ( -16.51473224551069308, -9.474510206698971260, 41.66557627198103120 ) ) ;
#109750=CARTESIAN_POINT ( 'NONE',  ( 4.379528057220339221, -16.55341960407611168, 107.7072429386476955 ) ) ;
#109751=CARTESIAN_POINT ( 'NONE',  ( 10.72451020669871369, 18.67979575497193778, 27.08442372801901854 ) ) ;
#109752=CARTESIAN_POINT ( 'NONE',  ( 5.153800228976335163, 19.02544592524342804, 109.7905762719810099 ) ) ;
#109753=CARTESIAN_POINT ( 'NONE',  ( 10.72451020669871369, 18.67979575497193778, 22.08442372801901143 ) ) ;
#109754=CARTESIAN_POINT ( 'NONE',  ( 0.05219959533909260263, 19.03943276465977164, 29.99890960531435979 ) ) ;
#109755=CARTESIAN_POINT ( 'NONE',  ( -10.72451020669898014, 18.67979575497178502, 100.4155762719810241 ) ) ;
#109756=CARTESIAN_POINT ( 'NONE',  ( 19.03943276465977164, 0.05219959533936151252, 51.25109039468567573 ) ) ;
#109757=CARTESIAN_POINT ( 'NONE',  ( -9.564922557960796823, -16.46253265017161027, 22.08224293864768839 ) ) ;
#109758=CARTESIAN_POINT ( 'NONE',  ( -19.02544592524342804, 5.153800228976336051, 26.04057627198103120 ) ) ;
#109760=CARTESIAN_POINT ( 'NONE',  ( 0.05219959533934541429, -16.53943276465976808, 65.00109039468568994 ) ) ;
#109761=CARTESIAN_POINT ( 'NONE',  ( 13.89961937509977652, -13.97604488694527269, 28.12390960531435624 ) ) ;
#109763=CARTESIAN_POINT ( 'NONE',  ( -13.89961937509977652, 13.97604488694528158, 75.62390960531438111 ) ) ;
#109764=CARTESIAN_POINT ( 'NONE',  ( -4.483927247898539470, -16.52544592524342804, 107.2905762719810525 ) ) ;
#109765=CARTESIAN_POINT ( 'NONE',  ( -10.81492255796078084, -18.62759615963271287, 42.08224293864769550 ) ) ;
#109766=CARTESIAN_POINT ( 'NONE',  ( 4.379528057220339221, -16.55341960407611168, 72.70724293864769550 ) ) ;
#109767=CARTESIAN_POINT ( 'NONE',  ( -0.05219959533934338120, 16.53943276465976808, 27.50109039468567929 ) ) ;
#109768=CARTESIAN_POINT ( 'NONE',  ( 5.719274019375673035, 21.55341960407619339, 82.29275706135234714 ) ) ;
#109769=CARTESIAN_POINT ( 'NONE',  ( -13.97604488694527625, -13.89961937509977652, 26.87390960531434558 ) ) ;
#109770=CARTESIAN_POINT ( 'NONE',  ( 12.14591786802327356, -12.06949235617739191, 110.6260903946857042 ) ) ;
#109771=CARTESIAN_POINT ( 'NONE',  ( -4.379528057220328563, 16.55341960407611168, 55.20724293864770260 ) ) ;
#109773=CARTESIAN_POINT ( 'NONE',  ( 19.02544592524343514, -5.153800228976328945, 58.54057627198102409 ) ) ;
#109774=CARTESIAN_POINT ( 'NONE',  ( 10.72451020669871369, 18.67979575497193778, 92.08442372801901854 ) ) ;
#109775=CARTESIAN_POINT ( 'NONE',  ( 10.81492255796078972, 18.62759615963270932, 109.5822429386476955 ) ) ;
#109776=CARTESIAN_POINT ( 'NONE',  ( -18.67979575497193778, 10.72451020669871902, 78.33442372801901854 ) ) ;
#109777=CARTESIAN_POINT ( 'NONE',  ( -16.53943276465976808, -0.05219959533934237506, 43.75109039468568284 ) ) ;
#109778=CARTESIAN_POINT ( 'NONE',  ( 14.29746914071049879, -8.314922557960816363, 83.33224293864769550 ) ) ;
#109779=CARTESIAN_POINT ( 'NONE',  ( 18.62759615963255655, 10.81492255796105972, 81.66775706135236135 ) ) ;
#109780=CARTESIAN_POINT ( 'NONE',  ( -12.06949235617739369, -12.14591786802326823, 109.3760903946857042 ) ) ;
#109781=CARTESIAN_POINT ( 'NONE',  ( -17.26172910966779739, 6.454744622555818268, 115.8064690864922710 ) ) ;
#109782=CARTESIAN_POINT ( 'NONE',  ( 4.379528057220092307, 16.55341960407617563, 42.29275706135235424 ) ) ;
#109783=CARTESIAN_POINT ( 'NONE',  ( -14.34966873604960291, -8.224510206698953496, 46.66557627198102409 ) ) ;
#109784=CARTESIAN_POINT ( 'NONE',  ( 8.224510206698742110, 14.34966873604972548, 87.08442372801901854 ) ) ;
#109785=CARTESIAN_POINT ( 'NONE',  ( 19.03943276465977164, -0.05219959533909143690, 103.7489096053143669 ) ) ;
#109786=CARTESIAN_POINT ( 'NONE',  ( 5.153800228976335163, 19.02544592524342804, 99.79057627198102409 ) ) ;
#109787=CARTESIAN_POINT ( 'NONE',  ( -5.719274019375665041, -21.55341960407619695, 94.79275706135234714 ) ) ;
#109788=CARTESIAN_POINT ( 'NONE',  ( -14.34966873604972548, 8.224510206698743886, 103.3344237280190043 ) ) ;
#109789=CARTESIAN_POINT ( 'NONE',  ( -16.53943276465976808, 0.05219959533911058130, 76.24890960531435269 ) ) ;
#109790=CARTESIAN_POINT ( 'NONE',  ( 19.03943276465977164, -0.05219959533909143690, 78.74890960531436690 ) ) ;
#109792=CARTESIAN_POINT ( 'NONE',  ( 14.34966873604972726, -8.224510206698740333, 20.83442372801901143 ) ) ;
#109793=CARTESIAN_POINT ( 'NONE',  ( -5.049401038298153566, 19.05341960407611168, 30.20724293864768839 ) ) ;
#109794=CARTESIAN_POINT ( 'NONE',  ( 9.474510206698971260, -16.51473224551069308, 97.91557627198102409 ) ) ;
#109795=CARTESIAN_POINT ( 'NONE',  ( 14.34966873604972726, -8.224510206698740333, 35.83442372801901143 ) ) ;
#109796=CARTESIAN_POINT ( 'NONE',  ( 17.50000000000000000, 5.499999999999997335, 106.7030961746582847 ) ) ;
#109797=CARTESIAN_POINT ( 'NONE',  ( 19.05341960407617918, -5.049401038297876454, 36.04275706135234003 ) ) ;
#109798=CARTESIAN_POINT ( 'NONE',  ( -16.53943276465976808, -0.05219959533934237506, 93.75109039468567573 ) ) ;
#109799=CARTESIAN_POINT ( 'NONE',  ( 5.049401038297881783, 19.05341960407617563, 107.2927570613523187 ) ) ;
#109800=CARTESIAN_POINT ( 'NONE',  ( -19.02544592524342804, 5.153800228976336051, 36.04057627198100988 ) ) ;
#109801=CARTESIAN_POINT ( 'NONE',  ( 0.05219959533934541429, -16.53943276465976808, 80.00109039468568994 ) ) ;
#109802=CARTESIAN_POINT ( 'NONE',  ( -14.34966873604972548, 8.224510206698743886, 68.33442372801900433 ) ) ;
#109803=CARTESIAN_POINT ( 'NONE',  ( -19.05341960407611168, -5.049401038298163336, 36.45724293864766707 ) ) ;
#109804=CARTESIAN_POINT ( 'NONE',  ( 13.89961937509957401, 13.97604488694547697, 71.87609039468567573 ) ) ;
#109805=CARTESIAN_POINT ( 'NONE',  ( 19.05341960407617918, -5.049401038297876454, 21.04275706135232582 ) ) ;
#109806=CARTESIAN_POINT ( 'NONE',  ( -16.46253265017160317, 9.564922557960807481, 50.83224293864770260 ) ) ;
#109807=CARTESIAN_POINT ( 'NONE',  ( 13.97604488694527802, 13.89961937509977652, 94.37390960531436690 ) ) ;
#109808=CARTESIAN_POINT ( 'NONE',  ( 12.06949235617757843, -12.14591786802309237, 83.12390960531436690 ) ) ;
#109810=CARTESIAN_POINT ( 'NONE',  ( -19.03943276465977164, -0.05219959533935918106, 48.75109039468566863 ) ) ;
#109811=CARTESIAN_POINT ( 'NONE',  ( -21.52544592524343514, 5.823673210054127303, 51.04057627198103120 ) ) ;
#109812=CARTESIAN_POINT ( 'NONE',  ( -18.62759615963255300, -10.81492255796106328, 104.1677570613523471 ) ) ;
#109813=CARTESIAN_POINT ( 'NONE',  ( 5.153800228976335163, 19.02544592524342804, 84.79057627198099567 ) ) ;
#109814=CARTESIAN_POINT ( 'NONE',  ( -16.46253265017146816, -9.564922557961047289, 19.16775706135233293 ) ) ;
#109815=CARTESIAN_POINT ( 'NONE',  ( 21.52544592524344225, -5.823673210054117533, 68.54057627198103830 ) ) ;
#109816=CARTESIAN_POINT ( 'NONE',  ( -16.51473224551069308, -9.474510206698971260, 111.6655762719810383 ) ) ;
#109817=CARTESIAN_POINT ( 'NONE',  ( 13.89961937509957401, 13.97604488694547697, 86.87609039468567573 ) ) ;
#109818=CARTESIAN_POINT ( 'NONE',  ( -9.474510206698964154, 16.51473224551069663, 115.4155762719810241 ) ) ;
#109819=CARTESIAN_POINT ( 'NONE',  ( -13.89961937509957401, -13.97604488694547875, 109.3760903946856331 ) ) ;
#109820=CARTESIAN_POINT ( 'NONE',  ( -5.153800228976328057, -19.02544592524343514, 22.29057627198102765 ) ) ;
#109821=CARTESIAN_POINT ( 'NONE',  ( 5.049401038298161559, -19.05341960407611168, 102.7072429386476955 ) ) ;
#109822=CARTESIAN_POINT ( 'NONE',  ( 10.81492255796078972, 18.62759615963270932, 79.58224293864769550 ) ) ;
#109823=CARTESIAN_POINT ( 'NONE',  ( 8.224510206698742110, 14.34966873604972548, 42.08442372801901854 ) ) ;
#109824=CARTESIAN_POINT ( 'NONE',  ( 15.80617190586769283, -15.72974639402175789, 45.62609039468567573 ) ) ;
#109825=CARTESIAN_POINT ( 'NONE',  ( -18.67979575497193778, 10.72451020669871902, 98.33442372801901854 ) ) ;
#109826=CARTESIAN_POINT ( 'NONE',  ( -0.05219959533934338120, 16.53943276465976808, 92.50109039468567573 ) ) ;
#109827=CARTESIAN_POINT ( 'NONE',  ( 19.02544592524343514, -5.153800228976328945, 88.54057627198102409 ) ) ;
#109828=CARTESIAN_POINT ( 'NONE',  ( 4.379528057220339221, -16.55341960407611168, 87.70724293864769550 ) ) ;
#109829=CARTESIAN_POINT ( 'NONE',  ( 4.483927247898545687, 16.52544592524342804, 39.79057627198103830 ) ) ;
#109830=CARTESIAN_POINT ( 'NONE',  ( 5.153800228976615827, -19.02544592524334988, 65.20942372801900433 ) ) ;
#109831=CARTESIAN_POINT ( 'NONE',  ( 21.52544592524334988, 5.823673210054432836, 51.45942372801901854 ) ) ;
#109832=CARTESIAN_POINT ( 'NONE',  ( 16.51473224551083163, -9.474510206698727899, 20.83442372801899722 ) ) ;
#109833=CARTESIAN_POINT ( 'NONE',  ( 4.483927247898545687, 16.52544592524342804, 89.79057627198103830 ) ) ;
#109834=CARTESIAN_POINT ( 'NONE',  ( -5.823673210054116645, -21.52544592524344225, 32.29057627198102409 ) ) ;
#109835=CARTESIAN_POINT ( 'NONE',  ( 14.34966873604972726, -8.224510206698740333, 110.8344237280190043 ) ) ;
#109836=CARTESIAN_POINT ( 'NONE',  ( 10.81492255796106328, -18.62759615963255655, 85.41775706135236135 ) ) ;
#109837=CARTESIAN_POINT ( 'NONE',  ( 16.55341960407618274, -4.379528057220086978, 61.04275706135234714 ) ) ;
#109838=CARTESIAN_POINT ( 'NONE',  ( -4.483927247898782831, 16.52544592524335698, 107.7094237280190328 ) ) ;
#109839=CARTESIAN_POINT ( 'NONE',  ( 5.823673210054444382, -21.52544592524334988, 55.20942372801902565 ) ) ;
#109840=CARTESIAN_POINT ( 'NONE',  ( 15.72974639402176855, 15.80617190586768217, 26.87609039468567218 ) ) ;
#109841=CARTESIAN_POINT ( 'NONE',  ( 0.05219959533910956823, 16.53943276465976808, 99.99890960531436690 ) ) ;
#109842=CARTESIAN_POINT ( 'NONE',  ( -0.05219959533909027116, -19.03943276465977164, 27.49890960531435624 ) ) ;
#109843=CARTESIAN_POINT ( 'NONE',  ( -16.52544592524342804, 4.483927247898546575, 71.04057627198103830 ) ) ;
#109844=CARTESIAN_POINT ( 'NONE',  ( -0.05219959533909027116, -19.03943276465977164, 67.49890960531436690 ) ) ;
#109845=CARTESIAN_POINT ( 'NONE',  ( 8.224510206698742110, 14.34966873604972548, 107.0844237280190043 ) ) ;
#109846=CARTESIAN_POINT ( 'NONE',  ( -10.81492255796078084, -18.62759615963271287, 62.08224293864769550 ) ) ;
#109847=CARTESIAN_POINT ( 'NONE',  ( 16.55341960407611168, 4.379528057220329451, 93.95724293864770971 ) ) ;
#109848=CARTESIAN_POINT ( 'NONE',  ( -15.80617190586745835, -15.72974639402198527, 96.87390960531436690 ) ) ;
#109849=CARTESIAN_POINT ( 'NONE',  ( -19.05341960407611168, -5.049401038298163336, 96.45724293864769550 ) ) ;
#109850=CARTESIAN_POINT ( 'NONE',  ( -9.474510206698964154, 16.51473224551069663, 50.41557627198102409 ) ) ;
#109851=CARTESIAN_POINT ( 'NONE',  ( -5.049401038297874678, -19.05341960407617918, 104.7927570613523471 ) ) ;
#109852=CARTESIAN_POINT ( 'NONE',  ( 15.72974639402199770, -15.80617190586745480, 38.12390960531436690 ) ) ;
#109853=CARTESIAN_POINT ( 'NONE',  ( 18.62759615963255655, 10.81492255796105972, 66.66775706135234714 ) ) ;
#109854=CARTESIAN_POINT ( 'NONE',  ( -13.97604488694527625, -13.89961937509977652, 61.87390960531435979 ) ) ;
#109855=CARTESIAN_POINT ( 'NONE',  ( -5.049401038298153566, 19.05341960407611168, 95.20724293864770971 ) ) ;
#109856=CARTESIAN_POINT ( 'NONE',  ( -0.05219959533934338120, 16.53943276465976808, 57.50109039468568994 ) ) ;
#109857=CARTESIAN_POINT ( 'NONE',  ( -5.719274019375665041, -21.55341960407619695, 49.79275706135234714 ) ) ;
#109858=CARTESIAN_POINT ( 'NONE',  ( -10.81492255796105439, 18.62759615963255655, 92.91775706135236135 ) ) ;
#109859=CARTESIAN_POINT ( 'NONE',  ( -15.72974639402197994, 15.80617190586746368, 105.6239096053143669 ) ) ;
#109860=CARTESIAN_POINT ( 'NONE',  ( -18.62759615963255300, -10.81492255796106328, 34.16775706135234714 ) ) ;
#109861=CARTESIAN_POINT ( 'NONE',  ( 16.55341960407618274, -4.379528057220086978, 81.04275706135236135 ) ) ;
#109862=CARTESIAN_POINT ( 'NONE',  ( 15.80617190586746368, 15.72974639402197994, 74.37390960531436690 ) ) ;
#109863=CARTESIAN_POINT ( 'NONE',  ( -16.51473224551082808, 9.474510206698731452, 28.33442372801900433 ) ) ;
#109864=CARTESIAN_POINT ( 'NONE',  ( 9.474510206698971260, -16.51473224551069308, 72.91557627198102409 ) ) ;
#109865=CARTESIAN_POINT ( 'NONE',  ( 16.52544592524342804, -4.483927247898539470, 28.54057627198103120 ) ) ;
#109867=CARTESIAN_POINT ( 'NONE',  ( -5.153800228976328057, -19.02544592524343514, 97.29057627198099567 ) ) ;
#109869=CARTESIAN_POINT ( 'NONE',  ( -0.05219959533936034679, 19.03943276465977164, 77.50109039468566152 ) ) ;
#109870=CARTESIAN_POINT ( 'NONE',  ( 18.67979575497178502, 10.72451020669898547, 64.16557627198102409 ) ) ;
#109871=CARTESIAN_POINT ( 'NONE',  ( 14.29746914071049879, -8.314922557960816363, 38.33224293864768839 ) ) ;
#109872=CARTESIAN_POINT ( 'NONE',  ( 9.474510206698729675, 16.51473224551082808, 112.0844237280190043 ) ) ;
#109873=CARTESIAN_POINT ( 'NONE',  ( -16.51473224551069308, -9.474510206698971260, 36.66557627198102409 ) ) ;
#109874=CARTESIAN_POINT ( 'NONE',  ( -19.02544592524334988, -5.153800228976617603, 103.9594237280190043 ) ) ;
#109875=CARTESIAN_POINT ( 'NONE',  ( 21.53943276465977519, -0.05219959533907433946, 103.7489096053143669 ) ) ;
#109876=CARTESIAN_POINT ( 'NONE',  ( -13.89961937509957401, -13.97604488694547875, 74.37609039468566152 ) ) ;
#109877=CARTESIAN_POINT ( 'NONE',  ( 14.29746914071037800, 8.314922557961029526, 86.66775706135234714 ) ) ;
#109878=CARTESIAN_POINT ( 'NONE',  ( -9.564922557960796823, -16.46253265017161027, 62.08224293864769550 ) ) ;
#109879=CARTESIAN_POINT ( 'NONE',  ( -8.224510206698948167, 14.34966873604960824, 70.41557627198102409 ) ) ;
#109880=EDGE_CURVE ( 'NONE', #125647, #96182, #139448, .T. ) ;
#109881=CARTESIAN_POINT ( 'NONE',  ( -19.03943276465977164, 0.05219959533909376836, 56.24890960531435979 ) ) ;
#109882=CARTESIAN_POINT ( 'NONE',  ( -4.483927247898539470, -16.52544592524342804, 62.29057627198102409 ) ) ;
#109883=CARTESIAN_POINT ( 'NONE',  ( -16.46253265017160317, 9.564922557960807481, 25.83224293864769194 ) ) ;
#109885=CARTESIAN_POINT ( 'NONE',  ( 16.55341960407611168, 4.379528057220329451, 38.95724293864768839 ) ) ;
#109886=CARTESIAN_POINT ( 'NONE',  ( -13.97604488694527625, -13.89961937509977652, 71.87390960531433848 ) ) ;
#109888=CARTESIAN_POINT ( 'NONE',  ( -16.46253265017146816, -9.564922557961047289, 34.16775706135233293 ) ) ;
#109889=CARTESIAN_POINT ( 'NONE',  ( 4.483927247898790824, -16.52544592524335698, 45.20942372801901854 ) ) ;
#109890=CARTESIAN_POINT ( 'NONE',  ( -10.81492255796078084, -18.62759615963271287, 62.08224293864769550 ) ) ;
#109891=CARTESIAN_POINT ( 'NONE',  ( -13.89961937509957401, -13.97604488694547875, 24.37609039468565442 ) ) ;
#109892=CARTESIAN_POINT ( 'NONE',  ( 9.564922557960805705, 16.46253265017160317, 74.58224293864769550 ) ) ;
#109894=CARTESIAN_POINT ( 'NONE',  ( -19.05341960407611168, -5.049401038298163336, 106.4572429386476955 ) ) ;
#109895=CARTESIAN_POINT ( 'NONE',  ( -19.03943276465977164, 0.05219959533909376836, 61.24890960531436690 ) ) ;
#109896=CARTESIAN_POINT ( 'NONE',  ( 5.719274019375673035, 21.55341960407619339, 32.29275706135235424 ) ) ;
#109897=CARTESIAN_POINT ( 'NONE',  ( -16.55341960407611168, -4.379528057220339221, 111.4572429386476813 ) ) ;
#109898=CARTESIAN_POINT ( 'NONE',  ( -21.53943276465977519, 0.05219959533907696930, 96.24890960531435269 ) ) ;
#109899=CARTESIAN_POINT ( 'NONE',  ( 13.89961937509977652, -13.97604488694527269, 83.12390960531436690 ) ) ;
#109901=CARTESIAN_POINT ( 'NONE',  ( -10.72451020669870658, -18.67979575497194134, 29.58442372801901854 ) ) ;
#109903=CARTESIAN_POINT ( 'NONE',  ( 16.46253265017160672, -9.564922557960803928, 93.33224293864769550 ) ) ;
#109904=CARTESIAN_POINT ( 'NONE',  ( 19.49149378614661643, -5.499999999999573674, 81.93757513605360998 ) ) ;
#109905=CARTESIAN_POINT ( 'NONE',  ( -18.62759615963270932, 10.81492255796079327, 100.8322429386477097 ) ) ;
#109906=CARTESIAN_POINT ( 'NONE',  ( -19.05341960407611168, -5.049401038298163336, 36.45724293864766707 ) ) ;
#109907=CARTESIAN_POINT ( 'NONE',  ( 16.51473224551083163, -9.474510206698727899, 100.8344237280190043 ) ) ;
#109909=CARTESIAN_POINT ( 'NONE',  ( 13.97604488694527802, 13.89961937509977652, 24.37390960531435624 ) ) ;
#109910=CARTESIAN_POINT ( 'NONE',  ( -18.62759615963255300, -10.81492255796106328, 84.16775706135234714 ) ) ;
#109911=CARTESIAN_POINT ( 'NONE',  ( -19.03943276465977164, 0.05219959533909376836, 81.24890960531436690 ) ) ;
#109912=CARTESIAN_POINT ( 'NONE',  ( 5.719274019375673035, 21.55341960407619339, 47.29275706135234003 ) ) ;
#109913=CARTESIAN_POINT ( 'NONE',  ( -5.823673210054431948, 21.52544592524334988, 22.70942372801901499 ) ) ;
#109915=CARTESIAN_POINT ( 'NONE',  ( -0.05219959533909027116, -19.03943276465977164, 87.49890960531436690 ) ) ;
#109917=CARTESIAN_POINT ( 'NONE',  ( 19.52851543214742591, 5.500000000000027534, 62.89357721762582543 ) ) ;
#109918=CARTESIAN_POINT ( 'NONE',  ( 12.14591786802327356, -12.06949235617739191, 40.62609039468567573 ) ) ;
#109919=CARTESIAN_POINT ( 'NONE',  ( 5.823673210054125526, 21.52544592524343514, 49.79057627198102409 ) ) ;
#109920=CARTESIAN_POINT ( 'NONE',  ( 21.52544592524334988, 5.823673210054432836, 46.45942372801901854 ) ) ;
#109921=CARTESIAN_POINT ( 'NONE',  ( 0.05219959533937995610, -21.53943276465977519, 80.00109039468568994 ) ) ;
#109924=CARTESIAN_POINT ( 'NONE',  ( -5.049401038297874678, -19.05341960407617918, 109.7927570613523187 ) ) ;
#109925=CARTESIAN_POINT ( 'NONE',  ( 5.049401038298161559, -19.05341960407611168, 57.70724293864769550 ) ) ;
#109926=CARTESIAN_POINT ( 'NONE',  ( 19.05341960407611168, 5.049401038298154454, 83.95724293864766707 ) ) ;
#109927=CARTESIAN_POINT ( 'NONE',  ( -0.05219959533910754901, -16.53943276465976808, 102.4989096053143811 ) ) ;
#109928=CARTESIAN_POINT ( 'NONE',  ( -14.29746914071049879, 8.314922557960819915, 105.8322429386476955 ) ) ;
#109929=CARTESIAN_POINT ( 'NONE',  ( 19.02544592524343514, -5.153800228976328945, 113.5405762719810241 ) ) ;
#109930=CARTESIAN_POINT ( 'NONE',  ( -0.05219959533934338120, 16.53943276465976808, 77.50109039468567573 ) ) ;
#109931=CARTESIAN_POINT ( 'NONE',  ( -16.55341960407611168, -4.379528057220339221, 71.45724293864769550 ) ) ;
#109932=CARTESIAN_POINT ( 'NONE',  ( -13.97604488694527625, -13.89961937509977652, 51.87390960531436690 ) ) ;
#109933=CARTESIAN_POINT ( 'NONE',  ( 5.823673210054444382, -21.52544592524334988, 80.20942372801901854 ) ) ;
#109934=CARTESIAN_POINT ( 'NONE',  ( -5.719274019375665041, -21.55341960407619695, 74.79275706135234714 ) ) ;
#109935=CARTESIAN_POINT ( 'NONE',  ( 5.049401038297881783, 19.05341960407617563, 112.2927570613523471 ) ) ;
#109936=CARTESIAN_POINT ( 'NONE',  ( -14.34966873604960291, -8.224510206698953496, 66.66557627198102409 ) ) ;
#109937=CARTESIAN_POINT ( 'NONE',  ( -5.719274019375665041, -21.55341960407619695, 34.79275706135235424 ) ) ;
#109938=CARTESIAN_POINT ( 'NONE',  ( -15.72974639402197994, 15.80617190586746368, 60.62390960531437401 ) ) ;
#109941=CARTESIAN_POINT ( 'NONE',  ( -19.03943276465977164, 0.05219959533909376836, 66.24890960531436690 ) ) ;
#109942=CARTESIAN_POINT ( 'NONE',  ( 4.483927247898545687, 16.52544592524342804, 39.79057627198103830 ) ) ;
#109944=CARTESIAN_POINT ( 'NONE',  ( -8.314922557960811034, -14.29746914071050412, 22.08224293864769194 ) ) ;
#109945=CARTESIAN_POINT ( 'NONE',  ( -0.05219959533934338120, 16.53943276465976808, 92.50109039468567573 ) ) ;
#109946=CARTESIAN_POINT ( 'NONE',  ( -19.02544592524334988, -5.153800228976617603, 53.95942372801898301 ) ) ;
#109947=CARTESIAN_POINT ( 'NONE',  ( 16.18388926212241685, 7.379444403734403579, 47.93953151366155652 ) ) ;
#109948=CARTESIAN_POINT ( 'NONE',  ( 19.05341960407611168, 5.049401038298154454, 108.9572429386477097 ) ) ;
#109949=CARTESIAN_POINT ( 'NONE',  ( 4.483927247898545687, 16.52544592524342804, 79.79057627198102409 ) ) ;
#109950=CARTESIAN_POINT ( 'NONE',  ( 0.05219959533936267826, -19.03943276465977164, 50.00109039468566863 ) ) ;
#109951=CARTESIAN_POINT ( 'NONE',  ( 17.48847506799970475, -5.747544572773726657, 103.3269743784328085 ) ) ;
#109952=CARTESIAN_POINT ( 'NONE',  ( -13.89961937509977652, 13.97604488694528158, 115.6239096053143669 ) ) ;
#109953=CARTESIAN_POINT ( 'NONE',  ( -5.823673210054116645, -21.52544592524344225, 52.29057627198102409 ) ) ;
#109955=CARTESIAN_POINT ( 'NONE',  ( 4.483927247898545687, 16.52544592524342804, 99.79057627198103830 ) ) ;
#109956=CARTESIAN_POINT ( 'NONE',  ( -16.55341960407617563, 4.379528057220093196, 53.54275706135234714 ) ) ;
#109957=CARTESIAN_POINT ( 'NONE',  ( 0.05219959533910956823, 16.53943276465976808, 89.99890960531438111 ) ) ;
#109958=CARTESIAN_POINT ( 'NONE',  ( 16.79531203550644847, -7.028104445595739769, 36.24755011779556924 ) ) ;
#109959=CARTESIAN_POINT ( 'NONE',  ( -17.26058549869090797, 6.457015423128607878, 48.62254162523932166 ) ) ;
#109960=CARTESIAN_POINT ( 'NONE',  ( 15.80617190586746368, 15.72974639402197994, 24.37390960531435979 ) ) ;
#109962=CARTESIAN_POINT ( 'NONE',  ( -15.49999999999999822, -5.500000000000000888, 118.0000000000000142 ) ) ;
#109963=CARTESIAN_POINT ( 'NONE',  ( 14.34966873604972726, -8.224510206698740333, 40.83442372801901854 ) ) ;
#109964=CARTESIAN_POINT ( 'NONE',  ( 14.29746914071049879, -8.314922557960816363, 23.33224293864769194 ) ) ;
#109965=CARTESIAN_POINT ( 'NONE',  ( 21.52544592524344225, -5.823673210054117533, 58.54057627198103120 ) ) ;
#109966=CARTESIAN_POINT ( 'NONE',  ( -0.05219959533936034679, 19.03943276465977164, 82.50109039468567573 ) ) ;
#109967=CARTESIAN_POINT ( 'NONE',  ( 21.55341960407610458, 5.719274019375980345, 48.95724293864770971 ) ) ;
#109968=CARTESIAN_POINT ( 'NONE',  ( -21.52544592524334988, -5.823673210054445271, 83.95942372801900433 ) ) ;
#109970=CARTESIAN_POINT ( 'NONE',  ( -16.52544592524335698, -4.483927247898792601, 38.95942372801901854 ) ) ;
#109971=CARTESIAN_POINT ( 'NONE',  ( -5.049401038298153566, 19.05341960407611168, 35.20724293864768839 ) ) ;
#109972=CARTESIAN_POINT ( 'NONE',  ( 19.03943276465977164, -0.05219959533909143690, 103.7489096053143669 ) ) ;
#109973=CARTESIAN_POINT ( 'NONE',  ( -5.049401038298153566, 19.05341960407611168, 30.20724293864768839 ) ) ;
#109974=CARTESIAN_POINT ( 'NONE',  ( -8.314922557960811034, -14.29746914071050412, 97.08224293864770971 ) ) ;
#109976=CARTESIAN_POINT ( 'NONE',  ( -5.049401038298153566, 19.05341960407611168, 105.2072429386476671 ) ) ;
#109978=CARTESIAN_POINT ( 'NONE',  ( 16.52544592524335698, 4.483927247898782831, 56.45942372801902565 ) ) ;
#109979=CARTESIAN_POINT ( 'NONE',  ( -10.81492255796078084, -18.62759615963271287, 87.08224293864769550 ) ) ;
#109980=CARTESIAN_POINT ( 'NONE',  ( -13.89961937509977652, 13.97604488694528158, 45.62390960531433848 ) ) ;
#109981=CARTESIAN_POINT ( 'NONE',  ( 10.72451020669871369, 18.67979575497193778, 27.08442372801901854 ) ) ;
#109982=CARTESIAN_POINT ( 'NONE',  ( -9.474510206698964154, 16.51473224551069663, 80.41557627198103830 ) ) ;
#109983=CARTESIAN_POINT ( 'NONE',  ( -5.049401038298153566, 19.05341960407611168, 115.2072429386477097 ) ) ;
#109985=CARTESIAN_POINT ( 'NONE',  ( 8.224510206698742110, 14.34966873604972548, 47.08442372801901854 ) ) ;
#109986=CARTESIAN_POINT ( 'NONE',  ( 10.81492255796106328, -18.62759615963255655, 20.41775706135234714 ) ) ;
#109987=CARTESIAN_POINT ( 'NONE',  ( -14.29746914071049879, 8.314922557960819915, 115.8322429386477097 ) ) ;
#109988=CARTESIAN_POINT ( 'NONE',  ( -9.564922557960796823, -16.46253265017161027, 97.08224293864769550 ) ) ;
#109989=CARTESIAN_POINT ( 'NONE',  ( -9.474510206698720793, -16.51473224551083518, 69.58442372801901854 ) ) ;
#109990=CARTESIAN_POINT ( 'NONE',  ( -9.564922557961040184, 16.46253265017147172, 32.91775706135233293 ) ) ;
#109991=CARTESIAN_POINT ( 'NONE',  ( 21.53943276465977519, -0.05219959533907433946, 83.74890960531435269 ) ) ;
#109992=CARTESIAN_POINT ( 'NONE',  ( 13.89961937509957401, 13.97604488694547697, 31.87609039468566863 ) ) ;
#109993=CARTESIAN_POINT ( 'NONE',  ( -4.379528057220086978, -16.55341960407618274, 84.79275706135234714 ) ) ;
#109994=CARTESIAN_POINT ( 'NONE',  ( 9.564922557960805705, 16.46253265017160317, 109.5822429386476955 ) ) ;
#109995=CARTESIAN_POINT ( 'NONE',  ( 19.02544592524343514, -5.153800228976328945, 63.54057627198103830 ) ) ;
#109996=CARTESIAN_POINT ( 'NONE',  ( -5.719274019375665041, -21.55341960407619695, 64.79275706135234714 ) ) ;
#109997=CARTESIAN_POINT ( 'NONE',  ( -21.52544592524334988, -5.823673210054445271, 73.95942372801901854 ) ) ;
#109998=CARTESIAN_POINT ( 'NONE',  ( -16.46253265017160317, 9.564922557960807481, 80.83224293864769550 ) ) ;
#109999=CARTESIAN_POINT ( 'NONE',  ( 5.823673210054444382, -21.52544592524334988, 45.20942372801901854 ) ) ;
#110000=CARTESIAN_POINT ( 'NONE',  ( 13.97604488694548053, -13.89961937509957401, 90.62609039468567573 ) ) ;
#110001=CARTESIAN_POINT ( 'NONE',  ( 13.97604488694527802, 13.89961937509977652, 59.37390960531434558 ) ) ;
#110002=CARTESIAN_POINT ( 'NONE',  ( -9.564922557960796823, -16.46253265017161027, 97.08224293864769550 ) ) ;
#110003=CARTESIAN_POINT ( 'NONE',  ( 0.05219959533909260263, 19.03943276465977164, 69.99890960531435269 ) ) ;
#110004=CARTESIAN_POINT ( 'NONE',  ( 5.153800228976335163, 19.02544592524342804, 114.7905762719810241 ) ) ;
#110005=CARTESIAN_POINT ( 'NONE',  ( -9.474510206698964154, 16.51473224551069663, 50.41557627198102409 ) ) ;
#110006=CARTESIAN_POINT ( 'NONE',  ( 15.80617190586746368, 15.72974639402197994, 99.37390960531436690 ) ) ;
#110007=CARTESIAN_POINT ( 'NONE',  ( 8.224510206698742110, 14.34966873604972548, 72.08442372801899012 ) ) ;
#110009=CARTESIAN_POINT ( 'NONE',  ( -16.51473224551082808, 9.474510206698731452, 28.33442372801900433 ) ) ;
#110010=CARTESIAN_POINT ( 'NONE',  ( -5.153800228976328057, -19.02544592524343514, 67.29057627198102409 ) ) ;
#110011=CARTESIAN_POINT ( 'NONE',  ( 16.55341960407611168, 4.379528057220329451, 63.95724293864770260 ) ) ;
#110012=CARTESIAN_POINT ( 'NONE',  ( -12.06949235617756955, 12.14591786802309770, 100.6239096053143811 ) ) ;
#110013=CARTESIAN_POINT ( 'NONE',  ( -0.05219959533909027116, -19.03943276465977164, 97.49890960531436690 ) ) ;
#110014=CARTESIAN_POINT ( 'NONE',  ( -0.05219959533909027116, -19.03943276465977164, 97.49890960531436690 ) ) ;
#110015=CARTESIAN_POINT ( 'NONE',  ( 15.72974639402176855, 15.80617190586768217, 56.87609039468568994 ) ) ;
#110016=CARTESIAN_POINT ( 'NONE',  ( -5.153800228976328057, -19.02544592524343514, 102.2905762719810383 ) ) ;
#110018=CARTESIAN_POINT ( 'NONE',  ( 15.72974639402176855, 15.80617190586768217, 111.8760903946856615 ) ) ;
#110019=CARTESIAN_POINT ( 'NONE',  ( -12.14591786802326823, 12.06949235617739902, 83.12609039468568994 ) ) ;
#110021=CARTESIAN_POINT ( 'NONE',  ( -18.67979575497193778, 10.72451020669871902, 43.33442372801901143 ) ) ;
#110022=CARTESIAN_POINT ( 'NONE',  ( 18.67979575497178502, 10.72451020669898547, 29.16557627198103120 ) ) ;
#110023=CARTESIAN_POINT ( 'NONE',  ( 0.05219959533907565091, 21.53943276465977519, 104.9989096053143669 ) ) ;
#110025=CARTESIAN_POINT ( 'NONE',  ( -14.34966873604960291, -8.224510206698953496, 61.66557627198103120 ) ) ;
#110026=CARTESIAN_POINT ( 'NONE',  ( 19.02544592524343514, -5.153800228976328945, 53.54057627198102409 ) ) ;
#110027=CARTESIAN_POINT ( 'NONE',  ( -16.55341960407611168, -4.379528057220339221, 86.45724293864770971 ) ) ;
#110028=CARTESIAN_POINT ( 'NONE',  ( 18.62759615963271287, -10.81492255796078972, 43.33224293864769550 ) ) ;
#110029=CARTESIAN_POINT ( 'NONE',  ( 19.03943276465977164, 0.05219959533936151252, 41.25109039468566152 ) ) ;
#110030=CARTESIAN_POINT ( 'NONE',  ( -0.05219959533909027116, -19.03943276465977164, 22.49890960531436690 ) ) ;
#110032=CARTESIAN_POINT ( 'NONE',  ( 14.29746914071037800, 8.314922557961029526, 71.66775706135234714 ) ) ;
#110033=CARTESIAN_POINT ( 'NONE',  ( 9.474510206698971260, -16.51473224551069308, 67.91557627198102409 ) ) ;
#110035=CARTESIAN_POINT ( 'NONE',  ( -0.05219959533910754901, -16.53943276465976808, 87.49890960531436690 ) ) ;
#110036=CARTESIAN_POINT ( 'NONE',  ( 18.62759615963271287, -10.81492255796078972, 33.33224293864769550 ) ) ;
#110037=CARTESIAN_POINT ( 'NONE',  ( 14.29746914071037800, 8.314922557961029526, 111.6677570613523613 ) ) ;
#110038=CARTESIAN_POINT ( 'NONE',  ( -16.52544592524335698, -4.483927247898792601, 23.95942372801901143 ) ) ;
#110039=CARTESIAN_POINT ( 'NONE',  ( -10.72451020669870658, -18.67979575497194134, 94.58442372801901854 ) ) ;
#110040=CARTESIAN_POINT ( 'NONE',  ( 19.03943276465977164, -0.05219959533909143690, 88.74890960531436690 ) ) ;
#110041=CARTESIAN_POINT ( 'NONE',  ( -10.72451020669898014, 18.67979575497178502, 110.4155762719810383 ) ) ;
#110042=CARTESIAN_POINT ( 'NONE',  ( 16.55341960407618274, -4.379528057220086978, 51.04275706135234714 ) ) ;
#110043=CARTESIAN_POINT ( 'NONE',  ( 16.51473224551069308, 9.474510206698969483, 29.16557627198103475 ) ) ;
#110044=CARTESIAN_POINT ( 'NONE',  ( 4.379528057220092307, 16.55341960407617563, 32.29275706135235424 ) ) ;
#110045=CARTESIAN_POINT ( 'NONE',  ( -13.89961937509957401, -13.97604488694547875, 94.37609039468566152 ) ) ;
#110046=CARTESIAN_POINT ( 'NONE',  ( -10.72451020669898014, 18.67979575497178502, 90.41557627198103830 ) ) ;
#110047=CARTESIAN_POINT ( 'NONE',  ( -16.46253265017146816, -9.564922557961047289, 74.16775706135234714 ) ) ;
#110049=CARTESIAN_POINT ( 'NONE',  ( 15.72974639402199770, -15.80617190586745480, 108.1239096053143811 ) ) ;
#110051=CARTESIAN_POINT ( 'NONE',  ( -16.51473224551069308, -9.474510206698971260, 81.66557627198103830 ) ) ;
#110052=CARTESIAN_POINT ( 'NONE',  ( 14.29746914071037800, 8.314922557961029526, 36.66775706135234714 ) ) ;
#110054=CARTESIAN_POINT ( 'NONE',  ( -16.51473224551082808, 9.474510206698731452, 58.33442372801900433 ) ) ;
#110055=CARTESIAN_POINT ( 'NONE',  ( 21.53943276465977519, 0.05219959533937863772, 21.25109039468567218 ) ) ;
#110056=CARTESIAN_POINT ( 'NONE',  ( 12.06949235617757843, -12.14591786802309237, 73.12390960531436690 ) ) ;
#110057=CARTESIAN_POINT ( 'NONE',  ( 5.153800228976335163, 19.02544592524342804, 84.79057627198099567 ) ) ;
#110058=CARTESIAN_POINT ( 'NONE',  ( -12.14591786802326823, 12.06949235617739902, 33.12609039468569705 ) ) ;
#110059=CARTESIAN_POINT ( 'NONE',  ( 13.97604488694548053, -13.89961937509957401, 35.62609039468567573 ) ) ;
#110060=CARTESIAN_POINT ( 'NONE',  ( 10.72451020669871369, 18.67979575497193778, 57.08442372801901854 ) ) ;
#110061=CARTESIAN_POINT ( 'NONE',  ( -19.05341960407617563, 5.049401038297882671, 108.5427570613523187 ) ) ;
#110062=CARTESIAN_POINT ( 'NONE',  ( -5.049401038298153566, 19.05341960407611168, 55.20724293864769550 ) ) ;
#110063=CARTESIAN_POINT ( 'NONE',  ( 0.05219959533936267826, -19.03943276465977164, 80.00109039468567573 ) ) ;
#110064=CARTESIAN_POINT ( 'NONE',  ( 4.379528057220092307, 16.55341960407617563, 57.29275706135234714 ) ) ;
#110065=CARTESIAN_POINT ( 'NONE',  ( 10.81492255796106328, -18.62759615963255655, 95.41775706135234714 ) ) ;
#110066=CARTESIAN_POINT ( 'NONE',  ( 19.03943276465977164, 0.05219959533936151252, 66.25109039468567573 ) ) ;
#110067=CARTESIAN_POINT ( 'NONE',  ( 9.564922557960805705, 16.46253265017160317, 34.58224293864770260 ) ) ;
#110068=CARTESIAN_POINT ( 'NONE',  ( -21.52544592524343514, 5.823673210054127303, 71.04057627198103830 ) ) ;
#110069=CARTESIAN_POINT ( 'NONE',  ( 16.53943276465976808, -0.05219959533910856209, 68.74890960531435269 ) ) ;
#110070=CARTESIAN_POINT ( 'NONE',  ( 0.05219959533936267826, -19.03943276465977164, 65.00109039468567573 ) ) ;
#110072=CARTESIAN_POINT ( 'NONE',  ( -16.51473224551082808, 9.474510206698731452, 38.33442372801899722 ) ) ;
#110073=CARTESIAN_POINT ( 'NONE',  ( -14.34966873604972548, 8.224510206698743886, 93.33442372801901854 ) ) ;
#110074=CARTESIAN_POINT ( 'NONE',  ( -0.05219959533910754901, -16.53943276465976808, 52.49890960531435979 ) ) ;
#110075=CARTESIAN_POINT ( 'NONE',  ( -5.719274019375665041, -21.55341960407619695, 89.79275706135236135 ) ) ;
#110077=CARTESIAN_POINT ( 'NONE',  ( -21.52544592524343514, 5.823673210054127303, 101.0405762719810383 ) ) ;
#110078=CARTESIAN_POINT ( 'NONE',  ( 19.05341960407611168, 5.049401038298154454, 53.95724293864770260 ) ) ;
#110079=CARTESIAN_POINT ( 'NONE',  ( 18.62759615963255655, 10.81492255796105972, 66.66775706135234714 ) ) ;
#110080=CARTESIAN_POINT ( 'NONE',  ( 5.153800228976335163, 19.02544592524342804, 49.79057627198100988 ) ) ;
#110082=CARTESIAN_POINT ( 'NONE',  ( 5.153800228976335163, 19.02544592524342804, 59.79057627198100988 ) ) ;
#110083=CARTESIAN_POINT ( 'NONE',  ( -16.53943276465976808, 0.05219959533911058130, 116.2489096053143669 ) ) ;
#110084=CARTESIAN_POINT ( 'NONE',  ( -10.81492255796078084, -18.62759615963271287, 22.08224293864769194 ) ) ;
#110085=CARTESIAN_POINT ( 'NONE',  ( 0.05219959533910956823, 16.53943276465976808, 54.99890960531435269 ) ) ;
#110086=CARTESIAN_POINT ( 'NONE',  ( 5.153800228976335163, 19.02544592524342804, 34.79057627198102409 ) ) ;
#110087=CARTESIAN_POINT ( 'NONE',  ( 0.05219959533910956823, 16.53943276465976808, 79.99890960531435269 ) ) ;
#110088=CARTESIAN_POINT ( 'NONE',  ( 15.80617190586746368, 15.72974639402197994, 99.37390960531436690 ) ) ;
#110089=CARTESIAN_POINT ( 'NONE',  ( 10.81492255796106328, -18.62759615963255655, 30.41775706135234358 ) ) ;
#110092=CARTESIAN_POINT ( 'NONE',  ( 8.224510206698742110, 14.34966873604972548, 57.08442372801901854 ) ) ;
#110093=CARTESIAN_POINT ( 'NONE',  ( -15.72974639402197994, 15.80617190586746368, 90.62390960531436690 ) ) ;
#110094=CARTESIAN_POINT ( 'NONE',  ( 18.67979575497194134, -10.72451020669871369, 110.8344237280190043 ) ) ;
#110095=CARTESIAN_POINT ( 'NONE',  ( 16.46253265017160672, -9.564922557960803928, 113.3322429386476955 ) ) ;
#110096=CARTESIAN_POINT ( 'NONE',  ( 18.62759615963255655, 10.81492255796105972, 46.66775706135234714 ) ) ;
#110097=CARTESIAN_POINT ( 'NONE',  ( -0.05219959533907301413, -21.53943276465977519, 42.49890960531435979 ) ) ;
#110098=CARTESIAN_POINT ( 'NONE',  ( -8.314922557961024197, 14.29746914071037800, 107.9177570613523471 ) ) ;
#110099=CARTESIAN_POINT ( 'NONE',  ( -15.72974639402176322, -15.80617190586768395, 59.37609039468568284 ) ) ;
#110100=CARTESIAN_POINT ( 'NONE',  ( 10.72451020669871369, 18.67979575497193778, 82.08442372801901854 ) ) ;
#110101=CARTESIAN_POINT ( 'NONE',  ( 0.05219959533936267826, -19.03943276465977164, 35.00109039468566863 ) ) ;
#110102=CARTESIAN_POINT ( 'NONE',  ( -16.55341960407617563, 4.379528057220093196, 83.54275706135234714 ) ) ;
#110103=CARTESIAN_POINT ( 'NONE',  ( 21.52544592524334988, 5.823673210054432836, 36.45942372801901143 ) ) ;
#110104=CARTESIAN_POINT ( 'NONE',  ( 0.05219959533909260263, 19.03943276465977164, 49.99890960531435979 ) ) ;
#110105=CARTESIAN_POINT ( 'NONE',  ( 13.89961937509957401, 13.97604488694547697, 21.87609039468566152 ) ) ;
#110106=CARTESIAN_POINT ( 'NONE',  ( -21.53943276465977519, 0.05219959533907696930, 31.24890960531435979 ) ) ;
#110108=CARTESIAN_POINT ( 'NONE',  ( 0.05219959533937995610, -21.53943276465977519, 20.00109039468568639 ) ) ;
#110109=CARTESIAN_POINT ( 'NONE',  ( -5.719274019375978568, 21.55341960407610458, 70.20724293864769550 ) ) ;
#110110=CARTESIAN_POINT ( 'NONE',  ( -17.72662750342724891, -5.500000000000087930, 61.40179492283743201 ) ) ;
#110111=CARTESIAN_POINT ( 'NONE',  ( -21.55341960407610458, -5.719274019375992779, 86.45724293864770971 ) ) ;
#110112=CARTESIAN_POINT ( 'NONE',  ( -4.379528057220086978, -16.55341960407618274, 59.79275706135234714 ) ) ;
#110113=CARTESIAN_POINT ( 'NONE',  ( -12.14591786802309592, -12.06949235617757132, 66.87390960531436690 ) ) ;
#110115=CARTESIAN_POINT ( 'NONE',  ( 16.51473224551083163, -9.474510206698727899, 95.83442372801900433 ) ) ;
#110117=CARTESIAN_POINT ( 'NONE',  ( -14.29746914071037622, -8.314922557961029526, 39.16775706135235424 ) ) ;
#110118=CARTESIAN_POINT ( 'NONE',  ( 5.719274019375991003, -21.55341960407610458, 92.70724293864770971 ) ) ;
#110119=CARTESIAN_POINT ( 'NONE',  ( -21.53943276465977519, 0.05219959533907696930, 81.24890960531436690 ) ) ;
#110120=CARTESIAN_POINT ( 'NONE',  ( -21.53943276465977519, 0.05219959533907696930, 21.24890960531436690 ) ) ;
#110121=CARTESIAN_POINT ( 'NONE',  ( 16.53943276465976808, 0.05219959533934440121, 61.25109039468567573 ) ) ;
#110122=CARTESIAN_POINT ( 'NONE',  ( -16.46253265017160317, 9.564922557960807481, 65.83224293864769550 ) ) ;
#110123=CARTESIAN_POINT ( 'NONE',  ( -21.52544592524334988, -5.823673210054445271, 38.95942372801901854 ) ) ;
#110124=CARTESIAN_POINT ( 'NONE',  ( 19.03943276465977164, 0.05219959533936151252, 111.2510903946856757 ) ) ;
#110125=CARTESIAN_POINT ( 'NONE',  ( 13.89961937509977652, -13.97604488694527269, 108.1239096053143669 ) ) ;
#110126=CARTESIAN_POINT ( 'NONE',  ( -0.05219959533936034679, 19.03943276465977164, 27.50109039468566507 ) ) ;
#110127=CARTESIAN_POINT ( 'NONE',  ( -12.14591786802326823, 12.06949235617739902, 38.12609039468567573 ) ) ;
#110128=CARTESIAN_POINT ( 'NONE',  ( -13.97604488694527625, -13.89961937509977652, 96.87390960531433848 ) ) ;
#110129=CARTESIAN_POINT ( 'NONE',  ( 21.53943276465977519, -0.05219959533907433946, 108.7489096053143669 ) ) ;
#110130=CARTESIAN_POINT ( 'NONE',  ( -5.049401038298153566, 19.05341960407611168, 55.20724293864769550 ) ) ;
#110131=CARTESIAN_POINT ( 'NONE',  ( -12.06949235617756955, 12.14591786802309770, 85.62390960531436690 ) ) ;
#110132=CARTESIAN_POINT ( 'NONE',  ( 10.72451020669898902, -18.67979575497178502, 27.91557627198103830 ) ) ;
#110133=CARTESIAN_POINT ( 'NONE',  ( -16.52216118717208104, 7.221426719304501418, 33.92400978953008206 ) ) ;
#110134=CARTESIAN_POINT ( 'NONE',  ( 10.81492255796078972, 18.62759615963270932, 109.5822429386476955 ) ) ;
#110135=CARTESIAN_POINT ( 'NONE',  ( -9.564922557961040184, 16.46253265017147172, 62.91775706135233293 ) ) ;
#110136=CARTESIAN_POINT ( 'NONE',  ( -16.51473224551069308, -9.474510206698971260, 111.6655762719810383 ) ) ;
#110137=CARTESIAN_POINT ( 'NONE',  ( 19.02544592524343514, -5.153800228976328945, 23.54057627198102054 ) ) ;
#110138=CARTESIAN_POINT ( 'NONE',  ( 10.72451020669898902, -18.67979575497178502, 57.91557627198103120 ) ) ;
#110139=CARTESIAN_POINT ( 'NONE',  ( 13.97604488694527802, 13.89961937509977652, 99.37390960531436690 ) ) ;
#110140=CARTESIAN_POINT ( 'NONE',  ( 5.719274019375673035, 21.55341960407619339, 77.29275706135234714 ) ) ;
#110141=CARTESIAN_POINT ( 'NONE',  ( 13.89961937509977652, -13.97604488694527269, 58.12390960531436690 ) ) ;
#110142=CARTESIAN_POINT ( 'NONE',  ( 8.224510206698953496, -14.34966873604960469, 87.91557627198103830 ) ) ;
#110143=CARTESIAN_POINT ( 'NONE',  ( 8.314922557961029526, -14.29746914071037800, 40.41775706135234714 ) ) ;
#110144=CARTESIAN_POINT ( 'NONE',  ( -18.67979575497193778, 10.72451020669871902, 68.33442372801900433 ) ) ;
#110146=CARTESIAN_POINT ( 'NONE',  ( 19.03943276465977164, 0.05219959533936151252, 21.25109039468565797 ) ) ;
#110147=CARTESIAN_POINT ( 'NONE',  ( -0.05219959533936034679, 19.03943276465977164, 82.50109039468567573 ) ) ;
#110148=CARTESIAN_POINT ( 'NONE',  ( 5.153800228976615827, -19.02544592524334988, 40.20942372801898301 ) ) ;
#110150=CARTESIAN_POINT ( 'NONE',  ( 5.719274019375673035, 21.55341960407619339, 37.29275706135235424 ) ) ;
#110152=CARTESIAN_POINT ( 'NONE',  ( 13.97604488694548053, -13.89961937509957401, 30.62609039468566863 ) ) ;
#110153=CARTESIAN_POINT ( 'NONE',  ( -19.03943276465977164, 0.05219959533909376836, 71.24890960531435269 ) ) ;
#110154=CARTESIAN_POINT ( 'NONE',  ( 4.379528057220339221, -16.55341960407611168, 22.70724293864769194 ) ) ;
#110155=CARTESIAN_POINT ( 'NONE',  ( -18.67979575497178146, -10.72451020669898902, 26.66557627198103475 ) ) ;
#110156=CARTESIAN_POINT ( 'NONE',  ( -18.67979575497193778, 10.72451020669871902, 88.33442372801901854 ) ) ;
#110159=CARTESIAN_POINT ( 'NONE',  ( -18.62759615963255300, -10.81492255796106328, 79.16775706135234714 ) ) ;
#110161=CARTESIAN_POINT ( 'NONE',  ( -19.02544592524342804, 5.153800228976336051, 106.0405762719810241 ) ) ;
#110163=CARTESIAN_POINT ( 'NONE',  ( 5.153800228976335163, 19.02544592524342804, 54.79057627198103120 ) ) ;
#110164=CARTESIAN_POINT ( 'NONE',  ( -21.52544592524343514, 5.823673210054127303, 51.04057627198103120 ) ) ;
#110165=CARTESIAN_POINT ( 'NONE',  ( 16.53943276465976808, -0.05219959533910856209, 28.74890960531435624 ) ) ;
#110166=CARTESIAN_POINT ( 'NONE',  ( 16.53943276465976808, -0.05219959533910856209, 108.7489096053143669 ) ) ;
#110167=CARTESIAN_POINT ( 'NONE',  ( -9.564922557960796823, -16.46253265017161027, 97.08224293864769550 ) ) ;
#110168=CARTESIAN_POINT ( 'NONE',  ( 18.67979575497194134, -10.72451020669871369, 110.8344237280190043 ) ) ;
#110169=CARTESIAN_POINT ( 'NONE',  ( 16.55341960407611168, 4.379528057220329451, 108.9572429386476955 ) ) ;
#110170=CARTESIAN_POINT ( 'NONE',  ( 10.81492255796106328, -18.62759615963255655, 65.41775706135234714 ) ) ;
#110172=CARTESIAN_POINT ( 'NONE',  ( -16.52544592524335698, -4.483927247898792601, 108.9594237280190185 ) ) ;
#110173=CARTESIAN_POINT ( 'NONE',  ( 9.564922557961047289, -16.46253265017146816, 60.41775706135233293 ) ) ;
#110175=CARTESIAN_POINT ( 'NONE',  ( -13.89961937509977652, 13.97604488694528158, 105.6239096053143527 ) ) ;
#110176=CARTESIAN_POINT ( 'NONE',  ( -14.29746914071049879, 8.314922557960819915, 70.83224293864770971 ) ) ;
#110177=CARTESIAN_POINT ( 'NONE',  ( 19.03943276465977164, 0.05219959533936151252, 56.25109039468566863 ) ) ;
#110178=CARTESIAN_POINT ( 'NONE',  ( 19.05341960407611168, 5.049401038298154454, 68.95724293864769550 ) ) ;
#110179=CARTESIAN_POINT ( 'NONE',  ( 16.53943276465976808, -0.05219959533910856209, 63.74890960531435979 ) ) ;
#110180=CARTESIAN_POINT ( 'NONE',  ( -5.153800228976607833, 19.02544592524334988, 87.70942372801897591 ) ) ;
#110181=CARTESIAN_POINT ( 'NONE',  ( -21.55341960407610458, -5.719274019375992779, 56.45724293864768839 ) ) ;
#110183=CARTESIAN_POINT ( 'NONE',  ( -16.55341960407611168, -4.379528057220339221, 111.4572429386476813 ) ) ;
#110185=CARTESIAN_POINT ( 'NONE',  ( -5.049401038298153566, 19.05341960407611168, 75.20724293864769550 ) ) ;
#110186=CARTESIAN_POINT ( 'NONE',  ( -21.52544592524343514, 5.823673210054127303, 61.04057627198103120 ) ) ;
#110187=CARTESIAN_POINT ( 'NONE',  ( 4.379528057220092307, 16.55341960407617563, 87.29275706135236135 ) ) ;
#110188=CARTESIAN_POINT ( 'NONE',  ( 5.049401038298161559, -19.05341960407611168, 72.70724293864768129 ) ) ;
#110189=CARTESIAN_POINT ( 'NONE',  ( -19.02544592524334988, -5.153800228976617603, 53.95942372801898301 ) ) ;
#110190=CARTESIAN_POINT ( 'NONE',  ( -10.81492255796105439, 18.62759615963255655, 82.91775706135234714 ) ) ;
#110191=CARTESIAN_POINT ( 'NONE',  ( -21.52544592524343514, 5.823673210054127303, 61.04057627198103120 ) ) ;
#110192=CARTESIAN_POINT ( 'NONE',  ( 9.474510206698971260, -16.51473224551069308, 102.9155762719810241 ) ) ;
#110193=CARTESIAN_POINT ( 'NONE',  ( -0.05219959533909027116, -19.03943276465977164, 32.49890960531435979 ) ) ;
#110194=CARTESIAN_POINT ( 'NONE',  ( 16.52544592524335698, 4.483927247898782831, 96.45942372801901854 ) ) ;
#110195=CARTESIAN_POINT ( 'NONE',  ( 0.05219959533934541429, -16.53943276465976808, 25.00109039468567218 ) ) ;
#110197=CARTESIAN_POINT ( 'NONE',  ( 10.81492255796106328, -18.62759615963255655, 90.41775706135236135 ) ) ;
#110198=CARTESIAN_POINT ( 'NONE',  ( -16.55341960407611168, -4.379528057220339221, 66.45724293864768129 ) ) ;
#110199=CARTESIAN_POINT ( 'NONE',  ( -8.224510206698948167, 14.34966873604960824, 75.41557627198102409 ) ) ;
#110200=CARTESIAN_POINT ( 'NONE',  ( 18.67979575497178502, 10.72451020669898547, 89.16557627198102409 ) ) ;
#110201=CARTESIAN_POINT ( 'NONE',  ( -10.72451020669898014, 18.67979575497178502, 85.41557627198102409 ) ) ;
#110202=CARTESIAN_POINT ( 'NONE',  ( 17.13100169013301155, -6.664070546373149995, 98.26789835699852915 ) ) ;
#110203=CARTESIAN_POINT ( 'NONE',  ( -21.52544592524343514, 5.823673210054127303, 51.04057627198103120 ) ) ;
#110204=CARTESIAN_POINT ( 'NONE',  ( 14.29746914071037800, 8.314922557961029526, 66.66775706135234714 ) ) ;
#110205=CARTESIAN_POINT ( 'NONE',  ( -14.29746914071049879, 8.314922557960819915, 95.83224293864770971 ) ) ;
#110206=CARTESIAN_POINT ( 'NONE',  ( -19.02544592524342804, 5.153800228976336051, 41.04057627198103120 ) ) ;
#110208=CARTESIAN_POINT ( 'NONE',  ( -0.05219959533934338120, 16.53943276465976808, 97.50109039468567573 ) ) ;
#110209=CARTESIAN_POINT ( 'NONE',  ( -21.55341960407619339, 5.719274019375674811, 38.54275706135234714 ) ) ;
#110210=CARTESIAN_POINT ( 'NONE',  ( 16.46253265017160672, -9.564922557960803928, 93.33224293864769550 ) ) ;
#110211=CARTESIAN_POINT ( 'NONE',  ( -18.67979575497193778, 10.72451020669871902, 63.33442372801900433 ) ) ;
#110213=CARTESIAN_POINT ( 'NONE',  ( 16.51473224551069308, 9.474510206698969483, 24.16557627198102765 ) ) ;
#110215=CARTESIAN_POINT ( 'NONE',  ( 0.05219959533937995610, -21.53943276465977519, 55.00109039468568284 ) ) ;
#110216=CARTESIAN_POINT ( 'NONE',  ( 0.05219959533909260263, 19.03943276465977164, 44.99890960531435979 ) ) ;
#110217=CARTESIAN_POINT ( 'NONE',  ( 16.51473224551069308, 9.474510206698969483, 24.16557627198102765 ) ) ;
#110218=CARTESIAN_POINT ( 'NONE',  ( -16.46253265017160317, 9.564922557960807481, 90.83224293864769550 ) ) ;
#110219=CARTESIAN_POINT ( 'NONE',  ( -13.97604488694547697, 13.89961937509957934, 73.12609039468568994 ) ) ;
#110220=CARTESIAN_POINT ( 'NONE',  ( -0.05219959533937732626, 21.53943276465977519, 32.50109039468568284 ) ) ;
#110221=CARTESIAN_POINT ( 'NONE',  ( 19.05341960407617918, -5.049401038297876454, 56.04275706135234714 ) ) ;
#110222=CARTESIAN_POINT ( 'NONE',  ( 19.05341960407611168, 5.049401038298154454, 33.95724293864769550 ) ) ;
#110223=CARTESIAN_POINT ( 'NONE',  ( 8.224510206698742110, 14.34966873604972548, 107.0844237280190043 ) ) ;
#110224=CARTESIAN_POINT ( 'NONE',  ( -19.02544592524334988, -5.153800228976617603, 78.95942372801900433 ) ) ;
#110225=CARTESIAN_POINT ( 'NONE',  ( 12.06949235617757843, -12.14591786802309237, 28.12390960531435979 ) ) ;
#110226=CARTESIAN_POINT ( 'NONE',  ( -9.474510206698720793, -16.51473224551083518, 44.58442372801900433 ) ) ;
#110227=CARTESIAN_POINT ( 'NONE',  ( -0.05219959533909027116, -19.03943276465977164, 102.4989096053143669 ) ) ;
#110228=CARTESIAN_POINT ( 'NONE',  ( -5.823673210054431948, 21.52544592524334988, 102.7094237280190185 ) ) ;
#110229=CARTESIAN_POINT ( 'NONE',  ( 19.03943276465977164, 0.05219959533936151252, 21.25109039468565797 ) ) ;
#110230=CARTESIAN_POINT ( 'NONE',  ( -9.564922557960796823, -16.46253265017161027, 32.08224293864769550 ) ) ;
#110231=CARTESIAN_POINT ( 'NONE',  ( 21.55341960407619695, -5.719274019375665929, 91.04275706135236135 ) ) ;
#110232=CARTESIAN_POINT ( 'NONE',  ( 14.34966873604972726, -8.224510206698740333, 35.83442372801901143 ) ) ;
#110233=CARTESIAN_POINT ( 'NONE',  ( -13.89961937509977652, 13.97604488694528158, 90.62390960531432427 ) ) ;
#110235=CARTESIAN_POINT ( 'NONE',  ( 13.89961937509977652, -13.97604488694527269, 83.12390960531436690 ) ) ;
#110236=CARTESIAN_POINT ( 'NONE',  ( -17.50000000000000000, 5.499999999999992895, 37.50000000000000000 ) ) ;
#110237=CARTESIAN_POINT ( 'NONE',  ( 9.474510206698729675, 16.51473224551082808, 67.08442372801900433 ) ) ;
#110238=CARTESIAN_POINT ( 'NONE',  ( 0.05219959533909260263, 19.03943276465977164, 99.99890960531436690 ) ) ;
#110239=CARTESIAN_POINT ( 'NONE',  ( 18.62759615963255655, 10.81492255796105972, 96.66775706135234714 ) ) ;
#110240=CARTESIAN_POINT ( 'NONE',  ( -14.34966873604960291, -8.224510206698953496, 96.66557627198102409 ) ) ;
#110241=CARTESIAN_POINT ( 'NONE',  ( 21.52544592524344225, -5.823673210054117533, 43.54057627198103830 ) ) ;
#110242=CARTESIAN_POINT ( 'NONE',  ( 18.67979575497178502, 10.72451020669898547, 34.16557627198102409 ) ) ;
#110243=CARTESIAN_POINT ( 'NONE',  ( -0.05219959533910754901, -16.53943276465976808, 102.4989096053143811 ) ) ;
#110244=LINE ( 'NONE', #47596, #108150 ) ;
#110245=CARTESIAN_POINT ( 'NONE',  ( -19.03943276465977164, -0.05219959533935918106, 63.75109039468566863 ) ) ;
#110246=CARTESIAN_POINT ( 'NONE',  ( 4.483927247898545687, 16.52544592524342804, 39.79057627198103830 ) ) ;
#110247=CARTESIAN_POINT ( 'NONE',  ( 15.80617190586746368, 15.72974639402197994, 24.37390960531435979 ) ) ;
#110249=CARTESIAN_POINT ( 'NONE',  ( -5.823673210054431948, 21.52544592524334988, 77.70942372801900433 ) ) ;
#110250=CARTESIAN_POINT ( 'NONE',  ( 21.52544592524344225, -5.823673210054117533, 73.54057627198102409 ) ) ;
#110251=CARTESIAN_POINT ( 'NONE',  ( 10.72451020669871369, 18.67979575497193778, 42.08442372801901854 ) ) ;
#110252=CARTESIAN_POINT ( 'NONE',  ( 21.53943276465977519, -0.05219959533907433946, 93.74890960531436690 ) ) ;
#110253=CARTESIAN_POINT ( 'NONE',  ( 5.719274019375673035, 21.55341960407619339, 57.29275706135234714 ) ) ;
#110254=CARTESIAN_POINT ( 'NONE',  ( 5.049401038298161559, -19.05341960407611168, 27.70724293864769550 ) ) ;
#110255=CARTESIAN_POINT ( 'NONE',  ( 9.474510206698971260, -16.51473224551069308, 82.91557627198103830 ) ) ;
#110256=CARTESIAN_POINT ( 'NONE',  ( -16.52544592524335698, -4.483927247898792601, 83.95942372801900433 ) ) ;
#110257=CARTESIAN_POINT ( 'NONE',  ( 12.14591786802309770, 12.06949235617756955, 109.3739096053143811 ) ) ;
#110258=CARTESIAN_POINT ( 'NONE',  ( -9.564922557960796823, -16.46253265017161027, 112.0822429386476955 ) ) ;
#110259=CARTESIAN_POINT ( 'NONE',  ( -8.314922557960811034, -14.29746914071050412, 52.08224293864768839 ) ) ;
#110260=CARTESIAN_POINT ( 'NONE',  ( -14.34966873604972548, 8.224510206698743886, 113.3344237280190328 ) ) ;
#110261=CARTESIAN_POINT ( 'NONE',  ( -19.05341960407611168, -5.049401038298163336, 71.45724293864766707 ) ) ;
#110262=CARTESIAN_POINT ( 'NONE',  ( -16.46253265017160317, 9.564922557960807481, 35.83224293864768839 ) ) ;
#110263=CARTESIAN_POINT ( 'NONE',  ( -10.72451020669898014, 18.67979575497178502, 45.41557627198103830 ) ) ;
#110264=CARTESIAN_POINT ( 'NONE',  ( -13.97604488694547697, 13.89961937509957934, 43.12609039468566152 ) ) ;
#110266=CARTESIAN_POINT ( 'NONE',  ( 16.55341960407611168, 4.379528057220329451, 33.95724293864769550 ) ) ;
#110267=CARTESIAN_POINT ( 'NONE',  ( -5.153800228976328057, -19.02544592524343514, 112.2905762719810099 ) ) ;
#110268=CARTESIAN_POINT ( 'NONE',  ( -21.53943276465977519, -0.05219959533937600094, 53.75109039468568994 ) ) ;
#110269=CARTESIAN_POINT ( 'NONE',  ( -16.46253265017160317, 9.564922557960807481, 115.8322429386477097 ) ) ;
#110270=CARTESIAN_POINT ( 'NONE',  ( -16.55341960407617563, 4.379528057220093196, 58.54275706135235424 ) ) ;
#110271=CARTESIAN_POINT ( 'NONE',  ( 13.89961937509957401, 13.97604488694547697, 61.87609039468566863 ) ) ;
#110273=CARTESIAN_POINT ( 'NONE',  ( -4.379528057220328563, 16.55341960407611168, 25.20724293864769550 ) ) ;
#110274=CARTESIAN_POINT ( 'NONE',  ( 16.19135201231364363, -7.376712067592015920, 52.31319145947973226 ) ) ;
#110275=CARTESIAN_POINT ( 'NONE',  ( 4.483927247898790824, -16.52544592524335698, 110.2094237280190185 ) ) ;
#110276=CARTESIAN_POINT ( 'NONE',  ( 19.02544592524343514, -5.153800228976328945, 38.54057627198103120 ) ) ;
#110277=CARTESIAN_POINT ( 'NONE',  ( 16.51473224551069308, 9.474510206698969483, 64.16557627198102409 ) ) ;
#110278=CARTESIAN_POINT ( 'NONE',  ( -9.564922557960796823, -16.46253265017161027, 32.08224293864769550 ) ) ;
#110279=CARTESIAN_POINT ( 'NONE',  ( 15.72974639402176855, 15.80617190586768217, 31.87609039468567929 ) ) ;
#110280=CARTESIAN_POINT ( 'NONE',  ( 13.89961937509977652, -13.97604488694527269, 48.12390960531435979 ) ) ;
#110282=CARTESIAN_POINT ( 'NONE',  ( -19.05341960407611168, -5.049401038298163336, 51.45724293864770260 ) ) ;
#110283=CARTESIAN_POINT ( 'NONE',  ( -18.62759615963270932, 10.81492255796079327, 25.83224293864769194 ) ) ;
#110284=CARTESIAN_POINT ( 'NONE',  ( 18.67979575497194134, -10.72451020669871369, 60.83442372801901854 ) ) ;
#110285=CARTESIAN_POINT ( 'NONE',  ( -19.05341960407611168, -5.049401038298163336, 26.45724293864769550 ) ) ;
#110286=CARTESIAN_POINT ( 'NONE',  ( -10.81492255796078084, -18.62759615963271287, 27.08224293864769550 ) ) ;
#110287=CARTESIAN_POINT ( 'NONE',  ( -14.34966873604972548, 8.224510206698743886, 73.33442372801901854 ) ) ;
#110288=CARTESIAN_POINT ( 'NONE',  ( -18.67979575497193778, 10.72451020669871902, 108.3344237280190185 ) ) ;
#110289=CARTESIAN_POINT ( 'NONE',  ( -14.34966873604972548, 8.224510206698743886, 53.33442372801901854 ) ) ;
#110290=CARTESIAN_POINT ( 'NONE',  ( 0.05219959533909260263, 19.03943276465977164, 94.99890960531436690 ) ) ;
#110291=CARTESIAN_POINT ( 'NONE',  ( 12.06949235617739724, 12.14591786802326823, 36.87609039468568994 ) ) ;
#110292=CARTESIAN_POINT ( 'NONE',  ( 8.314922557961029526, -14.29746914071037800, 20.41775706135234714 ) ) ;
#110293=CARTESIAN_POINT ( 'NONE',  ( 16.52544592524335698, 4.483927247898782831, 91.45942372801901854 ) ) ;
#110294=CARTESIAN_POINT ( 'NONE',  ( -5.719274019375665041, -21.55341960407619695, 59.79275706135234714 ) ) ;
#110295=CARTESIAN_POINT ( 'NONE',  ( 9.474510206698729675, 16.51473224551082808, 112.0844237280190043 ) ) ;
#110296=CARTESIAN_POINT ( 'NONE',  ( -10.81492255796078084, -18.62759615963271287, 107.0822429386476955 ) ) ;
#110297=CARTESIAN_POINT ( 'NONE',  ( 12.14591786802309770, 12.06949235617756955, 104.3739096053143669 ) ) ;
#110298=CARTESIAN_POINT ( 'NONE',  ( 13.97604488694548053, -13.89961937509957401, 105.6260903946856757 ) ) ;
#110299=CARTESIAN_POINT ( 'NONE',  ( 14.34966873604972726, -8.224510206698740333, 85.83442372801901854 ) ) ;
#110301=CARTESIAN_POINT ( 'NONE',  ( -9.564922557961040184, 16.46253265017147172, 77.91775706135234714 ) ) ;
#110302=CARTESIAN_POINT ( 'NONE',  ( -12.06949235617756955, 12.14591786802309770, 40.62390960531435269 ) ) ;
#110303=CARTESIAN_POINT ( 'NONE',  ( -14.34966873604960291, -8.224510206698953496, 46.66557627198102409 ) ) ;
#110304=CARTESIAN_POINT ( 'NONE',  ( 8.314922557960818139, 14.29746914071049879, 109.5822429386476955 ) ) ;
#110305=CARTESIAN_POINT ( 'NONE',  ( 9.564922557961047289, -16.46253265017146816, 50.41775706135233293 ) ) ;
#110306=CARTESIAN_POINT ( 'NONE',  ( -17.05587630539787369, 6.762274262135701264, 90.74180309037315340 ) ) ;
#110307=CARTESIAN_POINT ( 'NONE',  ( -0.05219959533937732626, 21.53943276465977519, 42.50109039468567573 ) ) ;
#110308=CARTESIAN_POINT ( 'NONE',  ( 5.153800228976615827, -19.02544592524334988, 110.2094237280189901 ) ) ;
#110310=CARTESIAN_POINT ( 'NONE',  ( -13.97604488694527625, -13.89961937509977652, 91.87390960531432427 ) ) ;
#110311=CARTESIAN_POINT ( 'NONE',  ( -9.474510206698964154, 16.51473224551069663, 95.41557627198102409 ) ) ;
#110312=CARTESIAN_POINT ( 'NONE',  ( -15.80617190586745835, -15.72974639402198527, 61.87390960531436690 ) ) ;
#110313=CARTESIAN_POINT ( 'NONE',  ( -8.224510206698948167, 14.34966873604960824, 90.41557627198103830 ) ) ;
#110314=CARTESIAN_POINT ( 'NONE',  ( 13.89961937509977652, -13.97604488694527269, 68.12390960531436690 ) ) ;
#110315=CARTESIAN_POINT ( 'NONE',  ( 19.03943276465977164, -0.05219959533909143690, 33.74890960531435979 ) ) ;
#110316=CARTESIAN_POINT ( 'NONE',  ( -10.81492255796105439, 18.62759615963255655, 42.91775706135235424 ) ) ;
#110317=CARTESIAN_POINT ( 'NONE',  ( -10.81492255796105439, 18.62759615963255655, 72.91775706135234714 ) ) ;
#110319=CARTESIAN_POINT ( 'NONE',  ( -14.29746914071037622, -8.314922557961029526, 89.16775706135236135 ) ) ;
#110320=CARTESIAN_POINT ( 'NONE',  ( 5.719274019375673035, 21.55341960407619339, 27.29275706135234358 ) ) ;
#110321=CARTESIAN_POINT ( 'NONE',  ( 5.823673210054444382, -21.52544592524334988, 25.20942372801901854 ) ) ;
#110322=CARTESIAN_POINT ( 'NONE',  ( -9.474510206698720793, -16.51473224551083518, 54.58442372801899722 ) ) ;
#110323=CARTESIAN_POINT ( 'NONE',  ( 13.97604488694527802, 13.89961937509977652, 84.37390960531433848 ) ) ;
#110324=CARTESIAN_POINT ( 'NONE',  ( 0.05219959533937995610, -21.53943276465977519, 85.00109039468568994 ) ) ;
#110325=CARTESIAN_POINT ( 'NONE',  ( -5.823673210054116645, -21.52544592524344225, 82.29057627198103830 ) ) ;
#110326=CARTESIAN_POINT ( 'NONE',  ( -4.483927247898539470, -16.52544592524342804, 47.29057627198103120 ) ) ;
#110327=CARTESIAN_POINT ( 'NONE',  ( -15.80617190586768217, 15.72974639402176855, 103.1260903946856757 ) ) ;
#110328=CARTESIAN_POINT ( 'NONE',  ( 14.34966873604960469, 8.224510206698951720, 79.16557627198103830 ) ) ;
#110329=CARTESIAN_POINT ( 'NONE',  ( 12.14591786802309770, 12.06949235617756955, 114.3739096053143527 ) ) ;
#110330=CARTESIAN_POINT ( 'NONE',  ( 16.46253265017146816, 9.564922557961045513, 76.66775706135234714 ) ) ;
#110331=CARTESIAN_POINT ( 'NONE',  ( -16.55341960407611168, -4.379528057220339221, 36.45724293864768839 ) ) ;
#110332=CARTESIAN_POINT ( 'NONE',  ( -5.823673210054431948, 21.52544592524334988, 87.70942372801901854 ) ) ;
#110333=CARTESIAN_POINT ( 'NONE',  ( -19.03943276465977164, 0.05219959533909376836, 91.24890960531436690 ) ) ;
#110334=CARTESIAN_POINT ( 'NONE',  ( 0.05219959533936267826, -19.03943276465977164, 60.00109039468566863 ) ) ;
#110335=CARTESIAN_POINT ( 'NONE',  ( 15.72974639402199770, -15.80617190586745480, 68.12390960531436690 ) ) ;
#110336=CARTESIAN_POINT ( 'NONE',  ( -10.72451020669870658, -18.67979575497194134, 19.58442372801901143 ) ) ;
#110337=CARTESIAN_POINT ( 'NONE',  ( -8.224510206698735004, -14.34966873604973081, 19.58442372801901143 ) ) ;
#110338=CARTESIAN_POINT ( 'NONE',  ( -14.34966873604972548, 8.224510206698743886, 73.33442372801901854 ) ) ;
#110340=CARTESIAN_POINT ( 'NONE',  ( -21.55341960407619339, 5.719274019375674811, 28.54275706135234358 ) ) ;
#110341=CARTESIAN_POINT ( 'NONE',  ( 12.14591786802309770, 12.06949235617756955, 99.37390960531436690 ) ) ;
#110343=CARTESIAN_POINT ( 'NONE',  ( -14.29746914071037622, -8.314922557961029526, 29.16775706135234003 ) ) ;
#110344=CARTESIAN_POINT ( 'NONE',  ( -21.55341960407610458, -5.719274019375992779, 56.45724293864768839 ) ) ;
#110345=CARTESIAN_POINT ( 'NONE',  ( -16.55341960407617563, 4.379528057220093196, 98.54275706135234714 ) ) ;
#110346=CARTESIAN_POINT ( 'NONE',  ( -4.379528057220086978, -16.55341960407618274, 39.79275706135235424 ) ) ;
#110347=CARTESIAN_POINT ( 'NONE',  ( 5.049401038298161559, -19.05341960407611168, 27.70724293864769550 ) ) ;
#110348=CARTESIAN_POINT ( 'NONE',  ( -8.314922557961024197, 14.29746914071037800, 82.91775706135234714 ) ) ;
#110349=CARTESIAN_POINT ( 'NONE',  ( -13.89961937509957401, -13.97604488694547875, 79.37609039468567573 ) ) ;
#110350=CARTESIAN_POINT ( 'NONE',  ( 15.72974639402199770, -15.80617190586745480, 58.12390960531435979 ) ) ;
#110351=CARTESIAN_POINT ( 'NONE',  ( -12.14591786802326823, 12.06949235617739902, 98.12609039468570415 ) ) ;
#110352=CARTESIAN_POINT ( 'NONE',  ( 15.72974639402176855, 15.80617190586768217, 76.87609039468567573 ) ) ;
#110353=CARTESIAN_POINT ( 'NONE',  ( 0.05219959533907565091, 21.53943276465977519, 54.99890960531435269 ) ) ;
#110354=CARTESIAN_POINT ( 'NONE',  ( -15.72974639402197994, 15.80617190586746368, 45.62390960531436690 ) ) ;
#110356=CARTESIAN_POINT ( 'NONE',  ( -16.55341960407617563, 4.379528057220093196, 78.54275706135236135 ) ) ;
#110357=CARTESIAN_POINT ( 'NONE',  ( -5.823673210054116645, -21.52544592524344225, 52.29057627198102409 ) ) ;
#110359=CARTESIAN_POINT ( 'NONE',  ( 19.05341960407611168, 5.049401038298154454, 98.95724293864766707 ) ) ;
#110361=CARTESIAN_POINT ( 'NONE',  ( -13.97604488694527625, -13.89961937509977652, 21.87390960531435979 ) ) ;
#110362=CARTESIAN_POINT ( 'NONE',  ( -10.72451020669898014, 18.67979575497178502, 65.41557627198102409 ) ) ;
#110363=CARTESIAN_POINT ( 'NONE',  ( -0.05219959533934338120, 16.53943276465976808, 107.5010903946856899 ) ) ;
#110364=CARTESIAN_POINT ( 'NONE',  ( 18.67979575497194134, -10.72451020669871369, 45.83442372801901854 ) ) ;
#110365=CARTESIAN_POINT ( 'NONE',  ( -9.474510206698720793, -16.51473224551083518, 109.5844237280190043 ) ) ;
#110366=CARTESIAN_POINT ( 'NONE',  ( -14.29746914071049879, 8.314922557960819915, 105.8322429386476955 ) ) ;
#110367=CARTESIAN_POINT ( 'NONE',  ( 9.564922557961047289, -16.46253265017146816, 110.4177570613523471 ) ) ;
#110368=CARTESIAN_POINT ( 'NONE',  ( 9.564922557960805705, 16.46253265017160317, 39.58224293864768839 ) ) ;
#110369=DIRECTION ( 'NONE',  ( 0.000000000000000000, 0.000000000000000000, -1.000000000000000000 ) ) ;
#110370=CARTESIAN_POINT ( 'NONE',  ( -19.03943276465977164, 0.05219959533909376836, 91.24890960531436690 ) ) ;
#110371=CARTESIAN_POINT ( 'NONE',  ( -14.34966873604972548, 8.224510206698743886, 78.33442372801901854 ) ) ;
#110372=CARTESIAN_POINT ( 'NONE',  ( 9.474510206698729675, 16.51473224551082808, 82.08442372801899012 ) ) ;
#110373=CARTESIAN_POINT ( 'NONE',  ( -18.67979575497193778, 10.72451020669871902, 103.3344237280190043 ) ) ;
#110374=CARTESIAN_POINT ( 'NONE',  ( -10.72451020669898014, 18.67979575497178502, 60.41557627198102409 ) ) ;
#110375=CARTESIAN_POINT ( 'NONE',  ( -0.05219959533934338120, 16.53943276465976808, 92.50109039468567573 ) ) ;
#110376=CARTESIAN_POINT ( 'NONE',  ( -5.049401038297874678, -19.05341960407617918, 74.79275706135231871 ) ) ;
#110377=CARTESIAN_POINT ( 'NONE',  ( 19.02544592524343514, -5.153800228976328945, 33.54057627198102409 ) ) ;
#110378=CARTESIAN_POINT ( 'NONE',  ( -9.564922557960796823, -16.46253265017161027, 72.08224293864770971 ) ) ;
#110379=CARTESIAN_POINT ( 'NONE',  ( 5.719274019375673035, 21.55341960407619339, 47.29275706135234003 ) ) ;
#110380=CARTESIAN_POINT ( 'NONE',  ( -0.05219959533909027116, -19.03943276465977164, 52.49890960531436690 ) ) ;
#110381=CARTESIAN_POINT ( 'NONE',  ( -9.564922557961040184, 16.46253265017147172, 67.91775706135233293 ) ) ;
#110382=B_SPLINE_CURVE_WITH_KNOTS ( 'NONE', 3,
 ( #1376, #20527, #98344, #21530, #35701, #17561 ),
 .UNSPECIFIED., .F., .F.,
 ( 4, 2, 4 ),
 ( 0.003239945802372225670, 0.003620412082092076995, 0.004000878361811928755 ),
 .UNSPECIFIED. ) ;
#110384=CARTESIAN_POINT ( 'NONE',  ( -9.474510206698964154, 16.51473224551069663, 105.4155762719810383 ) ) ;
#110385=CARTESIAN_POINT ( 'NONE',  ( 4.483927247898545687, 16.52544592524342804, 64.79057627198103830 ) ) ;
#110386=CARTESIAN_POINT ( 'NONE',  ( -15.80617190586745835, -15.72974639402198527, 61.87390960531436690 ) ) ;
#110388=CARTESIAN_POINT ( 'NONE',  ( -19.03943276465977164, -0.05219959533935918106, 23.75109039468566152 ) ) ;
#110390=CARTESIAN_POINT ( 'NONE',  ( -13.97604488694527625, -13.89961937509977652, 66.87390960531436690 ) ) ;
#110391=CARTESIAN_POINT ( 'NONE',  ( 16.51473224551069308, 9.474510206698969483, 74.16557627198103830 ) ) ;
#110392=CARTESIAN_POINT ( 'NONE',  ( 16.52544592524335698, 4.483927247898782831, 51.45942372801901854 ) ) ;
#110393=CARTESIAN_POINT ( 'NONE',  ( 19.50973618000806198, 5.499999999999992895, 37.50000000000000000 ) ) ;
#110395=CARTESIAN_POINT ( 'NONE',  ( -14.29746914071037622, -8.314922557961029526, 94.16775706135237556 ) ) ;
#110397=CARTESIAN_POINT ( 'NONE',  ( -4.483927247898782831, 16.52544592524335698, 62.70942372801902565 ) ) ;
#110398=CARTESIAN_POINT ( 'NONE',  ( -14.34966873604972548, 8.224510206698743886, 43.33442372801901143 ) ) ;
#110399=CARTESIAN_POINT ( 'NONE',  ( -5.049401038298153566, 19.05341960407611168, 55.20724293864769550 ) ) ;
#110401=CARTESIAN_POINT ( 'NONE',  ( 15.80617190586769283, -15.72974639402175789, 55.62609039468568284 ) ) ;
#110402=CARTESIAN_POINT ( 'NONE',  ( 16.46253265017146816, 9.564922557961045513, 66.66775706135233293 ) ) ;
#110403=CARTESIAN_POINT ( 'NONE',  ( -21.52544592524334988, -5.823673210054445271, 108.9594237280190185 ) ) ;
#110404=CARTESIAN_POINT ( 'NONE',  ( 16.46253265017160672, -9.564922557960803928, 33.33224293864770260 ) ) ;
#110405=CARTESIAN_POINT ( 'NONE',  ( 16.19062691409071064, 7.376977991747391883, 22.65583381035920141 ) ) ;
#110406=CARTESIAN_POINT ( 'NONE',  ( 0.05219959533907565091, 21.53943276465977519, 54.99890960531435269 ) ) ;
#110407=CARTESIAN_POINT ( 'NONE',  ( -9.564922557960796823, -16.46253265017161027, 112.0822429386476955 ) ) ;
#110408=CARTESIAN_POINT ( 'NONE',  ( -14.29746914071049879, 8.314922557960819915, 95.83224293864770971 ) ) ;
#110409=CARTESIAN_POINT ( 'NONE',  ( -16.52544592524335698, -4.483927247898792601, 43.95942372801902565 ) ) ;
#110410=CARTESIAN_POINT ( 'NONE',  ( 8.314922557960818139, 14.29746914071049879, 29.58224293864769905 ) ) ;
#110413=CARTESIAN_POINT ( 'NONE',  ( -21.53943276465977519, -0.05219959533937600094, 18.75109039468568639 ) ) ;
#110414=CARTESIAN_POINT ( 'NONE',  ( -4.379528057220328563, 16.55341960407611168, 35.20724293864768839 ) ) ;
#110415=CARTESIAN_POINT ( 'NONE',  ( -16.46253265017160317, 9.564922557960807481, 110.8322429386476955 ) ) ;
#110417=CARTESIAN_POINT ( 'NONE',  ( -13.97604488694547697, 13.89961937509957934, 93.12609039468566152 ) ) ;
#110418=CARTESIAN_POINT ( 'NONE',  ( 9.564922557961047289, -16.46253265017146816, 30.41775706135232937 ) ) ;
#110419=CARTESIAN_POINT ( 'NONE',  ( -8.224510206698948167, 14.34966873604960824, 30.41557627198101699 ) ) ;
#110420=CARTESIAN_POINT ( 'NONE',  ( 15.72974639402199770, -15.80617190586745480, 98.12390960531436690 ) ) ;
#110421=CARTESIAN_POINT ( 'NONE',  ( 21.53943276465977519, -0.05219959533907433946, 53.74890960531437401 ) ) ;
#110422=CARTESIAN_POINT ( 'NONE',  ( 9.474510206698971260, -16.51473224551069308, 77.91557627198103830 ) ) ;
#110423=CARTESIAN_POINT ( 'NONE',  ( 4.379528057220339221, -16.55341960407611168, 47.70724293864770260 ) ) ;
#110424=CARTESIAN_POINT ( 'NONE',  ( -13.89961937509977652, 13.97604488694528158, 90.62390960531432427 ) ) ;
#110426=CARTESIAN_POINT ( 'NONE',  ( 19.35543954521081744, 5.499999999999578115, 57.08901960356452321 ) ) ;
#110427=CARTESIAN_POINT ( 'NONE',  ( 16.51473224551083163, -9.474510206698727899, 45.83442372801900433 ) ) ;
#110428=CARTESIAN_POINT ( 'NONE',  ( 18.62759615963271287, -10.81492255796078972, 88.33224293864769550 ) ) ;
#110429=CARTESIAN_POINT ( 'NONE',  ( -12.14591786802309592, -12.06949235617757132, 96.87390960531436690 ) ) ;
#110430=CARTESIAN_POINT ( 'NONE',  ( 5.719274019375673035, 21.55341960407619339, 32.29275706135235424 ) ) ;
#110432=CARTESIAN_POINT ( 'NONE',  ( 4.483927247898790824, -16.52544592524335698, 105.2094237280190328 ) ) ;
#110433=CARTESIAN_POINT ( 'NONE',  ( -13.97604488694527625, -13.89961937509977652, 31.87390960531435979 ) ) ;
#110434=CARTESIAN_POINT ( 'NONE',  ( -0.05219959533909027116, -19.03943276465977164, 87.49890960531436690 ) ) ;
#110435=CARTESIAN_POINT ( 'NONE',  ( 5.719274019375991003, -21.55341960407610458, 62.70724293864769550 ) ) ;
#110437=CARTESIAN_POINT ( 'NONE',  ( -0.05219959533909027116, -19.03943276465977164, 37.49890960531436690 ) ) ;
#110438=CARTESIAN_POINT ( 'NONE',  ( -16.53943276465976808, 0.05219959533911058130, 41.24890960531435269 ) ) ;
#110439=CARTESIAN_POINT ( 'NONE',  ( -15.80617190586768217, 15.72974639402176855, 78.12609039468570415 ) ) ;
#110441=CARTESIAN_POINT ( 'NONE',  ( -12.14591786802326823, 12.06949235617739902, 63.12609039468568994 ) ) ;
#110442=CARTESIAN_POINT ( 'NONE',  ( -16.46253265017160317, 9.564922557960807481, 50.83224293864770260 ) ) ;
#110443=CARTESIAN_POINT ( 'NONE',  ( -13.89961937509977652, 13.97604488694528158, 65.62390960531436690 ) ) ;
#110444=ORIENTED_EDGE ( 'NONE', *, *, #179839, .T. ) ;
#110445=CARTESIAN_POINT ( 'NONE',  ( 15.80617190586769283, -15.72974639402175789, 105.6260903946856899 ) ) ;
#110446=CARTESIAN_POINT ( 'NONE',  ( 16.52544592524335698, 4.483927247898782831, 81.45942372801900433 ) ) ;
#110447=CARTESIAN_POINT ( 'NONE',  ( -0.05219959533937732626, 21.53943276465977519, 92.50109039468567573 ) ) ;
#110448=CARTESIAN_POINT ( 'NONE',  ( -19.02544592524342804, 5.153800228976336051, 61.04057627198103120 ) ) ;
#110449=CARTESIAN_POINT ( 'NONE',  ( -18.62759615963270932, 10.81492255796079327, 35.83224293864768839 ) ) ;
#110450=CARTESIAN_POINT ( 'NONE',  ( 5.049401038297881783, 19.05341960407617563, 107.2927570613523187 ) ) ;
#110451=CARTESIAN_POINT ( 'NONE',  ( -21.53943276465977519, -0.05219959533937600094, 78.75109039468568994 ) ) ;
#110452=CARTESIAN_POINT ( 'NONE',  ( 14.34966873604972726, -8.224510206698740333, 50.83442372801901143 ) ) ;
#110453=CARTESIAN_POINT ( 'NONE',  ( 5.719274019375991003, -21.55341960407610458, 97.70724293864772392 ) ) ;
#110454=CARTESIAN_POINT ( 'NONE',  ( 0.05219959533936267826, -19.03943276465977164, 105.0010903946856615 ) ) ;
#110455=CARTESIAN_POINT ( 'NONE',  ( 5.049401038298161559, -19.05341960407611168, 82.70724293864770971 ) ) ;
#110456=CARTESIAN_POINT ( 'NONE',  ( 9.564922557961047289, -16.46253265017146816, 105.4177570613523471 ) ) ;
#110457=CARTESIAN_POINT ( 'NONE',  ( -16.53943276465976808, -0.05219959533934237506, 18.75109039468568639 ) ) ;
#110458=CARTESIAN_POINT ( 'NONE',  ( 8.224510206698953496, -14.34966873604960469, 67.91557627198102409 ) ) ;
#110459=CARTESIAN_POINT ( 'NONE',  ( -4.379528057220086978, -16.55341960407618274, 69.79275706135234714 ) ) ;
#110460=CARTESIAN_POINT ( 'NONE',  ( 21.55341960407610458, 5.719274019375980345, 113.9572429386477239 ) ) ;
#110461=CARTESIAN_POINT ( 'NONE',  ( 13.89961937509977652, -13.97604488694527269, 58.12390960531436690 ) ) ;
#110462=CARTESIAN_POINT ( 'NONE',  ( 13.97604488694527802, 13.89961937509977652, 64.37390960531436690 ) ) ;
#110463=CARTESIAN_POINT ( 'NONE',  ( 12.06949235617739724, 12.14591786802326823, 66.87609039468568994 ) ) ;
#110466=CARTESIAN_POINT ( 'NONE',  ( 15.72974639402176855, 15.80617190586768217, 106.8760903946856899 ) ) ;
#110467=CARTESIAN_POINT ( 'NONE',  ( 5.153800228976335163, 19.02544592524342804, 39.79057627198100988 ) ) ;
#110468=ORIENTED_EDGE ( 'NONE', *, *, #131008, .T. ) ;
#110469=CARTESIAN_POINT ( 'NONE',  ( -8.314922557961024197, 14.29746914071037800, 32.91775706135234714 ) ) ;
#110470=CARTESIAN_POINT ( 'NONE',  ( 19.03943276465977164, 0.05219959533936151252, 41.25109039468566152 ) ) ;
#110471=CARTESIAN_POINT ( 'NONE',  ( -16.55341960407617563, 4.379528057220093196, 43.54275706135235424 ) ) ;
#110472=CARTESIAN_POINT ( 'NONE',  ( 16.51473224551069308, 9.474510206698969483, 44.16557627198103120 ) ) ;
#110473=CARTESIAN_POINT ( 'NONE',  ( 19.03943276465977164, -0.05219959533909143690, 63.74890960531435979 ) ) ;
#110474=CARTESIAN_POINT ( 'NONE',  ( 15.72974639402199770, -15.80617190586745480, 83.12390960531436690 ) ) ;
#110475=CARTESIAN_POINT ( 'NONE',  ( 19.05341960407611168, 5.049401038298154454, 78.95724293864769550 ) ) ;
#110476=CARTESIAN_POINT ( 'NONE',  ( -9.564922557960796823, -16.46253265017161027, 107.0822429386476955 ) ) ;
#110477=CARTESIAN_POINT ( 'NONE',  ( -9.564922557960796823, -16.46253265017161027, 52.08224293864768839 ) ) ;
#110479=CARTESIAN_POINT ( 'NONE',  ( 9.564922557961047289, -16.46253265017146816, 100.4177570613523329 ) ) ;
#110480=CARTESIAN_POINT ( 'NONE',  ( 10.72451020669898902, -18.67979575497178502, 77.91557627198102409 ) ) ;
#110481=CARTESIAN_POINT ( 'NONE',  ( -5.153800228976607833, 19.02544592524334988, 22.70942372801899012 ) ) ;
#110482=CARTESIAN_POINT ( 'NONE',  ( -0.05219959533910754901, -16.53943276465976808, 62.49890960531436690 ) ) ;
#110483=CARTESIAN_POINT ( 'NONE',  ( -5.823673210054431948, 21.52544592524334988, 87.70942372801901854 ) ) ;
#110484=CARTESIAN_POINT ( 'NONE',  ( -4.379528057220328563, 16.55341960407611168, 115.2072429386476955 ) ) ;
#110485=CARTESIAN_POINT ( 'NONE',  ( 12.06949235617757843, -12.14591786802309237, 33.12390960531435979 ) ) ;
#110486=CARTESIAN_POINT ( 'NONE',  ( 5.823673210054444382, -21.52544592524334988, 95.20942372801903275 ) ) ;
#110487=CARTESIAN_POINT ( 'NONE',  ( -5.153800228976328057, -19.02544592524343514, 82.29057627198103830 ) ) ;
#110489=CARTESIAN_POINT ( 'NONE',  ( 10.72451020669871369, 18.67979575497193778, 47.08442372801901854 ) ) ;
#110490=CARTESIAN_POINT ( 'NONE',  ( -16.51473224551069308, -9.474510206698971260, 76.66557627198103830 ) ) ;
#110491=CARTESIAN_POINT ( 'NONE',  ( -16.53943276465976808, 0.05219959533911058130, 91.24890960531436690 ) ) ;
#110492=CARTESIAN_POINT ( 'NONE',  ( -12.06949235617756955, 12.14591786802309770, 65.62390960531436690 ) ) ;
#110493=CARTESIAN_POINT ( 'NONE',  ( -21.55341960407610458, -5.719274019375992779, 71.45724293864769550 ) ) ;
#110494=CARTESIAN_POINT ( 'NONE',  ( 5.153800228976335163, 19.02544592524342804, 69.79057627198103830 ) ) ;
#110495=CARTESIAN_POINT ( 'NONE',  ( 18.62759615963271287, -10.81492255796078972, 83.33224293864769550 ) ) ;
#110496=CARTESIAN_POINT ( 'NONE',  ( 19.02544592524334988, 5.153800228976608722, 81.45942372801897591 ) ) ;
#110497=CARTESIAN_POINT ( 'NONE',  ( -16.51473224551082808, 9.474510206698731452, 33.33442372801899722 ) ) ;
#110498=CARTESIAN_POINT ( 'NONE',  ( -12.06949235617756955, 12.14591786802309770, 70.62390960531436690 ) ) ;
#110499=CARTESIAN_POINT ( 'NONE',  ( -21.52544592524343514, 5.823673210054127303, 56.04057627198102409 ) ) ;
#110501=CARTESIAN_POINT ( 'NONE',  ( 8.314922557961029526, -14.29746914071037800, 105.4177570613523613 ) ) ;
#110503=CARTESIAN_POINT ( 'NONE',  ( -19.05341960407617563, 5.049401038297882671, 103.5427570613523329 ) ) ;
#110505=CARTESIAN_POINT ( 'NONE',  ( 16.53943276465976808, -0.05219959533910856209, 78.74890960531436690 ) ) ;
#110506=CARTESIAN_POINT ( 'NONE',  ( -17.50000000000147793, 3.202012800152213678, 34.92822416027257759 ) ) ;
#110507=CARTESIAN_POINT ( 'NONE',  ( -19.02544592524342804, 5.153800228976336051, 71.04057627198099567 ) ) ;
#110508=CARTESIAN_POINT ( 'NONE',  ( 19.02544592524343514, -5.153800228976328945, 28.54057627198102409 ) ) ;
#110509=CARTESIAN_POINT ( 'NONE',  ( -0.05219959533910754901, -16.53943276465976808, 57.49890960531435979 ) ) ;
#110510=CARTESIAN_POINT ( 'NONE',  ( -19.02544592524342804, 5.153800228976336051, 106.0405762719810241 ) ) ;
#110511=CARTESIAN_POINT ( 'NONE',  ( 0.05219959533936267826, -19.03943276465977164, 90.00109039468567573 ) ) ;
#110512=CARTESIAN_POINT ( 'NONE',  ( -5.049401038298153566, 19.05341960407611168, 60.20724293864768129 ) ) ;
#110513=CARTESIAN_POINT ( 'NONE',  ( -16.53943276465976808, -0.05219959533934237506, 23.75109039468567929 ) ) ;
#110514=CARTESIAN_POINT ( 'NONE',  ( 9.474510206698971260, -16.51473224551069308, 82.91557627198103830 ) ) ;
#110515=CARTESIAN_POINT ( 'NONE',  ( 10.72451020669898902, -18.67979575497178502, 62.91557627198102409 ) ) ;
#110516=CARTESIAN_POINT ( 'NONE',  ( -16.55341960407617563, 4.379528057220093196, 58.54275706135235424 ) ) ;
#110517=CARTESIAN_POINT ( 'NONE',  ( 19.02544592524335343, 5.153800228976608722, 111.4594237280190043 ) ) ;
#110518=CARTESIAN_POINT ( 'NONE',  ( 13.89961937509977652, -13.97604488694527269, 68.12390960531436690 ) ) ;
#110519=CARTESIAN_POINT ( 'NONE',  ( 21.55341960407610458, 5.719274019375980345, 63.95724293864770260 ) ) ;
#110520=CARTESIAN_POINT ( 'NONE',  ( 16.51473224551083163, -9.474510206698727899, 90.83442372801900433 ) ) ;
#110521=CARTESIAN_POINT ( 'NONE',  ( -12.06949235617756955, 12.14591786802309770, 25.62390960531435624 ) ) ;
#110522=CARTESIAN_POINT ( 'NONE',  ( -15.80617190586768217, 15.72974639402176855, 48.12609039468568284 ) ) ;
#110524=CARTESIAN_POINT ( 'NONE',  ( 16.55341960407618274, -4.379528057220086978, 71.04275706135234714 ) ) ;
#110525=CARTESIAN_POINT ( 'NONE',  ( 9.474510206698971260, -16.51473224551069308, 102.9155762719810241 ) ) ;
#110526=CARTESIAN_POINT ( 'NONE',  ( 19.25663599770059164, -5.499999999999425349, 41.49419308057198208 ) ) ;
#110527=CARTESIAN_POINT ( 'NONE',  ( -16.88567814943160883, -6.947325034625784212, 36.29001122652586986 ) ) ;
#110528=CARTESIAN_POINT ( 'NONE',  ( 0.05219959533934541429, -16.53943276465976808, 100.0010903946857042 ) ) ;
#110529=CARTESIAN_POINT ( 'NONE',  ( -4.379528057220086978, -16.55341960407618274, 34.79275706135235424 ) ) ;
#110530=CARTESIAN_POINT ( 'NONE',  ( 5.153800228976335163, 19.02544592524342804, 49.79057627198100988 ) ) ;
#110531=CARTESIAN_POINT ( 'NONE',  ( 16.46253265017160672, -9.564922557960803928, 53.33224293864768839 ) ) ;
#110532=CARTESIAN_POINT ( 'NONE',  ( 5.049401038298161559, -19.05341960407611168, 62.70724293864769550 ) ) ;
#110533=CARTESIAN_POINT ( 'NONE',  ( 21.52544592524334988, 5.823673210054432836, 56.45942372801902565 ) ) ;
#110534=CARTESIAN_POINT ( 'NONE',  ( 8.224510206698742110, 14.34966873604972548, 57.08442372801901854 ) ) ;
#110535=CARTESIAN_POINT ( 'NONE',  ( -8.224510206698948167, 14.34966873604960824, 35.41557627198102409 ) ) ;
#110536=CARTESIAN_POINT ( 'NONE',  ( 19.05341960407611168, 5.049401038298154454, 38.95724293864767418 ) ) ;
#110537=CARTESIAN_POINT ( 'NONE',  ( 13.97604488694527802, 13.89961937509977652, 39.37390960531435269 ) ) ;
#110538=CARTESIAN_POINT ( 'NONE',  ( 12.06949235617739724, 12.14591786802326823, 26.87609039468567218 ) ) ;
#110539=CARTESIAN_POINT ( 'NONE',  ( -5.153800228976607833, 19.02544592524334988, 87.70942372801897591 ) ) ;
#110540=CARTESIAN_POINT ( 'NONE',  ( 16.52544592524342804, -4.483927247898539470, 88.54057627198103830 ) ) ;
#110541=CARTESIAN_POINT ( 'NONE',  ( -19.05341960407611168, -5.049401038298163336, 46.45724293864768129 ) ) ;
#110542=CARTESIAN_POINT ( 'NONE',  ( -13.97604488694547697, 13.89961937509957934, 88.12609039468563310 ) ) ;
#110543=CARTESIAN_POINT ( 'NONE',  ( 17.40805194822031154, -6.112264579159333522, 93.33371272510611050 ) ) ;
#110544=CARTESIAN_POINT ( 'NONE',  ( 21.53943276465977519, 0.05219959533937863772, 71.25109039468568994 ) ) ;
#110545=CARTESIAN_POINT ( 'NONE',  ( 8.224510206698742110, 14.34966873604972548, 57.08442372801901854 ) ) ;
#110547=CARTESIAN_POINT ( 'NONE',  ( 15.80617190586746368, 15.72974639402197994, 54.37390960531435979 ) ) ;
#110548=CARTESIAN_POINT ( 'NONE',  ( 0.05219959533934541429, -16.53943276465976808, 40.00109039468567573 ) ) ;
#110549=CARTESIAN_POINT ( 'NONE',  ( -13.97604488694527625, -13.89961937509977830, 21.87390960531435979 ) ) ;
#110550=CARTESIAN_POINT ( 'NONE',  ( -16.51473224551082808, 9.474510206698731452, 33.33442372801899722 ) ) ;
#110552=CARTESIAN_POINT ( 'NONE',  ( -19.05341960407611168, -5.049401038298163336, 56.45724293864768129 ) ) ;
#110554=CARTESIAN_POINT ( 'NONE',  ( -19.03943276465977164, 0.05219959533909376836, 66.24890960531436690 ) ) ;
#110556=CARTESIAN_POINT ( 'NONE',  ( 10.72451020669871369, 18.67979575497193778, 112.0844237280190185 ) ) ;
#110557=CARTESIAN_POINT ( 'NONE',  ( 4.379528057220339221, -16.55341960407611168, 37.70724293864769550 ) ) ;
#110558=CARTESIAN_POINT ( 'NONE',  ( 13.97604488694527802, 13.89961937509977652, 39.37390960531435269 ) ) ;
#110559=CARTESIAN_POINT ( 'NONE',  ( 5.153800228976335163, 19.02544592524342804, 99.79057627198102409 ) ) ;
#110560=CARTESIAN_POINT ( 'NONE',  ( 10.72451020669871369, 18.67979575497193778, 67.08442372801901854 ) ) ;
#110561=CARTESIAN_POINT ( 'NONE',  ( -19.03943276465977164, 0.05219959533909376836, 46.24890960531435979 ) ) ;
#110562=CARTESIAN_POINT ( 'NONE',  ( -18.62759615963255300, -10.81492255796106328, 64.16775706135234714 ) ) ;
#110563=CARTESIAN_POINT ( 'NONE',  ( 5.719274019375991003, -21.55341960407610458, 22.70724293864769194 ) ) ;
#110564=CARTESIAN_POINT ( 'NONE',  ( -19.02544592524342804, 5.153800228976336051, 31.04057627198102409 ) ) ;
#110565=CARTESIAN_POINT ( 'NONE',  ( 21.55341960407619695, -5.719274019375665929, 31.04275706135234714 ) ) ;
#110566=CARTESIAN_POINT ( 'NONE',  ( 9.564922557961047289, -16.46253265017146816, 50.41775706135233293 ) ) ;
#110567=CARTESIAN_POINT ( 'NONE',  ( 9.564922557960805705, 16.46253265017160317, 24.58224293864769194 ) ) ;
#110568=CARTESIAN_POINT ( 'NONE',  ( -13.97604488694527625, -13.89961937509977652, 61.87390960531435979 ) ) ;
#110569=CARTESIAN_POINT ( 'NONE',  ( -5.049401038297874678, -19.05341960407617918, 104.7927570613523471 ) ) ;
#110570=CARTESIAN_POINT ( 'NONE',  ( 4.483927247898545687, 16.52544592524342804, 69.79057627198102409 ) ) ;
#110571=CARTESIAN_POINT ( 'NONE',  ( -5.823673210054116645, -21.52544592524344225, 37.29057627198102409 ) ) ;
#110572=CARTESIAN_POINT ( 'NONE',  ( -13.89961937509957401, -13.97604488694547875, 104.3760903946856757 ) ) ;
#110573=CARTESIAN_POINT ( 'NONE',  ( -18.67979575497178146, -10.72451020669898902, 101.6655762719810383 ) ) ;
#110574=CARTESIAN_POINT ( 'NONE',  ( -21.52544592524334988, -5.823673210054445271, 53.95942372801900433 ) ) ;
#110575=CARTESIAN_POINT ( 'NONE',  ( -4.483927247898782831, 16.52544592524335698, 52.70942372801902565 ) ) ;
#110576=CARTESIAN_POINT ( 'NONE',  ( -8.224510206698735004, -14.34966873604973081, 59.58442372801901854 ) ) ;
#110577=CARTESIAN_POINT ( 'NONE',  ( 5.719274019375991003, -21.55341960407610458, 62.70724293864769550 ) ) ;
#110578=CARTESIAN_POINT ( 'NONE',  ( -9.564922557960796823, -16.46253265017161027, 42.08224293864769550 ) ) ;
#110579=CARTESIAN_POINT ( 'NONE',  ( -14.29746914071037622, -8.314922557961029526, 74.16775706135231871 ) ) ;
#110580=CARTESIAN_POINT ( 'NONE',  ( -15.80617190586745835, -15.72974639402198527, 101.8739096053143811 ) ) ;
#110581=CARTESIAN_POINT ( 'NONE',  ( -16.52544592524342804, 4.483927247898546575, 51.04057627198103120 ) ) ;
#110582=CARTESIAN_POINT ( 'NONE',  ( 19.05341960407611168, 5.049401038298154454, 78.95724293864769550 ) ) ;
#110583=CARTESIAN_POINT ( 'NONE',  ( 12.14591786802327356, -12.06949235617739191, 75.62609039468567573 ) ) ;
#110584=CARTESIAN_POINT ( 'NONE',  ( 9.474510206698729675, 16.51473224551082808, 112.0844237280190043 ) ) ;
#110585=CARTESIAN_POINT ( 'NONE',  ( -18.62759615963270932, 10.81492255796079327, 105.8322429386476955 ) ) ;
#110586=CARTESIAN_POINT ( 'NONE',  ( 16.52544592524342804, -4.483927247898539470, 38.54057627198103120 ) ) ;
#110588=CARTESIAN_POINT ( 'NONE',  ( 19.49149378614659511, -5.499999999999668709, 91.93757513605362419 ) ) ;
#110589=CARTESIAN_POINT ( 'NONE',  ( -21.52544592524343514, 5.823673210054127303, 91.04057627198103830 ) ) ;
#110590=CARTESIAN_POINT ( 'NONE',  ( -0.05219959533910754901, -16.53943276465976808, 22.49890960531436335 ) ) ;
#110591=ORIENTED_EDGE ( 'NONE', *, *, #155903, .T. ) ;
#110592=CARTESIAN_POINT ( 'NONE',  ( -17.31747979337947996, -6.344076630961018815, 56.37944868065183357 ) ) ;
#110593=CARTESIAN_POINT ( 'NONE',  ( 21.52544592524344225, -5.823673210054117533, 98.54057627198105251 ) ) ;
#110594=CARTESIAN_POINT ( 'NONE',  ( 16.46253265017160672, -9.564922557960803928, 113.3322429386476955 ) ) ;
#110595=CARTESIAN_POINT ( 'NONE',  ( -10.72451020669870658, -18.67979575497194134, 24.58442372801901499 ) ) ;
#110596=CARTESIAN_POINT ( 'NONE',  ( 12.14591786802309770, 12.06949235617756955, 54.37390960531435979 ) ) ;
#110597=CARTESIAN_POINT ( 'NONE',  ( 8.314922557961029526, -14.29746914071037800, 45.41775706135234003 ) ) ;
#110598=CARTESIAN_POINT ( 'NONE',  ( 16.51473224551069308, 9.474510206698969483, 59.16557627198102409 ) ) ;
#110599=CARTESIAN_POINT ( 'NONE',  ( 5.049401038297881783, 19.05341960407617563, 52.29275706135234003 ) ) ;
#110600=CARTESIAN_POINT ( 'NONE',  ( -19.02544592524342804, 5.153800228976336051, 81.04057627198103830 ) ) ;
#110601=CARTESIAN_POINT ( 'NONE',  ( -10.81492255796078084, -18.62759615963271287, 32.08224293864769550 ) ) ;
#110603=CARTESIAN_POINT ( 'NONE',  ( 0.05219959533934541429, -16.53943276465976808, 25.00109039468567218 ) ) ;
#110604=CARTESIAN_POINT ( 'NONE',  ( -19.05341960407617563, 5.049401038297882671, 68.54275706135230450 ) ) ;
#110605=CARTESIAN_POINT ( 'NONE',  ( -18.62759615963270932, 10.81492255796079327, 100.8322429386477097 ) ) ;
#110606=CARTESIAN_POINT ( 'NONE',  ( 8.314922557960818139, 14.29746914071049879, 39.58224293864769550 ) ) ;
#110607=CARTESIAN_POINT ( 'NONE',  ( 19.05341960407611168, 5.049401038298154454, 78.95724293864769550 ) ) ;
#110608=CARTESIAN_POINT ( 'NONE',  ( 10.72451020669898902, -18.67979575497178502, 62.91557627198102409 ) ) ;
#110609=CARTESIAN_POINT ( 'NONE',  ( -21.52544592524343514, 5.823673210054127303, 101.0405762719810383 ) ) ;
#110610=CARTESIAN_POINT ( 'NONE',  ( 16.52544592524335698, 4.483927247898782831, 21.45942372801901499 ) ) ;
#110612=CARTESIAN_POINT ( 'NONE',  ( 10.81492255796078972, 18.62759615963270932, 24.58224293864768839 ) ) ;
#110613=CARTESIAN_POINT ( 'NONE',  ( 10.72451020669871369, 18.67979575497193778, 87.08442372801901854 ) ) ;
#110614=CARTESIAN_POINT ( 'NONE',  ( 19.03943276465977164, -0.05219959533909143690, 93.74890960531435269 ) ) ;
#110615=CARTESIAN_POINT ( 'NONE',  ( -19.05341960407611168, -5.049401038298163336, 31.45724293864769550 ) ) ;
#110616=CARTESIAN_POINT ( 'NONE',  ( 19.03943276465977164, -0.05219959533909143690, 78.74890960531436690 ) ) ;
#110617=CARTESIAN_POINT ( 'NONE',  ( -0.05219959533910754901, -16.53943276465976808, 107.4989096053143669 ) ) ;
#110618=CARTESIAN_POINT ( 'NONE',  ( -13.97604488694527625, -13.89961937509977652, 61.87390960531435979 ) ) ;
#110619=CARTESIAN_POINT ( 'NONE',  ( 5.049401038297881783, 19.05341960407617563, 112.2927570613523471 ) ) ;
#110620=CARTESIAN_POINT ( 'NONE',  ( -17.59860650958993844, 7.585241751806885979, 43.42337014262493256 ) ) ;
#110621=CARTESIAN_POINT ( 'NONE',  ( 19.02544592524343514, -5.153800228976328945, 68.54057627198103830 ) ) ;
#110622=CARTESIAN_POINT ( 'NONE',  ( 5.719274019375673035, 21.55341960407619339, 102.2927570613523613 ) ) ;
#110623=CARTESIAN_POINT ( 'NONE',  ( 0.05219959533909260263, 19.03943276465977164, 109.9989096053143669 ) ) ;
#110624=CARTESIAN_POINT ( 'NONE',  ( -4.483927247898782831, 16.52544592524335698, 97.70942372801904696 ) ) ;
#110627=CARTESIAN_POINT ( 'NONE',  ( -5.153800228976607833, 19.02544592524334988, 72.70942372801900433 ) ) ;
#110628=CARTESIAN_POINT ( 'NONE',  ( -19.03943276465977164, -0.05219959533935918106, 23.75109039468566152 ) ) ;
#110630=CARTESIAN_POINT ( 'NONE',  ( 9.564922557960805705, 16.46253265017160317, 24.58224293864769194 ) ) ;
#110631=CARTESIAN_POINT ( 'NONE',  ( 16.55341960407611168, 4.379528057220329451, 33.95724293864769550 ) ) ;
#110633=CARTESIAN_POINT ( 'NONE',  ( -14.34966873604972548, 8.224510206698743886, 108.3344237280190185 ) ) ;
#110635=CARTESIAN_POINT ( 'NONE',  ( -12.06949235617739369, -12.14591786802326823, 84.37609039468570415 ) ) ;
#110636=CARTESIAN_POINT ( 'NONE',  ( 19.02544592524343514, -5.153800228976328945, 33.54057627198102409 ) ) ;
#110637=CARTESIAN_POINT ( 'NONE',  ( -15.80617190586768217, 15.72974639402176855, 98.12609039468570415 ) ) ;
#110638=CARTESIAN_POINT ( 'NONE',  ( -13.89961937509957401, -13.97604488694547875, 99.37609039468567573 ) ) ;
#110639=CARTESIAN_POINT ( 'NONE',  ( 21.52544592524334988, 5.823673210054432836, 81.45942372801900433 ) ) ;
#110640=CARTESIAN_POINT ( 'NONE',  ( -13.97604488694547697, 13.89961937509957934, 53.12609039468565442 ) ) ;
#110641=CARTESIAN_POINT ( 'NONE',  ( 5.153800228976335163, 19.02544592524342804, 74.79057627198103830 ) ) ;
#110642=CARTESIAN_POINT ( 'NONE',  ( 5.153800228976335163, 19.02544592524342804, 64.79057627198100988 ) ) ;
#110643=CARTESIAN_POINT ( 'NONE',  ( 17.12812012977027010, 6.668231424565943755, 73.85948759323143520 ) ) ;
#110644=CARTESIAN_POINT ( 'NONE',  ( 12.14591786802309770, 12.06949235617756955, 64.37390960531435269 ) ) ;
#110645=CARTESIAN_POINT ( 'NONE',  ( -10.81492255796078084, -18.62759615963271287, 62.08224293864769550 ) ) ;
#110646=CARTESIAN_POINT ( 'NONE',  ( -5.049401038298153566, 19.05341960407611168, 50.20724293864770260 ) ) ;
#110647=CARTESIAN_POINT ( 'NONE',  ( 15.72974639402199770, -15.80617190586745480, 83.12390960531436690 ) ) ;
#110648=CARTESIAN_POINT ( 'NONE',  ( 8.314922557961029526, -14.29746914071037800, 80.41775706135234714 ) ) ;
#110650=CARTESIAN_POINT ( 'NONE',  ( -9.564922557960796823, -16.46253265017161027, 52.08224293864768839 ) ) ;
#110652=CARTESIAN_POINT ( 'NONE',  ( -14.34966873604960291, -8.224510206698953496, 76.66557627198103830 ) ) ;
#110654=CARTESIAN_POINT ( 'NONE',  ( 5.049401038298161559, -19.05341960407611168, 52.70724293864767418 ) ) ;
#110655=CARTESIAN_POINT ( 'NONE',  ( -12.06949235617756955, 12.14591786802309770, 115.6239096053143669 ) ) ;
#110656=CARTESIAN_POINT ( 'NONE',  ( 5.049401038297881783, 19.05341960407617563, 72.29275706135234714 ) ) ;
#110657=CARTESIAN_POINT ( 'NONE',  ( 4.483927247898545687, 16.52544592524342804, 74.79057627198105251 ) ) ;
#110658=CARTESIAN_POINT ( 'NONE',  ( 5.719274019375673035, 21.55341960407619339, 42.29275706135235424 ) ) ;
#110659=CARTESIAN_POINT ( 'NONE',  ( 16.46253265017160672, -9.564922557960803928, 33.33224293864770260 ) ) ;
#110660=CARTESIAN_POINT ( 'NONE',  ( -15.72974639402197994, 15.80617190586746368, 105.6239096053143669 ) ) ;
#110661=CARTESIAN_POINT ( 'NONE',  ( 0.05219959533909260263, 19.03943276465977164, 114.9989096053143669 ) ) ;
#110662=CARTESIAN_POINT ( 'NONE',  ( -4.483927247898539470, -16.52544592524342804, 82.29057627198103830 ) ) ;
#110664=CARTESIAN_POINT ( 'NONE',  ( -9.474510206698964154, 16.51473224551069663, 50.41557627198102409 ) ) ;
#110666=CARTESIAN_POINT ( 'NONE',  ( -19.03943276465977164, -0.05219959533935918106, 83.75109039468567573 ) ) ;
#110667=CARTESIAN_POINT ( 'NONE',  ( 0.05219959533937995610, -21.53943276465977519, 30.00109039468568284 ) ) ;
#110668=CARTESIAN_POINT ( 'NONE',  ( 5.153800228976335163, 19.02544592524342804, 74.79057627198103830 ) ) ;
#110669=CARTESIAN_POINT ( 'NONE',  ( 19.02544592524334988, 5.153800228976608722, 51.45942372801900433 ) ) ;
#110670=CARTESIAN_POINT ( 'NONE',  ( 19.03943276465977164, -0.05219959533909143690, 43.74890960531435979 ) ) ;
#110671=CARTESIAN_POINT ( 'NONE',  ( 8.314922557960818139, 14.29746914071049879, 64.58224293864769550 ) ) ;
#110672=CARTESIAN_POINT ( 'NONE',  ( -12.14591786802309592, -12.06949235617757132, 71.87390960531438111 ) ) ;
#110673=CARTESIAN_POINT ( 'NONE',  ( -13.97604488694527625, -13.89961937509977652, 71.87390960531433848 ) ) ;
#110674=CARTESIAN_POINT ( 'NONE',  ( -21.52544592524343514, 5.823673210054127303, 101.0405762719810383 ) ) ;
#110675=CARTESIAN_POINT ( 'NONE',  ( 5.153800228976335163, 19.02544592524342804, 69.79057627198103830 ) ) ;
#110676=CARTESIAN_POINT ( 'NONE',  ( -0.05219959533937732626, 21.53943276465977519, 107.5010903946856899 ) ) ;
#110677=CARTESIAN_POINT ( 'NONE',  ( 16.51473224551069308, 9.474510206698969483, 39.16557627198103120 ) ) ;
#110678=CARTESIAN_POINT ( 'NONE',  ( 12.06949235617739724, 12.14591786802326823, 106.8760903946856899 ) ) ;
#110679=CARTESIAN_POINT ( 'NONE',  ( -4.483927247898539470, -16.52544592524342804, 92.29057627198103830 ) ) ;
#110680=CARTESIAN_POINT ( 'NONE',  ( 9.474510206698729675, 16.51473224551082808, 102.0844237280190043 ) ) ;
#110681=EDGE_LOOP ( 'NONE', ( #183357, #52720, #105188, #169041 ) ) ;
#110682=CARTESIAN_POINT ( 'NONE',  ( 15.72974639402176855, 15.80617190586768217, 36.87609039468568994 ) ) ;
#110683=CARTESIAN_POINT ( 'NONE',  ( -13.97604488694547697, 13.89961937509957934, 53.12609039468565442 ) ) ;
#110684=CARTESIAN_POINT ( 'NONE',  ( -16.52544592524335698, -4.483927247898792601, 108.9594237280190185 ) ) ;
#110685=CARTESIAN_POINT ( 'NONE',  ( -5.823673210054116645, -21.52544592524344225, 67.29057627198103830 ) ) ;
#110686=CARTESIAN_POINT ( 'NONE',  ( 13.89961937509977652, -13.97604488694527269, 108.1239096053143669 ) ) ;
#110687=CARTESIAN_POINT ( 'NONE',  ( -4.483927247898539470, -16.52544592524342804, 52.29057627198102409 ) ) ;
#110688=CARTESIAN_POINT ( 'NONE',  ( -19.03943276465977164, 0.05219959533909376836, 26.24890960531435624 ) ) ;
#110689=CARTESIAN_POINT ( 'NONE',  ( -5.049401038298153566, 19.05341960407611168, 40.20724293864768839 ) ) ;
#110690=CARTESIAN_POINT ( 'NONE',  ( 19.02544592524334988, 5.153800228976608722, 26.45942372801899722 ) ) ;
#110691=CARTESIAN_POINT ( 'NONE',  ( 14.34966873604972726, -8.224510206698740333, 95.83442372801903275 ) ) ;
#110692=CARTESIAN_POINT ( 'NONE',  ( 21.55341960407619695, -5.719274019375665929, 41.04275706135236135 ) ) ;
#110693=CARTESIAN_POINT ( 'NONE',  ( 14.29746914071037800, 8.314922557961029526, 41.66775706135235424 ) ) ;
#110694=CARTESIAN_POINT ( 'NONE',  ( -5.049401038298153566, 19.05341960407611168, 115.2072429386477097 ) ) ;
#110695=CARTESIAN_POINT ( 'NONE',  ( -13.97604488694527625, -13.89961937509977652, 56.87390960531434558 ) ) ;
#110696=CARTESIAN_POINT ( 'NONE',  ( -18.67979575497193778, 10.72451020669871902, 98.33442372801901854 ) ) ;
#110697=CARTESIAN_POINT ( 'NONE',  ( -19.05341960407611168, -5.049401038298163336, 76.45724293864769550 ) ) ;
#110698=CARTESIAN_POINT ( 'NONE',  ( 4.379528057220092307, 16.55341960407617563, 67.29275706135234714 ) ) ;
#110699=CARTESIAN_POINT ( 'NONE',  ( -4.483927247898539470, -16.52544592524342804, 102.2905762719810383 ) ) ;
#110700=CARTESIAN_POINT ( 'NONE',  ( -16.55341960407617563, 4.379528057220093196, 113.5427570613523756 ) ) ;
#110702=CARTESIAN_POINT ( 'NONE',  ( 10.81492255796106328, -18.62759615963255655, 70.41775706135236135 ) ) ;
#110703=CARTESIAN_POINT ( 'NONE',  ( -5.049401038298153566, 19.05341960407611168, 85.20724293864766707 ) ) ;
#110704=CARTESIAN_POINT ( 'NONE',  ( 9.564922557960805705, 16.46253265017160317, 79.58224293864769550 ) ) ;
#110705=CARTESIAN_POINT ( 'NONE',  ( -5.153800228976328057, -19.02544592524343514, 112.2905762719810099 ) ) ;
#110706=CARTESIAN_POINT ( 'NONE',  ( 12.14591786802309770, 12.06949235617756955, 64.37390960531435269 ) ) ;
#110707=CARTESIAN_POINT ( 'NONE',  ( -16.53943276465976808, -0.05219959533934237506, 108.7510903946857042 ) ) ;
#110708=EDGE_LOOP ( 'NONE', ( #47010, #135059, #44844, #127580 ) ) ;
#110709=CARTESIAN_POINT ( 'NONE',  ( 14.29746914071049879, -8.314922557960816363, 33.33224293864769550 ) ) ;
#110710=CARTESIAN_POINT ( 'NONE',  ( 12.06949235617739724, 12.14591786802326823, 36.87609039468568994 ) ) ;
#110712=CARTESIAN_POINT ( 'NONE',  ( -19.05341960407617563, 5.049401038297882671, 33.54275706135231871 ) ) ;
#110713=CARTESIAN_POINT ( 'NONE',  ( 13.97604488694527802, 13.89961937509977652, 74.37390960531436690 ) ) ;
#110714=CARTESIAN_POINT ( 'NONE',  ( 16.51473224551083163, -9.474510206698727899, 50.83442372801899722 ) ) ;
#110717=CARTESIAN_POINT ( 'NONE',  ( 19.03943276465977164, 0.05219959533936151252, 91.25109039468566152 ) ) ;
#110718=CARTESIAN_POINT ( 'NONE',  ( -8.314922557961024197, 14.29746914071037800, 77.91775706135231871 ) ) ;
#110719=CARTESIAN_POINT ( 'NONE',  ( 16.51473224551069308, 9.474510206698969483, 29.16557627198103475 ) ) ;
#110720=CARTESIAN_POINT ( 'NONE',  ( 0.05219959533909260263, 19.03943276465977164, 104.9989096053143669 ) ) ;
#110721=CARTESIAN_POINT ( 'NONE',  ( -21.53943276465977519, -0.05219959533937600094, 43.75109039468568284 ) ) ;
#110723=CARTESIAN_POINT ( 'NONE',  ( -9.564922557961040184, 16.46253265017147172, 92.91775706135233293 ) ) ;
#110724=CARTESIAN_POINT ( 'NONE',  ( 17.44270441346519362, 5.991230190322986537, 88.86335079264232206 ) ) ;
#110725=CARTESIAN_POINT ( 'NONE',  ( -13.97604488694527625, -13.89961937509977652, 51.87390960531436690 ) ) ;
#110726=CARTESIAN_POINT ( 'NONE',  ( 9.474510206698971260, -16.51473224551069308, 102.9155762719810241 ) ) ;
#110727=CARTESIAN_POINT ( 'NONE',  ( -8.314922557960811034, -14.29746914071050412, 57.08224293864769550 ) ) ;
#110728=CARTESIAN_POINT ( 'NONE',  ( 16.51473224551069308, 9.474510206698969483, 54.16557627198103120 ) ) ;
#110729=CARTESIAN_POINT ( 'NONE',  ( -9.474510206698964154, 16.51473224551069663, 60.41557627198102409 ) ) ;
#110730=CARTESIAN_POINT ( 'NONE',  ( 9.564922557961047289, -16.46253265017146816, 65.41775706135233293 ) ) ;
#110731=CARTESIAN_POINT ( 'NONE',  ( -13.89961937509957401, -13.97604488694547875, 34.37609039468566863 ) ) ;
#110732=CARTESIAN_POINT ( 'NONE',  ( -5.049401038298153566, 19.05341960407611168, 70.20724293864769550 ) ) ;
#110733=( BOUNDED_CURVE ( )  B_SPLINE_CURVE ( 2, ( #72258, #101583, #178448, #133936, #42922, #117766, #163271, #147103, #179459, #88408, #150104, #162262, #40924, #70262, #134943, #73273, #193614, #116757, #197598, #196620, #195626, #58090, #181444, #164283, #166272, #102597, #104587, #89413, #74258, #39915, #151102, #25776, #87422, #12594, #135928, #59064, #64034, #63031, #171218, #185392, #121724, #167258, #139862, #90394, #76214, #91363, #136901, #15552, #47883, #28757, #140864, #137893, #60056, #2353, #32707, #107539, #359, #125704, #75230, #30724, #199574, #94359, #92371, #14556, #109536, #156038, #187403, #77210, #152078, #13563, #105572, #170222, #183416 ),
 .UNSPECIFIED., .F., .T. ) 
 B_SPLINE_CURVE_WITH_KNOTS ( ( 3, 2, 2, 2, 2, 2, 2, 2, 2, 2, 2, 2, 2, 2, 2, 2, 2, 2, 2, 2, 2, 2, 2, 2, 2, 2, 2, 2, 2, 2, 2, 2, 2, 2, 2, 2, 3 ),
 ( 0.000000000000000000, 0.004385964912280701511, 0.008771929824561403022, 0.01315789473684210280, 0.01754385964912280604, 0.02192982456140350755, 0.02631578947368420560, 0.03070175438596491405, 0.03508771929824561209, 0.03947368421052631360, 0.04385964912280701511, 0.04824561403508771662, 0.05263157894736841119, 0.05701754385964912658, 0.06140350877192982809, 0.06578947368421052266, 0.07017543859649122417, 0.07456140350877192569, 0.07894736842105262720, 0.08333333333333332871, 0.08771929824561403022, 0.09210526315789473173, 0.09649122807017543324, 0.1008771929824561209, 0.1052631578947368224, 0.1096491228070175239, 0.1140350877192982532, 0.1184210526315789547, 0.1228070175438596562, 0.1271929824561403577, 0.1315789473684210453, 0.1359649122807017607, 0.1403508771929824483, 0.1447368421052631637, 0.1491228070175438514, 0.1535087719298245668, 0.1554186205929700415 ),
 .UNSPECIFIED. ) 
 CURVE ( )  GEOMETRIC_REPRESENTATION_ITEM ( )  RATIONAL_B_SPLINE_CURVE ( ( 1.000000000000000000, 0.9659258262890683122, 1.000000000000000000, 0.9659258262890683122, 1.000000000000000000, 0.9659258262890683122, 1.000000000000000000, 0.9659258262890683122, 1.000000000000000000, 0.9659258262890683122, 1.000000000000000000, 0.9659258262890683122, 1.000000000000000000, 0.9659258262890683122, 1.000000000000000000, 0.9659258262890683122, 1.000000000000000000, 0.9659258262890683122, 1.000000000000000000, 0.9659258262890683122, 1.000000000000000000, 0.9659258262890683122, 1.000000000000000000, 0.9659258262890683122, 1.000000000000000000, 0.9659258262890683122, 1.000000000000000000, 0.9659258262890683122, 1.000000000000000000, 0.9659258262890683122, 1.000000000000000000, 0.9659258262890683122, 1.000000000000000000, 0.9659258262890683122, 1.000000000000000000, 0.9659258262890683122, 1.000000000000000000, 0.9659258262890683122, 1.000000000000000000, 0.9659258262890683122, 1.000000000000000000, 0.9659258262890683122, 1.000000000000000000, 0.9659258262890683122, 1.000000000000000000, 0.9659258262890683122, 1.000000000000000000, 0.9659258262890683122, 1.000000000000000000, 0.9659258262890683122, 1.000000000000000000, 0.9659258262890683122, 1.000000000000000000, 0.9659258262890683122, 1.000000000000000000, 0.9659258262890683122, 1.000000000000000000, 0.9659258262890683122, 1.000000000000000000, 0.9659258262890683122, 1.000000000000000000, 0.9659258262890683122, 1.000000000000000000, 0.9659258262890683122, 1.000000000000000000, 0.9659258262890683122, 1.000000000000000000, 0.9659258262890683122, 1.000000000000000000, 0.9659258262890683122, 1.000000000000000000, 0.9851625545550090068, 0.9832469066685280978 ) ) 
 REPRESENTATION_ITEM ( '' )  );
#110734=CARTESIAN_POINT ( 'NONE',  ( -21.52544592524343514, 5.823673210054127303, 76.04057627198102409 ) ) ;
#110735=CARTESIAN_POINT ( 'NONE',  ( -12.06949235617756955, 12.14591786802309770, 70.62390960531436690 ) ) ;
#110736=CARTESIAN_POINT ( 'NONE',  ( 5.049401038297881783, 19.05341960407617563, 32.29275706135233293 ) ) ;
#110738=CARTESIAN_POINT ( 'NONE',  ( 18.62759615963271287, -10.81492255796078972, 43.33224293864769550 ) ) ;
#110739=CARTESIAN_POINT ( 'NONE',  ( -10.81492255796078084, -18.62759615963271287, 32.08224293864769550 ) ) ;
#110740=CARTESIAN_POINT ( 'NONE',  ( -19.05341960407611168, -5.049401038298163336, 66.45724293864769550 ) ) ;
#110741=CARTESIAN_POINT ( 'NONE',  ( 19.03943276465977164, -0.05219959533909143690, 38.74890960531436690 ) ) ;
#110742=CARTESIAN_POINT ( 'NONE',  ( 16.53943276465976808, -0.05219959533910856209, 103.7489096053143669 ) ) ;
#110743=CARTESIAN_POINT ( 'NONE',  ( -18.62759615963270932, 10.81492255796079327, 115.8322429386477097 ) ) ;
#110744=CARTESIAN_POINT ( 'NONE',  ( 16.51473224551069308, 9.474510206698969483, 114.1655762719810241 ) ) ;
#110745=CARTESIAN_POINT ( 'NONE',  ( 21.52544592524334988, 5.823673210054432836, 26.45942372801901854 ) ) ;
#110746=CARTESIAN_POINT ( 'NONE',  ( -5.153800228976328057, -19.02544592524343514, 27.29057627198103120 ) ) ;
#110747=CARTESIAN_POINT ( 'NONE',  ( -21.52544592524343514, 5.823673210054127303, 101.0405762719810383 ) ) ;
#110748=CARTESIAN_POINT ( 'NONE',  ( 5.153800228976615827, -19.02544592524334988, 45.20942372801901143 ) ) ;
#110749=CARTESIAN_POINT ( 'NONE',  ( 9.564922557960805705, 16.46253265017160317, 29.58224293864769550 ) ) ;
#110750=CARTESIAN_POINT ( 'NONE',  ( 18.22780087662122384, -5.500000000000022204, 76.01540105326107266 ) ) ;
#110752=CARTESIAN_POINT ( 'NONE',  ( -16.53943276465976808, -0.05219959533934237506, 43.75109039468568284 ) ) ;
#110753=CARTESIAN_POINT ( 'NONE',  ( -16.51473224551069308, -9.474510206698971260, 21.66557627198102765 ) ) ;
#110755=CARTESIAN_POINT ( 'NONE',  ( -16.51473224551069308, -9.474510206698971260, 71.66557627198102409 ) ) ;
#110756=CARTESIAN_POINT ( 'NONE',  ( 16.52544592524342804, -4.483927247898539470, 108.5405762719810241 ) ) ;
#110758=CARTESIAN_POINT ( 'NONE',  ( -10.72451020669898014, 18.67979575497178502, 40.41557627198103120 ) ) ;
#110759=CARTESIAN_POINT ( 'NONE',  ( -4.483927247898539470, -16.52544592524342804, 72.29057627198102409 ) ) ;
#110760=CARTESIAN_POINT ( 'NONE',  ( -12.06949235617739369, -12.14591786802326823, 34.37609039468568284 ) ) ;
#110761=CARTESIAN_POINT ( 'NONE',  ( 0.05219959533937995610, -21.53943276465977519, 80.00109039468568994 ) ) ;
#110762=CARTESIAN_POINT ( 'NONE',  ( -13.97604488694527625, -13.89961937509977652, 31.87390960531435979 ) ) ;
#110763=CARTESIAN_POINT ( 'NONE',  ( -14.34966873604960291, -8.224510206698953496, 21.66557627198102409 ) ) ;
#110764=CARTESIAN_POINT ( 'NONE',  ( -16.53943276465976808, 0.05219959533911058130, 56.24890960531436690 ) ) ;
#110765=CARTESIAN_POINT ( 'NONE',  ( 9.474510206698971260, -16.51473224551069308, 47.91557627198102409 ) ) ;
#110766=CARTESIAN_POINT ( 'NONE',  ( 5.719274019375673035, 21.55341960407619339, 102.2927570613523613 ) ) ;
#110767=CARTESIAN_POINT ( 'NONE',  ( 10.72451020669898902, -18.67979575497178502, 107.9155762719810241 ) ) ;
#110768=CARTESIAN_POINT ( 'NONE',  ( -18.62759615963255300, -10.81492255796106328, 69.16775706135234714 ) ) ;
#110769=CARTESIAN_POINT ( 'NONE',  ( -4.379528057220086978, -16.55341960407618274, 34.79275706135235424 ) ) ;
#110770=CARTESIAN_POINT ( 'NONE',  ( 8.224510206698953496, -14.34966873604960469, 77.91557627198102409 ) ) ;
#110771=CARTESIAN_POINT ( 'NONE',  ( -18.62759615963255300, -10.81492255796106328, 84.16775706135234714 ) ) ;
#110772=CARTESIAN_POINT ( 'NONE',  ( -0.05219959533934338120, 16.53943276465976808, 112.5010903946857042 ) ) ;
#110774=CARTESIAN_POINT ( 'NONE',  ( -18.39639308325436673, -5.500000000000039080, 66.48252246182197212 ) ) ;
#110775=CARTESIAN_POINT ( 'NONE',  ( 16.53943276465976808, -0.05219959533910856209, 38.74890960531435979 ) ) ;
#110776=CARTESIAN_POINT ( 'NONE',  ( 16.52544592524335698, 4.483927247898782831, 76.45942372801901854 ) ) ;
#110777=CARTESIAN_POINT ( 'NONE',  ( -19.05341960407611168, -5.049401038298163336, 91.45724293864766707 ) ) ;
#110778=CARTESIAN_POINT ( 'NONE',  ( -19.05341960407611168, -5.049401038298163336, 96.45724293864769550 ) ) ;
#110779=CARTESIAN_POINT ( 'NONE',  ( -10.72451020669870658, -18.67979575497194134, 99.58442372801900433 ) ) ;
#110781=CARTESIAN_POINT ( 'NONE',  ( -8.314922557961024197, 14.29746914071037800, 107.9177570613523471 ) ) ;
#110782=CARTESIAN_POINT ( 'NONE',  ( -14.29746914071049879, 8.314922557960819915, 70.83224293864770971 ) ) ;
#110783=CARTESIAN_POINT ( 'NONE',  ( -0.05219959533909027116, -19.03943276465977164, 77.49890960531435269 ) ) ;
#110785=CARTESIAN_POINT ( 'NONE',  ( -14.29746914071037622, -8.314922557961029526, 29.16775706135234003 ) ) ;
#110786=CARTESIAN_POINT ( 'NONE',  ( 5.049401038298161559, -19.05341960407611168, 27.70724293864769550 ) ) ;
#110787=CARTESIAN_POINT ( 'NONE',  ( -5.153800228976328057, -19.02544592524343514, 97.29057627198099567 ) ) ;
#110788=CARTESIAN_POINT ( 'NONE',  ( -4.483927247898782831, 16.52544592524335698, 27.70942372801901854 ) ) ;
#110790=CARTESIAN_POINT ( 'NONE',  ( -19.02544592524334988, -5.153800228976617603, 38.95942372801900433 ) ) ;
#110791=CARTESIAN_POINT ( 'NONE',  ( -8.224510206698735004, -14.34966873604973081, 99.58442372801900433 ) ) ;
#110792=CARTESIAN_POINT ( 'NONE',  ( 13.97604488694548053, -13.89961937509957401, 105.6260903946856757 ) ) ;
#110793=CARTESIAN_POINT ( 'NONE',  ( -9.564922557960796823, -16.46253265017161027, 27.08224293864769550 ) ) ;
#110794=CARTESIAN_POINT ( 'NONE',  ( 4.483927247898790824, -16.52544592524335698, 80.20942372801901854 ) ) ;
#110795=CARTESIAN_POINT ( 'NONE',  ( 16.53943276465976808, 0.05219959533934440121, 61.25109039468567573 ) ) ;
#110797=CARTESIAN_POINT ( 'NONE',  ( -9.564922557961040184, 16.46253265017147172, 62.91775706135233293 ) ) ;
#110798=CARTESIAN_POINT ( 'NONE',  ( 15.72974639402176855, 15.80617190586768217, 111.8760903946856615 ) ) ;
#110799=CARTESIAN_POINT ( 'NONE',  ( 16.51473224551069308, 9.474510206698969483, 44.16557627198103120 ) ) ;
#110800=CARTESIAN_POINT ( 'NONE',  ( -0.05219959533909027116, -19.03943276465977164, 87.49890960531436690 ) ) ;
#110801=CARTESIAN_POINT ( 'NONE',  ( 8.314922557960818139, 14.29746914071049879, 89.58224293864768129 ) ) ;
#110802=CARTESIAN_POINT ( 'NONE',  ( 5.153800228976615827, -19.02544592524334988, 55.20942372801899722 ) ) ;
#110803=CARTESIAN_POINT ( 'NONE',  ( 15.72974639402199770, -15.80617190586745480, 53.12390960531436690 ) ) ;
#110804=CARTESIAN_POINT ( 'NONE',  ( -10.81492255796105439, 18.62759615963255655, 107.9177570613523471 ) ) ;
#110805=CARTESIAN_POINT ( 'NONE',  ( 9.564922557960805705, 16.46253265017160317, 89.58224293864769550 ) ) ;
#110806=CARTESIAN_POINT ( 'NONE',  ( -16.51473224551082808, 9.474510206698731452, 23.33442372801900078 ) ) ;
#110807=CARTESIAN_POINT ( 'NONE',  ( 18.67979575497178502, 10.72451020669898547, 59.16557627198103120 ) ) ;
#110808=CARTESIAN_POINT ( 'NONE',  ( 5.153800228976335163, 19.02544592524342804, 109.7905762719810099 ) ) ;
#110809=CARTESIAN_POINT ( 'NONE',  ( 9.474510206698729675, 16.51473224551082808, 92.08442372801900433 ) ) ;
#110810=CARTESIAN_POINT ( 'NONE',  ( -17.50000000000014566, 3.417042746626926863, 110.1738039623247545 ) ) ;
#110811=CARTESIAN_POINT ( 'NONE',  ( 9.564922557961047289, -16.46253265017146816, 110.4177570613523471 ) ) ;
#110812=CARTESIAN_POINT ( 'NONE',  ( 19.03943276465977164, -0.05219959533909143690, 23.74890960531435269 ) ) ;
#110813=CARTESIAN_POINT ( 'NONE',  ( -9.474510206698964154, 16.51473224551069663, 85.41557627198102409 ) ) ;
#110814=CARTESIAN_POINT ( 'NONE',  ( 5.823673210054125526, 21.52544592524343514, 79.79057627198102409 ) ) ;
#110815=CARTESIAN_POINT ( 'NONE',  ( -14.34966873604972548, 8.224510206698743886, 43.33442372801901143 ) ) ;
#110816=CARTESIAN_POINT ( 'NONE',  ( 10.72451020669871369, 18.67979575497193778, 47.08442372801901854 ) ) ;
#110817=CARTESIAN_POINT ( 'NONE',  ( 18.67979575497194134, -10.72451020669871369, 95.83442372801903275 ) ) ;
#110818=CARTESIAN_POINT ( 'NONE',  ( 4.483927247898790824, -16.52544592524335698, 90.20942372801903275 ) ) ;
#110820=CARTESIAN_POINT ( 'NONE',  ( -0.05219959533909027116, -19.03943276465977164, 82.49890960531436690 ) ) ;
#110821=CARTESIAN_POINT ( 'NONE',  ( 4.483927247898545687, 16.52544592524342804, 89.79057627198103830 ) ) ;
#110822=CARTESIAN_POINT ( 'NONE',  ( 8.224510206698953496, -14.34966873604960469, 42.91557627198103120 ) ) ;
#110823=CARTESIAN_POINT ( 'NONE',  ( -5.049401038297874678, -19.05341960407617918, 74.79275706135231871 ) ) ;
#110824=CARTESIAN_POINT ( 'NONE',  ( -18.67979575497193778, 10.72451020669871902, 48.33442372801902565 ) ) ;
#110825=CARTESIAN_POINT ( 'NONE',  ( -5.153800228976607833, 19.02544592524334988, 27.70942372801899722 ) ) ;
#110826=CARTESIAN_POINT ( 'NONE',  ( -8.314922557960811034, -14.29746914071050412, 87.08224293864769550 ) ) ;
#110827=CARTESIAN_POINT ( 'NONE',  ( 19.02544592524343514, -5.153800228976328945, 108.5405762719810383 ) ) ;
#110828=CARTESIAN_POINT ( 'NONE',  ( 16.55341960407611168, 4.379528057220329451, 28.95724293864769905 ) ) ;
#110829=CARTESIAN_POINT ( 'NONE',  ( -18.62759615963255300, -10.81492255796106328, 84.16775706135234714 ) ) ;
#110830=CARTESIAN_POINT ( 'NONE',  ( -14.29746914071037622, -8.314922557961029526, 54.16775706135235424 ) ) ;
#110831=CARTESIAN_POINT ( 'NONE',  ( 16.53943276465976808, 0.05219959533934440121, 111.2510903946856899 ) ) ;
#110832=CARTESIAN_POINT ( 'NONE',  ( 5.823673210054444382, -21.52544592524334988, 50.20942372801901854 ) ) ;
#110833=VERTEX_POINT ( 'NONE', #61763 ) ;
#110834=CARTESIAN_POINT ( 'NONE',  ( -10.72451020669870658, -18.67979575497194134, 34.58442372801900433 ) ) ;
#110835=CARTESIAN_POINT ( 'NONE',  ( 4.483927247898545687, 16.52544592524342804, 109.7905762719810383 ) ) ;
#110837=CARTESIAN_POINT ( 'NONE',  ( -12.14591786802309592, -12.06949235617757132, 71.87390960531438111 ) ) ;
#110838=CARTESIAN_POINT ( 'NONE',  ( 16.46253265017160672, -9.564922557960803928, 78.33224293864769550 ) ) ;
#110839=CARTESIAN_POINT ( 'NONE',  ( -14.34966873604972548, 8.224510206698743886, 103.3344237280190043 ) ) ;
#110840=CARTESIAN_POINT ( 'NONE',  ( -5.049401038298153566, 19.05341960407611168, 35.20724293864768839 ) ) ;
#110841=CARTESIAN_POINT ( 'NONE',  ( 21.52544592524344225, -5.823673210054117533, 58.54057627198103120 ) ) ;
#110842=CARTESIAN_POINT ( 'NONE',  ( -16.53943276465976808, 0.05219959533911058130, 96.24890960531435269 ) ) ;
#110843=CARTESIAN_POINT ( 'NONE',  ( -18.67979575497178146, -10.72451020669898902, 96.66557627198102409 ) ) ;
#110844=CARTESIAN_POINT ( 'NONE',  ( -5.049401038298153566, 19.05341960407611168, 105.2072429386476671 ) ) ;
#110845=CARTESIAN_POINT ( 'NONE',  ( -9.564922557960796823, -16.46253265017161027, 52.08224293864768839 ) ) ;
#110846=CARTESIAN_POINT ( 'NONE',  ( -9.564922557961040184, 16.46253265017147172, 92.91775706135233293 ) ) ;
#110847=CARTESIAN_POINT ( 'NONE',  ( -18.62759615963270932, 10.81492255796079327, 40.83224293864769550 ) ) ;
#110848=CARTESIAN_POINT ( 'NONE',  ( 21.52544592524334988, 5.823673210054432836, 66.45942372801903275 ) ) ;
#110849=CARTESIAN_POINT ( 'NONE',  ( 16.46253265017160672, -9.564922557960803928, 53.33224293864768839 ) ) ;
#110850=CARTESIAN_POINT ( 'NONE',  ( -5.049401038298153566, 19.05341960407611168, 90.20724293864766707 ) ) ;
#110851=CARTESIAN_POINT ( 'NONE',  ( -16.52544592524335698, -4.483927247898792601, 63.95942372801901854 ) ) ;
#110852=CARTESIAN_POINT ( 'NONE',  ( 15.72974639402176855, 15.80617190586768217, 41.87609039468568284 ) ) ;
#110853=CARTESIAN_POINT ( 'NONE',  ( 21.55341960407619695, -5.719274019375665929, 91.04275706135236135 ) ) ;
#110854=CARTESIAN_POINT ( 'NONE',  ( -5.719274019375978568, 21.55341960407610458, 105.2072429386477097 ) ) ;
#110855=CARTESIAN_POINT ( 'NONE',  ( -21.52544592524334988, -5.823673210054445271, 43.95942372801902565 ) ) ;
#110856=CARTESIAN_POINT ( 'NONE',  ( 12.14591786802327356, -12.06949235617739191, 60.62609039468567573 ) ) ;
#110857=CARTESIAN_POINT ( 'NONE',  ( 10.81492255796078972, 18.62759615963270932, 69.58224293864769550 ) ) ;
#110858=CARTESIAN_POINT ( 'NONE',  ( -5.049401038297874678, -19.05341960407617918, 29.79275706135232227 ) ) ;
#110859=CARTESIAN_POINT ( 'NONE',  ( 19.02544592524343514, -5.153800228976328945, 73.54057627198103830 ) ) ;
#110860=CARTESIAN_POINT ( 'NONE',  ( 12.14591786802327356, -12.06949235617739191, 110.6260903946857042 ) ) ;
#110862=CARTESIAN_POINT ( 'NONE',  ( -16.51473224551069308, -9.474510206698971260, 101.6655762719810241 ) ) ;
#110864=CARTESIAN_POINT ( 'NONE',  ( 5.153800228976615827, -19.02544592524334988, 85.20942372801900433 ) ) ;
#110865=CARTESIAN_POINT ( 'NONE',  ( -15.80617190586745835, -15.72974639402198527, 61.87390960531436690 ) ) ;
#110866=CARTESIAN_POINT ( 'NONE',  ( 16.52544592524342804, -4.483927247898539470, 33.54057627198102409 ) ) ;
#110867=CARTESIAN_POINT ( 'NONE',  ( 4.379528057220092307, 16.55341960407617563, 22.29275706135235069 ) ) ;
#110868=CARTESIAN_POINT ( 'NONE',  ( 0.05219959533909260263, 19.03943276465977164, 34.99890960531435979 ) ) ;
#110869=CARTESIAN_POINT ( 'NONE',  ( 16.53943276465976808, 0.05219959533934440121, 21.25109039468567218 ) ) ;
#110870=CARTESIAN_POINT ( 'NONE',  ( 5.823673210054125526, 21.52544592524343514, 89.79057627198103830 ) ) ;
#110871=CARTESIAN_POINT ( 'NONE',  ( 16.51473224551083163, -9.474510206698727899, 65.83442372801900433 ) ) ;
#110872=CARTESIAN_POINT ( 'NONE',  ( -16.53943276465976808, -0.05219959533934237506, 83.75109039468568994 ) ) ;
#110873=CARTESIAN_POINT ( 'NONE',  ( 5.153800228976335163, 19.02544592524342804, 74.79057627198103830 ) ) ;
#110874=CARTESIAN_POINT ( 'NONE',  ( 8.224510206698953496, -14.34966873604960469, 72.91557627198103830 ) ) ;
#110875=CARTESIAN_POINT ( 'NONE',  ( 9.564922557960805705, 16.46253265017160317, 44.58224293864769550 ) ) ;
#110876=CARTESIAN_POINT ( 'NONE',  ( 16.52544592524342804, -4.483927247898539470, 53.54057627198103120 ) ) ;
#110879=CARTESIAN_POINT ( 'NONE',  ( 16.55341960407611168, 4.379528057220329451, 23.95724293864769550 ) ) ;
#110880=CARTESIAN_POINT ( 'NONE',  ( -0.05219959533909027116, -19.03943276465977164, 82.49890960531436690 ) ) ;
#110882=CARTESIAN_POINT ( 'NONE',  ( 9.474510206698729675, 16.51473224551082808, 37.08442372801899722 ) ) ;
#110883=CARTESIAN_POINT ( 'NONE',  ( -4.483927247898782831, 16.52544592524335698, 47.70942372801902565 ) ) ;
#110884=CARTESIAN_POINT ( 'NONE',  ( 18.67979575497178502, 10.72451020669898547, 59.16557627198103120 ) ) ;
#110885=CARTESIAN_POINT ( 'NONE',  ( 16.51473224551083163, -9.474510206698727899, 20.83442372801899722 ) ) ;
#110886=CARTESIAN_POINT ( 'NONE',  ( 19.03943276465977164, -0.05219959533909143690, 68.74890960531436690 ) ) ;
#110888=CARTESIAN_POINT ( 'NONE',  ( -19.02544592524342804, 5.153800228976336051, 111.0405762719810099 ) ) ;
#110889=CARTESIAN_POINT ( 'NONE',  ( 18.62759615963255655, 10.81492255796105972, 41.66775706135235424 ) ) ;
#110890=CARTESIAN_POINT ( 'NONE',  ( -12.14591786802309592, -12.06949235617757132, 106.8739096053143811 ) ) ;
#110891=CARTESIAN_POINT ( 'NONE',  ( 5.823673210054125526, 21.52544592524343514, 94.79057627198105251 ) ) ;
#110892=CARTESIAN_POINT ( 'NONE',  ( -19.02544592524342804, 5.153800228976336051, 76.04057627198102409 ) ) ;
#110894=CARTESIAN_POINT ( 'NONE',  ( 10.72451020669871369, 18.67979575497193778, 27.08442372801901854 ) ) ;
#110896=CARTESIAN_POINT ( 'NONE',  ( -5.153800228976328057, -19.02544592524343514, 87.29057627198103830 ) ) ;
#110897=CYLINDRICAL_SURFACE ( 'NONE', #20452, 2.000000000000001776 ) ;
#110898=CARTESIAN_POINT ( 'NONE',  ( 19.02544592524343514, -5.153800228976328945, 33.54057627198102409 ) ) ;
#110899=CARTESIAN_POINT ( 'NONE',  ( 13.97604488694548053, -13.89961937509957401, 105.6260903946856757 ) ) ;
#110901=CARTESIAN_POINT ( 'NONE',  ( 4.483927247898545687, 16.52544592524342804, 109.7905762719810383 ) ) ;
#110902=CARTESIAN_POINT ( 'NONE',  ( -15.72974639402176322, -15.80617190586768395, 89.37609039468568994 ) ) ;
#110903=CARTESIAN_POINT ( 'NONE',  ( 13.97604488694527802, 13.89961937509977652, 79.37390960531435269 ) ) ;
#110904=CARTESIAN_POINT ( 'NONE',  ( -10.81492255796105439, 18.62759615963255655, 47.91775706135234714 ) ) ;
#110905=CARTESIAN_POINT ( 'NONE',  ( -10.81492255796105439, 18.62759615963255655, 22.91775706135235069 ) ) ;
#110907=CARTESIAN_POINT ( 'NONE',  ( 19.02544592524343514, -5.153800228976328945, 83.54057627198100988 ) ) ;
#110909=CARTESIAN_POINT ( 'NONE',  ( -14.29746914071037622, -8.314922557961029526, 44.16775706135234714 ) ) ;
#110910=CARTESIAN_POINT ( 'NONE',  ( -10.72451020669898014, 18.67979575497178502, 50.41557627198103120 ) ) ;
#110911=CARTESIAN_POINT ( 'NONE',  ( 5.719274019375673035, 21.55341960407619339, 82.29275706135234714 ) ) ;
#110913=CARTESIAN_POINT ( 'NONE',  ( 16.51473224551083163, -9.474510206698727899, 110.8344237280190043 ) ) ;
#110914=CARTESIAN_POINT ( 'NONE',  ( 13.97604488694527802, 13.89961937509977652, 54.37390960531435979 ) ) ;
#110915=CARTESIAN_POINT ( 'NONE',  ( -9.474510206698964154, 16.51473224551069663, 80.41557627198103830 ) ) ;
#110916=CARTESIAN_POINT ( 'NONE',  ( 8.224510206698953496, -14.34966873604960469, 102.9155762719810383 ) ) ;
#110917=CARTESIAN_POINT ( 'NONE',  ( -12.06949235617756955, 12.14591786802309770, 110.6239096053143669 ) ) ;
#110918=CARTESIAN_POINT ( 'NONE',  ( -16.46253265017160317, 9.564922557960807481, 110.8322429386476955 ) ) ;
#110919=CARTESIAN_POINT ( 'NONE',  ( 16.52544592524335698, 4.483927247898782831, 81.45942372801900433 ) ) ;
#110920=CARTESIAN_POINT ( 'NONE',  ( -16.53943276465976808, 0.05219959533911058130, 56.24890960531436690 ) ) ;
#110921=CARTESIAN_POINT ( 'NONE',  ( 9.474510206698971260, -16.51473224551069308, 57.91557627198103120 ) ) ;
#110922=CARTESIAN_POINT ( 'NONE',  ( -18.67979575497193778, 10.72451020669871902, 83.33442372801903275 ) ) ;
#110923=CARTESIAN_POINT ( 'NONE',  ( 10.81492255796106328, -18.62759615963255655, 75.41775706135233293 ) ) ;
#110924=CARTESIAN_POINT ( 'NONE',  ( -9.474510206698720793, -16.51473224551083518, 89.58442372801900433 ) ) ;
#110925=CARTESIAN_POINT ( 'NONE',  ( 0.05219959533910956823, 16.53943276465976808, 64.99890960531435269 ) ) ;
#110926=CARTESIAN_POINT ( 'NONE',  ( 5.823673210054125526, 21.52544592524343514, 114.7905762719810383 ) ) ;
#110927=CARTESIAN_POINT ( 'NONE',  ( -21.52544592524343514, 5.823673210054127303, 66.04057627198103830 ) ) ;
#110930=CARTESIAN_POINT ( 'NONE',  ( 16.51473224551069308, 9.474510206698969483, 74.16557627198103830 ) ) ;
#110931=CARTESIAN_POINT ( 'NONE',  ( -14.34966873604960291, -8.224510206698953496, 36.66557627198103120 ) ) ;
#110932=CARTESIAN_POINT ( 'NONE',  ( -0.05219959533934338120, 16.53943276465976808, 112.5010903946857042 ) ) ;
#110933=CARTESIAN_POINT ( 'NONE',  ( 16.53943276465976808, 0.05219959533934440121, 101.2510903946856757 ) ) ;
#110934=CARTESIAN_POINT ( 'NONE',  ( -13.89961937509957401, -13.97604488694547875, 49.37609039468567573 ) ) ;
#110936=CARTESIAN_POINT ( 'NONE',  ( -16.46253265017160317, 9.564922557960807481, 85.83224293864769550 ) ) ;
#110937=CARTESIAN_POINT ( 'NONE',  ( 4.379528057220339221, -16.55341960407611168, 57.70724293864770260 ) ) ;
#110938=CARTESIAN_POINT ( 'NONE',  ( 16.38665767535053419, -7.295008042176110763, 102.7640086421455123 ) ) ;
#110939=CARTESIAN_POINT ( 'NONE',  ( -9.474510206698964154, 16.51473224551069663, 115.4155762719810241 ) ) ;
#110940=CARTESIAN_POINT ( 'NONE',  ( -18.62759615963270932, 10.81492255796079327, 55.83224293864770260 ) ) ;
#110941=ORIENTED_EDGE ( 'NONE', *, *, #197763, .T. ) ;
#110942=CARTESIAN_POINT ( 'NONE',  ( -4.483927247898539470, -16.52544592524342804, 92.29057627198103830 ) ) ;
#110943=CARTESIAN_POINT ( 'NONE',  ( 12.14591786802327356, -12.06949235617739191, 50.62609039468568994 ) ) ;
#110944=CARTESIAN_POINT ( 'NONE',  ( -8.224510206698948167, 14.34966873604960824, 85.41557627198102409 ) ) ;
#110946=CARTESIAN_POINT ( 'NONE',  ( 13.97604488694548053, -13.89961937509957401, 75.62609039468564731 ) ) ;
#110947=CARTESIAN_POINT ( 'NONE',  ( -5.823673210054116645, -21.52544592524344225, 27.29057627198103120 ) ) ;
#110949=CARTESIAN_POINT ( 'NONE',  ( -16.51473224551069308, -9.474510206698971260, 41.66557627198103120 ) ) ;
#110950=CARTESIAN_POINT ( 'NONE',  ( -4.483927247898782831, 16.52544592524335698, 32.70942372801900433 ) ) ;
#110951=CARTESIAN_POINT ( 'NONE',  ( -16.53943276465976808, 0.05219959533911058130, 36.24890960531435979 ) ) ;
#110952=CARTESIAN_POINT ( 'NONE',  ( -21.55341960407610458, -5.719274019375992779, 61.45724293864770260 ) ) ;
#110954=CARTESIAN_POINT ( 'NONE',  ( 16.51473224551083163, -9.474510206698727899, 90.83442372801900433 ) ) ;
#110955=CARTESIAN_POINT ( 'NONE',  ( -15.72974639402197994, 15.80617190586746368, 45.62390960531436690 ) ) ;
#110956=CARTESIAN_POINT ( 'NONE',  ( -10.81492255796105439, 18.62759615963255655, 77.91775706135231871 ) ) ;
#110958=CARTESIAN_POINT ( 'NONE',  ( -4.379528057220086978, -16.55341960407618274, 29.79275706135234358 ) ) ;
#110959=CARTESIAN_POINT ( 'NONE',  ( -16.46253265017160317, 9.564922557960807481, 40.83224293864769550 ) ) ;
#110960=CARTESIAN_POINT ( 'NONE',  ( 19.05341960407611168, 5.049401038298154454, 83.95724293864766707 ) ) ;
#110961=CARTESIAN_POINT ( 'NONE',  ( -5.153800228976328057, -19.02544592524343514, 37.29057627198102409 ) ) ;
#110962=CARTESIAN_POINT ( 'NONE',  ( -12.06949235617756955, 12.14591786802309770, 105.6239096053143669 ) ) ;
#110964=CARTESIAN_POINT ( 'NONE',  ( -19.03943276465977164, 0.05219959533909376836, 106.2489096053143669 ) ) ;
#110966=CARTESIAN_POINT ( 'NONE',  ( 12.06949235617739724, 12.14591786802326823, 61.87609039468568284 ) ) ;
#110967=CARTESIAN_POINT ( 'NONE',  ( -18.62759615963270932, 10.81492255796079327, 85.83224293864768129 ) ) ;
#110968=CARTESIAN_POINT ( 'NONE',  ( 9.564922557960805705, 16.46253265017160317, 49.58224293864770260 ) ) ;
#110969=CARTESIAN_POINT ( 'NONE',  ( -19.03943276465977164, -0.05219959533935918106, 78.75109039468567573 ) ) ;
#110970=CARTESIAN_POINT ( 'NONE',  ( -21.52544592524334988, -5.823673210054445271, 23.95942372801901143 ) ) ;
#110971=CARTESIAN_POINT ( 'NONE',  ( 9.474510206698971260, -16.51473224551069308, 77.91557627198103830 ) ) ;
#110972=CARTESIAN_POINT ( 'NONE',  ( -13.97604488694527625, -13.89961937509977652, 106.8739096053143669 ) ) ;
#110974=CARTESIAN_POINT ( 'NONE',  ( -16.52544592524335698, -4.483927247898792601, 33.95942372801901143 ) ) ;
#110975=CARTESIAN_POINT ( 'NONE',  ( 21.53943276465977519, -0.05219959533907433946, 113.7489096053143527 ) ) ;
#110976=CARTESIAN_POINT ( 'NONE',  ( -8.314922557960811034, -14.29746914071050412, 107.0822429386476955 ) ) ;
#110977=CARTESIAN_POINT ( 'NONE',  ( 13.89961937509977652, -13.97604488694527269, 93.12390960531436690 ) ) ;
#110978=CARTESIAN_POINT ( 'NONE',  ( 16.46253265017146816, 9.564922557961045513, 76.66775706135234714 ) ) ;
#110979=CARTESIAN_POINT ( 'NONE',  ( 19.02544592524334988, 5.153800228976608722, 31.45942372801900433 ) ) ;
#110980=CARTESIAN_POINT ( 'NONE',  ( 10.81492255796078972, 18.62759615963270932, 89.58224293864768129 ) ) ;
#110981=CARTESIAN_POINT ( 'NONE',  ( 0.05219959533936267826, -19.03943276465977164, 25.00109039468566152 ) ) ;
#110982=CARTESIAN_POINT ( 'NONE',  ( 16.52544592524335698, 4.483927247898782831, 81.45942372801900433 ) ) ;
#110983=CARTESIAN_POINT ( 'NONE',  ( 16.46253265017160672, -9.564922557960803928, 103.3322429386476955 ) ) ;
#110984=CARTESIAN_POINT ( 'NONE',  ( 19.03943276465977164, -0.05219959533909143690, 48.74890960531435979 ) ) ;
#110985=CARTESIAN_POINT ( 'NONE',  ( -21.53943276465977519, -0.05219959533937600094, 53.75109039468568994 ) ) ;
#110987=CARTESIAN_POINT ( 'NONE',  ( -10.81492255796105439, 18.62759615963255655, 62.91775706135236135 ) ) ;
#110988=CARTESIAN_POINT ( 'NONE',  ( 13.97604488694527802, 13.89961937509977652, 74.37390960531436690 ) ) ;
#110989=CARTESIAN_POINT ( 'NONE',  ( -15.72974639402176322, -15.80617190586768395, 54.37609039468568994 ) ) ;
#110990=CARTESIAN_POINT ( 'NONE',  ( -9.564922557961040184, 16.46253265017147172, 92.91775706135233293 ) ) ;
#110991=CARTESIAN_POINT ( 'NONE',  ( -9.474510206698964154, 16.51473224551069663, 50.41557627198102409 ) ) ;
#110992=CARTESIAN_POINT ( 'NONE',  ( 4.379528057220092307, 16.55341960407617563, 92.29275706135236135 ) ) ;
#110993=CARTESIAN_POINT ( 'NONE',  ( 16.51473224551069308, 9.474510206698969483, 69.16557627198102409 ) ) ;
#110994=FACE_OUTER_BOUND ( 'NONE', #128745, .T. ) ;
#110995=CARTESIAN_POINT ( 'NONE',  ( -16.51473224551069308, -9.474510206698971260, 51.66557627198102409 ) ) ;
#110996=CARTESIAN_POINT ( 'NONE',  ( 21.52544592524344225, -5.823673210054117533, 88.54057627198103830 ) ) ;
#110997=CARTESIAN_POINT ( 'NONE',  ( 4.379528057220092307, 16.55341960407617563, 72.29275706135236135 ) ) ;
#110999=CARTESIAN_POINT ( 'NONE',  ( 5.153800228976615827, -19.02544592524334988, 25.20942372801900433 ) ) ;
#111000=CARTESIAN_POINT ( 'NONE',  ( -19.05341960407611168, -5.049401038298163336, 71.45724293864766707 ) ) ;
#111001=CARTESIAN_POINT ( 'NONE',  ( -14.34966873604960291, -8.224510206698953496, 61.66557627198103120 ) ) ;
#111002=CARTESIAN_POINT ( 'NONE',  ( -0.05219959533910754901, -16.53943276465976808, 97.49890960531436690 ) ) ;
#111003=CARTESIAN_POINT ( 'NONE',  ( -9.474510206698964154, 16.51473224551069663, 95.41557627198102409 ) ) ;
#111004=CARTESIAN_POINT ( 'NONE',  ( -5.153800228976328057, -19.02544592524343514, 92.29057627198099567 ) ) ;
#111005=CARTESIAN_POINT ( 'NONE',  ( 21.52544592524334988, 5.823673210054432836, 46.45942372801901854 ) ) ;
#111006=CARTESIAN_POINT ( 'NONE',  ( 19.03943276465977164, -0.05219959533909143690, 103.7489096053143669 ) ) ;
#111007=CARTESIAN_POINT ( 'NONE',  ( 21.53943276465977519, 0.05219959533937863772, 111.2510903946856899 ) ) ;
#111008=CARTESIAN_POINT ( 'NONE',  ( 0.05219959533934541429, -16.53943276465976808, 75.00109039468568994 ) ) ;
#111009=CARTESIAN_POINT ( 'NONE',  ( 15.80617190586769283, -15.72974639402175789, 40.62609039468567573 ) ) ;
#111010=CARTESIAN_POINT ( 'NONE',  ( -5.719274019375978568, 21.55341960407610458, 35.20724293864768839 ) ) ;
#111011=CARTESIAN_POINT ( 'NONE',  ( -18.67979575497178146, -10.72451020669898902, 96.66557627198102409 ) ) ;
#111012=CARTESIAN_POINT ( 'NONE',  ( -16.55341960407611168, -4.379528057220339221, 66.45724293864768129 ) ) ;
#111013=CARTESIAN_POINT ( 'NONE',  ( 13.89961937509977652, -13.97604488694527269, 58.12390960531436690 ) ) ;
#111014=CARTESIAN_POINT ( 'NONE',  ( 16.53943276465976808, -0.05219959533910856209, 78.74890960531436690 ) ) ;
#111015=CARTESIAN_POINT ( 'NONE',  ( 18.62759615963271287, -10.81492255796078972, 38.33224293864768839 ) ) ;
#111016=CARTESIAN_POINT ( 'NONE',  ( 0.05219959533936267826, -19.03943276465977164, 40.00109039468566152 ) ) ;
#111017=EDGE_CURVE ( 'NONE', #78316, #658, #64083, .T. ) ;
#111018=CARTESIAN_POINT ( 'NONE',  ( -12.06949235617756955, 12.14591786802309770, 110.6239096053143669 ) ) ;
#111020=CARTESIAN_POINT ( 'NONE',  ( -8.314922557961024197, 14.29746914071037800, 72.91775706135234714 ) ) ;
#111021=CARTESIAN_POINT ( 'NONE',  ( 13.97604488694527802, 13.89961937509977652, 64.37390960531436690 ) ) ;
#111023=CARTESIAN_POINT ( 'NONE',  ( -14.29746914071049879, 8.314922557960819915, 85.83224293864768129 ) ) ;
#111024=CARTESIAN_POINT ( 'NONE',  ( -21.55341960407610458, -5.719274019375992779, 36.45724293864768839 ) ) ;
#111026=CARTESIAN_POINT ( 'NONE',  ( -8.224510206698735004, -14.34966873604973081, 109.5844237280190328 ) ) ;
#111027=CARTESIAN_POINT ( 'NONE',  ( 5.049401038297881783, 19.05341960407617563, 107.2927570613523187 ) ) ;
#111028=CARTESIAN_POINT ( 'NONE',  ( 21.52544592524334988, 5.823673210054432836, 81.45942372801900433 ) ) ;
#111029=CARTESIAN_POINT ( 'NONE',  ( -19.02544592524342804, 5.153800228976336051, 91.04057627198100988 ) ) ;
#111030=CARTESIAN_POINT ( 'NONE',  ( 5.823673210054125526, 21.52544592524343514, 99.79057627198103830 ) ) ;
#111031=CARTESIAN_POINT ( 'NONE',  ( 4.483927247898790824, -16.52544592524335698, 50.20942372801901854 ) ) ;
#111032=CARTESIAN_POINT ( 'NONE',  ( -19.03943276465977164, 0.05219959533909376836, 26.24890960531435624 ) ) ;
#111033=CARTESIAN_POINT ( 'NONE',  ( -16.53943276465976808, -0.05219959533934237506, 33.75109039468568284 ) ) ;
#111034=CARTESIAN_POINT ( 'NONE',  ( -19.05341960407617563, 5.049401038297882671, 93.54275706135234714 ) ) ;
#111036=CARTESIAN_POINT ( 'NONE',  ( -0.05219959533907301413, -21.53943276465977519, 87.49890960531436690 ) ) ;
#111037=CARTESIAN_POINT ( 'NONE',  ( -13.89961937509957401, -13.97604488694547875, 54.37609039468565442 ) ) ;
#111039=CARTESIAN_POINT ( 'NONE',  ( 21.52544592524344225, -5.823673210054117533, 103.5405762719810383 ) ) ;
#111041=CARTESIAN_POINT ( 'NONE',  ( 19.05341960407611168, 5.049401038298154454, 73.95724293864768129 ) ) ;
#111042=CARTESIAN_POINT ( 'NONE',  ( -4.483927247898782831, 16.52544592524335698, 37.70942372801900433 ) ) ;
#111044=CARTESIAN_POINT ( 'NONE',  ( -5.049401038297874678, -19.05341960407617918, 64.79275706135233293 ) ) ;
#111045=CARTESIAN_POINT ( 'NONE',  ( 18.62759615963255655, 10.81492255796105972, 21.66775706135235069 ) ) ;
#111046=CARTESIAN_POINT ( 'NONE',  ( 4.483927247898545687, 16.52544592524342804, 64.79057627198103830 ) ) ;
#111047=CARTESIAN_POINT ( 'NONE',  ( 9.474510206698971260, -16.51473224551069308, 72.91557627198102409 ) ) ;
#111048=CARTESIAN_POINT ( 'NONE',  ( -14.34966873604972548, 8.224510206698743886, 38.33442372801900433 ) ) ;
#111049=CARTESIAN_POINT ( 'NONE',  ( -13.89961937509957401, -13.97604488694547875, 39.37609039468566152 ) ) ;
#111050=CARTESIAN_POINT ( 'NONE',  ( 15.72974639402176855, 15.80617190586768217, 56.87609039468568994 ) ) ;
#111051=CARTESIAN_POINT ( 'NONE',  ( 0.05219959533934541429, -16.53943276465976808, 20.00109039468568639 ) ) ;
#111052=CARTESIAN_POINT ( 'NONE',  ( 13.97604488694527802, 13.89961937509977652, 49.37390960531434558 ) ) ;
#111053=CARTESIAN_POINT ( 'NONE',  ( -9.474510206698720793, -16.51473224551083518, 84.58442372801900433 ) ) ;
#111054=CARTESIAN_POINT ( 'NONE',  ( -21.53943276465977519, -0.05219959533937600094, 88.75109039468567573 ) ) ;
#111055=CARTESIAN_POINT ( 'NONE',  ( -19.03943276465977164, -0.05219959533935918106, 68.75109039468566152 ) ) ;
#111056=CARTESIAN_POINT ( 'NONE',  ( -0.05219959533909027116, -19.03943276465977164, 37.49890960531436690 ) ) ;
#111057=CARTESIAN_POINT ( 'NONE',  ( -21.55341960407610458, -5.719274019375992779, 51.45724293864770260 ) ) ;
#111058=CARTESIAN_POINT ( 'NONE',  ( -12.14591786802309592, -12.06949235617757132, 66.87390960531436690 ) ) ;
#111059=CARTESIAN_POINT ( 'NONE',  ( 16.51473224551083163, -9.474510206698727899, 70.83442372801900433 ) ) ;
#111060=CARTESIAN_POINT ( 'NONE',  ( -16.31925111598458500, -7.325300261831428905, 24.83575461032751264 ) ) ;
#111061=CARTESIAN_POINT ( 'NONE',  ( 19.03943276465977164, 0.05219959533936151252, 31.25109039468566863 ) ) ;
#111062=CARTESIAN_POINT ( 'NONE',  ( 16.55341960407618274, -4.379528057220086978, 101.0427570613523756 ) ) ;
#111063=CARTESIAN_POINT ( 'NONE',  ( 16.53943276465976808, -0.05219959533910856209, 53.74890960531437401 ) ) ;
#111064=CARTESIAN_POINT ( 'NONE',  ( 21.55341960407619695, -5.719274019375665929, 91.04275706135236135 ) ) ;
#111066=CARTESIAN_POINT ( 'NONE',  ( -21.55341960407610458, -5.719274019375992779, 101.4572429386476955 ) ) ;
#111067=CARTESIAN_POINT ( 'NONE',  ( -5.153800228976328057, -19.02544592524343514, 57.29057627198103120 ) ) ;
#111068=CARTESIAN_POINT ( 'NONE',  ( 18.62759615963255655, 10.81492255796105972, 71.66775706135234714 ) ) ;
#111069=CARTESIAN_POINT ( 'NONE',  ( -5.049401038298153566, 19.05341960407611168, 45.20724293864769550 ) ) ;
#111071=CARTESIAN_POINT ( 'NONE',  ( 0.05219959533909260263, 19.03943276465977164, 59.99890960531436690 ) ) ;
#111072=CARTESIAN_POINT ( 'NONE',  ( 4.483927247898545687, 16.52544592524342804, 109.7905762719810383 ) ) ;
#111073=CARTESIAN_POINT ( 'NONE',  ( -16.46253265017160317, 9.564922557960807481, 115.8322429386477097 ) ) ;
#111074=CARTESIAN_POINT ( 'NONE',  ( 12.06949235617757843, -12.14591786802309237, 58.12390960531435979 ) ) ;
#111075=CARTESIAN_POINT ( 'NONE',  ( 9.564922557960805705, 16.46253265017160317, 29.58224293864769550 ) ) ;
#111076=CARTESIAN_POINT ( 'NONE',  ( 8.224510206698953496, -14.34966873604960469, 87.91557627198103830 ) ) ;
#111077=CARTESIAN_POINT ( 'NONE',  ( -5.719274019375978568, 21.55341960407610458, 95.20724293864769550 ) ) ;
#111078=CARTESIAN_POINT ( 'NONE',  ( 10.81492255796106328, -18.62759615963255655, 35.41775706135234003 ) ) ;
#111079=CARTESIAN_POINT ( 'NONE',  ( 16.51473224551069308, 9.474510206698969483, 24.16557627198102765 ) ) ;
#111080=CARTESIAN_POINT ( 'NONE',  ( -14.29746914071037622, -8.314922557961029526, 34.16775706135234714 ) ) ;
#111081=CARTESIAN_POINT ( 'NONE',  ( 21.52544592524344225, -5.823673210054117533, 88.54057627198103830 ) ) ;
#111082=CARTESIAN_POINT ( 'NONE',  ( -21.52544592524334988, -5.823673210054445271, 108.9594237280190185 ) ) ;
#111083=CARTESIAN_POINT ( 'NONE',  ( 19.03943276465977164, -0.05219959533909143690, 88.74890960531436690 ) ) ;
#111084=CARTESIAN_POINT ( 'NONE',  ( -18.67979575497193778, 10.72451020669871902, 43.33442372801901143 ) ) ;
#111085=CARTESIAN_POINT ( 'NONE',  ( 18.67979575497178502, 10.72451020669898547, 29.16557627198103120 ) ) ;
#111086=CARTESIAN_POINT ( 'NONE',  ( 4.379528057220092307, 16.55341960407617563, 102.2927570613523613 ) ) ;
#111087=CARTESIAN_POINT ( 'NONE',  ( 18.67979575497194134, -10.72451020669871369, 55.83442372801901854 ) ) ;
#111088=CARTESIAN_POINT ( 'NONE',  ( 15.72974639402176855, 15.80617190586768217, 86.87609039468568994 ) ) ;
#111089=CARTESIAN_POINT ( 'NONE',  ( 9.474510206698729675, 16.51473224551082808, 27.08442372801900433 ) ) ;
#111090=CARTESIAN_POINT ( 'NONE',  ( 12.06949235617739724, 12.14591786802326823, 86.87609039468568994 ) ) ;
#111091=CARTESIAN_POINT ( 'NONE',  ( -21.55341960407619339, 5.719274019375674811, 38.54275706135234714 ) ) ;
#111092=CARTESIAN_POINT ( 'NONE',  ( -19.02544592524342804, 5.153800228976336051, 41.04057627198103120 ) ) ;
#111093=CARTESIAN_POINT ( 'NONE',  ( -10.72451020669870658, -18.67979575497194134, 99.58442372801900433 ) ) ;
#111094=CARTESIAN_POINT ( 'NONE',  ( -19.03943276465977164, 0.05219959533909376836, 101.2489096053143669 ) ) ;
#111095=CARTESIAN_POINT ( 'NONE',  ( -0.05219959533937732626, 21.53943276465977519, 22.50109039468567573 ) ) ;
#111096=CARTESIAN_POINT ( 'NONE',  ( 10.81492255796078972, 18.62759615963270932, 79.58224293864769550 ) ) ;
#111098=CARTESIAN_POINT ( 'NONE',  ( 18.67979575497178502, 10.72451020669898547, 64.16557627198102409 ) ) ;
#111099=CARTESIAN_POINT ( 'NONE',  ( -16.52544592524335698, -4.483927247898792601, 48.95942372801902565 ) ) ;
#111100=CARTESIAN_POINT ( 'NONE',  ( 8.224510206698953496, -14.34966873604960469, 62.91557627198102409 ) ) ;
#111102=CARTESIAN_POINT ( 'NONE',  ( -16.46253265017146816, -9.564922557961047289, 94.16775706135233293 ) ) ;
#111105=CARTESIAN_POINT ( 'NONE',  ( 4.483927247898790824, -16.52544592524335698, 25.20942372801901854 ) ) ;
#111106=CARTESIAN_POINT ( 'NONE',  ( 15.80617190586746368, 15.72974639402197994, 99.37390960531436690 ) ) ;
#111107=CARTESIAN_POINT ( 'NONE',  ( 10.81492255796078972, 18.62759615963270932, 79.58224293864769550 ) ) ;
#111108=CARTESIAN_POINT ( 'NONE',  ( -16.46253265017160317, 9.564922557960807481, 110.8322429386476955 ) ) ;
#111109=CARTESIAN_POINT ( 'NONE',  ( 12.06949235617739724, 12.14591786802326823, 61.87609039468568284 ) ) ;
#111110=CARTESIAN_POINT ( 'NONE',  ( 19.05341960407611168, 5.049401038298154454, 68.95724293864769550 ) ) ;
#111111=CARTESIAN_POINT ( 'NONE',  ( 18.62759615963255655, 10.81492255796105972, 46.66775706135234714 ) ) ;
#111112=CARTESIAN_POINT ( 'NONE',  ( -19.05341960407617563, 5.049401038297882671, 108.5427570613523187 ) ) ;
#111113=CARTESIAN_POINT ( 'NONE',  ( -5.153800228976328057, -19.02544592524343514, 102.2905762719810383 ) ) ;
#111114=CARTESIAN_POINT ( 'NONE',  ( -5.049401038298153566, 19.05341960407611168, 100.2072429386476955 ) ) ;
#111115=CARTESIAN_POINT ( 'NONE',  ( 10.72451020669898902, -18.67979575497178502, 97.91557627198103830 ) ) ;
#111116=CARTESIAN_POINT ( 'NONE',  ( 19.02544592524343514, -5.153800228976328945, 53.54057627198102409 ) ) ;
#111117=SPHERICAL_SURFACE ( 'NONE', #99177, 2.000000000000000000 ) ;
#111118=CARTESIAN_POINT ( 'NONE',  ( -14.29746914071049879, 8.314922557960819915, 75.83224293864769550 ) ) ;
#111119=CARTESIAN_POINT ( 'NONE',  ( -0.05219959533907301413, -21.53943276465977519, 27.49890960531435269 ) ) ;
#111120=CARTESIAN_POINT ( 'NONE',  ( 13.89961937509977652, -13.97604488694527269, 23.12390960531436335 ) ) ;
#111121=CARTESIAN_POINT ( 'NONE',  ( -5.719274019375978568, 21.55341960407610458, 100.2072429386476955 ) ) ;
#111122=CARTESIAN_POINT ( 'NONE',  ( -16.51473224551082808, 9.474510206698731452, 63.33442372801900433 ) ) ;
#111123=CARTESIAN_POINT ( 'NONE',  ( 15.72974639402199770, -15.80617190586745480, 23.12390960531436335 ) ) ;
#111124=CARTESIAN_POINT ( 'NONE',  ( 9.474510206698971260, -16.51473224551069308, 32.91557627198102409 ) ) ;
#111125=CARTESIAN_POINT ( 'NONE',  ( 15.80617190586746368, 15.72974639402197994, 49.37390960531436690 ) ) ;
#111127=CARTESIAN_POINT ( 'NONE',  ( 9.564922557960805705, 16.46253265017160317, 104.5822429386476955 ) ) ;
#111128=CARTESIAN_POINT ( 'NONE',  ( -21.53943276465977519, -0.05219959533937600094, 73.75109039468567573 ) ) ;
#111129=CARTESIAN_POINT ( 'NONE',  ( -13.89961937509977652, 13.97604488694528158, 55.62390960531434558 ) ) ;
#111130=CARTESIAN_POINT ( 'NONE',  ( 14.34966873604960469, 8.224510206698951720, 84.16557627198103830 ) ) ;
#111131=CARTESIAN_POINT ( 'NONE',  ( 12.14591786802327356, -12.06949235617739191, 35.62609039468568994 ) ) ;
#111132=CARTESIAN_POINT ( 'NONE',  ( 10.81492255796106328, -18.62759615963255655, 60.41775706135235424 ) ) ;
#111133=ORIENTED_EDGE ( 'NONE', *, *, #88147, .T. ) ;
#111134=CARTESIAN_POINT ( 'NONE',  ( -5.049401038297874678, -19.05341960407617918, 24.79275706135233648 ) ) ;
#111135=CARTESIAN_POINT ( 'NONE',  ( -16.46253265017146816, -9.564922557961047289, 84.16775706135233293 ) ) ;
#111136=CARTESIAN_POINT ( 'NONE',  ( 0.05219959533936267826, -19.03943276465977164, 40.00109039468566152 ) ) ;
#111138=CARTESIAN_POINT ( 'NONE',  ( 10.72451020669871369, 18.67979575497193778, 42.08442372801901854 ) ) ;
#111140=CARTESIAN_POINT ( 'NONE',  ( 9.474510206698729675, 16.51473224551082808, 32.08442372801900433 ) ) ;
#111141=CARTESIAN_POINT ( 'NONE',  ( -13.89961937509977652, 13.97604488694528158, 55.62390960531434558 ) ) ;
#111142=CARTESIAN_POINT ( 'NONE',  ( -19.05341960407617563, 5.049401038297882671, 33.54275706135231871 ) ) ;
#111143=CARTESIAN_POINT ( 'NONE',  ( -14.34966873604972548, 8.224510206698743886, 108.3344237280190185 ) ) ;
#111144=CARTESIAN_POINT ( 'NONE',  ( -0.05219959533907301413, -21.53943276465977519, 22.49890960531436335 ) ) ;
#111145=CARTESIAN_POINT ( 'NONE',  ( 10.81492255796106328, -18.62759615963255655, 80.41775706135234714 ) ) ;
#111148=CARTESIAN_POINT ( 'NONE',  ( 21.52544592524334988, 5.823673210054432836, 86.45942372801901854 ) ) ;
#111150=CARTESIAN_POINT ( 'NONE',  ( -16.51473224551069308, -9.474510206698971260, 101.6655762719810241 ) ) ;
#111151=EDGE_CURVE ( 'NONE', #14621, #50977, #114552, .T. ) ;
#111153=CARTESIAN_POINT ( 'NONE',  ( 13.97604488694527802, 13.89961937509977652, 54.37390960531435979 ) ) ;
#111154=CARTESIAN_POINT ( 'NONE',  ( -10.72451020669898014, 18.67979575497178502, 50.41557627198103120 ) ) ;
#111155=CARTESIAN_POINT ( 'NONE',  ( 0.05219959533910956823, 16.53943276465976808, 24.99890960531435624 ) ) ;
#111156=CARTESIAN_POINT ( 'NONE',  ( 12.14591786802309770, 12.06949235617756955, 99.37390960531436690 ) ) ;
#111157=CARTESIAN_POINT ( 'NONE',  ( 13.89961937509977652, -13.97604488694527269, 98.12390960531433848 ) ) ;
#111158=CARTESIAN_POINT ( 'NONE',  ( -9.474510206698720793, -16.51473224551083518, 24.58442372801900078 ) ) ;
#111159=CARTESIAN_POINT ( 'NONE',  ( -12.14591786802309592, -12.06949235617757132, 101.8739096053143811 ) ) ;
#111160=CARTESIAN_POINT ( 'NONE',  ( 18.67979575497194134, -10.72451020669871369, 55.83442372801901854 ) ) ;
#111161=CARTESIAN_POINT ( 'NONE',  ( -8.314922557961024197, 14.29746914071037800, 102.9177570613523756 ) ) ;
#111162=CARTESIAN_POINT ( 'NONE',  ( -5.153800228976607833, 19.02544592524334988, 67.70942372801900433 ) ) ;
#111164=CARTESIAN_POINT ( 'NONE',  ( -16.51473224551069308, -9.474510206698971260, 111.6655762719810383 ) ) ;
#111165=CARTESIAN_POINT ( 'NONE',  ( -8.224510206698948167, 14.34966873604960824, 70.41557627198102409 ) ) ;
#111166=CARTESIAN_POINT ( 'NONE',  ( 13.97604488694548053, -13.89961937509957401, 60.62609039468564731 ) ) ;
#111167=CARTESIAN_POINT ( 'NONE',  ( -13.97604488694527625, -13.89961937509977652, 56.87390960531434558 ) ) ;
#111168=CARTESIAN_POINT ( 'NONE',  ( 4.379528057220339221, -16.55341960407611168, 67.70724293864769550 ) ) ;
#111169=CARTESIAN_POINT ( 'NONE',  ( -13.97604488694547697, 13.89961937509957934, 93.12609039468566152 ) ) ;
#111170=CARTESIAN_POINT ( 'NONE',  ( 15.72974639402199770, -15.80617190586745480, 33.12390960531435979 ) ) ;
#111171=ORIENTED_EDGE ( 'NONE', *, *, #169970, .T. ) ;
#111172=CARTESIAN_POINT ( 'NONE',  ( 16.53943276465976808, -0.05219959533910856209, 98.74890960531438111 ) ) ;
#111173=CARTESIAN_POINT ( 'NONE',  ( -17.48853670773242897, -5.747243402303181981, 31.33328700250011778 ) ) ;
#111174=CARTESIAN_POINT ( 'NONE',  ( -16.51473224551069308, -9.474510206698971260, 61.66557627198103120 ) ) ;
#111175=CARTESIAN_POINT ( 'NONE',  ( 15.72974639402199770, -15.80617190586745480, 68.12390960531436690 ) ) ;
#111176=CARTESIAN_POINT ( 'NONE',  ( 13.89961937509977652, -13.97604488694527269, 48.12390960531435979 ) ) ;
#111177=CARTESIAN_POINT ( 'NONE',  ( 16.52544592524335698, 4.483927247898782831, 86.45942372801901854 ) ) ;
#111178=CARTESIAN_POINT ( 'NONE',  ( 19.05341960407611168, 5.049401038298154454, 68.95724293864769550 ) ) ;
#111179=CARTESIAN_POINT ( 'NONE',  ( -5.049401038297874678, -19.05341960407617918, 54.79275706135234003 ) ) ;
#111180=CARTESIAN_POINT ( 'NONE',  ( -10.81492255796105439, 18.62759615963255655, 87.91775706135234714 ) ) ;
#111181=CARTESIAN_POINT ( 'NONE',  ( -10.72451020669898014, 18.67979575497178502, 50.41557627198103120 ) ) ;
#111182=CARTESIAN_POINT ( 'NONE',  ( -13.89961937509977652, 13.97604488694528158, 110.6239096053143243 ) ) ;
#111183=CARTESIAN_POINT ( 'NONE',  ( -16.52544592524342804, 4.483927247898546575, 116.0405762719810383 ) ) ;
#111184=CARTESIAN_POINT ( 'NONE',  ( -16.53943276465976808, -0.05219959533934237506, 88.75109039468567573 ) ) ;
#111185=CARTESIAN_POINT ( 'NONE',  ( -13.89961937509957401, -13.97604488694547875, 109.3760903946856331 ) ) ;
#111186=CARTESIAN_POINT ( 'NONE',  ( -16.46253265017160317, 9.564922557960807481, 25.83224293864769194 ) ) ;
#111188=CARTESIAN_POINT ( 'NONE',  ( 10.72451020669871369, 18.67979575497193778, 102.0844237280190185 ) ) ;
#111189=CARTESIAN_POINT ( 'NONE',  ( -16.52544592524342804, 4.483927247898546575, 66.04057627198103830 ) ) ;
#111190=CARTESIAN_POINT ( 'NONE',  ( 0.05219959533910956823, 16.53943276465976808, 64.99890960531435269 ) ) ;
#111191=CARTESIAN_POINT ( 'NONE',  ( -18.62759615963270932, 10.81492255796079327, 100.8322429386477097 ) ) ;
#111192=CARTESIAN_POINT ( 'NONE',  ( 18.62759615963271287, -10.81492255796078972, 83.33224293864769550 ) ) ;
#111193=CARTESIAN_POINT ( 'NONE',  ( 16.62475595723697097, -7.163666690055294772, 98.02713351810470499 ) ) ;
#111194=CARTESIAN_POINT ( 'NONE',  ( -5.719274019375978568, 21.55341960407610458, 50.20724293864769550 ) ) ;
#111195=CARTESIAN_POINT ( 'NONE',  ( -8.314922557961024197, 14.29746914071037800, 67.91775706135234714 ) ) ;
#111196=CARTESIAN_POINT ( 'NONE',  ( 8.224510206698953496, -14.34966873604960469, 97.91557627198103830 ) ) ;
#111197=CARTESIAN_POINT ( 'NONE',  ( 19.03943276465977164, -0.05219959533909143690, 43.74890960531435979 ) ) ;
#111200=CARTESIAN_POINT ( 'NONE',  ( 14.29746914071037800, 8.314922557961029526, 101.6677570613523613 ) ) ;
#111201=CARTESIAN_POINT ( 'NONE',  ( -18.67979575497193778, 10.72451020669871902, 33.33442372801900433 ) ) ;
#111202=CARTESIAN_POINT ( 'NONE',  ( 5.049401038298161559, -19.05341960407611168, 87.70724293864769550 ) ) ;
#111203=CARTESIAN_POINT ( 'NONE',  ( -0.05219959533937732626, 21.53943276465977519, 67.50109039468568994 ) ) ;
#111205=CARTESIAN_POINT ( 'NONE',  ( -16.46253265017160317, 9.564922557960807481, 30.83224293864769550 ) ) ;
#111208=CARTESIAN_POINT ( 'NONE',  ( -10.81492255796105439, 18.62759615963255655, 57.91775706135234714 ) ) ;
#111209=CARTESIAN_POINT ( 'NONE',  ( -13.97604488694527625, -13.89961937509977652, 31.87390960531435979 ) ) ;
#111210=CARTESIAN_POINT ( 'NONE',  ( -16.51473224551069308, -9.474510206698971260, 21.66557627198102765 ) ) ;
#111211=CARTESIAN_POINT ( 'NONE',  ( -9.474510206698964154, 16.51473224551069663, 90.41557627198103830 ) ) ;
#111212=CARTESIAN_POINT ( 'NONE',  ( -5.153800228976607833, 19.02544592524334988, 62.70942372801899722 ) ) ;
#111213=CARTESIAN_POINT ( 'NONE',  ( -21.55341960407619339, 5.719274019375674811, 23.54275706135235424 ) ) ;
#111214=CARTESIAN_POINT ( 'NONE',  ( 5.153800228976615827, -19.02544592524334988, 55.20942372801899722 ) ) ;
#111215=CARTESIAN_POINT ( 'NONE',  ( 0.05219959533909260263, 19.03943276465977164, 44.99890960531435979 ) ) ;
#111216=CARTESIAN_POINT ( 'NONE',  ( -16.53943276465976808, -0.05219959533934237506, 103.7510903946857042 ) ) ;
#111217=CARTESIAN_POINT ( 'NONE',  ( -16.46253265017146816, -9.564922557961047289, 59.16775706135233293 ) ) ;
#111218=CARTESIAN_POINT ( 'NONE',  ( -4.483927247898539470, -16.52544592524342804, 27.29057627198103120 ) ) ;
#111219=CARTESIAN_POINT ( 'NONE',  ( -19.05341960407617563, 5.049401038297882671, 53.54275706135231871 ) ) ;
#111220=CARTESIAN_POINT ( 'NONE',  ( -19.03943276465977164, 0.05219959533909376836, 101.2489096053143669 ) ) ;
#111221=CARTESIAN_POINT ( 'NONE',  ( -15.72974639402176322, -15.80617190586768395, 109.3760903946857042 ) ) ;
#111222=CARTESIAN_POINT ( 'NONE',  ( -21.55341960407619339, 5.719274019375674811, 108.5427570613523756 ) ) ;
#111225=CARTESIAN_POINT ( 'NONE',  ( -15.72974639402176322, -15.80617190586768395, 84.37609039468570415 ) ) ;
#111226=CARTESIAN_POINT ( 'NONE',  ( -12.14591786802326823, 12.06949235617739902, 33.12609039468569705 ) ) ;
#111227=CARTESIAN_POINT ( 'NONE',  ( 16.46253265017160672, -9.564922557960803928, 98.33224293864769550 ) ) ;
#111229=CARTESIAN_POINT ( 'NONE',  ( 0.05219959533909260263, 19.03943276465977164, 74.99890960531435269 ) ) ;
#111232=CARTESIAN_POINT ( 'NONE',  ( -19.02544592524334988, -5.153800228976617603, 68.95942372801896170 ) ) ;
#111233=CARTESIAN_POINT ( 'NONE',  ( -13.89961937509977652, 13.97604488694528158, 110.6239096053143243 ) ) ;
#111234=CARTESIAN_POINT ( 'NONE',  ( -18.67979575497193778, 10.72451020669871902, 103.3344237280190043 ) ) ;
#111235=CARTESIAN_POINT ( 'NONE',  ( 16.55341960407611168, 4.379528057220329451, 93.95724293864770971 ) ) ;
#111236=CARTESIAN_POINT ( 'NONE',  ( -21.52544592524343514, 5.823673210054127303, 41.04057627198103120 ) ) ;
#111237=CARTESIAN_POINT ( 'NONE',  ( -5.719274019375978568, 21.55341960407610458, 40.20724293864769550 ) ) ;
#111238=CARTESIAN_POINT ( 'NONE',  ( -16.55341960407611168, -4.379528057220339221, 101.4572429386476955 ) ) ;
#111240=CARTESIAN_POINT ( 'NONE',  ( 16.51473224551083163, -9.474510206698727899, 60.83442372801900433 ) ) ;
#111241=CARTESIAN_POINT ( 'NONE',  ( 8.314922557960818139, 14.29746914071049879, 24.58224293864768839 ) ) ;
#111242=CARTESIAN_POINT ( 'NONE',  ( -16.46253265017160317, 9.564922557960807481, 105.8322429386476955 ) ) ;
#111243=CARTESIAN_POINT ( 'NONE',  ( 0.05219959533937995610, -21.53943276465977519, 80.00109039468568994 ) ) ;
#111244=CARTESIAN_POINT ( 'NONE',  ( 21.52544592524344225, -5.823673210054117533, 68.54057627198103830 ) ) ;
#111245=CARTESIAN_POINT ( 'NONE',  ( -15.72974639402176322, -15.80617190586768395, 39.37609039468567573 ) ) ;
#111246=CARTESIAN_POINT ( 'NONE',  ( -21.52544592524343514, 5.823673210054127303, 91.04057627198103830 ) ) ;
#111247=CARTESIAN_POINT ( 'NONE',  ( -0.05219959533937732626, 21.53943276465977519, 47.50109039468568994 ) ) ;
#111248=CARTESIAN_POINT ( 'NONE',  ( -19.05341960407611168, -5.049401038298163336, 31.45724293864769550 ) ) ;
#111249=CARTESIAN_POINT ( 'NONE',  ( -19.03943276465977164, 0.05219959533909376836, 81.24890960531436690 ) ) ;
#111250=CARTESIAN_POINT ( 'NONE',  ( 14.34966873604972726, -8.224510206698740333, 80.83442372801901854 ) ) ;
#111251=CARTESIAN_POINT ( 'NONE',  ( 12.14591786802309770, 12.06949235617756955, 99.37390960531436690 ) ) ;
#111252=CARTESIAN_POINT ( 'NONE',  ( 13.89961937509977652, -13.97604488694527269, 103.1239096053143527 ) ) ;
#111253=CARTESIAN_POINT ( 'NONE',  ( -16.55341960407611168, -4.379528057220339221, 51.45724293864770260 ) ) ;
#111254=CARTESIAN_POINT ( 'NONE',  ( -0.05219959533910754901, -16.53943276465976808, 22.49890960531436335 ) ) ;
#111255=CARTESIAN_POINT ( 'NONE',  ( 16.46253265017160672, -9.564922557960803928, 48.33224293864769550 ) ) ;
#111256=CARTESIAN_POINT ( 'NONE',  ( -13.97604488694527625, -13.89961937509977652, 31.87390960531435979 ) ) ;
#111257=CARTESIAN_POINT ( 'NONE',  ( -21.53943276465977519, 0.05219959533907696930, 41.24890960531435269 ) ) ;
#111258=CARTESIAN_POINT ( 'NONE',  ( 9.564922557961047289, -16.46253265017146816, 25.41775706135234003 ) ) ;
#111259=VECTOR ( 'NONE', #156752, 1000.000000000000000 ) ;
#111260=CARTESIAN_POINT ( 'NONE',  ( -17.48853670773242541, -5.747243402303178428, 41.33328700250010712 ) ) ;
#111261=CARTESIAN_POINT ( 'NONE',  ( 4.483927247898545687, 16.52544592524342804, 34.79057627198103120 ) ) ;
#111262=CARTESIAN_POINT ( 'NONE',  ( 15.80617190586769283, -15.72974639402175789, 40.62609039468567573 ) ) ;
#111264=CARTESIAN_POINT ( 'NONE',  ( 14.34966873604972726, -8.224510206698740333, 60.83442372801901854 ) ) ;
#111265=CARTESIAN_POINT ( 'NONE',  ( 19.03943276465977164, 0.05219959533936151252, 61.25109039468566863 ) ) ;
#111266=CARTESIAN_POINT ( 'NONE',  ( -8.314922557960811034, -14.29746914071050412, 27.08224293864769550 ) ) ;
#111267=CARTESIAN_POINT ( 'NONE',  ( 17.31747979337945154, -6.344076630961154706, 51.12055131934818775 ) ) ;
#111268=CARTESIAN_POINT ( 'NONE',  ( 12.14591786802327356, -12.06949235617739191, 105.6260903946856899 ) ) ;
#111269=CARTESIAN_POINT ( 'NONE',  ( 5.049401038298161559, -19.05341960407611168, 42.70724293864767418 ) ) ;
#111270=CARTESIAN_POINT ( 'NONE',  ( 16.46253265017160672, -9.564922557960803928, 63.33224293864769550 ) ) ;
#111271=CARTESIAN_POINT ( 'NONE',  ( 13.89961937509977652, -13.97604488694527269, 23.12390960531436335 ) ) ;
#111272=CARTESIAN_POINT ( 'NONE',  ( -0.05219959533937732626, 21.53943276465977519, 32.50109039468568284 ) ) ;
#111273=CARTESIAN_POINT ( 'NONE',  ( -16.46253265017160317, 9.564922557960807481, 50.83224293864770260 ) ) ;
#111275=CARTESIAN_POINT ( 'NONE',  ( 0.05219959533909260263, 19.03943276465977164, 49.99890960531435979 ) ) ;
#111276=CARTESIAN_POINT ( 'NONE',  ( 18.67979575497178502, 10.72451020669898547, 24.16557627198103120 ) ) ;
#111277=B_SPLINE_CURVE_WITH_KNOTS ( 'NONE', 3,
 ( #128685, #111541, #175211, #3363, #190382, #49876, #96359, #158047, #159026, #6340, #20519, #82167, #40694, #74031, #165045, #71033, #57865, #42696, #117530, #101346, #10368, #27541, #26538, #88182, #12368, #163035, #8357, #87196, #24542, #86192, #134713, #104357 ),
 .UNSPECIFIED., .F., .F.,
 ( 4, 2, 2, 2, 2, 2, 2, 2, 2, 2, 2, 2, 2, 2, 2, 4 ),
 ( 2.625112965618923374E-17, 0.0003712461730036961563, 0.0007424923460073660749, 0.001113738519011035939, 0.001484984692014705912, 0.002227477038022045858, 0.002598723211025716698, 0.002969969384029387104, 0.003341215557033057511, 0.003712461730036728785, 0.004083707903040398324, 0.004454954076044069164, 0.004826200249047740004, 0.005197446422051409977, 0.005568692595055081684, 0.005939938768058751657 ),
 .UNSPECIFIED. ) ;
#111278=CARTESIAN_POINT ( 'NONE',  ( -15.80617190586768217, 15.72974639402176855, 58.12609039468568994 ) ) ;
#111279=CARTESIAN_POINT ( 'NONE',  ( 14.29746914071049879, -8.314922557960816363, 98.33224293864769550 ) ) ;
#111280=CARTESIAN_POINT ( 'NONE',  ( 9.564922557960805705, 16.46253265017160317, 109.5822429386476955 ) ) ;
#111281=CARTESIAN_POINT ( 'NONE',  ( -0.05219959533934338120, 16.53943276465976808, 77.50109039468567573 ) ) ;
#111282=CARTESIAN_POINT ( 'NONE',  ( 18.62759615963255655, 10.81492255796105972, 96.66775706135234714 ) ) ;
#111283=CARTESIAN_POINT ( 'NONE',  ( 16.55341960407618274, -4.379528057220086978, 56.04275706135235424 ) ) ;
#111284=CARTESIAN_POINT ( 'NONE',  ( -5.049401038298153566, 19.05341960407611168, 95.20724293864770971 ) ) ;
#111285=CARTESIAN_POINT ( 'NONE',  ( 16.55341960407618274, -4.379528057220086978, 41.04275706135236135 ) ) ;
#111286=CARTESIAN_POINT ( 'NONE',  ( -12.14591786802326823, 12.06949235617739902, 28.12609039468568284 ) ) ;
#111287=CARTESIAN_POINT ( 'NONE',  ( -12.14591786802326823, 12.06949235617739902, 98.12609039468570415 ) ) ;
#111288=CARTESIAN_POINT ( 'NONE',  ( -21.52544592524334988, -5.823673210054445271, 48.95942372801902565 ) ) ;
#111289=CARTESIAN_POINT ( 'NONE',  ( 5.153800228976615827, -19.02544592524334988, 100.2094237280190043 ) ) ;
#111290=B_SPLINE_CURVE_WITH_KNOTS ( 'NONE', 3,
 ( #134467, #85943, #12128, #176981, #161790, #101100, #27294, #25305, #162786, #38451, #103120, #132455, #146609, #164801, #26296, #180975, #150632, #87937, #8102, #40445 ),
 .UNSPECIFIED., .F., .F.,
 ( 4, 2, 2, 2, 2, 2, 2, 2, 2, 4 ),
 ( 0.004000878361812008552, 0.004499404418916014975, 0.004997930476020021398, 0.005496456533124028689, 0.005994982590228035112, 0.006244245618780038323, 0.006493508647332041535, 0.006992034704436048825, 0.007490560761540055248, 0.007989086818644061672 ),
 .UNSPECIFIED. ) ;
#111291=CARTESIAN_POINT ( 'NONE',  ( 5.823673210054125526, 21.52544592524343514, 114.7905762719810383 ) ) ;
#111292=CARTESIAN_POINT ( 'NONE',  ( 12.14591786802309770, 12.06949235617756955, 109.3739096053143811 ) ) ;
#111293=CARTESIAN_POINT ( 'NONE',  ( 16.46253265017146816, 9.564922557961045513, 101.6677570613523329 ) ) ;
#111294=CARTESIAN_POINT ( 'NONE',  ( 8.224510206698742110, 14.34966873604972548, 72.08442372801899012 ) ) ;
#111296=CARTESIAN_POINT ( 'NONE',  ( -9.474510206698720793, -16.51473224551083518, 74.58442372801900433 ) ) ;
#111297=CARTESIAN_POINT ( 'NONE',  ( 4.483927247898545687, 16.52544592524342804, 39.79057627198103830 ) ) ;
#111298=CARTESIAN_POINT ( 'NONE',  ( 14.34966873604960469, 8.224510206698951720, 39.16557627198102409 ) ) ;
#111299=CARTESIAN_POINT ( 'NONE',  ( 12.14591786802309770, 12.06949235617756955, 99.37390960531436690 ) ) ;
#111300=CARTESIAN_POINT ( 'NONE',  ( -9.474510206698720793, -16.51473224551083518, 34.58442372801899722 ) ) ;
#111301=CARTESIAN_POINT ( 'NONE',  ( -17.48853670773247160, 5.747243402303041648, 88.66671299749997104 ) ) ;
#111302=CARTESIAN_POINT ( 'NONE',  ( 5.719274019375673035, 21.55341960407619339, 37.29275706135235424 ) ) ;
#111303=CARTESIAN_POINT ( 'NONE',  ( -0.05219959533936034679, 19.03943276465977164, 97.50109039468567573 ) ) ;
#111305=CARTESIAN_POINT ( 'NONE',  ( 5.049401038298161559, -19.05341960407611168, 92.70724293864769550 ) ) ;
#111306=CARTESIAN_POINT ( 'NONE',  ( -13.97604488694527625, -13.89961937509977652, 91.87390960531432427 ) ) ;
#111307=CARTESIAN_POINT ( 'NONE',  ( 21.55341960407610458, 5.719274019375980345, 53.95724293864770260 ) ) ;
#111308=CARTESIAN_POINT ( 'NONE',  ( -4.379528057220328563, 16.55341960407611168, 90.20724293864770971 ) ) ;
#111309=CARTESIAN_POINT ( 'NONE',  ( -5.049401038298153566, 19.05341960407611168, 70.20724293864769550 ) ) ;
#111310=CARTESIAN_POINT ( 'NONE',  ( 9.474510206698971260, -16.51473224551069308, 27.91557627198103120 ) ) ;
#111311=CARTESIAN_POINT ( 'NONE',  ( -5.719274019375665041, -21.55341960407619695, 44.79275706135234714 ) ) ;
#111312=CARTESIAN_POINT ( 'NONE',  ( -0.05219959533937732626, 21.53943276465977519, 77.50109039468567573 ) ) ;
#111313=CARTESIAN_POINT ( 'NONE',  ( -16.51473224551069308, -9.474510206698971260, 51.66557627198102409 ) ) ;
#111314=CARTESIAN_POINT ( 'NONE',  ( 14.34966873604972726, -8.224510206698740333, 85.83442372801901854 ) ) ;
#111315=CARTESIAN_POINT ( 'NONE',  ( -21.52544592524334988, -5.823673210054445271, 28.95942372801902209 ) ) ;
#111316=CARTESIAN_POINT ( 'NONE',  ( 15.72974639402176855, 15.80617190586768217, 21.87609039468567573 ) ) ;
#111317=CARTESIAN_POINT ( 'NONE',  ( 16.51473224551083163, -9.474510206698727899, 50.83442372801899722 ) ) ;
#111318=CARTESIAN_POINT ( 'NONE',  ( -19.03943276465977164, 0.05219959533909376836, 76.24890960531435269 ) ) ;
#111319=CARTESIAN_POINT ( 'NONE',  ( -15.72974639402176322, -15.80617190586768395, 79.37609039468567573 ) ) ;
#111320=CARTESIAN_POINT ( 'NONE',  ( 10.81492255796078972, 18.62759615963270932, 74.58224293864768129 ) ) ;
#111321=CARTESIAN_POINT ( 'NONE',  ( -12.06949235617756955, 12.14591786802309770, 45.62390960531436690 ) ) ;
#111322=CARTESIAN_POINT ( 'NONE',  ( -15.80617190586768217, 15.72974639402176855, 108.1260903946856757 ) ) ;
#111323=CARTESIAN_POINT ( 'NONE',  ( -9.564922557961040184, 16.46253265017147172, 27.91775706135232582 ) ) ;
#111324=CARTESIAN_POINT ( 'NONE',  ( -8.224510206698948167, 14.34966873604960824, 70.41557627198102409 ) ) ;
#111325=CARTESIAN_POINT ( 'NONE',  ( -8.314922557960811034, -14.29746914071050412, 112.0822429386477097 ) ) ;
#111326=CARTESIAN_POINT ( 'NONE',  ( -9.564922557961040184, 16.46253265017147172, 77.91775706135234714 ) ) ;
#111327=CARTESIAN_POINT ( 'NONE',  ( -8.224510206698948167, 14.34966873604960824, 35.41557627198102409 ) ) ;
#111328=CARTESIAN_POINT ( 'NONE',  ( 18.67979575497194134, -10.72451020669871369, 75.83442372801900433 ) ) ;
#111329=CARTESIAN_POINT ( 'NONE',  ( 0.05219959533909260263, 19.03943276465977164, 74.99890960531435269 ) ) ;
#111330=CARTESIAN_POINT ( 'NONE',  ( 16.46253265017146816, 9.564922557961045513, 41.66775706135234003 ) ) ;
#111331=CARTESIAN_POINT ( 'NONE',  ( -10.72451020669898014, 18.67979575497178502, 70.41557627198102409 ) ) ;
#111332=CARTESIAN_POINT ( 'NONE',  ( -21.52544592524343514, 5.823673210054127303, 111.0405762719810525 ) ) ;
#111333=CARTESIAN_POINT ( 'NONE',  ( 12.06949235617739724, 12.14591786802326823, 21.87609039468567573 ) ) ;
#111334=CARTESIAN_POINT ( 'NONE',  ( 16.52544592524335698, 4.483927247898782831, 71.45942372801901854 ) ) ;
#111335=CARTESIAN_POINT ( 'NONE',  ( 16.38665767535053064, 7.295008042176049479, 62.23599135785456582 ) ) ;
#111336=CARTESIAN_POINT ( 'NONE',  ( 21.53943276465977519, -0.05219959533907433946, 108.7489096053143669 ) ) ;
#111337=CARTESIAN_POINT ( 'NONE',  ( 8.224510206698953496, -14.34966873604960469, 107.9155762719810241 ) ) ;
#111338=CARTESIAN_POINT ( 'NONE',  ( 17.50000000000000000, -3.456093896842488800, 22.00000000000000711 ) ) ;
#111339=CARTESIAN_POINT ( 'NONE',  ( -16.53943276465976808, -0.05219959533934237506, 38.75109039468567573 ) ) ;
#111340=CARTESIAN_POINT ( 'NONE',  ( 15.80617190586746368, 15.72974639402197994, 59.37390960531436690 ) ) ;
#111341=CARTESIAN_POINT ( 'NONE',  ( 4.379528057220092307, 16.55341960407617563, 107.2927570613523471 ) ) ;
#111342=CARTESIAN_POINT ( 'NONE',  ( -19.02544592524342804, 5.153800228976336051, 36.04057627198100988 ) ) ;
#111343=CARTESIAN_POINT ( 'NONE',  ( -16.52544592524335698, -4.483927247898792601, 68.95942372801901854 ) ) ;
#111344=CARTESIAN_POINT ( 'NONE',  ( 5.153800228976615827, -19.02544592524334988, 65.20942372801900433 ) ) ;
#111345=CARTESIAN_POINT ( 'NONE',  ( -18.62759615963255300, -10.81492255796106328, 44.16775706135234714 ) ) ;
#111347=CARTESIAN_POINT ( 'NONE',  ( -10.72451020669898014, 18.67979575497178502, 55.41557627198102409 ) ) ;
#111348=CARTESIAN_POINT ( 'NONE',  ( 4.483927247898790824, -16.52544592524335698, 95.20942372801903275 ) ) ;
#111349=CARTESIAN_POINT ( 'NONE',  ( -21.52544592524334988, -5.823673210054445271, 88.95942372801901854 ) ) ;
#111350=CARTESIAN_POINT ( 'NONE',  ( -15.80617190586745835, -15.72974639402198527, 46.87390960531435979 ) ) ;
#111351=CARTESIAN_POINT ( 'NONE',  ( -15.72974639402197994, 15.80617190586746368, 30.62390960531436335 ) ) ;
#111352=VERTEX_POINT ( 'NONE', #48613 ) ;
#111354=CARTESIAN_POINT ( 'NONE',  ( -8.224510206698735004, -14.34966873604973081, 74.58442372801901854 ) ) ;
#111355=CARTESIAN_POINT ( 'NONE',  ( -21.55341960407610458, -5.719274019375992779, 41.45724293864769550 ) ) ;
#111357=CARTESIAN_POINT ( 'NONE',  ( 19.02544592524343514, -5.153800228976328945, 93.54057627198102409 ) ) ;
#111359=CARTESIAN_POINT ( 'NONE',  ( 9.474510206698971260, -16.51473224551069308, 27.91557627198103120 ) ) ;
#111360=CARTESIAN_POINT ( 'NONE',  ( -18.62759615963270932, 10.81492255796079327, 65.83224293864769550 ) ) ;
#111361=CARTESIAN_POINT ( 'NONE',  ( 16.52544592524335698, 4.483927247898782831, 91.45942372801901854 ) ) ;
#111362=CARTESIAN_POINT ( 'NONE',  ( -5.823673210054431948, 21.52544592524334988, 42.70942372801901854 ) ) ;
#111363=CARTESIAN_POINT ( 'NONE',  ( 5.153800228976615827, -19.02544592524334988, 100.2094237280190043 ) ) ;
#111364=CARTESIAN_POINT ( 'NONE',  ( -4.483927247898539470, -16.52544592524342804, 97.29057627198105251 ) ) ;
#111365=CARTESIAN_POINT ( 'NONE',  ( 8.224510206698742110, 14.34966873604972548, 22.08442372801901143 ) ) ;
#111366=VECTOR ( 'NONE', #117938, 1000.000000000000000 ) ;
#111367=CARTESIAN_POINT ( 'NONE',  ( -9.564922557960796823, -16.46253265017161027, 37.08224293864768839 ) ) ;
#111369=CARTESIAN_POINT ( 'NONE',  ( 13.97604488694527802, 13.89961937509977652, 89.37390960531436690 ) ) ;
#111370=CARTESIAN_POINT ( 'NONE',  ( 4.379528057220092307, 16.55341960407617563, 77.29275706135234714 ) ) ;
#111371=CARTESIAN_POINT ( 'NONE',  ( -0.05219959533937732626, 21.53943276465977519, 107.5010903946856899 ) ) ;
#111372=CARTESIAN_POINT ( 'NONE',  ( -10.81492255796078084, -18.62759615963271287, 67.08224293864770971 ) ) ;
#111373=CARTESIAN_POINT ( 'NONE',  ( 8.224510206698742110, 14.34966873604972548, 87.08442372801901854 ) ) ;
#111374=CARTESIAN_POINT ( 'NONE',  ( 16.51473224551083163, -9.474510206698727899, 75.83442372801900433 ) ) ;
#111375=CARTESIAN_POINT ( 'NONE',  ( -19.03943276465977164, 0.05219959533909376836, 36.24890960531436690 ) ) ;
#111376=CARTESIAN_POINT ( 'NONE',  ( 16.51473224551069308, 9.474510206698969483, 74.16557627198103830 ) ) ;
#111378=CARTESIAN_POINT ( 'NONE',  ( -9.474510206698964154, 16.51473224551069663, 35.41557627198102409 ) ) ;
#111379=CARTESIAN_POINT ( 'NONE',  ( 5.049401038297881783, 19.05341960407617563, 77.29275706135231871 ) ) ;
#111381=CARTESIAN_POINT ( 'NONE',  ( -9.564922557960796823, -16.46253265017161027, 107.0822429386476955 ) ) ;
#111382=CARTESIAN_POINT ( 'NONE',  ( -16.53943276465976808, 0.05219959533911058130, 66.24890960531436690 ) ) ;
#111383=CARTESIAN_POINT ( 'NONE',  ( -15.80617190586745835, -15.72974639402198527, 66.87390960531436690 ) ) ;
#111387=CARTESIAN_POINT ( 'NONE',  ( 9.564922557961047289, -16.46253265017146816, 25.41775706135234003 ) ) ;
#111389=CARTESIAN_POINT ( 'NONE',  ( 19.02544592524343514, -5.153800228976328945, 58.54057627198102409 ) ) ;
#111390=CARTESIAN_POINT ( 'NONE',  ( 0.05219959533909260263, 19.03943276465977164, 69.99890960531435269 ) ) ;
#111391=EDGE_CURVE ( 'NONE', #165125, #82999, #3089, .T. ) ;
#111392=CARTESIAN_POINT ( 'NONE',  ( -8.314922557961024197, 14.29746914071037800, 47.91775706135234714 ) ) ;
#111393=CARTESIAN_POINT ( 'NONE',  ( -19.34837522270366250, -5.499999999999802824, 100.8633768483257711 ) ) ;
#111395=CARTESIAN_POINT ( 'NONE',  ( 14.29746914071037800, 8.314922557961029526, 71.66775706135234714 ) ) ;
#111397=CARTESIAN_POINT ( 'NONE',  ( 16.52544592524335698, 4.483927247898782831, 66.45942372801903275 ) ) ;
#111398=CARTESIAN_POINT ( 'NONE',  ( -14.29746914071037622, -8.314922557961029526, 44.16775706135234714 ) ) ;
#111399=CARTESIAN_POINT ( 'NONE',  ( -13.97604488694527625, -13.89961937509977652, 51.87390960531436690 ) ) ;
#111401=CARTESIAN_POINT ( 'NONE',  ( -5.823673210054431948, 21.52544592524334988, 57.70942372801901143 ) ) ;
#111402=CARTESIAN_POINT ( 'NONE',  ( 5.153800228976615827, -19.02544592524334988, 60.20942372801899012 ) ) ;
#111403=CARTESIAN_POINT ( 'NONE',  ( -15.72974639402176322, -15.80617190586768395, 89.37609039468568994 ) ) ;
#111404=CARTESIAN_POINT ( 'NONE',  ( 13.97604488694527802, 13.89961937509977652, 29.37390960531435979 ) ) ;
#111406=CARTESIAN_POINT ( 'NONE',  ( -15.80617190586745835, -15.72974639402198527, 51.87390960531437401 ) ) ;
#111408=CARTESIAN_POINT ( 'NONE',  ( -5.049401038298153566, 19.05341960407611168, 105.2072429386476671 ) ) ;
#111409=CARTESIAN_POINT ( 'NONE',  ( -14.29746914071049879, 8.314922557960819915, 100.8322429386477097 ) ) ;
#111410=CARTESIAN_POINT ( 'NONE',  ( 14.29746914071037800, 8.314922557961029526, 36.66775706135234714 ) ) ;
#111411=CARTESIAN_POINT ( 'NONE',  ( 16.55341960407611168, 4.379528057220329451, 23.95724293864769550 ) ) ;
#111413=CARTESIAN_POINT ( 'NONE',  ( -15.80617190586745835, -15.72974639402198527, 106.8739096053143811 ) ) ;
#111414=CARTESIAN_POINT ( 'NONE',  ( -12.06949235617756955, 12.14591786802309770, 35.62390960531437401 ) ) ;
#111415=CARTESIAN_POINT ( 'NONE',  ( -18.22780087662123805, 5.499999999999981348, 86.01763182126894947 ) ) ;
#111416=CARTESIAN_POINT ( 'NONE',  ( -16.46253265017146816, -9.564922557961047289, 89.16775706135234714 ) ) ;
#111417=CARTESIAN_POINT ( 'NONE',  ( 19.03943276465977164, 0.05219959533936151252, 26.25109039468566507 ) ) ;
#111418=CARTESIAN_POINT ( 'NONE',  ( -4.379528057220328563, 16.55341960407611168, 25.20724293864769550 ) ) ;
#111419=CARTESIAN_POINT ( 'NONE',  ( -21.55341960407610458, -5.719274019375992779, 101.4572429386476955 ) ) ;
#111420=CARTESIAN_POINT ( 'NONE',  ( -10.81492255796078084, -18.62759615963271287, 47.08224293864770260 ) ) ;
#111421=CARTESIAN_POINT ( 'NONE',  ( 5.049401038298161559, -19.05341960407611168, 77.70724293864765286 ) ) ;
#111422=CARTESIAN_POINT ( 'NONE',  ( -14.29746914071049879, 8.314922557960819915, 35.83224293864768839 ) ) ;
#111423=CARTESIAN_POINT ( 'NONE',  ( 19.03943276465977164, -0.05219959533909143690, 88.74890960531436690 ) ) ;
#111425=CARTESIAN_POINT ( 'NONE',  ( 19.53091890409951858, 5.500000000000024869, 57.56097431831420153 ) ) ;
#111426=CARTESIAN_POINT ( 'NONE',  ( -19.02544592524334988, -5.153800228976617603, 43.95942372801899012 ) ) ;
#111427=CARTESIAN_POINT ( 'NONE',  ( 18.67979575497178502, 10.72451020669898547, 79.16557627198103830 ) ) ;
#111428=CARTESIAN_POINT ( 'NONE',  ( 12.14591786802309770, 12.06949235617756955, 94.37390960531436690 ) ) ;
#111429=CARTESIAN_POINT ( 'NONE',  ( -21.53943276465977519, -0.05219959533937600094, 38.75109039468567573 ) ) ;
#111431=CARTESIAN_POINT ( 'NONE',  ( 16.55341960407618274, -4.379528057220086978, 106.0427570613523471 ) ) ;
#111432=CARTESIAN_POINT ( 'NONE',  ( 13.89961937509977652, -13.97604488694527269, 38.12390960531436690 ) ) ;
#111433=CARTESIAN_POINT ( 'NONE',  ( -19.03943276465977164, 0.05219959533909376836, 81.24890960531436690 ) ) ;
#111435=CARTESIAN_POINT ( 'NONE',  ( -13.97604488694527625, -13.89961937509977652, 26.87390960531434558 ) ) ;
#111436=CARTESIAN_POINT ( 'NONE',  ( 16.52544592524342804, -4.483927247898539470, 38.54057627198103120 ) ) ;
#111437=CARTESIAN_POINT ( 'NONE',  ( 5.823673210054444382, -21.52544592524334988, 70.20942372801904696 ) ) ;
#111439=CARTESIAN_POINT ( 'NONE',  ( 16.53943276465976808, 0.05219959533934440121, 71.25109039468568994 ) ) ;
#111440=CARTESIAN_POINT ( 'NONE',  ( -9.474510206698964154, 16.51473224551069663, 50.41557627198102409 ) ) ;
#111441=CARTESIAN_POINT ( 'NONE',  ( 13.89961937509977652, -13.97604488694527269, 63.12390960531435979 ) ) ;
#111443=CARTESIAN_POINT ( 'NONE',  ( 10.72451020669871369, 18.67979575497193778, 102.0844237280190185 ) ) ;
#111444=CARTESIAN_POINT ( 'NONE',  ( 16.52544592524335698, 4.483927247898782831, 76.45942372801901854 ) ) ;
#111445=CARTESIAN_POINT ( 'NONE',  ( 5.719274019375673035, 21.55341960407619339, 97.29275706135234714 ) ) ;
#111446=CARTESIAN_POINT ( 'NONE',  ( -9.474510206698964154, 16.51473224551069663, 60.41557627198102409 ) ) ;
#111447=CARTESIAN_POINT ( 'NONE',  ( -15.72974639402197994, 15.80617190586746368, 35.62390960531437401 ) ) ;
#111448=CARTESIAN_POINT ( 'NONE',  ( 0.05219959533936267826, -19.03943276465977164, 105.0010903946856615 ) ) ;
#111449=CARTESIAN_POINT ( 'NONE',  ( 10.81492255796106328, -18.62759615963255655, 70.41775706135236135 ) ) ;
#111450=CARTESIAN_POINT ( 'NONE',  ( 16.55341960407618274, -4.379528057220086978, 56.04275706135235424 ) ) ;
#111452=CARTESIAN_POINT ( 'NONE',  ( -5.719274019375978568, 21.55341960407610458, 100.2072429386476955 ) ) ;
#111453=CARTESIAN_POINT ( 'NONE',  ( -13.89961937509957401, -13.97604488694547875, 94.37609039468566152 ) ) ;
#111454=CARTESIAN_POINT ( 'NONE',  ( -0.05219959533909027116, -19.03943276465977164, 77.49890960531435269 ) ) ;
#111455=CARTESIAN_POINT ( 'NONE',  ( 16.52544592524335698, 4.483927247898782831, 21.45942372801901499 ) ) ;
#111456=CARTESIAN_POINT ( 'NONE',  ( -14.29746914071037622, -8.314922557961029526, 19.16775706135234714 ) ) ;
#111457=CARTESIAN_POINT ( 'NONE',  ( -8.314922557960811034, -14.29746914071050412, 67.08224293864770971 ) ) ;
#111458=CARTESIAN_POINT ( 'NONE',  ( -16.52544592524335698, -4.483927247898792601, 78.95942372801901854 ) ) ;
#111460=CARTESIAN_POINT ( 'NONE',  ( -21.55341960407610458, -5.719274019375992779, 111.4572429386476813 ) ) ;
#111461=CARTESIAN_POINT ( 'NONE',  ( -16.46253265017160317, 9.564922557960807481, 50.83224293864770260 ) ) ;
#111462=CARTESIAN_POINT ( 'NONE',  ( 9.564922557960805705, 16.46253265017160317, 64.58224293864769550 ) ) ;
#111463=CARTESIAN_POINT ( 'NONE',  ( -16.55341960407617563, 4.379528057220093196, 78.54275706135236135 ) ) ;
#111466=CARTESIAN_POINT ( 'NONE',  ( -10.81492255796105439, 18.62759615963255655, 107.9177570613523471 ) ) ;
#111467=CARTESIAN_POINT ( 'NONE',  ( -13.89961937509977652, 13.97604488694528158, 35.62390960531435269 ) ) ;
#111469=CARTESIAN_POINT ( 'NONE',  ( 5.153800228976615827, -19.02544592524334988, 105.2094237280190185 ) ) ;
#111470=CARTESIAN_POINT ( 'NONE',  ( -16.46253265017146816, -9.564922557961047289, 39.16775706135234003 ) ) ;
#111471=CARTESIAN_POINT ( 'NONE',  ( 16.52544592524335698, 4.483927247898782831, 31.45942372801901854 ) ) ;
#111472=CARTESIAN_POINT ( 'NONE',  ( 19.02544592524343514, -5.153800228976328945, 43.54057627198103120 ) ) ;
#111473=CARTESIAN_POINT ( 'NONE',  ( -19.05341960407611168, -5.049401038298163336, 61.45724293864769550 ) ) ;
#111474=CARTESIAN_POINT ( 'NONE',  ( 5.823673210054125526, 21.52544592524343514, 79.79057627198102409 ) ) ;
#111476=CARTESIAN_POINT ( 'NONE',  ( -19.02544592524342804, 5.153800228976336051, 56.04057627198100988 ) ) ;
#111477=CARTESIAN_POINT ( 'NONE',  ( 17.50000000000000000, -5.500000000000000888, 120.0000000000000142 ) ) ;
#111478=CARTESIAN_POINT ( 'NONE',  ( -0.05219959533936034679, 19.03943276465977164, 92.50109039468566152 ) ) ;
#111479=CARTESIAN_POINT ( 'NONE',  ( 4.483927247898545687, 16.52544592524342804, 69.79057627198102409 ) ) ;
#111480=CARTESIAN_POINT ( 'NONE',  ( -0.05219959533936034679, 19.03943276465977164, 27.50109039468566507 ) ) ;
#111481=CARTESIAN_POINT ( 'NONE',  ( 8.314922557960818139, 14.29746914071049879, 59.58224293864770260 ) ) ;
#111482=CARTESIAN_POINT ( 'NONE',  ( -15.80617190586768217, 15.72974639402176855, 83.12609039468568994 ) ) ;
#111483=CARTESIAN_POINT ( 'NONE',  ( -5.153800228976328057, -19.02544592524343514, 27.29057627198103120 ) ) ;
#111484=CARTESIAN_POINT ( 'NONE',  ( 5.823673210054444382, -21.52544592524334988, 95.20942372801903275 ) ) ;
#111485=CARTESIAN_POINT ( 'NONE',  ( 8.314922557960818139, 14.29746914071049879, 24.58224293864768839 ) ) ;
#111486=CARTESIAN_POINT ( 'NONE',  ( 15.80617190586769283, -15.72974639402175789, 75.62609039468567573 ) ) ;
#111487=CARTESIAN_POINT ( 'NONE',  ( 13.97604488694527802, 13.89961937509977652, 84.37390960531433848 ) ) ;
#111488=CARTESIAN_POINT ( 'NONE',  ( 10.72451020669871369, 18.67979575497193778, 37.08442372801901143 ) ) ;
#111489=CARTESIAN_POINT ( 'NONE',  ( 5.049401038298161559, -19.05341960407611168, 77.70724293864765286 ) ) ;
#111490=CARTESIAN_POINT ( 'NONE',  ( -16.52544592524342804, 4.483927247898546575, 91.04057627198103830 ) ) ;
#111491=CARTESIAN_POINT ( 'NONE',  ( -14.34966873604960291, -8.224510206698953496, 66.66557627198102409 ) ) ;
#111492=CARTESIAN_POINT ( 'NONE',  ( 21.53943276465977519, -0.05219959533907433946, 68.74890960531435269 ) ) ;
#111493=CARTESIAN_POINT ( 'NONE',  ( -5.049401038298153566, 19.05341960407611168, 80.20724293864769550 ) ) ;
#111494=CARTESIAN_POINT ( 'NONE',  ( -10.72451020669898014, 18.67979575497178502, 85.41557627198102409 ) ) ;
#111495=CARTESIAN_POINT ( 'NONE',  ( 9.564922557961047289, -16.46253265017146816, 75.41775706135234714 ) ) ;
#111496=CARTESIAN_POINT ( 'NONE',  ( 13.89961937509957579, 13.97604488694547520, 31.87609039468566863 ) ) ;
#111497=CARTESIAN_POINT ( 'NONE',  ( -16.52544592524342804, 4.483927247898546575, 81.04057627198102409 ) ) ;
#111498=CARTESIAN_POINT ( 'NONE',  ( 0.05219959533907565091, 21.53943276465977519, 49.99890960531437401 ) ) ;
#111499=CARTESIAN_POINT ( 'NONE',  ( -18.09918380851992126, -5.500000000000039968, 41.48618307335612343 ) ) ;
#111500=CARTESIAN_POINT ( 'NONE',  ( -4.379528057220086978, -16.55341960407618274, 94.79275706135234714 ) ) ;
#111502=CARTESIAN_POINT ( 'NONE',  ( 13.97604488694548053, -13.89961937509957401, 105.6260903946856757 ) ) ;
#111503=CARTESIAN_POINT ( 'NONE',  ( -8.224510206698948167, 14.34966873604960824, 65.41557627198102409 ) ) ;
#111504=CARTESIAN_POINT ( 'NONE',  ( -19.01529144963335582, -5.500000000000032863, 96.23431955728437970 ) ) ;
#111505=CARTESIAN_POINT ( 'NONE',  ( 13.89961937509977652, -13.97604488694527269, 58.12390960531436690 ) ) ;
#111506=CARTESIAN_POINT ( 'NONE',  ( -4.379528057220328563, 16.55341960407611168, 50.20724293864769550 ) ) ;
#111507=CARTESIAN_POINT ( 'NONE',  ( 5.153800228976335163, 19.02544592524342804, 104.7905762719809957 ) ) ;
#111508=CARTESIAN_POINT ( 'NONE',  ( -0.05219959533936034679, 19.03943276465977164, 87.50109039468567573 ) ) ;
#111509=CARTESIAN_POINT ( 'NONE',  ( 9.564922557960805705, 16.46253265017160317, 69.58224293864770971 ) ) ;
#111510=CARTESIAN_POINT ( 'NONE',  ( 0.05219959533909260263, 19.03943276465977164, 89.99890960531436690 ) ) ;
#111511=CARTESIAN_POINT ( 'NONE',  ( -9.474510206698964154, 16.51473224551069663, 85.41557627198102409 ) ) ;
#111512=CARTESIAN_POINT ( 'NONE',  ( 21.52544592524344225, -5.823673210054117533, 58.54057627198103120 ) ) ;
#111513=CARTESIAN_POINT ( 'NONE',  ( -16.53943276465976808, -0.05219959533934237506, 58.75109039468568994 ) ) ;
#111515=CARTESIAN_POINT ( 'NONE',  ( 13.97604488694548053, -13.89961937509957401, 105.6260903946856757 ) ) ;
#111516=CARTESIAN_POINT ( 'NONE',  ( -13.89961937509977652, 13.97604488694528158, 60.62390960531436690 ) ) ;
#111517=CARTESIAN_POINT ( 'NONE',  ( 18.62759615963271287, -10.81492255796078972, 73.33224293864769550 ) ) ;
#111518=CARTESIAN_POINT ( 'NONE',  ( -19.02544592524334988, -5.153800228976617603, 98.95942372801900433 ) ) ;
#111519=CARTESIAN_POINT ( 'NONE',  ( -16.53943276465976808, 0.05219959533911058130, 26.24890960531435624 ) ) ;
#111520=CARTESIAN_POINT ( 'NONE',  ( 18.67979575497194134, -10.72451020669871369, 45.83442372801901854 ) ) ;
#111521=CARTESIAN_POINT ( 'NONE',  ( -19.05341960407617563, 5.049401038297882671, 43.54275706135232582 ) ) ;
#111523=CARTESIAN_POINT ( 'NONE',  ( -12.06949235617739369, -12.14591786802326823, 59.37609039468568284 ) ) ;
#111524=CARTESIAN_POINT ( 'NONE',  ( -16.52544592524335698, -4.483927247898792601, 93.95942372801903275 ) ) ;
#111526=CARTESIAN_POINT ( 'NONE',  ( 0.05219959533934541429, -16.53943276465976808, 80.00109039468568994 ) ) ;
#111527=CARTESIAN_POINT ( 'NONE',  ( -4.483927247898782831, 16.52544592524335698, 37.70942372801900433 ) ) ;
#111528=CARTESIAN_POINT ( 'NONE',  ( 19.03943276465977164, -0.05219959533909143690, 48.74890960531435979 ) ) ;
#111529=CARTESIAN_POINT ( 'NONE',  ( 19.02544592524343514, -5.153800228976328945, 53.54057627198102409 ) ) ;
#111530=CARTESIAN_POINT ( 'NONE',  ( 16.51473224551069308, 9.474510206698969483, 54.16557627198103120 ) ) ;
#111531=CARTESIAN_POINT ( 'NONE',  ( -10.72451020669870658, -18.67979575497194134, 59.58442372801901854 ) ) ;
#111532=CARTESIAN_POINT ( 'NONE',  ( -14.29746914071037622, -8.314922557961029526, 54.16775706135235424 ) ) ;
#111533=CARTESIAN_POINT ( 'NONE',  ( 12.06949235617757843, -12.14591786802309237, 23.12390960531436335 ) ) ;
#111534=CARTESIAN_POINT ( 'NONE',  ( 5.049401038298161559, -19.05341960407611168, 32.70724293864768129 ) ) ;
#111535=CARTESIAN_POINT ( 'NONE',  ( -9.474510206698964154, 16.51473224551069663, 40.41557627198103120 ) ) ;
#111536=CARTESIAN_POINT ( 'NONE',  ( -14.29746914071037622, -8.314922557961029526, 29.16775706135234003 ) ) ;
#111537=CARTESIAN_POINT ( 'NONE',  ( -5.049401038297874678, -19.05341960407617918, 84.79275706135233293 ) ) ;
#111538=CARTESIAN_POINT ( 'NONE',  ( 4.379528057220339221, -16.55341960407611168, 87.70724293864769550 ) ) ;
#111539=CARTESIAN_POINT ( 'NONE',  ( 19.03943276465977164, -0.05219959533909143690, 33.74890960531435979 ) ) ;
#111540=CARTESIAN_POINT ( 'NONE',  ( -9.474510206698720793, -16.51473224551083518, 74.58442372801900433 ) ) ;
#111541=CARTESIAN_POINT ( 'NONE',  ( 17.49999999999999645, 5.624438216177603422, 76.68329655085356933 ) ) ;
#111542=CARTESIAN_POINT ( 'NONE',  ( -15.80617190586768217, 15.72974639402176855, 78.12609039468570415 ) ) ;
#111543=CARTESIAN_POINT ( 'NONE',  ( 14.29746914071037800, 8.314922557961029526, 36.66775706135234714 ) ) ;
#111544=CARTESIAN_POINT ( 'NONE',  ( -17.49999999999998934, 3.471454075611624113, 24.48332581144370934 ) ) ;
#111545=CARTESIAN_POINT ( 'NONE',  ( 18.62759615963271287, -10.81492255796078972, 38.33224293864768839 ) ) ;
#111546=CARTESIAN_POINT ( 'NONE',  ( 12.14591786802327356, -12.06949235617739191, 20.62609039468568639 ) ) ;
#111547=CARTESIAN_POINT ( 'NONE',  ( 19.02544592524343514, -5.153800228976328945, 28.54057627198103120 ) ) ;
#111548=CARTESIAN_POINT ( 'NONE',  ( -13.97604488694547697, 13.89961937509957934, 33.12609039468566863 ) ) ;
#111550=CARTESIAN_POINT ( 'NONE',  ( 19.05341960407611168, 5.049401038298154454, 33.95724293864769550 ) ) ;
#111552=CARTESIAN_POINT ( 'NONE',  ( -19.05341960407611168, -5.049401038298163336, 66.45724293864769550 ) ) ;
#111553=CARTESIAN_POINT ( 'NONE',  ( 17.50000000000000000, -5.500000000000000000, 111.2176903769643559 ) ) ;
#111555=CARTESIAN_POINT ( 'NONE',  ( -10.72451020669870658, -18.67979575497194134, 109.5844237280190328 ) ) ;
#111556=CARTESIAN_POINT ( 'NONE',  ( -12.14591786802309592, -12.06949235617757132, 31.87390960531435979 ) ) ;
#111557=CARTESIAN_POINT ( 'NONE',  ( 9.564922557960805705, 16.46253265017160317, 44.58224293864769550 ) ) ;
#111558=CARTESIAN_POINT ( 'NONE',  ( -13.97604488694527625, -13.89961937509977652, 86.87390960531436690 ) ) ;
#111559=CARTESIAN_POINT ( 'NONE',  ( -18.62759615963255300, -10.81492255796106328, 69.16775706135234714 ) ) ;
#111560=CARTESIAN_POINT ( 'NONE',  ( -16.46253265017160317, 9.564922557960807481, 45.83224293864769550 ) ) ;
#111562=CARTESIAN_POINT ( 'NONE',  ( 21.53943276465977519, 0.05219959533937863772, 61.25109039468567573 ) ) ;
#111563=CARTESIAN_POINT ( 'NONE',  ( 21.53943276465977519, -0.05219959533907433946, 23.74890960531435269 ) ) ;
#111564=CARTESIAN_POINT ( 'NONE',  ( -13.97604488694527625, -13.89961937509977652, 31.87390960531435979 ) ) ;
#111565=CARTESIAN_POINT ( 'NONE',  ( -18.67979575497193778, 10.72451020669871902, 23.33442372801901499 ) ) ;
#111566=CARTESIAN_POINT ( 'NONE',  ( -16.51473224551082808, 9.474510206698731452, 48.33442372801900433 ) ) ;
#111567=CARTESIAN_POINT ( 'NONE',  ( -19.03943276465977164, 0.05219959533909376836, 21.24890960531436335 ) ) ;
#111568=CARTESIAN_POINT ( 'NONE',  ( -9.564922557960796823, -16.46253265017161027, 57.08224293864769550 ) ) ;
#111569=CARTESIAN_POINT ( 'NONE',  ( -19.03943276465977164, -0.05219959533935918106, 113.7510903946856757 ) ) ;
#111570=CARTESIAN_POINT ( 'NONE',  ( -8.314922557960811034, -14.29746914071050412, 82.08224293864768129 ) ) ;
#111571=CARTESIAN_POINT ( 'NONE',  ( 10.72451020669898902, -18.67979575497178502, 27.91557627198103830 ) ) ;
#111572=CARTESIAN_POINT ( 'NONE',  ( -16.46253265017146816, -9.564922557961047289, 99.16775706135233293 ) ) ;
#111573=CARTESIAN_POINT ( 'NONE',  ( 18.67979575497178502, 10.72451020669898547, 109.1655762719810383 ) ) ;
#111574=CARTESIAN_POINT ( 'NONE',  ( 18.62759615963255655, 10.81492255796105972, 51.66775706135234714 ) ) ;
#111575=CARTESIAN_POINT ( 'NONE',  ( 14.29746914071037800, 8.314922557961029526, 56.66775706135235424 ) ) ;
#111576=CARTESIAN_POINT ( 'NONE',  ( 8.314922557961029526, -14.29746914071037800, 55.41775706135234714 ) ) ;
#111577=CARTESIAN_POINT ( 'NONE',  ( -18.62759615963270932, 10.81492255796079327, 50.83224293864770971 ) ) ;
#111578=CARTESIAN_POINT ( 'NONE',  ( -16.51473224551069308, -9.474510206698971260, 51.66557627198102409 ) ) ;
#111579=CARTESIAN_POINT ( 'NONE',  ( 16.53943276465976808, 0.05219959533934440121, 81.25109039468568994 ) ) ;
#111580=CARTESIAN_POINT ( 'NONE',  ( 18.67979575497178502, 10.72451020669898547, 104.1655762719810241 ) ) ;
#111581=CARTESIAN_POINT ( 'NONE',  ( -16.52544592524342804, 4.483927247898546575, 46.04057627198103830 ) ) ;
#111582=CARTESIAN_POINT ( 'NONE',  ( 19.02544592524343514, -5.153800228976328945, 68.54057627198103830 ) ) ;
#111583=CARTESIAN_POINT ( 'NONE',  ( -14.29746914071037622, -8.314922557961029526, 79.16775706135234714 ) ) ;
#111584=CARTESIAN_POINT ( 'NONE',  ( -16.55341960407617563, 4.379528057220093196, 23.54275706135235424 ) ) ;
#111585=CARTESIAN_POINT ( 'NONE',  ( 21.52544592524344225, -5.823673210054117533, 98.54057627198105251 ) ) ;
#111586=CARTESIAN_POINT ( 'NONE',  ( 8.314922557960818139, 14.29746914071049879, 44.58224293864769550 ) ) ;
#111588=CARTESIAN_POINT ( 'NONE',  ( -16.61371651742600974, 7.165104196376139711, 73.85415069993000259 ) ) ;
#111589=CARTESIAN_POINT ( 'NONE',  ( -0.05219959533907301413, -21.53943276465977519, 82.49890960531436690 ) ) ;
#111590=CARTESIAN_POINT ( 'NONE',  ( -0.05219959533910754901, -16.53943276465976808, 32.49890960531435979 ) ) ;
#111593=CARTESIAN_POINT ( 'NONE',  ( 10.72451020669898902, -18.67979575497178502, 102.9155762719810383 ) ) ;
#111595=CARTESIAN_POINT ( 'NONE',  ( -13.97604488694527625, -13.89961937509977652, 96.87390960531433848 ) ) ;
#111596=CARTESIAN_POINT ( 'NONE',  ( 5.823673210054125526, 21.52544592524343514, 114.7905762719810383 ) ) ;
#111597=CARTESIAN_POINT ( 'NONE',  ( -4.483927247898539470, -16.52544592524342804, 37.29057627198102409 ) ) ;
#111599=CARTESIAN_POINT ( 'NONE',  ( -16.53943276465976808, -0.05219959533934237506, 43.75109039468568284 ) ) ;
#111600=CARTESIAN_POINT ( 'NONE',  ( -13.89961937509977652, 13.97604488694528158, 50.62390960531435979 ) ) ;
#111601=CARTESIAN_POINT ( 'NONE',  ( -5.049401038297874678, -19.05341960407617918, 49.79275706135231871 ) ) ;
#111602=CARTESIAN_POINT ( 'NONE',  ( 9.474510206698971260, -16.51473224551069308, 77.91557627198103830 ) ) ;
#111604=CARTESIAN_POINT ( 'NONE',  ( 5.823673210054125526, 21.52544592524343514, 29.79057627198102409 ) ) ;
#111606=CARTESIAN_POINT ( 'NONE',  ( 4.483927247898790824, -16.52544592524335698, 30.20942372801902565 ) ) ;
#111607=CARTESIAN_POINT ( 'NONE',  ( 5.049401038297881783, 19.05341960407617563, 47.29275706135231161 ) ) ;
#111608=CARTESIAN_POINT ( 'NONE',  ( 10.81492255796078972, 18.62759615963270932, 104.5822429386477097 ) ) ;
#111609=CARTESIAN_POINT ( 'NONE',  ( -12.06949235617756955, 12.14591786802309770, 30.62390960531436335 ) ) ;
#111610=CARTESIAN_POINT ( 'NONE',  ( 5.153800228976335163, 19.02544592524342804, 74.79057627198103830 ) ) ;
#111611=CARTESIAN_POINT ( 'NONE',  ( -5.719274019375978568, 21.55341960407610458, 55.20724293864770260 ) ) ;
#111612=CARTESIAN_POINT ( 'NONE',  ( 5.823673210054125526, 21.52544592524343514, 89.79057627198103830 ) ) ;
#111613=CARTESIAN_POINT ( 'NONE',  ( -16.53943276465976808, -0.05219959533934237506, 18.75109039468568639 ) ) ;
#111614=CARTESIAN_POINT ( 'NONE',  ( -21.53943276465977519, 0.05219959533907696930, 26.24890960531435624 ) ) ;
#111615=CARTESIAN_POINT ( 'NONE',  ( 15.72974639402176855, 15.80617190586768217, 91.87609039468568994 ) ) ;
#111616=CARTESIAN_POINT ( 'NONE',  ( -19.03943276465977164, 0.05219959533909376836, 76.24890960531435269 ) ) ;
#111617=CARTESIAN_POINT ( 'NONE',  ( -16.51473224551069308, -9.474510206698971260, 31.66557627198102054 ) ) ;
#111618=CARTESIAN_POINT ( 'NONE',  ( 0.05219959533909260263, 19.03943276465977164, 89.99890960531436690 ) ) ;
#111619=CARTESIAN_POINT ( 'NONE',  ( 14.34966873604960469, 8.224510206698951720, 109.1655762719810383 ) ) ;
#111620=CARTESIAN_POINT ( 'NONE',  ( 19.05341960407611168, 5.049401038298154454, 68.95724293864769550 ) ) ;
#111621=CARTESIAN_POINT ( 'NONE',  ( 9.564922557961047289, -16.46253265017146816, 100.4177570613523329 ) ) ;
#111622=CARTESIAN_POINT ( 'NONE',  ( 17.50000000000001421, 3.565345528327899416, 33.07505513193528657 ) ) ;
#111623=CARTESIAN_POINT ( 'NONE',  ( -5.049401038298153566, 19.05341960407611168, 70.20724293864769550 ) ) ;
#111624=CARTESIAN_POINT ( 'NONE',  ( 10.72451020669871369, 18.67979575497193778, 102.0844237280190185 ) ) ;
#111625=CARTESIAN_POINT ( 'NONE',  ( 15.80617190586746368, 15.72974639402197994, 24.37390960531435979 ) ) ;
#111626=CARTESIAN_POINT ( 'NONE',  ( -0.05219959533934338120, 16.53943276465976808, 97.50109039468567573 ) ) ;
#111628=CARTESIAN_POINT ( 'NONE',  ( 19.02544592524334988, 5.153800228976608722, 71.45942372801900433 ) ) ;
#111629=CARTESIAN_POINT ( 'NONE',  ( -18.67979575497193778, 10.72451020669871902, 108.3344237280190185 ) ) ;
#111630=DIRECTION ( 'NONE',  ( 0.5150380749100522682, 0.000000000000000000, -0.8571673007021134438 ) ) ;
#111631=CARTESIAN_POINT ( 'NONE',  ( 19.02544592524343514, -5.153800228976328945, 23.54057627198102054 ) ) ;
#111632=CARTESIAN_POINT ( 'NONE',  ( 12.06949235617757843, -12.14591786802309237, 23.12390960531436335 ) ) ;
#111634=CARTESIAN_POINT ( 'NONE',  ( 12.06949235617739724, 12.14591786802326823, 106.8760903946856899 ) ) ;
#111636=CARTESIAN_POINT ( 'NONE',  ( 8.314922557961029526, -14.29746914071037800, 75.41775706135233293 ) ) ;
#111637=CARTESIAN_POINT ( 'NONE',  ( -5.049401038298153566, 19.05341960407611168, 40.20724293864768839 ) ) ;
#111638=CARTESIAN_POINT ( 'NONE',  ( 18.62759615963255655, 10.81492255796105972, 91.66775706135234714 ) ) ;
#111639=CARTESIAN_POINT ( 'NONE',  ( -5.049401038297874678, -19.05341960407617918, 99.79275706135234714 ) ) ;
#111640=CARTESIAN_POINT ( 'NONE',  ( 21.55341960407619695, -5.719274019375665929, 66.04275706135236135 ) ) ;
#111641=CARTESIAN_POINT ( 'NONE',  ( -9.564922557961040184, 16.46253265017147172, 47.91775706135233293 ) ) ;
#111642=CARTESIAN_POINT ( 'NONE',  ( 5.049401038298161559, -19.05341960407611168, 72.70724293864768129 ) ) ;
#111643=CARTESIAN_POINT ( 'NONE',  ( -9.474510206698964154, 16.51473224551069663, 65.41557627198102409 ) ) ;
#111644=CARTESIAN_POINT ( 'NONE',  ( 17.49999999999999645, 5.624438216177600758, 71.68329655085361196 ) ) ;
#111645=CARTESIAN_POINT ( 'NONE',  ( -4.483927247898539470, -16.52544592524342804, 52.29057627198102409 ) ) ;
#111646=CARTESIAN_POINT ( 'NONE',  ( 10.72451020669898902, -18.67979575497178502, 42.91557627198103120 ) ) ;
#111647=CARTESIAN_POINT ( 'NONE',  ( -16.46253265017160317, 9.564922557960807481, 50.83224293864770260 ) ) ;
#111648=CARTESIAN_POINT ( 'NONE',  ( -10.81492255796078084, -18.62759615963271287, 82.08224293864768129 ) ) ;
#111649=CARTESIAN_POINT ( 'NONE',  ( 14.34966873604972726, -8.224510206698740333, 70.83442372801901854 ) ) ;
#111651=VERTEX_POINT ( 'NONE', #63773 ) ;
#111652=CARTESIAN_POINT ( 'NONE',  ( -16.52544592524342804, 4.483927247898546575, 76.04057627198102409 ) ) ;
#111654=CARTESIAN_POINT ( 'NONE',  ( 4.483927247898790824, -16.52544592524335698, 35.20942372801901854 ) ) ;
#111655=CARTESIAN_POINT ( 'NONE',  ( 13.89961937509977652, -13.97604488694527269, 28.12390960531435624 ) ) ;
#111656=CARTESIAN_POINT ( 'NONE',  ( -16.51473224551082808, 9.474510206698731452, 63.33442372801900433 ) ) ;
#111657=CARTESIAN_POINT ( 'NONE',  ( 16.55341960407611168, 4.379528057220329451, 68.95724293864769550 ) ) ;
#111658=CARTESIAN_POINT ( 'NONE',  ( -5.719274019375665041, -21.55341960407619695, 49.79275706135234714 ) ) ;
#111659=CARTESIAN_POINT ( 'NONE',  ( 5.153800228976335163, 19.02544592524342804, 24.79057627198102765 ) ) ;
#111660=CARTESIAN_POINT ( 'NONE',  ( -5.719274019375978568, 21.55341960407610458, 90.20724293864770971 ) ) ;
#111661=CARTESIAN_POINT ( 'NONE',  ( -19.02544592524342804, 5.153800228976336051, 111.0405762719810099 ) ) ;
#111662=CARTESIAN_POINT ( 'NONE',  ( 8.224510206698953496, -14.34966873604960469, 92.91557627198103830 ) ) ;
#111664=CARTESIAN_POINT ( 'NONE',  ( -5.153800228976328057, -19.02544592524343514, 47.29057627198102409 ) ) ;
#111666=CARTESIAN_POINT ( 'NONE',  ( 16.51473224551083163, -9.474510206698727899, 85.83442372801900433 ) ) ;
#111667=CARTESIAN_POINT ( 'NONE',  ( -21.53943276465977519, -0.05219959533937600094, 23.75109039468567929 ) ) ;
#111668=CARTESIAN_POINT ( 'NONE',  ( 5.049401038298161559, -19.05341960407611168, 67.70724293864769550 ) ) ;
#111669=CARTESIAN_POINT ( 'NONE',  ( 19.05341960407617918, -5.049401038297876454, 51.04275706135231871 ) ) ;
#111670=CARTESIAN_POINT ( 'NONE',  ( 19.05341960407611168, 5.049401038298154454, 48.95724293864768129 ) ) ;
#111672=CARTESIAN_POINT ( 'NONE',  ( -14.34966873604960291, -8.224510206698953496, 56.66557627198103830 ) ) ;
#111673=CARTESIAN_POINT ( 'NONE',  ( 0.05219959533910956823, 16.53943276465976808, 59.99890960531436690 ) ) ;
#111674=CARTESIAN_POINT ( 'NONE',  ( -13.97604488694527625, -13.89961937509977652, 76.87390960531433848 ) ) ;
#111675=CARTESIAN_POINT ( 'NONE',  ( -0.05219959533907301413, -21.53943276465977519, 107.4989096053143669 ) ) ;
#111676=CARTESIAN_POINT ( 'NONE',  ( 19.02544592524343514, -5.153800228976328945, 73.54057627198103830 ) ) ;
#111677=CARTESIAN_POINT ( 'NONE',  ( -18.67979575497178146, -10.72451020669898902, 81.66557627198103830 ) ) ;
#111678=CARTESIAN_POINT ( 'NONE',  ( 15.72974639402176855, 15.80617190586768217, 106.8760903946856899 ) ) ;
#111679=CARTESIAN_POINT ( 'NONE',  ( 9.564922557960805705, 16.46253265017160317, 39.58224293864768839 ) ) ;
#111680=CARTESIAN_POINT ( 'NONE',  ( -14.34966873604972548, 8.224510206698743886, 103.3344237280190043 ) ) ;
#111681=CARTESIAN_POINT ( 'NONE',  ( -8.314922557960811034, -14.29746914071050412, 102.0822429386476955 ) ) ;
#111682=CARTESIAN_POINT ( 'NONE',  ( -19.03943276465977164, -0.05219959533935918106, 103.7510903946856757 ) ) ;
#111683=ORIENTED_EDGE ( 'NONE', *, *, #79441, .F. ) ;
#111684=CARTESIAN_POINT ( 'NONE',  ( 18.62759615963255655, 10.81492255796105972, 36.66775706135234714 ) ) ;
#111685=CARTESIAN_POINT ( 'NONE',  ( -13.97604488694547697, 13.89961937509957934, 48.12609039468566863 ) ) ;
#111686=CARTESIAN_POINT ( 'NONE',  ( -16.53943276465976808, -0.05219959533934237506, 108.7510903946857042 ) ) ;
#111687=CARTESIAN_POINT ( 'NONE',  ( 21.52544592524344225, -5.823673210054117533, 73.54057627198102409 ) ) ;
#111688=CARTESIAN_POINT ( 'NONE',  ( -5.153800228976328057, -19.02544592524343514, 107.2905762719810383 ) ) ;
#111689=CARTESIAN_POINT ( 'NONE',  ( 8.314922557960818139, 14.29746914071049879, 59.58224293864770260 ) ) ;
#111690=CARTESIAN_POINT ( 'NONE',  ( 9.564922557960805705, 16.46253265017160317, 24.58224293864769194 ) ) ;
#111691=CARTESIAN_POINT ( 'NONE',  ( 13.89961937509977652, -13.97604488694527269, 28.12390960531435624 ) ) ;
#111692=CARTESIAN_POINT ( 'NONE',  ( -5.719274019375665041, -21.55341960407619695, 109.7927570613523613 ) ) ;
#111693=CARTESIAN_POINT ( 'NONE',  ( -12.14591786802326823, 12.06949235617739902, 88.12609039468570415 ) ) ;
#111694=CARTESIAN_POINT ( 'NONE',  ( -18.67979575497193778, 10.72451020669871902, 38.33442372801900433 ) ) ;
#111695=CARTESIAN_POINT ( 'NONE',  ( 8.314922557961029526, -14.29746914071037800, 40.41775706135234714 ) ) ;
#111696=CARTESIAN_POINT ( 'NONE',  ( 9.474510206698971260, -16.51473224551069308, 112.9155762719810383 ) ) ;
#111697=CARTESIAN_POINT ( 'NONE',  ( 13.89961937509977652, -13.97604488694527269, 53.12390960531434558 ) ) ;
#111698=CARTESIAN_POINT ( 'NONE',  ( 19.02544592524343514, -5.153800228976328945, 73.54057627198103830 ) ) ;
#111700=CARTESIAN_POINT ( 'NONE',  ( 4.379528057220092307, 16.55341960407617563, 62.29275706135236845 ) ) ;
#111701=CARTESIAN_POINT ( 'NONE',  ( -12.06949235617756955, 12.14591786802309770, 100.6239096053143811 ) ) ;
#111702=CARTESIAN_POINT ( 'NONE',  ( -14.29746914071049879, 8.314922557960819915, 25.83224293864769194 ) ) ;
#111704=CARTESIAN_POINT ( 'NONE',  ( 21.52544592524334988, 5.823673210054432836, 61.45942372801901854 ) ) ;
#111705=CARTESIAN_POINT ( 'NONE',  ( 9.564922557960805705, 16.46253265017160317, 94.58224293864769550 ) ) ;
#111706=CARTESIAN_POINT ( 'NONE',  ( 13.89961937509977652, -13.97604488694527269, 83.12390960531436690 ) ) ;
#111707=CARTESIAN_POINT ( 'NONE',  ( 16.46253265017160672, -9.564922557960803928, 108.3322429386476955 ) ) ;
#111708=CARTESIAN_POINT ( 'NONE',  ( -4.379528057220328563, 16.55341960407611168, 50.20724293864769550 ) ) ;
#111709=CARTESIAN_POINT ( 'NONE',  ( 4.379528057220092307, 16.55341960407617563, 112.2927570613523471 ) ) ;
#111710=CARTESIAN_POINT ( 'NONE',  ( -4.379528057220328563, 16.55341960407611168, 45.20724293864769550 ) ) ;
#111712=CARTESIAN_POINT ( 'NONE',  ( 16.46253265017146816, 9.564922557961045513, 31.66775706135232937 ) ) ;
#111713=CARTESIAN_POINT ( 'NONE',  ( -5.049401038298153566, 19.05341960407611168, 75.20724293864769550 ) ) ;
#111714=CARTESIAN_POINT ( 'NONE',  ( -13.97604488694547697, 13.89961937509957934, 58.12609039468566863 ) ) ;
#111717=CARTESIAN_POINT ( 'NONE',  ( -5.049401038297874678, -19.05341960407617918, 89.79275706135230450 ) ) ;
#111718=CARTESIAN_POINT ( 'NONE',  ( 14.29746914071037800, 8.314922557961029526, 71.66775706135234714 ) ) ;
#111719=CARTESIAN_POINT ( 'NONE',  ( 17.05587630539788435, 6.762274262135705705, 91.75819690962693187 ) ) ;
#111720=CARTESIAN_POINT ( 'NONE',  ( -13.97604488694527625, -13.89961937509977652, 101.8739096053143811 ) ) ;
#111721=CARTESIAN_POINT ( 'NONE',  ( 0.05219959533937995610, -21.53943276465977519, 30.00109039468568284 ) ) ;
#111722=CARTESIAN_POINT ( 'NONE',  ( 13.89961937509957401, 13.97604488694547697, 91.87609039468567573 ) ) ;
#111723=CARTESIAN_POINT ( 'NONE',  ( 16.51473224551069308, 9.474510206698969483, 114.1655762719810241 ) ) ;
#111724=CARTESIAN_POINT ( 'NONE',  ( -19.03943276465977164, 0.05219959533909376836, 51.24890960531436690 ) ) ;
#111725=CARTESIAN_POINT ( 'NONE',  ( 19.02544592524343514, -5.153800228976328945, 93.54057627198102409 ) ) ;
#111726=CARTESIAN_POINT ( 'NONE',  ( 16.53943276465976808, -0.05219959533910856209, 63.74890960531435979 ) ) ;
#111727=CARTESIAN_POINT ( 'NONE',  ( 5.153800228976335163, 19.02544592524342804, 54.79057627198103120 ) ) ;
#111728=CARTESIAN_POINT ( 'NONE',  ( -13.97604488694527625, -13.89961937509977652, 66.87390960531436690 ) ) ;
#111729=CARTESIAN_POINT ( 'NONE',  ( 19.02544592524334988, 5.153800228976608722, 66.45942372801899012 ) ) ;
#111730=CARTESIAN_POINT ( 'NONE',  ( 0.05219959533936267826, -19.03943276465977164, 25.00109039468566152 ) ) ;
#111731=CARTESIAN_POINT ( 'NONE',  ( 16.46253265017160672, -9.564922557960803928, 68.33224293864770971 ) ) ;
#111732=CARTESIAN_POINT ( 'NONE',  ( 18.62759615963271287, -10.81492255796078972, 63.33224293864770260 ) ) ;
#111733=CARTESIAN_POINT ( 'NONE',  ( 14.34966873604960469, 8.224510206698951720, 64.16557627198102409 ) ) ;
#111734=CARTESIAN_POINT ( 'NONE',  ( 5.153800228976615827, -19.02544592524334988, 35.20942372801899722 ) ) ;
#111736=CARTESIAN_POINT ( 'NONE',  ( -15.72974639402197994, 15.80617190586746368, 50.62390960531435979 ) ) ;
#111737=CARTESIAN_POINT ( 'NONE',  ( -18.62759615963270932, 10.81492255796079327, 25.83224293864769194 ) ) ;
#111738=CARTESIAN_POINT ( 'NONE',  ( -19.02544592524342804, 5.153800228976336051, 51.04057627198103120 ) ) ;
#111739=CARTESIAN_POINT ( 'NONE',  ( 19.05341960407611168, 5.049401038298154454, 33.95724293864769550 ) ) ;
#111740=CARTESIAN_POINT ( 'NONE',  ( -8.224510206698948167, 14.34966873604960824, 105.4155762719810383 ) ) ;
#111741=CARTESIAN_POINT ( 'NONE',  ( -5.823673210054116645, -21.52544592524344225, 107.2905762719810525 ) ) ;
#111742=CARTESIAN_POINT ( 'NONE',  ( -18.62759615963255300, -10.81492255796106328, 29.16775706135234003 ) ) ;
#111743=CARTESIAN_POINT ( 'NONE',  ( -4.379528057220328563, 16.55341960407611168, 110.2072429386477239 ) ) ;
#111744=CARTESIAN_POINT ( 'NONE',  ( 18.67979575497194134, -10.72451020669871369, 75.83442372801900433 ) ) ;
#111745=CARTESIAN_POINT ( 'NONE',  ( -10.81492255796078084, -18.62759615963271287, 87.08224293864769550 ) ) ;
#111746=CARTESIAN_POINT ( 'NONE',  ( 19.05341960407617918, -5.049401038297876454, 36.04275706135234003 ) ) ;
#111747=CARTESIAN_POINT ( 'NONE',  ( 17.72696623605159516, -5.500000000000042633, 76.09811031808418136 ) ) ;
#111750=CARTESIAN_POINT ( 'NONE',  ( -8.224510206698735004, -14.34966873604973081, 49.58442372801901143 ) ) ;
#111751=CARTESIAN_POINT ( 'NONE',  ( -8.224510206698948167, 14.34966873604960824, 110.4155762719810383 ) ) ;
#111753=CARTESIAN_POINT ( 'NONE',  ( -19.05341960407611168, -5.049401038298163336, 71.45724293864766707 ) ) ;
#111754=CARTESIAN_POINT ( 'NONE',  ( 12.06949235617757843, -12.14591786802309237, 98.12390960531436690 ) ) ;
#111755=CARTESIAN_POINT ( 'NONE',  ( -21.53943276465977519, 0.05219959533907696930, 46.24890960531435979 ) ) ;
#111756=CARTESIAN_POINT ( 'NONE',  ( -12.06949235617756955, 12.14591786802309770, 80.62390960531438111 ) ) ;
#111757=CARTESIAN_POINT ( 'NONE',  ( -14.34966873604972548, 8.224510206698743886, 28.33442372801902209 ) ) ;
#111758=CARTESIAN_POINT ( 'NONE',  ( 15.80617190586769283, -15.72974639402175789, 90.62609039468567573 ) ) ;
#111760=CARTESIAN_POINT ( 'NONE',  ( 12.14591786802327356, -12.06949235617739191, 100.6260903946857184 ) ) ;
#111761=CARTESIAN_POINT ( 'NONE',  ( 8.314922557960818139, 14.29746914071049879, 44.58224293864769550 ) ) ;
#111762=CARTESIAN_POINT ( 'NONE',  ( -13.89961937509977652, 13.97604488694528158, 35.62390960531435269 ) ) ;
#111763=CARTESIAN_POINT ( 'NONE',  ( 18.62759615963255655, 10.81492255796105972, 96.66775706135234714 ) ) ;
#111764=CARTESIAN_POINT ( 'NONE',  ( 15.80617190586746368, 15.72974639402197994, 104.3739096053143669 ) ) ;
#111765=CARTESIAN_POINT ( 'NONE',  ( 21.53943276465977519, 0.05219959533937863772, 61.25109039468567573 ) ) ;
#111766=CARTESIAN_POINT ( 'NONE',  ( -8.224510206698735004, -14.34966873604973081, 44.58442372801901854 ) ) ;
#111767=CARTESIAN_POINT ( 'NONE',  ( -8.224510206698948167, 14.34966873604960824, 70.41557627198102409 ) ) ;
#111768=CARTESIAN_POINT ( 'NONE',  ( -0.05219959533937732626, 21.53943276465977519, 87.50109039468568994 ) ) ;
#111769=CARTESIAN_POINT ( 'NONE',  ( 8.224510206698742110, 14.34966873604972548, 107.0844237280190043 ) ) ;
#111772=CARTESIAN_POINT ( 'NONE',  ( 8.314922557960818139, 14.29746914071049879, 29.58224293864769905 ) ) ;
#111773=CARTESIAN_POINT ( 'NONE',  ( 14.29746914071037800, 8.314922557961029526, 76.66775706135234714 ) ) ;
#111774=CARTESIAN_POINT ( 'NONE',  ( -9.564922557960796823, -16.46253265017161027, 87.08224293864769550 ) ) ;
#111775=CARTESIAN_POINT ( 'NONE',  ( -9.474510206698964154, 16.51473224551069663, 95.41557627198102409 ) ) ;
#111776=CARTESIAN_POINT ( 'NONE',  ( 0.05219959533937995610, -21.53943276465977519, 90.00109039468567573 ) ) ;
#111777=CARTESIAN_POINT ( 'NONE',  ( -14.34966873604972548, 8.224510206698743886, 83.33442372801903275 ) ) ;
#111778=CARTESIAN_POINT ( 'NONE',  ( 14.34966873604960469, 8.224510206698951720, 74.16557627198102409 ) ) ;
#111779=CARTESIAN_POINT ( 'NONE',  ( -9.564922557960796823, -16.46253265017161027, 67.08224293864769550 ) ) ;
#111781=CARTESIAN_POINT ( 'NONE',  ( -4.379528057220086978, -16.55341960407618274, 24.79275706135235779 ) ) ;
#111782=CARTESIAN_POINT ( 'NONE',  ( -9.564922557960796823, -16.46253265017161027, 22.08224293864768839 ) ) ;
#111783=CARTESIAN_POINT ( 'NONE',  ( 9.564922557960805705, 16.46253265017160317, 94.58224293864769550 ) ) ;
#111784=CARTESIAN_POINT ( 'NONE',  ( -16.51473224551082808, 9.474510206698731452, 113.3344237280190043 ) ) ;
#111786=CARTESIAN_POINT ( 'NONE',  ( 13.97604488694548053, -13.89961937509957401, 25.62609039468566507 ) ) ;
#111787=CARTESIAN_POINT ( 'NONE',  ( -12.14591786802326823, 12.06949235617739902, 98.12609039468570415 ) ) ;
#111788=CARTESIAN_POINT ( 'NONE',  ( 19.03943276465977164, 0.05219959533936151252, 106.2510903946856615 ) ) ;
#111789=CARTESIAN_POINT ( 'NONE',  ( 12.06949235617757843, -12.14591786802309237, 108.1239096053143811 ) ) ;
#111790=CARTESIAN_POINT ( 'NONE',  ( -16.53943276465976808, -0.05219959533934237506, 83.75109039468568994 ) ) ;
#111791=CARTESIAN_POINT ( 'NONE',  ( 16.52544592524335698, 4.483927247898782831, 51.45942372801901854 ) ) ;
#111793=CARTESIAN_POINT ( 'NONE',  ( -19.05341960407617563, 5.049401038297882671, 68.54275706135230450 ) ) ;
#111794=CARTESIAN_POINT ( 'NONE',  ( -19.02544592524334988, -5.153800228976617603, 18.95942372801899722 ) ) ;
#111795=CARTESIAN_POINT ( 'NONE',  ( -9.474510206698964154, 16.51473224551069663, 45.41557627198103120 ) ) ;
#111796=CARTESIAN_POINT ( 'NONE',  ( 0.05219959533909260263, 19.03943276465977164, 79.99890960531436690 ) ) ;
#111797=CARTESIAN_POINT ( 'NONE',  ( 16.52544592524342804, -4.483927247898539470, 88.54057627198103830 ) ) ;
#111798=CARTESIAN_POINT ( 'NONE',  ( 9.564922557961047289, -16.46253265017146816, 55.41775706135234003 ) ) ;
#111799=CARTESIAN_POINT ( 'NONE',  ( -10.81492255796078084, -18.62759615963271287, 52.08224293864768839 ) ) ;
#111800=CARTESIAN_POINT ( 'NONE',  ( -21.55341960407619339, 5.719274019375674811, 103.5427570613523613 ) ) ;
#111801=CARTESIAN_POINT ( 'NONE',  ( 16.46253265017160672, -9.564922557960803928, 88.33224293864769550 ) ) ;
#111802=EDGE_CURVE ( 'NONE', #129803, #60482, #104910, .T. ) ;
#111803=CARTESIAN_POINT ( 'NONE',  ( -15.72974639402176322, -15.80617190586768395, 104.3760903946856899 ) ) ;
#111804=CARTESIAN_POINT ( 'NONE',  ( 15.72974639402199770, -15.80617190586745480, 58.12390960531435979 ) ) ;
#111805=CARTESIAN_POINT ( 'NONE',  ( 19.03943276465977164, -0.05219959533909143690, 98.74890960531436690 ) ) ;
#111806=CARTESIAN_POINT ( 'NONE',  ( -13.97604488694547697, 13.89961937509957934, 93.12609039468566152 ) ) ;
#111807=CARTESIAN_POINT ( 'NONE',  ( 9.564922557960805705, 16.46253265017160317, 109.5822429386476955 ) ) ;
#111808=CARTESIAN_POINT ( 'NONE',  ( -19.05341960407617563, 5.049401038297882671, 103.5427570613523329 ) ) ;
#111809=CARTESIAN_POINT ( 'NONE',  ( -19.02544592524342804, 5.153800228976336051, 26.04057627198103120 ) ) ;
#111810=CARTESIAN_POINT ( 'NONE',  ( -16.51473224551069308, -9.474510206698971260, 81.66557627198103830 ) ) ;
#111811=CARTESIAN_POINT ( 'NONE',  ( 18.62759615963271287, -10.81492255796078972, 83.33224293864769550 ) ) ;
#111812=CARTESIAN_POINT ( 'NONE',  ( -8.314922557961024197, 14.29746914071037800, 47.91775706135234714 ) ) ;
#111813=CARTESIAN_POINT ( 'NONE',  ( 5.719274019375673035, 21.55341960407619339, 42.29275706135235424 ) ) ;
#111814=CARTESIAN_POINT ( 'NONE',  ( 15.72974639402176855, 15.80617190586768217, 101.8760903946857042 ) ) ;
#111815=CARTESIAN_POINT ( 'NONE',  ( -4.483927247898782831, 16.52544592524335698, 102.7094237280190185 ) ) ;
#111816=CARTESIAN_POINT ( 'NONE',  ( 13.97604488694527802, 13.89961937509977652, 89.37390960531436690 ) ) ;
#111817=CARTESIAN_POINT ( 'NONE',  ( -16.53943276465976808, 0.05219959533911058130, 91.24890960531436690 ) ) ;
#111818=CARTESIAN_POINT ( 'NONE',  ( -14.34966873604960291, -8.224510206698953496, 26.66557627198103475 ) ) ;
#111819=CARTESIAN_POINT ( 'NONE',  ( -19.02544592524334988, -5.153800228976617603, 68.95942372801896170 ) ) ;
#111820=CARTESIAN_POINT ( 'NONE',  ( 21.55341960407619695, -5.719274019375665929, 41.04275706135236135 ) ) ;
#111821=CARTESIAN_POINT ( 'NONE',  ( -16.52544592524342804, 4.483927247898546575, 91.04057627198103830 ) ) ;
#111822=CARTESIAN_POINT ( 'NONE',  ( 19.03943276465977164, -0.05219959533909143690, 108.7489096053143527 ) ) ;
#111823=CARTESIAN_POINT ( 'NONE',  ( 16.53943276465976808, -0.05219959533910856209, 28.74890960531435624 ) ) ;
#111824=CARTESIAN_POINT ( 'NONE',  ( -21.52544592524334988, -5.823673210054445271, 88.95942372801901854 ) ) ;
#111825=CARTESIAN_POINT ( 'NONE',  ( 4.379528057220092307, 16.55341960407617563, 52.29275706135236135 ) ) ;
#111826=CARTESIAN_POINT ( 'NONE',  ( -0.05219959533937732626, 21.53943276465977519, 37.50109039468568284 ) ) ;
#111828=CARTESIAN_POINT ( 'NONE',  ( 21.53943276465977519, 0.05219959533937863772, 31.25109039468568639 ) ) ;
#111829=CARTESIAN_POINT ( 'NONE',  ( 16.52544592524342804, -4.483927247898539470, 108.5405762719810241 ) ) ;
#111830=CARTESIAN_POINT ( 'NONE',  ( 19.02544592524343514, -5.153800228976328945, 28.54057627198102409 ) ) ;
#111831=CARTESIAN_POINT ( 'NONE',  ( -14.34966873604960291, -8.224510206698953496, 71.66557627198100988 ) ) ;
#111832=CARTESIAN_POINT ( 'NONE',  ( 13.89961937509977652, -13.97604488694527269, 73.12390960531436690 ) ) ;
#111833=CARTESIAN_POINT ( 'NONE',  ( -14.29746914071037622, -8.314922557961029526, 109.1677570613523613 ) ) ;
#111834=CARTESIAN_POINT ( 'NONE',  ( -13.89961937509977652, 13.97604488694528158, 40.62390960531435979 ) ) ;
#111835=CARTESIAN_POINT ( 'NONE',  ( -15.72974639402197994, 15.80617190586746368, 45.62390960531436690 ) ) ;
#111836=CARTESIAN_POINT ( 'NONE',  ( -4.379528057220328563, 16.55341960407611168, 85.20724293864770971 ) ) ;
#111838=CARTESIAN_POINT ( 'NONE',  ( 5.719274019375991003, -21.55341960407610458, 87.70724293864769550 ) ) ;
#111839=CARTESIAN_POINT ( 'NONE',  ( 19.03943276465977164, -0.05219959533909143690, 88.74890960531436690 ) ) ;
#111840=CARTESIAN_POINT ( 'NONE',  ( -19.03943276465977164, 0.05219959533909376836, 56.24890960531435979 ) ) ;
#111841=CARTESIAN_POINT ( 'NONE',  ( -19.02544592524334988, -5.153800228976617603, 98.95942372801900433 ) ) ;
#111842=CARTESIAN_POINT ( 'NONE',  ( -0.05219959533907301413, -21.53943276465977519, 47.49890960531435979 ) ) ;
#111843=CARTESIAN_POINT ( 'NONE',  ( -18.67979575497193778, 10.72451020669871902, 73.33442372801901854 ) ) ;
#111844=CARTESIAN_POINT ( 'NONE',  ( -19.05341960407611168, -5.049401038298163336, 51.45724293864770260 ) ) ;
#111845=CARTESIAN_POINT ( 'NONE',  ( 16.46253265017160672, -9.564922557960803928, 83.33224293864768129 ) ) ;
#111847=CARTESIAN_POINT ( 'NONE',  ( -4.483927247898782831, 16.52544592524335698, 67.70942372801901854 ) ) ;
#111848=CARTESIAN_POINT ( 'NONE',  ( 21.52544592524334988, 5.823673210054432836, 46.45942372801901854 ) ) ;
#111849=CARTESIAN_POINT ( 'NONE',  ( -21.55341960407619339, 5.719274019375674811, 68.54275706135234714 ) ) ;
#111850=CARTESIAN_POINT ( 'NONE',  ( -21.53943276465977519, 0.05219959533907696930, 21.24890960531436690 ) ) ;
#111851=CARTESIAN_POINT ( 'NONE',  ( 18.67979575497178502, 10.72451020669898547, 94.16557627198103830 ) ) ;
#111852=CARTESIAN_POINT ( 'NONE',  ( 21.52544592524334988, 5.823673210054432836, 36.45942372801901143 ) ) ;
#111853=CARTESIAN_POINT ( 'NONE',  ( -8.224510206698735004, -14.34966873604973081, 64.58442372801900433 ) ) ;
#111854=CARTESIAN_POINT ( 'NONE',  ( 15.80617190586746368, 15.72974639402197994, 59.37390960531436690 ) ) ;
#111855=CARTESIAN_POINT ( 'NONE',  ( -16.46253265017146816, -9.564922557961047289, 34.16775706135233293 ) ) ;
#111856=CARTESIAN_POINT ( 'NONE',  ( 16.51473224551069308, 9.474510206698969483, 69.16557627198102409 ) ) ;
#111857=CARTESIAN_POINT ( 'NONE',  ( 12.06949235617739724, 12.14591786802326823, 96.87609039468568994 ) ) ;
#111859=CARTESIAN_POINT ( 'NONE',  ( 19.03943276465977164, -0.05219959533909143690, 108.7489096053143527 ) ) ;
#111861=CARTESIAN_POINT ( 'NONE',  ( -16.51473224551082808, 9.474510206698731452, 83.33442372801899012 ) ) ;
#111862=CARTESIAN_POINT ( 'NONE',  ( 5.719274019375991003, -21.55341960407610458, 52.70724293864769550 ) ) ;
#111863=CARTESIAN_POINT ( 'NONE',  ( 16.55341960407611168, 4.379528057220329451, 38.95724293864768839 ) ) ;
#111864=CARTESIAN_POINT ( 'NONE',  ( -19.02544592524334988, -5.153800228976617603, 93.95942372801900433 ) ) ;
#111865=CARTESIAN_POINT ( 'NONE',  ( -5.153800228976328057, -19.02544592524343514, 27.29057627198103120 ) ) ;
#111866=CARTESIAN_POINT ( 'NONE',  ( 13.97604488694548053, -13.89961937509957401, 105.6260903946856757 ) ) ;
#111867=CARTESIAN_POINT ( 'NONE',  ( -10.72451020669898014, 18.67979575497178502, 90.41557627198103830 ) ) ;
#111868=CARTESIAN_POINT ( 'NONE',  ( 0.05219959533936267826, -19.03943276465977164, 55.00109039468566863 ) ) ;
#111869=CARTESIAN_POINT ( 'NONE',  ( -12.06949235617739369, -12.14591786802326823, 74.37609039468568994 ) ) ;
#111870=CARTESIAN_POINT ( 'NONE',  ( 9.474510206698971260, -16.51473224551069308, 67.91557627198102409 ) ) ;
#111871=CARTESIAN_POINT ( 'NONE',  ( 12.06949235617757843, -12.14591786802309237, 73.12390960531436690 ) ) ;
#111872=CARTESIAN_POINT ( 'NONE',  ( 0.05219959533909260263, 19.03943276465977164, 44.99890960531435979 ) ) ;
#111873=CARTESIAN_POINT ( 'NONE',  ( 16.55341960407611168, 4.379528057220329451, 48.95724293864770971 ) ) ;
#111874=CARTESIAN_POINT ( 'NONE',  ( -0.05219959533909027116, -19.03943276465977164, 22.49890960531436690 ) ) ;
#111876=CARTESIAN_POINT ( 'NONE',  ( 8.224510206698953496, -14.34966873604960469, 32.91557627198102409 ) ) ;
#111877=CARTESIAN_POINT ( 'NONE',  ( -19.03943276465977164, 0.05219959533909376836, 71.24890960531435269 ) ) ;
#111878=CARTESIAN_POINT ( 'NONE',  ( 17.50000000000000000, 5.500000000000011546, 68.78230962303564411 ) ) ;
#111879=CARTESIAN_POINT ( 'NONE',  ( -9.474510206698720793, -16.51473224551083518, 39.58442372801899722 ) ) ;
#111880=CARTESIAN_POINT ( 'NONE',  ( -12.14591786802326823, 12.06949235617739902, 48.12609039468568284 ) ) ;
#111881=CARTESIAN_POINT ( 'NONE',  ( 18.62759615963271287, -10.81492255796078972, 48.33224293864770260 ) ) ;
#111882=CARTESIAN_POINT ( 'NONE',  ( -5.823673210054431948, 21.52544592524334988, 112.7094237280190328 ) ) ;
#111883=CARTESIAN_POINT ( 'NONE',  ( 13.89961937509977652, -13.97604488694527269, 78.12390960531433848 ) ) ;
#111884=CARTESIAN_POINT ( 'NONE',  ( 0.05219959533909260263, 19.03943276465977164, 114.9989096053143669 ) ) ;
#111885=CARTESIAN_POINT ( 'NONE',  ( 13.89961937509977652, -13.97604488694527269, 113.1239096053143527 ) ) ;
#111886=CARTESIAN_POINT ( 'NONE',  ( 10.81492255796106328, -18.62759615963255655, 35.41775706135234003 ) ) ;
#111888=CARTESIAN_POINT ( 'NONE',  ( -12.06949235617756955, 12.14591786802309770, 100.6239096053143811 ) ) ;
#111889=CARTESIAN_POINT ( 'NONE',  ( 18.67979575497178502, 10.72451020669898547, 99.16557627198100988 ) ) ;
#111890=CARTESIAN_POINT ( 'NONE',  ( -19.03943276465977164, 0.05219959533909376836, 81.24890960531436690 ) ) ;
#111892=CARTESIAN_POINT ( 'NONE',  ( 21.52544592524334988, 5.823673210054432836, 26.45942372801901854 ) ) ;
#111895=CARTESIAN_POINT ( 'NONE',  ( 9.564922557960805705, 16.46253265017160317, 89.58224293864769550 ) ) ;
#111896=CARTESIAN_POINT ( 'NONE',  ( 19.26498983726237313, -5.499999999999792166, 83.05319577421998645 ) ) ;
#111897=CARTESIAN_POINT ( 'NONE',  ( -19.05341960407611168, -5.049401038298163336, 21.45724293864768839 ) ) ;
#111898=CARTESIAN_POINT ( 'NONE',  ( 16.51473224551069308, 9.474510206698969483, 34.16557627198102409 ) ) ;
#111899=CARTESIAN_POINT ( 'NONE',  ( -19.05341960407617563, 5.049401038297882671, 108.5427570613523187 ) ) ;
#111901=CARTESIAN_POINT ( 'NONE',  ( 8.224510206698953496, -14.34966873604960469, 107.9155762719810241 ) ) ;
#111902=CARTESIAN_POINT ( 'NONE',  ( 15.72974639402176855, 15.80617190586768217, 91.87609039468568994 ) ) ;
#111903=CARTESIAN_POINT ( 'NONE',  ( 13.97604488694527802, 13.89961937509977652, 64.37390960531436690 ) ) ;
#111904=CARTESIAN_POINT ( 'NONE',  ( 0.05219959533937995610, -21.53943276465977519, 35.00109039468568284 ) ) ;
#111905=CARTESIAN_POINT ( 'NONE',  ( 18.67979575497194134, -10.72451020669871369, 20.83442372801901143 ) ) ;
#111907=CARTESIAN_POINT ( 'NONE',  ( -9.474510206698964154, 16.51473224551069663, 90.41557627198103830 ) ) ;
#111909=CARTESIAN_POINT ( 'NONE',  ( -4.379528057220086978, -16.55341960407618274, 29.79275706135234358 ) ) ;
#111910=CARTESIAN_POINT ( 'NONE',  ( 0.05219959533907565091, 21.53943276465977519, 49.99890960531437401 ) ) ;
#111911=CARTESIAN_POINT ( 'NONE',  ( -21.52544592524334988, -5.823673210054445271, 78.95942372801901854 ) ) ;
#111912=CARTESIAN_POINT ( 'NONE',  ( -19.02544592524342804, 5.153800228976336051, 106.0405762719810241 ) ) ;
#111913=CARTESIAN_POINT ( 'NONE',  ( 9.474510206698729675, 16.51473224551082808, 102.0844237280190043 ) ) ;
#111914=CARTESIAN_POINT ( 'NONE',  ( 19.05341960407611168, 5.049401038298154454, 58.95724293864768129 ) ) ;
#111915=CARTESIAN_POINT ( 'NONE',  ( 0.05219959533909260263, 19.03943276465977164, 84.99890960531436690 ) ) ;
#111916=CARTESIAN_POINT ( 'NONE',  ( 14.29746914071049879, -8.314922557960816363, 88.33224293864769550 ) ) ;
#111917=CARTESIAN_POINT ( 'NONE',  ( -16.55341960407611168, -4.379528057220339221, 101.4572429386476955 ) ) ;
#111918=CARTESIAN_POINT ( 'NONE',  ( 16.46253265017160672, -9.564922557960803928, 108.3322429386476955 ) ) ;
#111920=CARTESIAN_POINT ( 'NONE',  ( 12.14591786802327356, -12.06949235617739191, 75.62609039468567573 ) ) ;
#111921=CARTESIAN_POINT ( 'NONE',  ( 14.29746914071049879, -8.314922557960816363, 58.33224293864768839 ) ) ;
#111923=CARTESIAN_POINT ( 'NONE',  ( -9.474510206698964154, 16.51473224551069663, 40.41557627198103120 ) ) ;
#111924=CARTESIAN_POINT ( 'NONE',  ( 21.52544592524334988, 5.823673210054432836, 66.45942372801903275 ) ) ;
#111925=CARTESIAN_POINT ( 'NONE',  ( 9.474510206698729675, 16.51473224551082808, 97.08442372801900433 ) ) ;
#111926=CARTESIAN_POINT ( 'NONE',  ( 14.29746914071049879, -8.314922557960816363, 63.33224293864770260 ) ) ;
#111927=CARTESIAN_POINT ( 'NONE',  ( -18.67979575497178146, -10.72451020669898902, 106.6655762719810383 ) ) ;
#111928=CARTESIAN_POINT ( 'NONE',  ( 21.52544592524344225, -5.823673210054117533, 48.54057627198103120 ) ) ;
#111929=CARTESIAN_POINT ( 'NONE',  ( -17.13100169013300444, -6.664070546373138448, 104.2321016430015135 ) ) ;
#111931=CARTESIAN_POINT ( 'NONE',  ( -19.05341960407611168, -5.049401038298163336, 66.45724293864769550 ) ) ;
#111932=CARTESIAN_POINT ( 'NONE',  ( 14.29746914071049879, -8.314922557960816363, 38.33224293864768839 ) ) ;
#111933=CARTESIAN_POINT ( 'NONE',  ( 16.55341960407618274, -4.379528057220086978, 111.0427570613523613 ) ) ;
#111934=CARTESIAN_POINT ( 'NONE',  ( 12.06949235617739724, 12.14591786802326823, 86.87609039468568994 ) ) ;
#111935=CARTESIAN_POINT ( 'NONE',  ( -13.89961937509957401, -13.97604488694547875, 39.37609039468566152 ) ) ;
#111937=CARTESIAN_POINT ( 'NONE',  ( 19.05341960407611168, 5.049401038298154454, 93.95724293864769550 ) ) ;
#111938=CARTESIAN_POINT ( 'NONE',  ( 19.05341960407611168, 5.049401038298154454, 48.95724293864768129 ) ) ;
#111939=CARTESIAN_POINT ( 'NONE',  ( -14.34966873604960291, -8.224510206698953496, 56.66557627198103830 ) ) ;
#111940=CARTESIAN_POINT ( 'NONE',  ( -19.03943276465977164, 0.05219959533909376836, 21.24890960531436335 ) ) ;
#111941=CARTESIAN_POINT ( 'NONE',  ( 5.153800228976335163, 19.02544592524342804, 114.7905762719810241 ) ) ;
#111942=CARTESIAN_POINT ( 'NONE',  ( 5.719274019375991003, -21.55341960407610458, 47.70724293864770260 ) ) ;
#111943=CARTESIAN_POINT ( 'NONE',  ( -14.34966873604960291, -8.224510206698953496, 91.66557627198103830 ) ) ;
#111944=CARTESIAN_POINT ( 'NONE',  ( -16.53943276465976808, -0.05219959533934237506, 33.75109039468568284 ) ) ;
#111945=CARTESIAN_POINT ( 'NONE',  ( 16.52544592524342804, -4.483927247898539470, 78.54057627198103830 ) ) ;
#111947=CARTESIAN_POINT ( 'NONE',  ( 16.51473224551083163, -9.474510206698727899, 75.83442372801900433 ) ) ;
#111948=CARTESIAN_POINT ( 'NONE',  ( 15.72974639402199770, -15.80617190586745480, 23.12390960531436335 ) ) ;
#111950=CARTESIAN_POINT ( 'NONE',  ( 17.58332526062526568, -7.635886036038552760, 43.42334959558467489 ) ) ;
#111951=CARTESIAN_POINT ( 'NONE',  ( 12.06949235617739724, 12.14591786802326823, 26.87609039468567218 ) ) ;
#111952=CARTESIAN_POINT ( 'NONE',  ( -14.34966873604972548, 8.224510206698743886, 108.3344237280190185 ) ) ;
#111953=CARTESIAN_POINT ( 'NONE',  ( 19.03943276465977164, 0.05219959533936151252, 66.25109039468567573 ) ) ;
#111954=CARTESIAN_POINT ( 'NONE',  ( -0.05219959533907301413, -21.53943276465977519, 47.49890960531435979 ) ) ;
#111955=CARTESIAN_POINT ( 'NONE',  ( 10.81492255796106328, -18.62759615963255655, 65.41775706135234714 ) ) ;
#111957=CARTESIAN_POINT ( 'NONE',  ( -16.55341960407617563, 4.379528057220093196, 38.54275706135234714 ) ) ;
#111958=CARTESIAN_POINT ( 'NONE',  ( 16.51473224551069308, 9.474510206698969483, 24.16557627198102765 ) ) ;
#111959=CARTESIAN_POINT ( 'NONE',  ( 13.89961937509977652, -13.97604488694527269, 83.12390960531436690 ) ) ;
#111960=CARTESIAN_POINT ( 'NONE',  ( 9.474510206698971260, -16.51473224551069308, 27.91557627198103120 ) ) ;
#111961=CARTESIAN_POINT ( 'NONE',  ( -8.224510206698948167, 14.34966873604960824, 105.4155762719810383 ) ) ;
#111962=CARTESIAN_POINT ( 'NONE',  ( -5.153800228976328057, -19.02544592524343514, 97.29057627198099567 ) ) ;
#111964=CARTESIAN_POINT ( 'NONE',  ( -12.06949235617739369, -12.14591786802326823, 54.37609039468568994 ) ) ;
#111965=CARTESIAN_POINT ( 'NONE',  ( 16.51473224551083163, -9.474510206698727899, 105.8344237280190043 ) ) ;
#111966=CARTESIAN_POINT ( 'NONE',  ( 10.81492255796078972, 18.62759615963270932, 79.58224293864769550 ) ) ;
#111967=CARTESIAN_POINT ( 'NONE',  ( 9.474510206698971260, -16.51473224551069308, 47.91557627198102409 ) ) ;
#111968=CARTESIAN_POINT ( 'NONE',  ( 5.153800228976615827, -19.02544592524334988, 75.20942372801896170 ) ) ;
#111969=CARTESIAN_POINT ( 'NONE',  ( 5.719274019375991003, -21.55341960407610458, 107.7072429386476955 ) ) ;
#111970=CARTESIAN_POINT ( 'NONE',  ( 0.05219959533909260263, 19.03943276465977164, 64.99890960531436690 ) ) ;
#111971=CARTESIAN_POINT ( 'NONE',  ( -5.049401038298153566, 19.05341960407611168, 100.2072429386476955 ) ) ;
#111973=CARTESIAN_POINT ( 'NONE',  ( -16.55341960407617563, 4.379528057220093196, 33.54275706135234714 ) ) ;
#111974=CARTESIAN_POINT ( 'NONE',  ( 10.81492255796078972, 18.62759615963270932, 109.5822429386476955 ) ) ;
#111975=CARTESIAN_POINT ( 'NONE',  ( -16.55341960407611168, -4.379528057220339221, 106.4572429386477097 ) ) ;
#111976=CARTESIAN_POINT ( 'NONE',  ( -19.03943276465977164, 0.05219959533909376836, 91.24890960531436690 ) ) ;
#111977=CARTESIAN_POINT ( 'NONE',  ( 13.97604488694548053, -13.89961937509957401, 80.62609039468567573 ) ) ;
#111978=CARTESIAN_POINT ( 'NONE',  ( -18.62759615963270932, 10.81492255796079327, 90.83224293864769550 ) ) ;
#111979=CARTESIAN_POINT ( 'NONE',  ( -8.314922557960811034, -14.29746914071050412, 47.08224293864770260 ) ) ;
#111980=CARTESIAN_POINT ( 'NONE',  ( -18.67979575497193778, 10.72451020669871902, 113.3344237280190328 ) ) ;
#111981=CARTESIAN_POINT ( 'NONE',  ( 14.34966873604972726, -8.224510206698740333, 70.83442372801901854 ) ) ;
#111982=CARTESIAN_POINT ( 'NONE',  ( 19.03943276465977164, -0.05219959533909143690, 88.74890960531436690 ) ) ;
#111983=CARTESIAN_POINT ( 'NONE',  ( -9.474510206698964154, 16.51473224551069663, 50.41557627198102409 ) ) ;
#111985=CARTESIAN_POINT ( 'NONE',  ( -15.72974639402176322, -15.80617190586768395, 59.37609039468568284 ) ) ;
#111986=CARTESIAN_POINT ( 'NONE',  ( 21.52544592524334988, 5.823673210054432836, 71.45942372801901854 ) ) ;
#111987=CARTESIAN_POINT ( 'NONE',  ( -5.049401038298153566, 19.05341960407611168, 60.20724293864768129 ) ) ;
#111988=CARTESIAN_POINT ( 'NONE',  ( -5.823673210054431948, 21.52544592524334988, 32.70942372801900433 ) ) ;
#111990=CARTESIAN_POINT ( 'NONE',  ( 9.474510206698729675, 16.51473224551082808, 82.08442372801899012 ) ) ;
#111991=CARTESIAN_POINT ( 'NONE',  ( -19.02544592524342804, 5.153800228976336051, 46.04057627198101699 ) ) ;
#111992=CARTESIAN_POINT ( 'NONE',  ( -16.52544592524335698, -4.483927247898792601, 83.95942372801900433 ) ) ;
#111993=CARTESIAN_POINT ( 'NONE',  ( -13.89961937509977652, 13.97604488694528158, 60.62390960531436690 ) ) ;
#111994=CARTESIAN_POINT ( 'NONE',  ( -0.05219959533909027116, -19.03943276465977164, 107.4989096053143527 ) ) ;
#111995=CARTESIAN_POINT ( 'NONE',  ( 9.474510206698971260, -16.51473224551069308, 42.91557627198103120 ) ) ;
#111996=CARTESIAN_POINT ( 'NONE',  ( -5.719274019375978568, 21.55341960407610458, 80.20724293864769550 ) ) ;
#111997=CARTESIAN_POINT ( 'NONE',  ( 12.06949235617739724, 12.14591786802326823, 71.87609039468568994 ) ) ;
#112000=CARTESIAN_POINT ( 'NONE',  ( 19.03943276465977164, 0.05219959533936151252, 31.25109039468566863 ) ) ;
#112002=CARTESIAN_POINT ( 'NONE',  ( 19.03943276465977164, -0.05219959533909143690, 63.74890960531435979 ) ) ;
#112003=CARTESIAN_POINT ( 'NONE',  ( 16.53943276465976808, -0.05219959533910856209, 38.74890960531435979 ) ) ;
#112004=CARTESIAN_POINT ( 'NONE',  ( 12.06949235617757843, -12.14591786802309237, 83.12390960531436690 ) ) ;
#112005=CARTESIAN_POINT ( 'NONE',  ( 0.05219959533909260263, 19.03943276465977164, 99.99890960531436690 ) ) ;
#112006=CARTESIAN_POINT ( 'NONE',  ( -19.03943276465977164, 0.05219959533909376836, 96.24890960531436690 ) ) ;
#112007=CARTESIAN_POINT ( 'NONE',  ( 10.81492255796106328, -18.62759615963255655, 50.41775706135235424 ) ) ;
#112008=CARTESIAN_POINT ( 'NONE',  ( -9.564922557960796823, -16.46253265017161027, 112.0822429386476955 ) ) ;
#112009=CARTESIAN_POINT ( 'NONE',  ( -0.05219959533936034679, 19.03943276465977164, 22.50109039468566152 ) ) ;
#112010=CARTESIAN_POINT ( 'NONE',  ( -8.224510206698735004, -14.34966873604973081, 74.58442372801901854 ) ) ;
#112011=CARTESIAN_POINT ( 'NONE',  ( 18.62759615963255655, 10.81492255796105972, 26.66775706135235424 ) ) ;
#112012=CARTESIAN_POINT ( 'NONE',  ( 5.049401038298161559, -19.05341960407611168, 107.7072429386476955 ) ) ;
#112013=CARTESIAN_POINT ( 'NONE',  ( -0.05219959533907301413, -21.53943276465977519, 107.4989096053143669 ) ) ;
#112014=CARTESIAN_POINT ( 'NONE',  ( 16.55341960407611168, 4.379528057220329451, 63.95724293864770260 ) ) ;
#112015=CARTESIAN_POINT ( 'NONE',  ( -9.564922557960796823, -16.46253265017161027, 47.08224293864769550 ) ) ;
#112016=CARTESIAN_POINT ( 'NONE',  ( 16.52544592524342804, -4.483927247898539470, 78.54057627198103830 ) ) ;
#112017=CARTESIAN_POINT ( 'NONE',  ( 10.72451020669898902, -18.67979575497178502, 27.91557627198103830 ) ) ;
#112018=CARTESIAN_POINT ( 'NONE',  ( 16.51473224551083163, -9.474510206698727899, 25.83442372801900078 ) ) ;
#112019=CARTESIAN_POINT ( 'NONE',  ( 8.314922557960818139, 14.29746914071049879, 109.5822429386476955 ) ) ;
#112021=CARTESIAN_POINT ( 'NONE',  ( -4.379528057220086978, -16.55341960407618274, 64.79275706135234714 ) ) ;
#112022=CARTESIAN_POINT ( 'NONE',  ( 16.46253265017160672, -9.564922557960803928, 63.33224293864769550 ) ) ;
#112024=CARTESIAN_POINT ( 'NONE',  ( -8.224510206698948167, 14.34966873604960824, 90.41557627198103830 ) ) ;
#112025=CARTESIAN_POINT ( 'NONE',  ( 0.05219959533907565091, 21.53943276465977519, 39.99890960531436690 ) ) ;
#112027=CARTESIAN_POINT ( 'NONE',  ( -14.34966873604972548, 8.224510206698743886, 113.3344237280190328 ) ) ;
#112028=CARTESIAN_POINT ( 'NONE',  ( 5.049401038297881783, 19.05341960407617563, 112.2927570613523471 ) ) ;
#112029=CARTESIAN_POINT ( 'NONE',  ( -10.72451020669870658, -18.67979575497194134, 74.58442372801901854 ) ) ;
#112030=CARTESIAN_POINT ( 'NONE',  ( -9.564922557960796823, -16.46253265017161027, 87.08224293864769550 ) ) ;
#112031=CARTESIAN_POINT ( 'NONE',  ( 15.72974639402199770, -15.80617190586745480, 98.12390960531436690 ) ) ;
#112032=CARTESIAN_POINT ( 'NONE',  ( -16.53943276465976808, -0.05219959533934237506, 48.75109039468568284 ) ) ;
#112033=CARTESIAN_POINT ( 'NONE',  ( 19.02544592524343514, -5.153800228976328945, 33.54057627198102409 ) ) ;
#112035=CARTESIAN_POINT ( 'NONE',  ( 16.53943276465976808, 0.05219959533934440121, 26.25109039468567573 ) ) ;
#112036=CARTESIAN_POINT ( 'NONE',  ( 0.05219959533936267826, -19.03943276465977164, 100.0010903946856757 ) ) ;
#112037=CARTESIAN_POINT ( 'NONE',  ( 15.72974639402199770, -15.80617190586745480, 93.12390960531436690 ) ) ;
#112038=CARTESIAN_POINT ( 'NONE',  ( 5.153800228976615827, -19.02544592524334988, 50.20942372801897591 ) ) ;
#112039=CARTESIAN_POINT ( 'NONE',  ( 19.26498983726236958, -5.499999999999793943, 88.05319577422001487 ) ) ;
#112040=CARTESIAN_POINT ( 'NONE',  ( 0.05219959533907565091, 21.53943276465977519, 99.99890960531436690 ) ) ;
#112042=CARTESIAN_POINT ( 'NONE',  ( 19.02544592524343514, -5.153800228976328945, 83.54057627198100988 ) ) ;
#112044=CARTESIAN_POINT ( 'NONE',  ( 8.224510206698742110, 14.34966873604972548, 32.08442372801901854 ) ) ;
#112046=CARTESIAN_POINT ( 'NONE',  ( -21.52544592524334988, -5.823673210054445271, 23.95942372801901143 ) ) ;
#112047=CARTESIAN_POINT ( 'NONE',  ( -14.29746914071049879, 8.314922557960819915, 60.83224293864769550 ) ) ;
#112048=CARTESIAN_POINT ( 'NONE',  ( 16.51473224551069308, 9.474510206698969483, 74.16557627198103830 ) ) ;
#112049=CARTESIAN_POINT ( 'NONE',  ( 8.314922557961029526, -14.29746914071037800, 35.41775706135234003 ) ) ;
#112050=CARTESIAN_POINT ( 'NONE',  ( 9.474510206698729675, 16.51473224551082808, 47.08442372801900433 ) ) ;
#112051=CARTESIAN_POINT ( 'NONE',  ( -10.81492255796105439, 18.62759615963255655, 47.91775706135234714 ) ) ;
#112052=CARTESIAN_POINT ( 'NONE',  ( 9.564922557961047289, -16.46253265017146816, 110.4177570613523471 ) ) ;
#112053=CARTESIAN_POINT ( 'NONE',  ( -9.564922557960796823, -16.46253265017161027, 57.08224293864769550 ) ) ;
#112054=CARTESIAN_POINT ( 'NONE',  ( 19.02544592524334988, 5.153800228976608722, 86.45942372801900433 ) ) ;
#112055=CARTESIAN_POINT ( 'NONE',  ( -10.81492255796105439, 18.62759615963255655, 82.91775706135234714 ) ) ;
#112056=CARTESIAN_POINT ( 'NONE',  ( 19.05341960407617918, -5.049401038297876454, 61.04275706135232582 ) ) ;
#112057=CARTESIAN_POINT ( 'NONE',  ( 19.02544592524343514, -5.153800228976328945, 43.54057627198103120 ) ) ;
#112058=CARTESIAN_POINT ( 'NONE',  ( 18.62759615963271287, -10.81492255796078972, 63.33224293864770260 ) ) ;
#112059=CARTESIAN_POINT ( 'NONE',  ( 14.29746914071049879, -8.314922557960816363, 58.33224293864768839 ) ) ;
#112060=CARTESIAN_POINT ( 'NONE',  ( -19.02544592524334988, -5.153800228976617603, 68.95942372801896170 ) ) ;
#112062=CARTESIAN_POINT ( 'NONE',  ( -16.46253265017146816, -9.564922557961047289, 34.16775706135233293 ) ) ;
#112063=CARTESIAN_POINT ( 'NONE',  ( -16.55341960407617563, 4.379528057220093196, 98.54275706135234714 ) ) ;
#112064=CARTESIAN_POINT ( 'NONE',  ( -12.14591786802309592, -12.06949235617757132, 56.87390960531436690 ) ) ;
#112065=CARTESIAN_POINT ( 'NONE',  ( 5.823673210054444382, -21.52544592524334988, 95.20942372801903275 ) ) ;
#112067=CARTESIAN_POINT ( 'NONE',  ( -5.823673210054431948, 21.52544592524334988, 97.70942372801904696 ) ) ;
#112068=CARTESIAN_POINT ( 'NONE',  ( -5.823673210054116645, -21.52544592524344225, 92.29057627198103830 ) ) ;
#112069=CARTESIAN_POINT ( 'NONE',  ( -19.03943276465977164, 0.05219959533909376836, 51.24890960531436690 ) ) ;
#112070=CARTESIAN_POINT ( 'NONE',  ( 21.55341960407619695, -5.719274019375665929, 71.04275706135234714 ) ) ;
#112071=CARTESIAN_POINT ( 'NONE',  ( 5.049401038298161559, -19.05341960407611168, 47.70724293864770260 ) ) ;
#112072=CARTESIAN_POINT ( 'NONE',  ( 19.02544592524343514, -5.153800228976328945, 68.54057627198103830 ) ) ;
#112073=CARTESIAN_POINT ( 'NONE',  ( -8.314922557960811034, -14.29746914071050412, 102.0822429386476955 ) ) ;
#112074=CARTESIAN_POINT ( 'NONE',  ( 0.05219959533909260263, 19.03943276465977164, 114.9989096053143669 ) ) ;
#112075=CARTESIAN_POINT ( 'NONE',  ( -4.379528057220328563, 16.55341960407611168, 60.20724293864768839 ) ) ;
#112076=CARTESIAN_POINT ( 'NONE',  ( -13.97604488694527625, -13.89961937509977652, 31.87390960531435979 ) ) ;
#112077=CARTESIAN_POINT ( 'NONE',  ( -8.224510206698948167, 14.34966873604960824, 65.41557627198102409 ) ) ;
#112078=CARTESIAN_POINT ( 'NONE',  ( 5.719274019375991003, -21.55341960407610458, 102.7072429386476955 ) ) ;
#112079=CARTESIAN_POINT ( 'NONE',  ( 10.81492255796106328, -18.62759615963255655, 40.41775706135234714 ) ) ;
#112081=CARTESIAN_POINT ( 'NONE',  ( -12.14591786802326823, 12.06949235617739902, 38.12609039468567573 ) ) ;
#112082=CARTESIAN_POINT ( 'NONE',  ( -21.52544592524343514, 5.823673210054127303, 86.04057627198102409 ) ) ;
#112083=CARTESIAN_POINT ( 'NONE',  ( -18.62759615963255300, -10.81492255796106328, 109.1677570613523613 ) ) ;
#112084=CARTESIAN_POINT ( 'NONE',  ( -13.97604488694527625, -13.89961937509977652, 86.87390960531436690 ) ) ;
#112085=CARTESIAN_POINT ( 'NONE',  ( 5.823673210054444382, -21.52544592524334988, 50.20942372801901854 ) ) ;
#112086=CARTESIAN_POINT ( 'NONE',  ( 15.80617190586746368, 15.72974639402197994, 24.37390960531435979 ) ) ;
#112087=CARTESIAN_POINT ( 'NONE',  ( -4.483927247898782831, 16.52544592524335698, 102.7094237280190185 ) ) ;
#112088=CARTESIAN_POINT ( 'NONE',  ( 18.67979575497194134, -10.72451020669871369, 45.83442372801901854 ) ) ;
#112089=CARTESIAN_POINT ( 'NONE',  ( 0.05219959533937995610, -21.53943276465977519, 90.00109039468567573 ) ) ;
#112090=CARTESIAN_POINT ( 'NONE',  ( -18.62759615963255300, -10.81492255796106328, 109.1677570613523613 ) ) ;
#112091=CARTESIAN_POINT ( 'NONE',  ( 16.52544592524335698, 4.483927247898782831, 91.45942372801901854 ) ) ;
#112092=CARTESIAN_POINT ( 'NONE',  ( -18.62759615963255300, -10.81492255796106328, 39.16775706135235424 ) ) ;
#112093=CARTESIAN_POINT ( 'NONE',  ( -19.03943276465977164, 0.05219959533909376836, 26.24890960531435624 ) ) ;
#112094=CARTESIAN_POINT ( 'NONE',  ( -5.719274019375665041, -21.55341960407619695, 104.7927570613523898 ) ) ;
#112095=CARTESIAN_POINT ( 'NONE',  ( -9.564922557960796823, -16.46253265017161027, 112.0822429386476955 ) ) ;
#112096=CARTESIAN_POINT ( 'NONE',  ( 21.53943276465977519, -0.05219959533907433946, 103.7489096053143669 ) ) ;
#112097=CARTESIAN_POINT ( 'NONE',  ( -17.97214573761830536, -5.500000000000087930, 61.46970049038655759 ) ) ;
#112098=CARTESIAN_POINT ( 'NONE',  ( -18.67979575497178146, -10.72451020669898902, 71.66557627198100988 ) ) ;
#112099=CARTESIAN_POINT ( 'NONE',  ( 16.55341960407618274, -4.379528057220086978, 56.04275706135235424 ) ) ;
#112100=CARTESIAN_POINT ( 'NONE',  ( -4.379528057220328563, 16.55341960407611168, 65.20724293864768129 ) ) ;
#112102=CARTESIAN_POINT ( 'NONE',  ( 9.474510206698729675, 16.51473224551082808, 92.08442372801900433 ) ) ;
#112104=CARTESIAN_POINT ( 'NONE',  ( 4.483927247898790824, -16.52544592524335698, 30.20942372801902565 ) ) ;
#112105=CARTESIAN_POINT ( 'NONE',  ( -21.55341960407610458, -5.719274019375992779, 101.4572429386476955 ) ) ;
#112106=CARTESIAN_POINT ( 'NONE',  ( 21.55341960407610458, 5.719274019375980345, 73.95724293864769550 ) ) ;
#112107=CARTESIAN_POINT ( 'NONE',  ( 0.05219959533907565091, 21.53943276465977519, 24.99890960531435624 ) ) ;
#112108=CARTESIAN_POINT ( 'NONE',  ( 8.314922557961029526, -14.29746914071037800, 55.41775706135234714 ) ) ;
#112109=CARTESIAN_POINT ( 'NONE',  ( 19.02544592524343514, -5.153800228976328945, 73.54057627198103830 ) ) ;
#112110=CARTESIAN_POINT ( 'NONE',  ( -5.719274019375665041, -21.55341960407619695, 34.79275706135235424 ) ) ;
#112111=CARTESIAN_POINT ( 'NONE',  ( 13.97604488694548053, -13.89961937509957401, 100.6260903946856615 ) ) ;
#112112=CARTESIAN_POINT ( 'NONE',  ( 19.05341960407611168, 5.049401038298154454, 103.9572429386476671 ) ) ;
#112113=CARTESIAN_POINT ( 'NONE',  ( -16.51473224551069308, -9.474510206698971260, 81.66557627198103830 ) ) ;
#112114=CARTESIAN_POINT ( 'NONE',  ( 18.67979575497178502, 10.72451020669898547, 84.16557627198103830 ) ) ;
#112115=CARTESIAN_POINT ( 'NONE',  ( -19.05341960407611168, -5.049401038298163336, 56.45724293864768129 ) ) ;
#112117=CARTESIAN_POINT ( 'NONE',  ( 14.29746914071049879, -8.314922557960816363, 63.33224293864770260 ) ) ;
#112118=CARTESIAN_POINT ( 'NONE',  ( -10.81492255796078084, -18.62759615963271287, 27.08224293864769550 ) ) ;
#112120=CARTESIAN_POINT ( 'NONE',  ( -15.72974639402197994, 15.80617190586746368, 110.6239096053143669 ) ) ;
#112121=CARTESIAN_POINT ( 'NONE',  ( 13.97604488694548053, -13.89961937509957401, 65.62609039468567573 ) ) ;
#112122=CARTESIAN_POINT ( 'NONE',  ( 18.67979575497178502, 10.72451020669898547, 24.16557627198103120 ) ) ;
#112123=( NAMED_UNIT ( * ) SI_UNIT ( $, .STERADIAN. ) SOLID_ANGLE_UNIT ( ) );
#112124=CARTESIAN_POINT ( 'NONE',  ( 5.823673210054125526, 21.52544592524343514, 59.79057627198103120 ) ) ;
#112125=AXIS2_PLACEMENT_3D ( 'NONE', #169414, #30919, #92567 ) ;
#112126=CARTESIAN_POINT ( 'NONE',  ( -16.46253265017160317, 9.564922557960807481, 90.83224293864769550 ) ) ;
#112127=CARTESIAN_POINT ( 'NONE',  ( 10.72451020669871369, 18.67979575497193778, 77.08442372801901854 ) ) ;
#112128=CARTESIAN_POINT ( 'NONE',  ( -9.564922557960796823, -16.46253265017161027, 47.08224293864769550 ) ) ;
#112129=CARTESIAN_POINT ( 'NONE',  ( 8.314922557960818139, 14.29746914071049879, 89.58224293864768129 ) ) ;
#112130=CARTESIAN_POINT ( 'NONE',  ( -16.52544592524335698, -4.483927247898792601, 33.95942372801901143 ) ) ;
#112131=CARTESIAN_POINT ( 'NONE',  ( -15.80617190586768217, 15.72974639402176855, 68.12609039468567573 ) ) ;
#112133=CARTESIAN_POINT ( 'NONE',  ( -9.564922557961040184, 16.46253265017147172, 27.91775706135232582 ) ) ;
#112134=CARTESIAN_POINT ( 'NONE',  ( -9.474510206698720793, -16.51473224551083518, 79.58442372801899012 ) ) ;
#112136=CARTESIAN_POINT ( 'NONE',  ( -21.53943276465977519, -0.05219959533937600094, 33.75109039468568284 ) ) ;
#112137=DIRECTION ( 'NONE',  ( -1.000000000000000000, -4.336808689942017736E-16, 0.000000000000000000 ) ) ;
#112138=CARTESIAN_POINT ( 'NONE',  ( -13.97604488694547697, 13.89961937509957934, 33.12609039468566863 ) ) ;
#112139=CARTESIAN_POINT ( 'NONE',  ( 13.97604488694527802, 13.89961937509977652, 59.37390960531434558 ) ) ;
#112140=CARTESIAN_POINT ( 'NONE',  ( 19.03943276465977164, 0.05219959533936151252, 26.25109039468566507 ) ) ;
#112141=CARTESIAN_POINT ( 'NONE',  ( 14.34966873604972726, -8.224510206698740333, 100.8344237280190185 ) ) ;
#112142=CARTESIAN_POINT ( 'NONE',  ( 9.564922557960805705, 16.46253265017160317, 114.5822429386476955 ) ) ;
#112143=CARTESIAN_POINT ( 'NONE',  ( 5.823673210054444382, -21.52544592524334988, 80.20942372801901854 ) ) ;
#112145=CARTESIAN_POINT ( 'NONE',  ( -17.49999999999995381, -3.850315288879052389, 35.73370869396556770 ) ) ;
#112146=CARTESIAN_POINT ( 'NONE',  ( -10.72451020669870658, -18.67979575497194134, 89.58442372801901854 ) ) ;
#112147=CARTESIAN_POINT ( 'NONE',  ( 17.05116617787827593, -6.768360034955678728, 41.15675553259200825 ) ) ;
#112148=CARTESIAN_POINT ( 'NONE',  ( -0.05219959533909027116, -19.03943276465977164, 97.49890960531436690 ) ) ;
#112152=DIRECTION ( 'NONE',  ( -0.000000000000000000, 1.000000000000000000, 0.000000000000000000 ) ) ;
#112153=CARTESIAN_POINT ( 'NONE',  ( -19.02544592524342804, 5.153800228976336051, 46.04057627198101699 ) ) ;
#112154=CARTESIAN_POINT ( 'NONE',  ( -5.823673210054116645, -21.52544592524344225, 62.29057627198102409 ) ) ;
#112156=CARTESIAN_POINT ( 'NONE',  ( -14.29746914071049879, 8.314922557960819915, 30.83224293864770260 ) ) ;
#112157=CARTESIAN_POINT ( 'NONE',  ( 16.52544592524342804, -4.483927247898539470, 93.54057627198103830 ) ) ;
#112158=CARTESIAN_POINT ( 'NONE',  ( -16.46253265017160317, 9.564922557960807481, 85.83224293864769550 ) ) ;
#112159=CARTESIAN_POINT ( 'NONE',  ( 9.474510206698729675, 16.51473224551082808, 22.08442372801899722 ) ) ;
#112160=CARTESIAN_POINT ( 'NONE',  ( 5.049401038298161559, -19.05341960407611168, 42.70724293864767418 ) ) ;
#112161=CARTESIAN_POINT ( 'NONE',  ( -16.52544592524342804, 4.483927247898546575, 101.0405762719810383 ) ) ;
#112162=CARTESIAN_POINT ( 'NONE',  ( 21.55341960407619695, -5.719274019375665929, 56.04275706135235424 ) ) ;
#112163=CARTESIAN_POINT ( 'NONE',  ( -10.72451020669898014, 18.67979575497178502, 85.41557627198102409 ) ) ;
#112164=CARTESIAN_POINT ( 'NONE',  ( 16.51473224551083163, -9.474510206698727899, 60.83442372801900433 ) ) ;
#112166=CARTESIAN_POINT ( 'NONE',  ( -19.05341960407611168, -5.049401038298163336, 111.4572429386476671 ) ) ;
#112167=CARTESIAN_POINT ( 'NONE',  ( -4.483927247898539470, -16.52544592524342804, 72.29057627198102409 ) ) ;
#112168=CARTESIAN_POINT ( 'NONE',  ( -16.51473224551082808, 9.474510206698731452, 48.33442372801900433 ) ) ;
#112170=CARTESIAN_POINT ( 'NONE',  ( -9.474510206698964154, 16.51473224551069663, 65.41557627198102409 ) ) ;
#112171=CARTESIAN_POINT ( 'NONE',  ( 0.05219959533910956823, 16.53943276465976808, 64.99890960531435269 ) ) ;
#112172=CARTESIAN_POINT ( 'NONE',  ( -16.46253265017146816, -9.564922557961047289, 79.16775706135234714 ) ) ;
#112173=CARTESIAN_POINT ( 'NONE',  ( 10.72451020669898902, -18.67979575497178502, 32.91557627198102409 ) ) ;
#112175=CARTESIAN_POINT ( 'NONE',  ( 4.379528057220339221, -16.55341960407611168, 102.7072429386476955 ) ) ;
#112176=CARTESIAN_POINT ( 'NONE',  ( -17.50000000000001421, -3.237210098469450070, 25.28763012620440520 ) ) ;
#112177=CARTESIAN_POINT ( 'NONE',  ( 5.153800228976335163, 19.02544592524342804, 59.79057627198100988 ) ) ;
#112178=CARTESIAN_POINT ( 'NONE',  ( 18.67979575497178502, 10.72451020669898547, 69.16557627198102409 ) ) ;
#112179=CARTESIAN_POINT ( 'NONE',  ( 16.46253265017160672, -9.564922557960803928, 38.33224293864768839 ) ) ;
#112180=CARTESIAN_POINT ( 'NONE',  ( 16.55341960407618274, -4.379528057220086978, 76.04275706135237556 ) ) ;
#112181=CARTESIAN_POINT ( 'NONE',  ( -13.97604488694527625, -13.89961937509977652, 71.87390960531433848 ) ) ;
#112182=CARTESIAN_POINT ( 'NONE',  ( 13.97604488694548053, -13.89961937509957401, 55.62609039468566863 ) ) ;
#112183=CARTESIAN_POINT ( 'NONE',  ( -18.67979575497193778, 10.72451020669871902, 68.33442372801900433 ) ) ;
#112184=CARTESIAN_POINT ( 'NONE',  ( 21.52544592524344225, -5.823673210054117533, 48.54057627198103120 ) ) ;
#112185=CARTESIAN_POINT ( 'NONE',  ( 4.379528057220339221, -16.55341960407611168, 112.7072429386476955 ) ) ;
#112186=CARTESIAN_POINT ( 'NONE',  ( 16.55341960407618274, -4.379528057220086978, 81.04275706135236135 ) ) ;
#112187=CARTESIAN_POINT ( 'NONE',  ( 9.474510206698729675, 16.51473224551082808, 107.0844237280190043 ) ) ;
#112188=CARTESIAN_POINT ( 'NONE',  ( 13.89961937509977652, -13.97604488694527269, 23.12390960531436335 ) ) ;
#112189=CARTESIAN_POINT ( 'NONE',  ( 18.09805431107247387, -5.500000000000095923, 43.51606229291886052 ) ) ;
#112190=CARTESIAN_POINT ( 'NONE',  ( 18.67979575497194134, -10.72451020669871369, 100.8344237280190185 ) ) ;
#112191=CARTESIAN_POINT ( 'NONE',  ( -8.224510206698948167, 14.34966873604960824, 50.41557627198103120 ) ) ;
#112192=CARTESIAN_POINT ( 'NONE',  ( -16.52544592524342804, 4.483927247898546575, 76.04057627198102409 ) ) ;
#112193=CARTESIAN_POINT ( 'NONE',  ( -21.53943276465977519, 0.05219959533907696930, 96.24890960531435269 ) ) ;
#112194=CARTESIAN_POINT ( 'NONE',  ( 10.81492255796078972, 18.62759615963270932, 94.58224293864769550 ) ) ;
#112195=CARTESIAN_POINT ( 'NONE',  ( 17.05587630539786304, -6.762274262135686165, 98.24180309037313918 ) ) ;
#112196=CARTESIAN_POINT ( 'NONE',  ( 5.719274019375991003, -21.55341960407610458, 32.70724293864770260 ) ) ;
#112197=CARTESIAN_POINT ( 'NONE',  ( 8.314922557961029526, -14.29746914071037800, 70.41775706135236135 ) ) ;
#112198=CARTESIAN_POINT ( 'NONE',  ( -0.05219959533910754901, -16.53943276465976808, 87.49890960531436690 ) ) ;
#112199=CARTESIAN_POINT ( 'NONE',  ( 9.474510206698971260, -16.51473224551069308, 42.91557627198103120 ) ) ;
#112201=CARTESIAN_POINT ( 'NONE',  ( 16.55341960407618274, -4.379528057220086978, 96.04275706135236135 ) ) ;
#112202=CARTESIAN_POINT ( 'NONE',  ( -10.72451020669870658, -18.67979575497194134, 34.58442372801900433 ) ) ;
#112203=CARTESIAN_POINT ( 'NONE',  ( 19.02544592524343514, -5.153800228976328945, 88.54057627198102409 ) ) ;
#112204=CARTESIAN_POINT ( 'NONE',  ( 21.52544592524334988, 5.823673210054432836, 66.45942372801903275 ) ) ;
#112205=CARTESIAN_POINT ( 'NONE',  ( 9.474510206698971260, -16.51473224551069308, 107.9155762719810383 ) ) ;
#112208=CARTESIAN_POINT ( 'NONE',  ( -21.53943276465977519, -0.05219959533937600094, 58.75109039468568994 ) ) ;
#112209=CARTESIAN_POINT ( 'NONE',  ( 16.46253265017160672, -9.564922557960803928, 33.33224293864770260 ) ) ;
#112210=CARTESIAN_POINT ( 'NONE',  ( -9.474510206698964154, 16.51473224551069663, 115.4155762719810241 ) ) ;
#112211=CARTESIAN_POINT ( 'NONE',  ( 13.89961937509957401, 13.97604488694547697, 71.87609039468567573 ) ) ;
#112212=CARTESIAN_POINT ( 'NONE',  ( 21.55341960407619695, -5.719274019375665929, 26.04275706135235779 ) ) ;
#112213=CARTESIAN_POINT ( 'NONE',  ( -16.51473224551082808, 9.474510206698731452, 63.33442372801900433 ) ) ;
#112214=CARTESIAN_POINT ( 'NONE',  ( -13.89961937509977652, 13.97604488694528158, 30.62390960531435269 ) ) ;
#112215=CARTESIAN_POINT ( 'NONE',  ( -4.379528057220086978, -16.55341960407618274, 89.79275706135236135 ) ) ;
#112216=CARTESIAN_POINT ( 'NONE',  ( 16.46253265017146816, 9.564922557961045513, 66.66775706135233293 ) ) ;
#112217=CARTESIAN_POINT ( 'NONE',  ( 16.55341960407611168, 4.379528057220329451, 28.95724293864769905 ) ) ;
#112218=CARTESIAN_POINT ( 'NONE',  ( -5.153800228976607833, 19.02544592524334988, 47.70942372801900433 ) ) ;
#112220=CARTESIAN_POINT ( 'NONE',  ( 9.474510206698971260, -16.51473224551069308, 82.91557627198103830 ) ) ;
#112221=CARTESIAN_POINT ( 'NONE',  ( 5.719274019375673035, 21.55341960407619339, 92.29275706135236135 ) ) ;
#112222=CARTESIAN_POINT ( 'NONE',  ( 15.80617190586769283, -15.72974639402175789, 105.6260903946856899 ) ) ;
#112224=CARTESIAN_POINT ( 'NONE',  ( 21.53943276465977519, 0.05219959533937863772, 91.25109039468568994 ) ) ;
#112225=CARTESIAN_POINT ( 'NONE',  ( 16.53943276465976808, 0.05219959533934440121, 36.25109039468567573 ) ) ;
#112226=CARTESIAN_POINT ( 'NONE',  ( 16.51473224551069308, 9.474510206698969483, 84.16557627198102409 ) ) ;
#112227=CARTESIAN_POINT ( 'NONE',  ( 18.67979575497178502, 10.72451020669898547, 29.16557627198103120 ) ) ;
#112229=CARTESIAN_POINT ( 'NONE',  ( -5.153800228976328057, -19.02544592524343514, 77.29057627198099567 ) ) ;
#112230=CARTESIAN_POINT ( 'NONE',  ( -19.49190055781009789, -5.500000000000055067, 40.56116087098780554 ) ) ;
#112231=CARTESIAN_POINT ( 'NONE',  ( 5.049401038297881783, 19.05341960407617563, 72.29275706135234714 ) ) ;
#112232=CARTESIAN_POINT ( 'NONE',  ( 5.153800228976335163, 19.02544592524342804, 104.7905762719809957 ) ) ;
#112233=CARTESIAN_POINT ( 'NONE',  ( -10.72451020669870658, -18.67979575497194134, 104.5844237280190185 ) ) ;
#112234=CARTESIAN_POINT ( 'NONE',  ( -14.29746914071049879, 8.314922557960819915, 95.83224293864770971 ) ) ;
#112235=CARTESIAN_POINT ( 'NONE',  ( 18.62759615963271287, -10.81492255796078972, 43.33224293864769550 ) ) ;
#112236=CARTESIAN_POINT ( 'NONE',  ( -5.823673210054116645, -21.52544592524344225, 32.29057627198102409 ) ) ;
#112237=CARTESIAN_POINT ( 'NONE',  ( 12.06949235617757843, -12.14591786802309237, 103.1239096053143811 ) ) ;
#112239=CARTESIAN_POINT ( 'NONE',  ( 5.049401038297881783, 19.05341960407617563, 52.29275706135234003 ) ) ;
#112240=CARTESIAN_POINT ( 'NONE',  ( -14.29746914071049879, 8.314922557960819915, 30.83224293864770260 ) ) ;
#112241=CARTESIAN_POINT ( 'NONE',  ( 16.46253265017160672, -9.564922557960803928, 108.3322429386476955 ) ) ;
#112242=CARTESIAN_POINT ( 'NONE',  ( 21.53943276465977519, 0.05219959533937863772, 76.25109039468568994 ) ) ;
#112243=CARTESIAN_POINT ( 'NONE',  ( 21.55341960407610458, 5.719274019375980345, 63.95724293864770260 ) ) ;
#112244=CARTESIAN_POINT ( 'NONE',  ( -5.719274019375665041, -21.55341960407619695, 49.79275706135234714 ) ) ;
#112245=CARTESIAN_POINT ( 'NONE',  ( -5.719274019375978568, 21.55341960407610458, 90.20724293864770971 ) ) ;
#112246=CARTESIAN_POINT ( 'NONE',  ( -15.72974639402176322, -15.80617190586768395, 44.37609039468567573 ) ) ;
#112247=CARTESIAN_POINT ( 'NONE',  ( 13.97604488694527802, 13.89961937509977652, 24.37390960531435624 ) ) ;
#112248=CARTESIAN_POINT ( 'NONE',  ( 16.51473224551069308, 9.474510206698969483, 89.16557627198103830 ) ) ;
#112249=CARTESIAN_POINT ( 'NONE',  ( -8.224510206698948167, 14.34966873604960824, 100.4155762719810241 ) ) ;
#112250=CARTESIAN_POINT ( 'NONE',  ( -13.97604488694527625, -13.89961937509977652, 111.8739096053143243 ) ) ;
#112251=CARTESIAN_POINT ( 'NONE',  ( -8.224510206698948167, 14.34966873604960824, 50.41557627198103120 ) ) ;
#112252=CARTESIAN_POINT ( 'NONE',  ( 16.53943276465976808, -0.05219959533910856209, 23.74890960531435269 ) ) ;
#112253=CARTESIAN_POINT ( 'NONE',  ( -0.05219959533909027116, -19.03943276465977164, 47.49890960531435979 ) ) ;
#112254=CARTESIAN_POINT ( 'NONE',  ( -0.05219959533909027116, -19.03943276465977164, 22.49890960531436690 ) ) ;
#112255=CARTESIAN_POINT ( 'NONE',  ( 15.80617190586746368, 15.72974639402197994, 49.37390960531436690 ) ) ;
#112256=CARTESIAN_POINT ( 'NONE',  ( 19.05341960407617918, -5.049401038297876454, 21.04275706135232582 ) ) ;
#112258=CARTESIAN_POINT ( 'NONE',  ( -12.06949235617756955, 12.14591786802309770, 40.62390960531435269 ) ) ;
#112259=CARTESIAN_POINT ( 'NONE',  ( 15.72974639402176855, 15.80617190586768217, 46.87609039468568994 ) ) ;
#112260=CARTESIAN_POINT ( 'NONE',  ( -5.049401038298153566, 19.05341960407611168, 115.2072429386477097 ) ) ;
#112261=CARTESIAN_POINT ( 'NONE',  ( 16.52544592524335698, 4.483927247898782831, 61.45942372801901854 ) ) ;
#112262=CARTESIAN_POINT ( 'NONE',  ( -9.564922557961040184, 16.46253265017147172, 62.91775706135233293 ) ) ;
#112263=CARTESIAN_POINT ( 'NONE',  ( -16.55341960407611168, -4.379528057220339221, 21.45724293864769550 ) ) ;
#112264=CARTESIAN_POINT ( 'NONE',  ( 16.52544592524335698, 4.483927247898782831, 106.4594237280190328 ) ) ;
#112265=CARTESIAN_POINT ( 'NONE',  ( 13.89961937509977652, -13.97604488694527269, 43.12390960531434558 ) ) ;
#112266=CARTESIAN_POINT ( 'NONE',  ( 19.02544592524343514, -5.153800228976328945, 58.54057627198102409 ) ) ;
#112267=CARTESIAN_POINT ( 'NONE',  ( -16.51473224551069308, -9.474510206698971260, 31.66557627198102054 ) ) ;
#112268=CARTESIAN_POINT ( 'NONE',  ( -21.52544592524334988, -5.823673210054445271, 38.95942372801901854 ) ) ;
#112269=CARTESIAN_POINT ( 'NONE',  ( -9.474510206698964154, 16.51473224551069663, 45.41557627198103120 ) ) ;
#112270=CARTESIAN_POINT ( 'NONE',  ( 9.564922557960805705, 16.46253265017160317, 114.5822429386476955 ) ) ;
#112271=CARTESIAN_POINT ( 'NONE',  ( -0.05219959533909027116, -19.03943276465977164, 52.49890960531436690 ) ) ;
#112272=CARTESIAN_POINT ( 'NONE',  ( 0.05219959533909260263, 19.03943276465977164, 114.9989096053143669 ) ) ;
#112273=CARTESIAN_POINT ( 'NONE',  ( -21.53943276465977519, -0.05219959533937600094, 58.75109039468568994 ) ) ;
#112274=CARTESIAN_POINT ( 'NONE',  ( 16.55341960407611168, 4.379528057220329451, 98.95724293864770971 ) ) ;
#112275=CARTESIAN_POINT ( 'NONE',  ( -5.049401038298153566, 19.05341960407611168, 110.2072429386476671 ) ) ;
#112276=CARTESIAN_POINT ( 'NONE',  ( -16.52544592524335698, -4.483927247898792601, 78.95942372801901854 ) ) ;
#112278=CARTESIAN_POINT ( 'NONE',  ( -0.05219959533937732626, 21.53943276465977519, 87.50109039468568994 ) ) ;
#112280=CARTESIAN_POINT ( 'NONE',  ( 4.483927247898790824, -16.52544592524335698, 50.20942372801901854 ) ) ;
#112281=CARTESIAN_POINT ( 'NONE',  ( -13.89961937509977652, 13.97604488694528158, 95.62390960531436690 ) ) ;
#112282=CARTESIAN_POINT ( 'NONE',  ( -16.52544592524335698, -4.483927247898792601, 38.95942372801901854 ) ) ;
#112283=CARTESIAN_POINT ( 'NONE',  ( -16.55341960407617563, 4.379528057220093196, 33.54275706135234714 ) ) ;
#112284=CARTESIAN_POINT ( 'NONE',  ( -12.14591786802326823, 12.06949235617739902, 88.12609039468570415 ) ) ;
#112285=CARTESIAN_POINT ( 'NONE',  ( -19.05341960407617563, 5.049401038297882671, 108.5427570613523187 ) ) ;
#112286=CARTESIAN_POINT ( 'NONE',  ( -10.81492255796078084, -18.62759615963271287, 102.0822429386476955 ) ) ;
#112287=CARTESIAN_POINT ( 'NONE',  ( -14.29746914071049879, 8.314922557960819915, 100.8322429386477097 ) ) ;
#112288=CARTESIAN_POINT ( 'NONE',  ( -19.05341960407617563, 5.049401038297882671, 98.54275706135233293 ) ) ;
#112289=CARTESIAN_POINT ( 'NONE',  ( 12.06949235617739724, 12.14591786802326823, 66.87609039468568994 ) ) ;
#112290=CARTESIAN_POINT ( 'NONE',  ( -17.12812012977051523, 6.668231424565586707, 43.64051240676855770 ) ) ;
#112291=CARTESIAN_POINT ( 'NONE',  ( 19.03943276465977164, 0.05219959533936151252, 76.25109039468566152 ) ) ;
#112292=CARTESIAN_POINT ( 'NONE',  ( -12.06949235617756955, 12.14591786802309770, 45.62390960531436690 ) ) ;
#112293=CARTESIAN_POINT ( 'NONE',  ( 8.224510206698953496, -14.34966873604960469, 27.91557627198103830 ) ) ;
#112294=CARTESIAN_POINT ( 'NONE',  ( 14.29746914071049879, -8.314922557960816363, 88.33224293864769550 ) ) ;
#112295=CARTESIAN_POINT ( 'NONE',  ( -19.03943276465977164, -0.05219959533935918106, 38.75109039468566152 ) ) ;
#112296=CARTESIAN_POINT ( 'NONE',  ( -17.40861289039000681, 6.110651285853376358, 88.62767529172568004 ) ) ;
#112297=CARTESIAN_POINT ( 'NONE',  ( 18.62759615963255655, 10.81492255796105972, 36.66775706135234714 ) ) ;
#112298=CARTESIAN_POINT ( 'NONE',  ( -19.02544592524334988, -5.153800228976617603, 98.95942372801900433 ) ) ;
#112300=CARTESIAN_POINT ( 'NONE',  ( -19.03943276465977164, 0.05219959533909376836, 91.24890960531436690 ) ) ;
#112301=CARTESIAN_POINT ( 'NONE',  ( 13.89961937509977652, -13.97604488694527269, 93.12390960531436690 ) ) ;
#112302=CARTESIAN_POINT ( 'NONE',  ( 5.719274019375991003, -21.55341960407610458, 62.70724293864769550 ) ) ;
#112303=CARTESIAN_POINT ( 'NONE',  ( 8.314922557960818139, 14.29746914071049879, 94.58224293864769550 ) ) ;
#112304=CARTESIAN_POINT ( 'NONE',  ( 0.05219959533909260263, 19.03943276465977164, 69.99890960531435269 ) ) ;
#112305=CARTESIAN_POINT ( 'NONE',  ( -0.05219959533909027116, -19.03943276465977164, 22.49890960531436690 ) ) ;
#112306=CARTESIAN_POINT ( 'NONE',  ( -10.72451020669870658, -18.67979575497194134, 34.58442372801900433 ) ) ;
#112307=CARTESIAN_POINT ( 'NONE',  ( 21.52544592524334988, 5.823673210054432836, 76.45942372801901854 ) ) ;
#112308=CARTESIAN_POINT ( 'NONE',  ( -16.46253265017160317, 9.564922557960807481, 60.83224293864769550 ) ) ;
#112309=CARTESIAN_POINT ( 'NONE',  ( -8.314922557961024197, 14.29746914071037800, 77.91775706135231871 ) ) ;
#112310=CARTESIAN_POINT ( 'NONE',  ( 18.62759615963255655, 10.81492255796105972, 26.66775706135235424 ) ) ;
#112311=CARTESIAN_POINT ( 'NONE',  ( -5.719274019375665041, -21.55341960407619695, 24.79275706135235779 ) ) ;
#112312=CARTESIAN_POINT ( 'NONE',  ( -13.97604488694547697, 13.89961937509957934, 58.12609039468566863 ) ) ;
#112313=CARTESIAN_POINT ( 'NONE',  ( 19.05341960407611168, 5.049401038298154454, 73.95724293864768129 ) ) ;
#112314=CARTESIAN_POINT ( 'NONE',  ( -5.153800228976607833, 19.02544592524334988, 32.70942372801899722 ) ) ;
#112315=CARTESIAN_POINT ( 'NONE',  ( -15.80617190586768217, 15.72974639402176855, 78.12609039468570415 ) ) ;
#112316=CARTESIAN_POINT ( 'NONE',  ( 10.72451020669898902, -18.67979575497178502, 67.91557627198102409 ) ) ;
#112317=CARTESIAN_POINT ( 'NONE',  ( 4.379528057220339221, -16.55341960407611168, 52.70724293864769550 ) ) ;
#112318=CARTESIAN_POINT ( 'NONE',  ( -21.53943276465977519, -0.05219959533937600094, 88.75109039468567573 ) ) ;
#112319=CARTESIAN_POINT ( 'NONE',  ( -13.89961937509957401, -13.97604488694547875, 24.37609039468565442 ) ) ;
#112320=CARTESIAN_POINT ( 'NONE',  ( 0.05219959533910956823, 16.53943276465976808, 64.99890960531435269 ) ) ;
#112321=CARTESIAN_POINT ( 'NONE',  ( -16.51473224551069308, -9.474510206698971260, 21.66557627198102765 ) ) ;
#112322=CARTESIAN_POINT ( 'NONE',  ( -16.51473224551082808, 9.474510206698731452, 68.33442372801900433 ) ) ;
#112323=CARTESIAN_POINT ( 'NONE',  ( -0.05219959533910754901, -16.53943276465976808, 37.49890960531436690 ) ) ;
#112324=CARTESIAN_POINT ( 'NONE',  ( 15.72974639402176855, 15.80617190586768217, 76.87609039468567573 ) ) ;
#112325=CARTESIAN_POINT ( 'NONE',  ( 13.89961937509977652, -13.97604488694527269, 73.12390960531436690 ) ) ;
#112326=CARTESIAN_POINT ( 'NONE',  ( -0.05219959533936034679, 19.03943276465977164, 47.50109039468566863 ) ) ;
#112327=CARTESIAN_POINT ( 'NONE',  ( 10.72451020669898902, -18.67979575497178502, 52.91557627198103830 ) ) ;
#112328=CARTESIAN_POINT ( 'NONE',  ( -15.72974639402176322, -15.80617190586768395, 39.37609039468567573 ) ) ;
#112329=CARTESIAN_POINT ( 'NONE',  ( -10.81492255796078084, -18.62759615963271287, 97.08224293864770971 ) ) ;
#112330=CARTESIAN_POINT ( 'NONE',  ( -14.29746914071037622, -8.314922557961029526, 19.16775706135234714 ) ) ;
#112331=CARTESIAN_POINT ( 'NONE',  ( -12.06949235617739369, -12.14591786802326823, 69.37609039468567573 ) ) ;
#112332=CARTESIAN_POINT ( 'NONE',  ( 17.50000000000000000, 5.500000000000013323, 63.78230962303565832 ) ) ;
#112333=CARTESIAN_POINT ( 'NONE',  ( -15.80617190586745835, -15.72974639402198527, 101.8739096053143811 ) ) ;
#112334=CARTESIAN_POINT ( 'NONE',  ( -0.05219959533910754901, -16.53943276465976808, 107.4989096053143669 ) ) ;
#112336=CARTESIAN_POINT ( 'NONE',  ( -4.483927247898782831, 16.52544592524335698, 32.70942372801900433 ) ) ;
#112337=CARTESIAN_POINT ( 'NONE',  ( -21.53943276465977519, 0.05219959533907696930, 66.24890960531436690 ) ) ;
#112338=CARTESIAN_POINT ( 'NONE',  ( -16.55341960407617563, 4.379528057220093196, 108.5427570613523756 ) ) ;
#112339=CARTESIAN_POINT ( 'NONE',  ( 13.89961937509977652, -13.97604488694527269, 33.12390960531434558 ) ) ;
#112340=CARTESIAN_POINT ( 'NONE',  ( 16.55341960407618274, -4.379528057220086978, 66.04275706135236135 ) ) ;
#112341=CARTESIAN_POINT ( 'NONE',  ( 9.474510206698729675, 16.51473224551082808, 62.08442372801899722 ) ) ;
#112342=CARTESIAN_POINT ( 'NONE',  ( 5.719274019375673035, 21.55341960407619339, 37.29275706135235424 ) ) ;
#112343=CARTESIAN_POINT ( 'NONE',  ( -18.67979575497178146, -10.72451020669898902, 61.66557627198103120 ) ) ;
#112344=CARTESIAN_POINT ( 'NONE',  ( 16.52544592524335698, 4.483927247898782831, 96.45942372801901854 ) ) ;
#112345=CARTESIAN_POINT ( 'NONE',  ( -5.719274019375665041, -21.55341960407619695, 64.79275706135234714 ) ) ;
#112346=CARTESIAN_POINT ( 'NONE',  ( 21.52544592524344225, -5.823673210054117533, 48.54057627198103120 ) ) ;
#112347=CARTESIAN_POINT ( 'NONE',  ( 21.55341960407610458, 5.719274019375980345, 33.95724293864769550 ) ) ;
#112348=EDGE_LOOP ( 'NONE', ( #156592, #141283, #73285, #191194 ) ) ;
#112349=EDGE_LOOP ( 'NONE', ( #191536, #81613, #131867, #104003 ) ) ;
#112350=CARTESIAN_POINT ( 'NONE',  ( -14.29746914071037622, -8.314922557961029526, 79.16775706135234714 ) ) ;
#112351=CARTESIAN_POINT ( 'NONE',  ( -15.80617190586745835, -15.72974639402198527, 26.87390960531435979 ) ) ;
#112352=ORIENTED_EDGE ( 'NONE', *, *, #138165, .T. ) ;
#112353=CARTESIAN_POINT ( 'NONE',  ( 13.89961937509977652, -13.97604488694527269, 93.12390960531436690 ) ) ;
#112354=CARTESIAN_POINT ( 'NONE',  ( -8.314922557960811034, -14.29746914071050412, 22.08224293864769194 ) ) ;
#112356=CARTESIAN_POINT ( 'NONE',  ( 4.483927247898545687, 16.52544592524342804, 104.7905762719810241 ) ) ;
#112357=CARTESIAN_POINT ( 'NONE',  ( -18.62759615963270932, 10.81492255796079327, 55.83224293864770260 ) ) ;
#112358=CARTESIAN_POINT ( 'NONE',  ( 14.29746914071037800, 8.314922557961029526, 96.66775706135234714 ) ) ;
#112359=CARTESIAN_POINT ( 'NONE',  ( 10.72451020669871369, 18.67979575497193778, 52.08442372801901854 ) ) ;
#112360=CARTESIAN_POINT ( 'NONE',  ( 9.474510206698729675, 16.51473224551082808, 102.0844237280190043 ) ) ;
#112361=CARTESIAN_POINT ( 'NONE',  ( 16.52544592524342804, -4.483927247898539470, 98.54057627198105251 ) ) ;
#112362=CARTESIAN_POINT ( 'NONE',  ( -19.03943276465977164, -0.05219959533935918106, 113.7510903946856757 ) ) ;
#112363=CARTESIAN_POINT ( 'NONE',  ( -19.02544592524342804, 5.153800228976336051, 31.04057627198102409 ) ) ;
#112365=CARTESIAN_POINT ( 'NONE',  ( 13.89961937509977652, -13.97604488694527269, 88.12390960531438111 ) ) ;
#112366=CARTESIAN_POINT ( 'NONE',  ( 16.55341960407618274, -4.379528057220086978, 71.04275706135234714 ) ) ;
#112367=CARTESIAN_POINT ( 'NONE',  ( 21.55341960407619695, -5.719274019375665929, 111.0427570613523613 ) ) ;
#112368=CARTESIAN_POINT ( 'NONE',  ( 5.719274019375991003, -21.55341960407610458, 62.70724293864769550 ) ) ;
#112369=CARTESIAN_POINT ( 'NONE',  ( -12.06949235617739369, -12.14591786802326823, 89.37609039468568994 ) ) ;
#112370=CARTESIAN_POINT ( 'NONE',  ( -9.474510206698720793, -16.51473224551083518, 79.58442372801899012 ) ) ;
#112371=CARTESIAN_POINT ( 'NONE',  ( -9.564922557960796823, -16.46253265017161027, 32.08224293864769550 ) ) ;
#112372=CARTESIAN_POINT ( 'NONE',  ( -19.03943276465977164, 0.05219959533909376836, 76.24890960531435269 ) ) ;
#112373=CARTESIAN_POINT ( 'NONE',  ( -5.153800228976328057, -19.02544592524343514, 27.29057627198103120 ) ) ;
#112374=CARTESIAN_POINT ( 'NONE',  ( 19.02544592524334988, 5.153800228976608722, 66.45942372801899012 ) ) ;
#112376=CARTESIAN_POINT ( 'NONE',  ( 13.89961937509977652, -13.97604488694527269, 98.12390960531433848 ) ) ;
#112377=CARTESIAN_POINT ( 'NONE',  ( -12.06949235617756955, 12.14591786802309770, 45.62390960531436690 ) ) ;
#112378=CARTESIAN_POINT ( 'NONE',  ( -10.72451020669898014, 18.67979575497178502, 65.41557627198102409 ) ) ;
#112380=CARTESIAN_POINT ( 'NONE',  ( -9.474510206698720793, -16.51473224551083518, 29.58442372801900433 ) ) ;
#112382=CARTESIAN_POINT ( 'NONE',  ( 5.153800228976335163, 19.02544592524342804, 49.79057627198100988 ) ) ;
#112383=CARTESIAN_POINT ( 'NONE',  ( 13.89961937509977652, -13.97604488694527269, 73.12390960531436690 ) ) ;
#112384=CARTESIAN_POINT ( 'NONE',  ( -8.314922557961024197, 14.29746914071037800, 37.91775706135235424 ) ) ;
#112385=CARTESIAN_POINT ( 'NONE',  ( -19.25918095147779852, -5.499999999999535483, 99.45284276293932635 ) ) ;
#112387=CARTESIAN_POINT ( 'NONE',  ( -0.05219959533934338120, 16.53943276465976808, 82.50109039468568994 ) ) ;
#112388=CARTESIAN_POINT ( 'NONE',  ( -21.52544592524343514, 5.823673210054127303, 96.04057627198102409 ) ) ;
#112390=CARTESIAN_POINT ( 'NONE',  ( -16.53943276465976808, -0.05219959533934237506, 43.75109039468568284 ) ) ;
#112391=CARTESIAN_POINT ( 'NONE',  ( 9.564922557960805705, 16.46253265017160317, 44.58224293864769550 ) ) ;
#112393=CARTESIAN_POINT ( 'NONE',  ( 5.823673210054444382, -21.52544592524334988, 50.20942372801901854 ) ) ;
#112394=CARTESIAN_POINT ( 'NONE',  ( 19.02544592524334988, 5.153800228976608722, 56.45942372801898301 ) ) ;
#112395=CARTESIAN_POINT ( 'NONE',  ( -5.719274019375665041, -21.55341960407619695, 99.79275706135234714 ) ) ;
#112396=CARTESIAN_POINT ( 'NONE',  ( 16.20579543436678449, 7.371946100355102338, 98.06520834171875833 ) ) ;
#112398=CARTESIAN_POINT ( 'NONE',  ( -21.53943276465977519, 0.05219959533907696930, 51.24890960531436690 ) ) ;
#112399=CARTESIAN_POINT ( 'NONE',  ( 13.89961937509977652, -13.97604488694527269, 98.12390960531433848 ) ) ;
#112400=CARTESIAN_POINT ( 'NONE',  ( -8.314922557960811034, -14.29746914071050412, 102.0822429386476955 ) ) ;
#112401=CARTESIAN_POINT ( 'NONE',  ( 4.379528057220092307, 16.55341960407617563, 22.29275706135235069 ) ) ;
#112402=CARTESIAN_POINT ( 'NONE',  ( 16.53943276465976808, 0.05219959533934440121, 106.2510903946856757 ) ) ;
#112403=VERTEX_POINT ( 'NONE', #9084 ) ;
#112404=CARTESIAN_POINT ( 'NONE',  ( -21.53943276465977519, 0.05219959533907696930, 96.24890960531435269 ) ) ;
#112405=CARTESIAN_POINT ( 'NONE',  ( 16.52544592524342804, -4.483927247898539470, 33.54057627198102409 ) ) ;
#112407=CARTESIAN_POINT ( 'NONE',  ( -13.97604488694547697, 13.89961937509957934, 88.12609039468563310 ) ) ;
#112408=CARTESIAN_POINT ( 'NONE',  ( -0.05219959533937732626, 21.53943276465977519, 107.5010903946856899 ) ) ;
#112409=CARTESIAN_POINT ( 'NONE',  ( -16.53943276465976808, 0.05219959533911058130, 31.24890960531435979 ) ) ;
#112410=CARTESIAN_POINT ( 'NONE',  ( -21.52544592524343514, 5.823673210054127303, 91.04057627198103830 ) ) ;
#112411=CARTESIAN_POINT ( 'NONE',  ( -21.53943276465977519, 0.05219959533907696930, 46.24890960531435979 ) ) ;
#112412=CARTESIAN_POINT ( 'NONE',  ( -19.05341960407611168, -5.049401038298163336, 61.45724293864769550 ) ) ;
#112413=CARTESIAN_POINT ( 'NONE',  ( 14.29746914071049879, -8.314922557960816363, 38.33224293864768839 ) ) ;
#112414=CARTESIAN_POINT ( 'NONE',  ( -9.474510206698964154, 16.51473224551069663, 95.41557627198102409 ) ) ;
#112416=CARTESIAN_POINT ( 'NONE',  ( 19.25918095147780917, 5.499999999999578115, 56.95284276293935477 ) ) ;
#112417=CARTESIAN_POINT ( 'NONE',  ( 5.049401038297881783, 19.05341960407617563, 42.29275706135234003 ) ) ;
#112418=CARTESIAN_POINT ( 'NONE',  ( -15.72974639402197994, 15.80617190586746368, 85.62390960531436690 ) ) ;
#112419=CARTESIAN_POINT ( 'NONE',  ( 16.53943276465976808, -0.05219959533910856209, 93.74890960531436690 ) ) ;
#112420=CARTESIAN_POINT ( 'NONE',  ( -18.67979575497193778, 10.72451020669871902, 43.33442372801901143 ) ) ;
#112423=CARTESIAN_POINT ( 'NONE',  ( -14.29746914071037622, -8.314922557961029526, 109.1677570613523613 ) ) ;
#112424=CARTESIAN_POINT ( 'NONE',  ( 19.03943276465977164, -0.05219959533909143690, 33.74890960531435979 ) ) ;
#112425=CARTESIAN_POINT ( 'NONE',  ( -9.474510206698964154, 16.51473224551069663, 85.41557627198102409 ) ) ;
#112426=CARTESIAN_POINT ( 'NONE',  ( 17.60769864724390388, -5.499999999999974243, 71.15024842019164453 ) ) ;
#112427=CARTESIAN_POINT ( 'NONE',  ( 16.51473224551069308, 9.474510206698969483, 29.16557627198103475 ) ) ;
#112428=CARTESIAN_POINT ( 'NONE',  ( 4.483927247898545687, 16.52544592524342804, 49.79057627198102409 ) ) ;
#112430=CARTESIAN_POINT ( 'NONE',  ( 10.72451020669871369, 18.67979575497193778, 67.08442372801901854 ) ) ;
#112432=CARTESIAN_POINT ( 'NONE',  ( -16.52544592524335698, -4.483927247898792601, 68.95942372801901854 ) ) ;
#112433=CARTESIAN_POINT ( 'NONE',  ( -16.51473224551069308, -9.474510206698971260, 56.66557627198103120 ) ) ;
#112434=CARTESIAN_POINT ( 'NONE',  ( 9.474510206698971260, -16.51473224551069308, 47.91557627198102409 ) ) ;
#112436=CARTESIAN_POINT ( 'NONE',  ( 5.719274019375673035, 21.55341960407619339, 107.2927570613523471 ) ) ;
#112437=CARTESIAN_POINT ( 'NONE',  ( -8.224510206698735004, -14.34966873604973081, 64.58442372801900433 ) ) ;
#112438=CARTESIAN_POINT ( 'NONE',  ( 15.72974639402176855, 15.80617190586768217, 101.8760903946857042 ) ) ;
#112439=CARTESIAN_POINT ( 'NONE',  ( 5.823673210054125526, 21.52544592524343514, 29.79057627198102409 ) ) ;
#112440=CARTESIAN_POINT ( 'NONE',  ( -13.97604488694547697, 13.89961937509957934, 113.1260903946856757 ) ) ;
#112441=CARTESIAN_POINT ( 'NONE',  ( -0.05219959533937732626, 21.53943276465977519, 72.50109039468568994 ) ) ;
#112442=CARTESIAN_POINT ( 'NONE',  ( 8.314922557961029526, -14.29746914071037800, 45.41775706135234003 ) ) ;
#112443=CARTESIAN_POINT ( 'NONE',  ( -21.53943276465977519, 0.05219959533907696930, 96.24890960531435269 ) ) ;
#112444=CARTESIAN_POINT ( 'NONE',  ( 19.05341960407617918, -5.049401038297876454, 101.0427570613523045 ) ) ;
#112445=CARTESIAN_POINT ( 'NONE',  ( -0.05219959533909027116, -19.03943276465977164, 62.49890960531435979 ) ) ;
#112446=CARTESIAN_POINT ( 'NONE',  ( 14.34966873604972726, -8.224510206698740333, 20.83442372801901143 ) ) ;
#112447=CARTESIAN_POINT ( 'NONE',  ( 13.97604488694548053, -13.89961937509957401, 105.6260903946856757 ) ) ;
#112448=CARTESIAN_POINT ( 'NONE',  ( -16.53943276465976808, 0.05219959533911058130, 66.24890960531436690 ) ) ;
#112449=CARTESIAN_POINT ( 'NONE',  ( 16.55341960407618274, -4.379528057220086978, 76.04275706135237556 ) ) ;
#112450=CARTESIAN_POINT ( 'NONE',  ( 5.823673210054125526, 21.52544592524343514, 114.7905762719810383 ) ) ;
#112451=CARTESIAN_POINT ( 'NONE',  ( -13.97604488694527625, -13.89961937509977652, 51.87390960531436690 ) ) ;
#112452=CARTESIAN_POINT ( 'NONE',  ( 19.03943276465977164, -0.05219959533909143690, 53.74890960531436690 ) ) ;
#112453=CARTESIAN_POINT ( 'NONE',  ( -4.483927247898782831, 16.52544592524335698, 72.70942372801901854 ) ) ;
#112456=CARTESIAN_POINT ( 'NONE',  ( 5.719274019375673035, 21.55341960407619339, 112.2927570613523471 ) ) ;
#112458=CARTESIAN_POINT ( 'NONE',  ( -8.224510206698735004, -14.34966873604973081, 19.58442372801901143 ) ) ;
#112459=CARTESIAN_POINT ( 'NONE',  ( 10.72451020669898902, -18.67979575497178502, 47.91557627198102409 ) ) ;
#112460=CARTESIAN_POINT ( 'NONE',  ( 16.46253265017146816, 9.564922557961045513, 46.66775706135233293 ) ) ;
#112461=CARTESIAN_POINT ( 'NONE',  ( -0.05219959533934338120, 16.53943276465976808, 32.50109039468568284 ) ) ;
#112462=CARTESIAN_POINT ( 'NONE',  ( 9.564922557960805705, 16.46253265017160317, 49.58224293864770260 ) ) ;
#112463=CARTESIAN_POINT ( 'NONE',  ( 19.02544592524343514, -5.153800228976328945, 48.54057627198103120 ) ) ;
#112464=CARTESIAN_POINT ( 'NONE',  ( -10.81492255796078084, -18.62759615963271287, 82.08224293864768129 ) ) ;
#112465=CARTESIAN_POINT ( 'NONE',  ( 13.89961937509977652, -13.97604488694527269, 108.1239096053143669 ) ) ;
#112466=CARTESIAN_POINT ( 'NONE',  ( -19.05341960407611168, -5.049401038298163336, 46.45724293864768129 ) ) ;
#112468=CARTESIAN_POINT ( 'NONE',  ( 0.05219959533936267826, -19.03943276465977164, 100.0010903946856757 ) ) ;
#112469=CARTESIAN_POINT ( 'NONE',  ( 0.05219959533910956823, 16.53943276465976808, 64.99890960531435269 ) ) ;
#112470=CARTESIAN_POINT ( 'NONE',  ( 16.46253265017146816, 9.564922557961045513, 26.66775706135234003 ) ) ;
#112471=CARTESIAN_POINT ( 'NONE',  ( 18.62759615963271287, -10.81492255796078972, 98.33224293864769550 ) ) ;
#112472=CARTESIAN_POINT ( 'NONE',  ( 15.80617190586769283, -15.72974639402175789, 80.62609039468567573 ) ) ;
#112473=CARTESIAN_POINT ( 'NONE',  ( -5.049401038298153566, 19.05341960407611168, 25.20724293864768484 ) ) ;
#112474=CARTESIAN_POINT ( 'NONE',  ( -21.53943276465977519, -0.05219959533937600094, 73.75109039468567573 ) ) ;
#112475=CARTESIAN_POINT ( 'NONE',  ( 16.52544592524342804, -4.483927247898539470, 23.54057627198102765 ) ) ;
#112476=CARTESIAN_POINT ( 'NONE',  ( 18.62759615963255655, 10.81492255796105972, 81.66775706135236135 ) ) ;
#112477=CARTESIAN_POINT ( 'NONE',  ( 16.51473224551069308, 9.474510206698969483, 69.16557627198102409 ) ) ;
#112478=CARTESIAN_POINT ( 'NONE',  ( 5.823673210054444382, -21.52544592524334988, 45.20942372801901854 ) ) ;
#112479=CARTESIAN_POINT ( 'NONE',  ( 13.97604488694527802, 13.89961937509977652, 84.37390960531433848 ) ) ;
#112480=CARTESIAN_POINT ( 'NONE',  ( 12.14591786802309770, 12.06949235617756955, 99.37390960531436690 ) ) ;
#112481=CARTESIAN_POINT ( 'NONE',  ( -12.14591786802309592, -12.06949235617757132, 61.87390960531436690 ) ) ;
#112482=CARTESIAN_POINT ( 'NONE',  ( -5.823673210054116645, -21.52544592524344225, 67.29057627198103830 ) ) ;
#112483=CARTESIAN_POINT ( 'NONE',  ( -9.474510206698964154, 16.51473224551069663, 80.41557627198103830 ) ) ;
#112484=CARTESIAN_POINT ( 'NONE',  ( -5.719274019375978568, 21.55341960407610458, 85.20724293864770971 ) ) ;
#112485=CARTESIAN_POINT ( 'NONE',  ( -19.02544592524334988, -5.153800228976617603, 63.95942372801899012 ) ) ;
#112486=CARTESIAN_POINT ( 'NONE',  ( 0.05219959533936267826, -19.03943276465977164, 35.00109039468566863 ) ) ;
#112487=CARTESIAN_POINT ( 'NONE',  ( 16.53943276465976808, -0.05219959533910856209, 73.74890960531433848 ) ) ;
#112488=CARTESIAN_POINT ( 'NONE',  ( 15.80617190586746368, 15.72974639402197994, 59.37390960531436690 ) ) ;
#112490=CARTESIAN_POINT ( 'NONE',  ( 4.379528057220092307, 16.55341960407617563, 92.29275706135236135 ) ) ;
#112492=CARTESIAN_POINT ( 'NONE',  ( -19.03943276465977164, -0.05219959533935918106, 98.75109039468567573 ) ) ;
#112493=CARTESIAN_POINT ( 'NONE',  ( 8.224510206698953496, -14.34966873604960469, 62.91557627198102409 ) ) ;
#112494=CARTESIAN_POINT ( 'NONE',  ( -17.50000000000002132, 3.471454075611629442, 34.48332581144360631 ) ) ;
#112495=CARTESIAN_POINT ( 'NONE',  ( -19.02544592524342804, 5.153800228976336051, 66.04057627198103830 ) ) ;
#112496=CARTESIAN_POINT ( 'NONE',  ( -14.29746914071049879, 8.314922557960819915, 50.83224293864770971 ) ) ;
#112497=CARTESIAN_POINT ( 'NONE',  ( 19.02544592524343514, -5.153800228976328945, 98.54057627198100988 ) ) ;
#112498=CARTESIAN_POINT ( 'NONE',  ( -9.474510206698720793, -16.51473224551083518, 79.58442372801899012 ) ) ;
#112499=CARTESIAN_POINT ( 'NONE',  ( 19.02544592524343514, -5.153800228976328945, 68.54057627198103830 ) ) ;
#112500=CARTESIAN_POINT ( 'NONE',  ( 9.474510206698971260, -16.51473224551069308, 82.91557627198103830 ) ) ;
#112501=CARTESIAN_POINT ( 'NONE',  ( -5.049401038298153566, 19.05341960407611168, 80.20724293864769550 ) ) ;
#112502=CARTESIAN_POINT ( 'NONE',  ( -15.80617190586745835, -15.72974639402198527, 56.87390960531436690 ) ) ;
#112503=CARTESIAN_POINT ( 'NONE',  ( 16.53943276465976808, 0.05219959533934440121, 51.25109039468568994 ) ) ;
#112504=CARTESIAN_POINT ( 'NONE',  ( 17.72662750342729510, 5.499999999999959144, 98.90179492283746754 ) ) ;
#112505=CARTESIAN_POINT ( 'NONE',  ( -16.46253265017160317, 9.564922557960807481, 55.83224293864769550 ) ) ;
#112506=CARTESIAN_POINT ( 'NONE',  ( 5.719274019375991003, -21.55341960407610458, 57.70724293864770260 ) ) ;
#112507=CARTESIAN_POINT ( 'NONE',  ( -0.05219959533936034679, 19.03943276465977164, 92.50109039468566152 ) ) ;
#112508=CARTESIAN_POINT ( 'NONE',  ( -4.483927247898539470, -16.52544592524342804, 27.29057627198103120 ) ) ;
#112509=CARTESIAN_POINT ( 'NONE',  ( 15.72974639402176855, 15.80617190586768217, 51.87609039468568284 ) ) ;
#112511=CARTESIAN_POINT ( 'NONE',  ( -5.049401038297874678, -19.05341960407617918, 34.79275706135233293 ) ) ;
#112512=CARTESIAN_POINT ( 'NONE',  ( -16.53943276465976808, -0.05219959533934237506, 53.75109039468568994 ) ) ;
#112513=CARTESIAN_POINT ( 'NONE',  ( -4.379528057220086978, -16.55341960407618274, 94.79275706135234714 ) ) ;
#112514=CARTESIAN_POINT ( 'NONE',  ( -18.22780087662122028, 5.500000000000031086, 53.51540105326106556 ) ) ;
#112515=CARTESIAN_POINT ( 'NONE',  ( 0.05219959533934541429, -16.53943276465976808, 75.00109039468568994 ) ) ;
#112516=CARTESIAN_POINT ( 'NONE',  ( 0.05219959533934541429, -16.53943276465976808, 35.00109039468568284 ) ) ;
#112517=CARTESIAN_POINT ( 'NONE',  ( 19.02544592524343514, -5.153800228976328945, 43.54057627198103120 ) ) ;
#112518=CARTESIAN_POINT ( 'NONE',  ( -16.46253265017160317, 9.564922557960807481, 45.83224293864769550 ) ) ;
#112519=CARTESIAN_POINT ( 'NONE',  ( -16.46253265017160317, 9.564922557960807481, 65.83224293864769550 ) ) ;
#112520=CARTESIAN_POINT ( 'NONE',  ( 10.81492255796106328, -18.62759615963255655, 35.41775706135234003 ) ) ;
#112521=CARTESIAN_POINT ( 'NONE',  ( 8.224510206698742110, 14.34966873604972548, 52.08442372801901854 ) ) ;
#112522=CARTESIAN_POINT ( 'NONE',  ( 4.379528057220092307, 16.55341960407617563, 107.2927570613523471 ) ) ;
#112523=CARTESIAN_POINT ( 'NONE',  ( 9.564922557960805705, 16.46253265017160317, 29.58224293864769550 ) ) ;
#112524=CARTESIAN_POINT ( 'NONE',  ( -18.67979575497193778, 10.72451020669871902, 108.3344237280190185 ) ) ;
#112525=CARTESIAN_POINT ( 'NONE',  ( 9.564922557961047289, -16.46253265017146816, 105.4177570613523471 ) ) ;
#112526=CARTESIAN_POINT ( 'NONE',  ( -19.02544592524334988, -5.153800228976617603, 63.95942372801899012 ) ) ;
#112527=CARTESIAN_POINT ( 'NONE',  ( 16.53943276465976808, -0.05219959533910856209, 73.74890960531433848 ) ) ;
#112528=CARTESIAN_POINT ( 'NONE',  ( -5.153800228976328057, -19.02544592524343514, 42.29057627198101699 ) ) ;
#112529=CARTESIAN_POINT ( 'NONE',  ( -16.51473224551082808, 9.474510206698731452, 73.33442372801900433 ) ) ;
#112530=CARTESIAN_POINT ( 'NONE',  ( 16.79531203550648399, -7.028104445595605654, 91.24755011779559766 ) ) ;
#112531=CARTESIAN_POINT ( 'NONE',  ( 10.81492255796106328, -18.62759615963255655, 75.41775706135233293 ) ) ;
#112532=CARTESIAN_POINT ( 'NONE',  ( 16.52544592524335698, 4.483927247898782831, 36.45942372801901143 ) ) ;
#112533=CARTESIAN_POINT ( 'NONE',  ( 16.29526858892878494, 7.335722546919996034, 38.29670597800206622 ) ) ;
#112534=CARTESIAN_POINT ( 'NONE',  ( -10.81492255796078084, -18.62759615963271287, 32.08224293864769550 ) ) ;
#112535=CARTESIAN_POINT ( 'NONE',  ( 4.483927247898790824, -16.52544592524335698, 20.20942372801900788 ) ) ;
#112536=CARTESIAN_POINT ( 'NONE',  ( -0.05219959533909027116, -19.03943276465977164, 22.49890960531436690 ) ) ;
#112537=CARTESIAN_POINT ( 'NONE',  ( -13.89961937509957401, -13.97604488694547875, 29.37609039468565797 ) ) ;
#112539=CARTESIAN_POINT ( 'NONE',  ( 13.89961937509977652, -13.97604488694527269, 33.12390960531434558 ) ) ;
#112540=CARTESIAN_POINT ( 'NONE',  ( 5.049401038297881783, 19.05341960407617918, 57.29275706135232582 ) ) ;
#112541=CARTESIAN_POINT ( 'NONE',  ( 9.474510206698971260, -16.51473224551069308, 67.91557627198102409 ) ) ;
#112542=CARTESIAN_POINT ( 'NONE',  ( -19.20446147854528718, -5.499999999999912959, 54.38999695167677828 ) ) ;
#112543=CARTESIAN_POINT ( 'NONE',  ( -13.89961937509957401, -13.97604488694547875, 19.37609039468566507 ) ) ;
#112544=CARTESIAN_POINT ( 'NONE',  ( 16.53943276465976808, 0.05219959533934440121, 111.2510903946856899 ) ) ;
#112545=CARTESIAN_POINT ( 'NONE',  ( 19.02544592524343514, -5.153800228976328945, 33.54057627198102409 ) ) ;
#112546=CARTESIAN_POINT ( 'NONE',  ( -16.51473224551069308, -9.474510206698971260, 86.66557627198102409 ) ) ;
#112547=CARTESIAN_POINT ( 'NONE',  ( -0.05219959533937732626, 21.53943276465977519, 67.50109039468568994 ) ) ;
#112548=CARTESIAN_POINT ( 'NONE',  ( -13.97604488694527625, -13.89961937509977652, 46.87390960531435979 ) ) ;
#112549=CARTESIAN_POINT ( 'NONE',  ( 21.55341960407619695, -5.719274019375665929, 61.04275706135234714 ) ) ;
#112550=CARTESIAN_POINT ( 'NONE',  ( 9.474510206698729675, 16.51473224551082808, 92.08442372801900433 ) ) ;
#112551=CARTESIAN_POINT ( 'NONE',  ( 10.81492255796078972, 18.62759615963270932, 24.58224293864768839 ) ) ;
#112552=CARTESIAN_POINT ( 'NONE',  ( 16.51473224551069308, 9.474510206698969483, 39.16557627198103120 ) ) ;
#112553=CARTESIAN_POINT ( 'NONE',  ( -21.52544592524334988, -5.823673210054445271, 18.95942372801901143 ) ) ;
#112554=CARTESIAN_POINT ( 'NONE',  ( -0.05219959533936034679, 19.03943276465977164, 37.50109039468567573 ) ) ;
#112555=CARTESIAN_POINT ( 'NONE',  ( -14.34966873604960291, -8.224510206698953496, 111.6655762719810525 ) ) ;
#112556=CARTESIAN_POINT ( 'NONE',  ( 0.05219959533909260263, 19.03943276465977164, 64.99890960531436690 ) ) ;
#112557=CARTESIAN_POINT ( 'NONE',  ( -5.153800228976607833, 19.02544592524334988, 112.7094237280190043 ) ) ;
#112558=CARTESIAN_POINT ( 'NONE',  ( 12.06949235617757843, -12.14591786802309237, 73.12390960531436690 ) ) ;
#112559=CARTESIAN_POINT ( 'NONE',  ( 18.67979575497178502, 10.72451020669898547, 24.16557627198103120 ) ) ;
#112560=CARTESIAN_POINT ( 'NONE',  ( 9.564922557961047289, -16.46253265017146816, 85.41775706135233293 ) ) ;
#112561=CARTESIAN_POINT ( 'NONE',  ( -18.62759615963270932, 10.81492255796079327, 95.83224293864770971 ) ) ;
#112562=CARTESIAN_POINT ( 'NONE',  ( -21.55341960407619339, 5.719274019375674811, 63.54275706135234003 ) ) ;
#112563=CARTESIAN_POINT ( 'NONE',  ( 16.55341960407618274, -4.379528057220086978, 56.04275706135235424 ) ) ;
#112564=CARTESIAN_POINT ( 'NONE',  ( 4.379528057220092307, 16.55341960407617563, 52.29275706135236135 ) ) ;
#112565=CARTESIAN_POINT ( 'NONE',  ( -15.72974639402176322, -15.80617190586768395, 54.37609039468568994 ) ) ;
#112566=CARTESIAN_POINT ( 'NONE',  ( -21.53943276465977519, 0.05219959533907696930, 51.24890960531436690 ) ) ;
#112567=CARTESIAN_POINT ( 'NONE',  ( 16.46253265017160672, -9.564922557960803928, 53.33224293864768839 ) ) ;
#112569=CARTESIAN_POINT ( 'NONE',  ( 4.483927247898790824, -16.52544592524335698, 80.20942372801901854 ) ) ;
#112571=CARTESIAN_POINT ( 'NONE',  ( 5.719274019375991003, -21.55341960407610458, 102.7072429386476955 ) ) ;
#112572=CARTESIAN_POINT ( 'NONE',  ( 16.52544592524342804, -4.483927247898539470, 53.54057627198103120 ) ) ;
#112573=CARTESIAN_POINT ( 'NONE',  ( 12.06949235617739724, 12.14591786802326823, 61.87609039468568284 ) ) ;
#112574=CARTESIAN_POINT ( 'NONE',  ( -19.05341960407617563, 5.049401038297882671, 98.54275706135233293 ) ) ;
#112575=CARTESIAN_POINT ( 'NONE',  ( -0.05219959533907301413, -21.53943276465977519, 102.4989096053143811 ) ) ;
#112576=CARTESIAN_POINT ( 'NONE',  ( 4.483927247898545687, 16.52544592524342804, 44.79057627198103120 ) ) ;
#112578=CARTESIAN_POINT ( 'NONE',  ( -17.50000000000001421, 5.622605283950874444, 73.68792689403892382 ) ) ;
#112579=CARTESIAN_POINT ( 'NONE',  ( 15.80617190586746368, 15.72974639402197994, 74.37390960531436690 ) ) ;
#112580=CARTESIAN_POINT ( 'NONE',  ( -12.06949235617756955, 12.14591786802309770, 30.62390960531436335 ) ) ;
#112582=CARTESIAN_POINT ( 'NONE',  ( -16.31925111598459566, -7.325300261831489301, 54.83575461032751264 ) ) ;
#112583=CARTESIAN_POINT ( 'NONE',  ( -10.72451020669898014, 18.67979575497178502, 95.41557627198102409 ) ) ;
#112584=CARTESIAN_POINT ( 'NONE',  ( -18.62759615963255300, -10.81492255796106328, 24.16775706135235424 ) ) ;
#112585=CARTESIAN_POINT ( 'NONE',  ( -0.05219959533910754901, -16.53943276465976808, 42.49890960531435979 ) ) ;
#112586=CARTESIAN_POINT ( 'NONE',  ( 14.29746914071037800, 8.314922557961029526, 46.66775706135234714 ) ) ;
#112587=CARTESIAN_POINT ( 'NONE',  ( -5.153800228976328057, -19.02544592524343514, 52.29057627198100988 ) ) ;
#112588=CARTESIAN_POINT ( 'NONE',  ( -0.05219959533909027116, -19.03943276465977164, 77.49890960531435269 ) ) ;
#112590=ADVANCED_FACE ( 'NONE', ( #160756 ), #70753, .T. ) ;
#112591=CARTESIAN_POINT ( 'NONE',  ( -5.823673210054116645, -21.52544592524344225, 32.29057627198102409 ) ) ;
#112593=CARTESIAN_POINT ( 'NONE',  ( 12.14591786802327356, -12.06949235617739191, 25.62609039468567929 ) ) ;
#112594=CARTESIAN_POINT ( 'NONE',  ( -16.51473224551082808, 9.474510206698731452, 53.33442372801900433 ) ) ;
#112595=CARTESIAN_POINT ( 'NONE',  ( 21.55341960407610458, 5.719274019375980345, 103.9572429386476813 ) ) ;
#112596=CARTESIAN_POINT ( 'NONE',  ( 14.29746914071049879, -8.314922557960816363, 33.33224293864769550 ) ) ;
#112597=CARTESIAN_POINT ( 'NONE',  ( -19.02544592524342804, 5.153800228976336051, 81.04057627198103830 ) ) ;
#112598=CARTESIAN_POINT ( 'NONE',  ( 21.55341960407610458, 5.719274019375980345, 63.95724293864770260 ) ) ;
#112599=CARTESIAN_POINT ( 'NONE',  ( -10.72451020669898014, 18.67979575497178502, 75.41557627198102409 ) ) ;
#112600=CARTESIAN_POINT ( 'NONE',  ( -0.05219959533934338120, 16.53943276465976808, 27.50109039468567929 ) ) ;
#112601=CARTESIAN_POINT ( 'NONE',  ( -5.823673210054116645, -21.52544592524344225, 27.29057627198103120 ) ) ;
#112602=CARTESIAN_POINT ( 'NONE',  ( 21.53943276465977519, 0.05219959533937863772, 81.25109039468568994 ) ) ;
#112603=CARTESIAN_POINT ( 'NONE',  ( -19.02544592524342804, 5.153800228976336051, 71.04057627198099567 ) ) ;
#112604=ADVANCED_FACE ( 'NONE', ( #22247 ), #55598, .T. ) ;
#112605=CARTESIAN_POINT ( 'NONE',  ( 19.03943276465977164, -0.05219959533909143690, 23.74890960531435269 ) ) ;
#112606=CARTESIAN_POINT ( 'NONE',  ( -19.03943276465977164, 0.05219959533909376836, 81.24890960531436690 ) ) ;
#112607=CARTESIAN_POINT ( 'NONE',  ( 4.379528057220339221, -16.55341960407611168, 87.70724293864769550 ) ) ;
#112608=VERTEX_POINT ( 'NONE', #125925 ) ;
#112609=CARTESIAN_POINT ( 'NONE',  ( -13.89961937509957401, -13.97604488694547875, 99.37609039468567573 ) ) ;
#112611=CARTESIAN_POINT ( 'NONE',  ( -0.05219959533909027116, -19.03943276465977164, 67.49890960531436690 ) ) ;
#112612=CARTESIAN_POINT ( 'NONE',  ( -21.55341960407619339, 5.719274019375674811, 98.54275706135234714 ) ) ;
#112613=CARTESIAN_POINT ( 'NONE',  ( -21.53943276465977519, 0.05219959533907696930, 21.24890960531436690 ) ) ;
#112614=CARTESIAN_POINT ( 'NONE',  ( 8.224510206698742110, 14.34966873604972548, 77.08442372801901854 ) ) ;
#112615=CARTESIAN_POINT ( 'NONE',  ( -17.50000000000002842, -5.499999999999952927, 76.28230962303568674 ) ) ;
#112616=CARTESIAN_POINT ( 'NONE',  ( 19.05341960407617918, -5.049401038297876454, 56.04275706135234714 ) ) ;
#112617=CARTESIAN_POINT ( 'NONE',  ( 18.62759615963255655, 10.81492255796105972, 106.6677570613523756 ) ) ;
#112619=CARTESIAN_POINT ( 'NONE',  ( -16.51473224551069308, -9.474510206698971260, 31.66557627198102054 ) ) ;
#112620=CARTESIAN_POINT ( 'NONE',  ( 12.06949235617739724, 12.14591786802326823, 111.8760903946856615 ) ) ;
#112622=CARTESIAN_POINT ( 'NONE',  ( -4.379528057220086978, -16.55341960407618274, 104.7927570613523898 ) ) ;
#112623=CARTESIAN_POINT ( 'NONE',  ( -19.34837522270366250, -5.499999999999857003, 85.86337684832578532 ) ) ;
#112624=CARTESIAN_POINT ( 'NONE',  ( 14.29746914071037800, 8.314922557961029526, 86.66775706135234714 ) ) ;
#112625=CARTESIAN_POINT ( 'NONE',  ( 16.51473224551069308, 9.474510206698969483, 29.16557627198103475 ) ) ;
#112626=CARTESIAN_POINT ( 'NONE',  ( -15.80617190586768217, 15.72974639402176855, 88.12609039468570415 ) ) ;
#112627=CARTESIAN_POINT ( 'NONE',  ( -0.05219959533936034679, 19.03943276465977164, 107.5010903946856615 ) ) ;
#112628=CARTESIAN_POINT ( 'NONE',  ( -5.823673210054431948, 21.52544592524334988, 62.70942372801902565 ) ) ;
#112629=CARTESIAN_POINT ( 'NONE',  ( -0.05219959533936034679, 19.03943276465977164, 42.50109039468566152 ) ) ;
#112630=CARTESIAN_POINT ( 'NONE',  ( 9.474510206698971260, -16.51473224551069308, 77.91557627198103830 ) ) ;
#112631=CARTESIAN_POINT ( 'NONE',  ( -13.97604488694527625, -13.89961937509977652, 71.87390960531433848 ) ) ;
#112633=CARTESIAN_POINT ( 'NONE',  ( -21.55341960407610458, -5.719274019375992779, 46.45724293864769550 ) ) ;
#112634=CARTESIAN_POINT ( 'NONE',  ( 9.564922557960805705, 16.46253265017160317, 44.58224293864769550 ) ) ;
#112635=CARTESIAN_POINT ( 'NONE',  ( -12.14591786802326823, 12.06949235617739902, 78.12609039468570415 ) ) ;
#112638=CARTESIAN_POINT ( 'NONE',  ( -4.379528057220328563, 16.55341960407611168, 85.20724293864770971 ) ) ;
#112640=CARTESIAN_POINT ( 'NONE',  ( -4.379528057220086978, -16.55341960407618274, 34.79275706135235424 ) ) ;
#112641=CARTESIAN_POINT ( 'NONE',  ( 4.483927247898545687, 16.52544592524342804, 109.7905762719810383 ) ) ;
#112642=CARTESIAN_POINT ( 'NONE',  ( 16.46253265017146816, 9.564922557961045513, 61.66775706135234003 ) ) ;
#112643=CARTESIAN_POINT ( 'NONE',  ( -0.05219959533910754901, -16.53943276465976808, 77.49890960531433848 ) ) ;
#112644=CARTESIAN_POINT ( 'NONE',  ( -21.53943276465977519, -0.05219959533937600094, 28.75109039468567929 ) ) ;
#112645=CARTESIAN_POINT ( 'NONE',  ( -15.49999999999999822, -5.500000000000000888, 120.0000000000000142 ) ) ;
#112646=CARTESIAN_POINT ( 'NONE',  ( -21.52544592524343514, 5.823673210054127303, 91.04057627198103830 ) ) ;
#112647=CARTESIAN_POINT ( 'NONE',  ( 13.89961937509977652, -13.97604488694527269, 103.1239096053143527 ) ) ;
#112648=CARTESIAN_POINT ( 'NONE',  ( 16.53943276465976808, -0.05219959533910856209, 78.74890960531436690 ) ) ;
#112650=CARTESIAN_POINT ( 'NONE',  ( -16.46253265017160317, 9.564922557960807481, 50.83224293864770260 ) ) ;
#112653=CARTESIAN_POINT ( 'NONE',  ( 16.46253265017146816, 9.564922557961045513, 81.66775706135233293 ) ) ;
#112654=CARTESIAN_POINT ( 'NONE',  ( 10.72451020669871369, 18.67979575497193778, 22.08442372801901143 ) ) ;
#112655=CARTESIAN_POINT ( 'NONE',  ( -16.51473224551069308, -9.474510206698971260, 76.66557627198103830 ) ) ;
#112656=CARTESIAN_POINT ( 'NONE',  ( 0.05219959533936267826, -19.03943276465977164, 50.00109039468566863 ) ) ;
#112657=CARTESIAN_POINT ( 'NONE',  ( -16.46253265017160317, 9.564922557960807481, 50.83224293864770260 ) ) ;
#112658=CARTESIAN_POINT ( 'NONE',  ( -4.379528057220328563, 16.55341960407611168, 65.20724293864768129 ) ) ;
#112659=CARTESIAN_POINT ( 'NONE',  ( 8.314922557960818139, 14.29746914071049879, 49.58224293864769550 ) ) ;
#112660=CARTESIAN_POINT ( 'NONE',  ( 13.97604488694527802, 13.89961937509977652, 74.37390960531436690 ) ) ;
#112661=CARTESIAN_POINT ( 'NONE',  ( -10.81492255796078084, -18.62759615963271287, 82.08224293864768129 ) ) ;
#112662=CARTESIAN_POINT ( 'NONE',  ( -19.02544592524342804, 5.153800228976336051, 71.04057627198099567 ) ) ;
#112663=CARTESIAN_POINT ( 'NONE',  ( 18.62759615963271287, -10.81492255796078972, 73.33224293864769550 ) ) ;
#112664=CARTESIAN_POINT ( 'NONE',  ( -19.05341960407617563, 5.049401038297882671, 23.54275706135233648 ) ) ;
#112665=CARTESIAN_POINT ( 'NONE',  ( -0.05219959533909027116, -19.03943276465977164, 22.49890960531436690 ) ) ;
#112666=CARTESIAN_POINT ( 'NONE',  ( 16.52544592524342804, -4.483927247898539470, 23.54057627198102765 ) ) ;
#112667=CARTESIAN_POINT ( 'NONE',  ( -8.314922557960811034, -14.29746914071050412, 92.08224293864769550 ) ) ;
#112668=CARTESIAN_POINT ( 'NONE',  ( -13.89961937509957401, -13.97604488694547875, 109.3760903946856331 ) ) ;
#112670=CARTESIAN_POINT ( 'NONE',  ( -15.72974639402197994, 15.80617190586746368, 115.6239096053143669 ) ) ;
#112671=CARTESIAN_POINT ( 'NONE',  ( 5.049401038297881783, 19.05341960407617563, 52.29275706135234003 ) ) ;
#112672=CARTESIAN_POINT ( 'NONE',  ( -0.05219959533910754901, -16.53943276465976808, 27.49890960531435269 ) ) ;
#112673=CARTESIAN_POINT ( 'NONE',  ( -10.81492255796078084, -18.62759615963271287, 72.08224293864769550 ) ) ;
#112674=CARTESIAN_POINT ( 'NONE',  ( 5.049401038298161559, -19.05341960407611168, 97.70724293864766707 ) ) ;
#112675=CARTESIAN_POINT ( 'NONE',  ( -4.483927247898539470, -16.52544592524342804, 57.29057627198103120 ) ) ;
#112676=LINE ( 'NONE', #174368, #79929 ) ;
#112677=CARTESIAN_POINT ( 'NONE',  ( -9.564922557960796823, -16.46253265017161027, 37.08224293864768839 ) ) ;
#112678=CARTESIAN_POINT ( 'NONE',  ( -10.81492255796105439, 18.62759615963255655, 102.9177570613523756 ) ) ;
#112679=CARTESIAN_POINT ( 'NONE',  ( -12.14591786802326823, 12.06949235617739902, 93.12609039468568994 ) ) ;
#112680=CARTESIAN_POINT ( 'NONE',  ( 15.80617190586769283, -15.72974639402175789, 45.62609039468567573 ) ) ;
#112681=CARTESIAN_POINT ( 'NONE',  ( -16.52544592524335698, -4.483927247898792601, 43.95942372801902565 ) ) ;
#112682=CARTESIAN_POINT ( 'NONE',  ( -5.823673210054116645, -21.52544592524344225, 27.29057627198103120 ) ) ;
#112683=CARTESIAN_POINT ( 'NONE',  ( 19.05341960407611168, 5.049401038298154454, 58.95724293864768129 ) ) ;
#112684=CARTESIAN_POINT ( 'NONE',  ( -5.049401038298153566, 19.05341960407611168, 60.20724293864768129 ) ) ;
#112685=CARTESIAN_POINT ( 'NONE',  ( 16.52544592524335698, 4.483927247898782831, 51.45942372801901854 ) ) ;
#112686=CARTESIAN_POINT ( 'NONE',  ( -12.06949235617756955, 12.14591786802309770, 105.6239096053143669 ) ) ;
#112687=CARTESIAN_POINT ( 'NONE',  ( 8.224510206698953496, -14.34966873604960469, 27.91557627198103830 ) ) ;
#112688=CARTESIAN_POINT ( 'NONE',  ( 18.22780087662121673, 5.500000000000056843, 48.98459894673892023 ) ) ;
#112689=CARTESIAN_POINT ( 'NONE',  ( 5.719274019375673035, 21.55341960407619339, 62.29275706135236845 ) ) ;
#112690=CARTESIAN_POINT ( 'NONE',  ( 0.05219959533909260263, 19.03943276465977164, 89.99890960531436690 ) ) ;
#112691=CARTESIAN_POINT ( 'NONE',  ( -0.05219959533909027116, -19.03943276465977164, 77.49890960531435269 ) ) ;
#112692=CARTESIAN_POINT ( 'NONE',  ( -9.564922557960796823, -16.46253265017161027, 102.0822429386477097 ) ) ;
#112693=CARTESIAN_POINT ( 'NONE',  ( 16.55341960407611168, 4.379528057220329451, 48.95724293864770971 ) ) ;
#112695=CARTESIAN_POINT ( 'NONE',  ( -8.224510206698735004, -14.34966873604973081, 109.5844237280190328 ) ) ;
#112696=CARTESIAN_POINT ( 'NONE',  ( -8.314922557960811034, -14.29746914071050412, 37.08224293864768129 ) ) ;
#112698=CARTESIAN_POINT ( 'NONE',  ( -0.05219959533936034679, 19.03943276465977164, 37.50109039468567573 ) ) ;
#112699=CARTESIAN_POINT ( 'NONE',  ( -19.03943276465977164, 0.05219959533909376836, 71.24890960531435269 ) ) ;
#112700=CARTESIAN_POINT ( 'NONE',  ( -19.03943276465977164, -0.05219959533935918106, 53.75109039468566863 ) ) ;
#112702=CARTESIAN_POINT ( 'NONE',  ( 13.89961937509978007, -13.97604488694527269, 68.12390960531436690 ) ) ;
#112703=CARTESIAN_POINT ( 'NONE',  ( -19.03943276465977164, -0.05219959533935918106, 78.75109039468567573 ) ) ;
#112704=CARTESIAN_POINT ( 'NONE',  ( -14.29746914071037622, -8.314922557961029526, 64.16775706135234714 ) ) ;
#112705=CARTESIAN_POINT ( 'NONE',  ( 16.79531203550646268, 7.028104445595615424, 93.75244988220441655 ) ) ;
#112706=CARTESIAN_POINT ( 'NONE',  ( 9.564922557960805705, 16.46253265017160317, 109.5822429386476955 ) ) ;
#112707=CARTESIAN_POINT ( 'NONE',  ( 0.05219959533937995610, -21.53943276465977519, 25.00109039468567218 ) ) ;
#112708=CARTESIAN_POINT ( 'NONE',  ( 16.51473224551083163, -9.474510206698727899, 90.83442372801900433 ) ) ;
#112709=CARTESIAN_POINT ( 'NONE',  ( -19.03943276465977164, 0.05219959533909376836, 116.2489096053143669 ) ) ;
#112710=CARTESIAN_POINT ( 'NONE',  ( 13.89961937509977652, -13.97604488694527269, 43.12390960531434558 ) ) ;
#112711=CARTESIAN_POINT ( 'NONE',  ( -16.51473224551069308, -9.474510206698971260, 91.66557627198103830 ) ) ;
#112712=CARTESIAN_POINT ( 'NONE',  ( 12.06949235617757843, -12.14591786802309237, 43.12390960531435269 ) ) ;
#112713=CARTESIAN_POINT ( 'NONE',  ( -19.05341960407611168, -5.049401038298163336, 51.45724293864770260 ) ) ;
#112714=CARTESIAN_POINT ( 'NONE',  ( 9.474510206698729675, 16.51473224551082808, 62.08442372801899722 ) ) ;
#112715=CARTESIAN_POINT ( 'NONE',  ( 19.05341960407617918, -5.049401038297876454, 36.04275706135234003 ) ) ;
#112716=CARTESIAN_POINT ( 'NONE',  ( 19.02544592524343514, -5.153800228976328945, 68.54057627198103830 ) ) ;
#112717=CARTESIAN_POINT ( 'NONE',  ( 15.80617190586746368, 15.72974639402197994, 59.37390960531436690 ) ) ;
#112718=CARTESIAN_POINT ( 'NONE',  ( -8.224510206698948167, 14.34966873604960824, 65.41557627198102409 ) ) ;
#112719=CARTESIAN_POINT ( 'NONE',  ( 18.62759615963255655, 10.81492255796105972, 111.6677570613523613 ) ) ;
#112721=CARTESIAN_POINT ( 'NONE',  ( 5.719274019375991003, -21.55341960407610458, 32.70724293864770260 ) ) ;
#112722=CARTESIAN_POINT ( 'NONE',  ( -16.46253265017160317, 9.564922557960807481, 50.83224293864770260 ) ) ;
#112723=CARTESIAN_POINT ( 'NONE',  ( 16.51473224551069308, 9.474510206698969483, 34.16557627198102409 ) ) ;
#112724=CARTESIAN_POINT ( 'NONE',  ( -16.55341960407611168, -4.379528057220339221, 96.45724293864770971 ) ) ;
#112725=CARTESIAN_POINT ( 'NONE',  ( 15.72974639402199770, -15.80617190586745480, 113.1239096053143953 ) ) ;
#112727=CARTESIAN_POINT ( 'NONE',  ( -5.823673210054431948, 21.52544592524334988, 32.70942372801900433 ) ) ;
#112728=CARTESIAN_POINT ( 'NONE',  ( 19.02544592524343514, -5.153800228976328945, 98.54057627198100988 ) ) ;
#112729=CARTESIAN_POINT ( 'NONE',  ( -13.97604488694527625, -13.89961937509977652, 21.87390960531435979 ) ) ;
#112730=CARTESIAN_POINT ( 'NONE',  ( 5.719274019375673035, 21.55341960407619339, 77.29275706135234714 ) ) ;
#112731=CARTESIAN_POINT ( 'NONE',  ( 5.823673210054125526, 21.52544592524343514, 99.79057627198103830 ) ) ;
#112735=CARTESIAN_POINT ( 'NONE',  ( 12.14591786802327356, -12.06949235617739191, 50.62609039468568994 ) ) ;
#112736=CARTESIAN_POINT ( 'NONE',  ( -4.483927247898539470, -16.52544592524342804, 107.2905762719810525 ) ) ;
#112738=CARTESIAN_POINT ( 'NONE',  ( -16.51473224551069308, -9.474510206698971260, 56.66557627198103120 ) ) ;
#112739=CARTESIAN_POINT ( 'NONE',  ( -14.29746914071049879, 8.314922557960819915, 90.83224293864769550 ) ) ;
#112740=CARTESIAN_POINT ( 'NONE',  ( -21.52544592524343514, 5.823673210054127303, 51.04057627198103120 ) ) ;
#112741=CARTESIAN_POINT ( 'NONE',  ( 16.53943276465976808, -0.05219959533910856209, 68.74890960531435269 ) ) ;
#112742=CARTESIAN_POINT ( 'NONE',  ( 9.564922557961047289, -16.46253265017146816, 110.4177570613523471 ) ) ;
#112743=CARTESIAN_POINT ( 'NONE',  ( -10.72451020669870658, -18.67979575497194134, 89.58442372801901854 ) ) ;
#112744=CARTESIAN_POINT ( 'NONE',  ( 16.18388926212238488, -7.379444403734518154, 77.06046848633846480 ) ) ;
#112745=CARTESIAN_POINT ( 'NONE',  ( -16.53943276465976808, -0.05219959533934237506, 93.75109039468567573 ) ) ;
#112746=CARTESIAN_POINT ( 'NONE',  ( 14.34966873604960469, 8.224510206698951720, 39.16557627198102409 ) ) ;
#112747=CARTESIAN_POINT ( 'NONE',  ( 19.03943276465977164, -0.05219959533909143690, 43.74890960531435979 ) ) ;
#112748=CARTESIAN_POINT ( 'NONE',  ( -19.03943276465977164, 0.05219959533909376836, 91.24890960531436690 ) ) ;
#112749=CARTESIAN_POINT ( 'NONE',  ( 15.80617190586746368, 15.72974639402197994, 94.37390960531436690 ) ) ;
#112750=CARTESIAN_POINT ( 'NONE',  ( -16.52544592524335698, -4.483927247898792601, 43.95942372801902565 ) ) ;
#112751=CARTESIAN_POINT ( 'NONE',  ( -12.14591786802309592, -12.06949235617757132, 66.87390960531436690 ) ) ;
#112752=CARTESIAN_POINT ( 'NONE',  ( -18.62759615963255300, -10.81492255796106328, 89.16775706135236135 ) ) ;
#112754=CARTESIAN_POINT ( 'NONE',  ( -14.34966873604972548, 8.224510206698743886, 98.33442372801901854 ) ) ;
#112755=CARTESIAN_POINT ( 'NONE',  ( 17.50000000000000000, 5.499999999999997335, 26.70309617465829888 ) ) ;
#112757=CARTESIAN_POINT ( 'NONE',  ( 16.53943276465976808, -0.05219959533910856209, 28.74890960531435624 ) ) ;
#112758=CARTESIAN_POINT ( 'NONE',  ( -12.06949235617739369, -12.14591786802326823, 79.37609039468567573 ) ) ;
#112759=CARTESIAN_POINT ( 'NONE',  ( 16.51473224551069308, 9.474510206698969483, 79.16557627198103830 ) ) ;
#112760=CARTESIAN_POINT ( 'NONE',  ( -5.153800228976328057, -19.02544592524343514, 102.2905762719810383 ) ) ;
#112761=CARTESIAN_POINT ( 'NONE',  ( -0.05219959533937732626, 21.53943276465977519, 87.50109039468568994 ) ) ;
#112762=CARTESIAN_POINT ( 'NONE',  ( 14.34966873604972726, -8.224510206698740333, 95.83442372801903275 ) ) ;
#112763=CARTESIAN_POINT ( 'NONE',  ( -12.14591786802309592, -12.06949235617757132, 61.87390960531436690 ) ) ;
#112764=CARTESIAN_POINT ( 'NONE',  ( 16.51473224551069308, 9.474510206698969483, 64.16557627198102409 ) ) ;
#112766=CARTESIAN_POINT ( 'NONE',  ( -13.89961937509957401, -13.97604488694547875, 104.3760903946856757 ) ) ;
#112767=CARTESIAN_POINT ( 'NONE',  ( 16.51473224551069308, 9.474510206698969483, 24.16557627198102765 ) ) ;
#112768=CARTESIAN_POINT ( 'NONE',  ( -5.153800228976328057, -19.02544592524343514, 72.29057627198102409 ) ) ;
#112769=CARTESIAN_POINT ( 'NONE',  ( 13.97604488694548053, -13.89961937509957401, 110.6260903946856615 ) ) ;
#112771=CARTESIAN_POINT ( 'NONE',  ( 0.05219959533936267826, -19.03943276465977164, 20.00109039468567218 ) ) ;
#112772=CARTESIAN_POINT ( 'NONE',  ( 12.14591786802327356, -12.06949235617739191, 85.62609039468568994 ) ) ;
#112773=CARTESIAN_POINT ( 'NONE',  ( -13.97604488694547697, 13.89961937509957934, 108.1260903946856331 ) ) ;
#112774=CARTESIAN_POINT ( 'NONE',  ( 12.14591786802309770, 12.06949235617756955, 114.3739096053143527 ) ) ;
#112775=CARTESIAN_POINT ( 'NONE',  ( 12.06949235617739724, 12.14591786802326823, 66.87609039468568994 ) ) ;
#112776=CARTESIAN_POINT ( 'NONE',  ( -16.55341960407617563, 4.379528057220093196, 53.54275706135234714 ) ) ;
#112777=CARTESIAN_POINT ( 'NONE',  ( -13.89961937509977652, 13.97604488694528158, 25.62390960531434558 ) ) ;
#112778=CARTESIAN_POINT ( 'NONE',  ( 19.03943276465977164, 0.05219959533936151252, 66.25109039468567573 ) ) ;
#112779=CARTESIAN_POINT ( 'NONE',  ( 5.153800228976615827, -19.02544592524334988, 20.20942372801899722 ) ) ;
#112780=CARTESIAN_POINT ( 'NONE',  ( 0.05219959533909260263, 19.03943276465977164, 29.99890960531435979 ) ) ;
#112781=CARTESIAN_POINT ( 'NONE',  ( -9.474510206698964154, 16.51473224551069663, 75.41557627198103830 ) ) ;
#112782=CARTESIAN_POINT ( 'NONE',  ( -16.53943276465976808, 0.05219959533911058130, 76.24890960531435269 ) ) ;
#112784=CARTESIAN_POINT ( 'NONE',  ( 16.46253265017146816, 9.564922557961045513, 46.66775706135233293 ) ) ;
#112785=CARTESIAN_POINT ( 'NONE',  ( -0.05219959533907301413, -21.53943276465977519, 37.49890960531436690 ) ) ;
#112786=CARTESIAN_POINT ( 'NONE',  ( 19.05341960407617918, -5.049401038297876454, 21.04275706135232582 ) ) ;
#112787=CARTESIAN_POINT ( 'NONE',  ( -5.049401038298153566, 19.05341960407611168, 95.20724293864770971 ) ) ;
#112788=CARTESIAN_POINT ( 'NONE',  ( 21.52544592524334988, 5.823673210054432836, 101.4594237280190185 ) ) ;
#112789=CARTESIAN_POINT ( 'NONE',  ( -15.80617190586745835, -15.72974639402198527, 66.87390960531436690 ) ) ;
#112790=CARTESIAN_POINT ( 'NONE',  ( 9.474510206698971260, -16.51473224551069308, 92.91557627198103830 ) ) ;
#112791=CARTESIAN_POINT ( 'NONE',  ( -9.474510206698720793, -16.51473224551083518, 94.58442372801900433 ) ) ;
#112792=CARTESIAN_POINT ( 'NONE',  ( -9.474510206698964154, 16.51473224551069663, 100.4155762719810241 ) ) ;
#112793=CARTESIAN_POINT ( 'NONE',  ( 5.153800228976615827, -19.02544592524334988, 100.2094237280190043 ) ) ;
#112794=CARTESIAN_POINT ( 'NONE',  ( -16.55341960407611168, -4.379528057220339221, 111.4572429386476813 ) ) ;
#112795=CARTESIAN_POINT ( 'NONE',  ( -5.153800228976328057, -19.02544592524343514, 87.29057627198103830 ) ) ;
#112796=CARTESIAN_POINT ( 'NONE',  ( 10.81492255796078972, 18.62759615963270932, 64.58224293864769550 ) ) ;
#112798=CARTESIAN_POINT ( 'NONE',  ( -14.34966873604972548, 8.224510206698743886, 38.33442372801900433 ) ) ;
#112799=CARTESIAN_POINT ( 'NONE',  ( -10.81492255796105439, 18.62759615963255655, 42.91775706135235424 ) ) ;
#112800=CARTESIAN_POINT ( 'NONE',  ( -0.05219959533937732626, 21.53943276465977519, 97.50109039468567573 ) ) ;
#112801=CARTESIAN_POINT ( 'NONE',  ( 8.224510206698742110, 14.34966873604972548, 97.08442372801904696 ) ) ;
#112802=CARTESIAN_POINT ( 'NONE',  ( 19.05341960407611168, 5.049401038298154454, 83.95724293864766707 ) ) ;
#112803=CARTESIAN_POINT ( 'NONE',  ( -12.06949235617756955, 12.14591786802309770, 85.62390960531436690 ) ) ;
#112804=CARTESIAN_POINT ( 'NONE',  ( 14.29746914071049879, -8.314922557960816363, 23.33224293864769194 ) ) ;
#112805=CARTESIAN_POINT ( 'NONE',  ( 19.03943276465977164, 0.05219959533936151252, 71.25109039468566152 ) ) ;
#112806=CARTESIAN_POINT ( 'NONE',  ( -21.53943276465977519, -0.05219959533937600094, 48.75109039468568284 ) ) ;
#112807=CARTESIAN_POINT ( 'NONE',  ( -14.29746914071049879, 8.314922557960819915, 90.83224293864769550 ) ) ;
#112808=CARTESIAN_POINT ( 'NONE',  ( 21.53943276465977519, -0.05219959533907433946, 23.74890960531435269 ) ) ;
#112809=CARTESIAN_POINT ( 'NONE',  ( 0.05219959533910956823, 16.53943276465976808, 24.99890960531435624 ) ) ;
#112810=CARTESIAN_POINT ( 'NONE',  ( -15.80617190586768217, 15.72974639402176855, 83.12609039468568994 ) ) ;
#112811=CARTESIAN_POINT ( 'NONE',  ( -16.52544592524335698, -4.483927247898792601, 48.95942372801902565 ) ) ;
#112812=CARTESIAN_POINT ( 'NONE',  ( -21.55341960407619339, 5.719274019375674811, 38.54275706135234714 ) ) ;
#112814=CARTESIAN_POINT ( 'NONE',  ( -5.719274019375978568, 21.55341960407610458, 115.2072429386476955 ) ) ;
#112815=CARTESIAN_POINT ( 'NONE',  ( -14.29746914071049879, 8.314922557960819915, 90.83224293864769550 ) ) ;
#112816=CARTESIAN_POINT ( 'NONE',  ( -19.20446147854529428, -5.499999999999913847, 49.38999695167678539 ) ) ;
#112817=CARTESIAN_POINT ( 'NONE',  ( -16.55341960407611168, -4.379528057220339221, 61.45724293864770260 ) ) ;
#112818=CARTESIAN_POINT ( 'NONE',  ( 9.474510206698971260, -16.51473224551069308, 62.91557627198102409 ) ) ;
#112819=CARTESIAN_POINT ( 'NONE',  ( -12.14591786802326823, 12.06949235617739902, 103.1260903946856757 ) ) ;
#112820=CARTESIAN_POINT ( 'NONE',  ( 9.474510206698971260, -16.51473224551069308, 37.91557627198102409 ) ) ;
#112821=CARTESIAN_POINT ( 'NONE',  ( 15.72974639402199770, -15.80617190586745480, 48.12390960531436690 ) ) ;
#112822=CARTESIAN_POINT ( 'NONE',  ( 12.14591786802309770, 12.06949235617756955, 84.37390960531438111 ) ) ;
#112824=CARTESIAN_POINT ( 'NONE',  ( -21.53943276465977519, 0.05219959533907696930, 81.24890960531436690 ) ) ;
#112825=CARTESIAN_POINT ( 'NONE',  ( 9.474510206698971260, -16.51473224551069308, 82.91557627198103830 ) ) ;
#112826=CARTESIAN_POINT ( 'NONE',  ( -16.51473224551069308, -9.474510206698971260, 36.66557627198102409 ) ) ;
#112827=CARTESIAN_POINT ( 'NONE',  ( -0.05219959533936034679, 19.03943276465977164, 87.50109039468567573 ) ) ;
#112828=CARTESIAN_POINT ( 'NONE',  ( 5.823673210054125526, 21.52544592524343514, 39.79057627198103830 ) ) ;
#112829=CARTESIAN_POINT ( 'NONE',  ( -15.72974639402176322, -15.80617190586768395, 69.37609039468567573 ) ) ;
#112830=CARTESIAN_POINT ( 'NONE',  ( 19.03943276465977164, -0.05219959533909143690, 53.74890960531436690 ) ) ;
#112831=CARTESIAN_POINT ( 'NONE',  ( -13.97604488694527625, -13.89961937509977652, 81.87390960531436690 ) ) ;
#112833=CARTESIAN_POINT ( 'NONE',  ( 8.224510206698742110, 14.34966873604972548, 67.08442372801901854 ) ) ;
#112834=CARTESIAN_POINT ( 'NONE',  ( 18.62759615963255655, 10.81492255796105972, 46.66775706135234714 ) ) ;
#112835=CARTESIAN_POINT ( 'NONE',  ( 10.72451020669871369, 18.67979575497193778, 67.08442372801901854 ) ) ;
#112836=CARTESIAN_POINT ( 'NONE',  ( 21.53943276465977519, -0.05219959533907433946, 28.74890960531435624 ) ) ;
#112837=CARTESIAN_POINT ( 'NONE',  ( 5.719274019375991003, -21.55341960407610458, 97.70724293864772392 ) ) ;
#112838=CARTESIAN_POINT ( 'NONE',  ( 21.55341960407619695, -5.719274019375665929, 41.04275706135236135 ) ) ;
#112839=CARTESIAN_POINT ( 'NONE',  ( 14.29746914071037800, 8.314922557961029526, 61.66775706135235424 ) ) ;
#112840=CARTESIAN_POINT ( 'NONE',  ( -0.05219959533907301413, -21.53943276465977519, 57.49890960531435979 ) ) ;
#112841=CARTESIAN_POINT ( 'NONE',  ( -0.05219959533936034679, 19.03943276465977164, 27.50109039468566507 ) ) ;
#112842=CARTESIAN_POINT ( 'NONE',  ( 13.97604488694527802, 13.89961937509977652, 64.37390960531436690 ) ) ;
#112843=CARTESIAN_POINT ( 'NONE',  ( -14.34966873604972548, 8.224510206698743886, 98.33442372801901854 ) ) ;
#112844=CARTESIAN_POINT ( 'NONE',  ( -17.50000000000001776, -4.658240926743213883, 106.0552958218320185 ) ) ;
#112846=CARTESIAN_POINT ( 'NONE',  ( 19.05341960407611168, 5.049401038298154454, 98.95724293864766707 ) ) ;
#112848=CARTESIAN_POINT ( 'NONE',  ( 9.564922557961047289, -16.46253265017146816, 75.41775706135234714 ) ) ;
#112849=CARTESIAN_POINT ( 'NONE',  ( 10.81492255796078972, 18.62759615963270932, 59.58224293864770260 ) ) ;
#112850=CARTESIAN_POINT ( 'NONE',  ( -4.483927247898539470, -16.52544592524342804, 32.29057627198102409 ) ) ;
#112851=CARTESIAN_POINT ( 'NONE',  ( 13.97604488694548053, -13.89961937509957401, 105.6260903946856757 ) ) ;
#112852=CARTESIAN_POINT ( 'NONE',  ( 5.153800228976335163, 19.02544592524342804, 24.79057627198102765 ) ) ;
#112853=CARTESIAN_POINT ( 'NONE',  ( 5.049401038297881783, 19.05341960407617563, 102.2927570613523045 ) ) ;
#112854=CARTESIAN_POINT ( 'NONE',  ( 10.72451020669898902, -18.67979575497178502, 82.91557627198103830 ) ) ;
#112855=CARTESIAN_POINT ( 'NONE',  ( 19.02544592524334988, 5.153800228976608722, 56.45942372801898301 ) ) ;
#112857=CARTESIAN_POINT ( 'NONE',  ( 5.153800228976335163, 19.02544592524342804, 69.79057627198103830 ) ) ;
#112858=CARTESIAN_POINT ( 'NONE',  ( -14.29746914071049879, 8.314922557960819915, 60.83224293864769550 ) ) ;
#112859=CARTESIAN_POINT ( 'NONE',  ( 9.474510206698971260, -16.51473224551069308, 42.91557627198103120 ) ) ;
#112860=CARTESIAN_POINT ( 'NONE',  ( 4.379528057220339221, -16.55341960407611168, 47.70724293864770260 ) ) ;
#112861=CARTESIAN_POINT ( 'NONE',  ( -5.153800228976328057, -19.02544592524343514, 22.29057627198102765 ) ) ;
#112863=CARTESIAN_POINT ( 'NONE',  ( 0.05219959533910956823, 16.53943276465976808, 34.99890960531435979 ) ) ;
#112864=CARTESIAN_POINT ( 'NONE',  ( 0.05219959533909260263, 19.03943276465977164, 69.99890960531435269 ) ) ;
#112866=CARTESIAN_POINT ( 'NONE',  ( -19.02544592524334988, -5.153800228976617603, 33.95942372801897591 ) ) ;
#112867=CARTESIAN_POINT ( 'NONE',  ( -14.34966873604972548, 8.224510206698743886, 43.33442372801901143 ) ) ;
#112868=CARTESIAN_POINT ( 'NONE',  ( -18.62759615963270932, 10.81492255796079327, 45.83224293864769550 ) ) ;
#112869=CARTESIAN_POINT ( 'NONE',  ( -21.53943276465977519, -0.05219959533937600094, 108.7510903946857042 ) ) ;
#112870=CARTESIAN_POINT ( 'NONE',  ( 19.05341960407611168, 5.049401038298154454, 78.95724293864769550 ) ) ;
#112872=CARTESIAN_POINT ( 'NONE',  ( -13.89961937509977652, 13.97604488694528158, 110.6239096053143243 ) ) ;
#112873=CARTESIAN_POINT ( 'NONE',  ( -15.80617190586768217, 15.72974639402176855, 38.12609039468567573 ) ) ;
#112874=CARTESIAN_POINT ( 'NONE',  ( 16.53943276465976808, -0.05219959533910856209, 93.74890960531436690 ) ) ;
#112875=CARTESIAN_POINT ( 'NONE',  ( 21.55341960407610458, 5.719274019375980345, 93.95724293864770971 ) ) ;
#112876=CARTESIAN_POINT ( 'NONE',  ( 13.89961937509977652, -13.97604488694527269, 78.12390960531433848 ) ) ;
#112878=CARTESIAN_POINT ( 'NONE',  ( -9.474510206698964154, 16.51473224551069663, 85.41557627198102409 ) ) ;
#112879=CARTESIAN_POINT ( 'NONE',  ( -21.53943276465977519, -0.05219959533937600094, 28.75109039468567929 ) ) ;
#112880=ORIENTED_EDGE ( 'NONE', *, *, #176690, .T. ) ;
#112881=CARTESIAN_POINT ( 'NONE',  ( 0.05219959533909260263, 19.03943276465977164, 89.99890960531436690 ) ) ;
#112882=CARTESIAN_POINT ( 'NONE',  ( 19.01533133064923931, -5.499999999999436007, 81.26586590595741200 ) ) ;
#112883=CARTESIAN_POINT ( 'NONE',  ( 16.46253265017160672, -9.564922557960803928, 28.33224293864769550 ) ) ;
#112884=CARTESIAN_POINT ( 'NONE',  ( -5.153800228976328057, -19.02544592524343514, 37.29057627198102409 ) ) ;
#112885=CARTESIAN_POINT ( 'NONE',  ( 19.03943276465977164, 0.05219959533936151252, 111.2510903946856757 ) ) ;
#112887=CARTESIAN_POINT ( 'NONE',  ( -14.29746914071049879, 8.314922557960819915, 115.8322429386477097 ) ) ;
#112888=CARTESIAN_POINT ( 'NONE',  ( 21.55341960407619695, -5.719274019375665929, 81.04275706135236135 ) ) ;
#112889=CARTESIAN_POINT ( 'NONE',  ( -5.049401038298153566, 19.05341960407611168, 60.20724293864768129 ) ) ;
#112890=CARTESIAN_POINT ( 'NONE',  ( 15.72974639402176855, 15.80617190586768217, 26.87609039468567218 ) ) ;
#112891=CARTESIAN_POINT ( 'NONE',  ( -18.62759615963270932, 10.81492255796079327, 105.8322429386476955 ) ) ;
#112893=CARTESIAN_POINT ( 'NONE',  ( -9.564922557960796823, -16.46253265017161027, 87.08224293864769550 ) ) ;
#112894=DIRECTION ( 'NONE',  ( -0.000000000000000000, -0.000000000000000000, 1.000000000000000000 ) ) ;
#112895=CARTESIAN_POINT ( 'NONE',  ( 8.314922557961029526, -14.29746914071037800, 20.41775706135234714 ) ) ;
#112896=CARTESIAN_POINT ( 'NONE',  ( 21.55341960407610458, 5.719274019375980345, 48.95724293864770971 ) ) ;
#112897=CARTESIAN_POINT ( 'NONE',  ( 10.81492255796106328, -18.62759615963255655, 60.41775706135235424 ) ) ;
#112898=CARTESIAN_POINT ( 'NONE',  ( -13.97604488694527625, -13.89961937509977652, 106.8739096053143669 ) ) ;
#112899=CARTESIAN_POINT ( 'NONE',  ( 13.89961937509957401, 13.97604488694547697, 91.87609039468567573 ) ) ;
#112900=CARTESIAN_POINT ( 'NONE',  ( 9.474510206698971260, -16.51473224551069308, 57.91557627198103120 ) ) ;
#112901=CARTESIAN_POINT ( 'NONE',  ( -16.51473224551069308, -9.474510206698971260, 86.66557627198102409 ) ) ;
#112902=CARTESIAN_POINT ( 'NONE',  ( 0.05219959533910956823, 16.53943276465976808, 94.99890960531436690 ) ) ;
#112903=CARTESIAN_POINT ( 'NONE',  ( 12.06949235617757843, -12.14591786802309237, 88.12390960531436690 ) ) ;
#112904=CARTESIAN_POINT ( 'NONE',  ( 19.05341960407611168, 5.049401038298154454, 108.9572429386477097 ) ) ;
#112905=CARTESIAN_POINT ( 'NONE',  ( -8.224510206698948167, 14.34966873604960824, 50.41557627198103120 ) ) ;
#112906=CARTESIAN_POINT ( 'NONE',  ( 16.46253265017160672, -9.564922557960803928, 43.33224293864769550 ) ) ;
#112907=CARTESIAN_POINT ( 'NONE',  ( -15.72974639402176322, -15.80617190586768395, 74.37609039468568994 ) ) ;
#112908=CARTESIAN_POINT ( 'NONE',  ( 16.46253265017146816, 9.564922557961045513, 96.66775706135233293 ) ) ;
#112909=CARTESIAN_POINT ( 'NONE',  ( -14.34966873604960291, -8.224510206698953496, 56.66557627198103830 ) ) ;
#112910=CARTESIAN_POINT ( 'NONE',  ( 10.81492255796078972, 18.62759615963270932, 114.5822429386477097 ) ) ;
#112911=CARTESIAN_POINT ( 'NONE',  ( 21.53943276465977519, -0.05219959533907433946, 48.74890960531435979 ) ) ;
#112912=CARTESIAN_POINT ( 'NONE',  ( 19.39720447994795549, 5.499999999999970690, 72.16317477297177163 ) ) ;
#112914=CARTESIAN_POINT ( 'NONE',  ( -9.564922557960796823, -16.46253265017161027, 62.08224293864769550 ) ) ;
#112915=CARTESIAN_POINT ( 'NONE',  ( 16.55341960407611168, 4.379528057220329451, 38.95724293864768839 ) ) ;
#112916=CARTESIAN_POINT ( 'NONE',  ( 16.53943276465976808, 0.05219959533934440121, 101.2510903946856757 ) ) ;
#112917=CARTESIAN_POINT ( 'NONE',  ( 14.34966873604972726, -8.224510206698740333, 80.83442372801901854 ) ) ;
#112918=CARTESIAN_POINT ( 'NONE',  ( 5.049401038297881783, 19.05341960407617563, 37.29275706135232582 ) ) ;
#112920=CARTESIAN_POINT ( 'NONE',  ( 0.05219959533909260263, 19.03943276465977164, 94.99890960531436690 ) ) ;
#112921=CARTESIAN_POINT ( 'NONE',  ( -16.51473224551069308, -9.474510206698971260, 46.66557627198102409 ) ) ;
#112922=CARTESIAN_POINT ( 'NONE',  ( 16.55341960407611168, 4.379528057220329451, 63.95724293864770260 ) ) ;
#112923=CARTESIAN_POINT ( 'NONE',  ( 17.50000000000000000, -5.499999999999992895, 101.2176903769643559 ) ) ;
#112924=CARTESIAN_POINT ( 'NONE',  ( 21.55341960407610458, 5.719274019375980345, 28.95724293864769905 ) ) ;
#112925=CARTESIAN_POINT ( 'NONE',  ( -10.72451020669898014, 18.67979575497178502, 35.41557627198102409 ) ) ;
#112926=CARTESIAN_POINT ( 'NONE',  ( -4.379528057220328563, 16.55341960407611168, 80.20724293864769550 ) ) ;
#112927=CARTESIAN_POINT ( 'NONE',  ( 16.55341960407618274, -4.379528057220086978, 36.04275706135234714 ) ) ;
#112928=EDGE_CURVE ( 'NONE', #101016, #88472, #1402, .T. ) ;
#112929=CARTESIAN_POINT ( 'NONE',  ( -8.314922557960811034, -14.29746914071050412, 82.08224293864768129 ) ) ;
#112931=CARTESIAN_POINT ( 'NONE',  ( 0.05219959533936267826, -19.03943276465977164, 80.00109039468567573 ) ) ;
#112932=CARTESIAN_POINT ( 'NONE',  ( -5.823673210054116645, -21.52544592524344225, 22.29057627198102765 ) ) ;
#112936=CARTESIAN_POINT ( 'NONE',  ( -16.52544592524335698, -4.483927247898792601, 23.95942372801901143 ) ) ;
#112937=CARTESIAN_POINT ( 'NONE',  ( -8.314922557960811034, -14.29746914071050412, 22.08224293864769194 ) ) ;
#112938=CARTESIAN_POINT ( 'NONE',  ( 9.564922557961047289, -16.46253265017146816, 65.41775706135233293 ) ) ;
#112939=CARTESIAN_POINT ( 'NONE',  ( 18.62759615963271287, -10.81492255796078972, 48.33224293864770260 ) ) ;
#112940=CARTESIAN_POINT ( 'NONE',  ( 15.72974639402176855, 15.80617190586768217, 61.87609039468568284 ) ) ;
#112942=CARTESIAN_POINT ( 'NONE',  ( -12.06949235617739369, -12.14591786802326823, 29.37609039468568284 ) ) ;
#112943=CARTESIAN_POINT ( 'NONE',  ( 5.049401038298161559, -19.05341960407611168, 22.70724293864769194 ) ) ;
#112944=CARTESIAN_POINT ( 'NONE',  ( 16.46253265017160672, -9.564922557960803928, 93.33224293864769550 ) ) ;
#112945=CARTESIAN_POINT ( 'NONE',  ( 19.02544592524343514, -5.153800228976328945, 28.54057627198102409 ) ) ;
#112946=CARTESIAN_POINT ( 'NONE',  ( 12.06949235617757843, -12.14591786802309237, 88.12390960531436690 ) ) ;
#112948=CARTESIAN_POINT ( 'NONE',  ( -16.51473224551069308, -9.474510206698971260, 96.66557627198102409 ) ) ;
#112950=CARTESIAN_POINT ( 'NONE',  ( 13.97604488694548053, -13.89961937509957401, 100.6260903946856615 ) ) ;
#112951=CARTESIAN_POINT ( 'NONE',  ( 5.719274019375991003, -21.55341960407610458, 72.70724293864769550 ) ) ;
#112952=CARTESIAN_POINT ( 'NONE',  ( 0.05219959533909260263, 19.03943276465977164, 44.99890960531435979 ) ) ;
#112953=CARTESIAN_POINT ( 'NONE',  ( -0.05219959533936034679, 19.03943276465977164, 67.50109039468566152 ) ) ;
#112954=CARTESIAN_POINT ( 'NONE',  ( 10.81492255796078972, 18.62759615963270932, 114.5822429386477097 ) ) ;
#112955=CARTESIAN_POINT ( 'NONE',  ( -19.05341960407611168, -5.049401038298163336, 71.45724293864766707 ) ) ;
#112956=CARTESIAN_POINT ( 'NONE',  ( 5.153800228976335163, 19.02544592524342804, 104.7905762719809957 ) ) ;
#112957=ORIENTED_EDGE ( 'NONE', *, *, #83145, .F. ) ;
#112958=CARTESIAN_POINT ( 'NONE',  ( -8.224510206698735004, -14.34966873604973081, 34.58442372801900433 ) ) ;
#112959=CARTESIAN_POINT ( 'NONE',  ( -0.05219959533907301413, -21.53943276465977519, 97.49890960531436690 ) ) ;
#112960=CARTESIAN_POINT ( 'NONE',  ( -16.55341960407611168, -4.379528057220339221, 111.4572429386476813 ) ) ;
#112961=CARTESIAN_POINT ( 'NONE',  ( 5.153800228976335163, 19.02544592524342804, 89.79057627198102409 ) ) ;
#112962=CARTESIAN_POINT ( 'NONE',  ( 13.89961937509957401, 13.97604488694547697, 56.87609039468564731 ) ) ;
#112963=CARTESIAN_POINT ( 'NONE',  ( 5.823673210054125526, 21.52544592524343514, 89.79057627198103830 ) ) ;
#112964=CARTESIAN_POINT ( 'NONE',  ( -12.14591786802309592, -12.06949235617757132, 51.87390960531437401 ) ) ;
#112965=CARTESIAN_POINT ( 'NONE',  ( -19.03943276465977164, -0.05219959533935918106, 23.75109039468566152 ) ) ;
#112966=CARTESIAN_POINT ( 'NONE',  ( 4.483927247898790824, -16.52544592524335698, 60.20942372801902565 ) ) ;
#112967=CARTESIAN_POINT ( 'NONE',  ( -19.03943276465977164, 0.05219959533909376836, 96.24890960531436690 ) ) ;
#112968=CARTESIAN_POINT ( 'NONE',  ( 13.89961937509977652, -13.97604488694527269, 43.12390960531434558 ) ) ;
#112970=CARTESIAN_POINT ( 'NONE',  ( -5.719274019375665041, -21.55341960407619695, 49.79275706135234714 ) ) ;
#112971=CARTESIAN_POINT ( 'NONE',  ( -21.55341960407619339, 5.719274019375674811, 68.54275706135234714 ) ) ;
#112972=CARTESIAN_POINT ( 'NONE',  ( 9.474510206698971260, -16.51473224551069308, 57.91557627198103120 ) ) ;
#112973=CARTESIAN_POINT ( 'NONE',  ( -21.52544592524334988, -5.823673210054445271, 33.95942372801901143 ) ) ;
#112974=CARTESIAN_POINT ( 'NONE',  ( -16.51473224551082808, 9.474510206698731452, 78.33442372801900433 ) ) ;
#112975=CARTESIAN_POINT ( 'NONE',  ( -9.474510206698964154, 16.51473224551069663, 40.41557627198103120 ) ) ;
#112976=CARTESIAN_POINT ( 'NONE',  ( -0.05219959533934338120, 16.53943276465976808, 87.50109039468568994 ) ) ;
#112977=CARTESIAN_POINT ( 'NONE',  ( 19.05341960407611168, 5.049401038298154454, 58.95724293864768129 ) ) ;
#112978=CARTESIAN_POINT ( 'NONE',  ( -0.05219959533909027116, -19.03943276465977164, 22.49890960531436690 ) ) ;
#112980=CARTESIAN_POINT ( 'NONE',  ( -19.02544592524342804, 5.153800228976336051, 36.04057627198100988 ) ) ;
#112981=CARTESIAN_POINT ( 'NONE',  ( -15.80617190586745835, -15.72974639402198527, 86.87390960531438111 ) ) ;
#112982=CARTESIAN_POINT ( 'NONE',  ( 0.05219959533934541429, -16.53943276465976808, 80.00109039468568994 ) ) ;
#112983=CARTESIAN_POINT ( 'NONE',  ( 30.00000000000000000, 5.499999999999992895, 37.50000000000000000 ) ) ;
#112984=CARTESIAN_POINT ( 'NONE',  ( 13.89961937509957401, 13.97604488694547697, 26.87609039468566507 ) ) ;
#112985=CARTESIAN_POINT ( 'NONE',  ( -5.153800228976328057, -19.02544592524343514, 52.29057627198100988 ) ) ;
#112986=CARTESIAN_POINT ( 'NONE',  ( -8.314922557960811034, -14.29746914071050412, 47.08224293864770260 ) ) ;
#112987=CARTESIAN_POINT ( 'NONE',  ( -8.224510206698948167, 14.34966873604960824, 75.41557627198102409 ) ) ;
#112988=CARTESIAN_POINT ( 'NONE',  ( -16.46253265017160317, 9.564922557960807481, 100.8322429386477097 ) ) ;
#112989=CARTESIAN_POINT ( 'NONE',  ( -13.97604488694527625, -13.89961937509977652, 81.87390960531436690 ) ) ;
#112990=CARTESIAN_POINT ( 'NONE',  ( 18.67979575497194134, -10.72451020669871369, 50.83442372801901143 ) ) ;
#112991=CARTESIAN_POINT ( 'NONE',  ( 16.46253265017160672, -9.564922557960803928, 93.33224293864769550 ) ) ;
#112992=CARTESIAN_POINT ( 'NONE',  ( -10.72451020669870658, -18.67979575497194134, 94.58442372801901854 ) ) ;
#112993=CARTESIAN_POINT ( 'NONE',  ( 0.05219959533934541429, -16.53943276465976808, 80.00109039468568994 ) ) ;
#112994=CARTESIAN_POINT ( 'NONE',  ( -5.719274019375665041, -21.55341960407619695, 29.79275706135234358 ) ) ;
#112995=CARTESIAN_POINT ( 'NONE',  ( -21.52544592524343514, 5.823673210054127303, 101.0405762719810383 ) ) ;
#112996=CARTESIAN_POINT ( 'NONE',  ( -16.55341960407611168, -4.379528057220339221, 46.45724293864769550 ) ) ;
#112997=CARTESIAN_POINT ( 'NONE',  ( -19.03943276465977164, 0.05219959533909376836, 36.24890960531436690 ) ) ;
#112998=CARTESIAN_POINT ( 'NONE',  ( -4.483927247898539470, -16.52544592524342804, 67.29057627198103830 ) ) ;
#112999=CARTESIAN_POINT ( 'NONE',  ( 5.719274019375991003, -21.55341960407610458, 27.70724293864769905 ) ) ;
#113000=CARTESIAN_POINT ( 'NONE',  ( -16.46253265017146816, -9.564922557961047289, 24.16775706135233648 ) ) ;
#113001=CARTESIAN_POINT ( 'NONE',  ( -8.224510206698948167, 14.34966873604960824, 105.4155762719810383 ) ) ;
#113002=VERTEX_POINT ( 'NONE', #143065 ) ;
#113003=CARTESIAN_POINT ( 'NONE',  ( 12.06949235617739724, 12.14591786802326823, 71.87609039468568994 ) ) ;
#113004=CARTESIAN_POINT ( 'NONE',  ( 9.564922557960805705, 16.46253265017160317, 74.58224293864769550 ) ) ;
#113005=CARTESIAN_POINT ( 'NONE',  ( -16.88471381081837208, -5.722258574975401579, 20.56778223399915007 ) ) ;
#113006=CARTESIAN_POINT ( 'NONE',  ( 4.379528057220339221, -16.55341960407611168, 92.70724293864770971 ) ) ;
#113007=CARTESIAN_POINT ( 'NONE',  ( 5.719274019375991003, -21.55341960407610458, 42.70724293864770260 ) ) ;
#113008=CARTESIAN_POINT ( 'NONE',  ( -16.52544592524335698, -4.483927247898792601, 88.95942372801901854 ) ) ;
#113009=CARTESIAN_POINT ( 'NONE',  ( 19.05341960407617918, -5.049401038297876454, 111.0427570613523329 ) ) ;
#113010=CARTESIAN_POINT ( 'NONE',  ( 10.81492255796106328, -18.62759615963255655, 80.41775706135234714 ) ) ;
#113011=CARTESIAN_POINT ( 'NONE',  ( 19.02544592524343514, -5.153800228976328945, 68.54057627198103830 ) ) ;
#113012=CARTESIAN_POINT ( 'NONE',  ( -0.05219959533907301413, -21.53943276465977519, 107.4989096053143669 ) ) ;
#113013=CARTESIAN_POINT ( 'NONE',  ( -16.53943276465976808, -0.05219959533934237506, 53.75109039468568994 ) ) ;
#113014=CARTESIAN_POINT ( 'NONE',  ( -14.29746914071049879, 8.314922557960819915, 115.8322429386477097 ) ) ;
#113015=CARTESIAN_POINT ( 'NONE',  ( -19.05341960407617563, 5.049401038297882671, 113.5427570613523471 ) ) ;
#113016=EDGE_CURVE ( 'NONE', #78253, #85061, #12741, .T. ) ;
#113017=CARTESIAN_POINT ( 'NONE',  ( 13.89961937509957401, 13.97604488694547697, 86.87609039468567573 ) ) ;
#113018=CARTESIAN_POINT ( 'NONE',  ( -15.72974639402197994, 15.80617190586746368, 70.62390960531436690 ) ) ;
#113019=CARTESIAN_POINT ( 'NONE',  ( 16.51473224551083163, -9.474510206698727899, 60.83442372801900433 ) ) ;
#113021=CARTESIAN_POINT ( 'NONE',  ( -0.05219959533907301413, -21.53943276465977519, 102.4989096053143811 ) ) ;
#113022=CARTESIAN_POINT ( 'NONE',  ( -17.44279575226822843, 5.990770900252458731, 85.83557567514317554 ) ) ;
#113023=CARTESIAN_POINT ( 'NONE',  ( -5.153800228976328057, -19.02544592524343514, 72.29057627198102409 ) ) ;
#113025=CARTESIAN_POINT ( 'NONE',  ( -14.34966873604972548, 8.224510206698743886, 28.33442372801902209 ) ) ;
#113027=CARTESIAN_POINT ( 'NONE',  ( 10.81492255796078972, 18.62759615963270932, 109.5822429386476955 ) ) ;
#113028=CARTESIAN_POINT ( 'NONE',  ( 8.224510206698953496, -14.34966873604960469, 67.91557627198102409 ) ) ;
#113029=CARTESIAN_POINT ( 'NONE',  ( 9.564922557960805705, 16.46253265017160317, 74.58224293864769550 ) ) ;
#113030=CARTESIAN_POINT ( 'NONE',  ( -5.719274019375665041, -21.55341960407619695, 89.79275706135236135 ) ) ;
#113031=CARTESIAN_POINT ( 'NONE',  ( 16.52544592524335698, 4.483927247898782831, 31.45942372801901854 ) ) ;
#113032=CARTESIAN_POINT ( 'NONE',  ( -5.153800228976607833, 19.02544592524334988, 42.70942372801901143 ) ) ;
#113033=CARTESIAN_POINT ( 'NONE',  ( 10.72451020669871369, 18.67979575497193778, 52.08442372801901854 ) ) ;
#113034=CARTESIAN_POINT ( 'NONE',  ( -5.823673210054116645, -21.52544592524344225, 57.29057627198103120 ) ) ;
#113035=CARTESIAN_POINT ( 'NONE',  ( -5.049401038297874678, -19.05341960407617918, 104.7927570613523471 ) ) ;
#113036=CARTESIAN_POINT ( 'NONE',  ( -16.46253265017160317, 9.564922557960807481, 60.83224293864769550 ) ) ;
#113037=CARTESIAN_POINT ( 'NONE',  ( 9.474510206698729675, 16.51473224551082808, 87.08442372801900433 ) ) ;
#113038=CARTESIAN_POINT ( 'NONE',  ( 18.67979575497194134, -10.72451020669871369, 90.83442372801901854 ) ) ;
#113039=CARTESIAN_POINT ( 'NONE',  ( -0.05219959533936034679, 19.03943276465977164, 62.50109039468566863 ) ) ;
#113040=CARTESIAN_POINT ( 'NONE',  ( -9.564922557960796823, -16.46253265017161027, 37.08224293864768839 ) ) ;
#113041=CARTESIAN_POINT ( 'NONE',  ( 21.55341960407610458, 5.719274019375980345, 58.95724293864770971 ) ) ;
#113042=CARTESIAN_POINT ( 'NONE',  ( -14.34966873604960291, -8.224510206698953496, 66.66557627198102409 ) ) ;
#113043=CARTESIAN_POINT ( 'NONE',  ( -17.49999999999998579, -5.499999999999973355, 101.2823096230356583 ) ) ;
#113044=CARTESIAN_POINT ( 'NONE',  ( 5.153800228976615827, -19.02544592524334988, 30.20942372801900433 ) ) ;
#113045=CARTESIAN_POINT ( 'NONE',  ( -0.05219959533934338120, 16.53943276465976808, 97.50109039468567573 ) ) ;
#113046=CARTESIAN_POINT ( 'NONE',  ( 14.34966873604960469, 8.224510206698951720, 54.16557627198103120 ) ) ;
#113047=CARTESIAN_POINT ( 'NONE',  ( 15.80617190586769283, -15.72974639402175789, 90.62609039468567573 ) ) ;
#113048=CARTESIAN_POINT ( 'NONE',  ( 10.72451020669871369, 18.67979575497193778, 87.08442372801901854 ) ) ;
#113049=CARTESIAN_POINT ( 'NONE',  ( -21.52544592524343514, 5.823673210054127303, 96.04057627198102409 ) ) ;
#113050=CARTESIAN_POINT ( 'NONE',  ( -16.51473224551069308, -9.474510206698971260, 51.66557627198102409 ) ) ;
#113051=CARTESIAN_POINT ( 'NONE',  ( 10.81492255796106328, -18.62759615963255655, 75.41775706135233293 ) ) ;
#113052=CARTESIAN_POINT ( 'NONE',  ( -19.02544592524342804, 5.153800228976336051, 41.04057627198103120 ) ) ;
#113053=CARTESIAN_POINT ( 'NONE',  ( -13.89961937509977652, 13.97604488694528158, 60.62390960531436690 ) ) ;
#113054=CARTESIAN_POINT ( 'NONE',  ( -16.52544592524342804, 4.483927247898546575, 101.0405762719810383 ) ) ;
#113055=CARTESIAN_POINT ( 'NONE',  ( -13.97604488694527625, -13.89961937509977652, 101.8739096053143811 ) ) ;
#113056=CARTESIAN_POINT ( 'NONE',  ( 8.314922557960818139, 14.29746914071049879, 59.58224293864770260 ) ) ;
#113057=CARTESIAN_POINT ( 'NONE',  ( 8.224510206698953496, -14.34966873604960469, 112.9155762719810383 ) ) ;
#113058=CARTESIAN_POINT ( 'NONE',  ( 10.81492255796078972, 18.62759615963270932, 79.58224293864769550 ) ) ;
#113059=CARTESIAN_POINT ( 'NONE',  ( -18.67979575497193778, 10.72451020669871902, 38.33442372801900433 ) ) ;
#113061=CARTESIAN_POINT ( 'NONE',  ( 12.06949235617739724, 12.14591786802326823, 36.87609039468568994 ) ) ;
#113062=CARTESIAN_POINT ( 'NONE',  ( 15.72974639402199770, -15.80617190586745480, 88.12390960531436690 ) ) ;
#113063=CARTESIAN_POINT ( 'NONE',  ( 5.719274019375673035, 21.55341960407619339, 102.2927570613523613 ) ) ;
#113064=CARTESIAN_POINT ( 'NONE',  ( 13.97604488694527802, 13.89961937509977652, 99.37390960531436690 ) ) ;
#113065=CARTESIAN_POINT ( 'NONE',  ( 10.81492255796106328, -18.62759615963255655, 30.41775706135234358 ) ) ;
#113066=CARTESIAN_POINT ( 'NONE',  ( 18.62759615963271287, -10.81492255796078972, 28.33224293864769550 ) ) ;
#113067=CARTESIAN_POINT ( 'NONE',  ( -16.52544592524335698, -4.483927247898792601, 103.9594237280190185 ) ) ;
#113068=CARTESIAN_POINT ( 'NONE',  ( -15.80617190586768217, 15.72974639402176855, 48.12609039468568284 ) ) ;
#113069=CARTESIAN_POINT ( 'NONE',  ( -21.55341960407619339, 5.719274019375674811, 83.54275706135234714 ) ) ;
#113070=CARTESIAN_POINT ( 'NONE',  ( -13.89961937509957401, -13.97604488694547875, 24.37609039468565442 ) ) ;
#113071=CARTESIAN_POINT ( 'NONE',  ( 16.53943276465976808, 0.05219959533934440121, 81.25109039468568994 ) ) ;
#113072=CARTESIAN_POINT ( 'NONE',  ( 10.81492255796106328, -18.62759615963255655, 40.41775706135234714 ) ) ;
#113073=CARTESIAN_POINT ( 'NONE',  ( -5.049401038298153566, 19.05341960407611168, 35.20724293864768839 ) ) ;
#113074=CARTESIAN_POINT ( 'NONE',  ( 15.72974639402176855, 15.80617190586768217, 96.87609039468568994 ) ) ;
#113075=CARTESIAN_POINT ( 'NONE',  ( -9.474510206698964154, 16.51473224551069663, 105.4155762719810383 ) ) ;
#113076=CARTESIAN_POINT ( 'NONE',  ( 21.55341960407610458, 5.719274019375980345, 108.9572429386476955 ) ) ;
#113077=CARTESIAN_POINT ( 'NONE',  ( 18.09805431107524498, -5.499999999999975131, 88.51606229291890315 ) ) ;
#113078=CARTESIAN_POINT ( 'NONE',  ( -21.53943276465977519, 0.05219959533907696930, 66.24890960531436690 ) ) ;
#113079=CARTESIAN_POINT ( 'NONE',  ( -4.483927247898782831, 16.52544592524335698, 47.70942372801902565 ) ) ;
#113080=CARTESIAN_POINT ( 'NONE',  ( 4.483927247898545687, 16.52544592524342804, 49.79057627198102409 ) ) ;
#113082=CARTESIAN_POINT ( 'NONE',  ( -5.049401038297874678, -19.05341960407617918, 84.79275706135233293 ) ) ;
#113084=CARTESIAN_POINT ( 'NONE',  ( -16.52544592524335698, -4.483927247898792601, 23.95942372801901143 ) ) ;
#113085=CARTESIAN_POINT ( 'NONE',  ( 5.823673210054125526, 21.52544592524343514, 99.79057627198103830 ) ) ;
#113086=CARTESIAN_POINT ( 'NONE',  ( -21.53943276465977519, 0.05219959533907696930, 71.24890960531435269 ) ) ;
#113087=CARTESIAN_POINT ( 'NONE',  ( 5.049401038298161559, -19.05341960407611168, 107.7072429386476955 ) ) ;
#113088=CARTESIAN_POINT ( 'NONE',  ( 8.224510206698742110, 14.34966873604972548, 42.08442372801901854 ) ) ;
#113089=CARTESIAN_POINT ( 'NONE',  ( -19.05341960407611168, -5.049401038298163336, 61.45724293864769550 ) ) ;
#113090=CARTESIAN_POINT ( 'NONE',  ( 5.823673210054444382, -21.52544592524334988, 25.20942372801901854 ) ) ;
#113091=CARTESIAN_POINT ( 'NONE',  ( -16.51473224551082808, 9.474510206698731452, 93.33442372801900433 ) ) ;
#113092=CARTESIAN_POINT ( 'NONE',  ( -13.89961937509977652, 13.97604488694528158, 105.6239096053143527 ) ) ;
#113093=( BOUNDED_SURFACE ( )  B_SPLINE_SURFACE ( 3, 2, ( 
 ( #101777, #72452, #150300, #166465, #42123, #71447, #163465, #136112, #56274, #164468, #26961, #179648, #196808, #41118, #195816, #102782, #57288, #25962, #149291, #134127, #118964, #103785, #73460, #58275, #12780, #119944, #74446, #197788, #182622, #123894, #18734, #199772, #108743, #187601, #171420, #2554, #156239, #106754, #168429, #183614, #76415, #141069, #169416, #154257, #107735, #138091, #60249, #140064, #64236, #92569, #79398, #170419, #139077, #95553, #32906, #155250, #49070, #62226, #29925, #157240, #153252, #31911, #91564, #14754, #110726, #77407, #555, #93564, #1555, #172407, #185593, #30921, #78388, #15748, #125902, #47082, #33896, #186608, #137097, #198783, #121920, #16739, #94560, #45097, #63231, #124910, #61239, #48080, #122911, #184599, #46080, #109736, #17741, #192563, #144044, #69205, #177408, #83363, #3539, #159206, #81358, #129853, #145039, #65217, #130873, #97519, #38879, #52039, #54046, #111725, #189577, #100536, #6521, #126877, #143042, #68200, #191551, #115720, #112711, #162215, #53028, #173411, #114709, #51049, #176402, #174404, #142053, #84359, #20700, #37877, #80381, #99535, #161217, #188583, #35873, #34882, #50064, #19716, #22712, #96537, #158226, #5526, #4520, #66213, #146037, #127873, #82356, #67206, #7521, #128864, #190564, #113695, #175391, #36859, #98526, #160219, #21709, #132877, #182384, #150053, #8538, #86372, #11559, #73225, #197550, #56036, #59018, #88360, #116710, #134896, #194566, #26721, #117714, #85362, #27722, #120685, #102548, #118724, #196573, #10547, #178400, #131883, #166221, #43862, #179410, #195576, #9548, #58043, #105527, #25728, #74211, #87374, #40875, #147054, #164232, #39864, #23714, #149059, #72211, #119713, #133885, #57049, #70216, #180412, #41884, #193568, #148057, #103551, #135879, #181397, #89365, #42875, #55040, #101530, #163222, #24723, #151054, #165226, #104540, #12545, #71214, #90346, #170175, #32659, #122670, #109489, #138834, #169169, #125657, #1303, #185346, #79145, #92326, #136854, #187354, #183373, #314, #60010, #121677, #17488, #107492, #30673, #61982, #31668, #140817, #154012, #137848, #108496, #184359, #94313, #15507, #155991, #16499, #167213, #2306, #28710, #152032, #13517, #62982, #77164, #45840, #44854, #123648, #63987, #124661, #186357, #171172, #48824, #93318, #106510, #46836, #78147, #76168, #155002, #139816, #47837, #199529, #75182, #198539, #168187, #29684, #14506, #91316, #153007, #60998, #64972, #175143, #97274, #37621, #111476, #99283, #20453, #3300, #114450, #160970, #22464, #36611, #96296, #6277, #130620, #157982, #51791, #127631, #19473, #190314, #144794, #82103, #158962, #110477, #173161, #98267, #33645, #172160, #128621, #159969, #34636, #52781, #84112, #21456, #65960, #143795, #83117, #50808, #5278, #66960, #191305, #81119, #49811, #95306, #142799, #113450, #67955, #189331, #7274, #4280, #112466, #129610, #176151, #141807, #174159, #126631, #188333, #192316, #145791, #35629, #68958, #156990, #18489, #80137, #12305, #119473, #104295, #164982, #103303, #55793, #117465, #150809, #26477, #149804, #181156, #42632, #194325, #178156, #87128, #11309, #86126, #165977, #41638, #88119, #89121, #39621, #85113, #69968, #177160, #147817, #195325, #27478, #25486, #72979, #146797, #115471, #73971, #38633, #100290, #134648, #118479, #161968, #135640, #70969, #53796, #148813, #23464, #8290, #162971, #131634, #180169, #193318, #116467, #196334, #57802, #54792, #9303, #101281, #24476, #132637, #179163, #40631, #56805, #102300, #163989, #10303, #71960, #133634, #92079, #108255, #184120, #151792, #105283, #139579, #170928, #167951, #168926, #183129, #74, #94074, #199288, #47595, #60755, #29450, #120442, #14261, #90108, #17251, #152769, #45602, #185105, #137605, #75930, #78904, #153768, #107255, #197310, #59768, #30432, #109248, #31426, #62739, #16261, #166971, #28474, #43619, #136610, #1064, #91082, #122428, #15263, #198291 ),
 ( #58774, #13283, #76921, #74947, #121436, #32419, #138592, #61744, #123412, #46595, #155753, #169935, #93079, #154763, #77912, #124419, #186115, #182136, #44612, #106267, #52549, #2071, #19246, #174913, #22225, #143558, #5041, #125424, #96066, #171925, #140581, #79908, #128387, #160733, #114210, #4049, #129380, #37386, #66727, #63750, #80893, #141579, #99043, #190083, #36377, #6044, #67722, #142570, #64744, #173927, #98031, #172929, #191076, #51559, #113223, #175915, #126406, #33414, #156761, #187120, #34408, #81867, #48592, #112237, #159728, #95073, #110243, #18255, #3067, #188102, #49575, #111238, #21224, #50577, #157755, #65726, #97047, #127395, #82880, #144558, #189104, #35396, #158729, #20219, #70735, #133396, #193082, #162734, #56568, #40394, #54557, #72743, #83874, #24242, #117231, #131394, #104062, #102065, #7034, #38393, #148576, #132402, #11065, #84874, #134414, #194095, #176922, #87881, #196100, #57570, #10066, #69726, #179933, #165743, #116230, #25250, #101049, #177921, #163750, #118242, #55557, #178924, #145556, #146551, #71726, #68716, #130373, #86892, #195086, #8047, #26242, #119240, #41400, #39389, #103065, #164747, #85891, #149569, #180924, #42399, #147579, #23230, #192071, #9065, #53552, #115231, #100049, #161735, #89884, #74723, #141099, #95586, #58550, #47114, #181906, #43385, #50096, #124942, #105057, #48110, #3571, #1587, #18766, #188615, #157270, #80413, #2586, #79428, #31942, #93596, #136386, #111756, #156271, #12077, #151567, #17773, #64266, #65249, #59529, #126909, #94593, #120216, #125932, #198063, #32938, #121207, #88886, #33928, #27237, #108773, #186639, #187631, #16772, #166741, #135412, #172440, #150578, #182898, #63262, #13056, #49101, #73740, #155282, #142085, #78420, #170451, #197083, #140096, #28244, #109766, #171450, #110759, #161249, #113728, #190595, #193601, #129884, #160252, #55073, #35904, #145071, #23748, #7553, #38910, #192595, #143074, #4552, #19747, #112741, #177440, #5558, #52072, #144077, #174434, #96569, #176435, #100567, #128896, #115752, #6553, #175425, #131917, #69239, #191584, #85397, #98558, #66245, #173445, #189607, #68231, #127905, #51081, #147090, #36893, #21742, #53062, #37909, #8574, #83394, #67237, #114741, #99568, #162249, #22743, #70249, #84392, #34913, #158257, #81388, #146068, #130905, #97550, #54078, #159238, #20732, #82389, #86406, #116743, #194599, #73259, #120717, #74243, #133921, #12578, #197583, #150087, #39901, #149093, #56071, #134928, #11591, #163257, #135912, #10583, #59050, #180447, #178433, #71248, #196605, #58076, #101566, #72244, #24759, #181429, #179444, #104573, #195612, #119746, #57084, #148091, #9582, #132912, #42907, #166255, #117751, #27755, #118758, #87408, #40910, #102583, #88394, #89398, #165260, #164267, #25762, #41919, #103585, #26754, #151087, #20380, #114376, #190242, #117392, #52712, #84043, #85039, #37549, #176080, #179091, #53725, #145722, #97204, #159897, #68887, #147743, #131561, #162896, #116390, #66884, #128545, #143723, #36538, #101207, #129538, #99212, #67885, #98194, #82027, #100217, #24405, #160900, #39548, #130547, #22393, #55720, #193245, #115401, #9230, #7203, #51719, #158890, #113382, #192244, #175072, #21386, #70897, #177089, #38561, #161898, #23393, #132564, #146720, #191238, #8217, #69893, #86054, #54718, #194253, #178080, #5203, #83044, #144719, #6205, #74878, #122354, #43548, #105214, #25414, #196263, #71889, #40560, #180098, #28401, #60679, #152696, #104223, #29379, #137530, #166901, #163918, #119402, #41566, #90040, #151722, #87056, #91010, #57732, #199212, #12237, #14185, #133559, #149732, #102229, #13215, #148741, #103229, #198221, #183057, #44541, #136540, #164911, #27402, #59693, #11233, #181085, #121364, #197241, #72907, #75854, #10229, #42560, #73899, #88044, #195250, #58702, #56734, #118404, #106196, #89047, #167880, #26405, #134576, #150737, #165904, #135569, #120372, #182065 ),
 ( #157677, #16184, #19167, #48518, #76847, #33339, #154689, #187048, #77839, #45526, #188028, #80816, #62663, #78830, #94999, #170856, #138518, #91998, #126331, #142494, #139506, #155681, #169858, #110172, #3972, #186038, #34331, #47521, #989, #107180, #124343, #30717, #65652, #109177, #32347, #171851, #94000, #17176, #184043, #140508, #1997, #168851, #46518, #63676, #95992, #18179, #49499, #2991, #153692, #15188, #30356, #123338, #111161, #125351, #156685, #79836, #185031, #61669, #141506, #172850, #64669, #108177, #31352, #93003, #81165, #19520, #52829, #22511, #67008, #68003, #188381, #157039, #130670, #18536, #80183, #141855, #3346, #129655, #5324, #50855, #49858, #51839, #7320, #114498, #65021, #174206, #96342, #144839, #160017, #126677, #145838, #112513, #53847, #128667, #69004, #111524, #4326, #115521, #21504, #173209, #158029, #83165, #6323, #192364, #127678, #177209, #191351, #34685, #176200, #66010, #98317, #189378, #142847, #99334, #95354, #35674, #190363, #37669, #82149, #97322, #159008, #161017, #20501, #143845, #113498, #175193, #84158, #36659, #40677, #89166, #102347, #9351, #162017, #55839, #131684, #58821, #194372, #25534, #26521, #179210, #117513, #120489, #195372, #87178, #38682, #101329, #10350, #150858, #73025, #104341, #57849, #8340, #70015, #85160, #178203, #42680, #71016, #164036, #132684, #39667, #23513, #41685, #166025, #148859, #181203, #72007, #134697, #86175, #100338, #119521, #12352, #133680, #193365, #146846, #54841, #56851, #116516, #163017, #74015, #118526, #180215, #103349, #165028, #135685, #88166, #149850, #11354, #196380, #27525, #197357, #24524, #147865, #182180, #94119, #43665, #60799, #16304, #63797, #185148, #46638, #167015, #137647, #13325, #105327, #121481, #169977, #2115, #155798, #45645, #170973, #78950, #108298, #77954, #153811, #30473, #28516, #44657, #31469, #90152, #151835, #117, #93121, #106310, #124464, #17296, #154806, #199334, #15306, #139621, #122472, #76965, #168968, #62783, #167996, #183175, #74990, #29492, #123456, #138636, #184163, #140625, #91125, #152815, #1109, #47642, #136654, #107296, #198335, #59811, #14307, #61786, #75974, #186161, #92123, #109294, #32466, #83922, #191122, #175962, #36419, #174956, #127440, #189146, #22271, #98075, #21268, #52596, #114257, #65771, #49621, #158773, #82925, #157799, #37431, #113264, #159773, #160783, #111283, #156807, #35438, #172973, #34452, #144603, #99091, #97090, #6088, #18299, #187166, #145603, #48637, #110289, #171971, #33459, #67767, #20262, #80937, #79955, #81908, #7082, #129424, #125469, #95117, #141624, #190125, #64789, #112280, #3113, #96111, #4092, #126450, #143601, #19290, #188148, #142613, #50619, #5085, #173970, #66767, #128428, #51600, #23275, #133440, #55600, #196141, #69770, #57613, #178968, #161780, #72786, #119281, #180964, #195130, #54598, #164790, #88930, #116272, #10110, #85933, #177962, #148619, #147622, #27284, #40435, #42441, #100096, #39430, #150622, #56611, #53601, #131438, #118285, #179976, #104104, #101090, #165787, #41444, #84919, #103109, #162776, #71770, #24284, #130421, #134456, #68763, #9110, #163792, #26284, #117274, #146599, #176971, #11111, #192119, #70776, #102107, #132445, #87926, #115277, #194136, #38440, #25294, #86936, #8092, #149613, #193124, #32232, #167765, #199094, #200088, #152580, #29263, #93890, #168736, #60561, #12118, #74764, #183927, #62551, #46400, #77728, #31238, #181947, #43430, #58590, #151607, #16070, #44425, #90894, #182942, #13099, #135454, #15071, #139394, #14070, #154574, #45412, #108059, #59573, #73782, #92887, #124227, #137413, #105099, #197123, #28286, #107065, #166785, #89926, #185923, #75737, #122237, #30240, #76732, #47408, #91883, #106079, #153574, #138408, #876, #61556, #109064, #123225, #120256, #170742, #136426, #184916, #169743, #198107, #121248, #158546, #140393, #111051, #186934, #155568, #94889, #143361, #175717, #67531 ),
 ( #79723, #97844, #129189, #4853, #172739, #127200, #81678, #95882, #188914, #142383, #36190, #141392, #156573, #17063, #2880, #96862, #112052, #34220, #52363, #18068, #64559, #66538, #21031, #48404, #157565, #110061, #171741, #37196, #50392, #33230, #173740, #190887, #35209, #144368, #114020, #82684, #5855, #128202, #189899, #19058, #80705, #78717, #51374, #113035, #1881, #63562, #3861, #126223, #20036, #174727, #187919, #125236, #159532, #49388, #65541, #23039, #130183, #8872, #84684, #146364, #56366, #26048, #70539, #71535, #191879, #160548, #134221, #22038, #83689, #145367, #6849, #133201, #132208, #54370, #53363, #55363, #10874, #118049, #179739, #41209, #102870, #163553, #38206, #85697, #148380, #7851, #177731, #194892, #117033, #69538, #87693, #98853, #39200, #193899, #131202, #119055, #178728, #68528, #115040, #25053, #147384, #149378, #99862, #72544, #40190, #176733, #164555, #195907, #57382, #86696, #192892, #180737, #161546, #116042, #101870, #100856, #162538, #9875, #24042, #13844, #90677, #42213, #104866, #168520, #165554, #103873, #45191, #136201, #27051, #46173, #139170, #121013, #137184, #153345, #29037, #196897, #150393, #184689, #15841, #12871, #75511, #28054, #106845, #647, #44196, #92659, #105855, #74536, #88697, #59344, #135225, #62317, #197876, #152359, #30018, #182711, #167542, #123987, #198872, #60339, #11889, #166555, #122013, #154348, #76509, #107826, #61332, #73552, #58364, #120031, #181716, #169510, #183704, #91656, #14846, #43199, #89695, #138185, #31010, #199868, #77500, #123003, #151381, #33002, #5622, #66308, #97612, #110823, #155346, #67301, #1651, #18831, #78486, #140159, #35965, #125996, #187694, #157336, #188680, #159301, #49164, #156336, #126972, #141163, #112805, #172505, #174498, #34980, #185685, #20797, #47175, #64329, #19809, #108834, #50160, #111819, #170514, #2652, #16835, #32004, #125007, #173507, #93661, #82452, #33992, #144140, #63329, #96633, #186702, #95648, #48173, #158321, #81450, #109830, #171513, #80476, #94656, #142149, #17836, #79494, #3633, #65312, #143137, #4616, #127968, #189671, #51144, #102649, #161315, #164334, #193667, #21806, #178500, #99633, #40980, #190660, #7619, #163327, #10650, #131982, #55138, #113793, #84455, #160316, #128960, #68298, #116808, #149160, #25828, #192659, #117819, #87473, #39966, #52136, #69303, #129949, #101636, #24823, #175488, #179512, #146133, #36960, #100632, #98622, #83458, #37975, #145136, #86472, #6619, #191649, #148157, #9649, #53128, #22809, #114806, #71315, #176499, #132978, #130969, #194668, #54142, #115816, #56138, #177506, #38975, #23814, #162313, #85464, #147153, #8641, #70313, #45939, #42976, #43964, #58145, #75285, #169272, #74313, #122770, #135980, #104641, #195680, #89467, #165330, #95156, #27825, #59117, #60111, #12646, #151156, #156844, #28810, #120783, #72312, #134997, #105626, #184459, #106614, #137947, #91421, #41986, #103652, #118829, #11660, #76269, #166328, #197651, #182483, #73326, #57151, #136956, #199630, #167314, #14612, #90451, #168289, #119813, #133989, #153108, #107594, #152135, #26822, #180513, #88463, #13618, #150159, #196676, #33497, #198645, #121779, #183472, #44957, #181498, #29785, #61097, #159815, #174009, #145643, #143641, #7123, #67810, #18339, #79994, #130464, #141662, #97129, #52637, #100137, #21310, #82967, #3154, #35480, #49659, #64827, #157839, #6127, #38480, #192162, #81949, #68805, #115319, #144644, #126489, #158813, #19330, #129465, #191164, #188187, #53642, #20301, #177011, #190165, #111323, #173013, #127480, #34492, #114302, #96150, #80978, #176004, #37473, #142653, #50658, #4132, #99134, #65811, #160824, #189185, #22312, #112319, #5124, #83963, #66806, #128469, #113305, #51641, #174996, #36461, #98118, #104145, #135494, #132485, #133478, #147662, #164830, #58630, #163832, #12159, #25334, #194174, #84957, #179007, #54636, #181989, #117311, #148662, #149654 ),
 ( #11152, #57654, #27324, #88971, #102147, #85972, #195170, #119320, #55638, #73824, #72826, #134495, #197164, #9149, #193164, #71810, #70816, #40475, #181007, #150661, #56651, #196182, #116311, #23313, #120296, #146639, #8132, #69810, #131477, #42482, #118324, #86975, #178000, #180017, #43471, #165827, #161818, #39467, #101128, #26326, #162814, #10150, #103149, #41484, #24323, #87966, #93928, #154612, #105139, #17102, #166825, #183964, #139432, #186973, #108097, #169782, #89965, #60601, #136465, #28326, #44465, #92926, #125276, #78754, #168775, #155607, #1921, #31275, #151645, #45451, #106119, #16107, #77765, #13140, #140431, #122276, #63600, #76772, #74802, #198145, #14110, #59615, #914, #121288, #167803, #62588, #124266, #182981, #137455, #29303, #185961, #90933, #47446, #75777, #109102, #199134, #152619, #170781, #107105, #30277, #200125, #32271, #91923, #153615, #15111, #138444, #61594, #123263, #184954, #46438, #51409, #145401, #50430, #98888, #112089, #19094, #171779, #65580, #141431, #68561, #3900, #35245, #36227, #188953, #127239, #130218, #4890, #96899, #48443, #111088, #20072, #160582, #82724, #114058, #67567, #18106, #79760, #94926, #187957, #52399, #80743, #173779, #142421, #49427, #33267, #113069, #175755, #158583, #190922, #81716, #144405, #95918, #110100, #129225, #22071, #143401, #2918, #156611, #64596, #66572, #126260, #172778, #83722, #128237, #189934, #174761, #97879, #6883, #159570, #21068, #5891, #37232, #34259, #157603, #163586, #178762, #72580, #116075, #131237, #53397, #39232, #133234, #148414, #147418, #88731, #54403, #100888, #102904, #57415, #23072, #8905, #146396, #7885, #11921, #86729, #69571, #9909, #165587, #25087, #180770, #150426, #119088, #42245, #164588, #41242, #193933, #55396, #73585, #26082, #87726, #103906, #27085, #132241, #177763, #71569, #149411, #24075, #191913, #179773, #10907, #115075, #162572, #84718, #101904, #85730, #70573, #134254, #176767, #194926, #195941, #192925, #38239, #99894, #161579, #117066, #40227, #56401, #118083, #45220, #90707, #89728, #91687, #47206, #92690, #154378, #77530, #139202, #199898, #74566, #122044, #184719, #44230, #13876, #107857, #153377, #105887, #124018, #135257, #75543, #168548, #182745, #155375, #14879, #58397, #151414, #61362, #183734, #62348, #136234, #185715, #106875, #28088, #677, #108865, #170544, #123033, #121050, #31041, #16864, #167574, #76540, #152390, #29068, #138216, #169542, #30046, #46203, #196929, #197908, #15872, #120063, #181751, #32035, #93692, #59378, #43233, #104899, #137217, #198904, #166588, #12902, #60372, #128990, #66337, #127998, #113820, #2681, #109857, #188709, #64358, #126027, #35993, #5651, #50191, #51174, #171542, #140189, #175515, #1681, #63359, #125036, #186732, #112834, #111848, #34022, #33030, #35007, #190688, #97640, #159329, #20825, #82482, #143166, #17867, #65341, #189701, #187723, #157366, #174526, #96662, #49194, #67328, #78515, #18860, #173538, #110852, #98651, #158349, #48203, #94685, #4646, #127001, #52163, #79522, #36989, #19838, #156364, #144166, #160345, #141192, #172536, #95680, #80506, #142179, #3663, #81479, #39002, #7646, #101663, #56165, #193695, #70341, #21834, #84483, #148183, #145164, #83486, #39992, #71342, #146160, #164360, #195707, #133005, #177533, #55164, #9677, #162340, #116834, #8668, #102675, #69330, #161344, #6648, #130996, #163354, #178525, #100658, #118856, #192688, #54171, #194695, #87499, #53156, #23841, #176529, #38005, #42013, #24850, #99660, #86499, #57179, #117846, #10676, #180539, #149187, #72340, #179539, #41008, #85490, #147179, #103677, #25855, #134015, #68326, #129976, #132008, #191676, #114835, #22836, #115844, #121804, #152159, #46966, #27852, #136980, #15633, #199657, #30804, #184487, #135026, #196701, #11687, #104669, #169298, #197675, #182509, #136004, #166354, #88491, #168315, #92453, #120810, #107620, #198669, #61123, #12671, #185476 ),
 ( #29811, #138960, #105650, #59140, #106642, #43989, #154141, #90477, #77290, #14638, #165356, #439, #26850, #167339, #122797, #150186, #91447, #153135, #73353, #28836, #58171, #119838, #89493, #76297, #181523, #62114, #13642, #123777, #43002, #137975, #151183, #75309, #74338, #45966, #60136, #183498, #44982, #125784, #67091, #80264, #159089, #139946, #17621, #128750, #34767, #93445, #171303, #96424, #158110, #82236, #140950, #143926, #173293, #1436, #19602, #79280, #111608, #2437, #170303, #112595, #5407, #187486, #3425, #81244, #95437, #63114, #16625, #50937, #190447, #64119, #141934, #94441, #142925, #108625, #110605, #20584, #172287, #48952, #31796, #33777, #124792, #155132, #157121, #78273, #65101, #186491, #47967, #18617, #109619, #4407, #32789, #156122, #66092, #127758, #126759, #188462, #49943, #189459, #174287, #35757, #97402, #54925, #145921, #113581, #55922, #148945, #130755, #146936, #163104, #38763, #6404, #160101, #194451, #25616, #22594, #23598, #37756, #116597, #10435, #53929, #102431, #115604, #84242, #175275, #69088, #144922, #72093, #7404, #100421, #39749, #192447, #177293, #133767, #8426, #162102, #51922, #114587, #85245, #164118, #86256, #117597, #71097, #21588, #83246, #98405, #191434, #179298, #70098, #131767, #193449, #52911, #36741, #178286, #40762, #101412, #87260, #24608, #147946, #99417, #68085, #132764, #129737, #9432, #176284, #161099, #11441, #28600, #88249, #149934, #45733, #135771, #197442, #167099, #198424, #169057, #58908, #166111, #136740, #150945, #122561, #120575, #184251, #44742, #195462, #107385, #56937, #74101, #29577, #77053, #59899, #121567, #180301, #12439, #26606, #118611, #134782, #183261, #15396, #30564, #182269, #92215, #153901, #106398, #41769, #43752, #196464, #168080, #91208, #103434, #165114, #105415, #90238, #152898, #73112, #57934, #119605, #181288, #42766, #104428, #27613, #14395, #151921, #13410, #89253, #75074, #76061, #137736, #199420, #60884, #81024, #3199, #78040, #125555, #188233, #47729, #17382, #111372, #95205, #109382, #127528, #138724, #79038, #172056, #186251, #158861, #156892, #61874, #93210, #64873, #187252, #65857, #139709, #189232, #48721, #31559, #142700, #50710, #112368, #126534, #124554, #34538, #20350, #171062, #80039, #155885, #32552, #18388, #173061, #110374, #33543, #205, #1196, #49706, #123544, #185237, #141708, #96197, #62873, #4179, #174059, #157886, #94205, #19375, #35528, #140713, #97176, #46729, #108391, #2203, #63884, #170068, #154895, #16393, #68857, #191211, #162866, #159866, #144691, #100187, #193214, #51692, #52686, #113354, #175046, #24374, #7174, #36511, #130516, #39518, #145692, #54688, #88761, #116361, #178050, #161869, #38531, #176054, #37521, #101178, #23363, #85009, #81998, #143691, #99183, #6176, #192212, #146689, #114349, #5173, #8185, #69861, #66856, #67856, #98166, #53695, #129511, #160872, #128518, #190213, #21359, #131530, #83016, #22362, #84014, #115372, #177061, #187894, #32208, #82656, #78691, #95855, #155543, #17037, #113007, #2853, #64531, #34194, #65514, #36164, #126198, #33204, #3835, #18042, #189872, #49361, #51347, #112025, #62525, #174700, #124198, #141366, #96837, #144340, #127175, #188885, #47383, #79696, #93865, #185898, #1855, #50366, #109038, #97816, #111024, #159505, #21001, #173714, #170717, #172710, #63537, #35182, #158521, #140368, #125212, #157539, #186908, #19033, #48379, #110036, #171714, #94862, #20009, #156543, #80679, #81652, #143336, #142355, #4823, #66511, #128173, #101582, #58089, #179458, #11604, #102596, #67504, #12593, #105571, #87421, #103598, #119759, #195625, #163270, #116756, #151101, #182430, #40923, #180460, #194612, #73272, #167257, #10596, #59063, #72257, #164282, #129161, #25775, #24772, #28756, #149106, #57098, #196619, #133935, #118772, #90393, #165273, #41932, #5828, #71261, #26767, #120730, #42921, #74257, #27769, #178447, #39914, #52335 ),
 ( #43909, #88407, #150103, #190858, #134942, #86419, #148105, #181443, #104586, #166271, #89412, #135927, #9596, #197597, #132925, #56084, #117765, #123693, #2352, #186405, #17534, #171217, #121723, #183415, #198587, #91362, #156037, #184404, #169214, #122714, #153053, #75229, #155049, #79194, #107538, #94358, #185391, #47882, #199573, #172206, #32706, #64033, #77209, #44899, #33691, #168233, #46882, #106556, #29729, #125703, #92370, #154056, #108542, #16544, #187402, #15551, #45885, #93362, #30723, #140863, #138878, #48870, #1350, #152077, #110525, #13562, #358, #109535, #136900, #78191, #139861, #60055, #62028, #14555, #76213, #137892, #63030, #61042, #170221, #31714, #124707, #138579, #140570, #156751, #189093, #59, #111227, #157744, #19234, #33403, #93065, #3057, #127382, #154752, #48580, #124409, #16249, #187110, #141569, #78891, #155742, #107242, #169922, #95062, #30418, #168912, #125413, #18245, #31414, #49563, #80882, #79898, #62726, #2060, #64734, #47584, #63739, #94063, #188092, #77901, #46581, #92066, #139568, #110233, #171914, #126395, #153754, #61732, #172919, #17239, #123400, #34398, #96056, #15249, #185092, #142559, #4037, #65715, #76908, #1052, #108243, #186103, #109236, #170915, #32408, #36365, #130359, #84860, #22212, #99030, #50566, #113211, #176909, #173916, #112226, #68703, #100036, #174900, #193067, #24225, #161722, #6030, #83861, #38380, #191063, #145543, #37372, #131379, #98017, #190071, #35385, #159712, #192057, #7021, #67709, #147564, #21210, #82867, #23217, #116216, #81853, #129367, #5029, #66714, #70719, #53539, #128375, #115216, #85876, #146537, #39375, #9049, #177907, #101034, #8031, #69712, #52536, #114196, #132387, #54543, #162719, #97037, #158717, #175901, #144545, #20207, #143543, #160720, #51547, #181891, #43369, #29207, #118226, #25235, #104046, #179917, #41384, #151551, #121191, #165726, #166725, #86876, #55543, #90841, #117215, #178908, #40376, #102050, #28229, #27222, #149553, #148560, #150563, #106024, #13041, #74708, #136371, #198048, #58535, #133379, #180908, #105041, #103049, #72724, #89869, #12062, #164731, #182884, #194080, #134397, #88870, #26225, #14013, #163735, #10051, #71711, #195069, #59514, #73724, #11048, #56549, #135397, #167711, #44367, #152526, #75679, #87865, #120201, #196084, #42383, #57554, #119224, #197068, #110001, #93832, #108001, #126166, #137358, #16015, #170687, #184861, #157507, #155512, #60507, #91827, #1824, #124165, #168684, #32176, #186877, #19001, #30185, #141334, #187861, #49330, #63506, #123173, #33171, #199037, #46344, #78659, #154518, #169687, #17007, #171682, #109008, #185867, #122182, #200036, #125181, #183874, #45359, #140334, #48347, #61504, #79663, #110991, #94830, #92833, #156508, #18009, #77672, #2821, #47353, #64499, #31182, #76678, #107011, #139341, #172676, #34161, #820, #95822, #62494, #153520, #15017, #138354, #111991, #97785, #35148, #96804, #100794, #175659, #158490, #98793, #54310, #52303, #69475, #39139, #146303, #131141, #191820, #130123, #82625, #144307, #177671, #53300, #176672, #7792, #192829, #20968, #4789, #113960, #38148, #112975, #115982, #68468, #114979, #162477, #66479, #173681, #190827, #128141, #189841, #99802, #80647, #37133, #161488, #19977, #142323, #3803, #65481, #127143, #188850, #159474, #22976, #50334, #83629, #145306, #81620, #36133, #143303, #51314, #174668, #84625, #5797, #67470, #129129, #160487, #21977, #6789, #10813, #102812, #24993, #73489, #88633, #8810, #74474, #41149, #182649, #195844, #136139, #55302, #133141, #44133, #150329, #70479, #86637, #11824, #135162, #197815, #56305, #59280, #196835, #116974, #58303, #194832, #26988, #117987, #85635, #27991, #120950, #164497, #118993, #119970, #72483, #178666, #132145, #166493, #105792, #179677, #57317, #9815, #181656, #23979, #25990, #147322, #87633, #149319, #193838, #134156, #40129, #101807, #180676, #42152, #43135, #103812 ) ),
 .UNSPECIFIED., .T., .F., .T. ) 
 B_SPLINE_SURFACE_WITH_KNOTS ( ( 4, 3, 4 ),
 ( 3, 2, 2, 2, 2, 2, 2, 2, 2, 2, 2, 2, 2, 2, 2, 2, 2, 2, 2, 2, 2, 2, 2, 2, 2, 2, 2, 2, 2, 2, 2, 2, 2, 2, 2, 2, 2, 2, 2, 2, 2, 2, 2, 2, 2, 2, 2, 2, 2, 2, 2, 2, 2, 2, 2, 2, 2, 2, 2, 2, 2, 2, 2, 2, 2, 2, 2, 2, 2, 2, 2, 2, 2, 2, 2, 2, 2, 2, 2, 2, 2, 2, 2, 2, 2, 2, 2, 2, 2, 2, 2, 2, 2, 2, 2, 2, 2, 2, 2, 2, 2, 2, 2, 2, 2, 2, 2, 2, 2, 2, 2, 2, 2, 2, 2, 2, 2, 2, 2, 2, 2, 2, 2, 2, 2, 2, 2, 2, 2, 2, 2, 2, 2, 2, 2, 2, 2, 2, 2, 2, 2, 2, 2, 2, 2, 2, 2, 2, 2, 2, 2, 2, 2, 2, 2, 2, 2, 2, 2, 2, 2, 2, 2, 2, 2, 2, 2, 2, 2, 2, 2, 2, 2, 2, 2, 2, 2, 2, 2, 2, 2, 2, 2, 2, 2, 2, 2, 2, 2, 2, 2, 2, 2, 2, 2, 2, 2, 2, 2, 2, 2, 2, 2, 2, 2, 2, 2, 2, 2, 2, 2, 2, 2, 2, 2, 2, 2, 2, 2, 2, 2, 2, 2, 2, 2, 2, 2, 2, 3 ),
 ( 0.000000000000000000, 0.5000000000000000000, 1.000000000000000000 ),
 ( 0.000000000000000000, 0.004385964912280701511, 0.008771929824561403022, 0.01315789473684210453, 0.01754385964912280604, 0.02192982456140350755, 0.02631578947368420907, 0.03070175438596491058, 0.03508771929824561209, 0.03947368421052631360, 0.04385964912280701511, 0.04824561403508771662, 0.05263157894736841813, 0.05701754385964911964, 0.06140350877192982115, 0.06578947368421052266, 0.07017543859649122417, 0.07456140350877192569, 0.07894736842105262720, 0.08333333333333332871, 0.08771929824561403022, 0.09210526315789473173, 0.09649122807017543324, 0.1008771929824561348, 0.1052631578947368363, 0.1096491228070175378, 0.1140350877192982393, 0.1184210526315789408, 0.1228070175438596423, 0.1271929824561403577, 0.1315789473684210453, 0.1359649122807017607, 0.1403508771929824483, 0.1447368421052631637, 0.1491228070175438514, 0.1535087719298245668, 0.1578947368421052544, 0.1622807017543859698, 0.1666666666666666574, 0.1710526315789473728, 0.1754385964912280604, 0.1798245614035087758, 0.1842105263157894635, 0.1885964912280701788, 0.1929824561403508665, 0.1973684210526315819, 0.2017543859649122695, 0.2061403508771929849, 0.2105263157894736725, 0.2149122807017543879, 0.2192982456140350755, 0.2236842105263157909, 0.2280701754385964786, 0.2324561403508771940, 0.2368421052631578816, 0.2412280701754385970, 0.2456140350877192846, 0.2500000000000000000, 0.2543859649122807154, 0.2587719298245614308, 0.2631578947368420907, 0.2675438596491228060, 0.2719298245614035214, 0.2763157894736842368, 0.2807017543859648967, 0.2850877192982456121, 0.2894736842105263275, 0.2938596491228070429, 0.2982456140350877027, 0.3026315789473684181, 0.3070175438596491335, 0.3114035087719298489, 0.3157894736842105088, 0.3201754385964912242, 0.3245614035087719396, 0.3289473684210526550, 0.3333333333333333148, 0.3377192982456140302, 0.3421052631578947456, 0.3464912280701754610, 0.3508771929824561209, 0.3552631578947368363, 0.3596491228070175517, 0.3640350877192982670, 0.3684210526315789269, 0.3728070175438596423, 0.3771929824561403577, 0.3815789473684210731, 0.3859649122807017330, 0.3903508771929824483, 0.3947368421052631637, 0.3991228070175438791, 0.4035087719298245390, 0.4078947368421052544, 0.4122807017543859698, 0.4166666666666666852, 0.4210526315789473450, 0.4254385964912280604, 0.4298245614035087758, 0.4342105263157894912, 0.4385964912280701511, 0.4429824561403508665, 0.4473684210526315819, 0.4517543859649122973, 0.4561403508771929571, 0.4605263157894736725, 0.4649122807017543879, 0.4692982456140351033, 0.4736842105263157632, 0.4780701754385964786, 0.4824561403508771940, 0.4868421052631579093, 0.4912280701754385692, 0.4956140350877192846, 0.5000000000000000000, 0.5043859649122807154, 0.5087719298245614308, 0.5131578947368421462, 0.5175438596491228616, 0.5219298245614034659, 0.5263157894736841813, 0.5307017543859648967, 0.5350877192982456121, 0.5394736842105263275, 0.5438596491228070429, 0.5482456140350877583, 0.5526315789473684736, 0.5570175438596490780, 0.5614035087719297934, 0.5657894736842105088, 0.5701754385964912242, 0.5745614035087719396, 0.5789473684210526550, 0.5833333333333333703, 0.5877192982456140857, 0.5921052631578946901, 0.5964912280701754055, 0.6008771929824561209, 0.6052631578947368363, 0.6096491228070175517, 0.6140350877192982670, 0.6184210526315789824, 0.6228070175438596978, 0.6271929824561403022, 0.6315789473684210176, 0.6359649122807017330, 0.6403508771929824483, 0.6447368421052631637, 0.6491228070175438791, 0.6535087719298245945, 0.6578947368421053099, 0.6622807017543859143, 0.6666666666666666297, 0.6710526315789473450, 0.6754385964912280604, 0.6798245614035087758, 0.6842105263157894912, 0.6885964912280702066, 0.6929824561403509220, 0.6973684210526315264, 0.7017543859649122417, 0.7061403508771929571, 0.7105263157894736725, 0.7149122807017543879, 0.7192982456140351033, 0.7236842105263158187, 0.7280701754385965341, 0.7324561403508771384, 0.7368421052631578538, 0.7412280701754385692, 0.7456140350877192846, 0.7500000000000000000, 0.7543859649122807154, 0.7587719298245614308, 0.7631578947368421462, 0.7675438596491228616, 0.7719298245614034659, 0.7763157894736841813, 0.7807017543859648967, 0.7850877192982456121, 0.7894736842105263275, 0.7938596491228070429, 0.7982456140350877583, 0.8026315789473684736, 0.8070175438596490780, 0.8114035087719297934, 0.8157894736842105088, 0.8201754385964912242, 0.8245614035087719396, 0.8289473684210526550, 0.8333333333333333703, 0.8377192982456140857, 0.8421052631578946901, 0.8464912280701754055, 0.8508771929824561209, 0.8552631578947368363, 0.8596491228070175517, 0.8640350877192982670, 0.8684210526315789824, 0.8728070175438596978, 0.8771929824561403022, 0.8815789473684210176, 0.8859649122807017330, 0.8903508771929824483, 0.8947368421052631637, 0.8991228070175438791, 0.9035087719298245945, 0.9078947368421053099, 0.9122807017543859143, 0.9166666666666666297, 0.9210526315789473450, 0.9254385964912280604, 0.9298245614035087758, 0.9342105263157894912, 0.9385964912280702066, 0.9429824561403509220, 0.9473684210526315264, 0.9517543859649122417, 0.9561403508771929571, 0.9605263157894736725, 0.9649122807017543879, 0.9692982456140351033, 0.9736842105263158187, 0.9780701754385965341, 0.9824561403508771384, 0.9868421052631578538, 0.9912280701754385692, 0.9956140350877192846, 1.000000000000000000 ),
 .UNSPECIFIED. ) 
 GEOMETRIC_REPRESENTATION_ITEM ( )  RATIONAL_B_SPLINE_SURFACE ( (
 ( 1.000000000000000000, 0.9659258262890683122, 1.000000000000000000, 0.9659258262890683122, 1.000000000000000000, 0.9659258262890683122, 1.000000000000000000, 0.9659258262890683122, 1.000000000000000000, 0.9659258262890683122, 1.000000000000000000, 0.9659258262890683122, 1.000000000000000000, 0.9659258262890683122, 1.000000000000000000, 0.9659258262890683122, 1.000000000000000000, 0.9659258262890683122, 1.000000000000000000, 0.9659258262890683122, 1.000000000000000000, 0.9659258262890683122, 1.000000000000000000, 0.9659258262890683122, 1.000000000000000000, 0.9659258262890683122, 1.000000000000000000, 0.9659258262890683122, 1.000000000000000000, 0.9659258262890683122, 1.000000000000000000, 0.9659258262890683122, 1.000000000000000000, 0.9659258262890683122, 1.000000000000000000, 0.9659258262890683122, 1.000000000000000000, 0.9659258262890683122, 1.000000000000000000, 0.9659258262890683122, 1.000000000000000000, 0.9659258262890683122, 1.000000000000000000, 0.9659258262890683122, 1.000000000000000000, 0.9659258262890683122, 1.000000000000000000, 0.9659258262890683122, 1.000000000000000000, 0.9659258262890683122, 1.000000000000000000, 0.9659258262890683122, 1.000000000000000000, 0.9659258262890683122, 1.000000000000000000, 0.9659258262890683122, 1.000000000000000000, 0.9659258262890683122, 1.000000000000000000, 0.9659258262890683122, 1.000000000000000000, 0.9659258262890683122, 1.000000000000000000, 0.9659258262890683122, 1.000000000000000000, 0.9659258262890683122, 1.000000000000000000, 0.9659258262890683122, 1.000000000000000000, 0.9659258262890683122, 1.000000000000000000, 0.9659258262890683122, 1.000000000000000000, 0.9659258262890683122, 1.000000000000000000, 0.9659258262890683122, 1.000000000000000000, 0.9659258262890683122, 1.000000000000000000, 0.9659258262890683122, 1.000000000000000000, 0.9659258262890683122, 1.000000000000000000, 0.9659258262890683122, 1.000000000000000000, 0.9659258262890683122, 1.000000000000000000, 0.9659258262890683122, 1.000000000000000000, 0.9659258262890683122, 1.000000000000000000, 0.9659258262890683122, 1.000000000000000000, 0.9659258262890683122, 1.000000000000000000, 0.9659258262890683122, 1.000000000000000000, 0.9659258262890683122, 1.000000000000000000, 0.9659258262890683122, 1.000000000000000000, 0.9659258262890683122, 1.000000000000000000, 0.9659258262890683122, 1.000000000000000000, 0.9659258262890683122, 1.000000000000000000, 0.9659258262890683122, 1.000000000000000000, 0.9659258262890683122, 1.000000000000000000, 0.9659258262890683122, 1.000000000000000000, 0.9659258262890683122, 1.000000000000000000, 0.9659258262890683122, 1.000000000000000000, 0.9659258262890683122, 1.000000000000000000, 0.9659258262890683122, 1.000000000000000000, 0.9659258262890683122, 1.000000000000000000, 0.9659258262890683122, 1.000000000000000000, 0.9659258262890683122, 1.000000000000000000, 0.9659258262890683122, 1.000000000000000000, 0.9659258262890683122, 1.000000000000000000, 0.9659258262890683122, 1.000000000000000000, 0.9659258262890683122, 1.000000000000000000, 0.9659258262890683122, 1.000000000000000000, 0.9659258262890683122, 1.000000000000000000, 0.9659258262890683122, 1.000000000000000000, 0.9659258262890683122, 1.000000000000000000, 0.9659258262890683122, 1.000000000000000000, 0.9659258262890683122, 1.000000000000000000, 0.9659258262890683122, 1.000000000000000000, 0.9659258262890683122, 1.000000000000000000, 0.9659258262890683122, 1.000000000000000000, 0.9659258262890683122, 1.000000000000000000, 0.9659258262890683122, 1.000000000000000000, 0.9659258262890683122, 1.000000000000000000, 0.9659258262890683122, 1.000000000000000000, 0.9659258262890683122, 1.000000000000000000, 0.9659258262890683122, 1.000000000000000000, 0.9659258262890683122, 1.000000000000000000, 0.9659258262890683122, 1.000000000000000000, 0.9659258262890683122, 1.000000000000000000, 0.9659258262890683122, 1.000000000000000000, 0.9659258262890683122, 1.000000000000000000, 0.9659258262890683122, 1.000000000000000000, 0.9659258262890683122, 1.000000000000000000, 0.9659258262890683122, 1.000000000000000000, 0.9659258262890683122, 1.000000000000000000, 0.9659258262890683122, 1.000000000000000000, 0.9659258262890683122, 1.000000000000000000, 0.9659258262890683122, 1.000000000000000000, 0.9659258262890683122, 1.000000000000000000, 0.9659258262890683122, 1.000000000000000000, 0.9659258262890683122, 1.000000000000000000, 0.9659258262890683122, 1.000000000000000000, 0.9659258262890683122, 1.000000000000000000, 0.9659258262890683122, 1.000000000000000000, 0.9659258262890683122, 1.000000000000000000, 0.9659258262890683122, 1.000000000000000000, 0.9659258262890683122, 1.000000000000000000, 0.9659258262890683122, 1.000000000000000000, 0.9659258262890683122, 1.000000000000000000, 0.9659258262890683122, 1.000000000000000000, 0.9659258262890683122, 1.000000000000000000, 0.9659258262890683122, 1.000000000000000000, 0.9659258262890683122, 1.000000000000000000, 0.9659258262890683122, 1.000000000000000000, 0.9659258262890683122, 1.000000000000000000, 0.9659258262890683122, 1.000000000000000000, 0.9659258262890683122, 1.000000000000000000, 0.9659258262890683122, 1.000000000000000000, 0.9659258262890683122, 1.000000000000000000, 0.9659258262890683122, 1.000000000000000000, 0.9659258262890683122, 1.000000000000000000, 0.9659258262890683122, 1.000000000000000000, 0.9659258262890683122, 1.000000000000000000, 0.9659258262890683122, 1.000000000000000000, 0.9659258262890683122, 1.000000000000000000, 0.9659258262890683122, 1.000000000000000000, 0.9659258262890683122, 1.000000000000000000, 0.9659258262890683122, 1.000000000000000000, 0.9659258262890683122, 1.000000000000000000, 0.9659258262890683122, 1.000000000000000000, 0.9659258262890683122, 1.000000000000000000, 0.9659258262890683122, 1.000000000000000000, 0.9659258262890683122, 1.000000000000000000, 0.9659258262890683122, 1.000000000000000000, 0.9659258262890683122, 1.000000000000000000, 0.9659258262890683122, 1.000000000000000000, 0.9659258262890683122, 1.000000000000000000, 0.9659258262890683122, 1.000000000000000000, 0.9659258262890683122, 1.000000000000000000, 0.9659258262890683122, 1.000000000000000000, 0.9659258262890683122, 1.000000000000000000, 0.9659258262890683122, 1.000000000000000000, 0.9659258262890683122, 1.000000000000000000, 0.9659258262890683122, 1.000000000000000000, 0.9659258262890683122, 1.000000000000000000, 0.9659258262890683122, 1.000000000000000000, 0.9659258262890683122, 1.000000000000000000, 0.9659258262890683122, 1.000000000000000000, 0.9659258262890683122, 1.000000000000000000, 0.9659258262890683122, 1.000000000000000000, 0.9659258262890683122, 1.000000000000000000, 0.9659258262890683122, 1.000000000000000000, 0.9659258262890683122, 1.000000000000000000, 0.9659258262890683122, 1.000000000000000000, 0.9659258262890683122, 1.000000000000000000, 0.9659258262890683122, 1.000000000000000000, 0.9659258262890683122, 1.000000000000000000, 0.9659258262890683122, 1.000000000000000000, 0.9659258262890683122, 1.000000000000000000, 0.9659258262890683122, 1.000000000000000000, 0.9659258262890683122, 1.000000000000000000, 0.9659258262890683122, 1.000000000000000000, 0.9659258262890683122, 1.000000000000000000, 0.9659258262890683122, 1.000000000000000000, 0.9659258262890683122, 1.000000000000000000, 0.9659258262890683122, 1.000000000000000000, 0.9659258262890683122, 1.000000000000000000, 0.9659258262890683122, 1.000000000000000000, 0.9659258262890683122, 1.000000000000000000, 0.9659258262890683122, 1.000000000000000000, 0.9659258262890683122, 1.000000000000000000, 0.9659258262890683122, 1.000000000000000000, 0.9659258262890683122, 1.000000000000000000, 0.9659258262890683122, 1.000000000000000000, 0.9659258262890683122, 1.000000000000000000, 0.9659258262890683122, 1.000000000000000000, 0.9659258262890683122, 1.000000000000000000, 0.9659258262890683122, 1.000000000000000000, 0.9659258262890683122, 1.000000000000000000, 0.9659258262890683122, 1.000000000000000000, 0.9659258262890683122, 1.000000000000000000, 0.9659258262890683122, 1.000000000000000000, 0.9659258262890683122, 1.000000000000000000, 0.9659258262890683122, 1.000000000000000000, 0.9659258262890683122, 1.000000000000000000, 0.9659258262890683122, 1.000000000000000000, 0.9659258262890683122, 1.000000000000000000, 0.9659258262890683122, 1.000000000000000000, 0.9659258262890683122, 1.000000000000000000, 0.9659258262890683122, 1.000000000000000000, 0.9659258262890683122, 1.000000000000000000, 0.9659258262890683122, 1.000000000000000000, 0.9659258262890683122, 1.000000000000000000, 0.9659258262890683122, 1.000000000000000000, 0.9659258262890683122, 1.000000000000000000, 0.9659258262890683122, 1.000000000000000000, 0.9659258262890683122, 1.000000000000000000, 0.9659258262890683122, 1.000000000000000000, 0.9659258262890683122, 1.000000000000000000, 0.9659258262890683122, 1.000000000000000000, 0.9659258262890683122, 1.000000000000000000, 0.9659258262890683122, 1.000000000000000000, 0.9659258262890683122, 1.000000000000000000, 0.9659258262890683122, 1.000000000000000000, 0.9659258262890683122, 1.000000000000000000, 0.9659258262890683122, 1.000000000000000000, 0.9659258262890683122, 1.000000000000000000, 0.9659258262890683122, 1.000000000000000000, 0.9659258262890683122, 1.000000000000000000, 0.9659258262890683122, 1.000000000000000000, 0.9659258262890683122, 1.000000000000000000, 0.9659258262890683122, 1.000000000000000000, 0.9659258262890683122, 1.000000000000000000, 0.9659258262890683122, 1.000000000000000000, 0.9659258262890683122, 1.000000000000000000, 0.9659258262890683122, 1.000000000000000000, 0.9659258262890683122, 1.000000000000000000, 0.9659258262890683122, 1.000000000000000000, 0.9659258262890683122, 1.000000000000000000, 0.9659258262890683122, 1.000000000000000000, 0.9659258262890683122, 1.000000000000000000, 0.9659258262890683122, 1.000000000000000000, 0.9659258262890683122, 1.000000000000000000, 0.9659258262890683122, 1.000000000000000000, 0.9659258262890683122, 1.000000000000000000, 0.9659258262890683122, 1.000000000000000000, 0.9659258262890683122, 1.000000000000000000, 0.9659258262890683122, 1.000000000000000000, 0.9659258262890683122, 1.000000000000000000, 0.9659258262890683122, 1.000000000000000000, 0.9659258262890683122, 1.000000000000000000, 0.9659258262890683122, 1.000000000000000000),
 ( 0.3333333333333333703, 0.3219752754296894559, 0.3333333333333333703, 0.3219752754296894559, 0.3333333333333333703, 0.3219752754296894559, 0.3333333333333333703, 0.3219752754296894559, 0.3333333333333333703, 0.3219752754296894559, 0.3333333333333333703, 0.3219752754296894559, 0.3333333333333333703, 0.3219752754296894559, 0.3333333333333333703, 0.3219752754296894559, 0.3333333333333333703, 0.3219752754296894559, 0.3333333333333333703, 0.3219752754296894559, 0.3333333333333333703, 0.3219752754296894559, 0.3333333333333333703, 0.3219752754296894559, 0.3333333333333333703, 0.3219752754296894559, 0.3333333333333333703, 0.3219752754296894559, 0.3333333333333333703, 0.3219752754296894559, 0.3333333333333333703, 0.3219752754296894559, 0.3333333333333333703, 0.3219752754296894559, 0.3333333333333333703, 0.3219752754296894559, 0.3333333333333333703, 0.3219752754296894559, 0.3333333333333333703, 0.3219752754296894559, 0.3333333333333333703, 0.3219752754296894559, 0.3333333333333333703, 0.3219752754296894559, 0.3333333333333333703, 0.3219752754296894559, 0.3333333333333333703, 0.3219752754296894559, 0.3333333333333333703, 0.3219752754296894559, 0.3333333333333333703, 0.3219752754296894559, 0.3333333333333333703, 0.3219752754296894559, 0.3333333333333333703, 0.3219752754296894559, 0.3333333333333333703, 0.3219752754296894559, 0.3333333333333333703, 0.3219752754296894559, 0.3333333333333333703, 0.3219752754296894559, 0.3333333333333333703, 0.3219752754296894559, 0.3333333333333333703, 0.3219752754296894559, 0.3333333333333333703, 0.3219752754296894559, 0.3333333333333333703, 0.3219752754296894559, 0.3333333333333333703, 0.3219752754296894559, 0.3333333333333333703, 0.3219752754296894559, 0.3333333333333333703, 0.3219752754296894559, 0.3333333333333333703, 0.3219752754296894559, 0.3333333333333333703, 0.3219752754296894559, 0.3333333333333333703, 0.3219752754296894559, 0.3333333333333333703, 0.3219752754296894559, 0.3333333333333333703, 0.3219752754296894559, 0.3333333333333333703, 0.3219752754296894559, 0.3333333333333333703, 0.3219752754296894559, 0.3333333333333333703, 0.3219752754296894559, 0.3333333333333333703, 0.3219752754296894559, 0.3333333333333333703, 0.3219752754296894559, 0.3333333333333333703, 0.3219752754296894559, 0.3333333333333333703, 0.3219752754296894559, 0.3333333333333333703, 0.3219752754296894559, 0.3333333333333333703, 0.3219752754296894559, 0.3333333333333333703, 0.3219752754296894559, 0.3333333333333333703, 0.3219752754296894559, 0.3333333333333333703, 0.3219752754296894559, 0.3333333333333333703, 0.3219752754296894559, 0.3333333333333333703, 0.3219752754296894559, 0.3333333333333333703, 0.3219752754296894559, 0.3333333333333333703, 0.3219752754296894559, 0.3333333333333333703, 0.3219752754296894559, 0.3333333333333333703, 0.3219752754296894559, 0.3333333333333333703, 0.3219752754296894559, 0.3333333333333333703, 0.3219752754296894559, 0.3333333333333333703, 0.3219752754296894559, 0.3333333333333333703, 0.3219752754296894559, 0.3333333333333333703, 0.3219752754296894559, 0.3333333333333333703, 0.3219752754296894559, 0.3333333333333333703, 0.3219752754296894559, 0.3333333333333333703, 0.3219752754296894559, 0.3333333333333333703, 0.3219752754296894559, 0.3333333333333333703, 0.3219752754296894559, 0.3333333333333333703, 0.3219752754296894559, 0.3333333333333333703, 0.3219752754296894559, 0.3333333333333333703, 0.3219752754296894559, 0.3333333333333333703, 0.3219752754296894559, 0.3333333333333333703, 0.3219752754296894559, 0.3333333333333333703, 0.3219752754296894559, 0.3333333333333333703, 0.3219752754296894559, 0.3333333333333333703, 0.3219752754296894559, 0.3333333333333333703, 0.3219752754296894559, 0.3333333333333333703, 0.3219752754296894559, 0.3333333333333333703, 0.3219752754296894559, 0.3333333333333333703, 0.3219752754296894559, 0.3333333333333333703, 0.3219752754296894559, 0.3333333333333333703, 0.3219752754296894559, 0.3333333333333333703, 0.3219752754296894559, 0.3333333333333333703, 0.3219752754296894559, 0.3333333333333333703, 0.3219752754296894559, 0.3333333333333333703, 0.3219752754296894559, 0.3333333333333333703, 0.3219752754296894559, 0.3333333333333333703, 0.3219752754296894559, 0.3333333333333333703, 0.3219752754296894559, 0.3333333333333333703, 0.3219752754296894559, 0.3333333333333333703, 0.3219752754296894559, 0.3333333333333333703, 0.3219752754296894559, 0.3333333333333333703, 0.3219752754296894559, 0.3333333333333333703, 0.3219752754296894559, 0.3333333333333333703, 0.3219752754296894559, 0.3333333333333333703, 0.3219752754296894559, 0.3333333333333333703, 0.3219752754296894559, 0.3333333333333333703, 0.3219752754296894559, 0.3333333333333333703, 0.3219752754296894559, 0.3333333333333333703, 0.3219752754296894559, 0.3333333333333333703, 0.3219752754296894559, 0.3333333333333333703, 0.3219752754296894559, 0.3333333333333333703, 0.3219752754296894559, 0.3333333333333333703, 0.3219752754296894559, 0.3333333333333333703, 0.3219752754296894559, 0.3333333333333333703, 0.3219752754296894559, 0.3333333333333333703, 0.3219752754296894559, 0.3333333333333333703, 0.3219752754296894559, 0.3333333333333333703, 0.3219752754296894559, 0.3333333333333333703, 0.3219752754296894559, 0.3333333333333333703, 0.3219752754296894559, 0.3333333333333333703, 0.3219752754296894559, 0.3333333333333333703, 0.3219752754296894559, 0.3333333333333333703, 0.3219752754296894559, 0.3333333333333333703, 0.3219752754296894559, 0.3333333333333333703, 0.3219752754296894559, 0.3333333333333333703, 0.3219752754296894559, 0.3333333333333333703, 0.3219752754296894559, 0.3333333333333333703, 0.3219752754296894559, 0.3333333333333333703, 0.3219752754296894559, 0.3333333333333333703, 0.3219752754296894559, 0.3333333333333333703, 0.3219752754296894559, 0.3333333333333333703, 0.3219752754296894559, 0.3333333333333333703, 0.3219752754296894559, 0.3333333333333333703, 0.3219752754296894559, 0.3333333333333333703, 0.3219752754296894559, 0.3333333333333333703, 0.3219752754296894559, 0.3333333333333333703, 0.3219752754296894559, 0.3333333333333333703, 0.3219752754296894559, 0.3333333333333333703, 0.3219752754296894559, 0.3333333333333333703, 0.3219752754296894559, 0.3333333333333333703, 0.3219752754296894559, 0.3333333333333333703, 0.3219752754296894559, 0.3333333333333333703, 0.3219752754296894559, 0.3333333333333333703, 0.3219752754296894559, 0.3333333333333333703, 0.3219752754296894559, 0.3333333333333333703, 0.3219752754296894559, 0.3333333333333333703, 0.3219752754296894559, 0.3333333333333333703, 0.3219752754296894559, 0.3333333333333333703, 0.3219752754296894559, 0.3333333333333333703, 0.3219752754296894559, 0.3333333333333333703, 0.3219752754296894559, 0.3333333333333333703, 0.3219752754296894559, 0.3333333333333333703, 0.3219752754296894559, 0.3333333333333333703, 0.3219752754296894559, 0.3333333333333333703, 0.3219752754296894559, 0.3333333333333333703, 0.3219752754296894559, 0.3333333333333333703, 0.3219752754296894559, 0.3333333333333333703, 0.3219752754296894559, 0.3333333333333333703, 0.3219752754296894559, 0.3333333333333333703, 0.3219752754296894559, 0.3333333333333333703, 0.3219752754296894559, 0.3333333333333333703, 0.3219752754296894559, 0.3333333333333333703, 0.3219752754296894559, 0.3333333333333333703, 0.3219752754296894559, 0.3333333333333333703, 0.3219752754296894559, 0.3333333333333333703, 0.3219752754296894559, 0.3333333333333333703, 0.3219752754296894559, 0.3333333333333333703, 0.3219752754296894559, 0.3333333333333333703, 0.3219752754296894559, 0.3333333333333333703, 0.3219752754296894559, 0.3333333333333333703, 0.3219752754296894559, 0.3333333333333333703, 0.3219752754296894559, 0.3333333333333333703, 0.3219752754296894559, 0.3333333333333333703, 0.3219752754296894559, 0.3333333333333333703, 0.3219752754296894559, 0.3333333333333333703, 0.3219752754296894559, 0.3333333333333333703, 0.3219752754296894559, 0.3333333333333333703, 0.3219752754296894559, 0.3333333333333333703, 0.3219752754296894559, 0.3333333333333333703, 0.3219752754296894559, 0.3333333333333333703, 0.3219752754296894559, 0.3333333333333333703, 0.3219752754296894559, 0.3333333333333333703, 0.3219752754296894559, 0.3333333333333333703, 0.3219752754296894559, 0.3333333333333333703, 0.3219752754296894559, 0.3333333333333333703, 0.3219752754296894559, 0.3333333333333333703, 0.3219752754296894559, 0.3333333333333333703, 0.3219752754296894559, 0.3333333333333333703, 0.3219752754296894559, 0.3333333333333333703, 0.3219752754296894559, 0.3333333333333333703, 0.3219752754296894559, 0.3333333333333333703, 0.3219752754296894559, 0.3333333333333333703, 0.3219752754296894559, 0.3333333333333333703, 0.3219752754296894559, 0.3333333333333333703, 0.3219752754296894559, 0.3333333333333333703, 0.3219752754296894559, 0.3333333333333333703, 0.3219752754296894559, 0.3333333333333333703, 0.3219752754296894559, 0.3333333333333333703, 0.3219752754296894559, 0.3333333333333333703, 0.3219752754296894559, 0.3333333333333333703, 0.3219752754296894559, 0.3333333333333333703, 0.3219752754296894559, 0.3333333333333333703, 0.3219752754296894559, 0.3333333333333333703, 0.3219752754296894559, 0.3333333333333333703, 0.3219752754296894559, 0.3333333333333333703, 0.3219752754296894559, 0.3333333333333333703, 0.3219752754296894559, 0.3333333333333333703, 0.3219752754296894559, 0.3333333333333333703, 0.3219752754296894559, 0.3333333333333333703, 0.3219752754296894559, 0.3333333333333333703, 0.3219752754296894559, 0.3333333333333333703, 0.3219752754296894559, 0.3333333333333333703, 0.3219752754296894559, 0.3333333333333333703, 0.3219752754296894559, 0.3333333333333333703, 0.3219752754296894559, 0.3333333333333333703, 0.3219752754296894559, 0.3333333333333333703, 0.3219752754296894559, 0.3333333333333333703, 0.3219752754296894559, 0.3333333333333333703, 0.3219752754296894559, 0.3333333333333333703, 0.3219752754296894559, 0.3333333333333333703, 0.3219752754296894559, 0.3333333333333333703, 0.3219752754296894559, 0.3333333333333333703, 0.3219752754296894559, 0.3333333333333333703, 0.3219752754296894559, 0.3333333333333333703, 0.3219752754296894559, 0.3333333333333333703, 0.3219752754296894559, 0.3333333333333333703, 0.3219752754296894559, 0.3333333333333333703, 0.3219752754296894559, 0.3333333333333333703, 0.3219752754296894559, 0.3333333333333333703, 0.3219752754296894559, 0.3333333333333333703, 0.3219752754296894559, 0.3333333333333333703, 0.3219752754296894559, 0.3333333333333333703, 0.3219752754296894559, 0.3333333333333333703, 0.3219752754296894559, 0.3333333333333333703),
 ( 0.3333333333333333703, 0.3219752754296894559, 0.3333333333333333703, 0.3219752754296894559, 0.3333333333333333703, 0.3219752754296894559, 0.3333333333333333703, 0.3219752754296894559, 0.3333333333333333703, 0.3219752754296894559, 0.3333333333333333703, 0.3219752754296894559, 0.3333333333333333703, 0.3219752754296894559, 0.3333333333333333703, 0.3219752754296894559, 0.3333333333333333703, 0.3219752754296894559, 0.3333333333333333703, 0.3219752754296894559, 0.3333333333333333703, 0.3219752754296894559, 0.3333333333333333703, 0.3219752754296894559, 0.3333333333333333703, 0.3219752754296894559, 0.3333333333333333703, 0.3219752754296894559, 0.3333333333333333703, 0.3219752754296894559, 0.3333333333333333703, 0.3219752754296894559, 0.3333333333333333703, 0.3219752754296894559, 0.3333333333333333703, 0.3219752754296894559, 0.3333333333333333703, 0.3219752754296894559, 0.3333333333333333703, 0.3219752754296894559, 0.3333333333333333703, 0.3219752754296894559, 0.3333333333333333703, 0.3219752754296894559, 0.3333333333333333703, 0.3219752754296894559, 0.3333333333333333703, 0.3219752754296894559, 0.3333333333333333703, 0.3219752754296894559, 0.3333333333333333703, 0.3219752754296894559, 0.3333333333333333703, 0.3219752754296894559, 0.3333333333333333703, 0.3219752754296894559, 0.3333333333333333703, 0.3219752754296894559, 0.3333333333333333703, 0.3219752754296894559, 0.3333333333333333703, 0.3219752754296894559, 0.3333333333333333703, 0.3219752754296894559, 0.3333333333333333703, 0.3219752754296894559, 0.3333333333333333703, 0.3219752754296894559, 0.3333333333333333703, 0.3219752754296894559, 0.3333333333333333703, 0.3219752754296894559, 0.3333333333333333703, 0.3219752754296894559, 0.3333333333333333703, 0.3219752754296894559, 0.3333333333333333703, 0.3219752754296894559, 0.3333333333333333703, 0.3219752754296894559, 0.3333333333333333703, 0.3219752754296894559, 0.3333333333333333703, 0.3219752754296894559, 0.3333333333333333703, 0.3219752754296894559, 0.3333333333333333703, 0.3219752754296894559, 0.3333333333333333703, 0.3219752754296894559, 0.3333333333333333703, 0.3219752754296894559, 0.3333333333333333703, 0.3219752754296894559, 0.3333333333333333703, 0.3219752754296894559, 0.3333333333333333703, 0.3219752754296894559, 0.3333333333333333703, 0.3219752754296894559, 0.3333333333333333703, 0.3219752754296894559, 0.3333333333333333703, 0.3219752754296894559, 0.3333333333333333703, 0.3219752754296894559, 0.3333333333333333703, 0.3219752754296894559, 0.3333333333333333703, 0.3219752754296894559, 0.3333333333333333703, 0.3219752754296894559, 0.3333333333333333703, 0.3219752754296894559, 0.3333333333333333703, 0.3219752754296894559, 0.3333333333333333703, 0.3219752754296894559, 0.3333333333333333703, 0.3219752754296894559, 0.3333333333333333703, 0.3219752754296894559, 0.3333333333333333703, 0.3219752754296894559, 0.3333333333333333703, 0.3219752754296894559, 0.3333333333333333703, 0.3219752754296894559, 0.3333333333333333703, 0.3219752754296894559, 0.3333333333333333703, 0.3219752754296894559, 0.3333333333333333703, 0.3219752754296894559, 0.3333333333333333703, 0.3219752754296894559, 0.3333333333333333703, 0.3219752754296894559, 0.3333333333333333703, 0.3219752754296894559, 0.3333333333333333703, 0.3219752754296894559, 0.3333333333333333703, 0.3219752754296894559, 0.3333333333333333703, 0.3219752754296894559, 0.3333333333333333703, 0.3219752754296894559, 0.3333333333333333703, 0.3219752754296894559, 0.3333333333333333703, 0.3219752754296894559, 0.3333333333333333703, 0.3219752754296894559, 0.3333333333333333703, 0.3219752754296894559, 0.3333333333333333703, 0.3219752754296894559, 0.3333333333333333703, 0.3219752754296894559, 0.3333333333333333703, 0.3219752754296894559, 0.3333333333333333703, 0.3219752754296894559, 0.3333333333333333703, 0.3219752754296894559, 0.3333333333333333703, 0.3219752754296894559, 0.3333333333333333703, 0.3219752754296894559, 0.3333333333333333703, 0.3219752754296894559, 0.3333333333333333703, 0.3219752754296894559, 0.3333333333333333703, 0.3219752754296894559, 0.3333333333333333703, 0.3219752754296894559, 0.3333333333333333703, 0.3219752754296894559, 0.3333333333333333703, 0.3219752754296894559, 0.3333333333333333703, 0.3219752754296894559, 0.3333333333333333703, 0.3219752754296894559, 0.3333333333333333703, 0.3219752754296894559, 0.3333333333333333703, 0.3219752754296894559, 0.3333333333333333703, 0.3219752754296894559, 0.3333333333333333703, 0.3219752754296894559, 0.3333333333333333703, 0.3219752754296894559, 0.3333333333333333703, 0.3219752754296894559, 0.3333333333333333703, 0.3219752754296894559, 0.3333333333333333703, 0.3219752754296894559, 0.3333333333333333703, 0.3219752754296894559, 0.3333333333333333703, 0.3219752754296894559, 0.3333333333333333703, 0.3219752754296894559, 0.3333333333333333703, 0.3219752754296894559, 0.3333333333333333703, 0.3219752754296894559, 0.3333333333333333703, 0.3219752754296894559, 0.3333333333333333703, 0.3219752754296894559, 0.3333333333333333703, 0.3219752754296894559, 0.3333333333333333703, 0.3219752754296894559, 0.3333333333333333703, 0.3219752754296894559, 0.3333333333333333703, 0.3219752754296894559, 0.3333333333333333703, 0.3219752754296894559, 0.3333333333333333703, 0.3219752754296894559, 0.3333333333333333703, 0.3219752754296894559, 0.3333333333333333703, 0.3219752754296894559, 0.3333333333333333703, 0.3219752754296894559, 0.3333333333333333703, 0.3219752754296894559, 0.3333333333333333703, 0.3219752754296894559, 0.3333333333333333703, 0.3219752754296894559, 0.3333333333333333703, 0.3219752754296894559, 0.3333333333333333703, 0.3219752754296894559, 0.3333333333333333703, 0.3219752754296894559, 0.3333333333333333703, 0.3219752754296894559, 0.3333333333333333703, 0.3219752754296894559, 0.3333333333333333703, 0.3219752754296894559, 0.3333333333333333703, 0.3219752754296894559, 0.3333333333333333703, 0.3219752754296894559, 0.3333333333333333703, 0.3219752754296894559, 0.3333333333333333703, 0.3219752754296894559, 0.3333333333333333703, 0.3219752754296894559, 0.3333333333333333703, 0.3219752754296894559, 0.3333333333333333703, 0.3219752754296894559, 0.3333333333333333703, 0.3219752754296894559, 0.3333333333333333703, 0.3219752754296894559, 0.3333333333333333703, 0.3219752754296894559, 0.3333333333333333703, 0.3219752754296894559, 0.3333333333333333703, 0.3219752754296894559, 0.3333333333333333703, 0.3219752754296894559, 0.3333333333333333703, 0.3219752754296894559, 0.3333333333333333703, 0.3219752754296894559, 0.3333333333333333703, 0.3219752754296894559, 0.3333333333333333703, 0.3219752754296894559, 0.3333333333333333703, 0.3219752754296894559, 0.3333333333333333703, 0.3219752754296894559, 0.3333333333333333703, 0.3219752754296894559, 0.3333333333333333703, 0.3219752754296894559, 0.3333333333333333703, 0.3219752754296894559, 0.3333333333333333703, 0.3219752754296894559, 0.3333333333333333703, 0.3219752754296894559, 0.3333333333333333703, 0.3219752754296894559, 0.3333333333333333703, 0.3219752754296894559, 0.3333333333333333703, 0.3219752754296894559, 0.3333333333333333703, 0.3219752754296894559, 0.3333333333333333703, 0.3219752754296894559, 0.3333333333333333703, 0.3219752754296894559, 0.3333333333333333703, 0.3219752754296894559, 0.3333333333333333703, 0.3219752754296894559, 0.3333333333333333703, 0.3219752754296894559, 0.3333333333333333703, 0.3219752754296894559, 0.3333333333333333703, 0.3219752754296894559, 0.3333333333333333703, 0.3219752754296894559, 0.3333333333333333703, 0.3219752754296894559, 0.3333333333333333703, 0.3219752754296894559, 0.3333333333333333703, 0.3219752754296894559, 0.3333333333333333703, 0.3219752754296894559, 0.3333333333333333703, 0.3219752754296894559, 0.3333333333333333703, 0.3219752754296894559, 0.3333333333333333703, 0.3219752754296894559, 0.3333333333333333703, 0.3219752754296894559, 0.3333333333333333703, 0.3219752754296894559, 0.3333333333333333703, 0.3219752754296894559, 0.3333333333333333703, 0.3219752754296894559, 0.3333333333333333703, 0.3219752754296894559, 0.3333333333333333703, 0.3219752754296894559, 0.3333333333333333703, 0.3219752754296894559, 0.3333333333333333703, 0.3219752754296894559, 0.3333333333333333703, 0.3219752754296894559, 0.3333333333333333703, 0.3219752754296894559, 0.3333333333333333703, 0.3219752754296894559, 0.3333333333333333703, 0.3219752754296894559, 0.3333333333333333703, 0.3219752754296894559, 0.3333333333333333703, 0.3219752754296894559, 0.3333333333333333703, 0.3219752754296894559, 0.3333333333333333703, 0.3219752754296894559, 0.3333333333333333703, 0.3219752754296894559, 0.3333333333333333703, 0.3219752754296894559, 0.3333333333333333703, 0.3219752754296894559, 0.3333333333333333703, 0.3219752754296894559, 0.3333333333333333703, 0.3219752754296894559, 0.3333333333333333703, 0.3219752754296894559, 0.3333333333333333703, 0.3219752754296894559, 0.3333333333333333703, 0.3219752754296894559, 0.3333333333333333703, 0.3219752754296894559, 0.3333333333333333703, 0.3219752754296894559, 0.3333333333333333703, 0.3219752754296894559, 0.3333333333333333703, 0.3219752754296894559, 0.3333333333333333703, 0.3219752754296894559, 0.3333333333333333703, 0.3219752754296894559, 0.3333333333333333703, 0.3219752754296894559, 0.3333333333333333703, 0.3219752754296894559, 0.3333333333333333703, 0.3219752754296894559, 0.3333333333333333703, 0.3219752754296894559, 0.3333333333333333703, 0.3219752754296894559, 0.3333333333333333703, 0.3219752754296894559, 0.3333333333333333703, 0.3219752754296894559, 0.3333333333333333703, 0.3219752754296894559, 0.3333333333333333703, 0.3219752754296894559, 0.3333333333333333703, 0.3219752754296894559, 0.3333333333333333703, 0.3219752754296894559, 0.3333333333333333703, 0.3219752754296894559, 0.3333333333333333703, 0.3219752754296894559, 0.3333333333333333703, 0.3219752754296894559, 0.3333333333333333703, 0.3219752754296894559, 0.3333333333333333703, 0.3219752754296894559, 0.3333333333333333703, 0.3219752754296894559, 0.3333333333333333703, 0.3219752754296894559, 0.3333333333333333703, 0.3219752754296894559, 0.3333333333333333703, 0.3219752754296894559, 0.3333333333333333703, 0.3219752754296894559, 0.3333333333333333703, 0.3219752754296894559, 0.3333333333333333703, 0.3219752754296894559, 0.3333333333333333703, 0.3219752754296894559, 0.3333333333333333703, 0.3219752754296894559, 0.3333333333333333703, 0.3219752754296894559, 0.3333333333333333703, 0.3219752754296894559, 0.3333333333333333703, 0.3219752754296894559, 0.3333333333333333703, 0.3219752754296894559, 0.3333333333333333703),
 ( 1.000000000000000000, 0.9659258262890683122, 1.000000000000000000, 0.9659258262890683122, 1.000000000000000000, 0.9659258262890683122, 1.000000000000000000, 0.9659258262890683122, 1.000000000000000000, 0.9659258262890683122, 1.000000000000000000, 0.9659258262890683122, 1.000000000000000000, 0.9659258262890683122, 1.000000000000000000, 0.9659258262890683122, 1.000000000000000000, 0.9659258262890683122, 1.000000000000000000, 0.9659258262890683122, 1.000000000000000000, 0.9659258262890683122, 1.000000000000000000, 0.9659258262890683122, 1.000000000000000000, 0.9659258262890683122, 1.000000000000000000, 0.9659258262890683122, 1.000000000000000000, 0.9659258262890683122, 1.000000000000000000, 0.9659258262890683122, 1.000000000000000000, 0.9659258262890683122, 1.000000000000000000, 0.9659258262890683122, 1.000000000000000000, 0.9659258262890683122, 1.000000000000000000, 0.9659258262890683122, 1.000000000000000000, 0.9659258262890683122, 1.000000000000000000, 0.9659258262890683122, 1.000000000000000000, 0.9659258262890683122, 1.000000000000000000, 0.9659258262890683122, 1.000000000000000000, 0.9659258262890683122, 1.000000000000000000, 0.9659258262890683122, 1.000000000000000000, 0.9659258262890683122, 1.000000000000000000, 0.9659258262890683122, 1.000000000000000000, 0.9659258262890683122, 1.000000000000000000, 0.9659258262890683122, 1.000000000000000000, 0.9659258262890683122, 1.000000000000000000, 0.9659258262890683122, 1.000000000000000000, 0.9659258262890683122, 1.000000000000000000, 0.9659258262890683122, 1.000000000000000000, 0.9659258262890683122, 1.000000000000000000, 0.9659258262890683122, 1.000000000000000000, 0.9659258262890683122, 1.000000000000000000, 0.9659258262890683122, 1.000000000000000000, 0.9659258262890683122, 1.000000000000000000, 0.9659258262890683122, 1.000000000000000000, 0.9659258262890683122, 1.000000000000000000, 0.9659258262890683122, 1.000000000000000000, 0.9659258262890683122, 1.000000000000000000, 0.9659258262890683122, 1.000000000000000000, 0.9659258262890683122, 1.000000000000000000, 0.9659258262890683122, 1.000000000000000000, 0.9659258262890683122, 1.000000000000000000, 0.9659258262890683122, 1.000000000000000000, 0.9659258262890683122, 1.000000000000000000, 0.9659258262890683122, 1.000000000000000000, 0.9659258262890683122, 1.000000000000000000, 0.9659258262890683122, 1.000000000000000000, 0.9659258262890683122, 1.000000000000000000, 0.9659258262890683122, 1.000000000000000000, 0.9659258262890683122, 1.000000000000000000, 0.9659258262890683122, 1.000000000000000000, 0.9659258262890683122, 1.000000000000000000, 0.9659258262890683122, 1.000000000000000000, 0.9659258262890683122, 1.000000000000000000, 0.9659258262890683122, 1.000000000000000000, 0.9659258262890683122, 1.000000000000000000, 0.9659258262890683122, 1.000000000000000000, 0.9659258262890683122, 1.000000000000000000, 0.9659258262890683122, 1.000000000000000000, 0.9659258262890683122, 1.000000000000000000, 0.9659258262890683122, 1.000000000000000000, 0.9659258262890683122, 1.000000000000000000, 0.9659258262890683122, 1.000000000000000000, 0.9659258262890683122, 1.000000000000000000, 0.9659258262890683122, 1.000000000000000000, 0.9659258262890683122, 1.000000000000000000, 0.9659258262890683122, 1.000000000000000000, 0.9659258262890683122, 1.000000000000000000, 0.9659258262890683122, 1.000000000000000000, 0.9659258262890683122, 1.000000000000000000, 0.9659258262890683122, 1.000000000000000000, 0.9659258262890683122, 1.000000000000000000, 0.9659258262890683122, 1.000000000000000000, 0.9659258262890683122, 1.000000000000000000, 0.9659258262890683122, 1.000000000000000000, 0.9659258262890683122, 1.000000000000000000, 0.9659258262890683122, 1.000000000000000000, 0.9659258262890683122, 1.000000000000000000, 0.9659258262890683122, 1.000000000000000000, 0.9659258262890683122, 1.000000000000000000, 0.9659258262890683122, 1.000000000000000000, 0.9659258262890683122, 1.000000000000000000, 0.9659258262890683122, 1.000000000000000000, 0.9659258262890683122, 1.000000000000000000, 0.9659258262890683122, 1.000000000000000000, 0.9659258262890683122, 1.000000000000000000, 0.9659258262890683122, 1.000000000000000000, 0.9659258262890683122, 1.000000000000000000, 0.9659258262890683122, 1.000000000000000000, 0.9659258262890683122, 1.000000000000000000, 0.9659258262890683122, 1.000000000000000000, 0.9659258262890683122, 1.000000000000000000, 0.9659258262890683122, 1.000000000000000000, 0.9659258262890683122, 1.000000000000000000, 0.9659258262890683122, 1.000000000000000000, 0.9659258262890683122, 1.000000000000000000, 0.9659258262890683122, 1.000000000000000000, 0.9659258262890683122, 1.000000000000000000, 0.9659258262890683122, 1.000000000000000000, 0.9659258262890683122, 1.000000000000000000, 0.9659258262890683122, 1.000000000000000000, 0.9659258262890683122, 1.000000000000000000, 0.9659258262890683122, 1.000000000000000000, 0.9659258262890683122, 1.000000000000000000, 0.9659258262890683122, 1.000000000000000000, 0.9659258262890683122, 1.000000000000000000, 0.9659258262890683122, 1.000000000000000000, 0.9659258262890683122, 1.000000000000000000, 0.9659258262890683122, 1.000000000000000000, 0.9659258262890683122, 1.000000000000000000, 0.9659258262890683122, 1.000000000000000000, 0.9659258262890683122, 1.000000000000000000, 0.9659258262890683122, 1.000000000000000000, 0.9659258262890683122, 1.000000000000000000, 0.9659258262890683122, 1.000000000000000000, 0.9659258262890683122, 1.000000000000000000, 0.9659258262890683122, 1.000000000000000000, 0.9659258262890683122, 1.000000000000000000, 0.9659258262890683122, 1.000000000000000000, 0.9659258262890683122, 1.000000000000000000, 0.9659258262890683122, 1.000000000000000000, 0.9659258262890683122, 1.000000000000000000, 0.9659258262890683122, 1.000000000000000000, 0.9659258262890683122, 1.000000000000000000, 0.9659258262890683122, 1.000000000000000000, 0.9659258262890683122, 1.000000000000000000, 0.9659258262890683122, 1.000000000000000000, 0.9659258262890683122, 1.000000000000000000, 0.9659258262890683122, 1.000000000000000000, 0.9659258262890683122, 1.000000000000000000, 0.9659258262890683122, 1.000000000000000000, 0.9659258262890683122, 1.000000000000000000, 0.9659258262890683122, 1.000000000000000000, 0.9659258262890683122, 1.000000000000000000, 0.9659258262890683122, 1.000000000000000000, 0.9659258262890683122, 1.000000000000000000, 0.9659258262890683122, 1.000000000000000000, 0.9659258262890683122, 1.000000000000000000, 0.9659258262890683122, 1.000000000000000000, 0.9659258262890683122, 1.000000000000000000, 0.9659258262890683122, 1.000000000000000000, 0.9659258262890683122, 1.000000000000000000, 0.9659258262890683122, 1.000000000000000000, 0.9659258262890683122, 1.000000000000000000, 0.9659258262890683122, 1.000000000000000000, 0.9659258262890683122, 1.000000000000000000, 0.9659258262890683122, 1.000000000000000000, 0.9659258262890683122, 1.000000000000000000, 0.9659258262890683122, 1.000000000000000000, 0.9659258262890683122, 1.000000000000000000, 0.9659258262890683122, 1.000000000000000000, 0.9659258262890683122, 1.000000000000000000, 0.9659258262890683122, 1.000000000000000000, 0.9659258262890683122, 1.000000000000000000, 0.9659258262890683122, 1.000000000000000000, 0.9659258262890683122, 1.000000000000000000, 0.9659258262890683122, 1.000000000000000000, 0.9659258262890683122, 1.000000000000000000, 0.9659258262890683122, 1.000000000000000000, 0.9659258262890683122, 1.000000000000000000, 0.9659258262890683122, 1.000000000000000000, 0.9659258262890683122, 1.000000000000000000, 0.9659258262890683122, 1.000000000000000000, 0.9659258262890683122, 1.000000000000000000, 0.9659258262890683122, 1.000000000000000000, 0.9659258262890683122, 1.000000000000000000, 0.9659258262890683122, 1.000000000000000000, 0.9659258262890683122, 1.000000000000000000, 0.9659258262890683122, 1.000000000000000000, 0.9659258262890683122, 1.000000000000000000, 0.9659258262890683122, 1.000000000000000000, 0.9659258262890683122, 1.000000000000000000, 0.9659258262890683122, 1.000000000000000000, 0.9659258262890683122, 1.000000000000000000, 0.9659258262890683122, 1.000000000000000000, 0.9659258262890683122, 1.000000000000000000, 0.9659258262890683122, 1.000000000000000000, 0.9659258262890683122, 1.000000000000000000, 0.9659258262890683122, 1.000000000000000000, 0.9659258262890683122, 1.000000000000000000, 0.9659258262890683122, 1.000000000000000000, 0.9659258262890683122, 1.000000000000000000, 0.9659258262890683122, 1.000000000000000000, 0.9659258262890683122, 1.000000000000000000, 0.9659258262890683122, 1.000000000000000000, 0.9659258262890683122, 1.000000000000000000, 0.9659258262890683122, 1.000000000000000000, 0.9659258262890683122, 1.000000000000000000, 0.9659258262890683122, 1.000000000000000000, 0.9659258262890683122, 1.000000000000000000, 0.9659258262890683122, 1.000000000000000000, 0.9659258262890683122, 1.000000000000000000, 0.9659258262890683122, 1.000000000000000000, 0.9659258262890683122, 1.000000000000000000, 0.9659258262890683122, 1.000000000000000000, 0.9659258262890683122, 1.000000000000000000, 0.9659258262890683122, 1.000000000000000000, 0.9659258262890683122, 1.000000000000000000, 0.9659258262890683122, 1.000000000000000000, 0.9659258262890683122, 1.000000000000000000, 0.9659258262890683122, 1.000000000000000000, 0.9659258262890683122, 1.000000000000000000, 0.9659258262890683122, 1.000000000000000000, 0.9659258262890683122, 1.000000000000000000, 0.9659258262890683122, 1.000000000000000000, 0.9659258262890683122, 1.000000000000000000, 0.9659258262890683122, 1.000000000000000000, 0.9659258262890683122, 1.000000000000000000, 0.9659258262890683122, 1.000000000000000000, 0.9659258262890683122, 1.000000000000000000, 0.9659258262890683122, 1.000000000000000000, 0.9659258262890683122, 1.000000000000000000, 0.9659258262890683122, 1.000000000000000000, 0.9659258262890683122, 1.000000000000000000, 0.9659258262890683122, 1.000000000000000000, 0.9659258262890683122, 1.000000000000000000, 0.9659258262890683122, 1.000000000000000000, 0.9659258262890683122, 1.000000000000000000, 0.9659258262890683122, 1.000000000000000000, 0.9659258262890683122, 1.000000000000000000, 0.9659258262890683122, 1.000000000000000000, 0.9659258262890683122, 1.000000000000000000, 0.9659258262890683122, 1.000000000000000000),
 ( 0.3333333333333333703, 0.3219752754296894559, 0.3333333333333333703, 0.3219752754296894559, 0.3333333333333333703, 0.3219752754296894559, 0.3333333333333333703, 0.3219752754296894559, 0.3333333333333333703, 0.3219752754296894559, 0.3333333333333333703, 0.3219752754296894559, 0.3333333333333333703, 0.3219752754296894559, 0.3333333333333333703, 0.3219752754296894559, 0.3333333333333333703, 0.3219752754296894559, 0.3333333333333333703, 0.3219752754296894559, 0.3333333333333333703, 0.3219752754296894559, 0.3333333333333333703, 0.3219752754296894559, 0.3333333333333333703, 0.3219752754296894559, 0.3333333333333333703, 0.3219752754296894559, 0.3333333333333333703, 0.3219752754296894559, 0.3333333333333333703, 0.3219752754296894559, 0.3333333333333333703, 0.3219752754296894559, 0.3333333333333333703, 0.3219752754296894559, 0.3333333333333333703, 0.3219752754296894559, 0.3333333333333333703, 0.3219752754296894559, 0.3333333333333333703, 0.3219752754296894559, 0.3333333333333333703, 0.3219752754296894559, 0.3333333333333333703, 0.3219752754296894559, 0.3333333333333333703, 0.3219752754296894559, 0.3333333333333333703, 0.3219752754296894559, 0.3333333333333333703, 0.3219752754296894559, 0.3333333333333333703, 0.3219752754296894559, 0.3333333333333333703, 0.3219752754296894559, 0.3333333333333333703, 0.3219752754296894559, 0.3333333333333333703, 0.3219752754296894559, 0.3333333333333333703, 0.3219752754296894559, 0.3333333333333333703, 0.3219752754296894559, 0.3333333333333333703, 0.3219752754296894559, 0.3333333333333333703, 0.3219752754296894559, 0.3333333333333333703, 0.3219752754296894559, 0.3333333333333333703, 0.3219752754296894559, 0.3333333333333333703, 0.3219752754296894559, 0.3333333333333333703, 0.3219752754296894559, 0.3333333333333333703, 0.3219752754296894559, 0.3333333333333333703, 0.3219752754296894559, 0.3333333333333333703, 0.3219752754296894559, 0.3333333333333333703, 0.3219752754296894559, 0.3333333333333333703, 0.3219752754296894559, 0.3333333333333333703, 0.3219752754296894559, 0.3333333333333333703, 0.3219752754296894559, 0.3333333333333333703, 0.3219752754296894559, 0.3333333333333333703, 0.3219752754296894559, 0.3333333333333333703, 0.3219752754296894559, 0.3333333333333333703, 0.3219752754296894559, 0.3333333333333333703, 0.3219752754296894559, 0.3333333333333333703, 0.3219752754296894559, 0.3333333333333333703, 0.3219752754296894559, 0.3333333333333333703, 0.3219752754296894559, 0.3333333333333333703, 0.3219752754296894559, 0.3333333333333333703, 0.3219752754296894559, 0.3333333333333333703, 0.3219752754296894559, 0.3333333333333333703, 0.3219752754296894559, 0.3333333333333333703, 0.3219752754296894559, 0.3333333333333333703, 0.3219752754296894559, 0.3333333333333333703, 0.3219752754296894559, 0.3333333333333333703, 0.3219752754296894559, 0.3333333333333333703, 0.3219752754296894559, 0.3333333333333333703, 0.3219752754296894559, 0.3333333333333333703, 0.3219752754296894559, 0.3333333333333333703, 0.3219752754296894559, 0.3333333333333333703, 0.3219752754296894559, 0.3333333333333333703, 0.3219752754296894559, 0.3333333333333333703, 0.3219752754296894559, 0.3333333333333333703, 0.3219752754296894559, 0.3333333333333333703, 0.3219752754296894559, 0.3333333333333333703, 0.3219752754296894559, 0.3333333333333333703, 0.3219752754296894559, 0.3333333333333333703, 0.3219752754296894559, 0.3333333333333333703, 0.3219752754296894559, 0.3333333333333333703, 0.3219752754296894559, 0.3333333333333333703, 0.3219752754296894559, 0.3333333333333333703, 0.3219752754296894559, 0.3333333333333333703, 0.3219752754296894559, 0.3333333333333333703, 0.3219752754296894559, 0.3333333333333333703, 0.3219752754296894559, 0.3333333333333333703, 0.3219752754296894559, 0.3333333333333333703, 0.3219752754296894559, 0.3333333333333333703, 0.3219752754296894559, 0.3333333333333333703, 0.3219752754296894559, 0.3333333333333333703, 0.3219752754296894559, 0.3333333333333333703, 0.3219752754296894559, 0.3333333333333333703, 0.3219752754296894559, 0.3333333333333333703, 0.3219752754296894559, 0.3333333333333333703, 0.3219752754296894559, 0.3333333333333333703, 0.3219752754296894559, 0.3333333333333333703, 0.3219752754296894559, 0.3333333333333333703, 0.3219752754296894559, 0.3333333333333333703, 0.3219752754296894559, 0.3333333333333333703, 0.3219752754296894559, 0.3333333333333333703, 0.3219752754296894559, 0.3333333333333333703, 0.3219752754296894559, 0.3333333333333333703, 0.3219752754296894559, 0.3333333333333333703, 0.3219752754296894559, 0.3333333333333333703, 0.3219752754296894559, 0.3333333333333333703, 0.3219752754296894559, 0.3333333333333333703, 0.3219752754296894559, 0.3333333333333333703, 0.3219752754296894559, 0.3333333333333333703, 0.3219752754296894559, 0.3333333333333333703, 0.3219752754296894559, 0.3333333333333333703, 0.3219752754296894559, 0.3333333333333333703, 0.3219752754296894559, 0.3333333333333333703, 0.3219752754296894559, 0.3333333333333333703, 0.3219752754296894559, 0.3333333333333333703, 0.3219752754296894559, 0.3333333333333333703, 0.3219752754296894559, 0.3333333333333333703, 0.3219752754296894559, 0.3333333333333333703, 0.3219752754296894559, 0.3333333333333333703, 0.3219752754296894559, 0.3333333333333333703, 0.3219752754296894559, 0.3333333333333333703, 0.3219752754296894559, 0.3333333333333333703, 0.3219752754296894559, 0.3333333333333333703, 0.3219752754296894559, 0.3333333333333333703, 0.3219752754296894559, 0.3333333333333333703, 0.3219752754296894559, 0.3333333333333333703, 0.3219752754296894559, 0.3333333333333333703, 0.3219752754296894559, 0.3333333333333333703, 0.3219752754296894559, 0.3333333333333333703, 0.3219752754296894559, 0.3333333333333333703, 0.3219752754296894559, 0.3333333333333333703, 0.3219752754296894559, 0.3333333333333333703, 0.3219752754296894559, 0.3333333333333333703, 0.3219752754296894559, 0.3333333333333333703, 0.3219752754296894559, 0.3333333333333333703, 0.3219752754296894559, 0.3333333333333333703, 0.3219752754296894559, 0.3333333333333333703, 0.3219752754296894559, 0.3333333333333333703, 0.3219752754296894559, 0.3333333333333333703, 0.3219752754296894559, 0.3333333333333333703, 0.3219752754296894559, 0.3333333333333333703, 0.3219752754296894559, 0.3333333333333333703, 0.3219752754296894559, 0.3333333333333333703, 0.3219752754296894559, 0.3333333333333333703, 0.3219752754296894559, 0.3333333333333333703, 0.3219752754296894559, 0.3333333333333333703, 0.3219752754296894559, 0.3333333333333333703, 0.3219752754296894559, 0.3333333333333333703, 0.3219752754296894559, 0.3333333333333333703, 0.3219752754296894559, 0.3333333333333333703, 0.3219752754296894559, 0.3333333333333333703, 0.3219752754296894559, 0.3333333333333333703, 0.3219752754296894559, 0.3333333333333333703, 0.3219752754296894559, 0.3333333333333333703, 0.3219752754296894559, 0.3333333333333333703, 0.3219752754296894559, 0.3333333333333333703, 0.3219752754296894559, 0.3333333333333333703, 0.3219752754296894559, 0.3333333333333333703, 0.3219752754296894559, 0.3333333333333333703, 0.3219752754296894559, 0.3333333333333333703, 0.3219752754296894559, 0.3333333333333333703, 0.3219752754296894559, 0.3333333333333333703, 0.3219752754296894559, 0.3333333333333333703, 0.3219752754296894559, 0.3333333333333333703, 0.3219752754296894559, 0.3333333333333333703, 0.3219752754296894559, 0.3333333333333333703, 0.3219752754296894559, 0.3333333333333333703, 0.3219752754296894559, 0.3333333333333333703, 0.3219752754296894559, 0.3333333333333333703, 0.3219752754296894559, 0.3333333333333333703, 0.3219752754296894559, 0.3333333333333333703, 0.3219752754296894559, 0.3333333333333333703, 0.3219752754296894559, 0.3333333333333333703, 0.3219752754296894559, 0.3333333333333333703, 0.3219752754296894559, 0.3333333333333333703, 0.3219752754296894559, 0.3333333333333333703, 0.3219752754296894559, 0.3333333333333333703, 0.3219752754296894559, 0.3333333333333333703, 0.3219752754296894559, 0.3333333333333333703, 0.3219752754296894559, 0.3333333333333333703, 0.3219752754296894559, 0.3333333333333333703, 0.3219752754296894559, 0.3333333333333333703, 0.3219752754296894559, 0.3333333333333333703, 0.3219752754296894559, 0.3333333333333333703, 0.3219752754296894559, 0.3333333333333333703, 0.3219752754296894559, 0.3333333333333333703, 0.3219752754296894559, 0.3333333333333333703, 0.3219752754296894559, 0.3333333333333333703, 0.3219752754296894559, 0.3333333333333333703, 0.3219752754296894559, 0.3333333333333333703, 0.3219752754296894559, 0.3333333333333333703, 0.3219752754296894559, 0.3333333333333333703, 0.3219752754296894559, 0.3333333333333333703, 0.3219752754296894559, 0.3333333333333333703, 0.3219752754296894559, 0.3333333333333333703, 0.3219752754296894559, 0.3333333333333333703, 0.3219752754296894559, 0.3333333333333333703, 0.3219752754296894559, 0.3333333333333333703, 0.3219752754296894559, 0.3333333333333333703, 0.3219752754296894559, 0.3333333333333333703, 0.3219752754296894559, 0.3333333333333333703, 0.3219752754296894559, 0.3333333333333333703, 0.3219752754296894559, 0.3333333333333333703, 0.3219752754296894559, 0.3333333333333333703, 0.3219752754296894559, 0.3333333333333333703, 0.3219752754296894559, 0.3333333333333333703, 0.3219752754296894559, 0.3333333333333333703, 0.3219752754296894559, 0.3333333333333333703, 0.3219752754296894559, 0.3333333333333333703, 0.3219752754296894559, 0.3333333333333333703, 0.3219752754296894559, 0.3333333333333333703, 0.3219752754296894559, 0.3333333333333333703, 0.3219752754296894559, 0.3333333333333333703, 0.3219752754296894559, 0.3333333333333333703, 0.3219752754296894559, 0.3333333333333333703, 0.3219752754296894559, 0.3333333333333333703, 0.3219752754296894559, 0.3333333333333333703, 0.3219752754296894559, 0.3333333333333333703, 0.3219752754296894559, 0.3333333333333333703, 0.3219752754296894559, 0.3333333333333333703, 0.3219752754296894559, 0.3333333333333333703, 0.3219752754296894559, 0.3333333333333333703, 0.3219752754296894559, 0.3333333333333333703, 0.3219752754296894559, 0.3333333333333333703, 0.3219752754296894559, 0.3333333333333333703, 0.3219752754296894559, 0.3333333333333333703, 0.3219752754296894559, 0.3333333333333333703, 0.3219752754296894559, 0.3333333333333333703, 0.3219752754296894559, 0.3333333333333333703, 0.3219752754296894559, 0.3333333333333333703, 0.3219752754296894559, 0.3333333333333333703, 0.3219752754296894559, 0.3333333333333333703, 0.3219752754296894559, 0.3333333333333333703, 0.3219752754296894559, 0.3333333333333333703, 0.3219752754296894559, 0.3333333333333333703),
 ( 0.3333333333333333703, 0.3219752754296894559, 0.3333333333333333703, 0.3219752754296894559, 0.3333333333333333703, 0.3219752754296894559, 0.3333333333333333703, 0.3219752754296894559, 0.3333333333333333703, 0.3219752754296894559, 0.3333333333333333703, 0.3219752754296894559, 0.3333333333333333703, 0.3219752754296894559, 0.3333333333333333703, 0.3219752754296894559, 0.3333333333333333703, 0.3219752754296894559, 0.3333333333333333703, 0.3219752754296894559, 0.3333333333333333703, 0.3219752754296894559, 0.3333333333333333703, 0.3219752754296894559, 0.3333333333333333703, 0.3219752754296894559, 0.3333333333333333703, 0.3219752754296894559, 0.3333333333333333703, 0.3219752754296894559, 0.3333333333333333703, 0.3219752754296894559, 0.3333333333333333703, 0.3219752754296894559, 0.3333333333333333703, 0.3219752754296894559, 0.3333333333333333703, 0.3219752754296894559, 0.3333333333333333703, 0.3219752754296894559, 0.3333333333333333703, 0.3219752754296894559, 0.3333333333333333703, 0.3219752754296894559, 0.3333333333333333703, 0.3219752754296894559, 0.3333333333333333703, 0.3219752754296894559, 0.3333333333333333703, 0.3219752754296894559, 0.3333333333333333703, 0.3219752754296894559, 0.3333333333333333703, 0.3219752754296894559, 0.3333333333333333703, 0.3219752754296894559, 0.3333333333333333703, 0.3219752754296894559, 0.3333333333333333703, 0.3219752754296894559, 0.3333333333333333703, 0.3219752754296894559, 0.3333333333333333703, 0.3219752754296894559, 0.3333333333333333703, 0.3219752754296894559, 0.3333333333333333703, 0.3219752754296894559, 0.3333333333333333703, 0.3219752754296894559, 0.3333333333333333703, 0.3219752754296894559, 0.3333333333333333703, 0.3219752754296894559, 0.3333333333333333703, 0.3219752754296894559, 0.3333333333333333703, 0.3219752754296894559, 0.3333333333333333703, 0.3219752754296894559, 0.3333333333333333703, 0.3219752754296894559, 0.3333333333333333703, 0.3219752754296894559, 0.3333333333333333703, 0.3219752754296894559, 0.3333333333333333703, 0.3219752754296894559, 0.3333333333333333703, 0.3219752754296894559, 0.3333333333333333703, 0.3219752754296894559, 0.3333333333333333703, 0.3219752754296894559, 0.3333333333333333703, 0.3219752754296894559, 0.3333333333333333703, 0.3219752754296894559, 0.3333333333333333703, 0.3219752754296894559, 0.3333333333333333703, 0.3219752754296894559, 0.3333333333333333703, 0.3219752754296894559, 0.3333333333333333703, 0.3219752754296894559, 0.3333333333333333703, 0.3219752754296894559, 0.3333333333333333703, 0.3219752754296894559, 0.3333333333333333703, 0.3219752754296894559, 0.3333333333333333703, 0.3219752754296894559, 0.3333333333333333703, 0.3219752754296894559, 0.3333333333333333703, 0.3219752754296894559, 0.3333333333333333703, 0.3219752754296894559, 0.3333333333333333703, 0.3219752754296894559, 0.3333333333333333703, 0.3219752754296894559, 0.3333333333333333703, 0.3219752754296894559, 0.3333333333333333703, 0.3219752754296894559, 0.3333333333333333703, 0.3219752754296894559, 0.3333333333333333703, 0.3219752754296894559, 0.3333333333333333703, 0.3219752754296894559, 0.3333333333333333703, 0.3219752754296894559, 0.3333333333333333703, 0.3219752754296894559, 0.3333333333333333703, 0.3219752754296894559, 0.3333333333333333703, 0.3219752754296894559, 0.3333333333333333703, 0.3219752754296894559, 0.3333333333333333703, 0.3219752754296894559, 0.3333333333333333703, 0.3219752754296894559, 0.3333333333333333703, 0.3219752754296894559, 0.3333333333333333703, 0.3219752754296894559, 0.3333333333333333703, 0.3219752754296894559, 0.3333333333333333703, 0.3219752754296894559, 0.3333333333333333703, 0.3219752754296894559, 0.3333333333333333703, 0.3219752754296894559, 0.3333333333333333703, 0.3219752754296894559, 0.3333333333333333703, 0.3219752754296894559, 0.3333333333333333703, 0.3219752754296894559, 0.3333333333333333703, 0.3219752754296894559, 0.3333333333333333703, 0.3219752754296894559, 0.3333333333333333703, 0.3219752754296894559, 0.3333333333333333703, 0.3219752754296894559, 0.3333333333333333703, 0.3219752754296894559, 0.3333333333333333703, 0.3219752754296894559, 0.3333333333333333703, 0.3219752754296894559, 0.3333333333333333703, 0.3219752754296894559, 0.3333333333333333703, 0.3219752754296894559, 0.3333333333333333703, 0.3219752754296894559, 0.3333333333333333703, 0.3219752754296894559, 0.3333333333333333703, 0.3219752754296894559, 0.3333333333333333703, 0.3219752754296894559, 0.3333333333333333703, 0.3219752754296894559, 0.3333333333333333703, 0.3219752754296894559, 0.3333333333333333703, 0.3219752754296894559, 0.3333333333333333703, 0.3219752754296894559, 0.3333333333333333703, 0.3219752754296894559, 0.3333333333333333703, 0.3219752754296894559, 0.3333333333333333703, 0.3219752754296894559, 0.3333333333333333703, 0.3219752754296894559, 0.3333333333333333703, 0.3219752754296894559, 0.3333333333333333703, 0.3219752754296894559, 0.3333333333333333703, 0.3219752754296894559, 0.3333333333333333703, 0.3219752754296894559, 0.3333333333333333703, 0.3219752754296894559, 0.3333333333333333703, 0.3219752754296894559, 0.3333333333333333703, 0.3219752754296894559, 0.3333333333333333703, 0.3219752754296894559, 0.3333333333333333703, 0.3219752754296894559, 0.3333333333333333703, 0.3219752754296894559, 0.3333333333333333703, 0.3219752754296894559, 0.3333333333333333703, 0.3219752754296894559, 0.3333333333333333703, 0.3219752754296894559, 0.3333333333333333703, 0.3219752754296894559, 0.3333333333333333703, 0.3219752754296894559, 0.3333333333333333703, 0.3219752754296894559, 0.3333333333333333703, 0.3219752754296894559, 0.3333333333333333703, 0.3219752754296894559, 0.3333333333333333703, 0.3219752754296894559, 0.3333333333333333703, 0.3219752754296894559, 0.3333333333333333703, 0.3219752754296894559, 0.3333333333333333703, 0.3219752754296894559, 0.3333333333333333703, 0.3219752754296894559, 0.3333333333333333703, 0.3219752754296894559, 0.3333333333333333703, 0.3219752754296894559, 0.3333333333333333703, 0.3219752754296894559, 0.3333333333333333703, 0.3219752754296894559, 0.3333333333333333703, 0.3219752754296894559, 0.3333333333333333703, 0.3219752754296894559, 0.3333333333333333703, 0.3219752754296894559, 0.3333333333333333703, 0.3219752754296894559, 0.3333333333333333703, 0.3219752754296894559, 0.3333333333333333703, 0.3219752754296894559, 0.3333333333333333703, 0.3219752754296894559, 0.3333333333333333703, 0.3219752754296894559, 0.3333333333333333703, 0.3219752754296894559, 0.3333333333333333703, 0.3219752754296894559, 0.3333333333333333703, 0.3219752754296894559, 0.3333333333333333703, 0.3219752754296894559, 0.3333333333333333703, 0.3219752754296894559, 0.3333333333333333703, 0.3219752754296894559, 0.3333333333333333703, 0.3219752754296894559, 0.3333333333333333703, 0.3219752754296894559, 0.3333333333333333703, 0.3219752754296894559, 0.3333333333333333703, 0.3219752754296894559, 0.3333333333333333703, 0.3219752754296894559, 0.3333333333333333703, 0.3219752754296894559, 0.3333333333333333703, 0.3219752754296894559, 0.3333333333333333703, 0.3219752754296894559, 0.3333333333333333703, 0.3219752754296894559, 0.3333333333333333703, 0.3219752754296894559, 0.3333333333333333703, 0.3219752754296894559, 0.3333333333333333703, 0.3219752754296894559, 0.3333333333333333703, 0.3219752754296894559, 0.3333333333333333703, 0.3219752754296894559, 0.3333333333333333703, 0.3219752754296894559, 0.3333333333333333703, 0.3219752754296894559, 0.3333333333333333703, 0.3219752754296894559, 0.3333333333333333703, 0.3219752754296894559, 0.3333333333333333703, 0.3219752754296894559, 0.3333333333333333703, 0.3219752754296894559, 0.3333333333333333703, 0.3219752754296894559, 0.3333333333333333703, 0.3219752754296894559, 0.3333333333333333703, 0.3219752754296894559, 0.3333333333333333703, 0.3219752754296894559, 0.3333333333333333703, 0.3219752754296894559, 0.3333333333333333703, 0.3219752754296894559, 0.3333333333333333703, 0.3219752754296894559, 0.3333333333333333703, 0.3219752754296894559, 0.3333333333333333703, 0.3219752754296894559, 0.3333333333333333703, 0.3219752754296894559, 0.3333333333333333703, 0.3219752754296894559, 0.3333333333333333703, 0.3219752754296894559, 0.3333333333333333703, 0.3219752754296894559, 0.3333333333333333703, 0.3219752754296894559, 0.3333333333333333703, 0.3219752754296894559, 0.3333333333333333703, 0.3219752754296894559, 0.3333333333333333703, 0.3219752754296894559, 0.3333333333333333703, 0.3219752754296894559, 0.3333333333333333703, 0.3219752754296894559, 0.3333333333333333703, 0.3219752754296894559, 0.3333333333333333703, 0.3219752754296894559, 0.3333333333333333703, 0.3219752754296894559, 0.3333333333333333703, 0.3219752754296894559, 0.3333333333333333703, 0.3219752754296894559, 0.3333333333333333703, 0.3219752754296894559, 0.3333333333333333703, 0.3219752754296894559, 0.3333333333333333703, 0.3219752754296894559, 0.3333333333333333703, 0.3219752754296894559, 0.3333333333333333703, 0.3219752754296894559, 0.3333333333333333703, 0.3219752754296894559, 0.3333333333333333703, 0.3219752754296894559, 0.3333333333333333703, 0.3219752754296894559, 0.3333333333333333703, 0.3219752754296894559, 0.3333333333333333703, 0.3219752754296894559, 0.3333333333333333703, 0.3219752754296894559, 0.3333333333333333703, 0.3219752754296894559, 0.3333333333333333703, 0.3219752754296894559, 0.3333333333333333703, 0.3219752754296894559, 0.3333333333333333703, 0.3219752754296894559, 0.3333333333333333703, 0.3219752754296894559, 0.3333333333333333703, 0.3219752754296894559, 0.3333333333333333703, 0.3219752754296894559, 0.3333333333333333703, 0.3219752754296894559, 0.3333333333333333703, 0.3219752754296894559, 0.3333333333333333703, 0.3219752754296894559, 0.3333333333333333703, 0.3219752754296894559, 0.3333333333333333703, 0.3219752754296894559, 0.3333333333333333703, 0.3219752754296894559, 0.3333333333333333703, 0.3219752754296894559, 0.3333333333333333703, 0.3219752754296894559, 0.3333333333333333703, 0.3219752754296894559, 0.3333333333333333703, 0.3219752754296894559, 0.3333333333333333703, 0.3219752754296894559, 0.3333333333333333703, 0.3219752754296894559, 0.3333333333333333703, 0.3219752754296894559, 0.3333333333333333703, 0.3219752754296894559, 0.3333333333333333703, 0.3219752754296894559, 0.3333333333333333703, 0.3219752754296894559, 0.3333333333333333703, 0.3219752754296894559, 0.3333333333333333703, 0.3219752754296894559, 0.3333333333333333703, 0.3219752754296894559, 0.3333333333333333703, 0.3219752754296894559, 0.3333333333333333703, 0.3219752754296894559, 0.3333333333333333703),
 ( 1.000000000000000000, 0.9659258262890683122, 1.000000000000000000, 0.9659258262890683122, 1.000000000000000000, 0.9659258262890683122, 1.000000000000000000, 0.9659258262890683122, 1.000000000000000000, 0.9659258262890683122, 1.000000000000000000, 0.9659258262890683122, 1.000000000000000000, 0.9659258262890683122, 1.000000000000000000, 0.9659258262890683122, 1.000000000000000000, 0.9659258262890683122, 1.000000000000000000, 0.9659258262890683122, 1.000000000000000000, 0.9659258262890683122, 1.000000000000000000, 0.9659258262890683122, 1.000000000000000000, 0.9659258262890683122, 1.000000000000000000, 0.9659258262890683122, 1.000000000000000000, 0.9659258262890683122, 1.000000000000000000, 0.9659258262890683122, 1.000000000000000000, 0.9659258262890683122, 1.000000000000000000, 0.9659258262890683122, 1.000000000000000000, 0.9659258262890683122, 1.000000000000000000, 0.9659258262890683122, 1.000000000000000000, 0.9659258262890683122, 1.000000000000000000, 0.9659258262890683122, 1.000000000000000000, 0.9659258262890683122, 1.000000000000000000, 0.9659258262890683122, 1.000000000000000000, 0.9659258262890683122, 1.000000000000000000, 0.9659258262890683122, 1.000000000000000000, 0.9659258262890683122, 1.000000000000000000, 0.9659258262890683122, 1.000000000000000000, 0.9659258262890683122, 1.000000000000000000, 0.9659258262890683122, 1.000000000000000000, 0.9659258262890683122, 1.000000000000000000, 0.9659258262890683122, 1.000000000000000000, 0.9659258262890683122, 1.000000000000000000, 0.9659258262890683122, 1.000000000000000000, 0.9659258262890683122, 1.000000000000000000, 0.9659258262890683122, 1.000000000000000000, 0.9659258262890683122, 1.000000000000000000, 0.9659258262890683122, 1.000000000000000000, 0.9659258262890683122, 1.000000000000000000, 0.9659258262890683122, 1.000000000000000000, 0.9659258262890683122, 1.000000000000000000, 0.9659258262890683122, 1.000000000000000000, 0.9659258262890683122, 1.000000000000000000, 0.9659258262890683122, 1.000000000000000000, 0.9659258262890683122, 1.000000000000000000, 0.9659258262890683122, 1.000000000000000000, 0.9659258262890683122, 1.000000000000000000, 0.9659258262890683122, 1.000000000000000000, 0.9659258262890683122, 1.000000000000000000, 0.9659258262890683122, 1.000000000000000000, 0.9659258262890683122, 1.000000000000000000, 0.9659258262890683122, 1.000000000000000000, 0.9659258262890683122, 1.000000000000000000, 0.9659258262890683122, 1.000000000000000000, 0.9659258262890683122, 1.000000000000000000, 0.9659258262890683122, 1.000000000000000000, 0.9659258262890683122, 1.000000000000000000, 0.9659258262890683122, 1.000000000000000000, 0.9659258262890683122, 1.000000000000000000, 0.9659258262890683122, 1.000000000000000000, 0.9659258262890683122, 1.000000000000000000, 0.9659258262890683122, 1.000000000000000000, 0.9659258262890683122, 1.000000000000000000, 0.9659258262890683122, 1.000000000000000000, 0.9659258262890683122, 1.000000000000000000, 0.9659258262890683122, 1.000000000000000000, 0.9659258262890683122, 1.000000000000000000, 0.9659258262890683122, 1.000000000000000000, 0.9659258262890683122, 1.000000000000000000, 0.9659258262890683122, 1.000000000000000000, 0.9659258262890683122, 1.000000000000000000, 0.9659258262890683122, 1.000000000000000000, 0.9659258262890683122, 1.000000000000000000, 0.9659258262890683122, 1.000000000000000000, 0.9659258262890683122, 1.000000000000000000, 0.9659258262890683122, 1.000000000000000000, 0.9659258262890683122, 1.000000000000000000, 0.9659258262890683122, 1.000000000000000000, 0.9659258262890683122, 1.000000000000000000, 0.9659258262890683122, 1.000000000000000000, 0.9659258262890683122, 1.000000000000000000, 0.9659258262890683122, 1.000000000000000000, 0.9659258262890683122, 1.000000000000000000, 0.9659258262890683122, 1.000000000000000000, 0.9659258262890683122, 1.000000000000000000, 0.9659258262890683122, 1.000000000000000000, 0.9659258262890683122, 1.000000000000000000, 0.9659258262890683122, 1.000000000000000000, 0.9659258262890683122, 1.000000000000000000, 0.9659258262890683122, 1.000000000000000000, 0.9659258262890683122, 1.000000000000000000, 0.9659258262890683122, 1.000000000000000000, 0.9659258262890683122, 1.000000000000000000, 0.9659258262890683122, 1.000000000000000000, 0.9659258262890683122, 1.000000000000000000, 0.9659258262890683122, 1.000000000000000000, 0.9659258262890683122, 1.000000000000000000, 0.9659258262890683122, 1.000000000000000000, 0.9659258262890683122, 1.000000000000000000, 0.9659258262890683122, 1.000000000000000000, 0.9659258262890683122, 1.000000000000000000, 0.9659258262890683122, 1.000000000000000000, 0.9659258262890683122, 1.000000000000000000, 0.9659258262890683122, 1.000000000000000000, 0.9659258262890683122, 1.000000000000000000, 0.9659258262890683122, 1.000000000000000000, 0.9659258262890683122, 1.000000000000000000, 0.9659258262890683122, 1.000000000000000000, 0.9659258262890683122, 1.000000000000000000, 0.9659258262890683122, 1.000000000000000000, 0.9659258262890683122, 1.000000000000000000, 0.9659258262890683122, 1.000000000000000000, 0.9659258262890683122, 1.000000000000000000, 0.9659258262890683122, 1.000000000000000000, 0.9659258262890683122, 1.000000000000000000, 0.9659258262890683122, 1.000000000000000000, 0.9659258262890683122, 1.000000000000000000, 0.9659258262890683122, 1.000000000000000000, 0.9659258262890683122, 1.000000000000000000, 0.9659258262890683122, 1.000000000000000000, 0.9659258262890683122, 1.000000000000000000, 0.9659258262890683122, 1.000000000000000000, 0.9659258262890683122, 1.000000000000000000, 0.9659258262890683122, 1.000000000000000000, 0.9659258262890683122, 1.000000000000000000, 0.9659258262890683122, 1.000000000000000000, 0.9659258262890683122, 1.000000000000000000, 0.9659258262890683122, 1.000000000000000000, 0.9659258262890683122, 1.000000000000000000, 0.9659258262890683122, 1.000000000000000000, 0.9659258262890683122, 1.000000000000000000, 0.9659258262890683122, 1.000000000000000000, 0.9659258262890683122, 1.000000000000000000, 0.9659258262890683122, 1.000000000000000000, 0.9659258262890683122, 1.000000000000000000, 0.9659258262890683122, 1.000000000000000000, 0.9659258262890683122, 1.000000000000000000, 0.9659258262890683122, 1.000000000000000000, 0.9659258262890683122, 1.000000000000000000, 0.9659258262890683122, 1.000000000000000000, 0.9659258262890683122, 1.000000000000000000, 0.9659258262890683122, 1.000000000000000000, 0.9659258262890683122, 1.000000000000000000, 0.9659258262890683122, 1.000000000000000000, 0.9659258262890683122, 1.000000000000000000, 0.9659258262890683122, 1.000000000000000000, 0.9659258262890683122, 1.000000000000000000, 0.9659258262890683122, 1.000000000000000000, 0.9659258262890683122, 1.000000000000000000, 0.9659258262890683122, 1.000000000000000000, 0.9659258262890683122, 1.000000000000000000, 0.9659258262890683122, 1.000000000000000000, 0.9659258262890683122, 1.000000000000000000, 0.9659258262890683122, 1.000000000000000000, 0.9659258262890683122, 1.000000000000000000, 0.9659258262890683122, 1.000000000000000000, 0.9659258262890683122, 1.000000000000000000, 0.9659258262890683122, 1.000000000000000000, 0.9659258262890683122, 1.000000000000000000, 0.9659258262890683122, 1.000000000000000000, 0.9659258262890683122, 1.000000000000000000, 0.9659258262890683122, 1.000000000000000000, 0.9659258262890683122, 1.000000000000000000, 0.9659258262890683122, 1.000000000000000000, 0.9659258262890683122, 1.000000000000000000, 0.9659258262890683122, 1.000000000000000000, 0.9659258262890683122, 1.000000000000000000, 0.9659258262890683122, 1.000000000000000000, 0.9659258262890683122, 1.000000000000000000, 0.9659258262890683122, 1.000000000000000000, 0.9659258262890683122, 1.000000000000000000, 0.9659258262890683122, 1.000000000000000000, 0.9659258262890683122, 1.000000000000000000, 0.9659258262890683122, 1.000000000000000000, 0.9659258262890683122, 1.000000000000000000, 0.9659258262890683122, 1.000000000000000000, 0.9659258262890683122, 1.000000000000000000, 0.9659258262890683122, 1.000000000000000000, 0.9659258262890683122, 1.000000000000000000, 0.9659258262890683122, 1.000000000000000000, 0.9659258262890683122, 1.000000000000000000, 0.9659258262890683122, 1.000000000000000000, 0.9659258262890683122, 1.000000000000000000, 0.9659258262890683122, 1.000000000000000000, 0.9659258262890683122, 1.000000000000000000, 0.9659258262890683122, 1.000000000000000000, 0.9659258262890683122, 1.000000000000000000, 0.9659258262890683122, 1.000000000000000000, 0.9659258262890683122, 1.000000000000000000, 0.9659258262890683122, 1.000000000000000000, 0.9659258262890683122, 1.000000000000000000, 0.9659258262890683122, 1.000000000000000000, 0.9659258262890683122, 1.000000000000000000, 0.9659258262890683122, 1.000000000000000000, 0.9659258262890683122, 1.000000000000000000, 0.9659258262890683122, 1.000000000000000000, 0.9659258262890683122, 1.000000000000000000, 0.9659258262890683122, 1.000000000000000000, 0.9659258262890683122, 1.000000000000000000, 0.9659258262890683122, 1.000000000000000000, 0.9659258262890683122, 1.000000000000000000, 0.9659258262890683122, 1.000000000000000000, 0.9659258262890683122, 1.000000000000000000, 0.9659258262890683122, 1.000000000000000000, 0.9659258262890683122, 1.000000000000000000, 0.9659258262890683122, 1.000000000000000000, 0.9659258262890683122, 1.000000000000000000, 0.9659258262890683122, 1.000000000000000000, 0.9659258262890683122, 1.000000000000000000, 0.9659258262890683122, 1.000000000000000000, 0.9659258262890683122, 1.000000000000000000, 0.9659258262890683122, 1.000000000000000000, 0.9659258262890683122, 1.000000000000000000, 0.9659258262890683122, 1.000000000000000000, 0.9659258262890683122, 1.000000000000000000, 0.9659258262890683122, 1.000000000000000000, 0.9659258262890683122, 1.000000000000000000, 0.9659258262890683122, 1.000000000000000000, 0.9659258262890683122, 1.000000000000000000, 0.9659258262890683122, 1.000000000000000000, 0.9659258262890683122, 1.000000000000000000, 0.9659258262890683122, 1.000000000000000000, 0.9659258262890683122, 1.000000000000000000, 0.9659258262890683122, 1.000000000000000000, 0.9659258262890683122, 1.000000000000000000, 0.9659258262890683122, 1.000000000000000000, 0.9659258262890683122, 1.000000000000000000, 0.9659258262890683122, 1.000000000000000000) ) ) 
 REPRESENTATION_ITEM ( '' )  SURFACE ( )  );
#113094=CARTESIAN_POINT ( 'NONE',  ( -9.474510206698964154, 16.51473224551069663, 90.41557627198103830 ) ) ;
#113095=CARTESIAN_POINT ( 'NONE',  ( 10.81492255796078972, 18.62759615963270932, 94.58224293864769550 ) ) ;
#113096=CARTESIAN_POINT ( 'NONE',  ( -16.46253265017160317, 9.564922557960807481, 65.83224293864769550 ) ) ;
#113097=CARTESIAN_POINT ( 'NONE',  ( -17.44270441346514033, -5.991230190323104665, 61.36335079264229364 ) ) ;
#113098=CARTESIAN_POINT ( 'NONE',  ( 4.483927247898545687, 16.52544592524342804, 74.79057627198105251 ) ) ;
#113099=CARTESIAN_POINT ( 'NONE',  ( 16.46253265017160672, -9.564922557960803928, 113.3322429386476955 ) ) ;
#113101=CARTESIAN_POINT ( 'NONE',  ( 21.52544592524344225, -5.823673210054117533, 88.54057627198103830 ) ) ;
#113102=CARTESIAN_POINT ( 'NONE',  ( -13.97604488694547697, 13.89961937509957934, 48.12609039468566863 ) ) ;
#113103=CARTESIAN_POINT ( 'NONE',  ( -5.153800228976328057, -19.02544592524343514, 112.2905762719810099 ) ) ;
#113105=CARTESIAN_POINT ( 'NONE',  ( -5.823673210054116645, -21.52544592524344225, 52.29057627198102409 ) ) ;
#113107=CARTESIAN_POINT ( 'NONE',  ( -5.049401038298153566, 19.05341960407611168, 80.20724293864769550 ) ) ;
#113108=CARTESIAN_POINT ( 'NONE',  ( 10.81492255796106328, -18.62759615963255655, 80.41775706135234714 ) ) ;
#113109=CARTESIAN_POINT ( 'NONE',  ( 19.02544592524343514, -5.153800228976328945, 38.54057627198103120 ) ) ;
#113110=CARTESIAN_POINT ( 'NONE',  ( -12.14591786802309592, -12.06949235617757132, 76.87390960531439532 ) ) ;
#113111=CARTESIAN_POINT ( 'NONE',  ( 4.379528057220092307, 16.55341960407617563, 22.29275706135235069 ) ) ;
#113112=CARTESIAN_POINT ( 'NONE',  ( -15.80617190586768217, 15.72974639402176855, 63.12609039468568994 ) ) ;
#113113=ORIENTED_EDGE ( 'NONE', *, *, #93672, .T. ) ;
#113114=CARTESIAN_POINT ( 'NONE',  ( -5.153800228976607833, 19.02544592524334988, 27.70942372801899722 ) ) ;
#113115=CARTESIAN_POINT ( 'NONE',  ( 13.97604488694548053, -13.89961937509957401, 75.62609039468564731 ) ) ;
#113117=CARTESIAN_POINT ( 'NONE',  ( -5.719274019375665041, -21.55341960407619695, 29.79275706135234358 ) ) ;
#113119=CARTESIAN_POINT ( 'NONE',  ( -18.89770734986052148, -5.499999999999912070, 44.10214472496640070 ) ) ;
#113120=CARTESIAN_POINT ( 'NONE',  ( -21.52544592524334988, -5.823673210054445271, 108.9594237280190185 ) ) ;
#113121=CARTESIAN_POINT ( 'NONE',  ( -0.05219959533909027116, -19.03943276465977164, 52.49890960531436690 ) ) ;
#113122=CARTESIAN_POINT ( 'NONE',  ( -13.97604488694547697, 13.89961937509957934, 33.12609039468566863 ) ) ;
#113123=CARTESIAN_POINT ( 'NONE',  ( -0.05219959533934338120, 16.53943276465976808, 97.50109039468567573 ) ) ;
#113124=CARTESIAN_POINT ( 'NONE',  ( 16.51473224551069308, 9.474510206698969483, 104.1655762719810241 ) ) ;
#113125=CARTESIAN_POINT ( 'NONE',  ( 18.62759615963255655, 10.81492255796105972, 76.66775706135234714 ) ) ;
#113127=CARTESIAN_POINT ( 'NONE',  ( 30.00000000000000000, -5.510910596163089556E-15, 45.00000000000000000 ) ) ;
#113128=CARTESIAN_POINT ( 'NONE',  ( 0.05219959533937995610, -21.53943276465977519, 80.00109039468568994 ) ) ;
#113129=CARTESIAN_POINT ( 'NONE',  ( -18.67979575497193778, 10.72451020669871902, 103.3344237280190043 ) ) ;
#113131=CARTESIAN_POINT ( 'NONE',  ( -9.474510206698964154, 16.51473224551069663, 105.4155762719810383 ) ) ;
#113132=CARTESIAN_POINT ( 'NONE',  ( -16.46253265017146816, -9.564922557961047289, 29.16775706135232937 ) ) ;
#113135=CARTESIAN_POINT ( 'NONE',  ( 5.153800228976335163, 19.02544592524342804, 44.79057627198103830 ) ) ;
#113136=CARTESIAN_POINT ( 'NONE',  ( -21.52544592524343514, 5.823673210054127303, 61.04057627198103120 ) ) ;
#113137=CARTESIAN_POINT ( 'NONE',  ( 8.224510206698953496, -14.34966873604960469, 22.91557627198102765 ) ) ;
#113138=CARTESIAN_POINT ( 'NONE',  ( -16.52544592524342804, 4.483927247898546575, 91.04057627198103830 ) ) ;
#113139=CARTESIAN_POINT ( 'NONE',  ( 5.049401038298161559, -19.05341960407611168, 82.70724293864770971 ) ) ;
#113140=CARTESIAN_POINT ( 'NONE',  ( -18.62759615963255300, -10.81492255796106328, 99.16775706135234714 ) ) ;
#113141=CARTESIAN_POINT ( 'NONE',  ( 13.89961937509977652, -13.97604488694527269, 43.12390960531434558 ) ) ;
#113142=CARTESIAN_POINT ( 'NONE',  ( 14.34966873604960469, 8.224510206698951720, 104.1655762719810241 ) ) ;
#113143=CARTESIAN_POINT ( 'NONE',  ( 10.72451020669871369, 18.67979575497193778, 57.08442372801901854 ) ) ;
#113144=CARTESIAN_POINT ( 'NONE',  ( 18.62759615963271287, -10.81492255796078972, 88.33224293864769550 ) ) ;
#113145=CARTESIAN_POINT ( 'NONE',  ( -16.46253265017146816, -9.564922557961047289, 54.16775706135234003 ) ) ;
#113147=CARTESIAN_POINT ( 'NONE',  ( 16.51473224551069308, 9.474510206698969483, 104.1655762719810241 ) ) ;
#113148=CARTESIAN_POINT ( 'NONE',  ( 8.314922557960818139, 14.29746914071049879, 74.58224293864768129 ) ) ;
#113149=CARTESIAN_POINT ( 'NONE',  ( -16.46253265017146816, -9.564922557961047289, 39.16775706135234003 ) ) ;
#113150=CARTESIAN_POINT ( 'NONE',  ( 16.46253265017160672, -9.564922557960803928, 68.33224293864770971 ) ) ;
#113151=CARTESIAN_POINT ( 'NONE',  ( -16.55341960407611168, -4.379528057220339221, 56.45724293864768839 ) ) ;
#113152=CARTESIAN_POINT ( 'NONE',  ( 5.153800228976615827, -19.02544592524334988, 80.20942372801901854 ) ) ;
#113153=CARTESIAN_POINT ( 'NONE',  ( -16.46253265017146816, -9.564922557961047289, 89.16775706135234714 ) ) ;
#113154=CARTESIAN_POINT ( 'NONE',  ( -5.719274019375978568, 21.55341960407610458, 30.20724293864769550 ) ) ;
#113155=CARTESIAN_POINT ( 'NONE',  ( -4.379528057220328563, 16.55341960407611168, 105.2072429386477097 ) ) ;
#113157=CARTESIAN_POINT ( 'NONE',  ( -13.89961937509977652, 13.97604488694528158, 55.62390960531434558 ) ) ;
#113158=CARTESIAN_POINT ( 'NONE',  ( 5.823673210054125526, 21.52544592524343514, 64.79057627198103830 ) ) ;
#113159=CARTESIAN_POINT ( 'NONE',  ( -5.153800228976328057, -19.02544592524343514, 27.29057627198103120 ) ) ;
#113160=CARTESIAN_POINT ( 'NONE',  ( 4.483927247898790824, -16.52544592524335698, 75.20942372801901854 ) ) ;
#113161=CARTESIAN_POINT ( 'NONE',  ( 5.049401038298161559, -19.05341960407611168, 62.70724293864769550 ) ) ;
#113162=CARTESIAN_POINT ( 'NONE',  ( 19.05341960407617918, -5.049401038297876454, 56.04275706135234714 ) ) ;
#113164=CARTESIAN_POINT ( 'NONE',  ( -18.62759615963255300, -10.81492255796106328, 64.16775706135234714 ) ) ;
#113165=CARTESIAN_POINT ( 'NONE',  ( 5.823673210054125526, 21.52544592524343514, 49.79057627198102409 ) ) ;
#113166=AXIS2_PLACEMENT_3D ( 'NONE', #126778, #93465, #139965 ) ;
#113167=CARTESIAN_POINT ( 'NONE',  ( 8.314922557960818139, 14.29746914071049879, 114.5822429386477097 ) ) ;
#113168=CARTESIAN_POINT ( 'NONE',  ( -4.483927247898782831, 16.52544592524335698, 87.70942372801901854 ) ) ;
#113169=CARTESIAN_POINT ( 'NONE',  ( 5.049401038297881783, 19.05341960407617563, 107.2927570613523187 ) ) ;
#113170=CARTESIAN_POINT ( 'NONE',  ( -18.22780087662122384, -5.500000000000025757, 96.48459894673894155 ) ) ;
#113172=CARTESIAN_POINT ( 'NONE',  ( -18.67979575497193778, 10.72451020669871902, 98.33442372801901854 ) ) ;
#113173=CARTESIAN_POINT ( 'NONE',  ( 12.06949235617757843, -12.14591786802309237, 53.12390960531436690 ) ) ;
#113174=CARTESIAN_POINT ( 'NONE',  ( -8.224510206698948167, 14.34966873604960824, 55.41557627198102409 ) ) ;
#113175=CARTESIAN_POINT ( 'NONE',  ( 15.80617190586746368, 15.72974639402197994, 94.37390960531436690 ) ) ;
#113176=CARTESIAN_POINT ( 'NONE',  ( 15.72974639402199770, -15.80617190586745480, 88.12390960531436690 ) ) ;
#113178=CARTESIAN_POINT ( 'NONE',  ( 18.62759615963271287, -10.81492255796078972, 33.33224293864769550 ) ) ;
#113179=CARTESIAN_POINT ( 'NONE',  ( 12.06949235617739724, 12.14591786802326823, 66.87609039468568994 ) ) ;
#113180=CARTESIAN_POINT ( 'NONE',  ( 4.483927247898545687, 16.52544592524342804, 74.79057627198105251 ) ) ;
#113181=CARTESIAN_POINT ( 'NONE',  ( 5.153800228976335163, 19.02544592524342804, 49.79057627198100988 ) ) ;
#113184=ORIENTED_EDGE ( 'NONE', *, *, #80571, .F. ) ;
#113185=CARTESIAN_POINT ( 'NONE',  ( -0.05219959533934338120, 16.53943276465976808, 92.50109039468567573 ) ) ;
#113186=CARTESIAN_POINT ( 'NONE',  ( 21.53943276465977519, 0.05219959533937863772, 26.25109039468567573 ) ) ;
#113187=CARTESIAN_POINT ( 'NONE',  ( -5.153800228976328057, -19.02544592524343514, 82.29057627198103830 ) ) ;
#113188=CARTESIAN_POINT ( 'NONE',  ( -18.67979575497193778, 10.72451020669871902, 48.33442372801902565 ) ) ;
#113189=CARTESIAN_POINT ( 'NONE',  ( -9.564922557960796823, -16.46253265017161027, 112.0822429386476955 ) ) ;
#113191=ORIENTED_EDGE ( 'NONE', *, *, #43597, .T. ) ;
#113192=CARTESIAN_POINT ( 'NONE',  ( 18.62759615963255655, 10.81492255796105972, 46.66775706135234714 ) ) ;
#113193=CARTESIAN_POINT ( 'NONE',  ( -0.05219959533909027116, -19.03943276465977164, 32.49890960531435979 ) ) ;
#113194=CARTESIAN_POINT ( 'NONE',  ( 9.474510206698971260, -16.51473224551069308, 112.9155762719810383 ) ) ;
#113195=CARTESIAN_POINT ( 'NONE',  ( -19.02544592524334988, -5.153800228976617603, 58.95942372801900433 ) ) ;
#113196=CARTESIAN_POINT ( 'NONE',  ( -18.67979575497193778, 10.72451020669871902, 33.33442372801900433 ) ) ;
#113197=CARTESIAN_POINT ( 'NONE',  ( -0.05219959533936034679, 19.03943276465977164, 52.50109039468566863 ) ) ;
#113198=CARTESIAN_POINT ( 'NONE',  ( 16.51473224551069308, 9.474510206698969483, 24.16557627198102765 ) ) ;
#113199=CARTESIAN_POINT ( 'NONE',  ( 12.06949235617739724, 12.14591786802326823, 91.87609039468568994 ) ) ;
#113200=CARTESIAN_POINT ( 'NONE',  ( -5.153800228976607833, 19.02544592524334988, 67.70942372801900433 ) ) ;
#113201=CARTESIAN_POINT ( 'NONE',  ( 4.483927247898790824, -16.52544592524335698, 100.2094237280190043 ) ) ;
#113203=CARTESIAN_POINT ( 'NONE',  ( 19.03943276465977164, -0.05219959533909143690, 88.74890960531436690 ) ) ;
#113204=CARTESIAN_POINT ( 'NONE',  ( 5.719274019375673035, 21.55341960407619339, 97.29275706135234714 ) ) ;
#113206=CARTESIAN_POINT ( 'NONE',  ( -5.719274019375665041, -21.55341960407619695, 104.7927570613523898 ) ) ;
#113208=CARTESIAN_POINT ( 'NONE',  ( 16.51473224551069308, 9.474510206698969483, 104.1655762719810241 ) ) ;
#113209=CARTESIAN_POINT ( 'NONE',  ( -5.823673210054431948, 21.52544592524334988, 72.70942372801901854 ) ) ;
#113210=CARTESIAN_POINT ( 'NONE',  ( -12.06949235617739369, -12.14591786802326823, 24.37609039468567573 ) ) ;
#113211=CARTESIAN_POINT ( 'NONE',  ( 5.153800228976335163, 19.02544592524342804, 84.79057627198099567 ) ) ;
#113212=CARTESIAN_POINT ( 'NONE',  ( 21.55341960407610458, 5.719274019375980345, 33.95724293864769550 ) ) ;
#113213=CARTESIAN_POINT ( 'NONE',  ( 19.02544592524343514, -5.153800228976328945, 93.54057627198102409 ) ) ;
#113215=CARTESIAN_POINT ( 'NONE',  ( -19.05341960407611168, -5.049401038298163336, 71.45724293864766707 ) ) ;
#113216=CARTESIAN_POINT ( 'NONE',  ( -14.34966873604960291, -8.224510206698953496, 26.66557627198103475 ) ) ;
#113218=CARTESIAN_POINT ( 'NONE',  ( -13.89961937509957401, -13.97604488694547875, 74.37609039468566152 ) ) ;
#113219=CARTESIAN_POINT ( 'NONE',  ( -19.03943276465977164, 0.05219959533909376836, 96.24890960531436690 ) ) ;
#113220=CARTESIAN_POINT ( 'NONE',  ( 12.06949235617757843, -12.14591786802309237, 88.12390960531436690 ) ) ;
#113221=CARTESIAN_POINT ( 'NONE',  ( 21.53943276465977519, -0.05219959533907433946, 43.74890960531435979 ) ) ;
#113222=CARTESIAN_POINT ( 'NONE',  ( -21.53943276465977519, 0.05219959533907696930, 26.24890960531435624 ) ) ;
#113223=CARTESIAN_POINT ( 'NONE',  ( 0.05219959533910956823, 16.53943276465976808, 104.9989096053143669 ) ) ;
#113224=CARTESIAN_POINT ( 'NONE',  ( -17.49999999999999289, 5.500000000000034639, 55.79690382534172954 ) ) ;
#113225=CARTESIAN_POINT ( 'NONE',  ( 16.51473224551083163, -9.474510206698727899, 50.83442372801899722 ) ) ;
#113226=CARTESIAN_POINT ( 'NONE',  ( 16.55341960407611168, 4.379528057220329451, 28.95724293864769905 ) ) ;
#113227=CARTESIAN_POINT ( 'NONE',  ( 16.51473224551069308, 9.474510206698969483, 99.16557627198102409 ) ) ;
#113228=CARTESIAN_POINT ( 'NONE',  ( -15.80617190586768217, 15.72974639402176855, 68.12609039468567573 ) ) ;
#113229=CARTESIAN_POINT ( 'NONE',  ( 15.72974639402199770, -15.80617190586745480, 53.12390960531436690 ) ) ;
#113230=CARTESIAN_POINT ( 'NONE',  ( -5.823673210054431948, 21.52544592524334988, 42.70942372801901854 ) ) ;
#113231=CARTESIAN_POINT ( 'NONE',  ( 0.05219959533907565091, 21.53943276465977519, 94.99890960531436690 ) ) ;
#113232=CARTESIAN_POINT ( 'NONE',  ( 15.80617190586769283, -15.72974639402175789, 40.62609039468567573 ) ) ;
#113233=CARTESIAN_POINT ( 'NONE',  ( -4.483927247898539470, -16.52544592524342804, 107.2905762719810525 ) ) ;
#113234=CARTESIAN_POINT ( 'NONE',  ( 19.05341960407617918, -5.049401038297876454, 76.04275706135230450 ) ) ;
#113235=CARTESIAN_POINT ( 'NONE',  ( 16.51473224551069308, 9.474510206698969483, 64.16557627198102409 ) ) ;
#113236=CARTESIAN_POINT ( 'NONE',  ( -16.53943276465976808, 0.05219959533911058130, 106.2489096053143811 ) ) ;
#113237=CARTESIAN_POINT ( 'NONE',  ( -0.05219959533909027116, -19.03943276465977164, 112.4989096053143669 ) ) ;
#113238=CARTESIAN_POINT ( 'NONE',  ( -4.483927247898539470, -16.52544592524342804, 42.29057627198103120 ) ) ;
#113239=CARTESIAN_POINT ( 'NONE',  ( -12.06949235617739369, -12.14591786802326823, 109.3760903946857042 ) ) ;
#113240=CARTESIAN_POINT ( 'NONE',  ( 13.97604488694527802, 13.89961937509977652, 59.37390960531434558 ) ) ;
#113241=CARTESIAN_POINT ( 'NONE',  ( 16.52544592524342804, -4.483927247898539470, 113.5405762719810383 ) ) ;
#113242=CARTESIAN_POINT ( 'NONE',  ( 19.03943276465977164, 0.05219959533936151252, 31.25109039468566863 ) ) ;
#113243=CARTESIAN_POINT ( 'NONE',  ( -16.88567814943164791, -6.947325034625598583, 41.29001122652586986 ) ) ;
#113244=CARTESIAN_POINT ( 'NONE',  ( -16.55341960407611168, -4.379528057220339221, 31.45724293864769550 ) ) ;
#113245=CARTESIAN_POINT ( 'NONE',  ( -15.72974639402176322, -15.80617190586768395, 44.37609039468567573 ) ) ;
#113246=ADVANCED_FACE ( 'NONE', ( #158249 ), #19739, .F. ) ;
#113248=CARTESIAN_POINT ( 'NONE',  ( -12.14591786802326823, 12.06949235617739902, 58.12609039468568994 ) ) ;
#113249=CARTESIAN_POINT ( 'NONE',  ( -4.483927247898539470, -16.52544592524342804, 27.29057627198103120 ) ) ;
#113250=CARTESIAN_POINT ( 'NONE',  ( 0.05219959533934541429, -16.53943276465976808, 110.0010903946856757 ) ) ;
#113251=CARTESIAN_POINT ( 'NONE',  ( -9.564922557960796823, -16.46253265017161027, 32.08224293864769550 ) ) ;
#113252=CARTESIAN_POINT ( 'NONE',  ( -9.564922557960796823, -16.46253265017161027, 52.08224293864768839 ) ) ;
#113253=CARTESIAN_POINT ( 'NONE',  ( -5.153800228976328057, -19.02544592524343514, 32.29057627198102409 ) ) ;
#113254=CARTESIAN_POINT ( 'NONE',  ( -15.80617190586768217, 15.72974639402176855, 38.12609039468567573 ) ) ;
#113255=CARTESIAN_POINT ( 'NONE',  ( 9.474510206698971260, -16.51473224551069308, 42.91557627198103120 ) ) ;
#113257=CARTESIAN_POINT ( 'NONE',  ( 5.153800228976335163, 19.02544592524342804, 34.79057627198102409 ) ) ;
#113258=CARTESIAN_POINT ( 'NONE',  ( -21.53943276465977519, 0.05219959533907696930, 26.24890960531435624 ) ) ;
#113259=CARTESIAN_POINT ( 'NONE',  ( 18.67979575497194134, -10.72451020669871369, 45.83442372801901854 ) ) ;
#113260=CARTESIAN_POINT ( 'NONE',  ( 12.06949235617757843, -12.14591786802309237, 108.1239096053143811 ) ) ;
#113261=CARTESIAN_POINT ( 'NONE',  ( 13.97604488694527802, 13.89961937509977652, 114.3739096053143669 ) ) ;
#113262=CARTESIAN_POINT ( 'NONE',  ( -16.52544592524335698, -4.483927247898792601, 83.95942372801900433 ) ) ;
#113263=CARTESIAN_POINT ( 'NONE',  ( 21.52544592524334988, 5.823673210054432836, 96.45942372801901854 ) ) ;
#113264=CARTESIAN_POINT ( 'NONE',  ( 14.29746914071037800, 8.314922557961029526, 56.66775706135235424 ) ) ;
#113265=CARTESIAN_POINT ( 'NONE',  ( 5.153800228976335163, 19.02544592524342804, 94.79057627198103830 ) ) ;
#113266=CARTESIAN_POINT ( 'NONE',  ( -0.05219959533934338120, 16.53943276465976808, 42.50109039468567573 ) ) ;
#113267=CARTESIAN_POINT ( 'NONE',  ( 14.34966873604972726, -8.224510206698740333, 30.83442372801902209 ) ) ;
#113268=CARTESIAN_POINT ( 'NONE',  ( -16.52544592524335698, -4.483927247898792601, 78.95942372801901854 ) ) ;
#113269=CARTESIAN_POINT ( 'NONE',  ( -5.153800228976607833, 19.02544592524334988, 107.7094237280189759 ) ) ;
#113270=CARTESIAN_POINT ( 'NONE',  ( 5.049401038298161559, -19.05341960407611168, 82.70724293864770971 ) ) ;
#113271=CARTESIAN_POINT ( 'NONE',  ( -18.62759615963270932, 10.81492255796079327, 95.83224293864770971 ) ) ;
#113272=CARTESIAN_POINT ( 'NONE',  ( -12.06949235617756955, 12.14591786802309770, 100.6239096053143811 ) ) ;
#113273=CARTESIAN_POINT ( 'NONE',  ( -19.05341960407617563, 5.049401038297882671, 103.5427570613523329 ) ) ;
#113274=CARTESIAN_POINT ( 'NONE',  ( 16.53943276465976808, 0.05219959533934440121, 71.25109039468568994 ) ) ;
#113276=CARTESIAN_POINT ( 'NONE',  ( 13.89961937509957401, 13.97604488694547697, 76.87609039468566152 ) ) ;
#113278=CARTESIAN_POINT ( 'NONE',  ( -8.314922557960811034, -14.29746914071050412, 52.08224293864768839 ) ) ;
#113279=CARTESIAN_POINT ( 'NONE',  ( -4.483927247898539470, -16.52544592524342804, 97.29057627198105251 ) ) ;
#113280=CARTESIAN_POINT ( 'NONE',  ( -16.51473224551082808, 9.474510206698731452, 38.33442372801899722 ) ) ;
#113281=CARTESIAN_POINT ( 'NONE',  ( -17.49999999999999645, -5.500000000000000888, 120.0000000000000142 ) ) ;
#113282=CARTESIAN_POINT ( 'NONE',  ( -21.53943276465977519, -0.05219959533937600094, 43.75109039468568284 ) ) ;
#113283=CARTESIAN_POINT ( 'NONE',  ( 19.05341960407617918, -5.049401038297876454, 101.0427570613523045 ) ) ;
#113284=CARTESIAN_POINT ( 'NONE',  ( 0.05219959533909260263, 19.03943276465977164, 114.9989096053143669 ) ) ;
#113285=CARTESIAN_POINT ( 'NONE',  ( 13.89961937509977652, -13.97604488694527269, 98.12390960531433848 ) ) ;
#113286=CARTESIAN_POINT ( 'NONE',  ( -21.55341960407619339, 5.719274019375674811, 108.5427570613523756 ) ) ;
#113287=CARTESIAN_POINT ( 'NONE',  ( -19.03943276465977164, 0.05219959533909376836, 86.24890960531436690 ) ) ;
#113288=CARTESIAN_POINT ( 'NONE',  ( 5.719274019375991003, -21.55341960407610458, 37.70724293864769550 ) ) ;
#113289=CARTESIAN_POINT ( 'NONE',  ( 14.29746914071049879, -8.314922557960816363, 93.33224293864769550 ) ) ;
#113290=CARTESIAN_POINT ( 'NONE',  ( -16.46253265017160317, 9.564922557960807481, 60.83224293864769550 ) ) ;
#113291=CARTESIAN_POINT ( 'NONE',  ( 12.06949235617757843, -12.14591786802309237, 113.1239096053143953 ) ) ;
#113292=CARTESIAN_POINT ( 'NONE',  ( 21.52544592524334988, 5.823673210054432836, 26.45942372801901854 ) ) ;
#113293=CARTESIAN_POINT ( 'NONE',  ( 15.72974639402176855, 15.80617190586768217, 76.87609039468567573 ) ) ;
#113294=CARTESIAN_POINT ( 'NONE',  ( -9.474510206698964154, 16.51473224551069663, 40.41557627198103120 ) ) ;
#113295=CARTESIAN_POINT ( 'NONE',  ( 0.05219959533934541429, -16.53943276465976808, 80.00109039468568994 ) ) ;
#113296=CARTESIAN_POINT ( 'NONE',  ( -21.53943276465977519, -0.05219959533937600094, 18.75109039468568639 ) ) ;
#113297=CARTESIAN_POINT ( 'NONE',  ( 0.05219959533937995610, -21.53943276465977519, 25.00109039468567218 ) ) ;
#113298=CARTESIAN_POINT ( 'NONE',  ( 9.474510206698729675, 16.51473224551082808, 52.08442372801900433 ) ) ;
#113299=CARTESIAN_POINT ( 'NONE',  ( -19.03943276465977164, 0.05219959533909376836, 71.24890960531435269 ) ) ;
#113300=CARTESIAN_POINT ( 'NONE',  ( 16.51473224551083163, -9.474510206698727899, 25.83442372801900078 ) ) ;
#113301=CARTESIAN_POINT ( 'NONE',  ( -21.55341960407619339, 5.719274019375674811, 83.54275706135234714 ) ) ;
#113302=CARTESIAN_POINT ( 'NONE',  ( -21.52544592524343514, 5.823673210054127303, 76.04057627198102409 ) ) ;
#113303=CARTESIAN_POINT ( 'NONE',  ( -4.483927247898539470, -16.52544592524342804, 52.29057627198102409 ) ) ;
#113304=CARTESIAN_POINT ( 'NONE',  ( 10.72451020669871369, 18.67979575497193778, 92.08442372801901854 ) ) ;
#113305=CARTESIAN_POINT ( 'NONE',  ( -16.51473224551082808, 9.474510206698731452, 23.33442372801900078 ) ) ;
#113306=CARTESIAN_POINT ( 'NONE',  ( 4.483927247898545687, 16.52544592524342804, 74.79057627198105251 ) ) ;
#113307=CARTESIAN_POINT ( 'NONE',  ( -13.97604488694527625, -13.89961937509977652, 21.87390960531435979 ) ) ;
#113308=CARTESIAN_POINT ( 'NONE',  ( -13.89961937509957401, -13.97604488694547875, 59.37609039468566863 ) ) ;
#113309=CARTESIAN_POINT ( 'NONE',  ( -0.05219959533910754901, -16.53943276465976808, 27.49890960531435269 ) ) ;
#113310=CARTESIAN_POINT ( 'NONE',  ( 5.719274019375673035, 21.55341960407619339, 87.29275706135236135 ) ) ;
#113311=CARTESIAN_POINT ( 'NONE',  ( -16.46253265017160317, 9.564922557960807481, 75.83224293864769550 ) ) ;
#113312=CARTESIAN_POINT ( 'NONE',  ( -9.474510206698720793, -16.51473224551083518, 44.58442372801900433 ) ) ;
#113313=CARTESIAN_POINT ( 'NONE',  ( -18.62759615963270932, 10.81492255796079327, 45.83224293864769550 ) ) ;
#113314=CARTESIAN_POINT ( 'NONE',  ( 21.53943276465977519, 0.05219959533937863772, 46.25109039468567573 ) ) ;
#113315=CARTESIAN_POINT ( 'NONE',  ( -18.67979575497178146, -10.72451020669898902, 106.6655762719810383 ) ) ;
#113316=CARTESIAN_POINT ( 'NONE',  ( -13.97604488694547697, 13.89961937509957934, 93.12609039468566152 ) ) ;
#113317=CARTESIAN_POINT ( 'NONE',  ( 14.34966873604972726, -8.224510206698740333, 60.83442372801901854 ) ) ;
#113319=CARTESIAN_POINT ( 'NONE',  ( 21.52544592524344225, -5.823673210054117533, 108.5405762719810241 ) ) ;
#113320=CARTESIAN_POINT ( 'NONE',  ( -16.55341960407611168, -4.379528057220339221, 96.45724293864770971 ) ) ;
#113321=CARTESIAN_POINT ( 'NONE',  ( -17.49999999999999645, 5.499999999999997335, 120.0000000000000142 ) ) ;
#113322=CARTESIAN_POINT ( 'NONE',  ( -4.379528057220086978, -16.55341960407618274, 29.79275706135234358 ) ) ;
#113323=CARTESIAN_POINT ( 'NONE',  ( -21.53943276465977519, 0.05219959533907696930, 61.24890960531435979 ) ) ;
#113324=CARTESIAN_POINT ( 'NONE',  ( -8.224510206698735004, -14.34966873604973081, 94.58442372801901854 ) ) ;
#113325=CARTESIAN_POINT ( 'NONE',  ( -5.153800228976328057, -19.02544592524343514, 27.29057627198103120 ) ) ;
#113326=CARTESIAN_POINT ( 'NONE',  ( -8.224510206698735004, -14.34966873604973081, 69.58442372801900433 ) ) ;
#113327=CARTESIAN_POINT ( 'NONE',  ( 19.02544592524334988, 5.153800228976608722, 61.45942372801900433 ) ) ;
#113328=CARTESIAN_POINT ( 'NONE',  ( 5.719274019375673035, 21.55341960407619339, 47.29275706135234003 ) ) ;
#113329=CARTESIAN_POINT ( 'NONE',  ( 0.05219959533907565091, 21.53943276465977519, 64.99890960531435269 ) ) ;
#113330=CARTESIAN_POINT ( 'NONE',  ( -0.05219959533934338120, 16.53943276465976808, 82.50109039468568994 ) ) ;
#113331=CARTESIAN_POINT ( 'NONE',  ( 5.719274019375673035, 21.55341960407619339, 67.29275706135234714 ) ) ;
#113332=CARTESIAN_POINT ( 'NONE',  ( 10.81492255796078972, 18.62759615963270932, 54.58224293864769550 ) ) ;
#113333=CARTESIAN_POINT ( 'NONE',  ( -15.72974639402197994, 15.80617190586746368, 35.62390960531437401 ) ) ;
#113335=CARTESIAN_POINT ( 'NONE',  ( 4.379528057220092307, 16.55341960407617563, 67.29275706135234714 ) ) ;
#113336=CARTESIAN_POINT ( 'NONE',  ( -10.81492255796078084, -18.62759615963271287, 27.08224293864769550 ) ) ;
#113338=CARTESIAN_POINT ( 'NONE',  ( 13.97604488694527802, 13.89961937509977652, 104.3739096053143385 ) ) ;
#113339=CARTESIAN_POINT ( 'NONE',  ( -0.05219959533934338120, 16.53943276465976808, 107.5010903946856899 ) ) ;
#113341=CARTESIAN_POINT ( 'NONE',  ( 12.06949235617757843, -12.14591786802309237, 103.1239096053143811 ) ) ;
#113342=CARTESIAN_POINT ( 'NONE',  ( -18.62759615963270932, 10.81492255796079327, 60.83224293864769550 ) ) ;
#113343=CARTESIAN_POINT ( 'NONE',  ( -16.46253265017160317, 9.564922557960807481, 50.83224293864770260 ) ) ;
#113344=CARTESIAN_POINT ( 'NONE',  ( 12.14591786802327356, -12.06949235617739191, 95.62609039468568994 ) ) ;
#113345=CARTESIAN_POINT ( 'NONE',  ( -18.67979575497193778, 10.72451020669871902, 33.33442372801900433 ) ) ;
#113346=CARTESIAN_POINT ( 'NONE',  ( 13.89961937509957401, 13.97604488694547697, 101.8760903946856331 ) ) ;
#113347=CARTESIAN_POINT ( 'NONE',  ( -14.34966873604960291, -8.224510206698953496, 101.6655762719810383 ) ) ;
#113348=CARTESIAN_POINT ( 'NONE',  ( 0.05219959533909260263, 19.03943276465977164, 54.99890960531435979 ) ) ;
#113349=CARTESIAN_POINT ( 'NONE',  ( -9.564922557960796823, -16.46253265017161027, 22.08224293864768839 ) ) ;
#113350=CARTESIAN_POINT ( 'NONE',  ( 17.48847506799968698, -5.747544572773780835, 38.32697437843281563 ) ) ;
#113351=CARTESIAN_POINT ( 'NONE',  ( -9.474510206698964154, 16.51473224551069663, 90.41557627198103830 ) ) ;
#113352=CARTESIAN_POINT ( 'NONE',  ( 8.224510206698742110, 14.34966873604972548, 77.08442372801901854 ) ) ;
#113353=CARTESIAN_POINT ( 'NONE',  ( 5.823673210054444382, -21.52544592524334988, 105.2094237280190328 ) ) ;
#113354=CARTESIAN_POINT ( 'NONE',  ( 18.62759615963271287, -10.81492255796078972, 53.33224293864769550 ) ) ;
#113355=CARTESIAN_POINT ( 'NONE',  ( -8.314922557961024197, 14.29746914071037800, 77.91775706135231871 ) ) ;
#113356=CARTESIAN_POINT ( 'NONE',  ( 9.474510206698729675, 16.51473224551082808, 77.08442372801900433 ) ) ;
#113358=CARTESIAN_POINT ( 'NONE',  ( 16.46253265017160672, -9.564922557960803928, 38.33224293864768839 ) ) ;
#113359=CARTESIAN_POINT ( 'NONE',  ( 16.51473224551069308, 9.474510206698969483, 79.16557627198103830 ) ) ;
#113360=CARTESIAN_POINT ( 'NONE',  ( -16.51473224551069308, -9.474510206698971260, 36.66557627198102409 ) ) ;
#113361=CARTESIAN_POINT ( 'NONE',  ( -5.153800228976607833, 19.02544592524334988, 77.70942372801900433 ) ) ;
#113362=CARTESIAN_POINT ( 'NONE',  ( -19.02544592524342804, 5.153800228976336051, 116.0405762719810383 ) ) ;
#113363=CARTESIAN_POINT ( 'NONE',  ( -0.05219959533909027116, -19.03943276465977164, 92.49890960531436690 ) ) ;
#113364=CARTESIAN_POINT ( 'NONE',  ( -8.314922557960811034, -14.29746914071050412, 47.08224293864770260 ) ) ;
#113365=CARTESIAN_POINT ( 'NONE',  ( 15.80617190586746368, 15.72974639402197994, 44.37390960531435979 ) ) ;
#113367=CARTESIAN_POINT ( 'NONE',  ( -13.97604488694547697, 13.89961937509957934, 33.12609039468566863 ) ) ;
#113368=CARTESIAN_POINT ( 'NONE',  ( -16.20579543436678449, -7.371946100355090792, 80.56520834171877254 ) ) ;
#113369=CARTESIAN_POINT ( 'NONE',  ( -13.89961937509977652, 13.97604488694528158, 50.62390960531435979 ) ) ;
#113370=CARTESIAN_POINT ( 'NONE',  ( -14.29746914071037622, -8.314922557961029526, 44.16775706135234714 ) ) ;
#113371=CARTESIAN_POINT ( 'NONE',  ( -19.39720447994794128, -5.500000000000030198, 99.66317477297174321 ) ) ;
#113372=CARTESIAN_POINT ( 'NONE',  ( -16.61371651742600974, 7.165104196376152146, 108.8541506999299884 ) ) ;
#113373=CARTESIAN_POINT ( 'NONE',  ( 0.05219959533934541429, -16.53943276465976808, 80.00109039468568994 ) ) ;
#113374=CARTESIAN_POINT ( 'NONE',  ( 21.53943276465977519, -0.05219959533907433946, 93.74890960531436690 ) ) ;
#113375=CARTESIAN_POINT ( 'NONE',  ( -4.483927247898782831, 16.52544592524335698, 47.70942372801902565 ) ) ;
#113376=CARTESIAN_POINT ( 'NONE',  ( 19.03943276465977164, -0.05219959533909143690, 38.74890960531436690 ) ) ;
#113378=CARTESIAN_POINT ( 'NONE',  ( -15.80617190586768217, 15.72974639402176855, 43.12609039468568284 ) ) ;
#113379=CARTESIAN_POINT ( 'NONE',  ( 9.474510206698729675, 16.51473224551082808, 47.08442372801900433 ) ) ;
#113380=CARTESIAN_POINT ( 'NONE',  ( -5.719274019375665041, -21.55341960407619695, 94.79275706135234714 ) ) ;
#113381=CARTESIAN_POINT ( 'NONE',  ( 17.44279575226823198, 5.990770900252457842, 96.66442432485682446 ) ) ;
#113382=CARTESIAN_POINT ( 'NONE',  ( 16.55341960407611168, 4.379528057220329451, 38.95724293864768839 ) ) ;
#113384=CARTESIAN_POINT ( 'NONE',  ( -21.52544592524343514, 5.823673210054127303, 51.04057627198103120 ) ) ;
#113386=CARTESIAN_POINT ( 'NONE',  ( 16.46253265017160672, -9.564922557960803928, 103.3322429386476955 ) ) ;
#113387=CARTESIAN_POINT ( 'NONE',  ( -0.05219959533910754901, -16.53943276465976808, 102.4989096053143811 ) ) ;
#113388=CARTESIAN_POINT ( 'NONE',  ( -16.51473224551082808, 9.474510206698731452, 113.3344237280190043 ) ) ;
#113389=CARTESIAN_POINT ( 'NONE',  ( -12.14591786802326823, 12.06949235617739902, 108.1260903946856757 ) ) ;
#113391=CARTESIAN_POINT ( 'NONE',  ( 0.05219959533909260263, 19.03943276465977164, 99.99890960531436690 ) ) ;
#113392=CARTESIAN_POINT ( 'NONE',  ( -21.53943276465977519, 0.05219959533907696930, 106.2489096053143811 ) ) ;
#113393=CARTESIAN_POINT ( 'NONE',  ( 8.314922557960818139, 14.29746914071049879, 24.58224293864768839 ) ) ;
#113394=CARTESIAN_POINT ( 'NONE',  ( 13.97604488694527802, 13.89961937509977652, 99.37390960531436690 ) ) ;
#113395=CARTESIAN_POINT ( 'NONE',  ( -5.153800228976607833, 19.02544592524334988, 97.70942372801900433 ) ) ;
#113396=CARTESIAN_POINT ( 'NONE',  ( 21.55341960407619695, -5.719274019375665929, 111.0427570613523613 ) ) ;
#113397=CARTESIAN_POINT ( 'NONE',  ( 0.05219959533907565091, 21.53943276465977519, 84.99890960531436690 ) ) ;
#113398=CARTESIAN_POINT ( 'NONE',  ( -0.05219959533907301413, -21.53943276465977519, 52.49890960531435979 ) ) ;
#113399=CARTESIAN_POINT ( 'NONE',  ( -16.46253265017160317, 9.564922557960807481, 65.83224293864769550 ) ) ;
#113400=CARTESIAN_POINT ( 'NONE',  ( 16.55341960407611168, 4.379528057220329451, 33.95724293864769550 ) ) ;
#113401=CARTESIAN_POINT ( 'NONE',  ( -16.46253265017160317, 9.564922557960807481, 70.83224293864770971 ) ) ;
#113402=CARTESIAN_POINT ( 'NONE',  ( 18.89770734986052503, 5.499999999999904077, 56.60214472496641491 ) ) ;
#113403=CARTESIAN_POINT ( 'NONE',  ( -9.564922557961040184, 16.46253265017147172, 37.91775706135233293 ) ) ;
#113404=CARTESIAN_POINT ( 'NONE',  ( 15.72974639402199770, -15.80617190586745480, 83.12390960531436690 ) ) ;
#113405=CARTESIAN_POINT ( 'NONE',  ( 12.06949235617757843, -12.14591786802309237, 88.12390960531436690 ) ) ;
#113406=CARTESIAN_POINT ( 'NONE',  ( -15.80617190586768217, 15.72974639402176855, 38.12609039468567573 ) ) ;
#113408=CARTESIAN_POINT ( 'NONE',  ( 4.379528057220092307, 16.55341960407617563, 112.2927570613523471 ) ) ;
#113409=CARTESIAN_POINT ( 'NONE',  ( -5.153800228976328057, -19.02544592524343514, 27.29057627198103120 ) ) ;
#113410=CARTESIAN_POINT ( 'NONE',  ( -13.89961937509977652, 13.97604488694528158, 85.62390960531433848 ) ) ;
#113412=CARTESIAN_POINT ( 'NONE',  ( -0.05219959533910754901, -16.53943276465976808, 42.49890960531435979 ) ) ;
#113413=CARTESIAN_POINT ( 'NONE',  ( -18.67979575497193778, 10.72451020669871902, 58.33442372801901143 ) ) ;
#113415=CARTESIAN_POINT ( 'NONE',  ( 5.049401038298161559, -19.05341960407611168, 37.70724293864768839 ) ) ;
#113416=CARTESIAN_POINT ( 'NONE',  ( -16.46253265017160317, 9.564922557960807481, 45.83224293864769550 ) ) ;
#113418=CARTESIAN_POINT ( 'NONE',  ( -5.823673210054431948, 21.52544592524334988, 102.7094237280190185 ) ) ;
#113419=CARTESIAN_POINT ( 'NONE',  ( 14.29746914071037800, 8.314922557961029526, 66.66775706135234714 ) ) ;
#113420=CARTESIAN_POINT ( 'NONE',  ( 15.80617190586769283, -15.72974639402175789, 90.62609039468567573 ) ) ;
#113421=CARTESIAN_POINT ( 'NONE',  ( 19.02544592524343514, -5.153800228976328945, 113.5405762719810241 ) ) ;
#113422=CARTESIAN_POINT ( 'NONE',  ( -13.97604488694547697, 13.89961937509957934, 88.12609039468563310 ) ) ;
#113423=CARTESIAN_POINT ( 'NONE',  ( 10.72451020669871369, 18.67979575497193778, 67.08442372801901854 ) ) ;
#113424=CARTESIAN_POINT ( 'NONE',  ( 8.224510206698742110, 14.34966873604972548, 32.08442372801901854 ) ) ;
#113425=CARTESIAN_POINT ( 'NONE',  ( -5.719274019375978568, 21.55341960407610458, 90.20724293864770971 ) ) ;
#113426=CARTESIAN_POINT ( 'NONE',  ( -13.97604488694547697, 13.89961937509957934, 98.12609039468566152 ) ) ;
#113427=CARTESIAN_POINT ( 'NONE',  ( 9.474510206698971260, -16.51473224551069308, 62.91557627198102409 ) ) ;
#113428=CARTESIAN_POINT ( 'NONE',  ( 0.05219959533936267826, -19.03943276465977164, 105.0010903946856615 ) ) ;
#113429=CARTESIAN_POINT ( 'NONE',  ( -5.049401038297874678, -19.05341960407617918, 99.79275706135234714 ) ) ;
#113430=CARTESIAN_POINT ( 'NONE',  ( 12.06949235617757843, -12.14591786802309237, 58.12390960531435979 ) ) ;
#113431=CARTESIAN_POINT ( 'NONE',  ( -9.564922557961040184, 16.46253265017147172, 72.91775706135233293 ) ) ;
#113432=CARTESIAN_POINT ( 'NONE',  ( -16.55341960407617563, 4.379528057220093196, 78.54275706135236135 ) ) ;
#113433=CARTESIAN_POINT ( 'NONE',  ( -5.823673210054116645, -21.52544592524344225, 112.2905762719810241 ) ) ;
#113434=CARTESIAN_POINT ( 'NONE',  ( -19.05341960407611168, -5.049401038298163336, 36.45724293864766707 ) ) ;
#113435=CARTESIAN_POINT ( 'NONE',  ( -16.46253265017160317, 9.564922557960807481, 50.83224293864770260 ) ) ;
#113436=CARTESIAN_POINT ( 'NONE',  ( -8.314922557961024197, 14.29746914071037800, 52.91775706135235424 ) ) ;
#113439=CARTESIAN_POINT ( 'NONE',  ( -19.05341960407611168, -5.049401038298163336, 111.4572429386476671 ) ) ;
#113442=CARTESIAN_POINT ( 'NONE',  ( 16.51473224551083163, -9.474510206698727899, 110.8344237280190043 ) ) ;
#113443=CARTESIAN_POINT ( 'NONE',  ( -0.05219959533907301413, -21.53943276465977519, 47.49890960531435979 ) ) ;
#113444=CARTESIAN_POINT ( 'NONE',  ( 0.05219959533936267826, -19.03943276465977164, 45.00109039468566863 ) ) ;
#113445=CARTESIAN_POINT ( 'NONE',  ( 14.34966873604972726, -8.224510206698740333, 30.83442372801902209 ) ) ;
#113446=CARTESIAN_POINT ( 'NONE',  ( -5.049401038298153566, 19.05341960407611168, 30.20724293864768839 ) ) ;
#113447=CARTESIAN_POINT ( 'NONE',  ( 9.564922557960805705, 16.46253265017160317, 54.58224293864769550 ) ) ;
#113448=CARTESIAN_POINT ( 'NONE',  ( -21.52544592524343514, 5.823673210054127303, 86.04057627198102409 ) ) ;
#113449=CARTESIAN_POINT ( 'NONE',  ( -16.46253265017160317, 9.564922557960807481, 105.8322429386476955 ) ) ;
#113450=CARTESIAN_POINT ( 'NONE',  ( -0.05219959533909027116, -19.03943276465977164, 47.49890960531435979 ) ) ;
#113451=CARTESIAN_POINT ( 'NONE',  ( -17.60769864724391098, 5.499999999999985789, 93.65024842019165874 ) ) ;
#113452=CARTESIAN_POINT ( 'NONE',  ( -5.049401038297874678, -19.05341960407617918, 89.79275706135230450 ) ) ;
#113453=CARTESIAN_POINT ( 'NONE',  ( -14.34966873604960291, -8.224510206698953496, 61.66557627198103120 ) ) ;
#113454=CARTESIAN_POINT ( 'NONE',  ( -15.80617190586768217, 15.72974639402176855, 103.1260903946856757 ) ) ;
#113455=CARTESIAN_POINT ( 'NONE',  ( -10.81492255796078084, -18.62759615963271287, 92.08224293864769550 ) ) ;
#113456=CARTESIAN_POINT ( 'NONE',  ( -21.52544592524334988, -5.823673210054445271, 88.95942372801901854 ) ) ;
#113457=CARTESIAN_POINT ( 'NONE',  ( -19.05341960407611168, -5.049401038298163336, 21.45724293864768839 ) ) ;
#113458=CARTESIAN_POINT ( 'NONE',  ( 21.53943276465977519, 0.05219959533937863772, 76.25109039468568994 ) ) ;
#113459=CARTESIAN_POINT ( 'NONE',  ( 19.05341960407611168, 5.049401038298154454, 103.9572429386476671 ) ) ;
#113460=CARTESIAN_POINT ( 'NONE',  ( 16.52544592524342804, -4.483927247898539470, 33.54057627198102409 ) ) ;
#113461=CARTESIAN_POINT ( 'NONE',  ( 0.05219959533937995610, -21.53943276465977519, 75.00109039468568994 ) ) ;
#113462=CARTESIAN_POINT ( 'NONE',  ( 13.89961937509977652, -13.97604488694527269, 63.12390960531435979 ) ) ;
#113463=CARTESIAN_POINT ( 'NONE',  ( 10.81492255796106328, -18.62759615963255655, 45.41775706135234003 ) ) ;
#113464=CARTESIAN_POINT ( 'NONE',  ( -19.05341960407611168, -5.049401038298163336, 86.45724293864769550 ) ) ;
#113465=CARTESIAN_POINT ( 'NONE',  ( 4.483927247898545687, 16.52544592524342804, 94.79057627198105251 ) ) ;
#113466=CARTESIAN_POINT ( 'NONE',  ( 0.05219959533910956823, 16.53943276465976808, 64.99890960531435269 ) ) ;
#113467=CARTESIAN_POINT ( 'NONE',  ( 18.67979575497178502, 10.72451020669898547, 74.16557627198102409 ) ) ;
#113468=CARTESIAN_POINT ( 'NONE',  ( -16.46253265017160317, 9.564922557960807481, 65.83224293864769550 ) ) ;
#113469=CARTESIAN_POINT ( 'NONE',  ( -15.80617190586745835, -15.72974639402198527, 71.87390960531438111 ) ) ;
#113470=CARTESIAN_POINT ( 'NONE',  ( 0.05219959533936267826, -19.03943276465977164, 60.00109039468566863 ) ) ;
#113471=CARTESIAN_POINT ( 'NONE',  ( 0.05219959533936267826, -19.03943276465977164, 30.00109039468566863 ) ) ;
#113472=CARTESIAN_POINT ( 'NONE',  ( -0.05219959533910754901, -16.53943276465976808, 77.49890960531433848 ) ) ;
#113473=CARTESIAN_POINT ( 'NONE',  ( -18.67979575497178146, -10.72451020669898902, 46.66557627198102409 ) ) ;
#113475=DIRECTION ( 'NONE',  ( -0.5150380737757255245, 0.000000000000000000, 0.8571673013836856869 ) ) ;
#113476=CARTESIAN_POINT ( 'NONE',  ( 14.34966873604972726, -8.224510206698740333, 100.8344237280190185 ) ) ;
#113478=CARTESIAN_POINT ( 'NONE',  ( -13.97604488694547697, 13.89961937509957934, 98.12609039468566152 ) ) ;
#113479=CARTESIAN_POINT ( 'NONE',  ( -14.29746914071049879, 8.314922557960819915, 70.83224293864770971 ) ) ;
#113481=CARTESIAN_POINT ( 'NONE',  ( 19.05341960407611168, 5.049401038298154454, 63.95724293864769550 ) ) ;
#113482=CARTESIAN_POINT ( 'NONE',  ( 12.14591786802309770, 12.06949235617756955, 54.37390960531435979 ) ) ;
#113483=CARTESIAN_POINT ( 'NONE',  ( 9.474510206698971260, -16.51473224551069308, 102.9155762719810241 ) ) ;
#113484=CARTESIAN_POINT ( 'NONE',  ( 19.03943276465977164, 0.05219959533936151252, 81.25109039468567573 ) ) ;
#113485=CARTESIAN_POINT ( 'NONE',  ( -9.474510206698964154, 16.51473224551069663, 65.41557627198102409 ) ) ;
#113486=CARTESIAN_POINT ( 'NONE',  ( 5.153800228976335163, 19.02544592524342804, 89.79057627198102409 ) ) ;
#113487=CARTESIAN_POINT ( 'NONE',  ( 9.474510206698971260, -16.51473224551069308, 67.91557627198102409 ) ) ;
#113488=CARTESIAN_POINT ( 'NONE',  ( -10.72451020669898014, 18.67979575497178502, 65.41557627198102409 ) ) ;
#113489=CARTESIAN_POINT ( 'NONE',  ( -12.14591786802326823, 12.06949235617739902, 58.12609039468568994 ) ) ;
#113491=CARTESIAN_POINT ( 'NONE',  ( 16.51473224551069308, 9.474510206698969483, 54.16557627198103120 ) ) ;
#113492=CARTESIAN_POINT ( 'NONE',  ( 15.72974639402199770, -15.80617190586745480, 48.12390960531436690 ) ) ;
#113493=CARTESIAN_POINT ( 'NONE',  ( -5.153800228976607833, 19.02544592524334988, 82.70942372801897591 ) ) ;
#113494=CARTESIAN_POINT ( 'NONE',  ( 14.29746914071049879, -8.314922557960816363, 28.33224293864769550 ) ) ;
#113495=CARTESIAN_POINT ( 'NONE',  ( -15.72974639402176322, -15.80617190586768395, 34.37609039468568284 ) ) ;
#113496=CARTESIAN_POINT ( 'NONE',  ( 5.153800228976615827, -19.02544592524334988, 40.20942372801898301 ) ) ;
#113497=CARTESIAN_POINT ( 'NONE',  ( -16.52544592524335698, -4.483927247898792601, 63.95942372801901854 ) ) ;
#113498=CARTESIAN_POINT ( 'NONE',  ( -8.314922557961024197, 14.29746914071037800, 87.91775706135234714 ) ) ;
#113500=CARTESIAN_POINT ( 'NONE',  ( -0.05219959533934338120, 16.53943276465976808, 77.50109039468567573 ) ) ;
#113501=CARTESIAN_POINT ( 'NONE',  ( 18.67979575497178502, 10.72451020669898547, 24.16557627198103120 ) ) ;
#113502=CARTESIAN_POINT ( 'NONE',  ( 16.55341960407618274, -4.379528057220086978, 31.04275706135234714 ) ) ;
#113503=CARTESIAN_POINT ( 'NONE',  ( 5.153800228976335163, 19.02544592524342804, 44.79057627198103830 ) ) ;
#113504=CARTESIAN_POINT ( 'NONE',  ( -13.89961937509977652, 13.97604488694528158, 55.62390960531434558 ) ) ;
#113505=CARTESIAN_POINT ( 'NONE',  ( 13.89961937509977652, -13.97604488694527269, 58.12390960531436690 ) ) ;
#113506=CARTESIAN_POINT ( 'NONE',  ( 18.62759615963255655, 10.81492255796105972, 36.66775706135234714 ) ) ;
#113507=CARTESIAN_POINT ( 'NONE',  ( 14.34966873604972726, -8.224510206698740333, 45.83442372801901854 ) ) ;
#113508=CARTESIAN_POINT ( 'NONE',  ( -12.14591786802326823, 12.06949235617739902, 113.1260903946856899 ) ) ;
#113509=CARTESIAN_POINT ( 'NONE',  ( 9.474510206698971260, -16.51473224551069308, 27.91557627198103120 ) ) ;
#113510=CARTESIAN_POINT ( 'NONE',  ( 21.53943276465977519, 0.05219959533937863772, 111.2510903946856899 ) ) ;
#113511=CARTESIAN_POINT ( 'NONE',  ( -19.02544592524334988, -5.153800228976617603, 103.9594237280190043 ) ) ;
#113513=CARTESIAN_POINT ( 'NONE',  ( -19.05341960407617563, 5.049401038297882671, 63.54275706135234003 ) ) ;
#113514=CARTESIAN_POINT ( 'NONE',  ( -4.379528057220328563, 16.55341960407611168, 70.20724293864769550 ) ) ;
#113515=CARTESIAN_POINT ( 'NONE',  ( -13.97604488694527625, -13.89961937509977652, 31.87390960531435979 ) ) ;
#113516=CARTESIAN_POINT ( 'NONE',  ( -16.51473224551082808, 9.474510206698731452, 78.33442372801900433 ) ) ;
#113518=CARTESIAN_POINT ( 'NONE',  ( 10.72451020669871369, 18.67979575497193778, 77.08442372801901854 ) ) ;
#113519=CARTESIAN_POINT ( 'NONE',  ( -12.06949235617739369, -12.14591786802326823, 44.37609039468567573 ) ) ;
#113520=CARTESIAN_POINT ( 'NONE',  ( 17.50000000000000000, 5.499999999999992895, 38.78230962303566542 ) ) ;
#113521=CARTESIAN_POINT ( 'NONE',  ( -18.62759615963270932, 10.81492255796079327, 40.83224293864769550 ) ) ;
#113522=CARTESIAN_POINT ( 'NONE',  ( 12.14591786802327356, -12.06949235617739191, 30.62609039468567929 ) ) ;
#113523=CARTESIAN_POINT ( 'NONE',  ( -19.05341960407611168, -5.049401038298164224, 21.45724293864768839 ) ) ;
#113524=CARTESIAN_POINT ( 'NONE',  ( 5.153800228976615827, -19.02544592524334988, 35.20942372801899722 ) ) ;
#113526=CARTESIAN_POINT ( 'NONE',  ( 9.474510206698971260, -16.51473224551069308, 32.91557627198102409 ) ) ;
#113528=CARTESIAN_POINT ( 'NONE',  ( 9.474510206698971260, -16.51473224551069308, 57.91557627198103120 ) ) ;
#113529=CARTESIAN_POINT ( 'NONE',  ( -18.87075004821569024, 5.499999999999997335, 98.67408112101047379 ) ) ;
#113530=CARTESIAN_POINT ( 'NONE',  ( -0.05219959533936034679, 19.03943276465977164, 22.50109039468566152 ) ) ;
#113531=CARTESIAN_POINT ( 'NONE',  ( 16.55341960407618274, -4.379528057220086978, 111.0427570613523613 ) ) ;
#113532=CARTESIAN_POINT ( 'NONE',  ( -13.97604488694527625, -13.89961937509977652, 26.87390960531434558 ) ) ;
#113533=CARTESIAN_POINT ( 'NONE',  ( -19.03943276465977164, 0.05219959533909376836, 91.24890960531436690 ) ) ;
#113534=CARTESIAN_POINT ( 'NONE',  ( -18.62759615963255300, -10.81492255796106328, 64.16775706135234714 ) ) ;
#113535=CARTESIAN_POINT ( 'NONE',  ( 5.049401038298161559, -19.05341960407611168, 37.70724293864768839 ) ) ;
#113536=CARTESIAN_POINT ( 'NONE',  ( -5.823673210054431948, 21.52544592524334988, 72.70942372801901854 ) ) ;
#113537=CARTESIAN_POINT ( 'NONE',  ( -19.02544592524334988, -5.153800228976617603, 93.95942372801900433 ) ) ;
#113538=CARTESIAN_POINT ( 'NONE',  ( -9.564922557960796823, -16.46253265017161027, 102.0822429386477097 ) ) ;
#113539=CARTESIAN_POINT ( 'NONE',  ( 13.97604488694527802, 13.89961937509977652, 39.37390960531435269 ) ) ;
#113540=CARTESIAN_POINT ( 'NONE',  ( -5.719274019375978568, 21.55341960407610458, 110.2072429386477239 ) ) ;
#113541=CARTESIAN_POINT ( 'NONE',  ( -5.153800228976607833, 19.02544592524334988, 37.70942372801899722 ) ) ;
#113542=CARTESIAN_POINT ( 'NONE',  ( -8.224510206698948167, 14.34966873604960824, 115.4155762719810241 ) ) ;
#113543=CARTESIAN_POINT ( 'NONE',  ( -16.51473224551069308, -9.474510206698971260, 61.66557627198103120 ) ) ;
#113544=CARTESIAN_POINT ( 'NONE',  ( 5.049401038297881783, 19.05341960407617563, 92.29275706135234714 ) ) ;
#113545=CARTESIAN_POINT ( 'NONE',  ( -16.53943276465976808, 0.05219959533911058130, 71.24890960531435269 ) ) ;
#113546=CARTESIAN_POINT ( 'NONE',  ( 21.55341960407610458, 5.719274019375980345, 28.95724293864769905 ) ) ;
#113547=CARTESIAN_POINT ( 'NONE',  ( 9.474510206698729675, 16.51473224551082808, 82.08442372801899012 ) ) ;
#113548=CARTESIAN_POINT ( 'NONE',  ( -21.55341960407610458, -5.719274019375992779, 86.45724293864770971 ) ) ;
#113549=CARTESIAN_POINT ( 'NONE',  ( -10.81492255796105439, 18.62759615963255655, 37.91775706135235424 ) ) ;
#113550=CARTESIAN_POINT ( 'NONE',  ( -16.53943276465976808, -0.05219959533934237506, 48.75109039468568284 ) ) ;
#113551=CARTESIAN_POINT ( 'NONE',  ( 8.224510206698742110, 14.34966873604972548, 52.08442372801901854 ) ) ;
#113552=CARTESIAN_POINT ( 'NONE',  ( -21.53943276465977519, -0.05219959533937600094, 53.75109039468568994 ) ) ;
#113553=CARTESIAN_POINT ( 'NONE',  ( -10.81492255796078084, -18.62759615963271287, 57.08224293864769550 ) ) ;
#113554=CARTESIAN_POINT ( 'NONE',  ( 0.05219959533909260263, 19.03943276465977164, 44.99890960531435979 ) ) ;
#113556=CARTESIAN_POINT ( 'NONE',  ( 8.224510206698742110, 14.34966873604972548, 77.08442372801901854 ) ) ;
#113557=CARTESIAN_POINT ( 'NONE',  ( -18.67979575497178146, -10.72451020669898902, 96.66557627198102409 ) ) ;
#113558=CARTESIAN_POINT ( 'NONE',  ( 4.483927247898545687, 16.52544592524342804, 34.79057627198103120 ) ) ;
#113559=CARTESIAN_POINT ( 'NONE',  ( 16.52544592524335698, 4.483927247898782831, 66.45942372801903275 ) ) ;
#113560=CARTESIAN_POINT ( 'NONE',  ( 16.46253265017146816, 9.564922557961045513, 101.6677570613523329 ) ) ;
#113561=CARTESIAN_POINT ( 'NONE',  ( 21.53943276465977519, -0.05219959533907433946, 103.7489096053143669 ) ) ;
#113562=CARTESIAN_POINT ( 'NONE',  ( 14.29746914071049879, -8.314922557960816363, 48.33224293864770260 ) ) ;
#113564=CARTESIAN_POINT ( 'NONE',  ( -16.55341960407617563, 4.379528057220093196, 73.54275706135234714 ) ) ;
#113565=CARTESIAN_POINT ( 'NONE',  ( 19.36337904590691394, -5.500000000000039080, 92.91494137495617167 ) ) ;
#113566=CARTESIAN_POINT ( 'NONE',  ( -21.52544592524343514, 5.823673210054127303, 71.04057627198103830 ) ) ;
#113567=CARTESIAN_POINT ( 'NONE',  ( 16.55341960407611168, 4.379528057220329451, 23.95724293864769550 ) ) ;
#113569=CARTESIAN_POINT ( 'NONE',  ( -17.48847506799969054, -5.747544572773812810, 54.17302562156721280 ) ) ;
#113570=CARTESIAN_POINT ( 'NONE',  ( 5.823673210054125526, 21.52544592524343514, 99.79057627198103830 ) ) ;
#113571=CARTESIAN_POINT ( 'NONE',  ( 15.80617190586746368, 15.72974639402197994, 109.3739096053143811 ) ) ;
#113572=CARTESIAN_POINT ( 'NONE',  ( 4.483927247898545687, 16.52544592524342804, 39.79057627198103830 ) ) ;
#113573=CARTESIAN_POINT ( 'NONE',  ( 16.52544592524335698, 4.483927247898782831, 46.45942372801901854 ) ) ;
#113574=CARTESIAN_POINT ( 'NONE',  ( 9.564922557960805705, 16.46253265017160317, 49.58224293864770260 ) ) ;
#113575=CARTESIAN_POINT ( 'NONE',  ( -13.97604488694527625, -13.89961937509977652, 71.87390960531433848 ) ) ;
#113576=VERTEX_POINT ( 'NONE', #161241 ) ;
#113577=CARTESIAN_POINT ( 'NONE',  ( 15.80617190586746368, 15.72974639402197994, 24.37390960531435979 ) ) ;
#113579=CARTESIAN_POINT ( 'NONE',  ( 13.97604488694548053, -13.89961937509957401, 100.6260903946856615 ) ) ;
#113580=CARTESIAN_POINT ( 'NONE',  ( -13.89961937509957401, -13.97604488694547875, 54.37609039468565442 ) ) ;
#113581=CARTESIAN_POINT ( 'NONE',  ( 5.823673210054125526, 21.52544592524343514, 94.79057627198105251 ) ) ;
#113582=CARTESIAN_POINT ( 'NONE',  ( -16.52544592524335698, -4.483927247898792601, 108.9594237280190185 ) ) ;
#113584=CARTESIAN_POINT ( 'NONE',  ( -13.89961937509977652, 13.97604488694528158, 75.62390960531438111 ) ) ;
#113585=CARTESIAN_POINT ( 'NONE',  ( -18.62759615963270932, 10.81492255796079327, 40.83224293864769550 ) ) ;
#113586=CARTESIAN_POINT ( 'NONE',  ( 21.53943276465977519, -0.05219959533907433946, 78.74890960531436690 ) ) ;
#113587=CARTESIAN_POINT ( 'NONE',  ( -16.52544592524335698, -4.483927247898792601, 28.95942372801902209 ) ) ;
#113588=CARTESIAN_POINT ( 'NONE',  ( 15.72974639402199770, -15.80617190586745480, 28.12390960531435979 ) ) ;
#113589=CARTESIAN_POINT ( 'NONE',  ( 10.81492255796106328, -18.62759615963255655, 80.41775706135234714 ) ) ;
#113590=CARTESIAN_POINT ( 'NONE',  ( 9.564922557960805705, 16.46253265017160317, 74.58224293864769550 ) ) ;
#113591=CARTESIAN_POINT ( 'NONE',  ( 9.474510206698971260, -16.51473224551069308, 22.91557627198102765 ) ) ;
#113592=CARTESIAN_POINT ( 'NONE',  ( 19.05341960407611168, 5.049401038298154454, 88.95724293864769550 ) ) ;
#113593=CARTESIAN_POINT ( 'NONE',  ( 14.34966873604960469, 8.224510206698951720, 89.16557627198102409 ) ) ;
#113595=CARTESIAN_POINT ( 'NONE',  ( 16.51473224551083163, -9.474510206698727899, 100.8344237280190043 ) ) ;
#113597=CARTESIAN_POINT ( 'NONE',  ( -19.03943276465977164, 0.05219959533909376836, 76.24890960531435269 ) ) ;
#113598=CARTESIAN_POINT ( 'NONE',  ( 5.823673210054444382, -21.52544592524334988, 80.20942372801901854 ) ) ;
#113599=CARTESIAN_POINT ( 'NONE',  ( -9.564922557960796823, -16.46253265017161027, 102.0822429386477097 ) ) ;
#113600=CARTESIAN_POINT ( 'NONE',  ( 4.379528057220092307, 16.55341960407617563, 77.29275706135234714 ) ) ;
#113602=CARTESIAN_POINT ( 'NONE',  ( 16.46253265017146816, 9.564922557961045513, 51.66775706135233293 ) ) ;
#113603=CARTESIAN_POINT ( 'NONE',  ( 16.51473224551083163, -9.474510206698727899, 20.83442372801899722 ) ) ;
#113607=CARTESIAN_POINT ( 'NONE',  ( -14.34966873604960291, -8.224510206698953496, 21.66557627198102409 ) ) ;
#113608=CARTESIAN_POINT ( 'NONE',  ( -17.49999999999999645, 5.499999999999992895, 102.5000000000000142 ) ) ;
#113609=CARTESIAN_POINT ( 'NONE',  ( 8.224510206698742110, 14.34966873604972548, 112.0844237280190185 ) ) ;
#113611=CARTESIAN_POINT ( 'NONE',  ( -16.52544592524335698, -4.483927247898792601, 78.95942372801901854 ) ) ;
#113612=CARTESIAN_POINT ( 'NONE',  ( -21.52544592524334988, -5.823673210054445271, 93.95942372801903275 ) ) ;
#113613=CARTESIAN_POINT ( 'NONE',  ( -16.46253265017146816, -9.564922557961047289, 99.16775706135233293 ) ) ;
#113614=CARTESIAN_POINT ( 'NONE',  ( -10.72451020669870658, -18.67979575497194134, 69.58442372801900433 ) ) ;
#113615=CARTESIAN_POINT ( 'NONE',  ( 16.51473224551083163, -9.474510206698727899, 40.83442372801900433 ) ) ;
#113616=CARTESIAN_POINT ( 'NONE',  ( -16.51473224551069308, -9.474510206698971260, 76.66557627198103830 ) ) ;
#113617=CARTESIAN_POINT ( 'NONE',  ( -16.51473224551069308, -9.474510206698971260, 56.66557627198103120 ) ) ;
#113619=CARTESIAN_POINT ( 'NONE',  ( 15.72974639402199770, -15.80617190586745480, 98.12390960531436690 ) ) ;
#113620=CARTESIAN_POINT ( 'NONE',  ( 0.05219959533907565091, 21.53943276465977519, 49.99890960531437401 ) ) ;
#113621=CARTESIAN_POINT ( 'NONE',  ( 13.97604488694527802, 13.89961937509977652, 49.37390960531434558 ) ) ;
#113622=CARTESIAN_POINT ( 'NONE',  ( 8.314922557961029526, -14.29746914071037800, 60.41775706135235424 ) ) ;
#113624=CARTESIAN_POINT ( 'NONE',  ( 15.80617190586769283, -15.72974639402175789, 50.62609039468568994 ) ) ;
#113625=CARTESIAN_POINT ( 'NONE',  ( -14.29746914071049879, 8.314922557960819915, 65.83224293864769550 ) ) ;
#113627=CARTESIAN_POINT ( 'NONE',  ( -12.14591786802326823, 12.06949235617739902, 38.12609039468567573 ) ) ;
#113628=CARTESIAN_POINT ( 'NONE',  ( 12.06949235617757843, -12.14591786802309237, 98.12390960531436690 ) ) ;
#113629=CARTESIAN_POINT ( 'NONE',  ( -9.564922557961040184, 16.46253265017147172, 47.91775706135233293 ) ) ;
#113630=CARTESIAN_POINT ( 'NONE',  ( 0.05219959533910956823, 16.53943276465976808, 64.99890960531435269 ) ) ;
#113631=CARTESIAN_POINT ( 'NONE',  ( 21.53943276465977519, 0.05219959533937863772, 36.25109039468567573 ) ) ;
#113632=CARTESIAN_POINT ( 'NONE',  ( -13.89961937509977652, 13.97604488694528158, 25.62390960531434558 ) ) ;
#113633=CARTESIAN_POINT ( 'NONE',  ( 5.823673210054125526, 21.52544592524343514, 89.79057627198103830 ) ) ;
#113634=CARTESIAN_POINT ( 'NONE',  ( 16.51473224551069308, 9.474510206698969483, 104.1655762719810241 ) ) ;
#113635=CARTESIAN_POINT ( 'NONE',  ( 8.224510206698953496, -14.34966873604960469, 72.91557627198103830 ) ) ;
#113638=CARTESIAN_POINT ( 'NONE',  ( 0.05219959533936267826, -19.03943276465977164, 80.00109039468567573 ) ) ;
#113639=CARTESIAN_POINT ( 'NONE',  ( 15.80617190586769283, -15.72974639402175789, 20.62609039468568639 ) ) ;
#113640=CARTESIAN_POINT ( 'NONE',  ( -13.97604488694527625, -13.89961937509977652, 71.87390960531433848 ) ) ;
#113641=CARTESIAN_POINT ( 'NONE',  ( -5.049401038297874678, -19.05341960407617918, 54.79275706135234003 ) ) ;
#113642=CARTESIAN_POINT ( 'NONE',  ( -13.97604488694527625, -13.89961937509977652, 36.87390960531436690 ) ) ;
#113644=CARTESIAN_POINT ( 'NONE',  ( -16.52544592524342804, 4.483927247898546575, 66.04057627198103830 ) ) ;
#113645=CARTESIAN_POINT ( 'NONE',  ( -8.314922557960811034, -14.29746914071050412, 52.08224293864768839 ) ) ;
#113646=CARTESIAN_POINT ( 'NONE',  ( -9.564922557960796823, -16.46253265017161027, 82.08224293864768129 ) ) ;
#113647=CARTESIAN_POINT ( 'NONE',  ( -5.719274019375978568, 21.55341960407610458, 90.20724293864770971 ) ) ;
#113648=CARTESIAN_POINT ( 'NONE',  ( 9.474510206698971260, -16.51473224551069308, 57.91557627198103120 ) ) ;
#113649=CARTESIAN_POINT ( 'NONE',  ( -21.55341960407610458, -5.719274019375992779, 81.45724293864769550 ) ) ;
#113650=CARTESIAN_POINT ( 'NONE',  ( -5.049401038297874678, -19.05341960407617918, 19.79275706135233293 ) ) ;
#113651=CARTESIAN_POINT ( 'NONE',  ( 9.564922557960805705, 16.46253265017160317, 29.58224293864769550 ) ) ;
#113652=CARTESIAN_POINT ( 'NONE',  ( -0.05219959533934338120, 16.53943276465976808, 107.5010903946856899 ) ) ;
#113653=CARTESIAN_POINT ( 'NONE',  ( -12.14591786802309592, -12.06949235617757132, 101.8739096053143811 ) ) ;
#113654=CARTESIAN_POINT ( 'NONE',  ( 9.474510206698729675, 16.51473224551082808, 92.08442372801900433 ) ) ;
#113656=CARTESIAN_POINT ( 'NONE',  ( 21.52544592524344225, -5.823673210054117533, 113.5405762719810383 ) ) ;
#113657=CARTESIAN_POINT ( 'NONE',  ( -19.03943276465977164, -0.05219959533935918106, 58.75109039468566863 ) ) ;
#113658=CARTESIAN_POINT ( 'NONE',  ( 4.483927247898790824, -16.52544592524335698, 105.2094237280190328 ) ) ;
#113659=CARTESIAN_POINT ( 'NONE',  ( -19.05341960407617563, 5.049401038297882671, 43.54275706135232582 ) ) ;
#113660=CARTESIAN_POINT ( 'NONE',  ( 16.46253265017160672, -9.564922557960803928, 108.3322429386476955 ) ) ;
#113661=CARTESIAN_POINT ( 'NONE',  ( -15.72974639402197994, 15.80617190586746368, 55.62390960531436690 ) ) ;
#113663=CARTESIAN_POINT ( 'NONE',  ( 5.049401038298161559, -19.05341960407611168, 32.70724293864768129 ) ) ;
#113664=CARTESIAN_POINT ( 'NONE',  ( 15.72974639402176855, 15.80617190586768217, 106.8760903946856899 ) ) ;
#113665=CARTESIAN_POINT ( 'NONE',  ( -8.224510206698735004, -14.34966873604973081, 79.58442372801903275 ) ) ;
#113666=CARTESIAN_POINT ( 'NONE',  ( -10.72451020669870658, -18.67979575497194134, 29.58442372801901854 ) ) ;
#113667=CARTESIAN_POINT ( 'NONE',  ( -16.53943276465976808, -0.05219959533934237506, 48.75109039468568284 ) ) ;
#113668=CARTESIAN_POINT ( 'NONE',  ( -19.02544592524342804, 5.153800228976336051, 111.0405762719810099 ) ) ;
#113669=CARTESIAN_POINT ( 'NONE',  ( 13.97604488694527802, 13.89961937509977652, 49.37390960531434558 ) ) ;
#113670=CARTESIAN_POINT ( 'NONE',  ( 13.89961937509977652, -13.97604488694527269, 68.12390960531436690 ) ) ;
#113671=CARTESIAN_POINT ( 'NONE',  ( -16.53943276465976808, -0.05219959533934237506, 43.75109039468568284 ) ) ;
#113672=CARTESIAN_POINT ( 'NONE',  ( 8.224510206698953496, -14.34966873604960469, 107.9155762719810241 ) ) ;
#113673=CARTESIAN_POINT ( 'NONE',  ( 16.55341960407618274, -4.379528057220086978, 111.0427570613523613 ) ) ;
#113675=CARTESIAN_POINT ( 'NONE',  ( -0.05219959533937732626, 21.53943276465977519, 62.50109039468568284 ) ) ;
#113676=CARTESIAN_POINT ( 'NONE',  ( 16.46253265017160672, -9.564922557960803928, 98.33224293864769550 ) ) ;
#113677=CARTESIAN_POINT ( 'NONE',  ( 5.153800228976335163, 19.02544592524342804, 64.79057627198100988 ) ) ;
#113678=CARTESIAN_POINT ( 'NONE',  ( 9.474510206698971260, -16.51473224551069308, 97.91557627198102409 ) ) ;
#113679=CARTESIAN_POINT ( 'NONE',  ( 4.483927247898545687, 16.52544592524342804, 49.79057627198102409 ) ) ;
#113680=CARTESIAN_POINT ( 'NONE',  ( 14.29746914071037800, 8.314922557961029526, 106.6677570613523756 ) ) ;
#113681=CARTESIAN_POINT ( 'NONE',  ( -4.483927247898539470, -16.52544592524342804, 37.29057627198102409 ) ) ;
#113682=CARTESIAN_POINT ( 'NONE',  ( 17.50000000000000000, 5.499999999999997335, 120.0000000000000142 ) ) ;
#113683=CARTESIAN_POINT ( 'NONE',  ( 5.049401038298161559, -19.05341960407611168, 62.70724293864769550 ) ) ;
#113684=CARTESIAN_POINT ( 'NONE',  ( -5.153800228976607833, 19.02544592524334988, 42.70942372801901143 ) ) ;
#113686=CARTESIAN_POINT ( 'NONE',  ( -9.564922557960796823, -16.46253265017161027, 67.08224293864769550 ) ) ;
#113687=CARTESIAN_POINT ( 'NONE',  ( 19.05341960407617918, -5.049401038297876454, 91.04275706135234714 ) ) ;
#113688=CARTESIAN_POINT ( 'NONE',  ( -16.53943276465976808, -0.05219959533934237506, 73.75109039468567573 ) ) ;
#113689=CARTESIAN_POINT ( 'NONE',  ( 16.18388926212238488, 7.379444403734540359, 92.93953151366149257 ) ) ;
#113690=CARTESIAN_POINT ( 'NONE',  ( -16.51473224551069308, -9.474510206698971260, 86.66557627198102409 ) ) ;
#113691=CARTESIAN_POINT ( 'NONE',  ( 10.72451020669871369, 18.67979575497193778, 32.08442372801901854 ) ) ;
#113692=CARTESIAN_POINT ( 'NONE',  ( 13.97604488694548053, -13.89961937509957401, 85.62609039468568994 ) ) ;
#113693=CARTESIAN_POINT ( 'NONE',  ( 16.20579543436678094, 7.371946100355120102, 88.06520834171882939 ) ) ;
#113694=CARTESIAN_POINT ( 'NONE',  ( -13.97604488694527625, -13.89961937509977652, 46.87390960531435979 ) ) ;
#113695=CARTESIAN_POINT ( 'NONE',  ( 5.153800228976335163, 19.02544592524342804, 84.79057627198099567 ) ) ;
#113696=CARTESIAN_POINT ( 'NONE',  ( -14.34966873604960291, -8.224510206698953496, 41.66557627198103120 ) ) ;
#113697=CARTESIAN_POINT ( 'NONE',  ( -19.02544592524342804, 5.153800228976336051, 51.04057627198103120 ) ) ;
#113698=CARTESIAN_POINT ( 'NONE',  ( 5.153800228976615827, -19.02544592524334988, 60.20942372801899012 ) ) ;
#113700=CARTESIAN_POINT ( 'NONE',  ( 12.14591786802309770, 12.06949235617756955, 84.37390960531438111 ) ) ;
#113701=CARTESIAN_POINT ( 'NONE',  ( -9.564922557961040184, 16.46253265017147172, 32.91775706135233293 ) ) ;
#113702=CARTESIAN_POINT ( 'NONE',  ( 5.049401038298161559, -19.05341960407611168, 62.70724293864769550 ) ) ;
#113703=CARTESIAN_POINT ( 'NONE',  ( 21.55341960407610458, 5.719274019375980345, 58.95724293864770971 ) ) ;
#113704=CARTESIAN_POINT ( 'NONE',  ( -14.34966873604960291, -8.224510206698953496, 61.66557627198103120 ) ) ;
#113705=CARTESIAN_POINT ( 'NONE',  ( 5.153800228976615827, -19.02544592524334988, 25.20942372801900433 ) ) ;
#113706=CARTESIAN_POINT ( 'NONE',  ( 13.89961937509977652, -13.97604488694527269, 103.1239096053143527 ) ) ;
#113707=CARTESIAN_POINT ( 'NONE',  ( -15.80617190586745835, -15.72974639402198527, 26.87390960531435979 ) ) ;
#113708=CARTESIAN_POINT ( 'NONE',  ( 13.97604488694527802, 13.89961937509977652, 59.37390960531434558 ) ) ;
#113709=CARTESIAN_POINT ( 'NONE',  ( -13.89961937509977652, 13.97604488694528158, 45.62390960531433848 ) ) ;
#113710=CARTESIAN_POINT ( 'NONE',  ( -14.34966873604960291, -8.224510206698953496, 101.6655762719810383 ) ) ;
#113711=CARTESIAN_POINT ( 'NONE',  ( -0.05219959533907301413, -21.53943276465977519, 112.4989096053143669 ) ) ;
#113712=CARTESIAN_POINT ( 'NONE',  ( -13.89961937509977652, 13.97604488694528158, 95.62390960531436690 ) ) ;
#113713=CARTESIAN_POINT ( 'NONE',  ( -10.81492255796105439, 18.62759615963255655, 22.91775706135235069 ) ) ;
#113714=CARTESIAN_POINT ( 'NONE',  ( 16.51473224551069308, 9.474510206698969483, 104.1655762719810241 ) ) ;
#113715=CARTESIAN_POINT ( 'NONE',  ( 19.03943276465977164, -0.05219959533909143690, 23.74890960531435269 ) ) ;
#113716=CARTESIAN_POINT ( 'NONE',  ( 21.55341960407619695, -5.719274019375665929, 81.04275706135236135 ) ) ;
#113717=CARTESIAN_POINT ( 'NONE',  ( -15.80617190586745835, -15.72974639402198527, 96.87390960531436690 ) ) ;
#113719=CARTESIAN_POINT ( 'NONE',  ( -17.49999999999999645, 5.499999999999997335, 120.0000000000000142 ) ) ;
#113720=CARTESIAN_POINT ( 'NONE',  ( 13.89961937509978007, -13.97604488694527269, 53.12390960531435269 ) ) ;
#113722=CARTESIAN_POINT ( 'NONE',  ( 14.34966873604972726, -8.224510206698740333, 50.83442372801901143 ) ) ;
#113723=CARTESIAN_POINT ( 'NONE',  ( 16.55341960407611168, 4.379528057220329451, 113.9572429386477239 ) ) ;
#113725=CARTESIAN_POINT ( 'NONE',  ( 9.474510206698971260, -16.51473224551069308, 62.91557627198102409 ) ) ;
#113726=CARTESIAN_POINT ( 'NONE',  ( 4.379528057220339221, -16.55341960407611168, 92.70724293864770971 ) ) ;
#113727=CARTESIAN_POINT ( 'NONE',  ( 0.05219959533907565091, 21.53943276465977519, 49.99890960531437401 ) ) ;
#113728=CARTESIAN_POINT ( 'NONE',  ( -12.14591786802309592, -12.06949235617757132, 71.87390960531438111 ) ) ;
#113729=CARTESIAN_POINT ( 'NONE',  ( -8.224510206698735004, -14.34966873604973081, 24.58442372801901499 ) ) ;
#113730=CARTESIAN_POINT ( 'NONE',  ( 10.72451020669871369, 18.67979575497193778, 77.08442372801901854 ) ) ;
#113731=CARTESIAN_POINT ( 'NONE',  ( -16.51473224551082808, 9.474510206698731452, 63.33442372801900433 ) ) ;
#113732=CARTESIAN_POINT ( 'NONE',  ( -8.314922557961024197, 14.29746914071037800, 92.91775706135236135 ) ) ;
#113733=CARTESIAN_POINT ( 'NONE',  ( -14.34966873604960291, -8.224510206698953496, 41.66557627198103120 ) ) ;
#113734=CARTESIAN_POINT ( 'NONE',  ( 9.564922557960805705, 16.46253265017160317, 39.58224293864768839 ) ) ;
#113735=CARTESIAN_POINT ( 'NONE',  ( 19.02544592524343514, -5.153800228976328945, 93.54057627198102409 ) ) ;
#113736=CARTESIAN_POINT ( 'NONE',  ( 21.52544592524344225, -5.823673210054117533, 88.54057627198103830 ) ) ;
#113737=CARTESIAN_POINT ( 'NONE',  ( 12.06949235617739724, 12.14591786802326823, 36.87609039468568994 ) ) ;
#113738=CARTESIAN_POINT ( 'NONE',  ( -16.55341960407611168, -4.379528057220339221, 71.45724293864769550 ) ) ;
#113739=CARTESIAN_POINT ( 'NONE',  ( -15.80617190586768217, 15.72974639402176855, 73.12609039468567573 ) ) ;
#113741=CARTESIAN_POINT ( 'NONE',  ( -16.55341960407617563, 4.379528057220093196, 103.5427570613523613 ) ) ;
#113744=CARTESIAN_POINT ( 'NONE',  ( 16.53943276465976808, -0.05219959533910856209, 23.74890960531435269 ) ) ;
#113745=CARTESIAN_POINT ( 'NONE',  ( -8.224510206698735004, -14.34966873604973081, 69.58442372801900433 ) ) ;
#113746=CARTESIAN_POINT ( 'NONE',  ( -19.02544592524342804, 5.153800228976336051, 91.04057627198100988 ) ) ;
#113747=CARTESIAN_POINT ( 'NONE',  ( -19.05341960407611168, -5.049401038298163336, 106.4572429386476955 ) ) ;
#113748=CARTESIAN_POINT ( 'NONE',  ( -21.53943276465977519, -0.05219959533937600094, 88.75109039468567573 ) ) ;
#113749=CARTESIAN_POINT ( 'NONE',  ( 12.14591786802327356, -12.06949235617739191, 95.62609039468568994 ) ) ;
#113750=CARTESIAN_POINT ( 'NONE',  ( -16.53943276465976808, 0.05219959533911058130, 61.24890960531435979 ) ) ;
#113751=CARTESIAN_POINT ( 'NONE',  ( 19.05341960407611168, 5.049401038298154454, 73.95724293864768129 ) ) ;
#113752=ORIENTED_EDGE ( 'NONE', *, *, #45027, .F. ) ;
#113753=CARTESIAN_POINT ( 'NONE',  ( 13.97604488694548053, -13.89961937509957401, 110.6260903946856615 ) ) ;
#113754=CARTESIAN_POINT ( 'NONE',  ( 12.14591786802309770, 12.06949235617756955, 109.3739096053143811 ) ) ;
#113755=CARTESIAN_POINT ( 'NONE',  ( -19.05341960407611168, -5.049401038298163336, 81.45724293864769550 ) ) ;
#113756=CARTESIAN_POINT ( 'NONE',  ( 0.05219959533934541429, -16.53943276465976808, 20.00109039468568639 ) ) ;
#113758=CARTESIAN_POINT ( 'NONE',  ( -15.80617190586768217, 15.72974639402176855, 113.1260903946856899 ) ) ;
#113759=CARTESIAN_POINT ( 'NONE',  ( 16.55341960407618274, -4.379528057220086978, 86.04275706135236135 ) ) ;
#113760=CARTESIAN_POINT ( 'NONE',  ( -19.05341960407617563, 5.049401038297882671, 103.5427570613523329 ) ) ;
#113761=CARTESIAN_POINT ( 'NONE',  ( -8.224510206698948167, 14.34966873604960824, 115.4155762719810241 ) ) ;
#113762=CARTESIAN_POINT ( 'NONE',  ( -0.05219959533934338120, 16.53943276465976808, 72.50109039468568994 ) ) ;
#113763=CARTESIAN_POINT ( 'NONE',  ( -8.314922557961024197, 14.29746914071037800, 57.91775706135234714 ) ) ;
#113765=CARTESIAN_POINT ( 'NONE',  ( -19.02544592524334988, -5.153800228976617603, 68.95942372801896170 ) ) ;
#113766=CARTESIAN_POINT ( 'NONE',  ( 21.55341960407619695, -5.719274019375665929, 101.0427570613523756 ) ) ;
#113767=CARTESIAN_POINT ( 'NONE',  ( 19.03943276465977164, -0.05219959533909143690, 28.74890960531435624 ) ) ;
#113768=CARTESIAN_POINT ( 'NONE',  ( 19.03943276465977164, -0.05219959533909143690, 78.74890960531436690 ) ) ;
#113769=CARTESIAN_POINT ( 'NONE',  ( -4.379528057220328563, 16.55341960407611168, 75.20724293864769550 ) ) ;
#113770=CARTESIAN_POINT ( 'NONE',  ( -5.823673210054431948, 21.52544592524334988, 92.70942372801901854 ) ) ;
#113771=CARTESIAN_POINT ( 'NONE',  ( 9.474510206698729675, 16.51473224551082808, 42.08442372801900433 ) ) ;
#113772=CARTESIAN_POINT ( 'NONE',  ( -18.67979575497178146, -10.72451020669898902, 31.66557627198102054 ) ) ;
#113773=CARTESIAN_POINT ( 'NONE',  ( 5.719274019375673035, 21.55341960407619339, 107.2927570613523471 ) ) ;
#113774=CARTESIAN_POINT ( 'NONE',  ( 9.564922557960805705, 16.46253265017160317, 79.58224293864769550 ) ) ;
#113775=CARTESIAN_POINT ( 'NONE',  ( 5.823673210054444382, -21.52544592524334988, 100.2094237280190043 ) ) ;
#113776=CARTESIAN_POINT ( 'NONE',  ( 18.67979575497178502, 10.72451020669898547, 69.16557627198102409 ) ) ;
#113777=CARTESIAN_POINT ( 'NONE',  ( 16.51473224551069308, 9.474510206698969483, 99.16557627198102409 ) ) ;
#113778=CARTESIAN_POINT ( 'NONE',  ( 5.049401038297881783, 19.05341960407617563, 72.29275706135234714 ) ) ;
#113779=CARTESIAN_POINT ( 'NONE',  ( 5.153800228976335163, 19.02544592524342804, 99.79057627198102409 ) ) ;
#113780=CARTESIAN_POINT ( 'NONE',  ( 19.05341960407617918, -5.049401038297876454, 91.04275706135234714 ) ) ;
#113781=CARTESIAN_POINT ( 'NONE',  ( -16.53943276465976808, -0.05219959533934237506, 58.75109039468568994 ) ) ;
#113782=CARTESIAN_POINT ( 'NONE',  ( -9.564922557960796823, -16.46253265017161027, 22.08224293864768839 ) ) ;
#113783=CARTESIAN_POINT ( 'NONE',  ( -16.51473224551069308, -9.474510206698971260, 86.66557627198102409 ) ) ;
#113784=CARTESIAN_POINT ( 'NONE',  ( -5.719274019375978568, 21.55341960407610458, 65.20724293864768129 ) ) ;
#113785=B_SPLINE_CURVE_WITH_KNOTS ( 'NONE', 3,
 ( #174972, #187183, #175978, #48654, #142629, #172990, #22287, #51616, #110306, #188165, #36436, #98091, #160799, #96127, #83938, #159789, #18316, #21284, #34468, #82941, #19306, #144619, #80954, #35455, #67783, #65787, #97106, #112296, #191139, #111301, #3131, #171988 ),
 .UNSPECIFIED., .F., .F.,
 ( 4, 2, 2, 2, 2, 2, 2, 2, 2, 2, 2, 2, 2, 2, 2, 4 ),
 ( 2.367436813247750825E-17, 0.0003712461730037028783, 0.0007424923460073820126, 0.001113738519011061310, 0.001484984692014740390, 0.002227477038022091828, 0.002598723211025753561, 0.002969969384029413993, 0.003341215557033075725, 0.003712461730036736591, 0.004083707903040397456, 0.004454954076044058756, 0.004826200249047720922, 0.005197446422051382221, 0.005568692595055043520, 0.005939938768058704820 ),
 .UNSPECIFIED. ) ;
#113786=CARTESIAN_POINT ( 'NONE',  ( 0.05219959533934541429, -16.53943276465976808, 35.00109039468568284 ) ) ;
#113787=CARTESIAN_POINT ( 'NONE',  ( -5.719274019375665041, -21.55341960407619695, 29.79275706135234358 ) ) ;
#113788=CARTESIAN_POINT ( 'NONE',  ( 18.62759615963255655, 10.81492255796105972, 81.66775706135236135 ) ) ;
#113789=CARTESIAN_POINT ( 'NONE',  ( -8.314922557961024197, 14.29746914071037800, 87.91775706135234714 ) ) ;
#113790=CARTESIAN_POINT ( 'NONE',  ( -19.05341960407611168, -5.049401038298163336, 81.45724293864769550 ) ) ;
#113791=CARTESIAN_POINT ( 'NONE',  ( -16.52544592524342804, 4.483927247898546575, 76.04057627198102409 ) ) ;
#113792=CARTESIAN_POINT ( 'NONE',  ( 4.379528057220339221, -16.55341960407611168, 22.70724293864769194 ) ) ;
#113793=CARTESIAN_POINT ( 'NONE',  ( -13.89961937509957401, -13.97604488694547875, 59.37609039468566863 ) ) ;
#113794=CARTESIAN_POINT ( 'NONE',  ( 18.67979575497194134, -10.72451020669871369, 40.83442372801901854 ) ) ;
#113795=CARTESIAN_POINT ( 'NONE',  ( 16.53943276465976808, -0.05219959533910856209, 88.74890960531436690 ) ) ;
#113796=CARTESIAN_POINT ( 'NONE',  ( -21.55341960407610458, -5.719274019375992779, 21.45724293864769550 ) ) ;
#113797=CARTESIAN_POINT ( 'NONE',  ( 14.34966873604972726, -8.224510206698740333, 105.8344237280190328 ) ) ;
#113798=CARTESIAN_POINT ( 'NONE',  ( -0.05219959533937732626, 21.53943276465977519, 82.50109039468568994 ) ) ;
#113799=CARTESIAN_POINT ( 'NONE',  ( -12.06949235617739369, -12.14591786802326823, 39.37609039468567573 ) ) ;
#113800=CARTESIAN_POINT ( 'NONE',  ( 5.719274019375673035, 21.55341960407619339, 37.29275706135235424 ) ) ;
#113801=EDGE_LOOP ( 'NONE', ( #148302, #12713 ) ) ;
#113802=CARTESIAN_POINT ( 'NONE',  ( 15.80617190586769283, -15.72974639402175789, 20.62609039468568639 ) ) ;
#113803=CARTESIAN_POINT ( 'NONE',  ( -14.29746914071049879, 8.314922557960819915, 95.83224293864770971 ) ) ;
#113805=CARTESIAN_POINT ( 'NONE',  ( -12.06949235617756955, 12.14591786802309770, 60.62390960531437401 ) ) ;
#113806=CARTESIAN_POINT ( 'NONE',  ( -16.55341960407617563, 4.379528057220093196, 93.54275706135234714 ) ) ;
#113807=CARTESIAN_POINT ( 'NONE',  ( -13.89961937509977652, 13.97604488694528158, 45.62390960531433848 ) ) ;
#113808=CARTESIAN_POINT ( 'NONE',  ( -18.62759615963270932, 10.81492255796079327, 45.83224293864769550 ) ) ;
#113809=CARTESIAN_POINT ( 'NONE',  ( -14.29746914071049879, 8.314922557960819915, 80.83224293864769550 ) ) ;
#113810=CARTESIAN_POINT ( 'NONE',  ( -21.52544592524343514, 5.823673210054127303, 76.04057627198102409 ) ) ;
#113811=CARTESIAN_POINT ( 'NONE',  ( -0.05219959533909027116, -19.03943276465977164, 82.49890960531436690 ) ) ;
#113812=CARTESIAN_POINT ( 'NONE',  ( -5.049401038298153566, 19.05341960407611168, 45.20724293864769550 ) ) ;
#113813=CARTESIAN_POINT ( 'NONE',  ( -19.05341960407617563, 5.049401038297882671, 93.54275706135234714 ) ) ;
#113814=CARTESIAN_POINT ( 'NONE',  ( 15.80617190586746368, 15.72974639402197994, 29.37390960531435269 ) ) ;
#113815=CARTESIAN_POINT ( 'NONE',  ( 5.719274019375673035, 21.55341960407619339, 57.29275706135234714 ) ) ;
#113816=CARTESIAN_POINT ( 'NONE',  ( 0.05219959533909260263, 19.03943276465977164, 59.99890960531436690 ) ) ;
#113817=CARTESIAN_POINT ( 'NONE',  ( -16.46253265017160317, 9.564922557960807481, 85.83224293864769550 ) ) ;
#113819=CARTESIAN_POINT ( 'NONE',  ( -0.05219959533934338120, 16.53943276465976808, 47.50109039468568994 ) ) ;
#113820=CARTESIAN_POINT ( 'NONE',  ( 5.823673210054444382, -21.52544592524334988, 50.20942372801901854 ) ) ;
#113821=CARTESIAN_POINT ( 'NONE',  ( -21.55341960407619339, 5.719274019375674811, 78.54275706135236135 ) ) ;
#113822=CARTESIAN_POINT ( 'NONE',  ( -18.67979575497178146, -10.72451020669898902, 21.66557627198102409 ) ) ;
#113823=CARTESIAN_POINT ( 'NONE',  ( 21.53943276465977519, -0.05219959533907433946, 83.74890960531435269 ) ) ;
#113824=CARTESIAN_POINT ( 'NONE',  ( 15.80617190586769283, -15.72974639402175789, 20.62609039468568639 ) ) ;
#113825=CARTESIAN_POINT ( 'NONE',  ( -12.06949235617739369, -12.14591786802326823, 59.37609039468568284 ) ) ;
#113826=CARTESIAN_POINT ( 'NONE',  ( 15.80617190586746368, 15.72974639402197994, 69.37390960531436690 ) ) ;
#113827=CARTESIAN_POINT ( 'NONE',  ( -19.03943276465977164, -0.05219959533935918106, 18.75109039468567218 ) ) ;
#113828=CARTESIAN_POINT ( 'NONE',  ( 5.049401038298161559, -19.05341960407611168, 62.70724293864769550 ) ) ;
#113829=CARTESIAN_POINT ( 'NONE',  ( -16.53943276465976808, -0.05219959533934237506, 103.7510903946857042 ) ) ;
#113831=CARTESIAN_POINT ( 'NONE',  ( 5.153800228976335163, 19.02544592524342804, 84.79057627198099567 ) ) ;
#113832=CARTESIAN_POINT ( 'NONE',  ( -17.59860650958993844, 7.585241751806885979, 53.42337014262493966 ) ) ;
#113833=CARTESIAN_POINT ( 'NONE',  ( -5.049401038297874678, -19.05341960407617918, 84.79275706135233293 ) ) ;
#113834=CARTESIAN_POINT ( 'NONE',  ( -15.72974639402197994, 15.80617190586746368, 55.62390960531436690 ) ) ;
#113835=CARTESIAN_POINT ( 'NONE',  ( -12.14591786802326823, 12.06949235617739902, 113.1260903946856899 ) ) ;
#113836=CARTESIAN_POINT ( 'NONE',  ( 16.51473224551083163, -9.474510206698727899, 105.8344237280190043 ) ) ;
#113838=CARTESIAN_POINT ( 'NONE',  ( 5.153800228976615827, -19.02544592524334988, 100.2094237280190043 ) ) ;
#113839=CARTESIAN_POINT ( 'NONE',  ( 18.67979575497178502, 10.72451020669898547, 89.16557627198102409 ) ) ;
#113840=CARTESIAN_POINT ( 'NONE',  ( -9.564922557961040184, 16.46253265017147172, 57.91775706135233293 ) ) ;
#113842=CARTESIAN_POINT ( 'NONE',  ( 19.05341960407611168, 5.049401038298154454, 48.95724293864768129 ) ) ;
#113843=CARTESIAN_POINT ( 'NONE',  ( -4.483927247898539470, -16.52544592524342804, 57.29057627198103120 ) ) ;
#113844=CARTESIAN_POINT ( 'NONE',  ( -5.153800228976328057, -19.02544592524343514, 47.29057627198102409 ) ) ;
#113845=CARTESIAN_POINT ( 'NONE',  ( -16.52544592524342804, 4.483927247898546575, 51.04057627198103120 ) ) ;
#113848=CARTESIAN_POINT ( 'NONE',  ( -4.483927247898539470, -16.52544592524342804, 32.29057627198102409 ) ) ;
#113849=CARTESIAN_POINT ( 'NONE',  ( -0.05219959533909027116, -19.03943276465977164, 62.49890960531435979 ) ) ;
#113850=CARTESIAN_POINT ( 'NONE',  ( 5.049401038297881783, 19.05341960407617918, 72.29275706135233293 ) ) ;
#113851=CARTESIAN_POINT ( 'NONE',  ( 13.89961937509957401, 13.97604488694547697, 41.87609039468566152 ) ) ;
#113852=CARTESIAN_POINT ( 'NONE',  ( 16.55341960407618274, -4.379528057220086978, 46.04275706135234714 ) ) ;
#113853=CARTESIAN_POINT ( 'NONE',  ( -21.55341960407610458, -5.719274019375992779, 56.45724293864768839 ) ) ;
#113854=CARTESIAN_POINT ( 'NONE',  ( -15.80617190586768217, 15.72974639402176855, 108.1260903946856757 ) ) ;
#113855=CARTESIAN_POINT ( 'NONE',  ( 9.474510206698971260, -16.51473224551069308, 77.91557627198103830 ) ) ;
#113856=DIRECTION ( 'NONE',  ( -0.000000000000000000, -0.000000000000000000, 1.000000000000000000 ) ) ;
#113857=CARTESIAN_POINT ( 'NONE',  ( -19.05341960407611168, -5.049401038298163336, 91.45724293864766707 ) ) ;
#113859=CARTESIAN_POINT ( 'NONE',  ( 15.72974639402176855, 15.80617190586768217, 31.87609039468567929 ) ) ;
#113860=CARTESIAN_POINT ( 'NONE',  ( -4.483927247898539470, -16.52544592524342804, 97.29057627198105251 ) ) ;
#113861=CARTESIAN_POINT ( 'NONE',  ( 10.72451020669898902, -18.67979575497178502, 92.91557627198103830 ) ) ;
#113862=CARTESIAN_POINT ( 'NONE',  ( -5.153800228976328057, -19.02544592524343514, 87.29057627198103830 ) ) ;
#113863=CARTESIAN_POINT ( 'NONE',  ( -5.049401038298153566, 19.05341960407611168, 85.20724293864766707 ) ) ;
#113864=CARTESIAN_POINT ( 'NONE',  ( 0.05219959533907565091, 21.53943276465977519, 109.9989096053143527 ) ) ;
#113866=CARTESIAN_POINT ( 'NONE',  ( 9.474510206698971260, -16.51473224551069308, 72.91557627198102409 ) ) ;
#113868=CARTESIAN_POINT ( 'NONE',  ( -16.52544592524342804, 4.483927247898546575, 116.0405762719810383 ) ) ;
#113869=CARTESIAN_POINT ( 'NONE',  ( -19.05341960407611168, -5.049401038298163336, 31.45724293864769550 ) ) ;
#113870=CARTESIAN_POINT ( 'NONE',  ( -16.46253265017146816, -9.564922557961047289, 89.16775706135234714 ) ) ;
#113871=CARTESIAN_POINT ( 'NONE',  ( -19.03943276465977164, 0.05219959533909376836, 21.24890960531436335 ) ) ;
#113872=CARTESIAN_POINT ( 'NONE',  ( -10.81492255796105439, 18.62759615963255655, 67.91775706135234714 ) ) ;
#113873=CARTESIAN_POINT ( 'NONE',  ( -9.474510206698964154, 16.51473224551069663, 60.41557627198102409 ) ) ;
#113874=CARTESIAN_POINT ( 'NONE',  ( -21.53943276465977519, -0.05219959533937600094, 33.75109039468568284 ) ) ;
#113875=CARTESIAN_POINT ( 'NONE',  ( 21.53943276465977519, -0.05219959533907433946, 113.7489096053143527 ) ) ;
#113877=CARTESIAN_POINT ( 'NONE',  ( 13.97604488694527802, 13.89961937509977652, 89.37390960531436690 ) ) ;
#113879=CARTESIAN_POINT ( 'NONE',  ( 16.52544592524335698, 4.483927247898782831, 31.45942372801901854 ) ) ;
#113880=CARTESIAN_POINT ( 'NONE',  ( -18.62759615963270932, 10.81492255796079327, 25.83224293864769194 ) ) ;
#113881=CARTESIAN_POINT ( 'NONE',  ( 21.55341960407619695, -5.719274019375665929, 61.04275706135234714 ) ) ;
#113882=CARTESIAN_POINT ( 'NONE',  ( -9.474510206698720793, -16.51473224551083518, 99.58442372801900433 ) ) ;
#113883=CARTESIAN_POINT ( 'NONE',  ( 16.46253265017160672, -9.564922557960803928, 43.33224293864769550 ) ) ;
#113884=CARTESIAN_POINT ( 'NONE',  ( -19.03943276465977164, 0.05219959533909376836, 81.24890960531436690 ) ) ;
#113886=CARTESIAN_POINT ( 'NONE',  ( -4.483927247898539470, -16.52544592524342804, 92.29057627198103830 ) ) ;
#113887=CARTESIAN_POINT ( 'NONE',  ( 16.51473224551069308, 9.474510206698969483, 114.1655762719810241 ) ) ;
#113888=CARTESIAN_POINT ( 'NONE',  ( -4.379528057220328563, 16.55341960407611168, 95.20724293864769550 ) ) ;
#113889=CARTESIAN_POINT ( 'NONE',  ( -19.03943276465977164, 0.05219959533909376836, 106.2489096053143669 ) ) ;
#113890=CARTESIAN_POINT ( 'NONE',  ( 16.55341960407611168, 4.379528057220329451, 58.95724293864770971 ) ) ;
#113891=CARTESIAN_POINT ( 'NONE',  ( 5.153800228976335163, 19.02544592524342804, 39.79057627198100988 ) ) ;
#113892=CARTESIAN_POINT ( 'NONE',  ( -18.67979575497193778, 10.72451020669871902, 58.33442372801901143 ) ) ;
#113893=CARTESIAN_POINT ( 'NONE',  ( 5.153800228976615827, -19.02544592524334988, 90.20942372801900433 ) ) ;
#113894=CARTESIAN_POINT ( 'NONE',  ( 12.06949235617757843, -12.14591786802309237, 48.12390960531436690 ) ) ;
#113895=CARTESIAN_POINT ( 'NONE',  ( 5.823673210054125526, 21.52544592524343514, 109.7905762719810383 ) ) ;
#113896=CARTESIAN_POINT ( 'NONE',  ( 21.52544592524344225, -5.823673210054117533, 53.54057627198103120 ) ) ;
#113897=CARTESIAN_POINT ( 'NONE',  ( -0.05219959533909027116, -19.03943276465977164, 107.4989096053143527 ) ) ;
#113899=CARTESIAN_POINT ( 'NONE',  ( -0.05219959533909027116, -19.03943276465977164, 52.49890960531436690 ) ) ;
#113900=CARTESIAN_POINT ( 'NONE',  ( 4.379528057220092307, 16.55341960407617563, 112.2927570613523471 ) ) ;
#113901=CARTESIAN_POINT ( 'NONE',  ( 14.34966873604972726, -8.224510206698740333, 95.83442372801903275 ) ) ;
#113902=CARTESIAN_POINT ( 'NONE',  ( -8.224510206698735004, -14.34966873604973081, 89.58442372801901854 ) ) ;
#113903=CARTESIAN_POINT ( 'NONE',  ( -9.564922557961040184, 16.46253265017147172, 32.91775706135233293 ) ) ;
#113904=CARTESIAN_POINT ( 'NONE',  ( -17.05587630539786659, 6.762274262135695935, 70.74180309037316761 ) ) ;
#113905=CARTESIAN_POINT ( 'NONE',  ( -19.03943276465977164, 0.05219959533909376836, 96.24890960531436690 ) ) ;
#113906=CARTESIAN_POINT ( 'NONE',  ( 19.05341960407611168, 5.049401038298154454, 53.95724293864770260 ) ) ;
#113907=CARTESIAN_POINT ( 'NONE',  ( -16.52544592524342804, 4.483927247898546575, 56.04057627198102409 ) ) ;
#113908=CARTESIAN_POINT ( 'NONE',  ( 16.88567814943161949, -6.947325034625689177, 101.2099887734741515 ) ) ;
#113909=CARTESIAN_POINT ( 'NONE',  ( 15.72974639402199770, -15.80617190586745480, 28.12390960531435979 ) ) ;
#113910=CARTESIAN_POINT ( 'NONE',  ( 21.53943276465977519, -0.05219959533907433946, 38.74890960531435979 ) ) ;
#113911=CARTESIAN_POINT ( 'NONE',  ( 4.483927247898545687, 16.52544592524342804, 79.79057627198102409 ) ) ;
#113912=CARTESIAN_POINT ( 'NONE',  ( 0.05219959533934541429, -16.53943276465976808, 40.00109039468567573 ) ) ;
#113914=CARTESIAN_POINT ( 'NONE',  ( -4.483927247898539470, -16.52544592524342804, 82.29057627198103830 ) ) ;
#113916=CARTESIAN_POINT ( 'NONE',  ( 9.564922557961047289, -16.46253265017146816, 80.41775706135234714 ) ) ;
#113917=CARTESIAN_POINT ( 'NONE',  ( 9.474510206698971260, -16.51473224551069308, 107.9155762719810383 ) ) ;
#113920=CARTESIAN_POINT ( 'NONE',  ( -12.06949235617739369, -12.14591786802326823, 29.37609039468568284 ) ) ;
#113921=CARTESIAN_POINT ( 'NONE',  ( 0.05219959533934541429, -16.53943276465976808, 110.0010903946856757 ) ) ;
#113922=CARTESIAN_POINT ( 'NONE',  ( 0.05219959533936267826, -19.03943276465977164, 65.00109039468567573 ) ) ;
#113923=CARTESIAN_POINT ( 'NONE',  ( 10.72451020669898902, -18.67979575497178502, 32.91557627198102409 ) ) ;
#113924=CARTESIAN_POINT ( 'NONE',  ( 18.67979575497194134, -10.72451020669871369, 65.83442372801900433 ) ) ;
#113926=CARTESIAN_POINT ( 'NONE',  ( 4.483927247898790824, -16.52544592524335698, 35.20942372801901854 ) ) ;
#113928=CARTESIAN_POINT ( 'NONE',  ( -13.89961937509977652, 13.97604488694528158, 85.62390960531433848 ) ) ;
#113930=CARTESIAN_POINT ( 'NONE',  ( 16.52544592524342804, -4.483927247898539470, 83.54057627198102409 ) ) ;
#113931=PRODUCT_CONTEXT ( 'NONE', #172025, 'mechanical' ) ;
#113932=CARTESIAN_POINT ( 'NONE',  ( -5.153800228976328057, -19.02544592524343514, 82.29057627198103830 ) ) ;
#113934=CARTESIAN_POINT ( 'NONE',  ( 19.05341960407617918, -5.049401038297876454, 111.0427570613523329 ) ) ;
#113935=CARTESIAN_POINT ( 'NONE',  ( -18.67979575497178146, -10.72451020669898902, 71.66557627198100988 ) ) ;
#113936=CARTESIAN_POINT ( 'NONE',  ( 16.51473224551069308, 9.474510206698969483, 39.16557627198103120 ) ) ;
#113937=CARTESIAN_POINT ( 'NONE',  ( 13.89961937509957401, 13.97604488694547697, 66.87609039468567573 ) ) ;
#113938=CARTESIAN_POINT ( 'NONE',  ( -15.72974639402197994, 15.80617190586746368, 115.6239096053143669 ) ) ;
#113939=CARTESIAN_POINT ( 'NONE',  ( 13.97604488694527802, 13.89961937509977652, 74.37390960531436690 ) ) ;
#113940=CARTESIAN_POINT ( 'NONE',  ( -9.564922557960796823, -16.46253265017161027, 112.0822429386476955 ) ) ;
#113942=CARTESIAN_POINT ( 'NONE',  ( 16.55341960407618274, -4.379528057220086978, 31.04275706135234714 ) ) ;
#113943=CARTESIAN_POINT ( 'NONE',  ( 21.55341960407610458, 5.719274019375980345, 108.9572429386476955 ) ) ;
#113944=CARTESIAN_POINT ( 'NONE',  ( -12.14591786802309592, -12.06949235617757132, 101.8739096053143811 ) ) ;
#113945=CARTESIAN_POINT ( 'NONE',  ( 9.474510206698971260, -16.51473224551069308, 87.91557627198102409 ) ) ;
#113946=CARTESIAN_POINT ( 'NONE',  ( -9.564922557961040184, 16.46253265017147172, 67.91775706135233293 ) ) ;
#113947=CARTESIAN_POINT ( 'NONE',  ( -15.80617190586745835, -15.72974639402198527, 86.87390960531438111 ) ) ;
#113948=CARTESIAN_POINT ( 'NONE',  ( -16.53943276465976808, 0.05219959533911058130, 46.24890960531435979 ) ) ;
#113949=CARTESIAN_POINT ( 'NONE',  ( 13.97604488694548053, -13.89961937509957401, 25.62609039468566507 ) ) ;
#113950=CARTESIAN_POINT ( 'NONE',  ( -4.379528057220086978, -16.55341960407618274, 64.79275706135234714 ) ) ;
#113951=CARTESIAN_POINT ( 'NONE',  ( 19.02544592524343514, -5.153800228976328945, 93.54057627198102409 ) ) ;
#113952=CARTESIAN_POINT ( 'NONE',  ( -13.97604488694527625, -13.89961937509977652, 41.87390960531435979 ) ) ;
#113953=CARTESIAN_POINT ( 'NONE',  ( -10.72451020669870658, -18.67979575497194134, 49.58442372801901143 ) ) ;
#113954=CARTESIAN_POINT ( 'NONE',  ( 10.72451020669871369, 18.67979575497193778, 72.08442372801899012 ) ) ;
#113955=CARTESIAN_POINT ( 'NONE',  ( -16.51473224551069308, -9.474510206698971260, 66.66557627198102409 ) ) ;
#113956=CARTESIAN_POINT ( 'NONE',  ( -15.80617190586768217, 15.72974639402176855, 38.12609039468567573 ) ) ;
#113958=CARTESIAN_POINT ( 'NONE',  ( -13.97604488694547697, 13.89961937509957934, 73.12609039468568994 ) ) ;
#113959=CARTESIAN_POINT ( 'NONE',  ( 5.049401038297881783, 19.05341960407617563, 67.29275706135234714 ) ) ;
#113960=CARTESIAN_POINT ( 'NONE',  ( -16.46253265017160317, 9.564922557960807481, 40.83224293864769550 ) ) ;
#113961=CARTESIAN_POINT ( 'NONE',  ( -16.53943276465976808, -0.05219959533934237506, 88.75109039468567573 ) ) ;
#113962=CARTESIAN_POINT ( 'NONE',  ( -19.05341960407611168, -5.049401038298163336, 46.45724293864768129 ) ) ;
#113964=CARTESIAN_POINT ( 'NONE',  ( -16.51473224551069308, -9.474510206698971260, 96.66557627198102409 ) ) ;
#113965=CARTESIAN_POINT ( 'NONE',  ( -19.05341960407611168, -5.049401038298163336, 36.45724293864766707 ) ) ;
#113966=CARTESIAN_POINT ( 'NONE',  ( 15.72974639402199770, -15.80617190586745480, 88.12390960531436690 ) ) ;
#113967=CARTESIAN_POINT ( 'NONE',  ( -16.55341960407617563, 4.379528057220093196, 58.54275706135235424 ) ) ;
#113968=CARTESIAN_POINT ( 'NONE',  ( 16.46253265017146816, 9.564922557961045513, 36.66775706135233293 ) ) ;
#113970=CARTESIAN_POINT ( 'NONE',  ( 9.564922557960805705, 16.46253265017160317, 54.58224293864769550 ) ) ;
#113971=CARTESIAN_POINT ( 'NONE',  ( 16.53943276465976808, -0.05219959533910856209, 48.74890960531435979 ) ) ;
#113972=CARTESIAN_POINT ( 'NONE',  ( 12.14591786802309770, 12.06949235617756955, 84.37390960531438111 ) ) ;
#113973=CARTESIAN_POINT ( 'NONE',  ( 13.89961937509977652, -13.97604488694527269, 83.12390960531436690 ) ) ;
#113974=CARTESIAN_POINT ( 'NONE',  ( 9.474510206698971260, -16.51473224551069308, 77.91557627198103830 ) ) ;
#113975=CARTESIAN_POINT ( 'NONE',  ( 10.72451020669871369, 18.67979575497193778, 42.08442372801901854 ) ) ;
#113976=CARTESIAN_POINT ( 'NONE',  ( 5.153800228976335163, 19.02544592524342804, 94.79057627198103830 ) ) ;
#113977=CARTESIAN_POINT ( 'NONE',  ( -18.62759615963255300, -10.81492255796106328, 94.16775706135237556 ) ) ;
#113978=CARTESIAN_POINT ( 'NONE',  ( 12.06949235617739724, 12.14591786802326823, 81.87609039468568994 ) ) ;
#113979=CARTESIAN_POINT ( 'NONE',  ( 21.55341960407619695, -5.719274019375665929, 31.04275706135234714 ) ) ;
#113980=CARTESIAN_POINT ( 'NONE',  ( -15.72974639402197994, 15.80617190586746368, 95.62390960531436690 ) ) ;
#113981=CARTESIAN_POINT ( 'NONE',  ( 16.52544592524342804, -4.483927247898539470, 43.54057627198103830 ) ) ;
#113982=CARTESIAN_POINT ( 'NONE',  ( 16.46253265017160672, -9.564922557960803928, 43.33224293864769550 ) ) ;
#113983=CARTESIAN_POINT ( 'NONE',  ( 16.55341960407611168, 4.379528057220329451, 68.95724293864769550 ) ) ;
#113984=CARTESIAN_POINT ( 'NONE',  ( 21.55341960407610458, 5.719274019375980345, 33.95724293864769550 ) ) ;
#113985=CARTESIAN_POINT ( 'NONE',  ( 19.03943276465977164, 0.05219959533936151252, 31.25109039468566863 ) ) ;
#113986=CARTESIAN_POINT ( 'NONE',  ( -16.52544592524342804, 4.483927247898546575, 96.04057627198102409 ) ) ;
#113987=CARTESIAN_POINT ( 'NONE',  ( -9.474510206698964154, 16.51473224551069663, 110.4155762719810383 ) ) ;
#113989=CARTESIAN_POINT ( 'NONE',  ( 14.34966873604972726, -8.224510206698740333, 50.83442372801901143 ) ) ;
#113990=CARTESIAN_POINT ( 'NONE',  ( -16.51473224551069308, -9.474510206698971260, 56.66557627198103120 ) ) ;
#113991=CARTESIAN_POINT ( 'NONE',  ( -17.49999999999999645, -5.500000000000000888, 120.0000000000000142 ) ) ;
#113992=CARTESIAN_POINT ( 'NONE',  ( -12.14591786802326823, 12.06949235617739902, 98.12609039468570415 ) ) ;
#113993=CARTESIAN_POINT ( 'NONE',  ( -19.05341960407617563, 5.049401038297882671, 108.5427570613523187 ) ) ;
#113994=CARTESIAN_POINT ( 'NONE',  ( -10.72451020669870658, -18.67979575497194134, 84.58442372801903275 ) ) ;
#113995=CARTESIAN_POINT ( 'NONE',  ( 16.51473224551069308, 9.474510206698969483, 69.16557627198102409 ) ) ;
#113996=CARTESIAN_POINT ( 'NONE',  ( 10.72451020669898902, -18.67979575497178502, 107.9155762719810241 ) ) ;
#113997=CARTESIAN_POINT ( 'NONE',  ( -16.52544592524335698, -4.483927247898792601, 58.95942372801902565 ) ) ;
#113998=CARTESIAN_POINT ( 'NONE',  ( 12.06949235617757843, -12.14591786802309237, 108.1239096053143811 ) ) ;
#113999=CARTESIAN_POINT ( 'NONE',  ( -16.52544592524335698, -4.483927247898792601, 23.95942372801901143 ) ) ;
#114000=CARTESIAN_POINT ( 'NONE',  ( -13.97604488694547697, 13.89961937509957934, 83.12609039468564731 ) ) ;
#114001=CARTESIAN_POINT ( 'NONE',  ( -21.55341960407610458, -5.719274019375992779, 81.45724293864769550 ) ) ;
#114002=CARTESIAN_POINT ( 'NONE',  ( 13.89961937509957401, 13.97604488694547697, 56.87609039468564731 ) ) ;
#114004=CARTESIAN_POINT ( 'NONE',  ( 15.72974639402199770, -15.80617190586745480, 103.1239096053143811 ) ) ;
#114005=CARTESIAN_POINT ( 'NONE',  ( 17.50000000000002132, 3.471454075611646761, 28.01667418855641856 ) ) ;
#114006=CARTESIAN_POINT ( 'NONE',  ( -5.049401038298153566, 19.05341960407611168, 70.20724293864769550 ) ) ;
#114008=CARTESIAN_POINT ( 'NONE',  ( 12.06949235617739724, 12.14591786802326823, 21.87609039468567573 ) ) ;
#114010=CARTESIAN_POINT ( 'NONE',  ( 18.62759615963271287, -10.81492255796078972, 103.3322429386476955 ) ) ;
#114011=CARTESIAN_POINT ( 'NONE',  ( -16.53943276465976808, 0.05219959533911058130, 61.24890960531435979 ) ) ;
#114012=CARTESIAN_POINT ( 'NONE',  ( 5.049401038298161559, -19.05341960407611168, 67.70724293864769550 ) ) ;
#114013=CARTESIAN_POINT ( 'NONE',  ( -21.53943276465977519, -0.05219959533937600094, 68.75109039468568994 ) ) ;
#114014=( BOUNDED_SURFACE ( )  B_SPLINE_SURFACE ( 3, 2, ( 
 ( #37277, #149454, #10950, #7932, #69616, #102948, #22116, #130262, #193980, #38284, #160625, #71613, #98934, #131282, #192970, #129272, #190966, #55442, #162619, #177808, #116119, #191958, #100935, #24125, #114101, #117113, #133279, #145446, #85777, #101950, #147464, #178807, #40277, #194970, #6928, #175804, #163631, #8954, #25134, #148461, #9954, #56449, #53444, #115119, #61407, #27127, #59420, #43274, #74608, #135297, #89771, #105929, #57458, #195985, #28131, #122087, #183778, #14924, #151456, #103949, #119130, #75585, #76584, #152431, #12943, #197950, #166629, #137264, #153426, #31088, #104943, #182788, #123078, #184764, #91730, #30089, #180811, #60414, #169590, #198947, #90748, #136275, #106918, #121094, #88774, #42290, #92736, #120104, #46249, #13919, #165628, #72624, #107903, #154424, #73627, #45264, #29110, #134299, #138260, #150467, #11962, #168591, #196969, #199943, #167614, #58437, #181794, #44271, #97689, #155419, #109903, #80551, #35052, #32081, #124065, #96706, #77576, #185766, #79568, #724, #2726, #174574, #81525, #139248, #141235, #64403, #112881, #19884, #111895, #47254, #36040, #65387, #173583, #143211, #126072, #15918, #33075, #187768, #62395, #110896, #93738, #17912, #49238, #158395, #172581, #34068, #95726, #156410, #171587, #157412, #16909, #18905, #4693, #108911, #125081, #50239, #142225, #170591, #78561, #140235, #63404, #128046, #3709, #1728, #186779, #189748, #48249, #94730, #127047, #188754, #66384, #51220, #117893, #41054, #100703, #37039, #55210, #54217, #56211, #163399, #101709, #159379, #98699, #53205, #23885, #178571, #175562, #67376, #40035, #20875, #129034, #22882, #144215, #146205, #179583, #24896, #82533, #84528, #7691, #5699, #86544, #116879, #190735, #52208, #8716, #148228, #9722, #69375, #113866, #176576, #131045, #160393, #115888, #21882, #161390, #192735, #71386, #177578, #39045, #162383, #99706, #114882, #85537, #83532, #147225, #133050, #145211, #68371, #6693, #70385, #132053, #193742, #194740, #130022, #191721, #38050, #61170, #75354, #135069, #43044, #167385, #44037, #105698, #196745, #74380, #91493, #57226, #89539, #73398, #104710, #165402, #119881, #136045, #87544, #25899, #58212, #152203, #13687, #45029, #181566, #134061, #149231, #28881, #106687, #182555, #166400, #27896, #151225, #90521, #183543, #122842, #12714, #197720, #153180, #14683, #121850, #60181, #10722, #137024, #199704, #198714, #120855, #59186, #168360, #29856, #76345, #138022, #184530, #102718, #164407, #72385, #180584, #195752, #118899, #42058, #11731, #103722, #26895, #88538, #150235, #98191, #172331, #52709, #15677, #7199, #21382, #78317, #186536, #110650, #187530, #48995, #139990, #17664, #37545, #484, #32833, #16668, #48009, #108670, #63157, #79323, #30851, #169342, #1478, #159894, #83041, #191235, #124836, #77337, #92498, #36535, #114373, #125827, #109665, #171345, #94484, #144716, #129535, #68883, #156166, #140993, #99209, #160897, #67882, #6202, #154187, #176077, #145718, #22389, #64162, #2481, #84039, #130543, #62157, #139004, #46010, #93491, #107665, #123821, #185519, #47011, #170348, #31840, #155177, #56731, #148738, #192241, #11230, #150734, #73896, #133556, #69888, #88041, #87053, #89044, #196260, #134573, #53721, #131557, #86051, #118401, #72904, #8213, #100214, #57729, #115398, #161894, #55717, #177086, #179088, #12234, #119399, #38557, #117389, #40557, #23390, #181082, #149729, #85036, #146717, #41563, #42557, #104220, #102226, #193242, #9227, #163915, #54715, #10226, #116387, #194250, #178077, #39544, #180095, #71886, #101203, #165901, #162893, #24402, #195247, #147740, #27399, #103226, #70894, #132561, #25411, #164908, #26402, #29376, #56566, #154686, #151719, #43545, #16181, #197238, #105211, #199209, #120369, #122351, #93997, #986, #58699, #60676, #184040, #32344, #139503, #31349, #166898, #155678, #185028, #93000, #62661, #45523, #17173, #152693, #107177, #135566 ),
 ( #77836, #182062, #44538, #28398, #168848, #108174, #30353, #46515, #61666, #124340, #90037, #13212, #169855, #167877, #75851, #123335, #76844, #138515, #91007, #91995, #186036, #74875, #153689, #106193, #137527, #198218, #14182, #15185, #136537, #59690, #47518, #109174, #170853, #121361, #183054, #110169, #125348, #81787, #21140, #158651, #95990, #3970, #172848, #143474, #159644, #37303, #49497, #189023, #129298, #190994, #97952, #36297, #1994, #66643, #175830, #4958, #96970, #34329, #113142, #142492, #33336, #187045, #98962, #126328, #52470, #20142, #171848, #78827, #114129, #111159, #80814, #141503, #157675, #112161, #63673, #48515, #19165, #128306, #190006, #82795, #65650, #94996, #156682, #51480, #144477, #174832, #127312, #50497, #173850, #5961, #67639, #160652, #35316, #140505, #18176, #79833, #2988, #64666, #188025, #9986, #119160, #148495, #40308, #116149, #56480, #85809, #176842, #130291, #180843, #69646, #134331, #163665, #53472, #22144, #196015, #103981, #23148, #86809, #178840, #83794, #41319, #42320, #145474, #25167, #99968, #118158, #117145, #6955, #26160, #164664, #68635, #161652, #177840, #71646, #102979, #38313, #191985, #87801, #115149, #84792, #147495, #146471, #8986, #7963, #149487, #131312, #70654, #132320, #193002, #10983, #179848, #54479, #39308, #133313, #72656, #57491, #194012, #100967, #162652, #55475, #24158, #101984, #195002, #167646, #29142, #46280, #90779, #152463, #183807, #105961, #59452, #75615, #43306, #13949, #61437, #62427, #74641, #135330, #137294, #138291, #198976, #14953, #91761, #169622, #197003, #124099, #199972, #197982, #60443, #30120, #106947, #168620, #121125, #122118, #154457, #120136, #45295, #153455, #76613, #123109, #184794, #104974, #182820, #12977, #185798, #107936, #31119, #58469, #11995, #92767, #15949, #77608, #47286, #139279, #756, #165660, #181827, #27158, #166661, #73658, #88805, #150498, #28162, #89804, #151486, #136307, #44302, #2756, #64432, #159408, #20903, #140267, #190762, #3739, #66412, #126102, #35082, #48281, #109936, #96735, #158424, #143240, #49267, #187798, #1759, #142255, #110925, #93769, #50268, #94762, #36069, #82561, #141266, #189777, #111926, #172611, #127077, #34098, #188785, #18936, #171618, #157441, #63437, #129061, #97718, #79597, #144243, #125113, #4723, #65416, #155450, #108942, #33106, #173612, #19912, #5727, #156444, #95756, #81554, #80581, #16940, #128074, #51249, #67406, #170623, #32112, #112909, #78594, #174603, #186811, #17943, #193772, #87573, #102748, #6721, #55241, #84556, #85569, #38078, #177607, #134093, #161418, #160421, #175592, #56242, #71414, #164436, #147255, #21910, #149260, #10752, #146234, #192762, #41085, #145240, #191751, #116909, #22910, #83561, #194768, #68399, #131073, #115917, #72416, #52237, #37068, #39075, #113894, #117923, #98727, #100732, #162413, #130051, #179612, #148257, #53234, #114910, #101742, #9750, #25930, #23915, #176604, #69407, #8746, #99734, #70416, #7721, #54245, #132083, #133078, #178602, #40065, #163430, #24928, #86573, #105729, #73428, #44069, #91525, #92531, #104741, #165432, #167416, #168392, #120887, #45060, #121882, #199735, #26927, #154220, #29887, #27927, #136077, #60212, #137057, #198747, #89570, #28912, #184561, #150267, #182586, #166432, #197751, #58243, #12746, #90552, #180615, #118930, #151256, #106718, #153212, #138054, #74411, #88569, #42088, #183575, #61201, #75385, #59218, #152234, #13719, #14717, #76377, #15710, #122873, #46042, #107697, #169376, #30884, #77370, #103753, #195783, #57256, #11761, #135099, #196775, #119911, #181597, #43074, #47046, #97480, #186570, #51011, #80341, #170382, #139038, #112672, #20661, #140025, #3502, #95514, #518, #158188, #159166, #62190, #142013, #16701, #34843, #33854, #35834, #143003, #81320, #123854, #78351, #32868, #65178, #19678, #155212, #108703, #4481, #185552, #31873, #2515, #96498, #157200, #93527, #66171 ),
 ( #64195, #18694, #141028, #1514, #172364, #127833, #174364, #63191, #124871, #125862, #189539, #49029, #48043, #94518, #126837, #109699, #171381, #156200, #188543, #17700, #50021, #79357, #187562, #110684, #111686, #173373, #5486, #86334, #101492, #132840, #177369, #190525, #117677, #40836, #176363, #22673, #71176, #175352, #21669, #147015, #191512, #113658, #24685, #51999, #161176, #145999, #102509, #164193, #85323, #115681, #130833, #69166, #83323, #37836, #129813, #82315, #8500, #148021, #36820, #128826, #9510, #84320, #194527, #144005, #38840, #192524, #7482, #98486, #67169, #160179, #145000, #54007, #100498, #6481, #55999, #162177, #68161, #23675, #99496, #70177, #179374, #52989, #114667, #131845, #193528, #39826, #55002, #116671, #178362, #163181, #151996, #13482, #59973, #166187, #104506, #57011, #58983, #27688, #10510, #167176, #11520, #152971, #137810, #58009, #106472, #28675, #119679, #43826, #181362, #105490, #135846, #199494, #42841, #168151, #90310, #89329, #75147, #151021, #136818, #197515, #165189, #74176, #180376, #45806, #14470, #196539, #76132, #118684, #121640, #182348, #72172, #107457, #26684, #120650, #198502, #60960, #88324, #12512, #183335, #44817, #133847, #29648, #91280, #122634, #25691, #184324, #87336, #149022, #195537, #41846, #103513, #150014, #73190, #134861, #123615, #110446, #1268, #2271, #154966, #94278, #50777, #78111, #77129, #92291, #173131, #188302, #19442, #63954, #138798, #4248, #127601, #62945, #109452, #157951, #61948, #108460, #33613, #139780, #279, #111444, #185310, #47802, #32624, #189300, #169133, #172127, #125623, #17453, #155956, #170137, #124625, #16462, #30638, #95276, #34606, #46801, #15472, #96265, #171135, #81090, #153975, #187321, #79109, #140782, #31632, #93281, #186320, #48792, #156959, #18456, #80107, #142768, #141775, #3269, #64941, #126600, #49779, #65928, #162938, #143763, #194294, #7242, #69937, #129577, #38601, #51758, #113419, #100257, #161938, #36579, #5244, #70937, #159937, #24445, #53765, #66924, #112437, #86094, #174126, #6245, #67924, #147785, #9271, #128588, #35597, #68927, #131601, #191274, #23433, #175111, #98234, #85080, #146764, #190282, #130589, #132605, #21424, #145760, #52749, #97243, #115439, #83084, #39590, #158931, #144760, #193286, #177130, #114418, #192284, #176119, #8257, #22431, #37590, #160939, #99252, #20420, #101249, #84081, #82070, #54760, #116434, #178122, #102271, #140303, #195292, #91795, #200005, #93802, #56773, #119442, #138323, #57772, #163959, #153489, #790, #32145, #55760, #155482, #181127, #108976, #165947, #47321, #11275, #61471, #16974, #170657, #10271, #123142, #88087, #14985, #41607, #42601, #117434, #164952, #25457, #179132, #62462, #77642, #78628, #76645, #87097, #40600, #148782, #149773, #196302, #71930, #133600, #118446, #184829, #26445, #180138, #124135, #103272, #134618, #104265, #72948, #27447, #46315, #107970, #169657, #31153, #92801, #154489, #15983, #139311, #185834, #144274, #94797, #48315, #5761, #142291, #67437, #83593, #35115, #188817, #65448, #171649, #160452, #17977, #109970, #3771, #111957, #64468, #129094, #96767, #1794, #81586, #143272, #18968, #127110, #95789, #66444, #82592, #21943, #172642, #173646, #52268, #113926, #20935, #159440, #125147, #189809, #98759, #128105, #19945, #157475, #33139, #50300, #126135, #156476, #63472, #49299, #175626, #4755, #79631, #186846, #37100, #141299, #2789, #51281, #158456, #187830, #190794, #110958, #34130, #112942, #80614, #97752, #174635, #36100, #149288, #87602, #26958, #84589, #39107, #9782, #164465, #161452, #53266, #25959, #6754, #114944, #8777, #130086, #132112, #103782, #10782, #68433, #70446, #193805, #42120, #72449, #41114, #176637, #165462, #194798, #102778, #134124, #55271, #145273, #162445, #116940, #191785, #40096, #22943, #147287, #178633, #195813, #101774, #163461, #24959, #85600, #100763, #86605, #146269, #148288, #57285 ),
 ( #71444, #133109, #56271, #117954, #177640, #179645, #118959, #99767, #180645, #115950, #38112, #7755, #23946, #69439, #131107, #192795, #54277, #138088, #199769, #30918, #105762, #119941, #135130, #91561, #92566, #153249, #107731, #104774, #196804, #169413, #150297, #58272, #152267, #73457, #75420, #47079, #154254, #11793, #13752, #137094, #185589, #15745, #184596, #181626, #108740, #61236, #46077, #77404, #198780, #170416, #167448, #60246, #88601, #183610, #166462, #90586, #121917, #139074, #45094, #106751, #168426, #28945, #182619, #29921, #27959, #14751, #552, #43106, #197785, #89600, #76412, #122908, #62223, #123891, #151288, #12777, #74442, #136109, #59251, #120920, #44104, #96533, #173408, #34879, #64233, #3537, #20697, #186605, #18730, #2551, #33893, #94557, #49067, #65214, #16737, #155247, #187598, #81355, #143039, #174400, #110723, #63227, #78385, #158223, #35870, #111722, #172404, #157237, #125898, #19713, #112708, #190561, #95550, #142050, #82353, #144041, #51046, #189574, #140061, #4517, #128861, #66210, #50061, #80378, #124907, #126874, #156236, #48077, #52035, #79395, #5523, #127870, #109733, #31908, #67203, #113692, #32903, #97516, #188580, #93561, #159203, #1552, #171417, #17738, #141065, #71211, #70213, #72208, #179407, #117711, #57046, #114706, #69202, #85358, #53025, #23711, #132874, #133882, #84356, #145036, #147051, #148054, #100533, #24720, #101527, #40871, #6518, #195573, #9545, #7517, #115717, #39861, #116707, #178397, #130870, #8534, #164228, #129849, #162212, #146034, #177405, #37874, #192560, #131880, #160216, #98523, #54043, #86369, #194563, #102545, #38876, #68197, #21706, #163218, #25725, #55037, #193565, #56033, #87371, #149056, #10544, #175388, #36856, #83360, #191548, #176399, #99532, #161214, #22709, #75179, #199526, #136851, #167210, #166218, #88357, #135876, #119710, #150050, #60994, #181394, #76165, #90343, #11556, #118720, #137845, #180409, #42872, #198536, #28707, #41881, #29680, #103548, #165223, #60007, #104537, #91312, #152028, #26718, #184356, #122668, #73222, #151051, #43859, #153004, #134893, #89362, #27719, #196569, #12542, #74207, #13514, #197547, #121674, #58040, #59015, #182381, #120682, #105524, #183369, #44851, #106507, #168184, #14503, #148712, #56702, #103201, #86026, #119373, #116363, #9203, #196235, #194225, #177063, #101180, #162868, #180069, #24376, #147715, #117364, #39520, #193216, #70868, #132536, #68859, #57704, #115374, #145694, #55690, #179060, #161871, #164882, #40529, #99185, #102200, #54690, #178052, #149704, #11202, #130518, #181056, #163888, #118375, #25385, #87027, #38533, #100189, #10200, #71860, #23365, #133529, #160874, #192214, #195221, #41537, #84016, #26377, #85011, #88016, #72878, #131532, #134546, #22364, #7176, #53697, #146691, #8187, #69863, #182038, #90981, #197213, #62639, #31325, #13187, #169832, #73872, #76821, #199184, #89019, #124315, #43520, #75826, #184017, #77812, #105186, #106169, #122325, #44513, #150710, #137504, #185004, #16158, #42532, #139481, #167852, #92977, #152668, #154662, #198194, #45499, #963, #104195, #58676, #107154, #74850, #60652, #28374, #29352, #165876, #151696, #12209, #27372, #46488, #61643, #135542, #168824, #120343, #166873, #90012, #136513, #183030, #59664, #121337, #14158, #30329, #91971, #153665, #108148, #15161, #138492, #200174, #123311, #67611, #188997, #19138, #34303, #172823, #125325, #79807, #33313, #144450, #50473, #128281, #78804, #32323, #189978, #126305, #51453, #186013, #80789, #141479, #94973, #5935, #112133, #113114, #140482, #93976, #174804, #188001, #36270, #47495, #142467, #95965, #49471, #155656, #109152, #1970, #17151, #111134, #157649, #48492, #97925, #3945, #170831, #65624, #2963, #64643, #159618, #21114, #63650, #187022, #127284, #143448, #173825, #35289, #110146, #171825, #96945, #158626, #156657, #20117, #82769, #18153, #81761, #4934, #66617, #147891, #24551 ),
 ( #89191, #57875, #39693, #196405, #100364, #103376, #25561, #115547, #150884, #8366, #102373, #10377, #104367, #70041, #132709, #148886, #71042, #177235, #164062, #11380, #42706, #69031, #166051, #194397, #119547, #179237, #181230, #86201, #72034, #27551, #130696, #23539, #133707, #101355, #87205, #54867, #55865, #192390, #178229, #38707, #53873, #73050, #88191, #162043, #195399, #85185, #146874, #131710, #163044, #9377, #193391, #116541, #117539, #56877, #40703, #118551, #134722, #180242, #41711, #165054, #26547, #149875, #15334, #45672, #60825, #199360, #151861, #107323, #170005, #29518, #138663, #13352, #75016, #144, #61813, #28542, #168996, #112067, #43691, #30500, #152841, #197383, #12379, #106336, #182207, #105353, #44683, #93149, #76992, #168022, #92151, #91152, #153837, #122499, #136681, #184190, #167040, #35223, #3877, #183201, #142398, #90178, #46666, #123483, #58848, #96876, #198363, #185175, #108325, #50407, #59838, #76000, #31496, #14335, #120515, #154833, #16332, #188929, #74041, #173755, #137674, #65556, #80720, #127215, #135712, #121507, #193911, #8884, #113048, #99874, #190900, #191891, #144381, #83701, #40203, #67544, #66551, #81692, #162550, #177743, #70552, #53375, #128215, #55375, #117045, #52376, #98865, #147396, #51387, #97857, #23051, #129202, #189912, #100868, #174740, #37209, #22050, #178740, #158559, #161558, #115053, #6861, #145379, #159546, #114033, #5868, #20049, #84696, #24054, #36203, #4866, #85710, #160560, #132219, #143374, #176745, #68540, #130195, #21044, #82697, #175730, #38218, #146376, #7863, #69550, #131214, #192905, #54382, #116054, #39212, #195918, #152370, #13855, #133213, #183715, #44207, #42224, #105866, #101883, #135236, #88708, #165565, #71547, #60350, #118061, #148393, #103885, #11900, #164567, #167553, #196908, #163565, #181729, #57393, #119066, #75522, #137197, #194904, #25065, #58375, #59356, #180748, #28065, #41221, #102882, #89706, #151392, #179751, #120042, #198883, #56378, #43210, #27062, #86708, #9887, #150404, #26061, #87704, #134233, #182722, #104877, #73563, #166566, #12882, #74547, #136212, #149389, #197887, #10885, #122024, #90688, #72555, #29048, #121025, #79503, #1662, #91666, #126980, #184699, #78496, #186713, #80485, #46183, #108844, #125017, #47185, #153356, #140169, #187703, #18840, #45201, #142159, #170525, #95657, #155356, #34001, #657, #48183, #3643, #157345, #199878, #109839, #77510, #63340, #31020, #32014, #106855, #154358, #14858, #168530, #49173, #64338, #65321, #171522, #76519, #30028, #138195, #139181, #185695, #61342, #123013, #107836, #33011, #15851, #169520, #110832, #92670, #123997, #93671, #62327, #16846, #94666, #156345, #17845, #141172, #2661, #126007, #172516, #147160, #191656, #130976, #81458, #34987, #145143, #85471, #19817, #21814, #128967, #173514, #188689, #82459, #158328, #143144, #20804, #69310, #53135, #144147, #6626, #5631, #68305, #98629, #127976, #36968, #4624, #8648, #177513, #159309, #115823, #66315, #22816, #129956, #96640, #70322, #189679, #83466, #114814, #23821, #51151, #52143, #176506, #190667, #112812, #37983, #192667, #162320, #50169, #111826, #113800, #38983, #160323, #100639, #67308, #99640, #174505, #35972, #97619, #161323, #175495, #84462, #146140, #7626, #54150, #40988, #39973, #55145, #135987, #151165, #182490, #26829, #101643, #167322, #90458, #25836, #72320, #120790, #24830, #71322, #196683, #102656, #163334, #74320, #86480, #10657, #195687, #152142, #13625, #135005, #165337, #180520, #118837, #132985, #87480, #179519, #131989, #58152, #197658, #148165, #178507, #59124, #133996, #43971, #193674, #88470, #41993, #57158, #9656, #116816, #194676, #56145, #103659, #150167, #117826, #105633, #11667, #164341, #73333, #149167, #119820, #28818, #181505, #42983, #104648, #166335, #89474, #27833, #12653, #14619, #76276, #1413, #124771, #91428, #172266, #184467, #44964, #123755, #47946, #418 ),
 ( #64095, #29792, #62092, #45946, #77269, #137954, #92432, #108604, #60118, #198652, #30785, #186469, #109597, #17598, #154119, #106622, #121786, #78251, #79257, #155110, #15612, #185454, #169279, #139924, #156100, #33756, #107601, #46944, #125763, #187463, #94420, #32768, #183480, #63092, #95415, #171280, #93423, #138938, #168296, #170281, #199638, #153115, #157100, #122777, #48931, #16604, #61104, #31775, #140929, #2415, #110585, #75292, #136963, #18596, #37734, #177272, #100401, #160080, #96403, #114566, #113561, #115584, #22574, #161079, #80244, #158090, #112575, #83227, #99396, #34744, #126738, #84221, #141914, #188441, #82215, #3405, #5388, #38743, #145900, #65080, #143906, #67071, #49920, #7384, #176263, #111585, #173270, #68064, #69068, #130735, #128730, #19582, #35737, #190426, #81225, #175255, #142906, #20564, #51902, #192427, #36721, #98383, #21567, #159070, #174269, #144902, #4387, #6385, #53909, #66072, #127738, #189440, #50917, #129718, #97384, #191415, #52891, #27591, #85224, #25597, #148924, #58886, #166088, #57912, #131747, #120552, #11419, #119584, #89229, #10413, #182245, #179276, #72071, #43730, #56914, #39730, #164098, #87241, #42744, #133744, #195439, #180279, #102411, #55903, #118589, #101391, #41749, #181267, #162082, #71078, #193429, #103413, #134760, #165091, #73089, #88228, #150923, #54905, #23576, #196442, #194432, #26585, #149912, #104406, #12416, #117576, #74078, #135749, #116578, #197420, #132744, #146915, #24588, #40741, #8404, #70079, #178267, #163084, #86236, #147926, #9412, #122536, #136719, #151899, #108365, #47706, #185212, #184227, #30538, #199397, #170043, #186225, #63859, #76038, #15372, #155860, #17358, #124530, #62846, #28580, #93186, #2179, #31533, #123519, #60861, #198400, #169032, #29555, #59878, #125530, #152877, #79013, #46703, #90216, #45708, #107359, #121544, #106376, #154871, #61850, #105392, #109356, #187227, #167078, #16368, #183239, #1171, #182, #13389, #171038, #32529, #75053, #44720, #92190, #78016, #94181, #168058, #153874, #91188, #14372, #139685, #140687, #137713, #77028, #138700, #142676, #113329, #129488, #7146, #19353, #158837, #99157, #160846, #67832, #6152, #172032, #36485, #145665, #175022, #66831, #4155, #80017, #112343, #173037, #141686, #68830, #96173, #22335, #190190, #33520, #127504, #65834, #64850, #49682, #98141, #5149, #48698, #191186, #130489, #110350, #51665, #126512, #144667, #143668, #95182, #52662, #114324, #156868, #188210, #189208, #159840, #176027, #111347, #18364, #37495, #3177, #34515, #174033, #157863, #35504, #81002, #83986, #50686, #97154, #20325, #81974, #128495, #21333, #82991, #150683, #41510, #149677, #196206, #179031, #12181, #9173, #102170, #88992, #86998, #69833, #194197, #55662, #72850, #117336, #40498, #10173, #132508, #85997, #163858, #131500, #25357, #87989, #73845, #101151, #161842, #148685, #164853, #71833, #103173, #118347, #57678, #23336, #192185, #26349, #24346, #133502, #56674, #195194, #180041, #147686, #11175, #181030, #146662, #134520, #162838, #119346, #54660, #70840, #42504, #177034, #115344, #104168, #165850, #27346, #53666, #38504, #100160, #84980, #8157, #193187, #116334, #178023, #39491, #136486, #199155, #15131, #137475, #43494, #168796, #77783, #109123, #17123, #170801, #60622, #185983, #45471, #124286, #90953, #76793, #32293, #47466, #89986, #138464, #167824, #30300, #121310, #122296, #135516, #44486, #105160, #58651, #139452, #154633, #93949, #91943, #166846, #155627, #197187, #29323, #75797, #120317, #28348, #74825, #200145, #106142, #151667, #933, #13161, #14130, #183986, #182011, #198166, #61615, #153636, #107125, #123283, #59636, #152640, #183002, #184974, #46459, #62607, #108119, #169802, #31295, #92947, #16128, #160600, #112107, #65599, #142441, #48463, #37250, #94946, #125297, #80763, #188972, #141452, #82743, #173798, #78775, #158601, #172797, #34278, #129244, #190940, #110120 ),
 ( #126279, #52417, #20091, #1941, #157623, #95937, #156630, #79780, #143421, #35264, #140451, #97898, #98907, #63621, #81735, #18125, #174779, #96919, #175776, #144423, #21086, #186993, #2937, #19113, #171798, #33286, #111108, #159589, #4908, #3919, #66591, #127259, #128255, #50448, #64617, #189953, #187976, #49445, #67586, #51427, #5909, #113087, #36245, #114075, #68580, #106651, #161597, #55415, #163605, #60145, #23091, #85750, #101923, #24096, #130236, #117086, #167348, #198678, #22090, #121813, #147437, #75318, #132261, #13651, #177781, #25106, #183508, #136989, #176785, #86750, #54423, #178781, #7905, #8925, #83740, #131256, #191932, #145419, #28845, #43999, #44991, #40249, #53416, #6901, #115093, #116093, #162591, #38258, #99912, #84736, #148433, #192944, #146414, #90486, #69589, #100907, #70593, #39251, #193952, #9928, #71587, #133253, #197684, #59149, #120819, #182519, #105661, #152168, #110614, #61132, #14646, #172296, #108633, #33785, #49952, #1444, #155141, #31804, #137984, #126767, #184495, #76306, #170311, #78281, #30812, #95445, #63122, #168323, #47975, #62122, #123785, #18625, #80272, #199667, #29820, #124801, #125792, #185484, #94450, #107628, #169306, #156130, #17629, #45974, #186499, #65109, #122805, #109627, #93453, #153144, #91456, #16634, #92461, #77299, #154149, #15641, #157129, #187494, #141942, #171311, #138969, #3433, #188471, #46974, #139954, #447, #32798, #79288, #140958, #2445, #64127, #48960, #81252, #190455, #175284, #131774, #193456, #114594, #144930, #160109, #98413, #50945, #5416, #159098, #70105, #176291, #53936, #4415, #158118, #115611, #51930, #177300, #111616, #6411, #21597, #36749, #142934, #173301, #127767, #19610, #113590, #83255, #174295, #38771, #68092, #34775, #191442, #67099, #128758, #162109, #23606, #66101, #96432, #129745, #69095, #52918, #37763, #112603, #35765, #99425, #161107, #189467, #22602, #8433, #97411, #84249, #145929, #20592, #82244, #7412, #143935, #130762, #192454, #100428, #85252, #146943, #73120, #10441, #134789, #165120, #194458, #103440, #9439, #75080, #43758, #25622, #182277, #86263, #89260, #11448, #101420, #136747, #55929, #88255, #196471, #90244, #117604, #118617, #57941, #56943, #163112, #149942, #197449, #28606, #54932, #151927, #180307, #105422, #26612, #167105, #72101, #119612, #13416, #116605, #71104, #181295, #87266, #42773, #40768, #41775, #148951, #104435, #179304, #133774, #166119, #39757, #178293, #195468, #27621, #150952, #58915, #12446, #147953, #24615, #74108, #120583, #135778, #132771, #102437, #164124, #62880, #79045, #156898, #169064, #108397, #48727, #110380, #17389, #155891, #121573, #186257, #95212, #124560, #16400, #92221, #29583, #61880, #122567, #91214, #18394, #45739, #172063, #139715, #183268, #77059, #153907, #14402, #199426, #47735, #154901, #198432, #140719, #80045, #59905, #1203, #76067, #94212, #93216, #44748, #2209, #63890, #106404, #137742, #15402, #109388, #125561, #60891, #168086, #187258, #152905, #184257, #123550, #107391, #185244, #30570, #33550, #138731, #46736, #170074, #211, #31565, #78046, #171068, #32558, #191217, #99190, #145698, #128524, #161876, #158867, #51697, #38538, #36516, #19380, #143698, #5180, #22369, #66861, #190218, #159873, #82004, #35533, #113360, #81029, #175052, #37527, #100194, #50715, #111378, #98171, #114355, #21364, #52691, #67862, #7180, #173066, #23370, #176060, #174065, #83022, #6182, #144696, #129517, #97181, #160878, #130523, #96202, #142705, #84020, #68864, #192220, #49713, #53702, #115379, #177067, #141714, #3204, #64878, #126539, #188238, #34543, #20356, #157891, #4184, #65863, #127535, #189237, #112373, #118379, #70873, #10205, #166877, #194229, #193221, #8193, #89023, #104199, #135546, #180073, #54695, #120347, #43525, #179065, #25390, #73876, #178056, #24381, #149708, #55695, #116368, #27377, #39524, #163894, #148717, #105190, #85015, #88020 ) ),
 .UNSPECIFIED., .T., .F., .T. ) 
 B_SPLINE_SURFACE_WITH_KNOTS ( ( 4, 3, 4 ),
 ( 3, 2, 2, 2, 2, 2, 2, 2, 2, 2, 2, 2, 2, 2, 2, 2, 2, 2, 2, 2, 2, 2, 2, 2, 2, 2, 2, 2, 2, 2, 2, 2, 2, 2, 2, 2, 2, 2, 2, 2, 2, 2, 2, 2, 2, 2, 2, 2, 2, 2, 2, 2, 2, 2, 2, 2, 2, 2, 2, 2, 2, 2, 2, 2, 2, 2, 2, 2, 2, 2, 2, 2, 2, 2, 2, 2, 2, 2, 2, 2, 2, 2, 2, 2, 2, 2, 2, 2, 2, 2, 2, 2, 2, 2, 2, 2, 2, 2, 2, 2, 2, 2, 2, 2, 2, 2, 2, 2, 2, 2, 2, 2, 2, 2, 2, 2, 2, 2, 2, 2, 2, 2, 2, 2, 2, 2, 2, 2, 2, 2, 2, 2, 2, 2, 2, 2, 2, 2, 2, 2, 2, 2, 2, 2, 2, 2, 2, 2, 2, 2, 2, 2, 2, 2, 2, 2, 2, 2, 2, 2, 2, 2, 2, 2, 2, 2, 2, 2, 2, 2, 2, 2, 2, 2, 2, 2, 2, 2, 2, 2, 2, 2, 2, 2, 2, 2, 2, 2, 2, 2, 2, 2, 2, 2, 2, 2, 2, 2, 2, 2, 2, 2, 2, 2, 2, 2, 2, 2, 2, 2, 2, 2, 2, 2, 2, 2, 2, 2, 2, 2, 2, 2, 2, 2, 2, 2, 2, 2, 3 ),
 ( 0.000000000000000000, 0.5000000000000000000, 1.000000000000000000 ),
 ( 0.000000000000000000, 0.004385964912280701511, 0.008771929824561403022, 0.01315789473684210453, 0.01754385964912280604, 0.02192982456140350755, 0.02631578947368420907, 0.03070175438596491058, 0.03508771929824561209, 0.03947368421052631360, 0.04385964912280701511, 0.04824561403508771662, 0.05263157894736841813, 0.05701754385964911964, 0.06140350877192982115, 0.06578947368421052266, 0.07017543859649122417, 0.07456140350877192569, 0.07894736842105262720, 0.08333333333333332871, 0.08771929824561403022, 0.09210526315789473173, 0.09649122807017543324, 0.1008771929824561348, 0.1052631578947368363, 0.1096491228070175378, 0.1140350877192982393, 0.1184210526315789408, 0.1228070175438596423, 0.1271929824561403577, 0.1315789473684210453, 0.1359649122807017607, 0.1403508771929824483, 0.1447368421052631637, 0.1491228070175438514, 0.1535087719298245668, 0.1578947368421052544, 0.1622807017543859698, 0.1666666666666666574, 0.1710526315789473728, 0.1754385964912280604, 0.1798245614035087758, 0.1842105263157894635, 0.1885964912280701788, 0.1929824561403508665, 0.1973684210526315819, 0.2017543859649122695, 0.2061403508771929849, 0.2105263157894736725, 0.2149122807017543879, 0.2192982456140350755, 0.2236842105263157909, 0.2280701754385964786, 0.2324561403508771940, 0.2368421052631578816, 0.2412280701754385970, 0.2456140350877192846, 0.2500000000000000000, 0.2543859649122807154, 0.2587719298245614308, 0.2631578947368420907, 0.2675438596491228060, 0.2719298245614035214, 0.2763157894736842368, 0.2807017543859648967, 0.2850877192982456121, 0.2894736842105263275, 0.2938596491228070429, 0.2982456140350877027, 0.3026315789473684181, 0.3070175438596491335, 0.3114035087719298489, 0.3157894736842105088, 0.3201754385964912242, 0.3245614035087719396, 0.3289473684210526550, 0.3333333333333333148, 0.3377192982456140302, 0.3421052631578947456, 0.3464912280701754610, 0.3508771929824561209, 0.3552631578947368363, 0.3596491228070175517, 0.3640350877192982670, 0.3684210526315789269, 0.3728070175438596423, 0.3771929824561403577, 0.3815789473684210731, 0.3859649122807017330, 0.3903508771929824483, 0.3947368421052631637, 0.3991228070175438791, 0.4035087719298245390, 0.4078947368421052544, 0.4122807017543859698, 0.4166666666666666852, 0.4210526315789473450, 0.4254385964912280604, 0.4298245614035087758, 0.4342105263157894912, 0.4385964912280701511, 0.4429824561403508665, 0.4473684210526315819, 0.4517543859649122973, 0.4561403508771929571, 0.4605263157894736725, 0.4649122807017543879, 0.4692982456140351033, 0.4736842105263157632, 0.4780701754385964786, 0.4824561403508771940, 0.4868421052631579093, 0.4912280701754385692, 0.4956140350877192846, 0.5000000000000000000, 0.5043859649122807154, 0.5087719298245614308, 0.5131578947368421462, 0.5175438596491228616, 0.5219298245614034659, 0.5263157894736841813, 0.5307017543859648967, 0.5350877192982456121, 0.5394736842105263275, 0.5438596491228070429, 0.5482456140350877583, 0.5526315789473684736, 0.5570175438596490780, 0.5614035087719297934, 0.5657894736842105088, 0.5701754385964912242, 0.5745614035087719396, 0.5789473684210526550, 0.5833333333333333703, 0.5877192982456140857, 0.5921052631578946901, 0.5964912280701754055, 0.6008771929824561209, 0.6052631578947368363, 0.6096491228070175517, 0.6140350877192982670, 0.6184210526315789824, 0.6228070175438596978, 0.6271929824561403022, 0.6315789473684210176, 0.6359649122807017330, 0.6403508771929824483, 0.6447368421052631637, 0.6491228070175438791, 0.6535087719298245945, 0.6578947368421053099, 0.6622807017543859143, 0.6666666666666666297, 0.6710526315789473450, 0.6754385964912280604, 0.6798245614035087758, 0.6842105263157894912, 0.6885964912280702066, 0.6929824561403509220, 0.6973684210526315264, 0.7017543859649122417, 0.7061403508771929571, 0.7105263157894736725, 0.7149122807017543879, 0.7192982456140351033, 0.7236842105263158187, 0.7280701754385965341, 0.7324561403508771384, 0.7368421052631578538, 0.7412280701754385692, 0.7456140350877192846, 0.7500000000000000000, 0.7543859649122807154, 0.7587719298245614308, 0.7631578947368421462, 0.7675438596491228616, 0.7719298245614034659, 0.7763157894736841813, 0.7807017543859648967, 0.7850877192982456121, 0.7894736842105263275, 0.7938596491228070429, 0.7982456140350877583, 0.8026315789473684736, 0.8070175438596490780, 0.8114035087719297934, 0.8157894736842105088, 0.8201754385964912242, 0.8245614035087719396, 0.8289473684210526550, 0.8333333333333333703, 0.8377192982456140857, 0.8421052631578946901, 0.8464912280701754055, 0.8508771929824561209, 0.8552631578947368363, 0.8596491228070175517, 0.8640350877192982670, 0.8684210526315789824, 0.8728070175438596978, 0.8771929824561403022, 0.8815789473684210176, 0.8859649122807017330, 0.8903508771929824483, 0.8947368421052631637, 0.8991228070175438791, 0.9035087719298245945, 0.9078947368421053099, 0.9122807017543859143, 0.9166666666666666297, 0.9210526315789473450, 0.9254385964912280604, 0.9298245614035087758, 0.9342105263157894912, 0.9385964912280702066, 0.9429824561403509220, 0.9473684210526315264, 0.9517543859649122417, 0.9561403508771929571, 0.9605263157894736725, 0.9649122807017543879, 0.9692982456140351033, 0.9736842105263158187, 0.9780701754385965341, 0.9824561403508771384, 0.9868421052631578538, 0.9912280701754385692, 0.9956140350877192846, 1.000000000000000000 ),
 .UNSPECIFIED. ) 
 GEOMETRIC_REPRESENTATION_ITEM ( )  RATIONAL_B_SPLINE_SURFACE ( (
 ( 1.000000000000000000, 0.9659258262890683122, 1.000000000000000000, 0.9659258262890683122, 1.000000000000000000, 0.9659258262890683122, 1.000000000000000000, 0.9659258262890683122, 1.000000000000000000, 0.9659258262890683122, 1.000000000000000000, 0.9659258262890683122, 1.000000000000000000, 0.9659258262890683122, 1.000000000000000000, 0.9659258262890683122, 1.000000000000000000, 0.9659258262890683122, 1.000000000000000000, 0.9659258262890683122, 1.000000000000000000, 0.9659258262890683122, 1.000000000000000000, 0.9659258262890683122, 1.000000000000000000, 0.9659258262890683122, 1.000000000000000000, 0.9659258262890683122, 1.000000000000000000, 0.9659258262890683122, 1.000000000000000000, 0.9659258262890683122, 1.000000000000000000, 0.9659258262890683122, 1.000000000000000000, 0.9659258262890683122, 1.000000000000000000, 0.9659258262890683122, 1.000000000000000000, 0.9659258262890683122, 1.000000000000000000, 0.9659258262890683122, 1.000000000000000000, 0.9659258262890683122, 1.000000000000000000, 0.9659258262890683122, 1.000000000000000000, 0.9659258262890683122, 1.000000000000000000, 0.9659258262890683122, 1.000000000000000000, 0.9659258262890683122, 1.000000000000000000, 0.9659258262890683122, 1.000000000000000000, 0.9659258262890683122, 1.000000000000000000, 0.9659258262890683122, 1.000000000000000000, 0.9659258262890683122, 1.000000000000000000, 0.9659258262890683122, 1.000000000000000000, 0.9659258262890683122, 1.000000000000000000, 0.9659258262890683122, 1.000000000000000000, 0.9659258262890683122, 1.000000000000000000, 0.9659258262890683122, 1.000000000000000000, 0.9659258262890683122, 1.000000000000000000, 0.9659258262890683122, 1.000000000000000000, 0.9659258262890683122, 1.000000000000000000, 0.9659258262890683122, 1.000000000000000000, 0.9659258262890683122, 1.000000000000000000, 0.9659258262890683122, 1.000000000000000000, 0.9659258262890683122, 1.000000000000000000, 0.9659258262890683122, 1.000000000000000000, 0.9659258262890683122, 1.000000000000000000, 0.9659258262890683122, 1.000000000000000000, 0.9659258262890683122, 1.000000000000000000, 0.9659258262890683122, 1.000000000000000000, 0.9659258262890683122, 1.000000000000000000, 0.9659258262890683122, 1.000000000000000000, 0.9659258262890683122, 1.000000000000000000, 0.9659258262890683122, 1.000000000000000000, 0.9659258262890683122, 1.000000000000000000, 0.9659258262890683122, 1.000000000000000000, 0.9659258262890683122, 1.000000000000000000, 0.9659258262890683122, 1.000000000000000000, 0.9659258262890683122, 1.000000000000000000, 0.9659258262890683122, 1.000000000000000000, 0.9659258262890683122, 1.000000000000000000, 0.9659258262890683122, 1.000000000000000000, 0.9659258262890683122, 1.000000000000000000, 0.9659258262890683122, 1.000000000000000000, 0.9659258262890683122, 1.000000000000000000, 0.9659258262890683122, 1.000000000000000000, 0.9659258262890683122, 1.000000000000000000, 0.9659258262890683122, 1.000000000000000000, 0.9659258262890683122, 1.000000000000000000, 0.9659258262890683122, 1.000000000000000000, 0.9659258262890683122, 1.000000000000000000, 0.9659258262890683122, 1.000000000000000000, 0.9659258262890683122, 1.000000000000000000, 0.9659258262890683122, 1.000000000000000000, 0.9659258262890683122, 1.000000000000000000, 0.9659258262890683122, 1.000000000000000000, 0.9659258262890683122, 1.000000000000000000, 0.9659258262890683122, 1.000000000000000000, 0.9659258262890683122, 1.000000000000000000, 0.9659258262890683122, 1.000000000000000000, 0.9659258262890683122, 1.000000000000000000, 0.9659258262890683122, 1.000000000000000000, 0.9659258262890683122, 1.000000000000000000, 0.9659258262890683122, 1.000000000000000000, 0.9659258262890683122, 1.000000000000000000, 0.9659258262890683122, 1.000000000000000000, 0.9659258262890683122, 1.000000000000000000, 0.9659258262890683122, 1.000000000000000000, 0.9659258262890683122, 1.000000000000000000, 0.9659258262890683122, 1.000000000000000000, 0.9659258262890683122, 1.000000000000000000, 0.9659258262890683122, 1.000000000000000000, 0.9659258262890683122, 1.000000000000000000, 0.9659258262890683122, 1.000000000000000000, 0.9659258262890683122, 1.000000000000000000, 0.9659258262890683122, 1.000000000000000000, 0.9659258262890683122, 1.000000000000000000, 0.9659258262890683122, 1.000000000000000000, 0.9659258262890683122, 1.000000000000000000, 0.9659258262890683122, 1.000000000000000000, 0.9659258262890683122, 1.000000000000000000, 0.9659258262890683122, 1.000000000000000000, 0.9659258262890683122, 1.000000000000000000, 0.9659258262890683122, 1.000000000000000000, 0.9659258262890683122, 1.000000000000000000, 0.9659258262890683122, 1.000000000000000000, 0.9659258262890683122, 1.000000000000000000, 0.9659258262890683122, 1.000000000000000000, 0.9659258262890683122, 1.000000000000000000, 0.9659258262890683122, 1.000000000000000000, 0.9659258262890683122, 1.000000000000000000, 0.9659258262890683122, 1.000000000000000000, 0.9659258262890683122, 1.000000000000000000, 0.9659258262890683122, 1.000000000000000000, 0.9659258262890683122, 1.000000000000000000, 0.9659258262890683122, 1.000000000000000000, 0.9659258262890683122, 1.000000000000000000, 0.9659258262890683122, 1.000000000000000000, 0.9659258262890683122, 1.000000000000000000, 0.9659258262890683122, 1.000000000000000000, 0.9659258262890683122, 1.000000000000000000, 0.9659258262890683122, 1.000000000000000000, 0.9659258262890683122, 1.000000000000000000, 0.9659258262890683122, 1.000000000000000000, 0.9659258262890683122, 1.000000000000000000, 0.9659258262890683122, 1.000000000000000000, 0.9659258262890683122, 1.000000000000000000, 0.9659258262890683122, 1.000000000000000000, 0.9659258262890683122, 1.000000000000000000, 0.9659258262890683122, 1.000000000000000000, 0.9659258262890683122, 1.000000000000000000, 0.9659258262890683122, 1.000000000000000000, 0.9659258262890683122, 1.000000000000000000, 0.9659258262890683122, 1.000000000000000000, 0.9659258262890683122, 1.000000000000000000, 0.9659258262890683122, 1.000000000000000000, 0.9659258262890683122, 1.000000000000000000, 0.9659258262890683122, 1.000000000000000000, 0.9659258262890683122, 1.000000000000000000, 0.9659258262890683122, 1.000000000000000000, 0.9659258262890683122, 1.000000000000000000, 0.9659258262890683122, 1.000000000000000000, 0.9659258262890683122, 1.000000000000000000, 0.9659258262890683122, 1.000000000000000000, 0.9659258262890683122, 1.000000000000000000, 0.9659258262890683122, 1.000000000000000000, 0.9659258262890683122, 1.000000000000000000, 0.9659258262890683122, 1.000000000000000000, 0.9659258262890683122, 1.000000000000000000, 0.9659258262890683122, 1.000000000000000000, 0.9659258262890683122, 1.000000000000000000, 0.9659258262890683122, 1.000000000000000000, 0.9659258262890683122, 1.000000000000000000, 0.9659258262890683122, 1.000000000000000000, 0.9659258262890683122, 1.000000000000000000, 0.9659258262890683122, 1.000000000000000000, 0.9659258262890683122, 1.000000000000000000, 0.9659258262890683122, 1.000000000000000000, 0.9659258262890683122, 1.000000000000000000, 0.9659258262890683122, 1.000000000000000000, 0.9659258262890683122, 1.000000000000000000, 0.9659258262890683122, 1.000000000000000000, 0.9659258262890683122, 1.000000000000000000, 0.9659258262890683122, 1.000000000000000000, 0.9659258262890683122, 1.000000000000000000, 0.9659258262890683122, 1.000000000000000000, 0.9659258262890683122, 1.000000000000000000, 0.9659258262890683122, 1.000000000000000000, 0.9659258262890683122, 1.000000000000000000, 0.9659258262890683122, 1.000000000000000000, 0.9659258262890683122, 1.000000000000000000, 0.9659258262890683122, 1.000000000000000000, 0.9659258262890683122, 1.000000000000000000, 0.9659258262890683122, 1.000000000000000000, 0.9659258262890683122, 1.000000000000000000, 0.9659258262890683122, 1.000000000000000000, 0.9659258262890683122, 1.000000000000000000, 0.9659258262890683122, 1.000000000000000000, 0.9659258262890683122, 1.000000000000000000, 0.9659258262890683122, 1.000000000000000000, 0.9659258262890683122, 1.000000000000000000, 0.9659258262890683122, 1.000000000000000000, 0.9659258262890683122, 1.000000000000000000, 0.9659258262890683122, 1.000000000000000000, 0.9659258262890683122, 1.000000000000000000, 0.9659258262890683122, 1.000000000000000000, 0.9659258262890683122, 1.000000000000000000, 0.9659258262890683122, 1.000000000000000000, 0.9659258262890683122, 1.000000000000000000, 0.9659258262890683122, 1.000000000000000000, 0.9659258262890683122, 1.000000000000000000, 0.9659258262890683122, 1.000000000000000000, 0.9659258262890683122, 1.000000000000000000, 0.9659258262890683122, 1.000000000000000000, 0.9659258262890683122, 1.000000000000000000, 0.9659258262890683122, 1.000000000000000000, 0.9659258262890683122, 1.000000000000000000, 0.9659258262890683122, 1.000000000000000000, 0.9659258262890683122, 1.000000000000000000, 0.9659258262890683122, 1.000000000000000000, 0.9659258262890683122, 1.000000000000000000, 0.9659258262890683122, 1.000000000000000000, 0.9659258262890683122, 1.000000000000000000, 0.9659258262890683122, 1.000000000000000000, 0.9659258262890683122, 1.000000000000000000, 0.9659258262890683122, 1.000000000000000000, 0.9659258262890683122, 1.000000000000000000, 0.9659258262890683122, 1.000000000000000000, 0.9659258262890683122, 1.000000000000000000, 0.9659258262890683122, 1.000000000000000000, 0.9659258262890683122, 1.000000000000000000, 0.9659258262890683122, 1.000000000000000000, 0.9659258262890683122, 1.000000000000000000, 0.9659258262890683122, 1.000000000000000000, 0.9659258262890683122, 1.000000000000000000, 0.9659258262890683122, 1.000000000000000000, 0.9659258262890683122, 1.000000000000000000, 0.9659258262890683122, 1.000000000000000000, 0.9659258262890683122, 1.000000000000000000, 0.9659258262890683122, 1.000000000000000000, 0.9659258262890683122, 1.000000000000000000, 0.9659258262890683122, 1.000000000000000000, 0.9659258262890683122, 1.000000000000000000, 0.9659258262890683122, 1.000000000000000000, 0.9659258262890683122, 1.000000000000000000, 0.9659258262890683122, 1.000000000000000000, 0.9659258262890683122, 1.000000000000000000, 0.9659258262890683122, 1.000000000000000000, 0.9659258262890683122, 1.000000000000000000, 0.9659258262890683122, 1.000000000000000000, 0.9659258262890683122, 1.000000000000000000),
 ( 0.3333333333333333703, 0.3219752754296894559, 0.3333333333333333703, 0.3219752754296894559, 0.3333333333333333703, 0.3219752754296894559, 0.3333333333333333703, 0.3219752754296894559, 0.3333333333333333703, 0.3219752754296894559, 0.3333333333333333703, 0.3219752754296894559, 0.3333333333333333703, 0.3219752754296894559, 0.3333333333333333703, 0.3219752754296894559, 0.3333333333333333703, 0.3219752754296894559, 0.3333333333333333703, 0.3219752754296894559, 0.3333333333333333703, 0.3219752754296894559, 0.3333333333333333703, 0.3219752754296894559, 0.3333333333333333703, 0.3219752754296894559, 0.3333333333333333703, 0.3219752754296894559, 0.3333333333333333703, 0.3219752754296894559, 0.3333333333333333703, 0.3219752754296894559, 0.3333333333333333703, 0.3219752754296894559, 0.3333333333333333703, 0.3219752754296894559, 0.3333333333333333703, 0.3219752754296894559, 0.3333333333333333703, 0.3219752754296894559, 0.3333333333333333703, 0.3219752754296894559, 0.3333333333333333703, 0.3219752754296894559, 0.3333333333333333703, 0.3219752754296894559, 0.3333333333333333703, 0.3219752754296894559, 0.3333333333333333703, 0.3219752754296894559, 0.3333333333333333703, 0.3219752754296894559, 0.3333333333333333703, 0.3219752754296894559, 0.3333333333333333703, 0.3219752754296894559, 0.3333333333333333703, 0.3219752754296894559, 0.3333333333333333703, 0.3219752754296894559, 0.3333333333333333703, 0.3219752754296894559, 0.3333333333333333703, 0.3219752754296894559, 0.3333333333333333703, 0.3219752754296894559, 0.3333333333333333703, 0.3219752754296894559, 0.3333333333333333703, 0.3219752754296894559, 0.3333333333333333703, 0.3219752754296894559, 0.3333333333333333703, 0.3219752754296894559, 0.3333333333333333703, 0.3219752754296894559, 0.3333333333333333703, 0.3219752754296894559, 0.3333333333333333703, 0.3219752754296894559, 0.3333333333333333703, 0.3219752754296894559, 0.3333333333333333703, 0.3219752754296894559, 0.3333333333333333703, 0.3219752754296894559, 0.3333333333333333703, 0.3219752754296894559, 0.3333333333333333703, 0.3219752754296894559, 0.3333333333333333703, 0.3219752754296894559, 0.3333333333333333703, 0.3219752754296894559, 0.3333333333333333703, 0.3219752754296894559, 0.3333333333333333703, 0.3219752754296894559, 0.3333333333333333703, 0.3219752754296894559, 0.3333333333333333703, 0.3219752754296894559, 0.3333333333333333703, 0.3219752754296894559, 0.3333333333333333703, 0.3219752754296894559, 0.3333333333333333703, 0.3219752754296894559, 0.3333333333333333703, 0.3219752754296894559, 0.3333333333333333703, 0.3219752754296894559, 0.3333333333333333703, 0.3219752754296894559, 0.3333333333333333703, 0.3219752754296894559, 0.3333333333333333703, 0.3219752754296894559, 0.3333333333333333703, 0.3219752754296894559, 0.3333333333333333703, 0.3219752754296894559, 0.3333333333333333703, 0.3219752754296894559, 0.3333333333333333703, 0.3219752754296894559, 0.3333333333333333703, 0.3219752754296894559, 0.3333333333333333703, 0.3219752754296894559, 0.3333333333333333703, 0.3219752754296894559, 0.3333333333333333703, 0.3219752754296894559, 0.3333333333333333703, 0.3219752754296894559, 0.3333333333333333703, 0.3219752754296894559, 0.3333333333333333703, 0.3219752754296894559, 0.3333333333333333703, 0.3219752754296894559, 0.3333333333333333703, 0.3219752754296894559, 0.3333333333333333703, 0.3219752754296894559, 0.3333333333333333703, 0.3219752754296894559, 0.3333333333333333703, 0.3219752754296894559, 0.3333333333333333703, 0.3219752754296894559, 0.3333333333333333703, 0.3219752754296894559, 0.3333333333333333703, 0.3219752754296894559, 0.3333333333333333703, 0.3219752754296894559, 0.3333333333333333703, 0.3219752754296894559, 0.3333333333333333703, 0.3219752754296894559, 0.3333333333333333703, 0.3219752754296894559, 0.3333333333333333703, 0.3219752754296894559, 0.3333333333333333703, 0.3219752754296894559, 0.3333333333333333703, 0.3219752754296894559, 0.3333333333333333703, 0.3219752754296894559, 0.3333333333333333703, 0.3219752754296894559, 0.3333333333333333703, 0.3219752754296894559, 0.3333333333333333703, 0.3219752754296894559, 0.3333333333333333703, 0.3219752754296894559, 0.3333333333333333703, 0.3219752754296894559, 0.3333333333333333703, 0.3219752754296894559, 0.3333333333333333703, 0.3219752754296894559, 0.3333333333333333703, 0.3219752754296894559, 0.3333333333333333703, 0.3219752754296894559, 0.3333333333333333703, 0.3219752754296894559, 0.3333333333333333703, 0.3219752754296894559, 0.3333333333333333703, 0.3219752754296894559, 0.3333333333333333703, 0.3219752754296894559, 0.3333333333333333703, 0.3219752754296894559, 0.3333333333333333703, 0.3219752754296894559, 0.3333333333333333703, 0.3219752754296894559, 0.3333333333333333703, 0.3219752754296894559, 0.3333333333333333703, 0.3219752754296894559, 0.3333333333333333703, 0.3219752754296894559, 0.3333333333333333703, 0.3219752754296894559, 0.3333333333333333703, 0.3219752754296894559, 0.3333333333333333703, 0.3219752754296894559, 0.3333333333333333703, 0.3219752754296894559, 0.3333333333333333703, 0.3219752754296894559, 0.3333333333333333703, 0.3219752754296894559, 0.3333333333333333703, 0.3219752754296894559, 0.3333333333333333703, 0.3219752754296894559, 0.3333333333333333703, 0.3219752754296894559, 0.3333333333333333703, 0.3219752754296894559, 0.3333333333333333703, 0.3219752754296894559, 0.3333333333333333703, 0.3219752754296894559, 0.3333333333333333703, 0.3219752754296894559, 0.3333333333333333703, 0.3219752754296894559, 0.3333333333333333703, 0.3219752754296894559, 0.3333333333333333703, 0.3219752754296894559, 0.3333333333333333703, 0.3219752754296894559, 0.3333333333333333703, 0.3219752754296894559, 0.3333333333333333703, 0.3219752754296894559, 0.3333333333333333703, 0.3219752754296894559, 0.3333333333333333703, 0.3219752754296894559, 0.3333333333333333703, 0.3219752754296894559, 0.3333333333333333703, 0.3219752754296894559, 0.3333333333333333703, 0.3219752754296894559, 0.3333333333333333703, 0.3219752754296894559, 0.3333333333333333703, 0.3219752754296894559, 0.3333333333333333703, 0.3219752754296894559, 0.3333333333333333703, 0.3219752754296894559, 0.3333333333333333703, 0.3219752754296894559, 0.3333333333333333703, 0.3219752754296894559, 0.3333333333333333703, 0.3219752754296894559, 0.3333333333333333703, 0.3219752754296894559, 0.3333333333333333703, 0.3219752754296894559, 0.3333333333333333703, 0.3219752754296894559, 0.3333333333333333703, 0.3219752754296894559, 0.3333333333333333703, 0.3219752754296894559, 0.3333333333333333703, 0.3219752754296894559, 0.3333333333333333703, 0.3219752754296894559, 0.3333333333333333703, 0.3219752754296894559, 0.3333333333333333703, 0.3219752754296894559, 0.3333333333333333703, 0.3219752754296894559, 0.3333333333333333703, 0.3219752754296894559, 0.3333333333333333703, 0.3219752754296894559, 0.3333333333333333703, 0.3219752754296894559, 0.3333333333333333703, 0.3219752754296894559, 0.3333333333333333703, 0.3219752754296894559, 0.3333333333333333703, 0.3219752754296894559, 0.3333333333333333703, 0.3219752754296894559, 0.3333333333333333703, 0.3219752754296894559, 0.3333333333333333703, 0.3219752754296894559, 0.3333333333333333703, 0.3219752754296894559, 0.3333333333333333703, 0.3219752754296894559, 0.3333333333333333703, 0.3219752754296894559, 0.3333333333333333703, 0.3219752754296894559, 0.3333333333333333703, 0.3219752754296894559, 0.3333333333333333703, 0.3219752754296894559, 0.3333333333333333703, 0.3219752754296894559, 0.3333333333333333703, 0.3219752754296894559, 0.3333333333333333703, 0.3219752754296894559, 0.3333333333333333703, 0.3219752754296894559, 0.3333333333333333703, 0.3219752754296894559, 0.3333333333333333703, 0.3219752754296894559, 0.3333333333333333703, 0.3219752754296894559, 0.3333333333333333703, 0.3219752754296894559, 0.3333333333333333703, 0.3219752754296894559, 0.3333333333333333703, 0.3219752754296894559, 0.3333333333333333703, 0.3219752754296894559, 0.3333333333333333703, 0.3219752754296894559, 0.3333333333333333703, 0.3219752754296894559, 0.3333333333333333703, 0.3219752754296894559, 0.3333333333333333703, 0.3219752754296894559, 0.3333333333333333703, 0.3219752754296894559, 0.3333333333333333703, 0.3219752754296894559, 0.3333333333333333703, 0.3219752754296894559, 0.3333333333333333703, 0.3219752754296894559, 0.3333333333333333703, 0.3219752754296894559, 0.3333333333333333703, 0.3219752754296894559, 0.3333333333333333703, 0.3219752754296894559, 0.3333333333333333703, 0.3219752754296894559, 0.3333333333333333703, 0.3219752754296894559, 0.3333333333333333703, 0.3219752754296894559, 0.3333333333333333703, 0.3219752754296894559, 0.3333333333333333703, 0.3219752754296894559, 0.3333333333333333703, 0.3219752754296894559, 0.3333333333333333703, 0.3219752754296894559, 0.3333333333333333703, 0.3219752754296894559, 0.3333333333333333703, 0.3219752754296894559, 0.3333333333333333703, 0.3219752754296894559, 0.3333333333333333703, 0.3219752754296894559, 0.3333333333333333703, 0.3219752754296894559, 0.3333333333333333703, 0.3219752754296894559, 0.3333333333333333703, 0.3219752754296894559, 0.3333333333333333703, 0.3219752754296894559, 0.3333333333333333703, 0.3219752754296894559, 0.3333333333333333703, 0.3219752754296894559, 0.3333333333333333703, 0.3219752754296894559, 0.3333333333333333703, 0.3219752754296894559, 0.3333333333333333703, 0.3219752754296894559, 0.3333333333333333703, 0.3219752754296894559, 0.3333333333333333703, 0.3219752754296894559, 0.3333333333333333703, 0.3219752754296894559, 0.3333333333333333703, 0.3219752754296894559, 0.3333333333333333703, 0.3219752754296894559, 0.3333333333333333703, 0.3219752754296894559, 0.3333333333333333703, 0.3219752754296894559, 0.3333333333333333703, 0.3219752754296894559, 0.3333333333333333703, 0.3219752754296894559, 0.3333333333333333703, 0.3219752754296894559, 0.3333333333333333703, 0.3219752754296894559, 0.3333333333333333703, 0.3219752754296894559, 0.3333333333333333703, 0.3219752754296894559, 0.3333333333333333703, 0.3219752754296894559, 0.3333333333333333703, 0.3219752754296894559, 0.3333333333333333703, 0.3219752754296894559, 0.3333333333333333703, 0.3219752754296894559, 0.3333333333333333703, 0.3219752754296894559, 0.3333333333333333703, 0.3219752754296894559, 0.3333333333333333703, 0.3219752754296894559, 0.3333333333333333703, 0.3219752754296894559, 0.3333333333333333703, 0.3219752754296894559, 0.3333333333333333703, 0.3219752754296894559, 0.3333333333333333703, 0.3219752754296894559, 0.3333333333333333703, 0.3219752754296894559, 0.3333333333333333703),
 ( 0.3333333333333333703, 0.3219752754296894559, 0.3333333333333333703, 0.3219752754296894559, 0.3333333333333333703, 0.3219752754296894559, 0.3333333333333333703, 0.3219752754296894559, 0.3333333333333333703, 0.3219752754296894559, 0.3333333333333333703, 0.3219752754296894559, 0.3333333333333333703, 0.3219752754296894559, 0.3333333333333333703, 0.3219752754296894559, 0.3333333333333333703, 0.3219752754296894559, 0.3333333333333333703, 0.3219752754296894559, 0.3333333333333333703, 0.3219752754296894559, 0.3333333333333333703, 0.3219752754296894559, 0.3333333333333333703, 0.3219752754296894559, 0.3333333333333333703, 0.3219752754296894559, 0.3333333333333333703, 0.3219752754296894559, 0.3333333333333333703, 0.3219752754296894559, 0.3333333333333333703, 0.3219752754296894559, 0.3333333333333333703, 0.3219752754296894559, 0.3333333333333333703, 0.3219752754296894559, 0.3333333333333333703, 0.3219752754296894559, 0.3333333333333333703, 0.3219752754296894559, 0.3333333333333333703, 0.3219752754296894559, 0.3333333333333333703, 0.3219752754296894559, 0.3333333333333333703, 0.3219752754296894559, 0.3333333333333333703, 0.3219752754296894559, 0.3333333333333333703, 0.3219752754296894559, 0.3333333333333333703, 0.3219752754296894559, 0.3333333333333333703, 0.3219752754296894559, 0.3333333333333333703, 0.3219752754296894559, 0.3333333333333333703, 0.3219752754296894559, 0.3333333333333333703, 0.3219752754296894559, 0.3333333333333333703, 0.3219752754296894559, 0.3333333333333333703, 0.3219752754296894559, 0.3333333333333333703, 0.3219752754296894559, 0.3333333333333333703, 0.3219752754296894559, 0.3333333333333333703, 0.3219752754296894559, 0.3333333333333333703, 0.3219752754296894559, 0.3333333333333333703, 0.3219752754296894559, 0.3333333333333333703, 0.3219752754296894559, 0.3333333333333333703, 0.3219752754296894559, 0.3333333333333333703, 0.3219752754296894559, 0.3333333333333333703, 0.3219752754296894559, 0.3333333333333333703, 0.3219752754296894559, 0.3333333333333333703, 0.3219752754296894559, 0.3333333333333333703, 0.3219752754296894559, 0.3333333333333333703, 0.3219752754296894559, 0.3333333333333333703, 0.3219752754296894559, 0.3333333333333333703, 0.3219752754296894559, 0.3333333333333333703, 0.3219752754296894559, 0.3333333333333333703, 0.3219752754296894559, 0.3333333333333333703, 0.3219752754296894559, 0.3333333333333333703, 0.3219752754296894559, 0.3333333333333333703, 0.3219752754296894559, 0.3333333333333333703, 0.3219752754296894559, 0.3333333333333333703, 0.3219752754296894559, 0.3333333333333333703, 0.3219752754296894559, 0.3333333333333333703, 0.3219752754296894559, 0.3333333333333333703, 0.3219752754296894559, 0.3333333333333333703, 0.3219752754296894559, 0.3333333333333333703, 0.3219752754296894559, 0.3333333333333333703, 0.3219752754296894559, 0.3333333333333333703, 0.3219752754296894559, 0.3333333333333333703, 0.3219752754296894559, 0.3333333333333333703, 0.3219752754296894559, 0.3333333333333333703, 0.3219752754296894559, 0.3333333333333333703, 0.3219752754296894559, 0.3333333333333333703, 0.3219752754296894559, 0.3333333333333333703, 0.3219752754296894559, 0.3333333333333333703, 0.3219752754296894559, 0.3333333333333333703, 0.3219752754296894559, 0.3333333333333333703, 0.3219752754296894559, 0.3333333333333333703, 0.3219752754296894559, 0.3333333333333333703, 0.3219752754296894559, 0.3333333333333333703, 0.3219752754296894559, 0.3333333333333333703, 0.3219752754296894559, 0.3333333333333333703, 0.3219752754296894559, 0.3333333333333333703, 0.3219752754296894559, 0.3333333333333333703, 0.3219752754296894559, 0.3333333333333333703, 0.3219752754296894559, 0.3333333333333333703, 0.3219752754296894559, 0.3333333333333333703, 0.3219752754296894559, 0.3333333333333333703, 0.3219752754296894559, 0.3333333333333333703, 0.3219752754296894559, 0.3333333333333333703, 0.3219752754296894559, 0.3333333333333333703, 0.3219752754296894559, 0.3333333333333333703, 0.3219752754296894559, 0.3333333333333333703, 0.3219752754296894559, 0.3333333333333333703, 0.3219752754296894559, 0.3333333333333333703, 0.3219752754296894559, 0.3333333333333333703, 0.3219752754296894559, 0.3333333333333333703, 0.3219752754296894559, 0.3333333333333333703, 0.3219752754296894559, 0.3333333333333333703, 0.3219752754296894559, 0.3333333333333333703, 0.3219752754296894559, 0.3333333333333333703, 0.3219752754296894559, 0.3333333333333333703, 0.3219752754296894559, 0.3333333333333333703, 0.3219752754296894559, 0.3333333333333333703, 0.3219752754296894559, 0.3333333333333333703, 0.3219752754296894559, 0.3333333333333333703, 0.3219752754296894559, 0.3333333333333333703, 0.3219752754296894559, 0.3333333333333333703, 0.3219752754296894559, 0.3333333333333333703, 0.3219752754296894559, 0.3333333333333333703, 0.3219752754296894559, 0.3333333333333333703, 0.3219752754296894559, 0.3333333333333333703, 0.3219752754296894559, 0.3333333333333333703, 0.3219752754296894559, 0.3333333333333333703, 0.3219752754296894559, 0.3333333333333333703, 0.3219752754296894559, 0.3333333333333333703, 0.3219752754296894559, 0.3333333333333333703, 0.3219752754296894559, 0.3333333333333333703, 0.3219752754296894559, 0.3333333333333333703, 0.3219752754296894559, 0.3333333333333333703, 0.3219752754296894559, 0.3333333333333333703, 0.3219752754296894559, 0.3333333333333333703, 0.3219752754296894559, 0.3333333333333333703, 0.3219752754296894559, 0.3333333333333333703, 0.3219752754296894559, 0.3333333333333333703, 0.3219752754296894559, 0.3333333333333333703, 0.3219752754296894559, 0.3333333333333333703, 0.3219752754296894559, 0.3333333333333333703, 0.3219752754296894559, 0.3333333333333333703, 0.3219752754296894559, 0.3333333333333333703, 0.3219752754296894559, 0.3333333333333333703, 0.3219752754296894559, 0.3333333333333333703, 0.3219752754296894559, 0.3333333333333333703, 0.3219752754296894559, 0.3333333333333333703, 0.3219752754296894559, 0.3333333333333333703, 0.3219752754296894559, 0.3333333333333333703, 0.3219752754296894559, 0.3333333333333333703, 0.3219752754296894559, 0.3333333333333333703, 0.3219752754296894559, 0.3333333333333333703, 0.3219752754296894559, 0.3333333333333333703, 0.3219752754296894559, 0.3333333333333333703, 0.3219752754296894559, 0.3333333333333333703, 0.3219752754296894559, 0.3333333333333333703, 0.3219752754296894559, 0.3333333333333333703, 0.3219752754296894559, 0.3333333333333333703, 0.3219752754296894559, 0.3333333333333333703, 0.3219752754296894559, 0.3333333333333333703, 0.3219752754296894559, 0.3333333333333333703, 0.3219752754296894559, 0.3333333333333333703, 0.3219752754296894559, 0.3333333333333333703, 0.3219752754296894559, 0.3333333333333333703, 0.3219752754296894559, 0.3333333333333333703, 0.3219752754296894559, 0.3333333333333333703, 0.3219752754296894559, 0.3333333333333333703, 0.3219752754296894559, 0.3333333333333333703, 0.3219752754296894559, 0.3333333333333333703, 0.3219752754296894559, 0.3333333333333333703, 0.3219752754296894559, 0.3333333333333333703, 0.3219752754296894559, 0.3333333333333333703, 0.3219752754296894559, 0.3333333333333333703, 0.3219752754296894559, 0.3333333333333333703, 0.3219752754296894559, 0.3333333333333333703, 0.3219752754296894559, 0.3333333333333333703, 0.3219752754296894559, 0.3333333333333333703, 0.3219752754296894559, 0.3333333333333333703, 0.3219752754296894559, 0.3333333333333333703, 0.3219752754296894559, 0.3333333333333333703, 0.3219752754296894559, 0.3333333333333333703, 0.3219752754296894559, 0.3333333333333333703, 0.3219752754296894559, 0.3333333333333333703, 0.3219752754296894559, 0.3333333333333333703, 0.3219752754296894559, 0.3333333333333333703, 0.3219752754296894559, 0.3333333333333333703, 0.3219752754296894559, 0.3333333333333333703, 0.3219752754296894559, 0.3333333333333333703, 0.3219752754296894559, 0.3333333333333333703, 0.3219752754296894559, 0.3333333333333333703, 0.3219752754296894559, 0.3333333333333333703, 0.3219752754296894559, 0.3333333333333333703, 0.3219752754296894559, 0.3333333333333333703, 0.3219752754296894559, 0.3333333333333333703, 0.3219752754296894559, 0.3333333333333333703, 0.3219752754296894559, 0.3333333333333333703, 0.3219752754296894559, 0.3333333333333333703, 0.3219752754296894559, 0.3333333333333333703, 0.3219752754296894559, 0.3333333333333333703, 0.3219752754296894559, 0.3333333333333333703, 0.3219752754296894559, 0.3333333333333333703, 0.3219752754296894559, 0.3333333333333333703, 0.3219752754296894559, 0.3333333333333333703, 0.3219752754296894559, 0.3333333333333333703, 0.3219752754296894559, 0.3333333333333333703, 0.3219752754296894559, 0.3333333333333333703, 0.3219752754296894559, 0.3333333333333333703, 0.3219752754296894559, 0.3333333333333333703, 0.3219752754296894559, 0.3333333333333333703, 0.3219752754296894559, 0.3333333333333333703, 0.3219752754296894559, 0.3333333333333333703, 0.3219752754296894559, 0.3333333333333333703, 0.3219752754296894559, 0.3333333333333333703, 0.3219752754296894559, 0.3333333333333333703, 0.3219752754296894559, 0.3333333333333333703, 0.3219752754296894559, 0.3333333333333333703, 0.3219752754296894559, 0.3333333333333333703, 0.3219752754296894559, 0.3333333333333333703, 0.3219752754296894559, 0.3333333333333333703, 0.3219752754296894559, 0.3333333333333333703, 0.3219752754296894559, 0.3333333333333333703, 0.3219752754296894559, 0.3333333333333333703, 0.3219752754296894559, 0.3333333333333333703, 0.3219752754296894559, 0.3333333333333333703, 0.3219752754296894559, 0.3333333333333333703, 0.3219752754296894559, 0.3333333333333333703, 0.3219752754296894559, 0.3333333333333333703, 0.3219752754296894559, 0.3333333333333333703, 0.3219752754296894559, 0.3333333333333333703, 0.3219752754296894559, 0.3333333333333333703, 0.3219752754296894559, 0.3333333333333333703, 0.3219752754296894559, 0.3333333333333333703, 0.3219752754296894559, 0.3333333333333333703, 0.3219752754296894559, 0.3333333333333333703, 0.3219752754296894559, 0.3333333333333333703, 0.3219752754296894559, 0.3333333333333333703, 0.3219752754296894559, 0.3333333333333333703, 0.3219752754296894559, 0.3333333333333333703, 0.3219752754296894559, 0.3333333333333333703, 0.3219752754296894559, 0.3333333333333333703, 0.3219752754296894559, 0.3333333333333333703, 0.3219752754296894559, 0.3333333333333333703, 0.3219752754296894559, 0.3333333333333333703, 0.3219752754296894559, 0.3333333333333333703, 0.3219752754296894559, 0.3333333333333333703, 0.3219752754296894559, 0.3333333333333333703, 0.3219752754296894559, 0.3333333333333333703, 0.3219752754296894559, 0.3333333333333333703),
 ( 1.000000000000000000, 0.9659258262890683122, 1.000000000000000000, 0.9659258262890683122, 1.000000000000000000, 0.9659258262890683122, 1.000000000000000000, 0.9659258262890683122, 1.000000000000000000, 0.9659258262890683122, 1.000000000000000000, 0.9659258262890683122, 1.000000000000000000, 0.9659258262890683122, 1.000000000000000000, 0.9659258262890683122, 1.000000000000000000, 0.9659258262890683122, 1.000000000000000000, 0.9659258262890683122, 1.000000000000000000, 0.9659258262890683122, 1.000000000000000000, 0.9659258262890683122, 1.000000000000000000, 0.9659258262890683122, 1.000000000000000000, 0.9659258262890683122, 1.000000000000000000, 0.9659258262890683122, 1.000000000000000000, 0.9659258262890683122, 1.000000000000000000, 0.9659258262890683122, 1.000000000000000000, 0.9659258262890683122, 1.000000000000000000, 0.9659258262890683122, 1.000000000000000000, 0.9659258262890683122, 1.000000000000000000, 0.9659258262890683122, 1.000000000000000000, 0.9659258262890683122, 1.000000000000000000, 0.9659258262890683122, 1.000000000000000000, 0.9659258262890683122, 1.000000000000000000, 0.9659258262890683122, 1.000000000000000000, 0.9659258262890683122, 1.000000000000000000, 0.9659258262890683122, 1.000000000000000000, 0.9659258262890683122, 1.000000000000000000, 0.9659258262890683122, 1.000000000000000000, 0.9659258262890683122, 1.000000000000000000, 0.9659258262890683122, 1.000000000000000000, 0.9659258262890683122, 1.000000000000000000, 0.9659258262890683122, 1.000000000000000000, 0.9659258262890683122, 1.000000000000000000, 0.9659258262890683122, 1.000000000000000000, 0.9659258262890683122, 1.000000000000000000, 0.9659258262890683122, 1.000000000000000000, 0.9659258262890683122, 1.000000000000000000, 0.9659258262890683122, 1.000000000000000000, 0.9659258262890683122, 1.000000000000000000, 0.9659258262890683122, 1.000000000000000000, 0.9659258262890683122, 1.000000000000000000, 0.9659258262890683122, 1.000000000000000000, 0.9659258262890683122, 1.000000000000000000, 0.9659258262890683122, 1.000000000000000000, 0.9659258262890683122, 1.000000000000000000, 0.9659258262890683122, 1.000000000000000000, 0.9659258262890683122, 1.000000000000000000, 0.9659258262890683122, 1.000000000000000000, 0.9659258262890683122, 1.000000000000000000, 0.9659258262890683122, 1.000000000000000000, 0.9659258262890683122, 1.000000000000000000, 0.9659258262890683122, 1.000000000000000000, 0.9659258262890683122, 1.000000000000000000, 0.9659258262890683122, 1.000000000000000000, 0.9659258262890683122, 1.000000000000000000, 0.9659258262890683122, 1.000000000000000000, 0.9659258262890683122, 1.000000000000000000, 0.9659258262890683122, 1.000000000000000000, 0.9659258262890683122, 1.000000000000000000, 0.9659258262890683122, 1.000000000000000000, 0.9659258262890683122, 1.000000000000000000, 0.9659258262890683122, 1.000000000000000000, 0.9659258262890683122, 1.000000000000000000, 0.9659258262890683122, 1.000000000000000000, 0.9659258262890683122, 1.000000000000000000, 0.9659258262890683122, 1.000000000000000000, 0.9659258262890683122, 1.000000000000000000, 0.9659258262890683122, 1.000000000000000000, 0.9659258262890683122, 1.000000000000000000, 0.9659258262890683122, 1.000000000000000000, 0.9659258262890683122, 1.000000000000000000, 0.9659258262890683122, 1.000000000000000000, 0.9659258262890683122, 1.000000000000000000, 0.9659258262890683122, 1.000000000000000000, 0.9659258262890683122, 1.000000000000000000, 0.9659258262890683122, 1.000000000000000000, 0.9659258262890683122, 1.000000000000000000, 0.9659258262890683122, 1.000000000000000000, 0.9659258262890683122, 1.000000000000000000, 0.9659258262890683122, 1.000000000000000000, 0.9659258262890683122, 1.000000000000000000, 0.9659258262890683122, 1.000000000000000000, 0.9659258262890683122, 1.000000000000000000, 0.9659258262890683122, 1.000000000000000000, 0.9659258262890683122, 1.000000000000000000, 0.9659258262890683122, 1.000000000000000000, 0.9659258262890683122, 1.000000000000000000, 0.9659258262890683122, 1.000000000000000000, 0.9659258262890683122, 1.000000000000000000, 0.9659258262890683122, 1.000000000000000000, 0.9659258262890683122, 1.000000000000000000, 0.9659258262890683122, 1.000000000000000000, 0.9659258262890683122, 1.000000000000000000, 0.9659258262890683122, 1.000000000000000000, 0.9659258262890683122, 1.000000000000000000, 0.9659258262890683122, 1.000000000000000000, 0.9659258262890683122, 1.000000000000000000, 0.9659258262890683122, 1.000000000000000000, 0.9659258262890683122, 1.000000000000000000, 0.9659258262890683122, 1.000000000000000000, 0.9659258262890683122, 1.000000000000000000, 0.9659258262890683122, 1.000000000000000000, 0.9659258262890683122, 1.000000000000000000, 0.9659258262890683122, 1.000000000000000000, 0.9659258262890683122, 1.000000000000000000, 0.9659258262890683122, 1.000000000000000000, 0.9659258262890683122, 1.000000000000000000, 0.9659258262890683122, 1.000000000000000000, 0.9659258262890683122, 1.000000000000000000, 0.9659258262890683122, 1.000000000000000000, 0.9659258262890683122, 1.000000000000000000, 0.9659258262890683122, 1.000000000000000000, 0.9659258262890683122, 1.000000000000000000, 0.9659258262890683122, 1.000000000000000000, 0.9659258262890683122, 1.000000000000000000, 0.9659258262890683122, 1.000000000000000000, 0.9659258262890683122, 1.000000000000000000, 0.9659258262890683122, 1.000000000000000000, 0.9659258262890683122, 1.000000000000000000, 0.9659258262890683122, 1.000000000000000000, 0.9659258262890683122, 1.000000000000000000, 0.9659258262890683122, 1.000000000000000000, 0.9659258262890683122, 1.000000000000000000, 0.9659258262890683122, 1.000000000000000000, 0.9659258262890683122, 1.000000000000000000, 0.9659258262890683122, 1.000000000000000000, 0.9659258262890683122, 1.000000000000000000, 0.9659258262890683122, 1.000000000000000000, 0.9659258262890683122, 1.000000000000000000, 0.9659258262890683122, 1.000000000000000000, 0.9659258262890683122, 1.000000000000000000, 0.9659258262890683122, 1.000000000000000000, 0.9659258262890683122, 1.000000000000000000, 0.9659258262890683122, 1.000000000000000000, 0.9659258262890683122, 1.000000000000000000, 0.9659258262890683122, 1.000000000000000000, 0.9659258262890683122, 1.000000000000000000, 0.9659258262890683122, 1.000000000000000000, 0.9659258262890683122, 1.000000000000000000, 0.9659258262890683122, 1.000000000000000000, 0.9659258262890683122, 1.000000000000000000, 0.9659258262890683122, 1.000000000000000000, 0.9659258262890683122, 1.000000000000000000, 0.9659258262890683122, 1.000000000000000000, 0.9659258262890683122, 1.000000000000000000, 0.9659258262890683122, 1.000000000000000000, 0.9659258262890683122, 1.000000000000000000, 0.9659258262890683122, 1.000000000000000000, 0.9659258262890683122, 1.000000000000000000, 0.9659258262890683122, 1.000000000000000000, 0.9659258262890683122, 1.000000000000000000, 0.9659258262890683122, 1.000000000000000000, 0.9659258262890683122, 1.000000000000000000, 0.9659258262890683122, 1.000000000000000000, 0.9659258262890683122, 1.000000000000000000, 0.9659258262890683122, 1.000000000000000000, 0.9659258262890683122, 1.000000000000000000, 0.9659258262890683122, 1.000000000000000000, 0.9659258262890683122, 1.000000000000000000, 0.9659258262890683122, 1.000000000000000000, 0.9659258262890683122, 1.000000000000000000, 0.9659258262890683122, 1.000000000000000000, 0.9659258262890683122, 1.000000000000000000, 0.9659258262890683122, 1.000000000000000000, 0.9659258262890683122, 1.000000000000000000, 0.9659258262890683122, 1.000000000000000000, 0.9659258262890683122, 1.000000000000000000, 0.9659258262890683122, 1.000000000000000000, 0.9659258262890683122, 1.000000000000000000, 0.9659258262890683122, 1.000000000000000000, 0.9659258262890683122, 1.000000000000000000, 0.9659258262890683122, 1.000000000000000000, 0.9659258262890683122, 1.000000000000000000, 0.9659258262890683122, 1.000000000000000000, 0.9659258262890683122, 1.000000000000000000, 0.9659258262890683122, 1.000000000000000000, 0.9659258262890683122, 1.000000000000000000, 0.9659258262890683122, 1.000000000000000000, 0.9659258262890683122, 1.000000000000000000, 0.9659258262890683122, 1.000000000000000000, 0.9659258262890683122, 1.000000000000000000, 0.9659258262890683122, 1.000000000000000000, 0.9659258262890683122, 1.000000000000000000, 0.9659258262890683122, 1.000000000000000000, 0.9659258262890683122, 1.000000000000000000, 0.9659258262890683122, 1.000000000000000000, 0.9659258262890683122, 1.000000000000000000, 0.9659258262890683122, 1.000000000000000000, 0.9659258262890683122, 1.000000000000000000, 0.9659258262890683122, 1.000000000000000000, 0.9659258262890683122, 1.000000000000000000, 0.9659258262890683122, 1.000000000000000000, 0.9659258262890683122, 1.000000000000000000, 0.9659258262890683122, 1.000000000000000000, 0.9659258262890683122, 1.000000000000000000, 0.9659258262890683122, 1.000000000000000000, 0.9659258262890683122, 1.000000000000000000, 0.9659258262890683122, 1.000000000000000000, 0.9659258262890683122, 1.000000000000000000, 0.9659258262890683122, 1.000000000000000000, 0.9659258262890683122, 1.000000000000000000, 0.9659258262890683122, 1.000000000000000000, 0.9659258262890683122, 1.000000000000000000, 0.9659258262890683122, 1.000000000000000000, 0.9659258262890683122, 1.000000000000000000, 0.9659258262890683122, 1.000000000000000000, 0.9659258262890683122, 1.000000000000000000, 0.9659258262890683122, 1.000000000000000000, 0.9659258262890683122, 1.000000000000000000, 0.9659258262890683122, 1.000000000000000000, 0.9659258262890683122, 1.000000000000000000, 0.9659258262890683122, 1.000000000000000000, 0.9659258262890683122, 1.000000000000000000, 0.9659258262890683122, 1.000000000000000000, 0.9659258262890683122, 1.000000000000000000, 0.9659258262890683122, 1.000000000000000000, 0.9659258262890683122, 1.000000000000000000, 0.9659258262890683122, 1.000000000000000000, 0.9659258262890683122, 1.000000000000000000, 0.9659258262890683122, 1.000000000000000000, 0.9659258262890683122, 1.000000000000000000, 0.9659258262890683122, 1.000000000000000000, 0.9659258262890683122, 1.000000000000000000, 0.9659258262890683122, 1.000000000000000000, 0.9659258262890683122, 1.000000000000000000, 0.9659258262890683122, 1.000000000000000000, 0.9659258262890683122, 1.000000000000000000),
 ( 0.3333333333333333703, 0.3219752754296894559, 0.3333333333333333703, 0.3219752754296894559, 0.3333333333333333703, 0.3219752754296894559, 0.3333333333333333703, 0.3219752754296894559, 0.3333333333333333703, 0.3219752754296894559, 0.3333333333333333703, 0.3219752754296894559, 0.3333333333333333703, 0.3219752754296894559, 0.3333333333333333703, 0.3219752754296894559, 0.3333333333333333703, 0.3219752754296894559, 0.3333333333333333703, 0.3219752754296894559, 0.3333333333333333703, 0.3219752754296894559, 0.3333333333333333703, 0.3219752754296894559, 0.3333333333333333703, 0.3219752754296894559, 0.3333333333333333703, 0.3219752754296894559, 0.3333333333333333703, 0.3219752754296894559, 0.3333333333333333703, 0.3219752754296894559, 0.3333333333333333703, 0.3219752754296894559, 0.3333333333333333703, 0.3219752754296894559, 0.3333333333333333703, 0.3219752754296894559, 0.3333333333333333703, 0.3219752754296894559, 0.3333333333333333703, 0.3219752754296894559, 0.3333333333333333703, 0.3219752754296894559, 0.3333333333333333703, 0.3219752754296894559, 0.3333333333333333703, 0.3219752754296894559, 0.3333333333333333703, 0.3219752754296894559, 0.3333333333333333703, 0.3219752754296894559, 0.3333333333333333703, 0.3219752754296894559, 0.3333333333333333703, 0.3219752754296894559, 0.3333333333333333703, 0.3219752754296894559, 0.3333333333333333703, 0.3219752754296894559, 0.3333333333333333703, 0.3219752754296894559, 0.3333333333333333703, 0.3219752754296894559, 0.3333333333333333703, 0.3219752754296894559, 0.3333333333333333703, 0.3219752754296894559, 0.3333333333333333703, 0.3219752754296894559, 0.3333333333333333703, 0.3219752754296894559, 0.3333333333333333703, 0.3219752754296894559, 0.3333333333333333703, 0.3219752754296894559, 0.3333333333333333703, 0.3219752754296894559, 0.3333333333333333703, 0.3219752754296894559, 0.3333333333333333703, 0.3219752754296894559, 0.3333333333333333703, 0.3219752754296894559, 0.3333333333333333703, 0.3219752754296894559, 0.3333333333333333703, 0.3219752754296894559, 0.3333333333333333703, 0.3219752754296894559, 0.3333333333333333703, 0.3219752754296894559, 0.3333333333333333703, 0.3219752754296894559, 0.3333333333333333703, 0.3219752754296894559, 0.3333333333333333703, 0.3219752754296894559, 0.3333333333333333703, 0.3219752754296894559, 0.3333333333333333703, 0.3219752754296894559, 0.3333333333333333703, 0.3219752754296894559, 0.3333333333333333703, 0.3219752754296894559, 0.3333333333333333703, 0.3219752754296894559, 0.3333333333333333703, 0.3219752754296894559, 0.3333333333333333703, 0.3219752754296894559, 0.3333333333333333703, 0.3219752754296894559, 0.3333333333333333703, 0.3219752754296894559, 0.3333333333333333703, 0.3219752754296894559, 0.3333333333333333703, 0.3219752754296894559, 0.3333333333333333703, 0.3219752754296894559, 0.3333333333333333703, 0.3219752754296894559, 0.3333333333333333703, 0.3219752754296894559, 0.3333333333333333703, 0.3219752754296894559, 0.3333333333333333703, 0.3219752754296894559, 0.3333333333333333703, 0.3219752754296894559, 0.3333333333333333703, 0.3219752754296894559, 0.3333333333333333703, 0.3219752754296894559, 0.3333333333333333703, 0.3219752754296894559, 0.3333333333333333703, 0.3219752754296894559, 0.3333333333333333703, 0.3219752754296894559, 0.3333333333333333703, 0.3219752754296894559, 0.3333333333333333703, 0.3219752754296894559, 0.3333333333333333703, 0.3219752754296894559, 0.3333333333333333703, 0.3219752754296894559, 0.3333333333333333703, 0.3219752754296894559, 0.3333333333333333703, 0.3219752754296894559, 0.3333333333333333703, 0.3219752754296894559, 0.3333333333333333703, 0.3219752754296894559, 0.3333333333333333703, 0.3219752754296894559, 0.3333333333333333703, 0.3219752754296894559, 0.3333333333333333703, 0.3219752754296894559, 0.3333333333333333703, 0.3219752754296894559, 0.3333333333333333703, 0.3219752754296894559, 0.3333333333333333703, 0.3219752754296894559, 0.3333333333333333703, 0.3219752754296894559, 0.3333333333333333703, 0.3219752754296894559, 0.3333333333333333703, 0.3219752754296894559, 0.3333333333333333703, 0.3219752754296894559, 0.3333333333333333703, 0.3219752754296894559, 0.3333333333333333703, 0.3219752754296894559, 0.3333333333333333703, 0.3219752754296894559, 0.3333333333333333703, 0.3219752754296894559, 0.3333333333333333703, 0.3219752754296894559, 0.3333333333333333703, 0.3219752754296894559, 0.3333333333333333703, 0.3219752754296894559, 0.3333333333333333703, 0.3219752754296894559, 0.3333333333333333703, 0.3219752754296894559, 0.3333333333333333703, 0.3219752754296894559, 0.3333333333333333703, 0.3219752754296894559, 0.3333333333333333703, 0.3219752754296894559, 0.3333333333333333703, 0.3219752754296894559, 0.3333333333333333703, 0.3219752754296894559, 0.3333333333333333703, 0.3219752754296894559, 0.3333333333333333703, 0.3219752754296894559, 0.3333333333333333703, 0.3219752754296894559, 0.3333333333333333703, 0.3219752754296894559, 0.3333333333333333703, 0.3219752754296894559, 0.3333333333333333703, 0.3219752754296894559, 0.3333333333333333703, 0.3219752754296894559, 0.3333333333333333703, 0.3219752754296894559, 0.3333333333333333703, 0.3219752754296894559, 0.3333333333333333703, 0.3219752754296894559, 0.3333333333333333703, 0.3219752754296894559, 0.3333333333333333703, 0.3219752754296894559, 0.3333333333333333703, 0.3219752754296894559, 0.3333333333333333703, 0.3219752754296894559, 0.3333333333333333703, 0.3219752754296894559, 0.3333333333333333703, 0.3219752754296894559, 0.3333333333333333703, 0.3219752754296894559, 0.3333333333333333703, 0.3219752754296894559, 0.3333333333333333703, 0.3219752754296894559, 0.3333333333333333703, 0.3219752754296894559, 0.3333333333333333703, 0.3219752754296894559, 0.3333333333333333703, 0.3219752754296894559, 0.3333333333333333703, 0.3219752754296894559, 0.3333333333333333703, 0.3219752754296894559, 0.3333333333333333703, 0.3219752754296894559, 0.3333333333333333703, 0.3219752754296894559, 0.3333333333333333703, 0.3219752754296894559, 0.3333333333333333703, 0.3219752754296894559, 0.3333333333333333703, 0.3219752754296894559, 0.3333333333333333703, 0.3219752754296894559, 0.3333333333333333703, 0.3219752754296894559, 0.3333333333333333703, 0.3219752754296894559, 0.3333333333333333703, 0.3219752754296894559, 0.3333333333333333703, 0.3219752754296894559, 0.3333333333333333703, 0.3219752754296894559, 0.3333333333333333703, 0.3219752754296894559, 0.3333333333333333703, 0.3219752754296894559, 0.3333333333333333703, 0.3219752754296894559, 0.3333333333333333703, 0.3219752754296894559, 0.3333333333333333703, 0.3219752754296894559, 0.3333333333333333703, 0.3219752754296894559, 0.3333333333333333703, 0.3219752754296894559, 0.3333333333333333703, 0.3219752754296894559, 0.3333333333333333703, 0.3219752754296894559, 0.3333333333333333703, 0.3219752754296894559, 0.3333333333333333703, 0.3219752754296894559, 0.3333333333333333703, 0.3219752754296894559, 0.3333333333333333703, 0.3219752754296894559, 0.3333333333333333703, 0.3219752754296894559, 0.3333333333333333703, 0.3219752754296894559, 0.3333333333333333703, 0.3219752754296894559, 0.3333333333333333703, 0.3219752754296894559, 0.3333333333333333703, 0.3219752754296894559, 0.3333333333333333703, 0.3219752754296894559, 0.3333333333333333703, 0.3219752754296894559, 0.3333333333333333703, 0.3219752754296894559, 0.3333333333333333703, 0.3219752754296894559, 0.3333333333333333703, 0.3219752754296894559, 0.3333333333333333703, 0.3219752754296894559, 0.3333333333333333703, 0.3219752754296894559, 0.3333333333333333703, 0.3219752754296894559, 0.3333333333333333703, 0.3219752754296894559, 0.3333333333333333703, 0.3219752754296894559, 0.3333333333333333703, 0.3219752754296894559, 0.3333333333333333703, 0.3219752754296894559, 0.3333333333333333703, 0.3219752754296894559, 0.3333333333333333703, 0.3219752754296894559, 0.3333333333333333703, 0.3219752754296894559, 0.3333333333333333703, 0.3219752754296894559, 0.3333333333333333703, 0.3219752754296894559, 0.3333333333333333703, 0.3219752754296894559, 0.3333333333333333703, 0.3219752754296894559, 0.3333333333333333703, 0.3219752754296894559, 0.3333333333333333703, 0.3219752754296894559, 0.3333333333333333703, 0.3219752754296894559, 0.3333333333333333703, 0.3219752754296894559, 0.3333333333333333703, 0.3219752754296894559, 0.3333333333333333703, 0.3219752754296894559, 0.3333333333333333703, 0.3219752754296894559, 0.3333333333333333703, 0.3219752754296894559, 0.3333333333333333703, 0.3219752754296894559, 0.3333333333333333703, 0.3219752754296894559, 0.3333333333333333703, 0.3219752754296894559, 0.3333333333333333703, 0.3219752754296894559, 0.3333333333333333703, 0.3219752754296894559, 0.3333333333333333703, 0.3219752754296894559, 0.3333333333333333703, 0.3219752754296894559, 0.3333333333333333703, 0.3219752754296894559, 0.3333333333333333703, 0.3219752754296894559, 0.3333333333333333703, 0.3219752754296894559, 0.3333333333333333703, 0.3219752754296894559, 0.3333333333333333703, 0.3219752754296894559, 0.3333333333333333703, 0.3219752754296894559, 0.3333333333333333703, 0.3219752754296894559, 0.3333333333333333703, 0.3219752754296894559, 0.3333333333333333703, 0.3219752754296894559, 0.3333333333333333703, 0.3219752754296894559, 0.3333333333333333703, 0.3219752754296894559, 0.3333333333333333703, 0.3219752754296894559, 0.3333333333333333703, 0.3219752754296894559, 0.3333333333333333703, 0.3219752754296894559, 0.3333333333333333703, 0.3219752754296894559, 0.3333333333333333703, 0.3219752754296894559, 0.3333333333333333703, 0.3219752754296894559, 0.3333333333333333703, 0.3219752754296894559, 0.3333333333333333703, 0.3219752754296894559, 0.3333333333333333703, 0.3219752754296894559, 0.3333333333333333703, 0.3219752754296894559, 0.3333333333333333703, 0.3219752754296894559, 0.3333333333333333703, 0.3219752754296894559, 0.3333333333333333703, 0.3219752754296894559, 0.3333333333333333703, 0.3219752754296894559, 0.3333333333333333703, 0.3219752754296894559, 0.3333333333333333703, 0.3219752754296894559, 0.3333333333333333703, 0.3219752754296894559, 0.3333333333333333703, 0.3219752754296894559, 0.3333333333333333703, 0.3219752754296894559, 0.3333333333333333703, 0.3219752754296894559, 0.3333333333333333703, 0.3219752754296894559, 0.3333333333333333703, 0.3219752754296894559, 0.3333333333333333703, 0.3219752754296894559, 0.3333333333333333703, 0.3219752754296894559, 0.3333333333333333703, 0.3219752754296894559, 0.3333333333333333703, 0.3219752754296894559, 0.3333333333333333703, 0.3219752754296894559, 0.3333333333333333703),
 ( 0.3333333333333333703, 0.3219752754296894559, 0.3333333333333333703, 0.3219752754296894559, 0.3333333333333333703, 0.3219752754296894559, 0.3333333333333333703, 0.3219752754296894559, 0.3333333333333333703, 0.3219752754296894559, 0.3333333333333333703, 0.3219752754296894559, 0.3333333333333333703, 0.3219752754296894559, 0.3333333333333333703, 0.3219752754296894559, 0.3333333333333333703, 0.3219752754296894559, 0.3333333333333333703, 0.3219752754296894559, 0.3333333333333333703, 0.3219752754296894559, 0.3333333333333333703, 0.3219752754296894559, 0.3333333333333333703, 0.3219752754296894559, 0.3333333333333333703, 0.3219752754296894559, 0.3333333333333333703, 0.3219752754296894559, 0.3333333333333333703, 0.3219752754296894559, 0.3333333333333333703, 0.3219752754296894559, 0.3333333333333333703, 0.3219752754296894559, 0.3333333333333333703, 0.3219752754296894559, 0.3333333333333333703, 0.3219752754296894559, 0.3333333333333333703, 0.3219752754296894559, 0.3333333333333333703, 0.3219752754296894559, 0.3333333333333333703, 0.3219752754296894559, 0.3333333333333333703, 0.3219752754296894559, 0.3333333333333333703, 0.3219752754296894559, 0.3333333333333333703, 0.3219752754296894559, 0.3333333333333333703, 0.3219752754296894559, 0.3333333333333333703, 0.3219752754296894559, 0.3333333333333333703, 0.3219752754296894559, 0.3333333333333333703, 0.3219752754296894559, 0.3333333333333333703, 0.3219752754296894559, 0.3333333333333333703, 0.3219752754296894559, 0.3333333333333333703, 0.3219752754296894559, 0.3333333333333333703, 0.3219752754296894559, 0.3333333333333333703, 0.3219752754296894559, 0.3333333333333333703, 0.3219752754296894559, 0.3333333333333333703, 0.3219752754296894559, 0.3333333333333333703, 0.3219752754296894559, 0.3333333333333333703, 0.3219752754296894559, 0.3333333333333333703, 0.3219752754296894559, 0.3333333333333333703, 0.3219752754296894559, 0.3333333333333333703, 0.3219752754296894559, 0.3333333333333333703, 0.3219752754296894559, 0.3333333333333333703, 0.3219752754296894559, 0.3333333333333333703, 0.3219752754296894559, 0.3333333333333333703, 0.3219752754296894559, 0.3333333333333333703, 0.3219752754296894559, 0.3333333333333333703, 0.3219752754296894559, 0.3333333333333333703, 0.3219752754296894559, 0.3333333333333333703, 0.3219752754296894559, 0.3333333333333333703, 0.3219752754296894559, 0.3333333333333333703, 0.3219752754296894559, 0.3333333333333333703, 0.3219752754296894559, 0.3333333333333333703, 0.3219752754296894559, 0.3333333333333333703, 0.3219752754296894559, 0.3333333333333333703, 0.3219752754296894559, 0.3333333333333333703, 0.3219752754296894559, 0.3333333333333333703, 0.3219752754296894559, 0.3333333333333333703, 0.3219752754296894559, 0.3333333333333333703, 0.3219752754296894559, 0.3333333333333333703, 0.3219752754296894559, 0.3333333333333333703, 0.3219752754296894559, 0.3333333333333333703, 0.3219752754296894559, 0.3333333333333333703, 0.3219752754296894559, 0.3333333333333333703, 0.3219752754296894559, 0.3333333333333333703, 0.3219752754296894559, 0.3333333333333333703, 0.3219752754296894559, 0.3333333333333333703, 0.3219752754296894559, 0.3333333333333333703, 0.3219752754296894559, 0.3333333333333333703, 0.3219752754296894559, 0.3333333333333333703, 0.3219752754296894559, 0.3333333333333333703, 0.3219752754296894559, 0.3333333333333333703, 0.3219752754296894559, 0.3333333333333333703, 0.3219752754296894559, 0.3333333333333333703, 0.3219752754296894559, 0.3333333333333333703, 0.3219752754296894559, 0.3333333333333333703, 0.3219752754296894559, 0.3333333333333333703, 0.3219752754296894559, 0.3333333333333333703, 0.3219752754296894559, 0.3333333333333333703, 0.3219752754296894559, 0.3333333333333333703, 0.3219752754296894559, 0.3333333333333333703, 0.3219752754296894559, 0.3333333333333333703, 0.3219752754296894559, 0.3333333333333333703, 0.3219752754296894559, 0.3333333333333333703, 0.3219752754296894559, 0.3333333333333333703, 0.3219752754296894559, 0.3333333333333333703, 0.3219752754296894559, 0.3333333333333333703, 0.3219752754296894559, 0.3333333333333333703, 0.3219752754296894559, 0.3333333333333333703, 0.3219752754296894559, 0.3333333333333333703, 0.3219752754296894559, 0.3333333333333333703, 0.3219752754296894559, 0.3333333333333333703, 0.3219752754296894559, 0.3333333333333333703, 0.3219752754296894559, 0.3333333333333333703, 0.3219752754296894559, 0.3333333333333333703, 0.3219752754296894559, 0.3333333333333333703, 0.3219752754296894559, 0.3333333333333333703, 0.3219752754296894559, 0.3333333333333333703, 0.3219752754296894559, 0.3333333333333333703, 0.3219752754296894559, 0.3333333333333333703, 0.3219752754296894559, 0.3333333333333333703, 0.3219752754296894559, 0.3333333333333333703, 0.3219752754296894559, 0.3333333333333333703, 0.3219752754296894559, 0.3333333333333333703, 0.3219752754296894559, 0.3333333333333333703, 0.3219752754296894559, 0.3333333333333333703, 0.3219752754296894559, 0.3333333333333333703, 0.3219752754296894559, 0.3333333333333333703, 0.3219752754296894559, 0.3333333333333333703, 0.3219752754296894559, 0.3333333333333333703, 0.3219752754296894559, 0.3333333333333333703, 0.3219752754296894559, 0.3333333333333333703, 0.3219752754296894559, 0.3333333333333333703, 0.3219752754296894559, 0.3333333333333333703, 0.3219752754296894559, 0.3333333333333333703, 0.3219752754296894559, 0.3333333333333333703, 0.3219752754296894559, 0.3333333333333333703, 0.3219752754296894559, 0.3333333333333333703, 0.3219752754296894559, 0.3333333333333333703, 0.3219752754296894559, 0.3333333333333333703, 0.3219752754296894559, 0.3333333333333333703, 0.3219752754296894559, 0.3333333333333333703, 0.3219752754296894559, 0.3333333333333333703, 0.3219752754296894559, 0.3333333333333333703, 0.3219752754296894559, 0.3333333333333333703, 0.3219752754296894559, 0.3333333333333333703, 0.3219752754296894559, 0.3333333333333333703, 0.3219752754296894559, 0.3333333333333333703, 0.3219752754296894559, 0.3333333333333333703, 0.3219752754296894559, 0.3333333333333333703, 0.3219752754296894559, 0.3333333333333333703, 0.3219752754296894559, 0.3333333333333333703, 0.3219752754296894559, 0.3333333333333333703, 0.3219752754296894559, 0.3333333333333333703, 0.3219752754296894559, 0.3333333333333333703, 0.3219752754296894559, 0.3333333333333333703, 0.3219752754296894559, 0.3333333333333333703, 0.3219752754296894559, 0.3333333333333333703, 0.3219752754296894559, 0.3333333333333333703, 0.3219752754296894559, 0.3333333333333333703, 0.3219752754296894559, 0.3333333333333333703, 0.3219752754296894559, 0.3333333333333333703, 0.3219752754296894559, 0.3333333333333333703, 0.3219752754296894559, 0.3333333333333333703, 0.3219752754296894559, 0.3333333333333333703, 0.3219752754296894559, 0.3333333333333333703, 0.3219752754296894559, 0.3333333333333333703, 0.3219752754296894559, 0.3333333333333333703, 0.3219752754296894559, 0.3333333333333333703, 0.3219752754296894559, 0.3333333333333333703, 0.3219752754296894559, 0.3333333333333333703, 0.3219752754296894559, 0.3333333333333333703, 0.3219752754296894559, 0.3333333333333333703, 0.3219752754296894559, 0.3333333333333333703, 0.3219752754296894559, 0.3333333333333333703, 0.3219752754296894559, 0.3333333333333333703, 0.3219752754296894559, 0.3333333333333333703, 0.3219752754296894559, 0.3333333333333333703, 0.3219752754296894559, 0.3333333333333333703, 0.3219752754296894559, 0.3333333333333333703, 0.3219752754296894559, 0.3333333333333333703, 0.3219752754296894559, 0.3333333333333333703, 0.3219752754296894559, 0.3333333333333333703, 0.3219752754296894559, 0.3333333333333333703, 0.3219752754296894559, 0.3333333333333333703, 0.3219752754296894559, 0.3333333333333333703, 0.3219752754296894559, 0.3333333333333333703, 0.3219752754296894559, 0.3333333333333333703, 0.3219752754296894559, 0.3333333333333333703, 0.3219752754296894559, 0.3333333333333333703, 0.3219752754296894559, 0.3333333333333333703, 0.3219752754296894559, 0.3333333333333333703, 0.3219752754296894559, 0.3333333333333333703, 0.3219752754296894559, 0.3333333333333333703, 0.3219752754296894559, 0.3333333333333333703, 0.3219752754296894559, 0.3333333333333333703, 0.3219752754296894559, 0.3333333333333333703, 0.3219752754296894559, 0.3333333333333333703, 0.3219752754296894559, 0.3333333333333333703, 0.3219752754296894559, 0.3333333333333333703, 0.3219752754296894559, 0.3333333333333333703, 0.3219752754296894559, 0.3333333333333333703, 0.3219752754296894559, 0.3333333333333333703, 0.3219752754296894559, 0.3333333333333333703, 0.3219752754296894559, 0.3333333333333333703, 0.3219752754296894559, 0.3333333333333333703, 0.3219752754296894559, 0.3333333333333333703, 0.3219752754296894559, 0.3333333333333333703, 0.3219752754296894559, 0.3333333333333333703, 0.3219752754296894559, 0.3333333333333333703, 0.3219752754296894559, 0.3333333333333333703, 0.3219752754296894559, 0.3333333333333333703, 0.3219752754296894559, 0.3333333333333333703, 0.3219752754296894559, 0.3333333333333333703, 0.3219752754296894559, 0.3333333333333333703, 0.3219752754296894559, 0.3333333333333333703, 0.3219752754296894559, 0.3333333333333333703, 0.3219752754296894559, 0.3333333333333333703, 0.3219752754296894559, 0.3333333333333333703, 0.3219752754296894559, 0.3333333333333333703, 0.3219752754296894559, 0.3333333333333333703, 0.3219752754296894559, 0.3333333333333333703, 0.3219752754296894559, 0.3333333333333333703, 0.3219752754296894559, 0.3333333333333333703, 0.3219752754296894559, 0.3333333333333333703, 0.3219752754296894559, 0.3333333333333333703, 0.3219752754296894559, 0.3333333333333333703, 0.3219752754296894559, 0.3333333333333333703, 0.3219752754296894559, 0.3333333333333333703, 0.3219752754296894559, 0.3333333333333333703, 0.3219752754296894559, 0.3333333333333333703, 0.3219752754296894559, 0.3333333333333333703, 0.3219752754296894559, 0.3333333333333333703, 0.3219752754296894559, 0.3333333333333333703, 0.3219752754296894559, 0.3333333333333333703, 0.3219752754296894559, 0.3333333333333333703, 0.3219752754296894559, 0.3333333333333333703, 0.3219752754296894559, 0.3333333333333333703, 0.3219752754296894559, 0.3333333333333333703, 0.3219752754296894559, 0.3333333333333333703, 0.3219752754296894559, 0.3333333333333333703, 0.3219752754296894559, 0.3333333333333333703, 0.3219752754296894559, 0.3333333333333333703, 0.3219752754296894559, 0.3333333333333333703, 0.3219752754296894559, 0.3333333333333333703, 0.3219752754296894559, 0.3333333333333333703, 0.3219752754296894559, 0.3333333333333333703, 0.3219752754296894559, 0.3333333333333333703),
 ( 1.000000000000000000, 0.9659258262890683122, 1.000000000000000000, 0.9659258262890683122, 1.000000000000000000, 0.9659258262890683122, 1.000000000000000000, 0.9659258262890683122, 1.000000000000000000, 0.9659258262890683122, 1.000000000000000000, 0.9659258262890683122, 1.000000000000000000, 0.9659258262890683122, 1.000000000000000000, 0.9659258262890683122, 1.000000000000000000, 0.9659258262890683122, 1.000000000000000000, 0.9659258262890683122, 1.000000000000000000, 0.9659258262890683122, 1.000000000000000000, 0.9659258262890683122, 1.000000000000000000, 0.9659258262890683122, 1.000000000000000000, 0.9659258262890683122, 1.000000000000000000, 0.9659258262890683122, 1.000000000000000000, 0.9659258262890683122, 1.000000000000000000, 0.9659258262890683122, 1.000000000000000000, 0.9659258262890683122, 1.000000000000000000, 0.9659258262890683122, 1.000000000000000000, 0.9659258262890683122, 1.000000000000000000, 0.9659258262890683122, 1.000000000000000000, 0.9659258262890683122, 1.000000000000000000, 0.9659258262890683122, 1.000000000000000000, 0.9659258262890683122, 1.000000000000000000, 0.9659258262890683122, 1.000000000000000000, 0.9659258262890683122, 1.000000000000000000, 0.9659258262890683122, 1.000000000000000000, 0.9659258262890683122, 1.000000000000000000, 0.9659258262890683122, 1.000000000000000000, 0.9659258262890683122, 1.000000000000000000, 0.9659258262890683122, 1.000000000000000000, 0.9659258262890683122, 1.000000000000000000, 0.9659258262890683122, 1.000000000000000000, 0.9659258262890683122, 1.000000000000000000, 0.9659258262890683122, 1.000000000000000000, 0.9659258262890683122, 1.000000000000000000, 0.9659258262890683122, 1.000000000000000000, 0.9659258262890683122, 1.000000000000000000, 0.9659258262890683122, 1.000000000000000000, 0.9659258262890683122, 1.000000000000000000, 0.9659258262890683122, 1.000000000000000000, 0.9659258262890683122, 1.000000000000000000, 0.9659258262890683122, 1.000000000000000000, 0.9659258262890683122, 1.000000000000000000, 0.9659258262890683122, 1.000000000000000000, 0.9659258262890683122, 1.000000000000000000, 0.9659258262890683122, 1.000000000000000000, 0.9659258262890683122, 1.000000000000000000, 0.9659258262890683122, 1.000000000000000000, 0.9659258262890683122, 1.000000000000000000, 0.9659258262890683122, 1.000000000000000000, 0.9659258262890683122, 1.000000000000000000, 0.9659258262890683122, 1.000000000000000000, 0.9659258262890683122, 1.000000000000000000, 0.9659258262890683122, 1.000000000000000000, 0.9659258262890683122, 1.000000000000000000, 0.9659258262890683122, 1.000000000000000000, 0.9659258262890683122, 1.000000000000000000, 0.9659258262890683122, 1.000000000000000000, 0.9659258262890683122, 1.000000000000000000, 0.9659258262890683122, 1.000000000000000000, 0.9659258262890683122, 1.000000000000000000, 0.9659258262890683122, 1.000000000000000000, 0.9659258262890683122, 1.000000000000000000, 0.9659258262890683122, 1.000000000000000000, 0.9659258262890683122, 1.000000000000000000, 0.9659258262890683122, 1.000000000000000000, 0.9659258262890683122, 1.000000000000000000, 0.9659258262890683122, 1.000000000000000000, 0.9659258262890683122, 1.000000000000000000, 0.9659258262890683122, 1.000000000000000000, 0.9659258262890683122, 1.000000000000000000, 0.9659258262890683122, 1.000000000000000000, 0.9659258262890683122, 1.000000000000000000, 0.9659258262890683122, 1.000000000000000000, 0.9659258262890683122, 1.000000000000000000, 0.9659258262890683122, 1.000000000000000000, 0.9659258262890683122, 1.000000000000000000, 0.9659258262890683122, 1.000000000000000000, 0.9659258262890683122, 1.000000000000000000, 0.9659258262890683122, 1.000000000000000000, 0.9659258262890683122, 1.000000000000000000, 0.9659258262890683122, 1.000000000000000000, 0.9659258262890683122, 1.000000000000000000, 0.9659258262890683122, 1.000000000000000000, 0.9659258262890683122, 1.000000000000000000, 0.9659258262890683122, 1.000000000000000000, 0.9659258262890683122, 1.000000000000000000, 0.9659258262890683122, 1.000000000000000000, 0.9659258262890683122, 1.000000000000000000, 0.9659258262890683122, 1.000000000000000000, 0.9659258262890683122, 1.000000000000000000, 0.9659258262890683122, 1.000000000000000000, 0.9659258262890683122, 1.000000000000000000, 0.9659258262890683122, 1.000000000000000000, 0.9659258262890683122, 1.000000000000000000, 0.9659258262890683122, 1.000000000000000000, 0.9659258262890683122, 1.000000000000000000, 0.9659258262890683122, 1.000000000000000000, 0.9659258262890683122, 1.000000000000000000, 0.9659258262890683122, 1.000000000000000000, 0.9659258262890683122, 1.000000000000000000, 0.9659258262890683122, 1.000000000000000000, 0.9659258262890683122, 1.000000000000000000, 0.9659258262890683122, 1.000000000000000000, 0.9659258262890683122, 1.000000000000000000, 0.9659258262890683122, 1.000000000000000000, 0.9659258262890683122, 1.000000000000000000, 0.9659258262890683122, 1.000000000000000000, 0.9659258262890683122, 1.000000000000000000, 0.9659258262890683122, 1.000000000000000000, 0.9659258262890683122, 1.000000000000000000, 0.9659258262890683122, 1.000000000000000000, 0.9659258262890683122, 1.000000000000000000, 0.9659258262890683122, 1.000000000000000000, 0.9659258262890683122, 1.000000000000000000, 0.9659258262890683122, 1.000000000000000000, 0.9659258262890683122, 1.000000000000000000, 0.9659258262890683122, 1.000000000000000000, 0.9659258262890683122, 1.000000000000000000, 0.9659258262890683122, 1.000000000000000000, 0.9659258262890683122, 1.000000000000000000, 0.9659258262890683122, 1.000000000000000000, 0.9659258262890683122, 1.000000000000000000, 0.9659258262890683122, 1.000000000000000000, 0.9659258262890683122, 1.000000000000000000, 0.9659258262890683122, 1.000000000000000000, 0.9659258262890683122, 1.000000000000000000, 0.9659258262890683122, 1.000000000000000000, 0.9659258262890683122, 1.000000000000000000, 0.9659258262890683122, 1.000000000000000000, 0.9659258262890683122, 1.000000000000000000, 0.9659258262890683122, 1.000000000000000000, 0.9659258262890683122, 1.000000000000000000, 0.9659258262890683122, 1.000000000000000000, 0.9659258262890683122, 1.000000000000000000, 0.9659258262890683122, 1.000000000000000000, 0.9659258262890683122, 1.000000000000000000, 0.9659258262890683122, 1.000000000000000000, 0.9659258262890683122, 1.000000000000000000, 0.9659258262890683122, 1.000000000000000000, 0.9659258262890683122, 1.000000000000000000, 0.9659258262890683122, 1.000000000000000000, 0.9659258262890683122, 1.000000000000000000, 0.9659258262890683122, 1.000000000000000000, 0.9659258262890683122, 1.000000000000000000, 0.9659258262890683122, 1.000000000000000000, 0.9659258262890683122, 1.000000000000000000, 0.9659258262890683122, 1.000000000000000000, 0.9659258262890683122, 1.000000000000000000, 0.9659258262890683122, 1.000000000000000000, 0.9659258262890683122, 1.000000000000000000, 0.9659258262890683122, 1.000000000000000000, 0.9659258262890683122, 1.000000000000000000, 0.9659258262890683122, 1.000000000000000000, 0.9659258262890683122, 1.000000000000000000, 0.9659258262890683122, 1.000000000000000000, 0.9659258262890683122, 1.000000000000000000, 0.9659258262890683122, 1.000000000000000000, 0.9659258262890683122, 1.000000000000000000, 0.9659258262890683122, 1.000000000000000000, 0.9659258262890683122, 1.000000000000000000, 0.9659258262890683122, 1.000000000000000000, 0.9659258262890683122, 1.000000000000000000, 0.9659258262890683122, 1.000000000000000000, 0.9659258262890683122, 1.000000000000000000, 0.9659258262890683122, 1.000000000000000000, 0.9659258262890683122, 1.000000000000000000, 0.9659258262890683122, 1.000000000000000000, 0.9659258262890683122, 1.000000000000000000, 0.9659258262890683122, 1.000000000000000000, 0.9659258262890683122, 1.000000000000000000, 0.9659258262890683122, 1.000000000000000000, 0.9659258262890683122, 1.000000000000000000, 0.9659258262890683122, 1.000000000000000000, 0.9659258262890683122, 1.000000000000000000, 0.9659258262890683122, 1.000000000000000000, 0.9659258262890683122, 1.000000000000000000, 0.9659258262890683122, 1.000000000000000000, 0.9659258262890683122, 1.000000000000000000, 0.9659258262890683122, 1.000000000000000000, 0.9659258262890683122, 1.000000000000000000, 0.9659258262890683122, 1.000000000000000000, 0.9659258262890683122, 1.000000000000000000, 0.9659258262890683122, 1.000000000000000000, 0.9659258262890683122, 1.000000000000000000, 0.9659258262890683122, 1.000000000000000000, 0.9659258262890683122, 1.000000000000000000, 0.9659258262890683122, 1.000000000000000000, 0.9659258262890683122, 1.000000000000000000, 0.9659258262890683122, 1.000000000000000000, 0.9659258262890683122, 1.000000000000000000, 0.9659258262890683122, 1.000000000000000000, 0.9659258262890683122, 1.000000000000000000, 0.9659258262890683122, 1.000000000000000000, 0.9659258262890683122, 1.000000000000000000, 0.9659258262890683122, 1.000000000000000000, 0.9659258262890683122, 1.000000000000000000, 0.9659258262890683122, 1.000000000000000000, 0.9659258262890683122, 1.000000000000000000, 0.9659258262890683122, 1.000000000000000000, 0.9659258262890683122, 1.000000000000000000, 0.9659258262890683122, 1.000000000000000000, 0.9659258262890683122, 1.000000000000000000, 0.9659258262890683122, 1.000000000000000000, 0.9659258262890683122, 1.000000000000000000, 0.9659258262890683122, 1.000000000000000000, 0.9659258262890683122, 1.000000000000000000, 0.9659258262890683122, 1.000000000000000000, 0.9659258262890683122, 1.000000000000000000, 0.9659258262890683122, 1.000000000000000000, 0.9659258262890683122, 1.000000000000000000, 0.9659258262890683122, 1.000000000000000000, 0.9659258262890683122, 1.000000000000000000, 0.9659258262890683122, 1.000000000000000000, 0.9659258262890683122, 1.000000000000000000, 0.9659258262890683122, 1.000000000000000000, 0.9659258262890683122, 1.000000000000000000, 0.9659258262890683122, 1.000000000000000000, 0.9659258262890683122, 1.000000000000000000, 0.9659258262890683122, 1.000000000000000000, 0.9659258262890683122, 1.000000000000000000, 0.9659258262890683122, 1.000000000000000000, 0.9659258262890683122, 1.000000000000000000, 0.9659258262890683122, 1.000000000000000000, 0.9659258262890683122, 1.000000000000000000, 0.9659258262890683122, 1.000000000000000000, 0.9659258262890683122, 1.000000000000000000) ) ) 
 REPRESENTATION_ITEM ( '' )  SURFACE ( )  );
#114015=CARTESIAN_POINT ( 'NONE',  ( 8.224510206698742110, 14.34966873604972548, 22.08442372801901143 ) ) ;
#114016=CARTESIAN_POINT ( 'NONE',  ( -9.474510206698720793, -16.51473224551083518, 44.58442372801900433 ) ) ;
#114017=CARTESIAN_POINT ( 'NONE',  ( 21.55341960407619695, -5.719274019375665929, 56.04275706135235424 ) ) ;
#114018=CARTESIAN_POINT ( 'NONE',  ( 5.823673210054125526, 21.52544592524343514, 109.7905762719810383 ) ) ;
#114019=CARTESIAN_POINT ( 'NONE',  ( -21.55341960407610458, -5.719274019375992779, 56.45724293864768839 ) ) ;
#114020=CARTESIAN_POINT ( 'NONE',  ( 16.46253265017146816, 9.564922557961045513, 106.6677570613523471 ) ) ;
#114021=CARTESIAN_POINT ( 'NONE',  ( 16.46253265017160672, -9.564922557960803928, 48.33224293864769550 ) ) ;
#114022=CARTESIAN_POINT ( 'NONE',  ( -19.05341960407617563, 5.049401038297882671, 73.54275706135233293 ) ) ;
#114023=CARTESIAN_POINT ( 'NONE',  ( 5.719274019375673035, 21.55341960407619339, 87.29275706135236135 ) ) ;
#114024=CARTESIAN_POINT ( 'NONE',  ( -9.474510206698720793, -16.51473224551083518, 59.58442372801900433 ) ) ;
#114025=CARTESIAN_POINT ( 'NONE',  ( -16.51473224551069308, -9.474510206698971260, 41.66557627198103120 ) ) ;
#114026=CARTESIAN_POINT ( 'NONE',  ( 15.72974639402199770, -15.80617190586745480, 58.12390960531435979 ) ) ;
#114027=CARTESIAN_POINT ( 'NONE',  ( -14.34966873604960291, -8.224510206698953496, 46.66557627198102409 ) ) ;
#114029=CARTESIAN_POINT ( 'NONE',  ( -5.153800228976607833, 19.02544592524334988, 32.70942372801899722 ) ) ;
#114030=CARTESIAN_POINT ( 'NONE',  ( 8.224510206698742110, 14.34966873604972548, 82.08442372801901854 ) ) ;
#114031=CARTESIAN_POINT ( 'NONE',  ( 4.483927247898545687, 16.52544592524342804, 59.79057627198103120 ) ) ;
#114032=CARTESIAN_POINT ( 'NONE',  ( 18.62759615963255655, 10.81492255796105972, 86.66775706135234714 ) ) ;
#114033=CARTESIAN_POINT ( 'NONE',  ( -10.72451020669870658, -18.67979575497194134, 79.58442372801903275 ) ) ;
#114034=CARTESIAN_POINT ( 'NONE',  ( -21.53943276465977519, 0.05219959533907696930, 86.24890960531436690 ) ) ;
#114035=CARTESIAN_POINT ( 'NONE',  ( -16.46253265017160317, 9.564922557960807481, 55.83224293864769550 ) ) ;
#114036=CARTESIAN_POINT ( 'NONE',  ( -10.81492255796105439, 18.62759615963255655, 52.91775706135235424 ) ) ;
#114037=CARTESIAN_POINT ( 'NONE',  ( -19.03943276465977164, 0.05219959533909376836, 41.24890960531435269 ) ) ;
#114039=CARTESIAN_POINT ( 'NONE',  ( -16.46253265017160317, 9.564922557960807481, 55.83224293864769550 ) ) ;
#114040=CARTESIAN_POINT ( 'NONE',  ( 14.34966873604960469, 8.224510206698951720, 104.1655762719810241 ) ) ;
#114041=CARTESIAN_POINT ( 'NONE',  ( 5.049401038298161559, -19.05341960407611168, 97.70724293864766707 ) ) ;
#114042=CARTESIAN_POINT ( 'NONE',  ( -4.483927247898539470, -16.52544592524342804, 52.29057627198102409 ) ) ;
#114043=CARTESIAN_POINT ( 'NONE',  ( -16.55341960407611168, -4.379528057220339221, 106.4572429386477097 ) ) ;
#114044=CARTESIAN_POINT ( 'NONE',  ( -15.80617190586745835, -15.72974639402198527, 81.87390960531435269 ) ) ;
#114045=CARTESIAN_POINT ( 'NONE',  ( -5.719274019375978568, 21.55341960407610458, 115.2072429386476955 ) ) ;
#114047=CARTESIAN_POINT ( 'NONE',  ( 14.29746914071037800, 8.314922557961029526, 41.66775706135235424 ) ) ;
#114049=CARTESIAN_POINT ( 'NONE',  ( 21.55341960407610458, 5.719274019375980345, 73.95724293864769550 ) ) ;
#114050=CARTESIAN_POINT ( 'NONE',  ( -0.05219959533937732626, 21.53943276465977519, 112.5010903946857042 ) ) ;
#114051=CARTESIAN_POINT ( 'NONE',  ( 5.153800228976335163, 19.02544592524342804, 99.79057627198102409 ) ) ;
#114052=CARTESIAN_POINT ( 'NONE',  ( 18.62759615963255655, 10.81492255796105972, 26.66775706135235424 ) ) ;
#114055=CARTESIAN_POINT ( 'NONE',  ( -18.67979575497178146, -10.72451020669898902, 31.66557627198102054 ) ) ;
#114056=CARTESIAN_POINT ( 'NONE',  ( -14.34966873604972548, 8.224510206698743886, 103.3344237280190043 ) ) ;
#114057=CARTESIAN_POINT ( 'NONE',  ( 18.67979575497194134, -10.72451020669871369, 50.83442372801901143 ) ) ;
#114058=CARTESIAN_POINT ( 'NONE',  ( 21.55341960407619695, -5.719274019375665929, 86.04275706135236135 ) ) ;
#114059=CARTESIAN_POINT ( 'NONE',  ( 5.823673210054444382, -21.52544592524334988, 110.2094237280190185 ) ) ;
#114060=CARTESIAN_POINT ( 'NONE',  ( 12.14591786802327356, -12.06949235617739191, 75.62609039468567573 ) ) ;
#114061=CARTESIAN_POINT ( 'NONE',  ( 15.80617190586769283, -15.72974639402175789, 35.62609039468568994 ) ) ;
#114062=CARTESIAN_POINT ( 'NONE',  ( -5.153800228976328057, -19.02544592524343514, 37.29057627198102409 ) ) ;
#114063=CARTESIAN_POINT ( 'NONE',  ( -21.53943276465977519, -0.05219959533937600094, 108.7510903946857042 ) ) ;
#114064=CARTESIAN_POINT ( 'NONE',  ( 19.02544592524343514, -5.153800228976328945, 103.5405762719809957 ) ) ;
#114065=CARTESIAN_POINT ( 'NONE',  ( 10.72451020669898902, -18.67979575497178502, 102.9155762719810383 ) ) ;
#114067=CARTESIAN_POINT ( 'NONE',  ( 21.55341960407610458, 5.719274019375980345, 63.95724293864770260 ) ) ;
#114068=CARTESIAN_POINT ( 'NONE',  ( -4.483927247898782831, 16.52544592524335698, 52.70942372801902565 ) ) ;
#114069=CARTESIAN_POINT ( 'NONE',  ( 4.379528057220339221, -16.55341960407611168, 52.70724293864769550 ) ) ;
#114070=CARTESIAN_POINT ( 'NONE',  ( -5.049401038297874678, -19.05341960407617918, 74.79275706135231871 ) ) ;
#114072=CARTESIAN_POINT ( 'NONE',  ( 16.52544592524335698, 4.483927247898782831, 26.45942372801901854 ) ) ;
#114073=CARTESIAN_POINT ( 'NONE',  ( 18.67979575497178502, 10.72451020669898547, 104.1655762719810241 ) ) ;
#114074=CARTESIAN_POINT ( 'NONE',  ( -16.55341960407611168, -4.379528057220339221, 61.45724293864770260 ) ) ;
#114075=CARTESIAN_POINT ( 'NONE',  ( -5.153800228976328057, -19.02544592524343514, 107.2905762719810383 ) ) ;
#114076=CARTESIAN_POINT ( 'NONE',  ( -14.34966873604972548, 8.224510206698743886, 43.33442372801901143 ) ) ;
#114077=CARTESIAN_POINT ( 'NONE',  ( -16.51473224551069308, -9.474510206698971260, 56.66557627198103120 ) ) ;
#114078=CARTESIAN_POINT ( 'NONE',  ( 0.05219959533937995610, -21.53943276465977519, 25.00109039468567218 ) ) ;
#114079=CARTESIAN_POINT ( 'NONE',  ( 5.049401038297881783, 19.05341960407617563, 97.29275706135233293 ) ) ;
#114080=CARTESIAN_POINT ( 'NONE',  ( 9.564922557960805705, 16.46253265017160317, 109.5822429386476955 ) ) ;
#114081=CARTESIAN_POINT ( 'NONE',  ( -9.564922557960796823, -16.46253265017161027, 87.08224293864769550 ) ) ;
#114082=CARTESIAN_POINT ( 'NONE',  ( -10.72451020669898014, 18.67979575497178502, 95.41557627198102409 ) ) ;
#114083=CARTESIAN_POINT ( 'NONE',  ( 9.474510206698971260, -16.51473224551069308, 62.91557627198102409 ) ) ;
#114085=CARTESIAN_POINT ( 'NONE',  ( -4.483927247898539470, -16.52544592524342804, 67.29057627198103830 ) ) ;
#114086=CARTESIAN_POINT ( 'NONE',  ( 16.46253265017160672, -9.564922557960803928, 98.33224293864769550 ) ) ;
#114088=CARTESIAN_POINT ( 'NONE',  ( -13.97604488694547697, 13.89961937509957934, 78.12609039468567573 ) ) ;
#114089=CARTESIAN_POINT ( 'NONE',  ( -0.05219959533907301413, -21.53943276465977519, 97.49890960531436690 ) ) ;
#114090=CARTESIAN_POINT ( 'NONE',  ( -5.049401038297874678, -19.05341960407617918, 54.79275706135234003 ) ) ;
#114091=CARTESIAN_POINT ( 'NONE',  ( -13.89961937509977652, 13.97604488694528158, 115.6239096053143669 ) ) ;
#114092=CARTESIAN_POINT ( 'NONE',  ( 18.22780087662122739, 5.500000000000000888, 76.48236817873106475 ) ) ;
#114093=CARTESIAN_POINT ( 'NONE',  ( -21.52544592524343514, 5.823673210054127303, 51.04057627198103120 ) ) ;
#114094=CARTESIAN_POINT ( 'NONE',  ( 19.05341960407611168, 5.049401038298154454, 88.95724293864769550 ) ) ;
#114095=CARTESIAN_POINT ( 'NONE',  ( 0.05219959533937995610, -21.53943276465977519, 75.00109039468568994 ) ) ;
#114096=CARTESIAN_POINT ( 'NONE',  ( -19.05341960407611168, -5.049401038298163336, 36.45724293864766707 ) ) ;
#114097=CARTESIAN_POINT ( 'NONE',  ( -4.379528057220328563, 16.55341960407611168, 75.20724293864769550 ) ) ;
#114098=CARTESIAN_POINT ( 'NONE',  ( -4.379528057220086978, -16.55341960407618274, 19.79275706135235069 ) ) ;
#114099=CARTESIAN_POINT ( 'NONE',  ( 21.53943276465977519, 0.05219959533937863772, 66.25109039468567573 ) ) ;
#114101=CARTESIAN_POINT ( 'NONE',  ( -19.03943276465977164, 0.05219959533909376836, 111.2489096053143669 ) ) ;
#114102=CARTESIAN_POINT ( 'NONE',  ( -19.03943276465977164, -0.05219959533935918106, 73.75109039468566152 ) ) ;
#114104=CARTESIAN_POINT ( 'NONE',  ( 21.53943276465977519, 0.05219959533937863772, 26.25109039468567573 ) ) ;
#114106=CARTESIAN_POINT ( 'NONE',  ( 19.02544592524334988, 5.153800228976608722, 21.45942372801899012 ) ) ;
#114107=CARTESIAN_POINT ( 'NONE',  ( -5.049401038298153566, 19.05341960407611168, 60.20724293864768129 ) ) ;
#114108=CARTESIAN_POINT ( 'NONE',  ( 5.719274019375673035, 21.55341960407619339, 107.2927570613523471 ) ) ;
#114109=CARTESIAN_POINT ( 'NONE',  ( 12.14591786802327356, -12.06949235617739191, 105.6260903946856899 ) ) ;
#114110=CARTESIAN_POINT ( 'NONE',  ( 19.03943276465977164, -0.05219959533909143690, 98.74890960531436690 ) ) ;
#114111=CARTESIAN_POINT ( 'NONE',  ( -5.719274019375665041, -21.55341960407619695, 79.79275706135236135 ) ) ;
#114114=CARTESIAN_POINT ( 'NONE',  ( 21.55341960407619695, -5.719274019375665929, 66.04275706135236135 ) ) ;
#114115=CARTESIAN_POINT ( 'NONE',  ( -21.52544592524334988, -5.823673210054445271, 98.95942372801903275 ) ) ;
#114116=VECTOR ( 'NONE', #152672, 1000.000000000000000 ) ;
#114118=CARTESIAN_POINT ( 'NONE',  ( 19.02544592524343514, -5.153800228976328945, 93.54057627198102409 ) ) ;
#114119=CARTESIAN_POINT ( 'NONE',  ( -19.02544592524334988, -5.153800228976617603, 28.95942372801900433 ) ) ;
#114121=CARTESIAN_POINT ( 'NONE',  ( -19.03943276465977164, 0.05219959533909376836, 36.24890960531436690 ) ) ;
#114122=CARTESIAN_POINT ( 'NONE',  ( 10.81492255796078972, 18.62759615963270932, 54.58224293864769550 ) ) ;
#114123=CARTESIAN_POINT ( 'NONE',  ( -12.14591786802326823, 12.06949235617739902, 103.1260903946856757 ) ) ;
#114124=CARTESIAN_POINT ( 'NONE',  ( -4.379528057220328563, 16.55341960407611168, 95.20724293864769550 ) ) ;
#114125=CARTESIAN_POINT ( 'NONE',  ( -13.97604488694527625, -13.89961937509977652, 76.87390960531433848 ) ) ;
#114126=CARTESIAN_POINT ( 'NONE',  ( 10.81492255796106328, -18.62759615963255655, 100.4177570613523471 ) ) ;
#114128=CARTESIAN_POINT ( 'NONE',  ( -19.03943276465977164, 0.05219959533909376836, 31.24890960531435979 ) ) ;
#114129=CARTESIAN_POINT ( 'NONE',  ( -8.314922557960811034, -14.29746914071050412, 102.0822429386476955 ) ) ;
#114130=CARTESIAN_POINT ( 'NONE',  ( 10.81492255796106328, -18.62759615963255655, 55.41775706135234714 ) ) ;
#114131=CARTESIAN_POINT ( 'NONE',  ( -10.72451020669898014, 18.67979575497178502, 90.41557627198103830 ) ) ;
#114132=CARTESIAN_POINT ( 'NONE',  ( 5.049401038297881783, 19.05341960407617563, 47.29275706135231161 ) ) ;
#114133=CARTESIAN_POINT ( 'NONE',  ( 16.46253265017160672, -9.564922557960803928, 48.33224293864769550 ) ) ;
#114134=CARTESIAN_POINT ( 'NONE',  ( 19.03943276465977164, -0.05219959533909143690, 93.74890960531435269 ) ) ;
#114135=CARTESIAN_POINT ( 'NONE',  ( -4.379528057220328563, 16.55341960407611168, 75.20724293864769550 ) ) ;
#114136=CARTESIAN_POINT ( 'NONE',  ( -19.03943276465977164, -0.05219959533935918106, 43.75109039468566863 ) ) ;
#114137=CARTESIAN_POINT ( 'NONE',  ( -19.05341960407611168, -5.049401038298163336, 61.45724293864769550 ) ) ;
#114138=CARTESIAN_POINT ( 'NONE',  ( 4.483927247898545687, 16.52544592524342804, 44.79057627198103120 ) ) ;
#114139=CARTESIAN_POINT ( 'NONE',  ( 9.564922557961047289, -16.46253265017146816, 85.41775706135233293 ) ) ;
#114140=CARTESIAN_POINT ( 'NONE',  ( -17.58332526062526213, -7.635886036038624702, 89.07665040441536064 ) ) ;
#114141=CARTESIAN_POINT ( 'NONE',  ( 10.81492255796078972, 18.62759615963270932, 39.58224293864769550 ) ) ;
#114142=EDGE_CURVE ( 'NONE', #135989, #65463, #197573, .T. ) ;
#114143=CARTESIAN_POINT ( 'NONE',  ( -16.52544592524342804, 4.483927247898546575, 106.0405762719810525 ) ) ;
#114144=CARTESIAN_POINT ( 'NONE',  ( -17.50000000000015277, -3.417042746627028560, 24.82619603767517447 ) ) ;
#114145=CARTESIAN_POINT ( 'NONE',  ( 9.564922557960805705, 16.46253265017160317, 54.58224293864769550 ) ) ;
#114146=CARTESIAN_POINT ( 'NONE',  ( -10.72451020669898014, 18.67979575497178502, 65.41557627198102409 ) ) ;
#114147=CARTESIAN_POINT ( 'NONE',  ( 19.03943276465977164, -0.05219959533909143690, 28.74890960531435624 ) ) ;
#114148=CARTESIAN_POINT ( 'NONE',  ( 16.52544592524335698, 4.483927247898782831, 76.45942372801901854 ) ) ;
#114149=CARTESIAN_POINT ( 'NONE',  ( 19.03943276465977164, -0.05219959533909143690, 63.74890960531435979 ) ) ;
#114150=CARTESIAN_POINT ( 'NONE',  ( 9.564922557961047289, -16.46253265017146816, 60.41775706135233293 ) ) ;
#114151=CARTESIAN_POINT ( 'NONE',  ( -21.53943276465977519, -0.05219959533937600094, 63.75109039468568284 ) ) ;
#114152=CARTESIAN_POINT ( 'NONE',  ( 5.719274019375991003, -21.55341960407610458, 52.70724293864769550 ) ) ;
#114153=CARTESIAN_POINT ( 'NONE',  ( 13.89961937509977652, -13.97604488694527269, 28.12390960531435624 ) ) ;
#114154=CARTESIAN_POINT ( 'NONE',  ( 0.05219959533934541429, -16.53943276465976808, 85.00109039468568994 ) ) ;
#114155=CARTESIAN_POINT ( 'NONE',  ( -19.02544592524334988, -5.153800228976617603, 98.95942372801900433 ) ) ;
#114156=CARTESIAN_POINT ( 'NONE',  ( 13.97604488694527802, 13.89961937509977652, 24.37390960531435624 ) ) ;
#114158=CARTESIAN_POINT ( 'NONE',  ( -5.823673210054116645, -21.52544592524344225, 52.29057627198102409 ) ) ;
#114159=CARTESIAN_POINT ( 'NONE',  ( 18.62759615963255655, 10.81492255796105972, 86.66775706135234714 ) ) ;
#114160=CARTESIAN_POINT ( 'NONE',  ( -0.05219959533910754901, -16.53943276465976808, 47.49890960531435979 ) ) ;
#114161=CARTESIAN_POINT ( 'NONE',  ( 0.05219959533910956823, 16.53943276465976808, 49.99890960531437401 ) ) ;
#114162=CARTESIAN_POINT ( 'NONE',  ( 0.05219959533907565091, 21.53943276465977519, 79.99890960531435269 ) ) ;
#114163=CARTESIAN_POINT ( 'NONE',  ( 15.80617190586746368, 15.72974639402197994, 84.37390960531438111 ) ) ;
#114165=CARTESIAN_POINT ( 'NONE',  ( 0.05219959533907565091, 21.53943276465977519, 34.99890960531435979 ) ) ;
#114166=CARTESIAN_POINT ( 'NONE',  ( 0.05219959533934541429, -16.53943276465976808, 65.00109039468568994 ) ) ;
#114167=CARTESIAN_POINT ( 'NONE',  ( 14.34966873604960469, 8.224510206698951720, 79.16557627198103830 ) ) ;
#114168=CARTESIAN_POINT ( 'NONE',  ( 5.049401038298161559, -19.05341960407611168, 37.70724293864768839 ) ) ;
#114170=DIRECTION ( 'NONE',  ( -0.5150380737757255245, 1.049727191973305394E-16, -0.8571673013836856869 ) ) ;
#114171=CARTESIAN_POINT ( 'NONE',  ( 0.05219959533934541429, -16.53943276465976808, 100.0010903946857042 ) ) ;
#114172=CARTESIAN_POINT ( 'NONE',  ( -21.55341960407610458, -5.719274019375992779, 111.4572429386476813 ) ) ;
#114173=CARTESIAN_POINT ( 'NONE',  ( -13.97604488694527625, -13.89961937509977652, 76.87390960531433848 ) ) ;
#114174=CARTESIAN_POINT ( 'NONE',  ( -10.81492255796105439, 18.62759615963255655, 47.91775706135234714 ) ) ;
#114175=CARTESIAN_POINT ( 'NONE',  ( 13.89961937509977652, -13.97604488694527269, 113.1239096053143527 ) ) ;
#114178=CARTESIAN_POINT ( 'NONE',  ( 21.52544592524334988, 5.823673210054432836, 41.45942372801901143 ) ) ;
#114179=CARTESIAN_POINT ( 'NONE',  ( -9.474510206698964154, 16.51473224551069663, 35.41557627198102409 ) ) ;
#114180=CARTESIAN_POINT ( 'NONE',  ( -5.153800228976328057, -19.02544592524343514, 97.29057627198099567 ) ) ;
#114181=CARTESIAN_POINT ( 'NONE',  ( -16.46253265017146816, -9.564922557961047289, 49.16775706135233293 ) ) ;
#114182=CARTESIAN_POINT ( 'NONE',  ( 21.53943276465977519, 0.05219959533937863772, 31.25109039468568639 ) ) ;
#114183=CARTESIAN_POINT ( 'NONE',  ( 5.153800228976615827, -19.02544592524334988, 50.20942372801897591 ) ) ;
#114184=CARTESIAN_POINT ( 'NONE',  ( 19.05341960407611168, 5.049401038298154454, 23.95724293864769194 ) ) ;
#114185=CARTESIAN_POINT ( 'NONE',  ( -14.29746914071037622, -8.314922557961029526, 94.16775706135237556 ) ) ;
#114186=CARTESIAN_POINT ( 'NONE',  ( -9.474510206698720793, -16.51473224551083518, 59.58442372801900433 ) ) ;
#114187=CARTESIAN_POINT ( 'NONE',  ( 14.34966873604972726, -8.224510206698740333, 100.8344237280190185 ) ) ;
#114189=CARTESIAN_POINT ( 'NONE',  ( 16.51473224551069308, 9.474510206698969483, 79.16557627198103830 ) ) ;
#114190=CARTESIAN_POINT ( 'NONE',  ( -10.81492255796105439, 18.62759615963255655, 92.91775706135236135 ) ) ;
#114191=CARTESIAN_POINT ( 'NONE',  ( 21.52544592524334988, 5.823673210054432836, 101.4594237280190185 ) ) ;
#114192=CARTESIAN_POINT ( 'NONE',  ( -13.97604488694527625, -13.89961937509977652, 21.87390960531435979 ) ) ;
#114193=CARTESIAN_POINT ( 'NONE',  ( -16.46253265017160317, 9.564922557960807481, 95.83224293864769550 ) ) ;
#114194=CARTESIAN_POINT ( 'NONE',  ( -21.52544592524334988, -5.823673210054445271, 78.95942372801901854 ) ) ;
#114195=CARTESIAN_POINT ( 'NONE',  ( 4.379528057220092307, 16.55341960407617563, 22.29275706135235069 ) ) ;
#114196=CARTESIAN_POINT ( 'NONE',  ( -5.049401038298153566, 19.05341960407611168, 75.20724293864769550 ) ) ;
#114197=CARTESIAN_POINT ( 'NONE',  ( -18.67979575497178146, -10.72451020669898902, 26.66557627198103475 ) ) ;
#114199=CARTESIAN_POINT ( 'NONE',  ( 5.153800228976335163, 19.02544592524342804, 89.79057627198102409 ) ) ;
#114200=LINE ( 'NONE', #145546, #17610 ) ;
#114201=CARTESIAN_POINT ( 'NONE',  ( 19.03943276465977164, -0.05219959533909143690, 73.74890960531435269 ) ) ;
#114202=CARTESIAN_POINT ( 'NONE',  ( 16.46253265017160672, -9.564922557960803928, 68.33224293864770971 ) ) ;
#114203=CARTESIAN_POINT ( 'NONE',  ( 16.55341960407618274, -4.379528057220086978, 96.04275706135236135 ) ) ;
#114205=CARTESIAN_POINT ( 'NONE',  ( -0.05219959533936034679, 19.03943276465977164, 77.50109039468566152 ) ) ;
#114206=CARTESIAN_POINT ( 'NONE',  ( -9.474510206698964154, 16.51473224551069663, 95.41557627198102409 ) ) ;
#114207=CARTESIAN_POINT ( 'NONE',  ( -12.14591786802309592, -12.06949235617757132, 81.87390960531435269 ) ) ;
#114208=CARTESIAN_POINT ( 'NONE',  ( -5.719274019375978568, 21.55341960407610458, 40.20724293864769550 ) ) ;
#114209=CARTESIAN_POINT ( 'NONE',  ( -18.67979575497178146, -10.72451020669898902, 21.66557627198102409 ) ) ;
#114210=CARTESIAN_POINT ( 'NONE',  ( 14.34966873604960469, 8.224510206698951720, 109.1655762719810383 ) ) ;
#114211=CARTESIAN_POINT ( 'NONE',  ( -16.52216118717207749, 7.221426719304497865, 53.92400978953007495 ) ) ;
#114212=CARTESIAN_POINT ( 'NONE',  ( 16.46253265017146816, 9.564922557961045513, 46.66775706135233293 ) ) ;
#114213=CARTESIAN_POINT ( 'NONE',  ( 4.379528057220339221, -16.55341960407611168, 32.70724293864770260 ) ) ;
#114214=CARTESIAN_POINT ( 'NONE',  ( 19.05341960407611168, 5.049401038298154454, 98.95724293864766707 ) ) ;
#114215=CARTESIAN_POINT ( 'NONE',  ( 15.80617190586769283, -15.72974639402175789, 60.62609039468567573 ) ) ;
#114216=CARTESIAN_POINT ( 'NONE',  ( 0.05219959533907565091, 21.53943276465977519, 54.99890960531435269 ) ) ;
#114217=CARTESIAN_POINT ( 'NONE',  ( -21.55341960407619339, 5.719274019375674811, 28.54275706135234358 ) ) ;
#114218=CARTESIAN_POINT ( 'NONE',  ( -18.62759615963270932, 10.81492255796079327, 80.83224293864769550 ) ) ;
#114219=CARTESIAN_POINT ( 'NONE',  ( -5.823673210054431948, 21.52544592524334988, 37.70942372801900433 ) ) ;
#114220=CARTESIAN_POINT ( 'NONE',  ( 16.55341960407611168, 4.379528057220329451, 113.9572429386477239 ) ) ;
#114221=CARTESIAN_POINT ( 'NONE',  ( 16.51473224551083163, -9.474510206698727899, 70.83442372801900433 ) ) ;
#114222=CARTESIAN_POINT ( 'NONE',  ( 5.049401038298161559, -19.05341960407611168, 47.70724293864770260 ) ) ;
#114223=CARTESIAN_POINT ( 'NONE',  ( -4.379528057220328563, 16.55341960407611168, 95.20724293864769550 ) ) ;
#114224=CARTESIAN_POINT ( 'NONE',  ( -13.89961937509977652, 13.97604488694528158, 100.6239096053143669 ) ) ;
#114225=CARTESIAN_POINT ( 'NONE',  ( -5.153800228976328057, -19.02544592524343514, 112.2905762719810099 ) ) ;
#114226=CARTESIAN_POINT ( 'NONE',  ( -9.564922557960796823, -16.46253265017161027, 32.08224293864769550 ) ) ;
#114227=CARTESIAN_POINT ( 'NONE',  ( 14.34966873604960469, 8.224510206698951720, 44.16557627198103120 ) ) ;
#114228=CARTESIAN_POINT ( 'NONE',  ( -4.483927247898782831, 16.52544592524335698, 97.70942372801904696 ) ) ;
#114229=CARTESIAN_POINT ( 'NONE',  ( 13.89961937509977652, -13.97604488694527269, 53.12390960531434558 ) ) ;
#114230=CARTESIAN_POINT ( 'NONE',  ( 4.379528057220339221, -16.55341960407611168, 112.7072429386476955 ) ) ;
#114231=CARTESIAN_POINT ( 'NONE',  ( 19.02544592524334988, 5.153800228976608722, 26.45942372801899722 ) ) ;
#114232=CARTESIAN_POINT ( 'NONE',  ( 19.05341960407611168, 5.049401038298154454, 108.9572429386477097 ) ) ;
#114233=CARTESIAN_POINT ( 'NONE',  ( -12.14591786802309592, -12.06949235617757132, 21.87390960531436690 ) ) ;
#114234=CARTESIAN_POINT ( 'NONE',  ( 21.53943276465977519, 0.05219959533937863772, 41.25109039468568284 ) ) ;
#114235=CARTESIAN_POINT ( 'NONE',  ( 5.049401038298161559, -19.05341960407611168, 112.7072429386476813 ) ) ;
#114236=CARTESIAN_POINT ( 'NONE',  ( -12.14591786802326823, 12.06949235617739902, 63.12609039468568994 ) ) ;
#114237=CARTESIAN_POINT ( 'NONE',  ( -14.29746914071049879, 8.314922557960819915, 30.83224293864770260 ) ) ;
#114238=CARTESIAN_POINT ( 'NONE',  ( -8.314922557961024197, 14.29746914071037800, 107.9177570613523471 ) ) ;
#114239=CARTESIAN_POINT ( 'NONE',  ( 0.05219959533934541429, -16.53943276465976808, 25.00109039468567218 ) ) ;
#114240=CARTESIAN_POINT ( 'NONE',  ( 19.02544592524343514, -5.153800228976328945, 43.54057627198103120 ) ) ;
#114241=CARTESIAN_POINT ( 'NONE',  ( 14.29746914071049879, -8.314922557960816363, 108.3322429386477097 ) ) ;
#114242=CARTESIAN_POINT ( 'NONE',  ( -21.53943276465977519, -0.05219959533937600094, 23.75109039468567929 ) ) ;
#114243=CARTESIAN_POINT ( 'NONE',  ( 0.05219959533909260263, 19.03943276465977164, 49.99890960531435979 ) ) ;
#114245=CARTESIAN_POINT ( 'NONE',  ( -9.564922557960796823, -16.46253265017161027, 27.08224293864769550 ) ) ;
#114247=CARTESIAN_POINT ( 'NONE',  ( -9.564922557960796823, -16.46253265017161027, 112.0822429386476955 ) ) ;
#114248=CARTESIAN_POINT ( 'NONE',  ( -17.50000000000001776, -5.622605283950791843, 36.31207310596109750 ) ) ;
#114249=CARTESIAN_POINT ( 'NONE',  ( -9.474510206698964154, 16.51473224551069663, 95.41557627198102409 ) ) ;
#114250=CARTESIAN_POINT ( 'NONE',  ( -5.823673210054431948, 21.52544592524334988, 42.70942372801901854 ) ) ;
#114251=CARTESIAN_POINT ( 'NONE',  ( 14.29746914071049879, -8.314922557960816363, 103.3322429386476955 ) ) ;
#114252=CARTESIAN_POINT ( 'NONE',  ( 19.03943276465977164, -0.05219959533909143690, 113.7489096053143669 ) ) ;
#114255=CARTESIAN_POINT ( 'NONE',  ( -12.06949235617739369, -12.14591786802326823, 84.37609039468570415 ) ) ;
#114256=CARTESIAN_POINT ( 'NONE',  ( 21.52544592524334988, 5.823673210054432836, 91.45942372801901854 ) ) ;
#114257=CARTESIAN_POINT ( 'NONE',  ( -12.14591786802326823, 12.06949235617739902, 58.12609039468568994 ) ) ;
#114258=CARTESIAN_POINT ( 'NONE',  ( -0.05219959533909027116, -19.03943276465977164, 92.49890960531436690 ) ) ;
#114260=CARTESIAN_POINT ( 'NONE',  ( 16.53943276465976808, 0.05219959533934440121, 46.25109039468567573 ) ) ;
#114261=CARTESIAN_POINT ( 'NONE',  ( 5.153800228976615827, -19.02544592524334988, 105.2094237280190185 ) ) ;
#114262=CARTESIAN_POINT ( 'NONE',  ( 4.379528057220092307, 16.55341960407617563, 77.29275706135234714 ) ) ;
#114263=CARTESIAN_POINT ( 'NONE',  ( -19.05341960407617563, 5.049401038297882671, 98.54275706135233293 ) ) ;
#114264=CARTESIAN_POINT ( 'NONE',  ( -16.51473224551069308, -9.474510206698971260, 71.66557627198102409 ) ) ;
#114265=CARTESIAN_POINT ( 'NONE',  ( -0.05219959533907301413, -21.53943276465977519, 97.49890960531436690 ) ) ;
#114266=CARTESIAN_POINT ( 'NONE',  ( -16.52544592524342804, 4.483927247898546575, 106.0405762719810525 ) ) ;
#114267=CARTESIAN_POINT ( 'NONE',  ( -19.03943276465977164, -0.05219959533935918106, 108.7510903946856615 ) ) ;
#114268=CARTESIAN_POINT ( 'NONE',  ( -14.34966873604972548, 8.224510206698743886, 73.33442372801901854 ) ) ;
#114270=CARTESIAN_POINT ( 'NONE',  ( -5.153800228976607833, 19.02544592524334988, 72.70942372801900433 ) ) ;
#114271=CARTESIAN_POINT ( 'NONE',  ( -8.314922557960811034, -14.29746914071050412, 37.08224293864768129 ) ) ;
#114272=CARTESIAN_POINT ( 'NONE',  ( -12.06949235617756955, 12.14591786802309770, 90.62390960531436690 ) ) ;
#114273=CARTESIAN_POINT ( 'NONE',  ( 5.153800228976615827, -19.02544592524334988, 30.20942372801900433 ) ) ;
#114275=CARTESIAN_POINT ( 'NONE',  ( 21.52544592524334988, 5.823673210054432836, 31.45942372801901854 ) ) ;
#114276=CARTESIAN_POINT ( 'NONE',  ( -9.564922557961040184, 16.46253265017147172, 92.91775706135233293 ) ) ;
#114278=CARTESIAN_POINT ( 'NONE',  ( -5.049401038298153566, 19.05341960407611168, 115.2072429386477097 ) ) ;
#114279=CARTESIAN_POINT ( 'NONE',  ( 5.049401038298161559, -19.05341960407611168, 87.70724293864769550 ) ) ;
#114280=CARTESIAN_POINT ( 'NONE',  ( -10.72451020669870658, -18.67979575497194134, 94.58442372801901854 ) ) ;
#114281=CARTESIAN_POINT ( 'NONE',  ( 5.153800228976335163, 19.02544592524342804, 74.79057627198103830 ) ) ;
#114282=CARTESIAN_POINT ( 'NONE',  ( -5.823673210054116645, -21.52544592524344225, 37.29057627198102409 ) ) ;
#114283=CARTESIAN_POINT ( 'NONE',  ( -14.34966873604960291, -8.224510206698953496, 91.66557627198103830 ) ) ;
#114284=CARTESIAN_POINT ( 'NONE',  ( 9.474510206698971260, -16.51473224551069308, 57.91557627198103120 ) ) ;
#114285=CARTESIAN_POINT ( 'NONE',  ( -13.97604488694527625, -13.89961937509977652, 21.87390960531435979 ) ) ;
#114286=VECTOR ( 'NONE', #6836, 1000.000000000000000 ) ;
#114287=CARTESIAN_POINT ( 'NONE',  ( 15.80617190586769283, -15.72974639402175789, 30.62609039468567929 ) ) ;
#114288=CARTESIAN_POINT ( 'NONE',  ( 10.81492255796106328, -18.62759615963255655, 60.41775706135235424 ) ) ;
#114289=CARTESIAN_POINT ( 'NONE',  ( -5.049401038298153566, 19.05341960407611168, 50.20724293864770260 ) ) ;
#114290=CARTESIAN_POINT ( 'NONE',  ( -14.29746914071037622, -8.314922557961029526, 79.16775706135234714 ) ) ;
#114291=CARTESIAN_POINT ( 'NONE',  ( 5.823673210054125526, 21.52544592524343514, 109.7905762719810383 ) ) ;
#114293=CARTESIAN_POINT ( 'NONE',  ( 10.81492255796106328, -18.62759615963255655, 25.41775706135235779 ) ) ;
#114294=CARTESIAN_POINT ( 'NONE',  ( 0.05219959533936267826, -19.03943276465977164, 50.00109039468566863 ) ) ;
#114295=CARTESIAN_POINT ( 'NONE',  ( -19.05341960407611168, -5.049401038298163336, 61.45724293864769550 ) ) ;
#114296=CARTESIAN_POINT ( 'NONE',  ( -13.89961937509957401, -13.97604488694547875, 34.37609039468566863 ) ) ;
#114297=CARTESIAN_POINT ( 'NONE',  ( 15.72974639402176855, 15.80617190586768217, 76.87609039468567573 ) ) ;
#114299=CARTESIAN_POINT ( 'NONE',  ( 18.62759615963271287, -10.81492255796078972, 73.33224293864769550 ) ) ;
#114300=CARTESIAN_POINT ( 'NONE',  ( -16.55341960407611168, -4.379528057220339221, 56.45724293864768839 ) ) ;
#114301=CARTESIAN_POINT ( 'NONE',  ( -10.81492255796105439, 18.62759615963255655, 92.91775706135236135 ) ) ;
#114302=CARTESIAN_POINT ( 'NONE',  ( 9.474510206698729675, 16.51473224551082808, 27.08442372801900433 ) ) ;
#114303=CARTESIAN_POINT ( 'NONE',  ( -14.34966873604960291, -8.224510206698953496, 66.66557627198102409 ) ) ;
#114304=CARTESIAN_POINT ( 'NONE',  ( -14.29746914071049879, 8.314922557960819915, 115.8322429386477097 ) ) ;
#114305=CARTESIAN_POINT ( 'NONE',  ( -19.03943276465977164, -0.05219959533935918106, 53.75109039468566863 ) ) ;
#114306=CARTESIAN_POINT ( 'NONE',  ( 4.379528057220339221, -16.55341960407611168, 27.70724293864769905 ) ) ;
#114307=CARTESIAN_POINT ( 'NONE',  ( 18.62759615963255655, 10.81492255796105972, 76.66775706135234714 ) ) ;
#114308=CARTESIAN_POINT ( 'NONE',  ( -19.05341960407617563, 5.049401038297882671, 43.54275706135232582 ) ) ;
#114309=CARTESIAN_POINT ( 'NONE',  ( 10.72451020669898902, -18.67979575497178502, 57.91557627198103120 ) ) ;
#114310=CARTESIAN_POINT ( 'NONE',  ( -0.05219959533937732626, 21.53943276465977519, 47.50109039468568994 ) ) ;
#114311=CARTESIAN_POINT ( 'NONE',  ( -15.72974639402197994, 15.80617190586746368, 95.62390960531436690 ) ) ;
#114312=CARTESIAN_POINT ( 'NONE',  ( 13.89961937509957401, 13.97604488694547697, 101.8760903946856331 ) ) ;
#114313=CARTESIAN_POINT ( 'NONE',  ( 0.05219959533934541429, -16.53943276465976808, 65.00109039468568994 ) ) ;
#114315=CARTESIAN_POINT ( 'NONE',  ( 15.72974639402199770, -15.80617190586745480, 103.1239096053143811 ) ) ;
#114316=CARTESIAN_POINT ( 'NONE',  ( 14.34966873604960469, 8.224510206698951720, 84.16557627198103830 ) ) ;
#114318=CARTESIAN_POINT ( 'NONE',  ( 16.52544592524335698, 4.483927247898782831, 36.45942372801901143 ) ) ;
#114319=CARTESIAN_POINT ( 'NONE',  ( -21.55341960407610458, -5.719274019375992779, 51.45724293864770260 ) ) ;
#114320=CARTESIAN_POINT ( 'NONE',  ( -12.14591786802326823, 12.06949235617739902, 93.12609039468568994 ) ) ;
#114321=CARTESIAN_POINT ( 'NONE',  ( -13.97604488694527625, -13.89961937509977652, 21.87390960531435979 ) ) ;
#114322=CARTESIAN_POINT ( 'NONE',  ( 14.29746914071037800, 8.314922557961029526, 71.66775706135234714 ) ) ;
#114323=CARTESIAN_POINT ( 'NONE',  ( -0.05219959533937732626, 21.53943276465977519, 42.50109039468567573 ) ) ;
#114324=CARTESIAN_POINT ( 'NONE',  ( -18.67979575497178146, -10.72451020669898902, 56.66557627198103830 ) ) ;
#114325=CARTESIAN_POINT ( 'NONE',  ( 12.14591786802327356, -12.06949235617739191, 90.62609039468567573 ) ) ;
#114326=CARTESIAN_POINT ( 'NONE',  ( -10.72451020669870658, -18.67979575497194134, 74.58442372801901854 ) ) ;
#114327=CARTESIAN_POINT ( 'NONE',  ( 18.62759615963271287, -10.81492255796078972, 48.33224293864770260 ) ) ;
#114328=CARTESIAN_POINT ( 'NONE',  ( 0.05219959533907565091, 21.53943276465977519, 34.99890960531435979 ) ) ;
#114330=CARTESIAN_POINT ( 'NONE',  ( -12.14591786802326823, 12.06949235617739902, 68.12609039468567573 ) ) ;
#114331=CARTESIAN_POINT ( 'NONE',  ( 18.67979575497178502, 10.72451020669898547, 39.16557627198102409 ) ) ;
#114333=CARTESIAN_POINT ( 'NONE',  ( -16.51473224551069308, -9.474510206698971260, 101.6655762719810241 ) ) ;
#114334=CARTESIAN_POINT ( 'NONE',  ( -8.314922557961024197, 14.29746914071037800, 112.9177570613523329 ) ) ;
#114336=CARTESIAN_POINT ( 'NONE',  ( 8.224510206698953496, -14.34966873604960469, 112.9155762719810383 ) ) ;
#114337=CARTESIAN_POINT ( 'NONE',  ( -10.72451020669898014, 18.67979575497178502, 45.41557627198103830 ) ) ;
#114338=CARTESIAN_POINT ( 'NONE',  ( 13.89961937509977652, -13.97604488694527269, 48.12390960531435979 ) ) ;
#114339=CARTESIAN_POINT ( 'NONE',  ( -14.34966873604972548, 8.224510206698743886, 93.33442372801901854 ) ) ;
#114340=CARTESIAN_POINT ( 'NONE',  ( -18.62759615963255300, -10.81492255796106328, 29.16775706135234003 ) ) ;
#114341=CARTESIAN_POINT ( 'NONE',  ( 13.97604488694548053, -13.89961937509957401, 95.62609039468563310 ) ) ;
#114342=CARTESIAN_POINT ( 'NONE',  ( 4.483927247898545687, 16.52544592524342804, 99.79057627198103830 ) ) ;
#114343=CARTESIAN_POINT ( 'NONE',  ( -16.51473224551069308, -9.474510206698971260, 56.66557627198103120 ) ) ;
#114344=CARTESIAN_POINT ( 'NONE',  ( 16.46253265017160672, -9.564922557960803928, 28.33224293864769550 ) ) ;
#114345=DIRECTION ( 'NONE',  ( 1.000000000000000000, -0.000000000000000000, -0.000000000000000000 ) ) ;
#114346=CARTESIAN_POINT ( 'NONE',  ( 5.049401038298161559, -19.05341960407611168, 72.70724293864768129 ) ) ;
#114347=CARTESIAN_POINT ( 'NONE',  ( 16.53943276465976808, 0.05219959533934440121, 66.25109039468567573 ) ) ;
#114348=CARTESIAN_POINT ( 'NONE',  ( -18.62759615963255300, -10.81492255796106328, 109.1677570613523613 ) ) ;
#114349=CARTESIAN_POINT ( 'NONE',  ( 15.72974639402199770, -15.80617190586745480, 48.12390960531436690 ) ) ;
#114350=CARTESIAN_POINT ( 'NONE',  ( 8.224510206698742110, 14.34966873604972548, 72.08442372801899012 ) ) ;
#114351=CARTESIAN_POINT ( 'NONE',  ( 5.153800228976615827, -19.02544592524334988, 70.20942372801899012 ) ) ;
#114353=CARTESIAN_POINT ( 'NONE',  ( -15.80617190586768217, 15.72974639402176855, 63.12609039468568994 ) ) ;
#114354=CARTESIAN_POINT ( 'NONE',  ( 13.97604488694527802, 13.89961937509977652, 64.37390960531436690 ) ) ;
#114355=CARTESIAN_POINT ( 'NONE',  ( 0.05219959533909260263, 19.03943276465977164, 34.99890960531435979 ) ) ;
#114356=CARTESIAN_POINT ( 'NONE',  ( -13.97604488694547697, 13.89961937509957934, 58.12609039468566863 ) ) ;
#114357=CARTESIAN_POINT ( 'NONE',  ( 16.51473224551069308, 9.474510206698969483, 109.1655762719810383 ) ) ;
#114358=CARTESIAN_POINT ( 'NONE',  ( -5.153800228976328057, -19.02544592524343514, 102.2905762719810383 ) ) ;
#114359=CARTESIAN_POINT ( 'NONE',  ( 4.379528057220339221, -16.55341960407611168, 52.70724293864769550 ) ) ;
#114360=CARTESIAN_POINT ( 'NONE',  ( 5.823673210054125526, 21.52544592524343514, 49.79057627198102409 ) ) ;
#114361=CARTESIAN_POINT ( 'NONE',  ( -17.50000000000002132, 4.658240926743188126, 103.9447041781680667 ) ) ;
#114362=CARTESIAN_POINT ( 'NONE',  ( 16.51473224551083163, -9.474510206698727899, 25.83442372801900078 ) ) ;
#114363=CARTESIAN_POINT ( 'NONE',  ( -19.03943276465977164, 0.05219959533909376836, 56.24890960531435979 ) ) ;
#114364=CARTESIAN_POINT ( 'NONE',  ( -18.89770734986049305, -5.499999999999956479, 99.10214472496639360 ) ) ;
#114366=CARTESIAN_POINT ( 'NONE',  ( -4.483927247898782831, 16.52544592524335698, 77.70942372801900433 ) ) ;
#114367=CARTESIAN_POINT ( 'NONE',  ( 21.53943276465977519, -0.05219959533907433946, 98.74890960531438111 ) ) ;
#114368=VECTOR ( 'NONE', #5141, 1000.000000000000000 ) ;
#114369=CARTESIAN_POINT ( 'NONE',  ( -19.05341960407611168, -5.049401038298163336, 46.45724293864768129 ) ) ;
#114370=FACE_OUTER_BOUND ( 'NONE', #99959, .T. ) ;
#114371=CARTESIAN_POINT ( 'NONE',  ( -5.719274019375665041, -21.55341960407619695, 39.79275706135235424 ) ) ;
#114372=CARTESIAN_POINT ( 'NONE',  ( 16.46253265017146816, 9.564922557961045513, 51.66775706135233293 ) ) ;
#114373=CARTESIAN_POINT ( 'NONE',  ( -5.153800228976328057, -19.02544592524343514, 47.29057627198102409 ) ) ;
#114374=CARTESIAN_POINT ( 'NONE',  ( 5.823673210054444382, -21.52544592524334988, 95.20942372801903275 ) ) ;
#114375=CARTESIAN_POINT ( 'NONE',  ( 16.21995358207304250, 7.366697692864176972, 97.56448998487843483 ) ) ;
#114376=CARTESIAN_POINT ( 'NONE',  ( -0.05219959533910754901, -16.53943276465976808, 47.49890960531435979 ) ) ;
#114378=CARTESIAN_POINT ( 'NONE',  ( 5.823673210054125526, 21.52544592524343514, 39.79057627198103830 ) ) ;
#114380=CARTESIAN_POINT ( 'NONE',  ( 19.02544592524343514, -5.153800228976328945, 103.5405762719809957 ) ) ;
#114381=CARTESIAN_POINT ( 'NONE',  ( 16.53943276465976808, -0.05219959533910856209, 88.74890960531436690 ) ) ;
#114382=CARTESIAN_POINT ( 'NONE',  ( -4.379528057220086978, -16.55341960407618274, 29.79275706135234358 ) ) ;
#114383=CARTESIAN_POINT ( 'NONE',  ( -14.29746914071037622, -8.314922557961029526, 104.1677570613523471 ) ) ;
#114386=B_SPLINE_CURVE_WITH_KNOTS ( 'NONE', 3,
 ( #120603, #148972, #197468, #133795, #181314, #106421, #121591, #195487, #182297, #43777, #103462, #164146, #180327, #183286, #56962, #165141, #28626, #44768, #26632, #168102, #102458, #25643, #42793, #87288, #88275, #118635, #149963, #104455, #167126, #11469, #73140, #134810 ),
 .UNSPECIFIED., .F., .F.,
 ( 4, 2, 2, 2, 2, 2, 2, 2, 2, 2, 2, 2, 2, 2, 2, 4 ),
 ( 1.346507514538369289E-17, 0.0003712461730036875911, 0.0007424923460073617381, 0.001113738519011035939, 0.001484984692014710032, 0.002227477038022060603, 0.002598723211025738382, 0.002969969384029416595, 0.003341215557033094807, 0.003712461730036773020, 0.004083707903040451233, 0.004454954076044129879, 0.004826200249047807658, 0.005197446422051485437, 0.005568692595055164084, 0.005939938768058842730 ),
 .UNSPECIFIED. ) ;
#114387=CARTESIAN_POINT ( 'NONE',  ( -19.02544592524342804, 5.153800228976336051, 96.04057627198103830 ) ) ;
#114388=CARTESIAN_POINT ( 'NONE',  ( 10.72451020669898902, -18.67979575497178502, 107.9155762719810241 ) ) ;
#114389=CARTESIAN_POINT ( 'NONE',  ( -14.34966873604972548, 8.224510206698743886, 113.3344237280190328 ) ) ;
#114390=CARTESIAN_POINT ( 'NONE',  ( -19.02544592524342804, 5.153800228976336051, 96.04057627198103830 ) ) ;
#114391=CARTESIAN_POINT ( 'NONE',  ( -19.03943276465977164, -0.05219959533935918106, 98.75109039468567573 ) ) ;
#114392=CARTESIAN_POINT ( 'NONE',  ( -5.823673210054431948, 21.52544592524334988, 112.7094237280190328 ) ) ;
#114393=CARTESIAN_POINT ( 'NONE',  ( -15.72974639402197994, 15.80617190586746368, 90.62390960531436690 ) ) ;
#114394=CARTESIAN_POINT ( 'NONE',  ( 18.62759615963271287, -10.81492255796078972, 48.33224293864770260 ) ) ;
#114396=CARTESIAN_POINT ( 'NONE',  ( 5.153800228976335163, 19.02544592524342804, 59.79057627198100988 ) ) ;
#114397=CARTESIAN_POINT ( 'NONE',  ( 4.379528057220339221, -16.55341960407611168, 37.70724293864769550 ) ) ;
#114398=CARTESIAN_POINT ( 'NONE',  ( -9.564922557960796823, -16.46253265017161027, 72.08224293864770971 ) ) ;
#114399=ORIENTED_EDGE ( 'NONE', *, *, #38764, .T. ) ;
#114400=CARTESIAN_POINT ( 'NONE',  ( 19.02130022317636104, -5.499999999999802824, 63.28188669246573284 ) ) ;
#114401=CARTESIAN_POINT ( 'NONE',  ( 16.51473224551083163, -9.474510206698727899, 40.83442372801900433 ) ) ;
#114402=CARTESIAN_POINT ( 'NONE',  ( 14.29746914071049879, -8.314922557960816363, 88.33224293864769550 ) ) ;
#114403=CARTESIAN_POINT ( 'NONE',  ( -21.52544592524334988, -5.823673210054445271, 28.95942372801902209 ) ) ;
#114405=CARTESIAN_POINT ( 'NONE',  ( -8.314922557961024197, 14.29746914071037800, 107.9177570613523471 ) ) ;
#114406=CARTESIAN_POINT ( 'NONE',  ( 14.29746914071049879, -8.314922557960816363, 113.3322429386476955 ) ) ;
#114407=CARTESIAN_POINT ( 'NONE',  ( -19.05341960407611168, -5.049401038298163336, 66.45724293864769550 ) ) ;
#114409=CARTESIAN_POINT ( 'NONE',  ( 12.14591786802309770, 12.06949235617756955, 49.37390960531436690 ) ) ;
#114411=CARTESIAN_POINT ( 'NONE',  ( -10.81492255796105439, 18.62759615963255655, 62.91775706135236135 ) ) ;
#114413=CARTESIAN_POINT ( 'NONE',  ( 5.823673210054444382, -21.52544592524334988, 90.20942372801903275 ) ) ;
#114414=CARTESIAN_POINT ( 'NONE',  ( -0.05219959533909027116, -19.03943276465977164, 37.49890960531436690 ) ) ;
#114415=CARTESIAN_POINT ( 'NONE',  ( -13.89961937509977652, 13.97604488694528158, 45.62390960531433848 ) ) ;
#114416=ORIENTED_EDGE ( 'NONE', *, *, #46491, .F. ) ;
#114417=CARTESIAN_POINT ( 'NONE',  ( 0.05219959533937995610, -21.53943276465977519, 90.00109039468567573 ) ) ;
#114418=CARTESIAN_POINT ( 'NONE',  ( -12.14591786802326823, 12.06949235617739902, 58.12609039468568994 ) ) ;
#114419=CARTESIAN_POINT ( 'NONE',  ( 10.81492255796106328, -18.62759615963255655, 85.41775706135236135 ) ) ;
#114420=CARTESIAN_POINT ( 'NONE',  ( 10.72451020669898902, -18.67979575497178502, 27.91557627198103830 ) ) ;
#114421=CARTESIAN_POINT ( 'NONE',  ( -19.02544592524334988, -5.153800228976617603, 98.95942372801900433 ) ) ;
#114422=CARTESIAN_POINT ( 'NONE',  ( -5.719274019375665041, -21.55341960407619695, 64.79275706135234714 ) ) ;
#114423=CARTESIAN_POINT ( 'NONE',  ( -12.06949235617739369, -12.14591786802326823, 39.37609039468567573 ) ) ;
#114424=CARTESIAN_POINT ( 'NONE',  ( 15.72974639402199770, -15.80617190586745480, 88.12390960531436690 ) ) ;
#114425=CARTESIAN_POINT ( 'NONE',  ( 19.03943276465977164, 0.05219959533936151252, 101.2510903946856757 ) ) ;
#114426=CARTESIAN_POINT ( 'NONE',  ( -16.51473224551069308, -9.474510206698971260, 61.66557627198103120 ) ) ;
#114427=CARTESIAN_POINT ( 'NONE',  ( 16.51473224551083163, -9.474510206698727899, 100.8344237280190043 ) ) ;
#114429=CARTESIAN_POINT ( 'NONE',  ( 16.46253265017146816, 9.564922557961045513, 96.66775706135233293 ) ) ;
#114430=CARTESIAN_POINT ( 'NONE',  ( -8.314922557960811034, -14.29746914071050412, 57.08224293864769550 ) ) ;
#114431=CARTESIAN_POINT ( 'NONE',  ( 13.89961937509957401, 13.97604488694547697, 71.87609039468567573 ) ) ;
#114432=CARTESIAN_POINT ( 'NONE',  ( 16.55341960407618274, -4.379528057220086978, 66.04275706135236135 ) ) ;
#114433=CARTESIAN_POINT ( 'NONE',  ( -21.52544592524343514, 5.823673210054127303, 116.0405762719810383 ) ) ;
#114434=CARTESIAN_POINT ( 'NONE',  ( 9.564922557960805705, 16.46253265017160317, 39.58224293864768839 ) ) ;
#114435=CARTESIAN_POINT ( 'NONE',  ( 9.474510206698971260, -16.51473224551069308, 57.91557627198103120 ) ) ;
#114436=CARTESIAN_POINT ( 'NONE',  ( 12.14591786802327356, -12.06949235617739191, 65.62609039468568994 ) ) ;
#114439=CARTESIAN_POINT ( 'NONE',  ( 9.564922557960805705, 16.46253265017160317, 109.5822429386476955 ) ) ;
#114440=CARTESIAN_POINT ( 'NONE',  ( -19.05341960407611168, -5.049401038298163336, 21.45724293864768839 ) ) ;
#114442=CARTESIAN_POINT ( 'NONE',  ( -9.564922557961040184, 16.46253265017147172, 112.9177570613523329 ) ) ;
#114443=CARTESIAN_POINT ( 'NONE',  ( -21.52544592524343514, 5.823673210054127303, 41.04057627198103120 ) ) ;
#114444=CARTESIAN_POINT ( 'NONE',  ( 16.46253265017146816, 9.564922557961045513, 26.66775706135234003 ) ) ;
#114445=CARTESIAN_POINT ( 'NONE',  ( -16.53943276465976808, -0.05219959533934237506, 33.75109039468568284 ) ) ;
#114446=CARTESIAN_POINT ( 'NONE',  ( -5.153800228976328057, -19.02544592524343514, 32.29057627198102409 ) ) ;
#114447=CARTESIAN_POINT ( 'NONE',  ( -16.51473224551069308, -9.474510206698971260, 46.66557627198102409 ) ) ;
#114448=CARTESIAN_POINT ( 'NONE',  ( -18.67979575497178146, -10.72451020669898902, 81.66557627198103830 ) ) ;
#114449=CARTESIAN_POINT ( 'NONE',  ( 19.03943276465977164, -0.05219959533909143690, 98.74890960531436690 ) ) ;
#114450=CARTESIAN_POINT ( 'NONE',  ( -5.049401038298153566, 19.05341960407611168, 55.20724293864769550 ) ) ;
#114452=CARTESIAN_POINT ( 'NONE',  ( 5.049401038297881783, 19.05341960407617563, 82.29275706135229029 ) ) ;
#114453=CARTESIAN_POINT ( 'NONE',  ( 12.06949235617757843, -12.14591786802309237, 73.12390960531436690 ) ) ;
#114454=CARTESIAN_POINT ( 'NONE',  ( 15.80617190586769283, -15.72974639402175789, 100.6260903946857184 ) ) ;
#114455=CARTESIAN_POINT ( 'NONE',  ( 15.72974639402199770, -15.80617190586745480, 103.1239096053143811 ) ) ;
#114456=CARTESIAN_POINT ( 'NONE',  ( -15.72974639402176322, -15.80617190586768395, 79.37609039468567573 ) ) ;
#114457=CARTESIAN_POINT ( 'NONE',  ( 21.55341960407619695, -5.719274019375665929, 76.04275706135237556 ) ) ;
#114458=CARTESIAN_POINT ( 'NONE',  ( -16.51473224551069308, -9.474510206698971260, 111.6655762719810383 ) ) ;
#114459=CARTESIAN_POINT ( 'NONE',  ( -16.53943276465976808, -0.05219959533934237506, 108.7510903946857042 ) ) ;
#114460=CARTESIAN_POINT ( 'NONE',  ( 10.72451020669871369, 18.67979575497193778, 82.08442372801901854 ) ) ;
#114461=CARTESIAN_POINT ( 'NONE',  ( -16.46253265017160317, 9.564922557960807481, 60.83224293864769550 ) ) ;
#114462=CARTESIAN_POINT ( 'NONE',  ( -21.52544592524334988, -5.823673210054445271, 48.95942372801902565 ) ) ;
#114463=CARTESIAN_POINT ( 'NONE',  ( -13.97604488694527625, -13.89961937509977652, 86.87390960531436690 ) ) ;
#114464=CARTESIAN_POINT ( 'NONE',  ( -8.224510206698948167, 14.34966873604960824, 75.41557627198102409 ) ) ;
#114465=CARTESIAN_POINT ( 'NONE',  ( 16.52544592524342804, -4.483927247898539470, 53.54057627198103120 ) ) ;
#114466=CARTESIAN_POINT ( 'NONE',  ( -10.72451020669898014, 18.67979575497178502, 55.41557627198102409 ) ) ;
#114467=CARTESIAN_POINT ( 'NONE',  ( -5.049401038298153566, 19.05341960407611168, 55.20724293864769550 ) ) ;
#114468=CARTESIAN_POINT ( 'NONE',  ( 10.72451020669898902, -18.67979575497178502, 67.91557627198102409 ) ) ;
#114469=CARTESIAN_POINT ( 'NONE',  ( 9.474510206698729675, 16.51473224551082808, 67.08442372801900433 ) ) ;
#114471=CARTESIAN_POINT ( 'NONE',  ( -16.55341960407611168, -4.379528057220339221, 71.45724293864769550 ) ) ;
#114472=CARTESIAN_POINT ( 'NONE',  ( 21.55341960407610458, 5.719274019375980345, 58.95724293864770971 ) ) ;
#114473=VERTEX_POINT ( 'NONE', #76191 ) ;
#114474=DIRECTION ( 'NONE',  ( -1.000000000000000000, -0.000000000000000000, -0.000000000000000000 ) ) ;
#114475=CARTESIAN_POINT ( 'NONE',  ( -4.483927247898782831, 16.52544592524335698, 102.7094237280190185 ) ) ;
#114477=CARTESIAN_POINT ( 'NONE',  ( 16.46253265017146816, 9.564922557961045513, 91.66775706135234714 ) ) ;
#114478=CARTESIAN_POINT ( 'NONE',  ( 4.483927247898545687, 16.52544592524342804, 64.79057627198103830 ) ) ;
#114480=CARTESIAN_POINT ( 'NONE',  ( 19.02544592524343514, -5.153800228976328945, 58.54057627198102409 ) ) ;
#114481=CARTESIAN_POINT ( 'NONE',  ( 8.314922557960818139, 14.29746914071049879, 59.58224293864770260 ) ) ;
#114482=CARTESIAN_POINT ( 'NONE',  ( 9.564922557960805705, 16.46253265017160317, 89.58224293864769550 ) ) ;
#114484=CARTESIAN_POINT ( 'NONE',  ( -5.153800228976607833, 19.02544592524334988, 77.70942372801900433 ) ) ;
#114485=CARTESIAN_POINT ( 'NONE',  ( -9.474510206698964154, 16.51473224551069663, 55.41557627198103120 ) ) ;
#114486=CARTESIAN_POINT ( 'NONE',  ( 5.153800228976335163, 19.02544592524342804, 84.79057627198099567 ) ) ;
#114487=CARTESIAN_POINT ( 'NONE',  ( -9.564922557960796823, -16.46253265017161027, 67.08224293864769550 ) ) ;
#114489=CARTESIAN_POINT ( 'NONE',  ( -18.62759615963270932, 10.81492255796079327, 60.83224293864769550 ) ) ;
#114490=CARTESIAN_POINT ( 'NONE',  ( -12.06949235617739369, -12.14591786802326823, 64.37609039468568994 ) ) ;
#114492=CARTESIAN_POINT ( 'NONE',  ( 5.153800228976335163, 19.02544592524342804, 54.79057627198103120 ) ) ;
#114493=CARTESIAN_POINT ( 'NONE',  ( -10.81492255796078084, -18.62759615963271287, 57.08224293864769550 ) ) ;
#114494=CARTESIAN_POINT ( 'NONE',  ( 5.153800228976615827, -19.02544592524334988, 75.20942372801896170 ) ) ;
#114495=CARTESIAN_POINT ( 'NONE',  ( -8.224510206698948167, 14.34966873604960824, 30.41557627198101699 ) ) ;
#114496=CARTESIAN_POINT ( 'NONE',  ( -16.46253265017146816, -9.564922557961047289, 39.16775706135234003 ) ) ;
#114497=CARTESIAN_POINT ( 'NONE',  ( -14.34966873604972548, 8.224510206698743886, 58.33442372801901143 ) ) ;
#114498=CARTESIAN_POINT ( 'NONE',  ( 16.52544592524335698, 4.483927247898782831, 96.45942372801901854 ) ) ;
#114499=CARTESIAN_POINT ( 'NONE',  ( -18.10062525802553424, 5.500000000000031086, 53.51383468041920111 ) ) ;
#114500=CARTESIAN_POINT ( 'NONE',  ( 14.34966873604972726, -8.224510206698740333, 85.83442372801901854 ) ) ;
#114501=CARTESIAN_POINT ( 'NONE',  ( 5.823673210054125526, 21.52544592524343514, 24.79057627198103120 ) ) ;
#114502=CARTESIAN_POINT ( 'NONE',  ( -5.049401038298153566, 19.05341960407611168, 40.20724293864768839 ) ) ;
#114503=CARTESIAN_POINT ( 'NONE',  ( -16.46253265017160317, 9.564922557960807481, 50.83224293864770260 ) ) ;
#114504=CARTESIAN_POINT ( 'NONE',  ( -19.05341960407611168, -5.049401038298163336, 41.45724293864769550 ) ) ;
#114505=CARTESIAN_POINT ( 'NONE',  ( -18.62759615963255300, -10.81492255796106328, 34.16775706135234714 ) ) ;
#114506=CARTESIAN_POINT ( 'NONE',  ( -4.379528057220086978, -16.55341960407618274, 54.79275706135235424 ) ) ;
#114507=CARTESIAN_POINT ( 'NONE',  ( 16.55341960407618274, -4.379528057220086978, 111.0427570613523613 ) ) ;
#114508=CARTESIAN_POINT ( 'NONE',  ( -9.474510206698964154, 16.51473224551069663, 25.41557627198103120 ) ) ;
#114509=CARTESIAN_POINT ( 'NONE',  ( -19.02544592524334988, -5.153800228976617603, 18.95942372801899722 ) ) ;
#114510=CARTESIAN_POINT ( 'NONE',  ( -16.51473224551082808, 9.474510206698731452, 108.3344237280190043 ) ) ;
#114512=CARTESIAN_POINT ( 'NONE',  ( 13.97604488694548053, -13.89961937509957401, 70.62609039468567573 ) ) ;
#114513=CARTESIAN_POINT ( 'NONE',  ( -16.52544592524342804, 4.483927247898546575, 66.04057627198103830 ) ) ;
#114514=CARTESIAN_POINT ( 'NONE',  ( -19.02544592524342804, 5.153800228976336051, 41.04057627198103120 ) ) ;
#114515=CARTESIAN_POINT ( 'NONE',  ( -19.05341960407617563, 5.049401038297882671, 78.54275706135233293 ) ) ;
#114517=CARTESIAN_POINT ( 'NONE',  ( -0.05219959533937732626, 21.53943276465977519, 72.50109039468568994 ) ) ;
#114518=CARTESIAN_POINT ( 'NONE',  ( 8.224510206698742110, 14.34966873604972548, 47.08442372801901854 ) ) ;
#114519=CARTESIAN_POINT ( 'NONE',  ( 18.87075004821571156, -5.499999999999887201, 56.17408112101048800 ) ) ;
#114520=CARTESIAN_POINT ( 'NONE',  ( -18.67979575497178146, -10.72451020669898902, 36.66557627198103120 ) ) ;
#114521=CARTESIAN_POINT ( 'NONE',  ( 16.55341960407618274, -4.379528057220086978, 31.04275706135234714 ) ) ;
#114523=CARTESIAN_POINT ( 'NONE',  ( 5.153800228976615827, -19.02544592524334988, 20.20942372801899722 ) ) ;
#114525=CARTESIAN_POINT ( 'NONE',  ( -0.05219959533909027116, -19.03943276465977164, 42.49890960531435269 ) ) ;
#114526=CARTESIAN_POINT ( 'NONE',  ( 16.46253265017146816, 9.564922557961045513, 56.66775706135233293 ) ) ;
#114527=CARTESIAN_POINT ( 'NONE',  ( -0.05219959533909027116, -19.03943276465977164, 62.49890960531435979 ) ) ;
#114528=CARTESIAN_POINT ( 'NONE',  ( -15.72974639402176322, -15.80617190586768395, 69.37609039468567573 ) ) ;
#114529=CARTESIAN_POINT ( 'NONE',  ( 16.51473224551083163, -9.474510206698727899, 20.83442372801899722 ) ) ;
#114530=CARTESIAN_POINT ( 'NONE',  ( -4.379528057220328563, 16.55341960407611168, 25.20724293864769550 ) ) ;
#114531=CARTESIAN_POINT ( 'NONE',  ( -5.049401038298153566, 19.05341960407611168, 30.20724293864768839 ) ) ;
#114533=CARTESIAN_POINT ( 'NONE',  ( 19.05341960407611168, 5.049401038298154454, 88.95724293864769550 ) ) ;
#114534=CARTESIAN_POINT ( 'NONE',  ( 21.52544592524334988, 5.823673210054432836, 56.45942372801902565 ) ) ;
#114535=CARTESIAN_POINT ( 'NONE',  ( 19.05341960407611168, 5.049401038298154454, 43.95724293864769550 ) ) ;
#114536=CARTESIAN_POINT ( 'NONE',  ( -15.80617190586768217, 15.72974639402176855, 68.12609039468567573 ) ) ;
#114537=CARTESIAN_POINT ( 'NONE',  ( 19.03943276465977164, 0.05219959533936151252, 91.25109039468566152 ) ) ;
#114538=CARTESIAN_POINT ( 'NONE',  ( -5.049401038298153566, 19.05341960407611168, 105.2072429386476671 ) ) ;
#114539=CARTESIAN_POINT ( 'NONE',  ( 8.224510206698953496, -14.34966873604960469, 112.9155762719810383 ) ) ;
#114540=CARTESIAN_POINT ( 'NONE',  ( -10.72451020669898014, 18.67979575497178502, 110.4155762719810383 ) ) ;
#114541=CARTESIAN_POINT ( 'NONE',  ( 9.564922557961047289, -16.46253265017146816, 40.41775706135234003 ) ) ;
#114542=CARTESIAN_POINT ( 'NONE',  ( -16.53943276465976808, 0.05219959533911058130, 111.2489096053143669 ) ) ;
#114543=CARTESIAN_POINT ( 'NONE',  ( 19.03943276465977164, -0.05219959533909143690, 58.74890960531435979 ) ) ;
#114544=CARTESIAN_POINT ( 'NONE',  ( -16.51473224551082808, 9.474510206698731452, 103.3344237280190043 ) ) ;
#114546=CARTESIAN_POINT ( 'NONE',  ( -14.29746914071049879, 8.314922557960819915, 60.83224293864769550 ) ) ;
#114547=CARTESIAN_POINT ( 'NONE',  ( 5.153800228976615827, -19.02544592524334988, 25.20942372801900433 ) ) ;
#114548=CARTESIAN_POINT ( 'NONE',  ( -9.474510206698964154, 16.51473224551069663, 115.4155762719810241 ) ) ;
#114549=CARTESIAN_POINT ( 'NONE',  ( 0.05219959533936267826, -19.03943276465977164, 90.00109039468567573 ) ) ;
#114550=CARTESIAN_POINT ( 'NONE',  ( -5.719274019375978568, 21.55341960407610458, 95.20724293864769550 ) ) ;
#114551=CARTESIAN_POINT ( 'NONE',  ( 10.72451020669871369, 18.67979575497193778, 47.08442372801901854 ) ) ;
#114552=B_SPLINE_CURVE_WITH_KNOTS ( 'NONE', 3,
 ( #19268, #81887, #157777, #36397, #190104, #155774 ),
 .UNSPECIFIED., .F., .F.,
 ( 4, 2, 4 ),
 ( 0.003989672132298030700, 0.004372778065220456548, 0.004755883998142883262 ),
 .UNSPECIFIED. ) ;
#114553=CARTESIAN_POINT ( 'NONE',  ( 14.34966873604972726, -8.224510206698740333, 40.83442372801901854 ) ) ;
#114554=CARTESIAN_POINT ( 'NONE',  ( -16.53943276465976808, -0.05219959533934237506, 108.7510903946857042 ) ) ;
#114555=CARTESIAN_POINT ( 'NONE',  ( 16.55341960407618274, -4.379528057220086978, 41.04275706135236135 ) ) ;
#114556=CARTESIAN_POINT ( 'NONE',  ( -5.719274019375665041, -21.55341960407619695, 44.79275706135234714 ) ) ;
#114557=CARTESIAN_POINT ( 'NONE',  ( -10.72451020669898014, 18.67979575497178502, 55.41557627198102409 ) ) ;
#114559=CARTESIAN_POINT ( 'NONE',  ( 13.97604488694527802, 13.89961937509977652, 39.37390960531435269 ) ) ;
#114561=CARTESIAN_POINT ( 'NONE',  ( -16.55341960407617563, 4.379528057220093196, 73.54275706135234714 ) ) ;
#114562=CARTESIAN_POINT ( 'NONE',  ( -21.55341960407610458, -5.719274019375992779, 91.45724293864769550 ) ) ;
#114563=CARTESIAN_POINT ( 'NONE',  ( -4.379528057220328563, 16.55341960407611168, 35.20724293864768839 ) ) ;
#114564=CARTESIAN_POINT ( 'NONE',  ( -8.224510206698735004, -14.34966873604973081, 64.58442372801900433 ) ) ;
#114565=CARTESIAN_POINT ( 'NONE',  ( 0.05219959533936267826, -19.03943276465977164, 105.0010903946856615 ) ) ;
#114566=CARTESIAN_POINT ( 'NONE',  ( 21.55341960407610458, 5.719274019375980345, 103.9572429386476813 ) ) ;
#114567=CARTESIAN_POINT ( 'NONE',  ( -14.29746914071049879, 8.314922557960819915, 25.83224293864769194 ) ) ;
#114569=CARTESIAN_POINT ( 'NONE',  ( -4.379528057220086978, -16.55341960407618274, 84.79275706135234714 ) ) ;
#114571=CARTESIAN_POINT ( 'NONE',  ( 18.62759615963271287, -10.81492255796078972, 73.33224293864769550 ) ) ;
#114572=CARTESIAN_POINT ( 'NONE',  ( 14.34966873604972726, -8.224510206698740333, 100.8344237280190185 ) ) ;
#114574=CARTESIAN_POINT ( 'NONE',  ( 19.19724070472095434, 5.499999999999968026, 88.56193348274382515 ) ) ;
#114575=CARTESIAN_POINT ( 'NONE',  ( -15.72974639402197994, 15.80617190586746368, 105.6239096053143669 ) ) ;
#114576=CARTESIAN_POINT ( 'NONE',  ( -10.81492255796078084, -18.62759615963271287, 112.0822429386477097 ) ) ;
#114577=CARTESIAN_POINT ( 'NONE',  ( -16.53943276465976808, 0.05219959533911058130, 36.24890960531435979 ) ) ;
#114578=CIRCLE ( 'NONE', #66227, 2.500000000000002220 ) ;
#114579=CARTESIAN_POINT ( 'NONE',  ( 4.379528057220092307, 16.55341960407617563, 32.29275706135235424 ) ) ;
#114580=CARTESIAN_POINT ( 'NONE',  ( 13.89961937509977652, -13.97604488694527269, 43.12390960531434558 ) ) ;
#114581=CARTESIAN_POINT ( 'NONE',  ( -19.03943276465977164, 0.05219959533909376836, 61.24890960531436690 ) ) ;
#114583=CARTESIAN_POINT ( 'NONE',  ( 21.52544592524344225, -5.823673210054117533, 23.54057627198102765 ) ) ;
#114584=DIRECTION ( 'NONE',  ( -1.000000000000000000, -0.000000000000000000, 0.000000000000000000 ) ) ;
#114585=CARTESIAN_POINT ( 'NONE',  ( -19.03943276465977164, -0.05219959533935918106, 103.7510903946856757 ) ) ;
#114586=CARTESIAN_POINT ( 'NONE',  ( 19.03943276465977164, 0.05219959533936151252, 56.25109039468566863 ) ) ;
#114587=CARTESIAN_POINT ( 'NONE',  ( 10.72451020669898902, -18.67979575497178502, 87.91557627198103830 ) ) ;
#114588=CARTESIAN_POINT ( 'NONE',  ( -12.14591786802326823, 12.06949235617739902, 108.1260903946856757 ) ) ;
#114589=CARTESIAN_POINT ( 'NONE',  ( -18.62759615963270932, 10.81492255796079327, 45.83224293864769550 ) ) ;
#114590=CARTESIAN_POINT ( 'NONE',  ( -15.72974639402197994, 15.80617190586746368, 80.62390960531438111 ) ) ;
#114591=CARTESIAN_POINT ( 'NONE',  ( 19.05341960407617918, -5.049401038297876454, 101.0427570613523045 ) ) ;
#114592=CARTESIAN_POINT ( 'NONE',  ( 21.53943276465977519, -0.05219959533907433946, 28.74890960531435624 ) ) ;
#114593=CARTESIAN_POINT ( 'NONE',  ( 15.72974639402176855, 15.80617190586768217, 76.87609039468567573 ) ) ;
#114594=CARTESIAN_POINT ( 'NONE',  ( 13.97604488694527802, 13.89961937509977652, 79.37390960531435269 ) ) ;
#114596=CARTESIAN_POINT ( 'NONE',  ( 19.05341960407611168, 5.049401038298154454, 68.95724293864769550 ) ) ;
#114597=CARTESIAN_POINT ( 'NONE',  ( -12.14591786802309592, -12.06949235617757132, 86.87390960531438111 ) ) ;
#114598=ORIENTED_EDGE ( 'NONE', *, *, #90799, .T. ) ;
#114599=CARTESIAN_POINT ( 'NONE',  ( -13.89961937509957401, -13.97604488694547875, 109.3760903946856331 ) ) ;
#114601=CARTESIAN_POINT ( 'NONE',  ( 9.474510206698971260, -16.51473224551069308, 77.91557627198103830 ) ) ;
#114602=CARTESIAN_POINT ( 'NONE',  ( 10.81492255796106328, -18.62759615963255655, 90.41775706135236135 ) ) ;
#114603=CARTESIAN_POINT ( 'NONE',  ( 13.97604488694527802, 13.89961937509977652, 94.37390960531436690 ) ) ;
#114604=CARTESIAN_POINT ( 'NONE',  ( -0.05219959533934338120, 16.53943276465976808, 82.50109039468568994 ) ) ;
#114606=CARTESIAN_POINT ( 'NONE',  ( -13.97604488694547697, 13.89961937509957934, 63.12609039468566152 ) ) ;
#114607=CARTESIAN_POINT ( 'NONE',  ( -19.02544592524334988, -5.153800228976617603, 23.95942372801900078 ) ) ;
#114610=CARTESIAN_POINT ( 'NONE',  ( -14.34966873604972548, 8.224510206698743886, 113.3344237280190328 ) ) ;
#114611=CARTESIAN_POINT ( 'NONE',  ( -17.49999999999999645, -5.500000000000000000, 111.2823096230356725 ) ) ;
#114612=CARTESIAN_POINT ( 'NONE',  ( 8.224510206698742110, 14.34966873604972548, 107.0844237280190043 ) ) ;
#114613=CARTESIAN_POINT ( 'NONE',  ( 17.48853670773247515, 5.747243402303057636, 68.83328700250008580 ) ) ;
#114614=CARTESIAN_POINT ( 'NONE',  ( 16.53943276465976808, 0.05219959533934440121, 81.25109039468568994 ) ) ;
#114615=CARTESIAN_POINT ( 'NONE',  ( -21.52544592524334988, -5.823673210054445271, 78.95942372801901854 ) ) ;
#114616=CARTESIAN_POINT ( 'NONE',  ( -5.153800228976607833, 19.02544592524334988, 87.70942372801897591 ) ) ;
#114617=CARTESIAN_POINT ( 'NONE',  ( -5.049401038297874678, -19.05341960407617918, 44.79275706135232582 ) ) ;
#114619=CARTESIAN_POINT ( 'NONE',  ( -19.03943276465977164, 0.05219959533909376836, 81.24890960531436690 ) ) ;
#114620=CARTESIAN_POINT ( 'NONE',  ( 0.05219959533909260263, 19.03943276465977164, 59.99890960531436690 ) ) ;
#114621=CARTESIAN_POINT ( 'NONE',  ( 18.22780087662114212, -5.499999999999987566, 41.01540105326107977 ) ) ;
#114622=CARTESIAN_POINT ( 'NONE',  ( -21.52544592524343514, 5.823673210054127303, 101.0405762719810383 ) ) ;
#114623=EDGE_CURVE ( 'NONE', #82599, #9179, #148459, .T. ) ;
#114624=CARTESIAN_POINT ( 'NONE',  ( 10.72451020669898902, -18.67979575497178502, 52.91557627198103830 ) ) ;
#114625=CARTESIAN_POINT ( 'NONE',  ( 9.564922557960805705, 16.46253265017160317, 34.58224293864770260 ) ) ;
#114626=CARTESIAN_POINT ( 'NONE',  ( 4.483927247898790824, -16.52544592524335698, 60.20942372801902565 ) ) ;
#114629=CARTESIAN_POINT ( 'NONE',  ( -21.53943276465977519, -0.05219959533937600094, 43.75109039468568284 ) ) ;
#114630=CARTESIAN_POINT ( 'NONE',  ( -4.483927247898539470, -16.52544592524342804, 72.29057627198102409 ) ) ;
#114632=CARTESIAN_POINT ( 'NONE',  ( -14.29746914071037622, -8.314922557961029526, 39.16775706135235424 ) ) ;
#114633=CARTESIAN_POINT ( 'NONE',  ( -12.14591786802309592, -12.06949235617757132, 96.87390960531436690 ) ) ;
#114634=CARTESIAN_POINT ( 'NONE',  ( -16.51473224551082808, 9.474510206698731452, 48.33442372801900433 ) ) ;
#114635=CARTESIAN_POINT ( 'NONE',  ( 16.52544592524342804, -4.483927247898539470, 58.54057627198103120 ) ) ;
#114636=CARTESIAN_POINT ( 'NONE',  ( -18.62759615963255300, -10.81492255796106328, 34.16775706135234714 ) ) ;
#114637=EDGE_CURVE ( 'NONE', #144727, #170830, #27804, .T. ) ;
#114639=CARTESIAN_POINT ( 'NONE',  ( 0.05219959533907565091, 21.53943276465977519, 84.99890960531436690 ) ) ;
#114640=CARTESIAN_POINT ( 'NONE',  ( -19.03943276465977164, 0.05219959533909376836, 106.2489096053143669 ) ) ;
#114641=CARTESIAN_POINT ( 'NONE',  ( 14.34966873604960469, 8.224510206698951720, 79.16557627198103830 ) ) ;
#114644=CARTESIAN_POINT ( 'NONE',  ( -13.97604488694547697, 13.89961937509957934, 88.12609039468563310 ) ) ;
#114645=CARTESIAN_POINT ( 'NONE',  ( 18.67979575497194134, -10.72451020669871369, 20.83442372801901143 ) ) ;
#114646=CARTESIAN_POINT ( 'NONE',  ( 0.05219959533909260263, 19.03943276465977164, 74.99890960531435269 ) ) ;
#114647=CARTESIAN_POINT ( 'NONE',  ( 19.02544592524334988, 5.153800228976608722, 61.45942372801900433 ) ) ;
#114648=CARTESIAN_POINT ( 'NONE',  ( 5.049401038298161559, -19.05341960407611168, 37.70724293864768839 ) ) ;
#114649=CARTESIAN_POINT ( 'NONE',  ( -15.72974639402176322, -15.80617190586768395, 79.37609039468567573 ) ) ;
#114651=CARTESIAN_POINT ( 'NONE',  ( -12.06949235617756955, 12.14591786802309770, 60.62390960531437401 ) ) ;
#114652=CARTESIAN_POINT ( 'NONE',  ( -19.05341960407611168, -5.049401038298163336, 66.45724293864769550 ) ) ;
#114654=CARTESIAN_POINT ( 'NONE',  ( -10.72451020669898014, 18.67979575497178502, 85.41557627198102409 ) ) ;
#114655=CARTESIAN_POINT ( 'NONE',  ( 16.51473224551069308, 9.474510206698969483, 54.16557627198103120 ) ) ;
#114657=CARTESIAN_POINT ( 'NONE',  ( -5.719274019375978568, 21.55341960407610458, 75.20724293864769550 ) ) ;
#114658=EDGE_CURVE ( 'NONE', #137960, #138821, #22490, .T. ) ;
#114659=CARTESIAN_POINT ( 'NONE',  ( 15.72974639402176855, 15.80617190586768217, 96.87609039468568994 ) ) ;
#114660=CARTESIAN_POINT ( 'NONE',  ( 16.46253265017160672, -9.564922557960803928, 23.33224293864769194 ) ) ;
#114661=CARTESIAN_POINT ( 'NONE',  ( 8.314922557961029526, -14.29746914071037800, 95.41775706135234714 ) ) ;
#114662=CARTESIAN_POINT ( 'NONE',  ( 8.314922557960818139, 14.29746914071049879, 99.58224293864770971 ) ) ;
#114663=CARTESIAN_POINT ( 'NONE',  ( 19.03943276465977164, 0.05219959533936151252, 91.25109039468566152 ) ) ;
#114664=EDGE_LOOP ( 'NONE', ( #92785, #12605, #58893, #110444, #43846 ) ) ;
#114665=CARTESIAN_POINT ( 'NONE',  ( 21.55341960407610458, 5.719274019375980345, 108.9572429386476955 ) ) ;
#114666=CARTESIAN_POINT ( 'NONE',  ( -16.46253265017146816, -9.564922557961047289, 54.16775706135234003 ) ) ;
#114667=CARTESIAN_POINT ( 'NONE',  ( 14.29746914071037800, 8.314922557961029526, 96.66775706135234714 ) ) ;
#114668=CARTESIAN_POINT ( 'NONE',  ( 5.049401038297881783, 19.05341960407617563, 32.29275706135233293 ) ) ;
#114669=CARTESIAN_POINT ( 'NONE',  ( 0.05219959533909260263, 19.03943276465977164, 99.99890960531436690 ) ) ;
#114670=CARTESIAN_POINT ( 'NONE',  ( 21.55341960407610458, 5.719274019375980345, 58.95724293864770971 ) ) ;
#114672=CARTESIAN_POINT ( 'NONE',  ( 19.03943276465977164, -0.05219959533909143690, 28.74890960531435624 ) ) ;
#114673=CARTESIAN_POINT ( 'NONE',  ( 21.52544592524334988, 5.823673210054432836, 106.4594237280190328 ) ) ;
#114674=CARTESIAN_POINT ( 'NONE',  ( 12.06949235617739724, 12.14591786802326823, 71.87609039468568994 ) ) ;
#114675=CARTESIAN_POINT ( 'NONE',  ( -21.53943276465977519, -0.05219959533937600094, 23.75109039468567929 ) ) ;
#114676=CARTESIAN_POINT ( 'NONE',  ( 14.29746914071037800, 8.314922557961029526, 46.66775706135234714 ) ) ;
#114677=CARTESIAN_POINT ( 'NONE',  ( 0.05219959533909260263, 19.03943276465977164, 99.99890960531436690 ) ) ;
#114678=CARTESIAN_POINT ( 'NONE',  ( 9.474510206698971260, -16.51473224551069308, 42.91557627198103120 ) ) ;
#114679=CARTESIAN_POINT ( 'NONE',  ( 5.049401038298161559, -19.05341960407611168, 62.70724293864769550 ) ) ;
#114680=CIRCLE ( 'NONE', #33868, 1.250000000000006439 ) ;
#114681=CARTESIAN_POINT ( 'NONE',  ( 16.52544592524335698, 4.483927247898782831, 46.45942372801901854 ) ) ;
#114682=CARTESIAN_POINT ( 'NONE',  ( 8.314922557960818139, 14.29746914071049879, 94.58224293864769550 ) ) ;
#114683=CARTESIAN_POINT ( 'NONE',  ( 16.53943276465976808, 0.05219959533934440121, 101.2510903946856757 ) ) ;
#114685=CARTESIAN_POINT ( 'NONE',  ( -21.55341960407619339, 5.719274019375674811, 53.54275706135234714 ) ) ;
#114686=CARTESIAN_POINT ( 'NONE',  ( -5.153800228976328057, -19.02544592524343514, 82.29057627198103830 ) ) ;
#114687=CARTESIAN_POINT ( 'NONE',  ( 13.97604488694527802, 13.89961937509977652, 69.37390960531436690 ) ) ;
#114688=CARTESIAN_POINT ( 'NONE',  ( 13.97604488694527802, 13.89961937509977652, 89.37390960531436690 ) ) ;
#114689=CARTESIAN_POINT ( 'NONE',  ( -14.34966873604960291, -8.224510206698953496, 51.66557627198102409 ) ) ;
#114690=CARTESIAN_POINT ( 'NONE',  ( 16.55341960407618274, -4.379528057220086978, 101.0427570613523756 ) ) ;
#114691=CARTESIAN_POINT ( 'NONE',  ( -0.05219959533910754901, -16.53943276465976808, 22.49890960531436335 ) ) ;
#114693=CARTESIAN_POINT ( 'NONE',  ( 19.02544592524334988, 5.153800228976608722, 46.45942372801899012 ) ) ;
#114694=CARTESIAN_POINT ( 'NONE',  ( -5.049401038298153566, 19.05341960407611168, 115.2072429386477097 ) ) ;
#114696=CARTESIAN_POINT ( 'NONE',  ( -13.97604488694527625, -13.89961937509977652, 61.87390960531435979 ) ) ;
#114697=CARTESIAN_POINT ( 'NONE',  ( -13.97604488694547697, 13.89961937509957934, 43.12609039468566152 ) ) ;
#114701=CARTESIAN_POINT ( 'NONE',  ( -9.474510206698720793, -16.51473224551083518, 84.58442372801900433 ) ) ;
#114702=CARTESIAN_POINT ( 'NONE',  ( -16.55341960407617563, 4.379528057220093196, 73.54275706135234714 ) ) ;
#114703=CARTESIAN_POINT ( 'NONE',  ( 16.81555441253553695, 7.025013491695490941, 91.86314554665746357 ) ) ;
#114704=CARTESIAN_POINT ( 'NONE',  ( -19.05341960407611168, -5.049401038298163336, 96.45724293864769550 ) ) ;
#114705=CARTESIAN_POINT ( 'NONE',  ( -10.81492255796105439, 18.62759615963255655, 22.91775706135235069 ) ) ;
#114706=CARTESIAN_POINT ( 'NONE',  ( 5.049401038297881783, 19.05341960407617563, 82.29275706135229029 ) ) ;
#114707=CARTESIAN_POINT ( 'NONE',  ( 16.38665767535054130, 7.295008042176063690, 87.23599135785460135 ) ) ;
#114708=CARTESIAN_POINT ( 'NONE',  ( -13.89961937509977652, 13.97604488694528158, 45.62390960531433848 ) ) ;
#114709=CARTESIAN_POINT ( 'NONE',  ( -16.46253265017160317, 9.564922557960807481, 90.83224293864769550 ) ) ;
#114710=CARTESIAN_POINT ( 'NONE',  ( 4.483927247898545687, 16.52544592524342804, 44.79057627198103120 ) ) ;
#114711=CARTESIAN_POINT ( 'NONE',  ( -5.049401038298153566, 19.05341960407611168, 40.20724293864768839 ) ) ;
#114712=CARTESIAN_POINT ( 'NONE',  ( -9.474510206698720793, -16.51473224551083518, 49.58442372801899722 ) ) ;
#114713=VERTEX_POINT ( 'NONE', #160995 ) ;
#114714=CARTESIAN_POINT ( 'NONE',  ( -14.34966873604960291, -8.224510206698953496, 91.66557627198103830 ) ) ;
#114715=CARTESIAN_POINT ( 'NONE',  ( -19.03943276465977164, -0.05219959533935918106, 33.75109039468566863 ) ) ;
#114716=CARTESIAN_POINT ( 'NONE',  ( 19.03943276465977164, -0.05219959533909143690, 63.74890960531435979 ) ) ;
#114717=CARTESIAN_POINT ( 'NONE',  ( -18.67979575497178146, -10.72451020669898902, 66.66557627198102409 ) ) ;
#114718=CARTESIAN_POINT ( 'NONE',  ( 14.29746914071049879, -8.314922557960816363, 53.33224293864769550 ) ) ;
#114719=CARTESIAN_POINT ( 'NONE',  ( -19.03943276465977164, -0.05219959533935918106, 18.75109039468567218 ) ) ;
#114720=CARTESIAN_POINT ( 'NONE',  ( -5.153800228976328057, -19.02544592524343514, 112.2905762719810099 ) ) ;
#114721=CARTESIAN_POINT ( 'NONE',  ( 21.53943276465977519, -0.05219959533907433946, 23.74890960531435269 ) ) ;
#114722=CARTESIAN_POINT ( 'NONE',  ( 5.049401038298161559, -19.05341960407611168, 57.70724293864769550 ) ) ;
#114723=CARTESIAN_POINT ( 'NONE',  ( 13.97604488694527802, 13.89961937509977652, 24.37390960531435624 ) ) ;
#114724=CARTESIAN_POINT ( 'NONE',  ( -14.34966873604960291, -8.224510206698953496, 96.66557627198102409 ) ) ;
#114725=CARTESIAN_POINT ( 'NONE',  ( -10.81492255796078084, -18.62759615963271287, 107.0822429386476955 ) ) ;
#114726=CARTESIAN_POINT ( 'NONE',  ( 19.03943276465977164, -0.05219959533909143690, 98.74890960531436690 ) ) ;
#114727=CARTESIAN_POINT ( 'NONE',  ( -15.80617190586745835, -15.72974639402198527, 106.8739096053143811 ) ) ;
#114728=CARTESIAN_POINT ( 'NONE',  ( 9.474510206698971260, -16.51473224551069308, 97.91557627198102409 ) ) ;
#114729=CARTESIAN_POINT ( 'NONE',  ( -12.14591786802309592, -12.06949235617757132, 111.8739096053143669 ) ) ;
#114730=CARTESIAN_POINT ( 'NONE',  ( -21.52544592524334988, -5.823673210054445271, 78.95942372801901854 ) ) ;
#114731=CARTESIAN_POINT ( 'NONE',  ( 10.81492255796078972, 18.62759615963270932, 89.58224293864768129 ) ) ;
#114732=CARTESIAN_POINT ( 'NONE',  ( 17.44270441346516520, -5.991230190323040716, 106.1366492073577064 ) ) ;
#114735=CARTESIAN_POINT ( 'NONE',  ( 14.34966873604972726, -8.224510206698740333, 40.83442372801901854 ) ) ;
#114736=CARTESIAN_POINT ( 'NONE',  ( 16.55341960407611168, 4.379528057220329451, 103.9572429386476813 ) ) ;
#114738=CARTESIAN_POINT ( 'NONE',  ( 9.564922557960805705, 16.46253265017160317, 64.58224293864769550 ) ) ;
#114739=CARTESIAN_POINT ( 'NONE',  ( 12.14591786802309770, 12.06949235617756955, 99.37390960531436690 ) ) ;
#114740=CARTESIAN_POINT ( 'NONE',  ( 18.62759615963271287, -10.81492255796078972, 38.33224293864768839 ) ) ;
#114741=CARTESIAN_POINT ( 'NONE',  ( -8.314922557960811034, -14.29746914071050412, 62.08224293864769550 ) ) ;
#114742=CARTESIAN_POINT ( 'NONE',  ( 5.049401038297881783, 19.05341960407617563, 112.2927570613523471 ) ) ;
#114743=CARTESIAN_POINT ( 'NONE',  ( -15.72974639402176322, -15.80617190586768395, 79.37609039468567573 ) ) ;
#114744=CARTESIAN_POINT ( 'NONE',  ( -18.22780087662122028, 5.500000000000031086, 63.51540105326107266 ) ) ;
#114745=CARTESIAN_POINT ( 'NONE',  ( -14.34966873604972548, 8.224510206698743886, 93.33442372801901854 ) ) ;
#114746=CARTESIAN_POINT ( 'NONE',  ( 14.29746914071049879, -8.314922557960816363, 38.33224293864768839 ) ) ;
#114747=CARTESIAN_POINT ( 'NONE',  ( 5.049401038298161559, -19.05341960407611168, 32.70724293864768129 ) ) ;
#114748=CARTESIAN_POINT ( 'NONE',  ( 9.564922557960805705, 16.46253265017160317, 94.58224293864769550 ) ) ;
#114749=CARTESIAN_POINT ( 'NONE',  ( 21.55341960407610458, 5.719274019375980345, 93.95724293864770971 ) ) ;
#114750=CARTESIAN_POINT ( 'NONE',  ( 8.314922557961029526, -14.29746914071037800, 20.41775706135234714 ) ) ;
#114751=CARTESIAN_POINT ( 'NONE',  ( -4.379528057220328563, 16.55341960407611168, 60.20724293864768839 ) ) ;
#114752=CARTESIAN_POINT ( 'NONE',  ( -21.52544592524334988, -5.823673210054445271, 68.95942372801901854 ) ) ;
#114753=CARTESIAN_POINT ( 'NONE',  ( 12.14591786802327356, -12.06949235617739191, 105.6260903946856899 ) ) ;
#114754=CARTESIAN_POINT ( 'NONE',  ( 17.05587630539785948, 6.762274262135715475, 26.75819690962688924 ) ) ;
#114755=CARTESIAN_POINT ( 'NONE',  ( -19.49671883438228193, -5.499999999999979572, 64.89279849105683695 ) ) ;
#114756=CARTESIAN_POINT ( 'NONE',  ( -8.224510206698948167, 14.34966873604960824, 30.41557627198101699 ) ) ;
#114757=CARTESIAN_POINT ( 'NONE',  ( 16.55341960407618274, -4.379528057220086978, 71.04275706135234714 ) ) ;
#114758=CARTESIAN_POINT ( 'NONE',  ( 9.474510206698971260, -16.51473224551069308, 82.91557627198103830 ) ) ;
#114759=CARTESIAN_POINT ( 'NONE',  ( -9.564922557960796823, -16.46253265017161027, 82.08224293864768129 ) ) ;
#114760=CARTESIAN_POINT ( 'NONE',  ( -5.823673210054431948, 21.52544592524334988, 87.70942372801901854 ) ) ;
#114761=CARTESIAN_POINT ( 'NONE',  ( -16.52544592524335698, -4.483927247898792601, 88.95942372801901854 ) ) ;
#114762=CARTESIAN_POINT ( 'NONE',  ( 12.14591786802309770, 12.06949235617756955, 59.37390960531436690 ) ) ;
#114763=CARTESIAN_POINT ( 'NONE',  ( -19.05341960407611168, -5.049401038298163336, 71.45724293864766707 ) ) ;
#114765=CARTESIAN_POINT ( 'NONE',  ( 5.049401038297881783, 19.05341960407617563, 107.2927570613523187 ) ) ;
#114766=CARTESIAN_POINT ( 'NONE',  ( -12.14591786802309592, -12.06949235617757132, 111.8739096053143669 ) ) ;
#114767=CARTESIAN_POINT ( 'NONE',  ( 0.05219959533909260263, 19.03943276465977164, 79.99890960531436690 ) ) ;
#114768=CARTESIAN_POINT ( 'NONE',  ( 5.153800228976615827, -19.02544592524334988, 110.2094237280189901 ) ) ;
#114770=CARTESIAN_POINT ( 'NONE',  ( 5.153800228976615827, -19.02544592524334988, 25.20942372801900433 ) ) ;
#114771=CARTESIAN_POINT ( 'NONE',  ( 14.29746914071037800, 8.314922557961029526, 86.66775706135234714 ) ) ;
#114772=CARTESIAN_POINT ( 'NONE',  ( 19.02544592524334988, 5.153800228976608722, 96.45942372801897591 ) ) ;
#114773=CARTESIAN_POINT ( 'NONE',  ( -8.314922557960811034, -14.29746914071050412, 112.0822429386477097 ) ) ;
#114774=CARTESIAN_POINT ( 'NONE',  ( 4.379528057220092307, 16.55341960407617563, 62.29275706135236845 ) ) ;
#114775=CARTESIAN_POINT ( 'NONE',  ( 14.29746914071037800, 8.314922557961029526, 56.66775706135235424 ) ) ;
#114776=CARTESIAN_POINT ( 'NONE',  ( -5.049401038298153566, 19.05341960407611168, 25.20724293864768484 ) ) ;
#114777=CARTESIAN_POINT ( 'NONE',  ( 13.97604488694548053, -13.89961937509957401, 50.62609039468566152 ) ) ;
#114779=CARTESIAN_POINT ( 'NONE',  ( 15.72974639402176855, 15.80617190586768217, 91.87609039468568994 ) ) ;
#114780=CARTESIAN_POINT ( 'NONE',  ( 13.89961937509977652, -13.97604488694527269, 28.12390960531435624 ) ) ;
#114781=CARTESIAN_POINT ( 'NONE',  ( -19.03943276465977164, 0.05219959533909376836, 81.24890960531436690 ) ) ;
#114782=CARTESIAN_POINT ( 'NONE',  ( 16.53943276465976808, -0.05219959533910856209, 78.74890960531436690 ) ) ;
#114783=CARTESIAN_POINT ( 'NONE',  ( -0.05219959533937732626, 21.53943276465977519, 87.50109039468568994 ) ) ;
#114784=CARTESIAN_POINT ( 'NONE',  ( -5.049401038297874678, -19.05341960407617918, 59.79275706135231871 ) ) ;
#114785=CARTESIAN_POINT ( 'NONE',  ( -13.89961937509957401, -13.97604488694547875, 39.37609039468566152 ) ) ;
#114786=CARTESIAN_POINT ( 'NONE',  ( 21.55341960407610458, 5.719274019375980345, 33.95724293864769550 ) ) ;
#114787=CARTESIAN_POINT ( 'NONE',  ( 10.72451020669871369, 18.67979575497193778, 92.08442372801901854 ) ) ;
#114788=CARTESIAN_POINT ( 'NONE',  ( -19.03943276465977164, 0.05219959533909376836, 71.24890960531435269 ) ) ;
#114789=CARTESIAN_POINT ( 'NONE',  ( 5.719274019375673035, 21.55341960407619339, 112.2927570613523471 ) ) ;
#114790=CARTESIAN_POINT ( 'NONE',  ( -15.72974639402197994, 15.80617190586746368, 55.62390960531436690 ) ) ;
#114791=CARTESIAN_POINT ( 'NONE',  ( 5.049401038298161559, -19.05341960407611168, 97.70724293864766707 ) ) ;
#114792=CARTESIAN_POINT ( 'NONE',  ( -5.153800228976607833, 19.02544592524334988, 77.70942372801900433 ) ) ;
#114793=CARTESIAN_POINT ( 'NONE',  ( -19.05341960407611168, -5.049401038298163336, 106.4572429386476955 ) ) ;
#114794=CARTESIAN_POINT ( 'NONE',  ( 0.05219959533936267826, -19.03943276465977164, 100.0010903946856757 ) ) ;
#114795=CARTESIAN_POINT ( 'NONE',  ( 4.483927247898790824, -16.52544592524335698, 40.20942372801901854 ) ) ;
#114796=CARTESIAN_POINT ( 'NONE',  ( 12.06949235617757843, -12.14591786802309237, 108.1239096053143811 ) ) ;
#114797=CARTESIAN_POINT ( 'NONE',  ( 5.049401038298161559, -19.05341960407611168, 77.70724293864765286 ) ) ;
#114798=CARTESIAN_POINT ( 'NONE',  ( 10.81492255796078972, 18.62759615963270932, 69.58224293864769550 ) ) ;
#114799=CARTESIAN_POINT ( 'NONE',  ( -16.55341960407617563, 4.379528057220093196, 38.54275706135234714 ) ) ;
#114800=CARTESIAN_POINT ( 'NONE',  ( 10.81492255796106328, -18.62759615963255655, 40.41775706135234714 ) ) ;
#114801=CARTESIAN_POINT ( 'NONE',  ( 15.72974639402176855, 15.80617190586768217, 86.87609039468568994 ) ) ;
#114802=CARTESIAN_POINT ( 'NONE',  ( -4.379528057220086978, -16.55341960407618274, 79.79275706135236135 ) ) ;
#114803=CARTESIAN_POINT ( 'NONE',  ( 9.564922557960805705, 16.46253265017160317, 74.58224293864769550 ) ) ;
#114804=CARTESIAN_POINT ( 'NONE',  ( -4.379528057220328563, 16.55341960407611168, 75.20724293864769550 ) ) ;
#114805=CARTESIAN_POINT ( 'NONE',  ( 12.06949235617757843, -12.14591786802309237, 23.12390960531436335 ) ) ;
#114806=CARTESIAN_POINT ( 'NONE',  ( -0.05219959533936034679, 19.03943276465977164, 52.50109039468566863 ) ) ;
#114808=CARTESIAN_POINT ( 'NONE',  ( -15.80617190586768217, 15.72974639402176855, 38.12609039468567573 ) ) ;
#114809=CARTESIAN_POINT ( 'NONE',  ( 4.379528057220339221, -16.55341960407611168, 72.70724293864769550 ) ) ;
#114810=CARTESIAN_POINT ( 'NONE',  ( -18.67979575497178146, -10.72451020669898902, 21.66557627198102409 ) ) ;
#114811=CARTESIAN_POINT ( 'NONE',  ( -4.483927247898782831, 16.52544592524335698, 107.7094237280190328 ) ) ;
#114812=CARTESIAN_POINT ( 'NONE',  ( -18.67979575497193778, 10.72451020669871902, 78.33442372801901854 ) ) ;
#114813=CARTESIAN_POINT ( 'NONE',  ( 4.379528057220092307, 16.55341960407617563, 42.29275706135235424 ) ) ;
#114814=CARTESIAN_POINT ( 'NONE',  ( -5.719274019375665041, -21.55341960407619695, 39.79275706135235424 ) ) ;
#114816=CARTESIAN_POINT ( 'NONE',  ( -10.81492255796078084, -18.62759615963271287, 112.0822429386477097 ) ) ;
#114817=CARTESIAN_POINT ( 'NONE',  ( -14.29746914071049879, 8.314922557960819915, 85.83224293864768129 ) ) ;
#114818=CARTESIAN_POINT ( 'NONE',  ( 17.49999999999996803, -3.512728167237031407, 27.72809995181124521 ) ) ;
#114819=CARTESIAN_POINT ( 'NONE',  ( -0.05219959533910754901, -16.53943276465976808, 47.49890960531435979 ) ) ;
#114820=CARTESIAN_POINT ( 'NONE',  ( -0.05219959533934338120, 16.53943276465976808, 92.50109039468567573 ) ) ;
#114821=CARTESIAN_POINT ( 'NONE',  ( -16.46253265017160317, 9.564922557960807481, 40.83224293864769550 ) ) ;
#114822=CARTESIAN_POINT ( 'NONE',  ( 5.719274019375991003, -21.55341960407610458, 47.70724293864770260 ) ) ;
#114823=CARTESIAN_POINT ( 'NONE',  ( 16.53943276465976808, -0.05219959533910856209, 78.74890960531436690 ) ) ;
#114824=CARTESIAN_POINT ( 'NONE',  ( 15.80617190586746368, 15.72974639402197994, 84.37390960531438111 ) ) ;
#114825=CARTESIAN_POINT ( 'NONE',  ( -16.51473224551069308, -9.474510206698971260, 81.66557627198103830 ) ) ;
#114826=CARTESIAN_POINT ( 'NONE',  ( 13.89961937509977652, -13.97604488694527269, 33.12390960531434558 ) ) ;
#114827=CARTESIAN_POINT ( 'NONE',  ( 5.153800228976615827, -19.02544592524334988, 90.20942372801900433 ) ) ;
#114828=CARTESIAN_POINT ( 'NONE',  ( -21.52544592524343514, 5.823673210054127303, 26.04057627198103475 ) ) ;
#114829=CARTESIAN_POINT ( 'NONE',  ( 21.53943276465977519, 0.05219959533937863772, 51.25109039468568994 ) ) ;
#114830=CARTESIAN_POINT ( 'NONE',  ( -0.05219959533907301413, -21.53943276465977519, 57.49890960531435979 ) ) ;
#114831=CARTESIAN_POINT ( 'NONE',  ( -9.474510206698964154, 16.51473224551069663, 55.41557627198103120 ) ) ;
#114832=CARTESIAN_POINT ( 'NONE',  ( -13.89961937509977652, 13.97604488694528158, 75.62390960531438111 ) ) ;
#114833=VERTEX_POINT ( 'NONE', #53824 ) ;
#114834=CARTESIAN_POINT ( 'NONE',  ( -8.224510206698735004, -14.34966873604973081, 44.58442372801901854 ) ) ;
#114835=CARTESIAN_POINT ( 'NONE',  ( -5.719274019375665041, -21.55341960407619695, 24.79275706135235779 ) ) ;
#114836=CARTESIAN_POINT ( 'NONE',  ( -5.719274019375665041, -21.55341960407619695, 79.79275706135236135 ) ) ;
#114837=CARTESIAN_POINT ( 'NONE',  ( 19.02544592524343514, -5.153800228976328945, 113.5405762719810241 ) ) ;
#114838=CARTESIAN_POINT ( 'NONE',  ( -0.05219959533907301413, -21.53943276465977519, 82.49890960531436690 ) ) ;
#114839=CARTESIAN_POINT ( 'NONE',  ( 21.55341960407619695, -5.719274019375665929, 26.04275706135235779 ) ) ;
#114840=CARTESIAN_POINT ( 'NONE',  ( 4.379528057220092307, 16.55341960407617563, 67.29275706135234714 ) ) ;
#114841=CARTESIAN_POINT ( 'NONE',  ( -5.719274019375978568, 21.55341960407610458, 65.20724293864768129 ) ) ;
#114842=CARTESIAN_POINT ( 'NONE',  ( 19.03943276465977164, 0.05219959533936151252, 21.25109039468565797 ) ) ;
#114843=CARTESIAN_POINT ( 'NONE',  ( -0.05219959533909027116, -19.03943276465977164, 57.49890960531435979 ) ) ;
#114844=CARTESIAN_POINT ( 'NONE',  ( 5.049401038298161559, -19.05341960407611168, 107.7072429386476955 ) ) ;
#114845=CARTESIAN_POINT ( 'NONE',  ( -9.474510206698964154, 16.51473224551069663, 95.41557627198102409 ) ) ;
#114846=CARTESIAN_POINT ( 'NONE',  ( 17.50000000000000355, 3.203707223489912881, 102.7268034735096904 ) ) ;
#114847=CARTESIAN_POINT ( 'NONE',  ( -19.03943276465977164, -0.05219959533935918106, 68.75109039468566152 ) ) ;
#114848=CARTESIAN_POINT ( 'NONE',  ( -21.55341960407610458, -5.719274019375992779, 46.45724293864769550 ) ) ;
#114849=CARTESIAN_POINT ( 'NONE',  ( -14.34966873604972548, 8.224510206698743886, 113.3344237280190328 ) ) ;
#114850=CARTESIAN_POINT ( 'NONE',  ( -5.049401038297874678, -19.05341960407617918, 99.79275706135234714 ) ) ;
#114851=CARTESIAN_POINT ( 'NONE',  ( 9.564922557960805705, 16.46253265017160317, 24.58224293864769194 ) ) ;
#114852=CARTESIAN_POINT ( 'NONE',  ( 9.564922557961047289, -16.46253265017146816, 20.41775706135233293 ) ) ;
#114853=CARTESIAN_POINT ( 'NONE',  ( 9.564922557961047289, -16.46253265017146816, 90.41775706135234714 ) ) ;
#114854=CARTESIAN_POINT ( 'NONE',  ( 10.72451020669898902, -18.67979575497178502, 87.91557627198103830 ) ) ;
#114855=CARTESIAN_POINT ( 'NONE',  ( -13.89961937509957401, -13.97604488694547875, 59.37609039468566863 ) ) ;
#114856=CARTESIAN_POINT ( 'NONE',  ( 16.38665767535055195, 7.295008042176104546, 107.2359913578545587 ) ) ;
#114857=CARTESIAN_POINT ( 'NONE',  ( 19.05341960407611168, 5.049401038298154454, 58.95724293864768129 ) ) ;
#114858=CARTESIAN_POINT ( 'NONE',  ( 12.06949235617757843, -12.14591786802309237, 68.12390960531436690 ) ) ;
#114859=CARTESIAN_POINT ( 'NONE',  ( -9.474510206698964154, 16.51473224551069663, 50.41557627198102409 ) ) ;
#114860=CARTESIAN_POINT ( 'NONE',  ( 4.483927247898545687, 16.52544592524342804, 49.79057627198102409 ) ) ;
#114861=CYLINDRICAL_SURFACE ( 'NONE', #100088, 2.000000000000001776 ) ;
#114862=CARTESIAN_POINT ( 'NONE',  ( -8.314922557960811034, -14.29746914071050412, 32.08224293864769550 ) ) ;
#114863=CARTESIAN_POINT ( 'NONE',  ( 19.05341960407611168, 5.049401038298154454, 63.95724293864769550 ) ) ;
#114864=CARTESIAN_POINT ( 'NONE',  ( 16.51473224551083163, -9.474510206698727899, 20.83442372801899722 ) ) ;
#114865=CARTESIAN_POINT ( 'NONE',  ( 8.314922557961029526, -14.29746914071037800, 30.41775706135234358 ) ) ;
#114866=CARTESIAN_POINT ( 'NONE',  ( 10.81492255796078972, 18.62759615963270932, 49.58224293864769550 ) ) ;
#114867=CARTESIAN_POINT ( 'NONE',  ( -18.62759615963255300, -10.81492255796106328, 99.16775706135234714 ) ) ;
#114868=ORIENTED_EDGE ( 'NONE', *, *, #12204, .T. ) ;
#114869=CARTESIAN_POINT ( 'NONE',  ( 19.05341960407611168, 5.049401038298154454, 58.95724293864768129 ) ) ;
#114871=CARTESIAN_POINT ( 'NONE',  ( 13.89961937509977652, -13.97604488694527269, 93.12390960531436690 ) ) ;
#114873=CARTESIAN_POINT ( 'NONE',  ( -21.52544592524334988, -5.823673210054445271, 23.95942372801901143 ) ) ;
#114875=CARTESIAN_POINT ( 'NONE',  ( -12.14591786802309592, -12.06949235617757132, 91.87390960531436690 ) ) ;
#114877=CARTESIAN_POINT ( 'NONE',  ( -18.67979575497178146, -10.72451020669898902, 91.66557627198103830 ) ) ;
#114878=CARTESIAN_POINT ( 'NONE',  ( -9.474510206698964154, 16.51473224551069663, 65.41557627198102409 ) ) ;
#114879=CARTESIAN_POINT ( 'NONE',  ( 0.05219959533909260263, 19.03943276465977164, 89.99890960531436690 ) ) ;
#114880=CARTESIAN_POINT ( 'NONE',  ( 5.823673210054125526, 21.52544592524343514, 104.7905762719810241 ) ) ;
#114882=CARTESIAN_POINT ( 'NONE',  ( -5.049401038298153566, 19.05341960407611168, 70.20724293864769550 ) ) ;
#114883=CARTESIAN_POINT ( 'NONE',  ( 19.35633801406909171, -5.499999999999674039, 96.63373818172770768 ) ) ;
#114884=CARTESIAN_POINT ( 'NONE',  ( -8.314922557960811034, -14.29746914071050412, 102.0822429386476955 ) ) ;
#114886=CARTESIAN_POINT ( 'NONE',  ( -19.05341960407617563, 5.049401038297882671, 98.54275706135233293 ) ) ;
#114887=CARTESIAN_POINT ( 'NONE',  ( -19.05341960407611168, -5.049401038298163336, 21.45724293864768839 ) ) ;
#114888=CARTESIAN_POINT ( 'NONE',  ( 15.80617190586769283, -15.72974639402175789, 65.62609039468568994 ) ) ;
#114889=CARTESIAN_POINT ( 'NONE',  ( 19.02544592524343514, -5.153800228976328945, 68.54057627198103830 ) ) ;
#114890=CARTESIAN_POINT ( 'NONE',  ( 21.53943276465977519, 0.05219959533937863772, 36.25109039468567573 ) ) ;
#114891=CARTESIAN_POINT ( 'NONE',  ( 10.81492255796078972, 18.62759615963270932, 104.5822429386477097 ) ) ;
#114893=CARTESIAN_POINT ( 'NONE',  ( 19.03943276465977164, -0.05219959533909143690, 68.74890960531436690 ) ) ;
#114895=CARTESIAN_POINT ( 'NONE',  ( 14.29746914071037800, 8.314922557961029526, 21.66775706135235069 ) ) ;
#114896=CARTESIAN_POINT ( 'NONE',  ( -21.52544592524343514, 5.823673210054127303, 26.04057627198103475 ) ) ;
#114897=CARTESIAN_POINT ( 'NONE',  ( 21.52544592524334988, 5.823673210054432836, 56.45942372801902565 ) ) ;
#114898=CARTESIAN_POINT ( 'NONE',  ( 5.049401038298161559, -19.05341960407611168, 112.7072429386476813 ) ) ;
#114899=CARTESIAN_POINT ( 'NONE',  ( 0.05219959533936267826, -19.03943276465977164, 90.00109039468567573 ) ) ;
#114900=CARTESIAN_POINT ( 'NONE',  ( 5.049401038298161559, -19.05341960407611168, 52.70724293864767418 ) ) ;
#114901=CARTESIAN_POINT ( 'NONE',  ( -5.153800228976328057, -19.02544592524343514, 67.29057627198102409 ) ) ;
#114902=CARTESIAN_POINT ( 'NONE',  ( 0.05219959533910956823, 16.53943276465976808, 99.99890960531436690 ) ) ;
#114903=CARTESIAN_POINT ( 'NONE',  ( -13.97604488694527625, -13.89961937509977652, 106.8739096053143669 ) ) ;
#114904=CARTESIAN_POINT ( 'NONE',  ( 8.224510206698953496, -14.34966873604960469, 87.91557627198103830 ) ) ;
#114905=CARTESIAN_POINT ( 'NONE',  ( -19.02544592524342804, 5.153800228976336051, 101.0405762719810241 ) ) ;
#114906=CARTESIAN_POINT ( 'NONE',  ( -0.05219959533910754901, -16.53943276465976808, 57.49890960531435979 ) ) ;
#114907=CARTESIAN_POINT ( 'NONE',  ( -9.564922557960796823, -16.46253265017161027, 47.08224293864769550 ) ) ;
#114908=CARTESIAN_POINT ( 'NONE',  ( -10.81492255796105439, 18.62759615963255655, 52.91775706135235424 ) ) ;
#114909=CARTESIAN_POINT ( 'NONE',  ( 13.89961937509957401, 13.97604488694547697, 91.87609039468567573 ) ) ;
#114910=CARTESIAN_POINT ( 'NONE',  ( -16.53943276465976808, 0.05219959533911058130, 46.24890960531435979 ) ) ;
#114911=CARTESIAN_POINT ( 'NONE',  ( -21.53943276465977519, 0.05219959533907696930, 96.24890960531435269 ) ) ;
#114912=CARTESIAN_POINT ( 'NONE',  ( 10.72451020669898902, -18.67979575497178502, 47.91557627198102409 ) ) ;
#114914=CARTESIAN_POINT ( 'NONE',  ( -9.474510206698964154, 16.51473224551069663, 110.4155762719810383 ) ) ;
#114915=CARTESIAN_POINT ( 'NONE',  ( -16.52544592524342804, 4.483927247898546575, 81.04057627198102409 ) ) ;
#114917=CARTESIAN_POINT ( 'NONE',  ( -19.02544592524342804, 5.153800228976336051, 56.04057627198100988 ) ) ;
#114918=CARTESIAN_POINT ( 'NONE',  ( 4.483927247898790824, -16.52544592524335698, 110.2094237280190185 ) ) ;
#114919=CARTESIAN_POINT ( 'NONE',  ( 4.483927247898790824, -16.52544592524335698, 95.20942372801903275 ) ) ;
#114920=CARTESIAN_POINT ( 'NONE',  ( -12.14591786802326823, 12.06949235617739902, 78.12609039468570415 ) ) ;
#114921=CARTESIAN_POINT ( 'NONE',  ( 0.05219959533936267826, -19.03943276465977164, 40.00109039468566152 ) ) ;
#114922=CARTESIAN_POINT ( 'NONE',  ( -16.81555441253551919, 7.025013491695477619, 70.63685445334257906 ) ) ;
#114923=CARTESIAN_POINT ( 'NONE',  ( 0.05219959533909260263, 19.03943276465977164, 109.9989096053143669 ) ) ;
#114924=CARTESIAN_POINT ( 'NONE',  ( 5.153800228976335163, 19.02544592524342804, 89.79057627198102409 ) ) ;
#114925=CARTESIAN_POINT ( 'NONE',  ( -19.03943276465977164, 0.05219959533909376836, 36.24890960531436690 ) ) ;
#114926=CARTESIAN_POINT ( 'NONE',  ( -16.53943276465976808, 0.05219959533911058130, 46.24890960531435979 ) ) ;
#114928=CARTESIAN_POINT ( 'NONE',  ( 0.05219959533909260263, 19.03943276465977164, 109.9989096053143669 ) ) ;
#114929=CARTESIAN_POINT ( 'NONE',  ( -15.80617190586745835, -15.72974639402198527, 36.87390960531435979 ) ) ;
#114930=CARTESIAN_POINT ( 'NONE',  ( -16.53943276465976808, 0.05219959533911058130, 91.24890960531436690 ) ) ;
#114931=CARTESIAN_POINT ( 'NONE',  ( -0.05219959533934338120, 16.53943276465976808, 42.50109039468567573 ) ) ;
#114932=CARTESIAN_POINT ( 'NONE',  ( 8.314922557960818139, 14.29746914071049879, 74.58224293864768129 ) ) ;
#114933=CARTESIAN_POINT ( 'NONE',  ( -18.87075004821570801, 5.499999999999902300, 63.67408112101044537 ) ) ;
#114934=CARTESIAN_POINT ( 'NONE',  ( 19.05341960407617918, -5.049401038297876454, 61.04275706135232582 ) ) ;
#114935=CARTESIAN_POINT ( 'NONE',  ( 9.474510206698971260, -16.51473224551069308, 102.9155762719810241 ) ) ;
#114936=CARTESIAN_POINT ( 'NONE',  ( -5.153800228976607833, 19.02544592524334988, 72.70942372801900433 ) ) ;
#114938=CARTESIAN_POINT ( 'NONE',  ( 8.314922557961029526, -14.29746914071037800, 30.41775706135234358 ) ) ;
#114939=CARTESIAN_POINT ( 'NONE',  ( -14.34966873604960291, -8.224510206698953496, 21.66557627198102409 ) ) ;
#114940=CARTESIAN_POINT ( 'NONE',  ( -13.97604488694547697, 13.89961937509957934, 68.12609039468563310 ) ) ;
#114941=CARTESIAN_POINT ( 'NONE',  ( 18.62759615963271287, -10.81492255796078972, 33.33224293864769550 ) ) ;
#114942=CARTESIAN_POINT ( 'NONE',  ( 0.05219959533937995610, -21.53943276465977519, 70.00109039468568994 ) ) ;
#114943=CARTESIAN_POINT ( 'NONE',  ( 18.93472913878450825, 5.499999999999855227, 38.78010116131535767 ) ) ;
#114944=CARTESIAN_POINT ( 'NONE',  ( 16.55341960407618274, -4.379528057220086978, 26.04275706135235779 ) ) ;
#114945=CARTESIAN_POINT ( 'NONE',  ( -19.03943276465977164, 0.05219959533909376836, 26.24890960531435624 ) ) ;
#114946=CARTESIAN_POINT ( 'NONE',  ( 5.049401038298161559, -19.05341960407611168, 92.70724293864769550 ) ) ;
#114948=CARTESIAN_POINT ( 'NONE',  ( -0.05219959533910754901, -16.53943276465976808, 87.49890960531436690 ) ) ;
#114949=CARTESIAN_POINT ( 'NONE',  ( -16.46253265017160317, 9.564922557960807481, 85.83224293864769550 ) ) ;
#114951=CARTESIAN_POINT ( 'NONE',  ( 9.564922557960805705, 16.46253265017160317, 89.58224293864769550 ) ) ;
#114952=ORIENTED_EDGE ( 'NONE', *, *, #56474, .F. ) ;
#114953=CARTESIAN_POINT ( 'NONE',  ( -5.049401038297874678, -19.05341960407617918, 84.79275706135233293 ) ) ;
#114954=CARTESIAN_POINT ( 'NONE',  ( -18.67979575497178146, -10.72451020669898902, 76.66557627198103830 ) ) ;
#114955=CARTESIAN_POINT ( 'NONE',  ( 0.05219959533909260263, 19.03943276465977164, 29.99890960531435979 ) ) ;
#114956=CARTESIAN_POINT ( 'NONE',  ( 0.05219959533936267826, -19.03943276465977164, 70.00109039468566152 ) ) ;
#114957=CARTESIAN_POINT ( 'NONE',  ( 0.05219959533907565091, 21.53943276465977519, 114.9989096053143669 ) ) ;
#114958=CARTESIAN_POINT ( 'NONE',  ( 13.89961937509977652, -13.97604488694527269, 68.12390960531436690 ) ) ;
#114959=CARTESIAN_POINT ( 'NONE',  ( -5.153800228976328057, -19.02544592524343514, 102.2905762719810383 ) ) ;
#114961=CARTESIAN_POINT ( 'NONE',  ( -21.55341960407610458, -5.719274019375992779, 101.4572429386476955 ) ) ;
#114962=CARTESIAN_POINT ( 'NONE',  ( 14.34966873604960469, 8.224510206698951720, 104.1655762719810241 ) ) ;
#114963=CARTESIAN_POINT ( 'NONE',  ( -5.153800228976328057, -19.02544592524343514, 82.29057627198103830 ) ) ;
#114964=CARTESIAN_POINT ( 'NONE',  ( -0.05219959533936034679, 19.03943276465977164, 62.50109039468566863 ) ) ;
#114965=CARTESIAN_POINT ( 'NONE',  ( 21.53943276465977519, -0.05219959533907433946, 88.74890960531436690 ) ) ;
#114966=CARTESIAN_POINT ( 'NONE',  ( -18.62759615963270932, 10.81492255796079327, 75.83224293864769550 ) ) ;
#114967=CARTESIAN_POINT ( 'NONE',  ( -14.34966873604960291, -8.224510206698953496, 41.66557627198103120 ) ) ;
#114968=CARTESIAN_POINT ( 'NONE',  ( 5.719274019375673035, 21.55341960407619339, 112.2927570613523471 ) ) ;
#114969=CARTESIAN_POINT ( 'NONE',  ( -16.55341960407617563, 4.379528057220093196, 68.54275706135234714 ) ) ;
#114971=CARTESIAN_POINT ( 'NONE',  ( -9.564922557960796823, -16.46253265017161027, 92.08224293864769550 ) ) ;
#114972=CARTESIAN_POINT ( 'NONE',  ( -5.153800228976328057, -19.02544592524343514, 47.29057627198102409 ) ) ;
#114973=CARTESIAN_POINT ( 'NONE',  ( -21.52544592524334988, -5.823673210054445271, 53.95942372801900433 ) ) ;
#114974=CARTESIAN_POINT ( 'NONE',  ( 18.62759615963255655, 10.81492255796105972, 56.66775706135235424 ) ) ;
#114975=CARTESIAN_POINT ( 'NONE',  ( -16.51473224551069308, -9.474510206698971260, 61.66557627198103120 ) ) ;
#114976=CARTESIAN_POINT ( 'NONE',  ( 15.80617190586769283, -15.72974639402175789, 35.62609039468568994 ) ) ;
#114977=CARTESIAN_POINT ( 'NONE',  ( 5.049401038297881783, 19.05341960407617563, 72.29275706135234714 ) ) ;
#114978=CARTESIAN_POINT ( 'NONE',  ( -5.049401038297874678, -19.05341960407617918, 74.79275706135231871 ) ) ;
#114979=CARTESIAN_POINT ( 'NONE',  ( 5.153800228976335163, 19.02544592524342804, 39.79057627198100988 ) ) ;
#114980=CARTESIAN_POINT ( 'NONE',  ( 14.34966873604972726, -8.224510206698740333, 80.83442372801901854 ) ) ;
#114981=CARTESIAN_POINT ( 'NONE',  ( -19.03943276465977164, 0.05219959533909376836, 51.24890960531436690 ) ) ;
#114983=CARTESIAN_POINT ( 'NONE',  ( 5.153800228976335163, 19.02544592524342804, 94.79057627198103830 ) ) ;
#114984=CARTESIAN_POINT ( 'NONE',  ( 19.03943276465977164, -0.05219959533909143690, 43.74890960531435979 ) ) ;
#114985=CARTESIAN_POINT ( 'NONE',  ( 5.823673210054125526, 21.52544592524343514, 84.79057627198102409 ) ) ;
#114986=CARTESIAN_POINT ( 'NONE',  ( 8.224510206698742110, 14.34966873604972548, 62.08442372801901143 ) ) ;
#114987=CARTESIAN_POINT ( 'NONE',  ( 18.62759615963255655, 10.81492255796105972, 106.6677570613523756 ) ) ;
#114988=CARTESIAN_POINT ( 'NONE',  ( 16.46253265017160672, -9.564922557960803928, 53.33224293864768839 ) ) ;
#114989=CARTESIAN_POINT ( 'NONE',  ( 16.52544592524342804, -4.483927247898539470, 43.54057627198103830 ) ) ;
#114990=CARTESIAN_POINT ( 'NONE',  ( 14.34966873604960469, 8.224510206698951720, 84.16557627198103830 ) ) ;
#114991=CARTESIAN_POINT ( 'NONE',  ( 0.05219959533909260263, 19.03943276465977164, 74.99890960531435269 ) ) ;
#114992=CARTESIAN_POINT ( 'NONE',  ( -21.52544592524334988, -5.823673210054445271, 33.95942372801901143 ) ) ;
#114993=CARTESIAN_POINT ( 'NONE',  ( 9.564922557960805705, 16.46253265017160317, 89.58224293864769550 ) ) ;
#114994=CARTESIAN_POINT ( 'NONE',  ( 5.823673210054444382, -21.52544592524334988, 100.2094237280190043 ) ) ;
#114995=CARTESIAN_POINT ( 'NONE',  ( 16.52544592524335698, 4.483927247898782831, 66.45942372801903275 ) ) ;
#114996=CARTESIAN_POINT ( 'NONE',  ( -21.53943276465977519, -0.05219959533937600094, 28.75109039468567929 ) ) ;
#114997=CARTESIAN_POINT ( 'NONE',  ( -5.049401038298153566, 19.05341960407611168, 110.2072429386476671 ) ) ;
#114999=CARTESIAN_POINT ( 'NONE',  ( -21.52544592524343514, 5.823673210054127303, 91.04057627198103830 ) ) ;
#115000=CARTESIAN_POINT ( 'NONE',  ( 12.06949235617757843, -12.14591786802309237, 48.12390960531436690 ) ) ;
#115001=CARTESIAN_POINT ( 'NONE',  ( -0.05219959533909027116, -19.03943276465977164, 47.49890960531435979 ) ) ;
#115002=CARTESIAN_POINT ( 'NONE',  ( 8.314922557960818139, 14.29746914071049879, 64.58224293864769550 ) ) ;
#115003=CARTESIAN_POINT ( 'NONE',  ( 15.80617190586746368, 15.72974639402197994, 34.37390960531435979 ) ) ;
#115004=CARTESIAN_POINT ( 'NONE',  ( 5.049401038297881783, 19.05341960407617563, 32.29275706135233293 ) ) ;
#115005=CARTESIAN_POINT ( 'NONE',  ( -12.06949235617756955, 12.14591786802309770, 100.6239096053143811 ) ) ;
#115006=CARTESIAN_POINT ( 'NONE',  ( 16.46253265017160672, -9.564922557960803928, 113.3322429386476955 ) ) ;
#115008=CARTESIAN_POINT ( 'NONE',  ( -14.34966873604972548, 8.224510206698743886, 53.33442372801901854 ) ) ;
#115009=CARTESIAN_POINT ( 'NONE',  ( -16.46253265017160317, 9.564922557960807481, 50.83224293864770260 ) ) ;
#115011=CARTESIAN_POINT ( 'NONE',  ( -0.05219959533934338120, 16.53943276465976808, 87.50109039468568994 ) ) ;
#115012=CARTESIAN_POINT ( 'NONE',  ( 12.14591786802327356, -12.06949235617739191, 20.62609039468568639 ) ) ;
#115013=CARTESIAN_POINT ( 'NONE',  ( -5.719274019375665041, -21.55341960407619695, 74.79275706135234714 ) ) ;
#115014=CARTESIAN_POINT ( 'NONE',  ( 5.153800228976335163, 19.02544592524342804, 74.79057627198103830 ) ) ;
#115015=CARTESIAN_POINT ( 'NONE',  ( 21.52544592524344225, -5.823673210054117533, 88.54057627198103830 ) ) ;
#115016=CARTESIAN_POINT ( 'NONE',  ( -0.05219959533934338120, 16.53943276465976808, 47.50109039468568994 ) ) ;
#115017=CARTESIAN_POINT ( 'NONE',  ( -16.53943276465976808, 0.05219959533911058130, 116.2489096053143669 ) ) ;
#115019=CARTESIAN_POINT ( 'NONE',  ( 8.224510206698742110, 14.34966873604972548, 22.08442372801901143 ) ) ;
#115020=CARTESIAN_POINT ( 'NONE',  ( -0.05219959533936034679, 19.03943276465977164, 82.50109039468567573 ) ) ;
#115021=CARTESIAN_POINT ( 'NONE',  ( -21.53943276465977519, 0.05219959533907696930, 76.24890960531435269 ) ) ;
#115022=CARTESIAN_POINT ( 'NONE',  ( -9.474510206698720793, -16.51473224551083518, 49.58442372801899722 ) ) ;
#115023=CARTESIAN_POINT ( 'NONE',  ( 19.52851543214744012, 5.499999999999982236, 97.89357721762578990 ) ) ;
#115024=CARTESIAN_POINT ( 'NONE',  ( 18.67979575497178502, 10.72451020669898547, 89.16557627198102409 ) ) ;
#115025=CARTESIAN_POINT ( 'NONE',  ( 17.97058386085787873, 5.500000000000054179, 61.50390968646219392 ) ) ;
#115026=CARTESIAN_POINT ( 'NONE',  ( 13.89961937509977652, -13.97604488694527269, 63.12390960531435979 ) ) ;
#115028=CARTESIAN_POINT ( 'NONE',  ( -19.03943276465977164, -0.05219959533935918106, 108.7510903946856615 ) ) ;
#115030=CARTESIAN_POINT ( 'NONE',  ( -10.81492255796105439, 18.62759615963255655, 52.91775706135235424 ) ) ;
#115031=CARTESIAN_POINT ( 'NONE',  ( -10.72451020669898014, 18.67979575497178502, 105.4155762719810383 ) ) ;
#115032=CARTESIAN_POINT ( 'NONE',  ( 16.53943276465976808, -0.05219959533910856209, 58.74890960531436690 ) ) ;
#115033=CARTESIAN_POINT ( 'NONE',  ( 16.46253265017160672, -9.564922557960803928, 73.33224293864769550 ) ) ;
#115034=CARTESIAN_POINT ( 'NONE',  ( -0.05219959533937732626, 21.53943276465977519, 67.50109039468568994 ) ) ;
#115035=CARTESIAN_POINT ( 'NONE',  ( -14.29746914071037622, -8.314922557961029526, 19.16775706135234714 ) ) ;
#115036=CARTESIAN_POINT ( 'NONE',  ( -9.474510206698720793, -16.51473224551083518, 29.58442372801900433 ) ) ;
#115037=CARTESIAN_POINT ( 'NONE',  ( -18.67979575497193778, 10.72451020669871902, 43.33442372801901143 ) ) ;
#115038=CARTESIAN_POINT ( 'NONE',  ( 10.72451020669898902, -18.67979575497178502, 107.9155762719810241 ) ) ;
#115039=CARTESIAN_POINT ( 'NONE',  ( -15.80617190586745835, -15.72974639402198527, 56.87390960531436690 ) ) ;
#115040=CARTESIAN_POINT ( 'NONE',  ( -16.51473224551082808, 9.474510206698731452, 93.33442372801900433 ) ) ;
#115041=EDGE_CURVE ( 'NONE', #658, #138021, #18100, .T. ) ;
#115042=CARTESIAN_POINT ( 'NONE',  ( -19.03943276465977164, -0.05219959533935918106, 63.75109039468566863 ) ) ;
#115043=CARTESIAN_POINT ( 'NONE',  ( 21.55341960407619695, -5.719274019375665929, 86.04275706135236135 ) ) ;
#115044=CARTESIAN_POINT ( 'NONE',  ( -5.049401038297874678, -19.05341960407617918, 59.79275706135231871 ) ) ;
#115045=CARTESIAN_POINT ( 'NONE',  ( 19.03943276465977164, -0.05219959533909143690, 23.74890960531435269 ) ) ;
#115046=CARTESIAN_POINT ( 'NONE',  ( -15.72974639402197994, 15.80617190586746368, 60.62390960531437401 ) ) ;
#115047=CARTESIAN_POINT ( 'NONE',  ( -0.05219959533910754901, -16.53943276465976808, 52.49890960531435979 ) ) ;
#115049=CARTESIAN_POINT ( 'NONE',  ( -13.89961937509957401, -13.97604488694547875, 34.37609039468566863 ) ) ;
#115050=CARTESIAN_POINT ( 'NONE',  ( -8.314922557961024197, 14.29746914071037800, 87.91775706135234714 ) ) ;
#115051=CARTESIAN_POINT ( 'NONE',  ( 8.224510206698953496, -14.34966873604960469, 37.91557627198102409 ) ) ;
#115052=CARTESIAN_POINT ( 'NONE',  ( 21.55341960407619695, -5.719274019375665929, 81.04275706135236135 ) ) ;
#115053=CARTESIAN_POINT ( 'NONE',  ( 10.81492255796106328, -18.62759615963255655, 80.41775706135234714 ) ) ;
#115054=CARTESIAN_POINT ( 'NONE',  ( -10.81492255796078084, -18.62759615963271287, 87.08224293864769550 ) ) ;
#115055=CARTESIAN_POINT ( 'NONE',  ( -19.02544592524342804, 5.153800228976336051, 41.04057627198103120 ) ) ;
#115056=CARTESIAN_POINT ( 'NONE',  ( -5.823673210054431948, 21.52544592524334988, 52.70942372801902565 ) ) ;
#115057=CARTESIAN_POINT ( 'NONE',  ( -19.02544592524342804, 5.153800228976336051, 31.04057627198102409 ) ) ;
#115058=CARTESIAN_POINT ( 'NONE',  ( -19.03943276465977164, 0.05219959533909376836, 46.24890960531435979 ) ) ;
#115059=CARTESIAN_POINT ( 'NONE',  ( -4.483927247898539470, -16.52544592524342804, 87.29057627198103830 ) ) ;
#115060=CARTESIAN_POINT ( 'NONE',  ( -16.51473224551069308, -9.474510206698971260, 101.6655762719810241 ) ) ;
#115062=CARTESIAN_POINT ( 'NONE',  ( -12.06949235617756955, 12.14591786802309770, 40.62390960531435269 ) ) ;
#115063=CARTESIAN_POINT ( 'NONE',  ( -8.224510206698948167, 14.34966873604960824, 115.4155762719810241 ) ) ;
#115064=CARTESIAN_POINT ( 'NONE',  ( 0.05219959533907565091, 21.53943276465977519, 79.99890960531435269 ) ) ;
#115066=CARTESIAN_POINT ( 'NONE',  ( 21.55341960407619695, -5.719274019375665929, 26.04275706135235779 ) ) ;
#115068=CARTESIAN_POINT ( 'NONE',  ( 8.224510206698742110, 14.34966873604972548, 32.08442372801901854 ) ) ;
#115069=CARTESIAN_POINT ( 'NONE',  ( 5.823673210054125526, 21.52544592524343514, 64.79057627198103830 ) ) ;
#115070=CARTESIAN_POINT ( 'NONE',  ( -15.72974639402176322, -15.80617190586768395, 99.37609039468568994 ) ) ;
#115071=CARTESIAN_POINT ( 'NONE',  ( -16.51473224551069308, -9.474510206698971260, 96.66557627198102409 ) ) ;
#115072=CARTESIAN_POINT ( 'NONE',  ( -10.72451020669870658, -18.67979575497194134, 29.58442372801901854 ) ) ;
#115073=CARTESIAN_POINT ( 'NONE',  ( -10.72451020669898014, 18.67979575497178502, 25.41557627198103120 ) ) ;
#115074=CARTESIAN_POINT ( 'NONE',  ( 8.224510206698742110, 14.34966873604972548, 87.08442372801901854 ) ) ;
#115075=CARTESIAN_POINT ( 'NONE',  ( -10.81492255796105439, 18.62759615963255655, 67.91775706135234714 ) ) ;
#115076=CARTESIAN_POINT ( 'NONE',  ( 5.719274019375673035, 21.55341960407619339, 112.2927570613523471 ) ) ;
#115077=CARTESIAN_POINT ( 'NONE',  ( -12.14591786802326823, 12.06949235617739902, 73.12609039468567573 ) ) ;
#115078=CARTESIAN_POINT ( 'NONE',  ( -18.62759615963255300, -10.81492255796106328, 24.16775706135235424 ) ) ;
#115079=CARTESIAN_POINT ( 'NONE',  ( 9.474510206698971260, -16.51473224551069308, 32.91557627198102409 ) ) ;
#115080=CARTESIAN_POINT ( 'NONE',  ( -21.52544592524334988, -5.823673210054445271, 103.9594237280190185 ) ) ;
#115081=CARTESIAN_POINT ( 'NONE',  ( 13.97604488694527802, 13.89961937509977652, 109.3739096053143669 ) ) ;
#115082=CARTESIAN_POINT ( 'NONE',  ( -10.81492255796078084, -18.62759615963271287, 102.0822429386476955 ) ) ;
#115084=CARTESIAN_POINT ( 'NONE',  ( 21.52544592524344225, -5.823673210054117533, 68.54057627198103830 ) ) ;
#115085=CARTESIAN_POINT ( 'NONE',  ( -16.55341960407617563, 4.379528057220093196, 53.54275706135234714 ) ) ;
#115086=CARTESIAN_POINT ( 'NONE',  ( -16.55341960407611168, -4.379528057220339221, 46.45724293864769550 ) ) ;
#115088=CARTESIAN_POINT ( 'NONE',  ( 16.46253265017146816, 9.564922557961045513, 81.66775706135233293 ) ) ;
#115089=CARTESIAN_POINT ( 'NONE',  ( -16.79531203550646268, 7.028104445595631411, 103.7475501177956261 ) ) ;
#115090=CARTESIAN_POINT ( 'NONE',  ( 8.224510206698742110, 14.34966873604972548, 27.08442372801901854 ) ) ;
#115091=CARTESIAN_POINT ( 'NONE',  ( -5.719274019375978568, 21.55341960407610458, 90.20724293864770971 ) ) ;
#115092=CARTESIAN_POINT ( 'NONE',  ( 8.224510206698953496, -14.34966873604960469, 62.91557627198102409 ) ) ;
#115093=CARTESIAN_POINT ( 'NONE',  ( 19.03943276465977164, -0.05219959533909143690, 98.74890960531436690 ) ) ;
#115094=CARTESIAN_POINT ( 'NONE',  ( 14.29746914071037800, 8.314922557961029526, 46.66775706135234714 ) ) ;
#115095=CARTESIAN_POINT ( 'NONE',  ( 13.97604488694527802, 13.89961937509977652, 54.37390960531435979 ) ) ;
#115096=CARTESIAN_POINT ( 'NONE',  ( -15.80617190586768217, 15.72974639402176855, 33.12609039468569705 ) ) ;
#115097=CARTESIAN_POINT ( 'NONE',  ( 19.05341960407617918, -5.049401038297876454, 101.0427570613523045 ) ) ;
#115098=CARTESIAN_POINT ( 'NONE',  ( -19.02544592524342804, 5.153800228976336051, 96.04057627198103830 ) ) ;
#115099=CARTESIAN_POINT ( 'NONE',  ( -16.51473224551069308, -9.474510206698971260, 91.66557627198103830 ) ) ;
#115100=CARTESIAN_POINT ( 'NONE',  ( -15.80617190586745835, -15.72974639402198527, 86.87390960531438111 ) ) ;
#115101=CARTESIAN_POINT ( 'NONE',  ( 13.89961937509977652, -13.97604488694527269, 48.12390960531435979 ) ) ;
#115102=CARTESIAN_POINT ( 'NONE',  ( -16.20579543436681291, -7.371946100354976217, 60.56520834171877254 ) ) ;
#115103=CARTESIAN_POINT ( 'NONE',  ( -14.29746914071049879, 8.314922557960819915, 65.83224293864769550 ) ) ;
#115104=CARTESIAN_POINT ( 'NONE',  ( 13.97604488694527802, 13.89961937509977652, 109.3739096053143669 ) ) ;
#115106=CARTESIAN_POINT ( 'NONE',  ( -13.89961937509957401, -13.97604488694547875, 69.37609039468564731 ) ) ;
#115107=CARTESIAN_POINT ( 'NONE',  ( 15.80617190586746368, 15.72974639402197994, 84.37390960531438111 ) ) ;
#115108=CARTESIAN_POINT ( 'NONE',  ( -19.05341960407617563, 5.049401038297882671, 43.54275706135232582 ) ) ;
#115109=CARTESIAN_POINT ( 'NONE',  ( 0.05219959533909260263, 19.03943276465977164, 99.99890960531436690 ) ) ;
#115110=CARTESIAN_POINT ( 'NONE',  ( -15.72974639402197994, 15.80617190586746368, 40.62390960531435269 ) ) ;
#115111=CARTESIAN_POINT ( 'NONE',  ( -16.46253265017160317, 9.564922557960807481, 85.83224293864769550 ) ) ;
#115112=CARTESIAN_POINT ( 'NONE',  ( -21.52544592524334988, -5.823673210054445271, 63.95942372801901854 ) ) ;
#115113=CARTESIAN_POINT ( 'NONE',  ( 9.474510206698971260, -16.51473224551069308, 32.91557627198102409 ) ) ;
#115114=EDGE_CURVE ( 'NONE', #658, #193741, #7299, .T. ) ;
#115115=CARTESIAN_POINT ( 'NONE',  ( -4.379528057220328563, 16.55341960407611168, 70.20724293864769550 ) ) ;
#115116=CARTESIAN_POINT ( 'NONE',  ( 14.29746914071037800, 8.314922557961029526, 26.66775706135235424 ) ) ;
#115117=CARTESIAN_POINT ( 'NONE',  ( -15.72974639402176322, -15.80617190586768395, 54.37609039468568994 ) ) ;
#115119=CARTESIAN_POINT ( 'NONE',  ( -5.153800228976328057, -19.02544592524343514, 107.2905762719810383 ) ) ;
#115120=CARTESIAN_POINT ( 'NONE',  ( -19.03943276465977164, -0.05219959533935918106, 68.75109039468566152 ) ) ;
#115122=CARTESIAN_POINT ( 'NONE',  ( 5.823673210054444382, -21.52544592524334988, 25.20942372801901854 ) ) ;
#115124=CARTESIAN_POINT ( 'NONE',  ( -19.02544592524334988, -5.153800228976617603, 18.95942372801899722 ) ) ;
#115125=CARTESIAN_POINT ( 'NONE',  ( -9.564922557960796823, -16.46253265017161027, 52.08224293864768839 ) ) ;
#115126=CARTESIAN_POINT ( 'NONE',  ( 5.049401038297881783, 19.05341960407617563, 22.29275706135233648 ) ) ;
#115127=CARTESIAN_POINT ( 'NONE',  ( -16.53943276465976808, -0.05219959533934237506, 103.7510903946857042 ) ) ;
#115128=EDGE_CURVE ( 'NONE', #164406, #40349, #130648, .T. ) ;
#115129=CARTESIAN_POINT ( 'NONE',  ( -5.049401038298153566, 19.05341960407611168, 105.2072429386476671 ) ) ;
#115130=CARTESIAN_POINT ( 'NONE',  ( 21.52544592524334988, 5.823673210054432836, 76.45942372801901854 ) ) ;
#115134=CARTESIAN_POINT ( 'NONE',  ( -8.314922557961024197, 14.29746914071037800, 67.91775706135234714 ) ) ;
#115135=CARTESIAN_POINT ( 'NONE',  ( 10.72451020669871369, 18.67979575497193778, 67.08442372801901854 ) ) ;
#115136=CARTESIAN_POINT ( 'NONE',  ( -21.52544592524334988, -5.823673210054445271, 108.9594237280190185 ) ) ;
#115138=CARTESIAN_POINT ( 'NONE',  ( -16.51473224551069308, -9.474510206698971260, 81.66557627198103830 ) ) ;
#115139=CARTESIAN_POINT ( 'NONE',  ( -13.89961937509977652, 13.97604488694528158, 110.6239096053143243 ) ) ;
#115142=CARTESIAN_POINT ( 'NONE',  ( -5.049401038298153566, 19.05341960407611168, 40.20724293864768839 ) ) ;
#115143=CARTESIAN_POINT ( 'NONE',  ( 5.823673210054125526, 21.52544592524343514, 44.79057627198103120 ) ) ;
#115144=CARTESIAN_POINT ( 'NONE',  ( 16.55341960407618274, -4.379528057220086978, 111.0427570613523613 ) ) ;
#115145=CARTESIAN_POINT ( 'NONE',  ( -12.06949235617756955, 12.14591786802309770, 100.6239096053143811 ) ) ;
#115146=CARTESIAN_POINT ( 'NONE',  ( -19.02544592524342804, 5.153800228976336051, 86.04057627198103830 ) ) ;
#115147=CARTESIAN_POINT ( 'NONE',  ( 5.823673210054444382, -21.52544592524334988, 110.2094237280190185 ) ) ;
#115148=CARTESIAN_POINT ( 'NONE',  ( -13.89961937509977652, 13.97604488694528158, 35.62390960531435269 ) ) ;
#115149=CARTESIAN_POINT ( 'NONE',  ( -0.05219959533910754901, -16.53943276465976808, 87.49890960531436690 ) ) ;
#115150=CARTESIAN_POINT ( 'NONE',  ( -21.55341960407619339, 5.719274019375674811, 48.54275706135234714 ) ) ;
#115151=CARTESIAN_POINT ( 'NONE',  ( -15.72974639402197994, 15.80617190586746368, 85.62390960531436690 ) ) ;
#115152=CARTESIAN_POINT ( 'NONE',  ( 16.51473224551083163, -9.474510206698727899, 45.83442372801900433 ) ) ;
#115153=CARTESIAN_POINT ( 'NONE',  ( -16.51473224551069308, -9.474510206698971260, 46.66557627198102409 ) ) ;
#115154=CARTESIAN_POINT ( 'NONE',  ( -13.89961937509977652, 13.97604488694528158, 100.6239096053143669 ) ) ;
#115155=CARTESIAN_POINT ( 'NONE',  ( -8.224510206698948167, 14.34966873604960824, 65.41557627198102409 ) ) ;
#115157=CARTESIAN_POINT ( 'NONE',  ( 19.03943276465977164, 0.05219959533936151252, 46.25109039468566863 ) ) ;
#115158=CARTESIAN_POINT ( 'NONE',  ( 8.314922557960818139, 14.29746914071049879, 49.58224293864769550 ) ) ;
#115159=CARTESIAN_POINT ( 'NONE',  ( -9.474510206698720793, -16.51473224551083518, 79.58442372801899012 ) ) ;
#115160=CARTESIAN_POINT ( 'NONE',  ( -9.474510206698720793, -16.51473224551083518, 89.58442372801900433 ) ) ;
#115161=CARTESIAN_POINT ( 'NONE',  ( -10.72451020669898014, 18.67979575497178502, 30.41557627198101699 ) ) ;
#115162=CARTESIAN_POINT ( 'NONE',  ( -16.55341960407611168, -4.379528057220339221, 96.45724293864770971 ) ) ;
#115164=CARTESIAN_POINT ( 'NONE',  ( 19.02544592524343514, -5.153800228976328945, 48.54057627198103120 ) ) ;
#115165=CARTESIAN_POINT ( 'NONE',  ( 10.81492255796078972, 18.62759615963270932, 54.58224293864769550 ) ) ;
#115166=CARTESIAN_POINT ( 'NONE',  ( 16.46253265017160672, -9.564922557960803928, 28.33224293864769550 ) ) ;
#115167=CARTESIAN_POINT ( 'NONE',  ( -8.224510206698735004, -14.34966873604973081, 79.58442372801903275 ) ) ;
#115168=CARTESIAN_POINT ( 'NONE',  ( 9.474510206698971260, -16.51473224551069308, 62.91557627198102409 ) ) ;
#115169=CARTESIAN_POINT ( 'NONE',  ( 13.89961937509957401, 13.97604488694547697, 36.87609039468565442 ) ) ;
#115170=CARTESIAN_POINT ( 'NONE',  ( -5.719274019375665041, -21.55341960407619695, 64.79275706135234714 ) ) ;
#115171=CARTESIAN_POINT ( 'NONE',  ( -5.823673210054116645, -21.52544592524344225, 47.29057627198103120 ) ) ;
#115172=CARTESIAN_POINT ( 'NONE',  ( 9.474510206698971260, -16.51473224551069308, 22.91557627198102765 ) ) ;
#115173=CARTESIAN_POINT ( 'NONE',  ( 19.05341960407617918, -5.049401038297876454, 101.0427570613523045 ) ) ;
#115176=CARTESIAN_POINT ( 'NONE',  ( -18.67979575497178146, -10.72451020669898902, 41.66557627198103120 ) ) ;
#115177=CARTESIAN_POINT ( 'NONE',  ( 16.79531203550645913, -7.028104445595738881, 66.24755011779559766 ) ) ;
#115178=CARTESIAN_POINT ( 'NONE',  ( -21.53943276465977519, -0.05219959533937600094, 88.75109039468567573 ) ) ;
#115179=CARTESIAN_POINT ( 'NONE',  ( -0.05219959533910754901, -16.53943276465976808, 42.49890960531435979 ) ) ;
#115180=CARTESIAN_POINT ( 'NONE',  ( -16.52544592524342804, 4.483927247898546575, 61.04057627198103120 ) ) ;
#115181=CARTESIAN_POINT ( 'NONE',  ( 10.72451020669898902, -18.67979575497178502, 87.91557627198103830 ) ) ;
#115182=CARTESIAN_POINT ( 'NONE',  ( -15.72974639402197994, 15.80617190586746368, 80.62390960531438111 ) ) ;
#115184=CARTESIAN_POINT ( 'NONE',  ( 18.62759615963271287, -10.81492255796078972, 38.33224293864768839 ) ) ;
#115185=CARTESIAN_POINT ( 'NONE',  ( -4.483927247898782831, 16.52544592524335698, 52.70942372801902565 ) ) ;
#115186=CARTESIAN_POINT ( 'NONE',  ( -4.483927247898539470, -16.52544592524342804, 82.29057627198103830 ) ) ;
#115187=CARTESIAN_POINT ( 'NONE',  ( -13.97604488694527625, -13.89961937509977652, 66.87390960531436690 ) ) ;
#115188=CARTESIAN_POINT ( 'NONE',  ( -19.03943276465977164, 0.05219959533909376836, 26.24890960531435624 ) ) ;
#115189=DIRECTION ( 'NONE',  ( -1.000000000000000000, 0.000000000000000000, -0.000000000000000000 ) ) ;
#115190=VERTEX_POINT ( 'NONE', #192342 ) ;
#115191=CARTESIAN_POINT ( 'NONE',  ( -8.314922557961024197, 14.29746914071037800, 77.91775706135231871 ) ) ;
#115192=CARTESIAN_POINT ( 'NONE',  ( 5.823673210054125526, 21.52544592524343514, 114.7905762719810383 ) ) ;
#115193=CARTESIAN_POINT ( 'NONE',  ( 13.97604488694527802, 13.89961937509977652, 84.37390960531433848 ) ) ;
#115194=CARTESIAN_POINT ( 'NONE',  ( 10.72451020669871369, 18.67979575497193778, 52.08442372801901854 ) ) ;
#115195=CARTESIAN_POINT ( 'NONE',  ( 16.46253265017160672, -9.564922557960803928, 108.3322429386476955 ) ) ;
#115197=VERTEX_POINT ( 'NONE', #141831 ) ;
#115198=CARTESIAN_POINT ( 'NONE',  ( 10.81492255796106328, -18.62759615963255655, 40.41775706135234714 ) ) ;
#115199=CARTESIAN_POINT ( 'NONE',  ( 16.46253265017160672, -9.564922557960803928, 38.33224293864768839 ) ) ;
#115200=CARTESIAN_POINT ( 'NONE',  ( -9.564922557960796823, -16.46253265017161027, 102.0822429386477097 ) ) ;
#115201=CARTESIAN_POINT ( 'NONE',  ( 5.153800228976615827, -19.02544592524334988, 50.20942372801897591 ) ) ;
#115202=CARTESIAN_POINT ( 'NONE',  ( -21.52544592524343514, 5.823673210054127303, 116.0405762719810383 ) ) ;
#115203=CARTESIAN_POINT ( 'NONE',  ( 13.89961937509957401, 13.97604488694547697, 41.87609039468566152 ) ) ;
#115204=CARTESIAN_POINT ( 'NONE',  ( -19.05341960407611168, -5.049401038298163336, 26.45724293864769550 ) ) ;
#115205=CARTESIAN_POINT ( 'NONE',  ( 8.224510206698742110, 14.34966873604972548, 97.08442372801904696 ) ) ;
#115206=CARTESIAN_POINT ( 'NONE',  ( 13.89961937509957401, 13.97604488694547697, 56.87609039468564731 ) ) ;
#115207=CARTESIAN_POINT ( 'NONE',  ( -8.224510206698735004, -14.34966873604973081, 104.5844237280190185 ) ) ;
#115209=CARTESIAN_POINT ( 'NONE',  ( -16.51473224551069308, -9.474510206698971260, 81.66557627198103830 ) ) ;
#115210=CARTESIAN_POINT ( 'NONE',  ( 18.67979575497194134, -10.72451020669871369, 90.83442372801901854 ) ) ;
#115211=CARTESIAN_POINT ( 'NONE',  ( 0.05219959533937995610, -21.53943276465977519, 110.0010903946856757 ) ) ;
#115212=CARTESIAN_POINT ( 'NONE',  ( -19.05341960407611168, -5.049401038298163336, 21.45724293864768839 ) ) ;
#115213=CARTESIAN_POINT ( 'NONE',  ( 9.474510206698971260, -16.51473224551069308, 102.9155762719810241 ) ) ;
#115214=CARTESIAN_POINT ( 'NONE',  ( -5.823673210054431948, 21.52544592524334988, 77.70942372801900433 ) ) ;
#115215=CARTESIAN_POINT ( 'NONE',  ( 4.483927247898790824, -16.52544592524335698, 25.20942372801901854 ) ) ;
#115216=CARTESIAN_POINT ( 'NONE',  ( -5.153800228976328057, -19.02544592524343514, 77.29057627198099567 ) ) ;
#115217=CARTESIAN_POINT ( 'NONE',  ( -21.52544592524343514, 5.823673210054127303, 36.04057627198102409 ) ) ;
#115219=CARTESIAN_POINT ( 'NONE',  ( -16.51473224551069308, -9.474510206698971260, 86.66557627198102409 ) ) ;
#115220=CARTESIAN_POINT ( 'NONE',  ( -16.21995358207303894, -7.366697692864244473, 90.06448998487844904 ) ) ;
#115221=CARTESIAN_POINT ( 'NONE',  ( -0.05219959533909027116, -19.03943276465977164, 82.49890960531436690 ) ) ;
#115222=CARTESIAN_POINT ( 'NONE',  ( -9.474510206698964154, 16.51473224551069663, 60.41557627198102409 ) ) ;
#115223=CARTESIAN_POINT ( 'NONE',  ( -4.483927247898782831, 16.52544592524335698, 97.70942372801904696 ) ) ;
#115224=CARTESIAN_POINT ( 'NONE',  ( -17.12812012977049747, 6.668231424565647991, 98.64051240676855059 ) ) ;
#115225=CARTESIAN_POINT ( 'NONE',  ( 19.03943276465977164, 0.05219959533936151252, 61.25109039468566863 ) ) ;
#115226=CARTESIAN_POINT ( 'NONE',  ( 0.05219959533909260263, 19.03943276465977164, 94.99890960531436690 ) ) ;
#115227=CARTESIAN_POINT ( 'NONE',  ( 14.34966873604960469, 8.224510206698951720, 79.16557627198103830 ) ) ;
#115228=CARTESIAN_POINT ( 'NONE',  ( -10.81492255796078084, -18.62759615963271287, 37.08224293864768129 ) ) ;
#115229=( BOUNDED_CURVE ( )  B_SPLINE_CURVE ( 2, ( #30745, #75252, #197620, #108566, #63052, #91387, #154080, #15574, #13585, #139884, #199598, #60078, #151123, #45908, #61065, #59085, #122737, #123718, #105593, #120752, #77232, #46906, #184428, #27793, #167279, #62053, #138901, #170244, #31738, #28777, #1373, #186429, #166297, #12616, #74280, #135950, #90416, #190388, #68026, #144863, #20525, #188404, #36682, #191375, #4349, #67032, #126700, #98342, #49882, #111547, #96365, #35699, #143869, #173232, #34708, #80207, #65044, #158053, #19543, #50878, #95377, #109559, #175217, #141878, #125727, #82173, #128691, #140887, #81188, #51863, #48894, #2377, #5348, #187426, #142870, #66034, #127701, #189401, #112536, #97346, #172230, #110549, #160041, #113523, #171240 ),
 .UNSPECIFIED., .F., .F. ) 
 B_SPLINE_CURVE_WITH_KNOTS ( ( 3, 2, 2, 2, 2, 2, 2, 2, 2, 2, 2, 2, 2, 2, 2, 2, 2, 2, 2, 2, 2, 2, 2, 2, 2, 2, 2, 2, 2, 2, 2, 2, 2, 2, 2, 2, 2, 2, 2, 2, 2, 2, 3 ),
 ( 0.8182199101112557216, 0.8201754385964912242, 0.8245614035087719396, 0.8289473684210526550, 0.8333333333333333703, 0.8377192982456140857, 0.8421052631578946901, 0.8464912280701754055, 0.8508771929824561209, 0.8552631578947368363, 0.8596491228070175517, 0.8640350877192982670, 0.8684210526315789824, 0.8728070175438596978, 0.8771929824561403022, 0.8815789473684210176, 0.8859649122807017330, 0.8903508771929824483, 0.8947368421052631637, 0.8991228070175438791, 0.9035087719298245945, 0.9078947368421053099, 0.9122807017543859143, 0.9166666666666666297, 0.9210526315789473450, 0.9254385964912280604, 0.9298245614035087758, 0.9342105263157894912, 0.9385964912280702066, 0.9429824561403509220, 0.9473684210526315264, 0.9517543859649122417, 0.9561403508771929571, 0.9605263157894736725, 0.9649122807017543879, 0.9692982456140351033, 0.9736842105263158187, 0.9780701754385965341, 0.9824561403508771384, 0.9868421052631578538, 0.9912280701754385692, 0.9956140350877192846, 1.000000000000000000 ),
 .UNSPECIFIED. ) 
 CURVE ( )  GEOMETRIC_REPRESENTATION_ITEM ( )  RATIONAL_B_SPLINE_CURVE ( ( 0.9831626618144007068, 0.9848076720550096308, 1.000000000000000000, 0.9659258262890683122, 1.000000000000000000, 0.9659258262890683122, 1.000000000000000000, 0.9659258262890683122, 1.000000000000000000, 0.9659258262890683122, 1.000000000000000000, 0.9659258262890683122, 1.000000000000000000, 0.9659258262890683122, 1.000000000000000000, 0.9659258262890683122, 1.000000000000000000, 0.9659258262890683122, 1.000000000000000000, 0.9659258262890683122, 1.000000000000000000, 0.9659258262890683122, 1.000000000000000000, 0.9659258262890683122, 1.000000000000000000, 0.9659258262890683122, 1.000000000000000000, 0.9659258262890683122, 1.000000000000000000, 0.9659258262890683122, 1.000000000000000000, 0.9659258262890683122, 1.000000000000000000, 0.9659258262890683122, 1.000000000000000000, 0.9659258262890683122, 1.000000000000000000, 0.9659258262890683122, 1.000000000000000000, 0.9659258262890683122, 1.000000000000000000, 0.9659258262890683122, 1.000000000000000000, 0.9659258262890683122, 1.000000000000000000, 0.9659258262890683122, 1.000000000000000000, 0.9659258262890683122, 1.000000000000000000, 0.9659258262890683122, 1.000000000000000000, 0.9659258262890683122, 1.000000000000000000, 0.9659258262890683122, 1.000000000000000000, 0.9659258262890683122, 1.000000000000000000, 0.9659258262890683122, 1.000000000000000000, 0.9659258262890683122, 1.000000000000000000, 0.9659258262890683122, 1.000000000000000000, 0.9659258262890683122, 1.000000000000000000, 0.9659258262890683122, 1.000000000000000000, 0.9659258262890683122, 1.000000000000000000, 0.9659258262890683122, 1.000000000000000000, 0.9659258262890683122, 1.000000000000000000, 0.9659258262890683122, 1.000000000000000000, 0.9659258262890683122, 1.000000000000000000, 0.9659258262890683122, 1.000000000000000000, 0.9659258262890683122, 1.000000000000000000, 0.9659258262890683122, 1.000000000000000000, 0.9659258262890683122, 1.000000000000000000 ) ) 
 REPRESENTATION_ITEM ( '' )  );
#115230=CARTESIAN_POINT ( 'NONE',  ( 0.05219959533907565091, 21.53943276465977519, 24.99890960531435624 ) ) ;
#115231=CARTESIAN_POINT ( 'NONE',  ( -16.52544592524342804, 4.483927247898546575, 86.04057627198102409 ) ) ;
#115232=CARTESIAN_POINT ( 'NONE',  ( -17.48847506799969054, 5.747544572773785276, 55.82697437843281563 ) ) ;
#115233=CARTESIAN_POINT ( 'NONE',  ( -9.474510206698720793, -16.51473224551083518, 39.58442372801899722 ) ) ;
#115234=CARTESIAN_POINT ( 'NONE',  ( -12.14591786802309592, -12.06949235617757132, 21.87390960531436690 ) ) ;
#115235=CARTESIAN_POINT ( 'NONE',  ( 19.03943276465977164, -0.05219959533909143690, 103.7489096053143669 ) ) ;
#115236=CARTESIAN_POINT ( 'NONE',  ( 21.55341960407619695, -5.719274019375665929, 66.04275706135236135 ) ) ;
#115237=CARTESIAN_POINT ( 'NONE',  ( -18.67979575497178146, -10.72451020669898902, 56.66557627198103830 ) ) ;
#115238=CARTESIAN_POINT ( 'NONE',  ( -10.81492255796105439, 18.62759615963255655, 32.91775706135234714 ) ) ;
#115239=CARTESIAN_POINT ( 'NONE',  ( 21.55341960407610458, 5.719274019375980345, 88.95724293864769550 ) ) ;
#115240=CARTESIAN_POINT ( 'NONE',  ( 0.05219959533937995610, -21.53943276465977519, 35.00109039468568284 ) ) ;
#115241=CARTESIAN_POINT ( 'NONE',  ( -14.34966873604960291, -8.224510206698953496, 106.6655762719810383 ) ) ;
#115242=CARTESIAN_POINT ( 'NONE',  ( -5.153800228976607833, 19.02544592524334988, 72.70942372801900433 ) ) ;
#115243=CARTESIAN_POINT ( 'NONE',  ( 16.46253265017160672, -9.564922557960803928, 43.33224293864769550 ) ) ;
#115244=CARTESIAN_POINT ( 'NONE',  ( -16.55341960407611168, -4.379528057220339221, 91.45724293864769550 ) ) ;
#115245=CARTESIAN_POINT ( 'NONE',  ( -16.46253265017160317, 9.564922557960807481, 90.83224293864769550 ) ) ;
#115246=CARTESIAN_POINT ( 'NONE',  ( -9.474510206698964154, 16.51473224551069663, 90.41557627198103830 ) ) ;
#115247=CARTESIAN_POINT ( 'NONE',  ( 4.379528057220339221, -16.55341960407611168, 107.7072429386476955 ) ) ;
#115248=CARTESIAN_POINT ( 'NONE',  ( -14.29746914071049879, 8.314922557960819915, 35.83224293864768839 ) ) ;
#115249=CARTESIAN_POINT ( 'NONE',  ( -4.379528057220086978, -16.55341960407618274, 104.7927570613523898 ) ) ;
#115250=CARTESIAN_POINT ( 'NONE',  ( 9.564922557960805705, 16.46253265017160317, 54.58224293864769550 ) ) ;
#115251=CARTESIAN_POINT ( 'NONE',  ( 14.34966873604960469, 8.224510206698951720, 114.1655762719810383 ) ) ;
#115252=CARTESIAN_POINT ( 'NONE',  ( 19.03943276465977164, 0.05219959533936151252, 26.25109039468566507 ) ) ;
#115253=CARTESIAN_POINT ( 'NONE',  ( 16.51473224551069308, 9.474510206698969483, 109.1655762719810383 ) ) ;
#115254=CARTESIAN_POINT ( 'NONE',  ( -14.34966873604960291, -8.224510206698953496, 21.66557627198102409 ) ) ;
#115255=CARTESIAN_POINT ( 'NONE',  ( 5.823673210054444382, -21.52544592524334988, 40.20942372801901854 ) ) ;
#115256=CARTESIAN_POINT ( 'NONE',  ( 9.474510206698971260, -16.51473224551069308, 107.9155762719810383 ) ) ;
#115257=CARTESIAN_POINT ( 'NONE',  ( -8.314922557961024197, 14.29746914071037800, 47.91775706135234714 ) ) ;
#115258=CARTESIAN_POINT ( 'NONE',  ( 4.379528057220092307, 16.55341960407617563, 107.2927570613523471 ) ) ;
#115259=CARTESIAN_POINT ( 'NONE',  ( -13.89961937509977652, 13.97604488694528158, 45.62390960531433848 ) ) ;
#115260=CARTESIAN_POINT ( 'NONE',  ( -16.53943276465976808, -0.05219959533934237506, 93.75109039468567573 ) ) ;
#115261=CARTESIAN_POINT ( 'NONE',  ( 8.314922557961029526, -14.29746914071037800, 20.41775706135234714 ) ) ;
#115262=CARTESIAN_POINT ( 'NONE',  ( -13.97604488694527625, -13.89961937509977652, 46.87390960531435979 ) ) ;
#115263=CARTESIAN_POINT ( 'NONE',  ( -0.05219959533910754901, -16.53943276465976808, 107.4989096053143669 ) ) ;
#115264=CARTESIAN_POINT ( 'NONE',  ( -18.62759615963270932, 10.81492255796079327, 110.8322429386476955 ) ) ;
#115265=CARTESIAN_POINT ( 'NONE',  ( 16.46253265017160672, -9.564922557960803928, 33.33224293864770260 ) ) ;
#115266=CARTESIAN_POINT ( 'NONE',  ( -9.474510206698964154, 16.51473224551069663, 100.4155762719810241 ) ) ;
#115267=CARTESIAN_POINT ( 'NONE',  ( -13.89961937509977652, 13.97604488694528158, 35.62390960531435269 ) ) ;
#115268=CARTESIAN_POINT ( 'NONE',  ( 5.153800228976335163, 19.02544592524342804, 99.79057627198102409 ) ) ;
#115269=CARTESIAN_POINT ( 'NONE',  ( -16.62475595723697808, -7.163666690055197073, 34.47286648189534475 ) ) ;
#115270=CARTESIAN_POINT ( 'NONE',  ( 9.564922557960805705, 16.46253265017160317, 94.58224293864769550 ) ) ;
#115271=CARTESIAN_POINT ( 'NONE',  ( -21.55341960407619339, 5.719274019375674811, 43.54275706135235424 ) ) ;
#115272=CARTESIAN_POINT ( 'NONE',  ( -14.34966873604960291, -8.224510206698953496, 101.6655762719810383 ) ) ;
#115273=CARTESIAN_POINT ( 'NONE',  ( -0.05219959533909027116, -19.03943276465977164, 107.4989096053143527 ) ) ;
#115274=CARTESIAN_POINT ( 'NONE',  ( 17.60769864724391098, -5.499999999999974243, 96.15024842019167295 ) ) ;
#115275=CARTESIAN_POINT ( 'NONE',  ( -16.52544592524335698, -4.483927247898792601, 63.95942372801901854 ) ) ;
#115276=CARTESIAN_POINT ( 'NONE',  ( -10.72451020669870658, -18.67979575497194134, 94.58442372801901854 ) ) ;
#115277=CARTESIAN_POINT ( 'NONE',  ( 8.314922557961029526, -14.29746914071037800, 35.41775706135234003 ) ) ;
#115278=CARTESIAN_POINT ( 'NONE',  ( 5.153800228976335163, 19.02544592524342804, 84.79057627198099567 ) ) ;
#115280=CARTESIAN_POINT ( 'NONE',  ( -9.564922557961040184, 16.46253265017147172, 112.9177570613523329 ) ) ;
#115281=CARTESIAN_POINT ( 'NONE',  ( 12.14591786802327356, -12.06949235617739191, 85.62609039468568994 ) ) ;
#115282=CARTESIAN_POINT ( 'NONE',  ( -19.02544592524334988, -5.153800228976617603, 88.95942372801897591 ) ) ;
#115283=CARTESIAN_POINT ( 'NONE',  ( 9.474510206698971260, -16.51473224551069308, 72.91557627198102409 ) ) ;
#115284=CARTESIAN_POINT ( 'NONE',  ( -15.72974639402197994, 15.80617190586746368, 100.6239096053143811 ) ) ;
#115285=CARTESIAN_POINT ( 'NONE',  ( -8.314922557960811034, -14.29746914071050412, 92.08224293864769550 ) ) ;
#115286=CARTESIAN_POINT ( 'NONE',  ( -13.97604488694547697, 13.89961937509957934, 88.12609039468563310 ) ) ;
#115287=CARTESIAN_POINT ( 'NONE',  ( 16.52544592524335698, 4.483927247898782831, 76.45942372801901854 ) ) ;
#115289=CARTESIAN_POINT ( 'NONE',  ( 9.474510206698729675, 16.51473224551082808, 72.08442372801900433 ) ) ;
#115290=CARTESIAN_POINT ( 'NONE',  ( 16.52544592524342804, -4.483927247898539470, 28.54057627198103120 ) ) ;
#115291=CARTESIAN_POINT ( 'NONE',  ( 14.34966873604960469, 8.224510206698951720, 94.16557627198103830 ) ) ;
#115292=CARTESIAN_POINT ( 'NONE',  ( -16.46253265017146816, -9.564922557961047289, 24.16775706135233648 ) ) ;
#115293=CARTESIAN_POINT ( 'NONE',  ( -19.02130022317638591, 5.499999999999807265, 90.78188669246574705 ) ) ;
#115294=CARTESIAN_POINT ( 'NONE',  ( -21.55341960407619339, 5.719274019375674811, 28.54275706135234358 ) ) ;
#115295=FACE_OUTER_BOUND ( 'NONE', #75407, .T. ) ;
#115296=CARTESIAN_POINT ( 'NONE',  ( -5.049401038298153566, 19.05341960407611168, 75.20724293864769550 ) ) ;
#115297=CARTESIAN_POINT ( 'NONE',  ( -21.55341960407619339, 5.719274019375674811, 98.54275706135234714 ) ) ;
#115298=CARTESIAN_POINT ( 'NONE',  ( -16.46253265017160317, 9.564922557960807481, 70.83224293864770971 ) ) ;
#115299=CARTESIAN_POINT ( 'NONE',  ( 5.719274019375991003, -21.55341960407610458, 42.70724293864770260 ) ) ;
#115300=CARTESIAN_POINT ( 'NONE',  ( 12.14591786802309770, 12.06949235617756955, 74.37390960531436690 ) ) ;
#115301=CARTESIAN_POINT ( 'NONE',  ( 9.564922557960805705, 16.46253265017160317, 54.58224293864769550 ) ) ;
#115302=CARTESIAN_POINT ( 'NONE',  ( -8.314922557960811034, -14.29746914071050412, 107.0822429386476955 ) ) ;
#115304=CARTESIAN_POINT ( 'NONE',  ( 15.72974639402176855, 15.80617190586768217, 31.87609039468567929 ) ) ;
#115305=CARTESIAN_POINT ( 'NONE',  ( -10.81492255796105439, 18.62759615963255655, 57.91775706135234714 ) ) ;
#115306=CARTESIAN_POINT ( 'NONE',  ( 16.51473224551069308, 9.474510206698969483, 44.16557627198103120 ) ) ;
#115307=CARTESIAN_POINT ( 'NONE',  ( -12.06949235617739369, -12.14591786802326823, 74.37609039468568994 ) ) ;
#115309=CARTESIAN_POINT ( 'NONE',  ( 15.72974639402199770, -15.80617190586745480, 108.1239096053143811 ) ) ;
#115310=VERTEX_POINT ( 'NONE', #21481 ) ;
#115311=CARTESIAN_POINT ( 'NONE',  ( 15.80617190586746368, 15.72974639402197994, 114.3739096053143527 ) ) ;
#115312=CARTESIAN_POINT ( 'NONE',  ( 0.05219959533936267826, -19.03943276465977164, 40.00109039468566152 ) ) ;
#115313=CARTESIAN_POINT ( 'NONE',  ( -0.05219959533909027116, -19.03943276465977164, 62.49890960531435979 ) ) ;
#115314=CARTESIAN_POINT ( 'NONE',  ( 9.564922557961047289, -16.46253265017146816, 30.41775706135232937 ) ) ;
#115315=CARTESIAN_POINT ( 'NONE',  ( 18.62759615963255655, 10.81492255796105972, 71.66775706135234714 ) ) ;
#115316=CARTESIAN_POINT ( 'NONE',  ( -21.55341960407610458, -5.719274019375992779, 66.45724293864768129 ) ) ;
#115317=CARTESIAN_POINT ( 'NONE',  ( -16.52544592524342804, 4.483927247898546575, 36.04057627198102409 ) ) ;
#115318=CARTESIAN_POINT ( 'NONE',  ( -21.53943276465977519, -0.05219959533937600094, 83.75109039468568994 ) ) ;
#115319=CARTESIAN_POINT ( 'NONE',  ( 9.564922557961047289, -16.46253265017146816, 30.41775706135232937 ) ) ;
#115320=CARTESIAN_POINT ( 'NONE',  ( 16.52544592524342804, -4.483927247898539470, 58.54057627198103120 ) ) ;
#115321=CARTESIAN_POINT ( 'NONE',  ( 14.34966873604960469, 8.224510206698951720, 109.1655762719810383 ) ) ;
#115322=CARTESIAN_POINT ( 'NONE',  ( -19.03943276465977164, -0.05219959533935918106, 58.75109039468566863 ) ) ;
#115323=CARTESIAN_POINT ( 'NONE',  ( -14.34966873604972548, 8.224510206698743886, 108.3344237280190185 ) ) ;
#115325=CARTESIAN_POINT ( 'NONE',  ( 10.81492255796106328, -18.62759615963255655, 65.41775706135234714 ) ) ;
#115326=CARTESIAN_POINT ( 'NONE',  ( 9.564922557960805705, 16.46253265017160317, 69.58224293864770971 ) ) ;
#115327=CARTESIAN_POINT ( 'NONE',  ( -19.05341960407617563, 5.049401038297882671, 53.54275706135231871 ) ) ;
#115328=CARTESIAN_POINT ( 'NONE',  ( -18.62759615963270932, 10.81492255796079327, 50.83224293864770971 ) ) ;
#115329=CARTESIAN_POINT ( 'NONE',  ( 10.72451020669871369, 18.67979575497193778, 47.08442372801901854 ) ) ;
#115330=CARTESIAN_POINT ( 'NONE',  ( -0.05219959533907301413, -21.53943276465977519, 102.4989096053143811 ) ) ;
#115331=CARTESIAN_POINT ( 'NONE',  ( 9.474510206698729675, 16.51473224551082808, 97.08442372801900433 ) ) ;
#115332=CARTESIAN_POINT ( 'NONE',  ( -16.53943276465976808, -0.05219959533934237506, 63.75109039468568284 ) ) ;
#115334=CARTESIAN_POINT ( 'NONE',  ( 10.81492255796078972, 18.62759615963270932, 109.5822429386476955 ) ) ;
#115335=CARTESIAN_POINT ( 'NONE',  ( -16.52544592524342804, 4.483927247898546575, 91.04057627198103830 ) ) ;
#115336=CARTESIAN_POINT ( 'NONE',  ( -16.38665767535054130, -7.295008042176132079, 99.73599135785453029 ) ) ;
#115337=CARTESIAN_POINT ( 'NONE',  ( -12.14591786802326823, 12.06949235617739902, 23.12609039468567573 ) ) ;
#115339=CARTESIAN_POINT ( 'NONE',  ( 5.823673210054125526, 21.52544592524343514, 44.79057627198103120 ) ) ;
#115340=CARTESIAN_POINT ( 'NONE',  ( -14.34966873604972548, 8.224510206698743886, 93.33442372801901854 ) ) ;
#115342=CARTESIAN_POINT ( 'NONE',  ( -4.379528057220086978, -16.55341960407618274, 64.79275706135234714 ) ) ;
#115343=CARTESIAN_POINT ( 'NONE',  ( 5.823673210054444382, -21.52544592524334988, 35.20942372801901854 ) ) ;
#115344=CARTESIAN_POINT ( 'NONE',  ( -21.53943276465977519, 0.05219959533907696930, 41.24890960531435269 ) ) ;
#115345=CARTESIAN_POINT ( 'NONE',  ( -16.52544592524335698, -4.483927247898792601, 83.95942372801900433 ) ) ;
#115346=CARTESIAN_POINT ( 'NONE',  ( -5.153800228976328057, -19.02544592524343514, 92.29057627198099567 ) ) ;
#115347=CARTESIAN_POINT ( 'NONE',  ( 18.62759615963255655, 10.81492255796105972, 66.66775706135234714 ) ) ;
#115348=CARTESIAN_POINT ( 'NONE',  ( 0.05219959533907565091, 21.53943276465977519, 34.99890960531435979 ) ) ;
#115349=CARTESIAN_POINT ( 'NONE',  ( 18.67979575497178502, 10.72451020669898547, 39.16557627198102409 ) ) ;
#115351=CARTESIAN_POINT ( 'NONE',  ( -19.02544592524334988, -5.153800228976617603, 48.95942372801900433 ) ) ;
#115352=CARTESIAN_POINT ( 'NONE',  ( -8.314922557961024197, 14.29746914071037800, 67.91775706135234714 ) ) ;
#115353=CARTESIAN_POINT ( 'NONE',  ( -21.52544592524343514, 5.823673210054127303, 36.04057627198102409 ) ) ;
#115355=CARTESIAN_POINT ( 'NONE',  ( -5.049401038298153566, 19.05341960407611168, 90.20724293864766707 ) ) ;
#115356=CARTESIAN_POINT ( 'NONE',  ( 14.29746914071037800, 8.314922557961029526, 111.6677570613523613 ) ) ;
#115358=CARTESIAN_POINT ( 'NONE',  ( 8.224510206698953496, -14.34966873604960469, 107.9155762719810241 ) ) ;
#115359=CARTESIAN_POINT ( 'NONE',  ( -15.80617190586745835, -15.72974639402198527, 51.87390960531437401 ) ) ;
#115360=CARTESIAN_POINT ( 'NONE',  ( -9.474510206698964154, 16.51473224551069663, 45.41557627198103120 ) ) ;
#115361=CARTESIAN_POINT ( 'NONE',  ( 12.06949235617739724, 12.14591786802326823, 86.87609039468568994 ) ) ;
#115362=CARTESIAN_POINT ( 'NONE',  ( 21.53943276465977519, 0.05219959533937863772, 36.25109039468567573 ) ) ;
#115363=CARTESIAN_POINT ( 'NONE',  ( -9.474510206698720793, -16.51473224551083518, 89.58442372801900433 ) ) ;
#115364=CARTESIAN_POINT ( 'NONE',  ( 16.52544592524342804, -4.483927247898539470, 88.54057627198103830 ) ) ;
#115365=CARTESIAN_POINT ( 'NONE',  ( 5.049401038298161559, -19.05341960407611168, 57.70724293864769550 ) ) ;
#115366=VECTOR ( 'NONE', #196955, 1000.000000000000000 ) ;
#115367=CARTESIAN_POINT ( 'NONE',  ( -0.05219959533909027116, -19.03943276465977164, 27.49890960531435624 ) ) ;
#115368=CARTESIAN_POINT ( 'NONE',  ( 18.67979575497194134, -10.72451020669871369, 105.8344237280190328 ) ) ;
#115369=CARTESIAN_POINT ( 'NONE',  ( -19.05341960407611168, -5.049401038298163336, 81.45724293864769550 ) ) ;
#115370=CARTESIAN_POINT ( 'NONE',  ( -12.06949235617739369, -12.14591786802326823, 64.37609039468568994 ) ) ;
#115371=CARTESIAN_POINT ( 'NONE',  ( -21.55341960407619339, 5.719274019375674811, 88.54275706135236135 ) ) ;
#115372=CARTESIAN_POINT ( 'NONE',  ( 10.81492255796078972, 18.62759615963270932, 44.58224293864769550 ) ) ;
#115373=CARTESIAN_POINT ( 'NONE',  ( -16.52544592524335698, -4.483927247898792601, 68.95942372801901854 ) ) ;
#115374=CARTESIAN_POINT ( 'NONE',  ( -13.89961937509957401, -13.97604488694547875, 54.37609039468565442 ) ) ;
#115375=CARTESIAN_POINT ( 'NONE',  ( 13.97604488694548053, -13.89961937509957401, 65.62609039468567573 ) ) ;
#115377=CARTESIAN_POINT ( 'NONE',  ( -18.67979575497193778, 10.72451020669871902, 58.33442372801901143 ) ) ;
#115378=CARTESIAN_POINT ( 'NONE',  ( -13.89961937509977652, 13.97604488694528158, 65.62390960531436690 ) ) ;
#115379=CARTESIAN_POINT ( 'NONE',  ( -5.049401038298153566, 19.05341960407611168, 30.20724293864768839 ) ) ;
#115380=CARTESIAN_POINT ( 'NONE',  ( -16.51473224551082808, 9.474510206698731452, 53.33442372801900433 ) ) ;
#115381=CARTESIAN_POINT ( 'NONE',  ( 0.05219959533909260263, 19.03943276465977164, 109.9989096053143669 ) ) ;
#115382=CARTESIAN_POINT ( 'NONE',  ( 0.05219959533909260263, 19.03943276465977164, 94.99890960531436690 ) ) ;
#115383=CARTESIAN_POINT ( 'NONE',  ( 0.05219959533910956823, 16.53943276465976808, 49.99890960531437401 ) ) ;
#115384=CARTESIAN_POINT ( 'NONE',  ( -18.67979575497178146, -10.72451020669898902, 41.66557627198103120 ) ) ;
#115385=CARTESIAN_POINT ( 'NONE',  ( 17.72696623605163424, -5.499999999999958256, 91.09811031808420978 ) ) ;
#115386=CARTESIAN_POINT ( 'NONE',  ( 0.05219959533936267826, -19.03943276465977164, 20.00109039468567218 ) ) ;
#115387=CARTESIAN_POINT ( 'NONE',  ( -16.18388926212238133, -7.379444403734535918, 80.43953151366153520 ) ) ;
#115388=CARTESIAN_POINT ( 'NONE',  ( -16.51473224551069308, -9.474510206698971260, 51.66557627198102409 ) ) ;
#115389=CARTESIAN_POINT ( 'NONE',  ( -19.39056639909674473, -5.500000000000012434, 100.7894878107434238 ) ) ;
#115390=CARTESIAN_POINT ( 'NONE',  ( -17.26058549869090797, 6.457015423128533271, 108.6225416252393359 ) ) ;
#115391=CARTESIAN_POINT ( 'NONE',  ( -4.379528057220086978, -16.55341960407618274, 79.79275706135236135 ) ) ;
#115392=CARTESIAN_POINT ( 'NONE',  ( 21.52544592524344225, -5.823673210054117533, 93.54057627198103830 ) ) ;
#115393=CARTESIAN_POINT ( 'NONE',  ( -4.483927247898539470, -16.52544592524342804, 47.29057627198103120 ) ) ;
#115394=CARTESIAN_POINT ( 'NONE',  ( -5.049401038298153566, 19.05341960407611168, 35.20724293864768839 ) ) ;
#115396=CARTESIAN_POINT ( 'NONE',  ( -0.05219959533937732626, 21.53943276465977519, 42.50109039468567573 ) ) ;
#115397=CARTESIAN_POINT ( 'NONE',  ( -5.049401038297874678, -19.05341960407617918, 54.79275706135234003 ) ) ;
#115398=CARTESIAN_POINT ( 'NONE',  ( -19.02544592524342804, 5.153800228976336051, 36.04057627198100988 ) ) ;
#115399=CARTESIAN_POINT ( 'NONE',  ( 18.62759615963255655, 10.81492255796105972, 91.66775706135234714 ) ) ;
#115400=CARTESIAN_POINT ( 'NONE',  ( -19.03943276465977164, 0.05219959533909376836, 21.24890960531436335 ) ) ;
#115401=CARTESIAN_POINT ( 'NONE',  ( 0.05219959533910956823, 16.53943276465976808, 39.99890960531436690 ) ) ;
#115403=CARTESIAN_POINT ( 'NONE',  ( -15.72974639402197994, 15.80617190586746368, 35.62390960531437401 ) ) ;
#115405=CARTESIAN_POINT ( 'NONE',  ( -9.564922557960796823, -16.46253265017161027, 107.0822429386476955 ) ) ;
#115406=CARTESIAN_POINT ( 'NONE',  ( -16.53943276465976808, 0.05219959533911058130, 91.24890960531436690 ) ) ;
#115407=CARTESIAN_POINT ( 'NONE',  ( 12.14591786802327356, -12.06949235617739191, 25.62609039468567929 ) ) ;
#115408=CARTESIAN_POINT ( 'NONE',  ( -14.34966873604972548, 8.224510206698743886, 113.3344237280190328 ) ) ;
#115410=CARTESIAN_POINT ( 'NONE',  ( 19.05341960407611168, 5.049401038298154454, 98.95724293864766707 ) ) ;
#115411=CARTESIAN_POINT ( 'NONE',  ( -10.72451020669898014, 18.67979575497178502, 90.41557627198103830 ) ) ;
#115412=CARTESIAN_POINT ( 'NONE',  ( -8.314922557960811034, -14.29746914071050412, 27.08224293864769550 ) ) ;
#115413=CARTESIAN_POINT ( 'NONE',  ( -19.05341960407611168, -5.049401038298163336, 106.4572429386476955 ) ) ;
#115414=CARTESIAN_POINT ( 'NONE',  ( 13.89961937509957401, 13.97604488694547697, 81.87609039468564731 ) ) ;
#115415=CARTESIAN_POINT ( 'NONE',  ( -0.05219959533937732626, 21.53943276465977519, 112.5010903946857042 ) ) ;
#115416=CARTESIAN_POINT ( 'NONE',  ( 21.55341960407610458, 5.719274019375980345, 93.95724293864770971 ) ) ;
#115417=CARTESIAN_POINT ( 'NONE',  ( -15.72974639402197994, 15.80617190586746368, 40.62390960531435269 ) ) ;
#115418=CARTESIAN_POINT ( 'NONE',  ( 9.564922557960805705, 16.46253265017160317, 64.58224293864769550 ) ) ;
#115419=CARTESIAN_POINT ( 'NONE',  ( 16.52544592524342804, -4.483927247898539470, 33.54057627198102409 ) ) ;
#115420=CARTESIAN_POINT ( 'NONE',  ( -5.153800228976328057, -19.02544592524343514, 77.29057627198099567 ) ) ;
#115421=ORIENTED_EDGE ( 'NONE', *, *, #138961, .T. ) ;
#115423=CARTESIAN_POINT ( 'NONE',  ( 19.03943276465977164, 0.05219959533936151252, 31.25109039468566863 ) ) ;
#115424=CARTESIAN_POINT ( 'NONE',  ( -12.14591786802309592, -12.06949235617757132, 86.87390960531438111 ) ) ;
#115425=CARTESIAN_POINT ( 'NONE',  ( 10.72451020669871369, 18.67979575497193778, 27.08442372801901854 ) ) ;
#115427=CARTESIAN_POINT ( 'NONE',  ( -8.224510206698735004, -14.34966873604973081, 89.58442372801901854 ) ) ;
#115428=CARTESIAN_POINT ( 'NONE',  ( -16.55341960407611168, -4.379528057220339221, 111.4572429386476813 ) ) ;
#115429=CARTESIAN_POINT ( 'NONE',  ( -16.51473224551069308, -9.474510206698971260, 71.66557627198102409 ) ) ;
#115431=CARTESIAN_POINT ( 'NONE',  ( 4.379528057220339221, -16.55341960407611168, 27.70724293864769905 ) ) ;
#115432=CARTESIAN_POINT ( 'NONE',  ( 21.55341960407619695, -5.719274019375665929, 61.04275706135234714 ) ) ;
#115434=CARTESIAN_POINT ( 'NONE',  ( -15.80617190586768217, 15.72974639402176855, 93.12609039468568994 ) ) ;
#115435=CARTESIAN_POINT ( 'NONE',  ( 13.89961937509977652, -13.97604488694527269, 43.12390960531434558 ) ) ;
#115436=CARTESIAN_POINT ( 'NONE',  ( 13.97604488694527802, 13.89961937509977652, 54.37390960531435979 ) ) ;
#115438=CARTESIAN_POINT ( 'NONE',  ( 10.72451020669871369, 18.67979575497193778, 97.08442372801904696 ) ) ;
#115439=CARTESIAN_POINT ( 'NONE',  ( -8.224510206698735004, -14.34966873604973081, 59.58442372801901854 ) ) ;
#115440=CARTESIAN_POINT ( 'NONE',  ( 15.72974639402176855, 15.80617190586768217, 81.87609039468568994 ) ) ;
#115441=CARTESIAN_POINT ( 'NONE',  ( -5.153800228976328057, -19.02544592524343514, 112.2905762719810099 ) ) ;
#115442=CARTESIAN_POINT ( 'NONE',  ( -9.474510206698720793, -16.51473224551083518, 99.58442372801900433 ) ) ;
#115443=CARTESIAN_POINT ( 'NONE',  ( 5.823673210054444382, -21.52544592524334988, 70.20942372801904696 ) ) ;
#115444=CARTESIAN_POINT ( 'NONE',  ( 8.224510206698742110, 14.34966873604972548, 37.08442372801901143 ) ) ;
#115445=CARTESIAN_POINT ( 'NONE',  ( 18.67979575497178502, 10.72451020669898547, 89.16557627198102409 ) ) ;
#115446=CARTESIAN_POINT ( 'NONE',  ( -5.049401038297874678, -19.05341960407617918, 89.79275706135230450 ) ) ;
#115447=CARTESIAN_POINT ( 'NONE',  ( 13.97604488694527802, 13.89961937509977652, 59.37390960531434558 ) ) ;
#115448=CARTESIAN_POINT ( 'NONE',  ( 19.02544592524334988, 5.153800228976608722, 96.45942372801897591 ) ) ;
#115450=CARTESIAN_POINT ( 'NONE',  ( -16.51473224551082808, 9.474510206698731452, 108.3344237280190043 ) ) ;
#115451=CARTESIAN_POINT ( 'NONE',  ( 16.52544592524342804, -4.483927247898539470, 58.54057627198103120 ) ) ;
#115452=CARTESIAN_POINT ( 'NONE',  ( -5.153800228976607833, 19.02544592524334988, 77.70942372801900433 ) ) ;
#115453=CARTESIAN_POINT ( 'NONE',  ( 14.29746914071037800, 8.314922557961029526, 61.66775706135235424 ) ) ;
#115454=CARTESIAN_POINT ( 'NONE',  ( 16.46253265017160672, -9.564922557960803928, 43.33224293864769550 ) ) ;
#115455=CARTESIAN_POINT ( 'NONE',  ( -16.46253265017160317, 9.564922557960807481, 60.83224293864769550 ) ) ;
#115456=CARTESIAN_POINT ( 'NONE',  ( 14.29746914071037800, 8.314922557961029526, 61.66775706135235424 ) ) ;
#115457=CARTESIAN_POINT ( 'NONE',  ( -18.22780087662119541, 5.500000000000102141, 46.01763182126894947 ) ) ;
#115460=CARTESIAN_POINT ( 'NONE',  ( -16.51473224551069308, -9.474510206698971260, 111.6655762719810383 ) ) ;
#115463=CARTESIAN_POINT ( 'NONE',  ( -16.51473224551082808, 9.474510206698731452, 113.3344237280190043 ) ) ;
#115464=CARTESIAN_POINT ( 'NONE',  ( -0.05219959533907301413, -21.53943276465977519, 32.49890960531435979 ) ) ;
#115465=CARTESIAN_POINT ( 'NONE',  ( 0.05219959533936267826, -19.03943276465977164, 30.00109039468566863 ) ) ;
#115466=CARTESIAN_POINT ( 'NONE',  ( 9.564922557961047289, -16.46253265017146816, 105.4177570613523471 ) ) ;
#115467=CARTESIAN_POINT ( 'NONE',  ( 5.049401038298161559, -19.05341960407611168, 27.70724293864769550 ) ) ;
#115468=CARTESIAN_POINT ( 'NONE',  ( -19.03943276465977164, 0.05219959533909376836, 51.24890960531436690 ) ) ;
#115469=CARTESIAN_POINT ( 'NONE',  ( 10.81492255796078972, 18.62759615963270932, 74.58224293864768129 ) ) ;
#115470=CARTESIAN_POINT ( 'NONE',  ( -19.02544592524342804, 5.153800228976336051, 96.04057627198103830 ) ) ;
#115471=CARTESIAN_POINT ( 'NONE',  ( -9.564922557960796823, -16.46253265017161027, 37.08224293864768839 ) ) ;
#115473=CARTESIAN_POINT ( 'NONE',  ( 5.153800228976615827, -19.02544592524334988, 85.20942372801900433 ) ) ;
#115474=CARTESIAN_POINT ( 'NONE',  ( 8.224510206698953496, -14.34966873604960469, 72.91557627198103830 ) ) ;
#115476=CARTESIAN_POINT ( 'NONE',  ( 15.80617190586746368, 15.72974639402197994, 49.37390960531436690 ) ) ;
#115477=CARTESIAN_POINT ( 'NONE',  ( 21.53943276465977519, 0.05219959533937863772, 111.2510903946856899 ) ) ;
#115478=CARTESIAN_POINT ( 'NONE',  ( 0.05219959533907565091, 21.53943276465977519, 94.99890960531436690 ) ) ;
#115479=CARTESIAN_POINT ( 'NONE',  ( -21.55341960407619339, 5.719274019375674811, 78.54275706135236135 ) ) ;
#115480=CARTESIAN_POINT ( 'NONE',  ( 21.53943276465977519, 0.05219959533937863772, 81.25109039468568994 ) ) ;
#115481=CARTESIAN_POINT ( 'NONE',  ( -19.02544592524342804, 5.153800228976336051, 106.0405762719810241 ) ) ;
#115482=CARTESIAN_POINT ( 'NONE',  ( 8.314922557961029526, -14.29746914071037800, 105.4177570613523613 ) ) ;
#115483=CARTESIAN_POINT ( 'NONE',  ( -15.80617190586768217, 15.72974639402176855, 83.12609039468568994 ) ) ;
#115484=CARTESIAN_POINT ( 'NONE',  ( 16.46253265017160672, -9.564922557960803928, 68.33224293864770971 ) ) ;
#115485=CARTESIAN_POINT ( 'NONE',  ( 19.03943276465977164, 0.05219959533936151252, 31.25109039468566863 ) ) ;
#115486=CARTESIAN_POINT ( 'NONE',  ( -21.55341960407619339, 5.719274019375674811, 28.54275706135234358 ) ) ;
#115487=CARTESIAN_POINT ( 'NONE',  ( -13.89961937509977652, 13.97604488694528158, 70.62390960531432427 ) ) ;
#115488=CARTESIAN_POINT ( 'NONE',  ( 8.224510206698953496, -14.34966873604960469, 82.91557627198103830 ) ) ;
#115489=CARTESIAN_POINT ( 'NONE',  ( 12.06949235617757843, -12.14591786802309237, 48.12390960531436690 ) ) ;
#115490=CARTESIAN_POINT ( 'NONE',  ( -18.62759615963270932, 10.81492255796079327, 60.83224293864769550 ) ) ;
#115491=CARTESIAN_POINT ( 'NONE',  ( 9.564922557960805705, 16.46253265017160317, 59.58224293864769550 ) ) ;
#115492=CARTESIAN_POINT ( 'NONE',  ( -5.823673210054116645, -21.52544592524344225, 77.29057627198102409 ) ) ;
#115493=CARTESIAN_POINT ( 'NONE',  ( -5.049401038297874678, -19.05341960407617918, 59.79275706135231871 ) ) ;
#115494=CARTESIAN_POINT ( 'NONE',  ( 19.05341960407618274, -5.049401038297876454, 26.04275706135233648 ) ) ;
#115495=CARTESIAN_POINT ( 'NONE',  ( -0.05219959533910754901, -16.53943276465976808, 67.49890960531436690 ) ) ;
#115497=CARTESIAN_POINT ( 'NONE',  ( -18.67979575497178146, -10.72451020669898902, 36.66557627198103120 ) ) ;
#115500=CARTESIAN_POINT ( 'NONE',  ( 16.52544592524335698, 4.483927247898782831, 91.45942372801901854 ) ) ;
#115502=CARTESIAN_POINT ( 'NONE',  ( -9.474510206698720793, -16.51473224551083518, 84.58442372801900433 ) ) ;
#115503=CARTESIAN_POINT ( 'NONE',  ( 12.06949235617757843, -12.14591786802309237, 68.12390960531436690 ) ) ;
#115505=CARTESIAN_POINT ( 'NONE',  ( -16.51473224551069308, -9.474510206698971260, 56.66557627198103120 ) ) ;
#115506=CARTESIAN_POINT ( 'NONE',  ( 16.55341960407611168, 4.379528057220329451, 43.95724293864769550 ) ) ;
#115507=CARTESIAN_POINT ( 'NONE',  ( -13.97604488694527625, -13.89961937509977652, 81.87390960531436690 ) ) ;
#115508=CARTESIAN_POINT ( 'NONE',  ( -0.05219959533936034679, 19.03943276465977164, 72.50109039468566152 ) ) ;
#115509=CARTESIAN_POINT ( 'NONE',  ( 16.51473224551069308, 9.474510206698969483, 49.16557627198102409 ) ) ;
#115510=CARTESIAN_POINT ( 'NONE',  ( 18.67979575497194134, -10.72451020669871369, 65.83442372801900433 ) ) ;
#115511=CARTESIAN_POINT ( 'NONE',  ( 9.474510206698971260, -16.51473224551069308, 87.91557627198102409 ) ) ;
#115512=CARTESIAN_POINT ( 'NONE',  ( -5.153800228976328057, -19.02544592524343514, 27.29057627198103120 ) ) ;
#115513=CARTESIAN_POINT ( 'NONE',  ( -16.46253265017160317, 9.564922557960807481, 75.83224293864769550 ) ) ;
#115514=CARTESIAN_POINT ( 'NONE',  ( -0.05219959533907301413, -21.53943276465977519, 47.49890960531435979 ) ) ;
#115515=CARTESIAN_POINT ( 'NONE',  ( 16.51473224551069308, 9.474510206698969483, 44.16557627198103120 ) ) ;
#115516=CARTESIAN_POINT ( 'NONE',  ( 0.05219959533907565091, 21.53943276465977519, 49.99890960531437401 ) ) ;
#115517=CARTESIAN_POINT ( 'NONE',  ( 19.05341960407617918, -5.049401038297876454, 86.04275706135233293 ) ) ;
#115518=CARTESIAN_POINT ( 'NONE',  ( 12.14591786802327356, -12.06949235617739191, 100.6260903946857184 ) ) ;
#115519=CARTESIAN_POINT ( 'NONE',  ( 0.05219959533936267826, -19.03943276465977164, 35.00109039468566863 ) ) ;
#115520=CARTESIAN_POINT ( 'NONE',  ( 12.14591786802327356, -12.06949235617739191, 65.62609039468568994 ) ) ;
#115521=CARTESIAN_POINT ( 'NONE',  ( -16.55341960407617563, 4.379528057220093196, 93.54275706135234714 ) ) ;
#115522=CARTESIAN_POINT ( 'NONE',  ( 18.22780087662122384, 5.500000000000018652, 98.98459894673892734 ) ) ;
#115523=CARTESIAN_POINT ( 'NONE',  ( 14.34966873604972726, -8.224510206698740333, 80.83442372801901854 ) ) ;
#115524=CARTESIAN_POINT ( 'NONE',  ( 5.719274019375991003, -21.55341960407610458, 32.70724293864770260 ) ) ;
#115525=CARTESIAN_POINT ( 'NONE',  ( -19.05341960407611168, -5.049401038298163336, 36.45724293864766707 ) ) ;
#115526=CARTESIAN_POINT ( 'NONE',  ( 4.379528057220092307, 16.55341960407617563, 32.29275706135235424 ) ) ;
#115527=CARTESIAN_POINT ( 'NONE',  ( -16.51473224551069308, -9.474510206698971260, 51.66557627198102409 ) ) ;
#115528=CARTESIAN_POINT ( 'NONE',  ( 5.823673210054444382, -21.52544592524334988, 45.20942372801901854 ) ) ;
#115529=CARTESIAN_POINT ( 'NONE',  ( -16.53943276465976808, -0.05219959533934237506, 38.75109039468567573 ) ) ;
#115530=CARTESIAN_POINT ( 'NONE',  ( -16.55341960407611168, -4.379528057220339221, 26.45724293864768839 ) ) ;
#115531=CARTESIAN_POINT ( 'NONE',  ( -19.03943276465977164, 0.05219959533909376836, 26.24890960531435624 ) ) ;
#115532=CARTESIAN_POINT ( 'NONE',  ( -16.46253265017146816, -9.564922557961047289, 19.16775706135233293 ) ) ;
#115533=CARTESIAN_POINT ( 'NONE',  ( -19.05341960407617563, 5.049401038297882671, 113.5427570613523471 ) ) ;
#115534=CARTESIAN_POINT ( 'NONE',  ( -0.05219959533936034679, 19.03943276465977164, 67.50109039468566152 ) ) ;
#115535=CARTESIAN_POINT ( 'NONE',  ( -16.53943276465976808, 0.05219959533911058130, 71.24890960531435269 ) ) ;
#115536=CARTESIAN_POINT ( 'NONE',  ( 9.474510206698971260, -16.51473224551069308, 37.91557627198102409 ) ) ;
#115537=CARTESIAN_POINT ( 'NONE',  ( 13.97604488694548053, -13.89961937509957401, 70.62609039468567573 ) ) ;
#115538=CARTESIAN_POINT ( 'NONE',  ( 17.26172910966779028, -6.454744622555846689, 93.30646908649222837 ) ) ;
#115539=CARTESIAN_POINT ( 'NONE',  ( 10.81492255796106328, -18.62759615963255655, 60.41775706135235424 ) ) ;
#115540=CARTESIAN_POINT ( 'NONE',  ( 0.05219959533934541429, -16.53943276465976808, 45.00109039468568284 ) ) ;
#115541=CARTESIAN_POINT ( 'NONE',  ( 18.56197773271730256, -5.499999999999888090, 56.05066217314453070 ) ) ;
#115542=CARTESIAN_POINT ( 'NONE',  ( -21.52544592524343514, 5.823673210054127303, 41.04057627198103120 ) ) ;
#115543=CARTESIAN_POINT ( 'NONE',  ( 4.379528057220092307, 16.55341960407617563, 22.29275706135235069 ) ) ;
#115544=CARTESIAN_POINT ( 'NONE',  ( 16.51473224551069308, 9.474510206698969483, 114.1655762719810241 ) ) ;
#115546=CARTESIAN_POINT ( 'NONE',  ( -16.51473224551069308, -9.474510206698971260, 41.66557627198103120 ) ) ;
#115547=CARTESIAN_POINT ( 'NONE',  ( 5.719274019375673035, 21.55341960407619339, 112.2927570613523471 ) ) ;
#115548=CARTESIAN_POINT ( 'NONE',  ( -5.153800228976328057, -19.02544592524343514, 62.29057627198100988 ) ) ;
#115549=CARTESIAN_POINT ( 'NONE',  ( -18.62759615963255300, -10.81492255796106328, 59.16775706135234714 ) ) ;
#115550=CARTESIAN_POINT ( 'NONE',  ( 5.823673210054444382, -21.52544592524334988, 100.2094237280190043 ) ) ;
#115551=CARTESIAN_POINT ( 'NONE',  ( 12.06949235617757843, -12.14591786802309237, 28.12390960531435979 ) ) ;
#115552=CARTESIAN_POINT ( 'NONE',  ( -0.05219959533909027116, -19.03943276465977164, 27.49890960531435624 ) ) ;
#115554=CARTESIAN_POINT ( 'NONE',  ( -19.03943276465977164, 0.05219959533909376836, 86.24890960531436690 ) ) ;
#115555=CARTESIAN_POINT ( 'NONE',  ( 21.53943276465977519, 0.05219959533937863772, 51.25109039468568994 ) ) ;
#115556=CARTESIAN_POINT ( 'NONE',  ( -5.153800228976328057, -19.02544592524343514, 37.29057627198102409 ) ) ;
#115557=CARTESIAN_POINT ( 'NONE',  ( -21.55341960407619339, 5.719274019375674811, 58.54275706135235424 ) ) ;
#115558=CARTESIAN_POINT ( 'NONE',  ( 19.05341960407617918, -5.049401038297876454, 91.04275706135234714 ) ) ;
#115559=CARTESIAN_POINT ( 'NONE',  ( -16.46253265017160317, 9.564922557960807481, 100.8322429386477097 ) ) ;
#115560=CARTESIAN_POINT ( 'NONE',  ( 16.46253265017160672, -9.564922557960803928, 28.33224293864769550 ) ) ;
#115561=CARTESIAN_POINT ( 'NONE',  ( -15.72974639402197994, 15.80617190586746368, 115.6239096053143669 ) ) ;
#115562=CARTESIAN_POINT ( 'NONE',  ( 0.05219959533936267826, -19.03943276465977164, 30.00109039468566863 ) ) ;
#115563=CARTESIAN_POINT ( 'NONE',  ( 0.05219959533910956823, 16.53943276465976808, 104.9989096053143669 ) ) ;
#115564=CARTESIAN_POINT ( 'NONE',  ( 16.51473224551069308, 9.474510206698969483, 44.16557627198103120 ) ) ;
#115565=CARTESIAN_POINT ( 'NONE',  ( -9.564922557961040184, 16.46253265017147172, 92.91775706135233293 ) ) ;
#115566=CARTESIAN_POINT ( 'NONE',  ( 12.06949235617757843, -12.14591786802309237, 63.12390960531435979 ) ) ;
#115567=CARTESIAN_POINT ( 'NONE',  ( -10.72451020669870658, -18.67979575497194134, 109.5844237280190328 ) ) ;
#115568=CARTESIAN_POINT ( 'NONE',  ( -10.72451020669898014, 18.67979575497178502, 25.41557627198103120 ) ) ;
#115569=CARTESIAN_POINT ( 'NONE',  ( -16.46253265017146816, -9.564922557961047289, 89.16775706135234714 ) ) ;
#115570=CARTESIAN_POINT ( 'NONE',  ( 10.81492255796078972, 18.62759615963270932, 94.58224293864769550 ) ) ;
#115571=CARTESIAN_POINT ( 'NONE',  ( -0.05219959533937732626, 21.53943276465977519, 37.50109039468568284 ) ) ;
#115572=CARTESIAN_POINT ( 'NONE',  ( -16.52544592524335698, -4.483927247898792601, 43.95942372801902565 ) ) ;
#115573=CARTESIAN_POINT ( 'NONE',  ( 16.52544592524335698, 4.483927247898782831, 106.4594237280190328 ) ) ;
#115574=CARTESIAN_POINT ( 'NONE',  ( 16.55341960407618274, -4.379528057220086978, 46.04275706135234714 ) ) ;
#115575=CARTESIAN_POINT ( 'NONE',  ( -5.823673210054431948, 21.52544592524334988, 52.70942372801902565 ) ) ;
#115576=CARTESIAN_POINT ( 'NONE',  ( 5.823673210054125526, 21.52544592524343514, 49.79057627198102409 ) ) ;
#115577=CARTESIAN_POINT ( 'NONE',  ( -19.03943276465977164, 0.05219959533909376836, 36.24890960531436690 ) ) ;
#115579=CARTESIAN_POINT ( 'NONE',  ( -16.53943276465976808, -0.05219959533934237506, 63.75109039468568284 ) ) ;
#115580=CARTESIAN_POINT ( 'NONE',  ( -5.823673210054116645, -21.52544592524344225, 87.29057627198103830 ) ) ;
#115581=CARTESIAN_POINT ( 'NONE',  ( 14.34966873604960469, 8.224510206698951720, 44.16557627198103120 ) ) ;
#115582=CARTESIAN_POINT ( 'NONE',  ( -0.05219959533934338120, 16.53943276465976808, 57.50109039468568994 ) ) ;
#115583=CARTESIAN_POINT ( 'NONE',  ( -0.05219959533936034679, 19.03943276465977164, 97.50109039468567573 ) ) ;
#115584=CARTESIAN_POINT ( 'NONE',  ( 21.52544592524344225, -5.823673210054117533, 103.5405762719810383 ) ) ;
#115585=CARTESIAN_POINT ( 'NONE',  ( -8.314922557960811034, -14.29746914071050412, 37.08224293864768129 ) ) ;
#115587=CARTESIAN_POINT ( 'NONE',  ( 4.379528057220092307, 16.55341960407617563, 72.29275706135236135 ) ) ;
#115589=CARTESIAN_POINT ( 'NONE',  ( 5.719274019375991003, -21.55341960407610458, 72.70724293864769550 ) ) ;
#115590=CARTESIAN_POINT ( 'NONE',  ( -8.314922557961024197, 14.29746914071037800, 107.9177570613523471 ) ) ;
#115593=CARTESIAN_POINT ( 'NONE',  ( -5.719274019375978568, 21.55341960407610458, 85.20724293864770971 ) ) ;
#115594=CARTESIAN_POINT ( 'NONE',  ( 18.62759615963271287, -10.81492255796078972, 113.3322429386476955 ) ) ;
#115595=CARTESIAN_POINT ( 'NONE',  ( 14.34966873604960469, 8.224510206698951720, 39.16557627198102409 ) ) ;
#115596=CARTESIAN_POINT ( 'NONE',  ( 8.224510206698742110, 14.34966873604972548, 37.08442372801901143 ) ) ;
#115598=CARTESIAN_POINT ( 'NONE',  ( 19.03943276465977164, -0.05219959533909143690, 48.74890960531435979 ) ) ;
#115599=CARTESIAN_POINT ( 'NONE',  ( 19.02544592524343514, -5.153800228976328945, 73.54057627198103830 ) ) ;
#115600=CARTESIAN_POINT ( 'NONE',  ( 16.46253265017160672, -9.564922557960803928, 113.3322429386476955 ) ) ;
#115601=CARTESIAN_POINT ( 'NONE',  ( -16.46253265017160317, 9.564922557960807481, 115.8322429386477097 ) ) ;
#115602=CARTESIAN_POINT ( 'NONE',  ( -19.05341960407617563, 5.049401038297882671, 108.5427570613523187 ) ) ;
#115603=CARTESIAN_POINT ( 'NONE',  ( 19.03943276465977164, 0.05219959533936151252, 46.25109039468566863 ) ) ;
#115604=CARTESIAN_POINT ( 'NONE',  ( -21.52544592524343514, 5.823673210054127303, 91.04057627198103830 ) ) ;
#115605=CARTESIAN_POINT ( 'NONE',  ( 8.314922557960818139, 14.29746914071049879, 24.58224293864768839 ) ) ;
#115606=CARTESIAN_POINT ( 'NONE',  ( -5.823673210054116645, -21.52544592524344225, 42.29057627198103120 ) ) ;
#115607=CARTESIAN_POINT ( 'NONE',  ( -21.55341960407610458, -5.719274019375992779, 81.45724293864769550 ) ) ;
#115608=CARTESIAN_POINT ( 'NONE',  ( -0.05219959533936034679, 19.03943276465977164, 107.5010903946856615 ) ) ;
#115609=CARTESIAN_POINT ( 'NONE',  ( 5.153800228976335163, 19.02544592524342804, 99.79057627198102409 ) ) ;
#115610=CARTESIAN_POINT ( 'NONE',  ( -21.53943276465977519, -0.05219959533937600094, 73.75109039468567573 ) ) ;
#115611=CARTESIAN_POINT ( 'NONE',  ( -13.97604488694527625, -13.89961937509977652, 76.87390960531433848 ) ) ;
#115612=CARTESIAN_POINT ( 'NONE',  ( -16.53943276465976808, 0.05219959533911058130, 101.2489096053143669 ) ) ;
#115614=CARTESIAN_POINT ( 'NONE',  ( 19.02544592524343514, -5.153800228976328945, 73.54057627198103830 ) ) ;
#115615=CARTESIAN_POINT ( 'NONE',  ( -8.314922557960811034, -14.29746914071050412, 92.08224293864769550 ) ) ;
#115616=VERTEX_POINT ( 'NONE', #67979 ) ;
#115617=CARTESIAN_POINT ( 'NONE',  ( -16.46253265017146816, -9.564922557961047289, 109.1677570613523471 ) ) ;
#115619=CARTESIAN_POINT ( 'NONE',  ( -13.89961937509977652, 13.97604488694528158, 55.62390960531434558 ) ) ;
#115621=CARTESIAN_POINT ( 'NONE',  ( -21.55341960407619339, 5.719274019375674811, 83.54275706135234714 ) ) ;
#115622=CARTESIAN_POINT ( 'NONE',  ( 16.46253265017160672, -9.564922557960803928, 103.3322429386476955 ) ) ;
#115623=CARTESIAN_POINT ( 'NONE',  ( -0.05219959533934338120, 16.53943276465976808, 72.50109039468568994 ) ) ;
#115625=CARTESIAN_POINT ( 'NONE',  ( -5.049401038297874678, -19.05341960407617918, 59.79275706135231871 ) ) ;
#115626=CARTESIAN_POINT ( 'NONE',  ( -18.62759615963255300, -10.81492255796106328, 94.16775706135237556 ) ) ;
#115629=CARTESIAN_POINT ( 'NONE',  ( 16.55341960407611168, 4.379528057220329451, 28.95724293864769905 ) ) ;
#115630=CARTESIAN_POINT ( 'NONE',  ( -17.58332526062526213, -7.635886036038624702, 74.07665040441536064 ) ) ;
#115631=CARTESIAN_POINT ( 'NONE',  ( -4.379528057220086978, -16.55341960407618274, 89.79275706135236135 ) ) ;
#115633=CARTESIAN_POINT ( 'NONE',  ( 12.06949235617739724, 12.14591786802326823, 71.87609039468568994 ) ) ;
#115634=CARTESIAN_POINT ( 'NONE',  ( -5.719274019375665041, -21.55341960407619695, 84.79275706135234714 ) ) ;
#115635=CARTESIAN_POINT ( 'NONE',  ( 16.51473224551083163, -9.474510206698727899, 85.83442372801900433 ) ) ;
#115636=CARTESIAN_POINT ( 'NONE',  ( -9.564922557961040184, 16.46253265017147172, 42.91775706135234003 ) ) ;
#115637=CARTESIAN_POINT ( 'NONE',  ( -19.03943276465977164, 0.05219959533909376836, 71.24890960531435269 ) ) ;
#115638=CARTESIAN_POINT ( 'NONE',  ( 19.02544592524343514, -5.153800228976328945, 63.54057627198103830 ) ) ;
#115640=CARTESIAN_POINT ( 'NONE',  ( -15.72974639402197994, 15.80617190586746368, 85.62390960531436690 ) ) ;
#115641=CARTESIAN_POINT ( 'NONE',  ( 21.55341960407610458, 5.719274019375980345, 53.95724293864770260 ) ) ;
#115642=CARTESIAN_POINT ( 'NONE',  ( 9.564922557960805705, 16.46253265017160317, 39.58224293864768839 ) ) ;
#115643=CARTESIAN_POINT ( 'NONE',  ( 8.224510206698742110, 14.34966873604972548, 67.08442372801901854 ) ) ;
#115645=CARTESIAN_POINT ( 'NONE',  ( 15.72974639402176855, 15.80617190586768217, 46.87609039468568994 ) ) ;
#115646=CARTESIAN_POINT ( 'NONE',  ( 12.14591786802309770, 12.06949235617756955, 59.37390960531436690 ) ) ;
#115648=CARTESIAN_POINT ( 'NONE',  ( -16.53943276465976808, -0.05219959533934237506, 33.75109039468568284 ) ) ;
#115649=CARTESIAN_POINT ( 'NONE',  ( -0.05219959533936034679, 19.03943276465977164, 47.50109039468566863 ) ) ;
#115650=CARTESIAN_POINT ( 'NONE',  ( -8.314922557960811034, -14.29746914071050412, 62.08224293864769550 ) ) ;
#115651=CARTESIAN_POINT ( 'NONE',  ( -15.72974639402176322, -15.80617190586768395, 29.37609039468568284 ) ) ;
#115652=EDGE_CURVE ( 'NONE', #30365, #99459, #138762, .T. ) ;
#115653=FACE_OUTER_BOUND ( 'NONE', #51528, .T. ) ;
#115654=CARTESIAN_POINT ( 'NONE',  ( 15.80617190586746368, 15.72974639402197994, 84.37390960531438111 ) ) ;
#115655=CARTESIAN_POINT ( 'NONE',  ( -19.02544592524342804, 5.153800228976336051, 106.0405762719810241 ) ) ;
#115656=CARTESIAN_POINT ( 'NONE',  ( 4.379528057220339221, -16.55341960407611168, 77.70724293864770971 ) ) ;
#115657=CARTESIAN_POINT ( 'NONE',  ( -19.02544592524342804, 5.153800228976336051, 111.0405762719810099 ) ) ;
#115659=CARTESIAN_POINT ( 'NONE',  ( -19.02544592524334988, -5.153800228976617603, 73.95942372801900433 ) ) ;
#115660=CARTESIAN_POINT ( 'NONE',  ( 0.05219959533907565091, 21.53943276465977519, 114.9989096053143669 ) ) ;
#115661=CARTESIAN_POINT ( 'NONE',  ( 0.05219959533909260263, 19.03943276465977164, 59.99890960531436690 ) ) ;
#115662=CARTESIAN_POINT ( 'NONE',  ( -5.153800228976607833, 19.02544592524334988, 42.70942372801901143 ) ) ;
#115663=CARTESIAN_POINT ( 'NONE',  ( -19.02544592524342804, 5.153800228976336051, 31.04057627198102409 ) ) ;
#115664=CARTESIAN_POINT ( 'NONE',  ( 10.72451020669871369, 18.67979575497193778, 67.08442372801901854 ) ) ;
#115665=CARTESIAN_POINT ( 'NONE',  ( -16.62475595723696742, -7.163666690055377373, 69.47286648189532343 ) ) ;
#115667=CARTESIAN_POINT ( 'NONE',  ( -16.53943276465976808, 0.05219959533911058130, 51.24890960531436690 ) ) ;
#115668=CARTESIAN_POINT ( 'NONE',  ( -13.97604488694527625, -13.89961937509977652, 66.87390960531436690 ) ) ;
#115669=CARTESIAN_POINT ( 'NONE',  ( 5.823673210054125526, 21.52544592524343514, 89.79057627198103830 ) ) ;
#115670=CARTESIAN_POINT ( 'NONE',  ( -13.97604488694527625, -13.89961937509977652, 51.87390960531436690 ) ) ;
#115672=CARTESIAN_POINT ( 'NONE',  ( -10.81492255796078084, -18.62759615963271287, 82.08224293864768129 ) ) ;
#115673=CARTESIAN_POINT ( 'NONE',  ( -18.62759615963255300, -10.81492255796106328, 104.1677570613523471 ) ) ;
#115674=CARTESIAN_POINT ( 'NONE',  ( 9.564922557960805705, 16.46253265017160317, 24.58224293864769194 ) ) ;
#115675=CARTESIAN_POINT ( 'NONE',  ( -4.483927247898782831, 16.52544592524335698, 102.7094237280190185 ) ) ;
#115676=CARTESIAN_POINT ( 'NONE',  ( 0.05219959533910956823, 16.53943276465976808, 79.99890960531435269 ) ) ;
#115677=CARTESIAN_POINT ( 'NONE',  ( -13.97604488694547697, 13.89961937509957934, 93.12609039468566152 ) ) ;
#115679=CARTESIAN_POINT ( 'NONE',  ( -10.72451020669898014, 18.67979575497178502, 115.4155762719810241 ) ) ;
#115680=CARTESIAN_POINT ( 'NONE',  ( -16.46253265017146816, -9.564922557961047289, 39.16775706135234003 ) ) ;
#115681=CARTESIAN_POINT ( 'NONE',  ( -16.55341960407617563, 4.379528057220093196, 103.5427570613523613 ) ) ;
#115682=CARTESIAN_POINT ( 'NONE',  ( -19.03943276465977164, -0.05219959533935918106, 33.75109039468566863 ) ) ;
#115683=CARTESIAN_POINT ( 'NONE',  ( -9.474510206698964154, 16.51473224551069663, 90.41557627198103830 ) ) ;
#115684=CARTESIAN_POINT ( 'NONE',  ( -5.823673210054116645, -21.52544592524344225, 57.29057627198103120 ) ) ;
#115685=CARTESIAN_POINT ( 'NONE',  ( -19.35633801406903487, 5.499999999999766409, 49.13373818172757979 ) ) ;
#115686=CARTESIAN_POINT ( 'NONE',  ( -14.29746914071049879, 8.314922557960819915, 115.8322429386477097 ) ) ;
#115687=CARTESIAN_POINT ( 'NONE',  ( 21.55341960407619695, -5.719274019375665929, 106.0427570613523471 ) ) ;
#115688=CARTESIAN_POINT ( 'NONE',  ( 8.314922557961029526, -14.29746914071037800, 75.41775706135233293 ) ) ;
#115689=CARTESIAN_POINT ( 'NONE',  ( 10.72451020669871369, 18.67979575497193778, 22.08442372801901143 ) ) ;
#115690=CARTESIAN_POINT ( 'NONE',  ( -12.14591786802326823, 12.06949235617739902, 33.12609039468569705 ) ) ;
#115691=CARTESIAN_POINT ( 'NONE',  ( 5.153800228976335163, 19.02544592524342804, 109.7905762719810099 ) ) ;
#115692=CARTESIAN_POINT ( 'NONE',  ( 19.05341960407611168, 5.049401038298154454, 38.95724293864767418 ) ) ;
#115693=CARTESIAN_POINT ( 'NONE',  ( 13.97604488694527802, 13.89961937509977652, 69.37390960531436690 ) ) ;
#115694=CARTESIAN_POINT ( 'NONE',  ( -8.314922557961024197, 14.29746914071037800, 42.91775706135235424 ) ) ;
#115695=CARTESIAN_POINT ( 'NONE',  ( -14.34966873604960291, -8.224510206698953496, 86.66557627198102409 ) ) ;
#115696=CARTESIAN_POINT ( 'NONE',  ( -12.06949235617739369, -12.14591786802326823, 104.3760903946856899 ) ) ;
#115697=CARTESIAN_POINT ( 'NONE',  ( 5.719274019375673035, 21.55341960407619339, 57.29275706135234714 ) ) ;
#115698=CARTESIAN_POINT ( 'NONE',  ( 9.474510206698971260, -16.51473224551069308, 82.91557627198103830 ) ) ;
#115699=CARTESIAN_POINT ( 'NONE',  ( 13.97604488694527802, 13.89961937509977652, 59.37390960531434558 ) ) ;
#115700=CARTESIAN_POINT ( 'NONE',  ( -13.97604488694527625, -13.89961937509977652, 101.8739096053143811 ) ) ;
#115701=CARTESIAN_POINT ( 'NONE',  ( 0.05219959533910956823, 16.53943276465976808, 39.99890960531436690 ) ) ;
#115702=CARTESIAN_POINT ( 'NONE',  ( -12.14591786802326823, 12.06949235617739902, 103.1260903946856757 ) ) ;
#115705=CARTESIAN_POINT ( 'NONE',  ( -13.97604488694547697, 13.89961937509957934, 43.12609039468566152 ) ) ;
#115706=CARTESIAN_POINT ( 'NONE',  ( 13.89961937509977652, -13.97604488694527269, 113.1239096053143527 ) ) ;
#115707=CARTESIAN_POINT ( 'NONE',  ( 19.03943276465977164, -0.05219959533909143690, 63.74890960531435979 ) ) ;
#115708=CARTESIAN_POINT ( 'NONE',  ( -16.46253265017146816, -9.564922557961047289, 44.16775706135232582 ) ) ;
#115710=CARTESIAN_POINT ( 'NONE',  ( -17.12812012977023812, -6.668231424566064547, 66.35948759323143520 ) ) ;
#115711=CARTESIAN_POINT ( 'NONE',  ( -14.34966873604972548, 8.224510206698743886, 53.33442372801901854 ) ) ;
#115712=CARTESIAN_POINT ( 'NONE',  ( 19.02544592524334988, 5.153800228976608722, 66.45942372801899012 ) ) ;
#115713=CARTESIAN_POINT ( 'NONE',  ( 8.224510206698742110, 14.34966873604972548, 67.08442372801901854 ) ) ;
#115714=CARTESIAN_POINT ( 'NONE',  ( 17.48853670773245383, 5.747243402303094051, 93.83328700250011423 ) ) ;
#115715=CARTESIAN_POINT ( 'NONE',  ( -9.564922557960796823, -16.46253265017161027, 97.08224293864769550 ) ) ;
#115716=CARTESIAN_POINT ( 'NONE',  ( 10.72451020669898902, -18.67979575497178502, 107.9155762719810241 ) ) ;
#115717=CARTESIAN_POINT ( 'NONE',  ( -16.51473224551082808, 9.474510206698731452, 78.33442372801900433 ) ) ;
#115718=CARTESIAN_POINT ( 'NONE',  ( 13.97604488694527802, 13.89961937509977652, 104.3739096053143385 ) ) ;
#115719=CARTESIAN_POINT ( 'NONE',  ( -5.049401038298153566, 19.05341960407611168, 35.20724293864768839 ) ) ;
#115720=CARTESIAN_POINT ( 'NONE',  ( -13.97604488694527625, -13.89961937509977652, 91.87390960531432427 ) ) ;
#115721=CARTESIAN_POINT ( 'NONE',  ( 14.34966873604960469, 8.224510206698951720, 54.16557627198103120 ) ) ;
#115722=CARTESIAN_POINT ( 'NONE',  ( 13.97604488694527802, 13.89961937509977652, 34.37390960531436690 ) ) ;
#115723=CARTESIAN_POINT ( 'NONE',  ( 5.153800228976615827, -19.02544592524334988, 45.20942372801901143 ) ) ;
#115724=ORIENTED_EDGE ( 'NONE', *, *, #186744, .F. ) ;
#115725=CARTESIAN_POINT ( 'NONE',  ( -0.05219959533910754901, -16.53943276465976808, 92.49890960531436690 ) ) ;
#115726=CARTESIAN_POINT ( 'NONE',  ( -0.05219959533937732626, 21.53943276465977519, 112.5010903946857042 ) ) ;
#115727=CARTESIAN_POINT ( 'NONE',  ( -5.153800228976328057, -19.02544592524343514, 52.29057627198100988 ) ) ;
#115728=CARTESIAN_POINT ( 'NONE',  ( 18.62759615963271287, -10.81492255796078972, 68.33224293864769550 ) ) ;
#115729=CARTESIAN_POINT ( 'NONE',  ( 16.53943276465976808, -0.05219959533910856209, 48.74890960531435979 ) ) ;
#115730=CARTESIAN_POINT ( 'NONE',  ( -21.55341960407619339, 5.719274019375674811, 113.5427570613523756 ) ) ;
#115731=CARTESIAN_POINT ( 'NONE',  ( -19.02544592524342804, 5.153800228976336051, 101.0405762719810241 ) ) ;
#115732=CARTESIAN_POINT ( 'NONE',  ( 16.46253265017160672, -9.564922557960803928, 108.3322429386476955 ) ) ;
#115733=CARTESIAN_POINT ( 'NONE',  ( 13.89961937509977652, -13.97604488694527269, 58.12390960531436690 ) ) ;
#115734=CARTESIAN_POINT ( 'NONE',  ( -9.564922557960796823, -16.46253265017161027, 22.08224293864768839 ) ) ;
#115735=CARTESIAN_POINT ( 'NONE',  ( 4.483927247898545687, 16.52544592524342804, 84.79057627198102409 ) ) ;
#115736=CARTESIAN_POINT ( 'NONE',  ( -5.823673210054116645, -21.52544592524344225, 92.29057627198103830 ) ) ;
#115737=CARTESIAN_POINT ( 'NONE',  ( -5.049401038298153566, 19.05341960407611168, 100.2072429386476955 ) ) ;
#115738=CARTESIAN_POINT ( 'NONE',  ( -21.53943276465977519, 0.05219959533907696930, 111.2489096053143669 ) ) ;
#115739=CARTESIAN_POINT ( 'NONE',  ( -5.153800228976328057, -19.02544592524343514, 102.2905762719810383 ) ) ;
#115740=CARTESIAN_POINT ( 'NONE',  ( 8.224510206698953496, -14.34966873604960469, 97.91557627198103830 ) ) ;
#115741=CARTESIAN_POINT ( 'NONE',  ( -21.52544592524334988, -5.823673210054445271, 73.95942372801901854 ) ) ;
#115742=CARTESIAN_POINT ( 'NONE',  ( -15.72974639402197994, 15.80617190586746368, 95.62390960531436690 ) ) ;
#115743=CARTESIAN_POINT ( 'NONE',  ( 17.05116617787824396, -6.768360034955795967, 106.1567555325920011 ) ) ;
#115744=DIRECTION ( 'NONE',  ( 6.718897857320949450E-15, -0.9991276842514722478, 0.04175967627138119087 ) ) ;
#115746=CARTESIAN_POINT ( 'NONE',  ( -16.55341960407617563, 4.379528057220093196, 28.54275706135234358 ) ) ;
#115747=CARTESIAN_POINT ( 'NONE',  ( 8.224510206698953496, -14.34966873604960469, 112.9155762719810383 ) ) ;
#115749=CARTESIAN_POINT ( 'NONE',  ( 0.05219959533909260263, 19.03943276465977164, 64.99890960531436690 ) ) ;
#115750=CARTESIAN_POINT ( 'NONE',  ( -4.483927247898539470, -16.52544592524342804, 92.29057627198103830 ) ) ;
#115751=CARTESIAN_POINT ( 'NONE',  ( 21.53943276465977519, -0.05219959533907433946, 33.74890960531436690 ) ) ;
#115752=CARTESIAN_POINT ( 'NONE',  ( -14.34966873604960291, -8.224510206698953496, 66.66557627198102409 ) ) ;
#115753=CARTESIAN_POINT ( 'NONE',  ( -4.379528057220086978, -16.55341960407618274, 24.79275706135235779 ) ) ;
#115754=CARTESIAN_POINT ( 'NONE',  ( -15.80617190586768217, 15.72974639402176855, 73.12609039468567573 ) ) ;
#115756=CARTESIAN_POINT ( 'NONE',  ( 13.89961937509977652, -13.97604488694527269, 113.1239096053143527 ) ) ;
#115757=CARTESIAN_POINT ( 'NONE',  ( 12.06949235617739724, 12.14591786802326823, 101.8760903946857042 ) ) ;
#115758=CARTESIAN_POINT ( 'NONE',  ( -19.05341960407611168, -5.049401038298163336, 36.45724293864766707 ) ) ;
#115759=CARTESIAN_POINT ( 'NONE',  ( 19.03943276465977164, -0.05219959533909143690, 88.74890960531436690 ) ) ;
#115760=CARTESIAN_POINT ( 'NONE',  ( 15.72974639402199770, -15.80617190586745480, 93.12390960531436690 ) ) ;
#115761=CARTESIAN_POINT ( 'NONE',  ( -12.14591786802326823, 12.06949235617739902, 28.12609039468568284 ) ) ;
#115762=CARTESIAN_POINT ( 'NONE',  ( -16.52544592524342804, 4.483927247898546575, 61.04057627198103120 ) ) ;
#115763=CARTESIAN_POINT ( 'NONE',  ( -10.81492255796105439, 18.62759615963255655, 67.91775706135234714 ) ) ;
#115765=CARTESIAN_POINT ( 'NONE',  ( 14.34966873604972726, -8.224510206698740333, 95.83442372801903275 ) ) ;
#115766=CARTESIAN_POINT ( 'NONE',  ( 17.26172910966717211, -6.454744622556960465, 48.30646908649207205 ) ) ;
#115767=CARTESIAN_POINT ( 'NONE',  ( 4.483927247898545687, 16.52544592524342804, 34.79057627198103120 ) ) ;
#115768=CARTESIAN_POINT ( 'NONE',  ( -16.55341960407617563, 4.379528057220093196, 58.54275706135235424 ) ) ;
#115769=CARTESIAN_POINT ( 'NONE',  ( 16.51473224551069308, 9.474510206698969483, 69.16557627198102409 ) ) ;
#115770=CARTESIAN_POINT ( 'NONE',  ( 19.05341960407611168, 5.049401038298154454, 88.95724293864769550 ) ) ;
#115771=CARTESIAN_POINT ( 'NONE',  ( -5.719274019375665041, -21.55341960407619695, 84.79275706135234714 ) ) ;
#115772=CARTESIAN_POINT ( 'NONE',  ( -4.379528057220086978, -16.55341960407618274, 89.79275706135236135 ) ) ;
#115773=CARTESIAN_POINT ( 'NONE',  ( 8.314922557960818139, 14.29746914071049879, 54.58224293864769550 ) ) ;
#115774=CARTESIAN_POINT ( 'NONE',  ( -9.564922557960796823, -16.46253265017161027, 72.08224293864770971 ) ) ;
#115776=CARTESIAN_POINT ( 'NONE',  ( -12.06949235617739369, -12.14591786802326823, 19.37609039468568639 ) ) ;
#115777=CARTESIAN_POINT ( 'NONE',  ( -0.05219959533910754901, -16.53943276465976808, 112.4989096053143669 ) ) ;
#115778=CARTESIAN_POINT ( 'NONE',  ( 13.89961937509977652, -13.97604488694527269, 83.12390960531436690 ) ) ;
#115779=CARTESIAN_POINT ( 'NONE',  ( -4.379528057220086978, -16.55341960407618274, 24.79275706135235779 ) ) ;
#115781=CARTESIAN_POINT ( 'NONE',  ( 5.823673210054444382, -21.52544592524334988, 110.2094237280190185 ) ) ;
#115782=CARTESIAN_POINT ( 'NONE',  ( 8.224510206698742110, 14.34966873604972548, 77.08442372801901854 ) ) ;
#115783=CARTESIAN_POINT ( 'NONE',  ( 16.46253265017146816, 9.564922557961045513, 86.66775706135233293 ) ) ;
#115784=CARTESIAN_POINT ( 'NONE',  ( -14.29746914071049879, 8.314922557960819915, 115.8322429386477097 ) ) ;
#115785=CARTESIAN_POINT ( 'NONE',  ( -14.34966873604972548, 8.224510206698743886, 63.33442372801900433 ) ) ;
#115787=CARTESIAN_POINT ( 'NONE',  ( -9.474510206698720793, -16.51473224551083518, 49.58442372801899722 ) ) ;
#115788=CARTESIAN_POINT ( 'NONE',  ( 15.80617190586769283, -15.72974639402175789, 95.62609039468568994 ) ) ;
#115789=CARTESIAN_POINT ( 'NONE',  ( 19.05341960407611168, 5.049401038298154454, 38.95724293864767418 ) ) ;
#115790=CARTESIAN_POINT ( 'NONE',  ( -16.46253265017160317, 9.564922557960807481, 80.83224293864769550 ) ) ;
#115791=CARTESIAN_POINT ( 'NONE',  ( -14.34966873604960291, -8.224510206698953496, 66.66557627198102409 ) ) ;
#115792=CARTESIAN_POINT ( 'NONE',  ( 21.53943276465977519, 0.05219959533937863772, 96.25109039468568994 ) ) ;
#115793=CARTESIAN_POINT ( 'NONE',  ( -19.05341960407617563, 5.049401038297882671, 48.54275706135233293 ) ) ;
#115794=CARTESIAN_POINT ( 'NONE',  ( 19.02544592524334988, 5.153800228976608722, 41.45942372801900433 ) ) ;
#115795=CARTESIAN_POINT ( 'NONE',  ( -21.55341960407610458, -5.719274019375992779, 41.45724293864769550 ) ) ;
#115796=CARTESIAN_POINT ( 'NONE',  ( -10.72451020669870658, -18.67979575497194134, 99.58442372801900433 ) ) ;
#115797=CARTESIAN_POINT ( 'NONE',  ( 9.474510206698971260, -16.51473224551069308, 77.91557627198103830 ) ) ;
#115798=CARTESIAN_POINT ( 'NONE',  ( 18.67979575497194134, -10.72451020669871369, 90.83442372801901854 ) ) ;
#115799=CARTESIAN_POINT ( 'NONE',  ( -15.80617190586745835, -15.72974639402198527, 51.87390960531437401 ) ) ;
#115800=CARTESIAN_POINT ( 'NONE',  ( -5.049401038298153566, 19.05341960407611168, 100.2072429386476955 ) ) ;
#115801=CARTESIAN_POINT ( 'NONE',  ( 0.05219959533936267826, -19.03943276465977164, 70.00109039468566152 ) ) ;
#115802=CARTESIAN_POINT ( 'NONE',  ( 9.564922557960805705, 16.46253265017160317, 104.5822429386476955 ) ) ;
#115803=CARTESIAN_POINT ( 'NONE',  ( 0.05219959533936267826, -19.03943276465977164, 95.00109039468567573 ) ) ;
#115804=CARTESIAN_POINT ( 'NONE',  ( -12.14591786802326823, 12.06949235617739902, 48.12609039468568284 ) ) ;
#115805=CARTESIAN_POINT ( 'NONE',  ( 14.29746914071049879, -8.314922557960816363, 98.33224293864769550 ) ) ;
#115806=CARTESIAN_POINT ( 'NONE',  ( -5.049401038298153566, 19.05341960407611168, 70.20724293864769550 ) ) ;
#115807=CARTESIAN_POINT ( 'NONE',  ( 21.53943276465977519, -0.05219959533907433946, 63.74890960531435979 ) ) ;
#115809=CARTESIAN_POINT ( 'NONE',  ( 16.52544592524335698, 4.483927247898782831, 36.45942372801901143 ) ) ;
#115810=CARTESIAN_POINT ( 'NONE',  ( -5.823673210054431948, 21.52544592524334988, 37.70942372801900433 ) ) ;
#115811=CARTESIAN_POINT ( 'NONE',  ( -10.81492255796105439, 18.62759615963255655, 87.91775706135234714 ) ) ;
#115812=CARTESIAN_POINT ( 'NONE',  ( 8.314922557961029526, -14.29746914071037800, 85.41775706135236135 ) ) ;
#115813=CARTESIAN_POINT ( 'NONE',  ( 5.153800228976335163, 19.02544592524342804, 69.79057627198103830 ) ) ;
#115814=CARTESIAN_POINT ( 'NONE',  ( -0.05219959533910754901, -16.53943276465976808, 72.49890960531435269 ) ) ;
#115815=CARTESIAN_POINT ( 'NONE',  ( 8.314922557960818139, 14.29746914071049879, 29.58224293864769905 ) ) ;
#115816=CARTESIAN_POINT ( 'NONE',  ( 19.05341960407617918, -5.049401038297876454, 51.04275706135231871 ) ) ;
#115817=CARTESIAN_POINT ( 'NONE',  ( 15.72974639402176855, 15.80617190586768217, 31.87609039468567929 ) ) ;
#115818=CARTESIAN_POINT ( 'NONE',  ( 4.483927247898545687, 16.52544592524342804, 79.79057627198102409 ) ) ;
#115819=CARTESIAN_POINT ( 'NONE',  ( 9.564922557960805705, 16.46253265017160317, 99.58224293864770971 ) ) ;
#115820=CARTESIAN_POINT ( 'NONE',  ( 14.29746914071037800, 8.314922557961029526, 106.6677570613523756 ) ) ;
#115821=CARTESIAN_POINT ( 'NONE',  ( 21.52544592524334988, 5.823673210054432836, 71.45942372801901854 ) ) ;
#115822=CARTESIAN_POINT ( 'NONE',  ( -16.55341960407617563, 4.379528057220093196, 48.54275706135234714 ) ) ;
#115823=CARTESIAN_POINT ( 'NONE',  ( 21.52544592524334988, 5.823673210054432836, 41.45942372801901143 ) ) ;
#115824=CARTESIAN_POINT ( 'NONE',  ( -4.379528057220328563, 16.55341960407611168, 65.20724293864768129 ) ) ;
#115826=ORIENTED_EDGE ( 'NONE', *, *, #130089, .T. ) ;
#115827=CARTESIAN_POINT ( 'NONE',  ( -5.719274019375665041, -21.55341960407619695, 19.79275706135235069 ) ) ;
#115828=CARTESIAN_POINT ( 'NONE',  ( 17.49999999999999645, -4.013004640162636250, 27.94605720994409737 ) ) ;
#115829=CARTESIAN_POINT ( 'NONE',  ( 12.14591786802309770, 12.06949235617756955, 54.37390960531435979 ) ) ;
#115830=CARTESIAN_POINT ( 'NONE',  ( 0.05219959533909260263, 19.03943276465977164, 24.99890960531435269 ) ) ;
#115831=CARTESIAN_POINT ( 'NONE',  ( 21.55341960407610458, 5.719274019375980345, 38.95724293864768839 ) ) ;
#115832=CARTESIAN_POINT ( 'NONE',  ( 16.55341960407611168, 4.379528057220329451, 78.95724293864769550 ) ) ;
#115834=CARTESIAN_POINT ( 'NONE',  ( 18.62759615963271287, -10.81492255796078972, 83.33224293864769550 ) ) ;
#115835=CARTESIAN_POINT ( 'NONE',  ( -19.02544592524342804, 5.153800228976336051, 86.04057627198103830 ) ) ;
#115836=CARTESIAN_POINT ( 'NONE',  ( -5.049401038298153566, 19.05341960407611168, 35.20724293864768839 ) ) ;
#115837=CARTESIAN_POINT ( 'NONE',  ( 19.02544592524334988, 5.153800228976608722, 81.45942372801897591 ) ) ;
#115838=CARTESIAN_POINT ( 'NONE',  ( -21.55341960407619339, 5.719274019375674811, 58.54275706135235424 ) ) ;
#115839=CARTESIAN_POINT ( 'NONE',  ( -5.823673210054116645, -21.52544592524344225, 57.29057627198103120 ) ) ;
#115840=CARTESIAN_POINT ( 'NONE',  ( 19.05341960407611168, 5.049401038298154454, 38.95724293864767418 ) ) ;
#115841=CARTESIAN_POINT ( 'NONE',  ( 9.564922557960805705, 16.46253265017160317, 69.58224293864770971 ) ) ;
#115843=CARTESIAN_POINT ( 'NONE',  ( -12.14591786802326823, 12.06949235617739902, 53.12609039468568284 ) ) ;
#115844=CARTESIAN_POINT ( 'NONE',  ( -15.72974639402176322, -15.80617190586768395, 24.37609039468567573 ) ) ;
#115845=CARTESIAN_POINT ( 'NONE',  ( -10.81492255796105439, 18.62759615963255655, 67.91775706135234714 ) ) ;
#115846=CARTESIAN_POINT ( 'NONE',  ( 16.46253265017160672, -9.564922557960803928, 98.33224293864769550 ) ) ;
#115847=CARTESIAN_POINT ( 'NONE',  ( -5.719274019375978568, 21.55341960407610458, 85.20724293864770971 ) ) ;
#115848=CARTESIAN_POINT ( 'NONE',  ( 15.80617190586769283, -15.72974639402175789, 30.62609039468567929 ) ) ;
#115849=CARTESIAN_POINT ( 'NONE',  ( -4.379528057220086978, -16.55341960407618274, 54.79275706135235424 ) ) ;
#115850=CARTESIAN_POINT ( 'NONE',  ( 15.80617190586746368, 15.72974639402197994, 49.37390960531436690 ) ) ;
#115851=CARTESIAN_POINT ( 'NONE',  ( 5.153800228976615827, -19.02544592524334988, 25.20942372801900433 ) ) ;
#115852=CARTESIAN_POINT ( 'NONE',  ( -19.05341960407611168, -5.049401038298163336, 51.45724293864770260 ) ) ;
#115853=CARTESIAN_POINT ( 'NONE',  ( 0.05219959533909260263, 19.03943276465977164, 114.9989096053143669 ) ) ;
#115854=CARTESIAN_POINT ( 'NONE',  ( 5.049401038298161559, -19.05341960407611168, 87.70724293864769550 ) ) ;
#115855=CARTESIAN_POINT ( 'NONE',  ( 18.22780087662126647, 5.499999999999818812, 51.48236817873107896 ) ) ;
#115856=CARTESIAN_POINT ( 'NONE',  ( 9.474510206698729675, 16.51473224551082808, 62.08442372801899722 ) ) ;
#115857=CARTESIAN_POINT ( 'NONE',  ( -5.823673210054116645, -21.52544592524344225, 47.29057627198103120 ) ) ;
#115858=CARTESIAN_POINT ( 'NONE',  ( -8.224510206698948167, 14.34966873604960824, 25.41557627198103120 ) ) ;
#115859=CARTESIAN_POINT ( 'NONE',  ( 19.05341960407617918, -5.049401038297876454, 101.0427570613523045 ) ) ;
#115861=CARTESIAN_POINT ( 'NONE',  ( 0.05219959533936267826, -19.03943276465977164, 20.00109039468567218 ) ) ;
#115862=CARTESIAN_POINT ( 'NONE',  ( 9.564922557961047289, -16.46253265017146816, 95.41775706135233293 ) ) ;
#115863=CARTESIAN_POINT ( 'NONE',  ( -0.05219959533907301413, -21.53943276465977519, 77.49890960531433848 ) ) ;
#115864=CARTESIAN_POINT ( 'NONE',  ( -9.474510206698720793, -16.51473224551083518, 59.58442372801900433 ) ) ;
#115866=CARTESIAN_POINT ( 'NONE',  ( 19.03943276465977164, -0.05219959533909143690, 53.74890960531436690 ) ) ;
#115867=CARTESIAN_POINT ( 'NONE',  ( 8.224510206698953496, -14.34966873604960469, 62.91557627198102409 ) ) ;
#115868=CARTESIAN_POINT ( 'NONE',  ( 19.02544592524343514, -5.153800228976328945, 38.54057627198103120 ) ) ;
#115869=CARTESIAN_POINT ( 'NONE',  ( -0.05219959533910754901, -16.53943276465976808, 37.49890960531436690 ) ) ;
#115871=CARTESIAN_POINT ( 'NONE',  ( -16.55341960407617563, 4.379528057220093196, 103.5427570613523613 ) ) ;
#115872=CARTESIAN_POINT ( 'NONE',  ( -0.05219959533909027116, -19.03943276465977164, 67.49890960531436690 ) ) ;
#115873=CARTESIAN_POINT ( 'NONE',  ( 19.03943276465977164, 0.05219959533936151252, 21.25109039468565797 ) ) ;
#115874=CARTESIAN_POINT ( 'NONE',  ( -16.55341960407617563, 4.379528057220093196, 33.54275706135234714 ) ) ;
#115875=CARTESIAN_POINT ( 'NONE',  ( 5.823673210054125526, 21.52544592524343514, 54.79057627198104541 ) ) ;
#115876=CARTESIAN_POINT ( 'NONE',  ( 5.823673210054444382, -21.52544592524334988, 110.2094237280190185 ) ) ;
#115877=CARTESIAN_POINT ( 'NONE',  ( -19.03943276465977164, 0.05219959533909376836, 61.24890960531436690 ) ) ;
#115878=CARTESIAN_POINT ( 'NONE',  ( 17.49999999999999289, 5.500000000000009770, 43.78230962303566542 ) ) ;
#115879=CARTESIAN_POINT ( 'NONE',  ( 19.03943276465977164, -0.05219959533909143690, 103.7489096053143669 ) ) ;
#115881=CARTESIAN_POINT ( 'NONE',  ( 21.55341960407619695, -5.719274019375665929, 26.04275706135235779 ) ) ;
#115882=CARTESIAN_POINT ( 'NONE',  ( 8.224510206698953496, -14.34966873604960469, 92.91557627198103830 ) ) ;
#115883=CARTESIAN_POINT ( 'NONE',  ( 15.72974639402199770, -15.80617190586745480, 88.12390960531436690 ) ) ;
#115884=CARTESIAN_POINT ( 'NONE',  ( 16.46253265017160672, -9.564922557960803928, 63.33224293864769550 ) ) ;
#115885=CARTESIAN_POINT ( 'NONE',  ( 5.049401038298161559, -19.05341960407611168, 67.70724293864769550 ) ) ;
#115886=CARTESIAN_POINT ( 'NONE',  ( 10.72451020669898902, -18.67979575497178502, 107.9155762719810241 ) ) ;
#115888=CARTESIAN_POINT ( 'NONE',  ( -9.564922557960796823, -16.46253265017161027, 72.08224293864770971 ) ) ;
#115890=CARTESIAN_POINT ( 'NONE',  ( 16.53943276465976808, -0.05219959533910856209, 103.7489096053143669 ) ) ;
#115891=CARTESIAN_POINT ( 'NONE',  ( -13.97604488694527625, -13.89961937509977652, 26.87390960531434558 ) ) ;
#115892=CARTESIAN_POINT ( 'NONE',  ( -9.564922557961040184, 16.46253265017147172, 87.91775706135233293 ) ) ;
#115893=CARTESIAN_POINT ( 'NONE',  ( 14.29746914071049879, -8.314922557960816363, 103.3322429386476955 ) ) ;
#115894=CARTESIAN_POINT ( 'NONE',  ( 21.53943276465977519, 0.05219959533937863772, 71.25109039468568994 ) ) ;
#115895=CARTESIAN_POINT ( 'NONE',  ( 19.03943276465977164, -0.05219959533909143690, 58.74890960531435979 ) ) ;
#115896=CARTESIAN_POINT ( 'NONE',  ( 5.823673210054444382, -21.52544592524334988, 30.20942372801902565 ) ) ;
#115897=CARTESIAN_POINT ( 'NONE',  ( -0.05219959533907301413, -21.53943276465977519, 112.4989096053143669 ) ) ;
#115899=CARTESIAN_POINT ( 'NONE',  ( -19.05341960407611168, -5.049401038298163336, 71.45724293864766707 ) ) ;
#115901=CARTESIAN_POINT ( 'NONE',  ( 14.29746914071037800, 8.314922557961029526, 26.66775706135235424 ) ) ;
#115902=CARTESIAN_POINT ( 'NONE',  ( -5.823673210054116645, -21.52544592524344225, 27.29057627198103120 ) ) ;
#115903=CARTESIAN_POINT ( 'NONE',  ( -21.53943276465977519, -0.05219959533937600094, 58.75109039468568994 ) ) ;
#115904=CARTESIAN_POINT ( 'NONE',  ( 0.05219959533909260263, 19.03943276465977164, 104.9989096053143669 ) ) ;
#115905=CARTESIAN_POINT ( 'NONE',  ( 13.89961937509957401, 13.97604488694547697, 101.8760903946856331 ) ) ;
#115906=CARTESIAN_POINT ( 'NONE',  ( -13.89961937509977652, 13.97604488694528158, 50.62390960531435979 ) ) ;
#115907=CARTESIAN_POINT ( 'NONE',  ( -19.02544592524342804, 5.153800228976336051, 71.04057627198099567 ) ) ;
#115908=CARTESIAN_POINT ( 'NONE',  ( 12.14591786802309770, 12.06949235617756955, 94.37390960531436690 ) ) ;
#115909=CARTESIAN_POINT ( 'NONE',  ( -13.97604488694527625, -13.89961937509977652, 101.8739096053143811 ) ) ;
#115910=CARTESIAN_POINT ( 'NONE',  ( -12.06949235617756955, 12.14591786802309770, 95.62390960531436690 ) ) ;
#115911=CARTESIAN_POINT ( 'NONE',  ( -5.049401038298153566, 19.05341960407611168, 95.20724293864770971 ) ) ;
#115912=CARTESIAN_POINT ( 'NONE',  ( 12.14591786802309770, 12.06949235617756955, 44.37390960531435979 ) ) ;
#115913=CARTESIAN_POINT ( 'NONE',  ( -9.564922557960796823, -16.46253265017161027, 37.08224293864768839 ) ) ;
#115915=CARTESIAN_POINT ( 'NONE',  ( -5.823673210054431948, 21.52544592524334988, 57.70942372801901143 ) ) ;
#115916=CARTESIAN_POINT ( 'NONE',  ( -13.89961937509957401, -13.97604488694547875, 84.37609039468567573 ) ) ;
#115917=CARTESIAN_POINT ( 'NONE',  ( 14.34966873604960469, 8.224510206698951720, 49.16557627198102409 ) ) ;
#115918=CARTESIAN_POINT ( 'NONE',  ( -21.52544592524343514, 5.823673210054127303, 101.0405762719810383 ) ) ;
#115919=CARTESIAN_POINT ( 'NONE',  ( -15.80617190586745835, -15.72974639402198527, 41.87390960531435979 ) ) ;
#115920=CARTESIAN_POINT ( 'NONE',  ( -5.049401038298153566, 19.05341960407611168, 110.2072429386476671 ) ) ;
#115921=CARTESIAN_POINT ( 'NONE',  ( 14.29746914071049879, -8.314922557960816363, 78.33224293864770971 ) ) ;
#115922=CARTESIAN_POINT ( 'NONE',  ( 13.97604488694527802, 13.89961937509977652, 59.37390960531434558 ) ) ;
#115923=CARTESIAN_POINT ( 'NONE',  ( 14.29746914071049879, -8.314922557960816363, 28.33224293864769550 ) ) ;
#115924=CARTESIAN_POINT ( 'NONE',  ( -14.29746914071037622, -8.314922557961029526, 104.1677570613523471 ) ) ;
#115925=CARTESIAN_POINT ( 'NONE',  ( 0.05219959533934541429, -16.53943276465976808, 70.00109039468568994 ) ) ;
#115926=CARTESIAN_POINT ( 'NONE',  ( -19.05341960407617563, 5.049401038297882671, 23.54275706135233648 ) ) ;
#115928=CARTESIAN_POINT ( 'NONE',  ( -16.51473224551069308, -9.474510206698971260, 111.6655762719810383 ) ) ;
#115929=CARTESIAN_POINT ( 'NONE',  ( 5.049401038298161559, -19.05341960407611168, 72.70724293864768129 ) ) ;
#115930=CARTESIAN_POINT ( 'NONE',  ( 13.89961937509977652, -13.97604488694527269, 38.12390960531436690 ) ) ;
#115931=CARTESIAN_POINT ( 'NONE',  ( 8.224510206698953496, -14.34966873604960469, 47.91557627198102409 ) ) ;
#115932=CARTESIAN_POINT ( 'NONE',  ( -0.05219959533909027116, -19.03943276465977164, 112.4989096053143669 ) ) ;
#115933=CARTESIAN_POINT ( 'NONE',  ( -16.51473224551069308, -9.474510206698971260, 101.6655762719810241 ) ) ;
#115934=CARTESIAN_POINT ( 'NONE',  ( -18.67979575497178146, -10.72451020669898902, 41.66557627198103120 ) ) ;
#115935=CARTESIAN_POINT ( 'NONE',  ( -8.314922557960811034, -14.29746914071050412, 82.08224293864768129 ) ) ;
#115936=CARTESIAN_POINT ( 'NONE',  ( 4.483927247898790824, -16.52544592524335698, 45.20942372801901854 ) ) ;
#115937=CARTESIAN_POINT ( 'NONE',  ( 16.55341960407611168, 4.379528057220329451, 58.95724293864770971 ) ) ;
#115939=CARTESIAN_POINT ( 'NONE',  ( 5.153800228976615827, -19.02544592524334988, 60.20942372801899012 ) ) ;
#115940=CARTESIAN_POINT ( 'NONE',  ( -5.153800228976328057, -19.02544592524343514, 102.2905762719810383 ) ) ;
#115941=CARTESIAN_POINT ( 'NONE',  ( 5.153800228976615827, -19.02544592524334988, 85.20942372801900433 ) ) ;
#115943=CARTESIAN_POINT ( 'NONE',  ( 5.153800228976617603, -19.02544592524335343, 95.20942372801899012 ) ) ;
#115944=CARTESIAN_POINT ( 'NONE',  ( 13.97604488694548053, -13.89961937509957401, 110.6260903946856615 ) ) ;
#115945=CARTESIAN_POINT ( 'NONE',  ( 8.224510206698953496, -14.34966873604960469, 22.91557627198102765 ) ) ;
#115946=CARTESIAN_POINT ( 'NONE',  ( -16.46253265017146816, -9.564922557961047289, 69.16775706135233293 ) ) ;
#115947=CARTESIAN_POINT ( 'NONE',  ( -0.05219959533907301413, -21.53943276465977519, 32.49890960531435979 ) ) ;
#115948=CARTESIAN_POINT ( 'NONE',  ( -10.72451020669870658, -18.67979575497194134, 64.58442372801900433 ) ) ;
#115950=CARTESIAN_POINT ( 'NONE',  ( 13.89961937509957401, 13.97604488694547697, 111.8760903946856757 ) ) ;
#115951=CARTESIAN_POINT ( 'NONE',  ( -13.97604488694527625, -13.89961937509977652, 26.87390960531434558 ) ) ;
#115952=CARTESIAN_POINT ( 'NONE',  ( -9.564922557960796823, -16.46253265017161027, 77.08224293864769550 ) ) ;
#115953=CARTESIAN_POINT ( 'NONE',  ( 5.049401038298161559, -19.05341960407611168, 22.70724293864769194 ) ) ;
#115954=CARTESIAN_POINT ( 'NONE',  ( -8.224510206698948167, 14.34966873604960824, 90.41557627198103830 ) ) ;
#115955=CARTESIAN_POINT ( 'NONE',  ( -16.51473224551069308, -9.474510206698971260, 81.66557627198103830 ) ) ;
#115956=CARTESIAN_POINT ( 'NONE',  ( -13.89961937509977652, 13.97604488694528158, 85.62390960531433848 ) ) ;
#115958=CARTESIAN_POINT ( 'NONE',  ( -16.46253265017146816, -9.564922557961047289, 94.16775706135233293 ) ) ;
#115959=CARTESIAN_POINT ( 'NONE',  ( -10.81492255796078084, -18.62759615963271287, 77.08224293864769550 ) ) ;
#115960=CARTESIAN_POINT ( 'NONE',  ( -13.89961937509977652, 13.97604488694528158, 25.62390960531434558 ) ) ;
#115961=CARTESIAN_POINT ( 'NONE',  ( 19.02544592524334988, 5.153800228976608722, 76.45942372801897591 ) ) ;
#115962=CARTESIAN_POINT ( 'NONE',  ( -16.51473224551069308, -9.474510206698971260, 66.66557627198102409 ) ) ;
#115963=CARTESIAN_POINT ( 'NONE',  ( -5.153800228976328057, -19.02544592524343514, 97.29057627198099567 ) ) ;
#115965=CARTESIAN_POINT ( 'NONE',  ( 21.53943276465977519, -0.05219959533907433946, 103.7489096053143669 ) ) ;
#115966=CARTESIAN_POINT ( 'NONE',  ( -4.483927247898539470, -16.52544592524342804, 92.29057627198103830 ) ) ;
#115967=CARTESIAN_POINT ( 'NONE',  ( -16.46253265017160317, 9.564922557960807481, 80.83224293864769550 ) ) ;
#115968=CARTESIAN_POINT ( 'NONE',  ( 13.89961937509957401, 13.97604488694547697, 61.87609039468566863 ) ) ;
#115969=CARTESIAN_POINT ( 'NONE',  ( 18.67979575497178502, 10.72451020669898547, 94.16557627198103830 ) ) ;
#115970=CARTESIAN_POINT ( 'NONE',  ( -15.72974639402197994, 15.80617190586746368, 70.62390960531436690 ) ) ;
#115971=CARTESIAN_POINT ( 'NONE',  ( 16.52544592524342804, -4.483927247898539470, 48.54057627198103120 ) ) ;
#115972=CARTESIAN_POINT ( 'NONE',  ( -15.72974639402176322, -15.80617190586768395, 109.3760903946857042 ) ) ;
#115973=CARTESIAN_POINT ( 'NONE',  ( 4.483927247898790824, -16.52544592524335698, 65.20942372801901854 ) ) ;
#115974=CARTESIAN_POINT ( 'NONE',  ( -9.474510206698964154, 16.51473224551069663, 95.41557627198102409 ) ) ;
#115975=CARTESIAN_POINT ( 'NONE',  ( -19.03943276465977164, 0.05219959533909376836, 31.24890960531435979 ) ) ;
#115976=CARTESIAN_POINT ( 'NONE',  ( -18.62759615963255300, -10.81492255796106328, 44.16775706135234714 ) ) ;
#115977=CARTESIAN_POINT ( 'NONE',  ( -5.719274019375665041, -21.55341960407619695, 59.79275706135234714 ) ) ;
#115978=CARTESIAN_POINT ( 'NONE',  ( 16.51473224551069308, 9.474510206698969483, 59.16557627198102409 ) ) ;
#115979=CARTESIAN_POINT ( 'NONE',  ( 21.53943276465977519, 0.05219959533937863772, 41.25109039468568284 ) ) ;
#115980=CARTESIAN_POINT ( 'NONE',  ( 5.153800228976615827, -19.02544592524334988, 75.20942372801896170 ) ) ;
#115981=CARTESIAN_POINT ( 'NONE',  ( 16.46253265017146816, 9.564922557961045513, 76.66775706135234714 ) ) ;
#115982=CARTESIAN_POINT ( 'NONE',  ( -5.049401038298153566, 19.05341960407611168, 40.20724293864768839 ) ) ;
#115983=CARTESIAN_POINT ( 'NONE',  ( 4.379528057220092307, 16.55341960407617563, 72.29275706135236135 ) ) ;
#115984=CARTESIAN_POINT ( 'NONE',  ( -0.05219959533909027116, -19.03943276465977164, 52.49890960531436690 ) ) ;
#115986=CARTESIAN_POINT ( 'NONE',  ( -0.05219959533909027116, -19.03943276465977164, 97.49890960531436690 ) ) ;
#115987=CARTESIAN_POINT ( 'NONE',  ( -16.51473224551069308, -9.474510206698971260, 41.66557627198103120 ) ) ;
#115988=CARTESIAN_POINT ( 'NONE',  ( 18.67979575497178502, 10.72451020669898547, 69.16557627198102409 ) ) ;
#115989=CARTESIAN_POINT ( 'NONE',  ( 0.05219959533934541429, -16.53943276465976808, 60.00109039468568284 ) ) ;
#115990=CARTESIAN_POINT ( 'NONE',  ( -9.474510206698720793, -16.51473224551083518, 19.58442372801899722 ) ) ;
#115991=CARTESIAN_POINT ( 'NONE',  ( 13.89961937509977652, -13.97604488694527269, 53.12390960531434558 ) ) ;
#115992=CARTESIAN_POINT ( 'NONE',  ( -0.05219959533910754901, -16.53943276465976808, 42.49890960531435979 ) ) ;
#115993=CARTESIAN_POINT ( 'NONE',  ( 8.224510206698953496, -14.34966873604960469, 87.91557627198103830 ) ) ;
#115994=CARTESIAN_POINT ( 'NONE',  ( -16.51473224551069308, -9.474510206698971260, 81.66557627198103830 ) ) ;
#115995=CARTESIAN_POINT ( 'NONE',  ( -15.72974639402176322, -15.80617190586768395, 39.37609039468567573 ) ) ;
#115996=CARTESIAN_POINT ( 'NONE',  ( 0.05219959533909260263, 19.03943276465977164, 89.99890960531436690 ) ) ;
#115997=CARTESIAN_POINT ( 'NONE',  ( -10.72451020669870658, -18.67979575497194134, 104.5844237280190185 ) ) ;
#115998=CARTESIAN_POINT ( 'NONE',  ( 8.224510206698742110, 14.34966873604972548, 62.08442372801901143 ) ) ;
#115999=CARTESIAN_POINT ( 'NONE',  ( -9.564922557960796823, -16.46253265017161027, 107.0822429386476955 ) ) ;
#116000=CARTESIAN_POINT ( 'NONE',  ( 15.72974639402199770, -15.80617190586745480, 83.12390960531436690 ) ) ;
#116001=CARTESIAN_POINT ( 'NONE',  ( -16.55341960407611168, -4.379528057220339221, 51.45724293864770260 ) ) ;
#116002=CARTESIAN_POINT ( 'NONE',  ( 5.049401038298161559, -19.05341960407611168, 42.70724293864767418 ) ) ;
#116003=CARTESIAN_POINT ( 'NONE',  ( -8.314922557960811034, -14.29746914071050412, 62.08224293864769550 ) ) ;
#116004=CARTESIAN_POINT ( 'NONE',  ( -21.53943276465977519, 0.05219959533907696930, 26.24890960531435624 ) ) ;
#116005=CARTESIAN_POINT ( 'NONE',  ( -21.53943276465977519, 0.05219959533907696930, 26.24890960531435624 ) ) ;
#116006=CARTESIAN_POINT ( 'NONE',  ( 13.89961937509957401, 13.97604488694547697, 31.87609039468566863 ) ) ;
#116007=CARTESIAN_POINT ( 'NONE',  ( -8.314922557960811034, -14.29746914071050412, 97.08224293864770971 ) ) ;
#116008=CARTESIAN_POINT ( 'NONE',  ( 13.97604488694527802, 13.89961937509977652, 104.3739096053143385 ) ) ;
#116010=CARTESIAN_POINT ( 'NONE',  ( 12.06949235617739724, 12.14591786802326823, 51.87609039468568284 ) ) ;
#116011=CARTESIAN_POINT ( 'NONE',  ( 13.89961937509977652, -13.97604488694527269, 58.12390960531436690 ) ) ;
#116013=CARTESIAN_POINT ( 'NONE',  ( 16.46253265017146816, 9.564922557961045513, 66.66775706135233293 ) ) ;
#116014=CARTESIAN_POINT ( 'NONE',  ( -4.483927247898782831, 16.52544592524335698, 92.70942372801901854 ) ) ;
#116015=CARTESIAN_POINT ( 'NONE',  ( -16.51473224551082808, 9.474510206698731452, 93.33442372801900433 ) ) ;
#116016=CARTESIAN_POINT ( 'NONE',  ( 5.823673210054444382, -21.52544592524334988, 70.20942372801904696 ) ) ;
#116017=CARTESIAN_POINT ( 'NONE',  ( -9.474510206698964154, 16.51473224551069663, 80.41557627198103830 ) ) ;
#116018=CARTESIAN_POINT ( 'NONE',  ( 15.72974639402199770, -15.80617190586745480, 93.12390960531436690 ) ) ;
#116019=CARTESIAN_POINT ( 'NONE',  ( -19.03943276465977164, 0.05219959533909376836, 21.24890960531436335 ) ) ;
#116020=VECTOR ( 'NONE', #186214, 1000.000000000000000 ) ;
#116021=CARTESIAN_POINT ( 'NONE',  ( -19.05341960407617563, 5.049401038297882671, 78.54275706135233293 ) ) ;
#116022=CARTESIAN_POINT ( 'NONE',  ( 18.62759615963271287, -10.81492255796078972, 73.33224293864769550 ) ) ;
#116023=CARTESIAN_POINT ( 'NONE',  ( 19.02544592524334988, 5.153800228976608722, 46.45942372801899012 ) ) ;
#116025=CARTESIAN_POINT ( 'NONE',  ( -18.62759615963270932, 10.81492255796079327, 90.83224293864769550 ) ) ;
#116026=CARTESIAN_POINT ( 'NONE',  ( 17.50000000000003553, 3.850315288878739750, 28.23370869396553573 ) ) ;
#116027=CARTESIAN_POINT ( 'NONE',  ( 9.564922557960805705, 16.46253265017160317, 69.58224293864770971 ) ) ;
#116029=CARTESIAN_POINT ( 'NONE',  ( 4.379528057220092307, 16.55341960407617563, 22.29275706135235069 ) ) ;
#116031=CARTESIAN_POINT ( 'NONE',  ( 9.474510206698971260, -16.51473224551069308, 42.91557627198103120 ) ) ;
#116032=CARTESIAN_POINT ( 'NONE',  ( -21.52544592524343514, 5.823673210054127303, 106.0405762719810525 ) ) ;
#116033=CARTESIAN_POINT ( 'NONE',  ( -8.224510206698948167, 14.34966873604960824, 55.41557627198102409 ) ) ;
#116034=CARTESIAN_POINT ( 'NONE',  ( 5.153800228976335163, 19.02544592524342804, 59.79057627198100988 ) ) ;
#116035=CARTESIAN_POINT ( 'NONE',  ( -15.80617190586768217, 15.72974639402176855, 78.12609039468570415 ) ) ;
#116036=CARTESIAN_POINT ( 'NONE',  ( -16.52544592524335698, -4.483927247898792601, 23.95942372801901143 ) ) ;
#116037=CARTESIAN_POINT ( 'NONE',  ( -13.89961937509957401, -13.97604488694547875, 24.37609039468565442 ) ) ;
#116038=CARTESIAN_POINT ( 'NONE',  ( 4.483927247898545687, 16.52544592524342804, 24.79057627198103120 ) ) ;
#116039=CARTESIAN_POINT ( 'NONE',  ( 5.823673210054444382, -21.52544592524334988, 35.20942372801901854 ) ) ;
#116040=CARTESIAN_POINT ( 'NONE',  ( 18.67979575497194134, -10.72451020669871369, 20.83442372801901143 ) ) ;
#116041=CARTESIAN_POINT ( 'NONE',  ( 21.52544592524344225, -5.823673210054117533, 53.54057627198103120 ) ) ;
#116042=CARTESIAN_POINT ( 'NONE',  ( 5.153800228976615827, -19.02544592524334988, 90.20942372801900433 ) ) ;
#116043=CARTESIAN_POINT ( 'NONE',  ( 9.564922557961047289, -16.46253265017146816, 75.41775706135234714 ) ) ;
#116044=CARTESIAN_POINT ( 'NONE',  ( -18.62759615963255300, -10.81492255796106328, 69.16775706135234714 ) ) ;
#116045=CARTESIAN_POINT ( 'NONE',  ( 9.474510206698729675, 16.51473224551082808, 52.08442372801900433 ) ) ;
#116046=CARTESIAN_POINT ( 'NONE',  ( 13.89961937509977652, -13.97604488694527269, 23.12390960531436335 ) ) ;
#116047=CARTESIAN_POINT ( 'NONE',  ( -15.80617190586745835, -15.72974639402198527, 46.87390960531435979 ) ) ;
#116048=CARTESIAN_POINT ( 'NONE',  ( 4.483927247898545687, 16.52544592524342804, 49.79057627198102409 ) ) ;
#116049=CARTESIAN_POINT ( 'NONE',  ( -19.25663599770060586, 5.499999999999445777, 93.99419308057203182 ) ) ;
#116050=CARTESIAN_POINT ( 'NONE',  ( -18.67979575497193778, 10.72451020669871902, 108.3344237280190185 ) ) ;
#116051=CARTESIAN_POINT ( 'NONE',  ( 8.314922557961029526, -14.29746914071037800, 90.41775706135236135 ) ) ;
#116052=CARTESIAN_POINT ( 'NONE',  ( -8.224510206698948167, 14.34966873604960824, 40.41557627198103120 ) ) ;
#116053=CARTESIAN_POINT ( 'NONE',  ( 21.52544592524334988, 5.823673210054432836, 81.45942372801900433 ) ) ;
#116054=CARTESIAN_POINT ( 'NONE',  ( -10.72451020669870658, -18.67979575497194134, 74.58442372801901854 ) ) ;
#116055=CARTESIAN_POINT ( 'NONE',  ( -15.80617190586745835, -15.72974639402198527, 86.87390960531438111 ) ) ;
#116057=CARTESIAN_POINT ( 'NONE',  ( 19.02544592524343514, -5.153800228976328945, 33.54057627198102409 ) ) ;
#116058=CARTESIAN_POINT ( 'NONE',  ( 18.67979575497194134, -10.72451020669871369, 60.83442372801901854 ) ) ;
#116059=CARTESIAN_POINT ( 'NONE',  ( -9.474510206698964154, 16.51473224551069663, 30.41557627198102054 ) ) ;
#116060=CARTESIAN_POINT ( 'NONE',  ( 9.474510206698971260, -16.51473224551069308, 52.91557627198102409 ) ) ;
#116061=CARTESIAN_POINT ( 'NONE',  ( -0.05219959533910754901, -16.53943276465976808, 92.49890960531436690 ) ) ;
#116062=CARTESIAN_POINT ( 'NONE',  ( -19.05341960407611168, -5.049401038298163336, 101.4572429386476955 ) ) ;
#116063=CARTESIAN_POINT ( 'NONE',  ( 16.55341960407611168, 4.379528057220329451, 33.95724293864769550 ) ) ;
#116064=CARTESIAN_POINT ( 'NONE',  ( -5.153800228976328057, -19.02544592524343514, 22.29057627198102765 ) ) ;
#116065=CARTESIAN_POINT ( 'NONE',  ( 5.823673210054125526, 21.52544592524343514, 79.79057627198102409 ) ) ;
#116066=CARTESIAN_POINT ( 'NONE',  ( 0.05219959533937995610, -21.53943276465977519, 25.00109039468567218 ) ) ;
#116068=CARTESIAN_POINT ( 'NONE',  ( -16.52544592524335698, -4.483927247898792601, 28.95942372801902209 ) ) ;
#116069=CARTESIAN_POINT ( 'NONE',  ( -21.52544592524343514, 5.823673210054127303, 71.04057627198103830 ) ) ;
#116070=CARTESIAN_POINT ( 'NONE',  ( -5.823673210054431948, 21.52544592524334988, 97.70942372801904696 ) ) ;
#116071=CARTESIAN_POINT ( 'NONE',  ( 0.05219959533909260263, 19.03943276465977164, 79.99890960531436690 ) ) ;
#116072=CARTESIAN_POINT ( 'NONE',  ( 15.72974639402176855, 15.80617190586768217, 36.87609039468568994 ) ) ;
#116073=CARTESIAN_POINT ( 'NONE',  ( -5.153800228976328057, -19.02544592524343514, 112.2905762719810099 ) ) ;
#116074=CARTESIAN_POINT ( 'NONE',  ( 16.52544592524335698, 4.483927247898782831, 86.45942372801901854 ) ) ;
#116075=CARTESIAN_POINT ( 'NONE',  ( 15.72974639402176855, 15.80617190586768217, 76.87609039468567573 ) ) ;
#116076=CARTESIAN_POINT ( 'NONE',  ( -19.02544592524334988, -5.153800228976617603, 18.95942372801899722 ) ) ;
#116077=CARTESIAN_POINT ( 'NONE',  ( 12.06949235617739724, 12.14591786802326823, 71.87609039468568994 ) ) ;
#116078=CARTESIAN_POINT ( 'NONE',  ( 15.72974639402176855, 15.80617190586768217, 26.87609039468567218 ) ) ;
#116079=CARTESIAN_POINT ( 'NONE',  ( 19.03943276465977164, -0.05219959533909143690, 38.74890960531436690 ) ) ;
#116080=CARTESIAN_POINT ( 'NONE',  ( 15.72974639402176855, 15.80617190586768217, 86.87609039468568994 ) ) ;
#116081=CARTESIAN_POINT ( 'NONE',  ( 16.51473224551069308, 9.474510206698969483, 89.16557627198103830 ) ) ;
#116082=CARTESIAN_POINT ( 'NONE',  ( 15.72974639402199770, -15.80617190586745480, 93.12390960531436690 ) ) ;
#116083=CARTESIAN_POINT ( 'NONE',  ( 19.25918095147779496, 5.499999999999574563, 81.95284276293932635 ) ) ;
#116084=CARTESIAN_POINT ( 'NONE',  ( 0.05219959533907565091, 21.53943276465977519, 49.99890960531437401 ) ) ;
#116085=CARTESIAN_POINT ( 'NONE',  ( -13.97604488694527625, -13.89961937509977652, 96.87390960531433848 ) ) ;
#116086=CARTESIAN_POINT ( 'NONE',  ( -4.379528057220328563, 16.55341960407611168, 45.20724293864769550 ) ) ;
#116088=CARTESIAN_POINT ( 'NONE',  ( -13.89961937509957401, -13.97604488694547875, 74.37609039468566152 ) ) ;
#116089=CARTESIAN_POINT ( 'NONE',  ( -17.31747979337946219, 6.344076630961073882, 103.6205513193481949 ) ) ;
#116090=CARTESIAN_POINT ( 'NONE',  ( -13.89961937509957401, -13.97604488694547875, 104.3760903946856757 ) ) ;
#116091=CARTESIAN_POINT ( 'NONE',  ( -10.81492255796078084, -18.62759615963271287, 87.08224293864769550 ) ) ;
#116092=CARTESIAN_POINT ( 'NONE',  ( 14.29746914071049879, -8.314922557960816363, 63.33224293864770260 ) ) ;
#116093=CARTESIAN_POINT ( 'NONE',  ( 19.02544592524343514, -5.153800228976328945, 98.54057627198100988 ) ) ;
#116094=CARTESIAN_POINT ( 'NONE',  ( 12.06949235617739724, 12.14591786802326823, 46.87609039468568994 ) ) ;
#116095=CARTESIAN_POINT ( 'NONE',  ( 13.89961937509977652, -13.97604488694527269, 63.12390960531435979 ) ) ;
#116096=CARTESIAN_POINT ( 'NONE',  ( 21.55341960407619695, -5.719274019375665929, 31.04275706135234714 ) ) ;
#116097=CARTESIAN_POINT ( 'NONE',  ( -9.474510206698720793, -16.51473224551083518, 99.58442372801900433 ) ) ;
#116098=CARTESIAN_POINT ( 'NONE',  ( -19.03943276465977164, 0.05219959533909376836, 96.24890960531436690 ) ) ;
#116099=CARTESIAN_POINT ( 'NONE',  ( -16.51473224551069308, -9.474510206698971260, 86.66557627198102409 ) ) ;
#116100=CARTESIAN_POINT ( 'NONE',  ( 18.67979575497178502, 10.72451020669898547, 94.16557627198103830 ) ) ;
#116101=CARTESIAN_POINT ( 'NONE',  ( 0.05219959533909260263, 19.03943276465977164, 39.99890960531436690 ) ) ;
#116102=CARTESIAN_POINT ( 'NONE',  ( -17.13100169013299379, -6.664070546373172199, 59.23210164300151348 ) ) ;
#116103=CARTESIAN_POINT ( 'NONE',  ( -0.05219959533910754901, -16.53943276465976808, 67.49890960531436690 ) ) ;
#116104=CARTESIAN_POINT ( 'NONE',  ( -19.02544592524342804, 5.153800228976336051, 101.0405762719810241 ) ) ;
#116106=CARTESIAN_POINT ( 'NONE',  ( -13.89961937509957401, -13.97604488694547875, 59.37609039468566863 ) ) ;
#116107=CARTESIAN_POINT ( 'NONE',  ( -18.62759615963270932, 10.81492255796079327, 90.83224293864769550 ) ) ;
#116108=CARTESIAN_POINT ( 'NONE',  ( -0.05219959533936034679, 19.03943276465977164, 47.50109039468566863 ) ) ;
#116109=CARTESIAN_POINT ( 'NONE',  ( -9.564922557960796823, -16.46253265017161027, 107.0822429386476955 ) ) ;
#116110=CARTESIAN_POINT ( 'NONE',  ( 18.87255363501903105, 5.499999999999943157, 68.82513748171827217 ) ) ;
#116111=CARTESIAN_POINT ( 'NONE',  ( -10.81492255796078084, -18.62759615963271287, 47.08224293864770260 ) ) ;
#116112=CARTESIAN_POINT ( 'NONE',  ( 19.02544592524343514, -5.153800228976328945, 88.54057627198102409 ) ) ;
#116113=CARTESIAN_POINT ( 'NONE',  ( 5.719274019375673035, 21.55341960407619339, 62.29275706135236845 ) ) ;
#116114=CARTESIAN_POINT ( 'NONE',  ( 16.46253265017160672, -9.564922557960803928, 38.33224293864768839 ) ) ;
#116115=CARTESIAN_POINT ( 'NONE',  ( 16.53943276465976808, -0.05219959533910856209, 68.74890960531435269 ) ) ;
#116116=CARTESIAN_POINT ( 'NONE',  ( 8.224510206698742110, 14.34966873604972548, 27.08442372801901854 ) ) ;
#116117=CARTESIAN_POINT ( 'NONE',  ( -18.62759615963255300, -10.81492255796106328, 49.16775706135234003 ) ) ;
#116119=CARTESIAN_POINT ( 'NONE',  ( -9.564922557960796823, -16.46253265017161027, 112.0822429386476955 ) ) ;
#116120=CARTESIAN_POINT ( 'NONE',  ( 9.564922557961047289, -16.46253265017146816, 60.41775706135233293 ) ) ;
#116122=CARTESIAN_POINT ( 'NONE',  ( -5.719274019375665041, -21.55341960407619695, 19.79275706135235069 ) ) ;
#116123=CARTESIAN_POINT ( 'NONE',  ( -13.89961937509977652, 13.97604488694528158, 55.62390960531434558 ) ) ;
#116125=CARTESIAN_POINT ( 'NONE',  ( 13.97604488694548053, -13.89961937509957401, 20.62609039468567573 ) ) ;
#116126=CARTESIAN_POINT ( 'NONE',  ( 9.474510206698971260, -16.51473224551069308, 47.91557627198102409 ) ) ;
#116127=CARTESIAN_POINT ( 'NONE',  ( 18.67979575497194134, -10.72451020669871369, 105.8344237280190328 ) ) ;
#116128=CARTESIAN_POINT ( 'NONE',  ( -12.14591786802326823, 12.06949235617739902, 88.12609039468570415 ) ) ;
#116129=CARTESIAN_POINT ( 'NONE',  ( -5.153800228976328057, -19.02544592524343514, 102.2905762719810383 ) ) ;
#116130=CARTESIAN_POINT ( 'NONE',  ( -0.05219959533937732626, 21.53943276465977519, 77.50109039468567573 ) ) ;
#116132=CARTESIAN_POINT ( 'NONE',  ( 19.05341960407611168, 5.049401038298154454, 108.9572429386477097 ) ) ;
#116134=CARTESIAN_POINT ( 'NONE',  ( -8.224510206698735004, -14.34966873604973081, 64.58442372801900433 ) ) ;
#116135=CARTESIAN_POINT ( 'NONE',  ( 5.823673210054444382, -21.52544592524334988, 65.20942372801901854 ) ) ;
#116136=CARTESIAN_POINT ( 'NONE',  ( -18.62759615963255300, -10.81492255796106328, 109.1677570613523613 ) ) ;
#116138=CARTESIAN_POINT ( 'NONE',  ( -9.474510206698964154, 16.51473224551069663, 80.41557627198103830 ) ) ;
#116139=CARTESIAN_POINT ( 'NONE',  ( -16.46253265017160317, 9.564922557960807481, 110.8322429386476955 ) ) ;
#116140=ORIENTED_EDGE ( 'NONE', *, *, #26049, .T. ) ;
#116141=DIRECTION ( 'NONE',  ( -1.000000000000000000, -0.000000000000000000, -0.000000000000000000 ) ) ;
#116142=CARTESIAN_POINT ( 'NONE',  ( 9.564922557960805705, 16.46253265017160317, 44.58224293864769550 ) ) ;
#116143=CARTESIAN_POINT ( 'NONE',  ( -5.823673210054116645, -21.52544592524344225, 37.29057627198102409 ) ) ;
#116144=CARTESIAN_POINT ( 'NONE',  ( 4.379528057220092307, 16.55341960407617563, 107.2927570613523471 ) ) ;
#116145=CARTESIAN_POINT ( 'NONE',  ( 16.53943276465976808, -0.05219959533910856209, 83.74890960531435269 ) ) ;
#116146=CARTESIAN_POINT ( 'NONE',  ( 5.049401038298161559, -19.05341960407611168, 77.70724293864765286 ) ) ;
#116147=CARTESIAN_POINT ( 'NONE',  ( 5.719274019375673035, 21.55341960407619339, 107.2927570613523471 ) ) ;
#116148=CARTESIAN_POINT ( 'NONE',  ( 5.049401038298161559, -19.05341960407611168, 37.70724293864768839 ) ) ;
#116149=CARTESIAN_POINT ( 'NONE',  ( 4.483927247898545687, 16.52544592524342804, 94.79057627198105251 ) ) ;
#116150=CARTESIAN_POINT ( 'NONE',  ( 21.53943276465977519, 0.05219959533937863772, 46.25109039468567573 ) ) ;
#116151=CARTESIAN_POINT ( 'NONE',  ( -0.05219959533907301413, -21.53943276465977519, 92.49890960531436690 ) ) ;
#116152=CARTESIAN_POINT ( 'NONE',  ( 13.97604488694548053, -13.89961937509957401, 50.62609039468566152 ) ) ;
#116154=CARTESIAN_POINT ( 'NONE',  ( -16.46253265017160317, 9.564922557960807481, 95.83224293864769550 ) ) ;
#116155=CARTESIAN_POINT ( 'NONE',  ( 16.52544592524342804, -4.483927247898539470, 63.54057627198103830 ) ) ;
#116157=CARTESIAN_POINT ( 'NONE',  ( 4.483927247898545687, 16.52544592524342804, 54.79057627198104541 ) ) ;
#116158=CARTESIAN_POINT ( 'NONE',  ( -14.34966873604960291, -8.224510206698953496, 31.66557627198102054 ) ) ;
#116159=CARTESIAN_POINT ( 'NONE',  ( 19.05341960407617918, -5.049401038297876454, 81.04275706135231871 ) ) ;
#116160=CARTESIAN_POINT ( 'NONE',  ( -18.39635199886970440, 5.499999999999980460, 86.01967076360000419 ) ) ;
#116161=CARTESIAN_POINT ( 'NONE',  ( 21.55341960407610458, 5.719274019375980345, 28.95724293864769905 ) ) ;
#116162=CARTESIAN_POINT ( 'NONE',  ( 14.29746914071049879, -8.314922557960816363, 88.33224293864769550 ) ) ;
#116164=CARTESIAN_POINT ( 'NONE',  ( -16.46253265017160317, 9.564922557960807481, 50.83224293864770260 ) ) ;
#116165=CARTESIAN_POINT ( 'NONE',  ( -5.719274019375978568, 21.55341960407610458, 45.20724293864769550 ) ) ;
#116166=CARTESIAN_POINT ( 'NONE',  ( 5.049401038298161559, -19.05341960407611168, 32.70724293864768129 ) ) ;
#116167=CARTESIAN_POINT ( 'NONE',  ( -4.483927247898782831, 16.52544592524335698, 72.70942372801901854 ) ) ;
#116168=CARTESIAN_POINT ( 'NONE',  ( 13.89961937509977652, -13.97604488694527269, 63.12390960531435979 ) ) ;
#116169=CARTESIAN_POINT ( 'NONE',  ( -9.564922557961040184, 16.46253265017147172, 42.91775706135234003 ) ) ;
#116170=CARTESIAN_POINT ( 'NONE',  ( 21.55341960407619695, -5.719274019375665929, 66.04275706135236135 ) ) ;
#116171=CARTESIAN_POINT ( 'NONE',  ( -10.72451020669898014, 18.67979575497178502, 30.41557627198101699 ) ) ;
#116172=CARTESIAN_POINT ( 'NONE',  ( -4.379528057220328563, 16.55341960407611168, 105.2072429386477097 ) ) ;
#116173=CARTESIAN_POINT ( 'NONE',  ( 19.03943276465977164, 0.05219959533936151252, 91.25109039468566152 ) ) ;
#116176=CARTESIAN_POINT ( 'NONE',  ( 0.05219959533907565091, 21.53943276465977519, 49.99890960531437401 ) ) ;
#116177=CARTESIAN_POINT ( 'NONE',  ( -0.05219959533909027116, -19.03943276465977164, 27.49890960531435624 ) ) ;
#116178=CARTESIAN_POINT ( 'NONE',  ( -10.72451020669870658, -18.67979575497194134, 84.58442372801903275 ) ) ;
#116179=CARTESIAN_POINT ( 'NONE',  ( -4.483927247898539470, -16.52544592524342804, 52.29057627198102409 ) ) ;
#116180=CARTESIAN_POINT ( 'NONE',  ( -16.53943276465976808, -0.05219959533934237506, 68.75109039468568994 ) ) ;
#116181=CARTESIAN_POINT ( 'NONE',  ( -0.05219959533910754901, -16.53943276465976808, 62.49890960531436690 ) ) ;
#116182=CARTESIAN_POINT ( 'NONE',  ( 18.67979575497178502, 10.72451020669898547, 79.16557627198103830 ) ) ;
#116183=CARTESIAN_POINT ( 'NONE',  ( -21.53943276465977519, 0.05219959533907696930, 76.24890960531435269 ) ) ;
#116185=CARTESIAN_POINT ( 'NONE',  ( 21.52544592524344225, -5.823673210054117533, 33.54057627198102409 ) ) ;
#116187=CARTESIAN_POINT ( 'NONE',  ( 16.52544592524335698, 4.483927247898782831, 51.45942372801901854 ) ) ;
#116188=CARTESIAN_POINT ( 'NONE',  ( 16.52544592524342804, -4.483927247898539470, 83.54057627198102409 ) ) ;
#116189=CARTESIAN_POINT ( 'NONE',  ( 19.03943276465977164, -0.05219959533909143690, 63.74890960531435979 ) ) ;
#116190=CARTESIAN_POINT ( 'NONE',  ( 9.474510206698971260, -16.51473224551069308, 32.91557627198102409 ) ) ;
#116193=CARTESIAN_POINT ( 'NONE',  ( 16.53943276465976808, 0.05219959533934440121, 81.25109039468568994 ) ) ;
#116194=CARTESIAN_POINT ( 'NONE',  ( 10.72451020669871369, 18.67979575497193778, 22.08442372801901143 ) ) ;
#116195=CARTESIAN_POINT ( 'NONE',  ( 5.049401038298161559, -19.05341960407611168, 67.70724293864769550 ) ) ;
#116196=CARTESIAN_POINT ( 'NONE',  ( 10.81492255796106328, -18.62759615963255655, 50.41775706135235424 ) ) ;
#116197=CARTESIAN_POINT ( 'NONE',  ( 16.51473224551069308, 9.474510206698969483, 114.1655762719810241 ) ) ;
#116200=CARTESIAN_POINT ( 'NONE',  ( 10.72451020669871369, 18.67979575497193778, 47.08442372801901854 ) ) ;
#116201=CARTESIAN_POINT ( 'NONE',  ( 9.564922557960805705, 16.46253265017160317, 114.5822429386476955 ) ) ;
#116202=CARTESIAN_POINT ( 'NONE',  ( -5.153800228976328057, -19.02544592524343514, 107.2905762719810383 ) ) ;
#116203=CARTESIAN_POINT ( 'NONE',  ( -19.05341960407617563, 5.049401038297882671, 53.54275706135231871 ) ) ;
#116204=CARTESIAN_POINT ( 'NONE',  ( 0.05219959533907565091, 21.53943276465977519, 109.9989096053143527 ) ) ;
#116205=CARTESIAN_POINT ( 'NONE',  ( -9.474510206698720793, -16.51473224551083518, 49.58442372801899722 ) ) ;
#116206=CARTESIAN_POINT ( 'NONE',  ( -9.564922557961040184, 16.46253265017147172, 42.91775706135234003 ) ) ;
#116207=CARTESIAN_POINT ( 'NONE',  ( 14.34966873604972726, -8.224510206698740333, 105.8344237280190328 ) ) ;
#116209=CARTESIAN_POINT ( 'NONE',  ( -16.51473224551069308, -9.474510206698971260, 91.66557627198103830 ) ) ;
#116210=CARTESIAN_POINT ( 'NONE',  ( -21.53943276465977519, -0.05219959533937600094, 93.75109039468567573 ) ) ;
#116211=CARTESIAN_POINT ( 'NONE',  ( -18.67979575497193778, 10.72451020669871902, 88.33442372801901854 ) ) ;
#116213=CARTESIAN_POINT ( 'NONE',  ( 9.564922557960805705, 16.46253265017160317, 99.58224293864770971 ) ) ;
#116214=CARTESIAN_POINT ( 'NONE',  ( 5.719274019375673035, 21.55341960407619339, 72.29275706135236135 ) ) ;
#116215=CARTESIAN_POINT ( 'NONE',  ( -8.224510206698735004, -14.34966873604973081, 24.58442372801901499 ) ) ;
#116216=CARTESIAN_POINT ( 'NONE',  ( 19.05341960407611168, 5.049401038298154454, 78.95724293864769550 ) ) ;
#116217=CARTESIAN_POINT ( 'NONE',  ( 21.55341960407610458, 5.719274019375980345, 28.95724293864769905 ) ) ;
#116218=CARTESIAN_POINT ( 'NONE',  ( -9.564922557960796823, -16.46253265017161027, 92.08224293864769550 ) ) ;
#116220=CARTESIAN_POINT ( 'NONE',  ( 16.46253265017160672, -9.564922557960803928, 73.33224293864769550 ) ) ;
#116221=CARTESIAN_POINT ( 'NONE',  ( -19.03943276465977164, 0.05219959533909376836, 66.24890960531436690 ) ) ;
#116222=CARTESIAN_POINT ( 'NONE',  ( -10.72451020669898014, 18.67979575497178502, 115.4155762719810241 ) ) ;
#116223=CARTESIAN_POINT ( 'NONE',  ( 16.52544592524335698, 4.483927247898782831, 96.45942372801901854 ) ) ;
#116224=CARTESIAN_POINT ( 'NONE',  ( -16.29526858892910823, 7.335722546919979159, 99.20329402199730850 ) ) ;
#116225=CARTESIAN_POINT ( 'NONE',  ( -0.05219959533936034679, 19.03943276465977164, 52.50109039468566863 ) ) ;
#116226=CARTESIAN_POINT ( 'NONE',  ( 19.03943276465977164, -0.05219959533909143690, 88.74890960531436690 ) ) ;
#116227=CARTESIAN_POINT ( 'NONE',  ( 16.53943276465976808, -0.05219959533910856209, 78.74890960531436690 ) ) ;
#116228=CARTESIAN_POINT ( 'NONE',  ( -10.81492255796078084, -18.62759615963271287, 32.08224293864769550 ) ) ;
#116229=CARTESIAN_POINT ( 'NONE',  ( 5.823673210054125526, 21.52544592524343514, 29.79057627198102409 ) ) ;
#116230=CARTESIAN_POINT ( 'NONE',  ( -0.05219959533910754901, -16.53943276465976808, 92.49890960531436690 ) ) ;
#116231=CARTESIAN_POINT ( 'NONE',  ( -16.21995358207306381, 7.366697692864088154, 54.93551001512158649 ) ) ;
#116232=CARTESIAN_POINT ( 'NONE',  ( 5.153800228976615827, -19.02544592524334988, 40.20942372801898301 ) ) ;
#116233=CARTESIAN_POINT ( 'NONE',  ( 16.55341960407618274, -4.379528057220086978, 106.0427570613523471 ) ) ;
#116234=CARTESIAN_POINT ( 'NONE',  ( -16.46253265017160317, 9.564922557960807481, 85.83224293864769550 ) ) ;
#116235=CARTESIAN_POINT ( 'NONE',  ( -10.81492255796105439, 18.62759615963255655, 72.91775706135234714 ) ) ;
#116236=CARTESIAN_POINT ( 'NONE',  ( 18.62759615963271287, -10.81492255796078972, 58.33224293864768839 ) ) ;
#116237=CARTESIAN_POINT ( 'NONE',  ( -15.80617190586768217, 15.72974639402176855, 28.12609039468568284 ) ) ;
#116238=CARTESIAN_POINT ( 'NONE',  ( 15.72974639402199770, -15.80617190586745480, 83.12390960531436690 ) ) ;
#116239=CARTESIAN_POINT ( 'NONE',  ( -16.52544592524342804, 4.483927247898546575, 106.0405762719810525 ) ) ;
#116240=CARTESIAN_POINT ( 'NONE',  ( 0.05219959533936267826, -19.03943276465977164, 70.00109039468566152 ) ) ;
#116241=CARTESIAN_POINT ( 'NONE',  ( -5.049401038298153566, 19.05341960407611168, 45.20724293864769550 ) ) ;
#116242=CARTESIAN_POINT ( 'NONE',  ( 5.049401038298161559, -19.05341960407611168, 97.70724293864766707 ) ) ;
#116243=CARTESIAN_POINT ( 'NONE',  ( -0.05219959533909027116, -19.03943276465977164, 92.49890960531436690 ) ) ;
#116244=CARTESIAN_POINT ( 'NONE',  ( -13.97604488694527625, -13.89961937509977652, 21.87390960531435979 ) ) ;
#116245=CARTESIAN_POINT ( 'NONE',  ( 8.314922557960818139, 14.29746914071049879, 39.58224293864769550 ) ) ;
#116246=CARTESIAN_POINT ( 'NONE',  ( 14.29746914071037800, 8.314922557961029526, 41.66775706135235424 ) ) ;
#116247=CARTESIAN_POINT ( 'NONE',  ( -18.67979575497193778, 10.72451020669871902, 108.3344237280190185 ) ) ;
#116248=CARTESIAN_POINT ( 'NONE',  ( 19.03943276465977164, -0.05219959533909143690, 113.7489096053143669 ) ) ;
#116249=CARTESIAN_POINT ( 'NONE',  ( -4.379528057220086978, -16.55341960407618274, 109.7927570613523613 ) ) ;
#116250=CARTESIAN_POINT ( 'NONE',  ( -15.72974639402176322, -15.80617190586768395, 29.37609039468568284 ) ) ;
#116251=CARTESIAN_POINT ( 'NONE',  ( 19.05341960407611168, 5.049401038298154454, 98.95724293864766707 ) ) ;
#116253=CARTESIAN_POINT ( 'NONE',  ( 12.06949235617739724, 12.14591786802326823, 101.8760903946857042 ) ) ;
#116254=CARTESIAN_POINT ( 'NONE',  ( 16.53943276465976808, 0.05219959533934440121, 91.25109039468568994 ) ) ;
#116255=CARTESIAN_POINT ( 'NONE',  ( -14.34966873604972548, 8.224510206698743886, 28.33442372801902209 ) ) ;
#116256=CARTESIAN_POINT ( 'NONE',  ( 19.05341960407611168, 5.049401038298154454, 48.95724293864768129 ) ) ;
#116257=CARTESIAN_POINT ( 'NONE',  ( -16.53943276465976808, 0.05219959533911058130, 111.2489096053143669 ) ) ;
#116258=CARTESIAN_POINT ( 'NONE',  ( -21.52544592524334988, -5.823673210054445271, 18.95942372801901143 ) ) ;
#116259=CARTESIAN_POINT ( 'NONE',  ( 19.03943276465977164, -0.05219959533909143690, 38.74890960531436690 ) ) ;
#116260=CARTESIAN_POINT ( 'NONE',  ( 19.03943276465977164, -0.05219959533909143690, 98.74890960531436690 ) ) ;
#116261=CARTESIAN_POINT ( 'NONE',  ( -16.46253265017160317, 9.564922557960807481, 30.83224293864769550 ) ) ;
#116262=CARTESIAN_POINT ( 'NONE',  ( -13.89961937509977652, 13.97604488694528158, 100.6239096053143669 ) ) ;
#116263=CARTESIAN_POINT ( 'NONE',  ( 17.49999999999999645, 5.500000000000010658, 88.78230962303567253 ) ) ;
#116265=CARTESIAN_POINT ( 'NONE',  ( 19.05341960407611168, 5.049401038298154454, 103.9572429386476671 ) ) ;
#116266=CARTESIAN_POINT ( 'NONE',  ( 10.81492255796106328, -18.62759615963255655, 50.41775706135235424 ) ) ;
#116267=CARTESIAN_POINT ( 'NONE',  ( -16.55341960407611168, -4.379528057220339221, 86.45724293864770971 ) ) ;
#116268=CARTESIAN_POINT ( 'NONE',  ( 5.049401038298161559, -19.05341960407611168, 97.70724293864766707 ) ) ;
#116270=CARTESIAN_POINT ( 'NONE',  ( 16.55341960407618274, -4.379528057220086978, 71.04275706135234714 ) ) ;
#116271=CARTESIAN_POINT ( 'NONE',  ( -18.62759615963255300, -10.81492255796106328, 79.16775706135234714 ) ) ;
#116272=CARTESIAN_POINT ( 'NONE',  ( -16.52544592524335698, -4.483927247898792601, 43.95942372801902565 ) ) ;
#116273=CARTESIAN_POINT ( 'NONE',  ( -13.97604488694527625, -13.89961937509977652, 86.87390960531436690 ) ) ;
#116274=CARTESIAN_POINT ( 'NONE',  ( -16.51473224551082808, 9.474510206698731452, 108.3344237280190043 ) ) ;
#116275=CARTESIAN_POINT ( 'NONE',  ( -8.314922557961024197, 14.29746914071037800, 87.91775706135234714 ) ) ;
#116276=CARTESIAN_POINT ( 'NONE',  ( -16.46253265017146816, -9.564922557961047289, 89.16775706135234714 ) ) ;
#116277=CARTESIAN_POINT ( 'NONE',  ( -0.05219959533909027116, -19.03943276465977164, 57.49890960531435979 ) ) ;
#116278=CARTESIAN_POINT ( 'NONE',  ( -15.80617190586745835, -15.72974639402198527, 96.87390960531436690 ) ) ;
#116279=CARTESIAN_POINT ( 'NONE',  ( -16.52544592524342804, 4.483927247898546575, 91.04057627198103830 ) ) ;
#116280=CARTESIAN_POINT ( 'NONE',  ( 19.05341960407617918, -5.049401038297876454, 91.04275706135234714 ) ) ;
#116281=CARTESIAN_POINT ( 'NONE',  ( -0.05219959533934338120, 16.53943276465976808, 57.50109039468568994 ) ) ;
#116282=CARTESIAN_POINT ( 'NONE',  ( 17.31728774477275934, -6.344390552232301417, 63.31906651689320142 ) ) ;
#116283=CARTESIAN_POINT ( 'NONE',  ( -9.564922557961040184, 16.46253265017147172, 52.91775706135233293 ) ) ;
#116284=CARTESIAN_POINT ( 'NONE',  ( -8.224510206698948167, 14.34966873604960824, 30.41557627198101699 ) ) ;
#116285=CARTESIAN_POINT ( 'NONE',  ( 16.55341960407611168, 4.379528057220329451, 73.95724293864769550 ) ) ;
#116286=CARTESIAN_POINT ( 'NONE',  ( 15.72974639402176855, 15.80617190586768217, 111.8760903946856615 ) ) ;
#116287=CARTESIAN_POINT ( 'NONE',  ( -17.50000000000000711, 5.622605283950841581, 38.68792689403890961 ) ) ;
#116288=CARTESIAN_POINT ( 'NONE',  ( 0.05219959533907565091, 21.53943276465977519, 114.9989096053143669 ) ) ;
#116290=CARTESIAN_POINT ( 'NONE',  ( -16.46253265017160317, 9.564922557960807481, 75.83224293864769550 ) ) ;
#116291=CARTESIAN_POINT ( 'NONE',  ( -0.05219959533937732626, 21.53943276465977519, 92.50109039468567573 ) ) ;
#116292=CARTESIAN_POINT ( 'NONE',  ( -13.89961937509977652, 13.97604488694528158, 70.62390960531432427 ) ) ;
#116293=CARTESIAN_POINT ( 'NONE',  ( 5.719274019375991003, -21.55341960407610458, 47.70724293864770260 ) ) ;
#116294=CARTESIAN_POINT ( 'NONE',  ( 0.05219959533910956823, 16.53943276465976808, 84.99890960531436690 ) ) ;
#116295=CARTESIAN_POINT ( 'NONE',  ( 16.46253265017160672, -9.564922557960803928, 53.33224293864768839 ) ) ;
#116296=CARTESIAN_POINT ( 'NONE',  ( -19.03943276465977164, 0.05219959533909376836, 21.24890960531436335 ) ) ;
#116297=CARTESIAN_POINT ( 'NONE',  ( -18.67979575497193778, 10.72451020669871902, 23.33442372801901499 ) ) ;
#116299=CARTESIAN_POINT ( 'NONE',  ( 15.80617190586769283, -15.72974639402175789, 55.62609039468568284 ) ) ;
#116300=CARTESIAN_POINT ( 'NONE',  ( 13.97604488694527802, 13.89961937509977652, 44.37390960531435269 ) ) ;
#116301=CARTESIAN_POINT ( 'NONE',  ( 12.14591786802327356, -12.06949235617739191, 70.62609039468567573 ) ) ;
#116302=CARTESIAN_POINT ( 'NONE',  ( 15.80617190586746368, 15.72974639402197994, 114.3739096053143527 ) ) ;
#116303=CARTESIAN_POINT ( 'NONE',  ( 18.67979575497178502, 10.72451020669898547, 114.1655762719810383 ) ) ;
#116304=CARTESIAN_POINT ( 'NONE',  ( -16.46253265017146816, -9.564922557961047289, 34.16775706135233293 ) ) ;
#116305=CARTESIAN_POINT ( 'NONE',  ( 9.564922557960805705, 16.46253265017160317, 69.58224293864770971 ) ) ;
#116307=CARTESIAN_POINT ( 'NONE',  ( 5.823673210054444382, -21.52544592524334988, 70.20942372801904696 ) ) ;
#116308=CARTESIAN_POINT ( 'NONE',  ( -10.72451020669898014, 18.67979575497178502, 50.41557627198103120 ) ) ;
#116309=CARTESIAN_POINT ( 'NONE',  ( -0.05219959533910754901, -16.53943276465976808, 32.49890960531435979 ) ) ;
#116310=CARTESIAN_POINT ( 'NONE',  ( 18.62759615963255655, 10.81492255796105972, 91.66775706135234714 ) ) ;
#116311=CARTESIAN_POINT ( 'NONE',  ( -18.62759615963255300, -10.81492255796106328, 109.1677570613523613 ) ) ;
#116312=CARTESIAN_POINT ( 'NONE',  ( -16.52544592524342804, 4.483927247898546575, 61.04057627198103120 ) ) ;
#116313=CARTESIAN_POINT ( 'NONE',  ( -8.224510206698948167, 14.34966873604960824, 105.4155762719810383 ) ) ;
#116314=CARTESIAN_POINT ( 'NONE',  ( 13.97604488694548053, -13.89961937509957401, 60.62609039468564731 ) ) ;
#116315=CARTESIAN_POINT ( 'NONE',  ( -4.483927247898782831, 16.52544592524335698, 112.7094237280190328 ) ) ;
#116316=CARTESIAN_POINT ( 'NONE',  ( -18.67979575497193778, 10.72451020669871902, 68.33442372801900433 ) ) ;
#116317=CARTESIAN_POINT ( 'NONE',  ( -16.46253265017160317, 9.564922557960807481, 70.83224293864770971 ) ) ;
#116318=CARTESIAN_POINT ( 'NONE',  ( 16.51473224551083163, -9.474510206698727899, 30.83442372801900433 ) ) ;
#116319=CARTESIAN_POINT ( 'NONE',  ( 21.52544592524344225, -5.823673210054117533, 48.54057627198103120 ) ) ;
#116320=CARTESIAN_POINT ( 'NONE',  ( 21.53943276465977519, 0.05219959533937863772, 51.25109039468568994 ) ) ;
#116321=CARTESIAN_POINT ( 'NONE',  ( 5.719274019375991003, -21.55341960407610458, 102.7072429386476955 ) ) ;
#116322=CARTESIAN_POINT ( 'NONE',  ( -19.05341960407617563, 5.049401038297882671, 93.54275706135234714 ) ) ;
#116323=CARTESIAN_POINT ( 'NONE',  ( 8.314922557961029526, -14.29746914071037800, 50.41775706135235424 ) ) ;
#116325=CARTESIAN_POINT ( 'NONE',  ( -5.719274019375978568, 21.55341960407610458, 100.2072429386476955 ) ) ;
#116326=CARTESIAN_POINT ( 'NONE',  ( -4.379528057220328563, 16.55341960407611168, 85.20724293864770971 ) ) ;
#116328=CARTESIAN_POINT ( 'NONE',  ( 5.049401038297881783, 19.05341960407617563, 112.2927570613523471 ) ) ;
#116329=CARTESIAN_POINT ( 'NONE',  ( -10.72451020669898014, 18.67979575497178502, 45.41557627198103830 ) ) ;
#116330=CARTESIAN_POINT ( 'NONE',  ( 16.55341960407618274, -4.379528057220086978, 86.04275706135236135 ) ) ;
#116332=CARTESIAN_POINT ( 'NONE',  ( -8.224510206698735004, -14.34966873604973081, 54.58442372801901143 ) ) ;
#116333=CARTESIAN_POINT ( 'NONE',  ( 15.72974639402176855, 15.80617190586768217, 21.87609039468567573 ) ) ;
#116334=CARTESIAN_POINT ( 'NONE',  ( 18.67979575497178502, 10.72451020669898547, 39.16557627198102409 ) ) ;
#116335=CARTESIAN_POINT ( 'NONE',  ( 0.05219959533934541429, -16.53943276465976808, 80.00109039468568994 ) ) ;
#116336=CARTESIAN_POINT ( 'NONE',  ( 9.564922557960805705, 16.46253265017160317, 104.5822429386476955 ) ) ;
#116337=CARTESIAN_POINT ( 'NONE',  ( -18.67979575497193778, 10.72451020669871902, 68.33442372801900433 ) ) ;
#116338=CARTESIAN_POINT ( 'NONE',  ( -15.72974639402197994, 15.80617190586746368, 35.62390960531437401 ) ) ;
#116339=CARTESIAN_POINT ( 'NONE',  ( 5.823673210054125526, 21.52544592524343514, 24.79057627198103120 ) ) ;
#116341=CARTESIAN_POINT ( 'NONE',  ( 19.03943276465977164, 0.05219959533936151252, 51.25109039468567573 ) ) ;
#116342=CARTESIAN_POINT ( 'NONE',  ( -4.379528057220086978, -16.55341960407618274, 69.79275706135234714 ) ) ;
#116343=CARTESIAN_POINT ( 'NONE',  ( -0.05219959533907301413, -21.53943276465977519, 27.49890960531435269 ) ) ;
#116345=CARTESIAN_POINT ( 'NONE',  ( 5.153800228976335163, 19.02544592524342804, 84.79057627198099567 ) ) ;
#116346=CARTESIAN_POINT ( 'NONE',  ( -16.52544592524335698, -4.483927247898792601, 108.9594237280190185 ) ) ;
#116348=CARTESIAN_POINT ( 'NONE',  ( -14.34966873604960291, -8.224510206698953496, 111.6655762719810525 ) ) ;
#116349=CARTESIAN_POINT ( 'NONE',  ( -21.55341960407610458, -5.719274019375992779, 46.45724293864769550 ) ) ;
#116350=CARTESIAN_POINT ( 'NONE',  ( 9.474510206698971260, -16.51473224551069308, 42.91557627198103120 ) ) ;
#116351=CARTESIAN_POINT ( 'NONE',  ( -0.05219959533934338120, 16.53943276465976808, 82.50109039468568994 ) ) ;
#116352=CARTESIAN_POINT ( 'NONE',  ( -18.67979575497193778, 10.72451020669871902, 38.33442372801900433 ) ) ;
#116353=CARTESIAN_POINT ( 'NONE',  ( 9.474510206698729675, 16.51473224551082808, 92.08442372801900433 ) ) ;
#116354=CARTESIAN_POINT ( 'NONE',  ( 8.224510206698953496, -14.34966873604960469, 92.91557627198103830 ) ) ;
#116355=CARTESIAN_POINT ( 'NONE',  ( 19.02544592524343514, -5.153800228976328945, 58.54057627198102409 ) ) ;
#116356=CARTESIAN_POINT ( 'NONE',  ( -5.153800228976328057, -19.02544592524343514, 32.29057627198102409 ) ) ;
#116357=CARTESIAN_POINT ( 'NONE',  ( -21.52544592524334988, -5.823673210054445271, 98.95942372801903275 ) ) ;
#116358=CARTESIAN_POINT ( 'NONE',  ( -19.02544592524342804, 5.153800228976336051, 81.04057627198103830 ) ) ;
#116359=CARTESIAN_POINT ( 'NONE',  ( 8.224510206698742110, 14.34966873604972548, 67.08442372801901854 ) ) ;
#116360=CARTESIAN_POINT ( 'NONE',  ( 21.55341960407619695, -5.719274019375665929, 91.04275706135236135 ) ) ;
#116361=CARTESIAN_POINT ( 'NONE',  ( -21.53943276465977519, 0.05219959533907696930, 51.24890960531436690 ) ) ;
#116362=CARTESIAN_POINT ( 'NONE',  ( -16.55341960407617563, 4.379528057220093196, 73.54275706135234714 ) ) ;
#116363=CARTESIAN_POINT ( 'NONE',  ( -9.564922557961040184, 16.46253265017147172, 57.91775706135233293 ) ) ;
#116364=CARTESIAN_POINT ( 'NONE',  ( -19.02544592524334988, -5.153800228976617603, 68.95942372801896170 ) ) ;
#116366=CARTESIAN_POINT ( 'NONE',  ( -0.05219959533937732626, 21.53943276465977519, 62.50109039468568284 ) ) ;
#116367=CARTESIAN_POINT ( 'NONE',  ( 0.05219959533909260263, 19.03943276465977164, 69.99890960531435269 ) ) ;
#116368=CARTESIAN_POINT ( 'NONE',  ( 5.049401038298161559, -19.05341960407611168, 22.70724293864769194 ) ) ;
#116369=CARTESIAN_POINT ( 'NONE',  ( 9.474510206698729675, 16.51473224551082808, 57.08442372801900433 ) ) ;
#116371=CARTESIAN_POINT ( 'NONE',  ( 5.153800228976335163, 19.02544592524342804, 99.79057627198102409 ) ) ;
#116372=CARTESIAN_POINT ( 'NONE',  ( 14.34966873604960469, 8.224510206698951720, 54.16557627198103120 ) ) ;
#116373=CARTESIAN_POINT ( 'NONE',  ( 21.55341960407610458, 5.719274019375980345, 43.95724293864769550 ) ) ;
#116375=CARTESIAN_POINT ( 'NONE',  ( -5.823673210054431948, 21.52544592524334988, 112.7094237280190328 ) ) ;
#116376=CARTESIAN_POINT ( 'NONE',  ( 19.02544592524343514, -5.153800228976328945, 53.54057627198102409 ) ) ;
#116377=CARTESIAN_POINT ( 'NONE',  ( -13.89961937509977652, 13.97604488694528158, 25.62390960531434558 ) ) ;
#116380=CARTESIAN_POINT ( 'NONE',  ( -12.06949235617739369, -12.14591786802326823, 59.37609039468568284 ) ) ;
#116381=CARTESIAN_POINT ( 'NONE',  ( -10.81492255796078084, -18.62759615963271287, 82.08224293864768129 ) ) ;
#116382=CARTESIAN_POINT ( 'NONE',  ( -16.52544592524342804, 4.483927247898546575, 56.04057627198102409 ) ) ;
#116383=CARTESIAN_POINT ( 'NONE',  ( 16.51473224551069308, 9.474510206698969483, 44.16557627198103120 ) ) ;
#116385=CARTESIAN_POINT ( 'NONE',  ( 15.80617190586769283, -15.72974639402175789, 40.62609039468567573 ) ) ;
#116386=CARTESIAN_POINT ( 'NONE',  ( 5.049401038297881783, 19.05341960407617563, 47.29275706135231161 ) ) ;
#116387=CARTESIAN_POINT ( 'NONE',  ( -19.02544592524342804, 5.153800228976336051, 31.04057627198102409 ) ) ;
#116388=CARTESIAN_POINT ( 'NONE',  ( 10.81492255796106328, -18.62759615963255655, 85.41775706135236135 ) ) ;
#116389=CARTESIAN_POINT ( 'NONE',  ( 17.05587630539788080, 6.762274262135702152, 96.75819690962687503 ) ) ;
#116390=CARTESIAN_POINT ( 'NONE',  ( 16.55341960407611168, 4.379528057220329451, 43.95724293864769550 ) ) ;
#116392=CARTESIAN_POINT ( 'NONE',  ( 21.52544592524344225, -5.823673210054117533, 38.54057627198103120 ) ) ;
#116393=ORIENTED_EDGE ( 'NONE', *, *, #199792, .T. ) ;
#116395=CARTESIAN_POINT ( 'NONE',  ( 9.474510206698971260, -16.51473224551069308, 92.91557627198103830 ) ) ;
#116396=CARTESIAN_POINT ( 'NONE',  ( -4.483927247898539470, -16.52544592524342804, 82.29057627198103830 ) ) ;
#116397=CARTESIAN_POINT ( 'NONE',  ( -8.224510206698735004, -14.34966873604973081, 24.58442372801901499 ) ) ;
#116398=CARTESIAN_POINT ( 'NONE',  ( 8.224510206698742110, 14.34966873604972548, 107.0844237280190043 ) ) ;
#116399=ORIENTED_EDGE ( 'NONE', *, *, #141236, .T. ) ;
#116400=CARTESIAN_POINT ( 'NONE',  ( -0.05219959533909027116, -19.03943276465977164, 37.49890960531436690 ) ) ;
#116401=CARTESIAN_POINT ( 'NONE',  ( -16.46253265017160317, 9.564922557960807481, 85.83224293864769550 ) ) ;
#116402=CARTESIAN_POINT ( 'NONE',  ( 5.719274019375991003, -21.55341960407610458, 87.70724293864769550 ) ) ;
#116403=CARTESIAN_POINT ( 'NONE',  ( 8.224510206698953496, -14.34966873604960469, 27.91557627198103830 ) ) ;
#116404=CARTESIAN_POINT ( 'NONE',  ( -5.153800228976328057, -19.02544592524343514, 102.2905762719810383 ) ) ;
#116405=CARTESIAN_POINT ( 'NONE',  ( -5.049401038297874678, -19.05341960407617918, 79.79275706135233293 ) ) ;
#116406=CARTESIAN_POINT ( 'NONE',  ( -18.67979575497193778, 10.72451020669871902, 108.3344237280190185 ) ) ;
#116407=CARTESIAN_POINT ( 'NONE',  ( -18.62759615963270932, 10.81492255796079327, 90.83224293864769550 ) ) ;
#116408=CARTESIAN_POINT ( 'NONE',  ( -15.80617190586745835, -15.72974639402198527, 31.87390960531435979 ) ) ;
#116409=CARTESIAN_POINT ( 'NONE',  ( -19.03943276465977164, 0.05219959533909376836, 66.24890960531436690 ) ) ;
#116410=CARTESIAN_POINT ( 'NONE',  ( 14.34966873604960469, 8.224510206698951720, 24.16557627198103120 ) ) ;
#116411=CARTESIAN_POINT ( 'NONE',  ( -5.153800228976328057, -19.02544592524343514, 82.29057627198103830 ) ) ;
#116414=CARTESIAN_POINT ( 'NONE',  ( 5.049401038297881783, 19.05341960407617563, 22.29275706135233648 ) ) ;
#116415=CARTESIAN_POINT ( 'NONE',  ( -8.224510206698948167, 14.34966873604960824, 90.41557627198103830 ) ) ;
#116416=( BOUNDED_SURFACE ( )  B_SPLINE_SURFACE ( 3, 2, ( 
 ( #112709, #173409, #22710, #65215, #83361, #84357, #129850, #146035, #144042, #7518, #111723, #5524, #34880, #174401, #96534, #158224, #19714, #52036, #143040, #159204, #190562, #102546, #85359, #134894, #192561, #178398, #42873, #164229, #163219, #195574, #11557, #24721, #118721, #89363, #133883, #73223, #23712, #41882, #147052, #40872, #87372, #9546, #149057, #10545, #57047, #86370, #130871, #8535, #181395, #132875, #25726, #193566, #196570, #72209, #54044, #180410, #148055, #115718, #119711, #71212, #58041, #12543, #103549, #88358, #194564, #165224, #70214, #131881, #26719, #150051, #104538, #56034, #117712, #55038, #166219, #27720, #162213, #151052, #116708, #177406, #38877, #100534, #179408, #39862, #101528, #92324, #29681, #154009, #184357, #120683, #198537, #74208, #32657, #182382, #16496, #122669, #121675, #43860, #45838, #170173, #62979, #13515, #107489, #15505, #109487, #169167, #312, #199527, #105525, #78145, #60995, #183370, #137846, #31666, #46834, #30671, #60008, #77162, #124659, #91313, #138832, #171170, #186355, #61980, #155000, #94311, #155989, #185343, #47835, #135877, #93316, #139813, #197548, #123646, #59016, #108494, #1301, #168185, #167211, #28708, #90344, #152029, #75180, #136852, #14504, #44852, #106508, #153005, #76166, #102054, #21214, #192061, #70724, #125655, #39379, #178913, #17486, #161726, #63985, #8035, #117219, #191067, #115221, #132391, #23221, #162724, #101038, #100040, #84864, #53543, #187352, #24229, #79143, #48822, #85880, #146542, #69716, #131383, #147568, #110475, #40380, #172157, #160724, #194084, #9053, #6034, #140814, #193072, #177911, #55546, #7025, #2304, #37377, #130364, #33643, #176913, #98022, #22216, #159717, #82871, #144549, #67713, #38384, #83865, #114201, #54547, #116220, #129371, #52540, #175905, #99034, #145547, #68707, #136375, #88874, #13045, #89873, #167714, #104050, #57558, #14017, #122186, #182888, #43373, #121195, #181895, #41388, #71715, #164735, #73728, #150567, #134401, #165730, #26230, #133383, #197072, #44371, #105045, #25239, #179921, #198052, #196088, #42387, #12066, #87869, #163739, #106028, #166729, #180912, #135401, #119228, #75683, #86880, #103053, #28233, #27226, #58539, #120205, #59518, #183878, #29211, #10055, #72728, #195074, #151555, #90845, #74712, #152530, #137362, #199041, #60511, #45363, #148565, #56553, #118230, #149557, #11053, #125185, #184865, #15021, #108005, #17011, #93836, #77676, #109012, #169691, #76682, #140338, #126170, #186881, #168688, #123177, #141338, #139345, #185871, #32180, #31185, #107015, #49333, #48351, #124169, #155516, #824, #171686, #187865, #65485, #142327, #18013, #95826, #30189, #110995, #64503, #91831, #94834, #3807, #33175, #110005, #62498, #2825, #170691, #61508, #138358, #78663, #172680, #47357, #79667, #200039, #153524, #19005, #188854, #92837, #1828, #157511, #46348, #34165, #127147, #154522, #156512, #16019, #80651, #63510, #20973, #145311, #162482, #53305, #192834, #131146, #130128, #114984, #83634, #158494, #69480, #111995, #19981, #54315, #191825, #176677, #161493, #115987, #143307, #147327, #4793, #190832, #23984, #39144, #36138, #8814, #99807, #7797, #177676, #37138, #70484, #67475, #160492, #132150, #6794, #128145, #52308, #100799, #82630, #50338, #189845, #85640, #113965, #21982, #112980, #173685, #68473, #35152, #38153, #144312, #96808, #81624, #129134, #66483, #51318, #22981, #174673, #175664, #84630, #97790, #159479, #146308, #5802, #98798, #134161, #72488, #133146, #89635, #58307, #24998, #135167, #179682, #120955, #105797, #178671, #87638, #194837, #10818, #11829, #149324, #73494, #103817, #40134, #117992, #193843, #152302, #101812, #136144, #42157, #41154, #163500, #165497, #151323, #182654, #56310, #26993, #196840, #28978, #88638, #119975, #118998, #86642, #197820, #180681, #102817, #57322, #12812, #166498, #150334, #164502, #181661, #44138, #195849, #43140, #90620, #167483 ),
 ( #104809, #13786, #27996, #74479, #55307, #59286, #75453, #148325, #25995, #116979, #9820, #71481, #79426, #108771, #91595, #141097, #198814, #184628, #49099, #170449, #169449, #1585, #17770, #30951, #124940, #95583, #140093, #2584, #29957, #48108, #153285, #47112, #93594, #15778, #155280, #16769, #63260, #110756, #31940, #92598, #186637, #64264, #154288, #109764, #157268, #171448, #125930, #14786, #32935, #76446, #78417, #94590, #77437, #156269, #187629, #172438, #139109, #137127, #138123, #33926, #583, #18764, #199804, #60279, #121952, #183645, #45127, #62254, #106785, #168460, #123923, #61271, #122941, #46110, #107764, #185622, #6550, #19745, #81386, #68229, #129882, #114739, #20730, #159235, #143071, #176433, #145069, #111754, #21740, #66243, #7550, #192593, #65247, #174432, #4550, #97548, #98556, #35902, #160250, #190593, #126907, #127903, #80411, #38908, #188613, #22741, #128893, #189605, #50094, #52069, #37907, #69237, #51078, #113726, #83392, #115750, #175422, #191581, #5556, #173442, #84389, #67235, #112739, #144075, #99566, #53060, #36891, #82387, #161247, #130903, #146066, #54076, #177438, #100565, #34911, #162245, #142083, #3569, #96567, #158255, #9580, #27753, #193599, #196603, #89396, #42905, #74241, #118756, #182414, #150085, #180445, #23745, #164265, #12575, #116741, #163255, #88391, #132910, #55071, #166253, #195609, #178431, #151084, #85395, #71246, #135910, #43894, #104570, #103583, #181427, #41917, #101564, #25760, #39896, #147088, #105557, #26752, #197581, #24757, #134926, #86404, #133919, #165258, #102581, #11589, #73256, #58074, #56068, #8572, #148089, #59048, #87406, #57082, #194597, #120714, #119744, #70247, #131915, #117748, #179442, #40908, #149091, #10581, #72242, #62012, #124693, #184389, #93348, #106541, #168218, #155034, #16529, #1334, #107523, #45870, #29715, #63014, #31699, #198571, #108527, #153038, #94343, #79177, #152063, #61028, #91347, #169199, #185375, #122700, #46866, #77195, #13548, #14538, #167243, #125687, #75214, #109520, #15537, #76199, #136885, #138864, #186390, #156022, #137878, #344, #170206, #2337, #123677, #78176, #92356, #60041, #171202, #154042, #199559, #30706, #47867, #139845, #32692, #17519, #140848, #64018, #187385, #48854, #28741, #90378, #121709, #183402, #44885, #143828, #96326, #35658, #158013, #114481, #80167, #83150, #176184, #129640, #161003, #5308, #68991, #36642, #66992, #110509, #50839, #99319, #3330, #49842, #175176, #19504, #141839, #52814, #82134, #65993, #51822, #145823, #22497, #65003, #113482, #142830, #128651, #81149, #97306, #4310, #37654, #126661, #144824, #84144, #191336, #7306, #190346, #130655, #98299, #160001, #172190, #112496, #192349, #188365, #111506, #21489, #127662, #173192, #33675, #6308, #34668, #95337, #157022, #189362, #18520, #67986, #174190, #158992, #20484, #146831, #53831, #12337, #56837, #196366, #8325, #165014, #70000, #164023, #10337, #132671, #71993, #133667, #180202, #86161, #115506, #131669, #104327, #55826, #25519, #116501, #57834, #87164, #177194, #195357, #147851, #38667, #42665, #194359, #181188, #135671, #148846, #11340, #71003, #41671, #193351, #54827, #103335, #26508, #88151, #117499, #179196, #178189, #149836, #118512, #85145, #73011, #39654, #166011, #27511, #100322, #9337, #101315, #40664, #134680, #102333, #119507, #89152, #162001, #163004, #23497, #74001, #24511, #150841, #45631, #44644, #167001, #107283, #93107, #186146, #136639, #30460, #138621, #32452, #168954, #123440, #122457, #105314, #1093, #184150, #106296, #60786, #154792, #169962, #153796, #183160, #92108, #47625, #94105, #185133, #15291, #91111, #31454, #76951, #151822, #28503, #102, #62769, #137634, #108284, #90137, #197343, #109279, #78935, #198321, #61772, #170958, #13311, #16290, #155784, #58806, #46624, #43651, #77940, #17281, #167982, #139607, #120474, #124450, #182166, #74977, #59798, #121468, #29480, #152801 ),
 ( #14293, #75960, #199321, #50605, #129407, #96096, #81894, #175944, #191104, #95103, #143587, #172959, #173956, #126436, #65756, #188134, #144585, #110275, #113250, #6071, #159757, #52578, #35423, #99074, #66753, #97076, #140611, #80922, #114238, #33444, #79940, #5070, #49605, #171956, #82907, #112264, #156792, #67749, #2101, #111268, #37414, #158757, #34437, #174940, #142598, #18285, #63782, #160764, #128414, #22254, #141610, #51585, #3097, #20246, #190110, #19275, #36403, #98057, #21252, #157785, #125454, #64774, #187150, #4078, #48623, #127425, #189133, #117255, #83903, #163774, #177945, #145586, #72768, #162757, #11091, #165767, #178947, #41424, #101072, #132426, #56593, #9090, #133421, #10092, #87907, #24266, #39412, #134438, #42422, #103090, #25275, #164771, #102089, #85915, #38422, #194118, #115260, #70758, #54581, #147603, #146581, #53583, #40418, #26266, #86917, #7064, #100078, #118267, #116254, #55581, #148600, #84901, #68745, #149594, #71752, #195110, #179957, #196123, #57593, #119263, #104085, #180946, #130403, #192101, #176953, #161763, #23258, #8075, #69751, #131420, #193107, #48144, #123958, #64300, #93632, #184664, #138159, #78456, #95620, #170485, #141133, #61307, #27262, #142120, #111790, #30984, #1621, #80447, #199840, #49136, #188651, #88911, #171484, #76482, #17807, #126943, #620, #124977, #3605, #32973, #172475, #110794, #109801, #94627, #63297, #122977, #33962, #150603, #46146, #157305, #156306, #79464, #2623, #18802, #107800, #50130, #169484, #31976, #65284, #14821, #15812, #92632, #125967, #187666, #154323, #16806, #77473, #47148, #140130, #139143, #186674, #62291, #155317, #185656, #108806, #96603, #51116, #191617, #113762, #67271, #83427, #146102, #193635, #69272, #19781, #82422, #143108, #38943, #66280, #70283, #127939, #175458, #147123, #162282, #159271, #131951, #22777, #130938, #177474, #160285, #55107, #190630, #145104, #173478, #68266, #112775, #36929, #192629, #85432, #158292, #174468, #53096, #98591, #128929, #6587, #7586, #34951, #54111, #81422, #144111, #4587, #21776, #115785, #129917, #84425, #99602, #100600, #114774, #52105, #23782, #189641, #8610, #176468, #35937, #37942, #161282, #97583, #20767, #5591, #103621, #87443, #118795, #179481, #86441, #150126, #135949, #134965, #178468, #132948, #151122, #149128, #195648, #41955, #117787, #116777, #59084, #196643, #133957, #165297, #10619, #181466, #197619, #75251, #152100, #27792, #105592, #39935, #120751, #74279, #101604, #104608, #13584, #42944, #58112, #72280, #12615, #180484, #71283, #24793, #26790, #182450, #57121, #89434, #148127, #163293, #28776, #198609, #40946, #88432, #167278, #9618, #43930, #136922, #194636, #119782, #56106, #166296, #102618, #11627, #73295, #90415, #164304, #25797, #140886, #139883, #124730, #93385, #168255, #79217, #121745, #29751, #64056, #1372, #63051, #171239, #186428, #95376, #31737, #47904, #185414, #91386, #125726, #46905, #169238, #123717, #17557, #32728, #16566, #45907, #170243, #48893, #15573, #109558, #157061, #110548, #14577, #94380, #92392, #155071, #107560, #108565, #30744, #187425, #153075, #156060, #172229, #2376, #33714, #78213, #18558, #80206, #141877, #60077, #380, #183437, #76235, #199597, #44922, #154079, #137915, #106578, #61064, #122736, #184427, #77231, #138900, #62052, #36681, #35698, #176222, #5347, #96364, #3368, #162039, #6345, #145860, #158052, #114521, #19542, #113522, #160040, #82172, #21527, #83188, #129676, #97345, #65043, #81187, #53869, #67031, #175216, #66033, #7342, #98341, #126699, #144862, #159031, #188403, #192386, #143868, #130692, #85181, #68025, #161039, #20524, #191374, #142869, #4348, #52850, #37691, #99356, #128690, #190387, #127700, #22533, #84180, #34707, #69027, #189400, #115543, #177231, #49881, #51862, #50877, #38703, #100360, #23535, #111546, #173231, #112535, #174229, #146870, #105349, #54863, #89188, #195395, #194394 ),
 ( #116537, #56873, #42702, #135708, #86197, #180238, #88187, #182202, #118548, #73046, #72030, #178225, #150880, #133703, #55861, #10373, #104363, #119543, #103372, #132705, #41707, #197379, #102369, #149871, #43687, #58844, #101351, #11376, #179233, #165050, #117535, #26543, #40699, #12374, #39689, #181226, #74037, #166047, #120511, #134718, #167036, #196401, #57871, #8362, #87201, #28538, #163040, #147887, #27547, #164058, #24547, #70037, #131706, #9373, #193387, #71038, #25557, #148882, #15329, #137669, #31492, #184186, #121503, #90174, #94142, #123479, #1132, #183197, #93144, #44679, #153833, #140, #45668, #61809, #138659, #46662, #199356, #151857, #168018, #109317, #168992, #76988, #152837, #62806, #185171, #13348, #108321, #107319, #136677, #170996, #30496, #47665, #75012, #170001, #124488, #92147, #154829, #14331, #75996, #16327, #77977, #186184, #139644, #32489, #60821, #155821, #198359, #29514, #59833, #106332, #91148, #122495, #55512, #164700, #10022, #87835, #88839, #26196, #150531, #180879, #117182, #72691, #42354, #133348, #74675, #104016, #70690, #12031, #149521, #132356, #59486, #11018, #198017, #152495, #165694, #28197, #134366, #197037, #71681, #195039, #58504, #120170, #105008, #196050, #57525, #56516, #166694, #135366, #102019, #73694, #118194, #121160, #182853, #178877, #119194, #179885, #27192, #181861, #43340, #89839, #151520, #40344, #41353, #194048, #29176, #163702, #13011, #136342, #103017, #25204, #44336, #105993, #167679, #90812, #86846, #148531, #98042, #55567, #100061, #146564, #85902, #113234, #117241, #174925, #160744, #194105, #9075, #6055, #178934, #69736, #177932, #24252, #7045, #40404, #37397, #130385, #102075, #115242, #159739, #22236, #39399, #132413, #143570, #21236, #38404, #83885, #114221, #192082, #193092, #20230, #116240, #66738, #129391, #190095, #68727, #54568, #145567, #131404, #8059, #147590, #53564, #175926, #70745, #81878, #101059, #161746, #162744, #23241, #99056, #36388, #176934, #51570, #84885, #191087, #5052, #82891, #144569, #128398, #67733, #52561, #25260, #179943, #198073, #134424, #42409, #88896, #164757, #163760, #133406, #136396, #167733, #182908, #14037, #58560, #122205, #89894, #120226, #86903, #104072, #152549, #56578, #103075, #28255, #72753, #195095, #106047, #135422, #118252, #29231, #148586, #11075, #75702, #197093, #196110, #59539, #165754, #41410, #10078, #183897, #166751, #90864, #26252, #74732, #87893, #73750, #181916, #27247, #43396, #105067, #151577, #57580, #71736, #149579, #137382, #150588, #13066, #119250, #199061, #121218, #180934, #44392, #12087, #60530, #45382, #185892, #34187, #188877, #1848, #64524, #124191, #33196, #46368, #108026, #94855, #156536, #141359, #47377, #109032, #169713, #2846, #171707, #138378, #48372, #92857, #95848, #19026, #91851, #846, #31206, #170711, #125205, #62519, #186901, #17030, #153544, #154544, #107035, #65507, #15041, #49354, #155535, #16039, #76702, #78684, #126191, #157532, #77697, #140360, #110029, #142348, #80672, #18035, #79689, #187887, #111016, #32202, #139365, #93858, #172703, #3828, #63530, #127168, #168707, #30209, #200058, #61527, #123196, #184886, #4816, #191844, #82650, #83654, #36158, #175683, #97810, #54335, #8836, #158514, #192856, #98817, #159499, #20002, #160511, #146327, #39163, #189866, #145332, #53325, #85661, #162504, #176698, #115004, #38172, #116006, #37158, #20995, #113985, #7816, #23004, #6814, #144332, #22001, #100821, #5821, #99827, #147348, #24005, #66503, #161512, #67497, #68492, #129154, #130147, #190851, #177695, #81645, #84650, #70504, #69500, #132172, #131166, #50359, #112018, #173707, #35175, #52328, #96830, #143329, #51340, #128166, #113000, #174694, #136168, #165521, #148345, #197843, #55328, #41174, #105820, #27017, #26016, #166521, #195873, #86661, #193863, #152324, #196864, #59309, #9841, #104832, #71500, #103840, #150357, #72511, #11854, #73519, #119998 ),
 ( #28019, #182676, #116999, #12836, #151347, #178694, #181684, #90642, #43165, #135190, #87660, #89661, #57346, #133167, #101832, #42180, #120978, #134186, #74502, #25018, #40156, #167507, #75476, #194858, #88661, #44160, #163519, #29002, #13810, #56331, #58330, #118013, #179702, #102837, #164523, #149345, #10841, #119021, #180704, #156292, #95606, #18788, #78442, #183667, #124963, #33948, #107786, #31962, #49122, #140116, #79449, #17793, #16792, #1607, #170472, #45152, #141119, #198837, #106808, #14808, #172461, #63283, #186660, #2609, #29980, #157291, #91619, #77459, #110779, #125953, #122964, #137149, #48130, #94613, #64286, #123945, #60301, #154310, #47135, #121975, #93617, #76469, #139130, #187651, #168482, #153307, #138146, #155302, #607, #30972, #108793, #109787, #199826, #32958, #61294, #46133, #184651, #185643, #171470, #62277, #169471, #92619, #15799, #20753, #174454, #130924, #38929, #99587, #160271, #37927, #98577, #97569, #34937, #128915, #111776, #67257, #51101, #82408, #143094, #50116, #113748, #161268, #21761, #142106, #96589, #114760, #112761, #159257, #5577, #81408, #80433, #22762, #83413, #144096, #190616, #35923, #145090, #84411, #100586, #115771, #191603, #69258, #3591, #146088, #7572, #65269, #68252, #177459, #6573, #129903, #52091, #176454, #175444, #158278, #188636, #36914, #192615, #53082, #54097, #173464, #126929, #162268, #19767, #4573, #66265, #127925, #189627, #9603, #185142, #73279, #181450, #27776, #10603, #46633, #40931, #133942, #123450, #118779, #101590, #25782, #42928, #138631, #147109, #163278, #41939, #164289, #117772, #195632, #196627, #108293, #119766, #70269, #132932, #193621, #72265, #58096, #149113, #134949, #150110, #92118, #87428, #179466, #76960, #23768, #104592, #103605, #166278, #165281, #102603, #178454, #57105, #55092, #180467, #194620, #26774, #86426, #116763, #88415, #153806, #11611, #85418, #39921, #15300, #56091, #112, #61781, #24779, #8595, #131937, #148112, #71268, #95112, #63791, #34446, #50614, #128423, #5080, #80932, #158768, #169972, #189141, #127435, #93116, #157794, #66762, #96105, #188143, #125464, #4087, #33453, #124459, #77949, #18294, #35433, #110284, #142608, #1102, #31464, #81903, #51595, #170968, #141619, #20257, #139616, #112273, #190119, #154801, #111278, #16299, #19285, #62778, #140620, #64784, #143596, #172968, #173965, #97085, #49615, #65765, #3108, #186156, #47635, #109289, #32461, #94114, #155793, #17290, #78944, #2110, #187161, #48632, #126445, #171966, #156801, #79949, #71764, #195123, #54592, #159768, #101084, #10104, #83915, #8086, #25287, #116266, #55593, #194130, #193118, #177956, #146592, #21263, #132439, #174951, #82919, #191116, #148613, #39424, #162769, #178961, #6082, #133434, #67761, #53595, #86930, #102101, #99085, #113259, #24278, #70770, #117268, #100090, #36414, #130414, #23269, #98068, #69763, #52590, #115271, #40430, #144596, #129418, #114250, #131432, #176964, #7076, #84913, #85927, #175956, #9103, #37425, #22265, #160776, #161774, #147616, #38434, #163786, #145597, #68757, #192113, #150616, #107059, #15065, #75731, #136420, #14064, #74758, #73775, #11105, #105093, #87920, #43424, #27276, #58584, #119275, #26278, #89919, #137407, #198100, #118279, #72780, #90888, #88924, #135448, #181941, #57606, #56605, #199087, #59566, #197117, #166779, #12112, #121241, #60555, #76726, #91876, #167758, #45406, #179970, #122230, #183921, #41436, #44418, #153568, #182935, #106071, #120250, #152574, #28280, #134450, #164784, #151601, #168730, #13092, #29256, #149607, #103103, #30234, #138401, #180958, #196135, #42435, #104098, #165781, #109058, #31232, #142376, #171735, #154568, #3855, #61550, #47402, #112046, #33223, #32226, #172732, #1875, #92881, #200082, #158540, #2874, #65534, #16064, #111045, #77722, #110055, #156564, #78711, #18062, #79717, #126217, #93884, #123219, #139388, #50386, #63556, #94883, #62545 ),
 ( #187913, #870, #124220, #49382, #34213, #95876, #140387, #125230, #185917, #157559, #64553, #170735, #141386, #155562, #127194, #173734, #184909, #17056, #186928, #48398, #19052, #80699, #188906, #35203, #46394, #96856, #108052, #20030, #169737, #81672, #191870, #190878, #113027, #53353, #39189, #132199, #82676, #176724, #84675, #178720, #55355, #69527, #146354, #7841, #147374, #68519, #52354, #6840, #100847, #116032, #99853, #129180, #115031, #193890, #98844, #131192, #40182, #117025, #97836, #192882, #175708, #38197, #114010, #130173, #37186, #8863, #174719, #177721, #70530, #162529, #101861, #161537, #163545, #54360, #23030, #143355, #83680, #21021, #145358, #24033, #25045, #66530, #144360, #85687, #4844, #160539, #128193, #189891, #51366, #36182, #159524, #22028, #5847, #67523, #59336, #11882, #136194, #12864, #90670, #27044, #180730, #137177, #45183, #105848, #166548, #44189, #104859, #103866, #41201, #135218, #118040, #73545, #57375, #88690, #149371, #56358, #120024, #167535, #28047, #148372, #102863, #121006, #119048, #165547, #196890, #87686, #86688, #29030, #89688, #150386, #58357, #42206, #151373, #152352, #106837, #122006, #197869, #75503, #9867, #13837, #198865, #71526, #74529, #183697, #182704, #60332, #181709, #168512, #43190, #164548, #194884, #133193, #179731, #26041, #10867, #72537, #134213, #195900, #111811, #31001, #1642, #80467, #138177, #49156, #188672, #30010, #171505, #76501, #17828, #126963, #638, #124999, #142141, #32994, #172497, #110814, #109822, #94648, #63319, #199858, #33984, #91648, #61324, #107818, #65304, #156328, #79486, #95640, #122995, #50152, #184681, #170504, #3625, #18823, #15831, #153337, #141155, #187686, #157328, #16826, #14838, #47166, #140150, #46164, #186694, #169502, #48164, #2644, #92650, #154339, #64320, #125988, #77491, #139161, #155337, #62308, #93652, #123978, #185676, #108825, #31994, #78477, #162305, #128951, #114798, #8633, #23805, #127960, #176491, #5614, #6611, #159292, #98614, #20789, #177497, #143128, #146125, #38967, #192651, #85456, #68290, #131974, #99625, #129941, #173499, #113784, #147145, #66300, #112796, #37967, #82444, #4608, #115807, #145127, #189663, #100623, #34972, #144132, #70305, #191640, #67293, #7610, #175480, #51136, #96624, #193658, #161306, #55130, #174490, #84447, #35957, #83450, #53120, #52128, #22801, #69295, #130961, #190652, #158313, #97604, #19801, #36952, #54134, #160308, #81442, #21798, #116800, #196668, #10643, #178491, #105618, #195673, #43956, #198636, #11652, #74304, #133982, #42968, #56130, #117812, #104631, #166320, #151147, #57144, #118821, #179505, #12638, #181490, #148150, #58136, #102642, #167306, #28802, #101629, #72304, #40972, #180506, #134989, #41978, #119805, #26815, #163319, #164327, #39958, #75277, #24816, #59109, #165323, #25820, #86465, #88455, #135972, #90441, #120774, #9641, #89458, #182475, #197643, #152127, #73318, #136947, #27817, #13609, #71308, #103645, #132971, #194661, #87466, #149153, #150151, #91412, #2400, #31760, #14604, #64079, #121770, #107586, #172252, #93409, #92417, #32754, #62076, #153100, #60102, #18582, #63078, #125749, #76260, #171266, #137938, #170266, #16589, #138923, #78237, #139908, #186453, #154103, #183463, #199622, #110571, #123741, #155095, #122761, #187449, #1398, #44949, #124757, #15597, #106604, #48917, #404, #33740, #141900, #47929, #17583, #77255, #109583, #61089, #184451, #94405, #156086, #79243, #185440, #46930, #45931, #140914, #95400, #169264, #157086, #30770, #80229, #168280, #29777, #108589, #142891, #20549, #21552, #159055, #83212, #113546, #49905, #127724, #3391, #162063, #111571, #145884, #51887, #50901, #173255, #175240, #99380, #192411, #4373, #36705, #144887, #38727, #115568, #129702, #6369, #68049, #7367, #128714, #112559, #67056, #161063, #176247, #160065, #189426, #98367, #53893, #82199, #191399, #100385, #177255, #158075, #52876, #35722 ),
 ( #188427, #97369, #66057, #143891, #114548, #5372, #37718, #22558, #34730, #174254, #65066, #23559, #96388, #69052, #84204, #190411, #19566, #130718, #85207, #126723, #81210, #180260, #88209, #182227, #58868, #73069, #149893, #11400, #150904, #72052, #55885, #10395, #104387, #119565, #103394, #132727, #56896, #135731, #102392, #134741, #43712, #197402, #101374, #196423, #179258, #41730, #194415, #133726, #117558, #12398, #116561, #165072, #87223, #40723, #118570, #181248, #167060, #42725, #193412, #164080, #178250, #195418, #166070, #26566, #57893, #27572, #74060, #148905, #25579, #120534, #105373, #89211, #28561, #146896, #8387, #70062, #163064, #131730, #39711, #54887, #24570, #86219, #9395, #147909, #71061, #109339, #108345, #151881, #106356, #124512, #60843, #169014, #15354, #91170, #90198, #32512, #170025, #107341, #77010, #184208, #154853, #171021, #48681, #125513, #1154, #78996, #13371, #94164, #47689, #75035, #77999, #187210, #16351, #31515, #45690, #186208, #153856, #44702, #198382, #140670, #110333, #155843, #93168, #17340, #139666, #30518, #168040, #138682, #121526, #163, #122518, #92170, #152859, #59859, #123501, #2162, #62829, #136701, #29537, #63841, #61831, #185194, #46685, #14354, #183221, #172014, #76019, #137694, #199379, #127486, #98124, #117058, #194917, #71561, #144650, #25078, #33503, #55388, #193925, #156850, #21316, #133226, #159821, #51647, #189191, #70565, #97136, #188193, #141669, #81955, #101896, #174015, #8897, #64833, #95162, #148406, #118074, #34498, #5130, #86721, #3160, #178753, #56392, #18345, #175003, #80000, #82974, #126495, #4138, #128475, #9901, #36467, #40217, #163578, #113311, #132233, #66813, #49665, #111329, #173019, #96156, #157845, #19337, #80984, #142659, #65817, #50665, #112325, #35486, #158819, #20307, #143647, #190171, #138209, #29060, #137210, #183727, #166581, #199891, #196922, #89721, #76533, #74559, #57407, #181743, #43225, #60365, #104892, #28081, #197901, #120056, #73577, #151406, #152383, #61355, #75535, #26074, #88723, #149403, #12895, #13868, #136226, #90700, #105880, #45213, #59370, #135250, #58389, #106867, #179765, #121042, #198897, #182738, #167567, #119079, #180761, #122037, #168541, #30039, #44222, #91678, #42237, #153370, #14872, #10898, #41234, #165579, #102895, #164580, #87718, #72571, #103898, #134246, #195932, #27077, #150419, #11914, #169534, #47198, #123026, #81471, #31034, #65334, #171535, #170537, #92683, #33023, #18853, #111840, #62340, #156357, #64351, #158341, #34999, #49187, #126020, #187716, #126994, #48196, #32027, #186725, #80499, #95672, #79515, #108858, #94678, #173529, #78508, #110845, #19830, #96654, #77523, #172529, #155368, #17859, #93685, #109850, #4638, #16857, #154371, #46196, #188701, #142172, #143158, #141185, #184711, #34015, #2674, #107849, #63352, #15865, #139195, #124010, #157359, #140181, #670, #50183, #3656, #185708, #1674, #125029, #113812, #178517, #99651, #98643, #38994, #68317, #159321, #66329, #24842, #69322, #8660, #20817, #177525, #82473, #176520, #22827, #145156, #84473, #146151, #192680, #160337, #127990, #144158, #116826, #129968, #37996, #128981, #70333, #161335, #189693, #7638, #21826, #51165, #55156, #175507, #39983, #130988, #83478, #100650, #191668, #5643, #112826, #86491, #54163, #132000, #67320, #162331, #190679, #115836, #23832, #6639, #85482, #147171, #193688, #53147, #174518, #52155, #101654, #114826, #163346, #36981, #148176, #35985, #97632, #119832, #118849, #71334, #105644, #42006, #182503, #75303, #135018, #135999, #180532, #166348, #25849, #87492, #104663, #27846, #12665, #103671, #165349, #149181, #74333, #89487, #179531, #181517, #10669, #43983, #167333, #132996, #26843, #72333, #88484, #42996, #150179, #151177, #11680, #194687, #134008, #9669, #56157, #164353, #28829, #58165, #73345, #195699, #197670, #120803, #152153, #57171, #59135, #90470, #117838, #41001, #13636 ) ),
 .UNSPECIFIED., .T., .F., .T. ) 
 B_SPLINE_SURFACE_WITH_KNOTS ( ( 4, 3, 4 ),
 ( 3, 2, 2, 2, 2, 2, 2, 2, 2, 2, 2, 2, 2, 2, 2, 2, 2, 2, 2, 2, 2, 2, 2, 2, 2, 2, 2, 2, 2, 2, 2, 2, 2, 2, 2, 2, 2, 2, 2, 2, 2, 2, 2, 2, 2, 2, 2, 2, 2, 2, 2, 2, 2, 2, 2, 2, 2, 2, 2, 2, 2, 2, 2, 2, 2, 2, 2, 2, 2, 2, 2, 2, 2, 2, 2, 2, 2, 2, 2, 2, 2, 2, 2, 2, 2, 2, 2, 2, 2, 2, 2, 2, 2, 2, 2, 2, 2, 2, 2, 2, 2, 2, 2, 2, 2, 2, 2, 2, 2, 2, 2, 2, 2, 2, 2, 2, 2, 2, 2, 2, 2, 2, 2, 2, 2, 2, 2, 2, 2, 2, 2, 2, 2, 2, 2, 2, 2, 2, 2, 2, 2, 2, 2, 2, 2, 2, 2, 2, 2, 2, 2, 2, 2, 2, 2, 2, 2, 2, 2, 2, 2, 2, 2, 2, 2, 2, 2, 2, 2, 2, 2, 2, 2, 2, 2, 2, 2, 2, 2, 2, 2, 2, 2, 2, 2, 2, 2, 2, 2, 2, 2, 2, 2, 2, 2, 2, 2, 2, 2, 2, 2, 2, 2, 2, 2, 2, 2, 2, 2, 2, 2, 2, 2, 2, 2, 2, 2, 2, 2, 2, 2, 2, 2, 2, 2, 2, 2, 2, 3 ),
 ( 0.000000000000000000, 0.5000000000000000000, 1.000000000000000000 ),
 ( 0.000000000000000000, 0.004385964912280701511, 0.008771929824561403022, 0.01315789473684210453, 0.01754385964912280604, 0.02192982456140350755, 0.02631578947368420907, 0.03070175438596491058, 0.03508771929824561209, 0.03947368421052631360, 0.04385964912280701511, 0.04824561403508771662, 0.05263157894736841813, 0.05701754385964911964, 0.06140350877192982115, 0.06578947368421052266, 0.07017543859649122417, 0.07456140350877192569, 0.07894736842105262720, 0.08333333333333332871, 0.08771929824561403022, 0.09210526315789473173, 0.09649122807017543324, 0.1008771929824561348, 0.1052631578947368363, 0.1096491228070175378, 0.1140350877192982393, 0.1184210526315789408, 0.1228070175438596423, 0.1271929824561403577, 0.1315789473684210453, 0.1359649122807017607, 0.1403508771929824483, 0.1447368421052631637, 0.1491228070175438514, 0.1535087719298245668, 0.1578947368421052544, 0.1622807017543859698, 0.1666666666666666574, 0.1710526315789473728, 0.1754385964912280604, 0.1798245614035087758, 0.1842105263157894635, 0.1885964912280701788, 0.1929824561403508665, 0.1973684210526315819, 0.2017543859649122695, 0.2061403508771929849, 0.2105263157894736725, 0.2149122807017543879, 0.2192982456140350755, 0.2236842105263157909, 0.2280701754385964786, 0.2324561403508771940, 0.2368421052631578816, 0.2412280701754385970, 0.2456140350877192846, 0.2500000000000000000, 0.2543859649122807154, 0.2587719298245614308, 0.2631578947368420907, 0.2675438596491228060, 0.2719298245614035214, 0.2763157894736842368, 0.2807017543859648967, 0.2850877192982456121, 0.2894736842105263275, 0.2938596491228070429, 0.2982456140350877027, 0.3026315789473684181, 0.3070175438596491335, 0.3114035087719298489, 0.3157894736842105088, 0.3201754385964912242, 0.3245614035087719396, 0.3289473684210526550, 0.3333333333333333148, 0.3377192982456140302, 0.3421052631578947456, 0.3464912280701754610, 0.3508771929824561209, 0.3552631578947368363, 0.3596491228070175517, 0.3640350877192982670, 0.3684210526315789269, 0.3728070175438596423, 0.3771929824561403577, 0.3815789473684210731, 0.3859649122807017330, 0.3903508771929824483, 0.3947368421052631637, 0.3991228070175438791, 0.4035087719298245390, 0.4078947368421052544, 0.4122807017543859698, 0.4166666666666666852, 0.4210526315789473450, 0.4254385964912280604, 0.4298245614035087758, 0.4342105263157894912, 0.4385964912280701511, 0.4429824561403508665, 0.4473684210526315819, 0.4517543859649122973, 0.4561403508771929571, 0.4605263157894736725, 0.4649122807017543879, 0.4692982456140351033, 0.4736842105263157632, 0.4780701754385964786, 0.4824561403508771940, 0.4868421052631579093, 0.4912280701754385692, 0.4956140350877192846, 0.5000000000000000000, 0.5043859649122807154, 0.5087719298245614308, 0.5131578947368421462, 0.5175438596491228616, 0.5219298245614034659, 0.5263157894736841813, 0.5307017543859648967, 0.5350877192982456121, 0.5394736842105263275, 0.5438596491228070429, 0.5482456140350877583, 0.5526315789473684736, 0.5570175438596490780, 0.5614035087719297934, 0.5657894736842105088, 0.5701754385964912242, 0.5745614035087719396, 0.5789473684210526550, 0.5833333333333333703, 0.5877192982456140857, 0.5921052631578946901, 0.5964912280701754055, 0.6008771929824561209, 0.6052631578947368363, 0.6096491228070175517, 0.6140350877192982670, 0.6184210526315789824, 0.6228070175438596978, 0.6271929824561403022, 0.6315789473684210176, 0.6359649122807017330, 0.6403508771929824483, 0.6447368421052631637, 0.6491228070175438791, 0.6535087719298245945, 0.6578947368421053099, 0.6622807017543859143, 0.6666666666666666297, 0.6710526315789473450, 0.6754385964912280604, 0.6798245614035087758, 0.6842105263157894912, 0.6885964912280702066, 0.6929824561403509220, 0.6973684210526315264, 0.7017543859649122417, 0.7061403508771929571, 0.7105263157894736725, 0.7149122807017543879, 0.7192982456140351033, 0.7236842105263158187, 0.7280701754385965341, 0.7324561403508771384, 0.7368421052631578538, 0.7412280701754385692, 0.7456140350877192846, 0.7500000000000000000, 0.7543859649122807154, 0.7587719298245614308, 0.7631578947368421462, 0.7675438596491228616, 0.7719298245614034659, 0.7763157894736841813, 0.7807017543859648967, 0.7850877192982456121, 0.7894736842105263275, 0.7938596491228070429, 0.7982456140350877583, 0.8026315789473684736, 0.8070175438596490780, 0.8114035087719297934, 0.8157894736842105088, 0.8201754385964912242, 0.8245614035087719396, 0.8289473684210526550, 0.8333333333333333703, 0.8377192982456140857, 0.8421052631578946901, 0.8464912280701754055, 0.8508771929824561209, 0.8552631578947368363, 0.8596491228070175517, 0.8640350877192982670, 0.8684210526315789824, 0.8728070175438596978, 0.8771929824561403022, 0.8815789473684210176, 0.8859649122807017330, 0.8903508771929824483, 0.8947368421052631637, 0.8991228070175438791, 0.9035087719298245945, 0.9078947368421053099, 0.9122807017543859143, 0.9166666666666666297, 0.9210526315789473450, 0.9254385964912280604, 0.9298245614035087758, 0.9342105263157894912, 0.9385964912280702066, 0.9429824561403509220, 0.9473684210526315264, 0.9517543859649122417, 0.9561403508771929571, 0.9605263157894736725, 0.9649122807017543879, 0.9692982456140351033, 0.9736842105263158187, 0.9780701754385965341, 0.9824561403508771384, 0.9868421052631578538, 0.9912280701754385692, 0.9956140350877192846, 1.000000000000000000 ),
 .UNSPECIFIED. ) 
 GEOMETRIC_REPRESENTATION_ITEM ( )  RATIONAL_B_SPLINE_SURFACE ( (
 ( 1.000000000000000000, 0.9659258262890683122, 1.000000000000000000, 0.9659258262890683122, 1.000000000000000000, 0.9659258262890683122, 1.000000000000000000, 0.9659258262890683122, 1.000000000000000000, 0.9659258262890683122, 1.000000000000000000, 0.9659258262890683122, 1.000000000000000000, 0.9659258262890683122, 1.000000000000000000, 0.9659258262890683122, 1.000000000000000000, 0.9659258262890683122, 1.000000000000000000, 0.9659258262890683122, 1.000000000000000000, 0.9659258262890683122, 1.000000000000000000, 0.9659258262890683122, 1.000000000000000000, 0.9659258262890683122, 1.000000000000000000, 0.9659258262890683122, 1.000000000000000000, 0.9659258262890683122, 1.000000000000000000, 0.9659258262890683122, 1.000000000000000000, 0.9659258262890683122, 1.000000000000000000, 0.9659258262890683122, 1.000000000000000000, 0.9659258262890683122, 1.000000000000000000, 0.9659258262890683122, 1.000000000000000000, 0.9659258262890683122, 1.000000000000000000, 0.9659258262890683122, 1.000000000000000000, 0.9659258262890683122, 1.000000000000000000, 0.9659258262890683122, 1.000000000000000000, 0.9659258262890683122, 1.000000000000000000, 0.9659258262890683122, 1.000000000000000000, 0.9659258262890683122, 1.000000000000000000, 0.9659258262890683122, 1.000000000000000000, 0.9659258262890683122, 1.000000000000000000, 0.9659258262890683122, 1.000000000000000000, 0.9659258262890683122, 1.000000000000000000, 0.9659258262890683122, 1.000000000000000000, 0.9659258262890683122, 1.000000000000000000, 0.9659258262890683122, 1.000000000000000000, 0.9659258262890683122, 1.000000000000000000, 0.9659258262890683122, 1.000000000000000000, 0.9659258262890683122, 1.000000000000000000, 0.9659258262890683122, 1.000000000000000000, 0.9659258262890683122, 1.000000000000000000, 0.9659258262890683122, 1.000000000000000000, 0.9659258262890683122, 1.000000000000000000, 0.9659258262890683122, 1.000000000000000000, 0.9659258262890683122, 1.000000000000000000, 0.9659258262890683122, 1.000000000000000000, 0.9659258262890683122, 1.000000000000000000, 0.9659258262890683122, 1.000000000000000000, 0.9659258262890683122, 1.000000000000000000, 0.9659258262890683122, 1.000000000000000000, 0.9659258262890683122, 1.000000000000000000, 0.9659258262890683122, 1.000000000000000000, 0.9659258262890683122, 1.000000000000000000, 0.9659258262890683122, 1.000000000000000000, 0.9659258262890683122, 1.000000000000000000, 0.9659258262890683122, 1.000000000000000000, 0.9659258262890683122, 1.000000000000000000, 0.9659258262890683122, 1.000000000000000000, 0.9659258262890683122, 1.000000000000000000, 0.9659258262890683122, 1.000000000000000000, 0.9659258262890683122, 1.000000000000000000, 0.9659258262890683122, 1.000000000000000000, 0.9659258262890683122, 1.000000000000000000, 0.9659258262890683122, 1.000000000000000000, 0.9659258262890683122, 1.000000000000000000, 0.9659258262890683122, 1.000000000000000000, 0.9659258262890683122, 1.000000000000000000, 0.9659258262890683122, 1.000000000000000000, 0.9659258262890683122, 1.000000000000000000, 0.9659258262890683122, 1.000000000000000000, 0.9659258262890683122, 1.000000000000000000, 0.9659258262890683122, 1.000000000000000000, 0.9659258262890683122, 1.000000000000000000, 0.9659258262890683122, 1.000000000000000000, 0.9659258262890683122, 1.000000000000000000, 0.9659258262890683122, 1.000000000000000000, 0.9659258262890683122, 1.000000000000000000, 0.9659258262890683122, 1.000000000000000000, 0.9659258262890683122, 1.000000000000000000, 0.9659258262890683122, 1.000000000000000000, 0.9659258262890683122, 1.000000000000000000, 0.9659258262890683122, 1.000000000000000000, 0.9659258262890683122, 1.000000000000000000, 0.9659258262890683122, 1.000000000000000000, 0.9659258262890683122, 1.000000000000000000, 0.9659258262890683122, 1.000000000000000000, 0.9659258262890683122, 1.000000000000000000, 0.9659258262890683122, 1.000000000000000000, 0.9659258262890683122, 1.000000000000000000, 0.9659258262890683122, 1.000000000000000000, 0.9659258262890683122, 1.000000000000000000, 0.9659258262890683122, 1.000000000000000000, 0.9659258262890683122, 1.000000000000000000, 0.9659258262890683122, 1.000000000000000000, 0.9659258262890683122, 1.000000000000000000, 0.9659258262890683122, 1.000000000000000000, 0.9659258262890683122, 1.000000000000000000, 0.9659258262890683122, 1.000000000000000000, 0.9659258262890683122, 1.000000000000000000, 0.9659258262890683122, 1.000000000000000000, 0.9659258262890683122, 1.000000000000000000, 0.9659258262890683122, 1.000000000000000000, 0.9659258262890683122, 1.000000000000000000, 0.9659258262890683122, 1.000000000000000000, 0.9659258262890683122, 1.000000000000000000, 0.9659258262890683122, 1.000000000000000000, 0.9659258262890683122, 1.000000000000000000, 0.9659258262890683122, 1.000000000000000000, 0.9659258262890683122, 1.000000000000000000, 0.9659258262890683122, 1.000000000000000000, 0.9659258262890683122, 1.000000000000000000, 0.9659258262890683122, 1.000000000000000000, 0.9659258262890683122, 1.000000000000000000, 0.9659258262890683122, 1.000000000000000000, 0.9659258262890683122, 1.000000000000000000, 0.9659258262890683122, 1.000000000000000000, 0.9659258262890683122, 1.000000000000000000, 0.9659258262890683122, 1.000000000000000000, 0.9659258262890683122, 1.000000000000000000, 0.9659258262890683122, 1.000000000000000000, 0.9659258262890683122, 1.000000000000000000, 0.9659258262890683122, 1.000000000000000000, 0.9659258262890683122, 1.000000000000000000, 0.9659258262890683122, 1.000000000000000000, 0.9659258262890683122, 1.000000000000000000, 0.9659258262890683122, 1.000000000000000000, 0.9659258262890683122, 1.000000000000000000, 0.9659258262890683122, 1.000000000000000000, 0.9659258262890683122, 1.000000000000000000, 0.9659258262890683122, 1.000000000000000000, 0.9659258262890683122, 1.000000000000000000, 0.9659258262890683122, 1.000000000000000000, 0.9659258262890683122, 1.000000000000000000, 0.9659258262890683122, 1.000000000000000000, 0.9659258262890683122, 1.000000000000000000, 0.9659258262890683122, 1.000000000000000000, 0.9659258262890683122, 1.000000000000000000, 0.9659258262890683122, 1.000000000000000000, 0.9659258262890683122, 1.000000000000000000, 0.9659258262890683122, 1.000000000000000000, 0.9659258262890683122, 1.000000000000000000, 0.9659258262890683122, 1.000000000000000000, 0.9659258262890683122, 1.000000000000000000, 0.9659258262890683122, 1.000000000000000000, 0.9659258262890683122, 1.000000000000000000, 0.9659258262890683122, 1.000000000000000000, 0.9659258262890683122, 1.000000000000000000, 0.9659258262890683122, 1.000000000000000000, 0.9659258262890683122, 1.000000000000000000, 0.9659258262890683122, 1.000000000000000000, 0.9659258262890683122, 1.000000000000000000, 0.9659258262890683122, 1.000000000000000000, 0.9659258262890683122, 1.000000000000000000, 0.9659258262890683122, 1.000000000000000000, 0.9659258262890683122, 1.000000000000000000, 0.9659258262890683122, 1.000000000000000000, 0.9659258262890683122, 1.000000000000000000, 0.9659258262890683122, 1.000000000000000000, 0.9659258262890683122, 1.000000000000000000, 0.9659258262890683122, 1.000000000000000000, 0.9659258262890683122, 1.000000000000000000, 0.9659258262890683122, 1.000000000000000000, 0.9659258262890683122, 1.000000000000000000, 0.9659258262890683122, 1.000000000000000000, 0.9659258262890683122, 1.000000000000000000, 0.9659258262890683122, 1.000000000000000000, 0.9659258262890683122, 1.000000000000000000, 0.9659258262890683122, 1.000000000000000000, 0.9659258262890683122, 1.000000000000000000, 0.9659258262890683122, 1.000000000000000000, 0.9659258262890683122, 1.000000000000000000, 0.9659258262890683122, 1.000000000000000000, 0.9659258262890683122, 1.000000000000000000, 0.9659258262890683122, 1.000000000000000000, 0.9659258262890683122, 1.000000000000000000, 0.9659258262890683122, 1.000000000000000000, 0.9659258262890683122, 1.000000000000000000, 0.9659258262890683122, 1.000000000000000000, 0.9659258262890683122, 1.000000000000000000, 0.9659258262890683122, 1.000000000000000000, 0.9659258262890683122, 1.000000000000000000, 0.9659258262890683122, 1.000000000000000000, 0.9659258262890683122, 1.000000000000000000, 0.9659258262890683122, 1.000000000000000000, 0.9659258262890683122, 1.000000000000000000, 0.9659258262890683122, 1.000000000000000000, 0.9659258262890683122, 1.000000000000000000, 0.9659258262890683122, 1.000000000000000000, 0.9659258262890683122, 1.000000000000000000, 0.9659258262890683122, 1.000000000000000000, 0.9659258262890683122, 1.000000000000000000, 0.9659258262890683122, 1.000000000000000000, 0.9659258262890683122, 1.000000000000000000, 0.9659258262890683122, 1.000000000000000000, 0.9659258262890683122, 1.000000000000000000, 0.9659258262890683122, 1.000000000000000000, 0.9659258262890683122, 1.000000000000000000, 0.9659258262890683122, 1.000000000000000000, 0.9659258262890683122, 1.000000000000000000, 0.9659258262890683122, 1.000000000000000000, 0.9659258262890683122, 1.000000000000000000, 0.9659258262890683122, 1.000000000000000000, 0.9659258262890683122, 1.000000000000000000, 0.9659258262890683122, 1.000000000000000000, 0.9659258262890683122, 1.000000000000000000, 0.9659258262890683122, 1.000000000000000000, 0.9659258262890683122, 1.000000000000000000, 0.9659258262890683122, 1.000000000000000000, 0.9659258262890683122, 1.000000000000000000, 0.9659258262890683122, 1.000000000000000000, 0.9659258262890683122, 1.000000000000000000, 0.9659258262890683122, 1.000000000000000000, 0.9659258262890683122, 1.000000000000000000, 0.9659258262890683122, 1.000000000000000000, 0.9659258262890683122, 1.000000000000000000, 0.9659258262890683122, 1.000000000000000000, 0.9659258262890683122, 1.000000000000000000, 0.9659258262890683122, 1.000000000000000000, 0.9659258262890683122, 1.000000000000000000, 0.9659258262890683122, 1.000000000000000000, 0.9659258262890683122, 1.000000000000000000, 0.9659258262890683122, 1.000000000000000000, 0.9659258262890683122, 1.000000000000000000, 0.9659258262890683122, 1.000000000000000000, 0.9659258262890683122, 1.000000000000000000, 0.9659258262890683122, 1.000000000000000000, 0.9659258262890683122, 1.000000000000000000, 0.9659258262890683122, 1.000000000000000000, 0.9659258262890683122, 1.000000000000000000, 0.9659258262890683122, 1.000000000000000000),
 ( 0.3333333333333333703, 0.3219752754296894559, 0.3333333333333333703, 0.3219752754296894559, 0.3333333333333333703, 0.3219752754296894559, 0.3333333333333333703, 0.3219752754296894559, 0.3333333333333333703, 0.3219752754296894559, 0.3333333333333333703, 0.3219752754296894559, 0.3333333333333333703, 0.3219752754296894559, 0.3333333333333333703, 0.3219752754296894559, 0.3333333333333333703, 0.3219752754296894559, 0.3333333333333333703, 0.3219752754296894559, 0.3333333333333333703, 0.3219752754296894559, 0.3333333333333333703, 0.3219752754296894559, 0.3333333333333333703, 0.3219752754296894559, 0.3333333333333333703, 0.3219752754296894559, 0.3333333333333333703, 0.3219752754296894559, 0.3333333333333333703, 0.3219752754296894559, 0.3333333333333333703, 0.3219752754296894559, 0.3333333333333333703, 0.3219752754296894559, 0.3333333333333333703, 0.3219752754296894559, 0.3333333333333333703, 0.3219752754296894559, 0.3333333333333333703, 0.3219752754296894559, 0.3333333333333333703, 0.3219752754296894559, 0.3333333333333333703, 0.3219752754296894559, 0.3333333333333333703, 0.3219752754296894559, 0.3333333333333333703, 0.3219752754296894559, 0.3333333333333333703, 0.3219752754296894559, 0.3333333333333333703, 0.3219752754296894559, 0.3333333333333333703, 0.3219752754296894559, 0.3333333333333333703, 0.3219752754296894559, 0.3333333333333333703, 0.3219752754296894559, 0.3333333333333333703, 0.3219752754296894559, 0.3333333333333333703, 0.3219752754296894559, 0.3333333333333333703, 0.3219752754296894559, 0.3333333333333333703, 0.3219752754296894559, 0.3333333333333333703, 0.3219752754296894559, 0.3333333333333333703, 0.3219752754296894559, 0.3333333333333333703, 0.3219752754296894559, 0.3333333333333333703, 0.3219752754296894559, 0.3333333333333333703, 0.3219752754296894559, 0.3333333333333333703, 0.3219752754296894559, 0.3333333333333333703, 0.3219752754296894559, 0.3333333333333333703, 0.3219752754296894559, 0.3333333333333333703, 0.3219752754296894559, 0.3333333333333333703, 0.3219752754296894559, 0.3333333333333333703, 0.3219752754296894559, 0.3333333333333333703, 0.3219752754296894559, 0.3333333333333333703, 0.3219752754296894559, 0.3333333333333333703, 0.3219752754296894559, 0.3333333333333333703, 0.3219752754296894559, 0.3333333333333333703, 0.3219752754296894559, 0.3333333333333333703, 0.3219752754296894559, 0.3333333333333333703, 0.3219752754296894559, 0.3333333333333333703, 0.3219752754296894559, 0.3333333333333333703, 0.3219752754296894559, 0.3333333333333333703, 0.3219752754296894559, 0.3333333333333333703, 0.3219752754296894559, 0.3333333333333333703, 0.3219752754296894559, 0.3333333333333333703, 0.3219752754296894559, 0.3333333333333333703, 0.3219752754296894559, 0.3333333333333333703, 0.3219752754296894559, 0.3333333333333333703, 0.3219752754296894559, 0.3333333333333333703, 0.3219752754296894559, 0.3333333333333333703, 0.3219752754296894559, 0.3333333333333333703, 0.3219752754296894559, 0.3333333333333333703, 0.3219752754296894559, 0.3333333333333333703, 0.3219752754296894559, 0.3333333333333333703, 0.3219752754296894559, 0.3333333333333333703, 0.3219752754296894559, 0.3333333333333333703, 0.3219752754296894559, 0.3333333333333333703, 0.3219752754296894559, 0.3333333333333333703, 0.3219752754296894559, 0.3333333333333333703, 0.3219752754296894559, 0.3333333333333333703, 0.3219752754296894559, 0.3333333333333333703, 0.3219752754296894559, 0.3333333333333333703, 0.3219752754296894559, 0.3333333333333333703, 0.3219752754296894559, 0.3333333333333333703, 0.3219752754296894559, 0.3333333333333333703, 0.3219752754296894559, 0.3333333333333333703, 0.3219752754296894559, 0.3333333333333333703, 0.3219752754296894559, 0.3333333333333333703, 0.3219752754296894559, 0.3333333333333333703, 0.3219752754296894559, 0.3333333333333333703, 0.3219752754296894559, 0.3333333333333333703, 0.3219752754296894559, 0.3333333333333333703, 0.3219752754296894559, 0.3333333333333333703, 0.3219752754296894559, 0.3333333333333333703, 0.3219752754296894559, 0.3333333333333333703, 0.3219752754296894559, 0.3333333333333333703, 0.3219752754296894559, 0.3333333333333333703, 0.3219752754296894559, 0.3333333333333333703, 0.3219752754296894559, 0.3333333333333333703, 0.3219752754296894559, 0.3333333333333333703, 0.3219752754296894559, 0.3333333333333333703, 0.3219752754296894559, 0.3333333333333333703, 0.3219752754296894559, 0.3333333333333333703, 0.3219752754296894559, 0.3333333333333333703, 0.3219752754296894559, 0.3333333333333333703, 0.3219752754296894559, 0.3333333333333333703, 0.3219752754296894559, 0.3333333333333333703, 0.3219752754296894559, 0.3333333333333333703, 0.3219752754296894559, 0.3333333333333333703, 0.3219752754296894559, 0.3333333333333333703, 0.3219752754296894559, 0.3333333333333333703, 0.3219752754296894559, 0.3333333333333333703, 0.3219752754296894559, 0.3333333333333333703, 0.3219752754296894559, 0.3333333333333333703, 0.3219752754296894559, 0.3333333333333333703, 0.3219752754296894559, 0.3333333333333333703, 0.3219752754296894559, 0.3333333333333333703, 0.3219752754296894559, 0.3333333333333333703, 0.3219752754296894559, 0.3333333333333333703, 0.3219752754296894559, 0.3333333333333333703, 0.3219752754296894559, 0.3333333333333333703, 0.3219752754296894559, 0.3333333333333333703, 0.3219752754296894559, 0.3333333333333333703, 0.3219752754296894559, 0.3333333333333333703, 0.3219752754296894559, 0.3333333333333333703, 0.3219752754296894559, 0.3333333333333333703, 0.3219752754296894559, 0.3333333333333333703, 0.3219752754296894559, 0.3333333333333333703, 0.3219752754296894559, 0.3333333333333333703, 0.3219752754296894559, 0.3333333333333333703, 0.3219752754296894559, 0.3333333333333333703, 0.3219752754296894559, 0.3333333333333333703, 0.3219752754296894559, 0.3333333333333333703, 0.3219752754296894559, 0.3333333333333333703, 0.3219752754296894559, 0.3333333333333333703, 0.3219752754296894559, 0.3333333333333333703, 0.3219752754296894559, 0.3333333333333333703, 0.3219752754296894559, 0.3333333333333333703, 0.3219752754296894559, 0.3333333333333333703, 0.3219752754296894559, 0.3333333333333333703, 0.3219752754296894559, 0.3333333333333333703, 0.3219752754296894559, 0.3333333333333333703, 0.3219752754296894559, 0.3333333333333333703, 0.3219752754296894559, 0.3333333333333333703, 0.3219752754296894559, 0.3333333333333333703, 0.3219752754296894559, 0.3333333333333333703, 0.3219752754296894559, 0.3333333333333333703, 0.3219752754296894559, 0.3333333333333333703, 0.3219752754296894559, 0.3333333333333333703, 0.3219752754296894559, 0.3333333333333333703, 0.3219752754296894559, 0.3333333333333333703, 0.3219752754296894559, 0.3333333333333333703, 0.3219752754296894559, 0.3333333333333333703, 0.3219752754296894559, 0.3333333333333333703, 0.3219752754296894559, 0.3333333333333333703, 0.3219752754296894559, 0.3333333333333333703, 0.3219752754296894559, 0.3333333333333333703, 0.3219752754296894559, 0.3333333333333333703, 0.3219752754296894559, 0.3333333333333333703, 0.3219752754296894559, 0.3333333333333333703, 0.3219752754296894559, 0.3333333333333333703, 0.3219752754296894559, 0.3333333333333333703, 0.3219752754296894559, 0.3333333333333333703, 0.3219752754296894559, 0.3333333333333333703, 0.3219752754296894559, 0.3333333333333333703, 0.3219752754296894559, 0.3333333333333333703, 0.3219752754296894559, 0.3333333333333333703, 0.3219752754296894559, 0.3333333333333333703, 0.3219752754296894559, 0.3333333333333333703, 0.3219752754296894559, 0.3333333333333333703, 0.3219752754296894559, 0.3333333333333333703, 0.3219752754296894559, 0.3333333333333333703, 0.3219752754296894559, 0.3333333333333333703, 0.3219752754296894559, 0.3333333333333333703, 0.3219752754296894559, 0.3333333333333333703, 0.3219752754296894559, 0.3333333333333333703, 0.3219752754296894559, 0.3333333333333333703, 0.3219752754296894559, 0.3333333333333333703, 0.3219752754296894559, 0.3333333333333333703, 0.3219752754296894559, 0.3333333333333333703, 0.3219752754296894559, 0.3333333333333333703, 0.3219752754296894559, 0.3333333333333333703, 0.3219752754296894559, 0.3333333333333333703, 0.3219752754296894559, 0.3333333333333333703, 0.3219752754296894559, 0.3333333333333333703, 0.3219752754296894559, 0.3333333333333333703, 0.3219752754296894559, 0.3333333333333333703, 0.3219752754296894559, 0.3333333333333333703, 0.3219752754296894559, 0.3333333333333333703, 0.3219752754296894559, 0.3333333333333333703, 0.3219752754296894559, 0.3333333333333333703, 0.3219752754296894559, 0.3333333333333333703, 0.3219752754296894559, 0.3333333333333333703, 0.3219752754296894559, 0.3333333333333333703, 0.3219752754296894559, 0.3333333333333333703, 0.3219752754296894559, 0.3333333333333333703, 0.3219752754296894559, 0.3333333333333333703, 0.3219752754296894559, 0.3333333333333333703, 0.3219752754296894559, 0.3333333333333333703, 0.3219752754296894559, 0.3333333333333333703, 0.3219752754296894559, 0.3333333333333333703, 0.3219752754296894559, 0.3333333333333333703, 0.3219752754296894559, 0.3333333333333333703, 0.3219752754296894559, 0.3333333333333333703, 0.3219752754296894559, 0.3333333333333333703, 0.3219752754296894559, 0.3333333333333333703, 0.3219752754296894559, 0.3333333333333333703, 0.3219752754296894559, 0.3333333333333333703, 0.3219752754296894559, 0.3333333333333333703, 0.3219752754296894559, 0.3333333333333333703, 0.3219752754296894559, 0.3333333333333333703, 0.3219752754296894559, 0.3333333333333333703, 0.3219752754296894559, 0.3333333333333333703, 0.3219752754296894559, 0.3333333333333333703, 0.3219752754296894559, 0.3333333333333333703, 0.3219752754296894559, 0.3333333333333333703, 0.3219752754296894559, 0.3333333333333333703, 0.3219752754296894559, 0.3333333333333333703, 0.3219752754296894559, 0.3333333333333333703, 0.3219752754296894559, 0.3333333333333333703, 0.3219752754296894559, 0.3333333333333333703, 0.3219752754296894559, 0.3333333333333333703, 0.3219752754296894559, 0.3333333333333333703, 0.3219752754296894559, 0.3333333333333333703, 0.3219752754296894559, 0.3333333333333333703, 0.3219752754296894559, 0.3333333333333333703, 0.3219752754296894559, 0.3333333333333333703, 0.3219752754296894559, 0.3333333333333333703, 0.3219752754296894559, 0.3333333333333333703, 0.3219752754296894559, 0.3333333333333333703, 0.3219752754296894559, 0.3333333333333333703, 0.3219752754296894559, 0.3333333333333333703, 0.3219752754296894559, 0.3333333333333333703, 0.3219752754296894559, 0.3333333333333333703, 0.3219752754296894559, 0.3333333333333333703, 0.3219752754296894559, 0.3333333333333333703),
 ( 0.3333333333333333703, 0.3219752754296894559, 0.3333333333333333703, 0.3219752754296894559, 0.3333333333333333703, 0.3219752754296894559, 0.3333333333333333703, 0.3219752754296894559, 0.3333333333333333703, 0.3219752754296894559, 0.3333333333333333703, 0.3219752754296894559, 0.3333333333333333703, 0.3219752754296894559, 0.3333333333333333703, 0.3219752754296894559, 0.3333333333333333703, 0.3219752754296894559, 0.3333333333333333703, 0.3219752754296894559, 0.3333333333333333703, 0.3219752754296894559, 0.3333333333333333703, 0.3219752754296894559, 0.3333333333333333703, 0.3219752754296894559, 0.3333333333333333703, 0.3219752754296894559, 0.3333333333333333703, 0.3219752754296894559, 0.3333333333333333703, 0.3219752754296894559, 0.3333333333333333703, 0.3219752754296894559, 0.3333333333333333703, 0.3219752754296894559, 0.3333333333333333703, 0.3219752754296894559, 0.3333333333333333703, 0.3219752754296894559, 0.3333333333333333703, 0.3219752754296894559, 0.3333333333333333703, 0.3219752754296894559, 0.3333333333333333703, 0.3219752754296894559, 0.3333333333333333703, 0.3219752754296894559, 0.3333333333333333703, 0.3219752754296894559, 0.3333333333333333703, 0.3219752754296894559, 0.3333333333333333703, 0.3219752754296894559, 0.3333333333333333703, 0.3219752754296894559, 0.3333333333333333703, 0.3219752754296894559, 0.3333333333333333703, 0.3219752754296894559, 0.3333333333333333703, 0.3219752754296894559, 0.3333333333333333703, 0.3219752754296894559, 0.3333333333333333703, 0.3219752754296894559, 0.3333333333333333703, 0.3219752754296894559, 0.3333333333333333703, 0.3219752754296894559, 0.3333333333333333703, 0.3219752754296894559, 0.3333333333333333703, 0.3219752754296894559, 0.3333333333333333703, 0.3219752754296894559, 0.3333333333333333703, 0.3219752754296894559, 0.3333333333333333703, 0.3219752754296894559, 0.3333333333333333703, 0.3219752754296894559, 0.3333333333333333703, 0.3219752754296894559, 0.3333333333333333703, 0.3219752754296894559, 0.3333333333333333703, 0.3219752754296894559, 0.3333333333333333703, 0.3219752754296894559, 0.3333333333333333703, 0.3219752754296894559, 0.3333333333333333703, 0.3219752754296894559, 0.3333333333333333703, 0.3219752754296894559, 0.3333333333333333703, 0.3219752754296894559, 0.3333333333333333703, 0.3219752754296894559, 0.3333333333333333703, 0.3219752754296894559, 0.3333333333333333703, 0.3219752754296894559, 0.3333333333333333703, 0.3219752754296894559, 0.3333333333333333703, 0.3219752754296894559, 0.3333333333333333703, 0.3219752754296894559, 0.3333333333333333703, 0.3219752754296894559, 0.3333333333333333703, 0.3219752754296894559, 0.3333333333333333703, 0.3219752754296894559, 0.3333333333333333703, 0.3219752754296894559, 0.3333333333333333703, 0.3219752754296894559, 0.3333333333333333703, 0.3219752754296894559, 0.3333333333333333703, 0.3219752754296894559, 0.3333333333333333703, 0.3219752754296894559, 0.3333333333333333703, 0.3219752754296894559, 0.3333333333333333703, 0.3219752754296894559, 0.3333333333333333703, 0.3219752754296894559, 0.3333333333333333703, 0.3219752754296894559, 0.3333333333333333703, 0.3219752754296894559, 0.3333333333333333703, 0.3219752754296894559, 0.3333333333333333703, 0.3219752754296894559, 0.3333333333333333703, 0.3219752754296894559, 0.3333333333333333703, 0.3219752754296894559, 0.3333333333333333703, 0.3219752754296894559, 0.3333333333333333703, 0.3219752754296894559, 0.3333333333333333703, 0.3219752754296894559, 0.3333333333333333703, 0.3219752754296894559, 0.3333333333333333703, 0.3219752754296894559, 0.3333333333333333703, 0.3219752754296894559, 0.3333333333333333703, 0.3219752754296894559, 0.3333333333333333703, 0.3219752754296894559, 0.3333333333333333703, 0.3219752754296894559, 0.3333333333333333703, 0.3219752754296894559, 0.3333333333333333703, 0.3219752754296894559, 0.3333333333333333703, 0.3219752754296894559, 0.3333333333333333703, 0.3219752754296894559, 0.3333333333333333703, 0.3219752754296894559, 0.3333333333333333703, 0.3219752754296894559, 0.3333333333333333703, 0.3219752754296894559, 0.3333333333333333703, 0.3219752754296894559, 0.3333333333333333703, 0.3219752754296894559, 0.3333333333333333703, 0.3219752754296894559, 0.3333333333333333703, 0.3219752754296894559, 0.3333333333333333703, 0.3219752754296894559, 0.3333333333333333703, 0.3219752754296894559, 0.3333333333333333703, 0.3219752754296894559, 0.3333333333333333703, 0.3219752754296894559, 0.3333333333333333703, 0.3219752754296894559, 0.3333333333333333703, 0.3219752754296894559, 0.3333333333333333703, 0.3219752754296894559, 0.3333333333333333703, 0.3219752754296894559, 0.3333333333333333703, 0.3219752754296894559, 0.3333333333333333703, 0.3219752754296894559, 0.3333333333333333703, 0.3219752754296894559, 0.3333333333333333703, 0.3219752754296894559, 0.3333333333333333703, 0.3219752754296894559, 0.3333333333333333703, 0.3219752754296894559, 0.3333333333333333703, 0.3219752754296894559, 0.3333333333333333703, 0.3219752754296894559, 0.3333333333333333703, 0.3219752754296894559, 0.3333333333333333703, 0.3219752754296894559, 0.3333333333333333703, 0.3219752754296894559, 0.3333333333333333703, 0.3219752754296894559, 0.3333333333333333703, 0.3219752754296894559, 0.3333333333333333703, 0.3219752754296894559, 0.3333333333333333703, 0.3219752754296894559, 0.3333333333333333703, 0.3219752754296894559, 0.3333333333333333703, 0.3219752754296894559, 0.3333333333333333703, 0.3219752754296894559, 0.3333333333333333703, 0.3219752754296894559, 0.3333333333333333703, 0.3219752754296894559, 0.3333333333333333703, 0.3219752754296894559, 0.3333333333333333703, 0.3219752754296894559, 0.3333333333333333703, 0.3219752754296894559, 0.3333333333333333703, 0.3219752754296894559, 0.3333333333333333703, 0.3219752754296894559, 0.3333333333333333703, 0.3219752754296894559, 0.3333333333333333703, 0.3219752754296894559, 0.3333333333333333703, 0.3219752754296894559, 0.3333333333333333703, 0.3219752754296894559, 0.3333333333333333703, 0.3219752754296894559, 0.3333333333333333703, 0.3219752754296894559, 0.3333333333333333703, 0.3219752754296894559, 0.3333333333333333703, 0.3219752754296894559, 0.3333333333333333703, 0.3219752754296894559, 0.3333333333333333703, 0.3219752754296894559, 0.3333333333333333703, 0.3219752754296894559, 0.3333333333333333703, 0.3219752754296894559, 0.3333333333333333703, 0.3219752754296894559, 0.3333333333333333703, 0.3219752754296894559, 0.3333333333333333703, 0.3219752754296894559, 0.3333333333333333703, 0.3219752754296894559, 0.3333333333333333703, 0.3219752754296894559, 0.3333333333333333703, 0.3219752754296894559, 0.3333333333333333703, 0.3219752754296894559, 0.3333333333333333703, 0.3219752754296894559, 0.3333333333333333703, 0.3219752754296894559, 0.3333333333333333703, 0.3219752754296894559, 0.3333333333333333703, 0.3219752754296894559, 0.3333333333333333703, 0.3219752754296894559, 0.3333333333333333703, 0.3219752754296894559, 0.3333333333333333703, 0.3219752754296894559, 0.3333333333333333703, 0.3219752754296894559, 0.3333333333333333703, 0.3219752754296894559, 0.3333333333333333703, 0.3219752754296894559, 0.3333333333333333703, 0.3219752754296894559, 0.3333333333333333703, 0.3219752754296894559, 0.3333333333333333703, 0.3219752754296894559, 0.3333333333333333703, 0.3219752754296894559, 0.3333333333333333703, 0.3219752754296894559, 0.3333333333333333703, 0.3219752754296894559, 0.3333333333333333703, 0.3219752754296894559, 0.3333333333333333703, 0.3219752754296894559, 0.3333333333333333703, 0.3219752754296894559, 0.3333333333333333703, 0.3219752754296894559, 0.3333333333333333703, 0.3219752754296894559, 0.3333333333333333703, 0.3219752754296894559, 0.3333333333333333703, 0.3219752754296894559, 0.3333333333333333703, 0.3219752754296894559, 0.3333333333333333703, 0.3219752754296894559, 0.3333333333333333703, 0.3219752754296894559, 0.3333333333333333703, 0.3219752754296894559, 0.3333333333333333703, 0.3219752754296894559, 0.3333333333333333703, 0.3219752754296894559, 0.3333333333333333703, 0.3219752754296894559, 0.3333333333333333703, 0.3219752754296894559, 0.3333333333333333703, 0.3219752754296894559, 0.3333333333333333703, 0.3219752754296894559, 0.3333333333333333703, 0.3219752754296894559, 0.3333333333333333703, 0.3219752754296894559, 0.3333333333333333703, 0.3219752754296894559, 0.3333333333333333703, 0.3219752754296894559, 0.3333333333333333703, 0.3219752754296894559, 0.3333333333333333703, 0.3219752754296894559, 0.3333333333333333703, 0.3219752754296894559, 0.3333333333333333703, 0.3219752754296894559, 0.3333333333333333703, 0.3219752754296894559, 0.3333333333333333703, 0.3219752754296894559, 0.3333333333333333703, 0.3219752754296894559, 0.3333333333333333703, 0.3219752754296894559, 0.3333333333333333703, 0.3219752754296894559, 0.3333333333333333703, 0.3219752754296894559, 0.3333333333333333703, 0.3219752754296894559, 0.3333333333333333703, 0.3219752754296894559, 0.3333333333333333703, 0.3219752754296894559, 0.3333333333333333703, 0.3219752754296894559, 0.3333333333333333703, 0.3219752754296894559, 0.3333333333333333703, 0.3219752754296894559, 0.3333333333333333703, 0.3219752754296894559, 0.3333333333333333703, 0.3219752754296894559, 0.3333333333333333703, 0.3219752754296894559, 0.3333333333333333703, 0.3219752754296894559, 0.3333333333333333703, 0.3219752754296894559, 0.3333333333333333703, 0.3219752754296894559, 0.3333333333333333703, 0.3219752754296894559, 0.3333333333333333703, 0.3219752754296894559, 0.3333333333333333703, 0.3219752754296894559, 0.3333333333333333703, 0.3219752754296894559, 0.3333333333333333703, 0.3219752754296894559, 0.3333333333333333703, 0.3219752754296894559, 0.3333333333333333703, 0.3219752754296894559, 0.3333333333333333703, 0.3219752754296894559, 0.3333333333333333703, 0.3219752754296894559, 0.3333333333333333703, 0.3219752754296894559, 0.3333333333333333703, 0.3219752754296894559, 0.3333333333333333703, 0.3219752754296894559, 0.3333333333333333703, 0.3219752754296894559, 0.3333333333333333703, 0.3219752754296894559, 0.3333333333333333703, 0.3219752754296894559, 0.3333333333333333703, 0.3219752754296894559, 0.3333333333333333703, 0.3219752754296894559, 0.3333333333333333703, 0.3219752754296894559, 0.3333333333333333703, 0.3219752754296894559, 0.3333333333333333703, 0.3219752754296894559, 0.3333333333333333703, 0.3219752754296894559, 0.3333333333333333703, 0.3219752754296894559, 0.3333333333333333703, 0.3219752754296894559, 0.3333333333333333703, 0.3219752754296894559, 0.3333333333333333703, 0.3219752754296894559, 0.3333333333333333703),
 ( 1.000000000000000000, 0.9659258262890683122, 1.000000000000000000, 0.9659258262890683122, 1.000000000000000000, 0.9659258262890683122, 1.000000000000000000, 0.9659258262890683122, 1.000000000000000000, 0.9659258262890683122, 1.000000000000000000, 0.9659258262890683122, 1.000000000000000000, 0.9659258262890683122, 1.000000000000000000, 0.9659258262890683122, 1.000000000000000000, 0.9659258262890683122, 1.000000000000000000, 0.9659258262890683122, 1.000000000000000000, 0.9659258262890683122, 1.000000000000000000, 0.9659258262890683122, 1.000000000000000000, 0.9659258262890683122, 1.000000000000000000, 0.9659258262890683122, 1.000000000000000000, 0.9659258262890683122, 1.000000000000000000, 0.9659258262890683122, 1.000000000000000000, 0.9659258262890683122, 1.000000000000000000, 0.9659258262890683122, 1.000000000000000000, 0.9659258262890683122, 1.000000000000000000, 0.9659258262890683122, 1.000000000000000000, 0.9659258262890683122, 1.000000000000000000, 0.9659258262890683122, 1.000000000000000000, 0.9659258262890683122, 1.000000000000000000, 0.9659258262890683122, 1.000000000000000000, 0.9659258262890683122, 1.000000000000000000, 0.9659258262890683122, 1.000000000000000000, 0.9659258262890683122, 1.000000000000000000, 0.9659258262890683122, 1.000000000000000000, 0.9659258262890683122, 1.000000000000000000, 0.9659258262890683122, 1.000000000000000000, 0.9659258262890683122, 1.000000000000000000, 0.9659258262890683122, 1.000000000000000000, 0.9659258262890683122, 1.000000000000000000, 0.9659258262890683122, 1.000000000000000000, 0.9659258262890683122, 1.000000000000000000, 0.9659258262890683122, 1.000000000000000000, 0.9659258262890683122, 1.000000000000000000, 0.9659258262890683122, 1.000000000000000000, 0.9659258262890683122, 1.000000000000000000, 0.9659258262890683122, 1.000000000000000000, 0.9659258262890683122, 1.000000000000000000, 0.9659258262890683122, 1.000000000000000000, 0.9659258262890683122, 1.000000000000000000, 0.9659258262890683122, 1.000000000000000000, 0.9659258262890683122, 1.000000000000000000, 0.9659258262890683122, 1.000000000000000000, 0.9659258262890683122, 1.000000000000000000, 0.9659258262890683122, 1.000000000000000000, 0.9659258262890683122, 1.000000000000000000, 0.9659258262890683122, 1.000000000000000000, 0.9659258262890683122, 1.000000000000000000, 0.9659258262890683122, 1.000000000000000000, 0.9659258262890683122, 1.000000000000000000, 0.9659258262890683122, 1.000000000000000000, 0.9659258262890683122, 1.000000000000000000, 0.9659258262890683122, 1.000000000000000000, 0.9659258262890683122, 1.000000000000000000, 0.9659258262890683122, 1.000000000000000000, 0.9659258262890683122, 1.000000000000000000, 0.9659258262890683122, 1.000000000000000000, 0.9659258262890683122, 1.000000000000000000, 0.9659258262890683122, 1.000000000000000000, 0.9659258262890683122, 1.000000000000000000, 0.9659258262890683122, 1.000000000000000000, 0.9659258262890683122, 1.000000000000000000, 0.9659258262890683122, 1.000000000000000000, 0.9659258262890683122, 1.000000000000000000, 0.9659258262890683122, 1.000000000000000000, 0.9659258262890683122, 1.000000000000000000, 0.9659258262890683122, 1.000000000000000000, 0.9659258262890683122, 1.000000000000000000, 0.9659258262890683122, 1.000000000000000000, 0.9659258262890683122, 1.000000000000000000, 0.9659258262890683122, 1.000000000000000000, 0.9659258262890683122, 1.000000000000000000, 0.9659258262890683122, 1.000000000000000000, 0.9659258262890683122, 1.000000000000000000, 0.9659258262890683122, 1.000000000000000000, 0.9659258262890683122, 1.000000000000000000, 0.9659258262890683122, 1.000000000000000000, 0.9659258262890683122, 1.000000000000000000, 0.9659258262890683122, 1.000000000000000000, 0.9659258262890683122, 1.000000000000000000, 0.9659258262890683122, 1.000000000000000000, 0.9659258262890683122, 1.000000000000000000, 0.9659258262890683122, 1.000000000000000000, 0.9659258262890683122, 1.000000000000000000, 0.9659258262890683122, 1.000000000000000000, 0.9659258262890683122, 1.000000000000000000, 0.9659258262890683122, 1.000000000000000000, 0.9659258262890683122, 1.000000000000000000, 0.9659258262890683122, 1.000000000000000000, 0.9659258262890683122, 1.000000000000000000, 0.9659258262890683122, 1.000000000000000000, 0.9659258262890683122, 1.000000000000000000, 0.9659258262890683122, 1.000000000000000000, 0.9659258262890683122, 1.000000000000000000, 0.9659258262890683122, 1.000000000000000000, 0.9659258262890683122, 1.000000000000000000, 0.9659258262890683122, 1.000000000000000000, 0.9659258262890683122, 1.000000000000000000, 0.9659258262890683122, 1.000000000000000000, 0.9659258262890683122, 1.000000000000000000, 0.9659258262890683122, 1.000000000000000000, 0.9659258262890683122, 1.000000000000000000, 0.9659258262890683122, 1.000000000000000000, 0.9659258262890683122, 1.000000000000000000, 0.9659258262890683122, 1.000000000000000000, 0.9659258262890683122, 1.000000000000000000, 0.9659258262890683122, 1.000000000000000000, 0.9659258262890683122, 1.000000000000000000, 0.9659258262890683122, 1.000000000000000000, 0.9659258262890683122, 1.000000000000000000, 0.9659258262890683122, 1.000000000000000000, 0.9659258262890683122, 1.000000000000000000, 0.9659258262890683122, 1.000000000000000000, 0.9659258262890683122, 1.000000000000000000, 0.9659258262890683122, 1.000000000000000000, 0.9659258262890683122, 1.000000000000000000, 0.9659258262890683122, 1.000000000000000000, 0.9659258262890683122, 1.000000000000000000, 0.9659258262890683122, 1.000000000000000000, 0.9659258262890683122, 1.000000000000000000, 0.9659258262890683122, 1.000000000000000000, 0.9659258262890683122, 1.000000000000000000, 0.9659258262890683122, 1.000000000000000000, 0.9659258262890683122, 1.000000000000000000, 0.9659258262890683122, 1.000000000000000000, 0.9659258262890683122, 1.000000000000000000, 0.9659258262890683122, 1.000000000000000000, 0.9659258262890683122, 1.000000000000000000, 0.9659258262890683122, 1.000000000000000000, 0.9659258262890683122, 1.000000000000000000, 0.9659258262890683122, 1.000000000000000000, 0.9659258262890683122, 1.000000000000000000, 0.9659258262890683122, 1.000000000000000000, 0.9659258262890683122, 1.000000000000000000, 0.9659258262890683122, 1.000000000000000000, 0.9659258262890683122, 1.000000000000000000, 0.9659258262890683122, 1.000000000000000000, 0.9659258262890683122, 1.000000000000000000, 0.9659258262890683122, 1.000000000000000000, 0.9659258262890683122, 1.000000000000000000, 0.9659258262890683122, 1.000000000000000000, 0.9659258262890683122, 1.000000000000000000, 0.9659258262890683122, 1.000000000000000000, 0.9659258262890683122, 1.000000000000000000, 0.9659258262890683122, 1.000000000000000000, 0.9659258262890683122, 1.000000000000000000, 0.9659258262890683122, 1.000000000000000000, 0.9659258262890683122, 1.000000000000000000, 0.9659258262890683122, 1.000000000000000000, 0.9659258262890683122, 1.000000000000000000, 0.9659258262890683122, 1.000000000000000000, 0.9659258262890683122, 1.000000000000000000, 0.9659258262890683122, 1.000000000000000000, 0.9659258262890683122, 1.000000000000000000, 0.9659258262890683122, 1.000000000000000000, 0.9659258262890683122, 1.000000000000000000, 0.9659258262890683122, 1.000000000000000000, 0.9659258262890683122, 1.000000000000000000, 0.9659258262890683122, 1.000000000000000000, 0.9659258262890683122, 1.000000000000000000, 0.9659258262890683122, 1.000000000000000000, 0.9659258262890683122, 1.000000000000000000, 0.9659258262890683122, 1.000000000000000000, 0.9659258262890683122, 1.000000000000000000, 0.9659258262890683122, 1.000000000000000000, 0.9659258262890683122, 1.000000000000000000, 0.9659258262890683122, 1.000000000000000000, 0.9659258262890683122, 1.000000000000000000, 0.9659258262890683122, 1.000000000000000000, 0.9659258262890683122, 1.000000000000000000, 0.9659258262890683122, 1.000000000000000000, 0.9659258262890683122, 1.000000000000000000, 0.9659258262890683122, 1.000000000000000000, 0.9659258262890683122, 1.000000000000000000, 0.9659258262890683122, 1.000000000000000000, 0.9659258262890683122, 1.000000000000000000, 0.9659258262890683122, 1.000000000000000000, 0.9659258262890683122, 1.000000000000000000, 0.9659258262890683122, 1.000000000000000000, 0.9659258262890683122, 1.000000000000000000, 0.9659258262890683122, 1.000000000000000000, 0.9659258262890683122, 1.000000000000000000, 0.9659258262890683122, 1.000000000000000000, 0.9659258262890683122, 1.000000000000000000, 0.9659258262890683122, 1.000000000000000000, 0.9659258262890683122, 1.000000000000000000, 0.9659258262890683122, 1.000000000000000000, 0.9659258262890683122, 1.000000000000000000, 0.9659258262890683122, 1.000000000000000000, 0.9659258262890683122, 1.000000000000000000, 0.9659258262890683122, 1.000000000000000000, 0.9659258262890683122, 1.000000000000000000, 0.9659258262890683122, 1.000000000000000000, 0.9659258262890683122, 1.000000000000000000, 0.9659258262890683122, 1.000000000000000000, 0.9659258262890683122, 1.000000000000000000, 0.9659258262890683122, 1.000000000000000000, 0.9659258262890683122, 1.000000000000000000, 0.9659258262890683122, 1.000000000000000000, 0.9659258262890683122, 1.000000000000000000, 0.9659258262890683122, 1.000000000000000000, 0.9659258262890683122, 1.000000000000000000, 0.9659258262890683122, 1.000000000000000000, 0.9659258262890683122, 1.000000000000000000, 0.9659258262890683122, 1.000000000000000000, 0.9659258262890683122, 1.000000000000000000, 0.9659258262890683122, 1.000000000000000000, 0.9659258262890683122, 1.000000000000000000, 0.9659258262890683122, 1.000000000000000000, 0.9659258262890683122, 1.000000000000000000, 0.9659258262890683122, 1.000000000000000000, 0.9659258262890683122, 1.000000000000000000, 0.9659258262890683122, 1.000000000000000000, 0.9659258262890683122, 1.000000000000000000, 0.9659258262890683122, 1.000000000000000000, 0.9659258262890683122, 1.000000000000000000, 0.9659258262890683122, 1.000000000000000000, 0.9659258262890683122, 1.000000000000000000, 0.9659258262890683122, 1.000000000000000000, 0.9659258262890683122, 1.000000000000000000, 0.9659258262890683122, 1.000000000000000000, 0.9659258262890683122, 1.000000000000000000, 0.9659258262890683122, 1.000000000000000000, 0.9659258262890683122, 1.000000000000000000, 0.9659258262890683122, 1.000000000000000000),
 ( 0.3333333333333333703, 0.3219752754296894559, 0.3333333333333333703, 0.3219752754296894559, 0.3333333333333333703, 0.3219752754296894559, 0.3333333333333333703, 0.3219752754296894559, 0.3333333333333333703, 0.3219752754296894559, 0.3333333333333333703, 0.3219752754296894559, 0.3333333333333333703, 0.3219752754296894559, 0.3333333333333333703, 0.3219752754296894559, 0.3333333333333333703, 0.3219752754296894559, 0.3333333333333333703, 0.3219752754296894559, 0.3333333333333333703, 0.3219752754296894559, 0.3333333333333333703, 0.3219752754296894559, 0.3333333333333333703, 0.3219752754296894559, 0.3333333333333333703, 0.3219752754296894559, 0.3333333333333333703, 0.3219752754296894559, 0.3333333333333333703, 0.3219752754296894559, 0.3333333333333333703, 0.3219752754296894559, 0.3333333333333333703, 0.3219752754296894559, 0.3333333333333333703, 0.3219752754296894559, 0.3333333333333333703, 0.3219752754296894559, 0.3333333333333333703, 0.3219752754296894559, 0.3333333333333333703, 0.3219752754296894559, 0.3333333333333333703, 0.3219752754296894559, 0.3333333333333333703, 0.3219752754296894559, 0.3333333333333333703, 0.3219752754296894559, 0.3333333333333333703, 0.3219752754296894559, 0.3333333333333333703, 0.3219752754296894559, 0.3333333333333333703, 0.3219752754296894559, 0.3333333333333333703, 0.3219752754296894559, 0.3333333333333333703, 0.3219752754296894559, 0.3333333333333333703, 0.3219752754296894559, 0.3333333333333333703, 0.3219752754296894559, 0.3333333333333333703, 0.3219752754296894559, 0.3333333333333333703, 0.3219752754296894559, 0.3333333333333333703, 0.3219752754296894559, 0.3333333333333333703, 0.3219752754296894559, 0.3333333333333333703, 0.3219752754296894559, 0.3333333333333333703, 0.3219752754296894559, 0.3333333333333333703, 0.3219752754296894559, 0.3333333333333333703, 0.3219752754296894559, 0.3333333333333333703, 0.3219752754296894559, 0.3333333333333333703, 0.3219752754296894559, 0.3333333333333333703, 0.3219752754296894559, 0.3333333333333333703, 0.3219752754296894559, 0.3333333333333333703, 0.3219752754296894559, 0.3333333333333333703, 0.3219752754296894559, 0.3333333333333333703, 0.3219752754296894559, 0.3333333333333333703, 0.3219752754296894559, 0.3333333333333333703, 0.3219752754296894559, 0.3333333333333333703, 0.3219752754296894559, 0.3333333333333333703, 0.3219752754296894559, 0.3333333333333333703, 0.3219752754296894559, 0.3333333333333333703, 0.3219752754296894559, 0.3333333333333333703, 0.3219752754296894559, 0.3333333333333333703, 0.3219752754296894559, 0.3333333333333333703, 0.3219752754296894559, 0.3333333333333333703, 0.3219752754296894559, 0.3333333333333333703, 0.3219752754296894559, 0.3333333333333333703, 0.3219752754296894559, 0.3333333333333333703, 0.3219752754296894559, 0.3333333333333333703, 0.3219752754296894559, 0.3333333333333333703, 0.3219752754296894559, 0.3333333333333333703, 0.3219752754296894559, 0.3333333333333333703, 0.3219752754296894559, 0.3333333333333333703, 0.3219752754296894559, 0.3333333333333333703, 0.3219752754296894559, 0.3333333333333333703, 0.3219752754296894559, 0.3333333333333333703, 0.3219752754296894559, 0.3333333333333333703, 0.3219752754296894559, 0.3333333333333333703, 0.3219752754296894559, 0.3333333333333333703, 0.3219752754296894559, 0.3333333333333333703, 0.3219752754296894559, 0.3333333333333333703, 0.3219752754296894559, 0.3333333333333333703, 0.3219752754296894559, 0.3333333333333333703, 0.3219752754296894559, 0.3333333333333333703, 0.3219752754296894559, 0.3333333333333333703, 0.3219752754296894559, 0.3333333333333333703, 0.3219752754296894559, 0.3333333333333333703, 0.3219752754296894559, 0.3333333333333333703, 0.3219752754296894559, 0.3333333333333333703, 0.3219752754296894559, 0.3333333333333333703, 0.3219752754296894559, 0.3333333333333333703, 0.3219752754296894559, 0.3333333333333333703, 0.3219752754296894559, 0.3333333333333333703, 0.3219752754296894559, 0.3333333333333333703, 0.3219752754296894559, 0.3333333333333333703, 0.3219752754296894559, 0.3333333333333333703, 0.3219752754296894559, 0.3333333333333333703, 0.3219752754296894559, 0.3333333333333333703, 0.3219752754296894559, 0.3333333333333333703, 0.3219752754296894559, 0.3333333333333333703, 0.3219752754296894559, 0.3333333333333333703, 0.3219752754296894559, 0.3333333333333333703, 0.3219752754296894559, 0.3333333333333333703, 0.3219752754296894559, 0.3333333333333333703, 0.3219752754296894559, 0.3333333333333333703, 0.3219752754296894559, 0.3333333333333333703, 0.3219752754296894559, 0.3333333333333333703, 0.3219752754296894559, 0.3333333333333333703, 0.3219752754296894559, 0.3333333333333333703, 0.3219752754296894559, 0.3333333333333333703, 0.3219752754296894559, 0.3333333333333333703, 0.3219752754296894559, 0.3333333333333333703, 0.3219752754296894559, 0.3333333333333333703, 0.3219752754296894559, 0.3333333333333333703, 0.3219752754296894559, 0.3333333333333333703, 0.3219752754296894559, 0.3333333333333333703, 0.3219752754296894559, 0.3333333333333333703, 0.3219752754296894559, 0.3333333333333333703, 0.3219752754296894559, 0.3333333333333333703, 0.3219752754296894559, 0.3333333333333333703, 0.3219752754296894559, 0.3333333333333333703, 0.3219752754296894559, 0.3333333333333333703, 0.3219752754296894559, 0.3333333333333333703, 0.3219752754296894559, 0.3333333333333333703, 0.3219752754296894559, 0.3333333333333333703, 0.3219752754296894559, 0.3333333333333333703, 0.3219752754296894559, 0.3333333333333333703, 0.3219752754296894559, 0.3333333333333333703, 0.3219752754296894559, 0.3333333333333333703, 0.3219752754296894559, 0.3333333333333333703, 0.3219752754296894559, 0.3333333333333333703, 0.3219752754296894559, 0.3333333333333333703, 0.3219752754296894559, 0.3333333333333333703, 0.3219752754296894559, 0.3333333333333333703, 0.3219752754296894559, 0.3333333333333333703, 0.3219752754296894559, 0.3333333333333333703, 0.3219752754296894559, 0.3333333333333333703, 0.3219752754296894559, 0.3333333333333333703, 0.3219752754296894559, 0.3333333333333333703, 0.3219752754296894559, 0.3333333333333333703, 0.3219752754296894559, 0.3333333333333333703, 0.3219752754296894559, 0.3333333333333333703, 0.3219752754296894559, 0.3333333333333333703, 0.3219752754296894559, 0.3333333333333333703, 0.3219752754296894559, 0.3333333333333333703, 0.3219752754296894559, 0.3333333333333333703, 0.3219752754296894559, 0.3333333333333333703, 0.3219752754296894559, 0.3333333333333333703, 0.3219752754296894559, 0.3333333333333333703, 0.3219752754296894559, 0.3333333333333333703, 0.3219752754296894559, 0.3333333333333333703, 0.3219752754296894559, 0.3333333333333333703, 0.3219752754296894559, 0.3333333333333333703, 0.3219752754296894559, 0.3333333333333333703, 0.3219752754296894559, 0.3333333333333333703, 0.3219752754296894559, 0.3333333333333333703, 0.3219752754296894559, 0.3333333333333333703, 0.3219752754296894559, 0.3333333333333333703, 0.3219752754296894559, 0.3333333333333333703, 0.3219752754296894559, 0.3333333333333333703, 0.3219752754296894559, 0.3333333333333333703, 0.3219752754296894559, 0.3333333333333333703, 0.3219752754296894559, 0.3333333333333333703, 0.3219752754296894559, 0.3333333333333333703, 0.3219752754296894559, 0.3333333333333333703, 0.3219752754296894559, 0.3333333333333333703, 0.3219752754296894559, 0.3333333333333333703, 0.3219752754296894559, 0.3333333333333333703, 0.3219752754296894559, 0.3333333333333333703, 0.3219752754296894559, 0.3333333333333333703, 0.3219752754296894559, 0.3333333333333333703, 0.3219752754296894559, 0.3333333333333333703, 0.3219752754296894559, 0.3333333333333333703, 0.3219752754296894559, 0.3333333333333333703, 0.3219752754296894559, 0.3333333333333333703, 0.3219752754296894559, 0.3333333333333333703, 0.3219752754296894559, 0.3333333333333333703, 0.3219752754296894559, 0.3333333333333333703, 0.3219752754296894559, 0.3333333333333333703, 0.3219752754296894559, 0.3333333333333333703, 0.3219752754296894559, 0.3333333333333333703, 0.3219752754296894559, 0.3333333333333333703, 0.3219752754296894559, 0.3333333333333333703, 0.3219752754296894559, 0.3333333333333333703, 0.3219752754296894559, 0.3333333333333333703, 0.3219752754296894559, 0.3333333333333333703, 0.3219752754296894559, 0.3333333333333333703, 0.3219752754296894559, 0.3333333333333333703, 0.3219752754296894559, 0.3333333333333333703, 0.3219752754296894559, 0.3333333333333333703, 0.3219752754296894559, 0.3333333333333333703, 0.3219752754296894559, 0.3333333333333333703, 0.3219752754296894559, 0.3333333333333333703, 0.3219752754296894559, 0.3333333333333333703, 0.3219752754296894559, 0.3333333333333333703, 0.3219752754296894559, 0.3333333333333333703, 0.3219752754296894559, 0.3333333333333333703, 0.3219752754296894559, 0.3333333333333333703, 0.3219752754296894559, 0.3333333333333333703, 0.3219752754296894559, 0.3333333333333333703, 0.3219752754296894559, 0.3333333333333333703, 0.3219752754296894559, 0.3333333333333333703, 0.3219752754296894559, 0.3333333333333333703, 0.3219752754296894559, 0.3333333333333333703, 0.3219752754296894559, 0.3333333333333333703, 0.3219752754296894559, 0.3333333333333333703, 0.3219752754296894559, 0.3333333333333333703, 0.3219752754296894559, 0.3333333333333333703, 0.3219752754296894559, 0.3333333333333333703, 0.3219752754296894559, 0.3333333333333333703, 0.3219752754296894559, 0.3333333333333333703, 0.3219752754296894559, 0.3333333333333333703, 0.3219752754296894559, 0.3333333333333333703, 0.3219752754296894559, 0.3333333333333333703, 0.3219752754296894559, 0.3333333333333333703, 0.3219752754296894559, 0.3333333333333333703, 0.3219752754296894559, 0.3333333333333333703, 0.3219752754296894559, 0.3333333333333333703, 0.3219752754296894559, 0.3333333333333333703, 0.3219752754296894559, 0.3333333333333333703, 0.3219752754296894559, 0.3333333333333333703, 0.3219752754296894559, 0.3333333333333333703, 0.3219752754296894559, 0.3333333333333333703, 0.3219752754296894559, 0.3333333333333333703, 0.3219752754296894559, 0.3333333333333333703, 0.3219752754296894559, 0.3333333333333333703, 0.3219752754296894559, 0.3333333333333333703, 0.3219752754296894559, 0.3333333333333333703, 0.3219752754296894559, 0.3333333333333333703, 0.3219752754296894559, 0.3333333333333333703, 0.3219752754296894559, 0.3333333333333333703, 0.3219752754296894559, 0.3333333333333333703, 0.3219752754296894559, 0.3333333333333333703, 0.3219752754296894559, 0.3333333333333333703, 0.3219752754296894559, 0.3333333333333333703, 0.3219752754296894559, 0.3333333333333333703, 0.3219752754296894559, 0.3333333333333333703),
 ( 0.3333333333333333703, 0.3219752754296894559, 0.3333333333333333703, 0.3219752754296894559, 0.3333333333333333703, 0.3219752754296894559, 0.3333333333333333703, 0.3219752754296894559, 0.3333333333333333703, 0.3219752754296894559, 0.3333333333333333703, 0.3219752754296894559, 0.3333333333333333703, 0.3219752754296894559, 0.3333333333333333703, 0.3219752754296894559, 0.3333333333333333703, 0.3219752754296894559, 0.3333333333333333703, 0.3219752754296894559, 0.3333333333333333703, 0.3219752754296894559, 0.3333333333333333703, 0.3219752754296894559, 0.3333333333333333703, 0.3219752754296894559, 0.3333333333333333703, 0.3219752754296894559, 0.3333333333333333703, 0.3219752754296894559, 0.3333333333333333703, 0.3219752754296894559, 0.3333333333333333703, 0.3219752754296894559, 0.3333333333333333703, 0.3219752754296894559, 0.3333333333333333703, 0.3219752754296894559, 0.3333333333333333703, 0.3219752754296894559, 0.3333333333333333703, 0.3219752754296894559, 0.3333333333333333703, 0.3219752754296894559, 0.3333333333333333703, 0.3219752754296894559, 0.3333333333333333703, 0.3219752754296894559, 0.3333333333333333703, 0.3219752754296894559, 0.3333333333333333703, 0.3219752754296894559, 0.3333333333333333703, 0.3219752754296894559, 0.3333333333333333703, 0.3219752754296894559, 0.3333333333333333703, 0.3219752754296894559, 0.3333333333333333703, 0.3219752754296894559, 0.3333333333333333703, 0.3219752754296894559, 0.3333333333333333703, 0.3219752754296894559, 0.3333333333333333703, 0.3219752754296894559, 0.3333333333333333703, 0.3219752754296894559, 0.3333333333333333703, 0.3219752754296894559, 0.3333333333333333703, 0.3219752754296894559, 0.3333333333333333703, 0.3219752754296894559, 0.3333333333333333703, 0.3219752754296894559, 0.3333333333333333703, 0.3219752754296894559, 0.3333333333333333703, 0.3219752754296894559, 0.3333333333333333703, 0.3219752754296894559, 0.3333333333333333703, 0.3219752754296894559, 0.3333333333333333703, 0.3219752754296894559, 0.3333333333333333703, 0.3219752754296894559, 0.3333333333333333703, 0.3219752754296894559, 0.3333333333333333703, 0.3219752754296894559, 0.3333333333333333703, 0.3219752754296894559, 0.3333333333333333703, 0.3219752754296894559, 0.3333333333333333703, 0.3219752754296894559, 0.3333333333333333703, 0.3219752754296894559, 0.3333333333333333703, 0.3219752754296894559, 0.3333333333333333703, 0.3219752754296894559, 0.3333333333333333703, 0.3219752754296894559, 0.3333333333333333703, 0.3219752754296894559, 0.3333333333333333703, 0.3219752754296894559, 0.3333333333333333703, 0.3219752754296894559, 0.3333333333333333703, 0.3219752754296894559, 0.3333333333333333703, 0.3219752754296894559, 0.3333333333333333703, 0.3219752754296894559, 0.3333333333333333703, 0.3219752754296894559, 0.3333333333333333703, 0.3219752754296894559, 0.3333333333333333703, 0.3219752754296894559, 0.3333333333333333703, 0.3219752754296894559, 0.3333333333333333703, 0.3219752754296894559, 0.3333333333333333703, 0.3219752754296894559, 0.3333333333333333703, 0.3219752754296894559, 0.3333333333333333703, 0.3219752754296894559, 0.3333333333333333703, 0.3219752754296894559, 0.3333333333333333703, 0.3219752754296894559, 0.3333333333333333703, 0.3219752754296894559, 0.3333333333333333703, 0.3219752754296894559, 0.3333333333333333703, 0.3219752754296894559, 0.3333333333333333703, 0.3219752754296894559, 0.3333333333333333703, 0.3219752754296894559, 0.3333333333333333703, 0.3219752754296894559, 0.3333333333333333703, 0.3219752754296894559, 0.3333333333333333703, 0.3219752754296894559, 0.3333333333333333703, 0.3219752754296894559, 0.3333333333333333703, 0.3219752754296894559, 0.3333333333333333703, 0.3219752754296894559, 0.3333333333333333703, 0.3219752754296894559, 0.3333333333333333703, 0.3219752754296894559, 0.3333333333333333703, 0.3219752754296894559, 0.3333333333333333703, 0.3219752754296894559, 0.3333333333333333703, 0.3219752754296894559, 0.3333333333333333703, 0.3219752754296894559, 0.3333333333333333703, 0.3219752754296894559, 0.3333333333333333703, 0.3219752754296894559, 0.3333333333333333703, 0.3219752754296894559, 0.3333333333333333703, 0.3219752754296894559, 0.3333333333333333703, 0.3219752754296894559, 0.3333333333333333703, 0.3219752754296894559, 0.3333333333333333703, 0.3219752754296894559, 0.3333333333333333703, 0.3219752754296894559, 0.3333333333333333703, 0.3219752754296894559, 0.3333333333333333703, 0.3219752754296894559, 0.3333333333333333703, 0.3219752754296894559, 0.3333333333333333703, 0.3219752754296894559, 0.3333333333333333703, 0.3219752754296894559, 0.3333333333333333703, 0.3219752754296894559, 0.3333333333333333703, 0.3219752754296894559, 0.3333333333333333703, 0.3219752754296894559, 0.3333333333333333703, 0.3219752754296894559, 0.3333333333333333703, 0.3219752754296894559, 0.3333333333333333703, 0.3219752754296894559, 0.3333333333333333703, 0.3219752754296894559, 0.3333333333333333703, 0.3219752754296894559, 0.3333333333333333703, 0.3219752754296894559, 0.3333333333333333703, 0.3219752754296894559, 0.3333333333333333703, 0.3219752754296894559, 0.3333333333333333703, 0.3219752754296894559, 0.3333333333333333703, 0.3219752754296894559, 0.3333333333333333703, 0.3219752754296894559, 0.3333333333333333703, 0.3219752754296894559, 0.3333333333333333703, 0.3219752754296894559, 0.3333333333333333703, 0.3219752754296894559, 0.3333333333333333703, 0.3219752754296894559, 0.3333333333333333703, 0.3219752754296894559, 0.3333333333333333703, 0.3219752754296894559, 0.3333333333333333703, 0.3219752754296894559, 0.3333333333333333703, 0.3219752754296894559, 0.3333333333333333703, 0.3219752754296894559, 0.3333333333333333703, 0.3219752754296894559, 0.3333333333333333703, 0.3219752754296894559, 0.3333333333333333703, 0.3219752754296894559, 0.3333333333333333703, 0.3219752754296894559, 0.3333333333333333703, 0.3219752754296894559, 0.3333333333333333703, 0.3219752754296894559, 0.3333333333333333703, 0.3219752754296894559, 0.3333333333333333703, 0.3219752754296894559, 0.3333333333333333703, 0.3219752754296894559, 0.3333333333333333703, 0.3219752754296894559, 0.3333333333333333703, 0.3219752754296894559, 0.3333333333333333703, 0.3219752754296894559, 0.3333333333333333703, 0.3219752754296894559, 0.3333333333333333703, 0.3219752754296894559, 0.3333333333333333703, 0.3219752754296894559, 0.3333333333333333703, 0.3219752754296894559, 0.3333333333333333703, 0.3219752754296894559, 0.3333333333333333703, 0.3219752754296894559, 0.3333333333333333703, 0.3219752754296894559, 0.3333333333333333703, 0.3219752754296894559, 0.3333333333333333703, 0.3219752754296894559, 0.3333333333333333703, 0.3219752754296894559, 0.3333333333333333703, 0.3219752754296894559, 0.3333333333333333703, 0.3219752754296894559, 0.3333333333333333703, 0.3219752754296894559, 0.3333333333333333703, 0.3219752754296894559, 0.3333333333333333703, 0.3219752754296894559, 0.3333333333333333703, 0.3219752754296894559, 0.3333333333333333703, 0.3219752754296894559, 0.3333333333333333703, 0.3219752754296894559, 0.3333333333333333703, 0.3219752754296894559, 0.3333333333333333703, 0.3219752754296894559, 0.3333333333333333703, 0.3219752754296894559, 0.3333333333333333703, 0.3219752754296894559, 0.3333333333333333703, 0.3219752754296894559, 0.3333333333333333703, 0.3219752754296894559, 0.3333333333333333703, 0.3219752754296894559, 0.3333333333333333703, 0.3219752754296894559, 0.3333333333333333703, 0.3219752754296894559, 0.3333333333333333703, 0.3219752754296894559, 0.3333333333333333703, 0.3219752754296894559, 0.3333333333333333703, 0.3219752754296894559, 0.3333333333333333703, 0.3219752754296894559, 0.3333333333333333703, 0.3219752754296894559, 0.3333333333333333703, 0.3219752754296894559, 0.3333333333333333703, 0.3219752754296894559, 0.3333333333333333703, 0.3219752754296894559, 0.3333333333333333703, 0.3219752754296894559, 0.3333333333333333703, 0.3219752754296894559, 0.3333333333333333703, 0.3219752754296894559, 0.3333333333333333703, 0.3219752754296894559, 0.3333333333333333703, 0.3219752754296894559, 0.3333333333333333703, 0.3219752754296894559, 0.3333333333333333703, 0.3219752754296894559, 0.3333333333333333703, 0.3219752754296894559, 0.3333333333333333703, 0.3219752754296894559, 0.3333333333333333703, 0.3219752754296894559, 0.3333333333333333703, 0.3219752754296894559, 0.3333333333333333703, 0.3219752754296894559, 0.3333333333333333703, 0.3219752754296894559, 0.3333333333333333703, 0.3219752754296894559, 0.3333333333333333703, 0.3219752754296894559, 0.3333333333333333703, 0.3219752754296894559, 0.3333333333333333703, 0.3219752754296894559, 0.3333333333333333703, 0.3219752754296894559, 0.3333333333333333703, 0.3219752754296894559, 0.3333333333333333703, 0.3219752754296894559, 0.3333333333333333703, 0.3219752754296894559, 0.3333333333333333703, 0.3219752754296894559, 0.3333333333333333703, 0.3219752754296894559, 0.3333333333333333703, 0.3219752754296894559, 0.3333333333333333703, 0.3219752754296894559, 0.3333333333333333703, 0.3219752754296894559, 0.3333333333333333703, 0.3219752754296894559, 0.3333333333333333703, 0.3219752754296894559, 0.3333333333333333703, 0.3219752754296894559, 0.3333333333333333703, 0.3219752754296894559, 0.3333333333333333703, 0.3219752754296894559, 0.3333333333333333703, 0.3219752754296894559, 0.3333333333333333703, 0.3219752754296894559, 0.3333333333333333703, 0.3219752754296894559, 0.3333333333333333703, 0.3219752754296894559, 0.3333333333333333703, 0.3219752754296894559, 0.3333333333333333703, 0.3219752754296894559, 0.3333333333333333703, 0.3219752754296894559, 0.3333333333333333703, 0.3219752754296894559, 0.3333333333333333703, 0.3219752754296894559, 0.3333333333333333703, 0.3219752754296894559, 0.3333333333333333703, 0.3219752754296894559, 0.3333333333333333703, 0.3219752754296894559, 0.3333333333333333703, 0.3219752754296894559, 0.3333333333333333703, 0.3219752754296894559, 0.3333333333333333703, 0.3219752754296894559, 0.3333333333333333703, 0.3219752754296894559, 0.3333333333333333703, 0.3219752754296894559, 0.3333333333333333703, 0.3219752754296894559, 0.3333333333333333703, 0.3219752754296894559, 0.3333333333333333703, 0.3219752754296894559, 0.3333333333333333703, 0.3219752754296894559, 0.3333333333333333703, 0.3219752754296894559, 0.3333333333333333703, 0.3219752754296894559, 0.3333333333333333703, 0.3219752754296894559, 0.3333333333333333703, 0.3219752754296894559, 0.3333333333333333703, 0.3219752754296894559, 0.3333333333333333703, 0.3219752754296894559, 0.3333333333333333703, 0.3219752754296894559, 0.3333333333333333703),
 ( 1.000000000000000000, 0.9659258262890683122, 1.000000000000000000, 0.9659258262890683122, 1.000000000000000000, 0.9659258262890683122, 1.000000000000000000, 0.9659258262890683122, 1.000000000000000000, 0.9659258262890683122, 1.000000000000000000, 0.9659258262890683122, 1.000000000000000000, 0.9659258262890683122, 1.000000000000000000, 0.9659258262890683122, 1.000000000000000000, 0.9659258262890683122, 1.000000000000000000, 0.9659258262890683122, 1.000000000000000000, 0.9659258262890683122, 1.000000000000000000, 0.9659258262890683122, 1.000000000000000000, 0.9659258262890683122, 1.000000000000000000, 0.9659258262890683122, 1.000000000000000000, 0.9659258262890683122, 1.000000000000000000, 0.9659258262890683122, 1.000000000000000000, 0.9659258262890683122, 1.000000000000000000, 0.9659258262890683122, 1.000000000000000000, 0.9659258262890683122, 1.000000000000000000, 0.9659258262890683122, 1.000000000000000000, 0.9659258262890683122, 1.000000000000000000, 0.9659258262890683122, 1.000000000000000000, 0.9659258262890683122, 1.000000000000000000, 0.9659258262890683122, 1.000000000000000000, 0.9659258262890683122, 1.000000000000000000, 0.9659258262890683122, 1.000000000000000000, 0.9659258262890683122, 1.000000000000000000, 0.9659258262890683122, 1.000000000000000000, 0.9659258262890683122, 1.000000000000000000, 0.9659258262890683122, 1.000000000000000000, 0.9659258262890683122, 1.000000000000000000, 0.9659258262890683122, 1.000000000000000000, 0.9659258262890683122, 1.000000000000000000, 0.9659258262890683122, 1.000000000000000000, 0.9659258262890683122, 1.000000000000000000, 0.9659258262890683122, 1.000000000000000000, 0.9659258262890683122, 1.000000000000000000, 0.9659258262890683122, 1.000000000000000000, 0.9659258262890683122, 1.000000000000000000, 0.9659258262890683122, 1.000000000000000000, 0.9659258262890683122, 1.000000000000000000, 0.9659258262890683122, 1.000000000000000000, 0.9659258262890683122, 1.000000000000000000, 0.9659258262890683122, 1.000000000000000000, 0.9659258262890683122, 1.000000000000000000, 0.9659258262890683122, 1.000000000000000000, 0.9659258262890683122, 1.000000000000000000, 0.9659258262890683122, 1.000000000000000000, 0.9659258262890683122, 1.000000000000000000, 0.9659258262890683122, 1.000000000000000000, 0.9659258262890683122, 1.000000000000000000, 0.9659258262890683122, 1.000000000000000000, 0.9659258262890683122, 1.000000000000000000, 0.9659258262890683122, 1.000000000000000000, 0.9659258262890683122, 1.000000000000000000, 0.9659258262890683122, 1.000000000000000000, 0.9659258262890683122, 1.000000000000000000, 0.9659258262890683122, 1.000000000000000000, 0.9659258262890683122, 1.000000000000000000, 0.9659258262890683122, 1.000000000000000000, 0.9659258262890683122, 1.000000000000000000, 0.9659258262890683122, 1.000000000000000000, 0.9659258262890683122, 1.000000000000000000, 0.9659258262890683122, 1.000000000000000000, 0.9659258262890683122, 1.000000000000000000, 0.9659258262890683122, 1.000000000000000000, 0.9659258262890683122, 1.000000000000000000, 0.9659258262890683122, 1.000000000000000000, 0.9659258262890683122, 1.000000000000000000, 0.9659258262890683122, 1.000000000000000000, 0.9659258262890683122, 1.000000000000000000, 0.9659258262890683122, 1.000000000000000000, 0.9659258262890683122, 1.000000000000000000, 0.9659258262890683122, 1.000000000000000000, 0.9659258262890683122, 1.000000000000000000, 0.9659258262890683122, 1.000000000000000000, 0.9659258262890683122, 1.000000000000000000, 0.9659258262890683122, 1.000000000000000000, 0.9659258262890683122, 1.000000000000000000, 0.9659258262890683122, 1.000000000000000000, 0.9659258262890683122, 1.000000000000000000, 0.9659258262890683122, 1.000000000000000000, 0.9659258262890683122, 1.000000000000000000, 0.9659258262890683122, 1.000000000000000000, 0.9659258262890683122, 1.000000000000000000, 0.9659258262890683122, 1.000000000000000000, 0.9659258262890683122, 1.000000000000000000, 0.9659258262890683122, 1.000000000000000000, 0.9659258262890683122, 1.000000000000000000, 0.9659258262890683122, 1.000000000000000000, 0.9659258262890683122, 1.000000000000000000, 0.9659258262890683122, 1.000000000000000000, 0.9659258262890683122, 1.000000000000000000, 0.9659258262890683122, 1.000000000000000000, 0.9659258262890683122, 1.000000000000000000, 0.9659258262890683122, 1.000000000000000000, 0.9659258262890683122, 1.000000000000000000, 0.9659258262890683122, 1.000000000000000000, 0.9659258262890683122, 1.000000000000000000, 0.9659258262890683122, 1.000000000000000000, 0.9659258262890683122, 1.000000000000000000, 0.9659258262890683122, 1.000000000000000000, 0.9659258262890683122, 1.000000000000000000, 0.9659258262890683122, 1.000000000000000000, 0.9659258262890683122, 1.000000000000000000, 0.9659258262890683122, 1.000000000000000000, 0.9659258262890683122, 1.000000000000000000, 0.9659258262890683122, 1.000000000000000000, 0.9659258262890683122, 1.000000000000000000, 0.9659258262890683122, 1.000000000000000000, 0.9659258262890683122, 1.000000000000000000, 0.9659258262890683122, 1.000000000000000000, 0.9659258262890683122, 1.000000000000000000, 0.9659258262890683122, 1.000000000000000000, 0.9659258262890683122, 1.000000000000000000, 0.9659258262890683122, 1.000000000000000000, 0.9659258262890683122, 1.000000000000000000, 0.9659258262890683122, 1.000000000000000000, 0.9659258262890683122, 1.000000000000000000, 0.9659258262890683122, 1.000000000000000000, 0.9659258262890683122, 1.000000000000000000, 0.9659258262890683122, 1.000000000000000000, 0.9659258262890683122, 1.000000000000000000, 0.9659258262890683122, 1.000000000000000000, 0.9659258262890683122, 1.000000000000000000, 0.9659258262890683122, 1.000000000000000000, 0.9659258262890683122, 1.000000000000000000, 0.9659258262890683122, 1.000000000000000000, 0.9659258262890683122, 1.000000000000000000, 0.9659258262890683122, 1.000000000000000000, 0.9659258262890683122, 1.000000000000000000, 0.9659258262890683122, 1.000000000000000000, 0.9659258262890683122, 1.000000000000000000, 0.9659258262890683122, 1.000000000000000000, 0.9659258262890683122, 1.000000000000000000, 0.9659258262890683122, 1.000000000000000000, 0.9659258262890683122, 1.000000000000000000, 0.9659258262890683122, 1.000000000000000000, 0.9659258262890683122, 1.000000000000000000, 0.9659258262890683122, 1.000000000000000000, 0.9659258262890683122, 1.000000000000000000, 0.9659258262890683122, 1.000000000000000000, 0.9659258262890683122, 1.000000000000000000, 0.9659258262890683122, 1.000000000000000000, 0.9659258262890683122, 1.000000000000000000, 0.9659258262890683122, 1.000000000000000000, 0.9659258262890683122, 1.000000000000000000, 0.9659258262890683122, 1.000000000000000000, 0.9659258262890683122, 1.000000000000000000, 0.9659258262890683122, 1.000000000000000000, 0.9659258262890683122, 1.000000000000000000, 0.9659258262890683122, 1.000000000000000000, 0.9659258262890683122, 1.000000000000000000, 0.9659258262890683122, 1.000000000000000000, 0.9659258262890683122, 1.000000000000000000, 0.9659258262890683122, 1.000000000000000000, 0.9659258262890683122, 1.000000000000000000, 0.9659258262890683122, 1.000000000000000000, 0.9659258262890683122, 1.000000000000000000, 0.9659258262890683122, 1.000000000000000000, 0.9659258262890683122, 1.000000000000000000, 0.9659258262890683122, 1.000000000000000000, 0.9659258262890683122, 1.000000000000000000, 0.9659258262890683122, 1.000000000000000000, 0.9659258262890683122, 1.000000000000000000, 0.9659258262890683122, 1.000000000000000000, 0.9659258262890683122, 1.000000000000000000, 0.9659258262890683122, 1.000000000000000000, 0.9659258262890683122, 1.000000000000000000, 0.9659258262890683122, 1.000000000000000000, 0.9659258262890683122, 1.000000000000000000, 0.9659258262890683122, 1.000000000000000000, 0.9659258262890683122, 1.000000000000000000, 0.9659258262890683122, 1.000000000000000000, 0.9659258262890683122, 1.000000000000000000, 0.9659258262890683122, 1.000000000000000000, 0.9659258262890683122, 1.000000000000000000, 0.9659258262890683122, 1.000000000000000000, 0.9659258262890683122, 1.000000000000000000, 0.9659258262890683122, 1.000000000000000000, 0.9659258262890683122, 1.000000000000000000, 0.9659258262890683122, 1.000000000000000000, 0.9659258262890683122, 1.000000000000000000, 0.9659258262890683122, 1.000000000000000000, 0.9659258262890683122, 1.000000000000000000, 0.9659258262890683122, 1.000000000000000000, 0.9659258262890683122, 1.000000000000000000, 0.9659258262890683122, 1.000000000000000000, 0.9659258262890683122, 1.000000000000000000, 0.9659258262890683122, 1.000000000000000000, 0.9659258262890683122, 1.000000000000000000, 0.9659258262890683122, 1.000000000000000000, 0.9659258262890683122, 1.000000000000000000, 0.9659258262890683122, 1.000000000000000000, 0.9659258262890683122, 1.000000000000000000, 0.9659258262890683122, 1.000000000000000000, 0.9659258262890683122, 1.000000000000000000, 0.9659258262890683122, 1.000000000000000000, 0.9659258262890683122, 1.000000000000000000, 0.9659258262890683122, 1.000000000000000000, 0.9659258262890683122, 1.000000000000000000, 0.9659258262890683122, 1.000000000000000000, 0.9659258262890683122, 1.000000000000000000, 0.9659258262890683122, 1.000000000000000000, 0.9659258262890683122, 1.000000000000000000, 0.9659258262890683122, 1.000000000000000000, 0.9659258262890683122, 1.000000000000000000, 0.9659258262890683122, 1.000000000000000000, 0.9659258262890683122, 1.000000000000000000, 0.9659258262890683122, 1.000000000000000000, 0.9659258262890683122, 1.000000000000000000, 0.9659258262890683122, 1.000000000000000000, 0.9659258262890683122, 1.000000000000000000, 0.9659258262890683122, 1.000000000000000000, 0.9659258262890683122, 1.000000000000000000, 0.9659258262890683122, 1.000000000000000000, 0.9659258262890683122, 1.000000000000000000, 0.9659258262890683122, 1.000000000000000000, 0.9659258262890683122, 1.000000000000000000, 0.9659258262890683122, 1.000000000000000000, 0.9659258262890683122, 1.000000000000000000, 0.9659258262890683122, 1.000000000000000000, 0.9659258262890683122, 1.000000000000000000, 0.9659258262890683122, 1.000000000000000000, 0.9659258262890683122, 1.000000000000000000, 0.9659258262890683122, 1.000000000000000000, 0.9659258262890683122, 1.000000000000000000, 0.9659258262890683122, 1.000000000000000000) ) ) 
 REPRESENTATION_ITEM ( '' )  SURFACE ( )  );
#116417=CARTESIAN_POINT ( 'NONE',  ( 18.62759615963255655, 10.81492255796105972, 21.66775706135235069 ) ) ;
#116419=CARTESIAN_POINT ( 'NONE',  ( -15.80617190586745835, -15.72974639402198527, 71.87390960531438111 ) ) ;
#116421=CARTESIAN_POINT ( 'NONE',  ( -16.52544592524335698, -4.483927247898792601, 88.95942372801901854 ) ) ;
#116422=CARTESIAN_POINT ( 'NONE',  ( -9.564922557960796823, -16.46253265017161027, 27.08224293864769550 ) ) ;
#116423=CARTESIAN_POINT ( 'NONE',  ( -13.97604488694527625, -13.89961937509977652, 66.87390960531436690 ) ) ;
#116424=CARTESIAN_POINT ( 'NONE',  ( 17.97182807773872426, -5.500000000000046185, 71.03038844047286204 ) ) ;
#116425=DIRECTION ( 'NONE',  ( -0.000000000000000000, -0.000000000000000000, 1.000000000000000000 ) ) ;
#116426=CARTESIAN_POINT ( 'NONE',  ( -8.224510206698948167, 14.34966873604960824, 30.41557627198101699 ) ) ;
#116427=CARTESIAN_POINT ( 'NONE',  ( 10.72451020669871369, 18.67979575497193778, 57.08442372801901854 ) ) ;
#116428=CARTESIAN_POINT ( 'NONE',  ( -5.049401038298153566, 19.05341960407611168, 105.2072429386476671 ) ) ;
#116429=CARTESIAN_POINT ( 'NONE',  ( 18.67979575497194134, -10.72451020669871369, 95.83442372801903275 ) ) ;
#116430=CARTESIAN_POINT ( 'NONE',  ( -13.89961937509977652, 13.97604488694528158, 45.62390960531433848 ) ) ;
#116431=CARTESIAN_POINT ( 'NONE',  ( 16.46253265017160672, -9.564922557960803928, 53.33224293864768839 ) ) ;
#116433=CARTESIAN_POINT ( 'NONE',  ( -5.823673210054431948, 21.52544592524334988, 92.70942372801901854 ) ) ;
#116434=CARTESIAN_POINT ( 'NONE',  ( 8.314922557961029526, -14.29746914071037800, 55.41775706135234714 ) ) ;
#116435=CARTESIAN_POINT ( 'NONE',  ( 0.05219959533937995610, -21.53943276465977519, 80.00109039468568994 ) ) ;
#116436=CARTESIAN_POINT ( 'NONE',  ( 21.55341960407610458, 5.719274019375980345, 23.95724293864769550 ) ) ;
#116437=CARTESIAN_POINT ( 'NONE',  ( 13.97604488694548053, -13.89961937509957401, 95.62609039468563310 ) ) ;
#116438=CARTESIAN_POINT ( 'NONE',  ( 15.72974639402176855, 15.80617190586768217, 51.87609039468568284 ) ) ;
#116439=CARTESIAN_POINT ( 'NONE',  ( -8.314922557961024197, 14.29746914071037800, 32.91775706135234714 ) ) ;
#116440=CARTESIAN_POINT ( 'NONE',  ( 15.80617190586746368, 15.72974639402197994, 89.37390960531435269 ) ) ;
#116441=CARTESIAN_POINT ( 'NONE',  ( 5.153800228976615827, -19.02544592524334988, 90.20942372801900433 ) ) ;
#116442=CARTESIAN_POINT ( 'NONE',  ( -16.46253265017160317, 9.564922557960807481, 70.83224293864770971 ) ) ;
#116443=CARTESIAN_POINT ( 'NONE',  ( -19.03943276465977164, -0.05219959533935918106, 93.75109039468566152 ) ) ;
#116445=CARTESIAN_POINT ( 'NONE',  ( 5.049401038297881783, 19.05341960407617563, 97.29275706135233293 ) ) ;
#116446=CARTESIAN_POINT ( 'NONE',  ( -16.53943276465976808, 0.05219959533911058130, 56.24890960531436690 ) ) ;
#116447=CARTESIAN_POINT ( 'NONE',  ( 16.46253265017146816, 9.564922557961045513, 81.66775706135233293 ) ) ;
#116448=CARTESIAN_POINT ( 'NONE',  ( -12.06949235617739369, -12.14591786802326823, 64.37609039468568994 ) ) ;
#116449=CARTESIAN_POINT ( 'NONE',  ( 9.564922557961047289, -16.46253265017146816, 40.41775706135234003 ) ) ;
#116450=CARTESIAN_POINT ( 'NONE',  ( -9.474510206698964154, 16.51473224551069663, 40.41557627198103120 ) ) ;
#116451=CARTESIAN_POINT ( 'NONE',  ( -9.474510206698964154, 16.51473224551069663, 45.41557627198103120 ) ) ;
#116452=EDGE_CURVE ( 'NONE', #164406, #38283, #159236, .T. ) ;
#116453=CARTESIAN_POINT ( 'NONE',  ( -16.52544592524335698, -4.483927247898792601, 63.95942372801901854 ) ) ;
#116454=CARTESIAN_POINT ( 'NONE',  ( -18.09805431107519880, 5.500000000000101252, 46.01606229291888894 ) ) ;
#116456=CARTESIAN_POINT ( 'NONE',  ( 19.05341960407611168, 5.049401038298154454, 108.9572429386477097 ) ) ;
#116457=CARTESIAN_POINT ( 'NONE',  ( 16.51473224551069308, 9.474510206698969483, 24.16557627198102765 ) ) ;
#116459=CARTESIAN_POINT ( 'NONE',  ( -16.51473224551082808, 9.474510206698731452, 98.33442372801900433 ) ) ;
#116460=CARTESIAN_POINT ( 'NONE',  ( 21.53943276465977519, -0.05219959533907433946, 33.74890960531436690 ) ) ;
#116461=CARTESIAN_POINT ( 'NONE',  ( 19.02544592524334988, 5.153800228976608722, 31.45942372801900433 ) ) ;
#116462=CARTESIAN_POINT ( 'NONE',  ( -5.153800228976607833, 19.02544592524334988, 107.7094237280189759 ) ) ;
#116463=CARTESIAN_POINT ( 'NONE',  ( 16.46253265017160672, -9.564922557960803928, 28.33224293864769550 ) ) ;
#116464=CARTESIAN_POINT ( 'NONE',  ( 5.049401038298161559, -19.05341960407611168, 52.70724293864767418 ) ) ;
#116465=CARTESIAN_POINT ( 'NONE',  ( -10.81492255796078084, -18.62759615963271287, 72.08224293864769550 ) ) ;
#116466=CARTESIAN_POINT ( 'NONE',  ( 19.03943276465977164, -0.05219959533909143690, 103.7489096053143669 ) ) ;
#116467=CARTESIAN_POINT ( 'NONE',  ( 19.02544592524343514, -5.153800228976328945, 33.54057627198102409 ) ) ;
#116469=CARTESIAN_POINT ( 'NONE',  ( -19.03943276465977164, -0.05219959533935918106, 78.75109039468567573 ) ) ;
#116470=CARTESIAN_POINT ( 'NONE',  ( -12.14591786802309592, -12.06949235617757132, 51.87390960531437401 ) ) ;
#116471=CARTESIAN_POINT ( 'NONE',  ( -0.05219959533907301413, -21.53943276465977519, 37.49890960531436690 ) ) ;
#116472=CARTESIAN_POINT ( 'NONE',  ( -15.80617190586768217, 15.72974639402176855, 108.1260903946856757 ) ) ;
#116473=CARTESIAN_POINT ( 'NONE',  ( -15.72974639402197994, 15.80617190586746368, 95.62390960531436690 ) ) ;
#116474=CARTESIAN_POINT ( 'NONE',  ( 21.53943276465977519, 0.05219959533937863772, 76.25109039468568994 ) ) ;
#116475=CARTESIAN_POINT ( 'NONE',  ( -10.72451020669870658, -18.67979575497194134, 74.58442372801901854 ) ) ;
#116476=CARTESIAN_POINT ( 'NONE',  ( -9.474510206698964154, 16.51473224551069663, 115.4155762719810241 ) ) ;
#116477=CARTESIAN_POINT ( 'NONE',  ( 12.06949235617739724, 12.14591786802326823, 111.8760903946856615 ) ) ;
#116478=CARTESIAN_POINT ( 'NONE',  ( -21.55341960407619339, 5.719274019375674811, 58.54275706135235424 ) ) ;
#116479=CARTESIAN_POINT ( 'NONE',  ( 13.89961937509977652, -13.97604488694527269, 73.12390960531436690 ) ) ;
#116480=CARTESIAN_POINT ( 'NONE',  ( -13.89961937509957401, -13.97604488694547875, 39.37609039468566152 ) ) ;
#116481=CARTESIAN_POINT ( 'NONE',  ( -10.72451020669870658, -18.67979575497194134, 34.58442372801900433 ) ) ;
#116482=CARTESIAN_POINT ( 'NONE',  ( 9.564922557960805705, 16.46253265017160317, 64.58224293864769550 ) ) ;
#116483=CARTESIAN_POINT ( 'NONE',  ( 16.52544592524342804, -4.483927247898539470, 78.54057627198103830 ) ) ;
#116484=CARTESIAN_POINT ( 'NONE',  ( 16.53943276465976808, -0.05219959533910856209, 53.74890960531437401 ) ) ;
#116485=CARTESIAN_POINT ( 'NONE',  ( 21.52544592524344225, -5.823673210054117533, 58.54057627198103120 ) ) ;
#116486=CARTESIAN_POINT ( 'NONE',  ( -0.05219959533909027116, -19.03943276465977164, 57.49890960531435979 ) ) ;
#116487=CARTESIAN_POINT ( 'NONE',  ( -0.05219959533907301413, -21.53943276465977519, 67.49890960531436690 ) ) ;
#116488=CARTESIAN_POINT ( 'NONE',  ( 5.153800228976615827, -19.02544592524334988, 65.20942372801900433 ) ) ;
#116489=CARTESIAN_POINT ( 'NONE',  ( 9.474510206698729675, 16.51473224551082808, 22.08442372801899722 ) ) ;
#116490=CARTESIAN_POINT ( 'NONE',  ( -16.55341960407611168, -4.379528057220339221, 61.45724293864770260 ) ) ;
#116491=CARTESIAN_POINT ( 'NONE',  ( -15.72974639402197994, 15.80617190586746368, 45.62390960531436690 ) ) ;
#116493=CARTESIAN_POINT ( 'NONE',  ( 16.88567814943161949, 6.947325034625699836, 103.7900112265258770 ) ) ;
#116494=CARTESIAN_POINT ( 'NONE',  ( -14.29746914071037622, -8.314922557961029526, 79.16775706135234714 ) ) ;
#116497=CARTESIAN_POINT ( 'NONE',  ( -5.049401038297874678, -19.05341960407617918, 84.79275706135233293 ) ) ;
#116498=CARTESIAN_POINT ( 'NONE',  ( 8.314922557960818139, 14.29746914071049879, 59.58224293864770260 ) ) ;
#116500=CARTESIAN_POINT ( 'NONE',  ( -19.02544592524342804, 5.153800228976336051, 46.04057627198101699 ) ) ;
#116501=CARTESIAN_POINT ( 'NONE',  ( 8.224510206698953496, -14.34966873604960469, 42.91557627198103120 ) ) ;
#116502=CARTESIAN_POINT ( 'NONE',  ( 16.46253265017160672, -9.564922557960803928, 93.33224293864769550 ) ) ;
#116503=CARTESIAN_POINT ( 'NONE',  ( 19.05341960407611168, 5.049401038298154454, 53.95724293864770260 ) ) ;
#116504=CARTESIAN_POINT ( 'NONE',  ( 15.80617190586769283, -15.72974639402175789, 65.62609039468568994 ) ) ;
#116505=CARTESIAN_POINT ( 'NONE',  ( -16.46253265017160317, 9.564922557960807481, 65.83224293864769550 ) ) ;
#116507=CARTESIAN_POINT ( 'NONE',  ( -9.564922557960796823, -16.46253265017161027, 72.08224293864770971 ) ) ;
#116508=CARTESIAN_POINT ( 'NONE',  ( 21.55341960407610458, 5.719274019375980345, 48.95724293864770971 ) ) ;
#116509=CARTESIAN_POINT ( 'NONE',  ( -16.46253265017160317, 9.564922557960807481, 50.83224293864770260 ) ) ;
#116510=CARTESIAN_POINT ( 'NONE',  ( 21.55341960407610458, 5.719274019375980345, 53.95724293864770260 ) ) ;
#116511=CARTESIAN_POINT ( 'NONE',  ( -9.474510206698720793, -16.51473224551083518, 79.58442372801899012 ) ) ;
#116513=CARTESIAN_POINT ( 'NONE',  ( -16.52544592524335698, -4.483927247898792601, 98.95942372801903275 ) ) ;
#116514=CARTESIAN_POINT ( 'NONE',  ( -19.02544592524334988, -5.153800228976617603, 23.95942372801900078 ) ) ;
#116515=CARTESIAN_POINT ( 'NONE',  ( -4.483927247898782831, 16.52544592524335698, 47.70942372801902565 ) ) ;
#116516=CARTESIAN_POINT ( 'NONE',  ( 8.224510206698742110, 14.34966873604972548, 77.08442372801901854 ) ) ;
#116517=CARTESIAN_POINT ( 'NONE',  ( -12.06949235617739369, -12.14591786802326823, 64.37609039468568994 ) ) ;
#116518=CARTESIAN_POINT ( 'NONE',  ( -21.53943276465977519, 0.05219959533907696930, 26.24890960531435624 ) ) ;
#116519=CARTESIAN_POINT ( 'NONE',  ( 16.51473224551069308, 9.474510206698969483, 34.16557627198102409 ) ) ;
#116520=CARTESIAN_POINT ( 'NONE',  ( 16.55341960407618274, -4.379528057220086978, 41.04275706135236135 ) ) ;
#116521=CARTESIAN_POINT ( 'NONE',  ( 9.474510206698971260, -16.51473224551069308, 42.91557627198103120 ) ) ;
#116522=CARTESIAN_POINT ( 'NONE',  ( 15.72974639402176855, 15.80617190586768217, 36.87609039468568994 ) ) ;
#116523=CARTESIAN_POINT ( 'NONE',  ( 14.34966873604972726, -8.224510206698740333, 35.83442372801901143 ) ) ;
#116524=CARTESIAN_POINT ( 'NONE',  ( 14.34966873604972726, -8.224510206698740333, 100.8344237280190185 ) ) ;
#116525=CARTESIAN_POINT ( 'NONE',  ( -19.03943276465977164, 0.05219959533909376836, 21.24890960531436335 ) ) ;
#116526=CARTESIAN_POINT ( 'NONE',  ( -21.52544592524334988, -5.823673210054445271, 103.9594237280190185 ) ) ;
#116527=CARTESIAN_POINT ( 'NONE',  ( -19.02544592524334988, -5.153800228976617603, 108.9594237280189759 ) ) ;
#116528=CARTESIAN_POINT ( 'NONE',  ( 5.153800228976615827, -19.02544592524334988, 70.20942372801899012 ) ) ;
#116529=CARTESIAN_POINT ( 'NONE',  ( -0.05219959533910754901, -16.53943276465976808, 67.49890960531436690 ) ) ;
#116530=CARTESIAN_POINT ( 'NONE',  ( 9.564922557960805705, 16.46253265017160317, 29.58224293864769550 ) ) ;
#116531=CARTESIAN_POINT ( 'NONE',  ( 5.049401038297881783, 19.05341960407617563, 62.29275706135234003 ) ) ;
#116532=CARTESIAN_POINT ( 'NONE',  ( 16.52216118717246829, -7.221426719304367303, 56.42400978952971258 ) ) ;
#116533=CARTESIAN_POINT ( 'NONE',  ( -10.72451020669870658, -18.67979575497194134, 64.58442372801900433 ) ) ;
#116534=CARTESIAN_POINT ( 'NONE',  ( -8.314922557961024197, 14.29746914071037800, 27.91775706135234358 ) ) ;
#116535=CARTESIAN_POINT ( 'NONE',  ( 19.52217212775657629, -5.500000000000104805, 57.43993709005260939 ) ) ;
#116536=CARTESIAN_POINT ( 'NONE',  ( -21.53943276465977519, 0.05219959533907696930, 26.24890960531435624 ) ) ;
#116537=CARTESIAN_POINT ( 'NONE',  ( -19.03943276465977164, -0.05219959533935918106, 113.7510903946856757 ) ) ;
#116538=CARTESIAN_POINT ( 'NONE',  ( -19.02544592524342804, 5.153800228976336051, 111.0405762719810099 ) ) ;
#116540=CARTESIAN_POINT ( 'NONE',  ( 5.153800228976335163, 19.02544592524342804, 24.79057627198102765 ) ) ;
#116541=CARTESIAN_POINT ( 'NONE',  ( -15.80617190586768217, 15.72974639402176855, 103.1260903946856757 ) ) ;
#116542=CARTESIAN_POINT ( 'NONE',  ( -9.474510206698964154, 16.51473224551069663, 50.41557627198102409 ) ) ;
#116543=CARTESIAN_POINT ( 'NONE',  ( 5.719274019375673035, 21.55341960407619339, 62.29275706135236845 ) ) ;
#116544=CARTESIAN_POINT ( 'NONE',  ( 10.72451020669871369, 18.67979575497193778, 102.0844237280190185 ) ) ;
#116545=CARTESIAN_POINT ( 'NONE',  ( 8.224510206698953496, -14.34966873604960469, 22.91557627198102765 ) ) ;
#116546=CARTESIAN_POINT ( 'NONE',  ( 0.05219959533909260263, 19.03943276465977164, 29.99890960531435979 ) ) ;
#116547=CARTESIAN_POINT ( 'NONE',  ( 19.03943276465977164, -0.05219959533909143690, 73.74890960531435269 ) ) ;
#116548=CARTESIAN_POINT ( 'NONE',  ( -21.53943276465977519, -0.05219959533937600094, 58.75109039468568994 ) ) ;
#116549=CARTESIAN_POINT ( 'NONE',  ( 16.51473224551069308, 9.474510206698969483, 39.16557627198103120 ) ) ;
#116550=CARTESIAN_POINT ( 'NONE',  ( 10.72451020669871369, 18.67979575497193778, 52.08442372801901854 ) ) ;
#116551=CARTESIAN_POINT ( 'NONE',  ( -19.03943276465977164, -0.05219959533935918106, 78.75109039468567573 ) ) ;
#116552=CARTESIAN_POINT ( 'NONE',  ( -5.049401038298153566, 19.05341960407611168, 110.2072429386476671 ) ) ;
#116553=CARTESIAN_POINT ( 'NONE',  ( -5.049401038298153566, 19.05341960407611168, 25.20724293864768484 ) ) ;
#116554=CARTESIAN_POINT ( 'NONE',  ( -10.81492255796078084, -18.62759615963271287, 107.0822429386476955 ) ) ;
#116555=CARTESIAN_POINT ( 'NONE',  ( 16.46253265017146816, 9.564922557961045513, 36.66775706135233293 ) ) ;
#116556=CARTESIAN_POINT ( 'NONE',  ( -12.06949235617756955, 12.14591786802309770, 95.62390960531436690 ) ) ;
#116557=CARTESIAN_POINT ( 'NONE',  ( 19.05341960407611168, 5.049401038298154454, 43.95724293864769550 ) ) ;
#116558=CARTESIAN_POINT ( 'NONE',  ( 13.89961937509957401, 13.97604488694547697, 96.87609039468566152 ) ) ;
#116559=CARTESIAN_POINT ( 'NONE',  ( -0.05219959533910754901, -16.53943276465976808, 57.49890960531435979 ) ) ;
#116560=CARTESIAN_POINT ( 'NONE',  ( 18.67979575497194134, -10.72451020669871369, 105.8344237280190328 ) ) ;
#116561=CARTESIAN_POINT ( 'NONE',  ( -16.46253265017160317, 9.564922557960807481, 105.8322429386476955 ) ) ;
#116562=CARTESIAN_POINT ( 'NONE',  ( -19.02544592524334988, -5.153800228976617603, 88.95942372801897591 ) ) ;
#116563=CARTESIAN_POINT ( 'NONE',  ( -21.52544592524343514, 5.823673210054127303, 91.04057627198103830 ) ) ;
#116564=CARTESIAN_POINT ( 'NONE',  ( -21.55341960407619339, 5.719274019375674811, 38.54275706135234714 ) ) ;
#116565=CARTESIAN_POINT ( 'NONE',  ( -16.52544592524335698, -4.483927247898792601, 48.95942372801902565 ) ) ;
#116566=CARTESIAN_POINT ( 'NONE',  ( 0.05219959533934541429, -16.53943276465976808, 110.0010903946856757 ) ) ;
#116567=CARTESIAN_POINT ( 'NONE',  ( 8.224510206698742110, 14.34966873604972548, 47.08442372801901854 ) ) ;
#116568=CARTESIAN_POINT ( 'NONE',  ( 5.719274019375673035, 21.55341960407619339, 47.29275706135234003 ) ) ;
#116569=CARTESIAN_POINT ( 'NONE',  ( 0.05219959533907565091, 21.53943276465977519, 44.99890960531435979 ) ) ;
#116570=CARTESIAN_POINT ( 'NONE',  ( -16.46253265017160317, 9.564922557960807481, 30.83224293864769550 ) ) ;
#116572=CARTESIAN_POINT ( 'NONE',  ( 12.14591786802327356, -12.06949235617739191, 60.62609039468567573 ) ) ;
#116573=CARTESIAN_POINT ( 'NONE',  ( 21.52544592524344225, -5.823673210054117533, 93.54057627198103830 ) ) ;
#116574=CARTESIAN_POINT ( 'NONE',  ( -4.379528057220328563, 16.55341960407611168, 45.20724293864769550 ) ) ;
#116575=CARTESIAN_POINT ( 'NONE',  ( -16.55341960407617563, 4.379528057220093196, 68.54275706135234714 ) ) ;
#116576=CARTESIAN_POINT ( 'NONE',  ( -0.05219959533909027116, -19.03943276465977164, 57.49890960531435979 ) ) ;
#116577=CARTESIAN_POINT ( 'NONE',  ( 19.03943276465977164, 0.05219959533936151252, 106.2510903946856615 ) ) ;
#116578=CARTESIAN_POINT ( 'NONE',  ( -21.53943276465977519, 0.05219959533907696930, 81.24890960531436690 ) ) ;
#116579=CARTESIAN_POINT ( 'NONE',  ( -0.05219959533910754901, -16.53943276465976808, 32.49890960531435979 ) ) ;
#116582=CARTESIAN_POINT ( 'NONE',  ( 21.53943276465977519, -0.05219959533907433946, 78.74890960531436690 ) ) ;
#116583=CARTESIAN_POINT ( 'NONE',  ( -12.14591786802326823, 12.06949235617739902, 108.1260903946856757 ) ) ;
#116585=CARTESIAN_POINT ( 'NONE',  ( 17.50000000000000711, -4.119547552397547108, 102.9808761550738296 ) ) ;
#116586=CARTESIAN_POINT ( 'NONE',  ( 18.67979575497178502, 10.72451020669898547, 89.16557627198102409 ) ) ;
#116587=CARTESIAN_POINT ( 'NONE',  ( 21.53943276465977519, -0.05219959533907433946, 103.7489096053143669 ) ) ;
#116588=CARTESIAN_POINT ( 'NONE',  ( 4.483927247898545687, 16.52544592524342804, 29.79057627198102409 ) ) ;
#116589=CARTESIAN_POINT ( 'NONE',  ( 16.53943276465976808, 0.05219959533934440121, 31.25109039468568639 ) ) ;
#116590=CARTESIAN_POINT ( 'NONE',  ( 16.51473224551069308, 9.474510206698969483, 29.16557627198103475 ) ) ;
#116591=CARTESIAN_POINT ( 'NONE',  ( 16.51473224551069308, 9.474510206698969483, 64.16557627198102409 ) ) ;
#116593=CARTESIAN_POINT ( 'NONE',  ( -21.55341960407610458, -5.719274019375992779, 21.45724293864769550 ) ) ;
#116595=CARTESIAN_POINT ( 'NONE',  ( -16.51473224551082808, 9.474510206698731452, 103.3344237280190043 ) ) ;
#116596=CARTESIAN_POINT ( 'NONE',  ( -19.02544592524334988, -5.153800228976617603, 33.95942372801897591 ) ) ;
#116597=CARTESIAN_POINT ( 'NONE',  ( -15.80617190586745835, -15.72974639402198527, 91.87390960531436690 ) ) ;
#116599=CARTESIAN_POINT ( 'NONE',  ( 4.379528057220092307, 16.55341960407617563, 112.2927570613523471 ) ) ;
#116600=CARTESIAN_POINT ( 'NONE',  ( -21.52544592524343514, 5.823673210054127303, 46.04057627198103830 ) ) ;
#116601=CARTESIAN_POINT ( 'NONE',  ( 21.55341960407610458, 5.719274019375980345, 78.95724293864769550 ) ) ;
#116602=CARTESIAN_POINT ( 'NONE',  ( 5.153800228976615827, -19.02544592524334988, 100.2094237280190043 ) ) ;
#116603=CARTESIAN_POINT ( 'NONE',  ( -19.05341960407611168, -5.049401038298163336, 106.4572429386476955 ) ) ;
#116604=CARTESIAN_POINT ( 'NONE',  ( 0.05219959533937995610, -21.53943276465977519, 70.00109039468568994 ) ) ;
#116605=CARTESIAN_POINT ( 'NONE',  ( 13.97604488694527802, 13.89961937509977652, 59.37390960531434558 ) ) ;
#116606=CARTESIAN_POINT ( 'NONE',  ( -4.483927247898539470, -16.52544592524342804, 97.29057627198105251 ) ) ;
#116608=CARTESIAN_POINT ( 'NONE',  ( -9.474510206698964154, 16.51473224551069663, 65.41557627198102409 ) ) ;
#116609=CARTESIAN_POINT ( 'NONE',  ( -4.379528057220328563, 16.55341960407611168, 90.20724293864770971 ) ) ;
#116610=ORIENTED_EDGE ( 'NONE', *, *, #113016, .F. ) ;
#116611=CARTESIAN_POINT ( 'NONE',  ( -9.564922557961040184, 16.46253265017147172, 87.91775706135233293 ) ) ;
#116613=CARTESIAN_POINT ( 'NONE',  ( -19.05341960407611168, -5.049401038298163336, 66.45724293864769550 ) ) ;
#116614=CARTESIAN_POINT ( 'NONE',  ( -18.67979575497193778, 10.72451020669871902, 78.33442372801901854 ) ) ;
#116615=CARTESIAN_POINT ( 'NONE',  ( 5.049401038298161559, -19.05341960407611168, 102.7072429386476955 ) ) ;
#116616=CARTESIAN_POINT ( 'NONE',  ( 16.55341960407618274, -4.379528057220086978, 81.04275706135236135 ) ) ;
#116617=CARTESIAN_POINT ( 'NONE',  ( -17.26172910966778318, -6.454744622555875999, 49.19353091350777873 ) ) ;
#116618=CARTESIAN_POINT ( 'NONE',  ( 0.05219959533936267826, -19.03943276465977164, 40.00109039468566152 ) ) ;
#116619=CARTESIAN_POINT ( 'NONE',  ( 10.81492255796106328, -18.62759615963255655, 95.41775706135234714 ) ) ;
#116622=CARTESIAN_POINT ( 'NONE',  ( -14.29746914071037622, -8.314922557961029526, 99.16775706135234714 ) ) ;
#116624=CARTESIAN_POINT ( 'NONE',  ( 16.52544592524335698, 4.483927247898782831, 96.45942372801901854 ) ) ;
#116626=CARTESIAN_POINT ( 'NONE',  ( -8.314922557961024197, 14.29746914071037800, 62.91775706135236135 ) ) ;
#116628=CARTESIAN_POINT ( 'NONE',  ( 21.53943276465977519, 0.05219959533937863772, 76.25109039468568994 ) ) ;
#116629=CARTESIAN_POINT ( 'NONE',  ( -13.89961937509957401, -13.97604488694547875, 84.37609039468567573 ) ) ;
#116630=CARTESIAN_POINT ( 'NONE',  ( 0.05219959533936267826, -19.03943276465977164, 40.00109039468566152 ) ) ;
#116631=CARTESIAN_POINT ( 'NONE',  ( -9.474510206698964154, 16.51473224551069663, 70.41557627198102409 ) ) ;
#116632=CARTESIAN_POINT ( 'NONE',  ( -19.05341960407611168, -5.049401038298163336, 56.45724293864768129 ) ) ;
#116633=CARTESIAN_POINT ( 'NONE',  ( -17.49999999999999645, 5.499999999999998224, 22.00000000000000711 ) ) ;
#116634=CARTESIAN_POINT ( 'NONE',  ( -15.72974639402197994, 15.80617190586746368, 75.62390960531439532 ) ) ;
#116635=CARTESIAN_POINT ( 'NONE',  ( 18.67979575497178502, 10.72451020669898547, 34.16557627198102409 ) ) ;
#116636=CARTESIAN_POINT ( 'NONE',  ( -19.03943276465977164, 0.05219959533909376836, 36.24890960531436690 ) ) ;
#116637=CARTESIAN_POINT ( 'NONE',  ( 4.379528057220092307, 16.55341960407617563, 62.29275706135236845 ) ) ;
#116638=VERTEX_POINT ( 'NONE', #151817 ) ;
#116639=CARTESIAN_POINT ( 'NONE',  ( 15.72974639402176855, 15.80617190586768217, 26.87609039468567218 ) ) ;
#116640=CARTESIAN_POINT ( 'NONE',  ( -4.379528057220328563, 16.55341960407611168, 70.20724293864769550 ) ) ;
#116642=CARTESIAN_POINT ( 'NONE',  ( -0.05219959533934338120, 16.53943276465976808, 22.50109039468567573 ) ) ;
#116643=CARTESIAN_POINT ( 'NONE',  ( 19.05341960407617918, -5.049401038297876454, 51.04275706135231871 ) ) ;
#116644=CARTESIAN_POINT ( 'NONE',  ( -12.06949235617756955, 12.14591786802309770, 60.62390960531437401 ) ) ;
#116645=CARTESIAN_POINT ( 'NONE',  ( -21.53943276465977519, -0.05219959533937600094, 33.75109039468568284 ) ) ;
#116646=CARTESIAN_POINT ( 'NONE',  ( 5.153800228976335163, 19.02544592524342804, 99.79057627198102409 ) ) ;
#116647=CARTESIAN_POINT ( 'NONE',  ( 18.67979575497178502, 10.72451020669898547, 84.16557627198103830 ) ) ;
#116648=CARTESIAN_POINT ( 'NONE',  ( 19.05341960407611168, 5.049401038298154454, 108.9572429386477097 ) ) ;
#116649=CARTESIAN_POINT ( 'NONE',  ( -4.379528057220328563, 16.55341960407611168, 80.20724293864769550 ) ) ;
#116651=CARTESIAN_POINT ( 'NONE',  ( -13.89961937509957401, -13.97604488694547875, 69.37609039468564731 ) ) ;
#116652=CARTESIAN_POINT ( 'NONE',  ( 0.05219959533907565091, 21.53943276465977519, 104.9989096053143669 ) ) ;
#116653=CARTESIAN_POINT ( 'NONE',  ( -9.564922557960796823, -16.46253265017161027, 57.08224293864769550 ) ) ;
#116654=CARTESIAN_POINT ( 'NONE',  ( 13.97604488694548053, -13.89961937509957401, 40.62609039468564731 ) ) ;
#116655=CARTESIAN_POINT ( 'NONE',  ( 19.05341960407611168, 5.049401038298154454, 33.95724293864769550 ) ) ;
#116656=CARTESIAN_POINT ( 'NONE',  ( -5.823673210054431948, 21.52544592524334988, 57.70942372801901143 ) ) ;
#116657=CARTESIAN_POINT ( 'NONE',  ( -17.50000000000001421, -5.499999999999944045, 71.28230962303567253 ) ) ;
#116658=CARTESIAN_POINT ( 'NONE',  ( -8.224510206698948167, 14.34966873604960824, 40.41557627198103120 ) ) ;
#116659=CARTESIAN_POINT ( 'NONE',  ( -19.05341960407611168, -5.049401038298163336, 56.45724293864768129 ) ) ;
#116660=CARTESIAN_POINT ( 'NONE',  ( -10.72451020669898014, 18.67979575497178502, 90.41557627198103830 ) ) ;
#116661=CARTESIAN_POINT ( 'NONE',  ( -0.05219959533909027116, -19.03943276465977164, 57.49890960531435979 ) ) ;
#116663=CARTESIAN_POINT ( 'NONE',  ( -18.62759615963270932, 10.81492255796079327, 60.83224293864769550 ) ) ;
#116664=CARTESIAN_POINT ( 'NONE',  ( 21.53943276465977519, 0.05219959533937863772, 96.25109039468568994 ) ) ;
#116666=CARTESIAN_POINT ( 'NONE',  ( 8.314922557961029526, -14.29746914071037800, 90.41775706135236135 ) ) ;
#116667=CARTESIAN_POINT ( 'NONE',  ( 16.52544592524342804, -4.483927247898539470, 88.54057627198103830 ) ) ;
#116668=CARTESIAN_POINT ( 'NONE',  ( 19.02544592524334988, 5.153800228976608722, 91.45942372801900433 ) ) ;
#116670=CARTESIAN_POINT ( 'NONE',  ( -13.89961937509957401, -13.97604488694547875, 39.37609039468566152 ) ) ;
#116671=CARTESIAN_POINT ( 'NONE',  ( 12.14591786802327356, -12.06949235617739191, 95.62609039468568994 ) ) ;
#116673=CARTESIAN_POINT ( 'NONE',  ( 19.05341960407617918, -5.049401038297876454, 31.04275706135232227 ) ) ;
#116674=CARTESIAN_POINT ( 'NONE',  ( 5.153800228976335163, 19.02544592524342804, 84.79057627198099567 ) ) ;
#116675=CARTESIAN_POINT ( 'NONE',  ( -0.05219959533907301413, -21.53943276465977519, 62.49890960531436690 ) ) ;
#116677=CARTESIAN_POINT ( 'NONE',  ( 9.564922557960805705, 16.46253265017160317, 24.58224293864769194 ) ) ;
#116678=CARTESIAN_POINT ( 'NONE',  ( -5.823673210054431948, 21.52544592524334988, 97.70942372801904696 ) ) ;
#116679=CARTESIAN_POINT ( 'NONE',  ( -4.483927247898782831, 16.52544592524335698, 72.70942372801901854 ) ) ;
#116680=CARTESIAN_POINT ( 'NONE',  ( -5.719274019375665041, -21.55341960407619695, 34.79275706135235424 ) ) ;
#116681=CARTESIAN_POINT ( 'NONE',  ( 8.224510206698742110, 14.34966873604972548, 27.08442372801901854 ) ) ;
#116682=CARTESIAN_POINT ( 'NONE',  ( 16.51473224551069308, 9.474510206698969483, 109.1655762719810383 ) ) ;
#116683=CARTESIAN_POINT ( 'NONE',  ( 0.05219959533909260263, 19.03943276465977164, 34.99890960531435979 ) ) ;
#116684=CARTESIAN_POINT ( 'NONE',  ( 13.89961937509977652, -13.97604488694527269, 53.12390960531434558 ) ) ;
#116685=CARTESIAN_POINT ( 'NONE',  ( -14.34966873604972548, 8.224510206698743886, 43.33442372801901143 ) ) ;
#116686=CARTESIAN_POINT ( 'NONE',  ( 4.483927247898545687, 16.52544592524342804, 89.79057627198103830 ) ) ;
#116687=CARTESIAN_POINT ( 'NONE',  ( -14.29746914071037622, -8.314922557961029526, 94.16775706135237556 ) ) ;
#116688=CARTESIAN_POINT ( 'NONE',  ( 18.67979575497194134, -10.72451020669871369, 45.83442372801901854 ) ) ;
#116689=CARTESIAN_POINT ( 'NONE',  ( -13.97604488694527625, -13.89961937509977652, 71.87390960531433848 ) ) ;
#116690=CARTESIAN_POINT ( 'NONE',  ( -19.05341960407611168, -5.049401038298163336, 66.45724293864769550 ) ) ;
#116691=CARTESIAN_POINT ( 'NONE',  ( 19.03943276465977164, -0.05219959533909143690, 93.74890960531435269 ) ) ;
#116693=CARTESIAN_POINT ( 'NONE',  ( -0.05219959533910754901, -16.53943276465976808, 37.49890960531436690 ) ) ;
#116694=CARTESIAN_POINT ( 'NONE',  ( 12.14591786802327356, -12.06949235617739191, 100.6260903946857184 ) ) ;
#116696=CARTESIAN_POINT ( 'NONE',  ( 5.153800228976615827, -19.02544592524334988, 40.20942372801898301 ) ) ;
#116697=CARTESIAN_POINT ( 'NONE',  ( -9.474510206698964154, 16.51473224551069663, 65.41557627198102409 ) ) ;
#116698=CARTESIAN_POINT ( 'NONE',  ( 5.153800228976615827, -19.02544592524334988, 40.20942372801898301 ) ) ;
#116700=CARTESIAN_POINT ( 'NONE',  ( 19.48894818550246555, -5.499999999999910294, 72.60307310435236161 ) ) ;
#116701=CARTESIAN_POINT ( 'NONE',  ( -16.52544592524335698, -4.483927247898792601, 48.95942372801902565 ) ) ;
#116702=CARTESIAN_POINT ( 'NONE',  ( 16.46253265017146816, 9.564922557961045513, 71.66775706135233293 ) ) ;
#116703=CARTESIAN_POINT ( 'NONE',  ( 8.224510206698742110, 14.34966873604972548, 62.08442372801901143 ) ) ;
#116704=CARTESIAN_POINT ( 'NONE',  ( -19.02544592524342804, 5.153800228976336051, 116.0405762719810383 ) ) ;
#116705=CARTESIAN_POINT ( 'NONE',  ( 19.05341960407611168, 5.049401038298154454, 93.95724293864769550 ) ) ;
#116706=CARTESIAN_POINT ( 'NONE',  ( 0.05219959533937995610, -21.53943276465977519, 20.00109039468568639 ) ) ;
#116707=CARTESIAN_POINT ( 'NONE',  ( -9.564922557961040184, 16.46253265017147172, 77.91775706135234714 ) ) ;
#116708=CARTESIAN_POINT ( 'NONE',  ( 0.05219959533909260263, 19.03943276465977164, 99.99890960531436690 ) ) ;
#116709=CARTESIAN_POINT ( 'NONE',  ( 16.46253265017160672, -9.564922557960803928, 33.33224293864770260 ) ) ;
#116710=CARTESIAN_POINT ( 'NONE',  ( -19.03943276465977164, 0.05219959533909376836, 81.24890960531436690 ) ) ;
#116711=CARTESIAN_POINT ( 'NONE',  ( -16.53943276465976808, 0.05219959533911058130, 51.24890960531436690 ) ) ;
#116712=CARTESIAN_POINT ( 'NONE',  ( -19.02544592524342804, 5.153800228976336051, 36.04057627198100988 ) ) ;
#116713=CARTESIAN_POINT ( 'NONE',  ( -0.05219959533936034679, 19.03943276465977164, 57.50109039468566863 ) ) ;
#116715=CARTESIAN_POINT ( 'NONE',  ( -14.34966873604960291, -8.224510206698953496, 86.66557627198102409 ) ) ;
#116716=CARTESIAN_POINT ( 'NONE',  ( 21.53943276465977519, 0.05219959533937863772, 106.2510903946856757 ) ) ;
#116717=CARTESIAN_POINT ( 'NONE',  ( 9.474510206698971260, -16.51473224551069308, 57.91557627198103120 ) ) ;
#116718=CARTESIAN_POINT ( 'NONE',  ( 18.62759615963271287, -10.81492255796078972, 53.33224293864769550 ) ) ;
#116719=CARTESIAN_POINT ( 'NONE',  ( -14.29746914071049879, 8.314922557960819915, 55.83224293864770260 ) ) ;
#116720=CARTESIAN_POINT ( 'NONE',  ( 5.153800228976615827, -19.02544592524334988, 20.20942372801899722 ) ) ;
#116721=CARTESIAN_POINT ( 'NONE',  ( -16.46253265017160317, 9.564922557960807481, 100.8322429386477097 ) ) ;
#116722=CARTESIAN_POINT ( 'NONE',  ( 5.153800228976335163, 19.02544592524342804, 114.7905762719810241 ) ) ;
#116723=CARTESIAN_POINT ( 'NONE',  ( 5.153800228976335163, 19.02544592524342804, 34.79057627198102409 ) ) ;
#116724=CARTESIAN_POINT ( 'NONE',  ( -0.05219959533909027116, -19.03943276465977164, 27.49890960531435624 ) ) ;
#116725=CARTESIAN_POINT ( 'NONE',  ( 14.34966873604960469, 8.224510206698951720, 84.16557627198103830 ) ) ;
#116726=CARTESIAN_POINT ( 'NONE',  ( -0.05219959533907301413, -21.53943276465977519, 97.49890960531436690 ) ) ;
#116727=CARTESIAN_POINT ( 'NONE',  ( -5.153800228976328057, -19.02544592524343514, 102.2905762719810383 ) ) ;
#116728=CARTESIAN_POINT ( 'NONE',  ( -15.72974639402197994, 15.80617190586746368, 110.6239096053143669 ) ) ;
#116729=CARTESIAN_POINT ( 'NONE',  ( 13.89961937509977652, -13.97604488694527269, 103.1239096053143527 ) ) ;
#116731=CARTESIAN_POINT ( 'NONE',  ( -8.314922557960811034, -14.29746914071050412, 102.0822429386476955 ) ) ;
#116732=CARTESIAN_POINT ( 'NONE',  ( 0.05219959533909260263, 19.03943276465977164, 64.99890960531436690 ) ) ;
#116733=CARTESIAN_POINT ( 'NONE',  ( 15.72974639402199770, -15.80617190586745480, 78.12390960531436690 ) ) ;
#116734=CARTESIAN_POINT ( 'NONE',  ( 16.31925111598456724, -7.325300261831551474, 107.6642453896725158 ) ) ;
#116736=CARTESIAN_POINT ( 'NONE',  ( 15.80617190586746368, 15.72974639402197994, 34.37390960531435979 ) ) ;
#116737=CARTESIAN_POINT ( 'NONE',  ( -4.379528057220086978, -16.55341960407618274, 34.79275706135235424 ) ) ;
#116738=CARTESIAN_POINT ( 'NONE',  ( 14.29746914071049879, -8.314922557960816363, 93.33224293864769550 ) ) ;
#116740=CARTESIAN_POINT ( 'NONE',  ( -19.03943276465977164, 0.05219959533909376836, 61.24890960531436690 ) ) ;
#116741=CARTESIAN_POINT ( 'NONE',  ( 14.34966873604960469, 8.224510206698951720, 84.16557627198103830 ) ) ;
#116742=CARTESIAN_POINT ( 'NONE',  ( -15.80617190586745835, -15.72974639402198527, 36.87390960531435979 ) ) ;
#116743=CARTESIAN_POINT ( 'NONE',  ( 16.52544592524342804, -4.483927247898539470, 58.54057627198103120 ) ) ;
#116744=CARTESIAN_POINT ( 'NONE',  ( 4.379528057220092307, 16.55341960407617563, 27.29275706135234358 ) ) ;
#116745=CARTESIAN_POINT ( 'NONE',  ( 10.72451020669871369, 18.67979575497193778, 72.08442372801899012 ) ) ;
#116747=CARTESIAN_POINT ( 'NONE',  ( 16.46253265017160672, -9.564922557960803928, 113.3322429386476955 ) ) ;
#116748=CARTESIAN_POINT ( 'NONE',  ( -16.52544592524335698, -4.483927247898792601, 78.95942372801901854 ) ) ;
#116749=CARTESIAN_POINT ( 'NONE',  ( -19.02544592524342804, 5.153800228976336051, 26.04057627198103120 ) ) ;
#116750=CARTESIAN_POINT ( 'NONE',  ( -5.153800228976328057, -19.02544592524343514, 87.29057627198103830 ) ) ;
#116751=CARTESIAN_POINT ( 'NONE',  ( 18.62759615963271287, -10.81492255796078972, 93.33224293864769550 ) ) ;
#116752=CARTESIAN_POINT ( 'NONE',  ( 16.53943276465976808, 0.05219959533934440121, 26.25109039468567573 ) ) ;
#116753=CARTESIAN_POINT ( 'NONE',  ( -14.34966873604960291, -8.224510206698953496, 56.66557627198103830 ) ) ;
#116754=CARTESIAN_POINT ( 'NONE',  ( 10.72451020669871369, 18.67979575497193778, 72.08442372801899012 ) ) ;
#116755=CARTESIAN_POINT ( 'NONE',  ( 4.483927247898790824, -16.52544592524335698, 105.2094237280190328 ) ) ;
#116756=CARTESIAN_POINT ( 'NONE',  ( 15.72974639402199770, -15.80617190586745480, 28.12390960531435979 ) ) ;
#116757=CARTESIAN_POINT ( 'NONE',  ( 5.049401038298163336, -19.05341960407611168, 112.7072429386476813 ) ) ;
#116759=CARTESIAN_POINT ( 'NONE',  ( 4.483927247898790824, -16.52544592524335698, 110.2094237280190185 ) ) ;
#116760=CARTESIAN_POINT ( 'NONE',  ( 14.34966873604972726, -8.224510206698740333, 60.83442372801901854 ) ) ;
#116761=CARTESIAN_POINT ( 'NONE',  ( -5.153800228976328057, -19.02544592524343514, 67.29057627198102409 ) ) ;
#116762=CARTESIAN_POINT ( 'NONE',  ( -16.51473224551069308, -9.474510206698971260, 86.66557627198102409 ) ) ;
#116763=CARTESIAN_POINT ( 'NONE',  ( -21.53943276465977519, -0.05219959533937600094, 68.75109039468568994 ) ) ;
#116764=CARTESIAN_POINT ( 'NONE',  ( -16.52544592524335698, -4.483927247898792601, 78.95942372801901854 ) ) ;
#116765=CARTESIAN_POINT ( 'NONE',  ( -14.34966873604960291, -8.224510206698953496, 61.66557627198103120 ) ) ;
#116766=CARTESIAN_POINT ( 'NONE',  ( -19.03943276465977164, 0.05219959533909376836, 61.24890960531436690 ) ) ;
#116768=CARTESIAN_POINT ( 'NONE',  ( 19.02544592524334988, 5.153800228976608722, 111.4594237280190043 ) ) ;
#116769=CARTESIAN_POINT ( 'NONE',  ( -12.06949235617756955, 12.14591786802309770, 110.6239096053143669 ) ) ;
#116770=CARTESIAN_POINT ( 'NONE',  ( 19.03943276465977164, -0.05219959533909143690, 83.74890960531436690 ) ) ;
#116771=CARTESIAN_POINT ( 'NONE',  ( 13.89961937509957401, 13.97604488694547697, 96.87609039468566152 ) ) ;
#116773=CARTESIAN_POINT ( 'NONE',  ( 5.823673210054444382, -21.52544592524334988, 105.2094237280190328 ) ) ;
#116774=CARTESIAN_POINT ( 'NONE',  ( 12.14591786802327356, -12.06949235617739191, 80.62609039468567573 ) ) ;
#116775=CARTESIAN_POINT ( 'NONE',  ( 19.02544592524334988, 5.153800228976608722, 91.45942372801900433 ) ) ;
#116776=CARTESIAN_POINT ( 'NONE',  ( 21.52544592524344225, -5.823673210054117533, 58.54057627198103120 ) ) ;
#116777=CARTESIAN_POINT ( 'NONE',  ( 14.29746914071037800, 8.314922557961029526, 56.66775706135235424 ) ) ;
#116779=CARTESIAN_POINT ( 'NONE',  ( 0.05219959533936267826, -19.03943276465977164, 50.00109039468566863 ) ) ;
#116780=CARTESIAN_POINT ( 'NONE',  ( 0.05219959533937995610, -21.53943276465977519, 95.00109039468568994 ) ) ;
#116781=CARTESIAN_POINT ( 'NONE',  ( 13.89961937509977652, -13.97604488694527269, 38.12390960531436690 ) ) ;
#116782=CARTESIAN_POINT ( 'NONE',  ( -13.97604488694527625, -13.89961937509977652, 71.87390960531433848 ) ) ;
#116783=CARTESIAN_POINT ( 'NONE',  ( -12.14591786802309592, -12.06949235617757132, 61.87390960531436690 ) ) ;
#116784=CARTESIAN_POINT ( 'NONE',  ( 5.823673210054444382, -21.52544592524334988, 90.20942372801903275 ) ) ;
#116785=CARTESIAN_POINT ( 'NONE',  ( -5.153800228976607833, 19.02544592524334988, 47.70942372801900433 ) ) ;
#116786=CARTESIAN_POINT ( 'NONE',  ( -13.97604488694547697, 13.89961937509957934, 48.12609039468566863 ) ) ;
#116787=CARTESIAN_POINT ( 'NONE',  ( -15.80617190586745835, -15.72974639402198527, 31.87390960531435979 ) ) ;
#116788=CARTESIAN_POINT ( 'NONE',  ( 15.80617190586769283, -15.72974639402175789, 100.6260903946857184 ) ) ;
#116789=CARTESIAN_POINT ( 'NONE',  ( 19.02544592524343514, -5.153800228976328945, 78.54057627198099567 ) ) ;
#116790=CARTESIAN_POINT ( 'NONE',  ( -0.05219959533937732626, 21.53943276465977519, 87.50109039468568994 ) ) ;
#116791=CARTESIAN_POINT ( 'NONE',  ( 21.55341960407610458, 5.719274019375980345, 53.95724293864770260 ) ) ;
#116792=CARTESIAN_POINT ( 'NONE',  ( 9.474510206698971260, -16.51473224551069308, 82.91557627198103830 ) ) ;
#116793=CARTESIAN_POINT ( 'NONE',  ( -13.97604488694547697, 13.89961937509957934, 78.12609039468567573 ) ) ;
#116794=CARTESIAN_POINT ( 'NONE',  ( 19.02544592524343514, -5.153800228976328945, 93.54057627198102409 ) ) ;
#116796=CARTESIAN_POINT ( 'NONE',  ( -13.97604488694547697, 13.89961937509957934, 98.12609039468566152 ) ) ;
#116797=CARTESIAN_POINT ( 'NONE',  ( -16.55341960407617563, 4.379528057220093196, 43.54275706135235424 ) ) ;
#116798=CARTESIAN_POINT ( 'NONE',  ( 8.224510206698953496, -14.34966873604960469, 107.9155762719810241 ) ) ;
#116799=CARTESIAN_POINT ( 'NONE',  ( 0.05219959533909260263, 19.03943276465977164, 74.99890960531435269 ) ) ;
#116800=CARTESIAN_POINT ( 'NONE',  ( -18.67979575497178146, -10.72451020669898902, 56.66557627198103830 ) ) ;
#116801=CARTESIAN_POINT ( 'NONE',  ( -16.52544592524335698, -4.483927247898792601, 28.95942372801902209 ) ) ;
#116802=CARTESIAN_POINT ( 'NONE',  ( 21.55341960407619695, -5.719274019375665929, 31.04275706135234714 ) ) ;
#116803=CARTESIAN_POINT ( 'NONE',  ( -5.823673210054431948, 21.52544592524334988, 77.70942372801900433 ) ) ;
#116804=CARTESIAN_POINT ( 'NONE',  ( 0.05219959533934541429, -16.53943276465976808, 85.00109039468568994 ) ) ;
#116805=CARTESIAN_POINT ( 'NONE',  ( -9.564922557960796823, -16.46253265017161027, 77.08224293864769550 ) ) ;
#116806=CARTESIAN_POINT ( 'NONE',  ( -16.55341960407611168, -4.379528057220339221, 76.45724293864769550 ) ) ;
#116807=CARTESIAN_POINT ( 'NONE',  ( -16.55341960407617563, 4.379528057220093196, 108.5427570613523756 ) ) ;
#116808=CARTESIAN_POINT ( 'NONE',  ( -16.51473224551082808, 9.474510206698731452, 58.33442372801900433 ) ) ;
#116809=CARTESIAN_POINT ( 'NONE',  ( 21.52544592524334988, 5.823673210054432836, 36.45942372801901143 ) ) ;
#116811=CARTESIAN_POINT ( 'NONE',  ( 8.314922557960818139, 14.29746914071049879, 84.58224293864769550 ) ) ;
#116812=CARTESIAN_POINT ( 'NONE',  ( -16.46253265017160317, 9.564922557960807481, 105.8322429386476955 ) ) ;
#116813=CARTESIAN_POINT ( 'NONE',  ( -0.05219959533934338120, 16.53943276465976808, 97.50109039468567573 ) ) ;
#116814=CARTESIAN_POINT ( 'NONE',  ( 18.67979575497194134, -10.72451020669871369, 75.83442372801900433 ) ) ;
#116815=CARTESIAN_POINT ( 'NONE',  ( -12.06949235617739369, -12.14591786802326823, 49.37609039468569705 ) ) ;
#116816=CARTESIAN_POINT ( 'NONE',  ( 0.05219959533937995610, -21.53943276465977519, 25.00109039468567218 ) ) ;
#116817=CARTESIAN_POINT ( 'NONE',  ( 4.379528057220339221, -16.55341960407611168, 77.70724293864770971 ) ) ;
#116819=CARTESIAN_POINT ( 'NONE',  ( 15.80617190586746368, 15.72974639402197994, 109.3739096053143811 ) ) ;
#116820=CARTESIAN_POINT ( 'NONE',  ( -14.34966873604960291, -8.224510206698953496, 56.66557627198103830 ) ) ;
#116821=CARTESIAN_POINT ( 'NONE',  ( -9.564922557960796823, -16.46253265017161027, 22.08224293864768839 ) ) ;
#116822=CARTESIAN_POINT ( 'NONE',  ( 5.719274019375991003, -21.55341960407610458, 32.70724293864770260 ) ) ;
#116823=CARTESIAN_POINT ( 'NONE',  ( -14.34966873604960291, -8.224510206698953496, 61.66557627198103120 ) ) ;
#116824=CARTESIAN_POINT ( 'NONE',  ( 21.53943276465977519, -0.05219959533907433946, 83.74890960531435269 ) ) ;
#116825=CARTESIAN_POINT ( 'NONE',  ( 5.049401038298161559, -19.05341960407611168, 72.70724293864768129 ) ) ;
#116826=CARTESIAN_POINT ( 'NONE',  ( -9.474510206698964154, 16.51473224551069663, 40.41557627198103120 ) ) ;
#116827=CARTESIAN_POINT ( 'NONE',  ( -0.05219959533936034679, 19.03943276465977164, 82.50109039468567573 ) ) ;
#116828=CARTESIAN_POINT ( 'NONE',  ( 15.80617190586769283, -15.72974639402175789, 50.62609039468568994 ) ) ;
#116829=CARTESIAN_POINT ( 'NONE',  ( -21.55341960407610458, -5.719274019375992779, 56.45724293864768839 ) ) ;
#116830=CARTESIAN_POINT ( 'NONE',  ( -19.03943276465977164, 0.05219959533909376836, 46.24890960531435979 ) ) ;
#116831=CARTESIAN_POINT ( 'NONE',  ( -5.153800228976328057, -19.02544592524343514, 72.29057627198102409 ) ) ;
#116833=CARTESIAN_POINT ( 'NONE',  ( -12.06949235617739369, -12.14591786802326823, 49.37609039468569705 ) ) ;
#116834=CARTESIAN_POINT ( 'NONE',  ( -15.80617190586768217, 15.72974639402176855, 33.12609039468569705 ) ) ;
#116836=CARTESIAN_POINT ( 'NONE',  ( 21.55341960407619695, -5.719274019375665929, 66.04275706135236135 ) ) ;
#116837=CARTESIAN_POINT ( 'NONE',  ( -9.474510206698964154, 16.51473224551069663, 110.4155762719810383 ) ) ;
#116838=CARTESIAN_POINT ( 'NONE',  ( 10.81492255796078972, 18.62759615963270932, 89.58224293864768129 ) ) ;
#116839=CARTESIAN_POINT ( 'NONE',  ( 0.05219959533937995610, -21.53943276465977519, 20.00109039468568639 ) ) ;
#116840=CARTESIAN_POINT ( 'NONE',  ( -14.29746914071037622, -8.314922557961029526, 54.16775706135235424 ) ) ;
#116841=CARTESIAN_POINT ( 'NONE',  ( 5.823673210054125526, 21.52544592524343514, 44.79057627198103120 ) ) ;
#116842=CARTESIAN_POINT ( 'NONE',  ( -10.81492255796105439, 18.62759615963255655, 112.9177570613523329 ) ) ;
#116843=CARTESIAN_POINT ( 'NONE',  ( -19.03943276465977164, 0.05219959533909376836, 61.24890960531436690 ) ) ;
#116844=CARTESIAN_POINT ( 'NONE',  ( 9.474510206698971260, -16.51473224551069308, 107.9155762719810383 ) ) ;
#116845=CARTESIAN_POINT ( 'NONE',  ( -13.97604488694527625, -13.89961937509977652, 86.87390960531436690 ) ) ;
#116847=CARTESIAN_POINT ( 'NONE',  ( -5.049401038297874678, -19.05341960407617918, 74.79275706135231871 ) ) ;
#116848=CARTESIAN_POINT ( 'NONE',  ( -0.05219959533907301413, -21.53943276465977519, 47.49890960531435979 ) ) ;
#116849=CARTESIAN_POINT ( 'NONE',  ( -0.05219959533910754901, -16.53943276465976808, 22.49890960531436335 ) ) ;
#116850=CARTESIAN_POINT ( 'NONE',  ( -5.153800228976607833, 19.02544592524334988, 87.70942372801897591 ) ) ;
#116851=CARTESIAN_POINT ( 'NONE',  ( -13.97604488694527625, -13.89961937509977652, 21.87390960531435979 ) ) ;
#116852=CARTESIAN_POINT ( 'NONE',  ( 10.72451020669871369, 18.67979575497193778, 112.0844237280190185 ) ) ;
#116853=CARTESIAN_POINT ( 'NONE',  ( -9.474510206698720793, -16.51473224551083518, 99.58442372801900433 ) ) ;
#116854=CARTESIAN_POINT ( 'NONE',  ( 5.049401038297881783, 19.05341960407617563, 42.29275706135234003 ) ) ;
#116856=CARTESIAN_POINT ( 'NONE',  ( -5.049401038298153566, 19.05341960407611168, 50.20724293864770260 ) ) ;
#116857=CARTESIAN_POINT ( 'NONE',  ( 14.34966873604960469, 8.224510206698951720, 64.16557627198102409 ) ) ;
#116858=CARTESIAN_POINT ( 'NONE',  ( 9.564922557960805705, 16.46253265017160317, 34.58224293864770260 ) ) ;
#116859=CARTESIAN_POINT ( 'NONE',  ( 14.34966873604960469, 8.224510206698951720, 34.16557627198102409 ) ) ;
#116860=CARTESIAN_POINT ( 'NONE',  ( 17.72696623605163779, -5.499999999999864997, 56.09811031808416715 ) ) ;
#116861=CARTESIAN_POINT ( 'NONE',  ( 8.224510206698742110, 14.34966873604972548, 102.0844237280190185 ) ) ;
#116862=CARTESIAN_POINT ( 'NONE',  ( -5.153800228976328057, -19.02544592524343514, 57.29057627198103120 ) ) ;
#116863=CARTESIAN_POINT ( 'NONE',  ( -9.564922557961040184, 16.46253265017147172, 27.91775706135232582 ) ) ;
#116864=CARTESIAN_POINT ( 'NONE',  ( 8.224510206698742110, 14.34966873604972548, 27.08442372801901854 ) ) ;
#116865=CARTESIAN_POINT ( 'NONE',  ( -21.55341960407610458, -5.719274019375992779, 41.45724293864769550 ) ) ;
#116866=CARTESIAN_POINT ( 'NONE',  ( -18.62759615963255300, -10.81492255796106328, 109.1677570613523613 ) ) ;
#116868=CARTESIAN_POINT ( 'NONE',  ( 9.564922557960805705, 16.46253265017160317, 64.58224293864769550 ) ) ;
#116869=CARTESIAN_POINT ( 'NONE',  ( -19.05341960407611168, -5.049401038298163336, 106.4572429386476955 ) ) ;
#116870=CARTESIAN_POINT ( 'NONE',  ( -19.05341960407611168, -5.049401038298163336, 101.4572429386476955 ) ) ;
#116872=CARTESIAN_POINT ( 'NONE',  ( -21.52544592524334988, -5.823673210054445271, 28.95942372801902209 ) ) ;
#116873=CARTESIAN_POINT ( 'NONE',  ( -16.55341960407611168, -4.379528057220339221, 96.45724293864770971 ) ) ;
#116874=CARTESIAN_POINT ( 'NONE',  ( 21.52544592524344225, -5.823673210054117533, 73.54057627198102409 ) ) ;
#116875=CARTESIAN_POINT ( 'NONE',  ( -5.153800228976328057, -19.02544592524343514, 72.29057627198102409 ) ) ;
#116876=CARTESIAN_POINT ( 'NONE',  ( 0.05219959533909260263, 19.03943276465977164, 79.99890960531436690 ) ) ;
#116877=CARTESIAN_POINT ( 'NONE',  ( -5.823673210054116645, -21.52544592524344225, 107.2905762719810525 ) ) ;
#116879=CARTESIAN_POINT ( 'NONE',  ( 13.97604488694527802, 13.89961937509977652, 74.37390960531436690 ) ) ;
#116881=CARTESIAN_POINT ( 'NONE',  ( -14.29746914071049879, 8.314922557960819915, 105.8322429386476955 ) ) ;
#116883=CARTESIAN_POINT ( 'NONE',  ( 0.05219959533909260263, 19.03943276465977164, 64.99890960531436690 ) ) ;
#116884=CARTESIAN_POINT ( 'NONE',  ( 16.51473224551083163, -9.474510206698727899, 90.83442372801900433 ) ) ;
#116885=CARTESIAN_POINT ( 'NONE',  ( 16.53943276465976808, -0.05219959533910856209, 93.74890960531436690 ) ) ;
#116886=CARTESIAN_POINT ( 'NONE',  ( 10.81492255796106328, -18.62759615963255655, 75.41775706135233293 ) ) ;
#116887=CARTESIAN_POINT ( 'NONE',  ( -9.474510206698964154, 16.51473224551069663, 45.41557627198103120 ) ) ;
#116888=CARTESIAN_POINT ( 'NONE',  ( -5.823673210054431948, 21.52544592524334988, 22.70942372801901499 ) ) ;
#116889=CARTESIAN_POINT ( 'NONE',  ( 10.72451020669898902, -18.67979575497178502, 107.9155762719810241 ) ) ;
#116891=CARTESIAN_POINT ( 'NONE',  ( -19.03943276465977164, 0.05219959533909376836, 66.24890960531436690 ) ) ;
#116892=CARTESIAN_POINT ( 'NONE',  ( 17.44279575226824974, 5.990770900252419651, 111.6644243248568245 ) ) ;
#116893=CARTESIAN_POINT ( 'NONE',  ( -5.153800228976607833, 19.02544592524334988, 102.7094237280189759 ) ) ;
#116894=CARTESIAN_POINT ( 'NONE',  ( -15.80617190586745835, -15.72974639402198527, 36.87390960531435979 ) ) ;
#116895=CARTESIAN_POINT ( 'NONE',  ( -21.55341960407619339, 5.719274019375674811, 58.54275706135235424 ) ) ;
#116896=CARTESIAN_POINT ( 'NONE',  ( 9.564922557960805705, 16.46253265017160317, 94.58224293864769550 ) ) ;
#116897=CARTESIAN_POINT ( 'NONE',  ( 16.51473224551083163, -9.474510206698727899, 80.83442372801899012 ) ) ;
#116898=CARTESIAN_POINT ( 'NONE',  ( -0.05219959533909027116, -19.03943276465977164, 52.49890960531436690 ) ) ;
#116899=CARTESIAN_POINT ( 'NONE',  ( 5.153800228976335163, 19.02544592524342804, 64.79057627198100988 ) ) ;
#116900=CARTESIAN_POINT ( 'NONE',  ( -16.52544592524342804, 4.483927247898546575, 86.04057627198102409 ) ) ;
#116901=CARTESIAN_POINT ( 'NONE',  ( -9.564922557960796823, -16.46253265017161027, 97.08224293864769550 ) ) ;
#116902=CARTESIAN_POINT ( 'NONE',  ( 8.314922557960818139, 14.29746914071049879, 94.58224293864769550 ) ) ;
#116903=CARTESIAN_POINT ( 'NONE',  ( -13.89961937509977652, 13.97604488694528158, 100.6239096053143669 ) ) ;
#116904=CARTESIAN_POINT ( 'NONE',  ( -16.53943276465976808, 0.05219959533911058130, 41.24890960531435269 ) ) ;
#116905=CARTESIAN_POINT ( 'NONE',  ( -5.153800228976328057, -19.02544592524343514, 32.29057627198102409 ) ) ;
#116907=CARTESIAN_POINT ( 'NONE',  ( -21.52544592524334988, -5.823673210054445271, 53.95942372801900433 ) ) ;
#116908=CARTESIAN_POINT ( 'NONE',  ( -13.89961937509957401, -13.97604488694547875, 74.37609039468566152 ) ) ;
#116909=CARTESIAN_POINT ( 'NONE',  ( -8.224510206698948167, 14.34966873604960824, 50.41557627198103120 ) ) ;
#116910=CARTESIAN_POINT ( 'NONE',  ( -18.67979575497178146, -10.72451020669898902, 101.6655762719810383 ) ) ;
#116911=CARTESIAN_POINT ( 'NONE',  ( -15.80617190586745835, -15.72974639402198527, 31.87390960531435979 ) ) ;
#116912=CARTESIAN_POINT ( 'NONE',  ( 12.06949235617757843, -12.14591786802309237, 88.12390960531436690 ) ) ;
#116913=CARTESIAN_POINT ( 'NONE',  ( -5.049401038298153566, 19.05341960407611168, 55.20724293864769550 ) ) ;
#116914=CARTESIAN_POINT ( 'NONE',  ( 0.05219959533910956823, 16.53943276465976808, 24.99890960531435624 ) ) ;
#116915=CARTESIAN_POINT ( 'NONE',  ( -4.379528057220086978, -16.55341960407618274, 99.79275706135234714 ) ) ;
#116916=CARTESIAN_POINT ( 'NONE',  ( 4.483927247898790824, -16.52544592524335698, 75.20942372801901854 ) ) ;
#116917=CARTESIAN_POINT ( 'NONE',  ( 0.05219959533936267826, -19.03943276465977164, 20.00109039468567218 ) ) ;
#116918=CARTESIAN_POINT ( 'NONE',  ( 5.153800228976335163, 19.02544592524342804, 99.79057627198102409 ) ) ;
#116919=CARTESIAN_POINT ( 'NONE',  ( -13.97604488694527625, -13.89961937509977652, 76.87390960531433848 ) ) ;
#116920=CARTESIAN_POINT ( 'NONE',  ( -16.46253265017160317, 9.564922557960807481, 40.83224293864769550 ) ) ;
#116921=CARTESIAN_POINT ( 'NONE',  ( 16.53943276465976808, -0.05219959533910856209, 43.74890960531435979 ) ) ;
#116922=CARTESIAN_POINT ( 'NONE',  ( 5.153800228976335163, 19.02544592524342804, 114.7905762719810241 ) ) ;
#116923=CARTESIAN_POINT ( 'NONE',  ( 13.97604488694527802, 13.89961937509977652, 109.3739096053143669 ) ) ;
#116924=CARTESIAN_POINT ( 'NONE',  ( 21.52544592524344225, -5.823673210054117533, 38.54057627198103120 ) ) ;
#116925=CARTESIAN_POINT ( 'NONE',  ( 8.314922557960818139, 14.29746914071049879, 74.58224293864768129 ) ) ;
#116926=CARTESIAN_POINT ( 'NONE',  ( 14.29746914071037800, 8.314922557961029526, 21.66775706135235069 ) ) ;
#116927=EDGE_LOOP ( 'NONE', ( #11959, #135427, #197425, #47827, #38985, #97999 ) ) ;
#116928=CARTESIAN_POINT ( 'NONE',  ( -16.55341960407611168, -4.379528057220339221, 61.45724293864770260 ) ) ;
#116930=CARTESIAN_POINT ( 'NONE',  ( -19.02544592524334988, -5.153800228976617603, 58.95942372801900433 ) ) ;
#116931=CARTESIAN_POINT ( 'NONE',  ( -9.564922557960796823, -16.46253265017161027, 102.0822429386477097 ) ) ;
#116932=CARTESIAN_POINT ( 'NONE',  ( -0.05219959533936034679, 19.03943276465977164, 77.50109039468566152 ) ) ;
#116934=CARTESIAN_POINT ( 'NONE',  ( 5.049401038297881783, 19.05341960407617563, 107.2927570613523187 ) ) ;
#116935=CARTESIAN_POINT ( 'NONE',  ( 12.14591786802327356, -12.06949235617739191, 100.6260903946857184 ) ) ;
#116936=CARTESIAN_POINT ( 'NONE',  ( -13.89961937509977652, 13.97604488694528158, 45.62390960531433848 ) ) ;
#116937=CARTESIAN_POINT ( 'NONE',  ( -10.72451020669898014, 18.67979575497178502, 35.41557627198102409 ) ) ;
#116938=CARTESIAN_POINT ( 'NONE',  ( -10.81492255796105439, 18.62759615963255655, 52.91775706135235424 ) ) ;
#116939=CARTESIAN_POINT ( 'NONE',  ( 19.33860699428957375, 5.500000000000045297, 38.39890772129063379 ) ) ;
#116940=CARTESIAN_POINT ( 'NONE',  ( 12.06949235617739724, 12.14591786802326823, 21.87609039468567573 ) ) ;
#116941=CARTESIAN_POINT ( 'NONE',  ( 17.50000000000000000, 4.189786006557876696, 22.00000000000000711 ) ) ;
#116942=CARTESIAN_POINT ( 'NONE',  ( 16.51473224551069308, 9.474510206698969483, 69.16557627198102409 ) ) ;
#116944=CARTESIAN_POINT ( 'NONE',  ( -12.14591786802309592, -12.06949235617757132, 86.87390960531438111 ) ) ;
#116945=CARTESIAN_POINT ( 'NONE',  ( -9.474510206698964154, 16.51473224551069663, 80.41557627198103830 ) ) ;
#116947=CARTESIAN_POINT ( 'NONE',  ( 9.474510206698971260, -16.51473224551069308, 92.91557627198103830 ) ) ;
#116949=CARTESIAN_POINT ( 'NONE',  ( 5.049401038297881783, 19.05341960407617563, 97.29275706135233293 ) ) ;
#116950=CARTESIAN_POINT ( 'NONE',  ( 10.81492255796078972, 18.62759615963270932, 64.58224293864769550 ) ) ;
#116951=CARTESIAN_POINT ( 'NONE',  ( -5.049401038298153566, 19.05341960407611168, 30.20724293864768839 ) ) ;
#116952=CARTESIAN_POINT ( 'NONE',  ( -19.05341960407617563, 5.049401038297882671, 53.54275706135231871 ) ) ;
#116953=CARTESIAN_POINT ( 'NONE',  ( 0.05219959533909260263, 19.03943276465977164, 49.99890960531435979 ) ) ;
#116954=CARTESIAN_POINT ( 'NONE',  ( 13.97604488694527802, 13.89961937509977652, 99.37390960531436690 ) ) ;
#116955=EDGE_CURVE ( 'NONE', #73688, #165524, #102396, .T. ) ;
#116957=CARTESIAN_POINT ( 'NONE',  ( -21.55341960407610458, -5.719274019375992779, 96.45724293864770971 ) ) ;
#116958=CARTESIAN_POINT ( 'NONE',  ( 12.14591786802309770, 12.06949235617756955, 89.37390960531435269 ) ) ;
#116959=CARTESIAN_POINT ( 'NONE',  ( -19.02544592524342804, 5.153800228976336051, 86.04057627198103830 ) ) ;
#116960=CARTESIAN_POINT ( 'NONE',  ( 0.05219959533936267826, -19.03943276465977164, 60.00109039468566863 ) ) ;
#116961=CARTESIAN_POINT ( 'NONE',  ( -21.55341960407610458, -5.719274019375992779, 86.45724293864770971 ) ) ;
#116962=CARTESIAN_POINT ( 'NONE',  ( 15.80617190586746368, 15.72974639402197994, 79.37390960531436690 ) ) ;
#116963=CARTESIAN_POINT ( 'NONE',  ( 8.314922557960818139, 14.29746914071049879, 29.58224293864769905 ) ) ;
#116964=CARTESIAN_POINT ( 'NONE',  ( 10.81492255796106328, -18.62759615963255655, 110.4177570613523756 ) ) ;
#116965=CARTESIAN_POINT ( 'NONE',  ( 12.06949235617739724, 12.14591786802326823, 51.87609039468568284 ) ) ;
#116966=CARTESIAN_POINT ( 'NONE',  ( -19.02544592524342804, 5.153800228976336051, 86.04057627198103830 ) ) ;
#116967=CARTESIAN_POINT ( 'NONE',  ( 19.02544592524343514, -5.153800228976328945, 28.54057627198102409 ) ) ;
#116968=CARTESIAN_POINT ( 'NONE',  ( -10.81492255796105439, 18.62759615963255655, 32.91775706135234714 ) ) ;
#116969=CARTESIAN_POINT ( 'NONE',  ( -18.62759615963255300, -10.81492255796106328, 54.16775706135235424 ) ) ;
#116970=CARTESIAN_POINT ( 'NONE',  ( -19.03943276465977164, 0.05219959533909376836, 46.24890960531435979 ) ) ;
#116971=CARTESIAN_POINT ( 'NONE',  ( -21.53943276465977519, -0.05219959533937600094, 18.75109039468568639 ) ) ;
#116972=CARTESIAN_POINT ( 'NONE',  ( 9.564922557961047289, -16.46253265017146816, 55.41775706135234003 ) ) ;
#116973=CARTESIAN_POINT ( 'NONE',  ( 19.05341960407617918, -5.049401038297876454, 71.04275706135234714 ) ) ;
#116974=CARTESIAN_POINT ( 'NONE',  ( 9.474510206698971260, -16.51473224551069308, 27.91557627198103120 ) ) ;
#116975=CARTESIAN_POINT ( 'NONE',  ( -4.483927247898782831, 16.52544592524335698, 77.70942372801900433 ) ) ;
#116976=CARTESIAN_POINT ( 'NONE',  ( 5.153800228976335163, 19.02544592524342804, 49.79057627198100988 ) ) ;
#116978=CARTESIAN_POINT ( 'NONE',  ( 5.049401038298161559, -19.05341960407611168, 92.70724293864769550 ) ) ;
#116979=CARTESIAN_POINT ( 'NONE',  ( 12.14591786802309770, 12.06949235617756955, 114.3739096053143527 ) ) ;
#116980=CARTESIAN_POINT ( 'NONE',  ( 21.55341960407610458, 5.719274019375980345, 78.95724293864769550 ) ) ;
#116981=CARTESIAN_POINT ( 'NONE',  ( 0.05219959533934541429, -16.53943276465976808, 55.00109039468568284 ) ) ;
#116982=CARTESIAN_POINT ( 'NONE',  ( 19.05341960407617918, -5.049401038297876454, 21.04275706135232582 ) ) ;
#116983=CARTESIAN_POINT ( 'NONE',  ( -0.05219959533909027116, -19.03943276465977164, 47.49890960531435979 ) ) ;
#116984=CARTESIAN_POINT ( 'NONE',  ( 4.379528057220339221, -16.55341960407611168, 32.70724293864770260 ) ) ;
#116985=CARTESIAN_POINT ( 'NONE',  ( 8.224510206698953496, -14.34966873604960469, 67.91557627198102409 ) ) ;
#116986=CARTESIAN_POINT ( 'NONE',  ( 5.153800228976335163, 19.02544592524342804, 79.79057627198102409 ) ) ;
#116987=CARTESIAN_POINT ( 'NONE',  ( -18.67979575497193778, 10.72451020669871902, 43.33442372801901143 ) ) ;
#116988=CARTESIAN_POINT ( 'NONE',  ( 13.89961937509977652, -13.97604488694527269, 93.12390960531436690 ) ) ;
#116989=CARTESIAN_POINT ( 'NONE',  ( 5.823673210054444382, -21.52544592524334988, 85.20942372801901854 ) ) ;
#116990=CARTESIAN_POINT ( 'NONE',  ( -16.53943276465976808, -0.05219959533934237506, 68.75109039468568994 ) ) ;
#116991=CARTESIAN_POINT ( 'NONE',  ( -5.153800228976328057, -19.02544592524343514, 112.2905762719810099 ) ) ;
#116992=CARTESIAN_POINT ( 'NONE',  ( 5.823673210054125526, 21.52544592524343514, 89.79057627198103830 ) ) ;
#116993=CARTESIAN_POINT ( 'NONE',  ( 14.29746914071049879, -8.314922557960816363, 43.33224293864769550 ) ) ;
#116994=CARTESIAN_POINT ( 'NONE',  ( -9.474510206698964154, 16.51473224551069663, 30.41557627198102054 ) ) ;
#116995=CARTESIAN_POINT ( 'NONE',  ( -16.52544592524335698, -4.483927247898792601, 53.95942372801900433 ) ) ;
#116996=CARTESIAN_POINT ( 'NONE',  ( 12.06949235617757843, -12.14591786802309237, 68.12390960531436690 ) ) ;
#116997=CARTESIAN_POINT ( 'NONE',  ( 0.05219959533909260263, 19.03943276465977164, 109.9989096053143669 ) ) ;
#116998=CARTESIAN_POINT ( 'NONE',  ( -15.80617190586745835, -15.72974639402198527, 36.87390960531435979 ) ) ;
#116999=CARTESIAN_POINT ( 'NONE',  ( -18.67979575497193778, 10.72451020669871902, 113.3344237280190328 ) ) ;
#117000=CARTESIAN_POINT ( 'NONE',  ( -8.314922557960811034, -14.29746914071050412, 102.0822429386476955 ) ) ;
#117001=CARTESIAN_POINT ( 'NONE',  ( 19.02544592524343514, -5.153800228976328945, 103.5405762719809957 ) ) ;
#117003=CARTESIAN_POINT ( 'NONE',  ( 16.52544592524335698, 4.483927247898782831, 56.45942372801902565 ) ) ;
#117004=CARTESIAN_POINT ( 'NONE',  ( -9.564922557960796823, -16.46253265017161027, 57.08224293864769550 ) ) ;
#117005=FACE_OUTER_BOUND ( 'NONE', #21341, .T. ) ;
#117006=CARTESIAN_POINT ( 'NONE',  ( 19.02544592524334988, 5.153800228976608722, 51.45942372801900433 ) ) ;
#117007=CARTESIAN_POINT ( 'NONE',  ( 14.29746914071037800, 8.314922557961029526, 96.66775706135234714 ) ) ;
#117008=CARTESIAN_POINT ( 'NONE',  ( -9.564922557961040184, 16.46253265017147172, 92.91775706135233293 ) ) ;
#117009=CARTESIAN_POINT ( 'NONE',  ( 21.55341960407619695, -5.719274019375665929, 61.04275706135234714 ) ) ;
#117010=CARTESIAN_POINT ( 'NONE',  ( -5.049401038298153566, 19.05341960407611168, 75.20724293864769550 ) ) ;
#117011=CARTESIAN_POINT ( 'NONE',  ( 10.81492255796078972, 18.62759615963270932, 89.58224293864768129 ) ) ;
#117012=CARTESIAN_POINT ( 'NONE',  ( -16.52544592524342804, 4.483927247898546575, 106.0405762719810525 ) ) ;
#117013=CARTESIAN_POINT ( 'NONE',  ( -19.03943276465977164, -0.05219959533935918106, 78.75109039468567573 ) ) ;
#117014=CARTESIAN_POINT ( 'NONE',  ( 5.719274019375991003, -21.55341960407610458, 77.70724293864770971 ) ) ;
#117015=CARTESIAN_POINT ( 'NONE',  ( -0.05219959533936034679, 19.03943276465977164, 37.50109039468567573 ) ) ;
#117017=CARTESIAN_POINT ( 'NONE',  ( -10.72451020669898014, 18.67979575497178502, 85.41557627198102409 ) ) ;
#117018=CARTESIAN_POINT ( 'NONE',  ( -19.52217212775657984, 5.500000000000115463, 54.93993709005259518 ) ) ;
#117019=CARTESIAN_POINT ( 'NONE',  ( 19.02544592524343514, -5.153800228976328945, 68.54057627198103830 ) ) ;
#117020=CARTESIAN_POINT ( 'NONE',  ( -17.59860650958991002, -7.585241751807008548, 91.57662985737506744 ) ) ;
#117021=CARTESIAN_POINT ( 'NONE',  ( 19.05341960407617918, -5.049401038297876454, 111.0427570613523329 ) ) ;
#117022=CARTESIAN_POINT ( 'NONE',  ( -16.51473224551082808, 9.474510206698731452, 98.33442372801900433 ) ) ;
#117023=CARTESIAN_POINT ( 'NONE',  ( 9.564922557960805705, 16.46253265017160317, 44.58224293864769550 ) ) ;
#117024=CARTESIAN_POINT ( 'NONE',  ( -5.823673210054116645, -21.52544592524344225, 22.29057627198102765 ) ) ;
#117025=CARTESIAN_POINT ( 'NONE',  ( 15.80617190586746368, 15.72974639402197994, 104.3739096053143669 ) ) ;
#117026=CARTESIAN_POINT ( 'NONE',  ( 0.05219959533910956823, 16.53943276465976808, 44.99890960531435979 ) ) ;
#117027=CARTESIAN_POINT ( 'NONE',  ( -21.55341960407619339, 5.719274019375674811, 78.54275706135236135 ) ) ;
#117028=CARTESIAN_POINT ( 'NONE',  ( 14.29746914071037800, 8.314922557961029526, 26.66775706135235424 ) ) ;
#117029=CARTESIAN_POINT ( 'NONE',  ( 13.89961937509957401, 13.97604488694547697, 31.87609039468566863 ) ) ;
#117030=CARTESIAN_POINT ( 'NONE',  ( -16.53943276465976808, 0.05219959533911058130, 31.24890960531435979 ) ) ;
#117031=CARTESIAN_POINT ( 'NONE',  ( 15.80617190586769283, -15.72974639402175789, 20.62609039468568639 ) ) ;
#117032=CARTESIAN_POINT ( 'NONE',  ( 12.14591786802309770, 12.06949235617756955, 44.37390960531435979 ) ) ;
#117033=CARTESIAN_POINT ( 'NONE',  ( 9.564922557961047289, -16.46253265017146816, 95.41775706135233293 ) ) ;
#117034=CARTESIAN_POINT ( 'NONE',  ( -19.05341960407617563, 5.049401038297882671, 68.54275706135230450 ) ) ;
#117035=CARTESIAN_POINT ( 'NONE',  ( -21.53943276465977519, -0.05219959533937600094, 73.75109039468567573 ) ) ;
#117036=CARTESIAN_POINT ( 'NONE',  ( 16.46253265017146816, 9.564922557961045513, 51.66775706135233293 ) ) ;
#117037=CARTESIAN_POINT ( 'NONE',  ( -5.153800228976328057, -19.02544592524343514, 27.29057627198103120 ) ) ;
#117038=CARTESIAN_POINT ( 'NONE',  ( -10.72451020669898014, 18.67979575497178502, 40.41557627198103120 ) ) ;
#117039=CARTESIAN_POINT ( 'NONE',  ( -4.379528057220328563, 16.55341960407611168, 45.20724293864769550 ) ) ;
#117040=CARTESIAN_POINT ( 'NONE',  ( -18.87580814761077264, 5.499999999999961808, 95.87172394265761000 ) ) ;
#117041=CARTESIAN_POINT ( 'NONE',  ( 5.153800228976615827, -19.02544592524334988, 20.20942372801899722 ) ) ;
#117042=CARTESIAN_POINT ( 'NONE',  ( 14.34966873604972726, -8.224510206698740333, 80.83442372801901854 ) ) ;
#117043=CARTESIAN_POINT ( 'NONE',  ( -16.52544592524342804, 4.483927247898546575, 46.04057627198103830 ) ) ;
#117044=CARTESIAN_POINT ( 'NONE',  ( -15.80617190586768217, 15.72974639402176855, 78.12609039468570415 ) ) ;
#117045=CARTESIAN_POINT ( 'NONE',  ( -21.53943276465977519, -0.05219959533937600094, 83.75109039468568994 ) ) ;
#117046=CARTESIAN_POINT ( 'NONE',  ( 18.67979575497178502, 10.72451020669898547, 79.16557627198103830 ) ) ;
#117047=CARTESIAN_POINT ( 'NONE',  ( -16.51473224551069308, -9.474510206698971260, 31.66557627198102054 ) ) ;
#117048=CARTESIAN_POINT ( 'NONE',  ( 15.80617190586769283, -15.72974639402175789, 55.62609039468568284 ) ) ;
#117049=CARTESIAN_POINT ( 'NONE',  ( -9.474510206698964154, 16.51473224551069663, 40.41557627198103120 ) ) ;
#117050=CARTESIAN_POINT ( 'NONE',  ( -16.51473224551069308, -9.474510206698971260, 56.66557627198103120 ) ) ;
#117051=CARTESIAN_POINT ( 'NONE',  ( -8.224510206698948167, 14.34966873604960824, 95.41557627198102409 ) ) ;
#117052=CARTESIAN_POINT ( 'NONE',  ( 19.05341960407611168, 5.049401038298154454, 93.95724293864769550 ) ) ;
#117053=CARTESIAN_POINT ( 'NONE',  ( 4.483927247898545687, 16.52544592524342804, 44.79057627198103120 ) ) ;
#117054=CARTESIAN_POINT ( 'NONE',  ( 12.06949235617757843, -12.14591786802309237, 108.1239096053143811 ) ) ;
#117055=CARTESIAN_POINT ( 'NONE',  ( -10.72451020669898014, 18.67979575497178502, 85.41557627198102409 ) ) ;
#117056=CARTESIAN_POINT ( 'NONE',  ( -18.67979575497193778, 10.72451020669871902, 23.33442372801901499 ) ) ;
#117058=CARTESIAN_POINT ( 'NONE',  ( 5.153800228976335163, 19.02544592524342804, 84.79057627198099567 ) ) ;
#117059=CARTESIAN_POINT ( 'NONE',  ( -19.03943276465977164, -0.05219959533935918106, 113.7510903946856757 ) ) ;
#117060=CARTESIAN_POINT ( 'NONE',  ( -18.62759615963270932, 10.81492255796079327, 70.83224293864770971 ) ) ;
#117061=CARTESIAN_POINT ( 'NONE',  ( -21.55341960407619339, 5.719274019375674811, 93.54275706135234714 ) ) ;
#117062=CARTESIAN_POINT ( 'NONE',  ( 19.02544592524343514, -5.153800228976328945, 78.54057627198099567 ) ) ;
#117063=CARTESIAN_POINT ( 'NONE',  ( -21.53943276465977519, -0.05219959533937600094, 28.75109039468567929 ) ) ;
#117064=CARTESIAN_POINT ( 'NONE',  ( 19.05341960407611168, 5.049401038298154454, 113.9572429386477097 ) ) ;
#117065=CARTESIAN_POINT ( 'NONE',  ( -8.314922557961024197, 14.29746914071037800, 92.91775706135236135 ) ) ;
#117066=CARTESIAN_POINT ( 'NONE',  ( 0.05219959533937995610, -21.53943276465977519, 65.00109039468568994 ) ) ;
#117067=CARTESIAN_POINT ( 'NONE',  ( 18.67979575497194134, -10.72451020669871369, 100.8344237280190185 ) ) ;
#117068=CARTESIAN_POINT ( 'NONE',  ( -14.29746914071037622, -8.314922557961029526, 79.16775706135234714 ) ) ;
#117069=CARTESIAN_POINT ( 'NONE',  ( -15.72974639402176322, -15.80617190586768395, 34.37609039468568284 ) ) ;
#117070=CARTESIAN_POINT ( 'NONE',  ( 5.049401038298161559, -19.05341960407611168, 22.70724293864769194 ) ) ;
#117071=CARTESIAN_POINT ( 'NONE',  ( 21.53943276465977519, 0.05219959533937863772, 96.25109039468568994 ) ) ;
#117072=CARTESIAN_POINT ( 'NONE',  ( 19.03943276465977164, -0.05219959533909143690, 88.74890960531436690 ) ) ;
#117073=CARTESIAN_POINT ( 'NONE',  ( 0.05219959533907565091, 21.53943276465977519, 84.99890960531436690 ) ) ;
#117074=CARTESIAN_POINT ( 'NONE',  ( 16.51473224551083163, -9.474510206698727899, 65.83442372801900433 ) ) ;
#117075=CARTESIAN_POINT ( 'NONE',  ( 19.25176906914650488, 5.499999999999744205, 83.49927264242278113 ) ) ;
#117076=CARTESIAN_POINT ( 'NONE',  ( -0.05219959533907301413, -21.53943276465977519, 47.49890960531435979 ) ) ;
#117077=CARTESIAN_POINT ( 'NONE',  ( -0.05219959533909027116, -19.03943276465977164, 97.49890960531436690 ) ) ;
#117078=CARTESIAN_POINT ( 'NONE',  ( -16.53943276465976808, 0.05219959533911058130, 46.24890960531435979 ) ) ;
#117081=CARTESIAN_POINT ( 'NONE',  ( 0.05219959533936267826, -19.03943276465977164, 80.00109039468567573 ) ) ;
#117082=CARTESIAN_POINT ( 'NONE',  ( -17.49999999999999645, 5.500000000000001776, 103.7176903769643701 ) ) ;
#117083=CARTESIAN_POINT ( 'NONE',  ( -19.03943276465977164, -0.05219959533935918106, 108.7510903946856615 ) ) ;
#117084=CARTESIAN_POINT ( 'NONE',  ( 21.52544592524344225, -5.823673210054117533, 88.54057627198103830 ) ) ;
#117085=CARTESIAN_POINT ( 'NONE',  ( -12.06949235617756955, 12.14591786802309770, 70.62390960531436690 ) ) ;
#117086=CARTESIAN_POINT ( 'NONE',  ( 5.153800228976335163, 19.02544592524342804, 104.7905762719809957 ) ) ;
#117087=CARTESIAN_POINT ( 'NONE',  ( 8.314922557961029526, -14.29746914071037800, 50.41775706135235424 ) ) ;
#117088=CARTESIAN_POINT ( 'NONE',  ( -5.153800228976328057, -19.02544592524343514, 57.29057627198103120 ) ) ;
#117089=CARTESIAN_POINT ( 'NONE',  ( 18.67979575497194134, -10.72451020669871369, 20.83442372801901143 ) ) ;
#117090=CARTESIAN_POINT ( 'NONE',  ( 0.05219959533936267826, -19.03943276465977164, 80.00109039468567573 ) ) ;
#117091=CARTESIAN_POINT ( 'NONE',  ( -0.05219959533909027116, -19.03943276465977164, 97.49890960531436690 ) ) ;
#117092=CARTESIAN_POINT ( 'NONE',  ( 0.05219959533909260263, 19.03943276465977164, 74.99890960531435269 ) ) ;
#117093=CARTESIAN_POINT ( 'NONE',  ( -18.67979575497178146, -10.72451020669898902, 81.66557627198103830 ) ) ;
#117094=CARTESIAN_POINT ( 'NONE',  ( -16.46253265017160317, 9.564922557960807481, 50.83224293864770260 ) ) ;
#117096=CARTESIAN_POINT ( 'NONE',  ( -12.14591786802309592, -12.06949235617757132, 51.87390960531437401 ) ) ;
#117097=CARTESIAN_POINT ( 'NONE',  ( -16.46253265017160317, 9.564922557960807481, 105.8322429386476955 ) ) ;
#117099=CARTESIAN_POINT ( 'NONE',  ( 19.02544592524334988, 5.153800228976608722, 66.45942372801899012 ) ) ;
#117100=CARTESIAN_POINT ( 'NONE',  ( -18.67979575497178146, -10.72451020669898902, 91.66557627198103830 ) ) ;
#117101=CARTESIAN_POINT ( 'NONE',  ( 19.02544592524334988, 5.153800228976608722, 56.45942372801898301 ) ) ;
#117102=CARTESIAN_POINT ( 'NONE',  ( 19.05341960407611168, 5.049401038298154454, 103.9572429386476671 ) ) ;
#117103=CARTESIAN_POINT ( 'NONE',  ( -17.49999999999999289, 3.850315288878790376, 114.2662913060345176 ) ) ;
#117104=CARTESIAN_POINT ( 'NONE',  ( -10.72451020669898014, 18.67979575497178502, 40.41557627198103120 ) ) ;
#117105=CARTESIAN_POINT ( 'NONE',  ( -5.049401038298153566, 19.05341960407611168, 70.20724293864769550 ) ) ;
#117106=CARTESIAN_POINT ( 'NONE',  ( 5.823673210054444382, -21.52544592524334988, 60.20942372801902565 ) ) ;
#117107=CARTESIAN_POINT ( 'NONE',  ( -5.049401038298153566, 19.05341960407611168, 35.20724293864768839 ) ) ;
#117108=CARTESIAN_POINT ( 'NONE',  ( 14.29746914071049879, -8.314922557960816363, 68.33224293864769550 ) ) ;
#117110=CARTESIAN_POINT ( 'NONE',  ( 0.05219959533934541429, -16.53943276465976808, 20.00109039468568639 ) ) ;
#117111=CARTESIAN_POINT ( 'NONE',  ( -10.72451020669870658, -18.67979575497194134, 54.58442372801901143 ) ) ;
#117113=CARTESIAN_POINT ( 'NONE',  ( -19.02544592524342804, 5.153800228976336051, 111.0405762719810099 ) ) ;
#117114=CARTESIAN_POINT ( 'NONE',  ( -13.97604488694547697, 13.89961937509957934, 63.12609039468566152 ) ) ;
#117116=CARTESIAN_POINT ( 'NONE',  ( 21.52544592524334988, 5.823673210054432836, 26.45942372801901854 ) ) ;
#117117=CARTESIAN_POINT ( 'NONE',  ( 0.05219959533909260263, 19.03943276465977164, 54.99890960531435979 ) ) ;
#117118=CARTESIAN_POINT ( 'NONE',  ( -12.06949235617739369, -12.14591786802326823, 34.37609039468568284 ) ) ;
#117120=CARTESIAN_POINT ( 'NONE',  ( -5.049401038297874678, -19.05341960407617918, 24.79275706135233648 ) ) ;
#117121=CARTESIAN_POINT ( 'NONE',  ( -19.02544592524342804, 5.153800228976336051, 41.04057627198103120 ) ) ;
#117122=CARTESIAN_POINT ( 'NONE',  ( 16.51473224551083163, -9.474510206698727899, 20.83442372801899722 ) ) ;
#117123=CARTESIAN_POINT ( 'NONE',  ( 0.05219959533934541429, -16.53943276465976808, 90.00109039468567573 ) ) ;
#117124=CARTESIAN_POINT ( 'NONE',  ( 0.05219959533909260263, 19.03943276465977164, 89.99890960531436690 ) ) ;
#117125=CARTESIAN_POINT ( 'NONE',  ( -21.53943276465977519, -0.05219959533937600094, 73.75109039468567573 ) ) ;
#117127=CARTESIAN_POINT ( 'NONE',  ( -19.05341960407611168, -5.049401038298163336, 106.4572429386476955 ) ) ;
#117129=CARTESIAN_POINT ( 'NONE',  ( 12.14591786802327356, -12.06949235617739191, 50.62609039468568994 ) ) ;
#117130=CARTESIAN_POINT ( 'NONE',  ( -5.823673210054431948, 21.52544592524334988, 77.70942372801900433 ) ) ;
#117131=CARTESIAN_POINT ( 'NONE',  ( 5.719274019375673035, 21.55341960407619339, 97.29275706135234714 ) ) ;
#117133=CARTESIAN_POINT ( 'NONE',  ( -8.224510206698735004, -14.34966873604973081, 29.58442372801901854 ) ) ;
#117134=CARTESIAN_POINT ( 'NONE',  ( 5.153800228976335163, 19.02544592524342804, 84.79057627198099567 ) ) ;
#117135=CARTESIAN_POINT ( 'NONE',  ( 5.153800228976335163, 19.02544592524342804, 114.7905762719810241 ) ) ;
#117137=CARTESIAN_POINT ( 'NONE',  ( 17.31747979337947640, 6.344076630961015262, 43.87944868065184068 ) ) ;
#117138=CARTESIAN_POINT ( 'NONE',  ( 9.474510206698971260, -16.51473224551069308, 32.91557627198102409 ) ) ;
#117139=CARTESIAN_POINT ( 'NONE',  ( -10.72451020669898014, 18.67979575497178502, 45.41557627198103830 ) ) ;
#117140=CARTESIAN_POINT ( 'NONE',  ( -8.224510206698735004, -14.34966873604973081, 104.5844237280190185 ) ) ;
#117141=CARTESIAN_POINT ( 'NONE',  ( 14.34966873604960469, 8.224510206698951720, 79.16557627198103830 ) ) ;
#117142=CARTESIAN_POINT ( 'NONE',  ( -19.02544592524342804, 5.153800228976336051, 71.04057627198099567 ) ) ;
#117143=CARTESIAN_POINT ( 'NONE',  ( -15.72974639402176322, -15.80617190586768395, 99.37609039468568994 ) ) ;
#117144=CARTESIAN_POINT ( 'NONE',  ( -12.06949235617739369, -12.14591786802326823, 19.37609039468568639 ) ) ;
#117145=CARTESIAN_POINT ( 'NONE',  ( 0.05219959533910956823, 16.53943276465976808, 89.99890960531438111 ) ) ;
#117146=CARTESIAN_POINT ( 'NONE',  ( -21.55341960407619339, 5.719274019375674811, 43.54275706135235424 ) ) ;
#117147=CARTESIAN_POINT ( 'NONE',  ( 10.72451020669898902, -18.67979575497178502, 77.91557627198102409 ) ) ;
#117148=CARTESIAN_POINT ( 'NONE',  ( -0.05219959533936034679, 19.03943276465977164, 47.50109039468566863 ) ) ;
#117150=CARTESIAN_POINT ( 'NONE',  ( -19.02544592524342804, 5.153800228976336051, 96.04057627198103830 ) ) ;
#117151=CARTESIAN_POINT ( 'NONE',  ( 16.53943276465976808, -0.05219959533910856209, 63.74890960531435979 ) ) ;
#117152=CARTESIAN_POINT ( 'NONE',  ( 12.06949235617757843, -12.14591786802309237, 53.12390960531436690 ) ) ;
#117153=CARTESIAN_POINT ( 'NONE',  ( 8.224510206698742110, 14.34966873604972548, 107.0844237280190043 ) ) ;
#117154=CARTESIAN_POINT ( 'NONE',  ( 9.474510206698729675, 16.51473224551082808, 67.08442372801900433 ) ) ;
#117156=CARTESIAN_POINT ( 'NONE',  ( 5.049401038298161559, -19.05341960407611168, 112.7072429386476813 ) ) ;
#117157=CARTESIAN_POINT ( 'NONE',  ( -8.224510206698948167, 14.34966873604960824, 85.41557627198102409 ) ) ;
#117159=CARTESIAN_POINT ( 'NONE',  ( -13.89961937509977652, 13.97604488694528158, 45.62390960531433848 ) ) ;
#117160=CARTESIAN_POINT ( 'NONE',  ( -15.72974639402197994, 15.80617190586746368, 55.62390960531436690 ) ) ;
#117161=CARTESIAN_POINT ( 'NONE',  ( 5.719274019375991003, -21.55341960407610458, 77.70724293864770971 ) ) ;
#117162=CARTESIAN_POINT ( 'NONE',  ( 0.05219959533909260263, 19.03943276465977164, 34.99890960531435979 ) ) ;
#117163=CARTESIAN_POINT ( 'NONE',  ( -14.29746914071037622, -8.314922557961029526, 64.16775706135234714 ) ) ;
#117164=CARTESIAN_POINT ( 'NONE',  ( 19.03943276465977164, -0.05219959533909143690, 58.74890960531435979 ) ) ;
#117165=CARTESIAN_POINT ( 'NONE',  ( 16.51473224551083163, -9.474510206698727899, 40.83442372801900433 ) ) ;
#117166=CARTESIAN_POINT ( 'NONE',  ( -18.62759615963255300, -10.81492255796106328, 49.16775706135234003 ) ) ;
#117167=CARTESIAN_POINT ( 'NONE',  ( -15.80617190586745835, -15.72974639402198527, 36.87390960531435979 ) ) ;
#117168=CARTESIAN_POINT ( 'NONE',  ( -16.53943276465976808, 0.05219959533911058130, 106.2489096053143811 ) ) ;
#117170=CARTESIAN_POINT ( 'NONE',  ( -16.46253265017146816, -9.564922557961047289, 94.16775706135233293 ) ) ;
#117172=CARTESIAN_POINT ( 'NONE',  ( 17.50000000000000711, 3.427582784589808362, 37.32655242534940498 ) ) ;
#117173=CARTESIAN_POINT ( 'NONE',  ( 21.55341960407610458, 5.719274019375980345, 48.95724293864770971 ) ) ;
#117174=CARTESIAN_POINT ( 'NONE',  ( -16.46253265017160317, 9.564922557960807481, 25.83224293864769194 ) ) ;
#117175=CARTESIAN_POINT ( 'NONE',  ( -10.81492255796105439, 18.62759615963255655, 82.91775706135234714 ) ) ;
#117176=CARTESIAN_POINT ( 'NONE',  ( -0.05219959533910754901, -16.53943276465976808, 27.49890960531435269 ) ) ;
#117177=CARTESIAN_POINT ( 'NONE',  ( 0.05219959533934541429, -16.53943276465976808, 60.00109039468568284 ) ) ;
#117178=CARTESIAN_POINT ( 'NONE',  ( 8.224510206698953496, -14.34966873604960469, 52.91557627198103830 ) ) ;
#117179=CARTESIAN_POINT ( 'NONE',  ( 15.72974639402199770, -15.80617190586745480, 78.12390960531436690 ) ) ;
#117180=CARTESIAN_POINT ( 'NONE',  ( -15.80617190586745835, -15.72974639402198527, 76.87390960531439532 ) ) ;
#117182=CARTESIAN_POINT ( 'NONE',  ( -19.03943276465977164, -0.05219959533935918106, 88.75109039468567573 ) ) ;
#117183=CARTESIAN_POINT ( 'NONE',  ( 10.81492255796078972, 18.62759615963270932, 24.58224293864768839 ) ) ;
#117185=CARTESIAN_POINT ( 'NONE',  ( 19.05341960407611168, 5.049401038298154454, 68.95724293864769550 ) ) ;
#117186=CARTESIAN_POINT ( 'NONE',  ( 9.564922557960805705, 16.46253265017160317, 34.58224293864770260 ) ) ;
#117190=CARTESIAN_POINT ( 'NONE',  ( -0.05219959533934338120, 16.53943276465976808, 82.50109039468568994 ) ) ;
#117191=CARTESIAN_POINT ( 'NONE',  ( -5.719274019375978568, 21.55341960407610458, 115.2072429386476955 ) ) ;
#117192=CARTESIAN_POINT ( 'NONE',  ( 16.46253265017160672, -9.564922557960803928, 73.33224293864769550 ) ) ;
#117193=CARTESIAN_POINT ( 'NONE',  ( -15.72974639402176322, -15.80617190586768395, 49.37609039468569705 ) ) ;
#117194=CARTESIAN_POINT ( 'NONE',  ( -16.51473224551069308, -9.474510206698971260, 96.66557627198102409 ) ) ;
#117198=CARTESIAN_POINT ( 'NONE',  ( 10.72451020669871369, 18.67979575497193778, 42.08442372801901854 ) ) ;
#117199=CARTESIAN_POINT ( 'NONE',  ( 13.89961937509977652, -13.97604488694527269, 23.12390960531436335 ) ) ;
#117200=CARTESIAN_POINT ( 'NONE',  ( 9.474510206698971260, -16.51473224551069308, 102.9155762719810241 ) ) ;
#117201=CARTESIAN_POINT ( 'NONE',  ( -13.89961937509957401, -13.97604488694547875, 54.37609039468565442 ) ) ;
#117202=CARTESIAN_POINT ( 'NONE',  ( 10.81492255796078972, 18.62759615963270932, 109.5822429386476955 ) ) ;
#117203=CARTESIAN_POINT ( 'NONE',  ( -19.05341960407617563, 5.049401038297882671, 43.54275706135232582 ) ) ;
#117204=CARTESIAN_POINT ( 'NONE',  ( -9.474510206698720793, -16.51473224551083518, 49.58442372801899722 ) ) ;
#117205=CARTESIAN_POINT ( 'NONE',  ( 8.224510206698742110, 14.34966873604972548, 107.0844237280190043 ) ) ;
#117208=CARTESIAN_POINT ( 'NONE',  ( -13.89961937509977652, 13.97604488694528158, 70.62390960531432427 ) ) ;
#117209=CARTESIAN_POINT ( 'NONE',  ( -5.719274019375665041, -21.55341960407619695, 74.79275706135234714 ) ) ;
#117210=CARTESIAN_POINT ( 'NONE',  ( -5.823673210054431948, 21.52544592524334988, 92.70942372801901854 ) ) ;
#117212=CARTESIAN_POINT ( 'NONE',  ( -16.51473224551069308, -9.474510206698971260, 81.66557627198103830 ) ) ;
#117213=CARTESIAN_POINT ( 'NONE',  ( -10.72451020669870658, -18.67979575497194134, 59.58442372801901854 ) ) ;
#117214=CARTESIAN_POINT ( 'NONE',  ( -19.02544592524334988, -5.153800228976617603, 108.9594237280189759 ) ) ;
#117215=CARTESIAN_POINT ( 'NONE',  ( 9.564922557960805705, 16.46253265017160317, 69.58224293864770971 ) ) ;
#117216=CARTESIAN_POINT ( 'NONE',  ( 13.97604488694527802, 13.89961937509977652, 109.3739096053143669 ) ) ;
#117217=CARTESIAN_POINT ( 'NONE',  ( -13.97604488694527625, -13.89961937509977652, 91.87390960531432427 ) ) ;
#117219=CARTESIAN_POINT ( 'NONE',  ( 9.474510206698971260, -16.51473224551069308, 82.91557627198103830 ) ) ;
#117220=CARTESIAN_POINT ( 'NONE',  ( 0.05219959533909260263, 19.03943276465977164, 64.99890960531436690 ) ) ;
#117221=CARTESIAN_POINT ( 'NONE',  ( -0.05219959533907301413, -21.53943276465977519, 112.4989096053143669 ) ) ;
#117222=CARTESIAN_POINT ( 'NONE',  ( -16.52544592524335698, -4.483927247898792601, 103.9594237280190185 ) ) ;
#117224=CARTESIAN_POINT ( 'NONE',  ( -5.153800228976607833, 19.02544592524334988, 62.70942372801899722 ) ) ;
#117225=CARTESIAN_POINT ( 'NONE',  ( 16.46253265017160672, -9.564922557960803928, 98.33224293864769550 ) ) ;
#117226=CARTESIAN_POINT ( 'NONE',  ( -16.53943276465976808, 0.05219959533911058130, 86.24890960531436690 ) ) ;
#117227=CARTESIAN_POINT ( 'NONE',  ( -16.52544592524342804, 4.483927247898546575, 106.0405762719810525 ) ) ;
#117228=CARTESIAN_POINT ( 'NONE',  ( 18.67979575497178502, 10.72451020669898547, 39.16557627198102409 ) ) ;
#117229=CARTESIAN_POINT ( 'NONE',  ( -10.81492255796078084, -18.62759615963271287, 27.08224293864769550 ) ) ;
#117231=CARTESIAN_POINT ( 'NONE',  ( -14.34966873604960291, -8.224510206698953496, 96.66557627198102409 ) ) ;
#117233=CARTESIAN_POINT ( 'NONE',  ( -19.05341960407617563, 5.049401038297882671, 38.54275706135233293 ) ) ;
#117234=CARTESIAN_POINT ( 'NONE',  ( -14.29746914071037622, -8.314922557961029526, 109.1677570613523613 ) ) ;
#117235=CARTESIAN_POINT ( 'NONE',  ( -16.51473224551069308, -9.474510206698971260, 91.66557627198103830 ) ) ;
#117236=CARTESIAN_POINT ( 'NONE',  ( -21.52544592524334988, -5.823673210054445271, 63.95942372801901854 ) ) ;
#117237=CARTESIAN_POINT ( 'NONE',  ( -15.80617190586745835, -15.72974639402198527, 41.87390960531435979 ) ) ;
#117238=CARTESIAN_POINT ( 'NONE',  ( 15.72974639402176855, 15.80617190586768217, 26.87609039468567218 ) ) ;
#117239=CARTESIAN_POINT ( 'NONE',  ( 15.72974639402199770, -15.80617190586745480, 88.12390960531436690 ) ) ;
#117240=CARTESIAN_POINT ( 'NONE',  ( 8.224510206698953496, -14.34966873604960469, 102.9155762719810383 ) ) ;
#117241=CARTESIAN_POINT ( 'NONE',  ( 16.51473224551083163, -9.474510206698727899, 75.83442372801900433 ) ) ;
#117242=CARTESIAN_POINT ( 'NONE',  ( 5.153800228976335163, 19.02544592524342804, 39.79057627198100988 ) ) ;
#117244=CARTESIAN_POINT ( 'NONE',  ( 5.153800228976335163, 19.02544592524342804, 99.79057627198102409 ) ) ;
#117245=CARTESIAN_POINT ( 'NONE',  ( -16.51473224551069308, -9.474510206698971260, 101.6655762719810241 ) ) ;
#117246=CARTESIAN_POINT ( 'NONE',  ( 9.564922557960805705, 16.46253265017160317, 24.58224293864769194 ) ) ;
#117247=CARTESIAN_POINT ( 'NONE',  ( -12.06949235617756955, 12.14591786802309770, 40.62390960531435269 ) ) ;
#117248=CARTESIAN_POINT ( 'NONE',  ( 16.52544592524335698, 4.483927247898782831, 46.45942372801901854 ) ) ;
#117249=CARTESIAN_POINT ( 'NONE',  ( 21.52544592524334988, 5.823673210054432836, 101.4594237280190185 ) ) ;
#117250=CARTESIAN_POINT ( 'NONE',  ( -19.03943276465977164, 0.05219959533909376836, 116.2489096053143669 ) ) ;
#117251=CARTESIAN_POINT ( 'NONE',  ( 4.483927247898545687, 16.52544592524342804, 29.79057627198102409 ) ) ;
#117252=CARTESIAN_POINT ( 'NONE',  ( -21.53943276465977519, -0.05219959533937600094, 33.75109039468568284 ) ) ;
#117253=CARTESIAN_POINT ( 'NONE',  ( -16.46253265017160317, 9.564922557960807481, 100.8322429386477097 ) ) ;
#117254=CARTESIAN_POINT ( 'NONE',  ( 0.05219959533934541429, -16.53943276465976808, 105.0010903946856757 ) ) ;
#117255=CARTESIAN_POINT ( 'NONE',  ( -4.379528057220086978, -16.55341960407618274, 99.79275706135234714 ) ) ;
#117256=CARTESIAN_POINT ( 'NONE',  ( -12.14591786802326823, 12.06949235617739902, 28.12609039468568284 ) ) ;
#117257=CARTESIAN_POINT ( 'NONE',  ( -16.46253265017160317, 9.564922557960807481, 45.83224293864769550 ) ) ;
#117259=CARTESIAN_POINT ( 'NONE',  ( 12.14591786802309770, 12.06949235617756955, 104.3739096053143669 ) ) ;
#117260=CARTESIAN_POINT ( 'NONE',  ( 18.67979575497178502, 10.72451020669898547, 114.1655762719810383 ) ) ;
#117261=CARTESIAN_POINT ( 'NONE',  ( -19.03943276465977164, 0.05219959533909376836, 26.24890960531435624 ) ) ;
#117262=CARTESIAN_POINT ( 'NONE',  ( 13.97604488694527802, 13.89961937509977652, 109.3739096053143669 ) ) ;
#117263=CARTESIAN_POINT ( 'NONE',  ( -15.80617190586768217, 15.72974639402176855, 38.12609039468567573 ) ) ;
#117264=CARTESIAN_POINT ( 'NONE',  ( 13.97604488694527802, 13.89961937509977652, 39.37390960531435269 ) ) ;
#117265=CARTESIAN_POINT ( 'NONE',  ( -5.049401038298153566, 19.05341960407611168, 110.2072429386476671 ) ) ;
#117266=CARTESIAN_POINT ( 'NONE',  ( -17.49999999999999645, -5.500000000000000888, 34.20309617465829177 ) ) ;
#117267=CARTESIAN_POINT ( 'NONE',  ( 0.05219959533909260263, 19.03943276465977164, 94.99890960531436690 ) ) ;
#117268=CARTESIAN_POINT ( 'NONE',  ( 5.823673210054444382, -21.52544592524334988, 45.20942372801901854 ) ) ;
#117269=CARTESIAN_POINT ( 'NONE',  ( -12.06949235617756955, 12.14591786802309770, 95.62390960531436690 ) ) ;
#117270=CARTESIAN_POINT ( 'NONE',  ( -19.03943276465977164, 0.05219959533909376836, 91.24890960531436690 ) ) ;
#117271=LINE ( 'NONE', #144599, #138502 ) ;
#117272=CARTESIAN_POINT ( 'NONE',  ( -16.52544592524335698, -4.483927247898792601, 68.95942372801901854 ) ) ;
#117273=CARTESIAN_POINT ( 'NONE',  ( 0.05219959533937995610, -21.53943276465977519, 80.00109039468568994 ) ) ;
#117274=CARTESIAN_POINT ( 'NONE',  ( 4.379528057220092307, 16.55341960407617563, 37.29275706135235424 ) ) ;
#117275=CARTESIAN_POINT ( 'NONE',  ( -0.05219959533909027116, -19.03943276465977164, 87.49890960531436690 ) ) ;
#117276=CARTESIAN_POINT ( 'NONE',  ( 0.05219959533936267826, -19.03943276465977164, 105.0010903946856615 ) ) ;
#117277=CARTESIAN_POINT ( 'NONE',  ( -16.55341960407617563, 4.379528057220093196, 73.54275706135234714 ) ) ;
#117278=CARTESIAN_POINT ( 'NONE',  ( 13.97604488694548053, -13.89961937509957401, 95.62609039468563310 ) ) ;
#117279=CARTESIAN_POINT ( 'NONE',  ( 9.474510206698971260, -16.51473224551069308, 57.91557627198103120 ) ) ;
#117280=CARTESIAN_POINT ( 'NONE',  ( -5.719274019375978568, 21.55341960407610458, 85.20724293864770971 ) ) ;
#117281=CARTESIAN_POINT ( 'NONE',  ( 16.52544592524342804, -4.483927247898539470, 88.54057627198103830 ) ) ;
#117282=CARTESIAN_POINT ( 'NONE',  ( -19.05341960407617563, 5.049401038297882671, 93.54275706135234714 ) ) ;
#117283=CARTESIAN_POINT ( 'NONE',  ( 14.34966873604972726, -8.224510206698740333, 65.83442372801900433 ) ) ;
#117284=CARTESIAN_POINT ( 'NONE',  ( 17.05587630539788080, -6.762274262135622216, 63.24180309037315340 ) ) ;
#117285=CARTESIAN_POINT ( 'NONE',  ( 13.89961937509957401, 13.97604488694547697, 56.87609039468564731 ) ) ;
#117286=CARTESIAN_POINT ( 'NONE',  ( 8.314922557960818139, 14.29746914071049879, 34.58224293864770260 ) ) ;
#117287=CARTESIAN_POINT ( 'NONE',  ( 14.34966873604960469, 8.224510206698951720, 79.16557627198103830 ) ) ;
#117288=CARTESIAN_POINT ( 'NONE',  ( -19.02544592524334988, -5.153800228976617603, 18.95942372801899722 ) ) ;
#117289=CARTESIAN_POINT ( 'NONE',  ( -18.22780087662126647, -5.499999999999827693, 43.98236817873107185 ) ) ;
#117290=CARTESIAN_POINT ( 'NONE',  ( 0.05219959533937995610, -21.53943276465977519, 20.00109039468568639 ) ) ;
#117291=CARTESIAN_POINT ( 'NONE',  ( 19.02544592524343514, -5.153800228976328945, 78.54057627198099567 ) ) ;
#117292=CARTESIAN_POINT ( 'NONE',  ( 21.52544592524334988, 5.823673210054432836, 91.45942372801901854 ) ) ;
#117293=CARTESIAN_POINT ( 'NONE',  ( -16.46253265017160317, 9.564922557960807481, 80.83224293864769550 ) ) ;
#117294=CARTESIAN_POINT ( 'NONE',  ( 21.53943276465977519, -0.05219959533907433946, 43.74890960531435979 ) ) ;
#117295=CARTESIAN_POINT ( 'NONE',  ( -4.483927247898539470, -16.52544592524342804, 77.29057627198102409 ) ) ;
#117296=CARTESIAN_POINT ( 'NONE',  ( 9.474510206698971260, -16.51473224551069308, 62.91557627198102409 ) ) ;
#117297=CARTESIAN_POINT ( 'NONE',  ( -8.314922557960811034, -14.29746914071050412, 92.08224293864769550 ) ) ;
#117298=CARTESIAN_POINT ( 'NONE',  ( -10.72451020669870658, -18.67979575497194134, 19.58442372801901143 ) ) ;
#117299=CARTESIAN_POINT ( 'NONE',  ( 10.72451020669871369, 18.67979575497193778, 62.08442372801901143 ) ) ;
#117300=CARTESIAN_POINT ( 'NONE',  ( 5.049401038298161559, -19.05341960407611168, 37.70724293864768839 ) ) ;
#117301=CARTESIAN_POINT ( 'NONE',  ( -4.483927247898782831, 16.52544592524335698, 62.70942372801902565 ) ) ;
#117302=CARTESIAN_POINT ( 'NONE',  ( 18.67979575497178502, 10.72451020669898547, 109.1655762719810383 ) ) ;
#117303=CARTESIAN_POINT ( 'NONE',  ( -15.80617190586745835, -15.72974639402198527, 111.8739096053143669 ) ) ;
#117304=CARTESIAN_POINT ( 'NONE',  ( 9.564922557961047289, -16.46253265017146816, 45.41775706135232582 ) ) ;
#117305=CARTESIAN_POINT ( 'NONE',  ( 13.89961937509977652, -13.97604488694527269, 68.12390960531436690 ) ) ;
#117306=LINE ( 'NONE', #196177, #124985 ) ;
#117307=CARTESIAN_POINT ( 'NONE',  ( -5.719274019375665041, -21.55341960407619695, 74.79275706135234714 ) ) ;
#117308=CARTESIAN_POINT ( 'NONE',  ( 21.55341960407610458, 5.719274019375980345, 53.95724293864770260 ) ) ;
#117309=CARTESIAN_POINT ( 'NONE',  ( -4.379528057220328563, 16.55341960407611168, 35.20724293864768839 ) ) ;
#117310=CARTESIAN_POINT ( 'NONE',  ( -18.67979575497193778, 10.72451020669871902, 83.33442372801903275 ) ) ;
#117311=CARTESIAN_POINT ( 'NONE',  ( -16.46253265017146816, -9.564922557961047289, 19.16775706135233293 ) ) ;
#117312=CARTESIAN_POINT ( 'NONE',  ( -12.06949235617756955, 12.14591786802309770, 60.62390960531437401 ) ) ;
#117313=CARTESIAN_POINT ( 'NONE',  ( 4.483927247898545687, 16.52544592524342804, 104.7905762719810241 ) ) ;
#117314=CARTESIAN_POINT ( 'NONE',  ( -0.05219959533936034679, 19.03943276465977164, 57.50109039468566863 ) ) ;
#117315=CARTESIAN_POINT ( 'NONE',  ( 16.52544592524335698, 4.483927247898782831, 111.4594237280190328 ) ) ;
#117316=CARTESIAN_POINT ( 'NONE',  ( 21.53943276465977519, 0.05219959533937863772, 66.25109039468567573 ) ) ;
#117317=CARTESIAN_POINT ( 'NONE',  ( 13.97604488694527802, 13.89961937509977652, 54.37390960531435979 ) ) ;
#117318=CARTESIAN_POINT ( 'NONE',  ( -9.564922557961040184, 16.46253265017147172, 37.91775706135233293 ) ) ;
#117319=CARTESIAN_POINT ( 'NONE',  ( -15.80617190586745835, -15.72974639402198527, 36.87390960531435979 ) ) ;
#117320=CARTESIAN_POINT ( 'NONE',  ( -10.81492255796105439, 18.62759615963255655, 37.91775706135235424 ) ) ;
#117321=CARTESIAN_POINT ( 'NONE',  ( 21.53943276465977519, -0.05219959533907433946, 93.74890960531436690 ) ) ;
#117322=CARTESIAN_POINT ( 'NONE',  ( -16.51473224551082808, 9.474510206698731452, 83.33442372801899012 ) ) ;
#117323=CARTESIAN_POINT ( 'NONE',  ( -14.29746914071037622, -8.314922557961029526, 54.16775706135235424 ) ) ;
#117325=CARTESIAN_POINT ( 'NONE',  ( 10.81492255796078972, 18.62759615963270932, 89.58224293864768129 ) ) ;
#117326=CARTESIAN_POINT ( 'NONE',  ( 16.52544592524342804, -4.483927247898539470, 83.54057627198102409 ) ) ;
#117328=CARTESIAN_POINT ( 'NONE',  ( -9.564922557961040184, 16.46253265017147172, 112.9177570613523329 ) ) ;
#117329=VECTOR ( 'NONE', #127289, 1000.000000000000000 ) ;
#117330=EDGE_CURVE ( 'NONE', #144387, #53443, #183154, .T. ) ;
#117331=CARTESIAN_POINT ( 'NONE',  ( 10.72451020669898902, -18.67979575497178502, 52.91557627198103830 ) ) ;
#117332=CARTESIAN_POINT ( 'NONE',  ( -16.52544592524335698, -4.483927247898792601, 93.95942372801903275 ) ) ;
#117333=CARTESIAN_POINT ( 'NONE',  ( 5.153800228976335163, 19.02544592524342804, 24.79057627198102765 ) ) ;
#117334=CARTESIAN_POINT ( 'NONE',  ( -12.06949235617739369, -12.14591786802326823, 49.37609039468569705 ) ) ;
#117335=CARTESIAN_POINT ( 'NONE',  ( -15.72974639402176322, -15.80617190586768395, 24.37609039468567573 ) ) ;
#117336=CARTESIAN_POINT ( 'NONE',  ( 21.55341960407610458, 5.719274019375980345, 48.95724293864770971 ) ) ;
#117337=CARTESIAN_POINT ( 'NONE',  ( -16.52544592524335698, -4.483927247898792601, 88.95942372801901854 ) ) ;
#117338=CARTESIAN_POINT ( 'NONE',  ( -5.153800228976328057, -19.02544592524343514, 97.29057627198099567 ) ) ;
#117339=CARTESIAN_POINT ( 'NONE',  ( -10.81492255796105439, 18.62759615963255655, 62.91775706135236135 ) ) ;
#117340=CARTESIAN_POINT ( 'NONE',  ( -0.05219959533907301413, -21.53943276465977519, 42.49890960531435979 ) ) ;
#117341=CARTESIAN_POINT ( 'NONE',  ( -16.46253265017160317, 9.564922557960807481, 110.8322429386476955 ) ) ;
#117342=ORIENTED_EDGE ( 'NONE', *, *, #52301, .T. ) ;
#117343=CARTESIAN_POINT ( 'NONE',  ( -5.049401038297874678, -19.05341960407617918, 34.79275706135233293 ) ) ;
#117344=CARTESIAN_POINT ( 'NONE',  ( 14.29746914071037800, 8.314922557961029526, 71.66775706135234714 ) ) ;
#117345=CARTESIAN_POINT ( 'NONE',  ( -5.153800228976328057, -19.02544592524343514, 112.2905762719810099 ) ) ;
#117347=CARTESIAN_POINT ( 'NONE',  ( 0.05219959533909260263, 19.03943276465977164, 79.99890960531436690 ) ) ;
#117348=CARTESIAN_POINT ( 'NONE',  ( 12.14591786802327356, -12.06949235617739191, 105.6260903946856899 ) ) ;
#117349=CARTESIAN_POINT ( 'NONE',  ( -17.97161686093727795, 5.499999999999980460, 85.99637206859166838 ) ) ;
#117350=CARTESIAN_POINT ( 'NONE',  ( -16.53943276465976808, 0.05219959533911058130, 96.24890960531435269 ) ) ;
#117351=CARTESIAN_POINT ( 'NONE',  ( -18.62759615963270932, 10.81492255796079327, 45.83224293864769550 ) ) ;
#117352=CARTESIAN_POINT ( 'NONE',  ( 0.05219959533909260263, 19.03943276465977164, 34.99890960531435979 ) ) ;
#117353=CARTESIAN_POINT ( 'NONE',  ( -16.52544592524335698, -4.483927247898792601, 83.95942372801900433 ) ) ;
#117354=CARTESIAN_POINT ( 'NONE',  ( -21.52544592524334988, -5.823673210054445271, 28.95942372801902209 ) ) ;
#117355=CARTESIAN_POINT ( 'NONE',  ( -16.46253265017146816, -9.564922557961047289, 89.16775706135234714 ) ) ;
#117356=CARTESIAN_POINT ( 'NONE',  ( 0.05219959533910956823, 16.53943276465976808, 89.99890960531438111 ) ) ;
#117357=CARTESIAN_POINT ( 'NONE',  ( 16.51473224551069308, 9.474510206698969483, 59.16557627198102409 ) ) ;
#117358=CARTESIAN_POINT ( 'NONE',  ( 19.03943276465977164, -0.05219959533909143690, 108.7489096053143527 ) ) ;
#117359=CARTESIAN_POINT ( 'NONE',  ( 21.53943276465977519, 0.05219959533937863772, 106.2510903946856757 ) ) ;
#117360=CARTESIAN_POINT ( 'NONE',  ( 19.02544592524343514, -5.153800228976328945, 73.54057627198103830 ) ) ;
#117361=CARTESIAN_POINT ( 'NONE',  ( -0.05219959533934338120, 16.53943276465976808, 67.50109039468568994 ) ) ;
#117362=CARTESIAN_POINT ( 'NONE',  ( -10.81492255796105439, 18.62759615963255655, 87.91775706135234714 ) ) ;
#117363=CARTESIAN_POINT ( 'NONE',  ( -0.05219959533934338120, 16.53943276465976808, 67.50109039468568994 ) ) ;
#117364=CARTESIAN_POINT ( 'NONE',  ( 16.51473224551083163, -9.474510206698727899, 55.83442372801899722 ) ) ;
#117365=CARTESIAN_POINT ( 'NONE',  ( 9.474510206698729675, 16.51473224551082808, 72.08442372801900433 ) ) ;
#117366=CARTESIAN_POINT ( 'NONE',  ( 18.67979575497194134, -10.72451020669871369, 60.83442372801901854 ) ) ;
#117367=CARTESIAN_POINT ( 'NONE',  ( 19.05341960407611168, 5.049401038298154454, 68.95724293864769550 ) ) ;
#117368=CARTESIAN_POINT ( 'NONE',  ( -9.564922557960796823, -16.46253265017161027, 57.08224293864769550 ) ) ;
#117369=CARTESIAN_POINT ( 'NONE',  ( 19.02544592524334988, 5.153800228976608722, 61.45942372801900433 ) ) ;
#117370=CARTESIAN_POINT ( 'NONE',  ( -13.97604488694527625, -13.89961937509977652, 111.8739096053143243 ) ) ;
#117371=CARTESIAN_POINT ( 'NONE',  ( 16.51473224551069308, 9.474510206698969483, 89.16557627198103830 ) ) ;
#117372=CARTESIAN_POINT ( 'NONE',  ( -8.224510206698948167, 14.34966873604960824, 35.41557627198102409 ) ) ;
#117373=CARTESIAN_POINT ( 'NONE',  ( 0.05219959533907565091, 21.53943276465977519, 44.99890960531435979 ) ) ;
#117375=CARTESIAN_POINT ( 'NONE',  ( 21.52544592524334988, 5.823673210054432836, 106.4594237280190328 ) ) ;
#117376=CARTESIAN_POINT ( 'NONE',  ( -16.31925111598456368, -7.325300261831607429, 79.83575461032749843 ) ) ;
#117377=CARTESIAN_POINT ( 'NONE',  ( -0.05219959533909027116, -19.03943276465977164, 32.49890960531435979 ) ) ;
#117378=CARTESIAN_POINT ( 'NONE',  ( 13.97604488694527802, 13.89961937509977652, 24.37390960531435624 ) ) ;
#117380=CARTESIAN_POINT ( 'NONE',  ( -21.55341960407619339, 5.719274019375674811, 63.54275706135234003 ) ) ;
#117382=CARTESIAN_POINT ( 'NONE',  ( -0.05219959533934338120, 16.53943276465976808, 62.50109039468568284 ) ) ;
#117383=CARTESIAN_POINT ( 'NONE',  ( -0.05219959533907301413, -21.53943276465977519, 82.49890960531436690 ) ) ;
#117384=CARTESIAN_POINT ( 'NONE',  ( 16.52544592524342804, -4.483927247898539470, 48.54057627198103120 ) ) ;
#117385=CARTESIAN_POINT ( 'NONE',  ( 19.03943276465977164, -0.05219959533909143690, 28.74890960531435624 ) ) ;
#117387=CARTESIAN_POINT ( 'NONE',  ( 18.62759615963255655, 10.81492255796105972, 41.66775706135235424 ) ) ;
#117388=CARTESIAN_POINT ( 'NONE',  ( 19.03943276465977164, 0.05219959533936151252, 46.25109039468566863 ) ) ;
#117389=CARTESIAN_POINT ( 'NONE',  ( 13.97604488694527802, 13.89961937509977652, 34.37390960531436690 ) ) ;
#117390=CARTESIAN_POINT ( 'NONE',  ( 10.72451020669871369, 18.67979575497193778, 87.08442372801901854 ) ) ;
#117391=CARTESIAN_POINT ( 'NONE',  ( 22.00000000000000000, -5.510910596163089556E-15, 42.49999999999999289 ) ) ;
#117392=CARTESIAN_POINT ( 'NONE',  ( -8.314922557960811034, -14.29746914071050412, 47.08224293864770260 ) ) ;
#117394=CARTESIAN_POINT ( 'NONE',  ( 21.52544592524344225, -5.823673210054117533, 43.54057627198103830 ) ) ;
#117396=CARTESIAN_POINT ( 'NONE',  ( -13.97604488694527625, -13.89961937509977652, 91.87390960531432427 ) ) ;
#117397=CARTESIAN_POINT ( 'NONE',  ( 4.379528057220339221, -16.55341960407611168, 82.70724293864770971 ) ) ;
#117398=CARTESIAN_POINT ( 'NONE',  ( -13.97604488694547697, 13.89961937509957934, 103.1260903946856473 ) ) ;
#117399=EDGE_CURVE ( 'NONE', #102413, #2480, #48451, .T. ) ;
#117400=CARTESIAN_POINT ( 'NONE',  ( 15.80617190586746368, 15.72974639402197994, 59.37390960531436690 ) ) ;
#117401=ORIENTED_EDGE ( 'NONE', *, *, #57096, .T. ) ;
#117402=CARTESIAN_POINT ( 'NONE',  ( 13.97604488694527802, 13.89961937509977652, 34.37390960531436690 ) ) ;
#117403=CARTESIAN_POINT ( 'NONE',  ( 16.51473224551069308, 9.474510206698969483, 79.16557627198103830 ) ) ;
#117404=CARTESIAN_POINT ( 'NONE',  ( 18.62759615963271287, -10.81492255796078972, 83.33224293864769550 ) ) ;
#117406=CARTESIAN_POINT ( 'NONE',  ( 8.314922557960818139, 14.29746914071049879, 29.58224293864769905 ) ) ;
#117407=CARTESIAN_POINT ( 'NONE',  ( -19.03943276465977164, 0.05219959533909376836, 101.2489096053143669 ) ) ;
#117408=CARTESIAN_POINT ( 'NONE',  ( 19.03943276465977164, 0.05219959533936151252, 81.25109039468567573 ) ) ;
#117409=CARTESIAN_POINT ( 'NONE',  ( -15.72974639402176322, -15.80617190586768395, 89.37609039468568994 ) ) ;
#117410=CARTESIAN_POINT ( 'NONE',  ( -15.72974639402197994, 15.80617190586746368, 80.62390960531438111 ) ) ;
#117411=CARTESIAN_POINT ( 'NONE',  ( -18.62759615963270932, 10.81492255796079327, 35.83224293864768839 ) ) ;
#117412=CARTESIAN_POINT ( 'NONE',  ( 13.97604488694527802, 13.89961937509977652, 54.37390960531435979 ) ) ;
#117413=CARTESIAN_POINT ( 'NONE',  ( 14.34966873604972726, -8.224510206698740333, 110.8344237280190043 ) ) ;
#117414=CARTESIAN_POINT ( 'NONE',  ( -19.02544592524342804, 5.153800228976336051, 71.04057627198099567 ) ) ;
#117415=ORIENTED_EDGE ( 'NONE', *, *, #130264, .F. ) ;
#117417=CARTESIAN_POINT ( 'NONE',  ( -19.05341960407617563, 5.049401038297882671, 33.54275706135231871 ) ) ;
#117418=CARTESIAN_POINT ( 'NONE',  ( -14.29746914071049879, 8.314922557960819915, 80.83224293864769550 ) ) ;
#117419=CARTESIAN_POINT ( 'NONE',  ( 0.05219959533937995610, -21.53943276465977519, 30.00109039468568284 ) ) ;
#117421=CARTESIAN_POINT ( 'NONE',  ( -18.62759615963270932, 10.81492255796079327, 55.83224293864770260 ) ) ;
#117422=CARTESIAN_POINT ( 'NONE',  ( -16.53943276465976808, -0.05219959533934237506, 93.75109039468567573 ) ) ;
#117423=CARTESIAN_POINT ( 'NONE',  ( 13.89961937509977652, -13.97604488694527269, 23.12390960531436335 ) ) ;
#117424=CARTESIAN_POINT ( 'NONE',  ( 16.51473224551069308, 9.474510206698969483, 69.16557627198102409 ) ) ;
#117426=CARTESIAN_POINT ( 'NONE',  ( 14.29746914071049879, -8.314922557960816363, 33.33224293864769550 ) ) ;
#117427=CARTESIAN_POINT ( 'NONE',  ( 15.80617190586769283, -15.72974639402175789, 65.62609039468568994 ) ) ;
#117428=CARTESIAN_POINT ( 'NONE',  ( -13.89961937509977652, 13.97604488694528158, 105.6239096053143527 ) ) ;
#117429=CARTESIAN_POINT ( 'NONE',  ( -18.62759615963255300, -10.81492255796106328, 89.16775706135236135 ) ) ;
#117430=CARTESIAN_POINT ( 'NONE',  ( -16.46253265017160317, 9.564922557960807481, 25.83224293864769194 ) ) ;
#117431=CARTESIAN_POINT ( 'NONE',  ( -13.89961937509977652, 13.97604488694528158, 35.62390960531435269 ) ) ;
#117433=CARTESIAN_POINT ( 'NONE',  ( 15.72974639402176855, 15.80617190586768217, 96.87609039468568994 ) ) ;
#117434=CARTESIAN_POINT ( 'NONE',  ( -16.53943276465976808, -0.05219959533934237506, 48.75109039468568284 ) ) ;
#117435=CARTESIAN_POINT ( 'NONE',  ( 21.52544592524334988, 5.823673210054432836, 91.45942372801901854 ) ) ;
#117436=CARTESIAN_POINT ( 'NONE',  ( -13.97604488694527625, -13.89961937509977652, 111.8739096053143243 ) ) ;
#117437=CARTESIAN_POINT ( 'NONE',  ( 9.564922557961047289, -16.46253265017146816, 90.41775706135234714 ) ) ;
#117438=CARTESIAN_POINT ( 'NONE',  ( 15.80617190586769283, -15.72974639402175789, 55.62609039468568284 ) ) ;
#117439=CARTESIAN_POINT ( 'NONE',  ( 12.06949235617739724, 12.14591786802326823, 21.87609039468567573 ) ) ;
#117440=CARTESIAN_POINT ( 'NONE',  ( -13.89961937509957401, -13.97604488694547875, 79.37609039468567573 ) ) ;
#117441=CARTESIAN_POINT ( 'NONE',  ( -9.564922557960796823, -16.46253265017161027, 52.08224293864768839 ) ) ;
#117442=CARTESIAN_POINT ( 'NONE',  ( -19.05341960407617563, 5.049401038297882671, 98.54275706135233293 ) ) ;
#117443=CARTESIAN_POINT ( 'NONE',  ( -19.03943276465977164, -0.05219959533935918106, 88.75109039468567573 ) ) ;
#117444=CARTESIAN_POINT ( 'NONE',  ( 14.34966873604960469, 8.224510206698951720, 54.16557627198103120 ) ) ;
#117445=CARTESIAN_POINT ( 'NONE',  ( 19.03943276465977164, 0.05219959533936151252, 71.25109039468566152 ) ) ;
#117446=CARTESIAN_POINT ( 'NONE',  ( -8.224510206698735004, -14.34966873604973081, 54.58442372801901143 ) ) ;
#117447=CARTESIAN_POINT ( 'NONE',  ( -21.55341960407619339, 5.719274019375674811, 113.5427570613523756 ) ) ;
#117448=CARTESIAN_POINT ( 'NONE',  ( 9.474510206698971260, -16.51473224551069308, 32.91557627198102409 ) ) ;
#117449=CARTESIAN_POINT ( 'NONE',  ( 0.05219959533909260263, 19.03943276465977164, 44.99890960531435979 ) ) ;
#117450=CARTESIAN_POINT ( 'NONE',  ( 12.06949235617739724, 12.14591786802326823, 56.87609039468568994 ) ) ;
#117451=CARTESIAN_POINT ( 'NONE',  ( -17.60728821187776205, 5.500000000000042633, 45.86690927743608626 ) ) ;
#117453=CARTESIAN_POINT ( 'NONE',  ( 13.97604488694527802, 13.89961937509977652, 109.3739096053143669 ) ) ;
#117454=CARTESIAN_POINT ( 'NONE',  ( -18.22780087662124160, -5.499999999999927169, 83.98236817873107896 ) ) ;
#117456=CARTESIAN_POINT ( 'NONE',  ( 5.049401038297881783, 19.05341960407617563, 92.29275706135234714 ) ) ;
#117457=CARTESIAN_POINT ( 'NONE',  ( 21.55341960407610458, 5.719274019375980345, 33.95724293864769550 ) ) ;
#117458=CARTESIAN_POINT ( 'NONE',  ( -16.46253265017146816, -9.564922557961047289, 29.16775706135232937 ) ) ;
#117459=CARTESIAN_POINT ( 'NONE',  ( -0.05219959533936034679, 19.03943276465977164, 107.5010903946856615 ) ) ;
#117460=CARTESIAN_POINT ( 'NONE',  ( -19.05341960407611168, -5.049401038298163336, 36.45724293864766707 ) ) ;
#117461=CARTESIAN_POINT ( 'NONE',  ( -13.97604488694527625, -13.89961937509977652, 36.87390960531436690 ) ) ;
#117462=CARTESIAN_POINT ( 'NONE',  ( -5.719274019375978568, 21.55341960407610458, 70.20724293864769550 ) ) ;
#117463=CARTESIAN_POINT ( 'NONE',  ( -9.564922557960796823, -16.46253265017161027, 102.0822429386477097 ) ) ;
#117465=CARTESIAN_POINT ( 'NONE',  ( -5.153800228976328057, -19.02544592524343514, 42.29057627198101699 ) ) ;
#117467=CARTESIAN_POINT ( 'NONE',  ( -0.05219959533936034679, 19.03943276465977164, 87.50109039468567573 ) ) ;
#117468=CARTESIAN_POINT ( 'NONE',  ( 4.379528057220339221, -16.55341960407611168, 57.70724293864770260 ) ) ;
#117469=CARTESIAN_POINT ( 'NONE',  ( 18.67979575497178502, 10.72451020669898547, 39.16557627198102409 ) ) ;
#117470=CARTESIAN_POINT ( 'NONE',  ( -0.05219959533937732626, 21.53943276465977519, 107.5010903946856899 ) ) ;
#117471=CARTESIAN_POINT ( 'NONE',  ( 15.80617190586746368, 15.72974639402197994, 79.37390960531436690 ) ) ;
#117472=CARTESIAN_POINT ( 'NONE',  ( -21.52544592524334988, -5.823673210054445271, 73.95942372801901854 ) ) ;
#117473=CARTESIAN_POINT ( 'NONE',  ( 18.62759615963255655, 10.81492255796105972, 66.66775706135234714 ) ) ;
#117474=CARTESIAN_POINT ( 'NONE',  ( -0.05219959533909027116, -19.03943276465977164, 112.4989096053143669 ) ) ;
#117475=CARTESIAN_POINT ( 'NONE',  ( -12.06949235617739369, -12.14591786802326823, 109.3760903946857042 ) ) ;
#117476=CARTESIAN_POINT ( 'NONE',  ( 21.53943276465977519, 0.05219959533937863772, 66.25109039468567573 ) ) ;
#117477=CARTESIAN_POINT ( 'NONE',  ( -16.51473224551069308, -9.474510206698971260, 56.66557627198103120 ) ) ;
#117478=CARTESIAN_POINT ( 'NONE',  ( -19.05341960407617563, 5.049401038297882671, 33.54275706135231871 ) ) ;
#117479=CARTESIAN_POINT ( 'NONE',  ( -18.62759615963255300, -10.81492255796106328, 24.16775706135235424 ) ) ;
#117480=CARTESIAN_POINT ( 'NONE',  ( 9.474510206698971260, -16.51473224551069308, 72.91557627198102409 ) ) ;
#117481=CARTESIAN_POINT ( 'NONE',  ( -0.05219959533910754901, -16.53943276465976808, 77.49890960531433848 ) ) ;
#117482=CARTESIAN_POINT ( 'NONE',  ( -12.14591786802309592, -12.06949235617757132, 51.87390960531437401 ) ) ;
#117483=CARTESIAN_POINT ( 'NONE',  ( 5.719274019375991003, -21.55341960407610458, 57.70724293864770260 ) ) ;
#117484=CARTESIAN_POINT ( 'NONE',  ( -5.049401038298153566, 19.05341960407611168, 65.20724293864765286 ) ) ;
#117485=CARTESIAN_POINT ( 'NONE',  ( -18.62759615963270932, 10.81492255796079327, 75.83224293864769550 ) ) ;
#117486=CARTESIAN_POINT ( 'NONE',  ( -13.89961937509957401, -13.97604488694547875, 54.37609039468565442 ) ) ;
#117489=CARTESIAN_POINT ( 'NONE',  ( 16.55341960407611168, 4.379528057220329451, 63.95724293864770260 ) ) ;
#117490=CARTESIAN_POINT ( 'NONE',  ( -21.53943276465977519, 0.05219959533907696930, 41.24890960531435269 ) ) ;
#117492=CARTESIAN_POINT ( 'NONE',  ( 16.31925111598457434, 7.325300261831544368, 102.3357546103274984 ) ) ;
#117493=CARTESIAN_POINT ( 'NONE',  ( -4.483927247898782831, 16.52544592524335698, 87.70942372801901854 ) ) ;
#117495=CARTESIAN_POINT ( 'NONE',  ( 0.05219959533936267826, -19.03943276465977164, 95.00109039468567573 ) ) ;
#117496=CARTESIAN_POINT ( 'NONE',  ( -4.379528057220328563, 16.55341960407611168, 50.20724293864769550 ) ) ;
#117498=CARTESIAN_POINT ( 'NONE',  ( 19.05341960407611168, 5.049401038298154454, 48.95724293864768129 ) ) ;
#117499=CARTESIAN_POINT ( 'NONE',  ( 16.53943276465976808, -0.05219959533910856209, 38.74890960531435979 ) ) ;
#117500=CARTESIAN_POINT ( 'NONE',  ( 19.05341960407611168, 5.049401038298154454, 83.95724293864766707 ) ) ;
#117501=CARTESIAN_POINT ( 'NONE',  ( -9.474510206698964154, 16.51473224551069663, 50.41557627198102409 ) ) ;
#117502=CARTESIAN_POINT ( 'NONE',  ( -21.53943276465977519, -0.05219959533937600094, 58.75109039468568994 ) ) ;
#117503=CARTESIAN_POINT ( 'NONE',  ( -13.89961937509977652, 13.97604488694528158, 70.62390960531432427 ) ) ;
#117504=CARTESIAN_POINT ( 'NONE',  ( 16.46253265017160672, -9.564922557960803928, 28.33224293864769550 ) ) ;
#117505=CARTESIAN_POINT ( 'NONE',  ( -5.049401038298153566, 19.05341960407611168, 70.20724293864769550 ) ) ;
#117506=CARTESIAN_POINT ( 'NONE',  ( 15.80617190586746368, 15.72974639402197994, 49.37390960531436690 ) ) ;
#117507=CARTESIAN_POINT ( 'NONE',  ( 9.474510206698971260, -16.51473224551069308, 37.91557627198102409 ) ) ;
#117508=CARTESIAN_POINT ( 'NONE',  ( -5.719274019375978568, 21.55341960407610458, 35.20724293864768839 ) ) ;
#117509=CARTESIAN_POINT ( 'NONE',  ( -12.06949235617739369, -12.14591786802326823, 109.3760903946857042 ) ) ;
#117510=CARTESIAN_POINT ( 'NONE',  ( -9.474510206698720793, -16.51473224551083518, 29.58442372801900433 ) ) ;
#117512=CARTESIAN_POINT ( 'NONE',  ( -16.52544592524335698, -4.483927247898792601, 43.95942372801902565 ) ) ;
#117513=CARTESIAN_POINT ( 'NONE',  ( -8.224510206698735004, -14.34966873604973081, 84.58442372801903275 ) ) ;
#117514=CARTESIAN_POINT ( 'NONE',  ( -13.89961937509977652, 13.97604488694528158, 115.6239096053143669 ) ) ;
#117515=CARTESIAN_POINT ( 'NONE',  ( 12.06949235617739724, 12.14591786802326823, 61.87609039468568284 ) ) ;
#117516=CARTESIAN_POINT ( 'NONE',  ( 19.05341960407611168, 5.049401038298154454, 108.9572429386477097 ) ) ;
#117517=CARTESIAN_POINT ( 'NONE',  ( -16.51473224551069308, -9.474510206698971260, 36.66557627198102409 ) ) ;
#117518=CARTESIAN_POINT ( 'NONE',  ( -16.55341960407617563, 4.379528057220093196, 33.54275706135234714 ) ) ;
#117519=CARTESIAN_POINT ( 'NONE',  ( 13.97604488694527802, 13.89961937509977652, 44.37390960531435269 ) ) ;
#117520=CARTESIAN_POINT ( 'NONE',  ( -21.52544592524334988, -5.823673210054445271, 23.95942372801901143 ) ) ;
#117521=CARTESIAN_POINT ( 'NONE',  ( 16.52544592524335698, 4.483927247898782831, 36.45942372801901143 ) ) ;
#117522=CARTESIAN_POINT ( 'NONE',  ( 8.224510206698742110, 14.34966873604972548, 102.0844237280190185 ) ) ;
#117524=CARTESIAN_POINT ( 'NONE',  ( 0.05219959533937995610, -21.53943276465977519, 95.00109039468568994 ) ) ;
#117525=CARTESIAN_POINT ( 'NONE',  ( 19.03943276465977164, 0.05219959533936151252, 101.2510903946856757 ) ) ;
#117526=CARTESIAN_POINT ( 'NONE',  ( -5.049401038297874678, -19.05341960407617918, 59.79275706135231871 ) ) ;
#117527=CARTESIAN_POINT ( 'NONE',  ( -8.314922557960811034, -14.29746914071050412, 62.08224293864769550 ) ) ;
#117528=CARTESIAN_POINT ( 'NONE',  ( 12.14591786802309770, 12.06949235617756955, 114.3739096053143527 ) ) ;
#117529=CARTESIAN_POINT ( 'NONE',  ( 19.02544592524334988, 5.153800228976608722, 61.45942372801900433 ) ) ;
#117530=CARTESIAN_POINT ( 'NONE',  ( 16.36317988757057762, 7.306389748694939179, 78.40210391636777842 ) ) ;
#117531=CARTESIAN_POINT ( 'NONE',  ( -21.52544592524334988, -5.823673210054445271, 63.95942372801901854 ) ) ;
#117532=CARTESIAN_POINT ( 'NONE',  ( -4.483927247898782831, 16.52544592524335698, 22.70942372801901499 ) ) ;
#117534=CARTESIAN_POINT ( 'NONE',  ( 15.80617190586746368, 15.72974639402197994, 24.37390960531435979 ) ) ;
#117535=CARTESIAN_POINT ( 'NONE',  ( -0.05219959533936034679, 19.03943276465977164, 107.5010903946856615 ) ) ;
#117538=CARTESIAN_POINT ( 'NONE',  ( -16.46253265017160317, 9.564922557960807481, 25.83224293864769194 ) ) ;
#117539=CARTESIAN_POINT ( 'NONE',  ( -10.81492255796105439, 18.62759615963255655, 102.9177570613523756 ) ) ;
#117540=CARTESIAN_POINT ( 'NONE',  ( 19.02544592524343514, -5.153800228976328945, 53.54057627198102409 ) ) ;
#117541=CARTESIAN_POINT ( 'NONE',  ( 0.05219959533937995610, -21.53943276465977519, 65.00109039468568994 ) ) ;
#117542=CARTESIAN_POINT ( 'NONE',  ( 21.52544592524334988, 5.823673210054432836, 101.4594237280190185 ) ) ;
#117543=CARTESIAN_POINT ( 'NONE',  ( -8.314922557961024197, 14.29746914071037800, 97.91775706135236135 ) ) ;
#117544=CARTESIAN_POINT ( 'NONE',  ( 16.46253265017160672, -9.564922557960803928, 73.33224293864769550 ) ) ;
#117545=CARTESIAN_POINT ( 'NONE',  ( -21.52544592524334988, -5.823673210054445271, 58.95942372801902565 ) ) ;
#117547=CARTESIAN_POINT ( 'NONE',  ( -18.62759615963255300, -10.81492255796106328, 54.16775706135235424 ) ) ;
#117548=CARTESIAN_POINT ( 'NONE',  ( -13.89961937509957401, -13.97604488694547875, 79.37609039468567573 ) ) ;
#117549=CARTESIAN_POINT ( 'NONE',  ( 9.564922557960805705, 16.46253265017160317, 104.5822429386476955 ) ) ;
#117550=CARTESIAN_POINT ( 'NONE',  ( -0.05219959533910754901, -16.53943276465976808, 112.4989096053143669 ) ) ;
#117551=CARTESIAN_POINT ( 'NONE',  ( -18.67979575497178146, -10.72451020669898902, 96.66557627198102409 ) ) ;
#117552=CARTESIAN_POINT ( 'NONE',  ( 13.97604488694548053, -13.89961937509957401, 20.62609039468567573 ) ) ;
#117553=CARTESIAN_POINT ( 'NONE',  ( -16.55341960407611168, -4.379528057220339221, 96.45724293864770971 ) ) ;
#117554=CARTESIAN_POINT ( 'NONE',  ( 19.02544592524343514, -5.153800228976328945, 53.54057627198102409 ) ) ;
#117555=CARTESIAN_POINT ( 'NONE',  ( 9.474510206698729675, 16.51473224551082808, 102.0844237280190043 ) ) ;
#117556=CARTESIAN_POINT ( 'NONE',  ( -0.05219959533910754901, -16.53943276465976808, 67.49890960531436690 ) ) ;
#117557=CARTESIAN_POINT ( 'NONE',  ( 21.52544592524334988, 5.823673210054432836, 111.4594237280190328 ) ) ;
#117558=CARTESIAN_POINT ( 'NONE',  ( -19.03943276465977164, 0.05219959533909376836, 106.2489096053143669 ) ) ;
#117559=CARTESIAN_POINT ( 'NONE',  ( -0.05219959533936034679, 19.03943276465977164, 72.50109039468566152 ) ) ;
#117560=CARTESIAN_POINT ( 'NONE',  ( 18.62759615963271287, -10.81492255796078972, 83.33224293864769550 ) ) ;
#117561=CARTESIAN_POINT ( 'NONE',  ( 10.81492255796106328, -18.62759615963255655, 50.41775706135235424 ) ) ;
#117562=CARTESIAN_POINT ( 'NONE',  ( -8.314922557961024197, 14.29746914071037800, 37.91775706135235424 ) ) ;
#117563=CARTESIAN_POINT ( 'NONE',  ( -16.55341960407617563, 4.379528057220093196, 93.54275706135234714 ) ) ;
#117564=CARTESIAN_POINT ( 'NONE',  ( -4.379528057220086978, -16.55341960407618274, 39.79275706135235424 ) ) ;
#117565=CARTESIAN_POINT ( 'NONE',  ( 21.52544592524334988, 5.823673210054432836, 36.45942372801901143 ) ) ;
#117566=CARTESIAN_POINT ( 'NONE',  ( -10.81492255796078084, -18.62759615963271287, 42.08224293864769550 ) ) ;
#117567=CARTESIAN_POINT ( 'NONE',  ( -9.474510206698964154, 16.51473224551069663, 40.41557627198103120 ) ) ;
#117569=CARTESIAN_POINT ( 'NONE',  ( 16.55341960407618274, -4.379528057220086978, 66.04275706135236135 ) ) ;
#117571=CARTESIAN_POINT ( 'NONE',  ( 0.05219959533907565091, 21.53943276465977519, 89.99890960531438111 ) ) ;
#117572=CARTESIAN_POINT ( 'NONE',  ( -12.06949235617756955, 12.14591786802309770, 40.62390960531435269 ) ) ;
#117573=CARTESIAN_POINT ( 'NONE',  ( -14.29746914071037622, -8.314922557961029526, 54.16775706135235424 ) ) ;
#117574=CARTESIAN_POINT ( 'NONE',  ( 19.03943276465977164, -0.05219959533909143690, 58.74890960531435979 ) ) ;
#117575=CARTESIAN_POINT ( 'NONE',  ( -9.564922557961040184, 16.46253265017147172, 82.91775706135233293 ) ) ;
#117576=CARTESIAN_POINT ( 'NONE',  ( -15.80617190586745835, -15.72974639402198527, 81.87390960531435269 ) ) ;
#117577=CARTESIAN_POINT ( 'NONE',  ( -4.379528057220328563, 16.55341960407611168, 30.20724293864769550 ) ) ;
#117581=CARTESIAN_POINT ( 'NONE',  ( -15.72974639402197994, 15.80617190586746368, 55.62390960531436690 ) ) ;
#117582=CARTESIAN_POINT ( 'NONE',  ( 0.05219959533934541429, -16.53943276465976808, 105.0010903946856757 ) ) ;
#117584=CARTESIAN_POINT ( 'NONE',  ( 18.39639308325437028, 5.500000000000035527, 88.98252246182197212 ) ) ;
#117585=CARTESIAN_POINT ( 'NONE',  ( 10.81492255796078972, 18.62759615963270932, 84.58224293864769550 ) ) ;
#117586=CARTESIAN_POINT ( 'NONE',  ( -4.483927247898539470, -16.52544592524342804, 22.29057627198102765 ) ) ;
#117587=CARTESIAN_POINT ( 'NONE',  ( 4.483927247898790824, -16.52544592524335698, 30.20942372801902565 ) ) ;
#117588=CARTESIAN_POINT ( 'NONE',  ( 5.049401038298161559, -19.05341960407611168, 32.70724293864768129 ) ) ;
#117589=CARTESIAN_POINT ( 'NONE',  ( 19.03943276465977164, -0.05219959533909143690, 68.74890960531436690 ) ) ;
#117591=CARTESIAN_POINT ( 'NONE',  ( -21.55341960407610458, -5.719274019375992779, 26.45724293864768839 ) ) ;
#117592=CARTESIAN_POINT ( 'NONE',  ( 18.09918380851993192, 5.500000000000035527, 78.98618307335611632 ) ) ;
#117594=CARTESIAN_POINT ( 'NONE',  ( -12.14591786802326823, 12.06949235617739902, 98.12609039468570415 ) ) ;
#117595=CARTESIAN_POINT ( 'NONE',  ( 13.97604488694548053, -13.89961937509957401, 105.6260903946856757 ) ) ;
#117596=CARTESIAN_POINT ( 'NONE',  ( 19.02544592524334988, 5.153800228976608722, 31.45942372801900433 ) ) ;
#117597=CARTESIAN_POINT ( 'NONE',  ( -10.81492255796078084, -18.62759615963271287, 87.08224293864769550 ) ) ;
#117598=CARTESIAN_POINT ( 'NONE',  ( -16.53943276465976808, 0.05219959533911058130, 21.24890960531436690 ) ) ;
#117599=CARTESIAN_POINT ( 'NONE',  ( 21.55341960407610458, 5.719274019375980345, 48.95724293864770971 ) ) ;
#117600=CARTESIAN_POINT ( 'NONE',  ( -16.46253265017146816, -9.564922557961047289, 109.1677570613523471 ) ) ;
#117601=CARTESIAN_POINT ( 'NONE',  ( 16.51473224551069308, 9.474510206698969483, 99.16557627198102409 ) ) ;
#117603=CARTESIAN_POINT ( 'NONE',  ( -21.52544592524334988, -5.823673210054445271, 63.95942372801901854 ) ) ;
#117604=CARTESIAN_POINT ( 'NONE',  ( 9.474510206698971260, -16.51473224551069308, 62.91557627198102409 ) ) ;
#117605=CARTESIAN_POINT ( 'NONE',  ( -16.52544592524342804, 4.483927247898546575, 96.04057627198102409 ) ) ;
#117607=CARTESIAN_POINT ( 'NONE',  ( -9.564922557960796823, -16.46253265017161027, 72.08224293864770971 ) ) ;
#117608=CARTESIAN_POINT ( 'NONE',  ( 16.55341960407611168, 4.379528057220329451, 78.95724293864769550 ) ) ;
#117610=CARTESIAN_POINT ( 'NONE',  ( 13.89961937509957401, 13.97604488694547697, 86.87609039468567573 ) ) ;
#117613=CARTESIAN_POINT ( 'NONE',  ( 19.39056639909674473, 5.500000000000001776, 93.28948781074345220 ) ) ;
#117614=CARTESIAN_POINT ( 'NONE',  ( -0.05219959533909027116, -19.03943276465977164, 57.49890960531435979 ) ) ;
#117616=CARTESIAN_POINT ( 'NONE',  ( -5.153800228976328057, -19.02544592524343514, 72.29057627198102409 ) ) ;
#117617=CARTESIAN_POINT ( 'NONE',  ( -5.049401038298153566, 19.05341960407611168, 105.2072429386476671 ) ) ;
#117618=CARTESIAN_POINT ( 'NONE',  ( -16.52544592524335698, -4.483927247898792601, 68.95942372801901854 ) ) ;
#117620=CARTESIAN_POINT ( 'NONE',  ( -5.153800228976607833, 19.02544592524334988, 47.70942372801900433 ) ) ;
#117621=CARTESIAN_POINT ( 'NONE',  ( -5.719274019375665041, -21.55341960407619695, 99.79275706135234714 ) ) ;
#117624=CARTESIAN_POINT ( 'NONE',  ( -0.05219959533934338120, 16.53943276465976808, 97.50109039468567573 ) ) ;
#117625=CARTESIAN_POINT ( 'NONE',  ( 13.97604488694548053, -13.89961937509957401, 75.62609039468566152 ) ) ;
#117626=CARTESIAN_POINT ( 'NONE',  ( 14.29746914071037800, 8.314922557961029526, 86.66775706135234714 ) ) ;
#117627=CARTESIAN_POINT ( 'NONE',  ( 16.29526858892874230, 7.335722546920140807, 68.29670597800208043 ) ) ;
#117628=CARTESIAN_POINT ( 'NONE',  ( 16.53943276465976808, 0.05219959533934440121, 71.25109039468568994 ) ) ;
#117629=ORIENTED_EDGE ( 'NONE', *, *, #12667, .F. ) ;
#117630=CARTESIAN_POINT ( 'NONE',  ( 21.52544592524334988, 5.823673210054432836, 76.45942372801901854 ) ) ;
#117631=CARTESIAN_POINT ( 'NONE',  ( -16.51473224551082808, 9.474510206698731452, 93.33442372801900433 ) ) ;
#117632=CARTESIAN_POINT ( 'NONE',  ( -16.46253265017146816, -9.564922557961047289, 24.16775706135233648 ) ) ;
#117633=CARTESIAN_POINT ( 'NONE',  ( 5.049401038298161559, -19.05341960407611168, 62.70724293864769550 ) ) ;
#117634=CARTESIAN_POINT ( 'NONE',  ( -5.049401038298153566, 19.05341960407611168, 60.20724293864768129 ) ) ;
#117636=CARTESIAN_POINT ( 'NONE',  ( -21.52544592524343514, 5.823673210054127303, 81.04057627198102409 ) ) ;
#117637=CIRCLE ( 'NONE', #191812, 2.000000000000001776 ) ;
#117638=CARTESIAN_POINT ( 'NONE',  ( 15.80617190586746368, 15.72974639402197994, 29.37390960531435269 ) ) ;
#117639=CARTESIAN_POINT ( 'NONE',  ( -9.474510206698964154, 16.51473224551069663, 35.41557627198102409 ) ) ;
#117640=CARTESIAN_POINT ( 'NONE',  ( -14.34966873604972548, 8.224510206698743886, 63.33442372801900433 ) ) ;
#117642=ORIENTED_EDGE ( 'NONE', *, *, #94206, .F. ) ;
#117643=CARTESIAN_POINT ( 'NONE',  ( 15.72974639402176855, 15.80617190586768217, 31.87609039468567929 ) ) ;
#117644=CARTESIAN_POINT ( 'NONE',  ( -0.05219959533910754901, -16.53943276465976808, 62.49890960531436690 ) ) ;
#117646=CARTESIAN_POINT ( 'NONE',  ( 4.483927247898790824, -16.52544592524335698, 20.20942372801900788 ) ) ;
#117647=CARTESIAN_POINT ( 'NONE',  ( -19.02544592524334988, -5.153800228976617603, 58.95942372801900433 ) ) ;
#117648=CARTESIAN_POINT ( 'NONE',  ( -14.29746914071049879, 8.314922557960819915, 60.83224293864769550 ) ) ;
#117649=CARTESIAN_POINT ( 'NONE',  ( -21.52544592524334988, -5.823673210054445271, 23.95942372801901143 ) ) ;
#117650=CARTESIAN_POINT ( 'NONE',  ( 13.97604488694527802, 13.89961937509977830, 99.37390960531436690 ) ) ;
#117651=CARTESIAN_POINT ( 'NONE',  ( 15.72974639402199770, -15.80617190586745480, 83.12390960531436690 ) ) ;
#117652=CARTESIAN_POINT ( 'NONE',  ( 9.474510206698971260, -16.51473224551069308, 92.91557627198103830 ) ) ;
#117653=CARTESIAN_POINT ( 'NONE',  ( -12.14591786802309592, -12.06949235617757132, 56.87390960531436690 ) ) ;
#117656=CARTESIAN_POINT ( 'NONE',  ( 5.049401038297881783, 19.05341960407617563, 72.29275706135234714 ) ) ;
#117657=CARTESIAN_POINT ( 'NONE',  ( 21.52544592524344225, -5.823673210054117533, 108.5405762719810241 ) ) ;
#117658=CARTESIAN_POINT ( 'NONE',  ( 19.03943276465977164, -0.05219959533909143690, 58.74890960531435979 ) ) ;
#117659=CARTESIAN_POINT ( 'NONE',  ( -13.89961937509957401, -13.97604488694547875, 39.37609039468566152 ) ) ;
#117660=CARTESIAN_POINT ( 'NONE',  ( -9.564922557960796823, -16.46253265017161027, 37.08224293864768839 ) ) ;
#117661=CARTESIAN_POINT ( 'NONE',  ( -0.05219959533937732626, 21.53943276465977519, 62.50109039468568284 ) ) ;
#117663=CARTESIAN_POINT ( 'NONE',  ( -16.55341960407611168, -4.379528057220339221, 41.45724293864769550 ) ) ;
#117664=CARTESIAN_POINT ( 'NONE',  ( 16.46253265017160672, -9.564922557960803928, 58.33224293864769550 ) ) ;
#117666=CARTESIAN_POINT ( 'NONE',  ( -21.53943276465977519, 0.05219959533907696930, 71.24890960531435269 ) ) ;
#117667=CARTESIAN_POINT ( 'NONE',  ( 19.02544592524343514, -5.153800228976328945, 58.54057627198102409 ) ) ;
#117669=CARTESIAN_POINT ( 'NONE',  ( 10.72451020669898902, -18.67979575497178502, 62.91557627198102409 ) ) ;
#117670=CARTESIAN_POINT ( 'NONE',  ( 10.81492255796106328, -18.62759615963255655, 95.41775706135234714 ) ) ;
#117672=CARTESIAN_POINT ( 'NONE',  ( 14.34966873604972726, -8.224510206698740333, 95.83442372801903275 ) ) ;
#117673=CARTESIAN_POINT ( 'NONE',  ( -0.05219959533910754901, -16.53943276465976808, 82.49890960531436690 ) ) ;
#117674=CARTESIAN_POINT ( 'NONE',  ( -13.89961937509957401, -13.97604488694547875, 89.37609039468563310 ) ) ;
#117675=ORIENTED_EDGE ( 'NONE', *, *, #182333, .F. ) ;
#117676=CARTESIAN_POINT ( 'NONE',  ( -9.564922557961040184, 16.46253265017147172, 37.91775706135233293 ) ) ;
#117677=CARTESIAN_POINT ( 'NONE',  ( 8.224510206698742110, 14.34966873604972548, 107.0844237280190043 ) ) ;
#117678=CARTESIAN_POINT ( 'NONE',  ( -5.153800228976607833, 19.02544592524334988, 27.70942372801899722 ) ) ;
#117679=CARTESIAN_POINT ( 'NONE',  ( 19.03943276465977164, -0.05219959533909143690, 88.74890960531436690 ) ) ;
#117680=CARTESIAN_POINT ( 'NONE',  ( -21.53943276465977519, 0.05219959533907696930, 66.24890960531436690 ) ) ;
#117682=CARTESIAN_POINT ( 'NONE',  ( -16.51473224551069308, -9.474510206698971260, 21.66557627198102765 ) ) ;
#117683=CARTESIAN_POINT ( 'NONE',  ( 0.05219959533937995610, -21.53943276465977519, 90.00109039468567573 ) ) ;
#117684=CARTESIAN_POINT ( 'NONE',  ( -14.29746914071037622, -8.314922557961029526, 74.16775706135231871 ) ) ;
#117685=CARTESIAN_POINT ( 'NONE',  ( 5.719274019375673035, 21.55341960407619339, 27.29275706135234358 ) ) ;
#117686=CARTESIAN_POINT ( 'NONE',  ( -12.06949235617739369, -12.14591786802326823, 34.37609039468568284 ) ) ;
#117687=CARTESIAN_POINT ( 'NONE',  ( -19.03943276465977164, 0.05219959533909376836, 106.2489096053143669 ) ) ;
#117688=CARTESIAN_POINT ( 'NONE',  ( 19.03943276465977164, -0.05219959533909143690, 33.74890960531435979 ) ) ;
#117689=CARTESIAN_POINT ( 'NONE',  ( -19.03943276465977164, 0.05219959533909376836, 51.24890960531436690 ) ) ;
#117690=CARTESIAN_POINT ( 'NONE',  ( 16.52544592524335698, 4.483927247898782831, 31.45942372801901854 ) ) ;
#117691=CARTESIAN_POINT ( 'NONE',  ( -16.53943276465976808, 0.05219959533911058130, 91.24890960531436690 ) ) ;
#117692=CARTESIAN_POINT ( 'NONE',  ( -8.224510206698735004, -14.34966873604973081, 104.5844237280190185 ) ) ;
#117693=CARTESIAN_POINT ( 'NONE',  ( -5.823673210054431948, 21.52544592524334988, 37.70942372801900433 ) ) ;
#117694=CARTESIAN_POINT ( 'NONE',  ( -16.51473224551069308, -9.474510206698971260, 76.66557627198103830 ) ) ;
#117695=CARTESIAN_POINT ( 'NONE',  ( 19.02544592524343514, -5.153800228976328945, 68.54057627198103830 ) ) ;
#117696=CARTESIAN_POINT ( 'NONE',  ( 16.46253265017160672, -9.564922557960803928, 83.33224293864768129 ) ) ;
#117697=CARTESIAN_POINT ( 'NONE',  ( 16.55341960407611168, 4.379528057220329451, 33.95724293864769550 ) ) ;
#117698=CARTESIAN_POINT ( 'NONE',  ( -0.05219959533934338120, 16.53943276465976808, 102.5010903946856899 ) ) ;
#117699=ORIENTED_EDGE ( 'NONE', *, *, #1307, .F. ) ;
#117700=CARTESIAN_POINT ( 'NONE',  ( -5.153800228976607833, 19.02544592524334988, 47.70942372801900433 ) ) ;
#117701=CARTESIAN_POINT ( 'NONE',  ( -19.05341960407611168, -5.049401038298163336, 106.4572429386476955 ) ) ;
#117702=CARTESIAN_POINT ( 'NONE',  ( 0.05219959533909260263, 19.03943276465977164, 54.99890960531435979 ) ) ;
#117703=CARTESIAN_POINT ( 'NONE',  ( 5.153800228976615827, -19.02544592524334988, 45.20942372801901143 ) ) ;
#117705=CARTESIAN_POINT ( 'NONE',  ( -12.06949235617739369, -12.14591786802326823, 39.37609039468567573 ) ) ;
#117706=CARTESIAN_POINT ( 'NONE',  ( 13.97604488694548053, -13.89961937509957401, 70.62609039468567573 ) ) ;
#117707=CARTESIAN_POINT ( 'NONE',  ( 16.52544592524335698, 4.483927247898782831, 56.45942372801902565 ) ) ;
#117708=CARTESIAN_POINT ( 'NONE',  ( 19.03943276465977164, -0.05219959533909143690, 113.7489096053143669 ) ) ;
#117709=CARTESIAN_POINT ( 'NONE',  ( 5.153800228976335163, 19.02544592524342804, 89.79057627198102409 ) ) ;
#117710=CARTESIAN_POINT ( 'NONE',  ( 18.67979575497178502, 10.72451020669898547, 109.1655762719810383 ) ) ;
#117711=CARTESIAN_POINT ( 'NONE',  ( -5.153800228976607833, 19.02544592524334988, 82.70942372801897591 ) ) ;
#117712=CARTESIAN_POINT ( 'NONE',  ( -19.03943276465977164, 0.05219959533909376836, 101.2489096053143669 ) ) ;
#117713=CARTESIAN_POINT ( 'NONE',  ( 19.05341960407611168, 5.049401038298154454, 33.95724293864769550 ) ) ;
#117714=CARTESIAN_POINT ( 'NONE',  ( -9.474510206698964154, 16.51473224551069663, 80.41557627198103830 ) ) ;
#117715=CARTESIAN_POINT ( 'NONE',  ( -4.483927247898539470, -16.52544592524342804, 37.29057627198102409 ) ) ;
#117716=CARTESIAN_POINT ( 'NONE',  ( 5.049401038298161559, -19.05341960407611168, 32.70724293864768129 ) ) ;
#117717=CARTESIAN_POINT ( 'NONE',  ( -19.02544592524334988, -5.153800228976617603, 48.95942372801900433 ) ) ;
#117718=CARTESIAN_POINT ( 'NONE',  ( -4.379528057220328563, 16.55341960407611168, 85.20724293864770971 ) ) ;
#117719=CARTESIAN_POINT ( 'NONE',  ( -5.153800228976607833, 19.02544592524334988, 22.70942372801899012 ) ) ;
#117720=CARTESIAN_POINT ( 'NONE',  ( -9.564922557960796823, -16.46253265017161027, 47.08224293864769550 ) ) ;
#117722=CARTESIAN_POINT ( 'NONE',  ( 21.55341960407610458, 5.719274019375980345, 43.95724293864769550 ) ) ;
#117723=CARTESIAN_POINT ( 'NONE',  ( 14.29746914071049879, -8.314922557960816363, 58.33224293864768839 ) ) ;
#117724=CARTESIAN_POINT ( 'NONE',  ( 10.72451020669871369, 18.67979575497193778, 97.08442372801904696 ) ) ;
#117725=CARTESIAN_POINT ( 'NONE',  ( 19.03943276465977164, -0.05219959533909143690, 103.7489096053143669 ) ) ;
#117726=CARTESIAN_POINT ( 'NONE',  ( -13.97604488694527625, -13.89961937509977652, 106.8739096053143669 ) ) ;
#117727=CARTESIAN_POINT ( 'NONE',  ( 0.05219959533909260263, 19.03943276465977164, 34.99890960531435979 ) ) ;
#117728=CARTESIAN_POINT ( 'NONE',  ( -19.02544592524342804, 5.153800228976336051, 31.04057627198102409 ) ) ;
#117729=CARTESIAN_POINT ( 'NONE',  ( -16.52544592524342804, 4.483927247898546575, 81.04057627198102409 ) ) ;
#117730=CARTESIAN_POINT ( 'NONE',  ( 15.72974639402199770, -15.80617190586745480, 93.12390960531436690 ) ) ;
#117731=CARTESIAN_POINT ( 'NONE',  ( 16.51473224551069308, 9.474510206698969483, 104.1655762719810241 ) ) ;
#117732=CARTESIAN_POINT ( 'NONE',  ( 0.05219959533937995610, -21.53943276465977519, 20.00109039468568639 ) ) ;
#117733=CARTESIAN_POINT ( 'NONE',  ( -13.97604488694527625, -13.89961937509977652, 96.87390960531433848 ) ) ;
#117734=CARTESIAN_POINT ( 'NONE',  ( 30.00000000000000000, 5.499999999999992895, 102.5000000000000142 ) ) ;
#117735=CARTESIAN_POINT ( 'NONE',  ( 4.483927247898545687, 16.52544592524342804, 99.79057627198103830 ) ) ;
#117736=CARTESIAN_POINT ( 'NONE',  ( -19.03943276465977164, 0.05219959533909376836, 76.24890960531435269 ) ) ;
#117737=CARTESIAN_POINT ( 'NONE',  ( 15.80617190586746368, 15.72974639402197994, 74.37390960531436690 ) ) ;
#117740=CARTESIAN_POINT ( 'NONE',  ( 5.719274019375991003, -21.55341960407610458, 32.70724293864770260 ) ) ;
#117742=CARTESIAN_POINT ( 'NONE',  ( -16.55341960407617563, 4.379528057220093196, 33.54275706135234714 ) ) ;
#117743=CARTESIAN_POINT ( 'NONE',  ( -12.06949235617756955, 12.14591786802309770, 95.62390960531436690 ) ) ;
#117746=CARTESIAN_POINT ( 'NONE',  ( -16.46253265017160317, 9.564922557960807481, 90.83224293864769550 ) ) ;
#117747=CARTESIAN_POINT ( 'NONE',  ( 19.05341960407611168, 5.049401038298154454, 48.95724293864768129 ) ) ;
#117748=CARTESIAN_POINT ( 'NONE',  ( 0.05219959533910956823, 16.53943276465976808, 74.99890960531435269 ) ) ;
#117750=CARTESIAN_POINT ( 'NONE',  ( 18.62759615963271287, -10.81492255796078972, 28.33224293864769550 ) ) ;
#117751=CARTESIAN_POINT ( 'NONE',  ( -14.29746914071049879, 8.314922557960819915, 50.83224293864770971 ) ) ;
#117752=CARTESIAN_POINT ( 'NONE',  ( 13.89961937509957401, 13.97604488694547697, 106.8760903946856757 ) ) ;
#117753=CARTESIAN_POINT ( 'NONE',  ( -15.72974639402176322, -15.80617190586768395, 69.37609039468567573 ) ) ;
#117756=CARTESIAN_POINT ( 'NONE',  ( -13.97604488694527625, -13.89961937509977652, 111.8739096053143243 ) ) ;
#117757=CARTESIAN_POINT ( 'NONE',  ( -12.14591786802326823, 12.06949235617739902, 83.12609039468568994 ) ) ;
#117758=CARTESIAN_POINT ( 'NONE',  ( 19.05341960407611168, 5.049401038298154454, 28.95724293864769550 ) ) ;
#117759=CARTESIAN_POINT ( 'NONE',  ( 9.474510206698971260, -16.51473224551069308, 77.91557627198103830 ) ) ;
#117760=CARTESIAN_POINT ( 'NONE',  ( -5.719274019375978568, 21.55341960407610458, 80.20724293864769550 ) ) ;
#117761=CARTESIAN_POINT ( 'NONE',  ( 0.05219959533934541429, -16.53943276465976808, 30.00109039468568284 ) ) ;
#117762=CARTESIAN_POINT ( 'NONE',  ( -0.05219959533910754901, -16.53943276465976808, 57.49890960531435979 ) ) ;
#117763=CARTESIAN_POINT ( 'NONE',  ( 15.80617190586769283, -15.72974639402175789, 70.62609039468567573 ) ) ;
#117764=CARTESIAN_POINT ( 'NONE',  ( 12.06949235617739724, 12.14591786802326823, 86.87609039468568994 ) ) ;
#117765=CARTESIAN_POINT ( 'NONE',  ( 9.474510206698971260, -16.51473224551069308, 112.9155762719810383 ) ) ;
#117766=CARTESIAN_POINT ( 'NONE',  ( -5.049401038298153566, 19.05341960407611168, 115.2072429386477097 ) ) ;
#117768=CARTESIAN_POINT ( 'NONE',  ( -14.29746914071037622, -8.314922557961029526, 104.1677570613523471 ) ) ;
#117769=CARTESIAN_POINT ( 'NONE',  ( 4.379528057220092307, 16.55341960407617563, 57.29275706135234714 ) ) ;
#117770=CARTESIAN_POINT ( 'NONE',  ( 16.46253265017160672, -9.564922557960803928, 73.33224293864769550 ) ) ;
#117771=CARTESIAN_POINT ( 'NONE',  ( 19.02544592524343514, -5.153800228976328945, 83.54057627198100988 ) ) ;
#117772=CARTESIAN_POINT ( 'NONE',  ( 0.05219959533937995610, -21.53943276465977519, 75.00109039468568994 ) ) ;
#117773=CARTESIAN_POINT ( 'NONE',  ( 4.483927247898790824, -16.52544592524335698, 80.20942372801901854 ) ) ;
#117774=CARTESIAN_POINT ( 'NONE',  ( -16.53943276465976808, 0.05219959533911058130, 41.24890960531435269 ) ) ;
#117775=CARTESIAN_POINT ( 'NONE',  ( 19.05341960407611168, 5.049401038298154454, 48.95724293864768129 ) ) ;
#117776=CARTESIAN_POINT ( 'NONE',  ( 19.02544592524343514, -5.153800228976328945, 43.54057627198103120 ) ) ;
#117778=CARTESIAN_POINT ( 'NONE',  ( 5.049401038297881783, 19.05341960407617563, 97.29275706135233293 ) ) ;
#117779=CARTESIAN_POINT ( 'NONE',  ( -8.224510206698948167, 14.34966873604960824, 115.4155762719810241 ) ) ;
#117780=CARTESIAN_POINT ( 'NONE',  ( 9.564922557960805705, 16.46253265017160317, 64.58224293864769550 ) ) ;
#117781=CARTESIAN_POINT ( 'NONE',  ( -5.049401038297874678, -19.05341960407617918, 104.7927570613523471 ) ) ;
#117783=CARTESIAN_POINT ( 'NONE',  ( 10.81492255796106328, -18.62759615963255655, 105.4177570613523613 ) ) ;
#117784=CARTESIAN_POINT ( 'NONE',  ( -16.52544592524335698, -4.483927247898792601, 63.95942372801901854 ) ) ;
#117785=CARTESIAN_POINT ( 'NONE',  ( -19.02544592524334988, -5.153800228976617603, 98.95942372801900433 ) ) ;
#117786=CARTESIAN_POINT ( 'NONE',  ( -15.80617190586745835, -15.72974639402198527, 56.87390960531436690 ) ) ;
#117787=CARTESIAN_POINT ( 'NONE',  ( 12.06949235617739724, 12.14591786802326823, 56.87609039468568994 ) ) ;
#117789=CARTESIAN_POINT ( 'NONE',  ( 19.02544592524334988, 5.153800228976608722, 61.45942372801900433 ) ) ;
#117790=CARTESIAN_POINT ( 'NONE',  ( 21.53943276465977519, 0.05219959533937863772, 96.25109039468568994 ) ) ;
#117791=CARTESIAN_POINT ( 'NONE',  ( -8.314922557960811034, -14.29746914071050412, 112.0822429386477097 ) ) ;
#117792=CARTESIAN_POINT ( 'NONE',  ( 19.05341960407611168, 5.049401038298154454, 63.95724293864769550 ) ) ;
#117793=CARTESIAN_POINT ( 'NONE',  ( -4.379528057220328563, 16.55341960407611168, 55.20724293864770260 ) ) ;
#117796=CARTESIAN_POINT ( 'NONE',  ( 10.81492255796106328, -18.62759615963255655, 95.41775706135234714 ) ) ;
#117797=CARTESIAN_POINT ( 'NONE',  ( 9.474510206698729675, 16.51473224551082808, 52.08442372801900433 ) ) ;
#117798=CARTESIAN_POINT ( 'NONE',  ( -19.02544592524334988, -5.153800228976617603, 33.95942372801897591 ) ) ;
#117799=CARTESIAN_POINT ( 'NONE',  ( 15.72974639402199770, -15.80617190586745480, 23.12390960531436335 ) ) ;
#117800=CARTESIAN_POINT ( 'NONE',  ( -0.05219959533937732626, 21.53943276465977519, 92.50109039468567573 ) ) ;
#117801=CARTESIAN_POINT ( 'NONE',  ( 19.02544592524343514, -5.153800228976328945, 73.54057627198103830 ) ) ;
#117802=CARTESIAN_POINT ( 'NONE',  ( 21.53943276465977519, 0.05219959533937863772, 91.25109039468568994 ) ) ;
#117803=CARTESIAN_POINT ( 'NONE',  ( 5.823673210054125526, 21.52544592524343514, 54.79057627198104541 ) ) ;
#117804=CARTESIAN_POINT ( 'NONE',  ( -9.564922557960796823, -16.46253265017161027, 77.08224293864769550 ) ) ;
#117805=CARTESIAN_POINT ( 'NONE',  ( -5.049401038297874678, -19.05341960407617918, 59.79275706135231871 ) ) ;
#117806=CARTESIAN_POINT ( 'NONE',  ( -5.153800228976328057, -19.02544592524343514, 37.29057627198102409 ) ) ;
#117807=CARTESIAN_POINT ( 'NONE',  ( -0.05219959533909027116, -19.03943276465977164, 92.49890960531436690 ) ) ;
#117808=CARTESIAN_POINT ( 'NONE',  ( -13.89961937509957401, -13.97604488694547875, 84.37609039468567573 ) ) ;
#117809=CARTESIAN_POINT ( 'NONE',  ( 4.379528057220092307, 16.55341960407617563, 47.29275706135234003 ) ) ;
#117810=CARTESIAN_POINT ( 'NONE',  ( 8.314922557960818139, 14.29746914071049879, 104.5822429386477097 ) ) ;
#117811=CARTESIAN_POINT ( 'NONE',  ( -19.02544592524342804, 5.153800228976336051, 66.04057627198103830 ) ) ;
#117812=CARTESIAN_POINT ( 'NONE',  ( 21.55341960407610458, 5.719274019375980345, 53.95724293864770260 ) ) ;
#117813=CARTESIAN_POINT ( 'NONE',  ( 4.483927247898790824, -16.52544592524335698, 25.20942372801901854 ) ) ;
#117814=CARTESIAN_POINT ( 'NONE',  ( -10.81492255796105439, 18.62759615963255655, 37.91775706135235424 ) ) ;
#117815=CARTESIAN_POINT ( 'NONE',  ( -21.52544592524334988, -5.823673210054445271, 88.95942372801901854 ) ) ;
#117816=CARTESIAN_POINT ( 'NONE',  ( 16.52544592524335698, 4.483927247898782831, 86.45942372801901854 ) ) ;
#117817=CARTESIAN_POINT ( 'NONE',  ( 9.564922557960805705, 16.46253265017160317, 79.58224293864769550 ) ) ;
#117818=CARTESIAN_POINT ( 'NONE',  ( -14.29746914071037622, -8.314922557961029526, 99.16775706135234714 ) ) ;
#117819=CARTESIAN_POINT ( 'NONE',  ( -0.05219959533936034679, 19.03943276465977164, 57.50109039468566863 ) ) ;
#117820=CARTESIAN_POINT ( 'NONE',  ( -21.55341960407619339, 5.719274019375674811, 28.54275706135234358 ) ) ;
#117821=CARTESIAN_POINT ( 'NONE',  ( 12.14591786802309770, 12.06949235617756955, 79.37390960531436690 ) ) ;
#117822=CARTESIAN_POINT ( 'NONE',  ( -19.02544592524342804, 5.153800228976336051, 96.04057627198103830 ) ) ;
#117823=CARTESIAN_POINT ( 'NONE',  ( -16.55341960407617563, 4.379528057220093196, 103.5427570613523613 ) ) ;
#117824=CARTESIAN_POINT ( 'NONE',  ( 18.62759615963255655, 10.81492255796105972, 71.66775706135234714 ) ) ;
#117825=CARTESIAN_POINT ( 'NONE',  ( -0.05219959533934338120, 16.53943276465976808, 32.50109039468568284 ) ) ;
#117826=CARTESIAN_POINT ( 'NONE',  ( -21.52544592524334988, -5.823673210054445271, 23.95942372801901143 ) ) ;
#117827=CARTESIAN_POINT ( 'NONE',  ( -16.52544592524342804, 4.483927247898546575, 76.04057627198102409 ) ) ;
#117829=CARTESIAN_POINT ( 'NONE',  ( -15.72974639402197994, 15.80617190586746368, 105.6239096053143669 ) ) ;
#117830=CARTESIAN_POINT ( 'NONE',  ( -16.52544592524342804, 4.483927247898546575, 51.04057627198103120 ) ) ;
#117832=CARTESIAN_POINT ( 'NONE',  ( 16.51473224551069308, 9.474510206698969483, 29.16557627198103475 ) ) ;
#117833=CARTESIAN_POINT ( 'NONE',  ( -21.55341960407610458, -5.719274019375992779, 26.45724293864768839 ) ) ;
#117834=CARTESIAN_POINT ( 'NONE',  ( -15.72974639402176322, -15.80617190586768395, 54.37609039468568994 ) ) ;
#117835=CARTESIAN_POINT ( 'NONE',  ( 14.34966873604960469, 8.224510206698951720, 59.16557627198103120 ) ) ;
#117836=CARTESIAN_POINT ( 'NONE',  ( -18.67979575497178146, -10.72451020669898902, 71.66557627198100988 ) ) ;
#117837=CARTESIAN_POINT ( 'NONE',  ( -0.05219959533909027116, -19.03943276465977164, 72.49890960531435269 ) ) ;
#117838=CARTESIAN_POINT ( 'NONE',  ( -16.51473224551069308, -9.474510206698971260, 21.66557627198102765 ) ) ;
#117839=CARTESIAN_POINT ( 'NONE',  ( -19.05341960407617563, 5.049401038297882671, 83.54275706135233293 ) ) ;
#117841=CARTESIAN_POINT ( 'NONE',  ( 15.72974639402176855, 15.80617190586768217, 51.87609039468568284 ) ) ;
#117842=CARTESIAN_POINT ( 'NONE',  ( -18.62759615963270932, 10.81492255796079327, 55.83224293864770260 ) ) ;
#117843=CARTESIAN_POINT ( 'NONE',  ( 19.05341960407611168, 5.049401038298154454, 43.95724293864769550 ) ) ;
#117844=CARTESIAN_POINT ( 'NONE',  ( -16.51473224551069308, -9.474510206698971260, 66.66557627198102409 ) ) ;
#117845=CARTESIAN_POINT ( 'NONE',  ( 12.06949235617739724, 12.14591786802326823, 56.87609039468568994 ) ) ;
#117846=CARTESIAN_POINT ( 'NONE',  ( -15.80617190586768217, 15.72974639402176855, 28.12609039468568284 ) ) ;
#117847=CARTESIAN_POINT ( 'NONE',  ( -5.823673210054431948, 21.52544592524334988, 57.70942372801901143 ) ) ;
#117848=CARTESIAN_POINT ( 'NONE',  ( 19.05341960407611168, 5.049401038298154454, 103.9572429386476671 ) ) ;
#117849=CARTESIAN_POINT ( 'NONE',  ( 10.81492255796078972, 18.62759615963270932, 79.58224293864769550 ) ) ;
#117850=CARTESIAN_POINT ( 'NONE',  ( -5.719274019375665041, -21.55341960407619695, 24.79275706135235779 ) ) ;
#117851=CARTESIAN_POINT ( 'NONE',  ( -16.52544592524335698, -4.483927247898792601, 53.95942372801900433 ) ) ;
#117852=CARTESIAN_POINT ( 'NONE',  ( -18.62759615963270932, 10.81492255796079327, 55.83224293864770260 ) ) ;
#117853=CARTESIAN_POINT ( 'NONE',  ( -13.97604488694547697, 13.89961937509957934, 23.12609039468565442 ) ) ;
#117854=CARTESIAN_POINT ( 'NONE',  ( 0.05219959533909260263, 19.03943276465977164, 59.99890960531436690 ) ) ;
#117855=CARTESIAN_POINT ( 'NONE',  ( 16.51473224551069308, 9.474510206698969483, 109.1655762719810383 ) ) ;
#117856=B_SPLINE_CURVE_WITH_KNOTS ( 'NONE', 3,
 ( #114092, #6919, #100924, #68597, #23108, #162609 ),
 .UNSPECIFIED., .F., .F.,
 ( 4, 2, 4 ),
 ( 0.003989672132298186825, 0.004372778065220602264, 0.004755883998143018571 ),
 .UNSPECIFIED. ) ;
#117857=CARTESIAN_POINT ( 'NONE',  ( 0.05219959533909260263, 19.03943276465977164, 94.99890960531436690 ) ) ;
#117860=CARTESIAN_POINT ( 'NONE',  ( -16.51473224551082808, 9.474510206698731452, 68.33442372801900433 ) ) ;
#117861=CARTESIAN_POINT ( 'NONE',  ( -5.719274019375978568, 21.55341960407610458, 45.20724293864769550 ) ) ;
#117862=CARTESIAN_POINT ( 'NONE',  ( 8.224510206698953496, -14.34966873604960469, 27.91557627198103830 ) ) ;
#117863=CARTESIAN_POINT ( 'NONE',  ( -13.97604488694547697, 13.89961937509957934, 83.12609039468564731 ) ) ;
#117864=CARTESIAN_POINT ( 'NONE',  ( -17.48853670773243252, 5.747243402303157112, 58.66671299749990709 ) ) ;
#117866=CARTESIAN_POINT ( 'NONE',  ( 19.05341960407617918, -5.049401038297876454, 26.04275706135233293 ) ) ;
#117867=CARTESIAN_POINT ( 'NONE',  ( 19.05341960407617918, -5.049401038297876454, 81.04275706135231871 ) ) ;
#117868=CARTESIAN_POINT ( 'NONE',  ( 19.05341960407617918, -5.049401038297876454, 51.04275706135231871 ) ) ;
#117870=CARTESIAN_POINT ( 'NONE',  ( -9.474510206698964154, 16.51473224551069663, 60.41557627198102409 ) ) ;
#117871=CARTESIAN_POINT ( 'NONE',  ( -12.14591786802309592, -12.06949235617757132, 51.87390960531437401 ) ) ;
#117872=CARTESIAN_POINT ( 'NONE',  ( 5.153800228976335163, 19.02544592524342804, 39.79057627198100988 ) ) ;
#117873=CARTESIAN_POINT ( 'NONE',  ( -16.52544592524342804, 4.483927247898546575, 46.04057627198103830 ) ) ;
#117874=CARTESIAN_POINT ( 'NONE',  ( 18.22780087662123805, 5.499999999999960032, 101.4823681787310647 ) ) ;
#117875=CARTESIAN_POINT ( 'NONE',  ( -14.34966873604960291, -8.224510206698953496, 21.66557627198102409 ) ) ;
#117876=CARTESIAN_POINT ( 'NONE',  ( -16.51473224551069308, -9.474510206698971260, 56.66557627198103120 ) ) ;
#117877=CARTESIAN_POINT ( 'NONE',  ( 13.89961937509957401, 13.97604488694547697, 26.87609039468566507 ) ) ;
#117878=CARTESIAN_POINT ( 'NONE',  ( -0.05219959533934338120, 16.53943276465976808, 32.50109039468568284 ) ) ;
#117879=CARTESIAN_POINT ( 'NONE',  ( -5.719274019375978568, 21.55341960407610458, 40.20724293864769550 ) ) ;
#117880=CARTESIAN_POINT ( 'NONE',  ( 21.53943276465977519, 0.05219959533937863772, 96.25109039468568994 ) ) ;
#117881=CARTESIAN_POINT ( 'NONE',  ( 5.049401038298161559, -19.05341960407611168, 62.70724293864769550 ) ) ;
#117882=CARTESIAN_POINT ( 'NONE',  ( 16.51473224551069308, 9.474510206698969483, 109.1655762719810383 ) ) ;
#117883=CARTESIAN_POINT ( 'NONE',  ( 16.46253265017160672, -9.564922557960803928, 98.33224293864769550 ) ) ;
#117885=CARTESIAN_POINT ( 'NONE',  ( 18.62759615963255655, 10.81492255796105972, 26.66775706135235424 ) ) ;
#117887=CARTESIAN_POINT ( 'NONE',  ( -8.224510206698948167, 14.34966873604960824, 75.41557627198102409 ) ) ;
#117888=CARTESIAN_POINT ( 'NONE',  ( -15.72974639402197994, 15.80617190586746368, 70.62390960531436690 ) ) ;
#117889=CARTESIAN_POINT ( 'NONE',  ( 19.03943276465977164, -0.05219959533909143690, 73.74890960531435269 ) ) ;
#117890=CARTESIAN_POINT ( 'NONE',  ( 5.153800228976335163, 19.02544592524342804, 74.79057627198103830 ) ) ;
#117891=CARTESIAN_POINT ( 'NONE',  ( 21.52544592524344225, -5.823673210054117533, 113.5405762719810383 ) ) ;
#117893=CARTESIAN_POINT ( 'NONE',  ( -9.474510206698964154, 16.51473224551069663, 80.41557627198103830 ) ) ;
#117894=CARTESIAN_POINT ( 'NONE',  ( 4.483927247898545687, 16.52544592524342804, 109.7905762719810383 ) ) ;
#117895=CARTESIAN_POINT ( 'NONE',  ( -13.89961937509977652, 13.97604488694528158, 25.62390960531434558 ) ) ;
#117896=CARTESIAN_POINT ( 'NONE',  ( 19.05341960407611168, 5.049401038298154454, 58.95724293864768129 ) ) ;
#117897=CARTESIAN_POINT ( 'NONE',  ( -5.153800228976607833, 19.02544592524334988, 87.70942372801897591 ) ) ;
#117899=CARTESIAN_POINT ( 'NONE',  ( -16.55341960407611168, -4.379528057220339221, 101.4572429386476955 ) ) ;
#117900=CARTESIAN_POINT ( 'NONE',  ( -0.05219959533937732626, 21.53943276465977519, 72.50109039468568994 ) ) ;
#117901=CARTESIAN_POINT ( 'NONE',  ( 19.02544592524343514, -5.153800228976328945, 43.54057627198103120 ) ) ;
#117902=CARTESIAN_POINT ( 'NONE',  ( 5.823673210054125526, 21.52544592524343514, 114.7905762719810383 ) ) ;
#117903=CARTESIAN_POINT ( 'NONE',  ( -14.29746914071049879, 8.314922557960819915, 95.83224293864770971 ) ) ;
#117905=CARTESIAN_POINT ( 'NONE',  ( 16.51473224551069308, 9.474510206698969483, 69.16557627198102409 ) ) ;
#117907=CARTESIAN_POINT ( 'NONE',  ( -5.049401038297874678, -19.05341960407617918, 109.7927570613523187 ) ) ;
#117908=CARTESIAN_POINT ( 'NONE',  ( 21.53943276465977519, -0.05219959533907433946, 33.74890960531436690 ) ) ;
#117909=CARTESIAN_POINT ( 'NONE',  ( -15.72974639402176322, -15.80617190586768395, 49.37609039468569705 ) ) ;
#117910=CARTESIAN_POINT ( 'NONE',  ( 13.97604488694527802, 13.89961937509977652, 99.37390960531436690 ) ) ;
#117911=CARTESIAN_POINT ( 'NONE',  ( -0.05219959533936034679, 19.03943276465977164, 77.50109039468566152 ) ) ;
#117912=CARTESIAN_POINT ( 'NONE',  ( -16.51473224551069308, -9.474510206698971260, 76.66557627198103830 ) ) ;
#117913=CARTESIAN_POINT ( 'NONE',  ( 12.06949235617757843, -12.14591786802309237, 78.12390960531436690 ) ) ;
#117914=CARTESIAN_POINT ( 'NONE',  ( 13.89961937509977652, -13.97604488694527269, 98.12390960531433848 ) ) ;
#117915=CARTESIAN_POINT ( 'NONE',  ( 8.224510206698953496, -14.34966873604960469, 72.91557627198103830 ) ) ;
#117916=CARTESIAN_POINT ( 'NONE',  ( -16.51473224551069308, -9.474510206698971260, 101.6655762719810241 ) ) ;
#117917=CARTESIAN_POINT ( 'NONE',  ( -19.03943276465977164, 0.05219959533909376836, 51.24890960531436690 ) ) ;
#117918=CARTESIAN_POINT ( 'NONE',  ( 4.483927247898545687, 16.52544592524342804, 49.79057627198102409 ) ) ;
#117919=CARTESIAN_POINT ( 'NONE',  ( 16.51473224551069308, 9.474510206698969483, 29.16557627198103475 ) ) ;
#117921=CARTESIAN_POINT ( 'NONE',  ( -10.72451020669870658, -18.67979575497194134, 59.58442372801901854 ) ) ;
#117922=CARTESIAN_POINT ( 'NONE',  ( -19.03943276465977164, -0.05219959533935918106, 83.75109039468567573 ) ) ;
#117923=CARTESIAN_POINT ( 'NONE',  ( 8.224510206698953496, -14.34966873604960469, 47.91557627198102409 ) ) ;
#117924=CARTESIAN_POINT ( 'NONE',  ( 18.62759615963271287, -10.81492255796078972, 93.33224293864769550 ) ) ;
#117925=CARTESIAN_POINT ( 'NONE',  ( 0.05219959533907565091, 21.53943276465977519, 39.99890960531436690 ) ) ;
#117926=CARTESIAN_POINT ( 'NONE',  ( 14.34966873604960469, 8.224510206698951720, 89.16557627198102409 ) ) ;
#117927=CARTESIAN_POINT ( 'NONE',  ( 16.46253265017160672, -9.564922557960803928, 38.33224293864768839 ) ) ;
#117928=CARTESIAN_POINT ( 'NONE',  ( -16.55341960407617563, 4.379528057220093196, 113.5427570613523756 ) ) ;
#117930=CARTESIAN_POINT ( 'NONE',  ( -14.34966873604972548, 8.224510206698743886, 93.33442372801901854 ) ) ;
#117931=CARTESIAN_POINT ( 'NONE',  ( 16.55341960407618274, -4.379528057220086978, 66.04275706135236135 ) ) ;
#117932=CARTESIAN_POINT ( 'NONE',  ( 19.03943276465977164, 0.05219959533936151252, 21.25109039468565797 ) ) ;
#117933=CARTESIAN_POINT ( 'NONE',  ( -5.049401038298153566, 19.05341960407611168, 90.20724293864766707 ) ) ;
#117934=CARTESIAN_POINT ( 'NONE',  ( 19.05341960407611168, 5.049401038298154454, 83.95724293864766707 ) ) ;
#117935=CARTESIAN_POINT ( 'NONE',  ( -16.55341960407617563, 4.379528057220093196, 88.54275706135236135 ) ) ;
#117936=CARTESIAN_POINT ( 'NONE',  ( 0.05219959533909260263, 19.03943276465977164, 39.99890960531436690 ) ) ;
#117937=CARTESIAN_POINT ( 'NONE',  ( -14.34966873604960291, -8.224510206698953496, 46.66557627198102409 ) ) ;
#117938=DIRECTION ( 'NONE',  ( -1.000000000000000000, -0.000000000000000000, -0.000000000000000000 ) ) ;
#117939=CARTESIAN_POINT ( 'NONE',  ( -19.02544592524342804, 5.153800228976336051, 111.0405762719810099 ) ) ;
#117940=CARTESIAN_POINT ( 'NONE',  ( -0.05219959533907301413, -21.53943276465977519, 32.49890960531435979 ) ) ;
#117941=CARTESIAN_POINT ( 'NONE',  ( 14.29746914071049879, -8.314922557960816363, 73.33224293864769550 ) ) ;
#117943=CARTESIAN_POINT ( 'NONE',  ( 8.314922557960818139, 14.29746914071049879, 64.58224293864769550 ) ) ;
#117945=CARTESIAN_POINT ( 'NONE',  ( 19.05341960407617918, -5.049401038297876454, 66.04275706135233293 ) ) ;
#117946=CARTESIAN_POINT ( 'NONE',  ( -16.46253265017160317, 9.564922557960807481, 105.8322429386476955 ) ) ;
#117947=CARTESIAN_POINT ( 'NONE',  ( 0.05219959533936267826, -19.03943276465977164, 80.00109039468567573 ) ) ;
#117949=CARTESIAN_POINT ( 'NONE',  ( 19.03943276465977164, 0.05219959533936151252, 106.2510903946856615 ) ) ;
#117950=CARTESIAN_POINT ( 'NONE',  ( 16.52544592524335698, 4.483927247898782831, 91.45942372801901854 ) ) ;
#117951=CARTESIAN_POINT ( 'NONE',  ( 19.05341960407611168, 5.049401038298154454, 33.95724293864769550 ) ) ;
#117952=CARTESIAN_POINT ( 'NONE',  ( -18.67979575497178146, -10.72451020669898902, 41.66557627198103120 ) ) ;
#117953=CARTESIAN_POINT ( 'NONE',  ( 5.823673210054444382, -21.52544592524334988, 60.20942372801902565 ) ) ;
#117954=CARTESIAN_POINT ( 'NONE',  ( -13.97604488694547697, 13.89961937509957934, 113.1260903946856757 ) ) ;
#117955=CARTESIAN_POINT ( 'NONE',  ( 17.49999999999996803, 3.285415412585594996, 22.44365530742415160 ) ) ;
#117956=CARTESIAN_POINT ( 'NONE',  ( 5.049401038298161559, -19.05341960407611168, 72.70724293864768129 ) ) ;
#117958=CARTESIAN_POINT ( 'NONE',  ( -4.379528057220328563, 16.55341960407611168, 80.20724293864769550 ) ) ;
#117959=CARTESIAN_POINT ( 'NONE',  ( -19.02544592524342804, 5.153800228976336051, 81.04057627198103830 ) ) ;
#117960=CARTESIAN_POINT ( 'NONE',  ( -9.564922557960796823, -16.46253265017161027, 87.08224293864769550 ) ) ;
#117962=CARTESIAN_POINT ( 'NONE',  ( -13.97604488694547697, 13.89961937509957934, 88.12609039468563310 ) ) ;
#117963=CARTESIAN_POINT ( 'NONE',  ( -5.823673210054116645, -21.52544592524344225, 62.29057627198102409 ) ) ;
#117964=CARTESIAN_POINT ( 'NONE',  ( -9.564922557960796823, -16.46253265017161027, 32.08224293864769550 ) ) ;
#117965=CARTESIAN_POINT ( 'NONE',  ( 13.89961937509957401, 13.97604488694547697, 56.87609039468564731 ) ) ;
#117966=CARTESIAN_POINT ( 'NONE',  ( -5.049401038298153566, 19.05341960407611168, 60.20724293864768129 ) ) ;
#117967=CARTESIAN_POINT ( 'NONE',  ( -5.049401038298153566, 19.05341960407611168, 95.20724293864770971 ) ) ;
#117969=CARTESIAN_POINT ( 'NONE',  ( -18.62759615963270932, 10.81492255796079327, 90.83224293864769550 ) ) ;
#117970=CARTESIAN_POINT ( 'NONE',  ( 12.14591786802309770, 12.06949235617756955, 99.37390960531436690 ) ) ;
#117971=CARTESIAN_POINT ( 'NONE',  ( -13.97604488694547697, 13.89961937509957934, 53.12609039468565442 ) ) ;
#117972=CARTESIAN_POINT ( 'NONE',  ( -15.72974639402197994, 15.80617190586746368, 95.62390960531436690 ) ) ;
#117973=CARTESIAN_POINT ( 'NONE',  ( 5.823673210054125526, 21.52544592524343514, 69.79057627198102409 ) ) ;
#117975=CARTESIAN_POINT ( 'NONE',  ( -16.55341960407611168, -4.379528057220339221, 26.45724293864768839 ) ) ;
#117976=CARTESIAN_POINT ( 'NONE',  ( 21.53943276465977519, 0.05219959533937863772, 106.2510903946856757 ) ) ;
#117977=CARTESIAN_POINT ( 'NONE',  ( -4.483927247898782831, 16.52544592524335698, 47.70942372801902565 ) ) ;
#117978=CARTESIAN_POINT ( 'NONE',  ( -0.05219959533909027116, -19.03943276465977164, 77.49890960531435269 ) ) ;
#117979=CARTESIAN_POINT ( 'NONE',  ( 19.03943276465977164, -0.05219959533909143690, 33.74890960531435979 ) ) ;
#117980=CARTESIAN_POINT ( 'NONE',  ( -18.67979575497193778, 10.72451020669871902, 43.33442372801901143 ) ) ;
#117981=CARTESIAN_POINT ( 'NONE',  ( 10.72451020669871369, 18.67979575497193778, 57.08442372801901854 ) ) ;
#117982=CARTESIAN_POINT ( 'NONE',  ( -0.05219959533909027116, -19.03943276465977164, 52.49890960531436690 ) ) ;
#117983=CARTESIAN_POINT ( 'NONE',  ( 5.823673210054125526, 21.52544592524343514, 114.7905762719810383 ) ) ;
#117984=CARTESIAN_POINT ( 'NONE',  ( 16.51473224551083163, -9.474510206698727899, 65.83442372801900433 ) ) ;
#117985=CARTESIAN_POINT ( 'NONE',  ( -9.564922557961040184, 16.46253265017147172, 77.91775706135234714 ) ) ;
#117986=CARTESIAN_POINT ( 'NONE',  ( 12.06949235617739724, 12.14591786802326823, 26.87609039468567218 ) ) ;
#117987=CARTESIAN_POINT ( 'NONE',  ( -9.564922557960796823, -16.46253265017161027, 27.08224293864769550 ) ) ;
#117988=CARTESIAN_POINT ( 'NONE',  ( 12.14591786802327356, -12.06949235617739191, 75.62609039468567573 ) ) ;
#117989=CARTESIAN_POINT ( 'NONE',  ( 5.153800228976335163, 19.02544592524342804, 39.79057627198100988 ) ) ;
#117991=CARTESIAN_POINT ( 'NONE',  ( -9.474510206698964154, 16.51473224551069663, 105.4155762719810383 ) ) ;
#117992=CARTESIAN_POINT ( 'NONE',  ( 9.474510206698971260, -16.51473224551069308, 27.91557627198103120 ) ) ;
#117993=ADVANCED_FACE ( 'NONE', ( #18280 ), #159754, .F. ) ;
#117994=CARTESIAN_POINT ( 'NONE',  ( -15.80617190586745835, -15.72974639402198527, 76.87390960531439532 ) ) ;
#117995=CARTESIAN_POINT ( 'NONE',  ( 16.53943276465976808, 0.05219959533934440121, 66.25109039468567573 ) ) ;
#117996=CARTESIAN_POINT ( 'NONE',  ( 15.72974639402176855, 15.80617190586768217, 111.8760903946856615 ) ) ;
#117997=CARTESIAN_POINT ( 'NONE',  ( 19.05341960407611168, 5.049401038298154454, 38.95724293864767418 ) ) ;
#117998=CARTESIAN_POINT ( 'NONE',  ( -8.314922557960811034, -14.29746914071050412, 37.08224293864768129 ) ) ;
#117999=CARTESIAN_POINT ( 'NONE',  ( -14.34966873604960291, -8.224510206698953496, 61.66557627198103120 ) ) ;
#118000=CARTESIAN_POINT ( 'NONE',  ( 19.03943276465977164, -0.05219959533909143690, 68.74890960531436690 ) ) ;
#118001=CARTESIAN_POINT ( 'NONE',  ( 15.80617190586769283, -15.72974639402175789, 105.6260903946856899 ) ) ;
#118002=CARTESIAN_POINT ( 'NONE',  ( 5.719274019375673035, 21.55341960407619339, 32.29275706135235424 ) ) ;
#118003=CARTESIAN_POINT ( 'NONE',  ( 13.97604488694527802, 13.89961937509977652, 74.37390960531436690 ) ) ;
#118004=CARTESIAN_POINT ( 'NONE',  ( 21.55341960407619695, -5.719274019375665929, 91.04275706135236135 ) ) ;
#118005=CARTESIAN_POINT ( 'NONE',  ( 16.53943276465976808, 0.05219959533934440121, 66.25109039468567573 ) ) ;
#118006=CARTESIAN_POINT ( 'NONE',  ( 13.89961937509977652, -13.97604488694527269, 103.1239096053143527 ) ) ;
#118007=CARTESIAN_POINT ( 'NONE',  ( 12.14591786802309770, 12.06949235617756955, 29.37390960531435269 ) ) ;
#118008=CARTESIAN_POINT ( 'NONE',  ( -5.153800228976328057, -19.02544592524343514, 27.29057627198103120 ) ) ;
#118009=CARTESIAN_POINT ( 'NONE',  ( -14.29746914071037622, -8.314922557961029526, 59.16775706135234714 ) ) ;
#118010=CARTESIAN_POINT ( 'NONE',  ( -16.55341960407611168, -4.379528057220339221, 61.45724293864770260 ) ) ;
#118011=CARTESIAN_POINT ( 'NONE',  ( -19.05341960407611168, -5.049401038298163336, 111.4572429386476671 ) ) ;
#118012=CARTESIAN_POINT ( 'NONE',  ( 21.52544592524344225, -5.823673210054117533, 33.54057627198102409 ) ) ;
#118013=CARTESIAN_POINT ( 'NONE',  ( 5.719274019375673035, 21.55341960407619339, 107.2927570613523471 ) ) ;
#118014=CARTESIAN_POINT ( 'NONE',  ( 14.34966873604960469, 8.224510206698951720, 89.16557627198102409 ) ) ;
#118015=CARTESIAN_POINT ( 'NONE',  ( -19.02544592524342804, 5.153800228976336051, 96.04057627198103830 ) ) ;
#118016=ORIENTED_EDGE ( 'NONE', *, *, #43597, .F. ) ;
#118017=CARTESIAN_POINT ( 'NONE',  ( -8.224510206698735004, -14.34966873604973081, 54.58442372801901143 ) ) ;
#118018=CARTESIAN_POINT ( 'NONE',  ( -19.02544592524342804, 5.153800228976336051, 51.04057627198103120 ) ) ;
#118019=LINE ( 'NONE', #149351, #11397 ) ;
#118020=CARTESIAN_POINT ( 'NONE',  ( 0.05219959533936267826, -19.03943276465977164, 45.00109039468566863 ) ) ;
#118021=CARTESIAN_POINT ( 'NONE',  ( -4.379528057220086978, -16.55341960407618274, 84.79275706135234714 ) ) ;
#118022=CARTESIAN_POINT ( 'NONE',  ( -19.05341960407617563, 5.049401038297882671, 98.54275706135233293 ) ) ;
#118023=CARTESIAN_POINT ( 'NONE',  ( -10.81492255796105439, 18.62759615963255655, 67.91775706135234714 ) ) ;
#118024=CARTESIAN_POINT ( 'NONE',  ( 5.049401038298161559, -19.05341960407611168, 67.70724293864769550 ) ) ;
#118025=CARTESIAN_POINT ( 'NONE',  ( -5.823673210054116645, -21.52544592524344225, 92.29057627198103830 ) ) ;
#118026=CARTESIAN_POINT ( 'NONE',  ( 8.224510206698953496, -14.34966873604960469, 102.9155762719810383 ) ) ;
#118028=CARTESIAN_POINT ( 'NONE',  ( 0.05219959533936267826, -19.03943276465977164, 70.00109039468566152 ) ) ;
#118029=CARTESIAN_POINT ( 'NONE',  ( -15.72974639402197994, 15.80617190586746368, 60.62390960531437401 ) ) ;
#118030=CARTESIAN_POINT ( 'NONE',  ( -5.049401038297874678, -19.05341960407617918, 39.79275706135232582 ) ) ;
#118031=CARTESIAN_POINT ( 'NONE',  ( 19.05341960407611168, 5.049401038298154454, 113.9572429386477097 ) ) ;
#118032=CARTESIAN_POINT ( 'NONE',  ( -15.80617190586745835, -15.72974639402198527, 91.87390960531436690 ) ) ;
#118033=CARTESIAN_POINT ( 'NONE',  ( -19.26498983726238023, 5.499999999999602096, 55.55319577422003618 ) ) ;
#118035=CARTESIAN_POINT ( 'NONE',  ( -9.474510206698720793, -16.51473224551083518, 109.5844237280190043 ) ) ;
#118036=CARTESIAN_POINT ( 'NONE',  ( -19.02130022317637525, 5.499999999999600320, 60.78188669246576836 ) ) ;
#118037=CARTESIAN_POINT ( 'NONE',  ( 12.14591786802327356, -12.06949235617739191, 30.62609039468567929 ) ) ;
#118038=CARTESIAN_POINT ( 'NONE',  ( 9.564922557960805705, 16.46253265017160317, 49.58224293864770260 ) ) ;
#118039=CARTESIAN_POINT ( 'NONE',  ( 13.89961937509977652, -13.97604488694527269, 108.1239096053143669 ) ) ;
#118040=CARTESIAN_POINT ( 'NONE',  ( 18.62759615963271287, -10.81492255796078972, 93.33224293864769550 ) ) ;
#118041=CARTESIAN_POINT ( 'NONE',  ( 14.34966873604960469, 8.224510206698951720, 54.16557627198103120 ) ) ;
#118043=CARTESIAN_POINT ( 'NONE',  ( 10.81492255796106328, -18.62759615963255655, 75.41775706135233293 ) ) ;
#118044=CARTESIAN_POINT ( 'NONE',  ( 4.379528057220092307, 16.55341960407617563, 22.29275706135235069 ) ) ;
#118045=CARTESIAN_POINT ( 'NONE',  ( -13.89961937509957401, -13.97604488694547875, 29.37609039468565797 ) ) ;
#118046=CARTESIAN_POINT ( 'NONE',  ( 4.483927247898545687, 16.52544592524342804, 34.79057627198103120 ) ) ;
#118047=CARTESIAN_POINT ( 'NONE',  ( 21.55341960407610458, 5.719274019375980345, 108.9572429386476955 ) ) ;
#118048=CARTESIAN_POINT ( 'NONE',  ( -12.14591786802309592, -12.06949235617757132, 46.87390960531435979 ) ) ;
#118049=CARTESIAN_POINT ( 'NONE',  ( -5.153800228976607833, 19.02544592524334988, 97.70942372801900433 ) ) ;
#118050=CARTESIAN_POINT ( 'NONE',  ( 19.03943276465977164, 0.05219959533936151252, 61.25109039468566863 ) ) ;
#118051=CARTESIAN_POINT ( 'NONE',  ( 15.72974639402176855, 15.80617190586768217, 71.87609039468568994 ) ) ;
#118052=CARTESIAN_POINT ( 'NONE',  ( 9.474510206698729675, 16.51473224551082808, 57.08442372801900433 ) ) ;
#118053=CARTESIAN_POINT ( 'NONE',  ( 16.51473224551069308, 9.474510206698969483, 29.16557627198103475 ) ) ;
#118054=CARTESIAN_POINT ( 'NONE',  ( 21.52544592524344225, -5.823673210054117533, 38.54057627198103120 ) ) ;
#118055=CARTESIAN_POINT ( 'NONE',  ( -8.314922557960811034, -14.29746914071050412, 52.08224293864768839 ) ) ;
#118056=CARTESIAN_POINT ( 'NONE',  ( -19.46398650005389186, 5.499999999999950262, 95.18269651486369298 ) ) ;
#118057=CARTESIAN_POINT ( 'NONE',  ( 19.02544592524334988, 5.153800228976608722, 21.45942372801899012 ) ) ;
#118058=CARTESIAN_POINT ( 'NONE',  ( -0.05219959533934338120, 16.53943276465976808, 87.50109039468568994 ) ) ;
#118059=CARTESIAN_POINT ( 'NONE',  ( -14.34966873604960291, -8.224510206698953496, 41.66557627198103120 ) ) ;
#118060=CARTESIAN_POINT ( 'NONE',  ( -10.72451020669870658, -18.67979575497194134, 74.58442372801901854 ) ) ;
#118061=CARTESIAN_POINT ( 'NONE',  ( 21.53943276465977519, 0.05219959533937863772, 71.25109039468568994 ) ) ;
#118062=CARTESIAN_POINT ( 'NONE',  ( -18.67979575497178146, -10.72451020669898902, 76.66557627198103830 ) ) ;
#118063=CARTESIAN_POINT ( 'NONE',  ( -13.89961937509977652, 13.97604488694528158, 40.62390960531435979 ) ) ;
#118064=CARTESIAN_POINT ( 'NONE',  ( 15.72974639402176855, 15.80617190586768217, 56.87609039468568994 ) ) ;
#118065=CARTESIAN_POINT ( 'NONE',  ( 9.564922557960805705, 16.46253265017160317, 29.58224293864769550 ) ) ;
#118066=CARTESIAN_POINT ( 'NONE',  ( -16.51473224551069308, -9.474510206698971260, 51.66557627198102409 ) ) ;
#118067=CARTESIAN_POINT ( 'NONE',  ( -16.55341960407611168, -4.379528057220339221, 91.45724293864769550 ) ) ;
#118068=CARTESIAN_POINT ( 'NONE',  ( -9.474510206698964154, 16.51473224551069663, 85.41557627198102409 ) ) ;
#118069=CARTESIAN_POINT ( 'NONE',  ( -8.314922557960811034, -14.29746914071050412, 42.08224293864769550 ) ) ;
#118070=CARTESIAN_POINT ( 'NONE',  ( 8.314922557960818139, 14.29746914071049879, 99.58224293864770971 ) ) ;
#118071=CARTESIAN_POINT ( 'NONE',  ( -10.81492255796078084, -18.62759615963271287, 72.08224293864769550 ) ) ;
#118072=CARTESIAN_POINT ( 'NONE',  ( -18.67979575497193778, 10.72451020669871902, 28.33442372801902209 ) ) ;
#118073=CARTESIAN_POINT ( 'NONE',  ( 13.89961937509977652, -13.97604488694527269, 113.1239096053143527 ) ) ;
#118074=CARTESIAN_POINT ( 'NONE',  ( 9.564922557960805705, 16.46253265017160317, 79.58224293864769550 ) ) ;
#118075=CARTESIAN_POINT ( 'NONE',  ( 8.224510206698742110, 14.34966873604972548, 27.08442372801901854 ) ) ;
#118076=ADVANCED_FACE ( 'NONE', ( #19271 ), #69768, .T. ) ;
#118077=CARTESIAN_POINT ( 'NONE',  ( -21.53943276465977519, 0.05219959533907696930, 71.24890960531435269 ) ) ;
#118078=CARTESIAN_POINT ( 'NONE',  ( -18.62759615963255300, -10.81492255796106328, 94.16775706135237556 ) ) ;
#118079=CARTESIAN_POINT ( 'NONE',  ( 19.05341960407611168, 5.049401038298154454, 73.95724293864768129 ) ) ;
#118080=CARTESIAN_POINT ( 'NONE',  ( 21.52544592524344225, -5.823673210054117533, 108.5405762719810241 ) ) ;
#118081=CARTESIAN_POINT ( 'NONE',  ( -13.97604488694527625, -13.89961937509977652, 111.8739096053143243 ) ) ;
#118082=CARTESIAN_POINT ( 'NONE',  ( -4.379528057220086978, -16.55341960407618274, 89.79275706135236135 ) ) ;
#118083=CARTESIAN_POINT ( 'NONE',  ( -15.72974639402176322, -15.80617190586768395, 64.37609039468568994 ) ) ;
#118084=CARTESIAN_POINT ( 'NONE',  ( -21.55341960407619339, 5.719274019375674811, 93.54275706135234714 ) ) ;
#118085=CARTESIAN_POINT ( 'NONE',  ( 16.52544592524335698, 4.483927247898782831, 56.45942372801902565 ) ) ;
#118086=CARTESIAN_POINT ( 'NONE',  ( -21.53943276465977519, -0.05219959533937600094, 28.75109039468567929 ) ) ;
#118087=CARTESIAN_POINT ( 'NONE',  ( 13.89961937509977652, -13.97604488694527269, 113.1239096053143527 ) ) ;
#118088=CARTESIAN_POINT ( 'NONE',  ( 5.823673210054444382, -21.52544592524334988, 90.20942372801903275 ) ) ;
#118089=CARTESIAN_POINT ( 'NONE',  ( -16.51473224551069308, -9.474510206698971260, 96.66557627198102409 ) ) ;
#118090=CARTESIAN_POINT ( 'NONE',  ( 18.62759615963271287, -10.81492255796078972, 93.33224293864769550 ) ) ;
#118091=CARTESIAN_POINT ( 'NONE',  ( 9.474510206698729675, 16.51473224551082808, 57.08442372801900433 ) ) ;
#118092=CARTESIAN_POINT ( 'NONE',  ( 5.719274019375991003, -21.55341960407610458, 52.70724293864769550 ) ) ;
#118093=CARTESIAN_POINT ( 'NONE',  ( -19.02544592524342804, 5.153800228976336051, 96.04057627198103830 ) ) ;
#118094=CARTESIAN_POINT ( 'NONE',  ( -4.483927247898539470, -16.52544592524342804, 42.29057627198103120 ) ) ;
#118096=CARTESIAN_POINT ( 'NONE',  ( 19.02544592524334988, 5.153800228976608722, 71.45942372801900433 ) ) ;
#118098=CARTESIAN_POINT ( 'NONE',  ( 5.153800228976615827, -19.02544592524334988, 110.2094237280189901 ) ) ;
#118099=CARTESIAN_POINT ( 'NONE',  ( -5.719274019375978568, 21.55341960407610458, 85.20724293864770971 ) ) ;
#118100=CARTESIAN_POINT ( 'NONE',  ( -16.53943276465976808, 0.05219959533911058130, 66.24890960531436690 ) ) ;
#118101=CARTESIAN_POINT ( 'NONE',  ( 14.29746914071037800, 8.314922557961029526, 36.66775706135234714 ) ) ;
#118102=CARTESIAN_POINT ( 'NONE',  ( -0.05219959533909027116, -19.03943276465977164, 47.49890960531435979 ) ) ;
#118103=CARTESIAN_POINT ( 'NONE',  ( 5.823673210054125526, 21.52544592524343514, 114.7905762719810383 ) ) ;
#118104=CARTESIAN_POINT ( 'NONE',  ( -5.153800228976607833, 19.02544592524334988, 87.70942372801897591 ) ) ;
#118106=CARTESIAN_POINT ( 'NONE',  ( -9.474510206698964154, 16.51473224551069663, 90.41557627198103830 ) ) ;
#118107=CARTESIAN_POINT ( 'NONE',  ( 19.02544592524343514, -5.153800228976328945, 68.54057627198103830 ) ) ;
#118108=CARTESIAN_POINT ( 'NONE',  ( 18.62759615963271287, -10.81492255796078972, 73.33224293864769550 ) ) ;
#118109=CARTESIAN_POINT ( 'NONE',  ( -5.049401038298153566, 19.05341960407611168, 45.20724293864769550 ) ) ;
#118111=CARTESIAN_POINT ( 'NONE',  ( 14.34966873604960469, 8.224510206698951720, 49.16557627198102409 ) ) ;
#118112=CARTESIAN_POINT ( 'NONE',  ( 19.05341960407611168, 5.049401038298154454, 108.9572429386477097 ) ) ;
#118114=CARTESIAN_POINT ( 'NONE',  ( 19.05341960407617918, -5.049401038297876454, 66.04275706135233293 ) ) ;
#118116=CARTESIAN_POINT ( 'NONE',  ( -15.80617190586745835, -15.72974639402198527, 81.87390960531435269 ) ) ;
#118117=CARTESIAN_POINT ( 'NONE',  ( 19.03943276465977164, 0.05219959533936151252, 31.25109039468566863 ) ) ;
#118118=CARTESIAN_POINT ( 'NONE',  ( -9.474510206698964154, 16.51473224551069663, 100.4155762719810241 ) ) ;
#118120=CARTESIAN_POINT ( 'NONE',  ( 18.62759615963271287, -10.81492255796078972, 43.33224293864769550 ) ) ;
#118121=CARTESIAN_POINT ( 'NONE',  ( 13.97604488694527802, 13.89961937509977652, 74.37390960531436690 ) ) ;
#118122=CARTESIAN_POINT ( 'NONE',  ( 0.05219959533937995610, -21.53943276465977519, 70.00109039468568994 ) ) ;
#118123=CARTESIAN_POINT ( 'NONE',  ( 13.89961937509977652, -13.97604488694527269, 28.12390960531435624 ) ) ;
#118124=CARTESIAN_POINT ( 'NONE',  ( -0.05219959533937732626, 21.53943276465977519, 22.50109039468567573 ) ) ;
#118126=CARTESIAN_POINT ( 'NONE',  ( 15.80617190586769283, -15.72974639402175789, 50.62609039468568994 ) ) ;
#118129=CARTESIAN_POINT ( 'NONE',  ( 19.03943276465977164, 0.05219959533936151252, 66.25109039468567573 ) ) ;
#118131=CARTESIAN_POINT ( 'NONE',  ( 15.80617190586746368, 15.72974639402197994, 114.3739096053143527 ) ) ;
#118132=CARTESIAN_POINT ( 'NONE',  ( 5.049401038298161559, -19.05341960407611168, 62.70724293864769550 ) ) ;
#118133=CARTESIAN_POINT ( 'NONE',  ( -16.55341960407617563, 4.379528057220093196, 43.54275706135235424 ) ) ;
#118135=CARTESIAN_POINT ( 'NONE',  ( 21.55341960407619695, -5.719274019375665929, 101.0427570613523756 ) ) ;
#118136=CARTESIAN_POINT ( 'NONE',  ( -0.05219959533909027116, -19.03943276465977164, 42.49890960531435269 ) ) ;
#118137=CARTESIAN_POINT ( 'NONE',  ( 5.719274019375673035, 21.55341960407619339, 112.2927570613523471 ) ) ;
#118138=CARTESIAN_POINT ( 'NONE',  ( -19.02544592524342804, 5.153800228976336051, 91.04057627198100988 ) ) ;
#118139=CARTESIAN_POINT ( 'NONE',  ( 15.80617190586769283, -15.72974639402175789, 60.62609039468567573 ) ) ;
#118140=CARTESIAN_POINT ( 'NONE',  ( -13.89961937509977652, 13.97604488694528158, 115.6239096053143669 ) ) ;
#118142=CARTESIAN_POINT ( 'NONE',  ( -8.314922557961024197, 14.29746914071037800, 47.91775706135234714 ) ) ;
#118143=CARTESIAN_POINT ( 'NONE',  ( -0.05219959533937732626, 21.53943276465977519, 72.50109039468568994 ) ) ;
#118144=CARTESIAN_POINT ( 'NONE',  ( 10.81492255796106328, -18.62759615963255655, 95.41775706135234714 ) ) ;
#118146=CARTESIAN_POINT ( 'NONE',  ( -16.53943276465976808, -0.05219959533934237506, 23.75109039468567929 ) ) ;
#118147=CARTESIAN_POINT ( 'NONE',  ( -19.05341960407611168, -5.049401038298163336, 86.45724293864769550 ) ) ;
#118148=CARTESIAN_POINT ( 'NONE',  ( 5.049401038298161559, -19.05341960407611168, 107.7072429386476955 ) ) ;
#118150=CARTESIAN_POINT ( 'NONE',  ( 17.26172910966777252, 6.454744622555864453, 41.69353091350778584 ) ) ;
#118151=CARTESIAN_POINT ( 'NONE',  ( -19.05341960407611168, -5.049401038298163336, 31.45724293864769550 ) ) ;
#118152=CARTESIAN_POINT ( 'NONE',  ( 0.05219959533907565091, 21.53943276465977519, 39.99890960531436690 ) ) ;
#118153=CARTESIAN_POINT ( 'NONE',  ( 4.483927247898790824, -16.52544592524335698, 110.2094237280190185 ) ) ;
#118154=CARTESIAN_POINT ( 'NONE',  ( 16.55341960407611168, 4.379528057220329451, 88.95724293864769550 ) ) ;
#118155=CARTESIAN_POINT ( 'NONE',  ( 16.51473224551069308, 9.474510206698969483, 69.16557627198102409 ) ) ;
#118156=CARTESIAN_POINT ( 'NONE',  ( 10.81492255796106328, -18.62759615963255655, 85.41775706135236135 ) ) ;
#118157=CARTESIAN_POINT ( 'NONE',  ( -14.34966873604972548, 8.224510206698743886, 23.33442372801901499 ) ) ;
#118158=CARTESIAN_POINT ( 'NONE',  ( -4.379528057220328563, 16.55341960407611168, 90.20724293864770971 ) ) ;
#118159=CARTESIAN_POINT ( 'NONE',  ( 15.72974639402176855, 15.80617190586768217, 46.87609039468568994 ) ) ;
#118160=CARTESIAN_POINT ( 'NONE',  ( -10.72451020669898014, 18.67979575497178502, 80.41557627198103830 ) ) ;
#118161=CARTESIAN_POINT ( 'NONE',  ( 9.564922557961047289, -16.46253265017146816, 40.41775706135234003 ) ) ;
#118163=CARTESIAN_POINT ( 'NONE',  ( -19.03943276465977164, 0.05219959533909376836, 101.2489096053143669 ) ) ;
#118164=CARTESIAN_POINT ( 'NONE',  ( -12.06949235617756955, 12.14591786802309770, 60.62390960531437401 ) ) ;
#118165=CARTESIAN_POINT ( 'NONE',  ( -4.379528057220328563, 16.55341960407611168, 35.20724293864768839 ) ) ;
#118166=CARTESIAN_POINT ( 'NONE',  ( 8.314922557961029526, -14.29746914071037800, 110.4177570613523756 ) ) ;
#118167=CARTESIAN_POINT ( 'NONE',  ( -9.564922557961040184, 16.46253265017147172, 67.91775706135233293 ) ) ;
#118168=CARTESIAN_POINT ( 'NONE',  ( 18.39639308325435962, 5.500000000000037303, 53.98252246182195790 ) ) ;
#118169=CARTESIAN_POINT ( 'NONE',  ( -13.89961937509977652, 13.97604488694528158, 115.6239096053143669 ) ) ;
#118170=CARTESIAN_POINT ( 'NONE',  ( -16.53943276465976808, 0.05219959533911058130, 91.24890960531436690 ) ) ;
#118172=CARTESIAN_POINT ( 'NONE',  ( -16.46253265017160317, 9.564922557960807481, 40.83224293864769550 ) ) ;
#118173=CARTESIAN_POINT ( 'NONE',  ( 18.62759615963271287, -10.81492255796078972, 48.33224293864770260 ) ) ;
#118174=CARTESIAN_POINT ( 'NONE',  ( -21.52544592524343514, 5.823673210054127303, 81.04057627198102409 ) ) ;
#118175=CARTESIAN_POINT ( 'NONE',  ( 16.52544592524342804, -4.483927247898539470, 113.5405762719810383 ) ) ;
#118176=CARTESIAN_POINT ( 'NONE',  ( 12.14591786802327356, -12.06949235617739191, 70.62609039468567573 ) ) ;
#118177=CARTESIAN_POINT ( 'NONE',  ( 5.153800228976335163, 19.02544592524342804, 49.79057627198100988 ) ) ;
#118178=CARTESIAN_POINT ( 'NONE',  ( 16.46253265017146816, 9.564922557961045513, 41.66775706135234003 ) ) ;
#118179=CARTESIAN_POINT ( 'NONE',  ( -21.55341960407619339, 5.719274019375674811, 58.54275706135235424 ) ) ;
#118180=CARTESIAN_POINT ( 'NONE',  ( 14.29746914071049879, -8.314922557960816363, 108.3322429386477097 ) ) ;
#118181=EDGE_CURVE ( 'NONE', #30166, #50977, #3742, .T. ) ;
#118182=CARTESIAN_POINT ( 'NONE',  ( 19.05341960407617918, -5.049401038297876454, 86.04275706135233293 ) ) ;
#118185=CARTESIAN_POINT ( 'NONE',  ( -15.72974639402197994, 15.80617190586746368, 45.62390960531436690 ) ) ;
#118186=CARTESIAN_POINT ( 'NONE',  ( -19.05341960407611168, -5.049401038298163336, 21.45724293864768839 ) ) ;
#118187=CARTESIAN_POINT ( 'NONE',  ( -10.81492255796105439, 18.62759615963255655, 87.91775706135234714 ) ) ;
#118188=CARTESIAN_POINT ( 'NONE',  ( 0.05219959533910956823, 16.53943276465976808, 29.99890960531435979 ) ) ;
#118189=CARTESIAN_POINT ( 'NONE',  ( 12.06949235617739724, 12.14591786802326823, 51.87609039468568284 ) ) ;
#118190=CARTESIAN_POINT ( 'NONE',  ( -12.06949235617756955, 12.14591786802309770, 40.62390960531435269 ) ) ;
#118191=CARTESIAN_POINT ( 'NONE',  ( -21.53943276465977519, 0.05219959533907696930, 86.24890960531436690 ) ) ;
#118192=CARTESIAN_POINT ( 'NONE',  ( -0.05219959533907301413, -21.53943276465977519, 72.49890960531435269 ) ) ;
#118194=CARTESIAN_POINT ( 'NONE',  ( -0.05219959533936034679, 19.03943276465977164, 82.50109039468567573 ) ) ;
#118195=CARTESIAN_POINT ( 'NONE',  ( -5.153800228976328057, -19.02544592524343514, 112.2905762719810099 ) ) ;
#118196=CARTESIAN_POINT ( 'NONE',  ( -5.153800228976328057, -19.02544592524343514, 52.29057627198100988 ) ) ;
#118197=CARTESIAN_POINT ( 'NONE',  ( -13.97604488694527625, -13.89961937509977652, 31.87390960531435979 ) ) ;
#118202=CARTESIAN_POINT ( 'NONE',  ( -4.483927247898782831, 16.52544592524335698, 87.70942372801901854 ) ) ;
#118203=CARTESIAN_POINT ( 'NONE',  ( -10.72451020669898014, 18.67979575497178502, 105.4155762719810383 ) ) ;
#118204=CARTESIAN_POINT ( 'NONE',  ( 19.05341960407611168, 5.049401038298154454, 68.95724293864769550 ) ) ;
#118205=CARTESIAN_POINT ( 'NONE',  ( 15.80617190586769283, -15.72974639402175789, 45.62609039468567573 ) ) ;
#118206=CARTESIAN_POINT ( 'NONE',  ( -19.03943276465977164, 0.05219959533909376836, 96.24890960531436690 ) ) ;
#118209=CARTESIAN_POINT ( 'NONE',  ( -5.823673210054431948, 21.52544592524334988, 27.70942372801901854 ) ) ;
#118210=CARTESIAN_POINT ( 'NONE',  ( 5.049401038298161559, -19.05341960407611168, 22.70724293864769194 ) ) ;
#118211=CARTESIAN_POINT ( 'NONE',  ( -9.474510206698964154, 16.51473224551069663, 100.4155762719810241 ) ) ;
#118212=CARTESIAN_POINT ( 'NONE',  ( 5.153800228976615827, -19.02544592524334988, 35.20942372801899722 ) ) ;
#118213=CARTESIAN_POINT ( 'NONE',  ( 5.823673210054125526, 21.52544592524343514, 109.7905762719810383 ) ) ;
#118214=CARTESIAN_POINT ( 'NONE',  ( -9.474510206698720793, -16.51473224551083518, 44.58442372801900433 ) ) ;
#118215=CARTESIAN_POINT ( 'NONE',  ( 5.153800228976615827, -19.02544592524334988, 55.20942372801899722 ) ) ;
#118216=CARTESIAN_POINT ( 'NONE',  ( 12.14591786802327356, -12.06949235617739191, 95.62609039468568994 ) ) ;
#118218=CARTESIAN_POINT ( 'NONE',  ( 9.474510206698971260, -16.51473224551069308, 77.91557627198103830 ) ) ;
#118220=CARTESIAN_POINT ( 'NONE',  ( -21.52544592524334988, -5.823673210054445271, 73.95942372801901854 ) ) ;
#118221=CARTESIAN_POINT ( 'NONE',  ( -21.52544592524334988, -5.823673210054445271, 88.95942372801901854 ) ) ;
#118223=CARTESIAN_POINT ( 'NONE',  ( -9.564922557960796823, -16.46253265017161027, 92.08224293864769550 ) ) ;
#118224=CARTESIAN_POINT ( 'NONE',  ( 10.72451020669871369, 18.67979575497193778, 62.08442372801901143 ) ) ;
#118225=CARTESIAN_POINT ( 'NONE',  ( -9.564922557961040184, 16.46253265017147172, 97.91775706135233293 ) ) ;
#118226=CARTESIAN_POINT ( 'NONE',  ( -9.564922557960796823, -16.46253265017161027, 72.08224293864770971 ) ) ;
#118227=CARTESIAN_POINT ( 'NONE',  ( -16.46253265017160317, 9.564922557960807481, 105.8322429386476955 ) ) ;
#118228=CARTESIAN_POINT ( 'NONE',  ( 16.51473224551069308, 9.474510206698969483, 84.16557627198102409 ) ) ;
#118229=CARTESIAN_POINT ( 'NONE',  ( -0.05219959533936034679, 19.03943276465977164, 87.50109039468567573 ) ) ;
#118230=CARTESIAN_POINT ( 'NONE',  ( 16.51473224551069308, 9.474510206698969483, 59.16557627198102409 ) ) ;
#118231=CARTESIAN_POINT ( 'NONE',  ( -5.049401038298153566, 19.05341960407611168, 50.20724293864770260 ) ) ;
#118232=CARTESIAN_POINT ( 'NONE',  ( 0.05219959533907565091, 21.53943276465977519, 114.9989096053143669 ) ) ;
#118233=CARTESIAN_POINT ( 'NONE',  ( -16.53943276465976808, -0.05219959533934237506, 103.7510903946857042 ) ) ;
#118236=CARTESIAN_POINT ( 'NONE',  ( -0.05219959533936034679, 19.03943276465977164, 57.50109039468566863 ) ) ;
#118237=CARTESIAN_POINT ( 'NONE',  ( -19.03943276465977164, 0.05219959533909376836, 86.24890960531436690 ) ) ;
#118238=CARTESIAN_POINT ( 'NONE',  ( -14.29746914071049879, 8.314922557960819915, 65.83224293864769550 ) ) ;
#118239=CARTESIAN_POINT ( 'NONE',  ( 0.05219959533910956823, 16.53943276465976808, 104.9989096053143669 ) ) ;
#118240=CARTESIAN_POINT ( 'NONE',  ( 10.72451020669898902, -18.67979575497178502, 27.91557627198103830 ) ) ;
#118241=CARTESIAN_POINT ( 'NONE',  ( -13.89961937509977652, 13.97604488694528158, 110.6239096053143243 ) ) ;
#118242=CARTESIAN_POINT ( 'NONE',  ( -16.55341960407611168, -4.379528057220339221, 91.45724293864769550 ) ) ;
#118243=CARTESIAN_POINT ( 'NONE',  ( 19.02544592524343514, -5.153800228976328945, 113.5405762719810241 ) ) ;
#118244=CARTESIAN_POINT ( 'NONE',  ( -19.02544592524334988, -5.153800228976617603, 33.95942372801897591 ) ) ;
#118245=CARTESIAN_POINT ( 'NONE',  ( -0.05219959533934338120, 16.53943276465976808, 112.5010903946857042 ) ) ;
#118246=CARTESIAN_POINT ( 'NONE',  ( 9.474510206698971260, -16.51473224551069308, 92.91557627198103830 ) ) ;
#118247=CARTESIAN_POINT ( 'NONE',  ( -10.81492255796105439, 18.62759615963255655, 47.91775706135234714 ) ) ;
#118248=CARTESIAN_POINT ( 'NONE',  ( 15.80617190586746368, 15.72974639402197994, 44.37390960531435979 ) ) ;
#118249=CARTESIAN_POINT ( 'NONE',  ( -10.72451020669870658, -18.67979575497194134, 34.58442372801900433 ) ) ;
#118250=CARTESIAN_POINT ( 'NONE',  ( 10.72451020669898902, -18.67979575497178502, 87.91557627198103830 ) ) ;
#118251=CARTESIAN_POINT ( 'NONE',  ( 16.53943276465976808, -0.05219959533910856209, 93.74890960531436690 ) ) ;
#118252=CARTESIAN_POINT ( 'NONE',  ( -13.97604488694547697, 13.89961937509957934, 58.12609039468566863 ) ) ;
#118253=CARTESIAN_POINT ( 'NONE',  ( 9.564922557960805705, 16.46253265017160317, 29.58224293864769550 ) ) ;
#118254=CARTESIAN_POINT ( 'NONE',  ( -19.03943276465977164, 0.05219959533909376836, 91.24890960531436690 ) ) ;
#118255=CARTESIAN_POINT ( 'NONE',  ( 5.049401038298161559, -19.05341960407611168, 92.70724293864769550 ) ) ;
#118256=CARTESIAN_POINT ( 'NONE',  ( -12.06949235617756955, 12.14591786802309770, 110.6239096053143669 ) ) ;
#118258=CARTESIAN_POINT ( 'NONE',  ( 16.52544592524342804, -4.483927247898539470, 28.54057627198103120 ) ) ;
#118259=CARTESIAN_POINT ( 'NONE',  ( -16.52544592524335698, -4.483927247898792601, 43.95942372801902565 ) ) ;
#118260=CARTESIAN_POINT ( 'NONE',  ( 21.53943276465977519, 0.05219959533937863772, 101.2510903946856757 ) ) ;
#118261=CARTESIAN_POINT ( 'NONE',  ( 5.153800228976335163, 19.02544592524342804, 114.7905762719810241 ) ) ;
#118262=CARTESIAN_POINT ( 'NONE',  ( 8.314922557961029526, -14.29746914071037800, 110.4177570613523756 ) ) ;
#118263=CARTESIAN_POINT ( 'NONE',  ( 21.55341960407619695, -5.719274019375665929, 36.04275706135234714 ) ) ;
#118264=CARTESIAN_POINT ( 'NONE',  ( -5.153800228976328057, -19.02544592524343514, 37.29057627198102409 ) ) ;
#118265=CARTESIAN_POINT ( 'NONE',  ( -12.14591786802326823, 12.06949235617739902, 38.12609039468567573 ) ) ;
#118266=CARTESIAN_POINT ( 'NONE',  ( -14.29746914071037622, -8.314922557961029526, 109.1677570613523613 ) ) ;
#118267=CARTESIAN_POINT ( 'NONE',  ( 16.52544592524335698, 4.483927247898782831, 91.45942372801901854 ) ) ;
#118268=CARTESIAN_POINT ( 'NONE',  ( 5.049401038297881783, 19.05341960407617563, 102.2927570613523045 ) ) ;
#118269=CARTESIAN_POINT ( 'NONE',  ( 0.05219959533909260263, 19.03943276465977164, 29.99890960531435979 ) ) ;
#118270=CARTESIAN_POINT ( 'NONE',  ( -16.55341960407611168, -4.379528057220339221, 111.4572429386476813 ) ) ;
#118271=CARTESIAN_POINT ( 'NONE',  ( -21.55341960407619339, 5.719274019375674811, 23.54275706135235424 ) ) ;
#118272=CARTESIAN_POINT ( 'NONE',  ( -19.05341960407611168, -5.049401038298163336, 31.45724293864769550 ) ) ;
#118273=CARTESIAN_POINT ( 'NONE',  ( 16.46253265017160672, -9.564922557960803928, 103.3322429386476955 ) ) ;
#118274=CARTESIAN_POINT ( 'NONE',  ( -10.81492255796105439, 18.62759615963255655, 37.91775706135235424 ) ) ;
#118275=CARTESIAN_POINT ( 'NONE',  ( 5.049401038298161559, -19.05341960407611168, 22.70724293864769194 ) ) ;
#118276=CARTESIAN_POINT ( 'NONE',  ( 0.05219959533909260263, 19.03943276465977164, 104.9989096053143669 ) ) ;
#118278=CARTESIAN_POINT ( 'NONE',  ( 19.03943276465977164, -0.05219959533909143690, 93.74890960531435269 ) ) ;
#118279=CARTESIAN_POINT ( 'NONE',  ( 0.05219959533937995610, -21.53943276465977519, 35.00109039468568284 ) ) ;
#118280=CARTESIAN_POINT ( 'NONE',  ( 14.29746914071049879, -8.314922557960816363, 93.33224293864769550 ) ) ;
#118281=CARTESIAN_POINT ( 'NONE',  ( -9.474510206698964154, 16.51473224551069663, 95.41557627198102409 ) ) ;
#118283=CARTESIAN_POINT ( 'NONE',  ( -4.379528057220086978, -16.55341960407618274, 64.79275706135234714 ) ) ;
#118284=CARTESIAN_POINT ( 'NONE',  ( -10.72451020669870658, -18.67979575497194134, 79.58442372801903275 ) ) ;
#118285=CARTESIAN_POINT ( 'NONE',  ( 14.34966873604972726, -8.224510206698740333, 40.83442372801901854 ) ) ;
#118286=CARTESIAN_POINT ( 'NONE',  ( -13.89961937509977652, 13.97604488694528158, 85.62390960531433848 ) ) ;
#118287=CARTESIAN_POINT ( 'NONE',  ( 13.97604488694548053, -13.89961937509957401, 105.6260903946856757 ) ) ;
#118288=CARTESIAN_POINT ( 'NONE',  ( 4.379528057220092307, 16.55341960407617563, 67.29275706135234714 ) ) ;
#118289=CARTESIAN_POINT ( 'NONE',  ( -21.55341960407619339, 5.719274019375674811, 113.5427570613523756 ) ) ;
#118290=CARTESIAN_POINT ( 'NONE',  ( -0.05219959533936034679, 19.03943276465977164, 97.50109039468567573 ) ) ;
#118291=CARTESIAN_POINT ( 'NONE',  ( -19.02544592524342804, 5.153800228976336051, 66.04057627198103830 ) ) ;
#118292=CARTESIAN_POINT ( 'NONE',  ( 15.72974639402199770, -15.80617190586745480, 83.12390960531436690 ) ) ;
#118293=CARTESIAN_POINT ( 'NONE',  ( -16.55341960407611168, -4.379528057220339221, 86.45724293864770971 ) ) ;
#118294=CARTESIAN_POINT ( 'NONE',  ( 19.02544592524334988, 5.153800228976608722, 91.45942372801900433 ) ) ;
#118295=CARTESIAN_POINT ( 'NONE',  ( 16.52544592524335698, 4.483927247898782831, 56.45942372801902565 ) ) ;
#118297=CARTESIAN_POINT ( 'NONE',  ( 19.03943276465977164, 0.05219959533936151252, 61.25109039468566863 ) ) ;
#118298=CARTESIAN_POINT ( 'NONE',  ( -12.14591786802309592, -12.06949235617757132, 26.87390960531435979 ) ) ;
#118299=CARTESIAN_POINT ( 'NONE',  ( 12.14591786802309770, 12.06949235617756955, 84.37390960531438111 ) ) ;
#118300=CARTESIAN_POINT ( 'NONE',  ( 16.51473224551083163, -9.474510206698727899, 20.83442372801899722 ) ) ;
#118301=CARTESIAN_POINT ( 'NONE',  ( -19.46398650005392028, 5.499999999999953815, 90.18269651486369298 ) ) ;
#118302=CARTESIAN_POINT ( 'NONE',  ( -15.80617190586768217, 15.72974639402176855, 28.12609039468568284 ) ) ;
#118303=CARTESIAN_POINT ( 'NONE',  ( 9.564922557960805705, 16.46253265017160317, 99.58224293864770971 ) ) ;
#118304=CARTESIAN_POINT ( 'NONE',  ( 9.564922557960805705, 16.46253265017160317, 74.58224293864769550 ) ) ;
#118305=CARTESIAN_POINT ( 'NONE',  ( -5.823673210054431948, 21.52544592524334988, 102.7094237280190185 ) ) ;
#118306=CARTESIAN_POINT ( 'NONE',  ( 13.89961937509977652, -13.97604488694527269, 73.12390960531436690 ) ) ;
#118307=CARTESIAN_POINT ( 'NONE',  ( -18.67979575497178146, -10.72451020669898902, 31.66557627198102054 ) ) ;
#118308=CARTESIAN_POINT ( 'NONE',  ( -12.14591786802309592, -12.06949235617757132, 86.87390960531438111 ) ) ;
#118309=CARTESIAN_POINT ( 'NONE',  ( 5.153800228976335163, 19.02544592524342804, 49.79057627198100988 ) ) ;
#118310=CARTESIAN_POINT ( 'NONE',  ( 16.55341960407611168, 4.379528057220329451, 98.95724293864770971 ) ) ;
#118311=CARTESIAN_POINT ( 'NONE',  ( -5.823673210054116645, -21.52544592524344225, 107.2905762719810525 ) ) ;
#118312=CARTESIAN_POINT ( 'NONE',  ( -21.55341960407619339, 5.719274019375674811, 58.54275706135235424 ) ) ;
#118313=CARTESIAN_POINT ( 'NONE',  ( -0.05219959533909027116, -19.03943276465977164, 32.49890960531435979 ) ) ;
#118314=CARTESIAN_POINT ( 'NONE',  ( 0.05219959533934541429, -16.53943276465976808, 65.00109039468568994 ) ) ;
#118315=CARTESIAN_POINT ( 'NONE',  ( -21.52544592524343514, 5.823673210054127303, 101.0405762719810383 ) ) ;
#118316=CARTESIAN_POINT ( 'NONE',  ( -15.72974639402197994, 15.80617190586746368, 105.6239096053143669 ) ) ;
#118317=CARTESIAN_POINT ( 'NONE',  ( 9.474510206698729675, 16.51473224551082808, 42.08442372801900433 ) ) ;
#118318=CARTESIAN_POINT ( 'NONE',  ( 13.97604488694527802, 13.89961937509977652, 54.37390960531435979 ) ) ;
#118319=CARTESIAN_POINT ( 'NONE',  ( 0.05219959533909260263, 19.03943276465977164, 114.9989096053143669 ) ) ;
#118320=CARTESIAN_POINT ( 'NONE',  ( -0.05219959533937732626, 21.53943276465977519, 52.50109039468567573 ) ) ;
#118321=CARTESIAN_POINT ( 'NONE',  ( -21.52544592524343514, 5.823673210054127303, 51.04057627198103120 ) ) ;
#118322=CARTESIAN_POINT ( 'NONE',  ( 12.06949235617757843, -12.14591786802309237, 43.12390960531435269 ) ) ;
#118323=CARTESIAN_POINT ( 'NONE',  ( 21.52544592524334988, 5.823673210054432836, 81.45942372801900433 ) ) ;
#118324=CARTESIAN_POINT ( 'NONE',  ( -0.05219959533937732626, 21.53943276465977519, 107.5010903946856899 ) ) ;
#118325=CARTESIAN_POINT ( 'NONE',  ( 12.06949235617757843, -12.14591786802309237, 53.12390960531436690 ) ) ;
#118326=CARTESIAN_POINT ( 'NONE',  ( -16.55341960407611168, -4.379528057220339221, 111.4572429386476813 ) ) ;
#118327=CARTESIAN_POINT ( 'NONE',  ( -13.97604488694547697, 13.89961937509957934, 43.12609039468566152 ) ) ;
#118328=CARTESIAN_POINT ( 'NONE',  ( -0.05219959533934338120, 16.53943276465976808, 102.5010903946856899 ) ) ;
#118329=CARTESIAN_POINT ( 'NONE',  ( -21.55341960407619339, 5.719274019375674811, 73.54275706135234714 ) ) ;
#118330=CARTESIAN_POINT ( 'NONE',  ( -13.89961937509977652, 13.97604488694528158, 60.62390960531436690 ) ) ;
#118331=CARTESIAN_POINT ( 'NONE',  ( -9.474510206698720793, -16.51473224551083518, 39.58442372801899722 ) ) ;
#118332=CARTESIAN_POINT ( 'NONE',  ( -21.53943276465977519, 0.05219959533907696930, 36.24890960531435979 ) ) ;
#118333=CARTESIAN_POINT ( 'NONE',  ( 18.62759615963255655, 10.81492255796105972, 31.66775706135234358 ) ) ;
#118334=CARTESIAN_POINT ( 'NONE',  ( -18.67979575497178146, -10.72451020669898902, 86.66557627198102409 ) ) ;
#118335=CARTESIAN_POINT ( 'NONE',  ( -13.97604488694547697, 13.89961937509957934, 88.12609039468563310 ) ) ;
#118336=CARTESIAN_POINT ( 'NONE',  ( -8.314922557961024197, 14.29746914071037800, 57.91775706135234714 ) ) ;
#118338=CARTESIAN_POINT ( 'NONE',  ( -5.719274019375978568, 21.55341960407610458, 95.20724293864769550 ) ) ;
#118339=CARTESIAN_POINT ( 'NONE',  ( 12.06949235617757843, -12.14591786802309237, 73.12390960531436690 ) ) ;
#118341=CARTESIAN_POINT ( 'NONE',  ( -16.53943276465976808, -0.05219959533934237506, 18.75109039468568639 ) ) ;
#118342=CARTESIAN_POINT ( 'NONE',  ( 18.67979575497178502, 10.72451020669898547, 44.16557627198103120 ) ) ;
#118343=CARTESIAN_POINT ( 'NONE',  ( -0.05219959533934338120, 16.53943276465976808, 77.50109039468567573 ) ) ;
#118344=CARTESIAN_POINT ( 'NONE',  ( 17.50000000000000000, -5.500000000000000888, 120.0000000000000142 ) ) ;
#118345=CARTESIAN_POINT ( 'NONE',  ( -14.29746914071037622, -8.314922557961029526, 54.16775706135235424 ) ) ;
#118346=CARTESIAN_POINT ( 'NONE',  ( 0.05219959533937995610, -21.53943276465977519, 25.00109039468567218 ) ) ;
#118347=CARTESIAN_POINT ( 'NONE',  ( -15.72974639402197994, 15.80617190586746368, 45.62390960531436690 ) ) ;
#118348=CARTESIAN_POINT ( 'NONE',  ( -14.29746914071037622, -8.314922557961029526, 74.16775706135231871 ) ) ;
#118349=CARTESIAN_POINT ( 'NONE',  ( -19.02544592524342804, 5.153800228976336051, 96.04057627198103830 ) ) ;
#118350=CARTESIAN_POINT ( 'NONE',  ( 21.55341960407619695, -5.719274019375665929, 56.04275706135235424 ) ) ;
#118351=CARTESIAN_POINT ( 'NONE',  ( 19.02544592524343514, -5.153800228976328945, 33.54057627198102409 ) ) ;
#118353=CARTESIAN_POINT ( 'NONE',  ( -5.823673210054116645, -21.52544592524344225, 42.29057627198103120 ) ) ;
#118354=CARTESIAN_POINT ( 'NONE',  ( 18.62759615963271287, -10.81492255796078972, 23.33224293864769194 ) ) ;
#118356=CARTESIAN_POINT ( 'NONE',  ( -9.564922557961040184, 16.46253265017147172, 32.91775706135233293 ) ) ;
#118357=CARTESIAN_POINT ( 'NONE',  ( 16.52544592524335698, 4.483927247898782831, 46.45942372801901854 ) ) ;
#118358=CARTESIAN_POINT ( 'NONE',  ( 13.97604488694527802, 13.89961937509977652, 109.3739096053143669 ) ) ;
#118360=CARTESIAN_POINT ( 'NONE',  ( 19.05341960407611168, 5.049401038298154454, 83.95724293864766707 ) ) ;
#118361=CARTESIAN_POINT ( 'NONE',  ( -8.224510206698735004, -14.34966873604973081, 99.58442372801900433 ) ) ;
#118363=CARTESIAN_POINT ( 'NONE',  ( 4.483927247898545687, 16.52544592524342804, 89.79057627198103830 ) ) ;
#118364=CARTESIAN_POINT ( 'NONE',  ( 0.05219959533907565091, 21.53943276465977519, 49.99890960531437401 ) ) ;
#118365=CARTESIAN_POINT ( 'NONE',  ( -5.153800228976328057, -19.02544592524343514, 27.29057627198103120 ) ) ;
#118366=CARTESIAN_POINT ( 'NONE',  ( 8.314922557961029526, -14.29746914071037800, 75.41775706135233293 ) ) ;
#118367=CARTESIAN_POINT ( 'NONE',  ( 18.67979575497194134, -10.72451020669871369, 25.83442372801901499 ) ) ;
#118368=CARTESIAN_POINT ( 'NONE',  ( 19.02544592524334988, 5.153800228976608722, 91.45942372801900433 ) ) ;
#118369=CARTESIAN_POINT ( 'NONE',  ( 5.153800228976335163, 19.02544592524342804, 44.79057627198103830 ) ) ;
#118370=CARTESIAN_POINT ( 'NONE',  ( 0.05219959533909260263, 19.03943276465977164, 109.9989096053143669 ) ) ;
#118371=CARTESIAN_POINT ( 'NONE',  ( -10.72451020669870658, -18.67979575497194134, 104.5844237280190185 ) ) ;
#118372=CARTESIAN_POINT ( 'NONE',  ( 16.46253265017160672, -9.564922557960803928, 78.33224293864769550 ) ) ;
#118373=CARTESIAN_POINT ( 'NONE',  ( 8.224510206698742110, 14.34966873604972548, 57.08442372801901854 ) ) ;
#118374=CARTESIAN_POINT ( 'NONE',  ( 5.823673210054444382, -21.52544592524334988, 90.20942372801903275 ) ) ;
#118375=CARTESIAN_POINT ( 'NONE',  ( 19.05341960407617918, -5.049401038297876454, 51.04275706135231871 ) ) ;
#118376=CARTESIAN_POINT ( 'NONE',  ( 16.46253265017146816, 9.564922557961045513, 71.66775706135233293 ) ) ;
#118378=CARTESIAN_POINT ( 'NONE',  ( -10.72451020669870658, -18.67979575497194134, 69.58442372801900433 ) ) ;
#118379=CARTESIAN_POINT ( 'NONE',  ( -9.564922557960796823, -16.46253265017161027, 27.08224293864769550 ) ) ;
#118380=CARTESIAN_POINT ( 'NONE',  ( 16.51473224551083163, -9.474510206698727899, 55.83442372801899722 ) ) ;
#118381=CARTESIAN_POINT ( 'NONE',  ( -19.03943276465977164, 0.05219959533909376836, 101.2489096053143669 ) ) ;
#118382=CARTESIAN_POINT ( 'NONE',  ( 13.89961937509977652, -13.97604488694527269, 88.12390960531438111 ) ) ;
#118383=CARTESIAN_POINT ( 'NONE',  ( -4.379528057220328563, 16.55341960407611168, 40.20724293864769550 ) ) ;
#118384=CARTESIAN_POINT ( 'NONE',  ( -15.80617190586745835, -15.72974639402198527, 31.87390960531435979 ) ) ;
#118387=CARTESIAN_POINT ( 'NONE',  ( -15.80617190586768217, 15.72974639402176855, 113.1260903946856899 ) ) ;
#118389=CARTESIAN_POINT ( 'NONE',  ( -9.564922557960796823, -16.46253265017161027, 42.08224293864769550 ) ) ;
#118390=CARTESIAN_POINT ( 'NONE',  ( -13.89961937509977830, 13.97604488694528158, 85.62390960531435269 ) ) ;
#118391=CARTESIAN_POINT ( 'NONE',  ( -17.72517630440434289, 5.499999999999979572, 80.92175719257211597 ) ) ;
#118392=CARTESIAN_POINT ( 'NONE',  ( 21.55341960407619695, -5.719274019375665929, 71.04275706135234714 ) ) ;
#118394=CARTESIAN_POINT ( 'NONE',  ( -12.06949235617739369, -12.14591786802326823, 64.37609039468568994 ) ) ;
#118395=CARTESIAN_POINT ( 'NONE',  ( -21.53943276465977519, 0.05219959533907696930, 81.24890960531436690 ) ) ;
#118396=CARTESIAN_POINT ( 'NONE',  ( 16.53943276465976808, -0.05219959533910856209, 58.74890960531436690 ) ) ;
#118397=CARTESIAN_POINT ( 'NONE',  ( 13.89961937509977652, -13.97604488694527269, 23.12390960531436335 ) ) ;
#118398=CARTESIAN_POINT ( 'NONE',  ( -5.153800228976328057, -19.02544592524343514, 102.2905762719810383 ) ) ;
#118399=CARTESIAN_POINT ( 'NONE',  ( 18.67979575497194134, -10.72451020669871369, 25.83442372801901499 ) ) ;
#118400=CARTESIAN_POINT ( 'NONE',  ( 19.03943276465977164, 0.05219959533936151252, 31.25109039468566863 ) ) ;
#118401=CARTESIAN_POINT ( 'NONE',  ( -9.564922557960796823, -16.46253265017161027, 37.08224293864768839 ) ) ;
#118402=CARTESIAN_POINT ( 'NONE',  ( -0.05219959533937732626, 21.53943276465977519, 82.50109039468568994 ) ) ;
#118404=CARTESIAN_POINT ( 'NONE',  ( 14.29746914071049879, -8.314922557960816363, 23.33224293864769194 ) ) ;
#118406=CARTESIAN_POINT ( 'NONE',  ( 21.53943276465977519, -0.05219959533907433946, 38.74890960531435979 ) ) ;
#118407=CARTESIAN_POINT ( 'NONE',  ( 16.53943276465976808, -0.05219959533910856209, 98.74890960531438111 ) ) ;
#118410=CARTESIAN_POINT ( 'NONE',  ( -13.89961937509977652, 13.97604488694528158, 90.62390960531432427 ) ) ;
#118411=CARTESIAN_POINT ( 'NONE',  ( -14.29746914071049879, 8.314922557960819915, 90.83224293864769550 ) ) ;
#118412=CARTESIAN_POINT ( 'NONE',  ( -13.89961937509957401, -13.97604488694547875, 104.3760903946856757 ) ) ;
#118413=CARTESIAN_POINT ( 'NONE',  ( -15.80617190586745835, -15.72974639402198527, 66.87390960531436690 ) ) ;
#118415=CARTESIAN_POINT ( 'NONE',  ( -16.51473224551069308, -9.474510206698971260, 26.66557627198103120 ) ) ;
#118416=CARTESIAN_POINT ( 'NONE',  ( -19.05341960407611168, -5.049401038298163336, 86.45724293864769550 ) ) ;
#118417=CARTESIAN_POINT ( 'NONE',  ( 5.823673210054125526, 21.52544592524343514, 94.79057627198105251 ) ) ;
#118418=CARTESIAN_POINT ( 'NONE',  ( -16.52544592524335698, -4.483927247898792601, 103.9594237280190185 ) ) ;
#118419=CARTESIAN_POINT ( 'NONE',  ( -5.153800228976328057, -19.02544592524343514, 82.29057627198103830 ) ) ;
#118420=CARTESIAN_POINT ( 'NONE',  ( 19.02544592524334988, 5.153800228976608722, 86.45942372801900433 ) ) ;
#118421=CARTESIAN_POINT ( 'NONE',  ( 18.67979575497194134, -10.72451020669871369, 95.83442372801903275 ) ) ;
#118422=CARTESIAN_POINT ( 'NONE',  ( 15.72974639402199770, -15.80617190586745480, 73.12390960531436690 ) ) ;
#118423=CARTESIAN_POINT ( 'NONE',  ( -10.81492255796078084, -18.62759615963271287, 37.08224293864768129 ) ) ;
#118424=CARTESIAN_POINT ( 'NONE',  ( -5.049401038298153566, 19.05341960407611168, 45.20724293864769550 ) ) ;
#118425=CARTESIAN_POINT ( 'NONE',  ( -0.05219959533934338120, 16.53943276465976808, 107.5010903946856899 ) ) ;
#118426=CARTESIAN_POINT ( 'NONE',  ( 9.564922557960805705, 16.46253265017160317, 64.58224293864769550 ) ) ;
#118429=CARTESIAN_POINT ( 'NONE',  ( -13.97604488694547697, 13.89961937509957934, 23.12609039468565442 ) ) ;
#118430=CARTESIAN_POINT ( 'NONE',  ( 8.224510206698953496, -14.34966873604960469, 67.91557627198102409 ) ) ;
#118431=CARTESIAN_POINT ( 'NONE',  ( -5.719274019375665041, -21.55341960407619695, 29.79275706135234358 ) ) ;
#118433=CARTESIAN_POINT ( 'NONE',  ( 21.55341960407610458, 5.719274019375980345, 53.95724293864770260 ) ) ;
#118434=CARTESIAN_POINT ( 'NONE',  ( -4.483927247898782831, 16.52544592524335698, 92.70942372801901854 ) ) ;
#118435=CARTESIAN_POINT ( 'NONE',  ( 0.05219959533910956823, 16.53943276465976808, 104.9989096053143669 ) ) ;
#118436=CARTESIAN_POINT ( 'NONE',  ( 0.05219959533909260263, 19.03943276465977164, 69.99890960531435269 ) ) ;
#118437=CARTESIAN_POINT ( 'NONE',  ( 14.29746914071049879, -8.314922557960816363, 28.33224293864769550 ) ) ;
#118438=CARTESIAN_POINT ( 'NONE',  ( -10.81492255796105439, 18.62759615963255655, 52.91775706135235424 ) ) ;
#118439=CARTESIAN_POINT ( 'NONE',  ( 16.46253265017160672, -9.564922557960803928, 113.3322429386476955 ) ) ;
#118440=CARTESIAN_POINT ( 'NONE',  ( 10.72451020669871369, 18.67979575497193778, 77.08442372801901854 ) ) ;
#118441=CARTESIAN_POINT ( 'NONE',  ( 9.564922557960805705, 16.46253265017160317, 24.58224293864769194 ) ) ;
#118442=CARTESIAN_POINT ( 'NONE',  ( -19.03943276465977164, 0.05219959533909376836, 36.24890960531436690 ) ) ;
#118445=CARTESIAN_POINT ( 'NONE',  ( 21.52544592524334988, 5.823673210054432836, 96.45942372801901854 ) ) ;
#118446=CARTESIAN_POINT ( 'NONE',  ( 12.14591786802327356, -12.06949235617739191, 45.62609039468567573 ) ) ;
#118447=CARTESIAN_POINT ( 'NONE',  ( -0.05219959533937732626, 21.53943276465977519, 72.50109039468568994 ) ) ;
#118448=CARTESIAN_POINT ( 'NONE',  ( -5.153800228976328057, -19.02544592524343514, 107.2905762719810383 ) ) ;
#118450=CARTESIAN_POINT ( 'NONE',  ( -19.03943276465977164, -0.05219959533935918106, 83.75109039468567573 ) ) ;
#118451=CARTESIAN_POINT ( 'NONE',  ( -10.72451020669870658, -18.67979575497194134, 49.58442372801901143 ) ) ;
#118452=CARTESIAN_POINT ( 'NONE',  ( -0.05219959533936034679, 19.03943276465977164, 112.5010903946856757 ) ) ;
#118453=CARTESIAN_POINT ( 'NONE',  ( 16.46253265017146816, 9.564922557961045513, 81.66775706135233293 ) ) ;
#118454=CARTESIAN_POINT ( 'NONE',  ( -19.02544592524342804, 5.153800228976336051, 46.04057627198101699 ) ) ;
#118455=CARTESIAN_POINT ( 'NONE',  ( -13.97604488694547697, 13.89961937509957934, 93.12609039468566152 ) ) ;
#118456=CARTESIAN_POINT ( 'NONE',  ( -0.05219959533934338120, 16.53943276465976808, 112.5010903946857042 ) ) ;
#118457=CARTESIAN_POINT ( 'NONE',  ( -16.51473224551082808, 9.474510206698731452, 83.33442372801899012 ) ) ;
#118458=CARTESIAN_POINT ( 'NONE',  ( 8.314922557960818139, 14.29746914071049879, 44.58224293864769550 ) ) ;
#118459=CARTESIAN_POINT ( 'NONE',  ( -19.05341960407617563, 5.049401038297882671, 58.54275706135234003 ) ) ;
#118460=CARTESIAN_POINT ( 'NONE',  ( -0.05219959533934338120, 16.53943276465976808, 47.50109039468568994 ) ) ;
#118461=CARTESIAN_POINT ( 'NONE',  ( -10.81492255796105439, 18.62759615963255655, 112.9177570613523329 ) ) ;
#118462=CARTESIAN_POINT ( 'NONE',  ( 16.46253265017160672, -9.564922557960803928, 28.33224293864769550 ) ) ;
#118463=CARTESIAN_POINT ( 'NONE',  ( 0.05219959533909260263, 19.03943276465977164, 39.99890960531436690 ) ) ;
#118464=CARTESIAN_POINT ( 'NONE',  ( -14.29746914071037622, -8.314922557961029526, 49.16775706135234003 ) ) ;
#118467=CARTESIAN_POINT ( 'NONE',  ( 9.564922557960805705, 16.46253265017160317, 89.58224293864769550 ) ) ;
#118470=CARTESIAN_POINT ( 'NONE',  ( -9.474510206698720793, -16.51473224551083518, 94.58442372801900433 ) ) ;
#118471=B_SPLINE_CURVE_WITH_KNOTS ( 'NONE', 3,
 ( #109553, #168250, #125721, #171234, #110543, #68020, #115538, #36676, #98336, #18553, #189395, #65038, #33709, #173226, #21522, #53864, #145855, #97340, #22528, #37686, #66028, #112530, #34702, #83183, #160035, #80201, #84175, #50872, #192381, #5342, #7337, #126694 ),
 .UNSPECIFIED., .F., .F.,
 ( 4, 2, 2, 2, 2, 2, 2, 2, 2, 2, 2, 2, 2, 2, 2, 4 ),
 ( 2.195984522899319715E-17, 0.0003712461730036815196, 0.0007424923460073411382, 0.001113738519011000594, 0.001484984692014660159, 0.002227477038021986010, 0.002598723211025666391, 0.002969969384029346772, 0.003341215557033026719, 0.003712461730036707968, 0.004083707903040387915, 0.004454954076044069164, 0.004826200249047748678, 0.005197446422051429926, 0.005568692595055110307, 0.005939938768058790688 ),
 .UNSPECIFIED. ) ;
#118472=CARTESIAN_POINT ( 'NONE',  ( 18.67979575497178502, 10.72451020669898547, 34.16557627198102409 ) ) ;
#118473=CARTESIAN_POINT ( 'NONE',  ( -0.05219959533936034679, 19.03943276465977164, 37.50109039468567573 ) ) ;
#118474=CARTESIAN_POINT ( 'NONE',  ( -13.89961937509957401, -13.97604488694547875, 109.3760903946856331 ) ) ;
#118475=CARTESIAN_POINT ( 'NONE',  ( 16.55341960407611168, 4.379528057220329451, 113.9572429386477239 ) ) ;
#118476=CARTESIAN_POINT ( 'NONE',  ( 5.049401038298161559, -19.05341960407611168, 42.70724293864767418 ) ) ;
#118477=CARTESIAN_POINT ( 'NONE',  ( 18.62759615963271287, -10.81492255796078972, 73.33224293864769550 ) ) ;
#118478=ADVANCED_FACE ( 'NONE', ( #184797 ), #158263, .F. ) ;
#118479=CARTESIAN_POINT ( 'NONE',  ( -19.02544592524342804, 5.153800228976336051, 36.04057627198100988 ) ) ;
#118481=CARTESIAN_POINT ( 'NONE',  ( 9.564922557961047289, -16.46253265017146816, 65.41775706135233293 ) ) ;
#118482=CARTESIAN_POINT ( 'NONE',  ( 4.483927247898545687, 16.52544592524342804, 59.79057627198103120 ) ) ;
#118483=CARTESIAN_POINT ( 'NONE',  ( 15.72974639402199770, -15.80617190586745480, 33.12390960531435979 ) ) ;
#118484=CARTESIAN_POINT ( 'NONE',  ( 21.53943276465977519, 0.05219959533937863772, 91.25109039468568994 ) ) ;
#118485=CARTESIAN_POINT ( 'NONE',  ( 18.62759615963271287, -10.81492255796078972, 78.33224293864770971 ) ) ;
#118486=CARTESIAN_POINT ( 'NONE',  ( -0.05219959533937732626, 21.53943276465977519, 72.50109039468568994 ) ) ;
#118487=CARTESIAN_POINT ( 'NONE',  ( -18.62759615963255300, -10.81492255796106328, 59.16775706135234714 ) ) ;
#118488=CARTESIAN_POINT ( 'NONE',  ( -13.89961937509977652, 13.97604488694528158, 95.62390960531436690 ) ) ;
#118489=CARTESIAN_POINT ( 'NONE',  ( 4.483927247898790824, -16.52544592524335698, 110.2094237280190185 ) ) ;
#118490=CARTESIAN_POINT ( 'NONE',  ( -18.67979575497193778, 10.72451020669871902, 63.33442372801900433 ) ) ;
#118491=CARTESIAN_POINT ( 'NONE',  ( -0.05219959533909027116, -19.03943276465977164, 52.49890960531436690 ) ) ;
#118492=CARTESIAN_POINT ( 'NONE',  ( -5.823673210054431948, 21.52544592524334988, 27.70942372801901854 ) ) ;
#118493=CARTESIAN_POINT ( 'NONE',  ( 9.474510206698971260, -16.51473224551069308, 62.91557627198102409 ) ) ;
#118494=CARTESIAN_POINT ( 'NONE',  ( -12.14591786802309592, -12.06949235617757132, 76.87390960531439532 ) ) ;
#118495=CARTESIAN_POINT ( 'NONE',  ( 0.05219959533910956823, 16.53943276465976808, 44.99890960531435979 ) ) ;
#118496=CARTESIAN_POINT ( 'NONE',  ( -15.72974639402197994, 15.80617190586746368, 55.62390960531436690 ) ) ;
#118497=CARTESIAN_POINT ( 'NONE',  ( 9.474510206698971260, -16.51473224551069308, 42.91557627198103120 ) ) ;
#118498=CARTESIAN_POINT ( 'NONE',  ( 18.62759615963271287, -10.81492255796078972, 53.33224293864769550 ) ) ;
#118499=CARTESIAN_POINT ( 'NONE',  ( 16.51473224551083163, -9.474510206698727899, 50.83442372801899722 ) ) ;
#118502=CARTESIAN_POINT ( 'NONE',  ( -16.52544592524342804, 4.483927247898546575, 61.04057627198103120 ) ) ;
#118503=CARTESIAN_POINT ( 'NONE',  ( -18.67979575497178146, -10.72451020669898902, 41.66557627198103120 ) ) ;
#118506=CARTESIAN_POINT ( 'NONE',  ( 12.06949235617739724, 12.14591786802326823, 91.87609039468568994 ) ) ;
#118508=CARTESIAN_POINT ( 'NONE',  ( 9.564922557961047289, -16.46253265017146816, 85.41775706135233293 ) ) ;
#118509=CARTESIAN_POINT ( 'NONE',  ( -4.379528057220328563, 16.55341960407611168, 60.20724293864768839 ) ) ;
#118511=CARTESIAN_POINT ( 'NONE',  ( 5.153800228976335163, 19.02544592524342804, 49.79057627198100988 ) ) ;
#118512=CARTESIAN_POINT ( 'NONE',  ( 8.224510206698953496, -14.34966873604960469, 37.91557627198102409 ) ) ;
#118513=CARTESIAN_POINT ( 'NONE',  ( 5.153800228976335163, 19.02544592524342804, 89.79057627198102409 ) ) ;
#118514=CARTESIAN_POINT ( 'NONE',  ( 13.97604488694527802, 13.89961937509977652, 59.37390960531434558 ) ) ;
#118515=CARTESIAN_POINT ( 'NONE',  ( 10.81492255796106328, -18.62759615963255655, 55.41775706135234714 ) ) ;
#118516=CARTESIAN_POINT ( 'NONE',  ( 16.51473224551069308, 9.474510206698969483, 69.16557627198102409 ) ) ;
#118517=CARTESIAN_POINT ( 'NONE',  ( -19.03943276465977164, 0.05219959533909376836, 31.24890960531435979 ) ) ;
#118519=CARTESIAN_POINT ( 'NONE',  ( -0.05219959533909027116, -19.03943276465977164, 62.49890960531435979 ) ) ;
#118520=CARTESIAN_POINT ( 'NONE',  ( -5.719274019375978568, 21.55341960407610458, 50.20724293864769550 ) ) ;
#118521=CARTESIAN_POINT ( 'NONE',  ( 9.564922557960805705, 16.46253265017160317, 29.58224293864769550 ) ) ;
#118522=CARTESIAN_POINT ( 'NONE',  ( 10.72451020669898902, -18.67979575497178502, 42.91557627198103120 ) ) ;
#118523=CARTESIAN_POINT ( 'NONE',  ( -4.483927247898782831, 16.52544592524335698, 107.7094237280190328 ) ) ;
#118524=CARTESIAN_POINT ( 'NONE',  ( -13.97604488694547697, 13.89961937509957934, 28.12609039468565797 ) ) ;
#118525=CARTESIAN_POINT ( 'NONE',  ( -12.06949235617739369, -12.14591786802326823, 49.37609039468569705 ) ) ;
#118526=CARTESIAN_POINT ( 'NONE',  ( 16.52544592524335698, 4.483927247898782831, 76.45942372801901854 ) ) ;
#118528=CARTESIAN_POINT ( 'NONE',  ( -8.224510206698735004, -14.34966873604973081, 69.58442372801900433 ) ) ;
#118529=CARTESIAN_POINT ( 'NONE',  ( 16.55341960407618274, -4.379528057220086978, 51.04275706135234714 ) ) ;
#118530=CARTESIAN_POINT ( 'NONE',  ( -19.05341960407611168, -5.049401038298163336, 106.4572429386476955 ) ) ;
#118531=CARTESIAN_POINT ( 'NONE',  ( 0.05219959533909260263, 19.03943276465977164, 29.99890960531435979 ) ) ;
#118532=CARTESIAN_POINT ( 'NONE',  ( 12.14591786802327356, -12.06949235617739191, 40.62609039468567573 ) ) ;
#118533=CARTESIAN_POINT ( 'NONE',  ( 19.02544592524343514, -5.153800228976328945, 53.54057627198102409 ) ) ;
#118534=CARTESIAN_POINT ( 'NONE',  ( -15.80617190586768217, 15.72974639402176855, 23.12609039468567573 ) ) ;
#118535=CARTESIAN_POINT ( 'NONE',  ( -8.224510206698735004, -14.34966873604973081, 39.58442372801901143 ) ) ;
#118536=CARTESIAN_POINT ( 'NONE',  ( -8.224510206698735004, -14.34966873604973081, 104.5844237280190185 ) ) ;
#118538=CARTESIAN_POINT ( 'NONE',  ( 15.72974639402176855, 15.80617190586768217, 101.8760903946857042 ) ) ;
#118539=CARTESIAN_POINT ( 'NONE',  ( -16.51473224551082808, 9.474510206698731452, 103.3344237280190043 ) ) ;
#118540=CARTESIAN_POINT ( 'NONE',  ( -16.52544592524342804, 4.483927247898546575, 56.04057627198102409 ) ) ;
#118541=CARTESIAN_POINT ( 'NONE',  ( 5.153800228976335163, 19.02544592524342804, 29.79057627198102409 ) ) ;
#118542=CARTESIAN_POINT ( 'NONE',  ( 13.97604488694548053, -13.89961937509957401, 65.62609039468567573 ) ) ;
#118543=CARTESIAN_POINT ( 'NONE',  ( 16.62475595723611121, -7.163666690055877417, 58.02713351810401576 ) ) ;
#118544=CARTESIAN_POINT ( 'NONE',  ( 10.81492255796106328, -18.62759615963255655, 70.41775706135236135 ) ) ;
#118545=CARTESIAN_POINT ( 'NONE',  ( 4.379528057220092307, 16.55341960407617563, 27.29275706135234358 ) ) ;
#118546=CARTESIAN_POINT ( 'NONE',  ( -17.72696623605163424, 5.499999999999875655, 63.59811031808420978 ) ) ;
#118547=CARTESIAN_POINT ( 'NONE',  ( 0.05219959533909260263, 19.03943276465977164, 114.9989096053143669 ) ) ;
#118548=CARTESIAN_POINT ( 'NONE',  ( 9.474510206698729675, 16.51473224551082808, 112.0844237280190043 ) ) ;
#118549=CARTESIAN_POINT ( 'NONE',  ( -19.03943276465977164, 0.05219959533909376836, 116.2489096053143669 ) ) ;
#118550=CARTESIAN_POINT ( 'NONE',  ( 13.89961937509977652, -13.97604488694527269, 23.12390960531436335 ) ) ;
#118551=CARTESIAN_POINT ( 'NONE',  ( 5.719274019375673035, 21.55341960407619339, 102.2927570613523613 ) ) ;
#118552=CARTESIAN_POINT ( 'NONE',  ( 19.02544592524343514, -5.153800228976328945, 38.54057627198103120 ) ) ;
#118554=CARTESIAN_POINT ( 'NONE',  ( 18.67979575497194134, -10.72451020669871369, 70.83442372801901854 ) ) ;
#118555=CARTESIAN_POINT ( 'NONE',  ( 0.05219959533937995610, -21.53943276465977519, 105.0010903946856757 ) ) ;
#118556=CARTESIAN_POINT ( 'NONE',  ( 4.483927247898790824, -16.52544592524335698, 100.2094237280190043 ) ) ;
#118557=CARTESIAN_POINT ( 'NONE',  ( 16.46253265017160672, -9.564922557960803928, 83.33224293864768129 ) ) ;
#118558=CARTESIAN_POINT ( 'NONE',  ( 5.719274019375673035, 21.55341960407619339, 62.29275706135236845 ) ) ;
#118559=CARTESIAN_POINT ( 'NONE',  ( 5.719274019375673035, 21.55341960407619339, 57.29275706135234714 ) ) ;
#118560=CARTESIAN_POINT ( 'NONE',  ( -16.46253265017146816, -9.564922557961047289, 74.16775706135234714 ) ) ;
#118561=CARTESIAN_POINT ( 'NONE',  ( -13.89961937509977652, 13.97604488694528158, 95.62390960531436690 ) ) ;
#118562=CARTESIAN_POINT ( 'NONE',  ( 13.97604488694527802, 13.89961937509977652, 24.37390960531435624 ) ) ;
#118563=CARTESIAN_POINT ( 'NONE',  ( 5.719274019375991003, -21.55341960407610458, 97.70724293864772392 ) ) ;
#118564=CARTESIAN_POINT ( 'NONE',  ( -0.05219959533937732626, 21.53943276465977519, 112.5010903946857042 ) ) ;
#118565=CARTESIAN_POINT ( 'NONE',  ( 12.06949235617757843, -12.14591786802309237, 103.1239096053143811 ) ) ;
#118566=CARTESIAN_POINT ( 'NONE',  ( 19.05341960407611168, 5.049401038298154454, 53.95724293864770260 ) ) ;
#118567=CARTESIAN_POINT ( 'NONE',  ( -19.03943276465977164, -0.05219959533935918106, 78.75109039468567573 ) ) ;
#118568=CARTESIAN_POINT ( 'NONE',  ( -4.483927247898539470, -16.52544592524342804, 57.29057627198103120 ) ) ;
#118569=CARTESIAN_POINT ( 'NONE',  ( 18.67979575497194134, -10.72451020669871369, 110.8344237280190043 ) ) ;
#118570=CARTESIAN_POINT ( 'NONE',  ( 0.05219959533909260263, 19.03943276465977164, 104.9989096053143669 ) ) ;
#118571=CARTESIAN_POINT ( 'NONE',  ( 19.02544592524334988, 5.153800228976608722, 76.45942372801897591 ) ) ;
#118572=CARTESIAN_POINT ( 'NONE',  ( 10.81492255796078972, 18.62759615963270932, 84.58224293864769550 ) ) ;
#118573=CARTESIAN_POINT ( 'NONE',  ( 21.55341960407619695, -5.719274019375665929, 26.04275706135235779 ) ) ;
#118574=CARTESIAN_POINT ( 'NONE',  ( -14.34966873604972548, 8.224510206698743886, 23.33442372801901499 ) ) ;
#118575=CARTESIAN_POINT ( 'NONE',  ( 14.34966873604972726, -8.224510206698740333, 95.83442372801903275 ) ) ;
#118576=CARTESIAN_POINT ( 'NONE',  ( -16.55341960407617563, 4.379528057220093196, 43.54275706135235424 ) ) ;
#118577=CARTESIAN_POINT ( 'NONE',  ( -10.81492255796105439, 18.62759615963255655, 32.91775706135234714 ) ) ;
#118578=CARTESIAN_POINT ( 'NONE',  ( 10.81492255796078972, 18.62759615963270932, 39.58224293864769550 ) ) ;
#118579=CARTESIAN_POINT ( 'NONE',  ( 16.51473224551069308, 9.474510206698969483, 34.16557627198102409 ) ) ;
#118581=CARTESIAN_POINT ( 'NONE',  ( 14.29746914071037800, 8.314922557961029526, 56.66775706135235424 ) ) ;
#118582=CARTESIAN_POINT ( 'NONE',  ( -16.52544592524342804, 4.483927247898546575, 91.04057627198103830 ) ) ;
#118583=CARTESIAN_POINT ( 'NONE',  ( 21.53943276465977519, -0.05219959533907433946, 88.74890960531436690 ) ) ;
#118584=CARTESIAN_POINT ( 'NONE',  ( -16.55341960407611168, -4.379528057220339221, 26.45724293864768839 ) ) ;
#118585=CARTESIAN_POINT ( 'NONE',  ( -8.314922557961024197, 14.29746914071037800, 42.91775706135235424 ) ) ;
#118586=CARTESIAN_POINT ( 'NONE',  ( 19.02544592524343514, -5.153800228976328945, 53.54057627198102409 ) ) ;
#118587=CARTESIAN_POINT ( 'NONE',  ( -12.14591786802326823, 12.06949235617739902, 88.12609039468570415 ) ) ;
#118588=CARTESIAN_POINT ( 'NONE',  ( 0.05219959533936267826, -19.03943276465977164, 90.00109039468567573 ) ) ;
#118589=CARTESIAN_POINT ( 'NONE',  ( -21.53943276465977519, 0.05219959533907696930, 86.24890960531436690 ) ) ;
#118590=CARTESIAN_POINT ( 'NONE',  ( 12.06949235617739724, 12.14591786802326823, 106.8760903946856899 ) ) ;
#118591=ORIENTED_EDGE ( 'NONE', *, *, #131511, .T. ) ;
#118592=FACE_OUTER_BOUND ( 'NONE', #189074, .T. ) ;
#118593=EDGE_CURVE ( 'NONE', #91492, #147765, #165309, .T. ) ;
#118594=CARTESIAN_POINT ( 'NONE',  ( -10.81492255796078084, -18.62759615963271287, 67.08224293864770971 ) ) ;
#118595=CARTESIAN_POINT ( 'NONE',  ( -0.05219959533934338120, 16.53943276465976808, 97.50109039468567573 ) ) ;
#118597=CARTESIAN_POINT ( 'NONE',  ( -15.72974639402197994, 15.80617190586746368, 25.62390960531435624 ) ) ;
#118599=CARTESIAN_POINT ( 'NONE',  ( -15.80617190586745835, -15.72974639402198527, 81.87390960531435269 ) ) ;
#118600=CARTESIAN_POINT ( 'NONE',  ( 12.14591786802309770, 12.06949235617756955, 29.37390960531435269 ) ) ;
#118601=CARTESIAN_POINT ( 'NONE',  ( 8.224510206698742110, 14.34966873604972548, 32.08442372801901854 ) ) ;
#118602=CARTESIAN_POINT ( 'NONE',  ( -9.564922557960796823, -16.46253265017161027, 37.08224293864768839 ) ) ;
#118603=CARTESIAN_POINT ( 'NONE',  ( 14.34966873604972726, -8.224510206698740333, 25.83442372801901499 ) ) ;
#118604=CARTESIAN_POINT ( 'NONE',  ( -19.02544592524342804, 5.153800228976336051, 51.04057627198103120 ) ) ;
#118606=CARTESIAN_POINT ( 'NONE',  ( 5.049401038298161559, -19.05341960407611168, 107.7072429386476955 ) ) ;
#118607=CARTESIAN_POINT ( 'NONE',  ( 18.22780087662121673, 5.500000000000056843, 78.98459894673892734 ) ) ;
#118608=CARTESIAN_POINT ( 'NONE',  ( -14.29746914071037622, -8.314922557961029526, 104.1677570613523471 ) ) ;
#118609=CARTESIAN_POINT ( 'NONE',  ( -5.049401038297874678, -19.05341960407617918, 89.79275706135230450 ) ) ;
#118610=CARTESIAN_POINT ( 'NONE',  ( 9.564922557961047289, -16.46253265017146816, 35.41775706135233293 ) ) ;
#118611=CARTESIAN_POINT ( 'NONE',  ( -18.62759615963270932, 10.81492255796079327, 75.83224293864769550 ) ) ;
#118612=CARTESIAN_POINT ( 'NONE',  ( 16.55341960407618274, -4.379528057220086978, 106.0427570613523471 ) ) ;
#118613=CARTESIAN_POINT ( 'NONE',  ( 21.52544592524344225, -5.823673210054117533, 38.54057627198103120 ) ) ;
#118614=CARTESIAN_POINT ( 'NONE',  ( 9.474510206698729675, 16.51473224551082808, 102.0844237280190043 ) ) ;
#118615=CARTESIAN_POINT ( 'NONE',  ( 0.05219959533909260263, 19.03943276465977164, 104.9989096053143669 ) ) ;
#118616=CARTESIAN_POINT ( 'NONE',  ( 21.55341960407619695, -5.719274019375665929, 61.04275706135234714 ) ) ;
#118617=CARTESIAN_POINT ( 'NONE',  ( 5.049401038298161559, -19.05341960407611168, 62.70724293864769550 ) ) ;
#118618=CARTESIAN_POINT ( 'NONE',  ( 4.379528057220339221, -16.55341960407611168, 102.7072429386476955 ) ) ;
#118620=CARTESIAN_POINT ( 'NONE',  ( -12.14591786802309592, -12.06949235617757132, 71.87390960531438111 ) ) ;
#118622=CARTESIAN_POINT ( 'NONE',  ( 19.02544592524334988, 5.153800228976608722, 86.45942372801900433 ) ) ;
#118623=CARTESIAN_POINT ( 'NONE',  ( 19.19724070472096855, 5.500000000000033751, 93.56193348274381094 ) ) ;
#118624=CARTESIAN_POINT ( 'NONE',  ( -19.05341960407611168, -5.049401038298163336, 61.45724293864769550 ) ) ;
#118625=CARTESIAN_POINT ( 'NONE',  ( 16.18388926212248435, -7.379444403734418678, 72.06046848633769741 ) ) ;
#118626=CARTESIAN_POINT ( 'NONE',  ( 13.89961937509977652, -13.97604488694527269, 73.12390960531436690 ) ) ;
#118627=CARTESIAN_POINT ( 'NONE',  ( -16.51473224551069308, -9.474510206698971260, 91.66557627198103830 ) ) ;
#118628=CARTESIAN_POINT ( 'NONE',  ( 4.483927247898790824, -16.52544592524335698, 70.20942372801904696 ) ) ;
#118629=CARTESIAN_POINT ( 'NONE',  ( -17.44279575226822132, -5.990770900252485376, 49.16442432485681024 ) ) ;
#118630=CARTESIAN_POINT ( 'NONE',  ( 16.51473224551083163, -9.474510206698727899, 40.83442372801900433 ) ) ;
#118632=CARTESIAN_POINT ( 'NONE',  ( 19.05341960407611168, 5.049401038298154454, 108.9572429386477097 ) ) ;
#118633=CARTESIAN_POINT ( 'NONE',  ( 12.14591786802327356, -12.06949235617739191, 105.6260903946856899 ) ) ;
#118634=CARTESIAN_POINT ( 'NONE',  ( 12.14591786802327356, -12.06949235617739191, 95.62609039468568994 ) ) ;
#118635=CARTESIAN_POINT ( 'NONE',  ( -17.26058549869089020, 6.457015423128606102, 28.62254162523932521 ) ) ;
#118636=CARTESIAN_POINT ( 'NONE',  ( 16.55341960407618274, -4.379528057220086978, 66.04275706135236135 ) ) ;
#118638=CARTESIAN_POINT ( 'NONE',  ( -18.67979575497193778, 10.72451020669871902, 68.33442372801900433 ) ) ;
#118639=CARTESIAN_POINT ( 'NONE',  ( 13.97604488694548053, -13.89961937509957401, 85.62609039468568994 ) ) ;
#118640=CARTESIAN_POINT ( 'NONE',  ( 9.474510206698729675, 16.51473224551082808, 32.08442372801900433 ) ) ;
#118641=CARTESIAN_POINT ( 'NONE',  ( -9.474510206698964154, 16.51473224551069663, 60.41557627198102409 ) ) ;
#118642=CARTESIAN_POINT ( 'NONE',  ( -0.05219959533909027116, -19.03943276465977164, 42.49890960531435269 ) ) ;
#118643=CARTESIAN_POINT ( 'NONE',  ( 16.51128444969438291, 7.226502650581850595, 22.09735981835456542 ) ) ;
#118644=CARTESIAN_POINT ( 'NONE',  ( -0.05219959533907301413, -21.53943276465977519, 87.49890960531436690 ) ) ;
#118646=CARTESIAN_POINT ( 'NONE',  ( -10.81492255796078084, -18.62759615963271287, 32.08224293864769550 ) ) ;
#118647=CARTESIAN_POINT ( 'NONE',  ( -16.46253265017160317, 9.564922557960807481, 30.83224293864769550 ) ) ;
#118648=CARTESIAN_POINT ( 'NONE',  ( 4.483927247898790824, -16.52544592524335698, 55.20942372801902565 ) ) ;
#118650=CARTESIAN_POINT ( 'NONE',  ( 15.80617190586769283, -15.72974639402175789, 25.62609039468567929 ) ) ;
#118651=CARTESIAN_POINT ( 'NONE',  ( 16.52544592524342804, -4.483927247898539470, 53.54057627198103120 ) ) ;
#118653=CARTESIAN_POINT ( 'NONE',  ( -16.55341960407617563, 4.379528057220093196, 23.54275706135235424 ) ) ;
#118654=CARTESIAN_POINT ( 'NONE',  ( 9.564922557961047289, -16.46253265017146816, 40.41775706135234003 ) ) ;
#118655=CARTESIAN_POINT ( 'NONE',  ( 16.52544592524342804, -4.483927247898539470, 53.54057627198103120 ) ) ;
#118656=CARTESIAN_POINT ( 'NONE',  ( 18.62759615963271287, -10.81492255796078972, 113.3322429386476955 ) ) ;
#118658=CARTESIAN_POINT ( 'NONE',  ( 18.67979575497178502, 10.72451020669898547, 74.16557627198102409 ) ) ;
#118659=CARTESIAN_POINT ( 'NONE',  ( -9.564922557960796823, -16.46253265017161027, 92.08224293864769550 ) ) ;
#118660=CARTESIAN_POINT ( 'NONE',  ( -4.483927247898539470, -16.52544592524342804, 62.29057627198102409 ) ) ;
#118661=CARTESIAN_POINT ( 'NONE',  ( 5.049401038298161559, -19.05341960407611168, 102.7072429386476955 ) ) ;
#118663=CARTESIAN_POINT ( 'NONE',  ( 9.474510206698729675, 16.51473224551082808, 67.08442372801900433 ) ) ;
#118664=CARTESIAN_POINT ( 'NONE',  ( -10.72451020669898014, 18.67979575497178502, 110.4155762719810383 ) ) ;
#118665=CARTESIAN_POINT ( 'NONE',  ( -0.05219959533909027116, -19.03943276465977164, 62.49890960531435979 ) ) ;
#118666=CARTESIAN_POINT ( 'NONE',  ( -5.153800228976607833, 19.02544592524334988, 47.70942372801900433 ) ) ;
#118667=CARTESIAN_POINT ( 'NONE',  ( 14.29746914071049879, -8.314922557960816363, 108.3322429386477097 ) ) ;
#118668=CARTESIAN_POINT ( 'NONE',  ( 21.55341960407619695, -5.719274019375665929, 61.04275706135234714 ) ) ;
#118670=CARTESIAN_POINT ( 'NONE',  ( -16.29526858892877073, -7.335722546920126597, 70.79670597800213727 ) ) ;
#118671=CARTESIAN_POINT ( 'NONE',  ( -8.224510206698948167, 14.34966873604960824, 45.41557627198103830 ) ) ;
#118672=CARTESIAN_POINT ( 'NONE',  ( 16.46253265017160672, -9.564922557960803928, 53.33224293864768839 ) ) ;
#118673=CARTESIAN_POINT ( 'NONE',  ( -0.05219959533907301413, -21.53943276465977519, 77.49890960531433848 ) ) ;
#118675=CARTESIAN_POINT ( 'NONE',  ( 9.474510206698971260, -16.51473224551069308, 47.91557627198102409 ) ) ;
#118676=CARTESIAN_POINT ( 'NONE',  ( -10.72451020669898014, 18.67979575497178502, 70.41557627198102409 ) ) ;
#118677=CARTESIAN_POINT ( 'NONE',  ( -5.719274019375665041, -21.55341960407619695, 104.7927570613523898 ) ) ;
#118678=CARTESIAN_POINT ( 'NONE',  ( 18.09918380851993192, 5.500000000000036415, 53.98618307335611632 ) ) ;
#118679=CARTESIAN_POINT ( 'NONE',  ( -12.06949235617739369, -12.14591786802326823, 94.37609039468568994 ) ) ;
#118680=CARTESIAN_POINT ( 'NONE',  ( 8.314922557960818139, 14.29746914071049879, 89.58224293864768129 ) ) ;
#118681=CARTESIAN_POINT ( 'NONE',  ( 19.05341960407611168, 5.049401038298154454, 73.95724293864768129 ) ) ;
#118683=CARTESIAN_POINT ( 'NONE',  ( -16.51473224551082808, 9.474510206698731452, 33.33442372801899722 ) ) ;
#118684=CARTESIAN_POINT ( 'NONE',  ( 4.379528057220092307, 16.55341960407617563, 87.29275706135236135 ) ) ;
#118685=CARTESIAN_POINT ( 'NONE',  ( 13.89961937509957401, 13.97604488694547697, 26.87609039468566507 ) ) ;
#118686=CARTESIAN_POINT ( 'NONE',  ( 13.97604488694527802, 13.89961937509977652, 89.37390960531436690 ) ) ;
#118687=CARTESIAN_POINT ( 'NONE',  ( -10.81492255796078084, -18.62759615963271287, 52.08224293864768839 ) ) ;
#118689=CARTESIAN_POINT ( 'NONE',  ( -13.89961937509977652, 13.97604488694528158, 25.62390960531434558 ) ) ;
#118690=CARTESIAN_POINT ( 'NONE',  ( -15.72974639402176322, -15.80617190586768395, 89.37609039468568994 ) ) ;
#118691=CARTESIAN_POINT ( 'NONE',  ( 8.314922557961029526, -14.29746914071037800, 60.41775706135235424 ) ) ;
#118692=CARTESIAN_POINT ( 'NONE',  ( 18.62759615963255655, 10.81492255796105972, 21.66775706135235069 ) ) ;
#118693=CARTESIAN_POINT ( 'NONE',  ( 16.55341960407618274, -4.379528057220086978, 31.04275706135234714 ) ) ;
#118694=CARTESIAN_POINT ( 'NONE',  ( 16.51473224551069308, 9.474510206698969483, 94.16557627198103830 ) ) ;
#118695=CARTESIAN_POINT ( 'NONE',  ( 5.153800228976335163, 19.02544592524342804, 39.79057627198100988 ) ) ;
#118696=CARTESIAN_POINT ( 'NONE',  ( 19.05341960407611168, 5.049401038298154454, 58.95724293864768129 ) ) ;
#118698=CARTESIAN_POINT ( 'NONE',  ( 16.55341960407618274, -4.379528057220086978, 31.04275706135234714 ) ) ;
#118699=CARTESIAN_POINT ( 'NONE',  ( 12.06949235617757843, -12.14591786802309237, 98.12390960531436690 ) ) ;
#118700=CARTESIAN_POINT ( 'NONE',  ( -0.05219959533934338120, 16.53943276465976808, 97.50109039468567573 ) ) ;
#118701=CARTESIAN_POINT ( 'NONE',  ( -21.53943276465977519, -0.05219959533937600094, 43.75109039468568284 ) ) ;
#118702=CARTESIAN_POINT ( 'NONE',  ( 16.51473224551069308, 9.474510206698969483, 69.16557627198102409 ) ) ;
#118703=CARTESIAN_POINT ( 'NONE',  ( -0.05219959533909027116, -19.03943276465977164, 52.49890960531436690 ) ) ;
#118704=CARTESIAN_POINT ( 'NONE',  ( -19.02544592524342804, 5.153800228976336051, 81.04057627198103830 ) ) ;
#118705=CARTESIAN_POINT ( 'NONE',  ( 14.29746914071049879, -8.314922557960816363, 38.33224293864768839 ) ) ;
#118706=CARTESIAN_POINT ( 'NONE',  ( -14.34966873604972548, 8.224510206698743886, 103.3344237280190043 ) ) ;
#118707=ORIENTED_EDGE ( 'NONE', *, *, #195934, .T. ) ;
#118708=CARTESIAN_POINT ( 'NONE',  ( 9.474510206698729675, 16.51473224551082808, 47.08442372801900433 ) ) ;
#118709=CARTESIAN_POINT ( 'NONE',  ( -16.46253265017160317, 9.564922557960807481, 110.8322429386476955 ) ) ;
#118710=CARTESIAN_POINT ( 'NONE',  ( 16.46253265017160672, -9.564922557960803928, 43.33224293864769550 ) ) ;
#118711=CARTESIAN_POINT ( 'NONE',  ( 9.474510206698729675, 16.51473224551082808, 32.08442372801900433 ) ) ;
#118713=CARTESIAN_POINT ( 'NONE',  ( 8.314922557961029526, -14.29746914071037800, 45.41775706135234003 ) ) ;
#118715=CARTESIAN_POINT ( 'NONE',  ( -19.02544592524334988, -5.153800228976617603, 68.95942372801896170 ) ) ;
#118716=CARTESIAN_POINT ( 'NONE',  ( 12.06949235617739724, 12.14591786802326823, 56.87609039468568994 ) ) ;
#118718=CARTESIAN_POINT ( 'NONE',  ( 0.05219959533909260263, 19.03943276465977164, 74.99890960531435269 ) ) ;
#118719=CARTESIAN_POINT ( 'NONE',  ( -18.62759615963270932, 10.81492255796079327, 115.8322429386477097 ) ) ;
#118720=CARTESIAN_POINT ( 'NONE',  ( 5.049401038297881783, 19.05341960407617563, 67.29275706135234714 ) ) ;
#118721=CARTESIAN_POINT ( 'NONE',  ( 9.564922557960805705, 16.46253265017160317, 109.5822429386476955 ) ) ;
#118722=CARTESIAN_POINT ( 'NONE',  ( 13.89961937509977652, -13.97604488694527269, 38.12390960531436690 ) ) ;
#118723=EDGE_CURVE ( 'NONE', #178804, #67326, #182121, .T. ) ;
#118724=CARTESIAN_POINT ( 'NONE',  ( 13.97604488694527802, 13.89961937509977652, 79.37390960531435269 ) ) ;
#118725=CARTESIAN_POINT ( 'NONE',  ( 12.06949235617757843, -12.14591786802309237, 28.12390960531435979 ) ) ;
#118726=CARTESIAN_POINT ( 'NONE',  ( 16.51473224551069308, 9.474510206698969483, 34.16557627198102409 ) ) ;
#118727=CARTESIAN_POINT ( 'NONE',  ( -5.153800228976607833, 19.02544592524334988, 57.70942372801899012 ) ) ;
#118728=CARTESIAN_POINT ( 'NONE',  ( -16.55341960407611168, -4.379528057220339221, 76.45724293864769550 ) ) ;
#118729=CARTESIAN_POINT ( 'NONE',  ( -5.823673210054431948, 21.52544592524334988, 112.7094237280190328 ) ) ;
#118730=CARTESIAN_POINT ( 'NONE',  ( -19.05341960407611168, -5.049401038298163336, 51.45724293864770260 ) ) ;
#118731=CARTESIAN_POINT ( 'NONE',  ( 0.05219959533907565091, 21.53943276465977519, 44.99890960531435979 ) ) ;
#118732=CARTESIAN_POINT ( 'NONE',  ( -14.29746914071049879, 8.314922557960819915, 50.83224293864770971 ) ) ;
#118733=CARTESIAN_POINT ( 'NONE',  ( -0.05219959533937732626, 21.53943276465977519, 107.5010903946856899 ) ) ;
#118734=CARTESIAN_POINT ( 'NONE',  ( -19.02544592524342804, 5.153800228976336051, 91.04057627198100988 ) ) ;
#118735=CARTESIAN_POINT ( 'NONE',  ( -9.474510206698964154, 16.51473224551069663, 105.4155762719810383 ) ) ;
#118736=CARTESIAN_POINT ( 'NONE',  ( 19.02544592524343514, -5.153800228976328945, 33.54057627198102409 ) ) ;
#118737=CARTESIAN_POINT ( 'NONE',  ( -9.564922557960796823, -16.46253265017161027, 32.08224293864769550 ) ) ;
#118738=CARTESIAN_POINT ( 'NONE',  ( 14.34966873604960469, 8.224510206698951720, 89.16557627198102409 ) ) ;
#118739=CARTESIAN_POINT ( 'NONE',  ( 18.67979575497178502, 10.72451020669898547, 99.16557627198100988 ) ) ;
#118740=CARTESIAN_POINT ( 'NONE',  ( -9.564922557960796823, -16.46253265017161027, 87.08224293864769550 ) ) ;
#118741=CARTESIAN_POINT ( 'NONE',  ( -5.719274019375978568, 21.55341960407610458, 110.2072429386477239 ) ) ;
#118742=CARTESIAN_POINT ( 'NONE',  ( -19.03943276465977164, 0.05219959533909376836, 86.24890960531436690 ) ) ;
#118744=CARTESIAN_POINT ( 'NONE',  ( -12.14591786802309592, -12.06949235617757132, 96.87390960531436690 ) ) ;
#118745=CARTESIAN_POINT ( 'NONE',  ( -5.049401038298153566, 19.05341960407611168, 75.20724293864769550 ) ) ;
#118746=CARTESIAN_POINT ( 'NONE',  ( -0.05219959533907301413, -21.53943276465977519, 82.49890960531436690 ) ) ;
#118749=CARTESIAN_POINT ( 'NONE',  ( 15.72974639402199770, -15.80617190586745480, 23.12390960531436335 ) ) ;
#118750=CARTESIAN_POINT ( 'NONE',  ( 18.39443945427639804, -5.500000000000021316, 66.01745347608652992 ) ) ;
#118751=CARTESIAN_POINT ( 'NONE',  ( -0.05219959533934338120, 16.53943276465976808, 32.50109039468568284 ) ) ;
#118752=CARTESIAN_POINT ( 'NONE',  ( 16.53943276465976808, -0.05219959533910856209, 93.74890960531436690 ) ) ;
#118753=CARTESIAN_POINT ( 'NONE',  ( -17.05587630539785238, -6.762274262135695935, 94.25819690962687503 ) ) ;
#118754=CARTESIAN_POINT ( 'NONE',  ( 13.89961937509977652, -13.97604488694527269, 93.12390960531436690 ) ) ;
#118755=CARTESIAN_POINT ( 'NONE',  ( -19.05341960407611168, -5.049401038298163336, 41.45724293864769550 ) ) ;
#118756=CARTESIAN_POINT ( 'NONE',  ( -12.06949235617756955, 12.14591786802309770, 85.62390960531436690 ) ) ;
#118757=CARTESIAN_POINT ( 'NONE',  ( 5.823673210054125526, 21.52544592524343514, 29.79057627198102409 ) ) ;
#118758=CARTESIAN_POINT ( 'NONE',  ( -8.224510206698948167, 14.34966873604960824, 50.41557627198103120 ) ) ;
#118759=CARTESIAN_POINT ( 'NONE',  ( -13.97604488694547697, 13.89961937509957934, 98.12609039468566152 ) ) ;
#118760=CARTESIAN_POINT ( 'NONE',  ( 15.72974639402176855, 15.80617190586768217, 61.87609039468568284 ) ) ;
#118762=CARTESIAN_POINT ( 'NONE',  ( -19.02544592524342804, 5.153800228976336051, 96.04057627198103830 ) ) ;
#118763=CARTESIAN_POINT ( 'NONE',  ( 4.483927247898790824, -16.52544592524335698, 90.20942372801903275 ) ) ;
#118764=CARTESIAN_POINT ( 'NONE',  ( -13.89961937509977652, 13.97604488694528158, 30.62390960531435269 ) ) ;
#118765=CARTESIAN_POINT ( 'NONE',  ( 13.89961937509977652, -13.97604488694527269, 78.12390960531433848 ) ) ;
#118766=CARTESIAN_POINT ( 'NONE',  ( -21.52544592524343514, 5.823673210054127303, 76.04057627198102409 ) ) ;
#118767=CARTESIAN_POINT ( 'NONE',  ( 12.06949235617739724, 12.14591786802326823, 21.87609039468567573 ) ) ;
#118768=CARTESIAN_POINT ( 'NONE',  ( 12.14591786802309770, 12.06949235617756955, 54.37390960531435979 ) ) ;
#118769=CARTESIAN_POINT ( 'NONE',  ( -21.52544592524334988, -5.823673210054445271, 63.95942372801901854 ) ) ;
#118770=B_SPLINE_CURVE_WITH_KNOTS ( 'NONE', 3,
 ( #41784, #183275, #135786, #75088, #13424, #134798, #136755, #198440, #106411, #150960, #59912, #60899, #56951, #30577, #92228, #118625, #120591, #58923, #72109, #165129, #168092, #121580, #57949, #26621, #122574, #180316, #182286, #29590, #149952, #88264, #197457, #11457 ),
 .UNSPECIFIED., .F., .F.,
 ( 4, 2, 2, 2, 2, 2, 2, 2, 2, 2, 2, 2, 2, 2, 2, 4 ),
 ( 1.644815183373819107E-15, 0.0003712461730052133888, 0.0007424923460087820429, 0.001113738519012350426, 0.001484984692015919134, 0.002227477038023074982, 0.002598723211026649979, 0.002969969384030225409, 0.003341215557033800406, 0.003712461730037375836, 0.004083707903040949966, 0.004454954076044525396, 0.004826200249048100827, 0.005197446422051676257, 0.005568692595055250820, 0.005939938768058826250 ),
 .UNSPECIFIED. ) ;
#118771=CARTESIAN_POINT ( 'NONE',  ( 12.06949235617739724, 12.14591786802326823, 81.87609039468568994 ) ) ;
#118772=CARTESIAN_POINT ( 'NONE',  ( 21.55341960407610458, 5.719274019375980345, 23.95724293864769550 ) ) ;
#118774=CARTESIAN_POINT ( 'NONE',  ( -17.31728774477273447, 6.344390552232389346, 80.81906651689321563 ) ) ;
#118775=CARTESIAN_POINT ( 'NONE',  ( 14.29746914071037800, 8.314922557961029526, 106.6677570613523756 ) ) ;
#118776=CARTESIAN_POINT ( 'NONE',  ( 14.29746914071037800, 8.314922557961029526, 61.66775706135235424 ) ) ;
#118777=CARTESIAN_POINT ( 'NONE',  ( 5.049401038298161559, -19.05341960407611168, 77.70724293864765286 ) ) ;
#118778=CARTESIAN_POINT ( 'NONE',  ( 5.049401038298161559, -19.05341960407611168, 87.70724293864769550 ) ) ;
#118779=CARTESIAN_POINT ( 'NONE',  ( 15.72974639402176855, 15.80617190586768217, 76.87609039468567573 ) ) ;
#118780=CARTESIAN_POINT ( 'NONE',  ( 12.14591786802327356, -12.06949235617739191, 70.62609039468567573 ) ) ;
#118781=CARTESIAN_POINT ( 'NONE',  ( -4.379528057220328563, 16.55341960407611168, 40.20724293864769550 ) ) ;
#118782=CARTESIAN_POINT ( 'NONE',  ( 19.02544592524343514, -5.153800228976328945, 58.54057627198102409 ) ) ;
#118783=CARTESIAN_POINT ( 'NONE',  ( -16.51473224551069308, -9.474510206698971260, 41.66557627198103120 ) ) ;
#118784=CARTESIAN_POINT ( 'NONE',  ( -16.52544592524335698, -4.483927247898792601, 38.95942372801901854 ) ) ;
#118786=CARTESIAN_POINT ( 'NONE',  ( -16.51473224551082808, 9.474510206698731452, 98.33442372801900433 ) ) ;
#118787=CARTESIAN_POINT ( 'NONE',  ( -0.05219959533910754901, -16.53943276465976808, 92.49890960531436690 ) ) ;
#118788=CARTESIAN_POINT ( 'NONE',  ( 19.03943276465977164, -0.05219959533909143690, 58.74890960531435979 ) ) ;
#118789=CARTESIAN_POINT ( 'NONE',  ( 5.153800228976615827, -19.02544592524334988, 105.2094237280190185 ) ) ;
#118791=CARTESIAN_POINT ( 'NONE',  ( 5.719274019375673035, 21.55341960407619339, 107.2927570613523471 ) ) ;
#118792=CARTESIAN_POINT ( 'NONE',  ( -14.29746914071037622, -8.314922557961029526, 64.16775706135234714 ) ) ;
#118794=CARTESIAN_POINT ( 'NONE',  ( 21.55341960407610458, 5.719274019375980345, 58.95724293864770971 ) ) ;
#118795=CARTESIAN_POINT ( 'NONE',  ( -12.06949235617739369, -12.14591786802326823, 59.37609039468568284 ) ) ;
#118797=CARTESIAN_POINT ( 'NONE',  ( 9.474510206698729675, 16.51473224551082808, 52.08442372801900433 ) ) ;
#118798=CARTESIAN_POINT ( 'NONE',  ( -16.46253265017160317, 9.564922557960807481, 85.83224293864769550 ) ) ;
#118799=CARTESIAN_POINT ( 'NONE',  ( -8.224510206698948167, 14.34966873604960824, 110.4155762719810383 ) ) ;
#118800=CARTESIAN_POINT ( 'NONE',  ( -19.03943276465977164, 0.05219959533909376836, 61.24890960531436690 ) ) ;
#118801=CARTESIAN_POINT ( 'NONE',  ( 16.55341960407611168, 4.379528057220329451, 53.95724293864770260 ) ) ;
#118803=CARTESIAN_POINT ( 'NONE',  ( 10.81492255796106328, -18.62759615963255655, 80.41775706135234714 ) ) ;
#118804=ADVANCED_FACE ( 'NONE', ( #51252 ), #6562, .T. ) ;
#118805=CARTESIAN_POINT ( 'NONE',  ( -19.05341960407617563, 5.049401038297882671, 53.54275706135231871 ) ) ;
#118806=CARTESIAN_POINT ( 'NONE',  ( -19.03943276465977164, -0.05219959533935918106, 28.75109039468566507 ) ) ;
#118807=CARTESIAN_POINT ( 'NONE',  ( -21.55341960407610458, -5.719274019375992779, 21.45724293864769550 ) ) ;
#118808=CARTESIAN_POINT ( 'NONE',  ( 21.53943276465977519, 0.05219959533937863772, 96.25109039468568994 ) ) ;
#118809=CARTESIAN_POINT ( 'NONE',  ( 16.51473224551069308, 9.474510206698969483, 59.16557627198102409 ) ) ;
#118810=CARTESIAN_POINT ( 'NONE',  ( 15.72974639402176855, 15.80617190586768217, 96.87609039468568994 ) ) ;
#118811=CARTESIAN_POINT ( 'NONE',  ( -15.72974639402197994, 15.80617190586746368, 45.62390960531436690 ) ) ;
#118812=CARTESIAN_POINT ( 'NONE',  ( -19.05341960407611168, -5.049401038298163336, 86.45724293864769550 ) ) ;
#118813=CARTESIAN_POINT ( 'NONE',  ( 13.89961937509957401, 13.97604488694547697, 61.87609039468566863 ) ) ;
#118814=CARTESIAN_POINT ( 'NONE',  ( -19.05341960407611168, -5.049401038298163336, 36.45724293864766707 ) ) ;
#118815=CARTESIAN_POINT ( 'NONE',  ( -16.46253265017160317, 9.564922557960807481, 90.83224293864769550 ) ) ;
#118816=CARTESIAN_POINT ( 'NONE',  ( -16.46253265017146816, -9.564922557961047289, 89.16775706135234714 ) ) ;
#118817=CARTESIAN_POINT ( 'NONE',  ( 8.224510206698742110, 14.34966873604972548, 47.08442372801901854 ) ) ;
#118818=CARTESIAN_POINT ( 'NONE',  ( -0.05219959533910754901, -16.53943276465976808, 97.49890960531436690 ) ) ;
#118819=CARTESIAN_POINT ( 'NONE',  ( -9.474510206698964154, 16.51473224551069663, 75.41557627198103830 ) ) ;
#118821=CARTESIAN_POINT ( 'NONE',  ( 10.72451020669898902, -18.67979575497178502, 52.91557627198103830 ) ) ;
#118822=CARTESIAN_POINT ( 'NONE',  ( -19.05341960407617563, 5.049401038297882671, 108.5427570613523187 ) ) ;
#118823=CARTESIAN_POINT ( 'NONE',  ( 15.80617190586746368, 15.72974639402197994, 114.3739096053143527 ) ) ;
#118824=CARTESIAN_POINT ( 'NONE',  ( 10.72451020669871369, 18.67979575497193778, 67.08442372801901854 ) ) ;
#118825=CARTESIAN_POINT ( 'NONE',  ( 16.53943276465976808, 0.05219959533934440121, 76.25109039468568994 ) ) ;
#118826=( BOUNDED_CURVE ( )  B_SPLINE_CURVE ( 2, ( #102104, #163789, #160779, #53598, #25290, #41439, #82922, #22268, #83918, #23272, #145600, #7079, #38437 ),
 .UNSPECIFIED., .F., .T. ) 
 B_SPLINE_CURVE_WITH_KNOTS ( ( 3, 2, 2, 2, 2, 2, 3 ),
 ( 0.4498445373017669335, 0.4517543859649122973, 0.4561403508771929571, 0.4605263157894736725, 0.4649122807017543879, 0.4692982456140351033, 0.4712537740992707724 ),
 .UNSPECIFIED. ) 
 CURVE ( )  GEOMETRIC_REPRESENTATION_ITEM ( )  RATIONAL_B_SPLINE_CURVE ( ( 0.9832469066685285419, 0.9851625545550100060, 1.000000000000000000, 0.9659258262890683122, 1.000000000000000000, 0.9659258262890683122, 1.000000000000000000, 0.9659258262890683122, 1.000000000000000000, 0.9659258262890683122, 1.000000000000000000, 0.9848076720550081875, 0.9831626618144004848 ) ) 
 REPRESENTATION_ITEM ( '' )  );
#118827=CARTESIAN_POINT ( 'NONE',  ( -16.51473224551069308, -9.474510206698971260, 71.66557627198102409 ) ) ;
#118828=CARTESIAN_POINT ( 'NONE',  ( -16.52544592524335698, -4.483927247898792601, 103.9594237280190185 ) ) ;
#118829=CARTESIAN_POINT ( 'NONE',  ( -0.05219959533936034679, 19.03943276465977164, 42.50109039468566152 ) ) ;
#118831=CARTESIAN_POINT ( 'NONE',  ( -15.80617190586768217, 15.72974639402176855, 33.12609039468569705 ) ) ;
#118832=CARTESIAN_POINT ( 'NONE',  ( -12.14591786802309592, -12.06949235617757132, 76.87390960531439532 ) ) ;
#118833=CARTESIAN_POINT ( 'NONE',  ( -19.05341960407611168, -5.049401038298163336, 96.45724293864769550 ) ) ;
#118834=CARTESIAN_POINT ( 'NONE',  ( -4.483927247898782831, 16.52544592524335698, 92.70942372801901854 ) ) ;
#118835=CARTESIAN_POINT ( 'NONE',  ( -18.67979575497193778, 10.72451020669871902, 68.33442372801900433 ) ) ;
#118836=CARTESIAN_POINT ( 'NONE',  ( -4.483927247898782831, 16.52544592524335698, 27.70942372801901854 ) ) ;
#118837=CARTESIAN_POINT ( 'NONE',  ( -21.55341960407619339, 5.719274019375674811, 28.54275706135234358 ) ) ;
#118838=CARTESIAN_POINT ( 'NONE',  ( -16.53943276465976808, 0.05219959533911058130, 71.24890960531435269 ) ) ;
#118840=CARTESIAN_POINT ( 'NONE',  ( 18.67979575497178502, 10.72451020669898547, 99.16557627198100988 ) ) ;
#118841=CARTESIAN_POINT ( 'NONE',  ( -4.379528057220328563, 16.55341960407611168, 50.20724293864769550 ) ) ;
#118843=CARTESIAN_POINT ( 'NONE',  ( -9.564922557960796823, -16.46253265017161027, 27.08224293864769550 ) ) ;
#118844=CARTESIAN_POINT ( 'NONE',  ( -15.80617190586745835, -15.72974639402198527, 31.87390960531435979 ) ) ;
#118845=CARTESIAN_POINT ( 'NONE',  ( -0.05219959533937732626, 21.53943276465977519, 42.50109039468567573 ) ) ;
#118846=CARTESIAN_POINT ( 'NONE',  ( 16.55341960407611168, 4.379528057220329451, 63.95724293864770260 ) ) ;
#118847=CARTESIAN_POINT ( 'NONE',  ( -15.80617190586745835, -15.72974639402198527, 66.87390960531436690 ) ) ;
#118848=CARTESIAN_POINT ( 'NONE',  ( 13.97604488694527802, 13.89961937509977652, 74.37390960531436690 ) ) ;
#118849=CARTESIAN_POINT ( 'NONE',  ( -16.51473224551069308, -9.474510206698971260, 31.66557627198102054 ) ) ;
#118850=CARTESIAN_POINT ( 'NONE',  ( 13.97604488694548053, -13.89961937509957401, 80.62609039468567573 ) ) ;
#118851=CARTESIAN_POINT ( 'NONE',  ( -15.80617190586745835, -15.72974639402198527, 61.87390960531436690 ) ) ;
#118852=CARTESIAN_POINT ( 'NONE',  ( -19.03943276465977164, 0.05219959533909376836, 36.24890960531436690 ) ) ;
#118853=CARTESIAN_POINT ( 'NONE',  ( 5.153800228976335163, 19.02544592524342804, 69.79057627198103830 ) ) ;
#118855=CARTESIAN_POINT ( 'NONE',  ( -4.483927247898782831, 16.52544592524335698, 32.70942372801900433 ) ) ;
#118856=CARTESIAN_POINT ( 'NONE',  ( 21.55341960407619695, -5.719274019375665929, 31.04275706135234714 ) ) ;
#118857=CARTESIAN_POINT ( 'NONE',  ( 21.52544592524334988, 5.823673210054432836, 66.45942372801903275 ) ) ;
#118858=CARTESIAN_POINT ( 'NONE',  ( -19.03943276465977164, 0.05219959533909376836, 106.2489096053143669 ) ) ;
#118859=CARTESIAN_POINT ( 'NONE',  ( 10.72451020669898902, -18.67979575497178502, 67.91557627198102409 ) ) ;
#118860=CARTESIAN_POINT ( 'NONE',  ( -21.53943276465977519, 0.05219959533907696930, 106.2489096053143811 ) ) ;
#118861=CARTESIAN_POINT ( 'NONE',  ( 8.224510206698742110, 14.34966873604972548, 57.08442372801901854 ) ) ;
#118862=CARTESIAN_POINT ( 'NONE',  ( 10.72451020669898902, -18.67979575497178502, 52.91557627198103830 ) ) ;
#118863=CARTESIAN_POINT ( 'NONE',  ( -21.52544592524334988, -5.823673210054445271, 103.9594237280190185 ) ) ;
#118864=CARTESIAN_POINT ( 'NONE',  ( -5.153800228976328057, -19.02544592524343514, 57.29057627198103120 ) ) ;
#118865=CARTESIAN_POINT ( 'NONE',  ( 5.153800228976335163, 19.02544592524342804, 104.7905762719809957 ) ) ;
#118866=CARTESIAN_POINT ( 'NONE',  ( 19.03943276465977164, -0.05219959533909143690, 78.74890960531436690 ) ) ;
#118867=CARTESIAN_POINT ( 'NONE',  ( 16.79531203550681440, -7.028104445595344529, 86.24755011779544134 ) ) ;
#118868=CARTESIAN_POINT ( 'NONE',  ( -9.474510206698720793, -16.51473224551083518, 64.58442372801900433 ) ) ;
#118869=CARTESIAN_POINT ( 'NONE',  ( 0.05219959533937995610, -21.53943276465977519, 110.0010903946856757 ) ) ;
#118870=CARTESIAN_POINT ( 'NONE',  ( 18.67979575497178502, 10.72451020669898547, 44.16557627198103120 ) ) ;
#118871=CARTESIAN_POINT ( 'NONE',  ( -12.06949235617739369, -12.14591786802326823, 99.37609039468568994 ) ) ;
#118872=CARTESIAN_POINT ( 'NONE',  ( -9.564922557961040184, 16.46253265017147172, 87.91775706135233293 ) ) ;
#118874=CARTESIAN_POINT ( 'NONE',  ( 5.049401038297881783, 19.05341960407617563, 27.29275706135232937 ) ) ;
#118875=CARTESIAN_POINT ( 'NONE',  ( -16.51473224551082808, 9.474510206698731452, 88.33442372801900433 ) ) ;
#118876=CARTESIAN_POINT ( 'NONE',  ( -13.89961937509957401, -13.97604488694547875, 49.37609039468567573 ) ) ;
#118878=CARTESIAN_POINT ( 'NONE',  ( -13.89961937509977652, 13.97604488694528158, 45.62390960531433848 ) ) ;
#118879=CARTESIAN_POINT ( 'NONE',  ( -16.53943276465976808, 0.05219959533911058130, 51.24890960531436690 ) ) ;
#118880=CARTESIAN_POINT ( 'NONE',  ( -13.89961937509977652, 13.97604488694528158, 35.62390960531435269 ) ) ;
#118881=CARTESIAN_POINT ( 'NONE',  ( 16.55341960407611168, 4.379528057220329451, 38.95724293864768839 ) ) ;
#118882=CARTESIAN_POINT ( 'NONE',  ( -15.49999999999999822, -7.500000000000000888, 120.0000000000000142 ) ) ;
#118883=CARTESIAN_POINT ( 'NONE',  ( -0.05219959533934338120, 16.53943276465976808, 107.5010903946856899 ) ) ;
#118884=CARTESIAN_POINT ( 'NONE',  ( 13.97604488694527802, 13.89961937509977652, 44.37390960531435269 ) ) ;
#118885=CARTESIAN_POINT ( 'NONE',  ( -13.97604488694547697, 13.89961937509957934, 28.12609039468565797 ) ) ;
#118886=CARTESIAN_POINT ( 'NONE',  ( 0.05219959533934541429, -16.53943276465976808, 30.00109039468568284 ) ) ;
#118887=CARTESIAN_POINT ( 'NONE',  ( -15.80617190586745835, -15.72974639402198527, 36.87390960531435979 ) ) ;
#118888=CARTESIAN_POINT ( 'NONE',  ( -21.52544592524334988, -5.823673210054445271, 93.95942372801903275 ) ) ;
#118889=CARTESIAN_POINT ( 'NONE',  ( -0.05219959533909027116, -19.03943276465977164, 107.4989096053143527 ) ) ;
#118890=CARTESIAN_POINT ( 'NONE',  ( -0.05219959533909027116, -19.03943276465977164, 77.49890960531435269 ) ) ;
#118892=CARTESIAN_POINT ( 'NONE',  ( -21.53943276465977519, 0.05219959533907696930, 111.2489096053143669 ) ) ;
#118893=CARTESIAN_POINT ( 'NONE',  ( -12.06949235617756955, 12.14591786802309770, 85.62390960531436690 ) ) ;
#118894=CARTESIAN_POINT ( 'NONE',  ( 21.53943276465977519, -0.05219959533907433946, 78.74890960531436690 ) ) ;
#118895=CARTESIAN_POINT ( 'NONE',  ( 5.153800228976335163, 19.02544592524342804, 69.79057627198103830 ) ) ;
#118896=CARTESIAN_POINT ( 'NONE',  ( -19.05341960407611168, -5.049401038298163336, 71.45724293864766707 ) ) ;
#118897=CARTESIAN_POINT ( 'NONE',  ( -18.67979575497178146, -10.72451020669898902, 96.66557627198102409 ) ) ;
#118899=CARTESIAN_POINT ( 'NONE',  ( -5.049401038298153566, 19.05341960407611168, 55.20724293864769550 ) ) ;
#118901=CARTESIAN_POINT ( 'NONE',  ( -16.55341960407611168, -4.379528057220339221, 111.4572429386476813 ) ) ;
#118902=CARTESIAN_POINT ( 'NONE',  ( -0.05219959533909027116, -19.03943276465977164, 22.49890960531436690 ) ) ;
#118903=CARTESIAN_POINT ( 'NONE',  ( -5.049401038298153566, 19.05341960407611168, 60.20724293864768129 ) ) ;
#118904=CARTESIAN_POINT ( 'NONE',  ( -9.474510206698720793, -16.51473224551083518, 84.58442372801900433 ) ) ;
#118905=CARTESIAN_POINT ( 'NONE',  ( 12.06949235617757843, -12.14591786802309237, 93.12390960531436690 ) ) ;
#118906=CARTESIAN_POINT ( 'NONE',  ( -15.80617190586768217, 15.72974639402176855, 58.12609039468568994 ) ) ;
#118907=CARTESIAN_POINT ( 'NONE',  ( -13.89961937509977652, 13.97604488694528158, 50.62390960531435979 ) ) ;
#118908=CARTESIAN_POINT ( 'NONE',  ( -21.52544592524343514, 5.823673210054127303, 111.0405762719810525 ) ) ;
#118909=CARTESIAN_POINT ( 'NONE',  ( 4.483927247898545687, 16.52544592524342804, 94.79057627198105251 ) ) ;
#118911=CARTESIAN_POINT ( 'NONE',  ( -13.89961937509977652, 13.97604488694528158, 75.62390960531438111 ) ) ;
#118913=CARTESIAN_POINT ( 'NONE',  ( -0.05219959533936034679, 19.03943276465977164, 107.5010903946856615 ) ) ;
#118914=CARTESIAN_POINT ( 'NONE',  ( -18.67979575497178146, -10.72451020669898902, 21.66557627198102409 ) ) ;
#118915=CARTESIAN_POINT ( 'NONE',  ( -21.52544592524334988, -5.823673210054445271, 53.95942372801900433 ) ) ;
#118916=CARTESIAN_POINT ( 'NONE',  ( 16.46253265017160672, -9.564922557960803928, 93.33224293864769550 ) ) ;
#118917=CARTESIAN_POINT ( 'NONE',  ( -19.02544592524334988, -5.153800228976617603, 78.95942372801900433 ) ) ;
#118918=CARTESIAN_POINT ( 'NONE',  ( 13.97604488694527802, 13.89961937509977652, 74.37390960531436690 ) ) ;
#118919=CARTESIAN_POINT ( 'NONE',  ( -14.34966873604960291, -8.224510206698953496, 76.66557627198103830 ) ) ;
#118920=CARTESIAN_POINT ( 'NONE',  ( 9.474510206698971260, -16.51473224551069308, 102.9155762719810241 ) ) ;
#118921=CARTESIAN_POINT ( 'NONE',  ( 12.14591786802309770, 12.06949235617756955, 84.37390960531438111 ) ) ;
#118922=CARTESIAN_POINT ( 'NONE',  ( -16.51473224551069308, -9.474510206698971260, 91.66557627198103830 ) ) ;
#118923=CARTESIAN_POINT ( 'NONE',  ( 5.153800228976615827, -19.02544592524334988, 40.20942372801898301 ) ) ;
#118924=CARTESIAN_POINT ( 'NONE',  ( 0.05219959533909260263, 19.03943276465977164, 44.99890960531435979 ) ) ;
#118925=CARTESIAN_POINT ( 'NONE',  ( 16.53943276465976808, -0.05219959533910856209, 38.74890960531435979 ) ) ;
#118926=CARTESIAN_POINT ( 'NONE',  ( -0.05219959533909027116, -19.03943276465977164, 27.49890960531435624 ) ) ;
#118928=CARTESIAN_POINT ( 'NONE',  ( 10.72451020669871369, 18.67979575497193778, 47.08442372801901854 ) ) ;
#118929=CARTESIAN_POINT ( 'NONE',  ( 19.02544592524334988, 5.153800228976608722, 86.45942372801900433 ) ) ;
#118930=CARTESIAN_POINT ( 'NONE',  ( -12.06949235617756955, 12.14591786802309770, 35.62390960531437401 ) ) ;
#118931=CARTESIAN_POINT ( 'NONE',  ( 5.719274019375991003, -21.55341960407610458, 97.70724293864772392 ) ) ;
#118932=CARTESIAN_POINT ( 'NONE',  ( 5.719274019375991003, -21.55341960407610458, 37.70724293864769550 ) ) ;
#118933=CARTESIAN_POINT ( 'NONE',  ( -14.29746914071049879, 8.314922557960819915, 80.83224293864769550 ) ) ;
#118934=CARTESIAN_POINT ( 'NONE',  ( -9.564922557960796823, -16.46253265017161027, 37.08224293864768839 ) ) ;
#118935=CARTESIAN_POINT ( 'NONE',  ( 16.52544592524335698, 4.483927247898782831, 101.4594237280190185 ) ) ;
#118936=CARTESIAN_POINT ( 'NONE',  ( 12.06949235617739724, 12.14591786802326823, 86.87609039468568994 ) ) ;
#118937=CARTESIAN_POINT ( 'NONE',  ( 0.05219959533934541429, -16.53943276465976808, 65.00109039468568994 ) ) ;
#118938=CARTESIAN_POINT ( 'NONE',  ( -16.46253265017146816, -9.564922557961047289, 29.16775706135232937 ) ) ;
#118939=CARTESIAN_POINT ( 'NONE',  ( 19.03943276465977164, -0.05219959533909143690, 93.74890960531435269 ) ) ;
#118940=CARTESIAN_POINT ( 'NONE',  ( -9.564922557960796823, -16.46253265017161027, 77.08224293864769550 ) ) ;
#118941=CARTESIAN_POINT ( 'NONE',  ( 16.53943276465976808, 0.05219959533934440121, 71.25109039468568994 ) ) ;
#118942=CARTESIAN_POINT ( 'NONE',  ( 19.02544592524343514, -5.153800228976328945, 33.54057627198102409 ) ) ;
#118943=CARTESIAN_POINT ( 'NONE',  ( 4.379528057220339221, -16.55341960407611168, 47.70724293864770260 ) ) ;
#118944=CARTESIAN_POINT ( 'NONE',  ( 19.02544592524343514, -5.153800228976328945, 113.5405762719810241 ) ) ;
#118945=CARTESIAN_POINT ( 'NONE',  ( 5.153800228976335163, 19.02544592524342804, 94.79057627198103830 ) ) ;
#118946=CARTESIAN_POINT ( 'NONE',  ( -10.81492255796078084, -18.62759615963271287, 32.08224293864769550 ) ) ;
#118947=CARTESIAN_POINT ( 'NONE',  ( -8.224510206698948167, 14.34966873604960824, 65.41557627198102409 ) ) ;
#118948=CARTESIAN_POINT ( 'NONE',  ( -14.29746914071049879, 8.314922557960819915, 60.83224293864769550 ) ) ;
#118950=CARTESIAN_POINT ( 'NONE',  ( -16.46253265017146816, -9.564922557961047289, 64.16775706135233293 ) ) ;
#118951=CARTESIAN_POINT ( 'NONE',  ( -19.02544592524342804, 5.153800228976336051, 96.04057627198103830 ) ) ;
#118952=CARTESIAN_POINT ( 'NONE',  ( 5.049401038297881783, 19.05341960407617563, 67.29275706135234714 ) ) ;
#118953=CARTESIAN_POINT ( 'NONE',  ( -13.89961937509957401, -13.97604488694547697, 39.37609039468566152 ) ) ;
#118954=CARTESIAN_POINT ( 'NONE',  ( 13.89961937509957401, 13.97604488694547697, 111.8760903946856757 ) ) ;
#118955=CARTESIAN_POINT ( 'NONE',  ( 12.06949235617739724, 12.14591786802326823, 96.87609039468568994 ) ) ;
#118956=CARTESIAN_POINT ( 'NONE',  ( 16.46253265017160672, -9.564922557960803928, 43.33224293864769550 ) ) ;
#118957=CARTESIAN_POINT ( 'NONE',  ( -15.80617190586745835, -15.72974639402198527, 26.87390960531435979 ) ) ;
#118958=CARTESIAN_POINT ( 'NONE',  ( 10.72451020669871369, 18.67979575497193778, 52.08442372801901854 ) ) ;
#118959=CARTESIAN_POINT ( 'NONE',  ( -0.05219959533936034679, 19.03943276465977164, 112.5010903946856757 ) ) ;
#118961=CARTESIAN_POINT ( 'NONE',  ( -5.153800228976328057, -19.02544592524343514, 77.29057627198099567 ) ) ;
#118964=CARTESIAN_POINT ( 'NONE',  ( -9.564922557960796823, -16.46253265017161027, 112.0822429386476955 ) ) ;
#118965=CARTESIAN_POINT ( 'NONE',  ( -8.224510206698948167, 14.34966873604960824, 70.41557627198102409 ) ) ;
#118966=CARTESIAN_POINT ( 'NONE',  ( 13.89961937509977652, -13.97604488694527269, 78.12390960531433848 ) ) ;
#118968=CARTESIAN_POINT ( 'NONE',  ( 16.51473224551069308, 9.474510206698969483, 74.16557627198103830 ) ) ;
#118969=CARTESIAN_POINT ( 'NONE',  ( -9.564922557961040184, 16.46253265017147172, 92.91775706135233293 ) ) ;
#118970=CARTESIAN_POINT ( 'NONE',  ( -5.719274019375978568, 21.55341960407610458, 70.20724293864769550 ) ) ;
#118971=CARTESIAN_POINT ( 'NONE',  ( 13.89961937509977652, -13.97604488694527269, 33.12390960531434558 ) ) ;
#118972=CARTESIAN_POINT ( 'NONE',  ( -19.03943276465977164, -0.05219959533935918106, 58.75109039468566863 ) ) ;
#118973=CARTESIAN_POINT ( 'NONE',  ( -0.05219959533909027116, -19.03943276465977164, 52.49890960531436690 ) ) ;
#118974=CARTESIAN_POINT ( 'NONE',  ( 13.97604488694527802, 13.89961937509977652, 89.37390960531436690 ) ) ;
#118976=CARTESIAN_POINT ( 'NONE',  ( -21.52544592524343514, 5.823673210054127303, 91.04057627198103830 ) ) ;
#118977=CARTESIAN_POINT ( 'NONE',  ( -16.55341960407611168, -4.379528057220339221, 96.45724293864770971 ) ) ;
#118978=CARTESIAN_POINT ( 'NONE',  ( 5.153800228976615827, -19.02544592524334988, 45.20942372801901143 ) ) ;
#118979=CARTESIAN_POINT ( 'NONE',  ( -18.67979575497178146, -10.72451020669898902, 91.66557627198103830 ) ) ;
#118980=CARTESIAN_POINT ( 'NONE',  ( 5.823673210054125526, 21.52544592524343514, 79.79057627198102409 ) ) ;
#118981=CARTESIAN_POINT ( 'NONE',  ( 4.379528057220339221, -16.55341960407611168, 32.70724293864770260 ) ) ;
#118982=CARTESIAN_POINT ( 'NONE',  ( -21.53943276465977519, -0.05219959533937600094, 103.7510903946857042 ) ) ;
#118983=CARTESIAN_POINT ( 'NONE',  ( 19.02544592524343514, -5.153800228976328945, 73.54057627198103830 ) ) ;
#118984=CARTESIAN_POINT ( 'NONE',  ( -16.51473224551069308, -9.474510206698971260, 31.66557627198102054 ) ) ;
#118985=CARTESIAN_POINT ( 'NONE',  ( 10.81492255796106328, -18.62759615963255655, 45.41775706135234003 ) ) ;
#118986=CARTESIAN_POINT ( 'NONE',  ( 15.80617190586769283, -15.72974639402175789, 55.62609039468568284 ) ) ;
#118987=CARTESIAN_POINT ( 'NONE',  ( -9.564922557960796823, -16.46253265017161027, 52.08224293864768839 ) ) ;
#118988=CARTESIAN_POINT ( 'NONE',  ( 5.719274019375673035, 21.55341960407619339, 27.29275706135234358 ) ) ;
#118989=CARTESIAN_POINT ( 'NONE',  ( 5.153800228976615827, -19.02544592524334988, 65.20942372801900433 ) ) ;
#118991=CARTESIAN_POINT ( 'NONE',  ( 19.05341960407611168, 5.049401038298154454, 33.95724293864769550 ) ) ;
#118992=CARTESIAN_POINT ( 'NONE',  ( -8.314922557961024197, 14.29746914071037800, 22.91775706135235069 ) ) ;
#118993=CARTESIAN_POINT ( 'NONE',  ( -19.02544592524342804, 5.153800228976336051, 26.04057627198103120 ) ) ;
#118994=CARTESIAN_POINT ( 'NONE',  ( -16.55341960407617563, 4.379528057220093196, 78.54275706135236135 ) ) ;
#118995=CARTESIAN_POINT ( 'NONE',  ( 0.05219959533909260263, 19.03943276465977164, 34.99890960531435979 ) ) ;
#118997=CARTESIAN_POINT ( 'NONE',  ( 19.02544592524343514, -5.153800228976328945, 88.54057627198102409 ) ) ;
#118998=CARTESIAN_POINT ( 'NONE',  ( 13.97604488694527802, 13.89961937509977652, 24.37390960531435624 ) ) ;
#118999=CARTESIAN_POINT ( 'NONE',  ( 5.719274019375991003, -21.55341960407610458, 77.70724293864770971 ) ) ;
#119000=CARTESIAN_POINT ( 'NONE',  ( 14.34966873604972726, -8.224510206698740333, 40.83442372801901854 ) ) ;
#119001=CARTESIAN_POINT ( 'NONE',  ( 19.03943276465977164, 0.05219959533936151252, 21.25109039468565797 ) ) ;
#119002=CARTESIAN_POINT ( 'NONE',  ( 13.89961937509977652, -13.97604488694527269, 33.12390960531434558 ) ) ;
#119003=CARTESIAN_POINT ( 'NONE',  ( -16.53943276465976808, 0.05219959533911058130, 31.24890960531435979 ) ) ;
#119004=CARTESIAN_POINT ( 'NONE',  ( -16.53943276465976808, 0.05219959533911058130, 66.24890960531436690 ) ) ;
#119005=CARTESIAN_POINT ( 'NONE',  ( -19.05341960407611168, -5.049401038298163336, 66.45724293864769550 ) ) ;
#119006=CARTESIAN_POINT ( 'NONE',  ( 21.55341960407619695, -5.719274019375665929, 106.0427570613523471 ) ) ;
#119007=CARTESIAN_POINT ( 'NONE',  ( 0.05219959533907565091, 21.53943276465977519, 114.9989096053143669 ) ) ;
#119008=CARTESIAN_POINT ( 'NONE',  ( 19.05341960407611168, 5.049401038298154454, 73.95724293864768129 ) ) ;
#119009=CARTESIAN_POINT ( 'NONE',  ( 18.62759615963255655, 10.81492255796105972, 91.66775706135234714 ) ) ;
#119010=CARTESIAN_POINT ( 'NONE',  ( -16.53943276465976808, -0.05219959533934237506, 63.75109039468568284 ) ) ;
#119011=CARTESIAN_POINT ( 'NONE',  ( 8.224510206698742110, 14.34966873604972548, 27.08442372801901854 ) ) ;
#119012=CARTESIAN_POINT ( 'NONE',  ( -16.53943276465976808, 0.05219959533911058130, 96.24890960531435269 ) ) ;
#119013=CARTESIAN_POINT ( 'NONE',  ( 19.03943276465977164, -0.05219959533909143690, 103.7489096053143669 ) ) ;
#119014=CARTESIAN_POINT ( 'NONE',  ( 4.379528057220339221, -16.55341960407611168, 27.70724293864769905 ) ) ;
#119015=CARTESIAN_POINT ( 'NONE',  ( 19.03943276465977164, -0.05219959533909143690, 28.74890960531435624 ) ) ;
#119016=CARTESIAN_POINT ( 'NONE',  ( 16.53943276465976808, 0.05219959533934440121, 51.25109039468568994 ) ) ;
#119017=CARTESIAN_POINT ( 'NONE',  ( 14.34966873604960469, 8.224510206698951720, 49.16557627198102409 ) ) ;
#119018=CARTESIAN_POINT ( 'NONE',  ( 16.55341960407618274, -4.379528057220086978, 106.0427570613523471 ) ) ;
#119019=CARTESIAN_POINT ( 'NONE',  ( -16.46253265017160317, 9.564922557960807481, 110.8322429386476955 ) ) ;
#119020=CARTESIAN_POINT ( 'NONE',  ( 15.72974639402199770, -15.80617190586745480, 28.12390960531435979 ) ) ;
#119021=CARTESIAN_POINT ( 'NONE',  ( 21.55341960407619695, -5.719274019375665929, 106.0427570613523471 ) ) ;
#119022=CARTESIAN_POINT ( 'NONE',  ( -16.52544592524342804, 4.483927247898546575, 81.04057627198102409 ) ) ;
#119023=CARTESIAN_POINT ( 'NONE',  ( 13.97604488694527802, 13.89961937509977652, 89.37390960531436690 ) ) ;
#119025=CARTESIAN_POINT ( 'NONE',  ( -14.29746914071037622, -8.314922557961029526, 34.16775706135234714 ) ) ;
#119026=CARTESIAN_POINT ( 'NONE',  ( 5.049401038298161559, -19.05341960407611168, 42.70724293864767418 ) ) ;
#119027=CARTESIAN_POINT ( 'NONE',  ( 0.05219959533934541429, -16.53943276465976808, 40.00109039468567573 ) ) ;
#119029=CARTESIAN_POINT ( 'NONE',  ( -5.153800228976607833, 19.02544592524334988, 47.70942372801900433 ) ) ;
#119030=CARTESIAN_POINT ( 'NONE',  ( -5.049401038298153566, 19.05341960407611168, 50.20724293864770260 ) ) ;
#119031=CARTESIAN_POINT ( 'NONE',  ( -8.314922557961024197, 14.29746914071037800, 82.91775706135234714 ) ) ;
#119032=CARTESIAN_POINT ( 'NONE',  ( 9.564922557961047289, -16.46253265017146816, 90.41775706135234714 ) ) ;
#119033=CARTESIAN_POINT ( 'NONE',  ( 19.02544592524343514, -5.153800228976328945, 63.54057627198103830 ) ) ;
#119034=CARTESIAN_POINT ( 'NONE',  ( 21.55341960407610458, 5.719274019375980345, 93.95724293864770971 ) ) ;
#119035=CARTESIAN_POINT ( 'NONE',  ( -4.379528057220328563, 16.55341960407611168, 95.20724293864769550 ) ) ;
#119037=CARTESIAN_POINT ( 'NONE',  ( -19.03943276465977164, -0.05219959533935918106, 68.75109039468566152 ) ) ;
#119038=CARTESIAN_POINT ( 'NONE',  ( -15.72974639402197994, 15.80617190586746368, 65.62390960531436690 ) ) ;
#119039=CARTESIAN_POINT ( 'NONE',  ( 0.05219959533936267826, -19.03943276465977164, 40.00109039468566152 ) ) ;
#119041=CARTESIAN_POINT ( 'NONE',  ( 21.53943276465977519, -0.05219959533907433946, 88.74890960531436690 ) ) ;
#119042=CARTESIAN_POINT ( 'NONE',  ( -17.49999999999999645, 5.499999999999992895, 83.71769037696435589 ) ) ;
#119043=CARTESIAN_POINT ( 'NONE',  ( -5.049401038297874678, -19.05341960407617918, 104.7927570613523471 ) ) ;
#119044=CARTESIAN_POINT ( 'NONE',  ( -17.60691670004650788, -5.500000000000026645, 99.13333313366442212 ) ) ;
#119045=CARTESIAN_POINT ( 'NONE',  ( -12.06949235617739369, -12.14591786802326823, 29.37609039468568284 ) ) ;
#119046=CARTESIAN_POINT ( 'NONE',  ( -0.05219959533909027116, -19.03943276465977164, 47.49890960531435979 ) ) ;
#119047=CARTESIAN_POINT ( 'NONE',  ( 16.51473224551069308, 9.474510206698969483, 109.1655762719810383 ) ) ;
#119048=CARTESIAN_POINT ( 'NONE',  ( -18.62759615963270932, 10.81492255796079327, 90.83224293864769550 ) ) ;
#119049=CARTESIAN_POINT ( 'NONE',  ( -21.52544592524334988, -5.823673210054445271, 58.95942372801902565 ) ) ;
#119050=CARTESIAN_POINT ( 'NONE',  ( 5.049401038297881783, 19.05341960407617563, 112.2927570613523471 ) ) ;
#119051=CARTESIAN_POINT ( 'NONE',  ( 0.05219959533937995610, -21.53943276465977519, 110.0010903946856757 ) ) ;
#119052=CARTESIAN_POINT ( 'NONE',  ( 8.314922557960818139, 14.29746914071049879, 34.58224293864770260 ) ) ;
#119053=CARTESIAN_POINT ( 'NONE',  ( -10.81492255796078084, -18.62759615963271287, 102.0822429386476955 ) ) ;
#119054=CARTESIAN_POINT ( 'NONE',  ( 8.314922557960818139, 14.29746914071049879, 49.58224293864769550 ) ) ;
#119055=CARTESIAN_POINT ( 'NONE',  ( -19.02544592524334988, -5.153800228976617603, 93.95942372801900433 ) ) ;
#119056=CARTESIAN_POINT ( 'NONE',  ( 16.46253265017146816, 9.564922557961045513, 51.66775706135233293 ) ) ;
#119057=CARTESIAN_POINT ( 'NONE',  ( -0.05219959533937732626, 21.53943276465977519, 67.50109039468568994 ) ) ;
#119058=CARTESIAN_POINT ( 'NONE',  ( 5.153800228976615827, -19.02544592524334988, 45.20942372801901143 ) ) ;
#119059=CARTESIAN_POINT ( 'NONE',  ( -8.224510206698948167, 14.34966873604960824, 115.4155762719810241 ) ) ;
#119060=CARTESIAN_POINT ( 'NONE',  ( 10.81492255796078972, 18.62759615963270932, 49.58224293864769550 ) ) ;
#119061=CARTESIAN_POINT ( 'NONE',  ( 4.379528057220339221, -16.55341960407611168, 42.70724293864770260 ) ) ;
#119062=CARTESIAN_POINT ( 'NONE',  ( -10.81492255796105439, 18.62759615963255655, 107.9177570613523471 ) ) ;
#119063=CARTESIAN_POINT ( 'NONE',  ( -12.14591786802326823, 12.06949235617739902, 73.12609039468567573 ) ) ;
#119064=CARTESIAN_POINT ( 'NONE',  ( -12.06949235617756955, 12.14591786802309770, 45.62390960531436690 ) ) ;
#119065=CARTESIAN_POINT ( 'NONE',  ( 10.81492255796106328, -18.62759615963255655, 70.41775706135236135 ) ) ;
#119066=CARTESIAN_POINT ( 'NONE',  ( -18.62759615963255300, -10.81492255796106328, 69.16775706135234714 ) ) ;
#119067=CARTESIAN_POINT ( 'NONE',  ( -18.67979575497178146, -10.72451020669898902, 61.66557627198103120 ) ) ;
#119068=CARTESIAN_POINT ( 'NONE',  ( 16.51473224551069308, 9.474510206698969483, 34.16557627198102409 ) ) ;
#119069=CARTESIAN_POINT ( 'NONE',  ( -21.53943276465977519, -0.05219959533937600094, 38.75109039468567573 ) ) ;
#119070=CARTESIAN_POINT ( 'NONE',  ( 16.55341960407611168, 4.379528057220329451, 113.9572429386477239 ) ) ;
#119071=CARTESIAN_POINT ( 'NONE',  ( 5.049401038298161559, -19.05341960407611168, 37.70724293864768839 ) ) ;
#119072=CARTESIAN_POINT ( 'NONE',  ( 8.224510206698953496, -14.34966873604960469, 87.91557627198103830 ) ) ;
#119073=CARTESIAN_POINT ( 'NONE',  ( 5.153800228976335163, 19.02544592524342804, 84.79057627198099567 ) ) ;
#119074=CARTESIAN_POINT ( 'NONE',  ( -16.53943276465976808, 0.05219959533911058130, 46.24890960531435979 ) ) ;
#119075=CARTESIAN_POINT ( 'NONE',  ( -16.53943276465976808, 0.05219959533911058130, 101.2489096053143669 ) ) ;
#119076=CARTESIAN_POINT ( 'NONE',  ( -10.72451020669898014, 18.67979575497178502, 75.41557627198102409 ) ) ;
#119077=CARTESIAN_POINT ( 'NONE',  ( -21.53943276465977519, 0.05219959533907696930, 111.2489096053143669 ) ) ;
#119078=CARTESIAN_POINT ( 'NONE',  ( -19.05341960407611168, -5.049401038298163336, 111.4572429386476671 ) ) ;
#119079=CARTESIAN_POINT ( 'NONE',  ( 16.46253265017160672, -9.564922557960803928, 63.33224293864769550 ) ) ;
#119080=CARTESIAN_POINT ( 'NONE',  ( 4.483927247898790824, -16.52544592524335698, 25.20942372801901854 ) ) ;
#119081=CARTESIAN_POINT ( 'NONE',  ( -5.719274019375978568, 21.55341960407610458, 55.20724293864770260 ) ) ;
#119082=CARTESIAN_POINT ( 'NONE',  ( 5.823673210054444382, -21.52544592524334988, 90.20942372801903275 ) ) ;
#119083=B_SPLINE_CURVE_WITH_KNOTS ( 'NONE', 3,
 ( #106669, #151209, #166382, #72367, #165384, #75337 ),
 .UNSPECIFIED., .F., .F.,
 ( 4, 2, 4 ),
 ( 0.003239945802372208323, 0.003620412082092052709, 0.004000878361811896662 ),
 .UNSPECIFIED. ) ;
#119084=CARTESIAN_POINT ( 'NONE',  ( -5.153800228976328057, -19.02544592524343514, 82.29057627198103830 ) ) ;
#119085=CARTESIAN_POINT ( 'NONE',  ( -10.72451020669898014, 18.67979575497178502, 115.4155762719810241 ) ) ;
#119086=CARTESIAN_POINT ( 'NONE',  ( 9.474510206698971260, -16.51473224551069308, 112.9155762719810383 ) ) ;
#119087=CARTESIAN_POINT ( 'NONE',  ( 0.05219959533934541429, -16.53943276465976808, 95.00109039468568994 ) ) ;
#119088=CARTESIAN_POINT ( 'NONE',  ( 15.72974639402176855, 15.80617190586768217, 71.87609039468568994 ) ) ;
#119089=CARTESIAN_POINT ( 'NONE',  ( -5.823673210054431948, 21.52544592524334988, 97.70942372801904696 ) ) ;
#119090=CARTESIAN_POINT ( 'NONE',  ( -16.52544592524335698, -4.483927247898792601, 58.95942372801902565 ) ) ;
#119091=CARTESIAN_POINT ( 'NONE',  ( -18.67979575497178146, -10.72451020669898902, 106.6655762719810383 ) ) ;
#119092=CARTESIAN_POINT ( 'NONE',  ( -16.46253265017160317, 9.564922557960807481, 110.8322429386476955 ) ) ;
#119093=CARTESIAN_POINT ( 'NONE',  ( 15.80617190586769283, -15.72974639402175789, 85.62609039468568994 ) ) ;
#119094=CARTESIAN_POINT ( 'NONE',  ( -21.55341960407610458, -5.719274019375992779, 91.45724293864769550 ) ) ;
#119095=CARTESIAN_POINT ( 'NONE',  ( 5.049401038297881783, 19.05341960407617563, 52.29275706135234003 ) ) ;
#119096=CARTESIAN_POINT ( 'NONE',  ( 10.72451020669898902, -18.67979575497178502, 57.91557627198103120 ) ) ;
#119097=CARTESIAN_POINT ( 'NONE',  ( 19.03943276465977164, -0.05219959533909143690, 98.74890960531436690 ) ) ;
#119098=CARTESIAN_POINT ( 'NONE',  ( 14.29746914071049879, -8.314922557960816363, 33.33224293864769550 ) ) ;
#119100=CARTESIAN_POINT ( 'NONE',  ( 16.46253265017146816, 9.564922557961045513, 66.66775706135233293 ) ) ;
#119101=CARTESIAN_POINT ( 'NONE',  ( 18.22780087662122384, -5.500000000000022204, 91.01540105326107266 ) ) ;
#119102=CARTESIAN_POINT ( 'NONE',  ( -19.05341960407617563, 5.049401038297882671, 103.5427570613523329 ) ) ;
#119103=CARTESIAN_POINT ( 'NONE',  ( -10.81492255796078084, -18.62759615963271287, 82.08224293864768129 ) ) ;
#119104=CARTESIAN_POINT ( 'NONE',  ( -4.379528057220328563, 16.55341960407611168, 50.20724293864769550 ) ) ;
#119105=CARTESIAN_POINT ( 'NONE',  ( 8.224510206698742110, 14.34966873604972548, 37.08442372801901143 ) ) ;
#119106=CARTESIAN_POINT ( 'NONE',  ( 5.153800228976335163, 19.02544592524342804, 39.79057627198100988 ) ) ;
#119107=CARTESIAN_POINT ( 'NONE',  ( 0.05219959533907565091, 21.53943276465977519, 109.9989096053143527 ) ) ;
#119108=CARTESIAN_POINT ( 'NONE',  ( 16.46253265017146816, 9.564922557961045513, 86.66775706135233293 ) ) ;
#119109=CARTESIAN_POINT ( 'NONE',  ( 5.153800228976335163, 19.02544592524342804, 79.79057627198102409 ) ) ;
#119110=CARTESIAN_POINT ( 'NONE',  ( -9.474510206698964154, 16.51473224551069663, 70.41557627198102409 ) ) ;
#119111=CARTESIAN_POINT ( 'NONE',  ( -21.53943276465977519, 0.05219959533907696930, 81.24890960531436690 ) ) ;
#119112=CARTESIAN_POINT ( 'NONE',  ( -16.51473224551069308, -9.474510206698971260, 51.66557627198102409 ) ) ;
#119114=CARTESIAN_POINT ( 'NONE',  ( -4.379528057220328563, 16.55341960407611168, 60.20724293864768839 ) ) ;
#119115=CARTESIAN_POINT ( 'NONE',  ( 5.153800228976335163, 19.02544592524342804, 89.79057627198102409 ) ) ;
#119117=CARTESIAN_POINT ( 'NONE',  ( -19.03943276465977164, -0.05219959533935918106, 63.75109039468566863 ) ) ;
#119118=CARTESIAN_POINT ( 'NONE',  ( -21.53943276465977519, 0.05219959533907696930, 71.24890960531435269 ) ) ;
#119119=CARTESIAN_POINT ( 'NONE',  ( 16.46253265017146816, 9.564922557961045513, 36.66775706135233293 ) ) ;
#119120=CARTESIAN_POINT ( 'NONE',  ( -5.153800228976328057, -19.02544592524343514, 97.29057627198099567 ) ) ;
#119122=CARTESIAN_POINT ( 'NONE',  ( -18.62759615963270932, 10.81492255796079327, 35.83224293864768839 ) ) ;
#119123=CARTESIAN_POINT ( 'NONE',  ( -0.05219959533909027116, -19.03943276465977164, 72.49890960531435269 ) ) ;
#119124=CARTESIAN_POINT ( 'NONE',  ( -5.823673210054431948, 21.52544592524334988, 67.70942372801901854 ) ) ;
#119125=CARTESIAN_POINT ( 'NONE',  ( 9.474510206698971260, -16.51473224551069308, 22.91557627198102765 ) ) ;
#119126=CARTESIAN_POINT ( 'NONE',  ( 15.72974639402199770, -15.80617190586745480, 108.1239096053143811 ) ) ;
#119128=CARTESIAN_POINT ( 'NONE',  ( -21.55341960407619339, 5.719274019375674811, 58.54275706135235424 ) ) ;
#119129=VERTEX_POINT ( 'NONE', #108891 ) ;
#119130=CARTESIAN_POINT ( 'NONE',  ( 19.03943276465977164, -0.05219959533909143690, 103.7489096053143669 ) ) ;
#119132=CARTESIAN_POINT ( 'NONE',  ( 13.97604488694527802, 13.89961937509977830, 89.37390960531435269 ) ) ;
#119133=CARTESIAN_POINT ( 'NONE',  ( 5.719274019375991003, -21.55341960407610458, 102.7072429386476955 ) ) ;
#119134=CARTESIAN_POINT ( 'NONE',  ( 19.03943276465977164, -0.05219959533909143690, 58.74890960531435979 ) ) ;
#119135=CARTESIAN_POINT ( 'NONE',  ( 14.29746914071037800, 8.314922557961029526, 36.66775706135234714 ) ) ;
#119137=CARTESIAN_POINT ( 'NONE',  ( 18.62759615963255655, 10.81492255796105972, 101.6677570613523613 ) ) ;
#119138=CARTESIAN_POINT ( 'NONE',  ( -16.51473224551069308, -9.474510206698971260, 41.66557627198103120 ) ) ;
#119139=CARTESIAN_POINT ( 'NONE',  ( -15.72974639402176322, -15.80617190586768395, 104.3760903946856899 ) ) ;
#119140=CARTESIAN_POINT ( 'NONE',  ( -9.564922557960796823, -16.46253265017161027, 92.08224293864769550 ) ) ;
#119141=CARTESIAN_POINT ( 'NONE',  ( -21.53943276465977519, -0.05219959533937600094, 58.75109039468568994 ) ) ;
#119143=CARTESIAN_POINT ( 'NONE',  ( -9.474510206698964154, 16.51473224551069663, 115.4155762719810241 ) ) ;
#119144=CARTESIAN_POINT ( 'NONE',  ( 18.22780087662126647, 5.499999999999818812, 46.48236817873107185 ) ) ;
#119145=CARTESIAN_POINT ( 'NONE',  ( 14.29746914071037800, 8.314922557961029526, 46.66775706135234714 ) ) ;
#119146=CARTESIAN_POINT ( 'NONE',  ( -15.72974639402176322, -15.80617190586768395, 54.37609039468568994 ) ) ;
#119147=CARTESIAN_POINT ( 'NONE',  ( -18.67979575497193778, 10.72451020669871902, 88.33442372801901854 ) ) ;
#119149=CARTESIAN_POINT ( 'NONE',  ( -0.05219959533934338120, 16.53943276465976808, 27.50109039468567929 ) ) ;
#119150=CARTESIAN_POINT ( 'NONE',  ( 9.474510206698971260, -16.51473224551069308, 67.91557627198102409 ) ) ;
#119151=CARTESIAN_POINT ( 'NONE',  ( -5.049401038298153566, 19.05341960407611168, 110.2072429386476671 ) ) ;
#119152=CARTESIAN_POINT ( 'NONE',  ( 16.29526858892879915, 7.335722546919997811, 43.29670597800208043 ) ) ;
#119153=CARTESIAN_POINT ( 'NONE',  ( 5.049401038298161559, -19.05341960407611168, 22.70724293864769194 ) ) ;
#119154=CARTESIAN_POINT ( 'NONE',  ( -15.80617190586745835, -15.72974639402198527, 41.87390960531435979 ) ) ;
#119155=CARTESIAN_POINT ( 'NONE',  ( 12.14591786802327356, -12.06949235617739191, 95.62609039468568994 ) ) ;
#119156=CARTESIAN_POINT ( 'NONE',  ( 8.314922557960818139, 14.29746914071049879, 79.58224293864769550 ) ) ;
#119157=CARTESIAN_POINT ( 'NONE',  ( 16.51473224551069308, 9.474510206698969483, 64.16557627198102409 ) ) ;
#119158=CARTESIAN_POINT ( 'NONE',  ( 10.81492255796106328, -18.62759615963255655, 95.41775706135234714 ) ) ;
#119159=CARTESIAN_POINT ( 'NONE',  ( -14.29746914071037622, -8.314922557961029526, 24.16775706135235424 ) ) ;
#119160=CARTESIAN_POINT ( 'NONE',  ( -8.224510206698948167, 14.34966873604960824, 95.41557627198102409 ) ) ;
#119161=CARTESIAN_POINT ( 'NONE',  ( 10.72451020669871369, 18.67979575497193778, 37.08442372801901143 ) ) ;
#119162=CARTESIAN_POINT ( 'NONE',  ( -18.62759615963270932, 10.81492255796079327, 70.83224293864770971 ) ) ;
#119163=CARTESIAN_POINT ( 'NONE',  ( -13.97604488694547697, 13.89961937509957934, 43.12609039468566152 ) ) ;
#119165=CARTESIAN_POINT ( 'NONE',  ( -0.05219959533909027116, -19.03943276465977164, 87.49890960531436690 ) ) ;
#119166=CARTESIAN_POINT ( 'NONE',  ( 14.34966873604960469, 8.224510206698951720, 59.16557627198103120 ) ) ;
#119167=CARTESIAN_POINT ( 'NONE',  ( -8.314922557960811034, -14.29746914071050412, 32.08224293864769550 ) ) ;
#119168=CARTESIAN_POINT ( 'NONE',  ( 12.14591786802309770, 12.06949235617756955, 24.37390960531435979 ) ) ;
#119169=CARTESIAN_POINT ( 'NONE',  ( 19.03943276465977164, 0.05219959533936151252, 71.25109039468566152 ) ) ;
#119170=CARTESIAN_POINT ( 'NONE',  ( 17.26172910966777607, 6.454744622555865341, 46.69353091350776452 ) ) ;
#119171=CARTESIAN_POINT ( 'NONE',  ( -0.05219959533907301413, -21.53943276465977519, 22.49890960531436335 ) ) ;
#119172=CARTESIAN_POINT ( 'NONE',  ( 8.224510206698953496, -14.34966873604960469, 87.91557627198103830 ) ) ;
#119174=CARTESIAN_POINT ( 'NONE',  ( -13.97604488694527625, -13.89961937509977652, 51.87390960531436690 ) ) ;
#119175=CARTESIAN_POINT ( 'NONE',  ( -5.823673210054116645, -21.52544592524344225, 47.29057627198103120 ) ) ;
#119176=CARTESIAN_POINT ( 'NONE',  ( -21.53943276465977519, 0.05219959533907696930, 66.24890960531436690 ) ) ;
#119177=CARTESIAN_POINT ( 'NONE',  ( -14.29746914071049879, 8.314922557960819915, 105.8322429386476955 ) ) ;
#119178=CARTESIAN_POINT ( 'NONE',  ( -14.29746914071037622, -8.314922557961029526, 59.16775706135234714 ) ) ;
#119179=CARTESIAN_POINT ( 'NONE',  ( 9.564922557960805705, 16.46253265017160317, 49.58224293864770260 ) ) ;
#119180=CARTESIAN_POINT ( 'NONE',  ( 5.719274019375673035, 21.55341960407619339, 52.29275706135236135 ) ) ;
#119181=CARTESIAN_POINT ( 'NONE',  ( 12.06949235617757843, -12.14591786802309237, 108.1239096053143811 ) ) ;
#119182=CARTESIAN_POINT ( 'NONE',  ( 19.03943276465977164, 0.05219959533936151252, 96.25109039468567573 ) ) ;
#119185=CARTESIAN_POINT ( 'NONE',  ( 5.823673210054125526, 21.52544592524343514, 29.79057627198102409 ) ) ;
#119186=CARTESIAN_POINT ( 'NONE',  ( 5.153800228976335163, 19.02544592524342804, 24.79057627198102765 ) ) ;
#119187=CARTESIAN_POINT ( 'NONE',  ( -5.719274019375665041, -21.55341960407619695, 74.79275706135234714 ) ) ;
#119189=CARTESIAN_POINT ( 'NONE',  ( -16.52544592524335698, -4.483927247898792601, 53.95942372801900433 ) ) ;
#119190=CARTESIAN_POINT ( 'NONE',  ( -8.314922557960811034, -14.29746914071050412, 47.08224293864770260 ) ) ;
#119191=CARTESIAN_POINT ( 'NONE',  ( 18.67979575497178502, 10.72451020669898547, 64.16557627198102409 ) ) ;
#119192=CARTESIAN_POINT ( 'NONE',  ( -18.62759615963270932, 10.81492255796079327, 75.83224293864769550 ) ) ;
#119194=CARTESIAN_POINT ( 'NONE',  ( 16.46253265017146816, 9.564922557961045513, 81.66775706135233293 ) ) ;
#119195=CARTESIAN_POINT ( 'NONE',  ( 21.52544592524344225, -5.823673210054117533, 23.54057627198102765 ) ) ;
#119196=CARTESIAN_POINT ( 'NONE',  ( -5.049401038298153566, 19.05341960407611168, 45.20724293864769550 ) ) ;
#119197=CARTESIAN_POINT ( 'NONE',  ( -14.29746914071049879, 8.314922557960819915, 110.8322429386476955 ) ) ;
#119198=CARTESIAN_POINT ( 'NONE',  ( 13.89961937509977652, -13.97604488694527269, 113.1239096053143527 ) ) ;
#119200=CARTESIAN_POINT ( 'NONE',  ( -16.53943276465976808, -0.05219959533934237506, 78.75109039468568994 ) ) ;
#119201=CARTESIAN_POINT ( 'NONE',  ( -15.72974639402197994, 15.80617190586746368, 100.6239096053143811 ) ) ;
#119202=CARTESIAN_POINT ( 'NONE',  ( 9.564922557960805705, 16.46253265017160317, 64.58224293864769550 ) ) ;
#119203=CARTESIAN_POINT ( 'NONE',  ( -10.81492255796105439, 18.62759615963255655, 37.91775706135235424 ) ) ;
#119204=CARTESIAN_POINT ( 'NONE',  ( -5.153800228976328057, -19.02544592524343514, 97.29057627198099567 ) ) ;
#119207=CARTESIAN_POINT ( 'NONE',  ( -5.823673210054431948, 21.52544592524334988, 37.70942372801900433 ) ) ;
#119208=CARTESIAN_POINT ( 'NONE',  ( 13.97604488694527802, 13.89961937509977652, 24.37390960531435624 ) ) ;
#119209=CARTESIAN_POINT ( 'NONE',  ( -9.564922557961040184, 16.46253265017147172, 92.91775706135233293 ) ) ;
#119210=CARTESIAN_POINT ( 'NONE',  ( -16.46253265017146816, -9.564922557961047289, 34.16775706135233293 ) ) ;
#119211=CARTESIAN_POINT ( 'NONE',  ( 5.719274019375991003, -21.55341960407610458, 112.7072429386476955 ) ) ;
#119212=CARTESIAN_POINT ( 'NONE',  ( -9.564922557961040184, 16.46253265017147172, 27.91775706135232582 ) ) ;
#119213=CARTESIAN_POINT ( 'NONE',  ( -13.89961937509957401, -13.97604488694547875, 54.37609039468565442 ) ) ;
#119214=CARTESIAN_POINT ( 'NONE',  ( -0.05219959533934338120, 16.53943276465976808, 87.50109039468568994 ) ) ;
#119216=CARTESIAN_POINT ( 'NONE',  ( -5.153800228976328057, -19.02544592524343514, 77.29057627198099567 ) ) ;
#119217=CARTESIAN_POINT ( 'NONE',  ( -21.53943276465977519, -0.05219959533937600094, 73.75109039468567573 ) ) ;
#119218=CARTESIAN_POINT ( 'NONE',  ( -15.80617190586768217, 15.72974639402176855, 98.12609039468570415 ) ) ;
#119220=CARTESIAN_POINT ( 'NONE',  ( -13.97604488694527625, -13.89961937509977652, 86.87390960531436690 ) ) ;
#119221=CARTESIAN_POINT ( 'NONE',  ( 15.80617190586769283, -15.72974639402175789, 60.62609039468567573 ) ) ;
#119222=CARTESIAN_POINT ( 'NONE',  ( 16.46253265017146816, 9.564922557961045513, 101.6677570613523329 ) ) ;
#119224=CARTESIAN_POINT ( 'NONE',  ( 5.153800228976335163, 19.02544592524342804, 59.79057627198100988 ) ) ;
#119225=CARTESIAN_POINT ( 'NONE',  ( 19.05341960407611168, 5.049401038298154454, 113.9572429386477097 ) ) ;
#119226=CARTESIAN_POINT ( 'NONE',  ( 19.03943276465977164, -0.05219959533909143690, 83.74890960531436690 ) ) ;
#119227=CARTESIAN_POINT ( 'NONE',  ( -18.22780087662123094, -5.499999999999984901, 76.48459894673894155 ) ) ;
#119228=CARTESIAN_POINT ( 'NONE',  ( 16.51473224551069308, 9.474510206698969483, 64.16557627198102409 ) ) ;
#119229=CARTESIAN_POINT ( 'NONE',  ( -19.03943276465977164, 0.05219959533909376836, 51.24890960531436690 ) ) ;
#119230=CARTESIAN_POINT ( 'NONE',  ( 0.05219959533937995610, -21.53943276465977519, 20.00109039468568639 ) ) ;
#119231=CARTESIAN_POINT ( 'NONE',  ( -4.483927247898782831, 16.52544592524335698, 92.70942372801901854 ) ) ;
#119232=CARTESIAN_POINT ( 'NONE',  ( -18.89770734986051437, -5.499999999999909406, 39.10214472496640781 ) ) ;
#119234=CARTESIAN_POINT ( 'NONE',  ( -16.51473224551082808, 9.474510206698731452, 58.33442372801900433 ) ) ;
#119235=CARTESIAN_POINT ( 'NONE',  ( -5.049401038298153566, 19.05341960407611168, 75.20724293864769550 ) ) ;
#119236=CARTESIAN_POINT ( 'NONE',  ( 16.55341960407611168, 4.379528057220329451, 68.95724293864769550 ) ) ;
#119237=CARTESIAN_POINT ( 'NONE',  ( -4.483927247898539470, -16.52544592524342804, 102.2905762719810383 ) ) ;
#119238=CARTESIAN_POINT ( 'NONE',  ( 13.97604488694527802, 13.89961937509977652, 109.3739096053143669 ) ) ;
#119239=CARTESIAN_POINT ( 'NONE',  ( 19.03943276465977164, -0.05219959533909143690, 108.7489096053143527 ) ) ;
#119240=CARTESIAN_POINT ( 'NONE',  ( 16.55341960407611168, 4.379528057220329451, 88.95724293864769550 ) ) ;
#119241=CARTESIAN_POINT ( 'NONE',  ( -17.59860650958991002, -7.585241751807008548, 81.57662985737506744 ) ) ;
#119242=CARTESIAN_POINT ( 'NONE',  ( -13.97604488694547697, 13.89961937509957934, 33.12609039468566863 ) ) ;
#119243=CARTESIAN_POINT ( 'NONE',  ( 16.52544592524335698, 4.483927247898782831, 101.4594237280190185 ) ) ;
#119244=CARTESIAN_POINT ( 'NONE',  ( -13.97604488694527625, -13.89961937509977652, 91.87390960531432427 ) ) ;
#119245=CARTESIAN_POINT ( 'NONE',  ( -5.719274019375665041, -21.55341960407619695, 59.79275706135234714 ) ) ;
#119246=CARTESIAN_POINT ( 'NONE',  ( -0.05219959533907301413, -21.53943276465977519, 47.49890960531435979 ) ) ;
#119247=CARTESIAN_POINT ( 'NONE',  ( -18.67979575497193778, 10.72451020669871902, 23.33442372801901499 ) ) ;
#119248=CARTESIAN_POINT ( 'NONE',  ( -15.72974639402197994, 15.80617190586746368, 75.62390960531439532 ) ) ;
#119249=CARTESIAN_POINT ( 'NONE',  ( 14.29746914071049879, -8.314922557960816363, 98.33224293864769550 ) ) ;
#119250=CARTESIAN_POINT ( 'NONE',  ( 9.474510206698729675, 16.51473224551082808, 52.08442372801900433 ) ) ;
#119251=CARTESIAN_POINT ( 'NONE',  ( 13.89961937509977652, -13.97604488694527269, 28.12390960531435624 ) ) ;
#119252=CARTESIAN_POINT ( 'NONE',  ( -19.05341960407611168, -5.049401038298163336, 86.45724293864769550 ) ) ;
#119253=CARTESIAN_POINT ( 'NONE',  ( 5.049401038298161559, -19.05341960407611168, 97.70724293864766707 ) ) ;
#119254=CARTESIAN_POINT ( 'NONE',  ( -12.06949235617756955, 12.14591786802309770, 115.6239096053143669 ) ) ;
#119255=CARTESIAN_POINT ( 'NONE',  ( -16.53943276465976808, 0.05219959533911058130, 21.24890960531436690 ) ) ;
#119256=CARTESIAN_POINT ( 'NONE',  ( -12.06949235617739369, -12.14591786802326823, 34.37609039468568284 ) ) ;
#119257=CARTESIAN_POINT ( 'NONE',  ( -10.81492255796105439, 18.62759615963255655, 107.9177570613523471 ) ) ;
#119258=CARTESIAN_POINT ( 'NONE',  ( -13.89961937509977652, 13.97604488694528158, 100.6239096053143669 ) ) ;
#119259=CARTESIAN_POINT ( 'NONE',  ( 21.53943276465977519, 0.05219959533937863772, 31.25109039468568639 ) ) ;
#119260=CARTESIAN_POINT ( 'NONE',  ( -9.474510206698964154, 16.51473224551069663, 50.41557627198102409 ) ) ;
#119261=CARTESIAN_POINT ( 'NONE',  ( 16.52544592524335698, 4.483927247898782831, 41.45942372801901143 ) ) ;
#119262=CARTESIAN_POINT ( 'NONE',  ( -4.483927247898782831, 16.52544592524335698, 112.7094237280190328 ) ) ;
#119263=CARTESIAN_POINT ( 'NONE',  ( -16.52544592524335698, -4.483927247898792601, 88.95942372801901854 ) ) ;
#119264=CARTESIAN_POINT ( 'NONE',  ( -19.03943276465977164, -0.05219959533935918106, 108.7510903946856615 ) ) ;
#119265=CARTESIAN_POINT ( 'NONE',  ( -13.89961937509977652, 13.97604488694528158, 30.62390960531435269 ) ) ;
#119266=CARTESIAN_POINT ( 'NONE',  ( 16.55341960407611168, 4.379528057220329451, 98.95724293864770971 ) ) ;
#119267=CARTESIAN_POINT ( 'NONE',  ( -10.72451020669898014, 18.67979575497178502, 100.4155762719810241 ) ) ;
#119268=CARTESIAN_POINT ( 'NONE',  ( 16.51473224551069308, 9.474510206698969483, 29.16557627198103475 ) ) ;
#119269=CARTESIAN_POINT ( 'NONE',  ( -13.97604488694527625, -13.89961937509977652, 111.8739096053143243 ) ) ;
#119270=CARTESIAN_POINT ( 'NONE',  ( -21.55341960407619339, 5.719274019375674811, 33.54275706135234714 ) ) ;
#119271=CARTESIAN_POINT ( 'NONE',  ( 19.05341960407611168, 5.049401038298154454, 23.95724293864769194 ) ) ;
#119272=CARTESIAN_POINT ( 'NONE',  ( -16.46253265017160317, 9.564922557960807481, 100.8322429386477097 ) ) ;
#119274=CARTESIAN_POINT ( 'NONE',  ( -9.564922557960796823, -16.46253265017161027, 87.08224293864769550 ) ) ;
#119275=CARTESIAN_POINT ( 'NONE',  ( 21.55341960407619695, -5.719274019375665929, 36.04275706135234714 ) ) ;
#119276=CARTESIAN_POINT ( 'NONE',  ( 14.29746914071049879, -8.314922557960816363, 88.33224293864769550 ) ) ;
#119277=CARTESIAN_POINT ( 'NONE',  ( 19.05341960407611168, 5.049401038298154454, 93.95724293864769550 ) ) ;
#119278=CARTESIAN_POINT ( 'NONE',  ( -19.02544592524334988, -5.153800228976617603, 23.95942372801900078 ) ) ;
#119279=CARTESIAN_POINT ( 'NONE',  ( 0.05219959533934541429, -16.53943276465976808, 65.00109039468568994 ) ) ;
#119280=CARTESIAN_POINT ( 'NONE',  ( 18.67979575497194134, -10.72451020669871369, 75.83442372801900433 ) ) ;
#119281=CARTESIAN_POINT ( 'NONE',  ( 4.483927247898790824, -16.52544592524335698, 45.20942372801901854 ) ) ;
#119282=CARTESIAN_POINT ( 'NONE',  ( 19.02544592524343514, -5.153800228976328945, 78.54057627198099567 ) ) ;
#119283=CARTESIAN_POINT ( 'NONE',  ( -9.564922557961040184, 16.46253265017147172, 97.91775706135233293 ) ) ;
#119284=CARTESIAN_POINT ( 'NONE',  ( -4.379528057220086978, -16.55341960407618274, 69.79275706135234714 ) ) ;
#119285=CARTESIAN_POINT ( 'NONE',  ( 10.72451020669871369, 18.67979575497193778, 112.0844237280190185 ) ) ;
#119286=CARTESIAN_POINT ( 'NONE',  ( -16.46253265017146816, -9.564922557961047289, 84.16775706135233293 ) ) ;
#119287=CARTESIAN_POINT ( 'NONE',  ( -19.05341960407611168, -5.049401038298163336, 61.45724293864769550 ) ) ;
#119288=CARTESIAN_POINT ( 'NONE',  ( -15.72974639402197994, 15.80617190586746368, 80.62390960531438111 ) ) ;
#119289=CARTESIAN_POINT ( 'NONE',  ( 8.314922557960818139, 14.29746914071049879, 74.58224293864768129 ) ) ;
#119290=CARTESIAN_POINT ( 'NONE',  ( 5.049401038297881783, 19.05341960407617563, 92.29275706135234714 ) ) ;
#119291=CARTESIAN_POINT ( 'NONE',  ( 16.55341960407618274, -4.379528057220086978, 56.04275706135235424 ) ) ;
#119293=CARTESIAN_POINT ( 'NONE',  ( 9.564922557961047289, -16.46253265017146816, 60.41775706135233293 ) ) ;
#119294=CARTESIAN_POINT ( 'NONE',  ( -8.314922557961024197, 14.29746914071037800, 112.9177570613523329 ) ) ;
#119295=CARTESIAN_POINT ( 'NONE',  ( -4.379528057220328563, 16.55341960407611168, 80.20724293864769550 ) ) ;
#119296=CARTESIAN_POINT ( 'NONE',  ( -19.03943276465977164, -0.05219959533935918106, 18.75109039468567218 ) ) ;
#119297=CARTESIAN_POINT ( 'NONE',  ( -16.79531203550682150, 7.028104445595347194, 38.74755011779544134 ) ) ;
#119298=CARTESIAN_POINT ( 'NONE',  ( -21.53943276465977519, 0.05219959533907696930, 106.2489096053143811 ) ) ;
#119299=CARTESIAN_POINT ( 'NONE',  ( -13.97604488694527625, -13.89961937509977652, 101.8739096053143811 ) ) ;
#119300=CARTESIAN_POINT ( 'NONE',  ( -0.05219959533909027116, -19.03943276465977164, 82.49890960531436690 ) ) ;
#119301=CARTESIAN_POINT ( 'NONE',  ( 18.62759615963255655, 10.81492255796105972, 86.66775706135234714 ) ) ;
#119302=CARTESIAN_POINT ( 'NONE',  ( 16.46253265017160672, -9.564922557960803928, 58.33224293864769550 ) ) ;
#119303=CARTESIAN_POINT ( 'NONE',  ( 10.72451020669898902, -18.67979575497178502, 27.91557627198103830 ) ) ;
#119304=CARTESIAN_POINT ( 'NONE',  ( 14.34966873604960469, 8.224510206698951720, 74.16557627198102409 ) ) ;
#119305=CARTESIAN_POINT ( 'NONE',  ( -5.153800228976328057, -19.02544592524343514, 37.29057627198102409 ) ) ;
#119306=CARTESIAN_POINT ( 'NONE',  ( -14.34966873604960291, -8.224510206698953496, 96.66557627198102409 ) ) ;
#119307=CARTESIAN_POINT ( 'NONE',  ( 21.55341960407610458, 5.719274019375980345, 103.9572429386476813 ) ) ;
#119308=CARTESIAN_POINT ( 'NONE',  ( -5.719274019375665041, -21.55341960407619695, 54.79275706135235424 ) ) ;
#119309=CARTESIAN_POINT ( 'NONE',  ( 5.049401038298161559, -19.05341960407611168, 32.70724293864768129 ) ) ;
#119310=CARTESIAN_POINT ( 'NONE',  ( 8.314922557961029526, -14.29746914071037800, 65.41775706135234714 ) ) ;
#119311=CARTESIAN_POINT ( 'NONE',  ( -15.72974639402197994, 15.80617190586746368, 105.6239096053143669 ) ) ;
#119312=CARTESIAN_POINT ( 'NONE',  ( -10.81492255796078084, -18.62759615963271287, 97.08224293864770971 ) ) ;
#119313=CARTESIAN_POINT ( 'NONE',  ( 9.564922557961047289, -16.46253265017146816, 35.41775706135233293 ) ) ;
#119314=CARTESIAN_POINT ( 'NONE',  ( -9.474510206698964154, 16.51473224551069663, 50.41557627198102409 ) ) ;
#119315=CARTESIAN_POINT ( 'NONE',  ( -19.02544592524342804, 5.153800228976336051, 116.0405762719810383 ) ) ;
#119316=CARTESIAN_POINT ( 'NONE',  ( -18.62759615963255300, -10.81492255796106328, 54.16775706135235424 ) ) ;
#119317=CARTESIAN_POINT ( 'NONE',  ( 18.62759615963271287, -10.81492255796078972, 63.33224293864770260 ) ) ;
#119318=CARTESIAN_POINT ( 'NONE',  ( -16.53943276465976808, 0.05219959533911058130, 31.24890960531435979 ) ) ;
#119319=CARTESIAN_POINT ( 'NONE',  ( -10.81492255796105439, 18.62759615963255655, 82.91775706135234714 ) ) ;
#119320=CARTESIAN_POINT ( 'NONE',  ( 5.719274019375673035, 21.55341960407619339, 112.2927570613523471 ) ) ;
#119321=CARTESIAN_POINT ( 'NONE',  ( 0.05219959533910956823, 16.53943276465976808, 59.99890960531436690 ) ) ;
#119322=CARTESIAN_POINT ( 'NONE',  ( 8.314922557960818139, 14.29746914071049879, 109.5822429386476955 ) ) ;
#119323=CARTESIAN_POINT ( 'NONE',  ( -13.97604488694547697, 13.89961937509957934, 38.12609039468566152 ) ) ;
#119324=CARTESIAN_POINT ( 'NONE',  ( 16.55341960407618274, -4.379528057220086978, 96.04275706135236135 ) ) ;
#119325=CARTESIAN_POINT ( 'NONE',  ( -15.72974639402176322, -15.80617190586768395, 69.37609039468567573 ) ) ;
#119326=ADVANCED_FACE ( 'NONE', ( #171567, #33056, #94711 ), #17893, .T. ) ;
#119327=CARTESIAN_POINT ( 'NONE',  ( -0.05219959533909027116, -19.03943276465977164, 62.49890960531435979 ) ) ;
#119328=CARTESIAN_POINT ( 'NONE',  ( 19.05341960407617918, -5.049401038297876454, 31.04275706135232227 ) ) ;
#119329=CARTESIAN_POINT ( 'NONE',  ( 21.52544592524344225, -5.823673210054117533, 38.54057627198103120 ) ) ;
#119330=CARTESIAN_POINT ( 'NONE',  ( 5.719274019375673035, 21.55341960407619339, 37.29275706135235424 ) ) ;
#119331=CARTESIAN_POINT ( 'NONE',  ( 18.62759615963271287, -10.81492255796078972, 88.33224293864769550 ) ) ;
#119332=CARTESIAN_POINT ( 'NONE',  ( -19.02544592524334988, -5.153800228976617603, 83.95942372801901854 ) ) ;
#119333=CARTESIAN_POINT ( 'NONE',  ( 4.483927247898790824, -16.52544592524335698, 55.20942372801902565 ) ) ;
#119334=CARTESIAN_POINT ( 'NONE',  ( 17.50000000000000000, -5.499999999999992895, 36.21769037696435589 ) ) ;
#119335=CARTESIAN_POINT ( 'NONE',  ( -18.62759615963270932, 10.81492255796079327, 95.83224293864770971 ) ) ;
#119336=CARTESIAN_POINT ( 'NONE',  ( 16.53943276465976808, 0.05219959533934440121, 76.25109039468568994 ) ) ;
#119337=CARTESIAN_POINT ( 'NONE',  ( -16.55341960407611168, -4.379528057220339221, 71.45724293864769550 ) ) ;
#119339=CARTESIAN_POINT ( 'NONE',  ( -8.224510206698735004, -14.34966873604973081, 24.58442372801901499 ) ) ;
#119340=CARTESIAN_POINT ( 'NONE',  ( 10.81492255796078972, 18.62759615963270932, 39.58224293864769550 ) ) ;
#119341=CARTESIAN_POINT ( 'NONE',  ( 12.14591786802327356, -12.06949235617739191, 75.62609039468567573 ) ) ;
#119344=CARTESIAN_POINT ( 'NONE',  ( 14.34966873604972726, -8.224510206698740333, 50.83442372801901143 ) ) ;
#119345=CARTESIAN_POINT ( 'NONE',  ( 5.719274019375673035, 21.55341960407619339, 27.29275706135234358 ) ) ;
#119346=CARTESIAN_POINT ( 'NONE',  ( -5.823673210054116645, -21.52544592524344225, 42.29057627198103120 ) ) ;
#119347=CARTESIAN_POINT ( 'NONE',  ( -8.224510206698735004, -14.34966873604973081, 64.58442372801900433 ) ) ;
#119348=CARTESIAN_POINT ( 'NONE',  ( -19.02544592524342804, 5.153800228976336051, 86.04057627198103830 ) ) ;
#119349=CARTESIAN_POINT ( 'NONE',  ( 15.80617190586769283, -15.72974639402175789, 60.62609039468567573 ) ) ;
#119350=CARTESIAN_POINT ( 'NONE',  ( -0.05219959533909027116, -19.03943276465977164, 27.49890960531435624 ) ) ;
#119351=CARTESIAN_POINT ( 'NONE',  ( -18.67979575497178146, -10.72451020669898902, 36.66557627198103120 ) ) ;
#119353=CARTESIAN_POINT ( 'NONE',  ( -19.03943276465977164, -0.05219959533935918106, 43.75109039468566863 ) ) ;
#119354=CARTESIAN_POINT ( 'NONE',  ( 12.14591786802327356, -12.06949235617739191, 50.62609039468568994 ) ) ;
#119355=CARTESIAN_POINT ( 'NONE',  ( -18.62759615963270932, 10.81492255796079327, 25.83224293864769194 ) ) ;
#119356=ORIENTED_EDGE ( 'NONE', *, *, #82183, .T. ) ;
#119357=CARTESIAN_POINT ( 'NONE',  ( 19.05341960407611168, 5.049401038298154454, 88.95724293864769550 ) ) ;
#119358=CARTESIAN_POINT ( 'NONE',  ( 16.52544592524335698, 4.483927247898782831, 106.4594237280190328 ) ) ;
#119360=CARTESIAN_POINT ( 'NONE',  ( -16.52544592524342804, 4.483927247898546575, 101.0405762719810383 ) ) ;
#119361=CARTESIAN_POINT ( 'NONE',  ( -18.62759615963270932, 10.81492255796079327, 30.83224293864770260 ) ) ;
#119362=CARTESIAN_POINT ( 'NONE',  ( -19.05341960407611168, -5.049401038298163336, 26.45724293864769550 ) ) ;
#119363=CARTESIAN_POINT ( 'NONE',  ( 16.55341960407618274, -4.379528057220086978, 76.04275706135237556 ) ) ;
#119364=CARTESIAN_POINT ( 'NONE',  ( -18.62759615963255300, -10.81492255796106328, 19.16775706135234714 ) ) ;
#119365=CARTESIAN_POINT ( 'NONE',  ( 13.89961937509957401, 13.97604488694547697, 71.87609039468567573 ) ) ;
#119366=CARTESIAN_POINT ( 'NONE',  ( 0.05219959533909260263, 19.03943276465977164, 34.99890960531435979 ) ) ;
#119368=CARTESIAN_POINT ( 'NONE',  ( -9.564922557960796823, -16.46253265017161027, 112.0822429386476955 ) ) ;
#119369=CARTESIAN_POINT ( 'NONE',  ( -5.823673210054431948, 21.52544592524334988, 107.7094237280190328 ) ) ;
#119370=CARTESIAN_POINT ( 'NONE',  ( -9.564922557960796823, -16.46253265017161027, 67.08224293864769550 ) ) ;
#119371=CARTESIAN_POINT ( 'NONE',  ( -16.52544592524335698, -4.483927247898792601, 53.95942372801900433 ) ) ;
#119372=CARTESIAN_POINT ( 'NONE',  ( -15.72974639402176322, -15.80617190586768395, 94.37609039468568994 ) ) ;
#119373=CARTESIAN_POINT ( 'NONE',  ( -13.97604488694547697, 13.89961937509957934, 58.12609039468566863 ) ) ;
#119374=EDGE_CURVE ( 'NONE', #179892, #66839, #164922, .T. ) ;
#119375=CARTESIAN_POINT ( 'NONE',  ( 19.03943276465977164, 0.05219959533936151252, 51.25109039468567573 ) ) ;
#119377=CARTESIAN_POINT ( 'NONE',  ( 21.52544592524334988, 5.823673210054432836, 46.45942372801901854 ) ) ;
#119378=CARTESIAN_POINT ( 'NONE',  ( -18.22780087662119897, 5.500000000000102141, 56.01763182126894947 ) ) ;
#119379=CARTESIAN_POINT ( 'NONE',  ( -9.474510206698720793, -16.51473224551083518, 39.58442372801899722 ) ) ;
#119380=CARTESIAN_POINT ( 'NONE',  ( -5.049401038298153566, 19.05341960407611168, 95.20724293864770971 ) ) ;
#119381=CARTESIAN_POINT ( 'NONE',  ( 9.564922557960805705, 16.46253265017160317, 84.58224293864769550 ) ) ;
#119382=CARTESIAN_POINT ( 'NONE',  ( -16.52544592524342804, 4.483927247898546575, 41.04057627198103120 ) ) ;
#119383=CARTESIAN_POINT ( 'NONE',  ( 5.719274019375991003, -21.55341960407610458, 27.70724293864769905 ) ) ;
#119386=CARTESIAN_POINT ( 'NONE',  ( -10.81492255796105439, 18.62759615963255655, 112.9177570613523329 ) ) ;
#119388=CARTESIAN_POINT ( 'NONE',  ( -16.46253265017160317, 9.564922557960807481, 30.83224293864769550 ) ) ;
#119389=CARTESIAN_POINT ( 'NONE',  ( -0.05219959533909027116, -19.03943276465977164, 27.49890960531435624 ) ) ;
#119392=CARTESIAN_POINT ( 'NONE',  ( 0.05219959533934541429, -16.53943276465976808, 60.00109039468568284 ) ) ;
#119393=CARTESIAN_POINT ( 'NONE',  ( -5.823673210054116645, -21.52544592524344225, 82.29057627198103830 ) ) ;
#119394=CARTESIAN_POINT ( 'NONE',  ( 8.224510206698953496, -14.34966873604960469, 42.91557627198103120 ) ) ;
#119395=CARTESIAN_POINT ( 'NONE',  ( -13.89961937509977652, 13.97604488694528158, 30.62390960531435269 ) ) ;
#119396=CARTESIAN_POINT ( 'NONE',  ( -16.46253265017160317, 9.564922557960807481, 110.8322429386476955 ) ) ;
#119397=CARTESIAN_POINT ( 'NONE',  ( -21.55341960407619339, 5.719274019375674811, 33.54275706135234714 ) ) ;
#119398=CARTESIAN_POINT ( 'NONE',  ( 9.564922557961047289, -16.46253265017146816, 30.41775706135232937 ) ) ;
#119399=CARTESIAN_POINT ( 'NONE',  ( 5.153800228976335163, 19.02544592524342804, 34.79057627198102409 ) ) ;
#119400=CARTESIAN_POINT ( 'NONE',  ( -15.80617190586768217, 15.72974639402176855, 78.12609039468570415 ) ) ;
#119401=CARTESIAN_POINT ( 'NONE',  ( 16.52216118717208815, -7.221426719304489872, 31.42400978953010338 ) ) ;
#119402=CARTESIAN_POINT ( 'NONE',  ( -14.29746914071049879, 8.314922557960819915, 30.83224293864770260 ) ) ;
#119404=CARTESIAN_POINT ( 'NONE',  ( -21.52544592524343514, 5.823673210054127303, 31.04057627198102409 ) ) ;
#119405=CARTESIAN_POINT ( 'NONE',  ( 16.52544592524342804, -4.483927247898539470, 108.5405762719810241 ) ) ;
#119407=CARTESIAN_POINT ( 'NONE',  ( 16.51473224551069308, 9.474510206698969483, 84.16557627198102409 ) ) ;
#119408=CARTESIAN_POINT ( 'NONE',  ( 16.53943276465976808, -0.05219959533910856209, 78.74890960531436690 ) ) ;
#119409=CARTESIAN_POINT ( 'NONE',  ( 5.153800228976615827, -19.02544592524334988, 100.2094237280190043 ) ) ;
#119410=CARTESIAN_POINT ( 'NONE',  ( 10.72451020669898902, -18.67979575497178502, 57.91557627198103120 ) ) ;
#119412=CARTESIAN_POINT ( 'NONE',  ( 13.97604488694527802, 13.89961937509977652, 39.37390960531435269 ) ) ;
#119413=CARTESIAN_POINT ( 'NONE',  ( -9.564922557960796823, -16.46253265017161027, 82.08224293864768129 ) ) ;
#119414=CARTESIAN_POINT ( 'NONE',  ( 5.719274019375991003, -21.55341960407610458, 92.70724293864770971 ) ) ;
#119415=CARTESIAN_POINT ( 'NONE',  ( 0.05219959533934541429, -16.53943276465976808, 100.0010903946857042 ) ) ;
#119416=CARTESIAN_POINT ( 'NONE',  ( 9.474510206698971260, -16.51473224551069308, 92.91557627198103830 ) ) ;
#119417=CARTESIAN_POINT ( 'NONE',  ( -19.05341960407617563, 5.049401038297882671, 78.54275706135233293 ) ) ;
#119418=CARTESIAN_POINT ( 'NONE',  ( -21.55341960407619339, 5.719274019375674811, 88.54275706135236135 ) ) ;
#119419=CARTESIAN_POINT ( 'NONE',  ( 18.67979575497178502, 10.72451020669898547, 79.16557627198103830 ) ) ;
#119420=CARTESIAN_POINT ( 'NONE',  ( 15.72974639402199770, -15.80617190586745480, 33.12390960531435979 ) ) ;
#119421=CARTESIAN_POINT ( 'NONE',  ( -19.05341960407611168, -5.049401038298163336, 56.45724293864768129 ) ) ;
#119422=CARTESIAN_POINT ( 'NONE',  ( 16.55341960407611168, 4.379528057220329451, 23.95724293864769550 ) ) ;
#119423=CARTESIAN_POINT ( 'NONE',  ( 9.564922557960805705, 16.46253265017160317, 59.58224293864769550 ) ) ;
#119425=CARTESIAN_POINT ( 'NONE',  ( -16.46253265017146816, -9.564922557961047289, 34.16775706135233293 ) ) ;
#119426=CARTESIAN_POINT ( 'NONE',  ( -14.34966873604960291, -8.224510206698953496, 71.66557627198100988 ) ) ;
#119427=CARTESIAN_POINT ( 'NONE',  ( 5.719274019375991003, -21.55341960407610458, 112.7072429386476955 ) ) ;
#119428=CARTESIAN_POINT ( 'NONE',  ( 0.05219959533937995610, -21.53943276465977519, 20.00109039468568639 ) ) ;
#119430=CARTESIAN_POINT ( 'NONE',  ( -21.52544592524343514, 5.823673210054127303, 61.04057627198103120 ) ) ;
#119431=CARTESIAN_POINT ( 'NONE',  ( 8.224510206698742110, 14.34966873604972548, 97.08442372801904696 ) ) ;
#119432=CARTESIAN_POINT ( 'NONE',  ( 14.29746914071049879, -8.314922557960816363, 108.3322429386477097 ) ) ;
#119433=CARTESIAN_POINT ( 'NONE',  ( -0.05219959533909027116, -19.03943276465977164, 57.49890960531435979 ) ) ;
#119434=CARTESIAN_POINT ( 'NONE',  ( 0.05219959533910956823, 16.53943276465976808, 29.99890960531435979 ) ) ;
#119435=CARTESIAN_POINT ( 'NONE',  ( -21.52544592524334988, -5.823673210054445271, 43.95942372801902565 ) ) ;
#119436=CARTESIAN_POINT ( 'NONE',  ( -9.564922557960796823, -16.46253265017161027, 107.0822429386476955 ) ) ;
#119437=CARTESIAN_POINT ( 'NONE',  ( 0.05219959533937995610, -21.53943276465977519, 80.00109039468568994 ) ) ;
#119438=CARTESIAN_POINT ( 'NONE',  ( 19.02544592524343514, -5.153800228976328945, 28.54057627198102409 ) ) ;
#119439=CARTESIAN_POINT ( 'NONE',  ( 16.46253265017160672, -9.564922557960803928, 38.33224293864768839 ) ) ;
#119441=CARTESIAN_POINT ( 'NONE',  ( 21.53943276465977519, 0.05219959533937863772, 81.25109039468568994 ) ) ;
#119442=CARTESIAN_POINT ( 'NONE',  ( -16.55341960407617563, 4.379528057220093196, 53.54275706135234714 ) ) ;
#119443=CARTESIAN_POINT ( 'NONE',  ( -10.72451020669870658, -18.67979575497194134, 69.58442372801900433 ) ) ;
#119444=CARTESIAN_POINT ( 'NONE',  ( -19.05341960407611168, -5.049401038298163336, 106.4572429386476955 ) ) ;
#119445=CARTESIAN_POINT ( 'NONE',  ( -9.564922557961040184, 16.46253265017147172, 82.91775706135233293 ) ) ;
#119446=CARTESIAN_POINT ( 'NONE',  ( 21.55341960407619695, -5.719274019375665929, 61.04275706135234714 ) ) ;
#119447=CARTESIAN_POINT ( 'NONE',  ( -16.55341960407617563, 4.379528057220093196, 28.54275706135234358 ) ) ;
#119448=CARTESIAN_POINT ( 'NONE',  ( -0.05219959533936034679, 19.03943276465977164, 72.50109039468566152 ) ) ;
#119449=CARTESIAN_POINT ( 'NONE',  ( -9.474510206698964154, 16.51473224551069663, 55.41557627198103120 ) ) ;
#119450=CARTESIAN_POINT ( 'NONE',  ( -19.05341960407617563, 5.049401038297882671, 88.54275706135230450 ) ) ;
#119451=CARTESIAN_POINT ( 'NONE',  ( -14.29746914071049879, 8.314922557960819915, 30.83224293864770260 ) ) ;
#119452=CARTESIAN_POINT ( 'NONE',  ( -19.03943276465977164, -0.05219959533935918106, 93.75109039468566152 ) ) ;
#119453=CARTESIAN_POINT ( 'NONE',  ( -4.379528057220328563, 16.55341960407611168, 35.20724293864768839 ) ) ;
#119455=CARTESIAN_POINT ( 'NONE',  ( 13.89961937509957401, 13.97604488694547697, 61.87609039468566863 ) ) ;
#119456=CARTESIAN_POINT ( 'NONE',  ( -4.379528057220086978, -16.55341960407618274, 49.79275706135234714 ) ) ;
#119457=CARTESIAN_POINT ( 'NONE',  ( 13.89961937509957401, 13.97604488694547697, 21.87609039468566152 ) ) ;
#119458=CARTESIAN_POINT ( 'NONE',  ( -5.049401038298153566, 19.05341960407611168, 45.20724293864769550 ) ) ;
#119459=CARTESIAN_POINT ( 'NONE',  ( 16.55341960407618274, -4.379528057220086978, 41.04275706135236135 ) ) ;
#119462=CARTESIAN_POINT ( 'NONE',  ( -19.02544592524342804, 5.153800228976336051, 86.04057627198103830 ) ) ;
#119465=CARTESIAN_POINT ( 'NONE',  ( 13.89961937509957401, 13.97604488694547697, 91.87609039468567573 ) ) ;
#119466=VECTOR ( 'NONE', #30832, 1000.000000000000000 ) ;
#119467=CARTESIAN_POINT ( 'NONE',  ( 21.52544592524344225, -5.823673210054117533, 23.54057627198102765 ) ) ;
#119468=CARTESIAN_POINT ( 'NONE',  ( -18.67979575497193778, 10.72451020669871902, 108.3344237280190185 ) ) ;
#119469=CARTESIAN_POINT ( 'NONE',  ( -19.05341960407617563, 5.049401038297882671, 113.5427570613523471 ) ) ;
#119470=CARTESIAN_POINT ( 'NONE',  ( -14.29746914071049879, 8.314922557960819915, 105.8322429386476955 ) ) ;
#119471=CARTESIAN_POINT ( 'NONE',  ( -16.51473224551069308, -9.474510206698971260, 41.66557627198103120 ) ) ;
#119472=CARTESIAN_POINT ( 'NONE',  ( -10.81492255796078084, -18.62759615963271287, 77.08224293864769550 ) ) ;
#119473=CARTESIAN_POINT ( 'NONE',  ( 16.46253265017160672, -9.564922557960803928, 43.33224293864769550 ) ) ;
#119474=CARTESIAN_POINT ( 'NONE',  ( -13.97604488694547520, 13.89961937509957934, 48.12609039468566863 ) ) ;
#119475=CARTESIAN_POINT ( 'NONE',  ( -9.564922557961040184, 16.46253265017147172, 67.91775706135233293 ) ) ;
#119476=CARTESIAN_POINT ( 'NONE',  ( 0.05219959533910956823, 16.53943276465976808, 59.99890960531436690 ) ) ;
#119477=CARTESIAN_POINT ( 'NONE',  ( -10.81492255796078084, -18.62759615963271287, 32.08224293864769550 ) ) ;
#119478=CARTESIAN_POINT ( 'NONE',  ( 18.62759615963255655, 10.81492255796105972, 96.66775706135234714 ) ) ;
#119479=CARTESIAN_POINT ( 'NONE',  ( 21.53943276465977519, -0.05219959533907433946, 88.74890960531436690 ) ) ;
#119480=CARTESIAN_POINT ( 'NONE',  ( 21.55341960407619695, -5.719274019375665929, 71.04275706135234714 ) ) ;
#119481=CARTESIAN_POINT ( 'NONE',  ( -21.52544592524334988, -5.823673210054445271, 68.95942372801901854 ) ) ;
#119483=CARTESIAN_POINT ( 'NONE',  ( -0.05219959533909027116, -19.03943276465977164, 102.4989096053143669 ) ) ;
#119484=CARTESIAN_POINT ( 'NONE',  ( -12.14591786802326823, 12.06949235617739902, 88.12609039468570415 ) ) ;
#119485=CARTESIAN_POINT ( 'NONE',  ( -21.55341960407619339, 5.719274019375674811, 68.54275706135234714 ) ) ;
#119486=CARTESIAN_POINT ( 'NONE',  ( -9.564922557960796823, -16.46253265017161027, 52.08224293864768839 ) ) ;
#119487=CARTESIAN_POINT ( 'NONE',  ( 16.51473224551069308, 9.474510206698969483, 29.16557627198103475 ) ) ;
#119488=CARTESIAN_POINT ( 'NONE',  ( -13.97604488694527625, -13.89961937509977652, 71.87390960531433848 ) ) ;
#119489=CARTESIAN_POINT ( 'NONE',  ( -16.53943276465976808, 0.05219959533911058130, 71.24890960531435269 ) ) ;
#119490=CARTESIAN_POINT ( 'NONE',  ( -14.34966873604960291, -8.224510206698953496, 36.66557627198103120 ) ) ;
#119491=CARTESIAN_POINT ( 'NONE',  ( -5.719274019375978568, 21.55341960407610458, 50.20724293864769550 ) ) ;
#119492=CARTESIAN_POINT ( 'NONE',  ( -16.51473224551069308, -9.474510206698971260, 41.66557627198103120 ) ) ;
#119493=CARTESIAN_POINT ( 'NONE',  ( 0.05219959533907565091, 21.53943276465977519, 64.99890960531435269 ) ) ;
#119494=CARTESIAN_POINT ( 'NONE',  ( -9.564922557961040184, 16.46253265017147172, 52.91775706135233293 ) ) ;
#119496=CARTESIAN_POINT ( 'NONE',  ( 14.29746914071049879, -8.314922557960816363, 63.33224293864770260 ) ) ;
#119497=CARTESIAN_POINT ( 'NONE',  ( 21.55341960407610458, 5.719274019375980345, 43.95724293864769550 ) ) ;
#119502=CARTESIAN_POINT ( 'NONE',  ( 16.53943276465976808, 0.05219959533934440121, 86.25109039468568994 ) ) ;
#119503=CARTESIAN_POINT ( 'NONE',  ( 16.51473224551083163, -9.474510206698727899, 80.83442372801899012 ) ) ;
#119504=CARTESIAN_POINT ( 'NONE',  ( 0.05219959533910956823, 16.53943276465976808, 49.99890960531437401 ) ) ;
#119506=CARTESIAN_POINT ( 'NONE',  ( 9.564922557960805705, 16.46253265017160317, 49.58224293864770260 ) ) ;
#119507=CARTESIAN_POINT ( 'NONE',  ( -8.224510206698948167, 14.34966873604960824, 35.41557627198102409 ) ) ;
#119508=CARTESIAN_POINT ( 'NONE',  ( 9.474510206698971260, -16.51473224551069308, 52.91557627198102409 ) ) ;
#119509=CARTESIAN_POINT ( 'NONE',  ( -0.05219959533909027116, -19.03943276465977164, 77.49890960531435269 ) ) ;
#119510=CARTESIAN_POINT ( 'NONE',  ( -0.05219959533909027116, -19.03943276465977164, 37.49890960531436690 ) ) ;
#119511=CARTESIAN_POINT ( 'NONE',  ( -0.05219959533937732626, 21.53943276465977519, 42.50109039468567573 ) ) ;
#119512=CARTESIAN_POINT ( 'NONE',  ( -5.049401038298153566, 19.05341960407611168, 70.20724293864769550 ) ) ;
#119513=CARTESIAN_POINT ( 'NONE',  ( 5.049401038298161559, -19.05341960407611168, 22.70724293864769194 ) ) ;
#119514=CARTESIAN_POINT ( 'NONE',  ( -5.049401038298153566, 19.05341960407611168, 65.20724293864765286 ) ) ;
#119515=CARTESIAN_POINT ( 'NONE',  ( -18.62759615963270932, 10.81492255796079327, 45.83224293864769550 ) ) ;
#119516=CARTESIAN_POINT ( 'NONE',  ( 19.03943276465977164, -0.05219959533909143690, 38.74890960531436690 ) ) ;
#119517=CARTESIAN_POINT ( 'NONE',  ( -10.81492255796078084, -18.62759615963271287, 42.08224293864769550 ) ) ;
#119518=CARTESIAN_POINT ( 'NONE',  ( 14.29746914071037800, 8.314922557961029526, 106.6677570613523756 ) ) ;
#119519=CARTESIAN_POINT ( 'NONE',  ( -19.05341960407617563, 5.049401038297882671, 28.54275706135232937 ) ) ;
#119520=CARTESIAN_POINT ( 'NONE',  ( -4.483927247898782831, 16.52544592524335698, 52.70942372801902565 ) ) ;
#119521=CARTESIAN_POINT ( 'NONE',  ( -16.55341960407617563, 4.379528057220093196, 78.54275706135236135 ) ) ;
#119523=CARTESIAN_POINT ( 'NONE',  ( -16.53943276465976808, -0.05219959533934237506, 63.75109039468568284 ) ) ;
#119524=CARTESIAN_POINT ( 'NONE',  ( -12.06949235617739369, -12.14591786802326823, 39.37609039468567573 ) ) ;
#119525=CARTESIAN_POINT ( 'NONE',  ( 9.564922557960805705, 16.46253265017160317, 104.5822429386476955 ) ) ;
#119526=CARTESIAN_POINT ( 'NONE',  ( 16.53943276465976808, 0.05219959533934440121, 41.25109039468568284 ) ) ;
#119527=CARTESIAN_POINT ( 'NONE',  ( -9.474510206698964154, 16.51473224551069663, 30.41557627198102054 ) ) ;
#119528=CARTESIAN_POINT ( 'NONE',  ( 0.05219959533937995610, -21.53943276465977519, 25.00109039468567218 ) ) ;
#119529=CARTESIAN_POINT ( 'NONE',  ( 16.55341960407618274, -4.379528057220086978, 31.04275706135234714 ) ) ;
#119530=CARTESIAN_POINT ( 'NONE',  ( -4.483927247898782831, 16.52544592524335698, 102.7094237280190185 ) ) ;
#119532=CARTESIAN_POINT ( 'NONE',  ( -21.53943276465977519, -0.05219959533937600094, 103.7510903946857042 ) ) ;
#119533=CARTESIAN_POINT ( 'NONE',  ( 19.03943276465977164, 0.05219959533936151252, 96.25109039468567573 ) ) ;
#119534=CARTESIAN_POINT ( 'NONE',  ( 4.483927247898545687, 16.52544592524342804, 59.79057627198103120 ) ) ;
#119535=CARTESIAN_POINT ( 'NONE',  ( -16.51473224551069308, -9.474510206698971260, 21.66557627198102765 ) ) ;
#119536=CARTESIAN_POINT ( 'NONE',  ( 13.89961937509957401, 13.97604488694547697, 66.87609039468567573 ) ) ;
#119537=CARTESIAN_POINT ( 'NONE',  ( 16.19135201231351218, -7.376712067592053224, 57.31319145947882987 ) ) ;
#119538=CARTESIAN_POINT ( 'NONE',  ( 0.05219959533937995610, -21.53943276465977519, 60.00109039468568284 ) ) ;
#119539=CARTESIAN_POINT ( 'NONE',  ( 0.05219959533934541429, -16.53943276465976808, 30.00109039468568284 ) ) ;
#119541=CARTESIAN_POINT ( 'NONE',  ( 19.03943276465977164, -0.05219959533909143690, 113.7489096053143669 ) ) ;
#119542=CARTESIAN_POINT ( 'NONE',  ( -5.719274019375978568, 21.55341960407610458, 75.20724293864769550 ) ) ;
#119543=CARTESIAN_POINT ( 'NONE',  ( 5.153800228976615827, -19.02544592524334988, 110.2094237280189901 ) ) ;
#119544=CARTESIAN_POINT ( 'NONE',  ( 9.564922557960805705, 16.46253265017160317, 104.5822429386476955 ) ) ;
#119546=CARTESIAN_POINT ( 'NONE',  ( -9.474510206698964154, 16.51473224551069663, 25.41557627198103120 ) ) ;
#119547=CARTESIAN_POINT ( 'NONE',  ( -21.53943276465977519, -0.05219959533937600094, 108.7510903946857042 ) ) ;
#119548=CARTESIAN_POINT ( 'NONE',  ( 5.153800228976335163, 19.02544592524342804, 44.79057627198103830 ) ) ;
#119549=CARTESIAN_POINT ( 'NONE',  ( -18.62759615963255300, -10.81492255796106328, 54.16775706135235424 ) ) ;
#119550=CARTESIAN_POINT ( 'NONE',  ( 18.62759615963255655, 10.81492255796105972, 96.66775706135234714 ) ) ;
#119551=CARTESIAN_POINT ( 'NONE',  ( -16.53943276465976808, -0.05219959533934237506, 108.7510903946857042 ) ) ;
#119552=CARTESIAN_POINT ( 'NONE',  ( 0.05219959533909260263, 19.03943276465977164, 84.99890960531436690 ) ) ;
#119553=CARTESIAN_POINT ( 'NONE',  ( -18.67979575497193778, 10.72451020669871902, 43.33442372801901143 ) ) ;
#119554=CARTESIAN_POINT ( 'NONE',  ( 15.80617190586769283, -15.72974639402175789, 55.62609039468568284 ) ) ;
#119555=CARTESIAN_POINT ( 'NONE',  ( 13.97604488694548053, -13.89961937509957401, 80.62609039468567573 ) ) ;
#119556=CARTESIAN_POINT ( 'NONE',  ( 9.474510206698971260, -16.51473224551069308, 87.91557627198102409 ) ) ;
#119557=CARTESIAN_POINT ( 'NONE',  ( 16.52544592524342804, -4.483927247898539470, 98.54057627198105251 ) ) ;
#119558=CARTESIAN_POINT ( 'NONE',  ( 0.05219959533907565091, 21.53943276465977519, 94.99890960531436690 ) ) ;
#119559=CARTESIAN_POINT ( 'NONE',  ( 15.72974639402176855, 15.80617190586768217, 111.8760903946856615 ) ) ;
#119560=CARTESIAN_POINT ( 'NONE',  ( -12.14591786802309592, -12.06949235617757132, 91.87390960531436690 ) ) ;
#119561=CARTESIAN_POINT ( 'NONE',  ( 19.05341960407611168, 5.049401038298154454, 48.95724293864768129 ) ) ;
#119562=CARTESIAN_POINT ( 'NONE',  ( 19.03943276465977164, 0.05219959533936151252, 81.25109039468567573 ) ) ;
#119563=CARTESIAN_POINT ( 'NONE',  ( 14.29746914071049879, -8.314922557960816363, 43.33224293864769550 ) ) ;
#119564=CARTESIAN_POINT ( 'NONE',  ( 15.72974639402176855, 15.80617190586768217, 101.8760903946857042 ) ) ;
#119565=CARTESIAN_POINT ( 'NONE',  ( 13.97604488694527802, 13.89961937509977652, 109.3739096053143669 ) ) ;
#119566=CARTESIAN_POINT ( 'NONE',  ( -9.474510206698720793, -16.51473224551083518, 69.58442372801901854 ) ) ;
#119567=CARTESIAN_POINT ( 'NONE',  ( 21.52544592524344225, -5.823673210054117533, 73.54057627198102409 ) ) ;
#119568=CARTESIAN_POINT ( 'NONE',  ( 18.67979575497194134, -10.72451020669871369, 35.83442372801901143 ) ) ;
#119569=CARTESIAN_POINT ( 'NONE',  ( 16.52544592524335698, 4.483927247898782831, 31.45942372801901854 ) ) ;
#119570=CARTESIAN_POINT ( 'NONE',  ( -8.224510206698735004, -14.34966873604973081, 94.58442372801901854 ) ) ;
#119571=CARTESIAN_POINT ( 'NONE',  ( 5.153800228976335163, 19.02544592524342804, 29.79057627198102409 ) ) ;
#119572=CARTESIAN_POINT ( 'NONE',  ( -18.67979575497193778, 10.72451020669871902, 38.33442372801900433 ) ) ;
#119573=CARTESIAN_POINT ( 'NONE',  ( 10.72451020669898902, -18.67979575497178502, 37.91557627198102409 ) ) ;
#119574=CARTESIAN_POINT ( 'NONE',  ( -13.97604488694527625, -13.89961937509977652, 21.87390960531435979 ) ) ;
#119576=CARTESIAN_POINT ( 'NONE',  ( 12.06949235617739724, 12.14591786802326823, 56.87609039468568994 ) ) ;
#119577=CARTESIAN_POINT ( 'NONE',  ( 14.34966873604960469, 8.224510206698951720, 94.16557627198103830 ) ) ;
#119578=CARTESIAN_POINT ( 'NONE',  ( 0.05219959533907565091, 21.53943276465977519, 69.99890960531435269 ) ) ;
#119579=CARTESIAN_POINT ( 'NONE',  ( -8.314922557960811034, -14.29746914071050412, 27.08224293864769550 ) ) ;
#119580=CARTESIAN_POINT ( 'NONE',  ( -14.34966873604972548, 8.224510206698743886, 43.33442372801901143 ) ) ;
#119581=CARTESIAN_POINT ( 'NONE',  ( -16.51473224551069308, -9.474510206698971260, 46.66557627198102409 ) ) ;
#119582=CARTESIAN_POINT ( 'NONE',  ( 4.379528057220092307, 16.55341960407617563, 97.29275706135234714 ) ) ;
#119583=CARTESIAN_POINT ( 'NONE',  ( 16.46253265017146816, 9.564922557961045513, 81.66775706135233293 ) ) ;
#119584=CARTESIAN_POINT ( 'NONE',  ( 5.823673210054125526, 21.52544592524343514, 89.79057627198103830 ) ) ;
#119585=CARTESIAN_POINT ( 'NONE',  ( 8.314922557961029526, -14.29746914071037800, 105.4177570613523613 ) ) ;
#119588=CARTESIAN_POINT ( 'NONE',  ( 18.67979575497178502, 10.72451020669898547, 64.16557627198102409 ) ) ;
#119589=CARTESIAN_POINT ( 'NONE',  ( -0.05219959533934338120, 16.53943276465976808, 87.50109039468568994 ) ) ;
#119590=ORIENTED_EDGE ( 'NONE', *, *, #106006, .F. ) ;
#119591=CARTESIAN_POINT ( 'NONE',  ( -21.55341960407610458, -5.719274019375992779, 31.45724293864769550 ) ) ;
#119593=CARTESIAN_POINT ( 'NONE',  ( -15.80617190586745835, -15.72974639402198527, 91.87390960531436690 ) ) ;
#119594=CARTESIAN_POINT ( 'NONE',  ( 0.05219959533910956823, 16.53943276465976808, 29.99890960531435979 ) ) ;
#119595=CARTESIAN_POINT ( 'NONE',  ( 5.153800228976615827, -19.02544592524334988, 110.2094237280189901 ) ) ;
#119596=CARTESIAN_POINT ( 'NONE',  ( -16.46253265017160317, 9.564922557960807481, 35.83224293864768839 ) ) ;
#119597=CARTESIAN_POINT ( 'NONE',  ( -16.55341960407617563, 4.379528057220093196, 23.54275706135235424 ) ) ;
#119598=CARTESIAN_POINT ( 'NONE',  ( 9.474510206698971260, -16.51473224551069308, 47.91557627198102409 ) ) ;
#119600=CARTESIAN_POINT ( 'NONE',  ( 19.05341960407611168, 5.049401038298154454, 103.9572429386476671 ) ) ;
#119601=CARTESIAN_POINT ( 'NONE',  ( 16.51473224551069308, 9.474510206698969483, 104.1655762719810241 ) ) ;
#119602=CARTESIAN_POINT ( 'NONE',  ( 8.224510206698742110, 14.34966873604972548, 92.08442372801901854 ) ) ;
#119603=CARTESIAN_POINT ( 'NONE',  ( -13.89961937509957401, -13.97604488694547875, 89.37609039468563310 ) ) ;
#119604=CARTESIAN_POINT ( 'NONE',  ( -5.153800228976607833, 19.02544592524334988, 37.70942372801899722 ) ) ;
#119605=CARTESIAN_POINT ( 'NONE',  ( -21.55341960407610458, -5.719274019375992779, 71.45724293864769550 ) ) ;
#119606=CARTESIAN_POINT ( 'NONE',  ( -8.314922557961024197, 14.29746914071037800, 97.91775706135236135 ) ) ;
#119607=CARTESIAN_POINT ( 'NONE',  ( -21.52544592524343514, 5.823673210054127303, 36.04057627198102409 ) ) ;
#119608=CARTESIAN_POINT ( 'NONE',  ( 5.049401038297881783, 19.05341960407617563, 87.29275706135234714 ) ) ;
#119609=CARTESIAN_POINT ( 'NONE',  ( -19.03943276465977164, 0.05219959533909376836, 51.24890960531436690 ) ) ;
#119610=CARTESIAN_POINT ( 'NONE',  ( 19.05341960407611168, 5.049401038298154454, 93.95724293864769550 ) ) ;
#119611=CARTESIAN_POINT ( 'NONE',  ( 0.05219959533937995610, -21.53943276465977519, 65.00109039468568994 ) ) ;
#119612=CARTESIAN_POINT ( 'NONE',  ( 5.153800228976335163, 19.02544592524342804, 59.79057627198100988 ) ) ;
#119613=CARTESIAN_POINT ( 'NONE',  ( -16.55341960407611168, -4.379528057220339221, 101.4572429386476955 ) ) ;
#119614=CARTESIAN_POINT ( 'NONE',  ( -17.40861289039003879, -6.110651285853240466, 86.37232470827434838 ) ) ;
#119615=CARTESIAN_POINT ( 'NONE',  ( -8.314922557960811034, -14.29746914071050412, 82.08224293864768129 ) ) ;
#119616=CARTESIAN_POINT ( 'NONE',  ( 21.52544592524344225, -5.823673210054117533, 68.54057627198103830 ) ) ;
#119617=CARTESIAN_POINT ( 'NONE',  ( -13.89961937509957401, -13.97604488694547875, 89.37609039468563310 ) ) ;
#119619=CARTESIAN_POINT ( 'NONE',  ( -16.51473224551069308, -9.474510206698971260, 56.66557627198103120 ) ) ;
#119621=CARTESIAN_POINT ( 'NONE',  ( 19.05341960407611168, 5.049401038298154454, 73.95724293864768129 ) ) ;
#119622=CARTESIAN_POINT ( 'NONE',  ( -19.03943276465977164, 0.05219959533909376836, 86.24890960531436690 ) ) ;
#119623=CARTESIAN_POINT ( 'NONE',  ( -14.29746914071037622, -8.314922557961029526, 69.16775706135234714 ) ) ;
#119625=CARTESIAN_POINT ( 'NONE',  ( -9.564922557961040184, 16.46253265017147172, 37.91775706135233293 ) ) ;
#119627=CARTESIAN_POINT ( 'NONE',  ( 16.46253265017160672, -9.564922557960803928, 113.3322429386476955 ) ) ;
#119628=CARTESIAN_POINT ( 'NONE',  ( -4.379528057220086978, -16.55341960407618274, 99.79275706135234714 ) ) ;
#119630=CARTESIAN_POINT ( 'NONE',  ( 8.314922557961029526, -14.29746914071037800, 95.41775706135234714 ) ) ;
#119632=CARTESIAN_POINT ( 'NONE',  ( 8.314922557961029526, -14.29746914071037800, 65.41775706135234714 ) ) ;
#119634=CARTESIAN_POINT ( 'NONE',  ( 21.55341960407619695, -5.719274019375665929, 66.04275706135236135 ) ) ;
#119635=CARTESIAN_POINT ( 'NONE',  ( -16.46253265017146816, -9.564922557961047289, 74.16775706135234714 ) ) ;
#119636=CARTESIAN_POINT ( 'NONE',  ( -5.049401038297874678, -19.05341960407617918, 29.79275706135232227 ) ) ;
#119637=CARTESIAN_POINT ( 'NONE',  ( 5.153800228976335163, 19.02544592524342804, 59.79057627198100988 ) ) ;
#119638=CARTESIAN_POINT ( 'NONE',  ( 19.05341960407611168, 5.049401038298154454, 38.95724293864767418 ) ) ;
#119640=CARTESIAN_POINT ( 'NONE',  ( -0.05219959533907301413, -21.53943276465977519, 82.49890960531436690 ) ) ;
#119642=CARTESIAN_POINT ( 'NONE',  ( 21.52544592524344225, -5.823673210054117533, 33.54057627198102409 ) ) ;
#119643=CARTESIAN_POINT ( 'NONE',  ( 8.314922557960818139, 14.29746914071049879, 109.5822429386476955 ) ) ;
#119644=CARTESIAN_POINT ( 'NONE',  ( 12.14591786802327356, -12.06949235617739191, 50.62609039468568994 ) ) ;
#119646=CARTESIAN_POINT ( 'NONE',  ( 15.80617190586769283, -15.72974639402175789, 30.62609039468567929 ) ) ;
#119647=CARTESIAN_POINT ( 'NONE',  ( -16.55341960407611168, -4.379528057220339221, 56.45724293864768839 ) ) ;
#119649=CARTESIAN_POINT ( 'NONE',  ( 16.53943276465976808, 0.05219959533934440121, 26.25109039468567573 ) ) ;
#119650=CARTESIAN_POINT ( 'NONE',  ( 13.89961937509957401, 13.97604488694547697, 36.87609039468565442 ) ) ;
#119651=CARTESIAN_POINT ( 'NONE',  ( 0.05219959533910956823, 16.53943276465976808, 49.99890960531437401 ) ) ;
#119652=CARTESIAN_POINT ( 'NONE',  ( -5.719274019375978568, 21.55341960407610458, 110.2072429386477239 ) ) ;
#119654=CARTESIAN_POINT ( 'NONE',  ( 5.719274019375991003, -21.55341960407610458, 77.70724293864770971 ) ) ;
#119655=CARTESIAN_POINT ( 'NONE',  ( -19.05341960407611168, -5.049401038298163336, 96.45724293864769550 ) ) ;
#119656=CARTESIAN_POINT ( 'NONE',  ( 8.224510206698953496, -14.34966873604960469, 62.91557627198102409 ) ) ;
#119657=CARTESIAN_POINT ( 'NONE',  ( 16.51473224551069308, 9.474510206698969483, 99.16557627198102409 ) ) ;
#119659=CARTESIAN_POINT ( 'NONE',  ( 19.03943276465977164, 0.05219959533936151252, 66.25109039468567573 ) ) ;
#119660=CARTESIAN_POINT ( 'NONE',  ( -18.67979575497178146, -10.72451020669898902, 106.6655762719810383 ) ) ;
#119661=CARTESIAN_POINT ( 'NONE',  ( -9.474510206698964154, 16.51473224551069663, 55.41557627198103120 ) ) ;
#119662=CARTESIAN_POINT ( 'NONE',  ( 5.049401038298161559, -19.05341960407611168, 22.70724293864769194 ) ) ;
#119663=CARTESIAN_POINT ( 'NONE',  ( -10.72451020669870658, -18.67979575497194134, 49.58442372801901143 ) ) ;
#119665=CARTESIAN_POINT ( 'NONE',  ( -0.05219959533910754901, -16.53943276465976808, 37.49890960531436690 ) ) ;
#119666=CARTESIAN_POINT ( 'NONE',  ( -0.05219959533909027116, -19.03943276465977164, 52.49890960531436690 ) ) ;
#119667=CARTESIAN_POINT ( 'NONE',  ( 5.153800228976335163, 19.02544592524342804, 109.7905762719810099 ) ) ;
#119668=CARTESIAN_POINT ( 'NONE',  ( 18.62759615963271287, -10.81492255796078972, 68.33224293864769550 ) ) ;
#119670=CARTESIAN_POINT ( 'NONE',  ( -16.46253265017160317, 9.564922557960807481, 50.83224293864770260 ) ) ;
#119671=CARTESIAN_POINT ( 'NONE',  ( 18.67979575497178502, 10.72451020669898547, 69.16557627198102409 ) ) ;
#119672=CARTESIAN_POINT ( 'NONE',  ( 15.72974639402176855, 15.80617190586768217, 86.87609039468568994 ) ) ;
#119673=CARTESIAN_POINT ( 'NONE',  ( 17.49999999999999645, 5.500000000000010658, 53.78230962303567964 ) ) ;
#119674=CARTESIAN_POINT ( 'NONE',  ( -16.53943276465976808, -0.05219959533934237506, 83.75109039468568994 ) ) ;
#119675=CARTESIAN_POINT ( 'NONE',  ( 16.52544592524342804, -4.483927247898539470, 83.54057627198102409 ) ) ;
#119676=CARTESIAN_POINT ( 'NONE',  ( -5.049401038298153566, 19.05341960407611168, 75.20724293864769550 ) ) ;
#119677=ORIENTED_EDGE ( 'NONE', *, *, #20984, .F. ) ;
#119678=CARTESIAN_POINT ( 'NONE',  ( -19.05341960407617563, 5.049401038297882671, 43.54275706135232582 ) ) ;
#119679=CARTESIAN_POINT ( 'NONE',  ( 14.29746914071037800, 8.314922557961029526, 91.66775706135234714 ) ) ;
#119680=CARTESIAN_POINT ( 'NONE',  ( -15.80617190586768217, 15.72974639402176855, 113.1260903946856899 ) ) ;
#119681=CARTESIAN_POINT ( 'NONE',  ( -0.05219959533909027116, -19.03943276465977164, 92.49890960531436690 ) ) ;
#119682=CARTESIAN_POINT ( 'NONE',  ( -5.719274019375978568, 21.55341960407610458, 45.20724293864769550 ) ) ;
#119683=CARTESIAN_POINT ( 'NONE',  ( 15.72974639402176855, 15.80617190586768217, 96.87609039468568994 ) ) ;
#119684=CARTESIAN_POINT ( 'NONE',  ( -14.29746914071037622, -8.314922557961029526, 59.16775706135234714 ) ) ;
#119685=CARTESIAN_POINT ( 'NONE',  ( 21.53943276465977519, -0.05219959533907433946, 108.7489096053143669 ) ) ;
#119686=CARTESIAN_POINT ( 'NONE',  ( 0.05219959533934541429, -16.53943276465976808, 30.00109039468568284 ) ) ;
#119687=CARTESIAN_POINT ( 'NONE',  ( -9.474510206698964154, 16.51473224551069663, 90.41557627198103830 ) ) ;
#119688=CARTESIAN_POINT ( 'NONE',  ( 16.55341960407618274, -4.379528057220086978, 31.04275706135234714 ) ) ;
#119689=CARTESIAN_POINT ( 'NONE',  ( 9.474510206698971260, -16.51473224551069308, 52.91557627198102409 ) ) ;
#119690=CARTESIAN_POINT ( 'NONE',  ( -8.314922557961024197, 14.29746914071037800, 27.91775706135234358 ) ) ;
#119691=CARTESIAN_POINT ( 'NONE',  ( -4.483927247898539470, -16.52544592524342804, 82.29057627198103830 ) ) ;
#119693=CARTESIAN_POINT ( 'NONE',  ( -14.34966873604972548, 8.224510206698743886, 93.33442372801901854 ) ) ;
#119694=CARTESIAN_POINT ( 'NONE',  ( 10.81492255796106328, -18.62759615963255655, 40.41775706135234714 ) ) ;
#119695=CARTESIAN_POINT ( 'NONE',  ( -19.05341960407611168, -5.049401038298163336, 71.45724293864766707 ) ) ;
#119696=CARTESIAN_POINT ( 'NONE',  ( 16.46253265017160672, -9.564922557960803928, 88.33224293864769550 ) ) ;
#119697=CARTESIAN_POINT ( 'NONE',  ( -16.52544592524342804, 4.483927247898546575, 36.04057627198102409 ) ) ;
#119698=CARTESIAN_POINT ( 'NONE',  ( 14.29746914071037800, 8.314922557961029526, 81.66775706135236135 ) ) ;
#119699=ORIENTED_EDGE ( 'NONE', *, *, #128937, .F. ) ;
#119700=CARTESIAN_POINT ( 'NONE',  ( 16.46253265017146816, 9.564922557961045513, 26.66775706135234003 ) ) ;
#119701=CARTESIAN_POINT ( 'NONE',  ( 19.03943276465977164, -0.05219959533909143690, 98.74890960531436690 ) ) ;
#119702=CARTESIAN_POINT ( 'NONE',  ( 16.46253265017160672, -9.564922557960803928, 48.33224293864769550 ) ) ;
#119704=CARTESIAN_POINT ( 'NONE',  ( -12.14591786802326823, 12.06949235617739902, 43.12609039468568284 ) ) ;
#119705=CARTESIAN_POINT ( 'NONE',  ( 19.02544592524334988, 5.153800228976608722, 71.45942372801900433 ) ) ;
#119706=CARTESIAN_POINT ( 'NONE',  ( -12.14591786802326823, 12.06949235617739902, 58.12609039468568994 ) ) ;
#119707=CARTESIAN_POINT ( 'NONE',  ( 13.89961937509977652, -13.97604488694527269, 113.1239096053143527 ) ) ;
#119708=CARTESIAN_POINT ( 'NONE',  ( -9.564922557960796823, -16.46253265017161027, 72.08224293864770971 ) ) ;
#119709=CARTESIAN_POINT ( 'NONE',  ( -10.81492255796078084, -18.62759615963271287, 112.0822429386477097 ) ) ;
#119710=CARTESIAN_POINT ( 'NONE',  ( -19.03943276465977164, -0.05219959533935918106, 68.75109039468566152 ) ) ;
#119711=CARTESIAN_POINT ( 'NONE',  ( 16.51473224551069308, 9.474510206698969483, 104.1655762719810241 ) ) ;
#119712=CARTESIAN_POINT ( 'NONE',  ( -19.02544592524342804, 5.153800228976336051, 31.04057627198102409 ) ) ;
#119713=CARTESIAN_POINT ( 'NONE',  ( 5.153800228976335163, 19.02544592524342804, 74.79057627198103830 ) ) ;
#119714=CARTESIAN_POINT ( 'NONE',  ( 8.224510206698953496, -14.34966873604960469, 32.91557627198102409 ) ) ;
#119716=CARTESIAN_POINT ( 'NONE',  ( 5.153800228976615827, -19.02544592524334988, 35.20942372801899722 ) ) ;
#119717=CARTESIAN_POINT ( 'NONE',  ( -12.06949235617756955, 12.14591786802309770, 70.62390960531436690 ) ) ;
#119718=CARTESIAN_POINT ( 'NONE',  ( -10.81492255796105439, 18.62759615963255655, 107.9177570613523471 ) ) ;
#119719=CARTESIAN_POINT ( 'NONE',  ( -0.05219959533909027116, -19.03943276465977164, 52.49890960531436690 ) ) ;
#119720=EDGE_CURVE ( 'NONE', #11730, #96182, #184112, .T. ) ;
#119721=CARTESIAN_POINT ( 'NONE',  ( -4.379528057220328563, 16.55341960407611168, 45.20724293864769550 ) ) ;
#119722=CARTESIAN_POINT ( 'NONE',  ( -10.81492255796105439, 18.62759615963255655, 102.9177570613523756 ) ) ;
#119723=CARTESIAN_POINT ( 'NONE',  ( 19.03943276465977164, -0.05219959533909143690, 88.74890960531436690 ) ) ;
#119724=CARTESIAN_POINT ( 'NONE',  ( 19.02544592524343514, -5.153800228976328945, 113.5405762719810241 ) ) ;
#119725=CARTESIAN_POINT ( 'NONE',  ( -13.89961937509977652, 13.97604488694528158, 40.62390960531435979 ) ) ;
#119726=CARTESIAN_POINT ( 'NONE',  ( 16.52544592524342804, -4.483927247898539470, 103.5405762719810383 ) ) ;
#119727=CARTESIAN_POINT ( 'NONE',  ( -16.52544592524342804, 4.483927247898546575, 91.04057627198103830 ) ) ;
#119728=CARTESIAN_POINT ( 'NONE',  ( 10.72451020669898902, -18.67979575497178502, 92.91557627198103830 ) ) ;
#119729=CARTESIAN_POINT ( 'NONE',  ( 9.474510206698971260, -16.51473224551069308, 87.91557627198102409 ) ) ;
#119730=CARTESIAN_POINT ( 'NONE',  ( 18.67979575497178502, 10.72451020669898547, 94.16557627198103830 ) ) ;
#119731=CARTESIAN_POINT ( 'NONE',  ( 0.05219959533909260263, 19.03943276465977164, 84.99890960531436690 ) ) ;
#119733=CARTESIAN_POINT ( 'NONE',  ( -16.53943276465976808, 0.05219959533911058130, 106.2489096053143811 ) ) ;
#119734=CARTESIAN_POINT ( 'NONE',  ( 19.02544592524343514, -5.153800228976328945, 73.54057627198103830 ) ) ;
#119735=CARTESIAN_POINT ( 'NONE',  ( 18.67979575497178502, 10.72451020669898547, 84.16557627198103830 ) ) ;
#119737=CARTESIAN_POINT ( 'NONE',  ( -5.823673210054116645, -21.52544592524344225, 27.29057627198103120 ) ) ;
#119738=CARTESIAN_POINT ( 'NONE',  ( 19.52837319214027900, -5.499999999999893419, 67.10471352585541638 ) ) ;
#119739=CARTESIAN_POINT ( 'NONE',  ( -16.52544592524335698, -4.483927247898792601, 33.95942372801901143 ) ) ;
#119740=CARTESIAN_POINT ( 'NONE',  ( 4.483927247898545687, 16.52544592524342804, 89.79057627198103830 ) ) ;
#119741=CARTESIAN_POINT ( 'NONE',  ( 18.22780087662123805, -5.499999999999989342, 53.51763182126895657 ) ) ;
#119742=CARTESIAN_POINT ( 'NONE',  ( 13.97604488694527802, 13.89961937509977652, 89.37390960531436690 ) ) ;
#119743=CARTESIAN_POINT ( 'NONE',  ( 5.153800228976335163, 19.02544592524342804, 39.79057627198100988 ) ) ;
#119744=CARTESIAN_POINT ( 'NONE',  ( -12.06949235617756955, 12.14591786802309770, 75.62390960531439532 ) ) ;
#119745=CARTESIAN_POINT ( 'NONE',  ( 5.719274019375991003, -21.55341960407610458, 22.70724293864769194 ) ) ;
#119746=CARTESIAN_POINT ( 'NONE',  ( -4.483927247898539470, -16.52544592524342804, 52.29057627198102409 ) ) ;
#119747=CARTESIAN_POINT ( 'NONE',  ( 19.03943276465977164, 0.05219959533936151252, 106.2510903946856615 ) ) ;
#119748=CARTESIAN_POINT ( 'NONE',  ( 21.53943276465977519, 0.05219959533937863772, 56.25109039468568284 ) ) ;
#119749=CARTESIAN_POINT ( 'NONE',  ( 17.50000000000000711, -5.499999999999978684, 41.21769037696436300 ) ) ;
#119750=CARTESIAN_POINT ( 'NONE',  ( -9.474510206698964154, 16.51473224551069663, 100.4155762719810241 ) ) ;
#119751=CARTESIAN_POINT ( 'NONE',  ( 12.14591786802327356, -12.06949235617739191, 80.62609039468567573 ) ) ;
#119752=CARTESIAN_POINT ( 'NONE',  ( 16.51473224551069308, 9.474510206698969483, 29.16557627198103475 ) ) ;
#119753=CARTESIAN_POINT ( 'NONE',  ( 9.564922557960805705, 16.46253265017160317, 74.58224293864769550 ) ) ;
#119754=CARTESIAN_POINT ( 'NONE',  ( -0.05219959533907301413, -21.53943276465977519, 82.49890960531436690 ) ) ;
#119755=CARTESIAN_POINT ( 'NONE',  ( 9.564922557961047289, -16.46253265017146816, 105.4177570613523471 ) ) ;
#119756=CARTESIAN_POINT ( 'NONE',  ( -0.05219959533910754901, -16.53943276465976808, 47.49890960531435979 ) ) ;
#119757=CARTESIAN_POINT ( 'NONE',  ( -18.67979575497193778, 10.72451020669871902, 58.33442372801901143 ) ) ;
#119758=CARTESIAN_POINT ( 'NONE',  ( -16.52544592524335698, -4.483927247898792601, 88.95942372801901854 ) ) ;
#119759=CARTESIAN_POINT ( 'NONE',  ( 21.53943276465977519, -0.05219959533907433946, 28.74890960531435624 ) ) ;
#119760=CARTESIAN_POINT ( 'NONE',  ( 17.48853670773242541, 5.747243402303174875, 28.83328700250010712 ) ) ;
#119762=CARTESIAN_POINT ( 'NONE',  ( 4.379528057220092307, 16.55341960407617563, 107.2927570613523471 ) ) ;
#119763=CARTESIAN_POINT ( 'NONE',  ( -8.224510206698735004, -14.34966873604973081, 59.58442372801901854 ) ) ;
#119764=CARTESIAN_POINT ( 'NONE',  ( -19.03943276465977164, 0.05219959533909376836, 76.24890960531435269 ) ) ;
#119765=CARTESIAN_POINT ( 'NONE',  ( 5.049401038298161559, -19.05341960407611168, 77.70724293864765286 ) ) ;
#119766=CARTESIAN_POINT ( 'NONE',  ( -18.62759615963255300, -10.81492255796106328, 74.16775706135231871 ) ) ;
#119767=CARTESIAN_POINT ( 'NONE',  ( -0.05219959533934338120, 16.53943276465976808, 72.50109039468568994 ) ) ;
#119768=CARTESIAN_POINT ( 'NONE',  ( 14.29746914071049879, -8.314922557960816363, 48.33224293864770260 ) ) ;
#119769=CARTESIAN_POINT ( 'NONE',  ( 5.153800228976335163, 19.02544592524342804, 54.79057627198103120 ) ) ;
#119770=CARTESIAN_POINT ( 'NONE',  ( 9.564922557960805705, 16.46253265017160317, 54.58224293864769550 ) ) ;
#119771=CARTESIAN_POINT ( 'NONE',  ( -14.29746914071037622, -8.314922557961029526, 39.16775706135235424 ) ) ;
#119772=VERTEX_POINT ( 'NONE', #117874 ) ;
#119773=CARTESIAN_POINT ( 'NONE',  ( 19.02544592524334988, 5.153800228976608722, 101.4594237280189759 ) ) ;
#119774=CARTESIAN_POINT ( 'NONE',  ( -16.55341960407611168, -4.379528057220339221, 96.45724293864770971 ) ) ;
#119775=CARTESIAN_POINT ( 'NONE',  ( 13.97604488694527802, 13.89961937509977652, 69.37390960531436690 ) ) ;
#119776=CARTESIAN_POINT ( 'NONE',  ( 19.03943276465977164, 0.05219959533936151252, 106.2510903946856615 ) ) ;
#119778=CARTESIAN_POINT ( 'NONE',  ( 18.62759615963255655, 10.81492255796105972, 101.6677570613523613 ) ) ;
#119779=CARTESIAN_POINT ( 'NONE',  ( 16.53943276465976808, 0.05219959533934440121, 71.25109039468568994 ) ) ;
#119781=CARTESIAN_POINT ( 'NONE',  ( -15.80617190586745835, -15.72974639402198527, 66.87390960531436690 ) ) ;
#119782=CARTESIAN_POINT ( 'NONE',  ( -14.34966873604972548, 8.224510206698743886, 48.33442372801902565 ) ) ;
#119784=CARTESIAN_POINT ( 'NONE',  ( 19.05341960407617918, -5.049401038297876454, 46.04275706135233293 ) ) ;
#119785=CARTESIAN_POINT ( 'NONE',  ( 13.89961937509977652, -13.97604488694527269, 93.12390960531436690 ) ) ;
#119786=CARTESIAN_POINT ( 'NONE',  ( 19.03943276465977164, -0.05219959533909143690, 23.74890960531435269 ) ) ;
#119787=CARTESIAN_POINT ( 'NONE',  ( -13.89961937509977652, 13.97604488694528158, 65.62390960531436690 ) ) ;
#119788=CARTESIAN_POINT ( 'NONE',  ( 21.53943276465977519, 0.05219959533937863772, 71.25109039468568994 ) ) ;
#119789=CARTESIAN_POINT ( 'NONE',  ( 19.05341960407617918, -5.049401038297876454, 46.04275706135233293 ) ) ;
#119790=CARTESIAN_POINT ( 'NONE',  ( -16.46253265017146816, -9.564922557961047289, 34.16775706135233293 ) ) ;
#119791=CARTESIAN_POINT ( 'NONE',  ( 0.05219959533909260263, 19.03943276465977164, 49.99890960531435979 ) ) ;
#119792=CARTESIAN_POINT ( 'NONE',  ( -21.53943276465977519, 0.05219959533907696930, 21.24890960531436690 ) ) ;
#119793=CARTESIAN_POINT ( 'NONE',  ( -0.05219959533937732626, 21.53943276465977519, 77.50109039468567573 ) ) ;
#119794=CARTESIAN_POINT ( 'NONE',  ( 19.02544592524343514, -5.153800228976328945, 63.54057627198103830 ) ) ;
#119795=CARTESIAN_POINT ( 'NONE',  ( -15.80617190586768217, 15.72974639402176855, 93.12609039468568994 ) ) ;
#119796=CARTESIAN_POINT ( 'NONE',  ( -0.05219959533907301413, -21.53943276465977519, 42.49890960531435979 ) ) ;
#119797=CARTESIAN_POINT ( 'NONE',  ( 19.05341960407611168, 5.049401038298154454, 88.95724293864769550 ) ) ;
#119798=CARTESIAN_POINT ( 'NONE',  ( -5.719274019375665041, -21.55341960407619695, 34.79275706135235424 ) ) ;
#119799=CARTESIAN_POINT ( 'NONE',  ( 16.46253265017146816, 9.564922557961045513, 61.66775706135234003 ) ) ;
#119800=CARTESIAN_POINT ( 'NONE',  ( -16.46253265017160317, 9.564922557960807481, 40.83224293864769550 ) ) ;
#119801=CARTESIAN_POINT ( 'NONE',  ( -13.89961937509977652, 13.97604488694528158, 90.62390960531432427 ) ) ;
#119802=CARTESIAN_POINT ( 'NONE',  ( 4.379528057220092307, 16.55341960407617563, 27.29275706135234358 ) ) ;
#119803=CARTESIAN_POINT ( 'NONE',  ( -14.29746914071049879, 8.314922557960819915, 85.83224293864768129 ) ) ;
#119804=CARTESIAN_POINT ( 'NONE',  ( 5.049401038298161559, -19.05341960407611168, 67.70724293864769550 ) ) ;
#119805=CARTESIAN_POINT ( 'NONE',  ( 5.823673210054125526, 21.52544592524343514, 49.79057627198102409 ) ) ;
#119806=CARTESIAN_POINT ( 'NONE',  ( -8.224510206698735004, -14.34966873604973081, 24.58442372801901499 ) ) ;
#119807=CARTESIAN_POINT ( 'NONE',  ( 18.62759615963255655, 10.81492255796105972, 26.66775706135235424 ) ) ;
#119808=CARTESIAN_POINT ( 'NONE',  ( -5.719274019375665041, -21.55341960407619695, 74.79275706135234714 ) ) ;
#119809=CARTESIAN_POINT ( 'NONE',  ( -4.379528057220086978, -16.55341960407618274, 64.79275706135234714 ) ) ;
#119810=CARTESIAN_POINT ( 'NONE',  ( -12.14591786802326823, 12.06949235617739902, 68.12609039468567573 ) ) ;
#119811=CARTESIAN_POINT ( 'NONE',  ( 5.049401038298161559, -19.05341960407611168, 67.70724293864769550 ) ) ;
#119812=CARTESIAN_POINT ( 'NONE',  ( 12.14591786802327356, -12.06949235617739191, 100.6260903946857184 ) ) ;
#119813=CARTESIAN_POINT ( 'NONE',  ( -9.474510206698720793, -16.51473224551083518, 39.58442372801899722 ) ) ;
#119814=CARTESIAN_POINT ( 'NONE',  ( 10.72451020669871369, 18.67979575497193778, 27.08442372801901854 ) ) ;
#119815=CARTESIAN_POINT ( 'NONE',  ( -16.53943276465976808, 0.05219959533911058130, 61.24890960531435979 ) ) ;
#119816=CARTESIAN_POINT ( 'NONE',  ( -9.564922557960796823, -16.46253265017161027, 102.0822429386477097 ) ) ;
#119817=CARTESIAN_POINT ( 'NONE',  ( 8.224510206698742110, 14.34966873604972548, 87.08442372801901854 ) ) ;
#119818=CARTESIAN_POINT ( 'NONE',  ( -5.719274019375665041, -21.55341960407619695, 59.79275706135234714 ) ) ;
#119819=CARTESIAN_POINT ( 'NONE',  ( 12.14591786802327356, -12.06949235617739191, 25.62609039468567929 ) ) ;
#119820=CARTESIAN_POINT ( 'NONE',  ( -5.823673210054431948, 21.52544592524334988, 22.70942372801901499 ) ) ;
#119821=CARTESIAN_POINT ( 'NONE',  ( 0.05219959533910956823, 16.53943276465976808, 54.99890960531435269 ) ) ;
#119823=CARTESIAN_POINT ( 'NONE',  ( -0.05219959533907301413, -21.53943276465977519, 107.4989096053143669 ) ) ;
#119824=CARTESIAN_POINT ( 'NONE',  ( 12.14591786802309770, 12.06949235617756955, 39.37390960531436690 ) ) ;
#119827=CARTESIAN_POINT ( 'NONE',  ( 5.823673210054125526, 21.52544592524343514, 29.79057627198102409 ) ) ;
#119828=CARTESIAN_POINT ( 'NONE',  ( 21.53943276465977519, 0.05219959533937863772, 31.25109039468568639 ) ) ;
#119829=CARTESIAN_POINT ( 'NONE',  ( 12.14591786802309770, 12.06949235617756955, 64.37390960531435269 ) ) ;
#119830=CARTESIAN_POINT ( 'NONE',  ( -5.719274019375978568, 21.55341960407610458, 60.20724293864768839 ) ) ;
#119831=CARTESIAN_POINT ( 'NONE',  ( 19.05341960407611168, 5.049401038298154454, 78.95724293864769550 ) ) ;
#119832=CARTESIAN_POINT ( 'NONE',  ( -13.97604488694527625, -13.89961937509977652, 31.87390960531435979 ) ) ;
#119833=CARTESIAN_POINT ( 'NONE',  ( -13.97604488694547697, 13.89961937509957934, 73.12609039468568994 ) ) ;
#119834=CARTESIAN_POINT ( 'NONE',  ( 10.72451020669898902, -18.67979575497178502, 42.91557627198103120 ) ) ;
#119835=CARTESIAN_POINT ( 'NONE',  ( 9.564922557960805705, 16.46253265017160317, 64.58224293864769550 ) ) ;
#119837=CARTESIAN_POINT ( 'NONE',  ( -14.34966873604972548, 8.224510206698743886, 43.33442372801901143 ) ) ;
#119838=CARTESIAN_POINT ( 'NONE',  ( -15.80617190586745835, -15.72974639402198527, 111.8739096053143669 ) ) ;
#119839=CARTESIAN_POINT ( 'NONE',  ( -0.05219959533910754901, -16.53943276465976808, 52.49890960531435979 ) ) ;
#119840=CARTESIAN_POINT ( 'NONE',  ( -13.97604488694527625, -13.89961937509977652, 101.8739096053143811 ) ) ;
#119841=CARTESIAN_POINT ( 'NONE',  ( -21.53943276465977519, 0.05219959533907696930, 76.24890960531435269 ) ) ;
#119842=CARTESIAN_POINT ( 'NONE',  ( 15.80617190586746368, 15.72974639402197994, 109.3739096053143811 ) ) ;
#119843=CARTESIAN_POINT ( 'NONE',  ( 16.55341960407618274, -4.379528057220086978, 36.04275706135234714 ) ) ;
#119844=CARTESIAN_POINT ( 'NONE',  ( -21.55341960407610458, -5.719274019375992779, 46.45724293864769550 ) ) ;
#119845=CARTESIAN_POINT ( 'NONE',  ( -0.05219959533937732626, 21.53943276465977519, 97.50109039468567573 ) ) ;
#119846=CARTESIAN_POINT ( 'NONE',  ( -5.049401038298153566, 19.05341960407611168, 40.20724293864768839 ) ) ;
#119847=CARTESIAN_POINT ( 'NONE',  ( -16.46253265017160317, 9.564922557960807481, 95.83224293864769550 ) ) ;
#119848=CARTESIAN_POINT ( 'NONE',  ( 13.97604488694527802, 13.89961937509977652, 79.37390960531435269 ) ) ;
#119850=ADVANCED_FACE ( 'NONE', ( #131025 ), #114861, .T. ) ;
#119851=CARTESIAN_POINT ( 'NONE',  ( 19.02544592524334988, 5.153800228976608722, 56.45942372801898301 ) ) ;
#119852=CARTESIAN_POINT ( 'NONE',  ( -15.80617190586768217, 15.72974639402176855, 108.1260903946856757 ) ) ;
#119853=CARTESIAN_POINT ( 'NONE',  ( -10.81492255796078084, -18.62759615963271287, 32.08224293864769550 ) ) ;
#119854=CARTESIAN_POINT ( 'NONE',  ( -16.55341960407617563, 4.379528057220093196, 98.54275706135234714 ) ) ;
#119855=CARTESIAN_POINT ( 'NONE',  ( 19.03943276465977164, 0.05219959533936151252, 81.25109039468567573 ) ) ;
#119856=CARTESIAN_POINT ( 'NONE',  ( -17.49999999999999645, 5.499999999999992895, 58.71769037696435589 ) ) ;
#119857=CARTESIAN_POINT ( 'NONE',  ( -19.02544592524334988, -5.153800228976617603, 78.95942372801900433 ) ) ;
#119858=CARTESIAN_POINT ( 'NONE',  ( 19.05341960407617918, -5.049401038297876454, 46.04275706135233293 ) ) ;
#119860=CARTESIAN_POINT ( 'NONE',  ( 9.474510206698971260, -16.51473224551069308, 47.91557627198102409 ) ) ;
#119861=CARTESIAN_POINT ( 'NONE',  ( -0.05219959533910754901, -16.53943276465976808, 47.49890960531435979 ) ) ;
#119862=CARTESIAN_POINT ( 'NONE',  ( -19.02544592524342804, 5.153800228976336051, 41.04057627198103120 ) ) ;
#119863=CARTESIAN_POINT ( 'NONE',  ( 12.14591786802309770, 12.06949235617756955, 39.37390960531436690 ) ) ;
#119865=CARTESIAN_POINT ( 'NONE',  ( -16.53943276465976808, 0.05219959533911058130, 21.24890960531436690 ) ) ;
#119866=CARTESIAN_POINT ( 'NONE',  ( 16.51473224551069308, 9.474510206698969483, 49.16557627198102409 ) ) ;
#119867=CARTESIAN_POINT ( 'NONE',  ( -18.67979575497193778, 10.72451020669871902, 113.3344237280190328 ) ) ;
#119868=CARTESIAN_POINT ( 'NONE',  ( 19.05341960407617918, -5.049401038297876454, 111.0427570613523329 ) ) ;
#119869=CARTESIAN_POINT ( 'NONE',  ( -21.52544592524343514, 5.823673210054127303, 36.04057627198102409 ) ) ;
#119870=CARTESIAN_POINT ( 'NONE',  ( 21.52544592524334988, 5.823673210054432836, 86.45942372801901854 ) ) ;
#119871=EDGE_LOOP ( 'NONE', ( #149914, #150264 ) ) ;
#119872=CARTESIAN_POINT ( 'NONE',  ( -19.03943276465977164, 0.05219959533909376836, 106.2489096053143669 ) ) ;
#119873=CARTESIAN_POINT ( 'NONE',  ( -19.02544592524342804, 5.153800228976336051, 81.04057627198103830 ) ) ;
#119875=CARTESIAN_POINT ( 'NONE',  ( -10.81492255796078084, -18.62759615963271287, 112.0822429386477097 ) ) ;
#119876=CARTESIAN_POINT ( 'NONE',  ( -4.379528057220328563, 16.55341960407611168, 85.20724293864770971 ) ) ;
#119877=CARTESIAN_POINT ( 'NONE',  ( -21.52544592524343514, 5.823673210054127303, 76.04057627198102409 ) ) ;
#119878=CARTESIAN_POINT ( 'NONE',  ( 16.51473224551069308, 9.474510206698969483, 69.16557627198102409 ) ) ;
#119879=CARTESIAN_POINT ( 'NONE',  ( 18.62759615963271287, -10.81492255796078972, 98.33224293864769550 ) ) ;
#119881=CARTESIAN_POINT ( 'NONE',  ( 19.05341960407611168, 5.049401038298154454, 63.95724293864769550 ) ) ;
#119882=CARTESIAN_POINT ( 'NONE',  ( -8.224510206698948167, 14.34966873604960824, 90.41557627198103830 ) ) ;
#119884=CARTESIAN_POINT ( 'NONE',  ( 19.02544592524343514, -5.153800228976328945, 68.54057627198103830 ) ) ;
#119885=CARTESIAN_POINT ( 'NONE',  ( 9.564922557961047289, -16.46253265017146816, 75.41775706135234714 ) ) ;
#119886=CARTESIAN_POINT ( 'NONE',  ( -16.55341960407611168, -4.379528057220339221, 91.45724293864769550 ) ) ;
#119887=CARTESIAN_POINT ( 'NONE',  ( -5.823673210054431948, 21.52544592524334988, 57.70942372801901143 ) ) ;
#119888=CARTESIAN_POINT ( 'NONE',  ( 5.049401038298161559, -19.05341960407611168, 47.70724293864770260 ) ) ;
#119889=CARTESIAN_POINT ( 'NONE',  ( 0.05219959533937995610, -21.53943276465977519, 25.00109039468567218 ) ) ;
#119890=CARTESIAN_POINT ( 'NONE',  ( -12.06949235617756955, 12.14591786802309770, 100.6239096053143811 ) ) ;
#119892=CARTESIAN_POINT ( 'NONE',  ( -19.03943276465977164, 0.05219959533909376836, 61.24890960531436690 ) ) ;
#119894=CARTESIAN_POINT ( 'NONE',  ( 0.05219959533936267826, -19.03943276465977164, 105.0010903946856615 ) ) ;
#119895=CARTESIAN_POINT ( 'NONE',  ( 19.05341960407611168, 5.049401038298154454, 108.9572429386477097 ) ) ;
#119896=CARTESIAN_POINT ( 'NONE',  ( -10.72451020669870658, -18.67979575497194134, 54.58442372801901143 ) ) ;
#119897=CARTESIAN_POINT ( 'NONE',  ( -16.51473224551069308, -9.474510206698971260, 96.66557627198102409 ) ) ;
#119898=CARTESIAN_POINT ( 'NONE',  ( -9.564922557961040184, 16.46253265017147172, 82.91775706135233293 ) ) ;
#119899=CARTESIAN_POINT ( 'NONE',  ( 9.474510206698971260, -16.51473224551069308, 57.91557627198103120 ) ) ;
#119900=CARTESIAN_POINT ( 'NONE',  ( 8.314922557960818139, 14.29746914071049879, 84.58224293864769550 ) ) ;
#119901=CARTESIAN_POINT ( 'NONE',  ( 19.03943276465977164, -0.05219959533909143690, 88.74890960531436690 ) ) ;
#119902=CARTESIAN_POINT ( 'NONE',  ( 14.29746914071049879, -8.314922557960816363, 83.33224293864769550 ) ) ;
#119903=CARTESIAN_POINT ( 'NONE',  ( -16.46253265017160317, 9.564922557960807481, 85.83224293864769550 ) ) ;
#119904=CARTESIAN_POINT ( 'NONE',  ( -16.51473224551082808, 9.474510206698731452, 28.33442372801900433 ) ) ;
#119905=CARTESIAN_POINT ( 'NONE',  ( 19.02544592524343514, -5.153800228976328945, 43.54057627198103120 ) ) ;
#119906=CARTESIAN_POINT ( 'NONE',  ( -14.29746914071049879, 8.314922557960819915, 40.83224293864769550 ) ) ;
#119907=CARTESIAN_POINT ( 'NONE',  ( 5.049401038298161559, -19.05341960407611168, 22.70724293864769194 ) ) ;
#119909=CARTESIAN_POINT ( 'NONE',  ( -0.05219959533937732626, 21.53943276465977519, 47.50109039468568994 ) ) ;
#119910=CARTESIAN_POINT ( 'NONE',  ( 13.89961937509957401, 13.97604488694547697, 81.87609039468564731 ) ) ;
#119911=CARTESIAN_POINT ( 'NONE',  ( 8.314922557960818139, 14.29746914071049879, 29.58224293864769905 ) ) ;
#119912=CARTESIAN_POINT ( 'NONE',  ( 21.53943276465977519, -0.05219959533907433946, 83.74890960531435269 ) ) ;
#119913=CARTESIAN_POINT ( 'NONE',  ( 10.81492255796078972, 18.62759615963270932, 29.58224293864769905 ) ) ;
#119914=CARTESIAN_POINT ( 'NONE',  ( 14.29746914071049879, -8.314922557960816363, 68.33224293864769550 ) ) ;
#119915=CARTESIAN_POINT ( 'NONE',  ( 16.46253265017160672, -9.564922557960803928, 43.33224293864769550 ) ) ;
#119916=CARTESIAN_POINT ( 'NONE',  ( 4.379528057220092307, 16.55341960407617563, 97.29275706135234714 ) ) ;
#119917=CARTESIAN_POINT ( 'NONE',  ( -14.29746914071037622, -8.314922557961029526, 64.16775706135234714 ) ) ;
#119918=CARTESIAN_POINT ( 'NONE',  ( -9.564922557961040184, 16.46253265017147172, 22.91775706135233648 ) ) ;
#119919=CARTESIAN_POINT ( 'NONE',  ( -9.474510206698964154, 16.51473224551069663, 90.41557627198103830 ) ) ;
#119920=CARTESIAN_POINT ( 'NONE',  ( 19.03943276465977164, -0.05219959533909143690, 73.74890960531435269 ) ) ;
#119921=CARTESIAN_POINT ( 'NONE',  ( -12.14591786802326823, 12.06949235617739902, 68.12609039468567573 ) ) ;
#119922=CARTESIAN_POINT ( 'NONE',  ( 19.03943276465977164, -0.05219959533909143690, 28.74890960531435624 ) ) ;
#119924=CARTESIAN_POINT ( 'NONE',  ( -14.34966873604960291, -8.224510206698953496, 31.66557627198102054 ) ) ;
#119925=CARTESIAN_POINT ( 'NONE',  ( 5.153800228976335163, 19.02544592524342804, 99.79057627198102409 ) ) ;
#119926=CARTESIAN_POINT ( 'NONE',  ( 9.564922557960805705, 16.46253265017160317, 84.58224293864769550 ) ) ;
#119927=CARTESIAN_POINT ( 'NONE',  ( -18.67979575497178146, -10.72451020669898902, 31.66557627198102054 ) ) ;
#119928=CARTESIAN_POINT ( 'NONE',  ( 14.34966873604960469, 8.224510206698951720, 74.16557627198102409 ) ) ;
#119929=CARTESIAN_POINT ( 'NONE',  ( -14.34966873604960291, -8.224510206698953496, 66.66557627198102409 ) ) ;
#119930=CARTESIAN_POINT ( 'NONE',  ( 16.53943276465976808, 0.05219959533934440121, 56.25109039468568284 ) ) ;
#119931=CARTESIAN_POINT ( 'NONE',  ( -16.46253265017146816, -9.564922557961047289, 59.16775706135233293 ) ) ;
#119932=CARTESIAN_POINT ( 'NONE',  ( -5.049401038297874678, -19.05341960407617918, 54.79275706135234003 ) ) ;
#119933=CARTESIAN_POINT ( 'NONE',  ( 13.89961937509977652, -13.97604488694527269, 93.12390960531436690 ) ) ;
#119934=CARTESIAN_POINT ( 'NONE',  ( -5.153800228976607833, 19.02544592524334988, 62.70942372801899722 ) ) ;
#119936=CARTESIAN_POINT ( 'NONE',  ( -9.564922557961040184, 16.46253265017147172, 112.9177570613523329 ) ) ;
#119937=CARTESIAN_POINT ( 'NONE',  ( -4.483927247898782831, 16.52544592524335698, 97.70942372801904696 ) ) ;
#119938=CARTESIAN_POINT ( 'NONE',  ( -0.05219959533909027116, -19.03943276465977164, 37.49890960531436690 ) ) ;
#119939=CARTESIAN_POINT ( 'NONE',  ( -16.46253265017160317, 9.564922557960807481, 115.8322429386477097 ) ) ;
#119940=CARTESIAN_POINT ( 'NONE',  ( 15.80617190586769283, -15.72974639402175789, 60.62609039468567573 ) ) ;
#119941=CARTESIAN_POINT ( 'NONE',  ( -13.89961937509957401, -13.97604488694547875, 109.3760903946856331 ) ) ;
#119943=CARTESIAN_POINT ( 'NONE',  ( 9.474510206698971260, -16.51473224551069308, 72.91557627198102409 ) ) ;
#119944=CARTESIAN_POINT ( 'NONE',  ( -19.02544592524342804, 5.153800228976336051, 111.0405762719810099 ) ) ;
#119945=CARTESIAN_POINT ( 'NONE',  ( -0.05219959533910754901, -16.53943276465976808, 72.49890960531435269 ) ) ;
#119946=CARTESIAN_POINT ( 'NONE',  ( 5.049401038298161559, -19.05341960407611168, 62.70724293864769550 ) ) ;
#119947=CARTESIAN_POINT ( 'NONE',  ( 19.03943276465977164, -0.05219959533909143690, 68.74890960531436690 ) ) ;
#119948=CARTESIAN_POINT ( 'NONE',  ( -19.05341960407617563, 5.049401038297882671, 73.54275706135233293 ) ) ;
#119949=CARTESIAN_POINT ( 'NONE',  ( -5.719274019375978568, 21.55341960407610458, 60.20724293864768839 ) ) ;
#119950=CARTESIAN_POINT ( 'NONE',  ( -16.53943276465976808, 0.05219959533911058130, 111.2489096053143669 ) ) ;
#119951=CARTESIAN_POINT ( 'NONE',  ( -19.05341960407617563, 5.049401038297882671, 58.54275706135234003 ) ) ;
#119952=CARTESIAN_POINT ( 'NONE',  ( 0.05219959533909260263, 19.03943276465977164, 54.99890960531435979 ) ) ;
#119953=CARTESIAN_POINT ( 'NONE',  ( -19.02544592524342804, 5.153800228976336051, 91.04057627198100988 ) ) ;
#119954=CARTESIAN_POINT ( 'NONE',  ( -18.67979575497178146, -10.72451020669898902, 91.66557627198103830 ) ) ;
#119955=CARTESIAN_POINT ( 'NONE',  ( 16.55341960407611168, 4.379528057220329451, 98.95724293864770971 ) ) ;
#119956=CARTESIAN_POINT ( 'NONE',  ( -16.46253265017146816, -9.564922557961047289, 49.16775706135233293 ) ) ;
#119957=CARTESIAN_POINT ( 'NONE',  ( -21.53943276465977519, 0.05219959533907696930, 76.24890960531435269 ) ) ;
#119958=CARTESIAN_POINT ( 'NONE',  ( 21.55341960407610458, 5.719274019375980345, 53.95724293864770260 ) ) ;
#119959=CARTESIAN_POINT ( 'NONE',  ( 8.224510206698953496, -14.34966873604960469, 37.91557627198102409 ) ) ;
#119960=CARTESIAN_POINT ( 'NONE',  ( -10.72451020669870658, -18.67979575497194134, 109.5844237280190328 ) ) ;
#119961=CARTESIAN_POINT ( 'NONE',  ( 9.564922557960805705, 16.46253265017160317, 74.58224293864769550 ) ) ;
#119962=CARTESIAN_POINT ( 'NONE',  ( 19.03943276465977164, -0.05219959533909143690, 38.74890960531436690 ) ) ;
#119963=CARTESIAN_POINT ( 'NONE',  ( -15.80617190586768217, 15.72974639402176855, 43.12609039468568284 ) ) ;
#119964=CARTESIAN_POINT ( 'NONE',  ( -21.55341960407619339, 5.719274019375674811, 43.54275706135235424 ) ) ;
#119965=CARTESIAN_POINT ( 'NONE',  ( -16.51473224551069308, -9.474510206698971260, 46.66557627198102409 ) ) ;
#119966=CARTESIAN_POINT ( 'NONE',  ( 5.823673210054444382, -21.52544592524334988, 20.20942372801900788 ) ) ;
#119967=CARTESIAN_POINT ( 'NONE',  ( -0.05219959533936034679, 19.03943276465977164, 67.50109039468566152 ) ) ;
#119968=CARTESIAN_POINT ( 'NONE',  ( -9.474510206698964154, 16.51473224551069663, 30.41557627198102054 ) ) ;
#119969=CARTESIAN_POINT ( 'NONE',  ( -4.483927247898782831, 16.52544592524335698, 32.70942372801900433 ) ) ;
#119970=CARTESIAN_POINT ( 'NONE',  ( -16.46253265017160317, 9.564922557960807481, 25.83224293864769194 ) ) ;
#119971=CARTESIAN_POINT ( 'NONE',  ( -12.06949235617739369, -12.14591786802326823, 79.37609039468567573 ) ) ;
#119972=CARTESIAN_POINT ( 'NONE',  ( 16.46253265017160672, -9.564922557960803928, 33.33224293864770260 ) ) ;
#119974=CARTESIAN_POINT ( 'NONE',  ( -5.049401038298153566, 19.05341960407611168, 90.20724293864766707 ) ) ;
#119975=CARTESIAN_POINT ( 'NONE',  ( 9.564922557960805705, 16.46253265017160317, 24.58224293864769194 ) ) ;
#119976=CARTESIAN_POINT ( 'NONE',  ( 18.67979575497178502, 10.72451020669898547, 79.16557627198103830 ) ) ;
#119977=CARTESIAN_POINT ( 'NONE',  ( -8.224510206698735004, -14.34966873604973081, 44.58442372801901854 ) ) ;
#119978=CARTESIAN_POINT ( 'NONE',  ( -0.05219959533937732626, 21.53943276465977519, 97.50109039468567573 ) ) ;
#119979=CARTESIAN_POINT ( 'NONE',  ( -16.51473224551069308, -9.474510206698971260, 36.66557627198102409 ) ) ;
#119980=CARTESIAN_POINT ( 'NONE',  ( 14.29746914071049879, -8.314922557960816363, 38.33224293864768839 ) ) ;
#119981=CARTESIAN_POINT ( 'NONE',  ( 8.314922557960818139, 14.29746914071049879, 69.58224293864769550 ) ) ;
#119982=CARTESIAN_POINT ( 'NONE',  ( -19.02544592524342804, 5.153800228976336051, 61.04057627198103120 ) ) ;
#119983=CARTESIAN_POINT ( 'NONE',  ( -13.89961937509957401, -13.97604488694547875, 19.37609039468566507 ) ) ;
#119984=CARTESIAN_POINT ( 'NONE',  ( -5.823673210054431948, 21.52544592524334988, 27.70942372801901854 ) ) ;
#119985=CARTESIAN_POINT ( 'NONE',  ( -19.05341960407611168, -5.049401038298163336, 81.45724293864769550 ) ) ;
#119986=CARTESIAN_POINT ( 'NONE',  ( 0.05219959533937995610, -21.53943276465977519, 80.00109039468568994 ) ) ;
#119987=CARTESIAN_POINT ( 'NONE',  ( -4.483927247898782831, 16.52544592524335698, 52.70942372801902565 ) ) ;
#119988=CARTESIAN_POINT ( 'NONE',  ( 0.05219959533934541429, -16.53943276465976808, 30.00109039468568284 ) ) ;
#119989=CARTESIAN_POINT ( 'NONE',  ( 16.53943276465976808, -0.05219959533910856209, 88.74890960531436690 ) ) ;
#119990=CARTESIAN_POINT ( 'NONE',  ( 5.719274019375673035, 21.55341960407619339, 102.2927570613523613 ) ) ;
#119991=CARTESIAN_POINT ( 'NONE',  ( -8.224510206698948167, 14.34966873604960824, 35.41557627198102409 ) ) ;
#119992=CARTESIAN_POINT ( 'NONE',  ( -19.03943276465977164, 0.05219959533909376836, 26.24890960531435624 ) ) ;
#119993=CARTESIAN_POINT ( 'NONE',  ( 14.34966873604972726, -8.224510206698740333, 55.83442372801901854 ) ) ;
#119994=CARTESIAN_POINT ( 'NONE',  ( 16.52544592524342804, -4.483927247898539470, 48.54057627198103120 ) ) ;
#119995=CARTESIAN_POINT ( 'NONE',  ( -16.53943276465976808, -0.05219959533934237506, 103.7510903946857042 ) ) ;
#119996=CARTESIAN_POINT ( 'NONE',  ( -9.474510206698964154, 16.51473224551069663, 115.4155762719810241 ) ) ;
#119997=CARTESIAN_POINT ( 'NONE',  ( 15.80617190586746368, 15.72974639402197994, 29.37390960531435269 ) ) ;
#119998=CARTESIAN_POINT ( 'NONE',  ( -19.03943276465977164, -0.05219959533935918106, 18.75109039468567218 ) ) ;
#119999=CARTESIAN_POINT ( 'NONE',  ( -4.379528057220328563, 16.55341960407611168, 85.20724293864770971 ) ) ;
#120000=CARTESIAN_POINT ( 'NONE',  ( -0.05219959533909027116, -19.03943276465977164, 97.49890960531436690 ) ) ;
#120002=CARTESIAN_POINT ( 'NONE',  ( -12.06949235617739369, -12.14591786802326823, 34.37609039468568284 ) ) ;
#120003=CARTESIAN_POINT ( 'NONE',  ( 19.03943276465977164, -0.05219959533909143690, 43.74890960531435979 ) ) ;
#120004=CARTESIAN_POINT ( 'NONE',  ( -8.224510206698735004, -14.34966873604973081, 49.58442372801901143 ) ) ;
#120005=DIRECTION ( 'NONE',  ( 0.000000000000000000, 0.000000000000000000, -1.000000000000000000 ) ) ;
#120006=CARTESIAN_POINT ( 'NONE',  ( 19.03943276465977164, 0.05219959533936151252, 46.25109039468566863 ) ) ;
#120007=CARTESIAN_POINT ( 'NONE',  ( -16.51473224551069308, -9.474510206698971260, 46.66557627198102409 ) ) ;
#120008=CARTESIAN_POINT ( 'NONE',  ( 12.14591786802327356, -12.06949235617739191, 75.62609039468567573 ) ) ;
#120009=CARTESIAN_POINT ( 'NONE',  ( 19.03943276465977164, 0.05219959533936151252, 81.25109039468567573 ) ) ;
#120010=CARTESIAN_POINT ( 'NONE',  ( 16.51473224551083163, -9.474510206698727899, 25.83442372801900078 ) ) ;
#120011=CARTESIAN_POINT ( 'NONE',  ( 16.46253265017160672, -9.564922557960803928, 58.33224293864769550 ) ) ;
#120012=CARTESIAN_POINT ( 'NONE',  ( -4.483927247898539470, -16.52544592524342804, 97.29057627198105251 ) ) ;
#120013=CARTESIAN_POINT ( 'NONE',  ( -19.02544592524334988, -5.153800228976617603, 63.95942372801899012 ) ) ;
#120014=CARTESIAN_POINT ( 'NONE',  ( 10.72451020669898902, -18.67979575497178502, 67.91557627198102409 ) ) ;
#120015=CARTESIAN_POINT ( 'NONE',  ( -19.03943276465977164, -0.05219959533935918106, 38.75109039468566152 ) ) ;
#120016=CARTESIAN_POINT ( 'NONE',  ( 19.03943276465977164, -0.05219959533909143690, 98.74890960531436690 ) ) ;
#120017=CARTESIAN_POINT ( 'NONE',  ( 21.55341960407610458, 5.719274019375980345, 73.95724293864769550 ) ) ;
#120018=CARTESIAN_POINT ( 'NONE',  ( -16.29526858892876007, 7.335722546920119491, 84.20329402199796220 ) ) ;
#120019=CARTESIAN_POINT ( 'NONE',  ( 19.02544592524334988, 5.153800228976608722, 96.45942372801897591 ) ) ;
#120020=CARTESIAN_POINT ( 'NONE',  ( 9.474510206698729675, 16.51473224551082808, 97.08442372801900433 ) ) ;
#120021=CARTESIAN_POINT ( 'NONE',  ( -14.29746914071037622, -8.314922557961029526, 34.16775706135234714 ) ) ;
#120022=CARTESIAN_POINT ( 'NONE',  ( -16.51473224551069308, -9.474510206698971260, 41.66557627198103120 ) ) ;
#120023=CARTESIAN_POINT ( 'NONE',  ( -13.97604488694527625, -13.89961937509977652, 106.8739096053143669 ) ) ;
#120024=CARTESIAN_POINT ( 'NONE',  ( -10.81492255796078084, -18.62759615963271287, 92.08224293864769550 ) ) ;
#120025=CARTESIAN_POINT ( 'NONE',  ( 18.67979575497194134, -10.72451020669871369, 55.83442372801901854 ) ) ;
#120026=CARTESIAN_POINT ( 'NONE',  ( -19.03943276465977164, -0.05219959533935918106, 103.7510903946856757 ) ) ;
#120027=CARTESIAN_POINT ( 'NONE',  ( 5.153800228976615827, -19.02544592524334988, 20.20942372801899722 ) ) ;
#120028=CARTESIAN_POINT ( 'NONE',  ( 4.483927247898790824, -16.52544592524335698, 105.2094237280190328 ) ) ;
#120029=CARTESIAN_POINT ( 'NONE',  ( 18.67979575497178502, 10.72451020669898547, 94.16557627198103830 ) ) ;
#120030=CARTESIAN_POINT ( 'NONE',  ( -16.55341960407611168, -4.379528057220339221, 46.45724293864769550 ) ) ;
#120031=CARTESIAN_POINT ( 'NONE',  ( -19.05341960407617563, 5.049401038297882671, 78.54275706135233293 ) ) ;
#120032=CARTESIAN_POINT ( 'NONE',  ( 13.97604488694548053, -13.89961937509957401, 60.62609039468564731 ) ) ;
#120033=CARTESIAN_POINT ( 'NONE',  ( 21.52544592524334988, 5.823673210054432836, 76.45942372801901854 ) ) ;
#120034=CARTESIAN_POINT ( 'NONE',  ( 13.89961937509957401, 13.97604488694547697, 41.87609039468566152 ) ) ;
#120035=CARTESIAN_POINT ( 'NONE',  ( 14.34966873604960469, 8.224510206698951720, 109.1655762719810383 ) ) ;
#120036=CARTESIAN_POINT ( 'NONE',  ( 21.53943276465977519, -0.05219959533907433946, 48.74890960531435979 ) ) ;
#120037=CARTESIAN_POINT ( 'NONE',  ( -16.53943276465976808, 0.05219959533911058130, 41.24890960531435269 ) ) ;
#120038=CARTESIAN_POINT ( 'NONE',  ( 18.67979575497194134, -10.72451020669871369, 105.8344237280190328 ) ) ;
#120039=CARTESIAN_POINT ( 'NONE',  ( -12.14591786802326823, 12.06949235617739902, 78.12609039468570415 ) ) ;
#120040=CARTESIAN_POINT ( 'NONE',  ( 0.05219959533910956823, 16.53943276465976808, 29.99890960531435979 ) ) ;
#120041=CARTESIAN_POINT ( 'NONE',  ( -10.72451020669870658, -18.67979575497194134, 64.58442372801900433 ) ) ;
#120042=CARTESIAN_POINT ( 'NONE',  ( 21.53943276465977519, 0.05219959533937863772, 66.25109039468567573 ) ) ;
#120043=CARTESIAN_POINT ( 'NONE',  ( 10.81492255796078972, 18.62759615963270932, 69.58224293864769550 ) ) ;
#120045=CARTESIAN_POINT ( 'NONE',  ( 19.03943276465977164, -0.05219959533909143690, 28.74890960531435624 ) ) ;
#120046=CARTESIAN_POINT ( 'NONE',  ( 18.67979575497194134, -10.72451020669871369, 45.83442372801901854 ) ) ;
#120047=CARTESIAN_POINT ( 'NONE',  ( -12.14591786802309592, -12.06949235617757132, 111.8739096053143669 ) ) ;
#120048=CARTESIAN_POINT ( 'NONE',  ( -5.153800228976328057, -19.02544592524343514, 37.29057627198102409 ) ) ;
#120049=CARTESIAN_POINT ( 'NONE',  ( 14.29746914071049879, -8.314922557960816363, 78.33224293864770971 ) ) ;
#120050=CARTESIAN_POINT ( 'NONE',  ( -19.03943276465977164, 0.05219959533909376836, 86.24890960531436690 ) ) ;
#120051=CARTESIAN_POINT ( 'NONE',  ( -14.34966873604960291, -8.224510206698953496, 26.66557627198103475 ) ) ;
#120052=CARTESIAN_POINT ( 'NONE',  ( 4.483927247898545687, 16.52544592524342804, 104.7905762719810241 ) ) ;
#120053=CARTESIAN_POINT ( 'NONE',  ( 15.80617190586746368, 15.72974639402197994, 74.37390960531436690 ) ) ;
#120054=CARTESIAN_POINT ( 'NONE',  ( 21.52544592524344225, -5.823673210054117533, 108.5405762719810241 ) ) ;
#120056=CARTESIAN_POINT ( 'NONE',  ( 16.46253265017160672, -9.564922557960803928, 68.33224293864770971 ) ) ;
#120057=CARTESIAN_POINT ( 'NONE',  ( 16.53943276465976808, 0.05219959533934440121, 21.25109039468567218 ) ) ;
#120058=CARTESIAN_POINT ( 'NONE',  ( 18.62759615963271287, -10.81492255796078972, 63.33224293864770260 ) ) ;
#120059=CARTESIAN_POINT ( 'NONE',  ( 0.05219959533937995610, -21.53943276465977519, 80.00109039468568994 ) ) ;
#120060=CARTESIAN_POINT ( 'NONE',  ( -13.97604488694527625, -13.89961937509977652, 81.87390960531436690 ) ) ;
#120061=CARTESIAN_POINT ( 'NONE',  ( 16.46253265017160672, -9.564922557960803928, 108.3322429386476955 ) ) ;
#120062=CARTESIAN_POINT ( 'NONE',  ( -14.34966873604972548, 8.224510206698743886, 83.33442372801903275 ) ) ;
#120063=CARTESIAN_POINT ( 'NONE',  ( -18.67979575497193778, 10.72451020669871902, 53.33442372801901854 ) ) ;
#120064=CARTESIAN_POINT ( 'NONE',  ( 0.05219959533937995610, -21.53943276465977519, 100.0010903946857042 ) ) ;
#120065=CARTESIAN_POINT ( 'NONE',  ( -16.52544592524335698, -4.483927247898792601, 63.95942372801901854 ) ) ;
#120066=CARTESIAN_POINT ( 'NONE',  ( 10.72451020669898902, -18.67979575497178502, 112.9155762719810383 ) ) ;
#120067=FACE_OUTER_BOUND ( 'NONE', #53013, .T. ) ;
#120068=CARTESIAN_POINT ( 'NONE',  ( -0.05219959533907301413, -21.53943276465977519, 92.49890960531436690 ) ) ;
#120069=CARTESIAN_POINT ( 'NONE',  ( -13.97604488694547697, 13.89961937509957934, 43.12609039468566152 ) ) ;
#120070=CARTESIAN_POINT ( 'NONE',  ( 18.62759615963271287, -10.81492255796078972, 53.33224293864769550 ) ) ;
#120071=CARTESIAN_POINT ( 'NONE',  ( 0.05219959533909260263, 19.03943276465977164, 99.99890960531436690 ) ) ;
#120072=CARTESIAN_POINT ( 'NONE',  ( 0.05219959533910956823, 16.53943276465976808, 39.99890960531436690 ) ) ;
#120073=CARTESIAN_POINT ( 'NONE',  ( -17.50000000000001421, 5.622605283950871780, 63.68792689403893093 ) ) ;
#120076=CARTESIAN_POINT ( 'NONE',  ( -13.97604488694547697, 13.89961937509957934, 98.12609039468566152 ) ) ;
#120077=CARTESIAN_POINT ( 'NONE',  ( -10.81492255796078084, -18.62759615963271287, 72.08224293864769550 ) ) ;
#120078=CARTESIAN_POINT ( 'NONE',  ( -12.06949235617756955, 12.14591786802309770, 55.62390960531436690 ) ) ;
#120079=CARTESIAN_POINT ( 'NONE',  ( 14.34966873604972726, -8.224510206698740333, 35.83442372801901143 ) ) ;
#120080=CARTESIAN_POINT ( 'NONE',  ( 19.05341960407611168, 5.049401038298154454, 43.95724293864769550 ) ) ;
#120081=CARTESIAN_POINT ( 'NONE',  ( 15.80617190586746368, 15.72974639402197994, 109.3739096053143811 ) ) ;
#120082=CARTESIAN_POINT ( 'NONE',  ( -19.02544592524334988, -5.153800228976617603, 88.95942372801897591 ) ) ;
#120083=CARTESIAN_POINT ( 'NONE',  ( 16.46253265017160672, -9.564922557960803928, 78.33224293864769550 ) ) ;
#120084=CARTESIAN_POINT ( 'NONE',  ( -5.049401038298153566, 19.05341960407611168, 80.20724293864769550 ) ) ;
#120085=CARTESIAN_POINT ( 'NONE',  ( -0.05219959533907301413, -21.53943276465977519, 72.49890960531435269 ) ) ;
#120086=CARTESIAN_POINT ( 'NONE',  ( 13.97604488694527802, 13.89961937509977652, 29.37390960531435979 ) ) ;
#120088=CARTESIAN_POINT ( 'NONE',  ( 8.224510206698953496, -14.34966873604960469, 57.91557627198103120 ) ) ;
#120089=CARTESIAN_POINT ( 'NONE',  ( -13.89961937509977652, 13.97604488694528158, 90.62390960531432427 ) ) ;
#120091=CARTESIAN_POINT ( 'NONE',  ( -19.02544592524334988, -5.153800228976617603, 53.95942372801898301 ) ) ;
#120092=CARTESIAN_POINT ( 'NONE',  ( 21.55341960407610458, 5.719274019375980345, 78.95724293864769550 ) ) ;
#120093=CARTESIAN_POINT ( 'NONE',  ( -19.03943276465977164, -0.05219959533935918106, 38.75109039468566152 ) ) ;
#120094=CARTESIAN_POINT ( 'NONE',  ( 16.46253265017160672, -9.564922557960803928, 93.33224293864769550 ) ) ;
#120096=CARTESIAN_POINT ( 'NONE',  ( 15.72974639402199770, -15.80617190586745480, 28.12390960531435979 ) ) ;
#120097=CARTESIAN_POINT ( 'NONE',  ( -19.02544592524342804, 5.153800228976336051, 76.04057627198102409 ) ) ;
#120098=CARTESIAN_POINT ( 'NONE',  ( 5.719274019375673035, 21.55341960407619339, 52.29275706135236135 ) ) ;
#120099=CARTESIAN_POINT ( 'NONE',  ( -13.97604488694527625, -13.89961937509977652, 21.87390960531435979 ) ) ;
#120100=CARTESIAN_POINT ( 'NONE',  ( -15.80617190586745835, -15.72974639402198527, 111.8739096053143669 ) ) ;
#120102=CARTESIAN_POINT ( 'NONE',  ( 21.53943276465977519, 0.05219959533937863772, 41.25109039468568284 ) ) ;
#120104=CARTESIAN_POINT ( 'NONE',  ( 13.89961937509977652, -13.97604488694527269, 98.12390960531433848 ) ) ;
#120105=VECTOR ( 'NONE', #62, 1000.000000000000000 ) ;
#120107=CARTESIAN_POINT ( 'NONE',  ( 21.55341960407610458, 5.719274019375980345, 108.9572429386476955 ) ) ;
#120108=CARTESIAN_POINT ( 'NONE',  ( 13.97604488694527802, 13.89961937509977652, 64.37390960531436690 ) ) ;
#120109=CARTESIAN_POINT ( 'NONE',  ( -19.05341960407617563, 5.049401038297882671, 113.5427570613523471 ) ) ;
#120111=CARTESIAN_POINT ( 'NONE',  ( 0.05219959533937995610, -21.53943276465977519, 105.0010903946856757 ) ) ;
#120112=CARTESIAN_POINT ( 'NONE',  ( -9.564922557960796823, -16.46253265017161027, 42.08224293864769550 ) ) ;
#120113=CARTESIAN_POINT ( 'NONE',  ( -5.719274019375665041, -21.55341960407619695, 94.79275706135234714 ) ) ;
#120114=CARTESIAN_POINT ( 'NONE',  ( -19.03943276465977164, 0.05219959533909376836, 86.24890960531436690 ) ) ;
#120115=CARTESIAN_POINT ( 'NONE',  ( 0.05219959533937995610, -21.53943276465977519, 60.00109039468568284 ) ) ;
#120117=CARTESIAN_POINT ( 'NONE',  ( 9.474510206698971260, -16.51473224551069308, 102.9155762719810241 ) ) ;
#120118=CARTESIAN_POINT ( 'NONE',  ( -17.49999999999999645, 3.471454075611625001, 29.48332581144368447 ) ) ;
#120119=CARTESIAN_POINT ( 'NONE',  ( 8.224510206698742110, 14.34966873604972548, 57.08442372801901854 ) ) ;
#120120=CARTESIAN_POINT ( 'NONE',  ( -12.06949235617739369, -12.14591786802326823, 69.37609039468567573 ) ) ;
#120121=CARTESIAN_POINT ( 'NONE',  ( -5.719274019375665041, -21.55341960407619695, 54.79275706135235424 ) ) ;
#120122=CARTESIAN_POINT ( 'NONE',  ( 5.823673210054444382, -21.52544592524334988, 90.20942372801903275 ) ) ;
#120124=CARTESIAN_POINT ( 'NONE',  ( -12.06949235617739369, -12.14591786802326823, 34.37609039468568284 ) ) ;
#120125=CARTESIAN_POINT ( 'NONE',  ( -19.02544592524342804, 5.153800228976336051, 71.04057627198099567 ) ) ;
#120126=CARTESIAN_POINT ( 'NONE',  ( 0.05219959533909260263, 19.03943276465977164, 94.99890960531436690 ) ) ;
#120127=CARTESIAN_POINT ( 'NONE',  ( 17.05587630539784527, 6.762274262135707481, 41.75819690962689634 ) ) ;
#120128=CARTESIAN_POINT ( 'NONE',  ( -13.97604488694527625, -13.89961937509977652, 31.87390960531435979 ) ) ;
#120129=CARTESIAN_POINT ( 'NONE',  ( 0.05219959533907565091, 21.53943276465977519, 24.99890960531435624 ) ) ;
#120130=CARTESIAN_POINT ( 'NONE',  ( -14.29746914071037622, -8.314922557961029526, 89.16775706135236135 ) ) ;
#120131=CARTESIAN_POINT ( 'NONE',  ( -12.06949235617756955, 12.14591786802309770, 85.62390960531436690 ) ) ;
#120132=CARTESIAN_POINT ( 'NONE',  ( 16.51473224551069308, 9.474510206698969483, 74.16557627198103830 ) ) ;
#120133=CARTESIAN_POINT ( 'NONE',  ( 5.823673210054444382, -21.52544592524334988, 90.20942372801903275 ) ) ;
#120135=CARTESIAN_POINT ( 'NONE',  ( -12.06949235617739369, -12.14591786802326823, 24.37609039468567573 ) ) ;
#120136=CARTESIAN_POINT ( 'NONE',  ( -12.06949235617756955, 12.14591786802309770, 75.62390960531439532 ) ) ;
#120137=CARTESIAN_POINT ( 'NONE',  ( -0.05219959533937732626, 21.53943276465977519, 37.50109039468568284 ) ) ;
#120138=CARTESIAN_POINT ( 'NONE',  ( 0.05219959533907565091, 21.53943276465977519, 69.99890960531435269 ) ) ;
#120139=CARTESIAN_POINT ( 'NONE',  ( 5.153800228976615827, -19.02544592524334988, 35.20942372801899722 ) ) ;
#120141=CARTESIAN_POINT ( 'NONE',  ( 9.564922557960805705, 16.46253265017160317, 79.58224293864769550 ) ) ;
#120142=CARTESIAN_POINT ( 'NONE',  ( -4.379528057220328563, 16.55341960407611168, 50.20724293864769550 ) ) ;
#120143=CARTESIAN_POINT ( 'NONE',  ( 8.224510206698953496, -14.34966873604960469, 32.91557627198102409 ) ) ;
#120144=CARTESIAN_POINT ( 'NONE',  ( 8.224510206698742110, 14.34966873604972548, 112.0844237280190185 ) ) ;
#120145=CARTESIAN_POINT ( 'NONE',  ( -9.474510206698720793, -16.51473224551083518, 69.58442372801901854 ) ) ;
#120146=CARTESIAN_POINT ( 'NONE',  ( 16.46253265017146816, 9.564922557961045513, 76.66775706135234714 ) ) ;
#120147=CARTESIAN_POINT ( 'NONE',  ( -21.55341960407610458, -5.719274019375992779, 26.45724293864768839 ) ) ;
#120149=CARTESIAN_POINT ( 'NONE',  ( -4.379528057220328563, 16.55341960407611168, 90.20724293864770971 ) ) ;
#120151=CARTESIAN_POINT ( 'NONE',  ( 19.02544592524343514, -5.153800228976328945, 28.54057627198102409 ) ) ;
#120152=CARTESIAN_POINT ( 'NONE',  ( -10.81492255796078084, -18.62759615963271287, 42.08224293864769550 ) ) ;
#120153=CARTESIAN_POINT ( 'NONE',  ( -0.05219959533907301413, -21.53943276465977519, 62.49890960531436690 ) ) ;
#120154=CARTESIAN_POINT ( 'NONE',  ( 14.34966873604960469, 8.224510206698951720, 114.1655762719810383 ) ) ;
#120155=CARTESIAN_POINT ( 'NONE',  ( -16.55341960407617563, 4.379528057220093196, 68.54275706135234714 ) ) ;
#120156=CARTESIAN_POINT ( 'NONE',  ( 5.049401038298161559, -19.05341960407611168, 47.70724293864770260 ) ) ;
#120157=CARTESIAN_POINT ( 'NONE',  ( -15.80617190586768217, 15.72974639402176855, 58.12609039468568994 ) ) ;
#120158=CARTESIAN_POINT ( 'NONE',  ( -16.52544592524342804, 4.483927247898546575, 111.0405762719810525 ) ) ;
#120159=CARTESIAN_POINT ( 'NONE',  ( 9.564922557961047289, -16.46253265017146816, 95.41775706135233293 ) ) ;
#120162=CARTESIAN_POINT ( 'NONE',  ( -0.05219959533907301413, -21.53943276465977519, 32.49890960531435979 ) ) ;
#120164=CARTESIAN_POINT ( 'NONE',  ( -5.719274019375665041, -21.55341960407619695, 64.79275706135234714 ) ) ;
#120165=CARTESIAN_POINT ( 'NONE',  ( -4.379528057220086978, -16.55341960407618274, 49.79275706135234714 ) ) ;
#120166=CARTESIAN_POINT ( 'NONE',  ( -12.14591786802309592, -12.06949235617757132, 41.87390960531435979 ) ) ;
#120167=CARTESIAN_POINT ( 'NONE',  ( 10.81492255796078972, 18.62759615963270932, 69.58224293864769550 ) ) ;
#120168=CARTESIAN_POINT ( 'NONE',  ( 18.62759615963271287, -10.81492255796078972, 63.33224293864770260 ) ) ;
#120170=CARTESIAN_POINT ( 'NONE',  ( -13.89961937509957401, -13.97604488694547875, 84.37609039468567573 ) ) ;
#120171=CARTESIAN_POINT ( 'NONE',  ( 0.05219959533909260263, 19.03943276465977164, 114.9989096053143669 ) ) ;
#120172=CARTESIAN_POINT ( 'NONE',  ( 13.97604488694527802, 13.89961937509977652, 54.37390960531435979 ) ) ;
#120173=CARTESIAN_POINT ( 'NONE',  ( 4.483927247898545687, 16.52544592524342804, 109.7905762719810383 ) ) ;
#120175=CARTESIAN_POINT ( 'NONE',  ( 19.02544592524343514, -5.153800228976328945, 108.5405762719810383 ) ) ;
#120177=CARTESIAN_POINT ( 'NONE',  ( 12.06949235617739724, 12.14591786802326823, 66.87609039468568994 ) ) ;
#120178=CARTESIAN_POINT ( 'NONE',  ( 10.72451020669898902, -18.67979575497178502, 97.91557627198103830 ) ) ;
#120179=CARTESIAN_POINT ( 'NONE',  ( -0.05219959533909027116, -19.03943276465977164, 67.49890960531436690 ) ) ;
#120180=CARTESIAN_POINT ( 'NONE',  ( -10.81492255796105439, 18.62759615963255655, 42.91775706135235424 ) ) ;
#120181=CARTESIAN_POINT ( 'NONE',  ( 19.02544592524343514, -5.153800228976328945, 98.54057627198100988 ) ) ;
#120184=CARTESIAN_POINT ( 'NONE',  ( 0.05219959533937995610, -21.53943276465977519, 30.00109039468568284 ) ) ;
#120185=CARTESIAN_POINT ( 'NONE',  ( -9.564922557960796823, -16.46253265017161027, 22.08224293864768839 ) ) ;
#120186=CARTESIAN_POINT ( 'NONE',  ( 16.46253265017146816, 9.564922557961045513, 86.66775706135233293 ) ) ;
#120187=CARTESIAN_POINT ( 'NONE',  ( 13.97604488694548053, -13.89961937509957401, 45.62609039468566863 ) ) ;
#120188=CARTESIAN_POINT ( 'NONE',  ( 5.719274019375991003, -21.55341960407610458, 97.70724293864772392 ) ) ;
#120189=CARTESIAN_POINT ( 'NONE',  ( 19.03943276465977164, 0.05219959533936151252, 31.25109039468566863 ) ) ;
#120190=CARTESIAN_POINT ( 'NONE',  ( -5.049401038297874678, -19.05341960407617918, 54.79275706135234003 ) ) ;
#120191=CARTESIAN_POINT ( 'NONE',  ( 4.379528057220092307, 16.55341960407617563, 87.29275706135236135 ) ) ;
#120194=CARTESIAN_POINT ( 'NONE',  ( 13.89961937509977652, -13.97604488694527269, 78.12390960531433848 ) ) ;
#120195=CARTESIAN_POINT ( 'NONE',  ( 15.80617190586769283, -15.72974639402175789, 80.62609039468567573 ) ) ;
#120196=CARTESIAN_POINT ( 'NONE',  ( 5.719274019375673035, 21.55341960407619339, 97.29275706135234714 ) ) ;
#120198=CARTESIAN_POINT ( 'NONE',  ( 16.46253265017160672, -9.564922557960803928, 93.33224293864769550 ) ) ;
#120199=CARTESIAN_POINT ( 'NONE',  ( 0.05219959533937995610, -21.53943276465977519, 60.00109039468568284 ) ) ;
#120200=CARTESIAN_POINT ( 'NONE',  ( -13.89961937509957401, -13.97604488694547875, 99.37609039468567573 ) ) ;
#120201=CARTESIAN_POINT ( 'NONE',  ( -13.89961937509977652, 13.97604488694528158, 60.62390960531436690 ) ) ;
#120202=CARTESIAN_POINT ( 'NONE',  ( 15.72974639402199770, -15.80617190586745480, 23.12390960531436335 ) ) ;
#120203=CARTESIAN_POINT ( 'NONE',  ( -9.564922557960796823, -16.46253265017161027, 77.08224293864769550 ) ) ;
#120205=CARTESIAN_POINT ( 'NONE',  ( 5.049401038298161559, -19.05341960407611168, 62.70724293864769550 ) ) ;
#120206=CARTESIAN_POINT ( 'NONE',  ( 0.05219959533909260263, 19.03943276465977164, 54.99890960531435979 ) ) ;
#120207=CARTESIAN_POINT ( 'NONE',  ( 21.55341960407610458, 5.719274019375980345, 113.9572429386477239 ) ) ;
#120208=CARTESIAN_POINT ( 'NONE',  ( 12.06949235617739724, 12.14591786802326823, 81.87609039468568994 ) ) ;
#120210=CARTESIAN_POINT ( 'NONE',  ( 16.46253265017146816, 9.564922557961045513, 46.66775706135233293 ) ) ;
#120211=CARTESIAN_POINT ( 'NONE',  ( -13.97604488694527625, -13.89961937509977652, 81.87390960531436690 ) ) ;
#120212=CARTESIAN_POINT ( 'NONE',  ( -8.314922557960811034, -14.29746914071050412, 67.08224293864770971 ) ) ;
#120213=CARTESIAN_POINT ( 'NONE',  ( 16.53943276465976808, -0.05219959533910856209, 108.7489096053143669 ) ) ;
#120214=CARTESIAN_POINT ( 'NONE',  ( 15.72974639402199770, -15.80617190586745480, 23.12390960531436335 ) ) ;
#120215=CARTESIAN_POINT ( 'NONE',  ( -5.049401038298153566, 19.05341960407611168, 105.2072429386476671 ) ) ;
#120216=CARTESIAN_POINT ( 'NONE',  ( 16.52544592524342804, -4.483927247898539470, 78.54057627198103830 ) ) ;
#120218=CARTESIAN_POINT ( 'NONE',  ( 19.03943276465977164, 0.05219959533936151252, 36.25109039468567573 ) ) ;
#120219=CARTESIAN_POINT ( 'NONE',  ( -4.379528057220086978, -16.55341960407618274, 99.79275706135234714 ) ) ;
#120220=CARTESIAN_POINT ( 'NONE',  ( 19.05341960407611168, 5.049401038298154454, 88.95724293864769550 ) ) ;
#120221=CARTESIAN_POINT ( 'NONE',  ( 15.72974639402176855, 15.80617190586768217, 56.87609039468568994 ) ) ;
#120222=CARTESIAN_POINT ( 'NONE',  ( -10.81492255796078084, -18.62759615963271287, 42.08224293864769550 ) ) ;
#120223=CARTESIAN_POINT ( 'NONE',  ( 0.05219959533907565091, 21.53943276465977519, 109.9989096053143527 ) ) ;
#120224=CARTESIAN_POINT ( 'NONE',  ( -0.05219959533907301413, -21.53943276465977519, 72.49890960531435269 ) ) ;
#120225=CARTESIAN_POINT ( 'NONE',  ( -12.06949235617756955, 12.14591786802309770, 100.6239096053143811 ) ) ;
#120226=CARTESIAN_POINT ( 'NONE',  ( 9.564922557961047289, -16.46253265017146816, 60.41775706135233293 ) ) ;
#120227=CARTESIAN_POINT ( 'NONE',  ( 5.049401038298161559, -19.05341960407611168, 32.70724293864768129 ) ) ;
#120228=CARTESIAN_POINT ( 'NONE',  ( -0.05219959533909027116, -19.03943276465977164, 87.49890960531436690 ) ) ;
#120229=CARTESIAN_POINT ( 'NONE',  ( -19.05341960407611168, -5.049401038298163336, 86.45724293864769550 ) ) ;
#120230=CARTESIAN_POINT ( 'NONE',  ( -12.14591786802309592, -12.06949235617757132, 96.87390960531436690 ) ) ;
#120231=CARTESIAN_POINT ( 'NONE',  ( 16.55341960407611168, 4.379528057220329451, 23.95724293864769550 ) ) ;
#120232=CARTESIAN_POINT ( 'NONE',  ( -4.379528057220086978, -16.55341960407618274, 44.79275706135234714 ) ) ;
#120233=CARTESIAN_POINT ( 'NONE',  ( 21.55341960407619695, -5.719274019375665929, 101.0427570613523756 ) ) ;
#120234=CARTESIAN_POINT ( 'NONE',  ( 5.049401038298161559, -19.05341960407611168, 107.7072429386476955 ) ) ;
#120235=CARTESIAN_POINT ( 'NONE',  ( -10.72451020669870658, -18.67979575497194134, 39.58442372801901143 ) ) ;
#120236=CARTESIAN_POINT ( 'NONE',  ( -19.03943276465977164, 0.05219959533909376836, 41.24890960531435269 ) ) ;
#120237=CARTESIAN_POINT ( 'NONE',  ( -8.224510206698735004, -14.34966873604973081, 39.58442372801901143 ) ) ;
#120238=CARTESIAN_POINT ( 'NONE',  ( -19.03943276465977164, -0.05219959533935918106, 103.7510903946856757 ) ) ;
#120239=EDGE_CURVE ( 'NONE', #9179, #123381, #57207, .T. ) ;
#120240=CARTESIAN_POINT ( 'NONE',  ( 13.89961937509977652, -13.97604488694527269, 33.12390960531434558 ) ) ;
#120241=CARTESIAN_POINT ( 'NONE',  ( -16.55341960407611168, -4.379528057220339221, 91.45724293864769550 ) ) ;
#120242=CARTESIAN_POINT ( 'NONE',  ( 21.55341960407610458, 5.719274019375980345, 108.9572429386476955 ) ) ;
#120243=CARTESIAN_POINT ( 'NONE',  ( 19.02544592524334988, 5.153800228976608722, 81.45942372801897591 ) ) ;
#120244=CARTESIAN_POINT ( 'NONE',  ( 9.474510206698971260, -16.51473224551069308, 97.91557627198102409 ) ) ;
#120245=CARTESIAN_POINT ( 'NONE',  ( 21.53943276465977519, 0.05219959533937863772, 36.25109039468567573 ) ) ;
#120247=CARTESIAN_POINT ( 'NONE',  ( -5.049401038298153566, 19.05341960407611168, 90.20724293864766707 ) ) ;
#120248=CARTESIAN_POINT ( 'NONE',  ( 16.20579543436677739, -7.371946100355105003, 111.9347916582813269 ) ) ;
#120249=CARTESIAN_POINT ( 'NONE',  ( 16.46253265017160672, -9.564922557960803928, 83.33224293864768129 ) ) ;
#120250=CARTESIAN_POINT ( 'NONE',  ( -15.72974639402176322, -15.80617190586768395, 29.37609039468568284 ) ) ;
#120251=CARTESIAN_POINT ( 'NONE',  ( 4.483927247898545687, 16.52544592524342804, 84.79057627198102409 ) ) ;
#120252=CARTESIAN_POINT ( 'NONE',  ( -0.05219959533909027116, -19.03943276465977164, 102.4989096053143669 ) ) ;
#120253=CARTESIAN_POINT ( 'NONE',  ( 19.03943276465977164, 0.05219959533936151252, 26.25109039468566507 ) ) ;
#120254=CARTESIAN_POINT ( 'NONE',  ( 16.52544592524335698, 4.483927247898782831, 51.45942372801901854 ) ) ;
#120255=CARTESIAN_POINT ( 'NONE',  ( 5.823673210054444382, -21.52544592524334988, 80.20942372801901854 ) ) ;
#120256=CARTESIAN_POINT ( 'NONE',  ( 12.06949235617739724, 12.14591786802326823, 21.87609039468567573 ) ) ;
#120257=CARTESIAN_POINT ( 'NONE',  ( -9.474510206698964154, 16.51473224551069663, 65.41557627198102409 ) ) ;
#120258=CARTESIAN_POINT ( 'NONE',  ( 5.153800228976615827, -19.02544592524334988, 100.2094237280190043 ) ) ;
#120259=CARTESIAN_POINT ( 'NONE',  ( -8.224510206698735004, -14.34966873604973081, 74.58442372801901854 ) ) ;
#120260=CARTESIAN_POINT ( 'NONE',  ( -21.53943276465977519, -0.05219959533937600094, 113.7510903946856757 ) ) ;
#120261=CARTESIAN_POINT ( 'NONE',  ( -19.05341960407617563, 5.049401038297882671, 83.54275706135233293 ) ) ;
#120262=CARTESIAN_POINT ( 'NONE',  ( 19.05341960407611168, 5.049401038298154454, 63.95724293864769550 ) ) ;
#120263=CARTESIAN_POINT ( 'NONE',  ( -18.67979575497178146, -10.72451020669898902, 81.66557627198103830 ) ) ;
#120264=CARTESIAN_POINT ( 'NONE',  ( 0.05219959533910956823, 16.53943276465976808, 69.99890960531435269 ) ) ;
#120265=CARTESIAN_POINT ( 'NONE',  ( -19.03943276465977164, -0.05219959533935918106, 73.75109039468566152 ) ) ;
#120266=CARTESIAN_POINT ( 'NONE',  ( -19.20446147854526231, -5.500000000000011546, 69.38999695167682091 ) ) ;
#120267=CARTESIAN_POINT ( 'NONE',  ( 19.05341960407617918, -5.049401038297876454, 51.04275706135231871 ) ) ;
#120268=CARTESIAN_POINT ( 'NONE',  ( 14.29746914071049879, -8.314922557960816363, 23.33224293864769194 ) ) ;
#120269=CARTESIAN_POINT ( 'NONE',  ( -4.379528057220328563, 16.55341960407611168, 85.20724293864770971 ) ) ;
#120270=CARTESIAN_POINT ( 'NONE',  ( -21.53943276465977519, -0.05219959533937600094, 103.7510903946857042 ) ) ;
#120272=CARTESIAN_POINT ( 'NONE',  ( 5.719274019375991003, -21.55341960407610458, 102.7072429386476955 ) ) ;
#120273=CARTESIAN_POINT ( 'NONE',  ( 13.97604488694527802, 13.89961937509977652, 99.37390960531436690 ) ) ;
#120274=CARTESIAN_POINT ( 'NONE',  ( 19.05341960407611168, 5.049401038298154454, 63.95724293864769550 ) ) ;
#120275=CARTESIAN_POINT ( 'NONE',  ( -18.62759615963255300, -10.81492255796106328, 79.16775706135234714 ) ) ;
#120276=CARTESIAN_POINT ( 'NONE',  ( 5.049401038298161559, -19.05341960407611168, 67.70724293864769550 ) ) ;
#120278=CARTESIAN_POINT ( 'NONE',  ( 0.05219959533909260263, 19.03943276465977164, 39.99890960531436690 ) ) ;
#120279=CARTESIAN_POINT ( 'NONE',  ( 18.62759615963271287, -10.81492255796078972, 33.33224293864769550 ) ) ;
#120280=CARTESIAN_POINT ( 'NONE',  ( 4.483927247898545687, 16.52544592524342804, 69.79057627198102409 ) ) ;
#120281=CARTESIAN_POINT ( 'NONE',  ( -9.564922557960796823, -16.46253265017161027, 42.08224293864769550 ) ) ;
#120282=CARTESIAN_POINT ( 'NONE',  ( 12.14591786802309770, 12.06949235617756955, 104.3739096053143669 ) ) ;
#120283=CARTESIAN_POINT ( 'NONE',  ( -5.719274019375978568, 21.55341960407610458, 115.2072429386476955 ) ) ;
#120284=CARTESIAN_POINT ( 'NONE',  ( -15.72974639402176322, -15.80617190586768395, 44.37609039468567573 ) ) ;
#120285=CARTESIAN_POINT ( 'NONE',  ( 9.564922557960805705, 16.46253265017160317, 29.58224293864769550 ) ) ;
#120286=CARTESIAN_POINT ( 'NONE',  ( 8.314922557961029526, -14.29746914071037800, 70.41775706135236135 ) ) ;
#120287=CARTESIAN_POINT ( 'NONE',  ( 21.55341960407610458, 5.719274019375980345, 103.9572429386476813 ) ) ;
#120288=CARTESIAN_POINT ( 'NONE',  ( 5.719274019375991003, -21.55341960407610458, 102.7072429386476955 ) ) ;
#120289=CARTESIAN_POINT ( 'NONE',  ( 19.05341960407617918, -5.049401038297876454, 21.04275706135232582 ) ) ;
#120290=CARTESIAN_POINT ( 'NONE',  ( 19.03943276465977164, -0.05219959533909143690, 53.74890960531436690 ) ) ;
#120291=CARTESIAN_POINT ( 'NONE',  ( -17.60728821187774429, 5.500000000000034639, 40.86690927743607205 ) ) ;
#120292=CARTESIAN_POINT ( 'NONE',  ( 15.80617190586769283, -15.72974639402175789, 60.62609039468567573 ) ) ;
#120293=CARTESIAN_POINT ( 'NONE',  ( -21.55341960407610458, -5.719274019375992779, 51.45724293864770260 ) ) ;
#120294=CARTESIAN_POINT ( 'NONE',  ( 4.483927247898545687, 16.52544592524342804, 29.79057627198102409 ) ) ;
#120295=CARTESIAN_POINT ( 'NONE',  ( -21.53943276465977519, -0.05219959533937600094, 78.75109039468568994 ) ) ;
#120296=CARTESIAN_POINT ( 'NONE',  ( -21.53943276465977519, -0.05219959533937600094, 108.7510903946857042 ) ) ;
#120297=CARTESIAN_POINT ( 'NONE',  ( -19.03943276465977164, -0.05219959533935918106, 48.75109039468566863 ) ) ;
#120298=CARTESIAN_POINT ( 'NONE',  ( -16.53943276465976808, -0.05219959533934237506, 98.75109039468568994 ) ) ;
#120299=CARTESIAN_POINT ( 'NONE',  ( 18.62759615963255655, 10.81492255796105972, 51.66775706135234714 ) ) ;
#120300=CARTESIAN_POINT ( 'NONE',  ( -16.51473224551069308, -9.474510206698971260, 61.66557627198103120 ) ) ;
#120301=CARTESIAN_POINT ( 'NONE',  ( 16.46253265017146816, 9.564922557961045513, 36.66775706135233293 ) ) ;
#120302=CARTESIAN_POINT ( 'NONE',  ( 5.823673210054125526, 21.52544592524343514, 44.79057627198103120 ) ) ;
#120303=CARTESIAN_POINT ( 'NONE',  ( -10.81492255796105439, 18.62759615963255655, 27.91775706135234358 ) ) ;
#120304=CARTESIAN_POINT ( 'NONE',  ( -15.80617190586745835, -15.72974639402198527, 86.87390960531438111 ) ) ;
#120305=CARTESIAN_POINT ( 'NONE',  ( 5.153800228976615827, -19.02544592524334988, 90.20942372801900433 ) ) ;
#120306=CARTESIAN_POINT ( 'NONE',  ( -14.34966873604972548, 8.224510206698743886, 48.33442372801902565 ) ) ;
#120308=CARTESIAN_POINT ( 'NONE',  ( 15.80617190586746368, 15.72974639402197994, 94.37390960531436690 ) ) ;
#120309=CARTESIAN_POINT ( 'NONE',  ( -12.06949235617739369, -12.14591786802326823, 84.37609039468570415 ) ) ;
#120310=CARTESIAN_POINT ( 'NONE',  ( -8.314922557960811034, -14.29746914071050412, 77.08224293864769550 ) ) ;
#120312=CARTESIAN_POINT ( 'NONE',  ( -5.049401038297874678, -19.05341960407617918, 104.7927570613523471 ) ) ;
#120313=CARTESIAN_POINT ( 'NONE',  ( -18.62759615963270932, 10.81492255796079327, 40.83224293864769550 ) ) ;
#120315=CARTESIAN_POINT ( 'NONE',  ( -14.29746914071037622, -8.314922557961029526, 49.16775706135234003 ) ) ;
#120316=CARTESIAN_POINT ( 'NONE',  ( -21.55341960407619339, 5.719274019375674811, 23.54275706135235424 ) ) ;
#120317=CARTESIAN_POINT ( 'NONE',  ( -18.62759615963270932, 10.81492255796079327, 30.83224293864770260 ) ) ;
#120318=CARTESIAN_POINT ( 'NONE',  ( -16.52544592524335698, -4.483927247898792601, 73.95942372801901854 ) ) ;
#120319=CARTESIAN_POINT ( 'NONE',  ( 9.474510206698971260, -16.51473224551069308, 82.91557627198103830 ) ) ;
#120320=CARTESIAN_POINT ( 'NONE',  ( 18.67979575497194134, -10.72451020669871369, 50.83442372801901143 ) ) ;
#120321=CARTESIAN_POINT ( 'NONE',  ( 19.03943276465977164, -0.05219959533909143690, 28.74890960531435624 ) ) ;
#120322=CARTESIAN_POINT ( 'NONE',  ( 18.62759615963271287, -10.81492255796078972, 28.33224293864769550 ) ) ;
#120323=CARTESIAN_POINT ( 'NONE',  ( 13.97604488694548053, -13.89961937509957401, 35.62609039468567573 ) ) ;
#120324=CARTESIAN_POINT ( 'NONE',  ( -8.314922557961024197, 14.29746914071037800, 52.91775706135235424 ) ) ;
#120325=CARTESIAN_POINT ( 'NONE',  ( 0.05219959533909260263, 19.03943276465977164, 114.9989096053143669 ) ) ;
#120326=CARTESIAN_POINT ( 'NONE',  ( 9.474510206698971260, -16.51473224551069308, 77.91557627198103830 ) ) ;
#120327=CARTESIAN_POINT ( 'NONE',  ( 14.34966873604972726, -8.224510206698740333, 105.8344237280190328 ) ) ;
#120328=CARTESIAN_POINT ( 'NONE',  ( -9.474510206698964154, 16.51473224551069663, 115.4155762719810241 ) ) ;
#120329=CARTESIAN_POINT ( 'NONE',  ( 14.34966873604960469, 8.224510206698951720, 99.16557627198100988 ) ) ;
#120330=CARTESIAN_POINT ( 'NONE',  ( 5.823673210054125526, 21.52544592524343514, 29.79057627198102409 ) ) ;
#120331=CARTESIAN_POINT ( 'NONE',  ( 19.03943276465977164, -0.05219959533909143690, 28.74890960531435624 ) ) ;
#120332=CARTESIAN_POINT ( 'NONE',  ( -14.29746914071037622, -8.314922557961029526, 64.16775706135234714 ) ) ;
#120333=CARTESIAN_POINT ( 'NONE',  ( -21.52544592524343514, 5.823673210054127303, 111.0405762719810525 ) ) ;
#120334=CARTESIAN_POINT ( 'NONE',  ( 5.049401038297881783, 19.05341960407617563, 82.29275706135229029 ) ) ;
#120335=CARTESIAN_POINT ( 'NONE',  ( 9.564922557960805705, 16.46253265017160317, 39.58224293864768839 ) ) ;
#120336=CARTESIAN_POINT ( 'NONE',  ( 21.52544592524344225, -5.823673210054117533, 68.54057627198103830 ) ) ;
#120337=CARTESIAN_POINT ( 'NONE',  ( -13.97604488694527625, -13.89961937509977652, 111.8739096053143243 ) ) ;
#120338=CARTESIAN_POINT ( 'NONE',  ( -18.67979575497193778, 10.72451020669871902, 88.33442372801901854 ) ) ;
#120339=CARTESIAN_POINT ( 'NONE',  ( -16.46253265017160317, 9.564922557960807481, 70.83224293864770971 ) ) ;
#120341=CARTESIAN_POINT ( 'NONE',  ( -16.55341960407617563, 4.379528057220093196, 48.54275706135234714 ) ) ;
#120342=CARTESIAN_POINT ( 'NONE',  ( -21.53943276465977519, -0.05219959533937600094, 78.75109039468568994 ) ) ;
#120343=CARTESIAN_POINT ( 'NONE',  ( 13.97604488694548053, -13.89961937509957401, 35.62609039468567573 ) ) ;
#120344=CARTESIAN_POINT ( 'NONE',  ( 16.51473224551083163, -9.474510206698727899, 50.83442372801899722 ) ) ;
#120345=ORIENTED_EDGE ( 'NONE', *, *, #166008, .F. ) ;
#120346=CARTESIAN_POINT ( 'NONE',  ( -21.52544592524334988, -5.823673210054445271, 43.95942372801902565 ) ) ;
#120347=CARTESIAN_POINT ( 'NONE',  ( 9.564922557960805705, 16.46253265017160317, 24.58224293864769194 ) ) ;
#120348=CARTESIAN_POINT ( 'NONE',  ( 9.564922557961047289, -16.46253265017146816, 50.41775706135233293 ) ) ;
#120349=CARTESIAN_POINT ( 'NONE',  ( 16.51473224551069308, 9.474510206698969483, 104.1655762719810241 ) ) ;
#120350=CARTESIAN_POINT ( 'NONE',  ( -16.46253265017160317, 9.564922557960807481, 85.83224293864769550 ) ) ;
#120351=CARTESIAN_POINT ( 'NONE',  ( 4.483927247898545687, 16.52544592524342804, 39.79057627198103830 ) ) ;
#120352=CARTESIAN_POINT ( 'NONE',  ( 21.53943276465977519, -0.05219959533907433946, 33.74890960531436690 ) ) ;
#120355=B_SPLINE_CURVE_WITH_KNOTS ( 'NONE', 3,
 ( #173729, #191864, #38191, #51361, #83674, #188900, #53346, #99847, #22022, #69521, #131186, #130167, #161531, #160533, #54354, #114005, #192876, #116026, #177715, #145352, #37179, #39183 ),
 .UNSPECIFIED., .F., .F.,
 ( 4, 2, 2, 2, 2, 2, 2, 2, 2, 2, 4 ),
 ( 2.110382192020081394E-17, 0.001309639967555352707, 0.001964459951333019736, 0.002291869943221851082, 0.002455574939166262852, 0.002619279935110674622, 0.002782984931055086392, 0.002946689926999498162, 0.003274099918888322136, 0.003928919902665964879, 0.005238559870221252100 ),
 .UNSPECIFIED. ) ;
#120356=CARTESIAN_POINT ( 'NONE',  ( 5.823673210054444382, -21.52544592524334988, 100.2094237280190043 ) ) ;
#120359=CARTESIAN_POINT ( 'NONE',  ( 19.02544592524343514, -5.153800228976328945, 38.54057627198103120 ) ) ;
#120360=CARTESIAN_POINT ( 'NONE',  ( -19.03943276465977164, 0.05219959533909376836, 116.2489096053143669 ) ) ;
#120362=CARTESIAN_POINT ( 'NONE',  ( 16.53943276465976808, 0.05219959533934440121, 56.25109039468568284 ) ) ;
#120363=CARTESIAN_POINT ( 'NONE',  ( 21.52544592524344225, -5.823673210054117533, 78.54057627198103830 ) ) ;
#120364=CARTESIAN_POINT ( 'NONE',  ( 0.05219959533910956823, 16.53943276465976808, 34.99890960531435979 ) ) ;
#120365=CARTESIAN_POINT ( 'NONE',  ( -19.03943276465977164, 0.05219959533909376836, 31.24890960531435979 ) ) ;
#120366=CARTESIAN_POINT ( 'NONE',  ( -16.46253265017160317, 9.564922557960807481, 105.8322429386476955 ) ) ;
#120367=CARTESIAN_POINT ( 'NONE',  ( -21.53943276465977519, -0.05219959533937600094, 33.75109039468568284 ) ) ;
#120368=CARTESIAN_POINT ( 'NONE',  ( -0.05219959533936034679, 19.03943276465977164, 37.50109039468567573 ) ) ;
#120369=CARTESIAN_POINT ( 'NONE',  ( -5.049401038298153566, 19.05341960407611168, 25.20724293864768484 ) ) ;
#120370=CARTESIAN_POINT ( 'NONE',  ( -0.05219959533937732626, 21.53943276465977519, 77.50109039468567573 ) ) ;
#120371=LINE ( 'NONE', #183056, #66326 ) ;
#120372=CARTESIAN_POINT ( 'NONE',  ( -16.55341960407611168, -4.379528057220339221, 21.45724293864769550 ) ) ;
#120373=CARTESIAN_POINT ( 'NONE',  ( 17.50000000000000000, 5.499999999999997335, 111.7030961746582847 ) ) ;
#120374=CARTESIAN_POINT ( 'NONE',  ( -5.823673210054116645, -21.52544592524344225, 22.29057627198102765 ) ) ;
#120375=CARTESIAN_POINT ( 'NONE',  ( -16.55341960407611168, -4.379528057220339221, 91.45724293864769550 ) ) ;
#120377=CARTESIAN_POINT ( 'NONE',  ( 19.05341960407611168, 5.049401038298154454, 73.95724293864768129 ) ) ;
#120378=CARTESIAN_POINT ( 'NONE',  ( 8.314922557960818139, 14.29746914071049879, 74.58224293864768129 ) ) ;
#120379=CARTESIAN_POINT ( 'NONE',  ( 19.02544592524334988, 5.153800228976608722, 111.4594237280190043 ) ) ;
#120380=CARTESIAN_POINT ( 'NONE',  ( -21.52544592524343514, 5.823673210054127303, 66.04057627198103830 ) ) ;
#120382=CARTESIAN_POINT ( 'NONE',  ( -9.564922557960796823, -16.46253265017161027, 37.08224293864768839 ) ) ;
#120383=CARTESIAN_POINT ( 'NONE',  ( 16.51473224551069308, 9.474510206698969483, 89.16557627198103830 ) ) ;
#120384=CARTESIAN_POINT ( 'NONE',  ( -15.72974639402197994, 15.80617190586746368, 75.62390960531439532 ) ) ;
#120385=CARTESIAN_POINT ( 'NONE',  ( 8.314922557961029526, -14.29746914071037800, 110.4177570613523756 ) ) ;
#120386=CARTESIAN_POINT ( 'NONE',  ( 16.46253265017160672, -9.564922557960803928, 83.33224293864768129 ) ) ;
#120387=CARTESIAN_POINT ( 'NONE',  ( 13.89961937509957401, 13.97604488694547697, 61.87609039468566863 ) ) ;
#120388=CARTESIAN_POINT ( 'NONE',  ( -15.80617190586768217, 15.72974639402176855, 98.12609039468570415 ) ) ;
#120389=CARTESIAN_POINT ( 'NONE',  ( 21.52544592524344225, -5.823673210054117533, 73.54057627198102409 ) ) ;
#120390=CARTESIAN_POINT ( 'NONE',  ( -15.72974639402197994, 15.80617190586746368, 25.62390960531435624 ) ) ;
#120391=CARTESIAN_POINT ( 'NONE',  ( -5.049401038298153566, 19.05341960407611168, 50.20724293864770260 ) ) ;
#120392=CARTESIAN_POINT ( 'NONE',  ( 8.224510206698953496, -14.34966873604960469, 22.91557627198102765 ) ) ;
#120393=CARTESIAN_POINT ( 'NONE',  ( 0.05219959533909260263, 19.03943276465977164, 64.99890960531436690 ) ) ;
#120394=CARTESIAN_POINT ( 'NONE',  ( 17.48847506799968343, 5.747544572773805704, 51.67302562156721280 ) ) ;
#120395=CARTESIAN_POINT ( 'NONE',  ( -19.02544592524334988, -5.153800228976617603, 18.95942372801899722 ) ) ;
#120396=CARTESIAN_POINT ( 'NONE',  ( -16.53943276465976808, 0.05219959533911058130, 71.24890960531435269 ) ) ;
#120398=CARTESIAN_POINT ( 'NONE',  ( -10.72451020669898014, 18.67979575497178502, 105.4155762719810383 ) ) ;
#120399=CARTESIAN_POINT ( 'NONE',  ( -10.81492255796078084, -18.62759615963271287, 102.0822429386476955 ) ) ;
#120401=CARTESIAN_POINT ( 'NONE',  ( 0.05219959533907565091, 21.53943276465977519, 59.99890960531436690 ) ) ;
#120402=CARTESIAN_POINT ( 'NONE',  ( -12.14591786802326823, 12.06949235617739902, 83.12609039468568994 ) ) ;
#120403=CARTESIAN_POINT ( 'NONE',  ( 12.06949235617757843, -12.14591786802309237, 98.12390960531436690 ) ) ;
#120404=CARTESIAN_POINT ( 'NONE',  ( -5.049401038298153566, 19.05341960407611168, 65.20724293864765286 ) ) ;
#120405=CARTESIAN_POINT ( 'NONE',  ( -16.53943276465976808, -0.05219959533934237506, 108.7510903946857042 ) ) ;
#120406=CARTESIAN_POINT ( 'NONE',  ( 5.823673210054444382, -21.52544592524334988, 40.20942372801901854 ) ) ;
#120407=CARTESIAN_POINT ( 'NONE',  ( -5.153800228976328057, -19.02544592524343514, 112.2905762719810099 ) ) ;
#120408=CARTESIAN_POINT ( 'NONE',  ( 15.72974639402176855, 15.80617190586768217, 81.87609039468568994 ) ) ;
#120409=CARTESIAN_POINT ( 'NONE',  ( 19.05341960407611168, 5.049401038298154454, 28.95724293864769550 ) ) ;
#120410=CARTESIAN_POINT ( 'NONE',  ( 13.89961937509977652, -13.97604488694527269, 38.12390960531436690 ) ) ;
#120412=CARTESIAN_POINT ( 'NONE',  ( -18.62759615963255300, -10.81492255796106328, 79.16775706135234714 ) ) ;
#120413=CARTESIAN_POINT ( 'NONE',  ( 0.05219959533937995610, -21.53943276465977519, 75.00109039468568994 ) ) ;
#120414=CARTESIAN_POINT ( 'NONE',  ( 19.02544592524343514, -5.153800228976328945, 98.54057627198100988 ) ) ;
#120415=CARTESIAN_POINT ( 'NONE',  ( -5.153800228976607833, 19.02544592524334988, 82.70942372801897591 ) ) ;
#120416=CARTESIAN_POINT ( 'NONE',  ( 18.62759615963255655, 10.81492255796105972, 61.66775706135235424 ) ) ;
#120417=CARTESIAN_POINT ( 'NONE',  ( -14.29746914071037622, -8.314922557961029526, 24.16775706135235424 ) ) ;
#120418=CARTESIAN_POINT ( 'NONE',  ( 9.474510206698729675, 16.51473224551082808, 77.08442372801900433 ) ) ;
#120419=CARTESIAN_POINT ( 'NONE',  ( -9.474510206698964154, 16.51473224551069663, 50.41557627198102409 ) ) ;
#120420=CARTESIAN_POINT ( 'NONE',  ( 13.89961937509957401, 13.97604488694547697, 76.87609039468566152 ) ) ;
#120421=CARTESIAN_POINT ( 'NONE',  ( -4.483927247898539470, -16.52544592524342804, 22.29057627198102765 ) ) ;
#120422=CARTESIAN_POINT ( 'NONE',  ( -19.05341960407617563, 5.049401038297882671, 88.54275706135230450 ) ) ;
#120423=CARTESIAN_POINT ( 'NONE',  ( -16.55341960407611168, -4.379528057220339221, 36.45724293864768839 ) ) ;
#120424=CARTESIAN_POINT ( 'NONE',  ( -16.51473224551082808, 9.474510206698731452, 58.33442372801900433 ) ) ;
#120425=CARTESIAN_POINT ( 'NONE',  ( -8.314922557961024197, 14.29746914071037800, 47.91775706135234714 ) ) ;
#120426=CARTESIAN_POINT ( 'NONE',  ( 16.51473224551083163, -9.474510206698727899, 20.83442372801899722 ) ) ;
#120427=CARTESIAN_POINT ( 'NONE',  ( 13.97604488694527802, 13.89961937509977652, 44.37390960531435269 ) ) ;
#120428=CARTESIAN_POINT ( 'NONE',  ( -17.49999999999998934, -5.622605283950889543, 66.31207310596113302 ) ) ;
#120429=CARTESIAN_POINT ( 'NONE',  ( -4.379528057220086978, -16.55341960407618274, 49.79275706135234714 ) ) ;
#120433=CARTESIAN_POINT ( 'NONE',  ( -13.89961937509977652, 13.97604488694528158, 95.62390960531436690 ) ) ;
#120435=CARTESIAN_POINT ( 'NONE',  ( -16.46253265017146816, -9.564922557961047289, 99.16775706135233293 ) ) ;
#120436=CARTESIAN_POINT ( 'NONE',  ( -9.474510206698964154, 16.51473224551069663, 115.4155762719810241 ) ) ;
#120437=CARTESIAN_POINT ( 'NONE',  ( -10.81492255796105439, 18.62759615963255655, 107.9177570613523471 ) ) ;
#120438=CARTESIAN_POINT ( 'NONE',  ( 9.564922557961047289, -16.46253265017146816, 100.4177570613523329 ) ) ;
#120439=CARTESIAN_POINT ( 'NONE',  ( 12.14591786802309770, 12.06949235617756955, 114.3739096053143527 ) ) ;
#120440=CARTESIAN_POINT ( 'NONE',  ( -19.03943276465977164, 0.05219959533909376836, 41.24890960531435269 ) ) ;
#120441=CARTESIAN_POINT ( 'NONE',  ( -10.72451020669898014, 18.67979575497178502, 65.41557627198102409 ) ) ;
#120442=CARTESIAN_POINT ( 'NONE',  ( -13.97604488694527625, -13.89961937509977652, 26.87390960531434558 ) ) ;
#120443=CARTESIAN_POINT ( 'NONE',  ( 16.46253265017146816, 9.564922557961045513, 46.66775706135233293 ) ) ;
#120444=CARTESIAN_POINT ( 'NONE',  ( 5.153800228976615827, -19.02544592524334988, 75.20942372801896170 ) ) ;
#120445=CARTESIAN_POINT ( 'NONE',  ( -4.483927247898539470, -16.52544592524342804, 57.29057627198103120 ) ) ;
#120446=CARTESIAN_POINT ( 'NONE',  ( 21.53943276465977519, -0.05219959533907433946, 33.74890960531436690 ) ) ;
#120447=CARTESIAN_POINT ( 'NONE',  ( 5.719274019375673035, 21.55341960407619339, 92.29275706135236135 ) ) ;
#120448=EDGE_CURVE ( 'NONE', #119129, #175270, #45993, .T. ) ;
#120449=CARTESIAN_POINT ( 'NONE',  ( -15.80617190586745835, -15.72974639402198527, 81.87390960531435269 ) ) ;
#120450=CARTESIAN_POINT ( 'NONE',  ( 0.05219959533937995610, -21.53943276465977519, 55.00109039468568284 ) ) ;
#120451=CARTESIAN_POINT ( 'NONE',  ( -18.62759615963255300, -10.81492255796106328, 69.16775706135234714 ) ) ;
#120452=CARTESIAN_POINT ( 'NONE',  ( 0.05219959533909260263, 19.03943276465977164, 89.99890960531436690 ) ) ;
#120453=CARTESIAN_POINT ( 'NONE',  ( 16.52544592524335698, 4.483927247898782831, 86.45942372801901854 ) ) ;
#120454=CARTESIAN_POINT ( 'NONE',  ( 18.62759615963255655, 10.81492255796105972, 61.66775706135235424 ) ) ;
#120455=CARTESIAN_POINT ( 'NONE',  ( 9.564922557960805705, 16.46253265017160317, 59.58224293864769550 ) ) ;
#120456=CARTESIAN_POINT ( 'NONE',  ( 19.02544592524343514, -5.153800228976328945, 28.54057627198102409 ) ) ;
#120457=CARTESIAN_POINT ( 'NONE',  ( -16.46253265017160317, 9.564922557960807481, 50.83224293864770260 ) ) ;
#120458=CARTESIAN_POINT ( 'NONE',  ( 12.06949235617757843, -12.14591786802309237, 63.12390960531435979 ) ) ;
#120459=CARTESIAN_POINT ( 'NONE',  ( 0.05219959533910956823, 16.53943276465976808, 34.99890960531435979 ) ) ;
#120460=CARTESIAN_POINT ( 'NONE',  ( -5.823673210054116645, -21.52544592524344225, 47.29057627198103120 ) ) ;
#120461=CARTESIAN_POINT ( 'NONE',  ( -9.474510206698964154, 16.51473224551069663, 45.41557627198103120 ) ) ;
#120462=CARTESIAN_POINT ( 'NONE',  ( -10.81492255796078084, -18.62759615963271287, 52.08224293864768839 ) ) ;
#120463=CARTESIAN_POINT ( 'NONE',  ( 13.89961937509957401, 13.97604488694547697, 56.87609039468564731 ) ) ;
#120464=CARTESIAN_POINT ( 'NONE',  ( -16.81555441253550498, -7.025013491695498047, 39.36314554665744936 ) ) ;
#120465=CARTESIAN_POINT ( 'NONE',  ( 4.483927247898545687, 16.52544592524342804, 44.79057627198103120 ) ) ;
#120466=CARTESIAN_POINT ( 'NONE',  ( 10.72451020669898902, -18.67979575497178502, 22.91557627198102765 ) ) ;
#120470=CARTESIAN_POINT ( 'NONE',  ( -16.53943276465976808, -0.05219959533934237506, 78.75109039468568994 ) ) ;
#120471=CARTESIAN_POINT ( 'NONE',  ( 16.46253265017146816, 9.564922557961045513, 76.66775706135234714 ) ) ;
#120472=CARTESIAN_POINT ( 'NONE',  ( 16.55341960407611168, 4.379528057220329451, 58.95724293864770971 ) ) ;
#120474=CARTESIAN_POINT ( 'NONE',  ( 4.379528057220339221, -16.55341960407611168, 22.70724293864769194 ) ) ;
#120475=CARTESIAN_POINT ( 'NONE',  ( -19.02544592524342804, 5.153800228976336051, 56.04057627198100988 ) ) ;
#120477=CARTESIAN_POINT ( 'NONE',  ( 0.05219959533909260263, 19.03943276465977164, 74.99890960531435269 ) ) ;
#120478=CARTESIAN_POINT ( 'NONE',  ( 19.05341960407611168, 5.049401038298154454, 33.95724293864769550 ) ) ;
#120479=CARTESIAN_POINT ( 'NONE',  ( -10.72451020669870658, -18.67979575497194134, 39.58442372801901143 ) ) ;
#120480=CARTESIAN_POINT ( 'NONE',  ( -13.97604488694527625, -13.89961937509977652, 66.87390960531436690 ) ) ;
#120482=CARTESIAN_POINT ( 'NONE',  ( 16.46253265017160672, -9.564922557960803928, 53.33224293864768839 ) ) ;
#120483=CARTESIAN_POINT ( 'NONE',  ( -21.53943276465977519, 0.05219959533907696930, 36.24890960531435979 ) ) ;
#120484=CARTESIAN_POINT ( 'NONE',  ( 5.049401038298161559, -19.05341960407611168, 32.70724293864768129 ) ) ;
#120485=CARTESIAN_POINT ( 'NONE',  ( 15.80617190586746368, 15.72974639402197994, 39.37390960531436690 ) ) ;
#120486=CARTESIAN_POINT ( 'NONE',  ( -16.53943276465976808, -0.05219959533934237506, 93.75109039468567573 ) ) ;
#120487=CARTESIAN_POINT ( 'NONE',  ( -5.049401038297874678, -19.05341960407617918, 24.79275706135233648 ) ) ;
#120488=CARTESIAN_POINT ( 'NONE',  ( -12.06949235617739369, -12.14591786802326823, 44.37609039468567573 ) ) ;
#120489=CARTESIAN_POINT ( 'NONE',  ( -12.06949235617739369, -12.14591786802326823, 84.37609039468570415 ) ) ;
#120490=CARTESIAN_POINT ( 'NONE',  ( 13.89961937509977652, -13.97604488694527269, 103.1239096053143527 ) ) ;
#120491=CARTESIAN_POINT ( 'NONE',  ( 16.55341960407618274, -4.379528057220086978, 66.04275706135236135 ) ) ;
#120492=CARTESIAN_POINT ( 'NONE',  ( 12.14591786802327356, -12.06949235617739191, 35.62609039468568994 ) ) ;
#120493=CARTESIAN_POINT ( 'NONE',  ( -16.46253265017160317, 9.564922557960807481, 105.8322429386476955 ) ) ;
#120494=CARTESIAN_POINT ( 'NONE',  ( -8.224510206698735004, -14.34966873604973081, 29.58442372801901854 ) ) ;
#120495=CARTESIAN_POINT ( 'NONE',  ( -19.03943276465977164, 0.05219959533909376836, 36.24890960531436690 ) ) ;
#120496=CARTESIAN_POINT ( 'NONE',  ( -15.72974639402176322, -15.80617190586768395, 29.37609039468568284 ) ) ;
#120497=CARTESIAN_POINT ( 'NONE',  ( -0.05219959533936034679, 19.03943276465977164, 112.5010903946856757 ) ) ;
#120498=CARTESIAN_POINT ( 'NONE',  ( 16.53943276465976808, 0.05219959533934440121, 96.25109039468568994 ) ) ;
#120500=CARTESIAN_POINT ( 'NONE',  ( 10.72451020669871369, 18.67979575497193778, 97.08442372801904696 ) ) ;
#120501=CARTESIAN_POINT ( 'NONE',  ( 13.89961937509957401, 13.97604488694547697, 91.87609039468567573 ) ) ;
#120502=CARTESIAN_POINT ( 'NONE',  ( -16.53943276465976808, 0.05219959533911058130, 61.24890960531435979 ) ) ;
#120503=CARTESIAN_POINT ( 'NONE',  ( -19.02544592524342804, 5.153800228976336051, 26.04057627198103120 ) ) ;
#120504=CARTESIAN_POINT ( 'NONE',  ( 16.46253265017146816, 9.564922557961045513, 66.66775706135233293 ) ) ;
#120506=CARTESIAN_POINT ( 'NONE',  ( -18.62759615963255300, -10.81492255796106328, 54.16775706135235424 ) ) ;
#120507=CARTESIAN_POINT ( 'NONE',  ( -16.55341960407617563, 4.379528057220093196, 28.54275706135234358 ) ) ;
#120509=CARTESIAN_POINT ( 'NONE',  ( -0.05219959533909027116, -19.03943276465977164, 112.4989096053143669 ) ) ;
#120510=CARTESIAN_POINT ( 'NONE',  ( 5.823673210054125526, 21.52544592524343514, 74.79057627198105251 ) ) ;
#120511=CARTESIAN_POINT ( 'NONE',  ( 16.51473224551083163, -9.474510206698727899, 105.8344237280190043 ) ) ;
#120512=CARTESIAN_POINT ( 'NONE',  ( -9.564922557960796823, -16.46253265017161027, 97.08224293864769550 ) ) ;
#120514=CARTESIAN_POINT ( 'NONE',  ( 19.05341960407611168, 5.049401038298154454, 28.95724293864769550 ) ) ;
#120515=CARTESIAN_POINT ( 'NONE',  ( 0.05219959533937995610, -21.53943276465977519, 90.00109039468567573 ) ) ;
#120516=CARTESIAN_POINT ( 'NONE',  ( 19.05341960407611168, 5.049401038298154454, 48.95724293864768129 ) ) ;
#120517=CARTESIAN_POINT ( 'NONE',  ( 5.823673210054444382, -21.52544592524334988, 55.20942372801902565 ) ) ;
#120518=CARTESIAN_POINT ( 'NONE',  ( -21.55341960407619339, 5.719274019375674811, 83.54275706135234714 ) ) ;
#120519=CARTESIAN_POINT ( 'NONE',  ( -4.379528057220086978, -16.55341960407618274, 99.79275706135234714 ) ) ;
#120520=CARTESIAN_POINT ( 'NONE',  ( 13.89961937509977652, -13.97604488694527269, 83.12390960531436690 ) ) ;
#120521=CARTESIAN_POINT ( 'NONE',  ( 15.80617190586769283, -15.72974639402175789, 45.62609039468567573 ) ) ;
#120522=CARTESIAN_POINT ( 'NONE',  ( 10.81492255796106328, -18.62759615963255655, 35.41775706135234003 ) ) ;
#120523=CARTESIAN_POINT ( 'NONE',  ( 13.89961937509957401, 13.97604488694547697, 81.87609039468564731 ) ) ;
#120524=CARTESIAN_POINT ( 'NONE',  ( -19.03943276465977164, 0.05219959533909376836, 91.24890960531436690 ) ) ;
#120525=CARTESIAN_POINT ( 'NONE',  ( -16.52544592524342804, 4.483927247898546575, 101.0405762719810383 ) ) ;
#120526=CARTESIAN_POINT ( 'NONE',  ( 5.719274019375991003, -21.55341960407610458, 102.7072429386476955 ) ) ;
#120527=CARTESIAN_POINT ( 'NONE',  ( -14.34966873604960291, -8.224510206698953496, 81.66557627198103830 ) ) ;
#120528=CARTESIAN_POINT ( 'NONE',  ( 0.05219959533936267826, -19.03943276465977164, 20.00109039468567218 ) ) ;
#120529=CARTESIAN_POINT ( 'NONE',  ( 14.29746914071049879, -8.314922557960816363, 93.33224293864769550 ) ) ;
#120530=CARTESIAN_POINT ( 'NONE',  ( -9.564922557960796823, -16.46253265017161027, 37.08224293864768839 ) ) ;
#120531=CARTESIAN_POINT ( 'NONE',  ( 5.153800228976615827, -19.02544592524334988, 85.20942372801900433 ) ) ;
#120532=CARTESIAN_POINT ( 'NONE',  ( 12.06949235617757843, -12.14591786802309237, 43.12390960531435269 ) ) ;
#120533=CARTESIAN_POINT ( 'NONE',  ( 0.05219959533937995610, -21.53943276465977519, 95.00109039468568994 ) ) ;
#120534=CARTESIAN_POINT ( 'NONE',  ( -13.97604488694527625, -13.89961937509977652, 101.8739096053143811 ) ) ;
#120535=CARTESIAN_POINT ( 'NONE',  ( 19.02544592524334988, 5.153800228976608722, 71.45942372801900433 ) ) ;
#120536=CARTESIAN_POINT ( 'NONE',  ( 15.80617190586746368, 15.72974639402197994, 84.37390960531438111 ) ) ;
#120537=CARTESIAN_POINT ( 'NONE',  ( 15.72974639402176855, 15.80617190586768217, 26.87609039468567218 ) ) ;
#120538=CARTESIAN_POINT ( 'NONE',  ( 8.224510206698742110, 14.34966873604972548, 32.08442372801901854 ) ) ;
#120539=CARTESIAN_POINT ( 'NONE',  ( -4.379528057220086978, -16.55341960407618274, 89.79275706135236135 ) ) ;
#120540=CARTESIAN_POINT ( 'NONE',  ( 19.02544592524343514, -5.153800228976328945, 23.54057627198102054 ) ) ;
#120541=CARTESIAN_POINT ( 'NONE',  ( 0.05219959533937995610, -21.53943276465977519, 30.00109039468568284 ) ) ;
#120542=CARTESIAN_POINT ( 'NONE',  ( -9.564922557960796823, -16.46253265017161027, 27.08224293864769550 ) ) ;
#120544=CARTESIAN_POINT ( 'NONE',  ( -12.14591786802326823, 12.06949235617739902, 48.12609039468568284 ) ) ;
#120545=CARTESIAN_POINT ( 'NONE',  ( -8.314922557960811034, -14.29746914071050412, 82.08224293864768129 ) ) ;
#120546=CARTESIAN_POINT ( 'NONE',  ( -18.67979575497178146, -10.72451020669898902, 71.66557627198100988 ) ) ;
#120547=CARTESIAN_POINT ( 'NONE',  ( -16.53943276465976808, -0.05219959533934237506, 113.7510903946856757 ) ) ;
#120548=CARTESIAN_POINT ( 'NONE',  ( 0.05219959533934541429, -16.53943276465976808, 50.00109039468568994 ) ) ;
#120549=CARTESIAN_POINT ( 'NONE',  ( -5.153800228976328057, -19.02544592524343514, 47.29057627198102409 ) ) ;
#120550=CARTESIAN_POINT ( 'NONE',  ( 8.224510206698742110, 14.34966873604972548, 92.08442372801901854 ) ) ;
#120551=CARTESIAN_POINT ( 'NONE',  ( -9.474510206698720793, -16.51473224551083518, 84.58442372801900433 ) ) ;
#120552=CARTESIAN_POINT ( 'NONE',  ( -5.719274019375978568, 21.55341960407610458, 90.20724293864770971 ) ) ;
#120553=CARTESIAN_POINT ( 'NONE',  ( 12.06949235617739724, 12.14591786802326823, 111.8760903946856615 ) ) ;
#120556=CARTESIAN_POINT ( 'NONE',  ( 15.72974639402199770, -15.80617190586745480, 58.12390960531435979 ) ) ;
#120558=CARTESIAN_POINT ( 'NONE',  ( 14.34966873604972726, -8.224510206698740333, 90.83442372801901854 ) ) ;
#120560=CARTESIAN_POINT ( 'NONE',  ( -15.80617190586745835, -15.72974639402198527, 31.87390960531435979 ) ) ;
#120561=CARTESIAN_POINT ( 'NONE',  ( 17.50000000000002842, 4.658240926743181909, 108.5552958218320043 ) ) ;
#120562=CARTESIAN_POINT ( 'NONE',  ( -21.55341960407610458, -5.719274019375992779, 76.45724293864769550 ) ) ;
#120563=CARTESIAN_POINT ( 'NONE',  ( -16.55341960407617563, 4.379528057220093196, 113.5427570613523756 ) ) ;
#120564=CARTESIAN_POINT ( 'NONE',  ( 4.379528057220092307, 16.55341960407617563, 27.29275706135234358 ) ) ;
#120565=CARTESIAN_POINT ( 'NONE',  ( 16.53943276465976808, -0.05219959533910856209, 113.7489096053143527 ) ) ;
#120566=CARTESIAN_POINT ( 'NONE',  ( 12.14591786802327356, -12.06949235617739191, 30.62609039468567929 ) ) ;
#120567=CARTESIAN_POINT ( 'NONE',  ( 0.05219959533909260263, 19.03943276465977164, 59.99890960531436690 ) ) ;
#120569=CARTESIAN_POINT ( 'NONE',  ( -16.46253265017160317, 9.564922557960807481, 105.8322429386476955 ) ) ;
#120570=CARTESIAN_POINT ( 'NONE',  ( -16.46253265017160317, 9.564922557960807481, 100.8322429386477097 ) ) ;
#120571=EDGE_CURVE ( 'NONE', #138821, #3778, #138002, .T. ) ;
#120572=CARTESIAN_POINT ( 'NONE',  ( -8.224510206698735004, -14.34966873604973081, 84.58442372801903275 ) ) ;
#120573=CARTESIAN_POINT ( 'NONE',  ( 9.564922557961047289, -16.46253265017146816, 95.41775706135233293 ) ) ;
#120574=CARTESIAN_POINT ( 'NONE',  ( -0.05219959533936034679, 19.03943276465977164, 37.50109039468567573 ) ) ;
#120575=CARTESIAN_POINT ( 'NONE',  ( 21.53943276465977519, -0.05219959533907433946, 78.74890960531436690 ) ) ;
#120576=CARTESIAN_POINT ( 'NONE',  ( -12.14591786802326823, 12.06949235617739902, 98.12609039468570415 ) ) ;
#120578=CARTESIAN_POINT ( 'NONE',  ( -18.62759615963270932, 10.81492255796079327, 35.83224293864768839 ) ) ;
#120579=CARTESIAN_POINT ( 'NONE',  ( -19.05341960407617563, 5.049401038297882671, 93.54275706135234714 ) ) ;
#120580=CARTESIAN_POINT ( 'NONE',  ( 9.564922557960805705, 16.46253265017160317, 44.58224293864769550 ) ) ;
#120581=CARTESIAN_POINT ( 'NONE',  ( -19.05341960407611168, -5.049401038298163336, 96.45724293864769550 ) ) ;
#120582=CARTESIAN_POINT ( 'NONE',  ( -21.53943276465977519, -0.05219959533937600094, 58.75109039468568994 ) ) ;
#120583=CARTESIAN_POINT ( 'NONE',  ( 5.153800228976335163, 19.02544592524342804, 54.79057627198103120 ) ) ;
#120584=CARTESIAN_POINT ( 'NONE',  ( -16.52544592524342804, 4.483927247898546575, 81.04057627198102409 ) ) ;
#120585=CARTESIAN_POINT ( 'NONE',  ( -17.12812012977030918, -6.668231424565924215, 86.35948759323143520 ) ) ;
#120586=CARTESIAN_POINT ( 'NONE',  ( 16.52544592524342804, -4.483927247898539470, 83.54057627198102409 ) ) ;
#120587=CARTESIAN_POINT ( 'NONE',  ( -21.55341960407610458, -5.719274019375992779, 71.45724293864769550 ) ) ;
#120588=CARTESIAN_POINT ( 'NONE',  ( -9.564922557961040184, 16.46253265017147172, 97.91775706135233293 ) ) ;
#120590=CARTESIAN_POINT ( 'NONE',  ( -19.02544592524334988, -5.153800228976617603, 48.95942372801900433 ) ) ;
#120591=CARTESIAN_POINT ( 'NONE',  ( 16.20579543436695502, -7.371946100355081022, 71.93479165828050270 ) ) ;
#120592=CARTESIAN_POINT ( 'NONE',  ( 9.564922557960805705, 16.46253265017160317, 74.58224293864769550 ) ) ;
#120593=CARTESIAN_POINT ( 'NONE',  ( 5.049401038298161559, -19.05341960407611168, 87.70724293864769550 ) ) ;
#120594=CARTESIAN_POINT ( 'NONE',  ( -4.483927247898782831, 16.52544592524335698, 67.70942372801901854 ) ) ;
#120595=CARTESIAN_POINT ( 'NONE',  ( -17.12812012977023457, -6.668231424566066323, 51.35948759323144230 ) ) ;
#120596=CARTESIAN_POINT ( 'NONE',  ( 13.89961937509957401, 13.97604488694547697, 41.87609039468566152 ) ) ;
#120598=CARTESIAN_POINT ( 'NONE',  ( 13.97604488694527802, 13.89961937509977652, 114.3739096053143669 ) ) ;
#120599=CARTESIAN_POINT ( 'NONE',  ( 14.29746914071037800, 8.314922557961029526, 106.6677570613523756 ) ) ;
#120600=EDGE_CURVE ( 'NONE', #188457, #184582, #119083, .T. ) ;
#120602=CARTESIAN_POINT ( 'NONE',  ( 8.314922557961029526, -14.29746914071037800, 75.41775706135233293 ) ) ;
#120603=CARTESIAN_POINT ( 'NONE',  ( -17.49999999999999645, 5.499999999999997335, 30.79690382534172599 ) ) ;
#120604=CARTESIAN_POINT ( 'NONE',  ( -14.29746914071037622, -8.314922557961029526, 49.16775706135234003 ) ) ;
#120606=CARTESIAN_POINT ( 'NONE',  ( -15.80617190586768217, 15.72974639402176855, 73.12609039468567573 ) ) ;
#120607=CARTESIAN_POINT ( 'NONE',  ( -16.51473224551082808, 9.474510206698731452, 78.33442372801900433 ) ) ;
#120608=CARTESIAN_POINT ( 'NONE',  ( -0.05219959533936034679, 19.03943276465977164, 22.50109039468566152 ) ) ;
#120609=CARTESIAN_POINT ( 'NONE',  ( 19.02544592524343514, -5.153800228976328945, 58.54057627198102409 ) ) ;
#120610=CARTESIAN_POINT ( 'NONE',  ( -5.153800228976328057, -19.02544592524343514, 47.29057627198102409 ) ) ;
#120612=CARTESIAN_POINT ( 'NONE',  ( -0.05219959533907301413, -21.53943276465977519, 67.49890960531436690 ) ) ;
#120613=CARTESIAN_POINT ( 'NONE',  ( 10.81492255796078972, 18.62759615963270932, 29.58224293864769905 ) ) ;
#120614=CARTESIAN_POINT ( 'NONE',  ( -14.34966873604960291, -8.224510206698953496, 111.6655762719810525 ) ) ;
#120615=CARTESIAN_POINT ( 'NONE',  ( 16.53943276465976808, 0.05219959533934440121, 51.25109039468568994 ) ) ;
#120617=CARTESIAN_POINT ( 'NONE',  ( -18.67979575497193778, 10.72451020669871902, 28.33442372801902209 ) ) ;
#120618=CARTESIAN_POINT ( 'NONE',  ( -8.314922557960811034, -14.29746914071050412, 47.08224293864770260 ) ) ;
#120620=CARTESIAN_POINT ( 'NONE',  ( 4.379528057220092307, 16.55341960407617563, 27.29275706135234358 ) ) ;
#120621=CARTESIAN_POINT ( 'NONE',  ( -9.564922557961040184, 16.46253265017147172, 37.91775706135233293 ) ) ;
#120622=CARTESIAN_POINT ( 'NONE',  ( 12.06949235617757843, -12.14591786802309237, 43.12390960531435269 ) ) ;
#120623=CARTESIAN_POINT ( 'NONE',  ( -15.72974639402176322, -15.80617190586768395, 19.37609039468568639 ) ) ;
#120624=CARTESIAN_POINT ( 'NONE',  ( 17.44279575226822843, 5.990770900252485376, 31.66442432485683867 ) ) ;
#120625=CARTESIAN_POINT ( 'NONE',  ( 5.719274019375991003, -21.55341960407610458, 72.70724293864769550 ) ) ;
#120626=CARTESIAN_POINT ( 'NONE',  ( -19.03943276465977164, 0.05219959533909376836, 96.24890960531436690 ) ) ;
#120627=CARTESIAN_POINT ( 'NONE',  ( 16.53943276465976808, -0.05219959533910856209, 63.74890960531435979 ) ) ;
#120628=CARTESIAN_POINT ( 'NONE',  ( 9.564922557960805705, 16.46253265017160317, 109.5822429386476955 ) ) ;
#120630=CARTESIAN_POINT ( 'NONE',  ( 13.97604488694548053, -13.89961937509957401, 50.62609039468566152 ) ) ;
#120631=CARTESIAN_POINT ( 'NONE',  ( 18.67979575497178502, 10.72451020669898547, 104.1655762719810241 ) ) ;
#120632=CARTESIAN_POINT ( 'NONE',  ( 19.05341960407611168, 5.049401038298154454, 48.95724293864768129 ) ) ;
#120633=CARTESIAN_POINT ( 'NONE',  ( 12.14591786802309770, 12.06949235617756955, 109.3739096053143811 ) ) ;
#120635=CARTESIAN_POINT ( 'NONE',  ( -10.72451020669870658, -18.67979575497194134, 54.58442372801901143 ) ) ;
#120636=CARTESIAN_POINT ( 'NONE',  ( 8.314922557960818139, 14.29746914071049879, 34.58224293864770260 ) ) ;
#120637=CARTESIAN_POINT ( 'NONE',  ( 9.474510206698971260, -16.51473224551069308, 42.91557627198103120 ) ) ;
#120638=CARTESIAN_POINT ( 'NONE',  ( 19.03943276465977164, -0.05219959533909143690, 103.7489096053143669 ) ) ;
#120639=CARTESIAN_POINT ( 'NONE',  ( 21.52544592524344225, -5.823673210054117533, 73.54057627198102409 ) ) ;
#120641=CARTESIAN_POINT ( 'NONE',  ( -13.89961937509977652, 13.97604488694528158, 45.62390960531433848 ) ) ;
#120642=CARTESIAN_POINT ( 'NONE',  ( -5.823673210054116645, -21.52544592524344225, 57.29057627198103120 ) ) ;
#120643=CARTESIAN_POINT ( 'NONE',  ( 5.719274019375673035, 21.55341960407619339, 87.29275706135236135 ) ) ;
#120645=CARTESIAN_POINT ( 'NONE',  ( -16.55341960407617563, 4.379528057220093196, 78.54275706135236135 ) ) ;
#120646=CARTESIAN_POINT ( 'NONE',  ( -4.379528057220328563, 16.55341960407611168, 65.20724293864768129 ) ) ;
#120647=CARTESIAN_POINT ( 'NONE',  ( 13.97604488694527802, 13.89961937509977652, 64.37390960531436690 ) ) ;
#120648=VERTEX_POINT ( 'NONE', #154169 ) ;
#120649=CARTESIAN_POINT ( 'NONE',  ( -16.51473224551082808, 9.474510206698731452, 28.33442372801900433 ) ) ;
#120650=CARTESIAN_POINT ( 'NONE',  ( 16.55341960407618274, -4.379528057220086978, 86.04275706135236135 ) ) ;
#120651=CARTESIAN_POINT ( 'NONE',  ( 18.67979575497194134, -10.72451020669871369, 105.8344237280190328 ) ) ;
#120652=CARTESIAN_POINT ( 'NONE',  ( 19.02544592524343514, -5.153800228976328945, 73.54057627198103830 ) ) ;
#120653=CARTESIAN_POINT ( 'NONE',  ( 21.52544592524344225, -5.823673210054117533, 48.54057627198103120 ) ) ;
#120654=CARTESIAN_POINT ( 'NONE',  ( -14.29746914071037622, -8.314922557961029526, 19.16775706135234714 ) ) ;
#120655=CARTESIAN_POINT ( 'NONE',  ( -18.67979575497193778, 10.72451020669871902, 98.33442372801901854 ) ) ;
#120656=CARTESIAN_POINT ( 'NONE',  ( -4.483927247898782831, 16.52544592524335698, 67.70942372801901854 ) ) ;
#120657=CARTESIAN_POINT ( 'NONE',  ( -21.53943276465977519, -0.05219959533937600094, 18.75109039468568639 ) ) ;
#120658=CARTESIAN_POINT ( 'NONE',  ( -19.02544592524334988, -5.153800228976617603, 108.9594237280189759 ) ) ;
#120659=CARTESIAN_POINT ( 'NONE',  ( -19.03943276465977164, 0.05219959533909376836, 96.24890960531436690 ) ) ;
#120660=CARTESIAN_POINT ( 'NONE',  ( -16.55341960407617563, 4.379528057220093196, 23.54275706135235424 ) ) ;
#120661=CARTESIAN_POINT ( 'NONE',  ( 9.564922557960805705, 16.46253265017160317, 54.58224293864769550 ) ) ;
#120662=CARTESIAN_POINT ( 'NONE',  ( -16.52544592524335698, -4.483927247898792601, 38.95942372801901854 ) ) ;
#120663=CARTESIAN_POINT ( 'NONE',  ( 12.14591786802309770, 12.06949235617756955, 74.37390960531436690 ) ) ;
#120664=CARTESIAN_POINT ( 'NONE',  ( 8.314922557961029526, -14.29746914071037800, 90.41775706135236135 ) ) ;
#120665=CARTESIAN_POINT ( 'NONE',  ( 15.80617190586769283, -15.72974639402175789, 45.62609039468567573 ) ) ;
#120666=CARTESIAN_POINT ( 'NONE',  ( -19.03943276465977164, 0.05219959533909376836, 66.24890960531436690 ) ) ;
#120667=CARTESIAN_POINT ( 'NONE',  ( 19.02544592524343514, -5.153800228976328945, 88.54057627198102409 ) ) ;
#120668=CARTESIAN_POINT ( 'NONE',  ( -16.53943276465976808, -0.05219959533934237506, 88.75109039468567573 ) ) ;
#120671=CARTESIAN_POINT ( 'NONE',  ( 16.46253265017146816, 9.564922557961045513, 36.66775706135233293 ) ) ;
#120672=CARTESIAN_POINT ( 'NONE',  ( -16.51473224551069308, -9.474510206698971260, 101.6655762719810241 ) ) ;
#120674=CARTESIAN_POINT ( 'NONE',  ( 19.03943276465977164, -0.05219959533909143690, 48.74890960531435979 ) ) ;
#120675=CARTESIAN_POINT ( 'NONE',  ( 19.02544592524343514, -5.153800228976328945, 108.5405762719810383 ) ) ;
#120676=CARTESIAN_POINT ( 'NONE',  ( -14.34966873604972548, 8.224510206698743886, 43.33442372801901143 ) ) ;
#120677=CARTESIAN_POINT ( 'NONE',  ( -13.97604488694547697, 13.89961937509957934, 63.12609039468566152 ) ) ;
#120678=CARTESIAN_POINT ( 'NONE',  ( 16.53943276465976808, 0.05219959533934440121, 61.25109039468567573 ) ) ;
#120679=CARTESIAN_POINT ( 'NONE',  ( -19.05341960407611168, -5.049401038298163336, 106.4572429386476955 ) ) ;
#120680=CARTESIAN_POINT ( 'NONE',  ( 9.564922557960805705, 16.46253265017160317, 79.58224293864769550 ) ) ;
#120681=CARTESIAN_POINT ( 'NONE',  ( 21.52544592524344225, -5.823673210054117533, 98.54057627198105251 ) ) ;
#120682=CARTESIAN_POINT ( 'NONE',  ( 9.564922557961047289, -16.46253265017146816, 60.41775706135233293 ) ) ;
#120683=CARTESIAN_POINT ( 'NONE',  ( 5.049401038298161559, -19.05341960407611168, 97.70724293864766707 ) ) ;
#120684=CARTESIAN_POINT ( 'NONE',  ( 16.51473224551069308, 9.474510206698969483, 24.16557627198102765 ) ) ;
#120685=CARTESIAN_POINT ( 'NONE',  ( 5.153800228976335163, 19.02544592524342804, 79.79057627198102409 ) ) ;
#120686=CARTESIAN_POINT ( 'NONE',  ( 14.34966873604960469, 8.224510206698951720, 39.16557627198102409 ) ) ;
#120687=CARTESIAN_POINT ( 'NONE',  ( 16.51473224551069308, 9.474510206698969483, 29.16557627198103475 ) ) ;
#120688=CARTESIAN_POINT ( 'NONE',  ( -0.05219959533936034679, 19.03943276465977164, 42.50109039468566152 ) ) ;
#120689=CARTESIAN_POINT ( 'NONE',  ( 16.53943276465976808, -0.05219959533910856209, 68.74890960531435269 ) ) ;
#120690=CARTESIAN_POINT ( 'NONE',  ( -10.81492255796105439, 18.62759615963255655, 102.9177570613523756 ) ) ;
#120691=CARTESIAN_POINT ( 'NONE',  ( -13.89961937509977652, 13.97604488694528158, 45.62390960531433848 ) ) ;
#120692=CARTESIAN_POINT ( 'NONE',  ( 4.483927247898545687, 16.52544592524342804, 34.79057627198103120 ) ) ;
#120693=CARTESIAN_POINT ( 'NONE',  ( -0.05219959533937732626, 21.53943276465977519, 102.5010903946856899 ) ) ;
#120694=CARTESIAN_POINT ( 'NONE',  ( -0.05219959533909027116, -19.03943276465977164, 92.49890960531436690 ) ) ;
#120695=CARTESIAN_POINT ( 'NONE',  ( 13.97604488694527802, 13.89961937509977652, 89.37390960531436690 ) ) ;
#120696=CARTESIAN_POINT ( 'NONE',  ( -5.153800228976328057, -19.02544592524343514, 27.29057627198103120 ) ) ;
#120697=CARTESIAN_POINT ( 'NONE',  ( -16.55341960407611168, -4.379528057220339221, 101.4572429386476955 ) ) ;
#120698=CARTESIAN_POINT ( 'NONE',  ( 4.483927247898545687, 16.52544592524342804, 74.79057627198105251 ) ) ;
#120699=CARTESIAN_POINT ( 'NONE',  ( -5.719274019375978568, 21.55341960407610458, 80.20724293864769550 ) ) ;
#120700=CARTESIAN_POINT ( 'NONE',  ( -5.049401038298153566, 19.05341960407611168, 90.20724293864766707 ) ) ;
#120701=CARTESIAN_POINT ( 'NONE',  ( 0.05219959533907565091, 21.53943276465977519, 104.9989096053143669 ) ) ;
#120702=CARTESIAN_POINT ( 'NONE',  ( 19.02544592524343514, -5.153800228976328945, 88.54057627198102409 ) ) ;
#120704=CARTESIAN_POINT ( 'NONE',  ( -16.52544592524342804, 4.483927247898546575, 86.04057627198102409 ) ) ;
#120705=CARTESIAN_POINT ( 'NONE',  ( -16.46253265017160317, 9.564922557960807481, 65.83224293864769550 ) ) ;
#120706=CARTESIAN_POINT ( 'NONE',  ( -5.823673210054116645, -21.52544592524344225, 62.29057627198102409 ) ) ;
#120707=CARTESIAN_POINT ( 'NONE',  ( 22.00000000000000000, -1.132798289211302014E-14, 97.50000000000000000 ) ) ;
#120708=CARTESIAN_POINT ( 'NONE',  ( -15.72974639402197994, 15.80617190586746368, 35.62390960531437401 ) ) ;
#120709=CARTESIAN_POINT ( 'NONE',  ( -19.03943276465977164, -0.05219959533935918106, 108.7510903946856615 ) ) ;
#120710=CARTESIAN_POINT ( 'NONE',  ( 14.29746914071049879, -8.314922557960816363, 98.33224293864769550 ) ) ;
#120711=CARTESIAN_POINT ( 'NONE',  ( -17.26172910966778318, -6.454744622555851130, 94.19353091350778584 ) ) ;
#120712=CARTESIAN_POINT ( 'NONE',  ( -9.564922557960796823, -16.46253265017161027, 87.08224293864769550 ) ) ;
#120713=CARTESIAN_POINT ( 'NONE',  ( -5.153800228976328057, -19.02544592524343514, 42.29057627198101699 ) ) ;
#120714=CARTESIAN_POINT ( 'NONE',  ( -14.29746914071049879, 8.314922557960819915, 75.83224293864769550 ) ) ;
#120716=CARTESIAN_POINT ( 'NONE',  ( -0.05219959533909027116, -19.03943276465977164, 112.4989096053143669 ) ) ;
#120717=CARTESIAN_POINT ( 'NONE',  ( 8.224510206698953496, -14.34966873604960469, 57.91557627198103120 ) ) ;
#120718=CARTESIAN_POINT ( 'NONE',  ( -19.02544592524334988, -5.153800228976617603, 108.9594237280189759 ) ) ;
#120719=CARTESIAN_POINT ( 'NONE',  ( 10.81492255796106328, -18.62759615963255655, 60.41775706135235424 ) ) ;
#120720=CARTESIAN_POINT ( 'NONE',  ( 13.89961937509977652, -13.97604488694527269, 98.12390960531433848 ) ) ;
#120721=CARTESIAN_POINT ( 'NONE',  ( -21.55341960407610458, -5.719274019375992779, 86.45724293864770971 ) ) ;
#120722=CARTESIAN_POINT ( 'NONE',  ( 8.224510206698742110, 14.34966873604972548, 87.08442372801901854 ) ) ;
#120723=CARTESIAN_POINT ( 'NONE',  ( -16.51473224551069308, -9.474510206698971260, 21.66557627198102765 ) ) ;
#120724=CARTESIAN_POINT ( 'NONE',  ( -0.05219959533909027116, -19.03943276465977164, 77.49890960531435269 ) ) ;
#120725=CARTESIAN_POINT ( 'NONE',  ( 18.67979575497178502, 10.72451020669898547, 79.16557627198103830 ) ) ;
#120726=CARTESIAN_POINT ( 'NONE',  ( -19.05341960407617563, 5.049401038297882671, 103.5427570613523329 ) ) ;
#120727=CARTESIAN_POINT ( 'NONE',  ( -16.53943276465976808, 0.05219959533911058130, 46.24890960531435979 ) ) ;
#120728=CARTESIAN_POINT ( 'NONE',  ( 10.72451020669871369, 18.67979575497193778, 62.08442372801901143 ) ) ;
#120729=CARTESIAN_POINT ( 'NONE',  ( -14.29746914071037622, -8.314922557961029526, 89.16775706135236135 ) ) ;
#120730=CARTESIAN_POINT ( 'NONE',  ( -0.05219959533907301413, -21.53943276465977519, 22.49890960531436335 ) ) ;
#120731=CARTESIAN_POINT ( 'NONE',  ( 17.44270441346512612, 5.991230190323099336, 28.86335079264228654 ) ) ;
#120733=CARTESIAN_POINT ( 'NONE',  ( 4.379528057220092307, 16.55341960407617563, 102.2927570613523613 ) ) ;
#120734=CARTESIAN_POINT ( 'NONE',  ( -14.34966873604972548, 8.224510206698743886, 43.33442372801901143 ) ) ;
#120735=CARTESIAN_POINT ( 'NONE',  ( 0.05219959533909260263, 19.03943276465977164, 64.99890960531436690 ) ) ;
#120736=CARTESIAN_POINT ( 'NONE',  ( 19.03943276465977164, -0.05219959533909143690, 73.74890960531435269 ) ) ;
#120737=CARTESIAN_POINT ( 'NONE',  ( -12.06949235617739369, -12.14591786802326823, 79.37609039468567573 ) ) ;
#120738=CARTESIAN_POINT ( 'NONE',  ( 4.379528057220339221, -16.55341960407611168, 42.70724293864770260 ) ) ;
#120739=CARTESIAN_POINT ( 'NONE',  ( -9.474510206698964154, 16.51473224551069663, 50.41557627198102409 ) ) ;
#120740=CARTESIAN_POINT ( 'NONE',  ( -19.02544592524342804, 5.153800228976336051, 51.04057627198103120 ) ) ;
#120741=CARTESIAN_POINT ( 'NONE',  ( -0.05219959533934338120, 16.53943276465976808, 42.50109039468567573 ) ) ;
#120742=CARTESIAN_POINT ( 'NONE',  ( 19.03943276465977164, 0.05219959533936151252, 91.25109039468566152 ) ) ;
#120743=CARTESIAN_POINT ( 'NONE',  ( 14.29746914071049879, -8.314922557960816363, 98.33224293864769550 ) ) ;
#120744=CARTESIAN_POINT ( 'NONE',  ( -0.05219959533909027116, -19.03943276465977164, 67.49890960531436690 ) ) ;
#120745=CARTESIAN_POINT ( 'NONE',  ( 9.474510206698729675, 16.51473224551082808, 102.0844237280190043 ) ) ;
#120747=CARTESIAN_POINT ( 'NONE',  ( 15.72974639402176855, 15.80617190586768217, 91.87609039468568994 ) ) ;
#120748=CARTESIAN_POINT ( 'NONE',  ( 14.34966873604972726, -8.224510206698740333, 65.83442372801900433 ) ) ;
#120750=CARTESIAN_POINT ( 'NONE',  ( 21.55341960407610458, 5.719274019375980345, 63.95724293864770260 ) ) ;
#120751=CARTESIAN_POINT ( 'NONE',  ( -16.52544592524335698, -4.483927247898792601, 53.95942372801900433 ) ) ;
#120752=CARTESIAN_POINT ( 'NONE',  ( 5.153800228976335163, 19.02544592524342804, 34.79057627198102409 ) ) ;
#120753=CARTESIAN_POINT ( 'NONE',  ( 16.46253265017146816, 9.564922557961045513, 36.66775706135233293 ) ) ;
#120754=CARTESIAN_POINT ( 'NONE',  ( 9.564922557960805705, 16.46253265017160317, 94.58224293864769550 ) ) ;
#120755=CARTESIAN_POINT ( 'NONE',  ( 4.483927247898545687, 16.52544592524342804, 114.7905762719810383 ) ) ;
#120756=CARTESIAN_POINT ( 'NONE',  ( 13.89961937509977652, -13.97604488694527269, 68.12390960531436690 ) ) ;
#120757=CARTESIAN_POINT ( 'NONE',  ( -18.67979575497193778, 10.72451020669871902, 83.33442372801903275 ) ) ;
#120758=CARTESIAN_POINT ( 'NONE',  ( 16.51473224551083163, -9.474510206698727899, 35.83442372801899722 ) ) ;
#120759=CARTESIAN_POINT ( 'NONE',  ( -13.97604488694547697, 13.89961937509957934, 23.12609039468565442 ) ) ;
#120760=CARTESIAN_POINT ( 'NONE',  ( 16.51473224551069308, 9.474510206698969483, 59.16557627198102409 ) ) ;
#120761=CARTESIAN_POINT ( 'NONE',  ( -10.72451020669898014, 18.67979575497178502, 30.41557627198101699 ) ) ;
#120762=CARTESIAN_POINT ( 'NONE',  ( -15.72974639402176322, -15.80617190586768395, 84.37609039468570415 ) ) ;
#120763=CARTESIAN_POINT ( 'NONE',  ( -13.89961937509977652, 13.97604488694528158, 65.62390960531436690 ) ) ;
#120764=CARTESIAN_POINT ( 'NONE',  ( -10.72451020669870658, -18.67979575497194134, 74.58442372801901854 ) ) ;
#120765=CARTESIAN_POINT ( 'NONE',  ( -5.719274019375978568, 21.55341960407610458, 40.20724293864769550 ) ) ;
#120766=CARTESIAN_POINT ( 'NONE',  ( -16.46253265017160317, 9.564922557960807481, 80.83224293864769550 ) ) ;
#120767=CARTESIAN_POINT ( 'NONE',  ( 21.55341960407619695, -5.719274019375665929, 36.04275706135234714 ) ) ;
#120768=CARTESIAN_POINT ( 'NONE',  ( -13.89961937509957401, -13.97604488694547875, 59.37609039468566863 ) ) ;
#120769=CARTESIAN_POINT ( 'NONE',  ( 0.05219959533909260263, 19.03943276465977164, 44.99890960531435979 ) ) ;
#120770=CARTESIAN_POINT ( 'NONE',  ( 5.153800228976335163, 19.02544592524342804, 84.79057627198099567 ) ) ;
#120771=CARTESIAN_POINT ( 'NONE',  ( 4.483927247898790824, -16.52544592524335698, 30.20942372801902565 ) ) ;
#120772=CARTESIAN_POINT ( 'NONE',  ( 8.314922557960818139, 14.29746914071049879, 89.58224293864768129 ) ) ;
#120773=CARTESIAN_POINT ( 'NONE',  ( 19.05341960407611168, 5.049401038298154454, 53.95724293864770260 ) ) ;
#120774=CARTESIAN_POINT ( 'NONE',  ( -15.80617190586745835, -15.72974639402198527, 46.87390960531435979 ) ) ;
#120775=CARTESIAN_POINT ( 'NONE',  ( 12.06949235617739724, 12.14591786802326823, 21.87609039468567573 ) ) ;
#120776=CARTESIAN_POINT ( 'NONE',  ( 10.72451020669871369, 18.67979575497193778, 22.08442372801901143 ) ) ;
#120777=CARTESIAN_POINT ( 'NONE',  ( -10.81492255796105439, 18.62759615963255655, 67.91775706135234714 ) ) ;
#120778=CARTESIAN_POINT ( 'NONE',  ( -12.14591786802326823, 12.06949235617739902, 63.12609039468568994 ) ) ;
#120779=CARTESIAN_POINT ( 'NONE',  ( 14.29746914071037800, 8.314922557961029526, 61.66775706135235424 ) ) ;
#120780=AXIS2_PLACEMENT_3D ( 'NONE', #116633, #35794, #86292 ) ;
#120781=CARTESIAN_POINT ( 'NONE',  ( 19.02544592524343514, -5.153800228976328945, 58.54057627198102409 ) ) ;
#120782=CARTESIAN_POINT ( 'NONE',  ( 16.55341960407618274, -4.379528057220086978, 91.04275706135236135 ) ) ;
#120783=CARTESIAN_POINT ( 'NONE',  ( -9.474510206698720793, -16.51473224551083518, 44.58442372801900433 ) ) ;
#120784=CARTESIAN_POINT ( 'NONE',  ( -10.72451020669870658, -18.67979575497194134, 19.58442372801901143 ) ) ;
#120785=CARTESIAN_POINT ( 'NONE',  ( 8.314922557960818139, 14.29746914071049879, 59.58224293864770260 ) ) ;
#120786=CARTESIAN_POINT ( 'NONE',  ( -9.564922557960796823, -16.46253265017161027, 87.08224293864769550 ) ) ;
#120787=CARTESIAN_POINT ( 'NONE',  ( 0.05219959533934541429, -16.53943276465976808, 90.00109039468567573 ) ) ;
#120788=CARTESIAN_POINT ( 'NONE',  ( -5.823673210054431948, 21.52544592524334988, 52.70942372801902565 ) ) ;
#120789=CARTESIAN_POINT ( 'NONE',  ( 14.34966873604972726, -8.224510206698740333, 35.83442372801901143 ) ) ;
#120790=CARTESIAN_POINT ( 'NONE',  ( 18.62759615963255655, 10.81492255796105972, 31.66775706135234358 ) ) ;
#120791=CARTESIAN_POINT ( 'NONE',  ( -14.34966873604960291, -8.224510206698953496, 51.66557627198102409 ) ) ;
#120792=EDGE_LOOP ( 'NONE', ( #7644, #174124 ) ) ;
#120794=CARTESIAN_POINT ( 'NONE',  ( 15.80617190586746368, 15.72974639402197994, 104.3739096053143669 ) ) ;
#120795=CARTESIAN_POINT ( 'NONE',  ( 4.483927247898545687, 16.52544592524342804, 39.79057627198103830 ) ) ;
#120798=CARTESIAN_POINT ( 'NONE',  ( -5.823673210054116645, -21.52544592524344225, 27.29057627198103120 ) ) ;
#120799=CARTESIAN_POINT ( 'NONE',  ( -18.62759615963255300, -10.81492255796106328, 34.16775706135234714 ) ) ;
#120800=CARTESIAN_POINT ( 'NONE',  ( -4.379528057220328563, 16.55341960407611168, 60.20724293864768839 ) ) ;
#120802=CARTESIAN_POINT ( 'NONE',  ( 5.153800228976335163, 19.02544592524342804, 74.79057627198103830 ) ) ;
#120803=CARTESIAN_POINT ( 'NONE',  ( 5.049401038298161559, -19.05341960407611168, 22.70724293864769194 ) ) ;
#120804=CARTESIAN_POINT ( 'NONE',  ( 16.46253265017146816, 9.564922557961045513, 71.66775706135233293 ) ) ;
#120805=CARTESIAN_POINT ( 'NONE',  ( 18.62759615963271287, -10.81492255796078972, 48.33224293864770260 ) ) ;
#120808=CARTESIAN_POINT ( 'NONE',  ( -19.02544592524342804, 5.153800228976336051, 61.04057627198103120 ) ) ;
#120809=CARTESIAN_POINT ( 'NONE',  ( -16.53943276465976808, -0.05219959533934237506, 33.75109039468568284 ) ) ;
#120810=CARTESIAN_POINT ( 'NONE',  ( -5.719274019375665041, -21.55341960407619695, 19.79275706135235069 ) ) ;
#120811=CARTESIAN_POINT ( 'NONE',  ( 12.14591786802309770, 12.06949235617756955, 44.37390960531435979 ) ) ;
#120813=CARTESIAN_POINT ( 'NONE',  ( -19.05341960407611168, -5.049401038298163336, 96.45724293864769550 ) ) ;
#120814=CARTESIAN_POINT ( 'NONE',  ( -21.52544592524343514, 5.823673210054127303, 71.04057627198103830 ) ) ;
#120815=CARTESIAN_POINT ( 'NONE',  ( -5.719274019375978568, 21.55341960407610458, 115.2072429386476955 ) ) ;
#120816=CARTESIAN_POINT ( 'NONE',  ( -8.314922557961024197, 14.29746914071037800, 32.91775706135234714 ) ) ;
#120817=CARTESIAN_POINT ( 'NONE',  ( -21.55341960407610458, -5.719274019375992779, 36.45724293864768839 ) ) ;
#120818=CARTESIAN_POINT ( 'NONE',  ( 15.72974639402176855, 15.80617190586768217, 106.8760903946856899 ) ) ;
#120819=CARTESIAN_POINT ( 'NONE',  ( 9.564922557960805705, 16.46253265017160317, 94.58224293864769550 ) ) ;
#120820=CARTESIAN_POINT ( 'NONE',  ( -16.46253265017160317, 9.564922557960807481, 45.83224293864769550 ) ) ;
#120821=CARTESIAN_POINT ( 'NONE',  ( -0.05219959533909027116, -19.03943276465977164, 92.49890960531436690 ) ) ;
#120822=CARTESIAN_POINT ( 'NONE',  ( -13.97604488694527625, -13.89961937509977652, 76.87390960531433848 ) ) ;
#120824=CARTESIAN_POINT ( 'NONE',  ( 13.89961937509957401, 13.97604488694547697, 51.87609039468566863 ) ) ;
#120825=CARTESIAN_POINT ( 'NONE',  ( -5.049401038297874678, -19.05341960407617918, 19.79275706135233293 ) ) ;
#120826=CARTESIAN_POINT ( 'NONE',  ( -18.62759615963270932, 10.81492255796079327, 25.83224293864769194 ) ) ;
#120827=CARTESIAN_POINT ( 'NONE',  ( 16.52544592524335698, 4.483927247898782831, 106.4594237280190328 ) ) ;
#120828=CARTESIAN_POINT ( 'NONE',  ( -9.474510206698720793, -16.51473224551083518, 89.58442372801900433 ) ) ;
#120829=CARTESIAN_POINT ( 'NONE',  ( -17.31747979337949772, 6.344076630960999275, 58.62055131934815222 ) ) ;
#120830=CARTESIAN_POINT ( 'NONE',  ( -19.02544592524334988, -5.153800228976617603, 83.95942372801901854 ) ) ;
#120831=CARTESIAN_POINT ( 'NONE',  ( -19.02544592524334988, -5.153800228976617603, 38.95942372801900433 ) ) ;
#120832=CARTESIAN_POINT ( 'NONE',  ( 16.52216118717204907, 7.221426719304542274, 108.5759902104699250 ) ) ;
#120833=CARTESIAN_POINT ( 'NONE',  ( 5.049401038298161559, -19.05341960407611168, 42.70724293864767418 ) ) ;
#120834=CARTESIAN_POINT ( 'NONE',  ( -16.52544592524342804, 4.483927247898546575, 46.04057627198103830 ) ) ;
#120836=CARTESIAN_POINT ( 'NONE',  ( -17.12812012977026654, -6.668231424565989052, 111.3594875932314636 ) ) ;
#120837=CARTESIAN_POINT ( 'NONE',  ( 16.53943276465976808, -0.05219959533910856209, 28.74890960531435624 ) ) ;
#120838=DIRECTION ( 'NONE',  ( 0.000000000000000000, 0.000000000000000000, -1.000000000000000000 ) ) ;
#120839=CARTESIAN_POINT ( 'NONE',  ( -8.224510206698735004, -14.34966873604973081, 89.58442372801901854 ) ) ;
#120840=CARTESIAN_POINT ( 'NONE',  ( -16.51473224551069308, -9.474510206698971260, 46.66557627198102409 ) ) ;
#120841=CARTESIAN_POINT ( 'NONE',  ( 5.719274019375673035, 21.55341960407619339, 102.2927570613523613 ) ) ;
#120842=CARTESIAN_POINT ( 'NONE',  ( -14.34966873604972548, 8.224510206698743886, 23.33442372801901499 ) ) ;
#120843=CARTESIAN_POINT ( 'NONE',  ( 18.62759615963255655, 10.81492255796105972, 91.66775706135234714 ) ) ;
#120845=CARTESIAN_POINT ( 'NONE',  ( 13.97604488694527802, 13.89961937509977652, 109.3739096053143669 ) ) ;
#120846=CARTESIAN_POINT ( 'NONE',  ( 9.474510206698971260, -16.51473224551069308, 82.91557627198103830 ) ) ;
#120848=CARTESIAN_POINT ( 'NONE',  ( 15.80617190586746368, 15.72974639402197994, 114.3739096053143527 ) ) ;
#120849=CARTESIAN_POINT ( 'NONE',  ( -0.05219959533910754901, -16.53943276465976808, 77.49890960531433848 ) ) ;
#120850=CARTESIAN_POINT ( 'NONE',  ( 0.05219959533907565091, 21.53943276465977519, 79.99890960531435269 ) ) ;
#120851=CARTESIAN_POINT ( 'NONE',  ( 19.02544592524343514, -5.153800228976328945, 63.54057627198103830 ) ) ;
#120852=CARTESIAN_POINT ( 'NONE',  ( -18.62759615963270932, 10.81492255796079327, 100.8322429386477097 ) ) ;
#120853=CARTESIAN_POINT ( 'NONE',  ( -4.483927247898782831, 16.52544592524335698, 87.70942372801901854 ) ) ;
#120855=CARTESIAN_POINT ( 'NONE',  ( 5.049401038298161559, -19.05341960407611168, 57.70724293864769550 ) ) ;
#120856=CARTESIAN_POINT ( 'NONE',  ( -8.314922557960811034, -14.29746914071050412, 87.08224293864769550 ) ) ;
#120858=CARTESIAN_POINT ( 'NONE',  ( 9.564922557960805705, 16.46253265017160317, 69.58224293864770971 ) ) ;
#120859=CARTESIAN_POINT ( 'NONE',  ( 19.02544592524334988, 5.153800228976608722, 81.45942372801897591 ) ) ;
#120860=CARTESIAN_POINT ( 'NONE',  ( -14.34966873604960291, -8.224510206698953496, 86.66557627198102409 ) ) ;
#120861=CARTESIAN_POINT ( 'NONE',  ( 18.62759615963255655, 10.81492255796105972, 56.66775706135235424 ) ) ;
#120862=CARTESIAN_POINT ( 'NONE',  ( 16.51473224551069308, 9.474510206698969483, 44.16557627198103120 ) ) ;
#120863=CARTESIAN_POINT ( 'NONE',  ( 5.823673210054444382, -21.52544592524334988, 20.20942372801900788 ) ) ;
#120864=CARTESIAN_POINT ( 'NONE',  ( 8.224510206698953496, -14.34966873604960469, 102.9155762719810383 ) ) ;
#120865=DIRECTION ( 'NONE',  ( 1.000000000000000000, -0.000000000000000000, 0.000000000000000000 ) ) ;
#120866=CARTESIAN_POINT ( 'NONE',  ( 13.97604488694527802, 13.89961937509977652, 54.37390960531435979 ) ) ;
#120868=CARTESIAN_POINT ( 'NONE',  ( 19.02544592524334988, 5.153800228976608722, 106.4594237280190185 ) ) ;
#120869=CARTESIAN_POINT ( 'NONE',  ( 9.474510206698971260, -16.51473224551069308, 112.9155762719810383 ) ) ;
#120870=CARTESIAN_POINT ( 'NONE',  ( 21.52544592524334988, 5.823673210054432836, 51.45942372801901854 ) ) ;
#120871=CARTESIAN_POINT ( 'NONE',  ( -19.02544592524342804, 5.153800228976336051, 101.0405762719810241 ) ) ;
#120872=CARTESIAN_POINT ( 'NONE',  ( -19.03943276465977164, -0.05219959533935918106, 83.75109039468567573 ) ) ;
#120873=CARTESIAN_POINT ( 'NONE',  ( 5.153800228976335163, 19.02544592524342804, 54.79057627198103120 ) ) ;
#120874=CARTESIAN_POINT ( 'NONE',  ( 8.314922557960818139, 14.29746914071049879, 74.58224293864768129 ) ) ;
#120875=CARTESIAN_POINT ( 'NONE',  ( 14.29746914071049879, -8.314922557960816363, 83.33224293864769550 ) ) ;
#120876=CARTESIAN_POINT ( 'NONE',  ( 9.564922557960805705, 16.46253265017160317, 84.58224293864769550 ) ) ;
#120877=CARTESIAN_POINT ( 'NONE',  ( -4.483927247898539470, -16.52544592524342804, 82.29057627198103830 ) ) ;
#120878=CARTESIAN_POINT ( 'NONE',  ( 0.05219959533909260263, 19.03943276465977164, 84.99890960531436690 ) ) ;
#120880=CARTESIAN_POINT ( 'NONE',  ( 0.05219959533936267826, -19.03943276465977164, 25.00109039468566152 ) ) ;
#120881=CARTESIAN_POINT ( 'NONE',  ( 16.51473224551069308, 9.474510206698969483, 54.16557627198103120 ) ) ;
#120882=CARTESIAN_POINT ( 'NONE',  ( 4.379528057220339221, -16.55341960407611168, 27.70724293864769905 ) ) ;
#120883=CARTESIAN_POINT ( 'NONE',  ( -13.89961937509977652, 13.97604488694528158, 30.62390960531435269 ) ) ;
#120885=CARTESIAN_POINT ( 'NONE',  ( 10.72451020669871369, 18.67979575497193778, 42.08442372801901854 ) ) ;
#120886=CARTESIAN_POINT ( 'NONE',  ( 19.03943276465977164, 0.05219959533936151252, 71.25109039468566152 ) ) ;
#120887=CARTESIAN_POINT ( 'NONE',  ( -8.224510206698948167, 14.34966873604960824, 40.41557627198103120 ) ) ;
#120888=CARTESIAN_POINT ( 'NONE',  ( -21.52544592524343514, 5.823673210054127303, 86.04057627198102409 ) ) ;
#120889=CARTESIAN_POINT ( 'NONE',  ( -18.67979575497178146, -10.72451020669898902, 31.66557627198102054 ) ) ;
#120890=CARTESIAN_POINT ( 'NONE',  ( -12.14591786802309592, -12.06949235617757132, 71.87390960531438111 ) ) ;
#120891=CARTESIAN_POINT ( 'NONE',  ( 13.89961937509977652, -13.97604488694527269, 48.12390960531435979 ) ) ;
#120892=CARTESIAN_POINT ( 'NONE',  ( 4.379528057220092307, 16.55341960407617563, 107.2927570613523471 ) ) ;
#120893=CARTESIAN_POINT ( 'NONE',  ( 14.29746914071037800, 8.314922557961029526, 56.66775706135235424 ) ) ;
#120894=CARTESIAN_POINT ( 'NONE',  ( -21.55341960407610458, -5.719274019375992779, 41.45724293864769550 ) ) ;
#120895=CARTESIAN_POINT ( 'NONE',  ( 21.52544592524334988, 5.823673210054432836, 111.4594237280190328 ) ) ;
#120896=CARTESIAN_POINT ( 'NONE',  ( -5.153800228976328057, -19.02544592524343514, 87.29057627198103830 ) ) ;
#120897=CARTESIAN_POINT ( 'NONE',  ( -8.314922557961024197, 14.29746914071037800, 77.91775706135231871 ) ) ;
#120898=CARTESIAN_POINT ( 'NONE',  ( 12.14591786802309770, 12.06949235617756955, 114.3739096053143527 ) ) ;
#120899=CARTESIAN_POINT ( 'NONE',  ( -16.53943276465976808, 0.05219959533911058130, 31.24890960531435979 ) ) ;
#120900=CARTESIAN_POINT ( 'NONE',  ( 19.03943276465977164, -0.05219959533909143690, 108.7489096053143527 ) ) ;
#120901=CARTESIAN_POINT ( 'NONE',  ( -0.05219959533909027116, -19.03943276465977164, 92.49890960531436690 ) ) ;
#120902=CARTESIAN_POINT ( 'NONE',  ( 15.80617190586746368, 15.72974639402197994, 29.37390960531435269 ) ) ;
#120904=CARTESIAN_POINT ( 'NONE',  ( -8.314922557960811034, -14.29746914071050412, 72.08224293864769550 ) ) ;
#120906=CARTESIAN_POINT ( 'NONE',  ( 8.224510206698953496, -14.34966873604960469, 57.91557627198103120 ) ) ;
#120907=CARTESIAN_POINT ( 'NONE',  ( -4.483927247898782831, 16.52544592524335698, 57.70942372801901143 ) ) ;
#120909=CARTESIAN_POINT ( 'NONE',  ( -19.02544592524334988, -5.153800228976617603, 48.95942372801900433 ) ) ;
#120910=CARTESIAN_POINT ( 'NONE',  ( -9.474510206698964154, 16.51473224551069663, 85.41557627198102409 ) ) ;
#120911=CARTESIAN_POINT ( 'NONE',  ( 16.46253265017146816, 9.564922557961045513, 66.66775706135233293 ) ) ;
#120913=CARTESIAN_POINT ( 'NONE',  ( -16.46253265017146816, -9.564922557961047289, 54.16775706135234003 ) ) ;
#120914=CARTESIAN_POINT ( 'NONE',  ( 16.51473224551083163, -9.474510206698727899, 100.8344237280190043 ) ) ;
#120915=CARTESIAN_POINT ( 'NONE',  ( 8.314922557961029526, -14.29746914071037800, 95.41775706135234714 ) ) ;
#120917=CARTESIAN_POINT ( 'NONE',  ( 5.153800228976335163, 19.02544592524342804, 44.79057627198103830 ) ) ;
#120918=CARTESIAN_POINT ( 'NONE',  ( -19.05341960407611168, -5.049401038298163336, 111.4572429386476671 ) ) ;
#120919=CARTESIAN_POINT ( 'NONE',  ( 10.81492255796106328, -18.62759615963255655, 55.41775706135234714 ) ) ;
#120920=CARTESIAN_POINT ( 'NONE',  ( 5.049401038297881783, 19.05341960407617563, 97.29275706135233293 ) ) ;
#120922=CARTESIAN_POINT ( 'NONE',  ( -16.46253265017160317, 9.564922557960807481, 55.83224293864769550 ) ) ;
#120924=CARTESIAN_POINT ( 'NONE',  ( 4.483927247898545687, 16.52544592524342804, 79.79057627198102409 ) ) ;
#120925=CARTESIAN_POINT ( 'NONE',  ( 13.89961937509977652, -13.97604488694527269, 63.12390960531435979 ) ) ;
#120926=CARTESIAN_POINT ( 'NONE',  ( 19.05341960407611168, 5.049401038298154454, 78.95724293864769550 ) ) ;
#120927=CARTESIAN_POINT ( 'NONE',  ( -16.46253265017146816, -9.564922557961047289, 79.16775706135234714 ) ) ;
#120928=CARTESIAN_POINT ( 'NONE',  ( -18.62759615963270932, 10.81492255796079327, 70.83224293864770971 ) ) ;
#120929=CARTESIAN_POINT ( 'NONE',  ( -16.52544592524342804, 4.483927247898546575, 116.0405762719810383 ) ) ;
#120930=CARTESIAN_POINT ( 'NONE',  ( -5.153800228976607833, 19.02544592524334988, 42.70942372801901143 ) ) ;
#120931=CARTESIAN_POINT ( 'NONE',  ( 16.51473224551069308, 9.474510206698969483, 49.16557627198102409 ) ) ;
#120932=CARTESIAN_POINT ( 'NONE',  ( 19.05341960407611168, 5.049401038298154454, 78.95724293864769550 ) ) ;
#120933=CARTESIAN_POINT ( 'NONE',  ( -0.05219959533907301413, -21.53943276465977519, 87.49890960531436690 ) ) ;
#120934=CARTESIAN_POINT ( 'NONE',  ( 14.29746914071049879, -8.314922557960816363, 78.33224293864770971 ) ) ;
#120935=CARTESIAN_POINT ( 'NONE',  ( 13.97604488694548053, -13.89961937509957401, 50.62609039468566152 ) ) ;
#120936=CARTESIAN_POINT ( 'NONE',  ( -10.72451020669898014, 18.67979575497178502, 80.41557627198103830 ) ) ;
#120937=CARTESIAN_POINT ( 'NONE',  ( -18.62759615963270932, 10.81492255796079327, 60.83224293864769550 ) ) ;
#120938=CARTESIAN_POINT ( 'NONE',  ( 14.29746914071049879, -8.314922557960816363, 33.33224293864769550 ) ) ;
#120939=CARTESIAN_POINT ( 'NONE',  ( 15.72974639402176855, 15.80617190586768217, 91.87609039468568994 ) ) ;
#120940=CARTESIAN_POINT ( 'NONE',  ( 16.46253265017160672, -9.564922557960803928, 78.33224293864769550 ) ) ;
#120941=CARTESIAN_POINT ( 'NONE',  ( 5.153800228976335163, 19.02544592524342804, 24.79057627198102765 ) ) ;
#120943=CARTESIAN_POINT ( 'NONE',  ( -21.52544592524334988, -5.823673210054445271, 23.95942372801901143 ) ) ;
#120944=CARTESIAN_POINT ( 'NONE',  ( -21.52544592524334988, -5.823673210054445271, 43.95942372801902565 ) ) ;
#120945=CARTESIAN_POINT ( 'NONE',  ( 16.51473224551069308, 9.474510206698969483, 44.16557627198103120 ) ) ;
#120946=CARTESIAN_POINT ( 'NONE',  ( 15.80617190586769283, -15.72974639402175789, 20.62609039468568639 ) ) ;
#120947=CARTESIAN_POINT ( 'NONE',  ( 0.05219959533936267826, -19.03943276465977164, 60.00109039468566863 ) ) ;
#120948=CARTESIAN_POINT ( 'NONE',  ( 19.03943276465977164, -0.05219959533909143690, 38.74890960531436690 ) ) ;
#120949=CARTESIAN_POINT ( 'NONE',  ( -12.06949235617739369, -12.14591786802326823, 29.37609039468568284 ) ) ;
#120950=CARTESIAN_POINT ( 'NONE',  ( -19.05341960407611168, -5.049401038298163336, 26.45724293864769550 ) ) ;
#120951=CARTESIAN_POINT ( 'NONE',  ( 8.314922557961029526, -14.29746914071037800, 60.41775706135235424 ) ) ;
#120952=CARTESIAN_POINT ( 'NONE',  ( -19.03943276465977164, 0.05219959533909376836, 41.24890960531435269 ) ) ;
#120954=CARTESIAN_POINT ( 'NONE',  ( -16.46253265017160317, 9.564922557960807481, 85.83224293864769550 ) ) ;
#120955=CARTESIAN_POINT ( 'NONE',  ( -5.049401038298153566, 19.05341960407611168, 30.20724293864768839 ) ) ;
#120956=CARTESIAN_POINT ( 'NONE',  ( 5.719274019375991003, -21.55341960407610458, 57.70724293864770260 ) ) ;
#120957=CARTESIAN_POINT ( 'NONE',  ( 4.379528057220092307, 16.55341960407617563, 52.29275706135236135 ) ) ;
#120958=CARTESIAN_POINT ( 'NONE',  ( -21.53943276465977519, -0.05219959533937600094, 93.75109039468567573 ) ) ;
#120959=CARTESIAN_POINT ( 'NONE',  ( 16.46253265017160672, -9.564922557960803928, 43.33224293864769550 ) ) ;
#120960=CARTESIAN_POINT ( 'NONE',  ( 4.483927247898545687, 16.52544592524342804, 29.79057627198102409 ) ) ;
#120961=CARTESIAN_POINT ( 'NONE',  ( 4.379528057220339221, -16.55341960407611168, 62.70724293864769550 ) ) ;
#120962=CARTESIAN_POINT ( 'NONE',  ( -16.51473224551069308, -9.474510206698971260, 61.66557627198103120 ) ) ;
#120963=CARTESIAN_POINT ( 'NONE',  ( 21.52544592524334988, 5.823673210054432836, 111.4594237280190328 ) ) ;
#120964=CARTESIAN_POINT ( 'NONE',  ( -5.823673210054431948, 21.52544592524334988, 22.70942372801901499 ) ) ;
#120965=CARTESIAN_POINT ( 'NONE',  ( -0.05219959533937732626, 21.53943276465977519, 92.50109039468567573 ) ) ;
#120966=CARTESIAN_POINT ( 'NONE',  ( -16.52544592524335698, -4.483927247898792601, 48.95942372801902565 ) ) ;
#120967=CARTESIAN_POINT ( 'NONE',  ( 4.483927247898790824, -16.52544592524335698, 25.20942372801901854 ) ) ;
#120968=EDGE_CURVE ( 'NONE', #194969, #163715, #105680, .T. ) ;
#120969=CARTESIAN_POINT ( 'NONE',  ( 8.224510206698953496, -14.34966873604960469, 97.91557627198103830 ) ) ;
#120970=CARTESIAN_POINT ( 'NONE',  ( 10.81492255796106328, -18.62759615963255655, 95.41775706135234714 ) ) ;
#120971=CARTESIAN_POINT ( 'NONE',  ( -4.379528057220328563, 16.55341960407611168, 40.20724293864769550 ) ) ;
#120972=CARTESIAN_POINT ( 'NONE',  ( -0.05219959533909027116, -19.03943276465977164, 22.49890960531436690 ) ) ;
#120973=CARTESIAN_POINT ( 'NONE',  ( 4.379528057220092307, 16.55341960407617563, 47.29275706135234003 ) ) ;
#120974=CARTESIAN_POINT ( 'NONE',  ( -4.379528057220328563, 16.55341960407611168, 60.20724293864768839 ) ) ;
#120975=CARTESIAN_POINT ( 'NONE',  ( -4.483927247898782831, 16.52544592524335698, 102.7094237280190185 ) ) ;
#120976=CARTESIAN_POINT ( 'NONE',  ( -5.049401038298153566, 19.05341960407611168, 115.2072429386477097 ) ) ;
#120977=CARTESIAN_POINT ( 'NONE',  ( -10.81492255796078084, -18.62759615963271287, 22.08224293864769194 ) ) ;
#120978=CARTESIAN_POINT ( 'NONE',  ( 10.81492255796106328, -18.62759615963255655, 110.4177570613523756 ) ) ;
#120979=CARTESIAN_POINT ( 'NONE',  ( 12.14591786802309770, 12.06949235617756955, 89.37390960531435269 ) ) ;
#120980=CARTESIAN_POINT ( 'NONE',  ( 19.03943276465977164, -0.05219959533909143690, 93.74890960531435269 ) ) ;
#120981=ORIENTED_EDGE ( 'NONE', *, *, #192276, .F. ) ;
#120982=CARTESIAN_POINT ( 'NONE',  ( -14.29746914071037622, -8.314922557961029526, 44.16775706135234714 ) ) ;
#120983=CARTESIAN_POINT ( 'NONE',  ( -13.89961937509977652, 13.97604488694528158, 40.62390960531435979 ) ) ;
#120984=CARTESIAN_POINT ( 'NONE',  ( -0.05219959533909027116, -19.03943276465977164, 107.4989096053143527 ) ) ;
#120985=CARTESIAN_POINT ( 'NONE',  ( -8.224510206698735004, -14.34966873604973081, 44.58442372801901854 ) ) ;
#120986=DIRECTION ( 'NONE',  ( -1.000000000000000000, 0.000000000000000000, 0.000000000000000000 ) ) ;
#120987=CARTESIAN_POINT ( 'NONE',  ( -16.51473224551082808, 9.474510206698731452, 53.33442372801900433 ) ) ;
#120988=CARTESIAN_POINT ( 'NONE',  ( -0.05219959533909027116, -19.03943276465977164, 52.49890960531436690 ) ) ;
#120989=CARTESIAN_POINT ( 'NONE',  ( 8.314922557961029526, -14.29746914071037800, 85.41775706135236135 ) ) ;
#120990=CARTESIAN_POINT ( 'NONE',  ( 16.46253265017146816, 9.564922557961045513, 86.66775706135233293 ) ) ;
#120991=CARTESIAN_POINT ( 'NONE',  ( 5.049401038297881783, 19.05341960407617563, 32.29275706135233293 ) ) ;
#120992=CARTESIAN_POINT ( 'NONE',  ( -0.05219959533909027116, -19.03943276465977164, 62.49890960531435979 ) ) ;
#120993=CARTESIAN_POINT ( 'NONE',  ( -8.224510206698948167, 14.34966873604960824, 105.4155762719810383 ) ) ;
#120994=CARTESIAN_POINT ( 'NONE',  ( -19.05341960407617563, 5.049401038297882671, 68.54275706135230450 ) ) ;
#120995=CARTESIAN_POINT ( 'NONE',  ( 15.72974639402199770, -15.80617190586745480, 63.12390960531435979 ) ) ;
#120996=CARTESIAN_POINT ( 'NONE',  ( -19.02544592524334988, -5.153800228976617603, 23.95942372801900078 ) ) ;
#120997=CARTESIAN_POINT ( 'NONE',  ( 9.474510206698971260, -16.51473224551069308, 97.91557627198102409 ) ) ;
#120999=CARTESIAN_POINT ( 'NONE',  ( -21.53943276465977519, 0.05219959533907696930, 81.24890960531436690 ) ) ;
#121000=CARTESIAN_POINT ( 'NONE',  ( -16.36317988757058828, 7.306389748694927633, 84.09789608363227842 ) ) ;
#121001=CARTESIAN_POINT ( 'NONE',  ( 19.02544592524334988, 5.153800228976608722, 106.4594237280190185 ) ) ;
#121002=CARTESIAN_POINT ( 'NONE',  ( -19.01533133064925707, 5.499999999999454658, 58.76586590595741910 ) ) ;
#121003=CARTESIAN_POINT ( 'NONE',  ( 14.29746914071037800, 8.314922557961029526, 31.66775706135234358 ) ) ;
#121004=CARTESIAN_POINT ( 'NONE',  ( 9.564922557960805705, 16.46253265017160317, 34.58224293864770260 ) ) ;
#121005=CARTESIAN_POINT ( 'NONE',  ( 16.46253265017160672, -9.564922557960803928, 113.3322429386476955 ) ) ;
#121006=CARTESIAN_POINT ( 'NONE',  ( -21.52544592524343514, 5.823673210054127303, 91.04057627198103830 ) ) ;
#121007=CARTESIAN_POINT ( 'NONE',  ( -18.62759615963255300, -10.81492255796106328, 54.16775706135235424 ) ) ;
#121008=CARTESIAN_POINT ( 'NONE',  ( -13.89961937509957401, -13.97604488694547875, 104.3760903946856757 ) ) ;
#121009=CARTESIAN_POINT ( 'NONE',  ( 18.62759615963255655, 10.81492255796105972, 106.6677570613523756 ) ) ;
#121010=CARTESIAN_POINT ( 'NONE',  ( -16.55341960407617563, 4.379528057220093196, 108.5427570613523756 ) ) ;
#121011=CARTESIAN_POINT ( 'NONE',  ( 18.62759615963271287, -10.81492255796078972, 98.33224293864769550 ) ) ;
#121012=CARTESIAN_POINT ( 'NONE',  ( 8.314922557960818139, 14.29746914071049879, 44.58224293864769550 ) ) ;
#121013=CARTESIAN_POINT ( 'NONE',  ( 19.02544592524334988, 5.153800228976608722, 86.45942372801900433 ) ) ;
#121014=CARTESIAN_POINT ( 'NONE',  ( 13.89961937509957401, 13.97604488694547697, 51.87609039468566863 ) ) ;
#121015=CARTESIAN_POINT ( 'NONE',  ( -15.72974639402176322, -15.80617190586768395, 64.37609039468568994 ) ) ;
#121016=CARTESIAN_POINT ( 'NONE',  ( -13.89961937509957401, -13.97604488694547875, 44.37609039468566863 ) ) ;
#121017=CARTESIAN_POINT ( 'NONE',  ( 0.05219959533910956823, 16.53943276465976808, 99.99890960531436690 ) ) ;
#121018=CARTESIAN_POINT ( 'NONE',  ( -15.80617190586745835, -15.72974639402198527, 36.87390960531435979 ) ) ;
#121019=CARTESIAN_POINT ( 'NONE',  ( -4.379528057220328563, 16.55341960407611168, 35.20724293864768839 ) ) ;
#121021=CARTESIAN_POINT ( 'NONE',  ( -21.53943276465977519, -0.05219959533937600094, 103.7510903946857042 ) ) ;
#121022=CARTESIAN_POINT ( 'NONE',  ( 12.14591786802327356, -12.06949235617739191, 75.62609039468567573 ) ) ;
#121023=CARTESIAN_POINT ( 'NONE',  ( -12.14591786802309592, -12.06949235617757132, 21.87390960531436690 ) ) ;
#121024=CARTESIAN_POINT ( 'NONE',  ( -21.55341960407619339, 5.719274019375674811, 63.54275706135234003 ) ) ;
#121025=CARTESIAN_POINT ( 'NONE',  ( 21.55341960407619695, -5.719274019375665929, 61.04275706135234714 ) ) ;
#121026=CARTESIAN_POINT ( 'NONE',  ( 21.53943276465977519, -0.05219959533907433946, 73.74890960531433848 ) ) ;
#121028=CARTESIAN_POINT ( 'NONE',  ( 17.58332526062529411, -7.635886036038503910, 63.42334959558468199 ) ) ;
#121029=CARTESIAN_POINT ( 'NONE',  ( -5.823673210054431948, 21.52544592524334988, 47.70942372801902565 ) ) ;
#121030=CARTESIAN_POINT ( 'NONE',  ( -19.03943276465977164, 0.05219959533909376836, 26.24890960531435624 ) ) ;
#121031=CARTESIAN_POINT ( 'NONE',  ( 9.474510206698971260, -16.51473224551069308, 37.91557627198102409 ) ) ;
#121032=CARTESIAN_POINT ( 'NONE',  ( -14.29746914071049879, 8.314922557960819915, 75.83224293864769550 ) ) ;
#121033=CARTESIAN_POINT ( 'NONE',  ( 0.05219959533909260263, 19.03943276465977164, 84.99890960531436690 ) ) ;
#121034=CARTESIAN_POINT ( 'NONE',  ( -0.05219959533910754901, -16.53943276465976808, 32.49890960531435979 ) ) ;
#121035=CARTESIAN_POINT ( 'NONE',  ( -16.55341960407611168, -4.379528057220339221, 101.4572429386476955 ) ) ;
#121036=CARTESIAN_POINT ( 'NONE',  ( -5.823673210054116645, -21.52544592524344225, 67.29057627198103830 ) ) ;
#121038=CARTESIAN_POINT ( 'NONE',  ( 0.05219959533907565091, 21.53943276465977519, 99.99890960531436690 ) ) ;
#121039=CARTESIAN_POINT ( 'NONE',  ( -5.049401038298153566, 19.05341960407611168, 115.2072429386477097 ) ) ;
#121042=CARTESIAN_POINT ( 'NONE',  ( 16.51473224551069308, 9.474510206698969483, 64.16557627198102409 ) ) ;
#121043=CARTESIAN_POINT ( 'NONE',  ( 0.05219959533936267826, -19.03943276465977164, 100.0010903946856757 ) ) ;
#121044=CARTESIAN_POINT ( 'NONE',  ( 15.80617190586746368, 15.72974639402197994, 59.37390960531436690 ) ) ;
#121045=CARTESIAN_POINT ( 'NONE',  ( 10.72451020669871369, 18.67979575497193778, 82.08442372801901854 ) ) ;
#121046=CARTESIAN_POINT ( 'NONE',  ( -19.03943276465977164, 0.05219959533909376836, 61.24890960531436690 ) ) ;
#121048=CARTESIAN_POINT ( 'NONE',  ( 19.05341960407611168, 5.049401038298154454, 98.95724293864766707 ) ) ;
#121049=CARTESIAN_POINT ( 'NONE',  ( -16.55341960407617563, 4.379528057220093196, 83.54275706135234714 ) ) ;
#121050=CARTESIAN_POINT ( 'NONE',  ( 21.53943276465977519, 0.05219959533937863772, 56.25109039468568284 ) ) ;
#121051=CARTESIAN_POINT ( 'NONE',  ( 10.72451020669871369, 18.67979575497193778, 97.08442372801904696 ) ) ;
#121052=CARTESIAN_POINT ( 'NONE',  ( 15.72974639402199770, -15.80617190586745480, 113.1239096053143953 ) ) ;
#121054=CARTESIAN_POINT ( 'NONE',  ( 15.72974639402199770, -15.80617190586745480, 73.12390960531436690 ) ) ;
#121055=CARTESIAN_POINT ( 'NONE',  ( 5.153800228976615827, -19.02544592524334988, 45.20942372801901143 ) ) ;
#121056=CARTESIAN_POINT ( 'NONE',  ( 10.81492255796078972, 18.62759615963270932, 39.58224293864769550 ) ) ;
#121058=CARTESIAN_POINT ( 'NONE',  ( -16.51473224551069308, -9.474510206698971260, 76.66557627198103830 ) ) ;
#121059=CARTESIAN_POINT ( 'NONE',  ( 4.379528057220339221, -16.55341960407611168, 32.70724293864770260 ) ) ;
#121060=DIRECTION ( 'NONE',  ( 0.000000000000000000, 0.000000000000000000, -1.000000000000000000 ) ) ;
#121061=CARTESIAN_POINT ( 'NONE',  ( -19.25918095147780562, -5.499999999999485745, 79.45284276293931214 ) ) ;
#121062=CARTESIAN_POINT ( 'NONE',  ( 5.049401038297881783, 19.05341960407617563, 92.29275706135234714 ) ) ;
#121063=CARTESIAN_POINT ( 'NONE',  ( 18.62759615963271287, -10.81492255796078972, 78.33224293864770971 ) ) ;
#121064=CARTESIAN_POINT ( 'NONE',  ( 16.52544592524342804, -4.483927247898539470, 58.54057627198103120 ) ) ;
#121065=CARTESIAN_POINT ( 'NONE',  ( 4.379528057220092307, 16.55341960407617563, 32.29275706135235424 ) ) ;
#121066=CARTESIAN_POINT ( 'NONE',  ( 13.97604488694527802, 13.89961937509977652, 44.37390960531435269 ) ) ;
#121067=CARTESIAN_POINT ( 'NONE',  ( 5.719274019375991003, -21.55341960407610458, 107.7072429386476955 ) ) ;
#121068=CARTESIAN_POINT ( 'NONE',  ( -19.02544592524334988, -5.153800228976617603, 83.95942372801901854 ) ) ;
#121069=CARTESIAN_POINT ( 'NONE',  ( -16.51473224551069308, -9.474510206698971260, 81.66557627198103830 ) ) ;
#121070=CARTESIAN_POINT ( 'NONE',  ( -12.06949235617756955, 12.14591786802309770, 90.62390960531436690 ) ) ;
#121071=CARTESIAN_POINT ( 'NONE',  ( -19.05341960407611168, -5.049401038298163336, 76.45724293864769550 ) ) ;
#121072=CARTESIAN_POINT ( 'NONE',  ( -14.34966873604960291, -8.224510206698953496, 61.66557627198103120 ) ) ;
#121073=CARTESIAN_POINT ( 'NONE',  ( -16.51473224551069308, -9.474510206698971260, 26.66557627198103120 ) ) ;
#121074=CARTESIAN_POINT ( 'NONE',  ( -17.22444507756011234, -5.345458043314972763, 20.98594102011676554 ) ) ;
#121075=CARTESIAN_POINT ( 'NONE',  ( -14.34966873604960291, -8.224510206698953496, 51.66557627198102409 ) ) ;
#121076=CARTESIAN_POINT ( 'NONE',  ( 19.02544592524343514, -5.153800228976328945, 88.54057627198102409 ) ) ;
#121077=CARTESIAN_POINT ( 'NONE',  ( -17.49999999999999645, 5.499999999999997335, 120.0000000000000142 ) ) ;
#121078=CARTESIAN_POINT ( 'NONE',  ( 19.02544592524334988, 5.153800228976608722, 56.45942372801898301 ) ) ;
#121079=CARTESIAN_POINT ( 'NONE',  ( -8.224510206698735004, -14.34966873604973081, 64.58442372801900433 ) ) ;
#121080=CARTESIAN_POINT ( 'NONE',  ( -21.53943276465977519, 0.05219959533907696930, 76.24890960531435269 ) ) ;
#121081=CARTESIAN_POINT ( 'NONE',  ( 16.51473224551083163, -9.474510206698727899, 40.83442372801900433 ) ) ;
#121082=CARTESIAN_POINT ( 'NONE',  ( -13.97604488694527625, -13.89961937509977652, 81.87390960531436690 ) ) ;
#121083=CARTESIAN_POINT ( 'NONE',  ( -17.60691670004652920, -5.499999999999996447, 74.13333313366439370 ) ) ;
#121084=CARTESIAN_POINT ( 'NONE',  ( -15.72974639402197994, 15.80617190586746368, 30.62390960531436335 ) ) ;
#121086=CARTESIAN_POINT ( 'NONE',  ( -13.89961937509977652, 13.97604488694528158, 70.62390960531432427 ) ) ;
#121087=CARTESIAN_POINT ( 'NONE',  ( -21.53943276465977519, -0.05219959533937600094, 53.75109039468568994 ) ) ;
#121088=CARTESIAN_POINT ( 'NONE',  ( -19.03943276465977164, 0.05219959533909376836, 21.24890960531436335 ) ) ;
#121089=CARTESIAN_POINT ( 'NONE',  ( 0.05219959533907565091, 21.53943276465977519, 109.9989096053143527 ) ) ;
#121090=CARTESIAN_POINT ( 'NONE',  ( -16.46253265017160317, 9.564922557960807481, 90.83224293864769550 ) ) ;
#121091=VERTEX_POINT ( 'NONE', #196728 ) ;
#121092=CARTESIAN_POINT ( 'NONE',  ( 18.67979575497194134, -10.72451020669871369, 35.83442372801901143 ) ) ;
#121093=VERTEX_POINT ( 'NONE', #60163 ) ;
#121094=CARTESIAN_POINT ( 'NONE',  ( 19.05341960407611168, 5.049401038298154454, 98.95724293864766707 ) ) ;
#121096=CARTESIAN_POINT ( 'NONE',  ( 15.80617190586746368, 15.72974639402197994, 104.3739096053143669 ) ) ;
#121097=CARTESIAN_POINT ( 'NONE',  ( -16.51473224551069308, -9.474510206698971260, 46.66557627198102409 ) ) ;
#121098=CARTESIAN_POINT ( 'NONE',  ( -4.483927247898782831, 16.52544592524335698, 27.70942372801901854 ) ) ;
#121100=CARTESIAN_POINT ( 'NONE',  ( 15.80617190586769283, -15.72974639402175789, 100.6260903946857184 ) ) ;
#121101=CARTESIAN_POINT ( 'NONE',  ( 19.02544592524343514, -5.153800228976328945, 33.54057627198102409 ) ) ;
#121102=CARTESIAN_POINT ( 'NONE',  ( 10.81492255796106328, -18.62759615963255655, 105.4177570613523613 ) ) ;
#121103=CARTESIAN_POINT ( 'NONE',  ( 9.564922557960805705, 16.46253265017160317, 84.58224293864769550 ) ) ;
#121104=CARTESIAN_POINT ( 'NONE',  ( -21.55341960407619339, 5.719274019375674811, 63.54275706135234003 ) ) ;
#121106=CARTESIAN_POINT ( 'NONE',  ( 5.153800228976335163, 19.02544592524342804, 99.79057627198102409 ) ) ;
#121107=CARTESIAN_POINT ( 'NONE',  ( 17.60691670004650788, 5.500000000000060396, 46.63333313366440791 ) ) ;
#121108=CARTESIAN_POINT ( 'NONE',  ( 14.34966873604972726, -8.224510206698740333, 55.83442372801901854 ) ) ;
#121109=CARTESIAN_POINT ( 'NONE',  ( 8.224510206698742110, 14.34966873604972548, 62.08442372801901143 ) ) ;
#121110=CARTESIAN_POINT ( 'NONE',  ( 18.62759615963255655, 10.81492255796105972, 51.66775706135234714 ) ) ;
#121111=CARTESIAN_POINT ( 'NONE',  ( 18.67979575497194134, -10.72451020669871369, 95.83442372801903275 ) ) ;
#121113=CARTESIAN_POINT ( 'NONE',  ( -16.55341960407617563, 4.379528057220093196, 28.54275706135234358 ) ) ;
#121114=CARTESIAN_POINT ( 'NONE',  ( 19.05341960407611168, 5.049401038298154454, 78.95724293864769550 ) ) ;
#121115=CARTESIAN_POINT ( 'NONE',  ( 19.05341960407611168, 5.049401038298154454, 93.95724293864769550 ) ) ;
#121116=CARTESIAN_POINT ( 'NONE',  ( -19.03943276465977164, 0.05219959533909376836, 111.2489096053143669 ) ) ;
#121117=CARTESIAN_POINT ( 'NONE',  ( -16.46253265017160317, 9.564922557960807481, 30.83224293864769550 ) ) ;
#121118=CARTESIAN_POINT ( 'NONE',  ( -10.72451020669898014, 18.67979575497178502, 30.41557627198101699 ) ) ;
#121119=CARTESIAN_POINT ( 'NONE',  ( 14.29746914071037800, 8.314922557961029526, 86.66775706135234714 ) ) ;
#121120=CARTESIAN_POINT ( 'NONE',  ( -12.14591786802309592, -12.06949235617757132, 66.87390960531436690 ) ) ;
#121121=CARTESIAN_POINT ( 'NONE',  ( -5.049401038298153566, 19.05341960407611168, 70.20724293864769550 ) ) ;
#121122=CARTESIAN_POINT ( 'NONE',  ( -21.52544592524334988, -5.823673210054445271, 93.95942372801903275 ) ) ;
#121124=CARTESIAN_POINT ( 'NONE',  ( 0.05219959533934541429, -16.53943276465976808, 25.00109039468567218 ) ) ;
#121125=CARTESIAN_POINT ( 'NONE',  ( -16.53943276465976808, 0.05219959533911058130, 76.24890960531435269 ) ) ;
#121126=CARTESIAN_POINT ( 'NONE',  ( -15.80617190586768217, 15.72974639402176855, 28.12609039468568284 ) ) ;
#121127=CARTESIAN_POINT ( 'NONE',  ( 5.719274019375991003, -21.55341960407610458, 72.70724293864769550 ) ) ;
#121129=CARTESIAN_POINT ( 'NONE',  ( -5.153800228976607833, 19.02544592524334988, 32.70942372801899722 ) ) ;
#121131=CARTESIAN_POINT ( 'NONE',  ( -19.02544592524342804, 5.153800228976336051, 81.04057627198103830 ) ) ;
#121132=CARTESIAN_POINT ( 'NONE',  ( 16.52544592524342804, -4.483927247898539470, 43.54057627198103830 ) ) ;
#121133=CARTESIAN_POINT ( 'NONE',  ( 4.483927247898545687, 16.52544592524342804, 39.79057627198103830 ) ) ;
#121134=CARTESIAN_POINT ( 'NONE',  ( 12.14591786802327356, -12.06949235617739191, 110.6260903946857042 ) ) ;
#121135=CARTESIAN_POINT ( 'NONE',  ( 16.46253265017146816, 9.564922557961045513, 61.66775706135234003 ) ) ;
#121136=CARTESIAN_POINT ( 'NONE',  ( 19.20446147854530139, 5.499999999999909406, 51.88999695167680670 ) ) ;
#121137=CARTESIAN_POINT ( 'NONE',  ( -9.474510206698964154, 16.51473224551069663, 100.4155762719810241 ) ) ;
#121138=CARTESIAN_POINT ( 'NONE',  ( 4.379528057220339221, -16.55341960407611168, 77.70724293864770971 ) ) ;
#121140=CARTESIAN_POINT ( 'NONE',  ( -16.51473224551069308, -9.474510206698971260, 26.66557627198103120 ) ) ;
#121141=CARTESIAN_POINT ( 'NONE',  ( -10.81492255796078084, -18.62759615963271287, 32.08224293864769550 ) ) ;
#121142=CARTESIAN_POINT ( 'NONE',  ( -21.55341960407610458, -5.719274019375992779, 71.45724293864769550 ) ) ;
#121143=CARTESIAN_POINT ( 'NONE',  ( -4.483927247898539470, -16.52544592524342804, 112.2905762719810241 ) ) ;
#121144=CARTESIAN_POINT ( 'NONE',  ( 14.34966873604972726, -8.224510206698740333, 60.83442372801901854 ) ) ;
#121145=CARTESIAN_POINT ( 'NONE',  ( -19.03943276465977164, 0.05219959533909376836, 51.24890960531436690 ) ) ;
#121147=CARTESIAN_POINT ( 'NONE',  ( 10.81492255796106328, -18.62759615963255655, 60.41775706135235424 ) ) ;
#121148=CARTESIAN_POINT ( 'NONE',  ( 16.53943276465976808, -0.05219959533910856209, 93.74890960531436690 ) ) ;
#121149=CARTESIAN_POINT ( 'NONE',  ( 16.36317988757058828, -7.306389748694915198, 36.59789608363225710 ) ) ;
#121151=CARTESIAN_POINT ( 'NONE',  ( 10.72451020669898902, -18.67979575497178502, 32.91557627198102409 ) ) ;
#121153=CARTESIAN_POINT ( 'NONE',  ( -21.52544592524334988, -5.823673210054445271, 63.95942372801901854 ) ) ;
#121154=CARTESIAN_POINT ( 'NONE',  ( -17.60769864724391098, 5.499999999999987566, 43.65024842019164453 ) ) ;
#121155=CARTESIAN_POINT ( 'NONE',  ( 12.14591786802327356, -12.06949235617739191, 60.62609039468567573 ) ) ;
#121156=CARTESIAN_POINT ( 'NONE',  ( -4.483927247898539470, -16.52544592524342804, 47.29057627198103120 ) ) ;
#121157=CARTESIAN_POINT ( 'NONE',  ( 15.80617190586746368, 15.72974639402197994, 69.37390960531436690 ) ) ;
#121158=CARTESIAN_POINT ( 'NONE',  ( -10.81492255796078084, -18.62759615963271287, 57.08224293864769550 ) ) ;
#121160=CARTESIAN_POINT ( 'NONE',  ( 5.049401038297881783, 19.05341960407617563, 82.29275706135229029 ) ) ;
#121161=CARTESIAN_POINT ( 'NONE',  ( 16.46253265017160672, -9.564922557960803928, 103.3322429386476955 ) ) ;
#121163=CARTESIAN_POINT ( 'NONE',  ( -9.474510206698964154, 16.51473224551069663, 45.41557627198103120 ) ) ;
#121164=CARTESIAN_POINT ( 'NONE',  ( -12.14591786802309592, -12.06949235617757132, 111.8739096053143669 ) ) ;
#121165=CARTESIAN_POINT ( 'NONE',  ( 19.05341960407611168, 5.049401038298154454, 108.9572429386477097 ) ) ;
#121166=ORIENTED_EDGE ( 'NONE', *, *, #171652, .T. ) ;
#121167=CARTESIAN_POINT ( 'NONE',  ( -14.34966873604972548, 8.224510206698743886, 63.33442372801900433 ) ) ;
#121168=CARTESIAN_POINT ( 'NONE',  ( 18.67979575497178502, 10.72451020669898547, 104.1655762719810241 ) ) ;
#121169=CARTESIAN_POINT ( 'NONE',  ( 19.05341960407611168, 5.049401038298154454, 58.95724293864768129 ) ) ;
#121170=CARTESIAN_POINT ( 'NONE',  ( -5.823673210054431948, 21.52544592524334988, 47.70942372801902565 ) ) ;
#121171=CARTESIAN_POINT ( 'NONE',  ( 5.049401038298161559, -19.05341960407611168, 92.70724293864769550 ) ) ;
#121174=CARTESIAN_POINT ( 'NONE',  ( 5.719274019375673035, 21.55341960407619339, 37.29275706135235424 ) ) ;
#121175=CARTESIAN_POINT ( 'NONE',  ( 5.049401038298161559, -19.05341960407611168, 102.7072429386476955 ) ) ;
#121176=CARTESIAN_POINT ( 'NONE',  ( -13.89961937509957401, -13.97604488694547875, 84.37609039468567573 ) ) ;
#121177=CARTESIAN_POINT ( 'NONE',  ( -0.05219959533936034679, 19.03943276465977164, 37.50109039468567573 ) ) ;
#121178=CARTESIAN_POINT ( 'NONE',  ( 18.67979575497178502, 10.72451020669898547, 94.16557627198103830 ) ) ;
#121179=CARTESIAN_POINT ( 'NONE',  ( -13.89961937509957401, -13.97604488694547875, 29.37609039468565797 ) ) ;
#121180=CARTESIAN_POINT ( 'NONE',  ( -0.05219959533936034679, 19.03943276465977164, 37.50109039468567573 ) ) ;
#121181=CARTESIAN_POINT ( 'NONE',  ( 16.52544592524335698, 4.483927247898782831, 86.45942372801901854 ) ) ;
#121182=CARTESIAN_POINT ( 'NONE',  ( 5.153800228976335163, 19.02544592524342804, 114.7905762719810241 ) ) ;
#121183=CARTESIAN_POINT ( 'NONE',  ( -19.02544592524342804, 5.153800228976336051, 66.04057627198103830 ) ) ;
#121185=CARTESIAN_POINT ( 'NONE',  ( -21.55341960407619339, 5.719274019375674811, 63.54275706135234003 ) ) ;
#121186=CARTESIAN_POINT ( 'NONE',  ( -15.72974639402176322, -15.80617190586768395, 74.37609039468568994 ) ) ;
#121188=CARTESIAN_POINT ( 'NONE',  ( 5.153800228976335163, 19.02544592524342804, 89.79057627198102409 ) ) ;
#121189=CARTESIAN_POINT ( 'NONE',  ( 18.62759615963255655, 10.81492255796105972, 66.66775706135234714 ) ) ;
#121190=CARTESIAN_POINT ( 'NONE',  ( -13.89961937509957401, -13.97604488694547875, 104.3760903946856757 ) ) ;
#121191=CARTESIAN_POINT ( 'NONE',  ( -16.46253265017160317, 9.564922557960807481, 70.83224293864770971 ) ) ;
#121192=CARTESIAN_POINT ( 'NONE',  ( 16.46253265017160672, -9.564922557960803928, 113.3322429386476955 ) ) ;
#121193=CARTESIAN_POINT ( 'NONE',  ( 13.89961937509977652, -13.97604488694527269, 83.12390960531436690 ) ) ;
#121195=CARTESIAN_POINT ( 'NONE',  ( 9.564922557960805705, 16.46253265017160317, 69.58224293864770971 ) ) ;
#121196=CARTESIAN_POINT ( 'NONE',  ( -9.564922557960796823, -16.46253265017161027, 57.08224293864769550 ) ) ;
#121197=CARTESIAN_POINT ( 'NONE',  ( 5.823673210054125526, 21.52544592524343514, 94.79057627198105251 ) ) ;
#121198=CARTESIAN_POINT ( 'NONE',  ( 16.52544592524335698, 4.483927247898782831, 81.45942372801900433 ) ) ;
#121200=CARTESIAN_POINT ( 'NONE',  ( -19.05341960407617563, 5.049401038297882671, 43.54275706135232582 ) ) ;
#121201=CARTESIAN_POINT ( 'NONE',  ( -16.46253265017160317, 9.564922557960807481, 75.83224293864769550 ) ) ;
#121202=CARTESIAN_POINT ( 'NONE',  ( 12.14591786802309770, 12.06949235617756955, 74.37390960531436690 ) ) ;
#121203=CARTESIAN_POINT ( 'NONE',  ( 16.55341960407611168, 4.379528057220329451, 113.9572429386477239 ) ) ;
#121204=B_SPLINE_CURVE_WITH_KNOTS ( 'NONE', 3,
 ( #113043, #33240, #188923, #35217, #95891, #96870 ),
 .UNSPECIFIED., .F., .F.,
 ( 4, 2, 4 ),
 ( 0.007228050697041513671, 0.007608510107495006572, 0.007988969517948500340 ),
 .UNSPECIFIED. ) ;
#121205=CARTESIAN_POINT ( 'NONE',  ( 19.02544592524343514, -5.153800228976328945, 108.5405762719810383 ) ) ;
#121206=CARTESIAN_POINT ( 'NONE',  ( 9.564922557960805705, 16.46253265017160317, 109.5822429386476955 ) ) ;
#121207=CARTESIAN_POINT ( 'NONE',  ( 4.379528057220339221, -16.55341960407611168, 77.70724293864770971 ) ) ;
#121208=CARTESIAN_POINT ( 'NONE',  ( 18.22780087662123805, -5.499999999999976019, 83.51763182126896368 ) ) ;
#121209=CARTESIAN_POINT ( 'NONE',  ( 5.049401038297881783, 19.05341960407617563, 32.29275706135233293 ) ) ;
#121210=CARTESIAN_POINT ( 'NONE',  ( -16.53943276465976808, -0.05219959533934237506, 98.75109039468568994 ) ) ;
#121211=CARTESIAN_POINT ( 'NONE',  ( -5.153800228976328057, -19.02544592524343514, 77.29057627198099567 ) ) ;
#121212=EDGE_CURVE ( 'NONE', #15707, #144387, #198697, .T. ) ;
#121213=CARTESIAN_POINT ( 'NONE',  ( 5.823673210054444382, -21.52544592524334988, 50.20942372801901854 ) ) ;
#121214=CARTESIAN_POINT ( 'NONE',  ( 10.72451020669898902, -18.67979575497178502, 42.91557627198103120 ) ) ;
#121215=CARTESIAN_POINT ( 'NONE',  ( -15.80617190586768217, 15.72974639402176855, 23.12609039468567573 ) ) ;
#121216=CARTESIAN_POINT ( 'NONE',  ( 18.67979575497178502, 10.72451020669898547, 69.16557627198102409 ) ) ;
#121217=CARTESIAN_POINT ( 'NONE',  ( -4.483927247898539470, -16.52544592524342804, 97.29057627198105251 ) ) ;
#121218=CARTESIAN_POINT ( 'NONE',  ( 16.46253265017146816, 9.564922557961045513, 51.66775706135233293 ) ) ;
#121219=CARTESIAN_POINT ( 'NONE',  ( -16.51473224551069308, -9.474510206698971260, 31.66557627198102054 ) ) ;
#121220=CARTESIAN_POINT ( 'NONE',  ( 9.564922557960805705, 16.46253265017160317, 89.58224293864769550 ) ) ;
#121221=CARTESIAN_POINT ( 'NONE',  ( -16.46253265017160317, 9.564922557960807481, 75.83224293864769550 ) ) ;
#121222=CARTESIAN_POINT ( 'NONE',  ( -12.06949235617756955, 12.14591786802309770, 95.62390960531436690 ) ) ;
#121223=ORIENTED_EDGE ( 'NONE', *, *, #59834, .T. ) ;
#121224=CARTESIAN_POINT ( 'NONE',  ( 16.53943276465976808, -0.05219959533910856209, 23.74890960531435269 ) ) ;
#121225=CARTESIAN_POINT ( 'NONE',  ( 14.34966873604972726, -8.224510206698740333, 25.83442372801901499 ) ) ;
#121226=CARTESIAN_POINT ( 'NONE',  ( -15.72974639402176322, -15.80617190586768395, 94.37609039468568994 ) ) ;
#121227=CARTESIAN_POINT ( 'NONE',  ( 5.153800228976335163, 19.02544592524342804, 99.79057627198102409 ) ) ;
#121228=CARTESIAN_POINT ( 'NONE',  ( -21.52544592524343514, 5.823673210054127303, 116.0405762719810383 ) ) ;
#121229=CARTESIAN_POINT ( 'NONE',  ( 9.564922557960805705, 16.46253265017160317, 44.58224293864769550 ) ) ;
#121230=CARTESIAN_POINT ( 'NONE',  ( -4.483927247898782831, 16.52544592524335698, 42.70942372801901854 ) ) ;
#121231=CARTESIAN_POINT ( 'NONE',  ( 5.049401038297881783, 19.05341960407617563, 107.2927570613523187 ) ) ;
#121232=CARTESIAN_POINT ( 'NONE',  ( 19.05341960407611168, 5.049401038298154454, 33.95724293864769550 ) ) ;
#121233=CARTESIAN_POINT ( 'NONE',  ( -12.14591786802309592, -12.06949235617757132, 96.87390960531436690 ) ) ;
#121234=CARTESIAN_POINT ( 'NONE',  ( -15.80617190586745835, -15.72974639402198527, 101.8739096053143811 ) ) ;
#121235=CARTESIAN_POINT ( 'NONE',  ( -19.02544592524334988, -5.153800228976617603, 68.95942372801896170 ) ) ;
#121236=CARTESIAN_POINT ( 'NONE',  ( -0.05219959533907301413, -21.53943276465977519, 112.4989096053143669 ) ) ;
#121238=CARTESIAN_POINT ( 'NONE',  ( -5.049401038298153566, 19.05341960407611168, 95.20724293864770971 ) ) ;
#121239=CARTESIAN_POINT ( 'NONE',  ( 16.19135201231366494, -7.376712067591912003, 112.3131914594796825 ) ) ;
#121240=CARTESIAN_POINT ( 'NONE',  ( -19.05341960407611168, -5.049401038298163336, 91.45724293864766707 ) ) ;
#121241=CARTESIAN_POINT ( 'NONE',  ( 5.719274019375673035, 21.55341960407619339, 32.29275706135235424 ) ) ;
#121242=CARTESIAN_POINT ( 'NONE',  ( 16.52544592524342804, -4.483927247898539470, 83.54057627198102409 ) ) ;
#121243=CARTESIAN_POINT ( 'NONE',  ( 9.474510206698971260, -16.51473224551069308, 77.91557627198103830 ) ) ;
#121244=CARTESIAN_POINT ( 'NONE',  ( -5.049401038297874678, -19.05341960407617918, 24.79275706135233648 ) ) ;
#121245=CARTESIAN_POINT ( 'NONE',  ( -8.224510206698735004, -14.34966873604973081, 44.58442372801901854 ) ) ;
#121246=CARTESIAN_POINT ( 'NONE',  ( 19.05341960407617918, -5.049401038297876454, 61.04275706135232582 ) ) ;
#121247=CARTESIAN_POINT ( 'NONE',  ( -18.67979575497193778, 10.72451020669871902, 68.33442372801900433 ) ) ;
#121248=CARTESIAN_POINT ( 'NONE',  ( 12.14591786802327356, -12.06949235617739191, 20.62609039468568639 ) ) ;
#121249=CARTESIAN_POINT ( 'NONE',  ( -13.89961937509977652, 13.97604488694528158, 70.62390960531432427 ) ) ;
#121250=CARTESIAN_POINT ( 'NONE',  ( 16.46253265017146816, 9.564922557961045513, 101.6677570613523329 ) ) ;
#121251=CARTESIAN_POINT ( 'NONE',  ( 8.314922557961029526, -14.29746914071037800, 65.41775706135234714 ) ) ;
#121252=CARTESIAN_POINT ( 'NONE',  ( 19.05341960407617918, -5.049401038297876454, 21.04275706135232582 ) ) ;
#121253=CARTESIAN_POINT ( 'NONE',  ( -16.51473224551082808, 9.474510206698731452, 73.33442372801900433 ) ) ;
#121254=CARTESIAN_POINT ( 'NONE',  ( -13.89961937509977652, 13.97604488694528158, 50.62390960531435979 ) ) ;
#121255=CARTESIAN_POINT ( 'NONE',  ( 21.52544592524344225, -5.823673210054117533, 83.54057627198102409 ) ) ;
#121256=CARTESIAN_POINT ( 'NONE',  ( 16.55341960407611168, 4.379528057220329451, 73.95724293864769550 ) ) ;
#121257=CARTESIAN_POINT ( 'NONE',  ( 5.049401038297881783, 19.05341960407617563, 72.29275706135234714 ) ) ;
#121258=DIRECTION ( 'NONE',  ( -1.000000000000000000, 0.000000000000000000, -8.673617379884026597E-16 ) ) ;
#121259=CARTESIAN_POINT ( 'NONE',  ( -5.153800228976607833, 19.02544592524334988, 47.70942372801900433 ) ) ;
#121260=CARTESIAN_POINT ( 'NONE',  ( -8.314922557961024197, 14.29746914071037800, 107.9177570613523471 ) ) ;
#121261=CARTESIAN_POINT ( 'NONE',  ( 16.52544592524342804, -4.483927247898539470, 63.54057627198103830 ) ) ;
#121262=CARTESIAN_POINT ( 'NONE',  ( -5.823673210054431948, 21.52544592524334988, 102.7094237280190185 ) ) ;
#121264=CARTESIAN_POINT ( 'NONE',  ( -15.80617190586745835, -15.72974639402198527, 101.8739096053143811 ) ) ;
#121265=CARTESIAN_POINT ( 'NONE',  ( -5.049401038298153566, 19.05341960407611168, 60.20724293864768129 ) ) ;
#121266=CARTESIAN_POINT ( 'NONE',  ( 5.719274019375673035, 21.55341960407619339, 77.29275706135234714 ) ) ;
#121267=CARTESIAN_POINT ( 'NONE',  ( 9.564922557960805705, 16.46253265017160317, 69.58224293864770971 ) ) ;
#121269=CARTESIAN_POINT ( 'NONE',  ( 9.564922557960805705, 16.46253265017160317, 24.58224293864769194 ) ) ;
#121270=CARTESIAN_POINT ( 'NONE',  ( -18.67979575497178146, -10.72451020669898902, 36.66557627198103120 ) ) ;
#121271=CARTESIAN_POINT ( 'NONE',  ( 14.29746914071049879, -8.314922557960816363, 63.33224293864770260 ) ) ;
#121272=CARTESIAN_POINT ( 'NONE',  ( 13.97604488694527802, 13.89961937509977652, 49.37390960531434558 ) ) ;
#121273=CARTESIAN_POINT ( 'NONE',  ( -4.483927247898539470, -16.52544592524342804, 92.29057627198103830 ) ) ;
#121274=CARTESIAN_POINT ( 'NONE',  ( 15.72974639402199770, -15.80617190586745480, 113.1239096053143953 ) ) ;
#121275=CARTESIAN_POINT ( 'NONE',  ( 10.81492255796106328, -18.62759615963255655, 55.41775706135234714 ) ) ;
#121276=CARTESIAN_POINT ( 'NONE',  ( -5.153800228976328057, -19.02544592524343514, 32.29057627198102409 ) ) ;
#121278=CARTESIAN_POINT ( 'NONE',  ( -16.53943276465976808, -0.05219959533934237506, 63.75109039468568284 ) ) ;
#121279=CARTESIAN_POINT ( 'NONE',  ( -10.81492255796078084, -18.62759615963271287, 107.0822429386476955 ) ) ;
#121280=CARTESIAN_POINT ( 'NONE',  ( 10.72451020669898902, -18.67979575497178502, 97.91557627198103830 ) ) ;
#121281=CARTESIAN_POINT ( 'NONE',  ( 9.564922557961047289, -16.46253265017146816, 20.41775706135233293 ) ) ;
#121282=CARTESIAN_POINT ( 'NONE',  ( 13.89961937509977652, -13.97604488694527269, 58.12390960531436690 ) ) ;
#121283=CARTESIAN_POINT ( 'NONE',  ( 9.474510206698971260, -16.51473224551069308, 102.9155762719810241 ) ) ;
#121284=CARTESIAN_POINT ( 'NONE',  ( 21.55341960407619695, -5.719274019375665929, 61.04275706135234714 ) ) ;
#121285=CARTESIAN_POINT ( 'NONE',  ( -21.52544592524343514, 5.823673210054127303, 41.04057627198103120 ) ) ;
#121286=CARTESIAN_POINT ( 'NONE',  ( -14.34966873604972548, 8.224510206698743886, 113.3344237280190328 ) ) ;
#121287=CARTESIAN_POINT ( 'NONE',  ( -18.62759615963255300, -10.81492255796106328, 59.16775706135234714 ) ) ;
#121288=CARTESIAN_POINT ( 'NONE',  ( 21.52544592524334988, 5.823673210054432836, 96.45942372801901854 ) ) ;
#121289=CARTESIAN_POINT ( 'NONE',  ( -19.02544592524334988, -5.153800228976617603, 48.95942372801900433 ) ) ;
#121290=CARTESIAN_POINT ( 'NONE',  ( -12.06949235617739369, -12.14591786802326823, 104.3760903946856899 ) ) ;
#121291=CARTESIAN_POINT ( 'NONE',  ( -10.72451020669870658, -18.67979575497194134, 49.58442372801901143 ) ) ;
#121292=CARTESIAN_POINT ( 'NONE',  ( 16.51473224551069308, 9.474510206698969483, 64.16557627198102409 ) ) ;
#121293=CARTESIAN_POINT ( 'NONE',  ( -9.474510206698720793, -16.51473224551083518, 19.58442372801899722 ) ) ;
#121294=CARTESIAN_POINT ( 'NONE',  ( 18.62759615963271287, -10.81492255796078972, 33.33224293864769550 ) ) ;
#121296=CARTESIAN_POINT ( 'NONE',  ( 5.823673210054444382, -21.52544592524334988, 30.20942372801902565 ) ) ;
#121297=CARTESIAN_POINT ( 'NONE',  ( -18.62759615963270932, 10.81492255796079327, 90.83224293864769550 ) ) ;
#121298=CARTESIAN_POINT ( 'NONE',  ( 5.049401038297881783, 19.05341960407617563, 87.29275706135234714 ) ) ;
#121299=CARTESIAN_POINT ( 'NONE',  ( 16.52544592524335698, 4.483927247898782831, 41.45942372801901143 ) ) ;
#121301=CARTESIAN_POINT ( 'NONE',  ( -10.81492255796078084, -18.62759615963271287, 77.08224293864769550 ) ) ;
#121302=CARTESIAN_POINT ( 'NONE',  ( -16.53943276465976808, -0.05219959533934237506, 63.75109039468568284 ) ) ;
#121303=CARTESIAN_POINT ( 'NONE',  ( 16.53943276465976808, -0.05219959533910856209, 78.74890960531436690 ) ) ;
#121305=CARTESIAN_POINT ( 'NONE',  ( 0.05219959533936267826, -19.03943276465977164, 105.0010903946856615 ) ) ;
#121306=CARTESIAN_POINT ( 'NONE',  ( 5.823673210054125526, 21.52544592524343514, 39.79057627198103830 ) ) ;
#121307=CARTESIAN_POINT ( 'NONE',  ( 9.564922557960805705, 16.46253265017160317, 94.58224293864769550 ) ) ;
#121308=CARTESIAN_POINT ( 'NONE',  ( -12.14591786802326823, 12.06949235617739902, 38.12609039468567573 ) ) ;
#121309=CARTESIAN_POINT ( 'NONE',  ( -5.823673210054116645, -21.52544592524344225, 107.2905762719810525 ) ) ;
#121310=CARTESIAN_POINT ( 'NONE',  ( 21.55341960407610458, 5.719274019375980345, 33.95724293864769550 ) ) ;
#121311=CARTESIAN_POINT ( 'NONE',  ( 12.14591786802327356, -12.06949235617739191, 65.62609039468568994 ) ) ;
#121312=CARTESIAN_POINT ( 'NONE',  ( 16.46253265017160672, -9.564922557960803928, 83.33224293864768129 ) ) ;
#121313=CARTESIAN_POINT ( 'NONE',  ( 5.823673210054444382, -21.52544592524334988, 55.20942372801902565 ) ) ;
#121314=CARTESIAN_POINT ( 'NONE',  ( 5.153800228976335163, 19.02544592524342804, 34.79057627198102409 ) ) ;
#121315=CARTESIAN_POINT ( 'NONE',  ( -19.02544592524342804, 5.153800228976336051, 116.0405762719810383 ) ) ;
#121317=CARTESIAN_POINT ( 'NONE',  ( -16.46253265017146816, -9.564922557961047289, 44.16775706135232582 ) ) ;
#121318=CARTESIAN_POINT ( 'NONE',  ( 16.53943276465976808, 0.05219959533934440121, 46.25109039468567573 ) ) ;
#121319=CARTESIAN_POINT ( 'NONE',  ( -13.89961937509977652, 13.97604488694528158, 110.6239096053143243 ) ) ;
#121320=CARTESIAN_POINT ( 'NONE',  ( -13.89961937509977652, 13.97604488694528158, 75.62390960531438111 ) ) ;
#121321=CARTESIAN_POINT ( 'NONE',  ( -4.379528057220086978, -16.55341960407618274, 94.79275706135234714 ) ) ;
#121323=CARTESIAN_POINT ( 'NONE',  ( 12.06949235617757843, -12.14591786802309237, 93.12390960531436690 ) ) ;
#121324=CARTESIAN_POINT ( 'NONE',  ( 21.52544592524344225, -5.823673210054117533, 28.54057627198103120 ) ) ;
#121325=CARTESIAN_POINT ( 'NONE',  ( -19.02544592524342804, 5.153800228976336051, 26.04057627198103120 ) ) ;
#121326=CARTESIAN_POINT ( 'NONE',  ( 12.06949235617739724, 12.14591786802326823, 61.87609039468568284 ) ) ;
#121327=CARTESIAN_POINT ( 'NONE',  ( 21.53943276465977519, 0.05219959533937863772, 21.25109039468567218 ) ) ;
#121328=CARTESIAN_POINT ( 'NONE',  ( -19.02544592524334988, -5.153800228976617603, 73.95942372801900433 ) ) ;
#121329=CARTESIAN_POINT ( 'NONE',  ( -13.89961937509977652, 13.97604488694528158, 40.62390960531435979 ) ) ;
#121330=CARTESIAN_POINT ( 'NONE',  ( -21.55341960407610458, -5.719274019375992779, 66.45724293864768129 ) ) ;
#121331=CARTESIAN_POINT ( 'NONE',  ( 16.51473224551069308, 9.474510206698969483, 114.1655762719810241 ) ) ;
#121332=CARTESIAN_POINT ( 'NONE',  ( 21.52544592524334988, 5.823673210054432836, 96.45942372801901854 ) ) ;
#121333=CARTESIAN_POINT ( 'NONE',  ( 0.05219959533909260263, 19.03943276465977164, 59.99890960531436690 ) ) ;
#121334=CARTESIAN_POINT ( 'NONE',  ( 16.53943276465976808, 0.05219959533934440121, 46.25109039468567573 ) ) ;
#121335=CARTESIAN_POINT ( 'NONE',  ( -13.97604488694527625, -13.89961937509977652, 61.87390960531435979 ) ) ;
#121336=CARTESIAN_POINT ( 'NONE',  ( -18.67979575497193778, 10.72451020669871902, 78.33442372801901854 ) ) ;
#121337=CARTESIAN_POINT ( 'NONE',  ( -13.89961937509957401, -13.97604488694547875, 34.37609039468566863 ) ) ;
#121338=CARTESIAN_POINT ( 'NONE',  ( -19.02544592524334988, -5.153800228976617603, 48.95942372801900433 ) ) ;
#121339=CARTESIAN_POINT ( 'NONE',  ( -18.62759615963255300, -10.81492255796106328, 54.16775706135235424 ) ) ;
#121341=CARTESIAN_POINT ( 'NONE',  ( 19.03943276465977164, 0.05219959533936151252, 51.25109039468567573 ) ) ;
#121342=CARTESIAN_POINT ( 'NONE',  ( 0.05219959533909260263, 19.03943276465977164, 99.99890960531436690 ) ) ;
#121343=CARTESIAN_POINT ( 'NONE',  ( 19.02544592524343514, -5.153800228976328945, 88.54057627198102409 ) ) ;
#121344=CARTESIAN_POINT ( 'NONE',  ( 16.55341960407611168, 4.379528057220329451, 33.95724293864769550 ) ) ;
#121345=CARTESIAN_POINT ( 'NONE',  ( 10.81492255796078972, 18.62759615963270932, 34.58224293864770260 ) ) ;
#121346=CARTESIAN_POINT ( 'NONE',  ( 5.823673210054444382, -21.52544592524334988, 100.2094237280190043 ) ) ;
#121348=CARTESIAN_POINT ( 'NONE',  ( 17.05116617787827238, 6.768360034955700044, 58.84324446740803438 ) ) ;
#121349=CARTESIAN_POINT ( 'NONE',  ( 21.55341960407619695, -5.719274019375665929, 101.0427570613523756 ) ) ;
#121351=CARTESIAN_POINT ( 'NONE',  ( -19.05341960407611168, -5.049401038298163336, 41.45724293864769550 ) ) ;
#121352=CARTESIAN_POINT ( 'NONE',  ( 5.049401038298161559, -19.05341960407611168, 112.7072429386476813 ) ) ;
#121354=CARTESIAN_POINT ( 'NONE',  ( 4.483927247898790824, -16.52544592524335698, 45.20942372801901854 ) ) ;
#121355=CARTESIAN_POINT ( 'NONE',  ( 15.72974639402199770, -15.80617190586745480, 68.12390960531436690 ) ) ;
#121356=CARTESIAN_POINT ( 'NONE',  ( 16.52544592524342804, -4.483927247898539470, 33.54057627198102409 ) ) ;
#121357=CARTESIAN_POINT ( 'NONE',  ( 5.153800228976335163, 19.02544592524342804, 29.79057627198102409 ) ) ;
#121358=CARTESIAN_POINT ( 'NONE',  ( -5.153800228976328057, -19.02544592524343514, 107.2905762719810383 ) ) ;
#121359=CARTESIAN_POINT ( 'NONE',  ( -21.55341960407619339, 5.719274019375674811, 23.54275706135235424 ) ) ;
#121360=CARTESIAN_POINT ( 'NONE',  ( 0.05219959533936267826, -19.03943276465977164, 35.00109039468566863 ) ) ;
#121361=CARTESIAN_POINT ( 'NONE',  ( 12.14591786802309770, 12.06949235617756955, 109.3739096053143811 ) ) ;
#121362=CARTESIAN_POINT ( 'NONE',  ( -15.80617190586768217, 15.72974639402176855, 63.12609039468568994 ) ) ;
#121363=CARTESIAN_POINT ( 'NONE',  ( 17.12812012977025589, -6.668231424566045007, 31.14051240676858967 ) ) ;
#121364=CARTESIAN_POINT ( 'NONE',  ( -12.06949235617756955, 12.14591786802309770, 25.62390960531435624 ) ) ;
#121365=CARTESIAN_POINT ( 'NONE',  ( -18.22780087662122028, 5.500000000000031086, 68.51540105326107266 ) ) ;
#121366=CARTESIAN_POINT ( 'NONE',  ( -5.823673210054116645, -21.52544592524344225, 32.29057627198102409 ) ) ;
#121367=CARTESIAN_POINT ( 'NONE',  ( 8.314922557960818139, 14.29746914071049879, 84.58224293864769550 ) ) ;
#121370=CARTESIAN_POINT ( 'NONE',  ( 16.46253265017160672, -9.564922557960803928, 73.33224293864769550 ) ) ;
#121371=CARTESIAN_POINT ( 'NONE',  ( -14.29746914071049879, 8.314922557960819915, 75.83224293864769550 ) ) ;
#121372=CARTESIAN_POINT ( 'NONE',  ( -16.51473224551082808, 9.474510206698731452, 108.3344237280190043 ) ) ;
#121373=CARTESIAN_POINT ( 'NONE',  ( -18.62759615963270932, 10.81492255796079327, 65.83224293864769550 ) ) ;
#121375=CARTESIAN_POINT ( 'NONE',  ( 16.51473224551069308, 9.474510206698969483, 24.16557627198102765 ) ) ;
#121376=EDGE_CURVE ( 'NONE', #40349, #132603, #87121, .T. ) ;
#121377=CARTESIAN_POINT ( 'NONE',  ( 0.05219959533909260263, 19.03943276465977164, 74.99890960531435269 ) ) ;
#121378=CARTESIAN_POINT ( 'NONE',  ( -10.72451020669898014, 18.67979575497178502, 75.41557627198102409 ) ) ;
#121379=CARTESIAN_POINT ( 'NONE',  ( 16.55341960407618274, -4.379528057220086978, 101.0427570613523756 ) ) ;
#121380=CARTESIAN_POINT ( 'NONE',  ( 16.46253265017160672, -9.564922557960803928, 93.33224293864769550 ) ) ;
#121381=CARTESIAN_POINT ( 'NONE',  ( 16.51473224551083163, -9.474510206698727899, 60.83442372801900433 ) ) ;
#121382=CARTESIAN_POINT ( 'NONE',  ( 21.52544592524334988, 5.823673210054432836, 101.4594237280190185 ) ) ;
#121383=CARTESIAN_POINT ( 'NONE',  ( -15.72974639402197994, 15.80617190586746368, 70.62390960531436690 ) ) ;
#121384=CARTESIAN_POINT ( 'NONE',  ( 13.97604488694527802, 13.89961937509977652, 114.3739096053143669 ) ) ;
#121385=CARTESIAN_POINT ( 'NONE',  ( 13.97604488694527802, 13.89961937509977652, 44.37390960531435269 ) ) ;
#121386=CARTESIAN_POINT ( 'NONE',  ( -12.06949235617739369, -12.14591786802326823, 94.37609039468568994 ) ) ;
#121387=CARTESIAN_POINT ( 'NONE',  ( -19.03943276465977164, 0.05219959533909376836, 66.24890960531436690 ) ) ;
#121388=CARTESIAN_POINT ( 'NONE',  ( 8.224510206698742110, 14.34966873604972548, 27.08442372801901854 ) ) ;
#121389=CARTESIAN_POINT ( 'NONE',  ( 17.05587630539785238, 6.762274262135711034, 51.75819690962690345 ) ) ;
#121390=CARTESIAN_POINT ( 'NONE',  ( 10.72451020669871369, 18.67979575497193778, 112.0844237280190185 ) ) ;
#121391=CARTESIAN_POINT ( 'NONE',  ( 8.314922557960818139, 14.29746914071049879, 74.58224293864768129 ) ) ;
#121392=CARTESIAN_POINT ( 'NONE',  ( 15.72974639402199770, -15.80617190586745480, 113.1239096053143953 ) ) ;
#121393=CARTESIAN_POINT ( 'NONE',  ( -0.05219959533907301413, -21.53943276465977519, 97.49890960531436690 ) ) ;
#121395=CARTESIAN_POINT ( 'NONE',  ( 21.53943276465977519, -0.05219959533907433946, 58.74890960531436690 ) ) ;
#121396=CARTESIAN_POINT ( 'NONE',  ( -14.34966873604972548, 8.224510206698743886, 78.33442372801901854 ) ) ;
#121397=CARTESIAN_POINT ( 'NONE',  ( 8.224510206698953496, -14.34966873604960469, 102.9155762719810383 ) ) ;
#121398=CARTESIAN_POINT ( 'NONE',  ( -0.05219959533909027116, -19.03943276465977164, 62.49890960531435979 ) ) ;
#121399=CARTESIAN_POINT ( 'NONE',  ( -8.224510206698735004, -14.34966873604973081, 109.5844237280190328 ) ) ;
#121400=CARTESIAN_POINT ( 'NONE',  ( 21.55341960407619695, -5.719274019375665929, 51.04275706135234714 ) ) ;
#121401=CARTESIAN_POINT ( 'NONE',  ( -9.474510206698964154, 16.51473224551069663, 95.41557627198102409 ) ) ;
#121402=CARTESIAN_POINT ( 'NONE',  ( -10.81492255796105439, 18.62759615963255655, 82.91775706135234714 ) ) ;
#121403=CARTESIAN_POINT ( 'NONE',  ( 0.05219959533909260263, 19.03943276465977164, 29.99890960531435979 ) ) ;
#121404=CARTESIAN_POINT ( 'NONE',  ( -9.474510206698964154, 16.51473224551069663, 40.41557627198103120 ) ) ;
#121405=ORIENTED_EDGE ( 'NONE', *, *, #76155, .T. ) ;
#121406=CARTESIAN_POINT ( 'NONE',  ( -18.62759615963255300, -10.81492255796106328, 74.16775706135231871 ) ) ;
#121407=CARTESIAN_POINT ( 'NONE',  ( 13.89961937509977652, -13.97604488694527269, 108.1239096053143669 ) ) ;
#121408=CARTESIAN_POINT ( 'NONE',  ( 0.05219959533936267826, -19.03943276465977164, 85.00109039468567573 ) ) ;
#121409=CARTESIAN_POINT ( 'NONE',  ( -21.53943276465977519, -0.05219959533937600094, 38.75109039468567573 ) ) ;
#121410=CARTESIAN_POINT ( 'NONE',  ( -16.53943276465976808, -0.05219959533934237506, 18.75109039468568639 ) ) ;
#121412=CARTESIAN_POINT ( 'NONE',  ( -19.05341960407617563, 5.049401038297882671, 68.54275706135230450 ) ) ;
#121413=CARTESIAN_POINT ( 'NONE',  ( -19.03943276465977164, 0.05219959533909376836, 51.24890960531436690 ) ) ;
#121414=CARTESIAN_POINT ( 'NONE',  ( 16.51473224551083163, -9.474510206698727899, 85.83442372801900433 ) ) ;
#121416=CARTESIAN_POINT ( 'NONE',  ( -12.14591786802309592, -12.06949235617757132, 31.87390960531435979 ) ) ;
#121417=CARTESIAN_POINT ( 'NONE',  ( -5.049401038297874678, -19.05341960407617918, 84.79275706135233293 ) ) ;
#121418=CARTESIAN_POINT ( 'NONE',  ( -8.224510206698948167, 14.34966873604960824, 35.41557627198102409 ) ) ;
#121419=CARTESIAN_POINT ( 'NONE',  ( -0.05219959533936034679, 19.03943276465977164, 57.50109039468566863 ) ) ;
#121420=CARTESIAN_POINT ( 'NONE',  ( -14.34966873604972548, 8.224510206698743886, 43.33442372801901143 ) ) ;
#121421=CARTESIAN_POINT ( 'NONE',  ( -13.89961937509957401, -13.97604488694547875, 24.37609039468565442 ) ) ;
#121422=CARTESIAN_POINT ( 'NONE',  ( -13.89961937509977652, 13.97604488694528158, 30.62390960531435269 ) ) ;
#121423=CARTESIAN_POINT ( 'NONE',  ( -16.36317988757057762, -7.306389748694952502, 65.90210391636775000 ) ) ;
#121424=CARTESIAN_POINT ( 'NONE',  ( -16.55341960407617563, 4.379528057220093196, 43.54275706135235424 ) ) ;
#121426=CARTESIAN_POINT ( 'NONE',  ( -0.05219959533909027116, -19.03943276465977164, 92.49890960531436690 ) ) ;
#121427=CARTESIAN_POINT ( 'NONE',  ( -17.60691670004653631, -5.500000000000000000, 69.13333313366437949 ) ) ;
#121429=CARTESIAN_POINT ( 'NONE',  ( -16.46253265017146816, -9.564922557961047289, 89.16775706135234714 ) ) ;
#121430=CARTESIAN_POINT ( 'NONE',  ( -5.719274019375978568, 21.55341960407610458, 25.20724293864769550 ) ) ;
#121431=CARTESIAN_POINT ( 'NONE',  ( 0.05219959533936267826, -19.03943276465977164, 20.00109039468567218 ) ) ;
#121432=CARTESIAN_POINT ( 'NONE',  ( 9.474510206698729675, 16.51473224551082808, 102.0844237280190043 ) ) ;
#121433=CARTESIAN_POINT ( 'NONE',  ( -4.379528057220328563, 16.55341960407611168, 110.2072429386477239 ) ) ;
#121434=CARTESIAN_POINT ( 'NONE',  ( -16.46253265017160317, 9.564922557960807481, 35.83224293864768839 ) ) ;
#121435=CARTESIAN_POINT ( 'NONE',  ( 18.62759615963271287, -10.81492255796078972, 63.33224293864770260 ) ) ;
#121436=CARTESIAN_POINT ( 'NONE',  ( -8.224510206698948167, 14.34966873604960824, 115.4155762719810241 ) ) ;
#121438=CARTESIAN_POINT ( 'NONE',  ( -5.153800228976607833, 19.02544592524334988, 72.70942372801900433 ) ) ;
#121439=CARTESIAN_POINT ( 'NONE',  ( 12.06949235617757843, -12.14591786802309237, 43.12390960531435269 ) ) ;
#121440=CARTESIAN_POINT ( 'NONE',  ( -16.46253265017160317, 9.564922557960807481, 115.8322429386477097 ) ) ;
#121442=CARTESIAN_POINT ( 'NONE',  ( -5.823673210054431948, 21.52544592524334988, 92.70942372801901854 ) ) ;
#121443=CARTESIAN_POINT ( 'NONE',  ( 15.72974639402199770, -15.80617190586745480, 83.12390960531436690 ) ) ;
#121444=CARTESIAN_POINT ( 'NONE',  ( 21.55341960407619695, -5.719274019375665929, 56.04275706135235424 ) ) ;
#121445=CARTESIAN_POINT ( 'NONE',  ( -0.05219959533937732626, 21.53943276465977519, 62.50109039468568284 ) ) ;
#121446=CARTESIAN_POINT ( 'NONE',  ( 16.46253265017160672, -9.564922557960803928, 93.33224293864769550 ) ) ;
#121447=CARTESIAN_POINT ( 'NONE',  ( 4.379528057220092307, 16.55341960407617563, 97.29275706135234714 ) ) ;
#121448=CARTESIAN_POINT ( 'NONE',  ( -5.719274019375665041, -21.55341960407619695, 54.79275706135235424 ) ) ;
#121449=CARTESIAN_POINT ( 'NONE',  ( 16.52544592524342804, -4.483927247898539470, 113.5405762719810383 ) ) ;
#121450=CARTESIAN_POINT ( 'NONE',  ( 16.52544592524342804, -4.483927247898539470, 73.54057627198102409 ) ) ;
#121451=CARTESIAN_POINT ( 'NONE',  ( -16.55341960407611168, -4.379528057220339221, 31.45724293864769550 ) ) ;
#121452=CARTESIAN_POINT ( 'NONE',  ( 21.55341960407610458, 5.719274019375980345, 48.95724293864770971 ) ) ;
#121453=CARTESIAN_POINT ( 'NONE',  ( -9.564922557960796823, -16.46253265017161027, 62.08224293864769550 ) ) ;
#121454=CARTESIAN_POINT ( 'NONE',  ( -13.97604488694527625, -13.89961937509977652, 46.87390960531435979 ) ) ;
#121455=CARTESIAN_POINT ( 'NONE',  ( 0.05219959533907565091, 21.53943276465977519, 59.99890960531436690 ) ) ;
#121456=CARTESIAN_POINT ( 'NONE',  ( -16.51473224551082808, 9.474510206698731452, 48.33442372801900433 ) ) ;
#121457=CARTESIAN_POINT ( 'NONE',  ( -16.29526858892878494, -7.335722546919999587, 40.79670597800206622 ) ) ;
#121458=CARTESIAN_POINT ( 'NONE',  ( -14.29746914071049879, 8.314922557960819915, 55.83224293864770260 ) ) ;
#121459=CARTESIAN_POINT ( 'NONE',  ( -13.89961937509977652, 13.97604488694528158, 115.6239096053143669 ) ) ;
#121463=CARTESIAN_POINT ( 'NONE',  ( -0.05219959533934338120, 16.53943276465976808, 72.50109039468568994 ) ) ;
#121464=CARTESIAN_POINT ( 'NONE',  ( 19.02544592524334988, 5.153800228976608722, 81.45942372801897591 ) ) ;
#121466=CARTESIAN_POINT ( 'NONE',  ( 0.05219959533910956823, 16.53943276465976808, 39.99890960531436690 ) ) ;
#121468=CARTESIAN_POINT ( 'NONE',  ( -14.34966873604960291, -8.224510206698953496, 21.66557627198102409 ) ) ;
#121469=CARTESIAN_POINT ( 'NONE',  ( -5.153800228976328057, -19.02544592524343514, 47.29057627198102409 ) ) ;
#121470=CARTESIAN_POINT ( 'NONE',  ( -9.474510206698964154, 16.51473224551069663, 80.41557627198103830 ) ) ;
#121471=CARTESIAN_POINT ( 'NONE',  ( 13.89961937509977652, -13.97604488694527269, 33.12390960531434558 ) ) ;
#121472=CARTESIAN_POINT ( 'NONE',  ( -5.823673210054431948, 21.52544592524334988, 47.70942372801902565 ) ) ;
#121473=CARTESIAN_POINT ( 'NONE',  ( 19.05341960407611168, 5.049401038298154454, 58.95724293864768129 ) ) ;
#121475=CARTESIAN_POINT ( 'NONE',  ( -5.049401038298153566, 19.05341960407611168, 55.20724293864769550 ) ) ;
#121476=CARTESIAN_POINT ( 'NONE',  ( -18.62759615963270932, 10.81492255796079327, 40.83224293864769550 ) ) ;
#121477=CARTESIAN_POINT ( 'NONE',  ( -4.379528057220328563, 16.55341960407611168, 115.2072429386476955 ) ) ;
#121478=CARTESIAN_POINT ( 'NONE',  ( -0.05219959533907301413, -21.53943276465977519, 47.49890960531435979 ) ) ;
#121479=CARTESIAN_POINT ( 'NONE',  ( 16.52544592524335698, 4.483927247898782831, 86.45942372801901854 ) ) ;
#121480=CARTESIAN_POINT ( 'NONE',  ( -5.823673210054431948, 21.52544592524334988, 107.7094237280190328 ) ) ;
#121481=CARTESIAN_POINT ( 'NONE',  ( 16.53943276465976808, 0.05219959533934440121, 71.25109039468568994 ) ) ;
#121482=CARTESIAN_POINT ( 'NONE',  ( 19.05341960407611168, 5.049401038298154454, 113.9572429386477097 ) ) ;
#121483=CARTESIAN_POINT ( 'NONE',  ( 12.06949235617739724, 12.14591786802326823, 56.87609039468568994 ) ) ;
#121484=CARTESIAN_POINT ( 'NONE',  ( 0.05219959533934541429, -16.53943276465976808, 35.00109039468568284 ) ) ;
#121485=CARTESIAN_POINT ( 'NONE',  ( 5.153800228976335163, 19.02544592524342804, 114.7905762719810241 ) ) ;
#121486=CARTESIAN_POINT ( 'NONE',  ( -14.29746914071037622, -8.314922557961029526, 19.16775706135234714 ) ) ;
#121487=CARTESIAN_POINT ( 'NONE',  ( 9.564922557960805705, 16.46253265017160317, 34.58224293864770260 ) ) ;
#121488=CARTESIAN_POINT ( 'NONE',  ( -5.823673210054431948, 21.52544592524334988, 22.70942372801901499 ) ) ;
#121489=CARTESIAN_POINT ( 'NONE',  ( -5.153800228976607833, 19.02544592524334988, 112.7094237280190043 ) ) ;
#121490=CARTESIAN_POINT ( 'NONE',  ( -14.34966873604972548, 8.224510206698743886, 88.33442372801901854 ) ) ;
#121492=CARTESIAN_POINT ( 'NONE',  ( -21.52544592524334988, -5.823673210054445271, 83.95942372801900433 ) ) ;
#121493=CARTESIAN_POINT ( 'NONE',  ( 16.51473224551083163, -9.474510206698727899, 90.83442372801900433 ) ) ;
#121494=CARTESIAN_POINT ( 'NONE',  ( 8.224510206698953496, -14.34966873604960469, 57.91557627198103120 ) ) ;
#121495=CARTESIAN_POINT ( 'NONE',  ( -8.224510206698948167, 14.34966873604960824, 110.4155762719810383 ) ) ;
#121496=CARTESIAN_POINT ( 'NONE',  ( -16.51473224551082808, 9.474510206698731452, 48.33442372801900433 ) ) ;
#121498=CARTESIAN_POINT ( 'NONE',  ( -5.823673210054431948, 21.52544592524334988, 47.70942372801902565 ) ) ;
#121499=CARTESIAN_POINT ( 'NONE',  ( -19.03943276465977164, -0.05219959533935918106, 108.7510903946856615 ) ) ;
#121500=CARTESIAN_POINT ( 'NONE',  ( 16.79531203550644491, 7.028104445595627858, 83.75244988220441655 ) ) ;
#121501=CARTESIAN_POINT ( 'NONE',  ( 9.564922557960805705, 16.46253265017160317, 104.5822429386476955 ) ) ;
#121502=CARTESIAN_POINT ( 'NONE',  ( -21.53943276465977519, 0.05219959533907696930, 66.24890960531436690 ) ) ;
#121503=CARTESIAN_POINT ( 'NONE',  ( 16.51473224551083163, -9.474510206698727899, 100.8344237280190043 ) ) ;
#121504=CARTESIAN_POINT ( 'NONE',  ( -5.153800228976328057, -19.02544592524343514, 107.2905762719810383 ) ) ;
#121506=CARTESIAN_POINT ( 'NONE',  ( -12.14591786802309592, -12.06949235617757132, 106.8739096053143811 ) ) ;
#121507=CARTESIAN_POINT ( 'NONE',  ( -5.823673210054431948, 21.52544592524334988, 87.70942372801901854 ) ) ;
#121508=CARTESIAN_POINT ( 'NONE',  ( -19.05341960407611168, -5.049401038298163336, 46.45724293864768129 ) ) ;
#121509=CARTESIAN_POINT ( 'NONE',  ( -21.55341960407619339, 5.719274019375674811, 58.54275706135235424 ) ) ;
#121510=CARTESIAN_POINT ( 'NONE',  ( -10.72451020669870658, -18.67979575497194134, 89.58442372801901854 ) ) ;
#121511=CARTESIAN_POINT ( 'NONE',  ( -14.29746914071037622, -8.314922557961029526, 109.1677570613523613 ) ) ;
#121512=CARTESIAN_POINT ( 'NONE',  ( 19.05341960407611168, 5.049401038298154454, 63.95724293864769550 ) ) ;
#121513=CARTESIAN_POINT ( 'NONE',  ( -5.823673210054431948, 21.52544592524334988, 37.70942372801900433 ) ) ;
#121514=CARTESIAN_POINT ( 'NONE',  ( -21.52544592524334988, -5.823673210054445271, 38.95942372801901854 ) ) ;
#121515=CARTESIAN_POINT ( 'NONE',  ( 16.46253265017146816, 9.564922557961045513, 66.66775706135233293 ) ) ;
#121516=CARTESIAN_POINT ( 'NONE',  ( -13.97604488694527625, -13.89961937509977652, 96.87390960531433848 ) ) ;
#121517=CARTESIAN_POINT ( 'NONE',  ( -12.06949235617756955, 12.14591786802309770, 110.6239096053143669 ) ) ;
#121518=CARTESIAN_POINT ( 'NONE',  ( 5.719274019375991003, -21.55341960407610458, 92.70724293864770971 ) ) ;
#121519=CARTESIAN_POINT ( 'NONE',  ( 8.314922557960818139, 14.29746914071049879, 64.58224293864769550 ) ) ;
#121520=CARTESIAN_POINT ( 'NONE',  ( 10.81492255796106328, -18.62759615963255655, 110.4177570613523756 ) ) ;
#121521=CARTESIAN_POINT ( 'NONE',  ( -4.483927247898539470, -16.52544592524342804, 87.29057627198103830 ) ) ;
#121522=CARTESIAN_POINT ( 'NONE',  ( -9.474510206698964154, 16.51473224551069663, 40.41557627198103120 ) ) ;
#121523=CARTESIAN_POINT ( 'NONE',  ( 19.02544592524334988, 5.153800228976608722, 86.45942372801900433 ) ) ;
#121524=CARTESIAN_POINT ( 'NONE',  ( 16.55341960407611168, 4.379528057220329451, 48.95724293864770971 ) ) ;
#121525=CARTESIAN_POINT ( 'NONE',  ( -18.62759615963255300, -10.81492255796106328, 99.16775706135234714 ) ) ;
#121526=CARTESIAN_POINT ( 'NONE',  ( 9.564922557960805705, 16.46253265017160317, 89.58224293864769550 ) ) ;
#121527=CARTESIAN_POINT ( 'NONE',  ( -16.51473224551082808, 9.474510206698731452, 73.33442372801900433 ) ) ;
#121528=CARTESIAN_POINT ( 'NONE',  ( 15.72974639402199770, -15.80617190586745480, 83.12390960531436690 ) ) ;
#121529=CARTESIAN_POINT ( 'NONE',  ( 0.05219959533937995610, -21.53943276465977519, 25.00109039468567218 ) ) ;
#121530=CARTESIAN_POINT ( 'NONE',  ( 8.314922557961029526, -14.29746914071037800, 35.41775706135234003 ) ) ;
#121531=CARTESIAN_POINT ( 'NONE',  ( -16.55341960407617563, 4.379528057220093196, 88.54275706135236135 ) ) ;
#121532=CARTESIAN_POINT ( 'NONE',  ( 0.05219959533909260263, 19.03943276465977164, 29.99890960531435979 ) ) ;
#121533=CARTESIAN_POINT ( 'NONE',  ( -18.62759615963255300, -10.81492255796106328, 24.16775706135235424 ) ) ;
#121534=CARTESIAN_POINT ( 'NONE',  ( -9.474510206698964154, 16.51473224551069663, 25.41557627198103120 ) ) ;
#121536=CARTESIAN_POINT ( 'NONE',  ( -8.224510206698735004, -14.34966873604973081, 54.58442372801901143 ) ) ;
#121537=CARTESIAN_POINT ( 'NONE',  ( -16.55341960407611168, -4.379528057220339221, 81.45724293864769550 ) ) ;
#121538=CARTESIAN_POINT ( 'NONE',  ( 15.80617190586746368, 15.72974639402197994, 79.37390960531436690 ) ) ;
#121539=CARTESIAN_POINT ( 'NONE',  ( -12.14591786802309592, -12.06949235617757132, 31.87390960531435979 ) ) ;
#121540=CARTESIAN_POINT ( 'NONE',  ( 12.06949235617739724, 12.14591786802326823, 46.87609039468568994 ) ) ;
#121541=CARTESIAN_POINT ( 'NONE',  ( -9.474510206698964154, 16.51473224551069663, 45.41557627198103120 ) ) ;
#121542=CARTESIAN_POINT ( 'NONE',  ( 16.52544592524335698, 4.483927247898782831, 81.45942372801900433 ) ) ;
#121543=CARTESIAN_POINT ( 'NONE',  ( -16.51473224551082808, 9.474510206698731452, 93.33442372801900433 ) ) ;
#121544=CARTESIAN_POINT ( 'NONE',  ( -21.53943276465977519, 0.05219959533907696930, 71.24890960531435269 ) ) ;
#121545=CARTESIAN_POINT ( 'NONE',  ( 14.29746914071049879, -8.314922557960816363, 23.33224293864769194 ) ) ;
#121548=CARTESIAN_POINT ( 'NONE',  ( -18.67979575497178146, -10.72451020669898902, 61.66557627198103120 ) ) ;
#121550=CARTESIAN_POINT ( 'NONE',  ( 12.14591786802327356, -12.06949235617739191, 85.62609039468568994 ) ) ;
#121552=CARTESIAN_POINT ( 'NONE',  ( 0.05219959533909260263, 19.03943276465977164, 114.9989096053143669 ) ) ;
#121553=CARTESIAN_POINT ( 'NONE',  ( 17.50000000000014566, 3.292511757969701858, 107.4347972978946615 ) ) ;
#121554=CARTESIAN_POINT ( 'NONE',  ( 18.67979575497178502, 10.72451020669898547, 69.16557627198102409 ) ) ;
#121555=CARTESIAN_POINT ( 'NONE',  ( 8.314922557961029526, -14.29746914071037800, 105.4177570613523613 ) ) ;
#121556=CARTESIAN_POINT ( 'NONE',  ( 8.224510206698742110, 14.34966873604972548, 22.08442372801901143 ) ) ;
#121557=CARTESIAN_POINT ( 'NONE',  ( -14.29746914071049879, 8.314922557960819915, 115.8322429386477097 ) ) ;
#121558=CARTESIAN_POINT ( 'NONE',  ( 12.14591786802327356, -12.06949235617739191, 25.62609039468567929 ) ) ;
#121559=AXIS2_PLACEMENT_3D ( 'NONE', #77864, #62688, #165928 ) ;
#121560=CARTESIAN_POINT ( 'NONE',  ( -19.05341960407611168, -5.049401038298163336, 56.45724293864768129 ) ) ;
#121562=CARTESIAN_POINT ( 'NONE',  ( -9.474510206698964154, 16.51473224551069663, 105.4155762719810383 ) ) ;
#121563=CARTESIAN_POINT ( 'NONE',  ( -16.53943276465976808, -0.05219959533934237506, 88.75109039468567573 ) ) ;
#121564=B_SPLINE_CURVE_WITH_KNOTS ( 'NONE', 3,
 ( #106408, #108402, #79051, #170079, #91218, #63896, #183272, #186263 ),
 .UNSPECIFIED., .F., .F.,
 ( 4, 2, 2, 4 ),
 ( 1.015220885719448636E-17, 0.002784256700436080808, 0.005568513400872152075, 0.01113702680174429374 ),
 .UNSPECIFIED. ) ;
#121565=CARTESIAN_POINT ( 'NONE',  ( 13.89961937509957401, 13.97604488694547697, 86.87609039468567573 ) ) ;
#121566=CARTESIAN_POINT ( 'NONE',  ( -9.474510206698720793, -16.51473224551083518, 24.58442372801900078 ) ) ;
#121567=CARTESIAN_POINT ( 'NONE',  ( -18.67979575497178146, -10.72451020669898902, 76.66557627198103830 ) ) ;
#121568=CARTESIAN_POINT ( 'NONE',  ( 4.379528057220092307, 16.55341960407617563, 102.2927570613523613 ) ) ;
#121569=CARTESIAN_POINT ( 'NONE',  ( -5.153800228976607833, 19.02544592524334988, 97.70942372801900433 ) ) ;
#121570=CARTESIAN_POINT ( 'NONE',  ( 16.46253265017160672, -9.564922557960803928, 43.33224293864769550 ) ) ;
#121571=CARTESIAN_POINT ( 'NONE',  ( 5.049401038298161559, -19.05341960407611168, 92.70724293864769550 ) ) ;
#121572=CARTESIAN_POINT ( 'NONE',  ( 21.55341960407619695, -5.719274019375665929, 56.04275706135235424 ) ) ;
#121573=CARTESIAN_POINT ( 'NONE',  ( -13.97604488694527625, -13.89961937509977652, 51.87390960531436690 ) ) ;
#121574=CARTESIAN_POINT ( 'NONE',  ( -17.49999999999999645, -5.499999999999992895, 84.20309617465829888 ) ) ;
#121575=CARTESIAN_POINT ( 'NONE',  ( -4.379528057220328563, 16.55341960407611168, 80.20724293864769550 ) ) ;
#121576=CARTESIAN_POINT ( 'NONE',  ( -5.823673210054116645, -21.52544592524344225, 77.29057627198102409 ) ) ;
#121578=CARTESIAN_POINT ( 'NONE',  ( 17.44270441346518652, -5.991230190322965221, 81.13664920735772057 ) ) ;
#121579=CARTESIAN_POINT ( 'NONE',  ( -9.564922557961040184, 16.46253265017147172, 37.91775706135233293 ) ) ;
#121580=CARTESIAN_POINT ( 'NONE',  ( 16.79531203550682861, -7.028104445595347194, 71.24755011779539871 ) ) ;
#121581=CARTESIAN_POINT ( 'NONE',  ( 19.03943276465977164, -0.05219959533909143690, 78.74890960531436690 ) ) ;
#121582=CARTESIAN_POINT ( 'NONE',  ( -19.03943276465977164, 0.05219959533909376836, 91.24890960531436690 ) ) ;
#121583=CARTESIAN_POINT ( 'NONE',  ( 12.06949235617739724, 12.14591786802326823, 61.87609039468568284 ) ) ;
#121585=CARTESIAN_POINT ( 'NONE',  ( -19.05341960407617563, 5.049401038297882671, 28.54275706135232937 ) ) ;
#121587=CARTESIAN_POINT ( 'NONE',  ( 0.05219959533909260263, 19.03943276465977164, 114.9989096053143669 ) ) ;
#121588=CARTESIAN_POINT ( 'NONE',  ( 8.314922557961029526, -14.29746914071037800, 85.41775706135236135 ) ) ;
#121590=CARTESIAN_POINT ( 'NONE',  ( -16.53943276465976808, -0.05219959533934237506, 73.75109039468567573 ) ) ;
#121591=CARTESIAN_POINT ( 'NONE',  ( -17.26172910966779739, 6.454744622555852018, 30.80646908649224258 ) ) ;
#121592=CARTESIAN_POINT ( 'NONE',  ( -16.53943276465976808, -0.05219959533934237506, 58.75109039468568994 ) ) ;
#121594=CARTESIAN_POINT ( 'NONE',  ( -5.823673210054431948, 21.52544592524334988, 72.70942372801901854 ) ) ;
#121595=CARTESIAN_POINT ( 'NONE',  ( -5.049401038297874678, -19.05341960407617918, 79.79275706135233293 ) ) ;
#121596=CARTESIAN_POINT ( 'NONE',  ( 9.564922557961047289, -16.46253265017146816, 25.41775706135234003 ) ) ;
#121597=CARTESIAN_POINT ( 'NONE',  ( 5.153800228976335163, 19.02544592524342804, 49.79057627198100988 ) ) ;
#121598=CARTESIAN_POINT ( 'NONE',  ( 0.05219959533909260263, 19.03943276465977164, 39.99890960531436690 ) ) ;
#121600=CARTESIAN_POINT ( 'NONE',  ( 21.52544592524344225, -5.823673210054117533, 63.54057627198103830 ) ) ;
#121601=CARTESIAN_POINT ( 'NONE',  ( 10.72451020669898902, -18.67979575497178502, 22.91557627198102765 ) ) ;
#121602=CARTESIAN_POINT ( 'NONE',  ( 9.564922557960805705, 16.46253265017160317, 24.58224293864769194 ) ) ;
#121603=CARTESIAN_POINT ( 'NONE',  ( 4.379528057220092307, 16.55341960407617563, 47.29275706135234003 ) ) ;
#121604=EDGE_LOOP ( 'NONE', ( #50547, #67559, #64532, #26832, #184289, #70621, #180071, #95804, #71080, #145094, #74688, #134640, #150834, #150466, #3012, #68861, #16908, #35991, #103023, #102608, #129725, #149795, #15254, #69892, #177577, #193253, #111683, #37737, #178353, #63094, #94729, #68185, #172093, #90223, #73211, #58491, #102024, #131534, #16429, #20200, #117675, #165718, #39736, #49800 ) ) ;
#121605=EDGE_CURVE ( 'NONE', #60482, #144727, #179631, .T. ) ;
#121606=CARTESIAN_POINT ( 'NONE',  ( 21.55341960407619695, -5.719274019375665929, 21.04275706135234714 ) ) ;
#121607=CARTESIAN_POINT ( 'NONE',  ( -0.05219959533910754901, -16.53943276465976808, 57.49890960531435979 ) ) ;
#121609=CARTESIAN_POINT ( 'NONE',  ( 19.03943276465977164, 0.05219959533936151252, 106.2510903946856615 ) ) ;
#121610=CARTESIAN_POINT ( 'NONE',  ( 19.02544592524334988, 5.153800228976608722, 36.45942372801900433 ) ) ;
#121611=CARTESIAN_POINT ( 'NONE',  ( 8.314922557960818139, 14.29746914071049879, 44.58224293864769550 ) ) ;
#121612=CARTESIAN_POINT ( 'NONE',  ( 0.05219959533937995610, -21.53943276465977519, 20.00109039468568639 ) ) ;
#121613=CARTESIAN_POINT ( 'NONE',  ( 17.44270441346512612, 5.991230190323098448, 33.86335079264229364 ) ) ;
#121614=CARTESIAN_POINT ( 'NONE',  ( -5.719274019375978568, 21.55341960407610458, 65.20724293864768129 ) ) ;
#121615=CARTESIAN_POINT ( 'NONE',  ( 9.564922557960805705, 16.46253265017160317, 84.58224293864769550 ) ) ;
#121616=CARTESIAN_POINT ( 'NONE',  ( 4.483927247898545687, 16.52544592524342804, 59.79057627198103120 ) ) ;
#121617=CARTESIAN_POINT ( 'NONE',  ( 19.05341960407611168, 5.049401038298154454, 103.9572429386476671 ) ) ;
#121618=LINE ( 'NONE', #45784, #40896 ) ;
#121619=CARTESIAN_POINT ( 'NONE',  ( -19.05341960407617563, 5.049401038297882671, 48.54275706135233293 ) ) ;
#121620=CARTESIAN_POINT ( 'NONE',  ( -18.67979575497178146, -10.72451020669898902, 96.66557627198102409 ) ) ;
#121621=CARTESIAN_POINT ( 'NONE',  ( -5.153800228976328057, -19.02544592524343514, 47.29057627198102409 ) ) ;
#121622=CARTESIAN_POINT ( 'NONE',  ( -8.224510206698948167, 14.34966873604960824, 115.4155762719810241 ) ) ;
#121623=CARTESIAN_POINT ( 'NONE',  ( 18.67979575497194134, -10.72451020669871369, 45.83442372801901854 ) ) ;
#121625=CARTESIAN_POINT ( 'NONE',  ( 16.52544592524342804, -4.483927247898539470, 23.54057627198102765 ) ) ;
#121626=CARTESIAN_POINT ( 'NONE',  ( 19.03943276465977164, -0.05219959533909143690, 53.74890960531436690 ) ) ;
#121627=CARTESIAN_POINT ( 'NONE',  ( 16.46253265017160672, -9.564922557960803928, 93.33224293864769550 ) ) ;
#121628=CARTESIAN_POINT ( 'NONE',  ( 0.05219959533907565091, 21.53943276465977519, 69.99890960531435269 ) ) ;
#121630=CARTESIAN_POINT ( 'NONE',  ( 13.97604488694527802, 13.89961937509977652, 39.37390960531435269 ) ) ;
#121631=CARTESIAN_POINT ( 'NONE',  ( -15.80617190586745835, -15.72974639402198527, 46.87390960531435979 ) ) ;
#121633=CARTESIAN_POINT ( 'NONE',  ( 21.53943276465977519, 0.05219959533937863772, 86.25109039468568994 ) ) ;
#121635=CARTESIAN_POINT ( 'NONE',  ( 12.06949235617739724, 12.14591786802326823, 81.87609039468568994 ) ) ;
#121636=CARTESIAN_POINT ( 'NONE',  ( -16.55341960407611168, -4.379528057220339221, 71.45724293864769550 ) ) ;
#121637=CARTESIAN_POINT ( 'NONE',  ( -16.51473224551069308, -9.474510206698971260, 66.66557627198102409 ) ) ;
#121638=ORIENTED_EDGE ( 'NONE', *, *, #127302, .F. ) ;
#121639=CARTESIAN_POINT ( 'NONE',  ( -13.97604488694547697, 13.89961937509957934, 23.12609039468565442 ) ) ;
#121640=CARTESIAN_POINT ( 'NONE',  ( 8.224510206698742110, 14.34966873604972548, 87.08442372801901854 ) ) ;
#121641=CARTESIAN_POINT ( 'NONE',  ( -10.81492255796105439, 18.62759615963255655, 107.9177570613523471 ) ) ;
#121642=CARTESIAN_POINT ( 'NONE',  ( 13.97604488694527802, 13.89961937509977652, 69.37390960531436690 ) ) ;
#121643=CARTESIAN_POINT ( 'NONE',  ( -15.72974639402197994, 15.80617190586746368, 45.62390960531436690 ) ) ;
#121644=CARTESIAN_POINT ( 'NONE',  ( 4.379528057220092307, 16.55341960407617563, 27.29275706135234358 ) ) ;
#121645=CARTESIAN_POINT ( 'NONE',  ( 21.55341960407619695, -5.719274019375665929, 81.04275706135236135 ) ) ;
#121646=CARTESIAN_POINT ( 'NONE',  ( 12.14591786802327356, -12.06949235617739191, 65.62609039468568994 ) ) ;
#121647=CARTESIAN_POINT ( 'NONE',  ( 18.62759615963271287, -10.81492255796078972, 113.3322429386476955 ) ) ;
#121648=CARTESIAN_POINT ( 'NONE',  ( -0.05219959533936034679, 19.03943276465977164, 112.5010903946856757 ) ) ;
#121649=CARTESIAN_POINT ( 'NONE',  ( -0.05219959533909027116, -19.03943276465977164, 97.49890960531436690 ) ) ;
#121650=CARTESIAN_POINT ( 'NONE',  ( -16.52544592524335698, -4.483927247898792601, 33.95942372801901143 ) ) ;
#121651=CARTESIAN_POINT ( 'NONE',  ( 16.51473224551069308, 9.474510206698969483, 44.16557627198103120 ) ) ;
#121653=CARTESIAN_POINT ( 'NONE',  ( 16.53943276465976808, 0.05219959533934440121, 36.25109039468567573 ) ) ;
#121654=CARTESIAN_POINT ( 'NONE',  ( 4.379528057220339221, -16.55341960407611168, 82.70724293864770971 ) ) ;
#121655=CARTESIAN_POINT ( 'NONE',  ( -8.314922557961024197, 14.29746914071037800, 87.91775706135234714 ) ) ;
#121656=CARTESIAN_POINT ( 'NONE',  ( -10.72451020669870658, -18.67979575497194134, 24.58442372801901499 ) ) ;
#121657=CARTESIAN_POINT ( 'NONE',  ( -19.05341960407611168, -5.049401038298163336, 61.45724293864769550 ) ) ;
#121658=CARTESIAN_POINT ( 'NONE',  ( -5.153800228976328057, -19.02544592524343514, 87.29057627198103830 ) ) ;
#121659=CARTESIAN_POINT ( 'NONE',  ( -8.314922557961024197, 14.29746914071037800, 82.91775706135234714 ) ) ;
#121663=CARTESIAN_POINT ( 'NONE',  ( -0.05219959533936034679, 19.03943276465977164, 37.50109039468567573 ) ) ;
#121664=CARTESIAN_POINT ( 'NONE',  ( 19.05341960407611168, 5.049401038298154454, 103.9572429386476671 ) ) ;
#121665=CARTESIAN_POINT ( 'NONE',  ( 5.153800228976335163, 19.02544592524342804, 49.79057627198100988 ) ) ;
#121666=CARTESIAN_POINT ( 'NONE',  ( 13.89961937509977652, -13.97604488694527269, 113.1239096053143527 ) ) ;
#121667=ORIENTED_EDGE ( 'NONE', *, *, #28410, .T. ) ;
#121668=CARTESIAN_POINT ( 'NONE',  ( 12.14591786802327356, -12.06949235617739191, 25.62609039468567929 ) ) ;
#121669=CARTESIAN_POINT ( 'NONE',  ( 19.05341960407617918, -5.049401038297876454, 56.04275706135234714 ) ) ;
#121670=CARTESIAN_POINT ( 'NONE',  ( 16.52544592524335698, 4.483927247898782831, 36.45942372801901143 ) ) ;
#121671=CARTESIAN_POINT ( 'NONE',  ( -9.564922557960796823, -16.46253265017161027, 102.0822429386477097 ) ) ;
#121672=CARTESIAN_POINT ( 'NONE',  ( 9.564922557960805705, 16.46253265017160317, 74.58224293864769550 ) ) ;
#121673=CARTESIAN_POINT ( 'NONE',  ( -18.67979575497178146, -10.72451020669898902, 96.66557627198102409 ) ) ;
#121674=CARTESIAN_POINT ( 'NONE',  ( 19.03943276465977164, 0.05219959533936151252, 61.25109039468566863 ) ) ;
#121675=CARTESIAN_POINT ( 'NONE',  ( -19.03943276465977164, 0.05219959533909376836, 96.24890960531436690 ) ) ;
#121676=CARTESIAN_POINT ( 'NONE',  ( 17.50000000000000000, -3.456093896842488800, 22.00000000000000711 ) ) ;
#121677=CARTESIAN_POINT ( 'NONE',  ( -16.51473224551069308, -9.474510206698971260, 66.66557627198102409 ) ) ;
#121678=CARTESIAN_POINT ( 'NONE',  ( -16.55341960407611168, -4.379528057220339221, 31.45724293864769550 ) ) ;
#121679=CARTESIAN_POINT ( 'NONE',  ( 19.05341960407611168, 5.049401038298154454, 28.95724293864769550 ) ) ;
#121680=CARTESIAN_POINT ( 'NONE',  ( 5.153800228976615827, -19.02544592524334988, 40.20942372801898301 ) ) ;
#121681=CARTESIAN_POINT ( 'NONE',  ( 14.34966873604960469, 8.224510206698951720, 79.16557627198103830 ) ) ;
#121682=CARTESIAN_POINT ( 'NONE',  ( 5.823673210054444382, -21.52544592524334988, 100.2094237280190043 ) ) ;
#121683=CARTESIAN_POINT ( 'NONE',  ( 13.89961937509977652, -13.97604488694527269, 33.12390960531434558 ) ) ;
#121684=CARTESIAN_POINT ( 'NONE',  ( 16.53943276465976808, 0.05219959533934440121, 56.25109039468568284 ) ) ;
#121685=CARTESIAN_POINT ( 'NONE',  ( 14.34966873604960469, 8.224510206698951720, 34.16557627198102409 ) ) ;
#121686=CARTESIAN_POINT ( 'NONE',  ( -15.80617190586768217, 15.72974639402176855, 98.12609039468570415 ) ) ;
#121687=CARTESIAN_POINT ( 'NONE',  ( -13.89961937509977652, 13.97604488694528158, 90.62390960531432427 ) ) ;
#121688=CARTESIAN_POINT ( 'NONE',  ( -16.46253265017160317, 9.564922557960807481, 95.83224293864769550 ) ) ;
#121689=CARTESIAN_POINT ( 'NONE',  ( -4.483927247898539470, -16.52544592524342804, 102.2905762719810383 ) ) ;
#121690=CARTESIAN_POINT ( 'NONE',  ( 16.55341960407611168, 4.379528057220329451, 68.95724293864769550 ) ) ;
#121691=CARTESIAN_POINT ( 'NONE',  ( 21.52544592524344225, -5.823673210054117533, 78.54057627198103830 ) ) ;
#121692=CARTESIAN_POINT ( 'NONE',  ( 9.564922557960805705, 16.46253265017160317, 84.58224293864769550 ) ) ;
#121693=CARTESIAN_POINT ( 'NONE',  ( 15.80617190586746368, 15.72974639402197994, 99.37390960531436690 ) ) ;
#121694=CARTESIAN_POINT ( 'NONE',  ( -16.51473224551069308, -9.474510206698971260, 96.66557627198102409 ) ) ;
#121695=CARTESIAN_POINT ( 'NONE',  ( 19.49149378614658090, -5.499999999999770850, 46.93757513605363130 ) ) ;
#121696=CARTESIAN_POINT ( 'NONE',  ( 16.53943276465976808, -0.05219959533910856209, 88.74890960531436690 ) ) ;
#121698=CARTESIAN_POINT ( 'NONE',  ( -9.564922557960796823, -16.46253265017161027, 62.08224293864769550 ) ) ;
#121699=CARTESIAN_POINT ( 'NONE',  ( 18.67979575497178502, 10.72451020669898547, 69.16557627198102409 ) ) ;
#121700=CARTESIAN_POINT ( 'NONE',  ( 17.50000000000000000, -5.500000000000000888, 28.29690382534172244 ) ) ;
#121701=CARTESIAN_POINT ( 'NONE',  ( 14.29746914071049879, -8.314922557960816363, 23.33224293864769194 ) ) ;
#121703=CARTESIAN_POINT ( 'NONE',  ( 13.89961937509957401, 13.97604488694547697, 111.8760903946856757 ) ) ;
#121704=EDGE_CURVE ( 'NONE', #23056, #69916, #42106, .T. ) ;
#121705=CARTESIAN_POINT ( 'NONE',  ( 14.29746914071049879, -8.314922557960816363, 83.33224293864769550 ) ) ;
#121706=CARTESIAN_POINT ( 'NONE',  ( -17.40805194822031865, -6.112264579159342404, 94.16628727489391792 ) ) ;
#121707=CARTESIAN_POINT ( 'NONE',  ( 0.05219959533909260263, 19.03943276465977164, 74.99890960531435269 ) ) ;
#121708=CARTESIAN_POINT ( 'NONE',  ( 13.97604488694527802, 13.89961937509977652, 44.37390960531435269 ) ) ;
#121709=CARTESIAN_POINT ( 'NONE',  ( -16.52544592524342804, 4.483927247898546575, 61.04057627198103120 ) ) ;
#121710=CARTESIAN_POINT ( 'NONE',  ( 16.51473224551069308, 9.474510206698969483, 109.1655762719810383 ) ) ;
#121711=CARTESIAN_POINT ( 'NONE',  ( -13.89961937509957401, -13.97604488694547875, 104.3760903946856757 ) ) ;
#121712=CARTESIAN_POINT ( 'NONE',  ( 16.46253265017160672, -9.564922557960803928, 98.33224293864769550 ) ) ;
#121713=CARTESIAN_POINT ( 'NONE',  ( 10.81492255796078972, 18.62759615963270932, 74.58224293864768129 ) ) ;
#121714=CARTESIAN_POINT ( 'NONE',  ( -4.483927247898782831, 16.52544592524335698, 72.70942372801901854 ) ) ;
#121715=CARTESIAN_POINT ( 'NONE',  ( -17.05116617787849975, 6.768360034955466453, 93.65675553259190167 ) ) ;
#121716=CARTESIAN_POINT ( 'NONE',  ( -9.474510206698964154, 16.51473224551069663, 70.41557627198102409 ) ) ;
#121717=CARTESIAN_POINT ( 'NONE',  ( 18.62759615963271287, -10.81492255796078972, 78.33224293864770971 ) ) ;
#121719=CARTESIAN_POINT ( 'NONE',  ( 13.89961937509957401, 13.97604488694547697, 111.8760903946856757 ) ) ;
#121720=CARTESIAN_POINT ( 'NONE',  ( -0.05219959533910754901, -16.53943276465976808, 42.49890960531435979 ) ) ;
#121721=CARTESIAN_POINT ( 'NONE',  ( -10.72451020669870658, -18.67979575497194134, 59.58442372801901854 ) ) ;
#121722=CARTESIAN_POINT ( 'NONE',  ( -16.53943276465976808, -0.05219959533934237506, 88.75109039468567573 ) ) ;
#121723=CARTESIAN_POINT ( 'NONE',  ( -16.51473224551069308, -9.474510206698971260, 111.6655762719810383 ) ) ;
#121724=CARTESIAN_POINT ( 'NONE',  ( 9.474510206698971260, -16.51473224551069308, 107.9155762719810383 ) ) ;
#121726=CARTESIAN_POINT ( 'NONE',  ( -16.52544592524335698, -4.483927247898792601, 88.95942372801901854 ) ) ;
#121727=CARTESIAN_POINT ( 'NONE',  ( 16.53943276465976808, 0.05219959533934440121, 41.25109039468568284 ) ) ;
#121728=CARTESIAN_POINT ( 'NONE',  ( 16.51473224551069308, 9.474510206698969483, 64.16557627198102409 ) ) ;
#121729=CARTESIAN_POINT ( 'NONE',  ( 9.564922557960805705, 16.46253265017160317, 79.58224293864769550 ) ) ;
#121730=CARTESIAN_POINT ( 'NONE',  ( 10.72451020669871369, 18.67979575497193778, 72.08442372801899012 ) ) ;
#121731=CARTESIAN_POINT ( 'NONE',  ( -16.53943276465976808, -0.05219959533934237506, 68.75109039468568994 ) ) ;
#121732=CARTESIAN_POINT ( 'NONE',  ( 0.05219959533910956823, 16.53943276465976808, 29.99890960531435979 ) ) ;
#121733=CARTESIAN_POINT ( 'NONE',  ( 5.049401038298161559, -19.05341960407611168, 42.70724293864767418 ) ) ;
#121734=CARTESIAN_POINT ( 'NONE',  ( 19.05341960407611168, 5.049401038298154454, 48.95724293864768129 ) ) ;
#121735=CARTESIAN_POINT ( 'NONE',  ( 16.52544592524335698, 4.483927247898782831, 46.45942372801901854 ) ) ;
#121736=CARTESIAN_POINT ( 'NONE',  ( -0.05219959533936034679, 19.03943276465977164, 97.50109039468567573 ) ) ;
#121737=CARTESIAN_POINT ( 'NONE',  ( 4.483927247898545687, 16.52544592524342804, 99.79057627198103830 ) ) ;
#121738=CARTESIAN_POINT ( 'NONE',  ( 0.05219959533909260263, 19.03943276465977164, 64.99890960531436690 ) ) ;
#121739=CARTESIAN_POINT ( 'NONE',  ( 9.474510206698729675, 16.51473224551082808, 87.08442372801900433 ) ) ;
#121741=CARTESIAN_POINT ( 'NONE',  ( -18.67979575497193778, 10.72451020669871902, 88.33442372801901854 ) ) ;
#121742=CARTESIAN_POINT ( 'NONE',  ( 14.34966873604972726, -8.224510206698740333, 60.83442372801901854 ) ) ;
#121744=CARTESIAN_POINT ( 'NONE',  ( 18.67979575497178502, 10.72451020669898547, 44.16557627198103120 ) ) ;
#121745=CARTESIAN_POINT ( 'NONE',  ( 4.483927247898790824, -16.52544592524335698, 45.20942372801901854 ) ) ;
#121746=CARTESIAN_POINT ( 'NONE',  ( -19.52217212775661537, 5.499999999999920064, 69.93993709005260939 ) ) ;
#121747=CARTESIAN_POINT ( 'NONE',  ( -19.03943276465977164, -0.05219959533935918106, 43.75109039468566863 ) ) ;
#121748=CARTESIAN_POINT ( 'NONE',  ( -13.89961937509977652, 13.97604488694528158, 85.62390960531433848 ) ) ;
#121749=CARTESIAN_POINT ( 'NONE',  ( 0.05219959533909260263, 19.03943276465977164, 24.99890960531435269 ) ) ;
#121750=CARTESIAN_POINT ( 'NONE',  ( 16.46253265017160672, -9.564922557960803928, 58.33224293864769550 ) ) ;
#121752=CARTESIAN_POINT ( 'NONE',  ( 0.05219959533937995610, -21.53943276465977519, 75.00109039468568994 ) ) ;
#121754=CARTESIAN_POINT ( 'NONE',  ( 16.46253265017146816, 9.564922557961045513, 31.66775706135232937 ) ) ;
#121755=CARTESIAN_POINT ( 'NONE',  ( -15.72974639402176322, -15.80617190586768395, 109.3760903946857042 ) ) ;
#121756=CARTESIAN_POINT ( 'NONE',  ( 14.29746914071049879, -8.314922557960816363, 48.33224293864770260 ) ) ;
#121757=CARTESIAN_POINT ( 'NONE',  ( -9.564922557960796823, -16.46253265017161027, 52.08224293864768839 ) ) ;
#121758=CARTESIAN_POINT ( 'NONE',  ( -5.049401038298153566, 19.05341960407611168, 115.2072429386477097 ) ) ;
#121759=CARTESIAN_POINT ( 'NONE',  ( -15.80617190586768217, 15.72974639402176855, 88.12609039468570415 ) ) ;
#121760=CARTESIAN_POINT ( 'NONE',  ( -19.05341960407611168, -5.049401038298163336, 61.45724293864769550 ) ) ;
#121761=CARTESIAN_POINT ( 'NONE',  ( 5.823673210054444382, -21.52544592524334988, 75.20942372801901854 ) ) ;
#121762=CARTESIAN_POINT ( 'NONE',  ( -0.05219959533907301413, -21.53943276465977519, 37.49890960531436690 ) ) ;
#121763=CARTESIAN_POINT ( 'NONE',  ( 10.81492255796106328, -18.62759615963255655, 40.41775706135234714 ) ) ;
#121764=CARTESIAN_POINT ( 'NONE',  ( -9.474510206698720793, -16.51473224551083518, 64.58442372801900433 ) ) ;
#121765=CARTESIAN_POINT ( 'NONE',  ( -9.564922557960796823, -16.46253265017161027, 32.08224293864769550 ) ) ;
#121766=CARTESIAN_POINT ( 'NONE',  ( 13.97604488694527802, 13.89961937509977652, 79.37390960531435269 ) ) ;
#121767=CARTESIAN_POINT ( 'NONE',  ( 8.314922557961029526, -14.29746914071037800, 35.41775706135234003 ) ) ;
#121768=CARTESIAN_POINT ( 'NONE',  ( 12.06949235617757843, -12.14591786802309237, 93.12390960531436690 ) ) ;
#121769=CARTESIAN_POINT ( 'NONE',  ( -0.05219959533909027116, -19.03943276465977164, 57.49890960531435979 ) ) ;
#121770=CARTESIAN_POINT ( 'NONE',  ( -5.823673210054116645, -21.52544592524344225, 42.29057627198103120 ) ) ;
#121771=CARTESIAN_POINT ( 'NONE',  ( -16.52544592524335698, -4.483927247898792601, 23.95942372801901143 ) ) ;
#121772=CARTESIAN_POINT ( 'NONE',  ( -5.719274019375665041, -21.55341960407619695, 19.79275706135235069 ) ) ;
#121773=CARTESIAN_POINT ( 'NONE',  ( -21.55341960407619339, 5.719274019375674811, 68.54275706135234714 ) ) ;
#121774=CARTESIAN_POINT ( 'NONE',  ( -4.483927247898782831, 16.52544592524335698, 67.70942372801901854 ) ) ;
#121775=CARTESIAN_POINT ( 'NONE',  ( 8.224510206698742110, 14.34966873604972548, 72.08442372801899012 ) ) ;
#121776=ORIENTED_EDGE ( 'NONE', *, *, #163633, .F. ) ;
#121777=CARTESIAN_POINT ( 'NONE',  ( 19.03943276465977164, -0.05219959533909143690, 63.74890960531435979 ) ) ;
#121778=CARTESIAN_POINT ( 'NONE',  ( 16.53943276465976808, 0.05219959533934440121, 86.25109039468568994 ) ) ;
#121779=CARTESIAN_POINT ( 'NONE',  ( 13.89961937509957401, 13.97604488694547697, 36.87609039468565442 ) ) ;
#121780=CARTESIAN_POINT ( 'NONE',  ( -21.52544592524343514, 5.823673210054127303, 116.0405762719810383 ) ) ;
#121781=CARTESIAN_POINT ( 'NONE',  ( -16.55341960407611168, -4.379528057220339221, 71.45724293864769550 ) ) ;
#121782=CARTESIAN_POINT ( 'NONE',  ( 0.05219959533909260263, 19.03943276465977164, 84.99890960531436690 ) ) ;
#121783=CARTESIAN_POINT ( 'NONE',  ( -4.483927247898782831, 16.52544592524335698, 87.70942372801901854 ) ) ;
#121784=CARTESIAN_POINT ( 'NONE',  ( 18.67979575497194134, -10.72451020669871369, 55.83442372801901854 ) ) ;
#121785=CARTESIAN_POINT ( 'NONE',  ( 4.483927247898790824, -16.52544592524335698, 30.20942372801902565 ) ) ;
#121786=CARTESIAN_POINT ( 'NONE',  ( 10.72451020669898902, -18.67979575497178502, 112.9155762719810383 ) ) ;
#121787=CARTESIAN_POINT ( 'NONE',  ( -14.29746914071049879, 8.314922557960819915, 60.83224293864769550 ) ) ;
#121789=CARTESIAN_POINT ( 'NONE',  ( -5.719274019375978568, 21.55341960407610458, 105.2072429386477097 ) ) ;
#121790=CARTESIAN_POINT ( 'NONE',  ( -14.29746914071049879, 8.314922557960819915, 40.83224293864769550 ) ) ;
#121791=ORIENTED_EDGE ( 'NONE', *, *, #127587, .T. ) ;
#121793=CARTESIAN_POINT ( 'NONE',  ( 13.89961937509977652, -13.97604488694527269, 113.1239096053143527 ) ) ;
#121794=CARTESIAN_POINT ( 'NONE',  ( 18.62759615963255655, 10.81492255796105972, 36.66775706135234714 ) ) ;
#121795=CARTESIAN_POINT ( 'NONE',  ( -16.55341960407611168, -4.379528057220339221, 56.45724293864768839 ) ) ;
#121797=CARTESIAN_POINT ( 'NONE',  ( 9.474510206698971260, -16.51473224551069308, 67.91557627198102409 ) ) ;
#121798=CARTESIAN_POINT ( 'NONE',  ( 19.05341960407617918, -5.049401038297876454, 71.04275706135234714 ) ) ;
#121799=CARTESIAN_POINT ( 'NONE',  ( 16.46253265017160672, -9.564922557960803928, 93.33224293864769550 ) ) ;
#121800=CARTESIAN_POINT ( 'NONE',  ( -15.80617190586745835, -15.72974639402198527, 46.87390960531435979 ) ) ;
#121802=CARTESIAN_POINT ( 'NONE',  ( 13.97604488694527802, 13.89961937509977652, 54.37390960531435979 ) ) ;
#121803=CARTESIAN_POINT ( 'NONE',  ( 8.224510206698742110, 14.34966873604972548, 42.08442372801901854 ) ) ;
#121804=CARTESIAN_POINT ( 'NONE',  ( -18.62759615963255300, -10.81492255796106328, 24.16775706135235424 ) ) ;
#121805=CARTESIAN_POINT ( 'NONE',  ( 12.06949235617757843, -12.14591786802309237, 48.12390960531436690 ) ) ;
#121806=CARTESIAN_POINT ( 'NONE',  ( -5.153800228976328057, -19.02544592524343514, 87.29057627198103830 ) ) ;
#121807=CARTESIAN_POINT ( 'NONE',  ( -10.81492255796078084, -18.62759615963271287, 67.08224293864770971 ) ) ;
#121808=CARTESIAN_POINT ( 'NONE',  ( -5.719274019375978568, 21.55341960407610458, 105.2072429386477097 ) ) ;
#121809=CARTESIAN_POINT ( 'NONE',  ( -12.06949235617739369, -12.14591786802326823, 39.37609039468567573 ) ) ;
#121811=CARTESIAN_POINT ( 'NONE',  ( -15.72974639402197994, 15.80617190586746368, 40.62390960531435269 ) ) ;
#121812=CARTESIAN_POINT ( 'NONE',  ( 15.80617190586769283, -15.72974639402175789, 100.6260903946857184 ) ) ;
#121813=CARTESIAN_POINT ( 'NONE',  ( 19.05341960407611168, 5.049401038298154454, 103.9572429386476671 ) ) ;
#121814=CARTESIAN_POINT ( 'NONE',  ( 19.03943276465977164, -0.05219959533909143690, 38.74890960531436690 ) ) ;
#121815=CARTESIAN_POINT ( 'NONE',  ( -19.02544592524342804, 5.153800228976336051, 96.04057627198103830 ) ) ;
#121816=CARTESIAN_POINT ( 'NONE',  ( -16.51473224551069308, -9.474510206698971260, 81.66557627198103830 ) ) ;
#121818=CARTESIAN_POINT ( 'NONE',  ( 9.564922557961047289, -16.46253265017146816, 60.41775706135233293 ) ) ;
#121820=CARTESIAN_POINT ( 'NONE',  ( 9.474510206698729675, 16.51473224551082808, 22.08442372801899722 ) ) ;
#121821=CARTESIAN_POINT ( 'NONE',  ( -21.55341960407610458, -5.719274019375992779, 36.45724293864768839 ) ) ;
#121822=CARTESIAN_POINT ( 'NONE',  ( 4.483927247898790824, -16.52544592524335698, 105.2094237280190328 ) ) ;
#121824=CARTESIAN_POINT ( 'NONE',  ( -17.40805194822032220, 6.112264579159342404, 60.83371272510612471 ) ) ;
#121825=CARTESIAN_POINT ( 'NONE',  ( -19.05341960407617563, 5.049401038297882671, 88.54275706135230450 ) ) ;
#121826=CARTESIAN_POINT ( 'NONE',  ( -5.049401038297874678, -19.05341960407617918, 29.79275706135232227 ) ) ;
#121828=CARTESIAN_POINT ( 'NONE',  ( -16.51473224551069308, -9.474510206698971260, 36.66557627198102409 ) ) ;
#121829=CARTESIAN_POINT ( 'NONE',  ( 16.52544592524342804, -4.483927247898539470, 43.54057627198103830 ) ) ;
#121830=CARTESIAN_POINT ( 'NONE',  ( -16.38665767535053774, -7.295008042176102769, 109.7359913578545303 ) ) ;
#121831=CARTESIAN_POINT ( 'NONE',  ( -12.06949235617756955, 12.14591786802309770, 25.62390960531435624 ) ) ;
#121833=CARTESIAN_POINT ( 'NONE',  ( 4.483927247898790824, -16.52544592524335698, 90.20942372801903275 ) ) ;
#121834=CARTESIAN_POINT ( 'NONE',  ( -19.05341960407611168, -5.049401038298163336, 51.45724293864770260 ) ) ;
#121835=CARTESIAN_POINT ( 'NONE',  ( -15.72974639402176322, -15.80617190586768395, 104.3760903946856899 ) ) ;
#121836=CARTESIAN_POINT ( 'NONE',  ( -13.89961937509957401, -13.97604488694547875, 109.3760903946856331 ) ) ;
#121837=CARTESIAN_POINT ( 'NONE',  ( 21.53943276465977519, 0.05219959533937863772, 91.25109039468568994 ) ) ;
#121838=CARTESIAN_POINT ( 'NONE',  ( 9.474510206698729675, 16.51473224551082808, 62.08442372801899722 ) ) ;
#121839=CARTESIAN_POINT ( 'NONE',  ( -13.89961937509977652, 13.97604488694528158, 90.62390960531432427 ) ) ;
#121840=CARTESIAN_POINT ( 'NONE',  ( 19.03943276465977164, -0.05219959533909143690, 83.74890960531436690 ) ) ;
#121842=CARTESIAN_POINT ( 'NONE',  ( 0.05219959533907565091, 21.53943276465977519, 109.9989096053143527 ) ) ;
#121844=CARTESIAN_POINT ( 'NONE',  ( -12.14591786802309592, -12.06949235617757132, 81.87390960531435269 ) ) ;
#121845=CARTESIAN_POINT ( 'NONE',  ( 10.72451020669898902, -18.67979575497178502, 57.91557627198103120 ) ) ;
#121846=CARTESIAN_POINT ( 'NONE',  ( 19.05341960407611168, 5.049401038298154454, 58.95724293864768129 ) ) ;
#121847=CARTESIAN_POINT ( 'NONE',  ( 10.81492255796078972, 18.62759615963270932, 94.58224293864769550 ) ) ;
#121848=CARTESIAN_POINT ( 'NONE',  ( 4.379528057220092307, 16.55341960407617563, 92.29275706135236135 ) ) ;
#121850=CARTESIAN_POINT ( 'NONE',  ( 19.05341960407611168, 5.049401038298154454, 58.95724293864768129 ) ) ;
#121852=CARTESIAN_POINT ( 'NONE',  ( -12.06949235617756955, 12.14591786802309770, 95.62390960531436690 ) ) ;
#121853=CARTESIAN_POINT ( 'NONE',  ( 15.50000000000000178, -7.500000000000000888, 118.0000000000000142 ) ) ;
#121854=CARTESIAN_POINT ( 'NONE',  ( -19.05341960407611168, -5.049401038298163336, 56.45724293864768129 ) ) ;
#121855=CARTESIAN_POINT ( 'NONE',  ( 13.97604488694548053, -13.89961937509957401, 80.62609039468567573 ) ) ;
#121856=CARTESIAN_POINT ( 'NONE',  ( 12.06949235617757843, -12.14591786802309237, 83.12390960531436690 ) ) ;
#121857=CARTESIAN_POINT ( 'NONE',  ( -0.05219959533937732626, 21.53943276465977519, 57.50109039468568994 ) ) ;
#121858=CARTESIAN_POINT ( 'NONE',  ( -16.46253265017160317, 9.564922557960807481, 30.83224293864769550 ) ) ;
#121859=CARTESIAN_POINT ( 'NONE',  ( 21.55341960407610458, 5.719274019375980345, 98.95724293864770971 ) ) ;
#121860=CARTESIAN_POINT ( 'NONE',  ( -8.314922557960811034, -14.29746914071050412, 102.0822429386476955 ) ) ;
#121861=CARTESIAN_POINT ( 'NONE',  ( 18.22780087662122384, 5.500000000000018652, 93.98459894673892734 ) ) ;
#121862=CARTESIAN_POINT ( 'NONE',  ( -5.049401038298153566, 19.05341960407611168, 60.20724293864768129 ) ) ;
#121864=CARTESIAN_POINT ( 'NONE',  ( 16.46253265017146816, 9.564922557961045513, 96.66775706135233293 ) ) ;
#121865=CARTESIAN_POINT ( 'NONE',  ( -19.02544592524342804, 5.153800228976336051, 106.0405762719810241 ) ) ;
#121866=CARTESIAN_POINT ( 'NONE',  ( 21.53943276465977519, 0.05219959533937863772, 56.25109039468568284 ) ) ;
#121867=CARTESIAN_POINT ( 'NONE',  ( 5.049401038298161559, -19.05341960407611168, 87.70724293864769550 ) ) ;
#121868=CARTESIAN_POINT ( 'NONE',  ( 19.05341960407617918, -5.049401038297876454, 71.04275706135234714 ) ) ;
#121869=CARTESIAN_POINT ( 'NONE',  ( -13.97604488694527625, -13.89961937509977652, 61.87390960531435979 ) ) ;
#121870=CARTESIAN_POINT ( 'NONE',  ( -14.34966873604960291, -8.224510206698953496, 81.66557627198103830 ) ) ;
#121871=CARTESIAN_POINT ( 'NONE',  ( 4.483927247898545687, 16.52544592524342804, 64.79057627198103830 ) ) ;
#121872=CARTESIAN_POINT ( 'NONE',  ( -5.049401038298153566, 19.05341960407611168, 95.20724293864770971 ) ) ;
#121873=CARTESIAN_POINT ( 'NONE',  ( -8.314922557960811034, -14.29746914071050412, 82.08224293864768129 ) ) ;
#121874=CARTESIAN_POINT ( 'NONE',  ( 0.05219959533909260263, 19.03943276465977164, 79.99890960531436690 ) ) ;
#121875=CARTESIAN_POINT ( 'NONE',  ( -19.03943276465977164, -0.05219959533935918106, 28.75109039468566507 ) ) ;
#121876=CARTESIAN_POINT ( 'NONE',  ( 5.153800228976335163, 19.02544592524342804, 49.79057627198100988 ) ) ;
#121877=CARTESIAN_POINT ( 'NONE',  ( 8.224510206698953496, -14.34966873604960469, 32.91557627198102409 ) ) ;
#121878=CARTESIAN_POINT ( 'NONE',  ( -16.53943276465976808, 0.05219959533911058130, 106.2489096053143811 ) ) ;
#121880=CARTESIAN_POINT ( 'NONE',  ( -21.55341960407619339, 5.719274019375674811, 38.54275706135234714 ) ) ;
#121881=CARTESIAN_POINT ( 'NONE',  ( -5.153800228976607833, 19.02544592524334988, 67.70942372801900433 ) ) ;
#121882=CARTESIAN_POINT ( 'NONE',  ( 0.05219959533910956823, 16.53943276465976808, 39.99890960531436690 ) ) ;
#121883=CARTESIAN_POINT ( 'NONE',  ( 10.81492255796078972, 18.62759615963270932, 79.58224293864769550 ) ) ;
#121884=CARTESIAN_POINT ( 'NONE',  ( 5.719274019375991003, -21.55341960407610458, 22.70724293864769194 ) ) ;
#121885=CARTESIAN_POINT ( 'NONE',  ( 4.379528057220339221, -16.55341960407611168, 72.70724293864769550 ) ) ;
#121886=CARTESIAN_POINT ( 'NONE',  ( 16.51473224551069308, 9.474510206698969483, 39.16557627198103120 ) ) ;
#121887=CARTESIAN_POINT ( 'NONE',  ( -13.97604488694547697, 13.89961937509957934, 43.12609039468566152 ) ) ;
#121888=CARTESIAN_POINT ( 'NONE',  ( 8.314922557961029526, -14.29746914071037800, 100.4177570613523471 ) ) ;
#121889=CARTESIAN_POINT ( 'NONE',  ( 8.314922557961029526, -14.29746914071037800, 60.41775706135235424 ) ) ;
#121890=CARTESIAN_POINT ( 'NONE',  ( -21.55341960407610458, -5.719274019375992779, 31.45724293864769550 ) ) ;
#121891=CARTESIAN_POINT ( 'NONE',  ( -21.52544592524334988, -5.823673210054445271, 103.9594237280190185 ) ) ;
#121892=CARTESIAN_POINT ( 'NONE',  ( 16.46253265017160672, -9.564922557960803928, 88.33224293864769550 ) ) ;
#121893=CARTESIAN_POINT ( 'NONE',  ( 0.05219959533934541429, -16.53943276465976808, 80.00109039468568994 ) ) ;
#121894=CARTESIAN_POINT ( 'NONE',  ( 9.474510206698971260, -16.51473224551069308, 27.91557627198103120 ) ) ;
#121895=CARTESIAN_POINT ( 'NONE',  ( 0.05219959533910956823, 16.53943276465976808, 34.99890960531435979 ) ) ;
#121896=CARTESIAN_POINT ( 'NONE',  ( -19.03943276465977164, 0.05219959533909376836, 111.2489096053143669 ) ) ;
#121897=CARTESIAN_POINT ( 'NONE',  ( -13.89961937509977652, 13.97604488694528158, 95.62390960531436690 ) ) ;
#121898=CARTESIAN_POINT ( 'NONE',  ( 5.823673210054125526, 21.52544592524343514, 24.79057627198103120 ) ) ;
#121899=CARTESIAN_POINT ( 'NONE',  ( 8.224510206698953496, -14.34966873604960469, 57.91557627198103120 ) ) ;
#121900=CARTESIAN_POINT ( 'NONE',  ( 12.06949235617757843, -12.14591786802309237, 28.12390960531435979 ) ) ;
#121901=B_SPLINE_CURVE_WITH_KNOTS ( 'NONE', 3,
 ( #146454, #7947, #109404, #33565, #156913, #69630 ),
 .UNSPECIFIED., .F., .F.,
 ( 4, 2, 4 ),
 ( 0.003989672132298142590, 0.004372778065220565835, 0.004755883998142989948 ),
 .UNSPECIFIED. ) ;
#121902=CARTESIAN_POINT ( 'NONE',  ( 12.06949235617757843, -12.14591786802309237, 58.12390960531435979 ) ) ;
#121904=CARTESIAN_POINT ( 'NONE',  ( 14.34966873604972726, -8.224510206698740333, 50.83442372801901143 ) ) ;
#121906=CARTESIAN_POINT ( 'NONE',  ( 19.05341960407617918, -5.049401038297876454, 51.04275706135231871 ) ) ;
#121907=CARTESIAN_POINT ( 'NONE',  ( 0.05219959533909260263, 19.03943276465977164, 94.99890960531436690 ) ) ;
#121908=CARTESIAN_POINT ( 'NONE',  ( -13.89961937509957401, -13.97604488694547875, 69.37609039468564731 ) ) ;
#121910=CARTESIAN_POINT ( 'NONE',  ( -9.474510206698720793, -16.51473224551083518, 59.58442372801900433 ) ) ;
#121911=CARTESIAN_POINT ( 'NONE',  ( -19.05341960407617563, 5.049401038297882671, 93.54275706135234714 ) ) ;
#121912=CARTESIAN_POINT ( 'NONE',  ( -0.05219959533934338120, 16.53943276465976808, 87.50109039468568994 ) ) ;
#121914=CARTESIAN_POINT ( 'NONE',  ( -19.02544592524342804, 5.153800228976336051, 31.04057627198102409 ) ) ;
#121915=CARTESIAN_POINT ( 'NONE',  ( -21.55341960407610458, -5.719274019375992779, 26.45724293864768839 ) ) ;
#121916=CARTESIAN_POINT ( 'NONE',  ( -15.72974639402176322, -15.80617190586768395, 44.37609039468567573 ) ) ;
#121917=CARTESIAN_POINT ( 'NONE',  ( 9.474510206698729675, 16.51473224551082808, 102.0844237280190043 ) ) ;
#121918=CARTESIAN_POINT ( 'NONE',  ( 17.50000000000000000, -3.565345528327946489, 106.9249448680647703 ) ) ;
#121919=CARTESIAN_POINT ( 'NONE',  ( -9.564922557960796823, -16.46253265017161027, 62.08224293864769550 ) ) ;
#121920=CARTESIAN_POINT ( 'NONE',  ( 9.564922557960805705, 16.46253265017160317, 99.58224293864770971 ) ) ;
#121921=CARTESIAN_POINT ( 'NONE',  ( -16.52544592524342804, 4.483927247898546575, 71.04057627198103830 ) ) ;
#121922=CARTESIAN_POINT ( 'NONE',  ( -19.05341960407611168, -5.049401038298163336, 61.45724293864769550 ) ) ;
#121923=CARTESIAN_POINT ( 'NONE',  ( -9.474510206698964154, 16.51473224551069663, 75.41557627198103830 ) ) ;
#121924=CARTESIAN_POINT ( 'NONE',  ( -19.03943276465977164, -0.05219959533935918106, 78.75109039468567573 ) ) ;
#121925=CARTESIAN_POINT ( 'NONE',  ( -10.81492255796078084, -18.62759615963271287, 47.08224293864770260 ) ) ;
#121926=CARTESIAN_POINT ( 'NONE',  ( 16.55341960407611168, 4.379528057220329451, 108.9572429386476955 ) ) ;
#121927=CARTESIAN_POINT ( 'NONE',  ( -19.02544592524334988, -5.153800228976617603, 38.95942372801900433 ) ) ;
#121928=CARTESIAN_POINT ( 'NONE',  ( 9.564922557960805705, 16.46253265017160317, 84.58224293864769550 ) ) ;
#121929=CARTESIAN_POINT ( 'NONE',  ( -0.05219959533907301413, -21.53943276465977519, 77.49890960531433848 ) ) ;
#121930=CARTESIAN_POINT ( 'NONE',  ( -4.379528057220328563, 16.55341960407611168, 85.20724293864770971 ) ) ;
#121931=CARTESIAN_POINT ( 'NONE',  ( -19.03943276465977164, -0.05219959533935918106, 48.75109039468566863 ) ) ;
#121932=CARTESIAN_POINT ( 'NONE',  ( 5.719274019375991003, -21.55341960407610458, 72.70724293864769550 ) ) ;
#121933=CARTESIAN_POINT ( 'NONE',  ( -21.52544592524343514, 5.823673210054127303, 56.04057627198102409 ) ) ;
#121934=CARTESIAN_POINT ( 'NONE',  ( -10.81492255796078084, -18.62759615963271287, 37.08224293864768129 ) ) ;
#121935=CARTESIAN_POINT ( 'NONE',  ( -5.823673210054431948, 21.52544592524334988, 97.70942372801904696 ) ) ;
#121936=CARTESIAN_POINT ( 'NONE',  ( -5.049401038298153566, 19.05341960407611168, 70.20724293864769550 ) ) ;
#121937=CARTESIAN_POINT ( 'NONE',  ( -0.05219959533910754901, -16.53943276465976808, 112.4989096053143669 ) ) ;
#121939=CARTESIAN_POINT ( 'NONE',  ( -5.719274019375665041, -21.55341960407619695, 19.79275706135235069 ) ) ;
#121941=CARTESIAN_POINT ( 'NONE',  ( 15.80617190586769283, -15.72974639402175789, 40.62609039468567573 ) ) ;
#121942=CARTESIAN_POINT ( 'NONE',  ( 19.02544592524343514, -5.153800228976328945, 28.54057627198102409 ) ) ;
#121943=CARTESIAN_POINT ( 'NONE',  ( 15.72974639402199770, -15.80617190586745480, 113.1239096053143953 ) ) ;
#121944=CARTESIAN_POINT ( 'NONE',  ( -5.153800228976607833, 19.02544592524334988, 52.70942372801900433 ) ) ;
#121945=CARTESIAN_POINT ( 'NONE',  ( -19.02544592524342804, 5.153800228976336051, 41.04057627198103120 ) ) ;
#121946=CARTESIAN_POINT ( 'NONE',  ( 16.46253265017160672, -9.564922557960803928, 23.33224293864769194 ) ) ;
#121947=DIRECTION ( 'NONE',  ( -0.000000000000000000, -0.000000000000000000, 1.000000000000000000 ) ) ;
#121948=CARTESIAN_POINT ( 'NONE',  ( -8.314922557961024197, 14.29746914071037800, 62.91775706135236135 ) ) ;
#121949=CARTESIAN_POINT ( 'NONE',  ( 9.474510206698971260, -16.51473224551069308, 32.91557627198102409 ) ) ;
#121951=CARTESIAN_POINT ( 'NONE',  ( -5.153800228976328057, -19.02544592524343514, 82.29057627198103830 ) ) ;
#121952=CARTESIAN_POINT ( 'NONE',  ( 8.224510206698953496, -14.34966873604960469, 102.9155762719810383 ) ) ;
#121953=CARTESIAN_POINT ( 'NONE',  ( 15.80617190586746368, 15.72974639402197994, 54.37390960531435979 ) ) ;
#121954=CARTESIAN_POINT ( 'NONE',  ( 14.34966873604972726, -8.224510206698740333, 50.83442372801901143 ) ) ;
#121955=CARTESIAN_POINT ( 'NONE',  ( -5.719274019375665041, -21.55341960407619695, 99.79275706135234714 ) ) ;
#121956=CARTESIAN_POINT ( 'NONE',  ( 13.97604488694527802, 13.89961937509977652, 39.37390960531435269 ) ) ;
#121957=CARTESIAN_POINT ( 'NONE',  ( 12.06949235617739724, 12.14591786802326823, 111.8760903946856615 ) ) ;
#121958=CARTESIAN_POINT ( 'NONE',  ( 12.14591786802309770, 12.06949235617756955, 54.37390960531435979 ) ) ;
#121959=CARTESIAN_POINT ( 'NONE',  ( 16.46253265017160672, -9.564922557960803928, 63.33224293864769550 ) ) ;
#121960=CARTESIAN_POINT ( 'NONE',  ( -21.53943276465977519, -0.05219959533937600094, 108.7510903946857042 ) ) ;
#121961=CARTESIAN_POINT ( 'NONE',  ( -5.719274019375978568, 21.55341960407610458, 115.2072429386476955 ) ) ;
#121962=CARTESIAN_POINT ( 'NONE',  ( 21.55341960407619695, -5.719274019375665929, 71.04275706135234714 ) ) ;
#121963=CARTESIAN_POINT ( 'NONE',  ( -14.34966873604972548, 8.224510206698743886, 53.33442372801901854 ) ) ;
#121964=CARTESIAN_POINT ( 'NONE',  ( -16.55341960407617563, 4.379528057220093196, 33.54275706135234714 ) ) ;
#121965=CARTESIAN_POINT ( 'NONE',  ( 14.29746914071049879, -8.314922557960816363, 78.33224293864770971 ) ) ;
#121966=CARTESIAN_POINT ( 'NONE',  ( -10.72451020669870658, -18.67979575497194134, 104.5844237280190185 ) ) ;
#121968=CARTESIAN_POINT ( 'NONE',  ( 4.379528057220339221, -16.55341960407611168, 37.70724293864769550 ) ) ;
#121969=CARTESIAN_POINT ( 'NONE',  ( -17.48847506799969054, 5.747544572773736427, 115.8269743784328654 ) ) ;
#121970=CARTESIAN_POINT ( 'NONE',  ( -14.34966873604972548, 8.224510206698743886, 43.33442372801901143 ) ) ;
#121971=CARTESIAN_POINT ( 'NONE',  ( -0.05219959533910754901, -16.53943276465976808, 52.49890960531435979 ) ) ;
#121972=CARTESIAN_POINT ( 'NONE',  ( 0.05219959533934541429, -16.53943276465976808, 85.00109039468568994 ) ) ;
#121973=CARTESIAN_POINT ( 'NONE',  ( 16.51473224551069308, 9.474510206698969483, 104.1655762719810241 ) ) ;
#121974=CARTESIAN_POINT ( 'NONE',  ( -0.05219959533909027116, -19.03943276465977164, 112.4989096053143669 ) ) ;
#121975=CARTESIAN_POINT ( 'NONE',  ( 5.719274019375673035, 21.55341960407619339, 97.29275706135234714 ) ) ;
#121977=CARTESIAN_POINT ( 'NONE',  ( 16.52544592524335698, 4.483927247898782831, 101.4594237280190185 ) ) ;
#121978=CARTESIAN_POINT ( 'NONE',  ( 14.29746914071049879, -8.314922557960816363, 93.33224293864769550 ) ) ;
#121979=CARTESIAN_POINT ( 'NONE',  ( 16.51473224551069308, 9.474510206698969483, 94.16557627198103830 ) ) ;
#121981=CARTESIAN_POINT ( 'NONE',  ( 16.55341960407618274, -4.379528057220086978, 41.04275706135236135 ) ) ;
#121983=CARTESIAN_POINT ( 'NONE',  ( 16.46253265017160672, -9.564922557960803928, 48.33224293864769550 ) ) ;
#121984=CARTESIAN_POINT ( 'NONE',  ( -19.02544592524342804, 5.153800228976336051, 111.0405762719810099 ) ) ;
#121985=CARTESIAN_POINT ( 'NONE',  ( -12.14591786802326823, 12.06949235617739902, 48.12609039468568284 ) ) ;
#121986=CARTESIAN_POINT ( 'NONE',  ( 17.60779699588839975, 5.500000000000013323, 68.84981316670106821 ) ) ;
#121987=CARTESIAN_POINT ( 'NONE',  ( 9.474510206698729675, 16.51473224551082808, 32.08442372801900433 ) ) ;
#121988=CARTESIAN_POINT ( 'NONE',  ( 19.03943276465977164, -0.05219959533909143690, 43.74890960531435979 ) ) ;
#121989=CARTESIAN_POINT ( 'NONE',  ( -16.53943276465976808, -0.05219959533934237506, 78.75109039468568994 ) ) ;
#121990=CARTESIAN_POINT ( 'NONE',  ( 16.46253265017146816, 9.564922557961045513, 76.66775706135234714 ) ) ;
#121991=CARTESIAN_POINT ( 'NONE',  ( -13.97604488694547697, 13.89961937509957934, 23.12609039468565442 ) ) ;
#121992=CARTESIAN_POINT ( 'NONE',  ( 5.153800228976335163, 19.02544592524342804, 54.79057627198103120 ) ) ;
#121994=CARTESIAN_POINT ( 'NONE',  ( -16.53943276465976808, 0.05219959533911058130, 96.24890960531435269 ) ) ;
#121995=CARTESIAN_POINT ( 'NONE',  ( -16.51473224551082808, 9.474510206698731452, 63.33442372801900433 ) ) ;
#121996=CARTESIAN_POINT ( 'NONE',  ( 10.72451020669898902, -18.67979575497178502, 62.91557627198102409 ) ) ;
#121997=CARTESIAN_POINT ( 'NONE',  ( 0.05219959533936267826, -19.03943276465977164, 30.00109039468566863 ) ) ;
#121998=CARTESIAN_POINT ( 'NONE',  ( 19.02544592524343514, -5.153800228976328945, 103.5405762719809957 ) ) ;
#121999=CARTESIAN_POINT ( 'NONE',  ( -21.55341960407610458, -5.719274019375992779, 71.45724293864769550 ) ) ;
#122000=CARTESIAN_POINT ( 'NONE',  ( 9.564922557960805705, 16.46253265017160317, 104.5822429386476955 ) ) ;
#122001=CARTESIAN_POINT ( 'NONE',  ( 0.05219959533936267826, -19.03943276465977164, 100.0010903946856757 ) ) ;
#122002=CARTESIAN_POINT ( 'NONE',  ( -16.46253265017160317, 9.564922557960807481, 110.8322429386476955 ) ) ;
#122003=CARTESIAN_POINT ( 'NONE',  ( -8.224510206698735004, -14.34966873604973081, 24.58442372801901499 ) ) ;
#122004=CARTESIAN_POINT ( 'NONE',  ( 13.89961937509977652, -13.97604488694527269, 38.12390960531436690 ) ) ;
#122005=CARTESIAN_POINT ( 'NONE',  ( 13.89961937509977652, -13.97604488694527269, 103.1239096053143527 ) ) ;
#122006=CARTESIAN_POINT ( 'NONE',  ( 15.72974639402199770, -15.80617190586745480, 88.12390960531436690 ) ) ;
#122007=CARTESIAN_POINT ( 'NONE',  ( -18.67979575497193778, 10.72451020669871902, 63.33442372801900433 ) ) ;
#122008=CARTESIAN_POINT ( 'NONE',  ( -9.564922557961040184, 16.46253265017147172, 107.9177570613523471 ) ) ;
#122009=CARTESIAN_POINT ( 'NONE',  ( -5.049401038297874678, -19.05341960407617918, 19.79275706135233293 ) ) ;
#122010=CARTESIAN_POINT ( 'NONE',  ( -16.52544592524335698, -4.483927247898792601, 108.9594237280190185 ) ) ;
#122011=CARTESIAN_POINT ( 'NONE',  ( -15.72974639402197994, 15.80617190586746368, 95.62390960531436690 ) ) ;
#122012=CARTESIAN_POINT ( 'NONE',  ( -4.379528057220328563, 16.55341960407611168, 30.20724293864769550 ) ) ;
#122013=CARTESIAN_POINT ( 'NONE',  ( 0.05219959533936267826, -19.03943276465977164, 80.00109039468567573 ) ) ;
#122014=CARTESIAN_POINT ( 'NONE',  ( -0.05219959533936034679, 19.03943276465977164, 57.50109039468566863 ) ) ;
#122015=CARTESIAN_POINT ( 'NONE',  ( -18.62759615963255300, -10.81492255796106328, 54.16775706135235424 ) ) ;
#122016=CARTESIAN_POINT ( 'NONE',  ( -13.89961937509957401, -13.97604488694547875, 39.37609039468566152 ) ) ;
#122017=CARTESIAN_POINT ( 'NONE',  ( 16.53943276465976808, -0.05219959533910856209, 103.7489096053143669 ) ) ;
#122018=CARTESIAN_POINT ( 'NONE',  ( 21.53943276465977519, -0.05219959533907433946, 33.74890960531436690 ) ) ;
#122019=CARTESIAN_POINT ( 'NONE',  ( -0.05219959533910754901, -16.53943276465976808, 42.49890960531435979 ) ) ;
#122020=CARTESIAN_POINT ( 'NONE',  ( -5.823673210054431948, 21.52544592524334988, 92.70942372801901854 ) ) ;
#122021=CARTESIAN_POINT ( 'NONE',  ( 4.483927247898790824, -16.52544592524335698, 70.20942372801904696 ) ) ;
#122022=CARTESIAN_POINT ( 'NONE',  ( -16.52544592524342804, 4.483927247898546575, 31.04057627198102409 ) ) ;
#122023=CARTESIAN_POINT ( 'NONE',  ( -10.81492255796105439, 18.62759615963255655, 67.91775706135234714 ) ) ;
#122024=CARTESIAN_POINT ( 'NONE',  ( 15.72974639402176855, 15.80617190586768217, 61.87609039468568284 ) ) ;
#122025=CARTESIAN_POINT ( 'NONE',  ( 21.52544592524344225, -5.823673210054117533, 63.54057627198103830 ) ) ;
#122027=CARTESIAN_POINT ( 'NONE',  ( 16.51473224551069308, 9.474510206698969483, 24.16557627198102765 ) ) ;
#122028=CARTESIAN_POINT ( 'NONE',  ( 15.80617190586769283, -15.72974639402175789, 45.62609039468567573 ) ) ;
#122029=CARTESIAN_POINT ( 'NONE',  ( 16.46253265017160672, -9.564922557960803928, 28.33224293864769550 ) ) ;
#122030=CARTESIAN_POINT ( 'NONE',  ( 13.97604488694527802, 13.89961937509977652, 44.37390960531435269 ) ) ;
#122031=CARTESIAN_POINT ( 'NONE',  ( 0.05219959533910956823, 16.53943276465976808, 74.99890960531435269 ) ) ;
#122032=CARTESIAN_POINT ( 'NONE',  ( 5.153800228976335163, 19.02544592524342804, 79.79057627198102409 ) ) ;
#122033=CARTESIAN_POINT ( 'NONE',  ( -12.14591786802309592, -12.06949235617757132, 26.87390960531435979 ) ) ;
#122034=CARTESIAN_POINT ( 'NONE',  ( 10.72451020669898902, -18.67979575497178502, 72.91557627198103830 ) ) ;
#122035=CARTESIAN_POINT ( 'NONE',  ( -0.05219959533907301413, -21.53943276465977519, 112.4989096053143669 ) ) ;
#122036=CARTESIAN_POINT ( 'NONE',  ( -16.51473224551069308, -9.474510206698971260, 101.6655762719810241 ) ) ;
#122037=CARTESIAN_POINT ( 'NONE',  ( 9.474510206698971260, -16.51473224551069308, 62.91557627198102409 ) ) ;
#122038=CARTESIAN_POINT ( 'NONE',  ( 16.46253265017146816, 9.564922557961045513, 101.6677570613523329 ) ) ;
#122039=CARTESIAN_POINT ( 'NONE',  ( 10.81492255796078972, 18.62759615963270932, 59.58224293864770260 ) ) ;
#122040=CARTESIAN_POINT ( 'NONE',  ( 15.80617190586769283, -15.72974639402175789, 75.62609039468567573 ) ) ;
#122041=CARTESIAN_POINT ( 'NONE',  ( -5.049401038298153566, 19.05341960407611168, 60.20724293864768129 ) ) ;
#122042=CARTESIAN_POINT ( 'NONE',  ( -0.05219959533909027116, -19.03943276465977164, 92.49890960531436690 ) ) ;
#122043=CARTESIAN_POINT ( 'NONE',  ( -12.14591786802326823, 12.06949235617739902, 83.12609039468568994 ) ) ;
#122044=CARTESIAN_POINT ( 'NONE',  ( 15.72974639402176855, 15.80617190586768217, 61.87609039468568284 ) ) ;
#122045=CARTESIAN_POINT ( 'NONE',  ( 10.72451020669871369, 18.67979575497193778, 82.08442372801901854 ) ) ;
#122046=CARTESIAN_POINT ( 'NONE',  ( -21.53943276465977519, -0.05219959533937600094, 18.75109039468568639 ) ) ;
#122047=CARTESIAN_POINT ( 'NONE',  ( -21.53943276465977519, 0.05219959533907696930, 71.24890960531435269 ) ) ;
#122048=CARTESIAN_POINT ( 'NONE',  ( -5.049401038297874678, -19.05341960407617918, 49.79275706135231871 ) ) ;
#122049=CARTESIAN_POINT ( 'NONE',  ( 21.55341960407610458, 5.719274019375980345, 43.95724293864769550 ) ) ;
#122050=CARTESIAN_POINT ( 'NONE',  ( 16.46253265017160672, -9.564922557960803928, 78.33224293864769550 ) ) ;
#122051=CARTESIAN_POINT ( 'NONE',  ( 12.14591786802309770, 12.06949235617756955, 39.37390960531436690 ) ) ;
#122052=CARTESIAN_POINT ( 'NONE',  ( -17.05116617787826883, 6.768360034955676952, 63.65675553259197983 ) ) ;
#122053=CARTESIAN_POINT ( 'NONE',  ( -21.53943276465977519, 0.05219959533907696930, 26.24890960531435624 ) ) ;
#122054=CARTESIAN_POINT ( 'NONE',  ( -18.22780087662123094, -5.499999999999984901, 81.48459894673892734 ) ) ;
#122055=CARTESIAN_POINT ( 'NONE',  ( -5.049401038297874678, -19.05341960407617918, 89.79275706135230450 ) ) ;
#122056=CARTESIAN_POINT ( 'NONE',  ( 21.53943276465977519, -0.05219959533907433946, 73.74890960531433848 ) ) ;
#122057=CARTESIAN_POINT ( 'NONE',  ( 16.55341960407611168, 4.379528057220329451, 53.95724293864770260 ) ) ;
#122058=CARTESIAN_POINT ( 'NONE',  ( -4.483927247898782831, 16.52544592524335698, 22.70942372801901499 ) ) ;
#122059=CARTESIAN_POINT ( 'NONE',  ( 0.05219959533909260263, 19.03943276465977164, 49.99890960531435979 ) ) ;
#122060=CARTESIAN_POINT ( 'NONE',  ( -18.62759615963270932, 10.81492255796079327, 105.8322429386476955 ) ) ;
#122061=CARTESIAN_POINT ( 'NONE',  ( 19.05341960407617918, -5.049401038297876454, 66.04275706135233293 ) ) ;
#122062=CARTESIAN_POINT ( 'NONE',  ( -19.05341960407611168, -5.049401038298163336, 81.45724293864769550 ) ) ;
#122063=CARTESIAN_POINT ( 'NONE',  ( 14.34966873604960469, 8.224510206698951720, 89.16557627198102409 ) ) ;
#122064=CARTESIAN_POINT ( 'NONE',  ( 13.89961937509977652, -13.97604488694527269, 58.12390960531436690 ) ) ;
#122065=CARTESIAN_POINT ( 'NONE',  ( -16.52544592524342804, 4.483927247898546575, 71.04057627198103830 ) ) ;
#122066=CARTESIAN_POINT ( 'NONE',  ( -13.89961937509977652, 13.97604488694528158, 35.62390960531435269 ) ) ;
#122067=CARTESIAN_POINT ( 'NONE',  ( -17.04537478617065815, -5.419303508143405779, 20.72959544958357725 ) ) ;
#122068=CARTESIAN_POINT ( 'NONE',  ( -14.29746914071049879, 8.314922557960819915, 45.83224293864769550 ) ) ;
#122069=CARTESIAN_POINT ( 'NONE',  ( 5.153800228976335163, 19.02544592524342804, 84.79057627198099567 ) ) ;
#122071=CARTESIAN_POINT ( 'NONE',  ( 5.153800228976615827, -19.02544592524334988, 50.20942372801897591 ) ) ;
#122072=CARTESIAN_POINT ( 'NONE',  ( 12.06949235617739724, 12.14591786802326823, 56.87609039468568994 ) ) ;
#122073=CARTESIAN_POINT ( 'NONE',  ( 18.67979575497178502, 10.72451020669898547, 79.16557627198103830 ) ) ;
#122074=CARTESIAN_POINT ( 'NONE',  ( 19.02544592524334988, 5.153800228976608722, 41.45942372801900433 ) ) ;
#122075=CARTESIAN_POINT ( 'NONE',  ( -0.05219959533909027116, -19.03943276465977164, 82.49890960531436690 ) ) ;
#122077=CARTESIAN_POINT ( 'NONE',  ( 10.81492255796078972, 18.62759615963270932, 34.58224293864770260 ) ) ;
#122078=VECTOR ( 'NONE', #67829, 1000.000000000000000 ) ;
#122079=CARTESIAN_POINT ( 'NONE',  ( 5.049401038298161559, -19.05341960407611168, 57.70724293864769550 ) ) ;
#122080=CARTESIAN_POINT ( 'NONE',  ( -15.72974639402176322, -15.80617190586768395, 49.37609039468569705 ) ) ;
#122081=CARTESIAN_POINT ( 'NONE',  ( -16.51473224551069308, -9.474510206698971260, 26.66557627198103120 ) ) ;
#122082=CARTESIAN_POINT ( 'NONE',  ( 5.823673210054444382, -21.52544592524334988, 20.20942372801900788 ) ) ;
#122083=CARTESIAN_POINT ( 'NONE',  ( -9.474510206698964154, 16.51473224551069663, 95.41557627198102409 ) ) ;
#122085=CARTESIAN_POINT ( 'NONE',  ( 21.53943276465977519, 0.05219959533937863772, 36.25109039468567573 ) ) ;
#122087=CARTESIAN_POINT ( 'NONE',  ( 5.153800228976335163, 19.02544592524342804, 104.7905762719809957 ) ) ;
#122089=CARTESIAN_POINT ( 'NONE',  ( -15.80617190586745835, -15.72974639402198527, 106.8739096053143811 ) ) ;
#122090=CARTESIAN_POINT ( 'NONE',  ( -5.153800228976328057, -19.02544592524343514, 42.29057627198101699 ) ) ;
#122091=CARTESIAN_POINT ( 'NONE',  ( 12.06949235617739724, 12.14591786802326823, 21.87609039468567573 ) ) ;
#122093=CARTESIAN_POINT ( 'NONE',  ( -19.05341960407611168, -5.049401038298163336, 26.45724293864769550 ) ) ;
#122094=CARTESIAN_POINT ( 'NONE',  ( 15.72974639402176855, 15.80617190586768217, 96.87609039468568994 ) ) ;
#122095=CARTESIAN_POINT ( 'NONE',  ( -13.89961937509977652, 13.97604488694528158, 80.62390960531436690 ) ) ;
#122096=CARTESIAN_POINT ( 'NONE',  ( -21.55341960407619339, 5.719274019375674811, 58.54275706135235424 ) ) ;
#122098=CARTESIAN_POINT ( 'NONE',  ( -19.02544592524342804, 5.153800228976336051, 96.04057627198103830 ) ) ;
#122099=B_SPLINE_CURVE_WITH_KNOTS ( 'NONE', 3,
 ( #97963, #23159, #40317, #129309, #68646, #175841, #176853, #145486, #128319, #22155, #85819, #163675, #159655, #7972, #132331, #177850, #54488, #130302, #116160, #53482 ),
 .UNSPECIFIED., .F., .F.,
 ( 4, 2, 2, 2, 2, 2, 2, 2, 2, 4 ),
 ( 0.004000878361811996409, 0.004499404418915992424, 0.004997930476019988438, 0.005496456533123985320, 0.005994982590227981335, 0.006244245618779979343, 0.006493508647331977350, 0.006992034704435974232, 0.007490560761539970247, 0.007989086818643966262 ),
 .UNSPECIFIED. ) ;
#122101=CARTESIAN_POINT ( 'NONE',  ( 8.224510206698742110, 14.34966873604972548, 42.08442372801901854 ) ) ;
#122102=CARTESIAN_POINT ( 'NONE',  ( -12.06949235617739369, -12.14591786802326823, 74.37609039468568994 ) ) ;
#122103=CARTESIAN_POINT ( 'NONE',  ( -10.72451020669870658, -18.67979575497194134, 64.58442372801900433 ) ) ;
#122104=CARTESIAN_POINT ( 'NONE',  ( -18.62759615963255300, -10.81492255796106328, 89.16775706135236135 ) ) ;
#122106=CARTESIAN_POINT ( 'NONE',  ( 13.97604488694548053, -13.89961937509957401, 105.6260903946856757 ) ) ;
#122107=CARTESIAN_POINT ( 'NONE',  ( 0.05219959533909260263, 19.03943276465977164, 69.99890960531435269 ) ) ;
#122108=CARTESIAN_POINT ( 'NONE',  ( -0.05219959533909027116, -19.03943276465977164, 92.49890960531436690 ) ) ;
#122110=CARTESIAN_POINT ( 'NONE',  ( 5.049401038298161559, -19.05341960407611168, 27.70724293864769550 ) ) ;
#122111=CARTESIAN_POINT ( 'NONE',  ( 15.72974639402199770, -15.80617190586745480, 23.12390960531436335 ) ) ;
#122112=CARTESIAN_POINT ( 'NONE',  ( -4.379528057220086978, -16.55341960407618274, 94.79275706135234714 ) ) ;
#122113=CARTESIAN_POINT ( 'NONE',  ( 16.55341960407611168, 4.379528057220329451, 63.95724293864770260 ) ) ;
#122114=CARTESIAN_POINT ( 'NONE',  ( -13.89961937509977652, 13.97604488694528158, 55.62390960531434558 ) ) ;
#122115=CARTESIAN_POINT ( 'NONE',  ( 15.80617190586769283, -15.72974639402175789, 95.62609039468568994 ) ) ;
#122117=CARTESIAN_POINT ( 'NONE',  ( 19.03943276465977164, 0.05219959533936151252, 111.2510903946856757 ) ) ;
#122118=CARTESIAN_POINT ( 'NONE',  ( -16.52544592524342804, 4.483927247898546575, 76.04057627198102409 ) ) ;
#122119=CARTESIAN_POINT ( 'NONE',  ( -21.53943276465977519, -0.05219959533937600094, 28.75109039468567929 ) ) ;
#122120=CARTESIAN_POINT ( 'NONE',  ( 15.80617190586746368, 15.72974639402197994, 59.37390960531436690 ) ) ;
#122121=CARTESIAN_POINT ( 'NONE',  ( 9.474510206698729675, 16.51473224551082808, 37.08442372801899722 ) ) ;
#122123=CARTESIAN_POINT ( 'NONE',  ( -19.02544592524342804, 5.153800228976336051, 86.04057627198103830 ) ) ;
#122124=CARTESIAN_POINT ( 'NONE',  ( -16.55341960407611168, -4.379528057220339221, 56.45724293864768839 ) ) ;
#122125=CARTESIAN_POINT ( 'NONE',  ( 14.29746914071049879, -8.314922557960816363, 38.33224293864768839 ) ) ;
#122126=CARTESIAN_POINT ( 'NONE',  ( 12.06949235617739724, 12.14591786802326823, 101.8760903946857042 ) ) ;
#122127=CARTESIAN_POINT ( 'NONE',  ( -19.05341960407617563, 5.049401038297882671, 48.54275706135233293 ) ) ;
#122128=B_SPLINE_CURVE_WITH_KNOTS ( 'NONE', 3,
 ( #153192, #92511, #199716, #76358, #156180, #75366, #198727, #60193, #498, #48022, #138035, #93506, #32848, #79337, #123834, #2495, #122854, #184542, #107678, #169355 ),
 .UNSPECIFIED., .F., .F.,
 ( 4, 2, 2, 2, 2, 2, 2, 2, 2, 4 ),
 ( 0.000000000000000000, 0.0004987090165372409355, 0.0009974180330744818711, 0.001246772541343112856, 0.001496127049611744274, 0.001994836066149007110, 0.002493545082686269513, 0.002742899590954893559, 0.002992254099223517604, 0.003989672132298028098 ),
 .UNSPECIFIED. ) ;
#122130=CARTESIAN_POINT ( 'NONE',  ( 16.46253265017160672, -9.564922557960803928, 108.3322429386476955 ) ) ;
#122131=CARTESIAN_POINT ( 'NONE',  ( 14.29746914071049879, -8.314922557960816363, 73.33224293864769550 ) ) ;
#122132=CARTESIAN_POINT ( 'NONE',  ( 19.05341960407617918, -5.049401038297876454, 41.04275706135233293 ) ) ;
#122133=CARTESIAN_POINT ( 'NONE',  ( -13.89961937509977652, 13.97604488694528158, 35.62390960531435269 ) ) ;
#122134=CARTESIAN_POINT ( 'NONE',  ( 15.80617190586746368, 15.72974639402197994, 34.37390960531435979 ) ) ;
#122135=CARTESIAN_POINT ( 'NONE',  ( 15.80617190586746368, 15.72974639402197994, 64.37390960531435269 ) ) ;
#122136=CARTESIAN_POINT ( 'NONE',  ( 8.314922557960818139, 14.29746914071049879, 114.5822429386477097 ) ) ;
#122137=CARTESIAN_POINT ( 'NONE',  ( -4.483927247898782831, 16.52544592524335698, 57.70942372801901143 ) ) ;
#122138=CARTESIAN_POINT ( 'NONE',  ( -5.719274019375665041, -21.55341960407619695, 39.79275706135235424 ) ) ;
#122139=CARTESIAN_POINT ( 'NONE',  ( 4.483927247898545687, 16.52544592524342804, 94.79057627198105251 ) ) ;
#122140=DIRECTION ( 'NONE',  ( 0.000000000000000000, 0.000000000000000000, -1.000000000000000000 ) ) ;
#122141=CARTESIAN_POINT ( 'NONE',  ( -16.62475595723696031, 7.163666690055234376, 50.52713351810466946 ) ) ;
#122142=CARTESIAN_POINT ( 'NONE',  ( -15.72974639402197994, 15.80617190586746368, 35.62390960531437401 ) ) ;
#122143=LINE ( 'NONE', #184820, #91357 ) ;
#122145=CARTESIAN_POINT ( 'NONE',  ( 12.06949235617739724, 12.14591786802326823, 41.87609039468568284 ) ) ;
#122146=CARTESIAN_POINT ( 'NONE',  ( 14.29746914071049879, -8.314922557960816363, 38.33224293864768839 ) ) ;
#122147=CARTESIAN_POINT ( 'NONE',  ( -5.823673210054116645, -21.52544592524344225, 72.29057627198102409 ) ) ;
#122148=CARTESIAN_POINT ( 'NONE',  ( -9.564922557961040184, 16.46253265017147172, 82.91775706135233293 ) ) ;
#122149=CARTESIAN_POINT ( 'NONE',  ( 10.72451020669898902, -18.67979575497178502, 62.91557627198102409 ) ) ;
#122151=CARTESIAN_POINT ( 'NONE',  ( 19.03943276465977164, -0.05219959533909143690, 38.74890960531436690 ) ) ;
#122152=CARTESIAN_POINT ( 'NONE',  ( 13.89961937509977652, -13.97604488694527269, 103.1239096053143527 ) ) ;
#122153=CARTESIAN_POINT ( 'NONE',  ( 19.05341960407611168, 5.049401038298154454, 43.95724293864769550 ) ) ;
#122154=CARTESIAN_POINT ( 'NONE',  ( 4.483927247898545687, 16.52544592524342804, 114.7905762719810383 ) ) ;
#122156=CARTESIAN_POINT ( 'NONE',  ( 19.05341960407611168, 5.049401038298154454, 113.9572429386477097 ) ) ;
#122158=CARTESIAN_POINT ( 'NONE',  ( 4.483927247898790824, -16.52544592524335698, 70.20942372801904696 ) ) ;
#122159=CARTESIAN_POINT ( 'NONE',  ( 15.80617190586746368, 15.72974639402197994, 109.3739096053143811 ) ) ;
#122160=CARTESIAN_POINT ( 'NONE',  ( 16.51473224551069308, 9.474510206698969483, 54.16557627198103120 ) ) ;
#122161=CARTESIAN_POINT ( 'NONE',  ( -15.80617190586768217, 15.72974639402176855, 28.12609039468568284 ) ) ;
#122162=CARTESIAN_POINT ( 'NONE',  ( 16.51473224551069308, 9.474510206698969483, 89.16557627198103830 ) ) ;
#122165=CARTESIAN_POINT ( 'NONE',  ( -10.81492255796105439, 18.62759615963255655, 27.91775706135234358 ) ) ;
#122166=CARTESIAN_POINT ( 'NONE',  ( 19.03943276465977164, -0.05219959533909143690, 23.74890960531435269 ) ) ;
#122167=CARTESIAN_POINT ( 'NONE',  ( 13.97604488694527802, 13.89961937509977652, 104.3739096053143385 ) ) ;
#122168=CARTESIAN_POINT ( 'NONE',  ( 9.474510206698729675, 16.51473224551082808, 82.08442372801899012 ) ) ;
#122169=CARTESIAN_POINT ( 'NONE',  ( 19.05341960407617918, -5.049401038297876454, 36.04275706135234003 ) ) ;
#122170=CARTESIAN_POINT ( 'NONE',  ( 21.55341960407610458, 5.719274019375980345, 103.9572429386476813 ) ) ;
#122171=CARTESIAN_POINT ( 'NONE',  ( -9.564922557961040184, 16.46253265017147172, 32.91775706135233293 ) ) ;
#122172=CARTESIAN_POINT ( 'NONE',  ( 13.97604488694548053, -13.89961937509957401, 40.62609039468564731 ) ) ;
#122173=CARTESIAN_POINT ( 'NONE',  ( -16.53943276465976808, -0.05219959533934237506, 88.75109039468567573 ) ) ;
#122174=CARTESIAN_POINT ( 'NONE',  ( -16.51473224551069308, -9.474510206698971260, 106.6655762719810383 ) ) ;
#122175=CARTESIAN_POINT ( 'NONE',  ( 0.05219959533909260263, 19.03943276465977164, 64.99890960531436690 ) ) ;
#122176=CARTESIAN_POINT ( 'NONE',  ( -5.823673210054431948, 21.52544592524334988, 62.70942372801902565 ) ) ;
#122177=CARTESIAN_POINT ( 'NONE',  ( 18.62759615963255655, 10.81492255796105972, 86.66775706135234714 ) ) ;
#122178=CARTESIAN_POINT ( 'NONE',  ( -5.049401038298153566, 19.05341960407611168, 115.2072429386477097 ) ) ;
#122179=CARTESIAN_POINT ( 'NONE',  ( -19.03943276465977164, 0.05219959533909376836, 81.24890960531436690 ) ) ;
#122180=CARTESIAN_POINT ( 'NONE',  ( -10.81492255796105439, 18.62759615963255655, 52.91775706135235424 ) ) ;
#122181=CARTESIAN_POINT ( 'NONE',  ( -16.46253265017146816, -9.564922557961047289, 99.16775706135233293 ) ) ;
#122182=CARTESIAN_POINT ( 'NONE',  ( -5.153800228976328057, -19.02544592524343514, 52.29057627198100988 ) ) ;
#122183=CARTESIAN_POINT ( 'NONE',  ( -5.153800228976328057, -19.02544592524343514, 97.29057627198099567 ) ) ;
#122184=CARTESIAN_POINT ( 'NONE',  ( 0.05219959533909260263, 19.03943276465977164, 79.99890960531436690 ) ) ;
#122186=CARTESIAN_POINT ( 'NONE',  ( -5.049401038298153566, 19.05341960407611168, 70.20724293864769550 ) ) ;
#122187=CARTESIAN_POINT ( 'NONE',  ( 21.53943276465977519, -0.05219959533907433946, 98.74890960531438111 ) ) ;
#122188=CARTESIAN_POINT ( 'NONE',  ( 4.483927247898790824, -16.52544592524335698, 85.20942372801901854 ) ) ;
#122190=CARTESIAN_POINT ( 'NONE',  ( 0.05219959533936267826, -19.03943276465977164, 45.00109039468566863 ) ) ;
#122191=CARTESIAN_POINT ( 'NONE',  ( 19.03943276465977164, -0.05219959533909143690, 73.74890960531435269 ) ) ;
#122192=CARTESIAN_POINT ( 'NONE',  ( 16.52544592524342804, -4.483927247898539470, 73.54057627198102409 ) ) ;
#122193=CARTESIAN_POINT ( 'NONE',  ( 8.314922557960818139, 14.29746914071049879, 99.58224293864770971 ) ) ;
#122194=CARTESIAN_POINT ( 'NONE',  ( -15.80617190586745835, -15.72974639402198527, 21.87390960531436690 ) ) ;
#122195=CARTESIAN_POINT ( 'NONE',  ( -19.05341960407611168, -5.049401038298163336, 101.4572429386476955 ) ) ;
#122196=CARTESIAN_POINT ( 'NONE',  ( -13.89961937509977652, 13.97604488694528158, 115.6239096053143669 ) ) ;
#122197=CARTESIAN_POINT ( 'NONE',  ( -0.05219959533936034679, 19.03943276465977164, 37.50109039468567573 ) ) ;
#122198=CARTESIAN_POINT ( 'NONE',  ( 14.29746914071037800, 8.314922557961029526, 96.66775706135234714 ) ) ;
#122199=CARTESIAN_POINT ( 'NONE',  ( -16.51473224551069308, -9.474510206698971260, 81.66557627198103830 ) ) ;
#122200=CARTESIAN_POINT ( 'NONE',  ( 15.80617190586769283, -15.72974639402175789, 55.62609039468568284 ) ) ;
#122201=CARTESIAN_POINT ( 'NONE',  ( -18.62759615963270932, 10.81492255796079327, 35.83224293864768839 ) ) ;
#122202=CARTESIAN_POINT ( 'NONE',  ( 10.81492255796106328, -18.62759615963255655, 20.41775706135234714 ) ) ;
#122203=CARTESIAN_POINT ( 'NONE',  ( -15.80617190586745835, -15.72974639402198527, 71.87390960531438111 ) ) ;
#122204=CARTESIAN_POINT ( 'NONE',  ( 8.314922557960818139, 14.29746914071049879, 99.58224293864770971 ) ) ;
#122205=CARTESIAN_POINT ( 'NONE',  ( 16.51473224551083163, -9.474510206698727899, 60.83442372801900433 ) ) ;
#122206=ADVANCED_FACE ( 'NONE', ( #192474 ), #41795, .T. ) ;
#122207=CARTESIAN_POINT ( 'NONE',  ( -0.05219959533909027116, -19.03943276465977164, 37.49890960531436690 ) ) ;
#122208=CARTESIAN_POINT ( 'NONE',  ( 13.97604488694527802, 13.89961937509977652, 89.37390960531436690 ) ) ;
#122209=CARTESIAN_POINT ( 'NONE',  ( 16.51473224551069308, 9.474510206698969483, 79.16557627198103830 ) ) ;
#122211=CARTESIAN_POINT ( 'NONE',  ( -4.483927247898539470, -16.52544592524342804, 97.29057627198105251 ) ) ;
#122212=ORIENTED_EDGE ( 'NONE', *, *, #122826, .T. ) ;
#122213=CARTESIAN_POINT ( 'NONE',  ( -0.05219959533910754901, -16.53943276465976808, 22.49890960531436335 ) ) ;
#122214=CARTESIAN_POINT ( 'NONE',  ( -12.14591786802326823, 12.06949235617739902, 23.12609039468567573 ) ) ;
#122215=CARTESIAN_POINT ( 'NONE',  ( -15.80617190586768217, 15.72974639402176855, 88.12609039468570415 ) ) ;
#122216=CARTESIAN_POINT ( 'NONE',  ( 13.97604488694527802, 13.89961937509977652, 99.37390960531436690 ) ) ;
#122217=CARTESIAN_POINT ( 'NONE',  ( -10.81492255796078084, -18.62759615963271287, 112.0822429386477097 ) ) ;
#122218=CARTESIAN_POINT ( 'NONE',  ( 13.97604488694527802, 13.89961937509977652, 49.37390960531434558 ) ) ;
#122219=CARTESIAN_POINT ( 'NONE',  ( 14.29746914071037800, 8.314922557961029526, 46.66775706135234714 ) ) ;
#122220=CARTESIAN_POINT ( 'NONE',  ( -5.153800228976607833, 19.02544592524334988, 107.7094237280189759 ) ) ;
#122221=CARTESIAN_POINT ( 'NONE',  ( -4.379528057220328563, 16.55341960407611168, 95.20724293864769550 ) ) ;
#122222=CARTESIAN_POINT ( 'NONE',  ( -21.53943276465977519, 0.05219959533907696930, 106.2489096053143811 ) ) ;
#122223=CARTESIAN_POINT ( 'NONE',  ( -9.474510206698720793, -16.51473224551083518, 74.58442372801900433 ) ) ;
#122225=CARTESIAN_POINT ( 'NONE',  ( -15.80617190586745835, -15.72974639402198527, 111.8739096053143669 ) ) ;
#122227=CARTESIAN_POINT ( 'NONE',  ( 0.05219959533909260263, 19.03943276465977164, 84.99890960531436690 ) ) ;
#122228=CARTESIAN_POINT ( 'NONE',  ( 17.49999999999999645, -5.622605283950884214, 111.1879268940389096 ) ) ;
#122229=CARTESIAN_POINT ( 'NONE',  ( 9.564922557960805705, 16.46253265017160317, 79.58224293864769550 ) ) ;
#122230=CARTESIAN_POINT ( 'NONE',  ( 18.67979575497194134, -10.72451020669871369, 30.83442372801902209 ) ) ;
#122231=CARTESIAN_POINT ( 'NONE',  ( -12.14591786802309592, -12.06949235617757132, 71.87390960531438111 ) ) ;
#122232=CARTESIAN_POINT ( 'NONE',  ( 16.46253265017160672, -9.564922557960803928, 88.33224293864769550 ) ) ;
#122233=CARTESIAN_POINT ( 'NONE',  ( -8.224510206698735004, -14.34966873604973081, 49.58442372801901143 ) ) ;
#122234=CARTESIAN_POINT ( 'NONE',  ( 5.153800228976615827, -19.02544592524334988, 50.20942372801897591 ) ) ;
#122235=CARTESIAN_POINT ( 'NONE',  ( 15.80617190586769283, -15.72974639402175789, 60.62609039468567573 ) ) ;
#122236=AXIS2_PLACEMENT_3D ( 'NONE', #95201, #114345, #110369 ) ;
#122237=CARTESIAN_POINT ( 'NONE',  ( -12.06949235617739369, -12.14591786802326823, 24.37609039468567573 ) ) ;
#122238=CARTESIAN_POINT ( 'NONE',  ( 5.153800228976335163, 19.02544592524342804, 64.79057627198100988 ) ) ;
#122239=CARTESIAN_POINT ( 'NONE',  ( 9.474510206698729675, 16.51473224551082808, 97.08442372801900433 ) ) ;
#122240=CARTESIAN_POINT ( 'NONE',  ( -8.224510206698735004, -14.34966873604973081, 54.58442372801901143 ) ) ;
#122241=CARTESIAN_POINT ( 'NONE',  ( 5.719274019375673035, 21.55341960407619339, 102.2927570613523613 ) ) ;
#122242=CARTESIAN_POINT ( 'NONE',  ( -19.05341960407617563, 5.049401038297882671, 78.54275706135233293 ) ) ;
#122243=CARTESIAN_POINT ( 'NONE',  ( -0.05219959533909027116, -19.03943276465977164, 47.49890960531435979 ) ) ;
#122244=CARTESIAN_POINT ( 'NONE',  ( -21.55341960407610458, -5.719274019375992779, 76.45724293864769550 ) ) ;
#122245=CARTESIAN_POINT ( 'NONE',  ( -16.52544592524342804, 4.483927247898546575, 81.04057627198102409 ) ) ;
#122246=CARTESIAN_POINT ( 'NONE',  ( -19.02544592524334988, -5.153800228976617603, 73.95942372801900433 ) ) ;
#122247=CARTESIAN_POINT ( 'NONE',  ( -19.49190055781011566, -5.499999999999970690, 70.56116087098779133 ) ) ;
#122248=CARTESIAN_POINT ( 'NONE',  ( -19.03943276465977164, -0.05219959533935918106, 38.75109039468566152 ) ) ;
#122249=CARTESIAN_POINT ( 'NONE',  ( 4.483927247898545687, 16.52544592524342804, 24.79057627198103120 ) ) ;
#122250=CARTESIAN_POINT ( 'NONE',  ( -16.55341960407611168, -4.379528057220339221, 71.45724293864769550 ) ) ;
#122251=CARTESIAN_POINT ( 'NONE',  ( 21.55341960407619695, -5.719274019375665929, 96.04275706135236135 ) ) ;
#122253=CARTESIAN_POINT ( 'NONE',  ( 10.81492255796078972, 18.62759615963270932, 109.5822429386476955 ) ) ;
#122254=CARTESIAN_POINT ( 'NONE',  ( -19.03943276465977164, 0.05219959533909376836, 66.24890960531436690 ) ) ;
#122255=CARTESIAN_POINT ( 'NONE',  ( -0.05219959533937732626, 21.53943276465977519, 87.50109039468568994 ) ) ;
#122256=CARTESIAN_POINT ( 'NONE',  ( -13.97604488694527625, -13.89961937509977652, 66.87390960531436690 ) ) ;
#122258=CARTESIAN_POINT ( 'NONE',  ( -12.06949235617756955, 12.14591786802309770, 115.6239096053143669 ) ) ;
#122259=CARTESIAN_POINT ( 'NONE',  ( 18.62759615963271287, -10.81492255796078972, 28.33224293864769550 ) ) ;
#122260=CARTESIAN_POINT ( 'NONE',  ( 14.34966873604960469, 8.224510206698951720, 64.16557627198102409 ) ) ;
#122261=CARTESIAN_POINT ( 'NONE',  ( -5.049401038298153566, 19.05341960407611168, 50.20724293864770260 ) ) ;
#122262=CARTESIAN_POINT ( 'NONE',  ( -14.34966873604960291, -8.224510206698953496, 86.66557627198102409 ) ) ;
#122263=CARTESIAN_POINT ( 'NONE',  ( 18.67979575497178502, 10.72451020669898547, 114.1655762719810383 ) ) ;
#122264=CARTESIAN_POINT ( 'NONE',  ( -18.62759615963255300, -10.81492255796106328, 54.16775706135235424 ) ) ;
#122265=CARTESIAN_POINT ( 'NONE',  ( 0.05219959533909260263, 19.03943276465977164, 29.99890960531435979 ) ) ;
#122266=CARTESIAN_POINT ( 'NONE',  ( 16.52544592524335698, 4.483927247898782831, 51.45942372801901854 ) ) ;
#122267=CARTESIAN_POINT ( 'NONE',  ( 15.80617190586746368, 15.72974639402197994, 104.3739096053143669 ) ) ;
#122268=CARTESIAN_POINT ( 'NONE',  ( -0.05219959533907301413, -21.53943276465977519, 92.49890960531436690 ) ) ;
#122269=CARTESIAN_POINT ( 'NONE',  ( -9.564922557961040184, 16.46253265017147172, 27.91775706135232582 ) ) ;
#122270=CARTESIAN_POINT ( 'NONE',  ( -5.153800228976328057, -19.02544592524343514, 52.29057627198100988 ) ) ;
#122271=CARTESIAN_POINT ( 'NONE',  ( 16.51473224551069308, 9.474510206698969483, 104.1655762719810241 ) ) ;
#122272=CARTESIAN_POINT ( 'NONE',  ( -18.67979575497193778, 10.72451020669871902, 58.33442372801901143 ) ) ;
#122273=CARTESIAN_POINT ( 'NONE',  ( -21.55341960407610458, -5.719274019375992779, 41.45724293864769550 ) ) ;
#122274=CARTESIAN_POINT ( 'NONE',  ( 12.06949235617757843, -12.14591786802309237, 23.12390960531436335 ) ) ;
#122275=CARTESIAN_POINT ( 'NONE',  ( -0.05219959533937732626, 21.53943276465977519, 57.50109039468568994 ) ) ;
#122276=CARTESIAN_POINT ( 'NONE',  ( -15.80617190586768217, 15.72974639402176855, 98.12609039468570415 ) ) ;
#122277=CARTESIAN_POINT ( 'NONE',  ( 19.05341960407617918, -5.049401038297876454, 51.04275706135231871 ) ) ;
#122278=CARTESIAN_POINT ( 'NONE',  ( 0.05219959533934541429, -16.53943276465976808, 100.0010903946857042 ) ) ;
#122279=CARTESIAN_POINT ( 'NONE',  ( 0.05219959533937995610, -21.53943276465977519, 55.00109039468568284 ) ) ;
#122280=CARTESIAN_POINT ( 'NONE',  ( -19.03943276465977164, 0.05219959533909376836, 41.24890960531435269 ) ) ;
#122281=CARTESIAN_POINT ( 'NONE',  ( -21.55341960407619339, 5.719274019375674811, 113.5427570613523756 ) ) ;
#122282=CARTESIAN_POINT ( 'NONE',  ( 21.53943276465977519, -0.05219959533907433946, 23.74890960531435269 ) ) ;
#122283=CARTESIAN_POINT ( 'NONE',  ( 18.62759615963271287, -10.81492255796078972, 113.3322429386476955 ) ) ;
#122284=CARTESIAN_POINT ( 'NONE',  ( -18.62759615963270932, 10.81492255796079327, 75.83224293864769550 ) ) ;
#122285=CARTESIAN_POINT ( 'NONE',  ( -8.314922557961024197, 14.29746914071037800, 37.91775706135235424 ) ) ;
#122287=CARTESIAN_POINT ( 'NONE',  ( 15.80617190586746368, 15.72974639402197994, 84.37390960531438111 ) ) ;
#122288=CARTESIAN_POINT ( 'NONE',  ( -16.55341960407617563, 4.379528057220093196, 63.54275706135234003 ) ) ;
#122289=CARTESIAN_POINT ( 'NONE',  ( -12.14591786802309592, -12.06949235617757132, 76.87390960531439532 ) ) ;
#122291=CARTESIAN_POINT ( 'NONE',  ( 16.51473224551083163, -9.474510206698727899, 105.8344237280190043 ) ) ;
#122292=CARTESIAN_POINT ( 'NONE',  ( -21.53943276465977519, 0.05219959533907696930, 31.24890960531435979 ) ) ;
#122294=CARTESIAN_POINT ( 'NONE',  ( -4.483927247898782831, 16.52544592524335698, 42.70942372801901854 ) ) ;
#122295=CARTESIAN_POINT ( 'NONE',  ( 15.80617190586769283, -15.72974639402175789, 20.62609039468568639 ) ) ;
#122296=CARTESIAN_POINT ( 'NONE',  ( 21.53943276465977519, -0.05219959533907433946, 33.74890960531436690 ) ) ;
#122297=CARTESIAN_POINT ( 'NONE',  ( 0.05219959533934541429, -16.53943276465976808, 70.00109039468568994 ) ) ;
#122298=CARTESIAN_POINT ( 'NONE',  ( 0.05219959533909260263, 19.03943276465977164, 79.99890960531436690 ) ) ;
#122299=CARTESIAN_POINT ( 'NONE',  ( 5.823673210054444382, -21.52544592524334988, 40.20942372801901854 ) ) ;
#122300=CARTESIAN_POINT ( 'NONE',  ( 19.05341960407611168, 5.049401038298154454, 23.95724293864769194 ) ) ;
#122301=CARTESIAN_POINT ( 'NONE',  ( -18.67979575497178146, -10.72451020669898902, 31.66557627198102054 ) ) ;
#122302=VERTEX_POINT ( 'NONE', #105441 ) ;
#122303=CARTESIAN_POINT ( 'NONE',  ( -0.05219959533936034679, 19.03943276465977164, 22.50109039468566152 ) ) ;
#122304=CARTESIAN_POINT ( 'NONE',  ( 8.314922557961029526, -14.29746914071037800, 50.41775706135235424 ) ) ;
#122305=CARTESIAN_POINT ( 'NONE',  ( -5.153800228976328057, -19.02544592524343514, 97.29057627198099567 ) ) ;
#122306=CARTESIAN_POINT ( 'NONE',  ( 10.72451020669898902, -18.67979575497178502, 102.9155762719810383 ) ) ;
#122307=CARTESIAN_POINT ( 'NONE',  ( -0.05219959533909027116, -19.03943276465977164, 72.49890960531435269 ) ) ;
#122310=CARTESIAN_POINT ( 'NONE',  ( -8.224510206698948167, 14.34966873604960824, 75.41557627198102409 ) ) ;
#122311=CARTESIAN_POINT ( 'NONE',  ( -10.72451020669898014, 18.67979575497178502, 40.41557627198103120 ) ) ;
#122313=CARTESIAN_POINT ( 'NONE',  ( 8.224510206698742110, 14.34966873604972548, 62.08442372801901143 ) ) ;
#122314=CARTESIAN_POINT ( 'NONE',  ( -21.53943276465977519, -0.05219959533937600094, 23.75109039468567929 ) ) ;
#122315=CARTESIAN_POINT ( 'NONE',  ( -5.153800228976607833, 19.02544592524334988, 82.70942372801897591 ) ) ;
#122316=CARTESIAN_POINT ( 'NONE',  ( -19.03943276465977164, 0.05219959533909376836, 26.24890960531435624 ) ) ;
#122317=CARTESIAN_POINT ( 'NONE',  ( 15.72974639402199770, -15.80617190586745480, 63.12390960531435979 ) ) ;
#122318=CARTESIAN_POINT ( 'NONE',  ( -5.153800228976328057, -19.02544592524343514, 102.2905762719810383 ) ) ;
#122319=CARTESIAN_POINT ( 'NONE',  ( 5.823673210054444382, -21.52544592524334988, 95.20942372801903275 ) ) ;
#122320=CARTESIAN_POINT ( 'NONE',  ( -0.05219959533909027116, -19.03943276465977164, 67.49890960531436690 ) ) ;
#122321=CARTESIAN_POINT ( 'NONE',  ( 4.379528057220092307, 16.55341960407617563, 52.29275706135236135 ) ) ;
#122322=CARTESIAN_POINT ( 'NONE',  ( -0.05219959533909027116, -19.03943276465977164, 57.49890960531435979 ) ) ;
#122323=CARTESIAN_POINT ( 'NONE',  ( 15.72974639402176855, 15.80617190586768217, 81.87609039468568994 ) ) ;
#122325=CARTESIAN_POINT ( 'NONE',  ( 13.89961937509957401, 13.97604488694547697, 41.87609039468566152 ) ) ;
#122326=CARTESIAN_POINT ( 'NONE',  ( -13.97604488694547697, 13.89961937509957934, 58.12609039468566863 ) ) ;
#122327=CARTESIAN_POINT ( 'NONE',  ( -15.80617190586768217, 15.72974639402176855, 53.12609039468568284 ) ) ;
#122329=CARTESIAN_POINT ( 'NONE',  ( 13.97604488694548053, -13.89961937509957401, 40.62609039468564731 ) ) ;
#122330=CARTESIAN_POINT ( 'NONE',  ( -19.02544592524342804, 5.153800228976336051, 96.04057627198103830 ) ) ;
#122331=CARTESIAN_POINT ( 'NONE',  ( -9.564922557960796823, -16.46253265017161027, 67.08224293864769550 ) ) ;
#122332=CARTESIAN_POINT ( 'NONE',  ( -0.05219959533934338120, 16.53943276465976808, 112.5010903946857042 ) ) ;
#122333=CARTESIAN_POINT ( 'NONE',  ( -15.72974639402197994, 15.80617190586746368, 40.62390960531435269 ) ) ;
#122334=CARTESIAN_POINT ( 'NONE',  ( -18.67979575497193778, 10.72451020669871902, 103.3344237280190043 ) ) ;
#122338=CARTESIAN_POINT ( 'NONE',  ( 21.53943276465977519, 0.05219959533937863772, 101.2510903946856757 ) ) ;
#122340=CARTESIAN_POINT ( 'NONE',  ( 13.89961937509977652, -13.97604488694527269, 28.12390960531435624 ) ) ;
#122341=CARTESIAN_POINT ( 'NONE',  ( -9.474510206698964154, 16.51473224551069663, 110.4155762719810383 ) ) ;
#122345=CARTESIAN_POINT ( 'NONE',  ( -8.224510206698735004, -14.34966873604973081, 54.58442372801901143 ) ) ;
#122346=CARTESIAN_POINT ( 'NONE',  ( -21.55341960407610458, -5.719274019375992779, 66.45724293864768129 ) ) ;
#122347=CARTESIAN_POINT ( 'NONE',  ( -14.34966873604960291, -8.224510206698953496, 41.66557627198103120 ) ) ;
#122348=CARTESIAN_POINT ( 'NONE',  ( -12.14591786802309592, -12.06949235617757132, 106.8739096053143811 ) ) ;
#122349=CARTESIAN_POINT ( 'NONE',  ( 19.03943276465977164, -0.05219959533909143690, 103.7489096053143669 ) ) ;
#122350=CARTESIAN_POINT ( 'NONE',  ( 9.564922557961047289, -16.46253265017146816, 35.41775706135233293 ) ) ;
#122351=CARTESIAN_POINT ( 'NONE',  ( 0.05219959533909260263, 19.03943276465977164, 24.99890960531435269 ) ) ;
#122352=CARTESIAN_POINT ( 'NONE',  ( -10.72451020669870658, -18.67979575497194134, 64.58442372801900433 ) ) ;
#122353=CARTESIAN_POINT ( 'NONE',  ( -5.153800228976328057, -19.02544592524343514, 112.2905762719810099 ) ) ;
#122354=CARTESIAN_POINT ( 'NONE',  ( 14.34966873604960469, 8.224510206698951720, 34.16557627198102409 ) ) ;
#122356=CARTESIAN_POINT ( 'NONE',  ( -18.62759615963270932, 10.81492255796079327, 25.83224293864769194 ) ) ;
#122357=CARTESIAN_POINT ( 'NONE',  ( 12.14591786802309770, 12.06949235617756955, 89.37390960531435269 ) ) ;
#122358=CARTESIAN_POINT ( 'NONE',  ( 9.474510206698729675, 16.51473224551082808, 57.08442372801900433 ) ) ;
#122359=CARTESIAN_POINT ( 'NONE',  ( -9.564922557960796823, -16.46253265017161027, 72.08224293864770971 ) ) ;
#122360=CARTESIAN_POINT ( 'NONE',  ( -8.224510206698948167, 14.34966873604960824, 80.41557627198103830 ) ) ;
#122361=CARTESIAN_POINT ( 'NONE',  ( 9.474510206698729675, 16.51473224551082808, 87.08442372801900433 ) ) ;
#122362=CARTESIAN_POINT ( 'NONE',  ( -15.80617190586745835, -15.72974639402198527, 51.87390960531437401 ) ) ;
#122364=CARTESIAN_POINT ( 'NONE',  ( 16.55341960407611168, 4.379528057220329451, 113.9572429386477239 ) ) ;
#122366=CARTESIAN_POINT ( 'NONE',  ( 5.049401038298161559, -19.05341960407611168, 67.70724293864769550 ) ) ;
#122367=CARTESIAN_POINT ( 'NONE',  ( 15.80617190586746368, 15.72974639402197994, 69.37390960531436690 ) ) ;
#122368=CARTESIAN_POINT ( 'NONE',  ( 0.05219959533934541429, -16.53943276465976808, 110.0010903946856757 ) ) ;
#122369=CARTESIAN_POINT ( 'NONE',  ( 16.46253265017160672, -9.564922557960803928, 88.33224293864769550 ) ) ;
#122370=CARTESIAN_POINT ( 'NONE',  ( 19.02544592524334988, 5.153800228976608722, 71.45942372801900433 ) ) ;
#122371=CARTESIAN_POINT ( 'NONE',  ( 5.823673210054444382, -21.52544592524334988, 80.20942372801901854 ) ) ;
#122372=CARTESIAN_POINT ( 'NONE',  ( -5.823673210054116645, -21.52544592524344225, 62.29057627198102409 ) ) ;
#122373=CARTESIAN_POINT ( 'NONE',  ( 21.55341960407610458, 5.719274019375980345, 23.95724293864769550 ) ) ;
#122374=CARTESIAN_POINT ( 'NONE',  ( 5.049401038298161559, -19.05341960407611168, 42.70724293864767418 ) ) ;
#122375=CARTESIAN_POINT ( 'NONE',  ( -14.29746914071037622, -8.314922557961029526, 94.16775706135237556 ) ) ;
#122376=CARTESIAN_POINT ( 'NONE',  ( 19.02544592524343514, -5.153800228976328945, 63.54057627198103830 ) ) ;
#122377=CARTESIAN_POINT ( 'NONE',  ( 19.02544592524334988, 5.153800228976608722, 111.4594237280190043 ) ) ;
#122379=CARTESIAN_POINT ( 'NONE',  ( -13.89961937509957401, -13.97604488694547875, 19.37609039468566507 ) ) ;
#122380=CARTESIAN_POINT ( 'NONE',  ( 4.483927247898545687, 16.52544592524342804, 74.79057627198105251 ) ) ;
#122381=CARTESIAN_POINT ( 'NONE',  ( 10.81492255796078972, 18.62759615963270932, 104.5822429386477097 ) ) ;
#122382=CARTESIAN_POINT ( 'NONE',  ( -18.67979575497178146, -10.72451020669898902, 96.66557627198102409 ) ) ;
#122383=CARTESIAN_POINT ( 'NONE',  ( 17.50000000000000000, -5.500000000000031086, 98.29690382534174375 ) ) ;
#122384=CARTESIAN_POINT ( 'NONE',  ( -0.05219959533907301413, -21.53943276465977519, 47.49890960531435979 ) ) ;
#122385=CARTESIAN_POINT ( 'NONE',  ( 8.224510206698742110, 14.34966873604972548, 77.08442372801901854 ) ) ;
#122386=CARTESIAN_POINT ( 'NONE',  ( 12.14591786802309770, 12.06949235617756955, 109.3739096053143811 ) ) ;
#122387=CARTESIAN_POINT ( 'NONE',  ( 0.05219959533909260263, 19.03943276465977164, 54.99890960531435979 ) ) ;
#122390=CARTESIAN_POINT ( 'NONE',  ( -0.05219959533934338120, 16.53943276465976808, 112.5010903946857042 ) ) ;
#122391=CARTESIAN_POINT ( 'NONE',  ( 0.05219959533937995610, -21.53943276465977519, 45.00109039468568284 ) ) ;
#122392=CARTESIAN_POINT ( 'NONE',  ( -16.51473224551069308, -9.474510206698971260, 101.6655762719810241 ) ) ;
#122393=CARTESIAN_POINT ( 'NONE',  ( 21.53943276465977519, 0.05219959533937863772, 76.25109039468568994 ) ) ;
#122394=LINE ( 'NONE', #169901, #153532 ) ;
#122395=CARTESIAN_POINT ( 'NONE',  ( -5.153800228976328057, -19.02544592524343514, 22.29057627198102765 ) ) ;
#122396=ORIENTED_EDGE ( 'NONE', *, *, #194696, .T. ) ;
#122397=CARTESIAN_POINT ( 'NONE',  ( 5.719274019375673035, 21.55341960407619339, 67.29275706135234714 ) ) ;
#122398=CARTESIAN_POINT ( 'NONE',  ( 19.02544592524343514, -5.153800228976328945, 53.54057627198102409 ) ) ;
#122399=CARTESIAN_POINT ( 'NONE',  ( 13.97604488694527802, 13.89961937509977652, 109.3739096053143669 ) ) ;
#122400=CARTESIAN_POINT ( 'NONE',  ( -0.05219959533936034679, 19.03943276465977164, 82.50109039468567573 ) ) ;
#122401=CARTESIAN_POINT ( 'NONE',  ( -18.67979575497193778, 10.72451020669871902, 43.33442372801901143 ) ) ;
#122402=CARTESIAN_POINT ( 'NONE',  ( -9.474510206698720793, -16.51473224551083518, 109.5844237280190043 ) ) ;
#122403=CARTESIAN_POINT ( 'NONE',  ( 19.05341960407617918, -5.049401038297876454, 66.04275706135233293 ) ) ;
#122404=CARTESIAN_POINT ( 'NONE',  ( 5.049401038298161559, -19.05341960407611168, 32.70724293864768129 ) ) ;
#122405=CARTESIAN_POINT ( 'NONE',  ( 0.05219959533936267826, -19.03943276465977164, 90.00109039468567573 ) ) ;
#122406=CARTESIAN_POINT ( 'NONE',  ( -16.53943276465976808, -0.05219959533934237506, 108.7510903946857042 ) ) ;
#122407=CARTESIAN_POINT ( 'NONE',  ( 9.564922557961047289, -16.46253265017146816, 75.41775706135234714 ) ) ;
#122408=CARTESIAN_POINT ( 'NONE',  ( 14.34966873604960469, 8.224510206698951720, 39.16557627198102409 ) ) ;
#122409=CARTESIAN_POINT ( 'NONE',  ( 5.153800228976615827, -19.02544592524334988, 60.20942372801899012 ) ) ;
#122410=CARTESIAN_POINT ( 'NONE',  ( 10.81492255796106328, -18.62759615963255655, 105.4177570613523613 ) ) ;
#122411=CARTESIAN_POINT ( 'NONE',  ( -9.564922557961040184, 16.46253265017147172, 27.91775706135232582 ) ) ;
#122412=EDGE_CURVE ( 'NONE', #177566, #17000, #114386, .T. ) ;
#122413=CARTESIAN_POINT ( 'NONE',  ( 9.474510206698971260, -16.51473224551069308, 27.91557627198103120 ) ) ;
#122414=CARTESIAN_POINT ( 'NONE',  ( -17.13100169013298668, -6.664070546373171311, 64.23210164300152769 ) ) ;
#122415=CARTESIAN_POINT ( 'NONE',  ( 8.314922557961029526, -14.29746914071037800, 45.41775706135234003 ) ) ;
#122417=CARTESIAN_POINT ( 'NONE',  ( 0.05219959533909260263, 19.03943276465977164, 94.99890960531436690 ) ) ;
#122418=CARTESIAN_POINT ( 'NONE',  ( -18.22780087662123805, 5.499999999999981348, 96.01763182126897789 ) ) ;
#122420=CARTESIAN_POINT ( 'NONE',  ( 0.05219959533936267826, -19.03943276465977164, 80.00109039468567573 ) ) ;
#122421=CARTESIAN_POINT ( 'NONE',  ( -21.55341960407610458, -5.719274019375992779, 26.45724293864768839 ) ) ;
#122422=CARTESIAN_POINT ( 'NONE',  ( 18.62759615963255655, 10.81492255796105972, 111.6677570613523613 ) ) ;
#122423=CARTESIAN_POINT ( 'NONE',  ( 16.51473224551083163, -9.474510206698727899, 95.83442372801900433 ) ) ;
#122424=CARTESIAN_POINT ( 'NONE',  ( 14.29746914071049879, -8.314922557960816363, 108.3322429386477097 ) ) ;
#122425=CARTESIAN_POINT ( 'NONE',  ( 13.89961937509977652, -13.97604488694527269, 28.12390960531435624 ) ) ;
#122426=CARTESIAN_POINT ( 'NONE',  ( -15.72974639402197994, 15.80617190586746368, 65.62390960531436690 ) ) ;
#122427=CARTESIAN_POINT ( 'NONE',  ( -21.53943276465977519, 0.05219959533907696930, 46.24890960531435979 ) ) ;
#122428=CARTESIAN_POINT ( 'NONE',  ( -16.51473224551069308, -9.474510206698971260, 21.66557627198102765 ) ) ;
#122430=CARTESIAN_POINT ( 'NONE',  ( -19.02544592524334988, -5.153800228976617603, 68.95942372801896170 ) ) ;
#122431=CARTESIAN_POINT ( 'NONE',  ( 16.53943276465976808, -0.05219959533910856209, 33.74890960531436690 ) ) ;
#122432=CARTESIAN_POINT ( 'NONE',  ( -0.05219959533909027116, -19.03943276465977164, 112.4989096053143669 ) ) ;
#122433=CARTESIAN_POINT ( 'NONE',  ( 0.05219959533937995610, -21.53943276465977519, 95.00109039468568994 ) ) ;
#122434=CARTESIAN_POINT ( 'NONE',  ( -18.62759615963270932, 10.81492255796079327, 65.83224293864769550 ) ) ;
#122435=CARTESIAN_POINT ( 'NONE',  ( -21.53943276465977519, -0.05219959533937600094, 53.75109039468568994 ) ) ;
#122436=CARTESIAN_POINT ( 'NONE',  ( -10.81492255796105439, 18.62759615963255655, 47.91775706135234714 ) ) ;
#122437=CARTESIAN_POINT ( 'NONE',  ( 13.97604488694527802, 13.89961937509977652, 99.37390960531436690 ) ) ;
#122438=CARTESIAN_POINT ( 'NONE',  ( 4.379528057220092307, 16.55341960407617563, 92.29275706135236135 ) ) ;
#122439=CARTESIAN_POINT ( 'NONE',  ( 18.67979575497194134, -10.72451020669871369, 45.83442372801901854 ) ) ;
#122440=CARTESIAN_POINT ( 'NONE',  ( -13.89961937509977652, 13.97604488694528158, 25.62390960531434558 ) ) ;
#122442=CARTESIAN_POINT ( 'NONE',  ( 4.379528057220339221, -16.55341960407611168, 67.70724293864769550 ) ) ;
#122443=CARTESIAN_POINT ( 'NONE',  ( 14.34966873604960469, 8.224510206698951720, 29.16557627198103120 ) ) ;
#122444=CARTESIAN_POINT ( 'NONE',  ( 9.474510206698971260, -16.51473224551069308, 67.91557627198102409 ) ) ;
#122445=CARTESIAN_POINT ( 'NONE',  ( 13.97604488694527802, 13.89961937509977652, 44.37390960531435269 ) ) ;
#122446=CARTESIAN_POINT ( 'NONE',  ( -10.72451020669898014, 18.67979575497178502, 60.41557627198102409 ) ) ;
#122447=CARTESIAN_POINT ( 'NONE',  ( 5.049401038297881783, 19.05341960407617563, 37.29275706135232582 ) ) ;
#122449=CARTESIAN_POINT ( 'NONE',  ( -0.05219959533910754901, -16.53943276465976808, 47.49890960531435979 ) ) ;
#122450=CARTESIAN_POINT ( 'NONE',  ( -15.72974639402197994, 15.80617190586746368, 30.62390960531436335 ) ) ;
#122453=CARTESIAN_POINT ( 'NONE',  ( 4.379528057220092307, 16.55341960407617563, 77.29275706135234714 ) ) ;
#122454=CARTESIAN_POINT ( 'NONE',  ( -9.564922557961040184, 16.46253265017147172, 77.91775706135234714 ) ) ;
#122455=CARTESIAN_POINT ( 'NONE',  ( 0.05219959533910956823, 16.53943276465976808, 44.99890960531435979 ) ) ;
#122456=CARTESIAN_POINT ( 'NONE',  ( 17.26172910966781515, -6.454744622555777411, 53.30646908649224969 ) ) ;
#122457=CARTESIAN_POINT ( 'NONE',  ( -16.53943276465976808, 0.05219959533911058130, 31.24890960531435979 ) ) ;
#122458=CARTESIAN_POINT ( 'NONE',  ( -16.46253265017160317, 9.564922557960807481, 55.83224293864769550 ) ) ;
#122459=CARTESIAN_POINT ( 'NONE',  ( -19.03943276465977164, 0.05219959533909376836, 81.24890960531436690 ) ) ;
#122460=CARTESIAN_POINT ( 'NONE',  ( -19.05341960407611168, -5.049401038298163336, 41.45724293864769550 ) ) ;
#122461=CARTESIAN_POINT ( 'NONE',  ( -21.55341960407619339, 5.719274019375674811, 43.54275706135235424 ) ) ;
#122462=CARTESIAN_POINT ( 'NONE',  ( 9.474510206698971260, -16.51473224551069308, 52.91557627198102409 ) ) ;
#122464=CARTESIAN_POINT ( 'NONE',  ( -13.97604488694527625, -13.89961937509977652, 56.87390960531434558 ) ) ;
#122465=CARTESIAN_POINT ( 'NONE',  ( 21.55341960407610458, 5.719274019375980345, 38.95724293864768839 ) ) ;
#122467=CARTESIAN_POINT ( 'NONE',  ( 13.89961937509977652, -13.97604488694527269, 23.12390960531436335 ) ) ;
#122468=CARTESIAN_POINT ( 'NONE',  ( -15.80617190586745835, -15.72974639402198527, 31.87390960531435979 ) ) ;
#122469=B_SPLINE_CURVE_WITH_KNOTS ( 'NONE', 3,
 ( #24545, #36679, #146868, #194392, #128688, #86195 ),
 .UNSPECIFIED., .F., .F.,
 ( 4, 2, 4 ),
 ( 0.000000000000000000, 0.0003837532665635277852, 0.0007675065331270555704 ),
 .UNSPECIFIED. ) ;
#122470=CARTESIAN_POINT ( 'NONE',  ( -8.224510206698735004, -14.34966873604973081, 84.58442372801903275 ) ) ;
#122471=CARTESIAN_POINT ( 'NONE',  ( -18.67979575497193778, 10.72451020669871902, 103.3344237280190043 ) ) ;
#122472=CARTESIAN_POINT ( 'NONE',  ( 16.55341960407618274, -4.379528057220086978, 66.04275706135236135 ) ) ;
#122473=CARTESIAN_POINT ( 'NONE',  ( -9.474510206698964154, 16.51473224551069663, 115.4155762719810241 ) ) ;
#122474=CARTESIAN_POINT ( 'NONE',  ( 12.14591786802327356, -12.06949235617739191, 60.62609039468567573 ) ) ;
#122475=CARTESIAN_POINT ( 'NONE',  ( 12.14591786802327356, -12.06949235617739191, 40.62609039468567573 ) ) ;
#122476=CARTESIAN_POINT ( 'NONE',  ( -14.34966873604972548, 8.224510206698743886, 93.33442372801901854 ) ) ;
#122477=CARTESIAN_POINT ( 'NONE',  ( -4.379528057220086978, -16.55341960407618274, 24.79275706135235779 ) ) ;
#122478=CARTESIAN_POINT ( 'NONE',  ( -19.02544592524342804, 5.153800228976336051, 31.04057627198102409 ) ) ;
#122479=CARTESIAN_POINT ( 'NONE',  ( 0.05219959533907565091, 21.53943276465977519, 104.9989096053143669 ) ) ;
#122480=CARTESIAN_POINT ( 'NONE',  ( -14.34966873604972548, 8.224510206698743886, 28.33442372801902209 ) ) ;
#122481=CARTESIAN_POINT ( 'NONE',  ( 12.14591786802327356, -12.06949235617739191, 80.62609039468567573 ) ) ;
#122483=CARTESIAN_POINT ( 'NONE',  ( -21.55341960407619339, 5.719274019375674811, 83.54275706135234714 ) ) ;
#122484=CARTESIAN_POINT ( 'NONE',  ( 13.97604488694548053, -13.89961937509957401, 85.62609039468568994 ) ) ;
#122485=CARTESIAN_POINT ( 'NONE',  ( -4.483927247898539470, -16.52544592524342804, 57.29057627198103120 ) ) ;
#122486=CARTESIAN_POINT ( 'NONE',  ( 8.314922557960818139, 14.29746914071049879, 49.58224293864769550 ) ) ;
#122487=CARTESIAN_POINT ( 'NONE',  ( -12.14591786802309592, -12.06949235617757132, 101.8739096053143811 ) ) ;
#122488=CARTESIAN_POINT ( 'NONE',  ( -5.153800228976607833, 19.02544592524334988, 42.70942372801901143 ) ) ;
#122489=CARTESIAN_POINT ( 'NONE',  ( 18.09805431107250584, -5.499999999999988454, 53.51606229291888184 ) ) ;
#122490=CARTESIAN_POINT ( 'NONE',  ( 21.52544592524334988, 5.823673210054432836, 46.45942372801901854 ) ) ;
#122491=CARTESIAN_POINT ( 'NONE',  ( -13.97604488694547697, 13.89961937509957934, 103.1260903946856473 ) ) ;
#122492=CARTESIAN_POINT ( 'NONE',  ( 17.44270441346518652, 5.991230190322986537, 83.86335079264230785 ) ) ;
#122493=CARTESIAN_POINT ( 'NONE',  ( 5.153800228976335163, 19.02544592524342804, 99.79057627198102409 ) ) ;
#122494=CARTESIAN_POINT ( 'NONE',  ( -18.62759615963270932, 10.81492255796079327, 70.83224293864770971 ) ) ;
#122495=CARTESIAN_POINT ( 'NONE',  ( 13.97604488694548053, -13.89961937509957401, 90.62609039468567573 ) ) ;
#122496=CARTESIAN_POINT ( 'NONE',  ( -13.97604488694527625, -13.89961937509977652, 106.8739096053143669 ) ) ;
#122498=CARTESIAN_POINT ( 'NONE',  ( -4.483927247898539470, -16.52544592524342804, 107.2905762719810525 ) ) ;
#122499=CARTESIAN_POINT ( 'NONE',  ( -15.72974639402176322, -15.80617190586768395, 94.37609039468568994 ) ) ;
#122500=CARTESIAN_POINT ( 'NONE',  ( 13.89961937509977652, -13.97604488694527269, 38.12390960531436690 ) ) ;
#122501=CARTESIAN_POINT ( 'NONE',  ( -18.67979575497193778, 10.72451020669871902, 48.33442372801902565 ) ) ;
#122503=CARTESIAN_POINT ( 'NONE',  ( -21.55341960407619339, 5.719274019375674811, 88.54275706135236135 ) ) ;
#122504=CARTESIAN_POINT ( 'NONE',  ( 16.52544592524335698, 4.483927247898782831, 96.45942372801901854 ) ) ;
#122505=CARTESIAN_POINT ( 'NONE',  ( -10.72451020669870658, -18.67979575497194134, 39.58442372801901143 ) ) ;
#122506=CARTESIAN_POINT ( 'NONE',  ( 15.80617190586769283, -15.72974639402175789, 40.62609039468567573 ) ) ;
#122507=CARTESIAN_POINT ( 'NONE',  ( -9.564922557961040184, 16.46253265017147172, 67.91775706135233293 ) ) ;
#122508=CARTESIAN_POINT ( 'NONE',  ( 9.564922557960805705, 16.46253265017160317, 89.58224293864769550 ) ) ;
#122509=CARTESIAN_POINT ( 'NONE',  ( -8.224510206698948167, 14.34966873604960824, 105.4155762719810383 ) ) ;
#122510=CARTESIAN_POINT ( 'NONE',  ( -5.719274019375978568, 21.55341960407610458, 80.20724293864769550 ) ) ;
#122511=CARTESIAN_POINT ( 'NONE',  ( 12.06949235617757843, -12.14591786802309237, 68.12390960531436690 ) ) ;
#122512=CARTESIAN_POINT ( 'NONE',  ( 0.05219959533937995610, -21.53943276465977519, 110.0010903946856757 ) ) ;
#122513=CARTESIAN_POINT ( 'NONE',  ( -14.29746914071049879, 8.314922557960819915, 85.83224293864768129 ) ) ;
#122514=CARTESIAN_POINT ( 'NONE',  ( -13.89961937509977652, 13.97604488694528158, 40.62390960531435979 ) ) ;
#122515=CARTESIAN_POINT ( 'NONE',  ( 13.89961937509957401, 13.97604488694547697, 86.87609039468567573 ) ) ;
#122516=CARTESIAN_POINT ( 'NONE',  ( 0.05219959533910956823, 16.53943276465976808, 54.99890960531435269 ) ) ;
#122517=CARTESIAN_POINT ( 'NONE',  ( -18.62759615963255300, -10.81492255796106328, 89.16775706135236135 ) ) ;
#122518=CARTESIAN_POINT ( 'NONE',  ( 16.51473224551069308, 9.474510206698969483, 89.16557627198103830 ) ) ;
#122519=CARTESIAN_POINT ( 'NONE',  ( -5.153800228976607833, 19.02544592524334988, 57.70942372801899012 ) ) ;
#122520=CARTESIAN_POINT ( 'NONE',  ( 18.67979575497178502, 10.72451020669898547, 59.16557627198103120 ) ) ;
#122521=CARTESIAN_POINT ( 'NONE',  ( 21.53943276465977519, -0.05219959533907433946, 113.7489096053143527 ) ) ;
#122522=CARTESIAN_POINT ( 'NONE',  ( 8.314922557961029526, -14.29746914071037800, 25.41775706135235779 ) ) ;
#122523=CARTESIAN_POINT ( 'NONE',  ( 16.55341960407618274, -4.379528057220086978, 76.04275706135237556 ) ) ;
#122524=CARTESIAN_POINT ( 'NONE',  ( -19.05341960407611168, -5.049401038298163336, 21.45724293864768839 ) ) ;
#122525=CARTESIAN_POINT ( 'NONE',  ( 21.53943276465977519, -0.05219959533907433946, 113.7489096053143527 ) ) ;
#122526=CARTESIAN_POINT ( 'NONE',  ( -16.51473224551069308, -9.474510206698971260, 21.66557627198102765 ) ) ;
#122528=CARTESIAN_POINT ( 'NONE',  ( 16.55341960407618274, -4.379528057220086978, 46.04275706135234714 ) ) ;
#122529=CARTESIAN_POINT ( 'NONE',  ( 14.34966873604960469, 8.224510206698951720, 84.16557627198103830 ) ) ;
#122530=CARTESIAN_POINT ( 'NONE',  ( 10.72451020669898902, -18.67979575497178502, 77.91557627198102409 ) ) ;
#122531=CARTESIAN_POINT ( 'NONE',  ( -16.53943276465976808, 0.05219959533911058130, 21.24890960531436690 ) ) ;
#122532=CARTESIAN_POINT ( 'NONE',  ( -8.224510206698735004, -14.34966873604973081, 39.58442372801901143 ) ) ;
#122533=CARTESIAN_POINT ( 'NONE',  ( 13.89961937509977652, -13.97604488694527269, 48.12390960531435979 ) ) ;
#122534=CARTESIAN_POINT ( 'NONE',  ( 16.55341960407618274, -4.379528057220086978, 76.04275706135237556 ) ) ;
#122535=CARTESIAN_POINT ( 'NONE',  ( 0.05219959533936267826, -19.03943276465977164, 80.00109039468567573 ) ) ;
#122536=CARTESIAN_POINT ( 'NONE',  ( 21.52544592524344225, -5.823673210054117533, 78.54057627198103830 ) ) ;
#122537=CARTESIAN_POINT ( 'NONE',  ( -16.55341960407617563, 4.379528057220093196, 113.5427570613523756 ) ) ;
#122538=VERTEX_POINT ( 'NONE', #166138 ) ;
#122540=CARTESIAN_POINT ( 'NONE',  ( 18.62759615963271287, -10.81492255796078972, 48.33224293864770260 ) ) ;
#122543=CARTESIAN_POINT ( 'NONE',  ( -16.55341960407617563, 4.379528057220093196, 93.54275706135234714 ) ) ;
#122544=CARTESIAN_POINT ( 'NONE',  ( 0.05219959533907565091, 21.53943276465977519, 39.99890960531436690 ) ) ;
#122546=CARTESIAN_POINT ( 'NONE',  ( 5.153800228976335163, 19.02544592524342804, 109.7905762719810099 ) ) ;
#122547=CARTESIAN_POINT ( 'NONE',  ( 17.49999999999999645, 3.209263204892610410, 107.7380317439373272 ) ) ;
#122548=CARTESIAN_POINT ( 'NONE',  ( -16.53943276465976808, 0.05219959533911058130, 116.2489096053143669 ) ) ;
#122549=CARTESIAN_POINT ( 'NONE',  ( -15.72974639402197994, 15.80617190586746368, 70.62390960531436690 ) ) ;
#122550=CARTESIAN_POINT ( 'NONE',  ( 16.52544592524335698, 4.483927247898782831, 101.4594237280190185 ) ) ;
#122551=CARTESIAN_POINT ( 'NONE',  ( -10.72451020669870658, -18.67979575497194134, 64.58442372801900433 ) ) ;
#122552=CARTESIAN_POINT ( 'NONE',  ( 13.97604488694548053, -13.89961937509957401, 110.6260903946856615 ) ) ;
#122553=CARTESIAN_POINT ( 'NONE',  ( -5.153800228976328057, -19.02544592524343514, 27.29057627198103120 ) ) ;
#122554=CARTESIAN_POINT ( 'NONE',  ( -0.05219959533934338120, 16.53943276465976808, 22.50109039468567573 ) ) ;
#122555=CARTESIAN_POINT ( 'NONE',  ( 16.46253265017160672, -9.564922557960803928, 53.33224293864768839 ) ) ;
#122557=CARTESIAN_POINT ( 'NONE',  ( -19.02544592524342804, 5.153800228976336051, 106.0405762719810241 ) ) ;
#122558=CARTESIAN_POINT ( 'NONE',  ( 16.53943276465976808, 0.05219959533934440121, 86.25109039468568994 ) ) ;
#122559=CARTESIAN_POINT ( 'NONE',  ( -0.05219959533936034679, 19.03943276465977164, 97.50109039468567573 ) ) ;
#122560=CARTESIAN_POINT ( 'NONE',  ( -9.564922557961040184, 16.46253265017147172, 27.91775706135232582 ) ) ;
#122561=CARTESIAN_POINT ( 'NONE',  ( 21.55341960407610458, 5.719274019375980345, 78.95724293864769550 ) ) ;
#122562=CARTESIAN_POINT ( 'NONE',  ( 0.05219959533934541429, -16.53943276465976808, 105.0010903946856757 ) ) ;
#122563=CARTESIAN_POINT ( 'NONE',  ( 19.02544592524334988, 5.153800228976608722, 91.45942372801900433 ) ) ;
#122564=CARTESIAN_POINT ( 'NONE',  ( 16.51473224551069308, 9.474510206698969483, 54.16557627198103120 ) ) ;
#122565=CARTESIAN_POINT ( 'NONE',  ( -13.97604488694527625, -13.89961937509977652, 91.87390960531432427 ) ) ;
#122566=CARTESIAN_POINT ( 'NONE',  ( 5.823673210054444382, -21.52544592524334988, 55.20942372801902565 ) ) ;
#122567=CARTESIAN_POINT ( 'NONE',  ( -5.049401038298153566, 19.05341960407611168, 50.20724293864770260 ) ) ;
#122569=CARTESIAN_POINT ( 'NONE',  ( 5.153800228976335163, 19.02544592524342804, 109.7905762719810099 ) ) ;
#122570=CARTESIAN_POINT ( 'NONE',  ( -4.379528057220328563, 16.55341960407611168, 65.20724293864768129 ) ) ;
#122571=CARTESIAN_POINT ( 'NONE',  ( -10.81492255796078084, -18.62759615963271287, 72.08224293864769550 ) ) ;
#122572=CARTESIAN_POINT ( 'NONE',  ( 17.50000000000000000, -5.500000000000000888, 23.29690382534171889 ) ) ;
#122573=CARTESIAN_POINT ( 'NONE',  ( -13.89961937509957401, -13.97604488694547875, 39.37609039468566152 ) ) ;
#122574=CARTESIAN_POINT ( 'NONE',  ( 17.12812012977047615, -6.668231424565698617, 71.14051240676850796 ) ) ;
#122575=CARTESIAN_POINT ( 'NONE',  ( 9.564922557960805705, 16.46253265017160317, 69.58224293864770971 ) ) ;
#122576=CARTESIAN_POINT ( 'NONE',  ( 13.97604488694527802, 13.89961937509977652, 84.37390960531433848 ) ) ;
#122578=CARTESIAN_POINT ( 'NONE',  ( -4.379528057220086978, -16.55341960407618274, 49.79275706135234714 ) ) ;
#122580=B_SPLINE_CURVE_WITH_KNOTS ( 'NONE', 3,
 ( #23176, #72684, #27185, #179877, #146499, #41345, #24186, #194040, #103007, #55504, #40336, #102011, #7990, #164692, #134359, #130319, #25195, #145503, #6984, #69673, #192016, #115177, #176870, #193028, #54505, #123134, #60468, #137320, #197030, #183831, #29169, #58497 ),
 .UNSPECIFIED., .F., .F.,
 ( 4, 2, 2, 2, 2, 2, 2, 2, 2, 2, 2, 2, 2, 2, 2, 4 ),
 ( 1.769077770938648657E-17, 0.0003712461730036916026, 0.0007424923460073655328, 0.001113738519011039409, 0.001484984692014713501, 0.002227477038022061036, 0.002598723211025738382, 0.002969969384029415727, 0.003341215557033093073, 0.003712461730036770418, 0.004083707903040446896, 0.004454954076044123808, 0.004826200249047801587, 0.005197446422051478498, 0.005568692595055156278, 0.005939938768058833189 ),
 .UNSPECIFIED. ) ;
#122581=CARTESIAN_POINT ( 'NONE',  ( -5.049401038297874678, -19.05341960407617918, 34.79275706135233293 ) ) ;
#122583=CARTESIAN_POINT ( 'NONE',  ( 14.34966873604972726, -8.224510206698740333, 90.83442372801901854 ) ) ;
#122585=CARTESIAN_POINT ( 'NONE',  ( -14.34966873604972548, 8.224510206698743886, 78.33442372801901854 ) ) ;
#122586=CARTESIAN_POINT ( 'NONE',  ( 16.55341960407618274, -4.379528057220086978, 61.04275706135234714 ) ) ;
#122587=CARTESIAN_POINT ( 'NONE',  ( -13.89961937509977652, 13.97604488694528158, 50.62390960531435979 ) ) ;
#122588=CARTESIAN_POINT ( 'NONE',  ( 17.59860650958989936, 7.585241751807028088, 74.07662985737508166 ) ) ;
#122589=CARTESIAN_POINT ( 'NONE',  ( 21.52544592524334988, 5.823673210054432836, 61.45942372801901854 ) ) ;
#122590=CARTESIAN_POINT ( 'NONE',  ( 19.03943276465977164, 0.05219959533936151252, 81.25109039468567573 ) ) ;
#122591=CARTESIAN_POINT ( 'NONE',  ( 10.81492255796106328, -18.62759615963255655, 110.4177570613523756 ) ) ;
#122592=CARTESIAN_POINT ( 'NONE',  ( 9.564922557960805705, 16.46253265017160317, 44.58224293864769550 ) ) ;
#122593=CARTESIAN_POINT ( 'NONE',  ( 17.50000000000000000, 5.499999999999997335, 23.78230962303566542 ) ) ;
#122594=CARTESIAN_POINT ( 'NONE',  ( 10.72451020669898902, -18.67979575497178502, 62.91557627198102409 ) ) ;
#122595=CARTESIAN_POINT ( 'NONE',  ( 0.05219959533909260263, 19.03943276465977164, 109.9989096053143669 ) ) ;
#122596=CARTESIAN_POINT ( 'NONE',  ( -9.564922557960796823, -16.46253265017161027, 22.08224293864768839 ) ) ;
#122597=CARTESIAN_POINT ( 'NONE',  ( 4.483927247898790824, -16.52544592524335698, 45.20942372801901854 ) ) ;
#122598=CARTESIAN_POINT ( 'NONE',  ( -4.483927247898539470, -16.52544592524342804, 32.29057627198102409 ) ) ;
#122600=CARTESIAN_POINT ( 'NONE',  ( 10.81492255796106328, -18.62759615963255655, 20.41775706135234714 ) ) ;
#122601=CARTESIAN_POINT ( 'NONE',  ( -12.14591786802309592, -12.06949235617757132, 51.87390960531437401 ) ) ;
#122603=CARTESIAN_POINT ( 'NONE',  ( 5.049401038297881783, 19.05341960407617563, 102.2927570613523045 ) ) ;
#122604=CARTESIAN_POINT ( 'NONE',  ( 16.46253265017146816, 9.564922557961045513, 41.66775706135234003 ) ) ;
#122605=CARTESIAN_POINT ( 'NONE',  ( 16.53943276465976808, -0.05219959533910856209, 43.74890960531435979 ) ) ;
#122606=CARTESIAN_POINT ( 'NONE',  ( -15.80617190586745835, -15.72974639402198527, 101.8739096053143811 ) ) ;
#122608=CARTESIAN_POINT ( 'NONE',  ( 15.72974639402199770, -15.80617190586745480, 68.12390960531436690 ) ) ;
#122609=CARTESIAN_POINT ( 'NONE',  ( 13.97604488694527802, 13.89961937509977652, 74.37390960531436690 ) ) ;
#122610=CARTESIAN_POINT ( 'NONE',  ( -4.483927247898539470, -16.52544592524342804, 47.29057627198103120 ) ) ;
#122611=CARTESIAN_POINT ( 'NONE',  ( -9.474510206698964154, 16.51473224551069663, 100.4155762719810241 ) ) ;
#122614=CARTESIAN_POINT ( 'NONE',  ( -19.05341960407617563, 5.049401038297882671, 58.54275706135234003 ) ) ;
#122615=CARTESIAN_POINT ( 'NONE',  ( -5.719274019375978568, 21.55341960407610458, 90.20724293864770971 ) ) ;
#122616=CARTESIAN_POINT ( 'NONE',  ( 16.46253265017160672, -9.564922557960803928, 48.33224293864769550 ) ) ;
#122617=CARTESIAN_POINT ( 'NONE',  ( -8.314922557960811034, -14.29746914071050412, 112.0822429386477097 ) ) ;
#122618=CARTESIAN_POINT ( 'NONE',  ( -5.719274019375665041, -21.55341960407619695, 54.79275706135235424 ) ) ;
#122620=CARTESIAN_POINT ( 'NONE',  ( -16.53943276465976808, 0.05219959533911058130, 21.24890960531436690 ) ) ;
#122621=CARTESIAN_POINT ( 'NONE',  ( 16.51473224551069308, 9.474510206698969483, 54.16557627198103120 ) ) ;
#122622=CARTESIAN_POINT ( 'NONE',  ( -5.153800228976328057, -19.02544592524343514, 102.2905762719810383 ) ) ;
#122623=CARTESIAN_POINT ( 'NONE',  ( -0.05219959533907301413, -21.53943276465977519, 62.49890960531436690 ) ) ;
#122625=CARTESIAN_POINT ( 'NONE',  ( 0.05219959533909260263, 19.03943276465977164, 49.99890960531435979 ) ) ;
#122626=CARTESIAN_POINT ( 'NONE',  ( 18.62759615963271287, -10.81492255796078972, 53.33224293864769550 ) ) ;
#122627=CARTESIAN_POINT ( 'NONE',  ( -5.823673210054431948, 21.52544592524334988, 87.70942372801901854 ) ) ;
#122629=CARTESIAN_POINT ( 'NONE',  ( -16.53943276465976808, -0.05219959533934237506, 78.75109039468568994 ) ) ;
#122630=CARTESIAN_POINT ( 'NONE',  ( -4.483927247898782831, 16.52544592524335698, 87.70942372801901854 ) ) ;
#122631=CARTESIAN_POINT ( 'NONE',  ( 13.97604488694527802, 13.89961937509977652, 74.37390960531436690 ) ) ;
#122633=CARTESIAN_POINT ( 'NONE',  ( -19.02544592524334988, -5.153800228976617603, 23.95942372801900078 ) ) ;
#122634=CARTESIAN_POINT ( 'NONE',  ( -16.52544592524335698, -4.483927247898792601, 83.95942372801900433 ) ) ;
#122635=CARTESIAN_POINT ( 'NONE',  ( 19.03943276465977164, 0.05219959533936151252, 21.25109039468565797 ) ) ;
#122636=CARTESIAN_POINT ( 'NONE',  ( -13.97604488694527625, -13.89961937509977652, 76.87390960531433848 ) ) ;
#122637=CARTESIAN_POINT ( 'NONE',  ( 18.67979575497178502, 10.72451020669898547, 54.16557627198103120 ) ) ;
#122638=CARTESIAN_POINT ( 'NONE',  ( -12.14591786802326823, 12.06949235617739902, 23.12609039468567573 ) ) ;
#122639=CARTESIAN_POINT ( 'NONE',  ( 21.53943276465977519, 0.05219959533937863772, 76.25109039468568994 ) ) ;
#122640=CARTESIAN_POINT ( 'NONE',  ( -8.224510206698735004, -14.34966873604973081, 64.58442372801900433 ) ) ;
#122641=CARTESIAN_POINT ( 'NONE',  ( -18.67979575497178146, -10.72451020669898902, 111.6655762719810525 ) ) ;
#122642=CARTESIAN_POINT ( 'NONE',  ( 0.05219959533936267826, -19.03943276465977164, 110.0010903946856757 ) ) ;
#122643=CARTESIAN_POINT ( 'NONE',  ( 13.89961937509977652, -13.97604488694527269, 98.12390960531433848 ) ) ;
#122644=CARTESIAN_POINT ( 'NONE',  ( -8.314922557961024197, 14.29746914071037800, 32.91775706135234714 ) ) ;
#122645=CARTESIAN_POINT ( 'NONE',  ( 13.89961937509977652, -13.97604488694527269, 43.12390960531434558 ) ) ;
#122647=CARTESIAN_POINT ( 'NONE',  ( 16.53943276465976808, 0.05219959533934440121, 21.25109039468567218 ) ) ;
#122648=CARTESIAN_POINT ( 'NONE',  ( 4.483927247898545687, 16.52544592524342804, 79.79057627198102409 ) ) ;
#122649=CARTESIAN_POINT ( 'NONE',  ( 12.14591786802327356, -12.06949235617739191, 85.62609039468568994 ) ) ;
#122651=CARTESIAN_POINT ( 'NONE',  ( 18.67979575497194134, -10.72451020669871369, 30.83442372801902209 ) ) ;
#122652=CARTESIAN_POINT ( 'NONE',  ( -16.46253265017160317, 9.564922557960807481, 60.83224293864769550 ) ) ;
#122653=CARTESIAN_POINT ( 'NONE',  ( -16.46253265017160317, 9.564922557960807481, 70.83224293864770971 ) ) ;
#122654=CARTESIAN_POINT ( 'NONE',  ( 16.53943276465976808, 0.05219959533934440121, 91.25109039468568994 ) ) ;
#122656=ORIENTED_EDGE ( 'NONE', *, *, #20347, .F. ) ;
#122657=ORIENTED_EDGE ( 'NONE', *, *, #61085, .T. ) ;
#122658=CARTESIAN_POINT ( 'NONE',  ( -0.05219959533936034679, 19.03943276465977164, 27.50109039468566507 ) ) ;
#122659=CARTESIAN_POINT ( 'NONE',  ( -13.89961937509977652, 13.97604488694528158, 40.62390960531435979 ) ) ;
#122660=CARTESIAN_POINT ( 'NONE',  ( 15.50000000000000355, 7.499999999999998224, 120.0000000000000142 ) ) ;
#122661=ORIENTED_EDGE ( 'NONE', *, *, #190681, .T. ) ;
#122662=CARTESIAN_POINT ( 'NONE',  ( -12.06949235617739369, -12.14591786802326823, 24.37609039468567573 ) ) ;
#122663=CARTESIAN_POINT ( 'NONE',  ( 19.03943276465977164, 0.05219959533936151252, 61.25109039468566863 ) ) ;
#122664=CARTESIAN_POINT ( 'NONE',  ( -14.34966873604972548, 8.224510206698743886, 43.33442372801901143 ) ) ;
#122665=CARTESIAN_POINT ( 'NONE',  ( -9.564922557960796823, -16.46253265017161027, 112.0822429386476955 ) ) ;
#122666=CARTESIAN_POINT ( 'NONE',  ( -9.564922557960796823, -16.46253265017161027, 77.08224293864769550 ) ) ;
#122667=CARTESIAN_POINT ( 'NONE',  ( 5.719274019375991003, -21.55341960407610458, 102.7072429386476955 ) ) ;
#122668=CARTESIAN_POINT ( 'NONE',  ( -19.02544592524334988, -5.153800228976617603, 63.95942372801899012 ) ) ;
#122669=CARTESIAN_POINT ( 'NONE',  ( -19.05341960407611168, -5.049401038298163336, 96.45724293864769550 ) ) ;
#122670=CARTESIAN_POINT ( 'NONE',  ( 9.564922557960805705, 16.46253265017160317, 69.58224293864770971 ) ) ;
#122671=CARTESIAN_POINT ( 'NONE',  ( -16.55341960407611168, -4.379528057220339221, 21.45724293864769550 ) ) ;
#122672=CARTESIAN_POINT ( 'NONE',  ( -16.46253265017160317, 9.564922557960807481, 70.83224293864770971 ) ) ;
#122673=CARTESIAN_POINT ( 'NONE',  ( 0.05219959533936267826, -19.03943276465977164, 35.00109039468566863 ) ) ;
#122674=CARTESIAN_POINT ( 'NONE',  ( 14.34966873604960469, 8.224510206698951720, 69.16557627198102409 ) ) ;
#122675=CARTESIAN_POINT ( 'NONE',  ( -5.823673210054431948, 21.52544592524334988, 97.70942372801904696 ) ) ;
#122676=CARTESIAN_POINT ( 'NONE',  ( -13.89961937509977652, 13.97604488694528158, 35.62390960531435269 ) ) ;
#122677=CARTESIAN_POINT ( 'NONE',  ( -4.379528057220086978, -16.55341960407618274, 49.79275706135234714 ) ) ;
#122678=CARTESIAN_POINT ( 'NONE',  ( 0.05219959533910956823, 16.53943276465976808, 44.99890960531435979 ) ) ;
#122679=CARTESIAN_POINT ( 'NONE',  ( 15.72974639402176855, 15.80617190586768217, 86.87609039468568994 ) ) ;
#122680=CARTESIAN_POINT ( 'NONE',  ( 13.97604488694527802, 13.89961937509977652, 79.37390960531435269 ) ) ;
#122681=CARTESIAN_POINT ( 'NONE',  ( -16.51473224551069308, -9.474510206698971260, 91.66557627198103830 ) ) ;
#122682=CARTESIAN_POINT ( 'NONE',  ( -0.05219959533910754901, -16.53943276465976808, 112.4989096053143669 ) ) ;
#122683=CARTESIAN_POINT ( 'NONE',  ( 16.55341960407611168, 4.379528057220329451, 78.95724293864769550 ) ) ;
#122684=CARTESIAN_POINT ( 'NONE',  ( -5.823673210054116645, -21.52544592524344225, 77.29057627198102409 ) ) ;
#122685=CARTESIAN_POINT ( 'NONE',  ( -5.049401038298153566, 19.05341960407611168, 85.20724293864766707 ) ) ;
#122686=CARTESIAN_POINT ( 'NONE',  ( 5.719274019375991003, -21.55341960407610458, 97.70724293864772392 ) ) ;
#122687=CARTESIAN_POINT ( 'NONE',  ( -16.46253265017146816, -9.564922557961047289, 74.16775706135234714 ) ) ;
#122688=CARTESIAN_POINT ( 'NONE',  ( -13.89961937509957401, -13.97604488694547697, 64.37609039468567573 ) ) ;
#122689=CARTESIAN_POINT ( 'NONE',  ( -16.55341960407611168, -4.379528057220339221, 91.45724293864769550 ) ) ;
#122690=CARTESIAN_POINT ( 'NONE',  ( 5.049401038298161559, -19.05341960407611168, 52.70724293864767418 ) ) ;
#122691=CARTESIAN_POINT ( 'NONE',  ( -5.719274019375978568, 21.55341960407610458, 60.20724293864768839 ) ) ;
#122692=CARTESIAN_POINT ( 'NONE',  ( 16.81555441253552985, -7.025013491695481171, 28.13685445334258262 ) ) ;
#122693=CARTESIAN_POINT ( 'NONE',  ( 16.53943276465976808, 0.05219959533934440121, 106.2510903946856757 ) ) ;
#122695=CARTESIAN_POINT ( 'NONE',  ( -0.05219959533936034679, 19.03943276465977164, 112.5010903946856757 ) ) ;
#122696=CARTESIAN_POINT ( 'NONE',  ( -16.55341960407611168, -4.379528057220339221, 76.45724293864769550 ) ) ;
#122697=DIRECTION ( 'NONE',  ( 1.000000000000000000, -0.000000000000000000, -0.000000000000000000 ) ) ;
#122698=CARTESIAN_POINT ( 'NONE',  ( 16.51473224551069308, 9.474510206698969483, 69.16557627198102409 ) ) ;
#122699=CARTESIAN_POINT ( 'NONE',  ( -16.46253265017160317, 9.564922557960807481, 30.83224293864769550 ) ) ;
#122700=CARTESIAN_POINT ( 'NONE',  ( 16.53943276465976808, -0.05219959533910856209, 68.74890960531435269 ) ) ;
#122701=CARTESIAN_POINT ( 'NONE',  ( -13.89961937509977652, 13.97604488694528158, 115.6239096053143669 ) ) ;
#122702=CARTESIAN_POINT ( 'NONE',  ( -13.97604488694547697, 13.89961937509957934, 83.12609039468564731 ) ) ;
#122703=CARTESIAN_POINT ( 'NONE',  ( 5.153800228976335163, 19.02544592524342804, 99.79057627198102409 ) ) ;
#122704=CARTESIAN_POINT ( 'NONE',  ( -21.55341960407610458, -5.719274019375992779, 71.45724293864769550 ) ) ;
#122705=CARTESIAN_POINT ( 'NONE',  ( 14.29746914071037800, 8.314922557961029526, 66.66775706135234714 ) ) ;
#122706=CARTESIAN_POINT ( 'NONE',  ( 9.474510206698729675, 16.51473224551082808, 107.0844237280190043 ) ) ;
#122707=CARTESIAN_POINT ( 'NONE',  ( 16.51473224551069308, 9.474510206698969483, 59.16557627198102409 ) ) ;
#122708=CARTESIAN_POINT ( 'NONE',  ( -15.80617190586745835, -15.72974639402198527, 66.87390960531436690 ) ) ;
#122709=CARTESIAN_POINT ( 'NONE',  ( 13.89961937509957401, 13.97604488694547697, 106.8760903946856757 ) ) ;
#122710=CARTESIAN_POINT ( 'NONE',  ( 12.06949235617757843, -12.14591786802309237, 43.12390960531435269 ) ) ;
#122711=CARTESIAN_POINT ( 'NONE',  ( 15.80617190586769283, -15.72974639402175789, 65.62609039468568994 ) ) ;
#122712=CARTESIAN_POINT ( 'NONE',  ( 13.89961937509957579, 13.97604488694547520, 71.87609039468567573 ) ) ;
#122713=CARTESIAN_POINT ( 'NONE',  ( -4.483927247898782831, 16.52544592524335698, 72.70942372801901854 ) ) ;
#122714=CARTESIAN_POINT ( 'NONE',  ( -5.049401038298153566, 19.05341960407611168, 110.2072429386476671 ) ) ;
#122716=CARTESIAN_POINT ( 'NONE',  ( -17.40861289039002813, 6.110651285853254677, 78.62767529172566583 ) ) ;
#122717=CARTESIAN_POINT ( 'NONE',  ( 0.05219959533934541429, -16.53943276465976808, 95.00109039468568994 ) ) ;
#122718=CARTESIAN_POINT ( 'NONE',  ( 8.224510206698742110, 14.34966873604972548, 47.08442372801901854 ) ) ;
#122719=CARTESIAN_POINT ( 'NONE',  ( -13.97604488694527625, -13.89961937509977652, 61.87390960531435979 ) ) ;
#122720=CARTESIAN_POINT ( 'NONE',  ( -9.474510206698964154, 16.51473224551069663, 70.41557627198102409 ) ) ;
#122721=CARTESIAN_POINT ( 'NONE',  ( -15.72974639402176322, -15.80617190586768395, 64.37609039468568994 ) ) ;
#122722=CARTESIAN_POINT ( 'NONE',  ( -16.52544592524335698, -4.483927247898792601, 58.95942372801902565 ) ) ;
#122723=CARTESIAN_POINT ( 'NONE',  ( 14.29746914071049879, -8.314922557960816363, 33.33224293864769550 ) ) ;
#122724=CARTESIAN_POINT ( 'NONE',  ( 5.153800228976335163, 19.02544592524342804, 44.79057627198103830 ) ) ;
#122725=CARTESIAN_POINT ( 'NONE',  ( 19.03943276465977164, -0.05219959533909143690, 33.74890960531435979 ) ) ;
#122726=CARTESIAN_POINT ( 'NONE',  ( -14.34966873604972548, 8.224510206698743886, 23.33442372801901499 ) ) ;
#122727=CARTESIAN_POINT ( 'NONE',  ( -19.03943276465977164, -0.05219959533935918106, 78.75109039468567573 ) ) ;
#122728=CARTESIAN_POINT ( 'NONE',  ( 0.05219959533910956823, 16.53943276465976808, 99.99890960531436690 ) ) ;
#122729=CARTESIAN_POINT ( 'NONE',  ( 13.97604488694527802, 13.89961937509977652, 49.37390960531434558 ) ) ;
#122730=CARTESIAN_POINT ( 'NONE',  ( 13.97604488694548053, -13.89961937509957401, 90.62609039468567573 ) ) ;
#122732=CARTESIAN_POINT ( 'NONE',  ( -5.823673210054431948, 21.52544592524334988, 92.70942372801901854 ) ) ;
#122733=CARTESIAN_POINT ( 'NONE',  ( 14.29746914071037800, 8.314922557961029526, 56.66775706135235424 ) ) ;
#122734=CARTESIAN_POINT ( 'NONE',  ( -17.49999999999999645, 5.499999999999997335, 25.79690382534172244 ) ) ;
#122735=CARTESIAN_POINT ( 'NONE',  ( 15.72974639402199770, -15.80617190586745480, 43.12390960531435269 ) ) ;
#122736=CARTESIAN_POINT ( 'NONE',  ( -14.29746914071037622, -8.314922557961029526, 34.16775706135234714 ) ) ;
#122737=CARTESIAN_POINT ( 'NONE',  ( -9.474510206698964154, 16.51473224551069663, 35.41557627198102409 ) ) ;
#122738=CARTESIAN_POINT ( 'NONE',  ( 9.474510206698729675, 16.51473224551082808, 47.08442372801900433 ) ) ;
#122739=CARTESIAN_POINT ( 'NONE',  ( -13.97604488694527625, -13.89961937509977652, 86.87390960531436690 ) ) ;
#122740=CARTESIAN_POINT ( 'NONE',  ( 9.564922557960805705, 16.46253265017160317, 49.58224293864770260 ) ) ;
#122742=CARTESIAN_POINT ( 'NONE',  ( -10.81492255796105439, 18.62759615963255655, 72.91775706135234714 ) ) ;
#122744=CARTESIAN_POINT ( 'NONE',  ( 13.89961937509957401, 13.97604488694547697, 36.87609039468565442 ) ) ;
#122745=CARTESIAN_POINT ( 'NONE',  ( 21.53943276465977519, 0.05219959533937863772, 106.2510903946856757 ) ) ;
#122746=CARTESIAN_POINT ( 'NONE',  ( -12.14591786802309592, -12.06949235617757132, 56.87390960531436690 ) ) ;
#122747=CARTESIAN_POINT ( 'NONE',  ( -19.02544592524342804, 5.153800228976336051, 56.04057627198100988 ) ) ;
#122748=CARTESIAN_POINT ( 'NONE',  ( -5.153800228976328057, -19.02544592524343514, 107.2905762719810383 ) ) ;
#122749=CARTESIAN_POINT ( 'NONE',  ( 5.719274019375673035, 21.55341960407619339, 87.29275706135236135 ) ) ;
#122750=CARTESIAN_POINT ( 'NONE',  ( -19.03943276465977164, 0.05219959533909376836, 66.24890960531436690 ) ) ;
#122751=EDGE_CURVE ( 'NONE', #46822, #129974, #117271, .T. ) ;
#122752=CARTESIAN_POINT ( 'NONE',  ( -5.719274019375665041, -21.55341960407619695, 84.79275706135234714 ) ) ;
#122753=CARTESIAN_POINT ( 'NONE',  ( -15.80617190586745835, -15.72974639402198527, 36.87390960531435979 ) ) ;
#122754=CARTESIAN_POINT ( 'NONE',  ( -0.05219959533937732626, 21.53943276465977519, 27.50109039468567929 ) ) ;
#122755=CARTESIAN_POINT ( 'NONE',  ( -9.564922557961040184, 16.46253265017147172, 52.91775706135233293 ) ) ;
#122756=CARTESIAN_POINT ( 'NONE',  ( 5.153800228976335163, 19.02544592524342804, 34.79057627198102409 ) ) ;
#122757=CARTESIAN_POINT ( 'NONE',  ( -5.049401038298153566, 19.05341960407611168, 70.20724293864769550 ) ) ;
#122758=CARTESIAN_POINT ( 'NONE',  ( -0.05219959533934338120, 16.53943276465976808, 32.50109039468568284 ) ) ;
#122759=CARTESIAN_POINT ( 'NONE',  ( 0.05219959533910956823, 16.53943276465976808, 84.99890960531436690 ) ) ;
#122760=CARTESIAN_POINT ( 'NONE',  ( 13.89961937509977652, -13.97604488694527269, 53.12390960531434558 ) ) ;
#122761=CARTESIAN_POINT ( 'NONE',  ( -18.67979575497178146, -10.72451020669898902, 36.66557627198103120 ) ) ;
#122762=VECTOR ( 'NONE', #173615, 1000.000000000000000 ) ;
#122763=CARTESIAN_POINT ( 'NONE',  ( 5.049401038297881783, 19.05341960407617563, 107.2927570613523187 ) ) ;
#122764=CARTESIAN_POINT ( 'NONE',  ( -5.719274019375978568, 21.55341960407610458, 110.2072429386477239 ) ) ;
#122765=CARTESIAN_POINT ( 'NONE',  ( 5.823673210054444382, -21.52544592524334988, 75.20942372801901854 ) ) ;
#122766=CARTESIAN_POINT ( 'NONE',  ( 4.379528057220092307, 16.55341960407617563, 67.29275706135234714 ) ) ;
#122767=CARTESIAN_POINT ( 'NONE',  ( 16.53943276465976808, 0.05219959533934440121, 66.25109039468567573 ) ) ;
#122768=CARTESIAN_POINT ( 'NONE',  ( -5.153800228976328057, -19.02544592524343514, 62.29057627198100988 ) ) ;
#122769=CARTESIAN_POINT ( 'NONE',  ( -12.06949235617739369, -12.14591786802326823, 94.37609039468568994 ) ) ;
#122770=CARTESIAN_POINT ( 'NONE',  ( -0.05219959533936034679, 19.03943276465977164, 47.50109039468566863 ) ) ;
#122771=CARTESIAN_POINT ( 'NONE',  ( -15.80617190586768217, 15.72974639402176855, 23.12609039468567573 ) ) ;
#122772=CARTESIAN_POINT ( 'NONE',  ( 14.29746914071049879, -8.314922557960816363, 68.33224293864769550 ) ) ;
#122773=CARTESIAN_POINT ( 'NONE',  ( -0.05219959533909027116, -19.03943276465977164, 82.49890960531436690 ) ) ;
#122774=CARTESIAN_POINT ( 'NONE',  ( -4.483927247898782831, 16.52544592524335698, 72.70942372801901854 ) ) ;
#122775=CARTESIAN_POINT ( 'NONE',  ( 18.62759615963255655, 10.81492255796105972, 56.66775706135235424 ) ) ;
#122776=CARTESIAN_POINT ( 'NONE',  ( 13.89961937509957401, 13.97604488694547697, 111.8760903946856757 ) ) ;
#122777=CARTESIAN_POINT ( 'NONE',  ( -5.823673210054116645, -21.52544592524344225, 107.2905762719810525 ) ) ;
#122778=CARTESIAN_POINT ( 'NONE',  ( -16.52544592524342804, 4.483927247898546575, 56.04057627198102409 ) ) ;
#122779=ORIENTED_EDGE ( 'NONE', *, *, #134567, .F. ) ;
#122780=CARTESIAN_POINT ( 'NONE',  ( -5.719274019375978568, 21.55341960407610458, 90.20724293864770971 ) ) ;
#122781=CARTESIAN_POINT ( 'NONE',  ( -16.55341960407611168, -4.379528057220339221, 41.45724293864769550 ) ) ;
#122784=CARTESIAN_POINT ( 'NONE',  ( -5.719274019375665041, -21.55341960407619695, 19.79275706135235069 ) ) ;
#122785=CARTESIAN_POINT ( 'NONE',  ( 13.97604488694527802, 13.89961937509977652, 114.3739096053143669 ) ) ;
#122786=CARTESIAN_POINT ( 'NONE',  ( 5.719274019375673035, 21.55341960407619339, 32.29275706135235424 ) ) ;
#122787=CARTESIAN_POINT ( 'NONE',  ( -16.52544592524342804, 4.483927247898546575, 46.04057627198103830 ) ) ;
#122789=CARTESIAN_POINT ( 'NONE',  ( -0.05219959533909027116, -19.03943276465977164, 62.49890960531435979 ) ) ;
#122790=CARTESIAN_POINT ( 'NONE',  ( 16.51473224551083163, -9.474510206698727899, 60.83442372801900433 ) ) ;
#122791=CARTESIAN_POINT ( 'NONE',  ( 19.03943276465977164, -0.05219959533909143690, 98.74890960531436690 ) ) ;
#122792=CARTESIAN_POINT ( 'NONE',  ( -0.05219959533907301413, -21.53943276465977519, 42.49890960531435979 ) ) ;
#122794=CARTESIAN_POINT ( 'NONE',  ( 13.89961937509977652, -13.97604488694527269, 53.12390960531434558 ) ) ;
#122795=CARTESIAN_POINT ( 'NONE',  ( 16.55341960407618274, -4.379528057220086978, 36.04275706135234714 ) ) ;
#122796=CARTESIAN_POINT ( 'NONE',  ( -9.564922557961040184, 16.46253265017147172, 67.91775706135233293 ) ) ;
#122797=CARTESIAN_POINT ( 'NONE',  ( 18.62759615963271287, -10.81492255796078972, 113.3322429386476955 ) ) ;
#122798=CARTESIAN_POINT ( 'NONE',  ( -14.34966873604960291, -8.224510206698953496, 46.66557627198102409 ) ) ;
#122799=CARTESIAN_POINT ( 'NONE',  ( -19.02544592524342804, 5.153800228976336051, 91.04057627198100988 ) ) ;
#122800=CARTESIAN_POINT ( 'NONE',  ( -15.80617190586745835, -15.72974639402198527, 76.87390960531439532 ) ) ;
#122801=CARTESIAN_POINT ( 'NONE',  ( 21.55341960407610458, 5.719274019375980345, 113.9572429386477239 ) ) ;
#122802=CARTESIAN_POINT ( 'NONE',  ( -12.14591786802326823, 12.06949235617739902, 43.12609039468568284 ) ) ;
#122803=CARTESIAN_POINT ( 'NONE',  ( -18.67979575497178146, -10.72451020669898902, 36.66557627198103120 ) ) ;
#122804=CARTESIAN_POINT ( 'NONE',  ( -15.80617190586768217, 15.72974639402176855, 108.1260903946856757 ) ) ;
#122805=CARTESIAN_POINT ( 'NONE',  ( -16.46253265017160317, 9.564922557960807481, 85.83224293864769550 ) ) ;
#122806=CARTESIAN_POINT ( 'NONE',  ( 5.049401038298161559, -19.05341960407611168, 47.70724293864770260 ) ) ;
#122807=CARTESIAN_POINT ( 'NONE',  ( 13.89961937509977652, -13.97604488694527269, 98.12390960531433848 ) ) ;
#122808=CARTESIAN_POINT ( 'NONE',  ( -16.51473224551069308, -9.474510206698971260, 76.66557627198103830 ) ) ;
#122809=CARTESIAN_POINT ( 'NONE',  ( -12.06949235617739369, -12.14591786802326823, 24.37609039468567573 ) ) ;
#122810=CARTESIAN_POINT ( 'NONE',  ( 17.49999999999997513, 3.805241302050415442, 32.12647527217407628 ) ) ;
#122811=CARTESIAN_POINT ( 'NONE',  ( -9.564922557961040184, 16.46253265017147172, 52.91775706135233293 ) ) ;
#122812=CARTESIAN_POINT ( 'NONE',  ( -19.03943276465977164, -0.05219959533935918106, 18.75109039468567218 ) ) ;
#122813=CARTESIAN_POINT ( 'NONE',  ( 5.823673210054125526, 21.52544592524343514, 29.79057627198102409 ) ) ;
#122814=CARTESIAN_POINT ( 'NONE',  ( 4.483927247898790824, -16.52544592524335698, 100.2094237280190043 ) ) ;
#122816=CARTESIAN_POINT ( 'NONE',  ( -13.89961937509957401, -13.97604488694547875, 69.37609039468564731 ) ) ;
#122817=CARTESIAN_POINT ( 'NONE',  ( 19.05341960407617918, -5.049401038297876454, 26.04275706135233293 ) ) ;
#122818=CARTESIAN_POINT ( 'NONE',  ( -16.79531203550650176, -7.028104445595492855, 46.25244988220443787 ) ) ;
#122819=CARTESIAN_POINT ( 'NONE',  ( -9.474510206698964154, 16.51473224551069663, 35.41557627198102409 ) ) ;
#122820=CARTESIAN_POINT ( 'NONE',  ( -16.52544592524342804, 4.483927247898546575, 31.04057627198102409 ) ) ;
#122821=CARTESIAN_POINT ( 'NONE',  ( -16.18388926212238843, -7.379444403734516378, 110.4395315136615068 ) ) ;
#122822=CARTESIAN_POINT ( 'NONE',  ( 12.14591786802309770, 12.06949235617756955, 29.37390960531435269 ) ) ;
#122823=DIRECTION ( 'NONE',  ( -0.000000000000000000, -0.000000000000000000, 1.000000000000000000 ) ) ;
#122824=CARTESIAN_POINT ( 'NONE',  ( -14.34966873604972548, 8.224510206698743886, 98.33442372801901854 ) ) ;
#122825=CARTESIAN_POINT ( 'NONE',  ( 13.97604488694527802, 13.89961937509977652, 34.37390960531436690 ) ) ;
#122826=EDGE_CURVE ( 'NONE', #115310, #169831, #131232, .T. ) ;
#122827=CARTESIAN_POINT ( 'NONE',  ( -10.81492255796105439, 18.62759615963255655, 107.9177570613523471 ) ) ;
#122828=CARTESIAN_POINT ( 'NONE',  ( -12.14591786802326823, 12.06949235617739902, 23.12609039468567573 ) ) ;
#122829=CARTESIAN_POINT ( 'NONE',  ( -21.55341960407619339, 5.719274019375674811, 78.54275706135236135 ) ) ;
#122830=CARTESIAN_POINT ( 'NONE',  ( -9.474510206698720793, -16.51473224551083518, 59.58442372801900433 ) ) ;
#122831=CARTESIAN_POINT ( 'NONE',  ( 5.049401038298161559, -19.05341960407611168, 97.70724293864766707 ) ) ;
#122832=CARTESIAN_POINT ( 'NONE',  ( -19.03943276465977164, 0.05219959533909376836, 81.24890960531436690 ) ) ;
#122834=CARTESIAN_POINT ( 'NONE',  ( -15.80617190586745835, -15.72974639402198527, 106.8739096053143811 ) ) ;
#122835=CARTESIAN_POINT ( 'NONE',  ( 16.53943276465976808, -0.05219959533910856209, 63.74890960531435979 ) ) ;
#122836=CARTESIAN_POINT ( 'NONE',  ( -21.53943276465977519, 0.05219959533907696930, 56.24890960531436690 ) ) ;
#122837=CARTESIAN_POINT ( 'NONE',  ( 9.564922557960805705, 16.46253265017160317, 59.58224293864769550 ) ) ;
#122838=CARTESIAN_POINT ( 'NONE',  ( -10.81492255796078084, -18.62759615963271287, 92.08224293864769550 ) ) ;
#122839=CARTESIAN_POINT ( 'NONE',  ( -14.29746914071037622, -8.314922557961029526, 89.16775706135236135 ) ) ;
#122842=CARTESIAN_POINT ( 'NONE',  ( 0.05219959533909260263, 19.03943276465977164, 59.99890960531436690 ) ) ;
#122843=CARTESIAN_POINT ( 'NONE',  ( -12.06949235617756955, 12.14591786802309770, 90.62390960531436690 ) ) ;
#122845=CARTESIAN_POINT ( 'NONE',  ( -16.46253265017160317, 9.564922557960807481, 55.83224293864769550 ) ) ;
#122846=CARTESIAN_POINT ( 'NONE',  ( -9.564922557961040184, 16.46253265017147172, 77.91775706135234714 ) ) ;
#122847=CARTESIAN_POINT ( 'NONE',  ( 12.14591786802309770, 12.06949235617756955, 84.37390960531438111 ) ) ;
#122848=CARTESIAN_POINT ( 'NONE',  ( 15.80617190586769283, -15.72974639402175789, 40.62609039468567573 ) ) ;
#122849=CARTESIAN_POINT ( 'NONE',  ( -9.474510206698964154, 16.51473224551069663, 40.41557627198103120 ) ) ;
#122850=CARTESIAN_POINT ( 'NONE',  ( -10.72451020669898014, 18.67979575497178502, 100.4155762719810241 ) ) ;
#122851=CARTESIAN_POINT ( 'NONE',  ( 14.29746914071049879, -8.314922557960816363, 93.33224293864769550 ) ) ;
#122853=CARTESIAN_POINT ( 'NONE',  ( -5.049401038298153566, 19.05341960407611168, 55.20724293864769550 ) ) ;
#122854=CARTESIAN_POINT ( 'NONE',  ( 19.20446147854529073, 5.499999999999904965, 46.88999695167679960 ) ) ;
#122855=CARTESIAN_POINT ( 'NONE',  ( 19.05341960407617918, -5.049401038297876454, 96.04275706135231871 ) ) ;
#122856=CARTESIAN_POINT ( 'NONE',  ( 5.153800228976335163, 19.02544592524342804, 114.7905762719810241 ) ) ;
#122857=CARTESIAN_POINT ( 'NONE',  ( -0.05219959533937732626, 21.53943276465977519, 37.50109039468568284 ) ) ;
#122858=CARTESIAN_POINT ( 'NONE',  ( 16.51473224551069308, 9.474510206698969483, 84.16557627198102409 ) ) ;
#122859=CARTESIAN_POINT ( 'NONE',  ( -13.89961937509957401, -13.97604488694547875, 64.37609039468567573 ) ) ;
#122860=CARTESIAN_POINT ( 'NONE',  ( -16.51473224551069308, -9.474510206698971260, 56.66557627198103120 ) ) ;
#122861=CARTESIAN_POINT ( 'NONE',  ( 4.379528057220339221, -16.55341960407611168, 77.70724293864770971 ) ) ;
#122862=CARTESIAN_POINT ( 'NONE',  ( 8.224510206698953496, -14.34966873604960469, 62.91557627198102409 ) ) ;
#122863=CARTESIAN_POINT ( 'NONE',  ( -19.03943276465977164, 0.05219959533909376836, 91.24890960531436690 ) ) ;
#122864=CARTESIAN_POINT ( 'NONE',  ( 18.62759615963271287, -10.81492255796078972, 98.33224293864769550 ) ) ;
#122865=CARTESIAN_POINT ( 'NONE',  ( 13.89961937509977652, -13.97604488694527269, 88.12390960531438111 ) ) ;
#122866=CARTESIAN_POINT ( 'NONE',  ( 5.153800228976615827, -19.02544592524334988, 30.20942372801900433 ) ) ;
#122867=CARTESIAN_POINT ( 'NONE',  ( -5.153800228976328057, -19.02544592524343514, 42.29057627198101699 ) ) ;
#122868=CARTESIAN_POINT ( 'NONE',  ( -12.14591786802309592, -12.06949235617757132, 36.87390960531435979 ) ) ;
#122869=CARTESIAN_POINT ( 'NONE',  ( 12.14591786802309770, 12.06949235617756955, 114.3739096053143527 ) ) ;
#122871=CARTESIAN_POINT ( 'NONE',  ( -5.823673210054431948, 21.52544592524334988, 27.70942372801901854 ) ) ;
#122872=CARTESIAN_POINT ( 'NONE',  ( 19.02544592524334988, 5.153800228976608722, 61.45942372801900433 ) ) ;
#122873=CARTESIAN_POINT ( 'NONE',  ( -8.314922557960811034, -14.29746914071050412, 32.08224293864769550 ) ) ;
#122874=CARTESIAN_POINT ( 'NONE',  ( -15.72974639402197994, 15.80617190586746368, 85.62390960531436690 ) ) ;
#122875=CARTESIAN_POINT ( 'NONE',  ( -19.02544592524342804, 5.153800228976336051, 116.0405762719810383 ) ) ;
#122876=CARTESIAN_POINT ( 'NONE',  ( 16.53943276465976808, -0.05219959533910856209, 73.74890960531433848 ) ) ;
#122877=CARTESIAN_POINT ( 'NONE',  ( -13.97604488694527625, -13.89961937509977652, 31.87390960531435979 ) ) ;
#122878=CARTESIAN_POINT ( 'NONE',  ( -13.89961937509957401, -13.97604488694547875, 24.37609039468565442 ) ) ;
#122879=CARTESIAN_POINT ( 'NONE',  ( 16.55341960407618274, -4.379528057220086978, 106.0427570613523471 ) ) ;
#122880=CARTESIAN_POINT ( 'NONE',  ( 16.55341960407618274, -4.379528057220086978, 56.04275706135235424 ) ) ;
#122881=CARTESIAN_POINT ( 'NONE',  ( -21.52544592524343514, 5.823673210054127303, 41.04057627198103120 ) ) ;
#122882=CARTESIAN_POINT ( 'NONE',  ( 21.53943276465977519, 0.05219959533937863772, 101.2510903946856757 ) ) ;
#122883=CARTESIAN_POINT ( 'NONE',  ( -0.05219959533909027116, -19.03943276465977164, 77.49890960531435269 ) ) ;
#122884=CARTESIAN_POINT ( 'NONE',  ( 4.379528057220092307, 16.55341960407617563, 77.29275706135234714 ) ) ;
#122885=CARTESIAN_POINT ( 'NONE',  ( -13.97604488694527625, -13.89961937509977652, 21.87390960531435979 ) ) ;
#122886=CARTESIAN_POINT ( 'NONE',  ( -16.53943276465976808, 0.05219959533911058130, 41.24890960531435269 ) ) ;
#122887=CARTESIAN_POINT ( 'NONE',  ( 16.46253265017160672, -9.564922557960803928, 103.3322429386476955 ) ) ;
#122888=CARTESIAN_POINT ( 'NONE',  ( 13.89961937509977652, -13.97604488694527269, 88.12390960531438111 ) ) ;
#122889=CARTESIAN_POINT ( 'NONE',  ( -19.02544592524342804, 5.153800228976336051, 106.0405762719810241 ) ) ;
#122890=CARTESIAN_POINT ( 'NONE',  ( -4.483927247898539470, -16.52544592524342804, 62.29057627198102409 ) ) ;
#122891=CARTESIAN_POINT ( 'NONE',  ( 14.34966873604960469, 8.224510206698951720, 29.16557627198103120 ) ) ;
#122893=CARTESIAN_POINT ( 'NONE',  ( 4.379528057220339221, -16.55341960407611168, 57.70724293864770260 ) ) ;
#122894=CARTESIAN_POINT ( 'NONE',  ( 14.29746914071037800, 8.314922557961029526, 46.66775706135234714 ) ) ;
#122896=CARTESIAN_POINT ( 'NONE',  ( 16.51473224551083163, -9.474510206698727899, 55.83442372801899722 ) ) ;
#122897=CARTESIAN_POINT ( 'NONE',  ( 19.03943276465977164, -0.05219959533909143690, 88.74890960531436690 ) ) ;
#122898=CARTESIAN_POINT ( 'NONE',  ( 9.564922557961047289, -16.46253265017146816, 70.41775706135233293 ) ) ;
#122900=CARTESIAN_POINT ( 'NONE',  ( 13.97604488694548053, -13.89961937509957401, 60.62609039468564731 ) ) ;
#122901=CARTESIAN_POINT ( 'NONE',  ( 9.474510206698729675, 16.51473224551082808, 92.08442372801900433 ) ) ;
#122902=CARTESIAN_POINT ( 'NONE',  ( -12.06949235617739369, -12.14591786802326823, 84.37609039468570415 ) ) ;
#122904=CARTESIAN_POINT ( 'NONE',  ( 16.46253265017160672, -9.564922557960803928, 28.33224293864769550 ) ) ;
#122905=( BOUNDED_SURFACE ( )  B_SPLINE_SURFACE ( 3, 2, ( 
 ( #16987, #168665, #13995, #30165, #48328, #109983, #33152, #156489, #106005, #137339, #152506, #91809, #153501, #14998, #76658, #138337, #61484, #161467, #82606, #81601, #113940, #130102, #143285, #37113, #51295, #6769, #188831, #142305, #160466, #65462, #159453, #5776, #128120, #67451, #129109, #175639, #4771, #49312, #127125, #99782, #176652, #22957, #97766, #84605, #144287, #110972, #190808, #66458, #172656, #38128, #189823, #146284, #131121, #52282, #68448, #112956, #7771, #174649, #36114, #20949, #98772, #83607, #21957, #145286, #19959, #191799, #53280, #114959, #69454, #35130, #34144, #95803, #157489, #18982, #80628, #3785, #50315, #111971, #173663, #96782, #158471, #116954, #192809, #151301, #166474, #180657, #102792, #100775, #103794, #149301, #56285, #115963, #132125, #25972, #134137, #27972, #177651, #147301, #85614, #89612, #196817, #117967, #101787, #179658, #150309, #165474, #10795, #178646, #11806, #73470, #87615, #58284, #12790, #43118, #8790, #195826, #24972, #72463, #40109, #41128, #163475, #119953, #162458, #26970, #181638, #135143, #104786, #57297, #74455, #118974, #42133, #54291, #133122, #39119, #70460, #193818, #88613, #86618, #23959, #55283, #148301, #9795, #164478, #71457, #194811, #76423, #14762, #106762, #91572, #138099, #184607, #77415, #121928, #63237, #48086, #94567, #47089, #199780, #108750, #154265, #153260, #15756, #46088, #182631, #60257, #136121, #156246, #109742, #123901, #107743, #44115, #170426, #92577, #61247, #59263, #75431, #169424, #139085, #171426, #120932, #90597, #28956, #32913, #140071, #122919, #45105, #30929, #93572, #31918, #562, #183622, #155257, #16746, #62233, #1562, #17748, #186614, #152279, #185600, #168437, #78395, #29933, #124916, #197797, #105773, #167460, #13763, #137105, #198791, #129859, #174409, #37884, #5533, #35878, #79404, #19721, #68206, #172414, #18740, #144051, #188589, #110732, #21716, #161224, #2560, #83369, #80387, #126883, #191557, #112716, #111731, #67212, #160225, #173418, #128870, #81363, #36866, #142059, #33902, #190570, #95559, #189582, #97524, #158231, #159212, #20706, #52046, #34888, #141075, #157246, #53034, #6527, #114716, #127878, #176408, #82362, #64242, #113702, #96543, #125909, #99542, #143047, #187607, #49076, #175398, #98532, #4525, #3545, #66218, #65223, #145046, #50070, #51054, #148063, #23720, #22718, #41890, #104546, #26727, #196579, #116717, #87380, #103557, #181403, #58049, #133891, #11565, #84366, #165232, #180418, #146043, #10553, #149065, #131890, #195583, #192569, #57055, #86378, #177414, #130879, #134902, #55046, #179416, #7527, #54052, #69211, #119719, #115727, #88366, #178406, #38885, #118730, #150059, #42881, #100542, #164238, #162221, #72217, #85368, #193574, #40881, #147062, #8544, #70222, #9554, #73231, #25734, #39870, #101536, #163229, #24729, #71220, #117720, #132883, #194572, #56042, #102554, #59024, #62990, #120691, #106516, #139822, #155009, #152038, #14513, #45846, #1311, #15513, #153013, #186364, #183379, #76174, #124668, #61004, #43868, #168194, #185352, #78154, #89371, #105533, #184365, #29691, #60016, #137854, #138840, #47844, #61988, #12551, #75188, #135885, #199534, #320, #91322, #77170, #92332, #170182, #31676, #151060, #74217, #197556, #46843, #107499, #123654, #169175, #167219, #182390, #28716, #122676, #30680, #154018, #16506, #108502, #90353, #93325, #166227, #27728, #13523, #136860, #198546, #121683, #44861, #65968, #188340, #127638, #189338, #35636, #141814, #109497, #187362, #159976, #36618, #85888, #157989, #24238, #142807, #171179, #50816, #3307, #32667, #98275, #49819, #147576, #194092, #4287, #66968, #126638, #9062, #111483, #173168, #96303, #97281, #143802, #34644, #19480, #80144, #64980, #81126, #112473, #174166, #95313, #70732, #132399, #94320, #20461, #158969, #82111, #5285, #128628, #190321, #51798, #155998, #33652, #17494, #79152, #140823, #113457, #175150 ),
 ( #2312, #63993, #18496, #125664, #48831, #110484, #172167, #156998, #74720, #136383, #88883, #121203, #90852, #106035, #10063, #197080, #87878, #150575, #41397, #180921, #103062, #59526, #25247, #28241, #182895, #198060, #167721, #12074, #14024, #181903, #73736, #55554, #196097, #44379, #148573, #195083, #120213, #164744, #86888, #29219, #137369, #178921, #152537, #56563, #26239, #75690, #135409, #149566, #43381, #117227, #11062, #105053, #57567, #13053, #118239, #58547, #40389, #166737, #102062, #71723, #89881, #72738, #134411, #42396, #179930, #163747, #133392, #119237, #104059, #165739, #27234, #151564, #79674, #157518, #34173, #110012, #187872, #199048, #18021, #156521, #122193, #186888, #63517, #108013, #171693, #168695, #33182, #62506, #153531, #107023, #111002, #31192, #155523, #60518, #30196, #183885, #172688, #80658, #64510, #92844, #15028, #94841, #141345, #19012, #45370, #140347, #91838, #48358, #95834, #169698, #17018, #76689, #138365, #200046, #185878, #2832, #1835, #125192, #61515, #126177, #123184, #184873, #93844, #49340, #46355, #154529, #16026, #77684, #139352, #832, #124177, #47364, #109019, #170698, #32187, #78671, #115993, #191831, #129141, #162489, #159485, #52314, #39150, #37145, #19988, #144319, #161499, #54321, #65492, #81631, #160498, #82636, #36145, #113972, #114990, #23990, #38159, #188862, #51326, #112004, #190838, #176684, #67482, #53312, #68479, #146314, #7803, #127154, #50345, #173693, #22989, #21988, #99813, #83640, #143314, #35160, #4801, #175670, #98804, #6801, #192841, #130134, #96815, #3814, #158501, #145318, #131152, #66490, #84637, #69487, #128153, #100806, #189853, #5808, #177682, #142334, #112987, #174680, #97797, #20979, #135173, #72494, #105803, #102823, #195856, #182660, #180687, #163506, #87644, #104815, #197826, #8821, #25004, #103823, #26002, #179688, #57328, #58313, #167490, #181667, #132156, #194843, #55314, #134168, #119981, #10824, #196846, #11836, #89642, #151330, #70490, #193849, #116985, #166504, #165503, #43146, #26999, #86648, #178678, #148331, #119004, #42163, #150340, #136151, #73501, #40141, #88644, #28002, #12818, #147334, #101818, #74485, #56317, #164508, #59292, #9827, #85647, #120961, #71487, #44144, #133153, #41160, #117999, #149330, #187636, #64271, #140101, #17778, #28985, #48115, #186644, #152308, #16777, #93601, #138129, #1592, #198820, #63267, #92604, #183651, #137133, #141104, #61277, #185628, #90626, #60285, #13794, #2592, #110764, #94598, #122948, #45134, #124948, #109771, #49106, #75459, #170456, #121958, #78426, #125937, #199810, #47120, #106792, #168466, #29964, #15784, #171455, #31947, #155287, #91602, #32943, #153291, #156277, #14792, #184636, #79433, #76452, #46117, #107770, #169456, #30957, #154294, #77443, #139115, #591, #62262, #123930, #108778, #52077, #80418, #175430, #127910, #3576, #18771, #129889, #19752, #20738, #33933, #142090, #172445, #53068, #95591, #68236, #4558, #111761, #36899, #83398, #157275, #65254, #98563, #173450, #145076, #126914, #174439, #160257, #188620, #50101, #158262, #113733, #37913, #6558, #191589, #81393, #34918, #143079, #66250, #21747, #96574, #51086, #189612, #112746, #67242, #35909, #128901, #114746, #97555, #159243, #176440, #82394, #144082, #5563, #190600, #139744, #173097, #170102, #62911, #49742, #47766, #30601, #154930, #172092, #64907, #76096, #92254, #171098, #93245, #46767, #124591, #125589, #34574, #48757, #199456, #61910, #122598, #1232, #187286, #78075, #2237, #79076, #156927, #18424, #137771, #60924, #184288, #33579, #32590, #110410, #94243, #153938, #45769, #15433, #186286, #109419, #17419, #3233, #140749, #107421, #155923, #95242, #63920, #14433, #169094, #80074, #123580, #31596, #141743, #77091, #152934, #126568, #138760, #188267, #185275, #242, #111411, #108426, #16428, #38568, #35563, #143731, #8224, #129545, #128553, #160907, #177096, #190249, #84051, #98201 ),
 ( #97211, #96231, #115408, #178087, #100224, #69901, #51726, #22400, #161906, #54725, #131568, #7210, #85046, #157919, #23399, #53733, #19409, #145729, #68894, #5210, #130554, #65892, #192251, #159905, #50744, #4214, #193252, #113389, #52719, #81058, #127567, #142735, #116398, #189268, #146727, #175079, #112402, #174094, #158897, #20387, #82034, #37557, #66891, #36545, #21393, #83052, #114383, #144726, #6213, #67892, #191245, #176087, #99219, #49625, #121, #94123, #2119, #96115, #45649, #15310, #153815, #157803, #64793, #186165, #169982, #124468, #18303, #33463, #17300, #46642, #79959, #141628, #155802, #126454, #19294, #111287, #76969, #63801, #93125, #78954, #108302, #47647, #31473, #188152, #30477, #95121, #172977, #3118, #34456, #140629, #80942, #187170, #125474, #60803, #1113, #142617, #138640, #154810, #122476, #61790, #184167, #107300, #168972, #109298, #92128, #48641, #123460, #110293, #16308, #185152, #77958, #139625, #62787, #170977, #171975, #32470, #156811, #131441, #144607, #98079, #38443, #67771, #158778, #112284, #116275, #36424, #160787, #65775, #35442, #4096, #177965, #85936, #69773, #159777, #20266, #115281, #23278, #162779, #127444, #145607, #50623, #192124, #101093, #174960, #22275, #189150, #173974, #97094, #84922, #83926, #68767, #37435, #81912, #146602, #143605, #5089, #99095, #193128, #66771, #100099, #54601, #128432, #24287, #190129, #6092, #39433, #51604, #113268, #52600, #7086, #21272, #53605, #191126, #82929, #129428, #114262, #175966, #130425, #176974, #161783, #8095, #59577, #70780, #25297, #165790, #87929, #41447, #57616, #120259, #167768, #43433, #194139, #56614, #117277, #196144, #181951, #72789, #197126, #73785, #151610, #13102, #132448, #55603, #178971, #166788, #27287, #105102, #88933, #86939, #40438, #148623, #119284, #180967, #12121, #198110, #135457, #102110, #42444, #28289, #150625, #9113, #163795, #89929, #118288, #179979, #10113, #58593, #74767, #106082, #29266, #136429, #71773, #121251, #44428, #103112, #104108, #147625, #133443, #195133, #182945, #164793, #26288, #149616, #11114, #134459, #152583, #60564, #185926, #82441, #14073, #186937, #159289, #183930, #190649, #45415, #31241, #67290, #144129, #76735, #139397, #170746, #128948, #140396, #77731, #113781, #108062, #879, #52125, #47411, #168739, #92891, #110064, #5611, #75740, #30243, #109067, #154577, #184919, #62554, #63565, #175477, #48408, #137417, #200091, #122240, #124230, #125239, #16073, #1884, #17066, #97601, #20786, #199097, #107068, #91886, #171744, #32235, #33233, #93893, #153577, #15075, #138411, #155571, #78720, #90897, #61559, #123228, #46403, #169746, #56127, #55127, #98611, #53117, #71305, #7606, #115804, #162302, #37964, #36949, #117809, #118817, #40968, #10640, #130958, #101626, #179502, #195670, #72301, #148147, #25817, #160305, #102639, #194658, #21795, #24813, #133979, #163315, #116797, #192648, #132968, #100620, #191637, #145124, #149150, #69292, #193655, #83447, #68287, #6608, #57141, #129938, #164324, #86462, #114795, #9638, #178488, #54131, #87463, #23802, #176488, #99622, #161303, #177494, #39955, #22798, #84444, #146122, #38964, #85452, #147142, #8630, #70302, #131971, #199619, #138920, #62073, #121767, #26812, #168277, #77252, #151144, #136944, #180503, #41975, #165320, #61086, #60099, #44946, #13606, #88452, #122758, #103642, #150148, #75274, #169260, #11649, #76257, #45928, #73315, #401, #134986, #120771, #154100, #30767, #166317, #28799, #183460, #15594, #29774, #167303, #196664, #197640, #90438, #58133, #198633, #119802, #182472, #184448, #92414, #181487, #42965, #106601, #43953, #74300, #152124, #153097, #104628, #137935, #27814, #89455, #12635, #91409, #14601, #105615, #107583, #135969, #59106, #189424, #108587, #170264, #31758, #142889, #3389, #81208, #141898, #1395, #93407, #124755, #33737, #157084, #188425, #174252, #49902, #155093, #18580, #4371, #65064 ),
 ( #111569, #66054, #82196, #159053, #34728, #112557, #123738, #127722, #50899, #46927, #16587, #47927, #185437, #143889, #97367, #173253, #95398, #78235, #139906, #172250, #19564, #35720, #63076, #80227, #126721, #20547, #186451, #109581, #171264, #5370, #32752, #48915, #94403, #187447, #156084, #96386, #158073, #17580, #79241, #140912, #2398, #64077, #125747, #110569, #21550, #8384, #99377, #100382, #52873, #192408, #114544, #71058, #36703, #39708, #132724, #86216, #117555, #162060, #25576, #193409, #23556, #67054, #7364, #55882, #160063, #6367, #131727, #176244, #98364, #9392, #148902, #190409, #194412, #68047, #37715, #179254, #85204, #161060, #54884, #147906, #22555, #116558, #69049, #24567, #129699, #83210, #178247, #144885, #177252, #146892, #145881, #70059, #101371, #163060, #84201, #128712, #191396, #40720, #102389, #164077, #115565, #87220, #51885, #113544, #175238, #130714, #53890, #38724, #89208, #137691, #92167, #105370, #168037, #27568, #136698, #149890, #11396, #198379, #59856, #44699, #150901, #12395, #181245, #166067, #74057, #58865, #151878, #196420, #199376, #122515, #169011, #121523, #135728, #183218, #28558, #197399, #90195, #120531, #182224, #57890, #14351, #180257, #106353, #76016, #29534, #60840, #167057, #30515, #91167, #13368, #10392, #43708, #184205, #103391, #73066, #75032, #119562, #41727, #152856, #72049, #133723, #45687, #134738, #42722, #107338, #195415, #104384, #56893, #118567, #165069, #26563, #88206, #111326, #93165, #46682, #64830, #170022, #63837, #110330, #32509, #172011, #33500, #79997, #186204, #153853, #31512, #4135, #80981, #127483, #2159, #65814, #187207, #15351, #95159, #47686, #77007, #142656, #94161, #189188, #35483, #48678, #173016, #171018, #141665, #154850, #16347, #3157, #126492, #188190, #155840, #17337, #124509, #109336, #78993, #125510, #156847, #139663, #50661, #112322, #174012, #49662, #140667, #34495, #18342, #96153, #157842, #19333, #159, #77996, #138679, #61828, #123498, #185191, #108341, #1151, #62826, #145646, #193167, #85975, #36464, #130467, #38483, #132488, #81952, #51644, #190168, #194177, #101131, #22315, #6130, #160827, #54639, #69813, #53645, #82970, #116314, #178003, #192165, #162817, #55641, #147665, #113308, #100140, #129468, #115322, #144647, #70819, #191167, #161821, #39470, #117314, #179010, #8135, #9153, #97132, #24326, #158816, #20304, #84960, #143644, #23316, #177014, #52640, #131480, #83966, #174999, #5127, #66809, #114305, #146642, #128472, #98121, #159818, #21313, #67813, #176007, #37476, #99137, #7126, #68808, #199135, #122277, #181990, #86978, #28327, #137456, #11155, #197165, #40478, #102150, #25337, #121289, #120297, #105140, #73825, #148665, #59616, #163835, #10153, #135495, #29304, #71813, #136466, #106120, #133481, #60602, #195173, #181010, #14111, #90934, #26329, #88972, #43472, #75778, #89966, #27326, #56654, #57657, #150662, #118327, #58631, #180020, #42484, #182982, #152620, #41487, #103152, #166826, #104147, #134499, #12160, #13141, #164833, #198146, #87969, #149657, #72829, #151646, #74803, #165829, #44466, #167804, #196185, #119323, #168776, #30278, #91924, #2919, #63601, #141432, #1922, #61595, #153616, #184955, #93929, #17103, #48444, #34260, #110101, #15112, #78755, #64597, #125277, #45452, #200126, #18107, #154613, #62589, #109103, #46439, #183965, #126261, #65581, #187958, #142422, #94927, #124267, #156612, #186974, #139433, #171780, #155608, #76773, #108098, #107106, #3901, #157604, #33268, #140432, #138445, #123264, #32272, #79761, #172779, #169783, #49428, #111089, #19095, #31276, #92927, #16108, #80744, #95919, #170782, #77766, #47447, #915, #185962, #83723, #113070, #146397, #7886, #160583, #192926, #162573, #177764, #81717, #68562, #159571, #22072, #174762, #52400, #36228, #131238, #96900, #99895, #54404, #69572, #39233, #145402, #85732, #53398, #6884, #127240, #67568, #116076, #20073 ),
 ( #4891, #35247, #128238, #37233, #130219, #191914, #100889, #115076, #158584, #176768, #24076, #38240, #188954, #143402, #161580, #97880, #5892, #114059, #189935, #50431, #147419, #8906, #112090, #173780, #21069, #23074, #66573, #51410, #82725, #84719, #144406, #129226, #190923, #175756, #98889, #58398, #167575, #196930, #88732, #164589, #104900, #134255, #25088, #178763, #182746, #102905, #27086, #132242, #101905, #70574, #44231, #152391, #136235, #105888, #103907, #193934, #150427, #26083, #55397, #59379, #149412, #197909, #117067, #165588, #28089, #87727, #120064, #9910, #71570, #181752, #43234, #166589, #10908, #72581, #41243, #195942, #57416, #119089, #11922, #56402, #121051, #29069, #90708, #89729, #180771, #151415, #73586, #42246, #135258, #12903, #40228, #194927, #163587, #86730, #148415, #74567, #133235, #118084, #179774, #62349, #109858, #2682, #153378, #47207, #155376, #49195, #198905, #168549, #106876, #110853, #17868, #139203, #123034, #77531, #171543, #186733, #170545, #199899, #33031, #94687, #108866, #79523, #172538, #64359, #30047, #16865, #46204, #32036, #61363, #678, #184720, #141193, #183735, #48204, #126028, #156365, #187724, #93693, #34023, #140190, #78516, #13877, #154379, #95681, #91688, #14880, #1682, #107858, #45221, #75544, #137218, #60373, #122045, #76541, #169543, #138217, #63360, #31042, #125037, #92691, #15873, #124019, #185716, #114836, #96663, #50193, #68327, #173539, #67329, #113821, #35994, #175516, #36991, #83488, #189702, #157367, #35008, #7647, #84484, #130997, #5653, #177534, #174527, #128991, #54172, #52164, #158350, #159330, #176530, #69331, #80507, #19839, #98652, #97641, #51175, #190689, #129977, #39004, #53158, #3664, #66338, #127002, #160346, #191677, #82483, #6649, #145165, #161346, #22837, #142180, #65342, #188710, #38006, #21835, #99661, #146161, #81480, #111849, #143167, #192689, #115845, #18861, #4647, #128000, #112835, #20827, #144167, #118857, #162341, #116836, #137726, #71343, #179540, #25856, #101665, #100659, #122551, #185227, #107375, #77043, #194697, #165358, #184241, #61864, #138714, #14384, #92205, #23842, #45722, #60874, #85492, #88493, #195, #26852, #180540, #56166, #199410, #164361, #55165, #8669, #15386, #133006, #57180, #147180, #132009, #70342, #123533, #193696, #169047, #117847, #178526, #76050, #30553, #39993, #163355, #42014, #24851, #150190, #86500, #41009, #103679, #148184, #9678, #102676, #153889, #87500, #149188, #134016, #10677, #72342, #195708, #16383, #141699, #35519, #170057, #142690, #112359, #139699, #143682, #1185, #187241, #20340, #97167, #32542, #95195, #126525, #81989, #96188, #33533, #5163, #62862, #48711, #66846, #158852, #94195, #156881, #188224, #128509, #157877, #18378, #46718, #63874, #80030, #108381, #3190, #124544, #110364, #65848, #31548, #93200, #186241, #64863, #172046, #140702, #49697, #19366, #154885, #4170, #78030, #155875, #47719, #111362, #81015, #173051, #127518, #34528, #50700, #174050, #109370, #171052, #17372, #189222, #79027, #2192, #125545, #67847, #98156, #191202, #100178, #23354, #54678, #40518, #116352, #159856, #84999, #9192, #8175, #51683, #6167, #24364, #160863, #68848, #115362, #52677, #190204, #70857, #71852, #194215, #163877, #84005, #178041, #132526, #148704, #25376, #101169, #179050, #113345, #55680, #147704, #175037, #39509, #87018, #162857, #69851, #145683, #86015, #53685, #144682, #21349, #102189, #22353, #146680, #36502, #83007, #129502, #10192, #114340, #117354, #7165, #176043, #37511, #99173, #130507, #192203, #131519, #177052, #38522, #161860, #193205, #90003, #15148, #133521, #118367, #14148, #13177, #198183, #166863, #41529, #152658, #195213, #103192, #28365, #122314, #56693, #29342, #199173, #26368, #180060, #151685, #90971, #150701, #59653, #72869, #134538, #121327, #183019, #167841, #73864, #12199, #104186, #89010, #135533, #182028, #74840, #119364, #60640, #45488 ),
 ( #44503, #43511, #164873, #88008, #105177, #75815, #184005, #196226, #136503, #106159, #168813, #149696, #11194, #57696, #30317, #137493, #58667, #42523, #197204, #107143, #91960, #153653, #181048, #165868, #27364, #120333, #142454, #112120, #127272, #31311, #18140, #109138, #110134, #62624, #1957, #124302, #80776, #46476, #49459, #3932, #95952, #188986, #171813, #35277, #2951, #33301, #76810, #17138, #65612, #169820, #16145, #141467, #185999, #108136, #19126, #158614, #200162, #50461, #77800, #47481, #173812, #94960, #170817, #64630, #157637, #32309, #126292, #78790, #34291, #139469, #92964, #187989, #154650, #187008, #156645, #155643, #79794, #111121, #172811, #93963, #138481, #949, #96932, #61632, #123300, #125312, #184992, #140468, #63636, #48478, #114089, #81748, #8939, #98922, #147451, #36258, #54437, #190954, #160614, #145433, #21102, #20104, #39265, #101938, #24110, #193966, #175790, #84751, #100921, #178795, #55429, #131270, #70608, #143435, #162606, #177795, #4922, #7919, #117100, #146429, #38272, #37264, #116107, #83754, #174792, #128268, #132275, #52431, #176799, #66604, #51441, #189966, #40264, #113101, #85765, #22104, #97912, #192958, #159603, #82757, #144437, #161611, #5923, #69604, #67600, #6916, #99926, #129259, #68594, #130250, #191945, #23105, #53431, #115107, #71601, #182775, #25120, #133267, #58425, #152418, #86764, #59406, #29096, #56435, #60401, #118116, #103936, #137248, #13906, #149442, #11950, #43261, #198934, #12930, #150455, #183765, #180799, #73614, #122073, #120092, #41273, #165616, #44258, #75572, #148447, #102935, #181780, #27115, #57445, #135285, #136262, #45251, #121080, #9942, #72611, #194958, #196957, #197937, #88762, #74594, #89757, #167601, #90735, #179804, #164620, #26114, #105915, #104929, #163619, #166616, #87757, #10938, #134286, #28118, #151443, #195973, #119118, #42278, #76571, #140222, #126059, #125068, #168578, #157400, #34055, #80539, #155406, #18893, #1715, #106905, #186765, #710, #30076, #95713, #185751, #142213, #188742, #63391, #64391, #124052, #33063, #46236, #107890, #94718, #156396, #141223, #47240, #108898, #77563, #62382, #170577, #16896, #48235, #92722, #3696, #65375, #127035, #17900, #32068, #79555, #109890, #93724, #171574, #78547, #153411, #31075, #91717, #14910, #138246, #2714, #187756, #199930, #61393, #49226, #110884, #123065, #169577, #172569, #184751, #154411, #15905, #139235, #143199, #85522, #54203, #175549, #159364, #113853, #7677, #22867, #6679, #36026, #69361, #131030, #83519, #115875, #147210, #100688, #4680, #191707, #82518, #145196, #97675, #37024, #20861, #177564, #19872, #84514, #39033, #192719, #162370, #68357, #8701, #176561, #130008, #50227, #190722, #23871, #66372, #189734, #114866, #144200, #81512, #70371, #132039, #173571, #111881, #51207, #5686, #35040, #53191, #67362, #38036, #96694, #129021, #99692, #52195, #158383, #112868, #128032, #161376, #174559, #160378, #146192, #98685, #21869, #180571, #88525, #41039, #193728, #9708, #42045, #55196, #26882, #25886, #178556, #12702, #149218, #89525, #116865, #165389, #166387, #10709, #196733, #56196, #117879, #135057, #58201, #43033, #134046, #72372, #87531, #195739, #57212, #103709, #11718, #102705, #74368, #197708, #40022, #181554, #118887, #104699, #73385, #150221, #119869, #27883, #86530, #164393, #101695, #163384, #24881, #151214, #136034, #194726, #179569, #59174, #148214, #71372, #133036, #7323, #115524, #9354, #159011, #128670, #67011, #71019, #178206, #99337, #83168, #37672, #131687, #146849, #130673, #160020, #193368, #54844, #69007, #39670, #132687, #24527, #190366, #177212, #6326, #192367, #21507, #161020, #144842, #101332, #143848, #8343, #163020, #116518, #86178, #53850, #194375, #100341, #38685, #174209, #114501, #147868, #51842, #113501, #162020, #68006, #5327, #55842, #35677, #97325, #20504, #175196, #129658, #82152, #23516, #191354, #85162, #36661 ),
 ( #52832, #176203, #22514, #98320, #84161, #145841, #70018, #121485, #91129, #90156, #74019, #103354, #136659, #198339, #150862, #183179, #152819, #168000, #72011, #58826, #149854, #12356, #165032, #42684, #26525, #44661, #87182, #151839, #106314, #59815, #29496, #135689, #75978, #43669, #197361, #117516, #57853, #14312, #10354, #56855, #182184, #88170, #148863, #137651, #199338, #40680, #179213, #118530, #11358, #102350, #120493, #73029, #105331, #164039, #134701, #167019, #119525, #74994, #180219, #133684, #28520, #195376, #27529, #13329, #196384, #25538, #41689, #181208, #104345, #166029, #89170, #103916, #41252, #178773, #86740, #55407, #26092, #42254, #120071, #196937, #72590, #150434, #161589, #180779, #119097, #84728, #149421, #58405, #87736, #179783, #117077, #195951, #25098, #116085, #69581, #73593, #193944, #118093, #23083, #192936, #146406, #135266, #43241, #27094, #40239, #177773, #134264, #165596, #181759, #7896, #102914, #131247, #10917, #54413, #132253, #164598, #39243, #100899, #162583, #88740, #57424, #11929, #194937, #24087, #85742, #147429, #8916, #56413, #70584, #101915, #163597, #148425, #9920, #71579, #133245, #45228, #78522, #13882, #168555, #62356, #77538, #61369, #90713, #124026, #185725, #138223, #170552, #140196, #155382, #59384, #46210, #137225, #199905, #152396, #30053, #75549, #108872, #74572, #139210, #32042, #47214, #16871, #123040, #63366, #31048, #184726, #104908, #106882, #93699, #197914, #44236, #169550, #198910, #136240, #1690, #186739, #28096, #125043, #105893, #60378, #166596, #107864, #122050, #92697, #89735, #183741, #154385, #91694, #151421, #167580, #121058, #15880, #182752, #14886, #685, #153386, #12908, #29074, #76547, #80514, #48210, #126034, #98659, #50201, #158358, #110859, #52171, #81487, #109864, #128007, #142187, #171549, #36998, #127009, #175523, #129984, #143174, #5660, #65349, #174534, #187730, #49201, #36001, #97648, #82491, #188717, #111856, #18868, #3671, #173546, #96670, #189709, #34029, #160353, #21843, #6656, #159337, #35015, #20834, #66345, #19846, #51182, #4654, #94693, #172544, #33038, #68334, #83495, #144174, #112842, #156371, #17875, #67336, #128998, #145172, #95687, #190696, #113828, #79529, #141199, #2688, #64365, #157375, #195715, #116843, #57188, #10685, #42021, #86507, #150197, #117854, #148192, #191684, #132016, #180548, #84491, #131004, #56173, #100666, #22844, #134023, #73362, #114843, #118864, #192696, #39011, #103686, #24858, #23849, #179547, #72349, #85499, #41017, #193704, #149195, #54179, #146169, #102683, #7654, #101672, #9685, #70349, #71350, #133014, #164369, #147187, #53165, #69338, #165365, #55173, #163362, #115852, #26859, #194704, #176537, #25863, #8677, #38013, #88501, #178533, #11695, #99669, #87507, #161353, #40000, #177542, #162348, #136012, #61134, #122806, #169307, #75319, #13652, #105662, #90487, #136990, #183510, #76307, #120820, #62123, #46975, #93455, #45975, #198679, #107629, #153145, #152169, #14647, #44993, #181531, #59150, #135034, #155142, #108634, #184496, #106652, #43010, #104677, #168324, #30813, #123786, #74346, #29821, #137985, #170312, #119846, #89502, #27861, #31805, #138970, #60146, #44001, #121814, #92462, #154150, #91457, #182520, #15642, #77301, #199668, #448, #16635, #185485, #151191, #196710, #167349, #58179, #28847, #166364, #12680, #197685, #47976, #50946, #67100, #171312, #17630, #142935, #187495, #109629, #20593, #160110, #1445, #82245, #79290, #125793, #190458, #111617, #110615, #4416, #159099, #172297, #66102, #80273, #35766, #140959, #32799, #189468, #94451, #188472, #34777, #157131, #96433, #158120, #127768, #33786, #78282, #156131, #128759, #141944, #49953, #2446, #143936, #173302, #139955, #19611, #95446, #63123, #51931, #18626, #5417, #124802, #81253, #97412, #3434, #112605, #64128, #48961, #174297, #113591, #175285, #65110, #126768, #36750, #98414, #186500, #52919, #21598 ) ),
 .UNSPECIFIED., .T., .F., .F. ) 
 B_SPLINE_SURFACE_WITH_KNOTS ( ( 4, 3, 4 ),
 ( 3, 2, 2, 2, 2, 2, 2, 2, 2, 2, 2, 2, 2, 2, 2, 2, 2, 2, 2, 2, 2, 2, 2, 2, 2, 2, 2, 2, 2, 2, 2, 2, 2, 2, 2, 2, 2, 2, 2, 2, 2, 2, 2, 2, 2, 2, 2, 2, 2, 2, 2, 2, 2, 2, 2, 2, 2, 2, 2, 2, 2, 2, 2, 2, 2, 2, 2, 2, 2, 2, 2, 2, 2, 2, 2, 2, 2, 2, 2, 2, 2, 2, 2, 2, 2, 2, 2, 2, 2, 2, 2, 2, 2, 2, 2, 2, 2, 2, 2, 2, 2, 2, 2, 2, 2, 2, 2, 2, 2, 2, 2, 2, 2, 2, 2, 2, 2, 2, 2, 2, 2, 2, 2, 2, 2, 2, 2, 2, 2, 2, 2, 2, 2, 2, 2, 2, 2, 2, 2, 2, 2, 2, 2, 2, 2, 2, 2, 2, 2, 2, 2, 2, 2, 2, 2, 2, 2, 2, 2, 2, 2, 2, 2, 2, 2, 2, 2, 2, 2, 2, 2, 2, 2, 2, 2, 2, 2, 2, 2, 2, 2, 2, 2, 2, 2, 2, 2, 2, 2, 2, 2, 2, 2, 2, 2, 2, 2, 2, 2, 2, 2, 2, 2, 2, 2, 2, 2, 2, 2, 2, 2, 2, 2, 2, 2, 2, 2, 2, 2, 2, 2, 2, 2, 2, 2, 2, 2, 2, 3 ),
 ( 0.000000000000000000, 0.5000000000000000000, 1.000000000000000000 ),
 ( 0.000000000000000000, 0.004385964912280701511, 0.008771929824561403022, 0.01315789473684210453, 0.01754385964912280604, 0.02192982456140350755, 0.02631578947368420907, 0.03070175438596491058, 0.03508771929824561209, 0.03947368421052631360, 0.04385964912280701511, 0.04824561403508771662, 0.05263157894736841813, 0.05701754385964911964, 0.06140350877192982115, 0.06578947368421052266, 0.07017543859649122417, 0.07456140350877192569, 0.07894736842105262720, 0.08333333333333332871, 0.08771929824561403022, 0.09210526315789473173, 0.09649122807017543324, 0.1008771929824561348, 0.1052631578947368363, 0.1096491228070175378, 0.1140350877192982393, 0.1184210526315789408, 0.1228070175438596423, 0.1271929824561403577, 0.1315789473684210453, 0.1359649122807017607, 0.1403508771929824483, 0.1447368421052631637, 0.1491228070175438514, 0.1535087719298245668, 0.1578947368421052544, 0.1622807017543859698, 0.1666666666666666574, 0.1710526315789473728, 0.1754385964912280604, 0.1798245614035087758, 0.1842105263157894635, 0.1885964912280701788, 0.1929824561403508665, 0.1973684210526315819, 0.2017543859649122695, 0.2061403508771929849, 0.2105263157894736725, 0.2149122807017543879, 0.2192982456140350755, 0.2236842105263157909, 0.2280701754385964786, 0.2324561403508771940, 0.2368421052631578816, 0.2412280701754385970, 0.2456140350877192846, 0.2500000000000000000, 0.2543859649122807154, 0.2587719298245614308, 0.2631578947368420907, 0.2675438596491228060, 0.2719298245614035214, 0.2763157894736842368, 0.2807017543859648967, 0.2850877192982456121, 0.2894736842105263275, 0.2938596491228070429, 0.2982456140350877027, 0.3026315789473684181, 0.3070175438596491335, 0.3114035087719298489, 0.3157894736842105088, 0.3201754385964912242, 0.3245614035087719396, 0.3289473684210526550, 0.3333333333333333148, 0.3377192982456140302, 0.3421052631578947456, 0.3464912280701754610, 0.3508771929824561209, 0.3552631578947368363, 0.3596491228070175517, 0.3640350877192982670, 0.3684210526315789269, 0.3728070175438596423, 0.3771929824561403577, 0.3815789473684210731, 0.3859649122807017330, 0.3903508771929824483, 0.3947368421052631637, 0.3991228070175438791, 0.4035087719298245390, 0.4078947368421052544, 0.4122807017543859698, 0.4166666666666666852, 0.4210526315789473450, 0.4254385964912280604, 0.4298245614035087758, 0.4342105263157894912, 0.4385964912280701511, 0.4429824561403508665, 0.4473684210526315819, 0.4517543859649122973, 0.4561403508771929571, 0.4605263157894736725, 0.4649122807017543879, 0.4692982456140351033, 0.4736842105263157632, 0.4780701754385964786, 0.4824561403508771940, 0.4868421052631579093, 0.4912280701754385692, 0.4956140350877192846, 0.5000000000000000000, 0.5043859649122807154, 0.5087719298245614308, 0.5131578947368421462, 0.5175438596491228616, 0.5219298245614034659, 0.5263157894736841813, 0.5307017543859648967, 0.5350877192982456121, 0.5394736842105263275, 0.5438596491228070429, 0.5482456140350877583, 0.5526315789473684736, 0.5570175438596490780, 0.5614035087719297934, 0.5657894736842105088, 0.5701754385964912242, 0.5745614035087719396, 0.5789473684210526550, 0.5833333333333333703, 0.5877192982456140857, 0.5921052631578946901, 0.5964912280701754055, 0.6008771929824561209, 0.6052631578947368363, 0.6096491228070175517, 0.6140350877192982670, 0.6184210526315789824, 0.6228070175438596978, 0.6271929824561403022, 0.6315789473684210176, 0.6359649122807017330, 0.6403508771929824483, 0.6447368421052631637, 0.6491228070175438791, 0.6535087719298245945, 0.6578947368421053099, 0.6622807017543859143, 0.6666666666666666297, 0.6710526315789473450, 0.6754385964912280604, 0.6798245614035087758, 0.6842105263157894912, 0.6885964912280702066, 0.6929824561403509220, 0.6973684210526315264, 0.7017543859649122417, 0.7061403508771929571, 0.7105263157894736725, 0.7149122807017543879, 0.7192982456140351033, 0.7236842105263158187, 0.7280701754385965341, 0.7324561403508771384, 0.7368421052631578538, 0.7412280701754385692, 0.7456140350877192846, 0.7500000000000000000, 0.7543859649122807154, 0.7587719298245614308, 0.7631578947368421462, 0.7675438596491228616, 0.7719298245614034659, 0.7763157894736841813, 0.7807017543859648967, 0.7850877192982456121, 0.7894736842105263275, 0.7938596491228070429, 0.7982456140350877583, 0.8026315789473684736, 0.8070175438596490780, 0.8114035087719297934, 0.8157894736842105088, 0.8201754385964912242, 0.8245614035087719396, 0.8289473684210526550, 0.8333333333333333703, 0.8377192982456140857, 0.8421052631578946901, 0.8464912280701754055, 0.8508771929824561209, 0.8552631578947368363, 0.8596491228070175517, 0.8640350877192982670, 0.8684210526315789824, 0.8728070175438596978, 0.8771929824561403022, 0.8815789473684210176, 0.8859649122807017330, 0.8903508771929824483, 0.8947368421052631637, 0.8991228070175438791, 0.9035087719298245945, 0.9078947368421053099, 0.9122807017543859143, 0.9166666666666666297, 0.9210526315789473450, 0.9254385964912280604, 0.9298245614035087758, 0.9342105263157894912, 0.9385964912280702066, 0.9429824561403509220, 0.9473684210526315264, 0.9517543859649122417, 0.9561403508771929571, 0.9605263157894736725, 0.9649122807017543879, 0.9692982456140351033, 0.9736842105263158187, 0.9780701754385965341, 0.9824561403508771384, 0.9868421052631578538, 0.9912280701754385692, 0.9956140350877192846, 1.000000000000000000 ),
 .UNSPECIFIED. ) 
 GEOMETRIC_REPRESENTATION_ITEM ( )  RATIONAL_B_SPLINE_SURFACE ( (
 ( 1.000000000000000000, 0.9659258262890683122, 1.000000000000000000, 0.9659258262890683122, 1.000000000000000000, 0.9659258262890683122, 1.000000000000000000, 0.9659258262890683122, 1.000000000000000000, 0.9659258262890683122, 1.000000000000000000, 0.9659258262890683122, 1.000000000000000000, 0.9659258262890683122, 1.000000000000000000, 0.9659258262890683122, 1.000000000000000000, 0.9659258262890683122, 1.000000000000000000, 0.9659258262890683122, 1.000000000000000000, 0.9659258262890683122, 1.000000000000000000, 0.9659258262890683122, 1.000000000000000000, 0.9659258262890683122, 1.000000000000000000, 0.9659258262890683122, 1.000000000000000000, 0.9659258262890683122, 1.000000000000000000, 0.9659258262890683122, 1.000000000000000000, 0.9659258262890683122, 1.000000000000000000, 0.9659258262890683122, 1.000000000000000000, 0.9659258262890683122, 1.000000000000000000, 0.9659258262890683122, 1.000000000000000000, 0.9659258262890683122, 1.000000000000000000, 0.9659258262890683122, 1.000000000000000000, 0.9659258262890683122, 1.000000000000000000, 0.9659258262890683122, 1.000000000000000000, 0.9659258262890683122, 1.000000000000000000, 0.9659258262890683122, 1.000000000000000000, 0.9659258262890683122, 1.000000000000000000, 0.9659258262890683122, 1.000000000000000000, 0.9659258262890683122, 1.000000000000000000, 0.9659258262890683122, 1.000000000000000000, 0.9659258262890683122, 1.000000000000000000, 0.9659258262890683122, 1.000000000000000000, 0.9659258262890683122, 1.000000000000000000, 0.9659258262890683122, 1.000000000000000000, 0.9659258262890683122, 1.000000000000000000, 0.9659258262890683122, 1.000000000000000000, 0.9659258262890683122, 1.000000000000000000, 0.9659258262890683122, 1.000000000000000000, 0.9659258262890683122, 1.000000000000000000, 0.9659258262890683122, 1.000000000000000000, 0.9659258262890683122, 1.000000000000000000, 0.9659258262890683122, 1.000000000000000000, 0.9659258262890683122, 1.000000000000000000, 0.9659258262890683122, 1.000000000000000000, 0.9659258262890683122, 1.000000000000000000, 0.9659258262890683122, 1.000000000000000000, 0.9659258262890683122, 1.000000000000000000, 0.9659258262890683122, 1.000000000000000000, 0.9659258262890683122, 1.000000000000000000, 0.9659258262890683122, 1.000000000000000000, 0.9659258262890683122, 1.000000000000000000, 0.9659258262890683122, 1.000000000000000000, 0.9659258262890683122, 1.000000000000000000, 0.9659258262890683122, 1.000000000000000000, 0.9659258262890683122, 1.000000000000000000, 0.9659258262890683122, 1.000000000000000000, 0.9659258262890683122, 1.000000000000000000, 0.9659258262890683122, 1.000000000000000000, 0.9659258262890683122, 1.000000000000000000, 0.9659258262890683122, 1.000000000000000000, 0.9659258262890683122, 1.000000000000000000, 0.9659258262890683122, 1.000000000000000000, 0.9659258262890683122, 1.000000000000000000, 0.9659258262890683122, 1.000000000000000000, 0.9659258262890683122, 1.000000000000000000, 0.9659258262890683122, 1.000000000000000000, 0.9659258262890683122, 1.000000000000000000, 0.9659258262890683122, 1.000000000000000000, 0.9659258262890683122, 1.000000000000000000, 0.9659258262890683122, 1.000000000000000000, 0.9659258262890683122, 1.000000000000000000, 0.9659258262890683122, 1.000000000000000000, 0.9659258262890683122, 1.000000000000000000, 0.9659258262890683122, 1.000000000000000000, 0.9659258262890683122, 1.000000000000000000, 0.9659258262890683122, 1.000000000000000000, 0.9659258262890683122, 1.000000000000000000, 0.9659258262890683122, 1.000000000000000000, 0.9659258262890683122, 1.000000000000000000, 0.9659258262890683122, 1.000000000000000000, 0.9659258262890683122, 1.000000000000000000, 0.9659258262890683122, 1.000000000000000000, 0.9659258262890683122, 1.000000000000000000, 0.9659258262890683122, 1.000000000000000000, 0.9659258262890683122, 1.000000000000000000, 0.9659258262890683122, 1.000000000000000000, 0.9659258262890683122, 1.000000000000000000, 0.9659258262890683122, 1.000000000000000000, 0.9659258262890683122, 1.000000000000000000, 0.9659258262890683122, 1.000000000000000000, 0.9659258262890683122, 1.000000000000000000, 0.9659258262890683122, 1.000000000000000000, 0.9659258262890683122, 1.000000000000000000, 0.9659258262890683122, 1.000000000000000000, 0.9659258262890683122, 1.000000000000000000, 0.9659258262890683122, 1.000000000000000000, 0.9659258262890683122, 1.000000000000000000, 0.9659258262890683122, 1.000000000000000000, 0.9659258262890683122, 1.000000000000000000, 0.9659258262890683122, 1.000000000000000000, 0.9659258262890683122, 1.000000000000000000, 0.9659258262890683122, 1.000000000000000000, 0.9659258262890683122, 1.000000000000000000, 0.9659258262890683122, 1.000000000000000000, 0.9659258262890683122, 1.000000000000000000, 0.9659258262890683122, 1.000000000000000000, 0.9659258262890683122, 1.000000000000000000, 0.9659258262890683122, 1.000000000000000000, 0.9659258262890683122, 1.000000000000000000, 0.9659258262890683122, 1.000000000000000000, 0.9659258262890683122, 1.000000000000000000, 0.9659258262890683122, 1.000000000000000000, 0.9659258262890683122, 1.000000000000000000, 0.9659258262890683122, 1.000000000000000000, 0.9659258262890683122, 1.000000000000000000, 0.9659258262890683122, 1.000000000000000000, 0.9659258262890683122, 1.000000000000000000, 0.9659258262890683122, 1.000000000000000000, 0.9659258262890683122, 1.000000000000000000, 0.9659258262890683122, 1.000000000000000000, 0.9659258262890683122, 1.000000000000000000, 0.9659258262890683122, 1.000000000000000000, 0.9659258262890683122, 1.000000000000000000, 0.9659258262890683122, 1.000000000000000000, 0.9659258262890683122, 1.000000000000000000, 0.9659258262890683122, 1.000000000000000000, 0.9659258262890683122, 1.000000000000000000, 0.9659258262890683122, 1.000000000000000000, 0.9659258262890683122, 1.000000000000000000, 0.9659258262890683122, 1.000000000000000000, 0.9659258262890683122, 1.000000000000000000, 0.9659258262890683122, 1.000000000000000000, 0.9659258262890683122, 1.000000000000000000, 0.9659258262890683122, 1.000000000000000000, 0.9659258262890683122, 1.000000000000000000, 0.9659258262890683122, 1.000000000000000000, 0.9659258262890683122, 1.000000000000000000, 0.9659258262890683122, 1.000000000000000000, 0.9659258262890683122, 1.000000000000000000, 0.9659258262890683122, 1.000000000000000000, 0.9659258262890683122, 1.000000000000000000, 0.9659258262890683122, 1.000000000000000000, 0.9659258262890683122, 1.000000000000000000, 0.9659258262890683122, 1.000000000000000000, 0.9659258262890683122, 1.000000000000000000, 0.9659258262890683122, 1.000000000000000000, 0.9659258262890683122, 1.000000000000000000, 0.9659258262890683122, 1.000000000000000000, 0.9659258262890683122, 1.000000000000000000, 0.9659258262890683122, 1.000000000000000000, 0.9659258262890683122, 1.000000000000000000, 0.9659258262890683122, 1.000000000000000000, 0.9659258262890683122, 1.000000000000000000, 0.9659258262890683122, 1.000000000000000000, 0.9659258262890683122, 1.000000000000000000, 0.9659258262890683122, 1.000000000000000000, 0.9659258262890683122, 1.000000000000000000, 0.9659258262890683122, 1.000000000000000000, 0.9659258262890683122, 1.000000000000000000, 0.9659258262890683122, 1.000000000000000000, 0.9659258262890683122, 1.000000000000000000, 0.9659258262890683122, 1.000000000000000000, 0.9659258262890683122, 1.000000000000000000, 0.9659258262890683122, 1.000000000000000000, 0.9659258262890683122, 1.000000000000000000, 0.9659258262890683122, 1.000000000000000000, 0.9659258262890683122, 1.000000000000000000, 0.9659258262890683122, 1.000000000000000000, 0.9659258262890683122, 1.000000000000000000, 0.9659258262890683122, 1.000000000000000000, 0.9659258262890683122, 1.000000000000000000, 0.9659258262890683122, 1.000000000000000000, 0.9659258262890683122, 1.000000000000000000, 0.9659258262890683122, 1.000000000000000000, 0.9659258262890683122, 1.000000000000000000, 0.9659258262890683122, 1.000000000000000000, 0.9659258262890683122, 1.000000000000000000, 0.9659258262890683122, 1.000000000000000000, 0.9659258262890683122, 1.000000000000000000, 0.9659258262890683122, 1.000000000000000000, 0.9659258262890683122, 1.000000000000000000, 0.9659258262890683122, 1.000000000000000000, 0.9659258262890683122, 1.000000000000000000, 0.9659258262890683122, 1.000000000000000000, 0.9659258262890683122, 1.000000000000000000, 0.9659258262890683122, 1.000000000000000000, 0.9659258262890683122, 1.000000000000000000, 0.9659258262890683122, 1.000000000000000000, 0.9659258262890683122, 1.000000000000000000, 0.9659258262890683122, 1.000000000000000000, 0.9659258262890683122, 1.000000000000000000, 0.9659258262890683122, 1.000000000000000000, 0.9659258262890683122, 1.000000000000000000, 0.9659258262890683122, 1.000000000000000000, 0.9659258262890683122, 1.000000000000000000, 0.9659258262890683122, 1.000000000000000000, 0.9659258262890683122, 1.000000000000000000, 0.9659258262890683122, 1.000000000000000000, 0.9659258262890683122, 1.000000000000000000, 0.9659258262890683122, 1.000000000000000000, 0.9659258262890683122, 1.000000000000000000, 0.9659258262890683122, 1.000000000000000000, 0.9659258262890683122, 1.000000000000000000, 0.9659258262890683122, 1.000000000000000000, 0.9659258262890683122, 1.000000000000000000, 0.9659258262890683122, 1.000000000000000000, 0.9659258262890683122, 1.000000000000000000, 0.9659258262890683122, 1.000000000000000000, 0.9659258262890683122, 1.000000000000000000, 0.9659258262890683122, 1.000000000000000000, 0.9659258262890683122, 1.000000000000000000, 0.9659258262890683122, 1.000000000000000000, 0.9659258262890683122, 1.000000000000000000, 0.9659258262890683122, 1.000000000000000000, 0.9659258262890683122, 1.000000000000000000, 0.9659258262890683122, 1.000000000000000000, 0.9659258262890683122, 1.000000000000000000, 0.9659258262890683122, 1.000000000000000000, 0.9659258262890683122, 1.000000000000000000, 0.9659258262890683122, 1.000000000000000000, 0.9659258262890683122, 1.000000000000000000, 0.9659258262890683122, 1.000000000000000000, 0.9659258262890683122, 1.000000000000000000, 0.9659258262890683122, 1.000000000000000000, 0.9659258262890683122, 1.000000000000000000, 0.9659258262890683122, 1.000000000000000000, 0.9659258262890683122, 1.000000000000000000, 0.9659258262890683122, 1.000000000000000000),
 ( 0.3333333333333333703, 0.3219752754296894559, 0.3333333333333333703, 0.3219752754296894559, 0.3333333333333333703, 0.3219752754296894559, 0.3333333333333333703, 0.3219752754296894559, 0.3333333333333333703, 0.3219752754296894559, 0.3333333333333333703, 0.3219752754296894559, 0.3333333333333333703, 0.3219752754296894559, 0.3333333333333333703, 0.3219752754296894559, 0.3333333333333333703, 0.3219752754296894559, 0.3333333333333333703, 0.3219752754296894559, 0.3333333333333333703, 0.3219752754296894559, 0.3333333333333333703, 0.3219752754296894559, 0.3333333333333333703, 0.3219752754296894559, 0.3333333333333333703, 0.3219752754296894559, 0.3333333333333333703, 0.3219752754296894559, 0.3333333333333333703, 0.3219752754296894559, 0.3333333333333333703, 0.3219752754296894559, 0.3333333333333333703, 0.3219752754296894559, 0.3333333333333333703, 0.3219752754296894559, 0.3333333333333333703, 0.3219752754296894559, 0.3333333333333333703, 0.3219752754296894559, 0.3333333333333333703, 0.3219752754296894559, 0.3333333333333333703, 0.3219752754296894559, 0.3333333333333333703, 0.3219752754296894559, 0.3333333333333333703, 0.3219752754296894559, 0.3333333333333333703, 0.3219752754296894559, 0.3333333333333333703, 0.3219752754296894559, 0.3333333333333333703, 0.3219752754296894559, 0.3333333333333333703, 0.3219752754296894559, 0.3333333333333333703, 0.3219752754296894559, 0.3333333333333333703, 0.3219752754296894559, 0.3333333333333333703, 0.3219752754296894559, 0.3333333333333333703, 0.3219752754296894559, 0.3333333333333333703, 0.3219752754296894559, 0.3333333333333333703, 0.3219752754296894559, 0.3333333333333333703, 0.3219752754296894559, 0.3333333333333333703, 0.3219752754296894559, 0.3333333333333333703, 0.3219752754296894559, 0.3333333333333333703, 0.3219752754296894559, 0.3333333333333333703, 0.3219752754296894559, 0.3333333333333333703, 0.3219752754296894559, 0.3333333333333333703, 0.3219752754296894559, 0.3333333333333333703, 0.3219752754296894559, 0.3333333333333333703, 0.3219752754296894559, 0.3333333333333333703, 0.3219752754296894559, 0.3333333333333333703, 0.3219752754296894559, 0.3333333333333333703, 0.3219752754296894559, 0.3333333333333333703, 0.3219752754296894559, 0.3333333333333333703, 0.3219752754296894559, 0.3333333333333333703, 0.3219752754296894559, 0.3333333333333333703, 0.3219752754296894559, 0.3333333333333333703, 0.3219752754296894559, 0.3333333333333333703, 0.3219752754296894559, 0.3333333333333333703, 0.3219752754296894559, 0.3333333333333333703, 0.3219752754296894559, 0.3333333333333333703, 0.3219752754296894559, 0.3333333333333333703, 0.3219752754296894559, 0.3333333333333333703, 0.3219752754296894559, 0.3333333333333333703, 0.3219752754296894559, 0.3333333333333333703, 0.3219752754296894559, 0.3333333333333333703, 0.3219752754296894559, 0.3333333333333333703, 0.3219752754296894559, 0.3333333333333333703, 0.3219752754296894559, 0.3333333333333333703, 0.3219752754296894559, 0.3333333333333333703, 0.3219752754296894559, 0.3333333333333333703, 0.3219752754296894559, 0.3333333333333333703, 0.3219752754296894559, 0.3333333333333333703, 0.3219752754296894559, 0.3333333333333333703, 0.3219752754296894559, 0.3333333333333333703, 0.3219752754296894559, 0.3333333333333333703, 0.3219752754296894559, 0.3333333333333333703, 0.3219752754296894559, 0.3333333333333333703, 0.3219752754296894559, 0.3333333333333333703, 0.3219752754296894559, 0.3333333333333333703, 0.3219752754296894559, 0.3333333333333333703, 0.3219752754296894559, 0.3333333333333333703, 0.3219752754296894559, 0.3333333333333333703, 0.3219752754296894559, 0.3333333333333333703, 0.3219752754296894559, 0.3333333333333333703, 0.3219752754296894559, 0.3333333333333333703, 0.3219752754296894559, 0.3333333333333333703, 0.3219752754296894559, 0.3333333333333333703, 0.3219752754296894559, 0.3333333333333333703, 0.3219752754296894559, 0.3333333333333333703, 0.3219752754296894559, 0.3333333333333333703, 0.3219752754296894559, 0.3333333333333333703, 0.3219752754296894559, 0.3333333333333333703, 0.3219752754296894559, 0.3333333333333333703, 0.3219752754296894559, 0.3333333333333333703, 0.3219752754296894559, 0.3333333333333333703, 0.3219752754296894559, 0.3333333333333333703, 0.3219752754296894559, 0.3333333333333333703, 0.3219752754296894559, 0.3333333333333333703, 0.3219752754296894559, 0.3333333333333333703, 0.3219752754296894559, 0.3333333333333333703, 0.3219752754296894559, 0.3333333333333333703, 0.3219752754296894559, 0.3333333333333333703, 0.3219752754296894559, 0.3333333333333333703, 0.3219752754296894559, 0.3333333333333333703, 0.3219752754296894559, 0.3333333333333333703, 0.3219752754296894559, 0.3333333333333333703, 0.3219752754296894559, 0.3333333333333333703, 0.3219752754296894559, 0.3333333333333333703, 0.3219752754296894559, 0.3333333333333333703, 0.3219752754296894559, 0.3333333333333333703, 0.3219752754296894559, 0.3333333333333333703, 0.3219752754296894559, 0.3333333333333333703, 0.3219752754296894559, 0.3333333333333333703, 0.3219752754296894559, 0.3333333333333333703, 0.3219752754296894559, 0.3333333333333333703, 0.3219752754296894559, 0.3333333333333333703, 0.3219752754296894559, 0.3333333333333333703, 0.3219752754296894559, 0.3333333333333333703, 0.3219752754296894559, 0.3333333333333333703, 0.3219752754296894559, 0.3333333333333333703, 0.3219752754296894559, 0.3333333333333333703, 0.3219752754296894559, 0.3333333333333333703, 0.3219752754296894559, 0.3333333333333333703, 0.3219752754296894559, 0.3333333333333333703, 0.3219752754296894559, 0.3333333333333333703, 0.3219752754296894559, 0.3333333333333333703, 0.3219752754296894559, 0.3333333333333333703, 0.3219752754296894559, 0.3333333333333333703, 0.3219752754296894559, 0.3333333333333333703, 0.3219752754296894559, 0.3333333333333333703, 0.3219752754296894559, 0.3333333333333333703, 0.3219752754296894559, 0.3333333333333333703, 0.3219752754296894559, 0.3333333333333333703, 0.3219752754296894559, 0.3333333333333333703, 0.3219752754296894559, 0.3333333333333333703, 0.3219752754296894559, 0.3333333333333333703, 0.3219752754296894559, 0.3333333333333333703, 0.3219752754296894559, 0.3333333333333333703, 0.3219752754296894559, 0.3333333333333333703, 0.3219752754296894559, 0.3333333333333333703, 0.3219752754296894559, 0.3333333333333333703, 0.3219752754296894559, 0.3333333333333333703, 0.3219752754296894559, 0.3333333333333333703, 0.3219752754296894559, 0.3333333333333333703, 0.3219752754296894559, 0.3333333333333333703, 0.3219752754296894559, 0.3333333333333333703, 0.3219752754296894559, 0.3333333333333333703, 0.3219752754296894559, 0.3333333333333333703, 0.3219752754296894559, 0.3333333333333333703, 0.3219752754296894559, 0.3333333333333333703, 0.3219752754296894559, 0.3333333333333333703, 0.3219752754296894559, 0.3333333333333333703, 0.3219752754296894559, 0.3333333333333333703, 0.3219752754296894559, 0.3333333333333333703, 0.3219752754296894559, 0.3333333333333333703, 0.3219752754296894559, 0.3333333333333333703, 0.3219752754296894559, 0.3333333333333333703, 0.3219752754296894559, 0.3333333333333333703, 0.3219752754296894559, 0.3333333333333333703, 0.3219752754296894559, 0.3333333333333333703, 0.3219752754296894559, 0.3333333333333333703, 0.3219752754296894559, 0.3333333333333333703, 0.3219752754296894559, 0.3333333333333333703, 0.3219752754296894559, 0.3333333333333333703, 0.3219752754296894559, 0.3333333333333333703, 0.3219752754296894559, 0.3333333333333333703, 0.3219752754296894559, 0.3333333333333333703, 0.3219752754296894559, 0.3333333333333333703, 0.3219752754296894559, 0.3333333333333333703, 0.3219752754296894559, 0.3333333333333333703, 0.3219752754296894559, 0.3333333333333333703, 0.3219752754296894559, 0.3333333333333333703, 0.3219752754296894559, 0.3333333333333333703, 0.3219752754296894559, 0.3333333333333333703, 0.3219752754296894559, 0.3333333333333333703, 0.3219752754296894559, 0.3333333333333333703, 0.3219752754296894559, 0.3333333333333333703, 0.3219752754296894559, 0.3333333333333333703, 0.3219752754296894559, 0.3333333333333333703, 0.3219752754296894559, 0.3333333333333333703, 0.3219752754296894559, 0.3333333333333333703, 0.3219752754296894559, 0.3333333333333333703, 0.3219752754296894559, 0.3333333333333333703, 0.3219752754296894559, 0.3333333333333333703, 0.3219752754296894559, 0.3333333333333333703, 0.3219752754296894559, 0.3333333333333333703, 0.3219752754296894559, 0.3333333333333333703, 0.3219752754296894559, 0.3333333333333333703, 0.3219752754296894559, 0.3333333333333333703, 0.3219752754296894559, 0.3333333333333333703, 0.3219752754296894559, 0.3333333333333333703, 0.3219752754296894559, 0.3333333333333333703, 0.3219752754296894559, 0.3333333333333333703, 0.3219752754296894559, 0.3333333333333333703, 0.3219752754296894559, 0.3333333333333333703, 0.3219752754296894559, 0.3333333333333333703, 0.3219752754296894559, 0.3333333333333333703, 0.3219752754296894559, 0.3333333333333333703, 0.3219752754296894559, 0.3333333333333333703, 0.3219752754296894559, 0.3333333333333333703, 0.3219752754296894559, 0.3333333333333333703, 0.3219752754296894559, 0.3333333333333333703, 0.3219752754296894559, 0.3333333333333333703, 0.3219752754296894559, 0.3333333333333333703, 0.3219752754296894559, 0.3333333333333333703, 0.3219752754296894559, 0.3333333333333333703, 0.3219752754296894559, 0.3333333333333333703, 0.3219752754296894559, 0.3333333333333333703, 0.3219752754296894559, 0.3333333333333333703, 0.3219752754296894559, 0.3333333333333333703, 0.3219752754296894559, 0.3333333333333333703, 0.3219752754296894559, 0.3333333333333333703, 0.3219752754296894559, 0.3333333333333333703, 0.3219752754296894559, 0.3333333333333333703, 0.3219752754296894559, 0.3333333333333333703, 0.3219752754296894559, 0.3333333333333333703, 0.3219752754296894559, 0.3333333333333333703, 0.3219752754296894559, 0.3333333333333333703, 0.3219752754296894559, 0.3333333333333333703, 0.3219752754296894559, 0.3333333333333333703, 0.3219752754296894559, 0.3333333333333333703, 0.3219752754296894559, 0.3333333333333333703, 0.3219752754296894559, 0.3333333333333333703, 0.3219752754296894559, 0.3333333333333333703, 0.3219752754296894559, 0.3333333333333333703, 0.3219752754296894559, 0.3333333333333333703, 0.3219752754296894559, 0.3333333333333333703, 0.3219752754296894559, 0.3333333333333333703, 0.3219752754296894559, 0.3333333333333333703, 0.3219752754296894559, 0.3333333333333333703, 0.3219752754296894559, 0.3333333333333333703, 0.3219752754296894559, 0.3333333333333333703, 0.3219752754296894559, 0.3333333333333333703),
 ( 0.3333333333333333703, 0.3219752754296894559, 0.3333333333333333703, 0.3219752754296894559, 0.3333333333333333703, 0.3219752754296894559, 0.3333333333333333703, 0.3219752754296894559, 0.3333333333333333703, 0.3219752754296894559, 0.3333333333333333703, 0.3219752754296894559, 0.3333333333333333703, 0.3219752754296894559, 0.3333333333333333703, 0.3219752754296894559, 0.3333333333333333703, 0.3219752754296894559, 0.3333333333333333703, 0.3219752754296894559, 0.3333333333333333703, 0.3219752754296894559, 0.3333333333333333703, 0.3219752754296894559, 0.3333333333333333703, 0.3219752754296894559, 0.3333333333333333703, 0.3219752754296894559, 0.3333333333333333703, 0.3219752754296894559, 0.3333333333333333703, 0.3219752754296894559, 0.3333333333333333703, 0.3219752754296894559, 0.3333333333333333703, 0.3219752754296894559, 0.3333333333333333703, 0.3219752754296894559, 0.3333333333333333703, 0.3219752754296894559, 0.3333333333333333703, 0.3219752754296894559, 0.3333333333333333703, 0.3219752754296894559, 0.3333333333333333703, 0.3219752754296894559, 0.3333333333333333703, 0.3219752754296894559, 0.3333333333333333703, 0.3219752754296894559, 0.3333333333333333703, 0.3219752754296894559, 0.3333333333333333703, 0.3219752754296894559, 0.3333333333333333703, 0.3219752754296894559, 0.3333333333333333703, 0.3219752754296894559, 0.3333333333333333703, 0.3219752754296894559, 0.3333333333333333703, 0.3219752754296894559, 0.3333333333333333703, 0.3219752754296894559, 0.3333333333333333703, 0.3219752754296894559, 0.3333333333333333703, 0.3219752754296894559, 0.3333333333333333703, 0.3219752754296894559, 0.3333333333333333703, 0.3219752754296894559, 0.3333333333333333703, 0.3219752754296894559, 0.3333333333333333703, 0.3219752754296894559, 0.3333333333333333703, 0.3219752754296894559, 0.3333333333333333703, 0.3219752754296894559, 0.3333333333333333703, 0.3219752754296894559, 0.3333333333333333703, 0.3219752754296894559, 0.3333333333333333703, 0.3219752754296894559, 0.3333333333333333703, 0.3219752754296894559, 0.3333333333333333703, 0.3219752754296894559, 0.3333333333333333703, 0.3219752754296894559, 0.3333333333333333703, 0.3219752754296894559, 0.3333333333333333703, 0.3219752754296894559, 0.3333333333333333703, 0.3219752754296894559, 0.3333333333333333703, 0.3219752754296894559, 0.3333333333333333703, 0.3219752754296894559, 0.3333333333333333703, 0.3219752754296894559, 0.3333333333333333703, 0.3219752754296894559, 0.3333333333333333703, 0.3219752754296894559, 0.3333333333333333703, 0.3219752754296894559, 0.3333333333333333703, 0.3219752754296894559, 0.3333333333333333703, 0.3219752754296894559, 0.3333333333333333703, 0.3219752754296894559, 0.3333333333333333703, 0.3219752754296894559, 0.3333333333333333703, 0.3219752754296894559, 0.3333333333333333703, 0.3219752754296894559, 0.3333333333333333703, 0.3219752754296894559, 0.3333333333333333703, 0.3219752754296894559, 0.3333333333333333703, 0.3219752754296894559, 0.3333333333333333703, 0.3219752754296894559, 0.3333333333333333703, 0.3219752754296894559, 0.3333333333333333703, 0.3219752754296894559, 0.3333333333333333703, 0.3219752754296894559, 0.3333333333333333703, 0.3219752754296894559, 0.3333333333333333703, 0.3219752754296894559, 0.3333333333333333703, 0.3219752754296894559, 0.3333333333333333703, 0.3219752754296894559, 0.3333333333333333703, 0.3219752754296894559, 0.3333333333333333703, 0.3219752754296894559, 0.3333333333333333703, 0.3219752754296894559, 0.3333333333333333703, 0.3219752754296894559, 0.3333333333333333703, 0.3219752754296894559, 0.3333333333333333703, 0.3219752754296894559, 0.3333333333333333703, 0.3219752754296894559, 0.3333333333333333703, 0.3219752754296894559, 0.3333333333333333703, 0.3219752754296894559, 0.3333333333333333703, 0.3219752754296894559, 0.3333333333333333703, 0.3219752754296894559, 0.3333333333333333703, 0.3219752754296894559, 0.3333333333333333703, 0.3219752754296894559, 0.3333333333333333703, 0.3219752754296894559, 0.3333333333333333703, 0.3219752754296894559, 0.3333333333333333703, 0.3219752754296894559, 0.3333333333333333703, 0.3219752754296894559, 0.3333333333333333703, 0.3219752754296894559, 0.3333333333333333703, 0.3219752754296894559, 0.3333333333333333703, 0.3219752754296894559, 0.3333333333333333703, 0.3219752754296894559, 0.3333333333333333703, 0.3219752754296894559, 0.3333333333333333703, 0.3219752754296894559, 0.3333333333333333703, 0.3219752754296894559, 0.3333333333333333703, 0.3219752754296894559, 0.3333333333333333703, 0.3219752754296894559, 0.3333333333333333703, 0.3219752754296894559, 0.3333333333333333703, 0.3219752754296894559, 0.3333333333333333703, 0.3219752754296894559, 0.3333333333333333703, 0.3219752754296894559, 0.3333333333333333703, 0.3219752754296894559, 0.3333333333333333703, 0.3219752754296894559, 0.3333333333333333703, 0.3219752754296894559, 0.3333333333333333703, 0.3219752754296894559, 0.3333333333333333703, 0.3219752754296894559, 0.3333333333333333703, 0.3219752754296894559, 0.3333333333333333703, 0.3219752754296894559, 0.3333333333333333703, 0.3219752754296894559, 0.3333333333333333703, 0.3219752754296894559, 0.3333333333333333703, 0.3219752754296894559, 0.3333333333333333703, 0.3219752754296894559, 0.3333333333333333703, 0.3219752754296894559, 0.3333333333333333703, 0.3219752754296894559, 0.3333333333333333703, 0.3219752754296894559, 0.3333333333333333703, 0.3219752754296894559, 0.3333333333333333703, 0.3219752754296894559, 0.3333333333333333703, 0.3219752754296894559, 0.3333333333333333703, 0.3219752754296894559, 0.3333333333333333703, 0.3219752754296894559, 0.3333333333333333703, 0.3219752754296894559, 0.3333333333333333703, 0.3219752754296894559, 0.3333333333333333703, 0.3219752754296894559, 0.3333333333333333703, 0.3219752754296894559, 0.3333333333333333703, 0.3219752754296894559, 0.3333333333333333703, 0.3219752754296894559, 0.3333333333333333703, 0.3219752754296894559, 0.3333333333333333703, 0.3219752754296894559, 0.3333333333333333703, 0.3219752754296894559, 0.3333333333333333703, 0.3219752754296894559, 0.3333333333333333703, 0.3219752754296894559, 0.3333333333333333703, 0.3219752754296894559, 0.3333333333333333703, 0.3219752754296894559, 0.3333333333333333703, 0.3219752754296894559, 0.3333333333333333703, 0.3219752754296894559, 0.3333333333333333703, 0.3219752754296894559, 0.3333333333333333703, 0.3219752754296894559, 0.3333333333333333703, 0.3219752754296894559, 0.3333333333333333703, 0.3219752754296894559, 0.3333333333333333703, 0.3219752754296894559, 0.3333333333333333703, 0.3219752754296894559, 0.3333333333333333703, 0.3219752754296894559, 0.3333333333333333703, 0.3219752754296894559, 0.3333333333333333703, 0.3219752754296894559, 0.3333333333333333703, 0.3219752754296894559, 0.3333333333333333703, 0.3219752754296894559, 0.3333333333333333703, 0.3219752754296894559, 0.3333333333333333703, 0.3219752754296894559, 0.3333333333333333703, 0.3219752754296894559, 0.3333333333333333703, 0.3219752754296894559, 0.3333333333333333703, 0.3219752754296894559, 0.3333333333333333703, 0.3219752754296894559, 0.3333333333333333703, 0.3219752754296894559, 0.3333333333333333703, 0.3219752754296894559, 0.3333333333333333703, 0.3219752754296894559, 0.3333333333333333703, 0.3219752754296894559, 0.3333333333333333703, 0.3219752754296894559, 0.3333333333333333703, 0.3219752754296894559, 0.3333333333333333703, 0.3219752754296894559, 0.3333333333333333703, 0.3219752754296894559, 0.3333333333333333703, 0.3219752754296894559, 0.3333333333333333703, 0.3219752754296894559, 0.3333333333333333703, 0.3219752754296894559, 0.3333333333333333703, 0.3219752754296894559, 0.3333333333333333703, 0.3219752754296894559, 0.3333333333333333703, 0.3219752754296894559, 0.3333333333333333703, 0.3219752754296894559, 0.3333333333333333703, 0.3219752754296894559, 0.3333333333333333703, 0.3219752754296894559, 0.3333333333333333703, 0.3219752754296894559, 0.3333333333333333703, 0.3219752754296894559, 0.3333333333333333703, 0.3219752754296894559, 0.3333333333333333703, 0.3219752754296894559, 0.3333333333333333703, 0.3219752754296894559, 0.3333333333333333703, 0.3219752754296894559, 0.3333333333333333703, 0.3219752754296894559, 0.3333333333333333703, 0.3219752754296894559, 0.3333333333333333703, 0.3219752754296894559, 0.3333333333333333703, 0.3219752754296894559, 0.3333333333333333703, 0.3219752754296894559, 0.3333333333333333703, 0.3219752754296894559, 0.3333333333333333703, 0.3219752754296894559, 0.3333333333333333703, 0.3219752754296894559, 0.3333333333333333703, 0.3219752754296894559, 0.3333333333333333703, 0.3219752754296894559, 0.3333333333333333703, 0.3219752754296894559, 0.3333333333333333703, 0.3219752754296894559, 0.3333333333333333703, 0.3219752754296894559, 0.3333333333333333703, 0.3219752754296894559, 0.3333333333333333703, 0.3219752754296894559, 0.3333333333333333703, 0.3219752754296894559, 0.3333333333333333703, 0.3219752754296894559, 0.3333333333333333703, 0.3219752754296894559, 0.3333333333333333703, 0.3219752754296894559, 0.3333333333333333703, 0.3219752754296894559, 0.3333333333333333703, 0.3219752754296894559, 0.3333333333333333703, 0.3219752754296894559, 0.3333333333333333703, 0.3219752754296894559, 0.3333333333333333703, 0.3219752754296894559, 0.3333333333333333703, 0.3219752754296894559, 0.3333333333333333703, 0.3219752754296894559, 0.3333333333333333703, 0.3219752754296894559, 0.3333333333333333703, 0.3219752754296894559, 0.3333333333333333703, 0.3219752754296894559, 0.3333333333333333703, 0.3219752754296894559, 0.3333333333333333703, 0.3219752754296894559, 0.3333333333333333703, 0.3219752754296894559, 0.3333333333333333703, 0.3219752754296894559, 0.3333333333333333703, 0.3219752754296894559, 0.3333333333333333703, 0.3219752754296894559, 0.3333333333333333703, 0.3219752754296894559, 0.3333333333333333703, 0.3219752754296894559, 0.3333333333333333703, 0.3219752754296894559, 0.3333333333333333703, 0.3219752754296894559, 0.3333333333333333703, 0.3219752754296894559, 0.3333333333333333703, 0.3219752754296894559, 0.3333333333333333703, 0.3219752754296894559, 0.3333333333333333703, 0.3219752754296894559, 0.3333333333333333703, 0.3219752754296894559, 0.3333333333333333703, 0.3219752754296894559, 0.3333333333333333703, 0.3219752754296894559, 0.3333333333333333703, 0.3219752754296894559, 0.3333333333333333703, 0.3219752754296894559, 0.3333333333333333703, 0.3219752754296894559, 0.3333333333333333703, 0.3219752754296894559, 0.3333333333333333703, 0.3219752754296894559, 0.3333333333333333703, 0.3219752754296894559, 0.3333333333333333703),
 ( 1.000000000000000000, 0.9659258262890683122, 1.000000000000000000, 0.9659258262890683122, 1.000000000000000000, 0.9659258262890683122, 1.000000000000000000, 0.9659258262890683122, 1.000000000000000000, 0.9659258262890683122, 1.000000000000000000, 0.9659258262890683122, 1.000000000000000000, 0.9659258262890683122, 1.000000000000000000, 0.9659258262890683122, 1.000000000000000000, 0.9659258262890683122, 1.000000000000000000, 0.9659258262890683122, 1.000000000000000000, 0.9659258262890683122, 1.000000000000000000, 0.9659258262890683122, 1.000000000000000000, 0.9659258262890683122, 1.000000000000000000, 0.9659258262890683122, 1.000000000000000000, 0.9659258262890683122, 1.000000000000000000, 0.9659258262890683122, 1.000000000000000000, 0.9659258262890683122, 1.000000000000000000, 0.9659258262890683122, 1.000000000000000000, 0.9659258262890683122, 1.000000000000000000, 0.9659258262890683122, 1.000000000000000000, 0.9659258262890683122, 1.000000000000000000, 0.9659258262890683122, 1.000000000000000000, 0.9659258262890683122, 1.000000000000000000, 0.9659258262890683122, 1.000000000000000000, 0.9659258262890683122, 1.000000000000000000, 0.9659258262890683122, 1.000000000000000000, 0.9659258262890683122, 1.000000000000000000, 0.9659258262890683122, 1.000000000000000000, 0.9659258262890683122, 1.000000000000000000, 0.9659258262890683122, 1.000000000000000000, 0.9659258262890683122, 1.000000000000000000, 0.9659258262890683122, 1.000000000000000000, 0.9659258262890683122, 1.000000000000000000, 0.9659258262890683122, 1.000000000000000000, 0.9659258262890683122, 1.000000000000000000, 0.9659258262890683122, 1.000000000000000000, 0.9659258262890683122, 1.000000000000000000, 0.9659258262890683122, 1.000000000000000000, 0.9659258262890683122, 1.000000000000000000, 0.9659258262890683122, 1.000000000000000000, 0.9659258262890683122, 1.000000000000000000, 0.9659258262890683122, 1.000000000000000000, 0.9659258262890683122, 1.000000000000000000, 0.9659258262890683122, 1.000000000000000000, 0.9659258262890683122, 1.000000000000000000, 0.9659258262890683122, 1.000000000000000000, 0.9659258262890683122, 1.000000000000000000, 0.9659258262890683122, 1.000000000000000000, 0.9659258262890683122, 1.000000000000000000, 0.9659258262890683122, 1.000000000000000000, 0.9659258262890683122, 1.000000000000000000, 0.9659258262890683122, 1.000000000000000000, 0.9659258262890683122, 1.000000000000000000, 0.9659258262890683122, 1.000000000000000000, 0.9659258262890683122, 1.000000000000000000, 0.9659258262890683122, 1.000000000000000000, 0.9659258262890683122, 1.000000000000000000, 0.9659258262890683122, 1.000000000000000000, 0.9659258262890683122, 1.000000000000000000, 0.9659258262890683122, 1.000000000000000000, 0.9659258262890683122, 1.000000000000000000, 0.9659258262890683122, 1.000000000000000000, 0.9659258262890683122, 1.000000000000000000, 0.9659258262890683122, 1.000000000000000000, 0.9659258262890683122, 1.000000000000000000, 0.9659258262890683122, 1.000000000000000000, 0.9659258262890683122, 1.000000000000000000, 0.9659258262890683122, 1.000000000000000000, 0.9659258262890683122, 1.000000000000000000, 0.9659258262890683122, 1.000000000000000000, 0.9659258262890683122, 1.000000000000000000, 0.9659258262890683122, 1.000000000000000000, 0.9659258262890683122, 1.000000000000000000, 0.9659258262890683122, 1.000000000000000000, 0.9659258262890683122, 1.000000000000000000, 0.9659258262890683122, 1.000000000000000000, 0.9659258262890683122, 1.000000000000000000, 0.9659258262890683122, 1.000000000000000000, 0.9659258262890683122, 1.000000000000000000, 0.9659258262890683122, 1.000000000000000000, 0.9659258262890683122, 1.000000000000000000, 0.9659258262890683122, 1.000000000000000000, 0.9659258262890683122, 1.000000000000000000, 0.9659258262890683122, 1.000000000000000000, 0.9659258262890683122, 1.000000000000000000, 0.9659258262890683122, 1.000000000000000000, 0.9659258262890683122, 1.000000000000000000, 0.9659258262890683122, 1.000000000000000000, 0.9659258262890683122, 1.000000000000000000, 0.9659258262890683122, 1.000000000000000000, 0.9659258262890683122, 1.000000000000000000, 0.9659258262890683122, 1.000000000000000000, 0.9659258262890683122, 1.000000000000000000, 0.9659258262890683122, 1.000000000000000000, 0.9659258262890683122, 1.000000000000000000, 0.9659258262890683122, 1.000000000000000000, 0.9659258262890683122, 1.000000000000000000, 0.9659258262890683122, 1.000000000000000000, 0.9659258262890683122, 1.000000000000000000, 0.9659258262890683122, 1.000000000000000000, 0.9659258262890683122, 1.000000000000000000, 0.9659258262890683122, 1.000000000000000000, 0.9659258262890683122, 1.000000000000000000, 0.9659258262890683122, 1.000000000000000000, 0.9659258262890683122, 1.000000000000000000, 0.9659258262890683122, 1.000000000000000000, 0.9659258262890683122, 1.000000000000000000, 0.9659258262890683122, 1.000000000000000000, 0.9659258262890683122, 1.000000000000000000, 0.9659258262890683122, 1.000000000000000000, 0.9659258262890683122, 1.000000000000000000, 0.9659258262890683122, 1.000000000000000000, 0.9659258262890683122, 1.000000000000000000, 0.9659258262890683122, 1.000000000000000000, 0.9659258262890683122, 1.000000000000000000, 0.9659258262890683122, 1.000000000000000000, 0.9659258262890683122, 1.000000000000000000, 0.9659258262890683122, 1.000000000000000000, 0.9659258262890683122, 1.000000000000000000, 0.9659258262890683122, 1.000000000000000000, 0.9659258262890683122, 1.000000000000000000, 0.9659258262890683122, 1.000000000000000000, 0.9659258262890683122, 1.000000000000000000, 0.9659258262890683122, 1.000000000000000000, 0.9659258262890683122, 1.000000000000000000, 0.9659258262890683122, 1.000000000000000000, 0.9659258262890683122, 1.000000000000000000, 0.9659258262890683122, 1.000000000000000000, 0.9659258262890683122, 1.000000000000000000, 0.9659258262890683122, 1.000000000000000000, 0.9659258262890683122, 1.000000000000000000, 0.9659258262890683122, 1.000000000000000000, 0.9659258262890683122, 1.000000000000000000, 0.9659258262890683122, 1.000000000000000000, 0.9659258262890683122, 1.000000000000000000, 0.9659258262890683122, 1.000000000000000000, 0.9659258262890683122, 1.000000000000000000, 0.9659258262890683122, 1.000000000000000000, 0.9659258262890683122, 1.000000000000000000, 0.9659258262890683122, 1.000000000000000000, 0.9659258262890683122, 1.000000000000000000, 0.9659258262890683122, 1.000000000000000000, 0.9659258262890683122, 1.000000000000000000, 0.9659258262890683122, 1.000000000000000000, 0.9659258262890683122, 1.000000000000000000, 0.9659258262890683122, 1.000000000000000000, 0.9659258262890683122, 1.000000000000000000, 0.9659258262890683122, 1.000000000000000000, 0.9659258262890683122, 1.000000000000000000, 0.9659258262890683122, 1.000000000000000000, 0.9659258262890683122, 1.000000000000000000, 0.9659258262890683122, 1.000000000000000000, 0.9659258262890683122, 1.000000000000000000, 0.9659258262890683122, 1.000000000000000000, 0.9659258262890683122, 1.000000000000000000, 0.9659258262890683122, 1.000000000000000000, 0.9659258262890683122, 1.000000000000000000, 0.9659258262890683122, 1.000000000000000000, 0.9659258262890683122, 1.000000000000000000, 0.9659258262890683122, 1.000000000000000000, 0.9659258262890683122, 1.000000000000000000, 0.9659258262890683122, 1.000000000000000000, 0.9659258262890683122, 1.000000000000000000, 0.9659258262890683122, 1.000000000000000000, 0.9659258262890683122, 1.000000000000000000, 0.9659258262890683122, 1.000000000000000000, 0.9659258262890683122, 1.000000000000000000, 0.9659258262890683122, 1.000000000000000000, 0.9659258262890683122, 1.000000000000000000, 0.9659258262890683122, 1.000000000000000000, 0.9659258262890683122, 1.000000000000000000, 0.9659258262890683122, 1.000000000000000000, 0.9659258262890683122, 1.000000000000000000, 0.9659258262890683122, 1.000000000000000000, 0.9659258262890683122, 1.000000000000000000, 0.9659258262890683122, 1.000000000000000000, 0.9659258262890683122, 1.000000000000000000, 0.9659258262890683122, 1.000000000000000000, 0.9659258262890683122, 1.000000000000000000, 0.9659258262890683122, 1.000000000000000000, 0.9659258262890683122, 1.000000000000000000, 0.9659258262890683122, 1.000000000000000000, 0.9659258262890683122, 1.000000000000000000, 0.9659258262890683122, 1.000000000000000000, 0.9659258262890683122, 1.000000000000000000, 0.9659258262890683122, 1.000000000000000000, 0.9659258262890683122, 1.000000000000000000, 0.9659258262890683122, 1.000000000000000000, 0.9659258262890683122, 1.000000000000000000, 0.9659258262890683122, 1.000000000000000000, 0.9659258262890683122, 1.000000000000000000, 0.9659258262890683122, 1.000000000000000000, 0.9659258262890683122, 1.000000000000000000, 0.9659258262890683122, 1.000000000000000000, 0.9659258262890683122, 1.000000000000000000, 0.9659258262890683122, 1.000000000000000000, 0.9659258262890683122, 1.000000000000000000, 0.9659258262890683122, 1.000000000000000000, 0.9659258262890683122, 1.000000000000000000, 0.9659258262890683122, 1.000000000000000000, 0.9659258262890683122, 1.000000000000000000, 0.9659258262890683122, 1.000000000000000000, 0.9659258262890683122, 1.000000000000000000, 0.9659258262890683122, 1.000000000000000000, 0.9659258262890683122, 1.000000000000000000, 0.9659258262890683122, 1.000000000000000000, 0.9659258262890683122, 1.000000000000000000, 0.9659258262890683122, 1.000000000000000000, 0.9659258262890683122, 1.000000000000000000, 0.9659258262890683122, 1.000000000000000000, 0.9659258262890683122, 1.000000000000000000, 0.9659258262890683122, 1.000000000000000000, 0.9659258262890683122, 1.000000000000000000, 0.9659258262890683122, 1.000000000000000000, 0.9659258262890683122, 1.000000000000000000, 0.9659258262890683122, 1.000000000000000000, 0.9659258262890683122, 1.000000000000000000, 0.9659258262890683122, 1.000000000000000000, 0.9659258262890683122, 1.000000000000000000, 0.9659258262890683122, 1.000000000000000000, 0.9659258262890683122, 1.000000000000000000, 0.9659258262890683122, 1.000000000000000000, 0.9659258262890683122, 1.000000000000000000, 0.9659258262890683122, 1.000000000000000000, 0.9659258262890683122, 1.000000000000000000, 0.9659258262890683122, 1.000000000000000000, 0.9659258262890683122, 1.000000000000000000, 0.9659258262890683122, 1.000000000000000000),
 ( 0.3333333333333333703, 0.3219752754296894559, 0.3333333333333333703, 0.3219752754296894559, 0.3333333333333333703, 0.3219752754296894559, 0.3333333333333333703, 0.3219752754296894559, 0.3333333333333333703, 0.3219752754296894559, 0.3333333333333333703, 0.3219752754296894559, 0.3333333333333333703, 0.3219752754296894559, 0.3333333333333333703, 0.3219752754296894559, 0.3333333333333333703, 0.3219752754296894559, 0.3333333333333333703, 0.3219752754296894559, 0.3333333333333333703, 0.3219752754296894559, 0.3333333333333333703, 0.3219752754296894559, 0.3333333333333333703, 0.3219752754296894559, 0.3333333333333333703, 0.3219752754296894559, 0.3333333333333333703, 0.3219752754296894559, 0.3333333333333333703, 0.3219752754296894559, 0.3333333333333333703, 0.3219752754296894559, 0.3333333333333333703, 0.3219752754296894559, 0.3333333333333333703, 0.3219752754296894559, 0.3333333333333333703, 0.3219752754296894559, 0.3333333333333333703, 0.3219752754296894559, 0.3333333333333333703, 0.3219752754296894559, 0.3333333333333333703, 0.3219752754296894559, 0.3333333333333333703, 0.3219752754296894559, 0.3333333333333333703, 0.3219752754296894559, 0.3333333333333333703, 0.3219752754296894559, 0.3333333333333333703, 0.3219752754296894559, 0.3333333333333333703, 0.3219752754296894559, 0.3333333333333333703, 0.3219752754296894559, 0.3333333333333333703, 0.3219752754296894559, 0.3333333333333333703, 0.3219752754296894559, 0.3333333333333333703, 0.3219752754296894559, 0.3333333333333333703, 0.3219752754296894559, 0.3333333333333333703, 0.3219752754296894559, 0.3333333333333333703, 0.3219752754296894559, 0.3333333333333333703, 0.3219752754296894559, 0.3333333333333333703, 0.3219752754296894559, 0.3333333333333333703, 0.3219752754296894559, 0.3333333333333333703, 0.3219752754296894559, 0.3333333333333333703, 0.3219752754296894559, 0.3333333333333333703, 0.3219752754296894559, 0.3333333333333333703, 0.3219752754296894559, 0.3333333333333333703, 0.3219752754296894559, 0.3333333333333333703, 0.3219752754296894559, 0.3333333333333333703, 0.3219752754296894559, 0.3333333333333333703, 0.3219752754296894559, 0.3333333333333333703, 0.3219752754296894559, 0.3333333333333333703, 0.3219752754296894559, 0.3333333333333333703, 0.3219752754296894559, 0.3333333333333333703, 0.3219752754296894559, 0.3333333333333333703, 0.3219752754296894559, 0.3333333333333333703, 0.3219752754296894559, 0.3333333333333333703, 0.3219752754296894559, 0.3333333333333333703, 0.3219752754296894559, 0.3333333333333333703, 0.3219752754296894559, 0.3333333333333333703, 0.3219752754296894559, 0.3333333333333333703, 0.3219752754296894559, 0.3333333333333333703, 0.3219752754296894559, 0.3333333333333333703, 0.3219752754296894559, 0.3333333333333333703, 0.3219752754296894559, 0.3333333333333333703, 0.3219752754296894559, 0.3333333333333333703, 0.3219752754296894559, 0.3333333333333333703, 0.3219752754296894559, 0.3333333333333333703, 0.3219752754296894559, 0.3333333333333333703, 0.3219752754296894559, 0.3333333333333333703, 0.3219752754296894559, 0.3333333333333333703, 0.3219752754296894559, 0.3333333333333333703, 0.3219752754296894559, 0.3333333333333333703, 0.3219752754296894559, 0.3333333333333333703, 0.3219752754296894559, 0.3333333333333333703, 0.3219752754296894559, 0.3333333333333333703, 0.3219752754296894559, 0.3333333333333333703, 0.3219752754296894559, 0.3333333333333333703, 0.3219752754296894559, 0.3333333333333333703, 0.3219752754296894559, 0.3333333333333333703, 0.3219752754296894559, 0.3333333333333333703, 0.3219752754296894559, 0.3333333333333333703, 0.3219752754296894559, 0.3333333333333333703, 0.3219752754296894559, 0.3333333333333333703, 0.3219752754296894559, 0.3333333333333333703, 0.3219752754296894559, 0.3333333333333333703, 0.3219752754296894559, 0.3333333333333333703, 0.3219752754296894559, 0.3333333333333333703, 0.3219752754296894559, 0.3333333333333333703, 0.3219752754296894559, 0.3333333333333333703, 0.3219752754296894559, 0.3333333333333333703, 0.3219752754296894559, 0.3333333333333333703, 0.3219752754296894559, 0.3333333333333333703, 0.3219752754296894559, 0.3333333333333333703, 0.3219752754296894559, 0.3333333333333333703, 0.3219752754296894559, 0.3333333333333333703, 0.3219752754296894559, 0.3333333333333333703, 0.3219752754296894559, 0.3333333333333333703, 0.3219752754296894559, 0.3333333333333333703, 0.3219752754296894559, 0.3333333333333333703, 0.3219752754296894559, 0.3333333333333333703, 0.3219752754296894559, 0.3333333333333333703, 0.3219752754296894559, 0.3333333333333333703, 0.3219752754296894559, 0.3333333333333333703, 0.3219752754296894559, 0.3333333333333333703, 0.3219752754296894559, 0.3333333333333333703, 0.3219752754296894559, 0.3333333333333333703, 0.3219752754296894559, 0.3333333333333333703, 0.3219752754296894559, 0.3333333333333333703, 0.3219752754296894559, 0.3333333333333333703, 0.3219752754296894559, 0.3333333333333333703, 0.3219752754296894559, 0.3333333333333333703, 0.3219752754296894559, 0.3333333333333333703, 0.3219752754296894559, 0.3333333333333333703, 0.3219752754296894559, 0.3333333333333333703, 0.3219752754296894559, 0.3333333333333333703, 0.3219752754296894559, 0.3333333333333333703, 0.3219752754296894559, 0.3333333333333333703, 0.3219752754296894559, 0.3333333333333333703, 0.3219752754296894559, 0.3333333333333333703, 0.3219752754296894559, 0.3333333333333333703, 0.3219752754296894559, 0.3333333333333333703, 0.3219752754296894559, 0.3333333333333333703, 0.3219752754296894559, 0.3333333333333333703, 0.3219752754296894559, 0.3333333333333333703, 0.3219752754296894559, 0.3333333333333333703, 0.3219752754296894559, 0.3333333333333333703, 0.3219752754296894559, 0.3333333333333333703, 0.3219752754296894559, 0.3333333333333333703, 0.3219752754296894559, 0.3333333333333333703, 0.3219752754296894559, 0.3333333333333333703, 0.3219752754296894559, 0.3333333333333333703, 0.3219752754296894559, 0.3333333333333333703, 0.3219752754296894559, 0.3333333333333333703, 0.3219752754296894559, 0.3333333333333333703, 0.3219752754296894559, 0.3333333333333333703, 0.3219752754296894559, 0.3333333333333333703, 0.3219752754296894559, 0.3333333333333333703, 0.3219752754296894559, 0.3333333333333333703, 0.3219752754296894559, 0.3333333333333333703, 0.3219752754296894559, 0.3333333333333333703, 0.3219752754296894559, 0.3333333333333333703, 0.3219752754296894559, 0.3333333333333333703, 0.3219752754296894559, 0.3333333333333333703, 0.3219752754296894559, 0.3333333333333333703, 0.3219752754296894559, 0.3333333333333333703, 0.3219752754296894559, 0.3333333333333333703, 0.3219752754296894559, 0.3333333333333333703, 0.3219752754296894559, 0.3333333333333333703, 0.3219752754296894559, 0.3333333333333333703, 0.3219752754296894559, 0.3333333333333333703, 0.3219752754296894559, 0.3333333333333333703, 0.3219752754296894559, 0.3333333333333333703, 0.3219752754296894559, 0.3333333333333333703, 0.3219752754296894559, 0.3333333333333333703, 0.3219752754296894559, 0.3333333333333333703, 0.3219752754296894559, 0.3333333333333333703, 0.3219752754296894559, 0.3333333333333333703, 0.3219752754296894559, 0.3333333333333333703, 0.3219752754296894559, 0.3333333333333333703, 0.3219752754296894559, 0.3333333333333333703, 0.3219752754296894559, 0.3333333333333333703, 0.3219752754296894559, 0.3333333333333333703, 0.3219752754296894559, 0.3333333333333333703, 0.3219752754296894559, 0.3333333333333333703, 0.3219752754296894559, 0.3333333333333333703, 0.3219752754296894559, 0.3333333333333333703, 0.3219752754296894559, 0.3333333333333333703, 0.3219752754296894559, 0.3333333333333333703, 0.3219752754296894559, 0.3333333333333333703, 0.3219752754296894559, 0.3333333333333333703, 0.3219752754296894559, 0.3333333333333333703, 0.3219752754296894559, 0.3333333333333333703, 0.3219752754296894559, 0.3333333333333333703, 0.3219752754296894559, 0.3333333333333333703, 0.3219752754296894559, 0.3333333333333333703, 0.3219752754296894559, 0.3333333333333333703, 0.3219752754296894559, 0.3333333333333333703, 0.3219752754296894559, 0.3333333333333333703, 0.3219752754296894559, 0.3333333333333333703, 0.3219752754296894559, 0.3333333333333333703, 0.3219752754296894559, 0.3333333333333333703, 0.3219752754296894559, 0.3333333333333333703, 0.3219752754296894559, 0.3333333333333333703, 0.3219752754296894559, 0.3333333333333333703, 0.3219752754296894559, 0.3333333333333333703, 0.3219752754296894559, 0.3333333333333333703, 0.3219752754296894559, 0.3333333333333333703, 0.3219752754296894559, 0.3333333333333333703, 0.3219752754296894559, 0.3333333333333333703, 0.3219752754296894559, 0.3333333333333333703, 0.3219752754296894559, 0.3333333333333333703, 0.3219752754296894559, 0.3333333333333333703, 0.3219752754296894559, 0.3333333333333333703, 0.3219752754296894559, 0.3333333333333333703, 0.3219752754296894559, 0.3333333333333333703, 0.3219752754296894559, 0.3333333333333333703, 0.3219752754296894559, 0.3333333333333333703, 0.3219752754296894559, 0.3333333333333333703, 0.3219752754296894559, 0.3333333333333333703, 0.3219752754296894559, 0.3333333333333333703, 0.3219752754296894559, 0.3333333333333333703, 0.3219752754296894559, 0.3333333333333333703, 0.3219752754296894559, 0.3333333333333333703, 0.3219752754296894559, 0.3333333333333333703, 0.3219752754296894559, 0.3333333333333333703, 0.3219752754296894559, 0.3333333333333333703, 0.3219752754296894559, 0.3333333333333333703, 0.3219752754296894559, 0.3333333333333333703, 0.3219752754296894559, 0.3333333333333333703, 0.3219752754296894559, 0.3333333333333333703, 0.3219752754296894559, 0.3333333333333333703, 0.3219752754296894559, 0.3333333333333333703, 0.3219752754296894559, 0.3333333333333333703, 0.3219752754296894559, 0.3333333333333333703, 0.3219752754296894559, 0.3333333333333333703, 0.3219752754296894559, 0.3333333333333333703, 0.3219752754296894559, 0.3333333333333333703, 0.3219752754296894559, 0.3333333333333333703, 0.3219752754296894559, 0.3333333333333333703, 0.3219752754296894559, 0.3333333333333333703, 0.3219752754296894559, 0.3333333333333333703, 0.3219752754296894559, 0.3333333333333333703, 0.3219752754296894559, 0.3333333333333333703, 0.3219752754296894559, 0.3333333333333333703, 0.3219752754296894559, 0.3333333333333333703, 0.3219752754296894559, 0.3333333333333333703, 0.3219752754296894559, 0.3333333333333333703, 0.3219752754296894559, 0.3333333333333333703, 0.3219752754296894559, 0.3333333333333333703, 0.3219752754296894559, 0.3333333333333333703, 0.3219752754296894559, 0.3333333333333333703, 0.3219752754296894559, 0.3333333333333333703),
 ( 0.3333333333333333703, 0.3219752754296894559, 0.3333333333333333703, 0.3219752754296894559, 0.3333333333333333703, 0.3219752754296894559, 0.3333333333333333703, 0.3219752754296894559, 0.3333333333333333703, 0.3219752754296894559, 0.3333333333333333703, 0.3219752754296894559, 0.3333333333333333703, 0.3219752754296894559, 0.3333333333333333703, 0.3219752754296894559, 0.3333333333333333703, 0.3219752754296894559, 0.3333333333333333703, 0.3219752754296894559, 0.3333333333333333703, 0.3219752754296894559, 0.3333333333333333703, 0.3219752754296894559, 0.3333333333333333703, 0.3219752754296894559, 0.3333333333333333703, 0.3219752754296894559, 0.3333333333333333703, 0.3219752754296894559, 0.3333333333333333703, 0.3219752754296894559, 0.3333333333333333703, 0.3219752754296894559, 0.3333333333333333703, 0.3219752754296894559, 0.3333333333333333703, 0.3219752754296894559, 0.3333333333333333703, 0.3219752754296894559, 0.3333333333333333703, 0.3219752754296894559, 0.3333333333333333703, 0.3219752754296894559, 0.3333333333333333703, 0.3219752754296894559, 0.3333333333333333703, 0.3219752754296894559, 0.3333333333333333703, 0.3219752754296894559, 0.3333333333333333703, 0.3219752754296894559, 0.3333333333333333703, 0.3219752754296894559, 0.3333333333333333703, 0.3219752754296894559, 0.3333333333333333703, 0.3219752754296894559, 0.3333333333333333703, 0.3219752754296894559, 0.3333333333333333703, 0.3219752754296894559, 0.3333333333333333703, 0.3219752754296894559, 0.3333333333333333703, 0.3219752754296894559, 0.3333333333333333703, 0.3219752754296894559, 0.3333333333333333703, 0.3219752754296894559, 0.3333333333333333703, 0.3219752754296894559, 0.3333333333333333703, 0.3219752754296894559, 0.3333333333333333703, 0.3219752754296894559, 0.3333333333333333703, 0.3219752754296894559, 0.3333333333333333703, 0.3219752754296894559, 0.3333333333333333703, 0.3219752754296894559, 0.3333333333333333703, 0.3219752754296894559, 0.3333333333333333703, 0.3219752754296894559, 0.3333333333333333703, 0.3219752754296894559, 0.3333333333333333703, 0.3219752754296894559, 0.3333333333333333703, 0.3219752754296894559, 0.3333333333333333703, 0.3219752754296894559, 0.3333333333333333703, 0.3219752754296894559, 0.3333333333333333703, 0.3219752754296894559, 0.3333333333333333703, 0.3219752754296894559, 0.3333333333333333703, 0.3219752754296894559, 0.3333333333333333703, 0.3219752754296894559, 0.3333333333333333703, 0.3219752754296894559, 0.3333333333333333703, 0.3219752754296894559, 0.3333333333333333703, 0.3219752754296894559, 0.3333333333333333703, 0.3219752754296894559, 0.3333333333333333703, 0.3219752754296894559, 0.3333333333333333703, 0.3219752754296894559, 0.3333333333333333703, 0.3219752754296894559, 0.3333333333333333703, 0.3219752754296894559, 0.3333333333333333703, 0.3219752754296894559, 0.3333333333333333703, 0.3219752754296894559, 0.3333333333333333703, 0.3219752754296894559, 0.3333333333333333703, 0.3219752754296894559, 0.3333333333333333703, 0.3219752754296894559, 0.3333333333333333703, 0.3219752754296894559, 0.3333333333333333703, 0.3219752754296894559, 0.3333333333333333703, 0.3219752754296894559, 0.3333333333333333703, 0.3219752754296894559, 0.3333333333333333703, 0.3219752754296894559, 0.3333333333333333703, 0.3219752754296894559, 0.3333333333333333703, 0.3219752754296894559, 0.3333333333333333703, 0.3219752754296894559, 0.3333333333333333703, 0.3219752754296894559, 0.3333333333333333703, 0.3219752754296894559, 0.3333333333333333703, 0.3219752754296894559, 0.3333333333333333703, 0.3219752754296894559, 0.3333333333333333703, 0.3219752754296894559, 0.3333333333333333703, 0.3219752754296894559, 0.3333333333333333703, 0.3219752754296894559, 0.3333333333333333703, 0.3219752754296894559, 0.3333333333333333703, 0.3219752754296894559, 0.3333333333333333703, 0.3219752754296894559, 0.3333333333333333703, 0.3219752754296894559, 0.3333333333333333703, 0.3219752754296894559, 0.3333333333333333703, 0.3219752754296894559, 0.3333333333333333703, 0.3219752754296894559, 0.3333333333333333703, 0.3219752754296894559, 0.3333333333333333703, 0.3219752754296894559, 0.3333333333333333703, 0.3219752754296894559, 0.3333333333333333703, 0.3219752754296894559, 0.3333333333333333703, 0.3219752754296894559, 0.3333333333333333703, 0.3219752754296894559, 0.3333333333333333703, 0.3219752754296894559, 0.3333333333333333703, 0.3219752754296894559, 0.3333333333333333703, 0.3219752754296894559, 0.3333333333333333703, 0.3219752754296894559, 0.3333333333333333703, 0.3219752754296894559, 0.3333333333333333703, 0.3219752754296894559, 0.3333333333333333703, 0.3219752754296894559, 0.3333333333333333703, 0.3219752754296894559, 0.3333333333333333703, 0.3219752754296894559, 0.3333333333333333703, 0.3219752754296894559, 0.3333333333333333703, 0.3219752754296894559, 0.3333333333333333703, 0.3219752754296894559, 0.3333333333333333703, 0.3219752754296894559, 0.3333333333333333703, 0.3219752754296894559, 0.3333333333333333703, 0.3219752754296894559, 0.3333333333333333703, 0.3219752754296894559, 0.3333333333333333703, 0.3219752754296894559, 0.3333333333333333703, 0.3219752754296894559, 0.3333333333333333703, 0.3219752754296894559, 0.3333333333333333703, 0.3219752754296894559, 0.3333333333333333703, 0.3219752754296894559, 0.3333333333333333703, 0.3219752754296894559, 0.3333333333333333703, 0.3219752754296894559, 0.3333333333333333703, 0.3219752754296894559, 0.3333333333333333703, 0.3219752754296894559, 0.3333333333333333703, 0.3219752754296894559, 0.3333333333333333703, 0.3219752754296894559, 0.3333333333333333703, 0.3219752754296894559, 0.3333333333333333703, 0.3219752754296894559, 0.3333333333333333703, 0.3219752754296894559, 0.3333333333333333703, 0.3219752754296894559, 0.3333333333333333703, 0.3219752754296894559, 0.3333333333333333703, 0.3219752754296894559, 0.3333333333333333703, 0.3219752754296894559, 0.3333333333333333703, 0.3219752754296894559, 0.3333333333333333703, 0.3219752754296894559, 0.3333333333333333703, 0.3219752754296894559, 0.3333333333333333703, 0.3219752754296894559, 0.3333333333333333703, 0.3219752754296894559, 0.3333333333333333703, 0.3219752754296894559, 0.3333333333333333703, 0.3219752754296894559, 0.3333333333333333703, 0.3219752754296894559, 0.3333333333333333703, 0.3219752754296894559, 0.3333333333333333703, 0.3219752754296894559, 0.3333333333333333703, 0.3219752754296894559, 0.3333333333333333703, 0.3219752754296894559, 0.3333333333333333703, 0.3219752754296894559, 0.3333333333333333703, 0.3219752754296894559, 0.3333333333333333703, 0.3219752754296894559, 0.3333333333333333703, 0.3219752754296894559, 0.3333333333333333703, 0.3219752754296894559, 0.3333333333333333703, 0.3219752754296894559, 0.3333333333333333703, 0.3219752754296894559, 0.3333333333333333703, 0.3219752754296894559, 0.3333333333333333703, 0.3219752754296894559, 0.3333333333333333703, 0.3219752754296894559, 0.3333333333333333703, 0.3219752754296894559, 0.3333333333333333703, 0.3219752754296894559, 0.3333333333333333703, 0.3219752754296894559, 0.3333333333333333703, 0.3219752754296894559, 0.3333333333333333703, 0.3219752754296894559, 0.3333333333333333703, 0.3219752754296894559, 0.3333333333333333703, 0.3219752754296894559, 0.3333333333333333703, 0.3219752754296894559, 0.3333333333333333703, 0.3219752754296894559, 0.3333333333333333703, 0.3219752754296894559, 0.3333333333333333703, 0.3219752754296894559, 0.3333333333333333703, 0.3219752754296894559, 0.3333333333333333703, 0.3219752754296894559, 0.3333333333333333703, 0.3219752754296894559, 0.3333333333333333703, 0.3219752754296894559, 0.3333333333333333703, 0.3219752754296894559, 0.3333333333333333703, 0.3219752754296894559, 0.3333333333333333703, 0.3219752754296894559, 0.3333333333333333703, 0.3219752754296894559, 0.3333333333333333703, 0.3219752754296894559, 0.3333333333333333703, 0.3219752754296894559, 0.3333333333333333703, 0.3219752754296894559, 0.3333333333333333703, 0.3219752754296894559, 0.3333333333333333703, 0.3219752754296894559, 0.3333333333333333703, 0.3219752754296894559, 0.3333333333333333703, 0.3219752754296894559, 0.3333333333333333703, 0.3219752754296894559, 0.3333333333333333703, 0.3219752754296894559, 0.3333333333333333703, 0.3219752754296894559, 0.3333333333333333703, 0.3219752754296894559, 0.3333333333333333703, 0.3219752754296894559, 0.3333333333333333703, 0.3219752754296894559, 0.3333333333333333703, 0.3219752754296894559, 0.3333333333333333703, 0.3219752754296894559, 0.3333333333333333703, 0.3219752754296894559, 0.3333333333333333703, 0.3219752754296894559, 0.3333333333333333703, 0.3219752754296894559, 0.3333333333333333703, 0.3219752754296894559, 0.3333333333333333703, 0.3219752754296894559, 0.3333333333333333703, 0.3219752754296894559, 0.3333333333333333703, 0.3219752754296894559, 0.3333333333333333703, 0.3219752754296894559, 0.3333333333333333703, 0.3219752754296894559, 0.3333333333333333703, 0.3219752754296894559, 0.3333333333333333703, 0.3219752754296894559, 0.3333333333333333703, 0.3219752754296894559, 0.3333333333333333703, 0.3219752754296894559, 0.3333333333333333703, 0.3219752754296894559, 0.3333333333333333703, 0.3219752754296894559, 0.3333333333333333703, 0.3219752754296894559, 0.3333333333333333703, 0.3219752754296894559, 0.3333333333333333703, 0.3219752754296894559, 0.3333333333333333703, 0.3219752754296894559, 0.3333333333333333703, 0.3219752754296894559, 0.3333333333333333703, 0.3219752754296894559, 0.3333333333333333703, 0.3219752754296894559, 0.3333333333333333703, 0.3219752754296894559, 0.3333333333333333703, 0.3219752754296894559, 0.3333333333333333703, 0.3219752754296894559, 0.3333333333333333703, 0.3219752754296894559, 0.3333333333333333703, 0.3219752754296894559, 0.3333333333333333703, 0.3219752754296894559, 0.3333333333333333703, 0.3219752754296894559, 0.3333333333333333703, 0.3219752754296894559, 0.3333333333333333703, 0.3219752754296894559, 0.3333333333333333703, 0.3219752754296894559, 0.3333333333333333703, 0.3219752754296894559, 0.3333333333333333703, 0.3219752754296894559, 0.3333333333333333703, 0.3219752754296894559, 0.3333333333333333703, 0.3219752754296894559, 0.3333333333333333703, 0.3219752754296894559, 0.3333333333333333703, 0.3219752754296894559, 0.3333333333333333703, 0.3219752754296894559, 0.3333333333333333703, 0.3219752754296894559, 0.3333333333333333703, 0.3219752754296894559, 0.3333333333333333703, 0.3219752754296894559, 0.3333333333333333703, 0.3219752754296894559, 0.3333333333333333703, 0.3219752754296894559, 0.3333333333333333703, 0.3219752754296894559, 0.3333333333333333703),
 ( 1.000000000000000000, 0.9659258262890683122, 1.000000000000000000, 0.9659258262890683122, 1.000000000000000000, 0.9659258262890683122, 1.000000000000000000, 0.9659258262890683122, 1.000000000000000000, 0.9659258262890683122, 1.000000000000000000, 0.9659258262890683122, 1.000000000000000000, 0.9659258262890683122, 1.000000000000000000, 0.9659258262890683122, 1.000000000000000000, 0.9659258262890683122, 1.000000000000000000, 0.9659258262890683122, 1.000000000000000000, 0.9659258262890683122, 1.000000000000000000, 0.9659258262890683122, 1.000000000000000000, 0.9659258262890683122, 1.000000000000000000, 0.9659258262890683122, 1.000000000000000000, 0.9659258262890683122, 1.000000000000000000, 0.9659258262890683122, 1.000000000000000000, 0.9659258262890683122, 1.000000000000000000, 0.9659258262890683122, 1.000000000000000000, 0.9659258262890683122, 1.000000000000000000, 0.9659258262890683122, 1.000000000000000000, 0.9659258262890683122, 1.000000000000000000, 0.9659258262890683122, 1.000000000000000000, 0.9659258262890683122, 1.000000000000000000, 0.9659258262890683122, 1.000000000000000000, 0.9659258262890683122, 1.000000000000000000, 0.9659258262890683122, 1.000000000000000000, 0.9659258262890683122, 1.000000000000000000, 0.9659258262890683122, 1.000000000000000000, 0.9659258262890683122, 1.000000000000000000, 0.9659258262890683122, 1.000000000000000000, 0.9659258262890683122, 1.000000000000000000, 0.9659258262890683122, 1.000000000000000000, 0.9659258262890683122, 1.000000000000000000, 0.9659258262890683122, 1.000000000000000000, 0.9659258262890683122, 1.000000000000000000, 0.9659258262890683122, 1.000000000000000000, 0.9659258262890683122, 1.000000000000000000, 0.9659258262890683122, 1.000000000000000000, 0.9659258262890683122, 1.000000000000000000, 0.9659258262890683122, 1.000000000000000000, 0.9659258262890683122, 1.000000000000000000, 0.9659258262890683122, 1.000000000000000000, 0.9659258262890683122, 1.000000000000000000, 0.9659258262890683122, 1.000000000000000000, 0.9659258262890683122, 1.000000000000000000, 0.9659258262890683122, 1.000000000000000000, 0.9659258262890683122, 1.000000000000000000, 0.9659258262890683122, 1.000000000000000000, 0.9659258262890683122, 1.000000000000000000, 0.9659258262890683122, 1.000000000000000000, 0.9659258262890683122, 1.000000000000000000, 0.9659258262890683122, 1.000000000000000000, 0.9659258262890683122, 1.000000000000000000, 0.9659258262890683122, 1.000000000000000000, 0.9659258262890683122, 1.000000000000000000, 0.9659258262890683122, 1.000000000000000000, 0.9659258262890683122, 1.000000000000000000, 0.9659258262890683122, 1.000000000000000000, 0.9659258262890683122, 1.000000000000000000, 0.9659258262890683122, 1.000000000000000000, 0.9659258262890683122, 1.000000000000000000, 0.9659258262890683122, 1.000000000000000000, 0.9659258262890683122, 1.000000000000000000, 0.9659258262890683122, 1.000000000000000000, 0.9659258262890683122, 1.000000000000000000, 0.9659258262890683122, 1.000000000000000000, 0.9659258262890683122, 1.000000000000000000, 0.9659258262890683122, 1.000000000000000000, 0.9659258262890683122, 1.000000000000000000, 0.9659258262890683122, 1.000000000000000000, 0.9659258262890683122, 1.000000000000000000, 0.9659258262890683122, 1.000000000000000000, 0.9659258262890683122, 1.000000000000000000, 0.9659258262890683122, 1.000000000000000000, 0.9659258262890683122, 1.000000000000000000, 0.9659258262890683122, 1.000000000000000000, 0.9659258262890683122, 1.000000000000000000, 0.9659258262890683122, 1.000000000000000000, 0.9659258262890683122, 1.000000000000000000, 0.9659258262890683122, 1.000000000000000000, 0.9659258262890683122, 1.000000000000000000, 0.9659258262890683122, 1.000000000000000000, 0.9659258262890683122, 1.000000000000000000, 0.9659258262890683122, 1.000000000000000000, 0.9659258262890683122, 1.000000000000000000, 0.9659258262890683122, 1.000000000000000000, 0.9659258262890683122, 1.000000000000000000, 0.9659258262890683122, 1.000000000000000000, 0.9659258262890683122, 1.000000000000000000, 0.9659258262890683122, 1.000000000000000000, 0.9659258262890683122, 1.000000000000000000, 0.9659258262890683122, 1.000000000000000000, 0.9659258262890683122, 1.000000000000000000, 0.9659258262890683122, 1.000000000000000000, 0.9659258262890683122, 1.000000000000000000, 0.9659258262890683122, 1.000000000000000000, 0.9659258262890683122, 1.000000000000000000, 0.9659258262890683122, 1.000000000000000000, 0.9659258262890683122, 1.000000000000000000, 0.9659258262890683122, 1.000000000000000000, 0.9659258262890683122, 1.000000000000000000, 0.9659258262890683122, 1.000000000000000000, 0.9659258262890683122, 1.000000000000000000, 0.9659258262890683122, 1.000000000000000000, 0.9659258262890683122, 1.000000000000000000, 0.9659258262890683122, 1.000000000000000000, 0.9659258262890683122, 1.000000000000000000, 0.9659258262890683122, 1.000000000000000000, 0.9659258262890683122, 1.000000000000000000, 0.9659258262890683122, 1.000000000000000000, 0.9659258262890683122, 1.000000000000000000, 0.9659258262890683122, 1.000000000000000000, 0.9659258262890683122, 1.000000000000000000, 0.9659258262890683122, 1.000000000000000000, 0.9659258262890683122, 1.000000000000000000, 0.9659258262890683122, 1.000000000000000000, 0.9659258262890683122, 1.000000000000000000, 0.9659258262890683122, 1.000000000000000000, 0.9659258262890683122, 1.000000000000000000, 0.9659258262890683122, 1.000000000000000000, 0.9659258262890683122, 1.000000000000000000, 0.9659258262890683122, 1.000000000000000000, 0.9659258262890683122, 1.000000000000000000, 0.9659258262890683122, 1.000000000000000000, 0.9659258262890683122, 1.000000000000000000, 0.9659258262890683122, 1.000000000000000000, 0.9659258262890683122, 1.000000000000000000, 0.9659258262890683122, 1.000000000000000000, 0.9659258262890683122, 1.000000000000000000, 0.9659258262890683122, 1.000000000000000000, 0.9659258262890683122, 1.000000000000000000, 0.9659258262890683122, 1.000000000000000000, 0.9659258262890683122, 1.000000000000000000, 0.9659258262890683122, 1.000000000000000000, 0.9659258262890683122, 1.000000000000000000, 0.9659258262890683122, 1.000000000000000000, 0.9659258262890683122, 1.000000000000000000, 0.9659258262890683122, 1.000000000000000000, 0.9659258262890683122, 1.000000000000000000, 0.9659258262890683122, 1.000000000000000000, 0.9659258262890683122, 1.000000000000000000, 0.9659258262890683122, 1.000000000000000000, 0.9659258262890683122, 1.000000000000000000, 0.9659258262890683122, 1.000000000000000000, 0.9659258262890683122, 1.000000000000000000, 0.9659258262890683122, 1.000000000000000000, 0.9659258262890683122, 1.000000000000000000, 0.9659258262890683122, 1.000000000000000000, 0.9659258262890683122, 1.000000000000000000, 0.9659258262890683122, 1.000000000000000000, 0.9659258262890683122, 1.000000000000000000, 0.9659258262890683122, 1.000000000000000000, 0.9659258262890683122, 1.000000000000000000, 0.9659258262890683122, 1.000000000000000000, 0.9659258262890683122, 1.000000000000000000, 0.9659258262890683122, 1.000000000000000000, 0.9659258262890683122, 1.000000000000000000, 0.9659258262890683122, 1.000000000000000000, 0.9659258262890683122, 1.000000000000000000, 0.9659258262890683122, 1.000000000000000000, 0.9659258262890683122, 1.000000000000000000, 0.9659258262890683122, 1.000000000000000000, 0.9659258262890683122, 1.000000000000000000, 0.9659258262890683122, 1.000000000000000000, 0.9659258262890683122, 1.000000000000000000, 0.9659258262890683122, 1.000000000000000000, 0.9659258262890683122, 1.000000000000000000, 0.9659258262890683122, 1.000000000000000000, 0.9659258262890683122, 1.000000000000000000, 0.9659258262890683122, 1.000000000000000000, 0.9659258262890683122, 1.000000000000000000, 0.9659258262890683122, 1.000000000000000000, 0.9659258262890683122, 1.000000000000000000, 0.9659258262890683122, 1.000000000000000000, 0.9659258262890683122, 1.000000000000000000, 0.9659258262890683122, 1.000000000000000000, 0.9659258262890683122, 1.000000000000000000, 0.9659258262890683122, 1.000000000000000000, 0.9659258262890683122, 1.000000000000000000, 0.9659258262890683122, 1.000000000000000000, 0.9659258262890683122, 1.000000000000000000, 0.9659258262890683122, 1.000000000000000000, 0.9659258262890683122, 1.000000000000000000, 0.9659258262890683122, 1.000000000000000000, 0.9659258262890683122, 1.000000000000000000, 0.9659258262890683122, 1.000000000000000000, 0.9659258262890683122, 1.000000000000000000, 0.9659258262890683122, 1.000000000000000000, 0.9659258262890683122, 1.000000000000000000, 0.9659258262890683122, 1.000000000000000000, 0.9659258262890683122, 1.000000000000000000, 0.9659258262890683122, 1.000000000000000000, 0.9659258262890683122, 1.000000000000000000, 0.9659258262890683122, 1.000000000000000000, 0.9659258262890683122, 1.000000000000000000, 0.9659258262890683122, 1.000000000000000000, 0.9659258262890683122, 1.000000000000000000, 0.9659258262890683122, 1.000000000000000000, 0.9659258262890683122, 1.000000000000000000, 0.9659258262890683122, 1.000000000000000000, 0.9659258262890683122, 1.000000000000000000, 0.9659258262890683122, 1.000000000000000000, 0.9659258262890683122, 1.000000000000000000, 0.9659258262890683122, 1.000000000000000000, 0.9659258262890683122, 1.000000000000000000, 0.9659258262890683122, 1.000000000000000000, 0.9659258262890683122, 1.000000000000000000, 0.9659258262890683122, 1.000000000000000000, 0.9659258262890683122, 1.000000000000000000, 0.9659258262890683122, 1.000000000000000000, 0.9659258262890683122, 1.000000000000000000, 0.9659258262890683122, 1.000000000000000000, 0.9659258262890683122, 1.000000000000000000, 0.9659258262890683122, 1.000000000000000000, 0.9659258262890683122, 1.000000000000000000, 0.9659258262890683122, 1.000000000000000000, 0.9659258262890683122, 1.000000000000000000, 0.9659258262890683122, 1.000000000000000000, 0.9659258262890683122, 1.000000000000000000, 0.9659258262890683122, 1.000000000000000000, 0.9659258262890683122, 1.000000000000000000, 0.9659258262890683122, 1.000000000000000000, 0.9659258262890683122, 1.000000000000000000, 0.9659258262890683122, 1.000000000000000000, 0.9659258262890683122, 1.000000000000000000, 0.9659258262890683122, 1.000000000000000000, 0.9659258262890683122, 1.000000000000000000, 0.9659258262890683122, 1.000000000000000000) ) ) 
 REPRESENTATION_ITEM ( '' )  SURFACE ( )  );
#122906=CARTESIAN_POINT ( 'NONE',  ( 21.52544592524344225, -5.823673210054117533, 23.54057627198102765 ) ) ;
#122907=CARTESIAN_POINT ( 'NONE',  ( 21.55341960407619695, -5.719274019375665929, 36.04275706135234714 ) ) ;
#122908=CARTESIAN_POINT ( 'NONE',  ( -19.02544592524334988, -5.153800228976617603, 98.95942372801900433 ) ) ;
#122910=CARTESIAN_POINT ( 'NONE',  ( -19.02544592524342804, 5.153800228976336051, 66.04057627198103830 ) ) ;
#122911=CARTESIAN_POINT ( 'NONE',  ( 9.474510206698971260, -16.51473224551069308, 97.91557627198102409 ) ) ;
#122912=CARTESIAN_POINT ( 'NONE',  ( -0.05219959533910754901, -16.53943276465976808, 67.49890960531436690 ) ) ;
#122913=CARTESIAN_POINT ( 'NONE',  ( -13.97604488694527625, -13.89961937509977652, 61.87390960531435979 ) ) ;
#122914=CARTESIAN_POINT ( 'NONE',  ( 19.05341960407611168, 5.049401038298154454, 68.95724293864769550 ) ) ;
#122915=CARTESIAN_POINT ( 'NONE',  ( 13.97604488694548053, -13.89961937509957401, 75.62609039468564731 ) ) ;
#122916=CARTESIAN_POINT ( 'NONE',  ( -21.53943276465977519, 0.05219959533907696930, 56.24890960531436690 ) ) ;
#122917=CARTESIAN_POINT ( 'NONE',  ( -16.51473224551069308, -9.474510206698971260, 21.66557627198102765 ) ) ;
#122918=CARTESIAN_POINT ( 'NONE',  ( 0.05219959533936267826, -19.03943276465977164, 40.00109039468566152 ) ) ;
#122919=CARTESIAN_POINT ( 'NONE',  ( 9.474510206698971260, -16.51473224551069308, 77.91557627198103830 ) ) ;
#122920=CARTESIAN_POINT ( 'NONE',  ( -10.72451020669898014, 18.67979575497178502, 70.41557627198102409 ) ) ;
#122921=CARTESIAN_POINT ( 'NONE',  ( 12.06949235617757843, -12.14591786802309237, 78.12390960531436690 ) ) ;
#122922=CARTESIAN_POINT ( 'NONE',  ( 9.564922557961047289, -16.46253265017146816, 35.41775706135233293 ) ) ;
#122923=CARTESIAN_POINT ( 'NONE',  ( -21.55341960407610458, -5.719274019375992779, 66.45724293864768129 ) ) ;
#122924=CARTESIAN_POINT ( 'NONE',  ( -15.80617190586745835, -15.72974639402198527, 41.87390960531435979 ) ) ;
#122925=CARTESIAN_POINT ( 'NONE',  ( 18.67979575497194134, -10.72451020669871369, 90.83442372801901854 ) ) ;
#122926=CARTESIAN_POINT ( 'NONE',  ( -16.46253265017160317, 9.564922557960807481, 60.83224293864769550 ) ) ;
#122927=CARTESIAN_POINT ( 'NONE',  ( -4.483927247898539470, -16.52544592524342804, 112.2905762719810241 ) ) ;
#122928=CARTESIAN_POINT ( 'NONE',  ( 15.80617190586769283, -15.72974639402175789, 25.62609039468567929 ) ) ;
#122930=CARTESIAN_POINT ( 'NONE',  ( -5.719274019375665041, -21.55341960407619695, 44.79275706135234714 ) ) ;
#122931=CARTESIAN_POINT ( 'NONE',  ( 0.05219959533909260263, 19.03943276465977164, 39.99890960531436690 ) ) ;
#122932=CARTESIAN_POINT ( 'NONE',  ( -0.05219959533907301413, -21.53943276465977519, 102.4989096053143811 ) ) ;
#122933=CARTESIAN_POINT ( 'NONE',  ( 19.03943276465977164, 0.05219959533936151252, 41.25109039468566152 ) ) ;
#122934=CARTESIAN_POINT ( 'NONE',  ( 16.46253265017160672, -9.564922557960803928, 38.33224293864768839 ) ) ;
#122935=CARTESIAN_POINT ( 'NONE',  ( 19.02544592524343514, -5.153800228976328945, 23.54057627198102054 ) ) ;
#122936=CARTESIAN_POINT ( 'NONE',  ( 17.31090126489389291, -5.922914322405134158, 21.23212116175356456 ) ) ;
#122937=CARTESIAN_POINT ( 'NONE',  ( -8.224510206698735004, -14.34966873604973081, 64.58442372801900433 ) ) ;
#122938=CARTESIAN_POINT ( 'NONE',  ( 19.03943276465977164, -0.05219959533909143690, 23.74890960531435269 ) ) ;
#122940=CARTESIAN_POINT ( 'NONE',  ( -19.05341960407611168, -5.049401038298163336, 86.45724293864769550 ) ) ;
#122941=CARTESIAN_POINT ( 'NONE',  ( -16.53943276465976808, 0.05219959533911058130, 101.2489096053143669 ) ) ;
#122942=CARTESIAN_POINT ( 'NONE',  ( 21.55341960407610458, 5.719274019375980345, 53.95724293864770260 ) ) ;
#122943=CARTESIAN_POINT ( 'NONE',  ( -12.06949235617739369, -12.14591786802326823, 44.37609039468567573 ) ) ;
#122944=CARTESIAN_POINT ( 'NONE',  ( -10.72451020669870658, -18.67979575497194134, 94.58442372801901854 ) ) ;
#122946=CARTESIAN_POINT ( 'NONE',  ( -16.46253265017160317, 9.564922557960807481, 30.83224293864769550 ) ) ;
#122947=CARTESIAN_POINT ( 'NONE',  ( -16.53943276465976808, 0.05219959533911058130, 21.24890960531436690 ) ) ;
#122948=CARTESIAN_POINT ( 'NONE',  ( -14.29746914071049879, 8.314922557960819915, 55.83224293864770260 ) ) ;
#122949=CARTESIAN_POINT ( 'NONE',  ( -5.153800228976328057, -19.02544592524343514, 47.29057627198102409 ) ) ;
#122950=CARTESIAN_POINT ( 'NONE',  ( 5.823673210054444382, -21.52544592524334988, 90.20942372801903275 ) ) ;
#122951=CARTESIAN_POINT ( 'NONE',  ( 5.719274019375673035, 21.55341960407619339, 22.29275706135235069 ) ) ;
#122952=CARTESIAN_POINT ( 'NONE',  ( 15.80617190586769283, -15.72974639402175789, 70.62609039468567573 ) ) ;
#122953=CARTESIAN_POINT ( 'NONE',  ( -8.314922557961024197, 14.29746914071037800, 57.91775706135234714 ) ) ;
#122954=CARTESIAN_POINT ( 'NONE',  ( 4.483927247898545687, 16.52544592524342804, 79.79057627198102409 ) ) ;
#122955=CARTESIAN_POINT ( 'NONE',  ( -15.72974639402176322, -15.80617190586768395, 99.37609039468568994 ) ) ;
#122956=EDGE_CURVE ( 'NONE', #163173, #78021, #118826, .T. ) ;
#122957=CARTESIAN_POINT ( 'NONE',  ( 0.05219959533934541429, -16.53943276465976808, 110.0010903946856757 ) ) ;
#122959=CARTESIAN_POINT ( 'NONE',  ( 12.14591786802327356, -12.06949235617739191, 35.62609039468568994 ) ) ;
#122960=CARTESIAN_POINT ( 'NONE',  ( -0.05219959533910754901, -16.53943276465976808, 37.49890960531436690 ) ) ;
#122961=CARTESIAN_POINT ( 'NONE',  ( -12.06949235617739369, -12.14591786802326823, 84.37609039468570415 ) ) ;
#122962=CARTESIAN_POINT ( 'NONE',  ( -5.153800228976328057, -19.02544592524343514, 102.2905762719810383 ) ) ;
#122963=CARTESIAN_POINT ( 'NONE',  ( 5.719274019375991003, -21.55341960407610458, 22.70724293864769194 ) ) ;
#122964=CARTESIAN_POINT ( 'NONE',  ( -18.62759615963255300, -10.81492255796106328, 99.16775706135234714 ) ) ;
#122965=CARTESIAN_POINT ( 'NONE',  ( 12.14591786802327356, -12.06949235617739191, 100.6260903946857184 ) ) ;
#122966=CARTESIAN_POINT ( 'NONE',  ( -8.224510206698948167, 14.34966873604960824, 70.41557627198102409 ) ) ;
#122967=CARTESIAN_POINT ( 'NONE',  ( -9.474510206698964154, 16.51473224551069663, 80.41557627198103830 ) ) ;
#122969=CARTESIAN_POINT ( 'NONE',  ( -4.379528057220086978, -16.55341960407618274, 34.79275706135235424 ) ) ;
#122970=CARTESIAN_POINT ( 'NONE',  ( 16.51473224551069308, 9.474510206698969483, 39.16557627198103120 ) ) ;
#122971=CARTESIAN_POINT ( 'NONE',  ( -16.51473224551069308, -9.474510206698971260, 91.66557627198103830 ) ) ;
#122972=CARTESIAN_POINT ( 'NONE',  ( 4.483927247898790824, -16.52544592524335698, 30.20942372801902565 ) ) ;
#122974=CARTESIAN_POINT ( 'NONE',  ( -19.05341960407617563, 5.049401038297882671, 33.54275706135231871 ) ) ;
#122975=CARTESIAN_POINT ( 'NONE',  ( -8.314922557961024197, 14.29746914071037800, 97.91775706135236135 ) ) ;
#122976=CARTESIAN_POINT ( 'NONE',  ( 9.564922557960805705, 16.46253265017160317, 34.58224293864770260 ) ) ;
#122977=CARTESIAN_POINT ( 'NONE',  ( -12.06949235617739369, -12.14591786802326823, 79.37609039468567573 ) ) ;
#122978=CARTESIAN_POINT ( 'NONE',  ( 8.314922557961029526, -14.29746914071037800, 65.41775706135234714 ) ) ;
#122979=CARTESIAN_POINT ( 'NONE',  ( -0.05219959533936034679, 19.03943276465977164, 82.50109039468567573 ) ) ;
#122980=CARTESIAN_POINT ( 'NONE',  ( 13.89961937509957401, 13.97604488694547697, 26.87609039468566507 ) ) ;
#122981=CARTESIAN_POINT ( 'NONE',  ( 9.564922557960805705, 16.46253265017160317, 54.58224293864769550 ) ) ;
#122982=CARTESIAN_POINT ( 'NONE',  ( 14.34966873604960469, 8.224510206698951720, 89.16557627198102409 ) ) ;
#122983=CARTESIAN_POINT ( 'NONE',  ( 5.049401038297881783, 19.05341960407617563, 57.29275706135231871 ) ) ;
#122984=CARTESIAN_POINT ( 'NONE',  ( 21.53943276465977519, -0.05219959533907433946, 48.74890960531435979 ) ) ;
#122985=CARTESIAN_POINT ( 'NONE',  ( -13.97604488694547697, 13.89961937509957934, 28.12609039468565797 ) ) ;
#122986=CARTESIAN_POINT ( 'NONE',  ( -9.474510206698964154, 16.51473224551069663, 110.4155762719810383 ) ) ;
#122988=CARTESIAN_POINT ( 'NONE',  ( -21.53943276465977519, 0.05219959533907696930, 76.24890960531435269 ) ) ;
#122989=CARTESIAN_POINT ( 'NONE',  ( 13.97604488694527802, 13.89961937509977652, 114.3739096053143669 ) ) ;
#122990=CARTESIAN_POINT ( 'NONE',  ( -0.05219959533936034679, 19.03943276465977164, 102.5010903946856757 ) ) ;
#122991=CARTESIAN_POINT ( 'NONE',  ( -19.02544592524342804, 5.153800228976336051, 116.0405762719810383 ) ) ;
#122992=CARTESIAN_POINT ( 'NONE',  ( 19.03943276465977164, 0.05219959533936151252, 111.2510903946856757 ) ) ;
#122993=CARTESIAN_POINT ( 'NONE',  ( -19.03943276465977164, 0.05219959533909376836, 36.24890960531436690 ) ) ;
#122994=CARTESIAN_POINT ( 'NONE',  ( -19.05341960407611168, -5.049401038298163336, 101.4572429386476955 ) ) ;
#122995=CARTESIAN_POINT ( 'NONE',  ( -10.81492255796078084, -18.62759615963271287, 77.08224293864769550 ) ) ;
#122996=CARTESIAN_POINT ( 'NONE',  ( -12.14591786802326823, 12.06949235617739902, 63.12609039468568994 ) ) ;
#122997=CARTESIAN_POINT ( 'NONE',  ( -21.55341960407619339, 5.719274019375674811, 58.54275706135235424 ) ) ;
#122998=CARTESIAN_POINT ( 'NONE',  ( 16.51473224551083163, -9.474510206698727899, 105.8344237280190043 ) ) ;
#122999=CARTESIAN_POINT ( 'NONE',  ( 15.72974639402176855, 15.80617190586768217, 111.8760903946856615 ) ) ;
#123000=CARTESIAN_POINT ( 'NONE',  ( -12.14591786802326823, 12.06949235617739902, 108.1260903946856757 ) ) ;
#123001=CARTESIAN_POINT ( 'NONE',  ( 18.62759615963271287, -10.81492255796078972, 103.3322429386476955 ) ) ;
#123002=CARTESIAN_POINT ( 'NONE',  ( -4.379528057220328563, 16.55341960407611168, 35.20724293864768839 ) ) ;
#123003=CARTESIAN_POINT ( 'NONE',  ( 19.05341960407617918, -5.049401038297876454, 76.04275706135230450 ) ) ;
#123004=CARTESIAN_POINT ( 'NONE',  ( -5.719274019375665041, -21.55341960407619695, 54.79275706135235424 ) ) ;
#123005=CARTESIAN_POINT ( 'NONE',  ( -19.03943276465977164, -0.05219959533935918106, 33.75109039468566863 ) ) ;
#123006=CARTESIAN_POINT ( 'NONE',  ( 12.06949235617757843, -12.14591786802309237, 103.1239096053143811 ) ) ;
#123007=CARTESIAN_POINT ( 'NONE',  ( 0.05219959533907565091, 21.53943276465977519, 29.99890960531435979 ) ) ;
#123008=CARTESIAN_POINT ( 'NONE',  ( 16.52544592524342804, -4.483927247898539470, 38.54057627198103120 ) ) ;
#123009=CARTESIAN_POINT ( 'NONE',  ( -18.62759615963255300, -10.81492255796106328, 104.1677570613523471 ) ) ;
#123010=CARTESIAN_POINT ( 'NONE',  ( -12.06949235617739369, -12.14591786802326823, 59.37609039468568284 ) ) ;
#123011=CARTESIAN_POINT ( 'NONE',  ( -16.52544592524342804, 4.483927247898546575, 26.04057627198103475 ) ) ;
#123012=CARTESIAN_POINT ( 'NONE',  ( -18.62759615963255300, -10.81492255796106328, 69.16775706135234714 ) ) ;
#123013=CARTESIAN_POINT ( 'NONE',  ( 21.53943276465977519, 0.05219959533937863772, 51.25109039468568994 ) ) ;
#123015=CARTESIAN_POINT ( 'NONE',  ( -19.05341960407611168, -5.049401038298163336, 21.45724293864768839 ) ) ;
#123016=CARTESIAN_POINT ( 'NONE',  ( -10.81492255796105439, 18.62759615963255655, 47.91775706135234714 ) ) ;
#123017=CARTESIAN_POINT ( 'NONE',  ( -12.06949235617756955, 12.14591786802309770, 110.6239096053143669 ) ) ;
#123018=CARTESIAN_POINT ( 'NONE',  ( 19.02544592524343514, -5.153800228976328945, 43.54057627198103120 ) ) ;
#123019=CARTESIAN_POINT ( 'NONE',  ( 4.379528057220339221, -16.55341960407611168, 82.70724293864770971 ) ) ;
#123020=CARTESIAN_POINT ( 'NONE',  ( -16.51473224551069308, -9.474510206698971260, 71.66557627198102409 ) ) ;
#123021=CARTESIAN_POINT ( 'NONE',  ( 12.06949235617757843, -12.14591786802309237, 28.12390960531435979 ) ) ;
#123022=CARTESIAN_POINT ( 'NONE',  ( -21.55341960407610458, -5.719274019375992779, 56.45724293864768839 ) ) ;
#123023=CARTESIAN_POINT ( 'NONE',  ( 0.05219959533910956823, 16.53943276465976808, 89.99890960531438111 ) ) ;
#123024=CARTESIAN_POINT ( 'NONE',  ( 5.719274019375991003, -21.55341960407610458, 107.7072429386476955 ) ) ;
#123025=CARTESIAN_POINT ( 'NONE',  ( -9.474510206698964154, 16.51473224551069663, 100.4155762719810241 ) ) ;
#123026=CARTESIAN_POINT ( 'NONE',  ( 13.89961937509977652, -13.97604488694527269, 58.12390960531436690 ) ) ;
#123027=CARTESIAN_POINT ( 'NONE',  ( 5.153800228976615827, -19.02544592524334988, 110.2094237280189901 ) ) ;
#123028=CARTESIAN_POINT ( 'NONE',  ( 5.719274019375991003, -21.55341960407610458, 62.70724293864769550 ) ) ;
#123029=CARTESIAN_POINT ( 'NONE',  ( 5.823673210054444382, -21.52544592524334988, 80.20942372801901854 ) ) ;
#123030=CARTESIAN_POINT ( 'NONE',  ( 9.564922557960805705, 16.46253265017160317, 69.58224293864770971 ) ) ;
#123031=CARTESIAN_POINT ( 'NONE',  ( -5.049401038298153566, 19.05341960407611168, 100.2072429386476955 ) ) ;
#123032=CARTESIAN_POINT ( 'NONE',  ( -4.483927247898782831, 16.52544592524335698, 82.70942372801900433 ) ) ;
#123033=CARTESIAN_POINT ( 'NONE',  ( 21.52544592524334988, 5.823673210054432836, 56.45942372801902565 ) ) ;
#123034=CARTESIAN_POINT ( 'NONE',  ( 10.81492255796106328, -18.62759615963255655, 90.41775706135236135 ) ) ;
#123035=CARTESIAN_POINT ( 'NONE',  ( -15.72974639402197994, 15.80617190586746368, 110.6239096053143669 ) ) ;
#123036=CARTESIAN_POINT ( 'NONE',  ( -14.34966873604972548, 8.224510206698743886, 83.33442372801903275 ) ) ;
#123037=CARTESIAN_POINT ( 'NONE',  ( -18.67979575497178146, -10.72451020669898902, 71.66557627198100988 ) ) ;
#123038=CARTESIAN_POINT ( 'NONE',  ( -19.05341960407617563, 5.049401038297882671, 43.54275706135232582 ) ) ;
#123039=CARTESIAN_POINT ( 'NONE',  ( 0.05219959533907565091, 21.53943276465977519, 44.99890960531435979 ) ) ;
#123040=CARTESIAN_POINT ( 'NONE',  ( -0.05219959533909027116, -19.03943276465977164, 82.49890960531436690 ) ) ;
#123041=CARTESIAN_POINT ( 'NONE',  ( -16.53943276465976808, 0.05219959533911058130, 26.24890960531435624 ) ) ;
#123042=CARTESIAN_POINT ( 'NONE',  ( -16.19135201231369692, 7.376712067591781441, 64.81319145947969673 ) ) ;
#123043=CARTESIAN_POINT ( 'NONE',  ( -9.564922557960796823, -16.46253265017161027, 112.0822429386476955 ) ) ;
#123044=CARTESIAN_POINT ( 'NONE',  ( 18.22780087662122384, -5.500000000000022204, 46.01540105326107266 ) ) ;
#123045=CARTESIAN_POINT ( 'NONE',  ( -19.05341960407617563, 5.049401038297882671, 88.54275706135230450 ) ) ;
#123046=CARTESIAN_POINT ( 'NONE',  ( 18.62759615963271287, -10.81492255796078972, 73.33224293864769550 ) ) ;
#123047=CARTESIAN_POINT ( 'NONE',  ( 14.29746914071049879, -8.314922557960816363, 48.33224293864770260 ) ) ;
#123048=CARTESIAN_POINT ( 'NONE',  ( 13.89961937509957401, 13.97604488694547697, 111.8760903946856757 ) ) ;
#123049=CARTESIAN_POINT ( 'NONE',  ( -16.46253265017160317, 9.564922557960807481, 35.83224293864768839 ) ) ;
#123050=CARTESIAN_POINT ( 'NONE',  ( 16.51473224551083163, -9.474510206698727899, 105.8344237280190043 ) ) ;
#123051=CARTESIAN_POINT ( 'NONE',  ( -5.823673210054116645, -21.52544592524344225, 102.2905762719810383 ) ) ;
#123052=CARTESIAN_POINT ( 'NONE',  ( 5.153800228976615827, -19.02544592524334988, 65.20942372801900433 ) ) ;
#123053=CARTESIAN_POINT ( 'NONE',  ( -14.29746914071037622, -8.314922557961029526, 74.16775706135231871 ) ) ;
#123054=CARTESIAN_POINT ( 'NONE',  ( -19.05341960407611168, -5.049401038298163336, 86.45724293864769550 ) ) ;
#123055=CARTESIAN_POINT ( 'NONE',  ( 8.314922557960818139, 14.29746914071049879, 74.58224293864768129 ) ) ;
#123056=CARTESIAN_POINT ( 'NONE',  ( -13.97604488694527625, -13.89961937509977652, 56.87390960531434558 ) ) ;
#123057=CARTESIAN_POINT ( 'NONE',  ( -16.55341960407611168, -4.379528057220339221, 71.45724293864769550 ) ) ;
#123058=CARTESIAN_POINT ( 'NONE',  ( 16.51473224551069308, 9.474510206698969483, 29.16557627198103475 ) ) ;
#123060=CARTESIAN_POINT ( 'NONE',  ( -16.55341960407611168, -4.379528057220339221, 46.45724293864769550 ) ) ;
#123061=CARTESIAN_POINT ( 'NONE',  ( 9.564922557960805705, 16.46253265017160317, 89.58224293864769550 ) ) ;
#123063=CARTESIAN_POINT ( 'NONE',  ( 5.153800228976615827, -19.02544592524334988, 55.20942372801899722 ) ) ;
#123064=CARTESIAN_POINT ( 'NONE',  ( 12.06949235617739724, 12.14591786802326823, 61.87609039468568284 ) ) ;
#123065=CARTESIAN_POINT ( 'NONE',  ( 21.55341960407610458, 5.719274019375980345, 58.95724293864770971 ) ) ;
#123066=CARTESIAN_POINT ( 'NONE',  ( 19.02544592524334988, 5.153800228976608722, 26.45942372801899722 ) ) ;
#123067=CARTESIAN_POINT ( 'NONE',  ( 9.474510206698971260, -16.51473224551069308, 92.91557627198103830 ) ) ;
#123069=CARTESIAN_POINT ( 'NONE',  ( -10.72451020669898014, 18.67979575497178502, 25.41557627198103120 ) ) ;
#123070=CARTESIAN_POINT ( 'NONE',  ( -19.02544592524342804, 5.153800228976336051, 61.04057627198103120 ) ) ;
#123071=CARTESIAN_POINT ( 'NONE',  ( 18.67979575497194134, -10.72451020669871369, 50.83442372801901143 ) ) ;
#123072=CARTESIAN_POINT ( 'NONE',  ( 14.29746914071049879, -8.314922557960816363, 103.3322429386476955 ) ) ;
#123073=CARTESIAN_POINT ( 'NONE',  ( 10.81492255796078972, 18.62759615963270932, 104.5822429386477097 ) ) ;
#123074=CARTESIAN_POINT ( 'NONE',  ( 5.153800228976335163, 19.02544592524342804, 99.79057627198102409 ) ) ;
#123076=CARTESIAN_POINT ( 'NONE',  ( -5.719274019375665041, -21.55341960407619695, 34.79275706135235424 ) ) ;
#123077=VERTEX_POINT ( 'NONE', #62885 ) ;
#123078=CARTESIAN_POINT ( 'NONE',  ( -19.03943276465977164, 0.05219959533909376836, 101.2489096053143669 ) ) ;
#123080=CARTESIAN_POINT ( 'NONE',  ( 18.67979575497178502, 10.72451020669898547, 94.16557627198103830 ) ) ;
#123081=CARTESIAN_POINT ( 'NONE',  ( -9.564922557960796823, -16.46253265017161027, 42.08224293864769550 ) ) ;
#123082=CARTESIAN_POINT ( 'NONE',  ( -8.224510206698735004, -14.34966873604973081, 19.58442372801901143 ) ) ;
#123084=CARTESIAN_POINT ( 'NONE',  ( 16.46253265017160672, -9.564922557960803928, 28.33224293864769550 ) ) ;
#123085=CARTESIAN_POINT ( 'NONE',  ( 18.67979575497194134, -10.72451020669871369, 100.8344237280190185 ) ) ;
#123086=CARTESIAN_POINT ( 'NONE',  ( 16.51473224551069308, 9.474510206698969483, 74.16557627198103830 ) ) ;
#123087=CARTESIAN_POINT ( 'NONE',  ( -0.05219959533937732626, 21.53943276465977519, 47.50109039468568994 ) ) ;
#123088=CARTESIAN_POINT ( 'NONE',  ( -0.05219959533937732626, 21.53943276465977519, 27.50109039468567929 ) ) ;
#123090=CARTESIAN_POINT ( 'NONE',  ( 19.02544592524343514, -5.153800228976328945, 103.5405762719809957 ) ) ;
#123092=CARTESIAN_POINT ( 'NONE',  ( -16.52544592524335698, -4.483927247898792601, 33.95942372801901143 ) ) ;
#123093=CARTESIAN_POINT ( 'NONE',  ( 16.55341960407618274, -4.379528057220086978, 71.04275706135234714 ) ) ;
#123094=CARTESIAN_POINT ( 'NONE',  ( -21.52544592524334988, -5.823673210054445271, 53.95942372801900433 ) ) ;
#123095=CARTESIAN_POINT ( 'NONE',  ( 21.55341960407619695, -5.719274019375665929, 81.04275706135236135 ) ) ;
#123097=CARTESIAN_POINT ( 'NONE',  ( -19.03943276465977164, -0.05219959533935918106, 103.7510903946856757 ) ) ;
#123098=CARTESIAN_POINT ( 'NONE',  ( 19.05341960407611168, 5.049401038298154454, 73.95724293864768129 ) ) ;
#123099=CARTESIAN_POINT ( 'NONE',  ( 19.03943276465977164, -0.05219959533909143690, 93.74890960531435269 ) ) ;
#123100=CARTESIAN_POINT ( 'NONE',  ( 12.14591786802309770, 12.06949235617756955, 109.3739096053143811 ) ) ;
#123101=CARTESIAN_POINT ( 'NONE',  ( -18.62759615963270932, 10.81492255796079327, 25.83224293864769194 ) ) ;
#123102=EDGE_CURVE ( 'NONE', #123348, #114473, #121564, .T. ) ;
#123103=CARTESIAN_POINT ( 'NONE',  ( 4.379528057220092307, 16.55341960407617563, 87.29275706135236135 ) ) ;
#123104=CARTESIAN_POINT ( 'NONE',  ( 8.224510206698953496, -14.34966873604960469, 72.91557627198103830 ) ) ;
#123105=CARTESIAN_POINT ( 'NONE',  ( -16.46253265017160317, 9.564922557960807481, 50.83224293864770260 ) ) ;
#123106=CARTESIAN_POINT ( 'NONE',  ( -18.62759615963255300, -10.81492255796106328, 74.16775706135231871 ) ) ;
#123108=CARTESIAN_POINT ( 'NONE',  ( -13.97604488694547697, 13.89961937509957934, 108.1260903946856331 ) ) ;
#123109=CARTESIAN_POINT ( 'NONE',  ( 4.483927247898545687, 16.52544592524342804, 74.79057627198105251 ) ) ;
#123110=CARTESIAN_POINT ( 'NONE',  ( 18.67979575497194134, -10.72451020669871369, 25.83442372801901499 ) ) ;
#123111=CARTESIAN_POINT ( 'NONE',  ( 15.72974639402199770, -15.80617190586745480, 63.12390960531435979 ) ) ;
#123112=CARTESIAN_POINT ( 'NONE',  ( -16.36317988757055630, -7.306389748694962272, 105.9021039163677358 ) ) ;
#123114=CARTESIAN_POINT ( 'NONE',  ( -19.05341960407611168, -5.049401038298163336, 86.45724293864769550 ) ) ;
#123115=CARTESIAN_POINT ( 'NONE',  ( -14.29746914071049879, 8.314922557960819915, 50.83224293864770971 ) ) ;
#123116=CARTESIAN_POINT ( 'NONE',  ( 12.14591786802309770, 12.06949235617756955, 24.37390960531435979 ) ) ;
#123117=CARTESIAN_POINT ( 'NONE',  ( 4.483927247898790824, -16.52544592524335698, 95.20942372801903275 ) ) ;
#123118=CARTESIAN_POINT ( 'NONE',  ( 5.049401038297881783, 19.05341960407617563, 52.29275706135234003 ) ) ;
#123120=CARTESIAN_POINT ( 'NONE',  ( -13.89961937509977652, 13.97604488694528158, 105.6239096053143527 ) ) ;
#123121=CARTESIAN_POINT ( 'NONE',  ( -16.53943276465976808, 0.05219959533911058130, 76.24890960531435269 ) ) ;
#123122=CARTESIAN_POINT ( 'NONE',  ( -0.05219959533936034679, 19.03943276465977164, 37.50109039468567573 ) ) ;
#123123=CARTESIAN_POINT ( 'NONE',  ( 9.564922557960805705, 16.46253265017160317, 34.58224293864770260 ) ) ;
#123124=CARTESIAN_POINT ( 'NONE',  ( 18.62759615963271287, -10.81492255796078972, 33.33224293864769550 ) ) ;
#123125=CARTESIAN_POINT ( 'NONE',  ( -21.53943276465977519, 0.05219959533907696930, 71.24890960531435269 ) ) ;
#123126=ORIENTED_EDGE ( 'NONE', *, *, #111802, .F. ) ;
#123127=CARTESIAN_POINT ( 'NONE',  ( 14.29746914071049879, -8.314922557960816363, 103.3322429386476955 ) ) ;
#123128=CARTESIAN_POINT ( 'NONE',  ( -0.05219959533934338120, 16.53943276465976808, 47.50109039468568994 ) ) ;
#123129=CARTESIAN_POINT ( 'NONE',  ( -21.55341960407619339, 5.719274019375674811, 43.54275706135235424 ) ) ;
#123130=CARTESIAN_POINT ( 'NONE',  ( 16.52544592524342804, -4.483927247898539470, 98.54057627198105251 ) ) ;
#123133=CARTESIAN_POINT ( 'NONE',  ( -18.62759615963270932, 10.81492255796079327, 30.83224293864770260 ) ) ;
#123134=CARTESIAN_POINT ( 'NONE',  ( 17.26058549869091507, -6.457015423128606102, 66.12254162523933587 ) ) ;
#123136=CARTESIAN_POINT ( 'NONE',  ( -8.314922557961024197, 14.29746914071037800, 37.91775706135235424 ) ) ;
#123137=CARTESIAN_POINT ( 'NONE',  ( 8.224510206698953496, -14.34966873604960469, 27.91557627198103830 ) ) ;
#123138=CARTESIAN_POINT ( 'NONE',  ( -10.81492255796078084, -18.62759615963271287, 57.08224293864769550 ) ) ;
#123139=CARTESIAN_POINT ( 'NONE',  ( 19.05341960407617918, -5.049401038297876454, 81.04275706135231871 ) ) ;
#123140=CARTESIAN_POINT ( 'NONE',  ( 15.80617190586746368, 15.72974639402197994, 59.37390960531436690 ) ) ;
#123142=CARTESIAN_POINT ( 'NONE',  ( -4.379528057220086978, -16.55341960407618274, 49.79275706135234714 ) ) ;
#123143=CARTESIAN_POINT ( 'NONE',  ( -0.05219959533909027116, -19.03943276465977164, 32.49890960531435979 ) ) ;
#123144=CARTESIAN_POINT ( 'NONE',  ( -9.474510206698964154, 16.51473224551069663, 105.4155762719810383 ) ) ;
#123145=CARTESIAN_POINT ( 'NONE',  ( -9.564922557960796823, -16.46253265017161027, 42.08224293864769550 ) ) ;
#123146=CARTESIAN_POINT ( 'NONE',  ( -5.049401038298153566, 19.05341960407611168, 25.20724293864768484 ) ) ;
#123148=CARTESIAN_POINT ( 'NONE',  ( -13.97604488694527625, -13.89961937509977652, 111.8739096053143243 ) ) ;
#123150=CARTESIAN_POINT ( 'NONE',  ( 16.55341960407618274, -4.379528057220086978, 66.04275706135236135 ) ) ;
#123151=CARTESIAN_POINT ( 'NONE',  ( 15.72974639402199770, -15.80617190586745480, 88.12390960531436690 ) ) ;
#123152=CARTESIAN_POINT ( 'NONE',  ( -5.049401038298153566, 19.05341960407611168, 55.20724293864769550 ) ) ;
#123153=CARTESIAN_POINT ( 'NONE',  ( -10.81492255796105439, 18.62759615963255655, 22.91775706135235069 ) ) ;
#123154=CARTESIAN_POINT ( 'NONE',  ( -0.05219959533909027116, -19.03943276465977164, 82.49890960531436690 ) ) ;
#123156=ORIENTED_EDGE ( 'NONE', *, *, #131013, .T. ) ;
#123157=CARTESIAN_POINT ( 'NONE',  ( 0.05219959533907565091, 21.53943276465977519, 114.9989096053143669 ) ) ;
#123158=CARTESIAN_POINT ( 'NONE',  ( 12.14591786802309770, 12.06949235617756955, 114.3739096053143527 ) ) ;
#123159=CARTESIAN_POINT ( 'NONE',  ( -5.049401038298153566, 19.05341960407611168, 110.2072429386476671 ) ) ;
#123160=CARTESIAN_POINT ( 'NONE',  ( -5.153800228976607833, 19.02544592524334988, 72.70942372801900433 ) ) ;
#123161=CARTESIAN_POINT ( 'NONE',  ( 13.97604488694548053, -13.89961937509957401, 30.62609039468566863 ) ) ;
#123162=CARTESIAN_POINT ( 'NONE',  ( -0.05219959533907301413, -21.53943276465977519, 97.49890960531436690 ) ) ;
#123163=CARTESIAN_POINT ( 'NONE',  ( 5.049401038297881783, 19.05341960407617563, 37.29275706135232582 ) ) ;
#123164=CARTESIAN_POINT ( 'NONE',  ( -12.14591786802326823, 12.06949235617739902, 83.12609039468568994 ) ) ;
#123165=CARTESIAN_POINT ( 'NONE',  ( -19.05341960407611168, -5.049401038298163336, 106.4572429386476955 ) ) ;
#123166=CARTESIAN_POINT ( 'NONE',  ( 16.46253265017160672, -9.564922557960803928, 53.33224293864768839 ) ) ;
#123167=CARTESIAN_POINT ( 'NONE',  ( 21.55341960407619695, -5.719274019375665929, 61.04275706135234714 ) ) ;
#123168=CARTESIAN_POINT ( 'NONE',  ( -21.52544592524334988, -5.823673210054445271, 78.95942372801901854 ) ) ;
#123169=CARTESIAN_POINT ( 'NONE',  ( -18.09867054820433907, -5.499999999999827693, 53.98393025253585620 ) ) ;
#123170=CARTESIAN_POINT ( 'NONE',  ( -19.05341960407611168, -5.049401038298163336, 71.45724293864766707 ) ) ;
#123171=CARTESIAN_POINT ( 'NONE',  ( -5.719274019375665041, -21.55341960407619695, 44.79275706135234714 ) ) ;
#123172=CARTESIAN_POINT ( 'NONE',  ( -13.89961937509957401, -13.97604488694547875, 89.37609039468563310 ) ) ;
#123173=CARTESIAN_POINT ( 'NONE',  ( 9.564922557960805705, 16.46253265017160317, 54.58224293864769550 ) ) ;
#123174=CARTESIAN_POINT ( 'NONE',  ( 9.474510206698971260, -16.51473224551069308, 92.91557627198103830 ) ) ;
#123175=CARTESIAN_POINT ( 'NONE',  ( -5.049401038298153566, 19.05341960407611168, 60.20724293864768129 ) ) ;
#123176=CARTESIAN_POINT ( 'NONE',  ( -17.26058549869094350, -6.457015423128473763, 91.37745837476069255 ) ) ;
#123177=CARTESIAN_POINT ( 'NONE',  ( -13.89961937509977652, 13.97604488694528158, 55.62390960531434558 ) ) ;
#123178=CARTESIAN_POINT ( 'NONE',  ( 21.52544592524344225, -5.823673210054117533, 103.5405762719810383 ) ) ;
#123179=CARTESIAN_POINT ( 'NONE',  ( -0.05219959533934338120, 16.53943276465976808, 92.50109039468567573 ) ) ;
#123181=CARTESIAN_POINT ( 'NONE',  ( 16.51473224551083163, -9.474510206698727899, 50.83442372801899722 ) ) ;
#123182=CARTESIAN_POINT ( 'NONE',  ( -19.05341960407611168, -5.049401038298163336, 61.45724293864769550 ) ) ;
#123183=CARTESIAN_POINT ( 'NONE',  ( 16.55341960407611168, 4.379528057220329451, 58.95724293864770971 ) ) ;
#123184=CARTESIAN_POINT ( 'NONE',  ( -16.53943276465976808, 0.05219959533911058130, 91.24890960531436690 ) ) ;
#123185=CARTESIAN_POINT ( 'NONE',  ( 10.72451020669898902, -18.67979575497178502, 22.91557627198102765 ) ) ;
#123186=CARTESIAN_POINT ( 'NONE',  ( 13.89961937509977652, -13.97604488694527269, 98.12390960531433848 ) ) ;
#123187=CARTESIAN_POINT ( 'NONE',  ( 19.05341960407611168, 5.049401038298154454, 103.9572429386476671 ) ) ;
#123188=CARTESIAN_POINT ( 'NONE',  ( 0.05219959533936267826, -19.03943276465977164, 20.00109039468567218 ) ) ;
#123189=CARTESIAN_POINT ( 'NONE',  ( -16.53943276465976808, -0.05219959533934237506, 88.75109039468567573 ) ) ;
#123190=CARTESIAN_POINT ( 'NONE',  ( -13.97604488694527625, -13.89961937509977652, 71.87390960531433848 ) ) ;
#123191=CARTESIAN_POINT ( 'NONE',  ( -18.67979575497193778, 10.72451020669871902, 38.33442372801900433 ) ) ;
#123192=CARTESIAN_POINT ( 'NONE',  ( 5.719274019375991003, -21.55341960407610458, 27.70724293864769905 ) ) ;
#123193=CARTESIAN_POINT ( 'NONE',  ( 15.72974639402199770, -15.80617190586745480, 113.1239096053143953 ) ) ;
#123194=CARTESIAN_POINT ( 'NONE',  ( -5.823673210054116645, -21.52544592524344225, 72.29057627198102409 ) ) ;
#123195=CARTESIAN_POINT ( 'NONE',  ( 14.29746914071049879, -8.314922557960816363, 78.33224293864770971 ) ) ;
#123196=CARTESIAN_POINT ( 'NONE',  ( -0.05219959533936034679, 19.03943276465977164, 37.50109039468567573 ) ) ;
#123197=CARTESIAN_POINT ( 'NONE',  ( 8.314922557960818139, 14.29746914071049879, 114.5822429386477097 ) ) ;
#123198=CARTESIAN_POINT ( 'NONE',  ( -16.51473224551069308, -9.474510206698971260, 86.66557627198102409 ) ) ;
#123199=CARTESIAN_POINT ( 'NONE',  ( 19.02544592524343514, -5.153800228976328945, 78.54057627198099567 ) ) ;
#123201=CARTESIAN_POINT ( 'NONE',  ( 0.05219959533910956823, 16.53943276465976808, 94.99890960531436690 ) ) ;
#123202=ORIENTED_EDGE ( 'NONE', *, *, #48034, .F. ) ;
#123203=CARTESIAN_POINT ( 'NONE',  ( -14.29746914071037622, -8.314922557961029526, 109.1677570613523613 ) ) ;
#123204=CARTESIAN_POINT ( 'NONE',  ( 16.55341960407618274, -4.379528057220086978, 26.04275706135235779 ) ) ;
#123205=CARTESIAN_POINT ( 'NONE',  ( 10.72451020669871369, 18.67979575497193778, 87.08442372801901854 ) ) ;
#123206=CARTESIAN_POINT ( 'NONE',  ( -13.97604488694527625, -13.89961937509977652, 106.8739096053143669 ) ) ;
#123207=CARTESIAN_POINT ( 'NONE',  ( 21.52544592524334988, 5.823673210054432836, 21.45942372801901499 ) ) ;
#123208=CARTESIAN_POINT ( 'NONE',  ( 16.46253265017160672, -9.564922557960803928, 33.33224293864770260 ) ) ;
#123209=CARTESIAN_POINT ( 'NONE',  ( -14.29746914071037622, -8.314922557961029526, 34.16775706135234714 ) ) ;
#123210=CARTESIAN_POINT ( 'NONE',  ( -19.05341960407617563, 5.049401038297882671, 98.54275706135233293 ) ) ;
#123211=CARTESIAN_POINT ( 'NONE',  ( -21.53943276465977519, 0.05219959533907696930, 91.24890960531436690 ) ) ;
#123212=CARTESIAN_POINT ( 'NONE',  ( -19.03943276465977164, -0.05219959533935918106, 73.75109039468566152 ) ) ;
#123213=CARTESIAN_POINT ( 'NONE',  ( 9.474510206698971260, -16.51473224551069308, 22.91557627198102765 ) ) ;
#123214=CARTESIAN_POINT ( 'NONE',  ( -15.72974639402197994, 15.80617190586746368, 110.6239096053143669 ) ) ;
#123216=CARTESIAN_POINT ( 'NONE',  ( 13.97604488694527802, 13.89961937509977652, 89.37390960531436690 ) ) ;
#123218=CARTESIAN_POINT ( 'NONE',  ( -5.153800228976328057, -19.02544592524343514, 82.29057627198103830 ) ) ;
#123219=CARTESIAN_POINT ( 'NONE',  ( -5.719274019375665041, -21.55341960407619695, 19.79275706135235069 ) ) ;
#123220=CARTESIAN_POINT ( 'NONE',  ( -16.53943276465976808, 0.05219959533911058130, 81.24890960531436690 ) ) ;
#123221=CARTESIAN_POINT ( 'NONE',  ( 5.049401038298161559, -19.05341960407611168, 82.70724293864770971 ) ) ;
#123222=CARTESIAN_POINT ( 'NONE',  ( 4.379528057220092307, 16.55341960407617563, 52.29275706135236135 ) ) ;
#123223=CARTESIAN_POINT ( 'NONE',  ( -16.51473224551082808, 9.474510206698731452, 53.33442372801900433 ) ) ;
#123224=CARTESIAN_POINT ( 'NONE',  ( 15.72974639402176855, 15.80617190586768217, 61.87609039468568284 ) ) ;
#123225=CARTESIAN_POINT ( 'NONE',  ( 8.224510206698742110, 14.34966873604972548, 22.08442372801901143 ) ) ;
#123226=CARTESIAN_POINT ( 'NONE',  ( 5.153800228976335163, 19.02544592524342804, 74.79057627198103830 ) ) ;
#123227=CARTESIAN_POINT ( 'NONE',  ( -5.049401038297874678, -19.05341960407617918, 89.79275706135230450 ) ) ;
#123228=CARTESIAN_POINT ( 'NONE',  ( 0.05219959533934541429, -16.53943276465976808, 50.00109039468568994 ) ) ;
#123229=CARTESIAN_POINT ( 'NONE',  ( 21.52544592524334988, 5.823673210054432836, 91.45942372801901854 ) ) ;
#123230=CARTESIAN_POINT ( 'NONE',  ( 16.51473224551083163, -9.474510206698727899, 75.83442372801900433 ) ) ;
#123231=CARTESIAN_POINT ( 'NONE',  ( -19.05341960407611168, -5.049401038298163336, 46.45724293864768129 ) ) ;
#123232=CARTESIAN_POINT ( 'NONE',  ( 21.53943276465977519, -0.05219959533907433946, 73.74890960531433848 ) ) ;
#123233=CARTESIAN_POINT ( 'NONE',  ( -14.34966873604960291, -8.224510206698953496, 71.66557627198100988 ) ) ;
#123234=CARTESIAN_POINT ( 'NONE',  ( -13.97604488694547697, 13.89961937509957934, 83.12609039468564731 ) ) ;
#123236=CARTESIAN_POINT ( 'NONE',  ( 9.474510206698729675, 16.51473224551082808, 42.08442372801900433 ) ) ;
#123237=CARTESIAN_POINT ( 'NONE',  ( -8.314922557960811034, -14.29746914071050412, 22.08224293864769194 ) ) ;
#123238=CARTESIAN_POINT ( 'NONE',  ( 12.14591786802309770, 12.06949235617756955, 69.37390960531436690 ) ) ;
#123239=CARTESIAN_POINT ( 'NONE',  ( -18.67979575497193778, 10.72451020669871902, 108.3344237280190185 ) ) ;
#123241=CARTESIAN_POINT ( 'NONE',  ( -10.81492255796078084, -18.62759615963271287, 107.0822429386476955 ) ) ;
#123242=CARTESIAN_POINT ( 'NONE',  ( 19.03943276465977164, -0.05219959533909143690, 63.74890960531435979 ) ) ;
#123243=CARTESIAN_POINT ( 'NONE',  ( 18.67979575497194134, -10.72451020669871369, 80.83442372801901854 ) ) ;
#123244=CARTESIAN_POINT ( 'NONE',  ( 19.05341960407611168, 5.049401038298154454, 58.95724293864768129 ) ) ;
#123245=ORIENTED_EDGE ( 'NONE', *, *, #53412, .F. ) ;
#123246=CARTESIAN_POINT ( 'NONE',  ( -13.89961937509977652, 13.97604488694528158, 25.62390960531434558 ) ) ;
#123247=CARTESIAN_POINT ( 'NONE',  ( -5.153800228976328057, -19.02544592524343514, 112.2905762719810099 ) ) ;
#123248=CARTESIAN_POINT ( 'NONE',  ( 4.379528057220339221, -16.55341960407611168, 67.70724293864769550 ) ) ;
#123249=CARTESIAN_POINT ( 'NONE',  ( 5.153800228976335163, 19.02544592524342804, 24.79057627198102765 ) ) ;
#123250=CARTESIAN_POINT ( 'NONE',  ( -4.379528057220328563, 16.55341960407611168, 80.20724293864769550 ) ) ;
#123251=CARTESIAN_POINT ( 'NONE',  ( -18.67979575497178146, -10.72451020669898902, 96.66557627198102409 ) ) ;
#123252=CARTESIAN_POINT ( 'NONE',  ( -21.52544592524334988, -5.823673210054445271, 43.95942372801902565 ) ) ;
#123254=CARTESIAN_POINT ( 'NONE',  ( 14.29746914071037800, 8.314922557961029526, 56.66775706135235424 ) ) ;
#123255=CARTESIAN_POINT ( 'NONE',  ( 0.05219959533907565091, 21.53943276465977519, 94.99890960531436690 ) ) ;
#123256=CARTESIAN_POINT ( 'NONE',  ( -9.564922557961040184, 16.46253265017147172, 22.91775706135233648 ) ) ;
#123257=CARTESIAN_POINT ( 'NONE',  ( -16.46253265017160317, 9.564922557960807481, 100.8322429386477097 ) ) ;
#123258=CARTESIAN_POINT ( 'NONE',  ( 21.52544592524334988, 5.823673210054432836, 41.45942372801901143 ) ) ;
#123259=CARTESIAN_POINT ( 'NONE',  ( 18.62759615963271287, -10.81492255796078972, 38.33224293864768839 ) ) ;
#123260=CARTESIAN_POINT ( 'NONE',  ( -16.55341960407611168, -4.379528057220339221, 26.45724293864768839 ) ) ;
#123262=CARTESIAN_POINT ( 'NONE',  ( -15.72974639402176322, -15.80617190586768395, 64.37609039468568994 ) ) ;
#123263=CARTESIAN_POINT ( 'NONE',  ( 21.52544592524334988, 5.823673210054432836, 91.45942372801901854 ) ) ;
#123264=CARTESIAN_POINT ( 'NONE',  ( -16.51473224551082808, 9.474510206698731452, 28.33442372801900433 ) ) ;
#123265=CARTESIAN_POINT ( 'NONE',  ( -4.483927247898782831, 16.52544592524335698, 87.70942372801901854 ) ) ;
#123266=CARTESIAN_POINT ( 'NONE',  ( 21.52544592524334988, 5.823673210054432836, 56.45942372801902565 ) ) ;
#123267=CARTESIAN_POINT ( 'NONE',  ( 5.049401038298161559, -19.05341960407611168, 42.70724293864767418 ) ) ;
#123268=CARTESIAN_POINT ( 'NONE',  ( 9.474510206698729675, 16.51473224551082808, 27.08442372801900433 ) ) ;
#123269=CARTESIAN_POINT ( 'NONE',  ( -21.52544592524343514, 5.823673210054127303, 31.04057627198102409 ) ) ;
#123270=CARTESIAN_POINT ( 'NONE',  ( -10.72451020669870658, -18.67979575497194134, 19.58442372801901143 ) ) ;
#123271=CARTESIAN_POINT ( 'NONE',  ( 15.72974639402199770, -15.80617190586745480, 73.12390960531436690 ) ) ;
#123272=CARTESIAN_POINT ( 'NONE',  ( 8.224510206698742110, 14.34966873604972548, 37.08442372801901143 ) ) ;
#123274=CARTESIAN_POINT ( 'NONE',  ( -15.80617190586745835, -15.72974639402198527, 86.87390960531438111 ) ) ;
#123275=CARTESIAN_POINT ( 'NONE',  ( -0.05219959533934338120, 16.53943276465976808, 62.50109039468568284 ) ) ;
#123276=CARTESIAN_POINT ( 'NONE',  ( -0.05219959533910754901, -16.53943276465976808, 57.49890960531435979 ) ) ;
#123278=CARTESIAN_POINT ( 'NONE',  ( -13.89961937509957401, -13.97604488694547875, 99.37609039468567573 ) ) ;
#123279=CARTESIAN_POINT ( 'NONE',  ( 21.52544592524344225, -5.823673210054117533, 33.54057627198102409 ) ) ;
#123281=CARTESIAN_POINT ( 'NONE',  ( -8.224510206698735004, -14.34966873604973081, 44.58442372801901854 ) ) ;
#123282=CARTESIAN_POINT ( 'NONE',  ( 21.52544592524344225, -5.823673210054117533, 108.5405762719810241 ) ) ;
#123283=CARTESIAN_POINT ( 'NONE',  ( 5.719274019375991003, -21.55341960407610458, 27.70724293864769905 ) ) ;
#123284=CARTESIAN_POINT ( 'NONE',  ( 8.314922557961029526, -14.29746914071037800, 60.41775706135235424 ) ) ;
#123285=CARTESIAN_POINT ( 'NONE',  ( -9.474510206698964154, 16.51473224551069663, 85.41557627198102409 ) ) ;
#123286=CARTESIAN_POINT ( 'NONE',  ( 18.62759615963255655, 10.81492255796105972, 36.66775706135234714 ) ) ;
#123287=CARTESIAN_POINT ( 'NONE',  ( 19.02544592524334988, 5.153800228976608722, 111.4594237280190043 ) ) ;
#123288=CARTESIAN_POINT ( 'NONE',  ( 10.72451020669898902, -18.67979575497178502, 32.91557627198102409 ) ) ;
#123290=CARTESIAN_POINT ( 'NONE',  ( 19.03943276465977164, 0.05219959533936151252, 26.25109039468566507 ) ) ;
#123291=CARTESIAN_POINT ( 'NONE',  ( 4.483927247898790824, -16.52544592524335698, 45.20942372801901854 ) ) ;
#123292=CARTESIAN_POINT ( 'NONE',  ( 5.049401038298161559, -19.05341960407611168, 102.7072429386476955 ) ) ;
#123293=CARTESIAN_POINT ( 'NONE',  ( -0.05219959533907301413, -21.53943276465977519, 107.4989096053143669 ) ) ;
#123294=CARTESIAN_POINT ( 'NONE',  ( 9.564922557960805705, 16.46253265017160317, 74.58224293864769550 ) ) ;
#123295=CARTESIAN_POINT ( 'NONE',  ( -16.52216118717207749, 7.221426719304501418, 23.92400978953008917 ) ) ;
#123296=CARTESIAN_POINT ( 'NONE',  ( -0.05219959533910754901, -16.53943276465976808, 82.49890960531436690 ) ) ;
#123297=CARTESIAN_POINT ( 'NONE',  ( -15.72974639402197994, 15.80617190586746368, 35.62390960531437401 ) ) ;
#123298=CARTESIAN_POINT ( 'NONE',  ( -17.50000000000000000, 5.622605283950870891, 33.68792689403888119 ) ) ;
#123299=CARTESIAN_POINT ( 'NONE',  ( 4.379528057220092307, 16.55341960407617563, 62.29275706135236845 ) ) ;
#123300=CARTESIAN_POINT ( 'NONE',  ( 21.53943276465977519, -0.05219959533907433946, 98.74890960531438111 ) ) ;
#123301=CARTESIAN_POINT ( 'NONE',  ( -13.97604488694547697, 13.89961937509957934, 78.12609039468567573 ) ) ;
#123302=CARTESIAN_POINT ( 'NONE',  ( -13.97604488694527625, -13.89961937509977652, 31.87390960531435979 ) ) ;
#123303=CARTESIAN_POINT ( 'NONE',  ( -5.823673210054116645, -21.52544592524344225, 72.29057627198102409 ) ) ;
#123304=CARTESIAN_POINT ( 'NONE',  ( 5.153800228976335163, 19.02544592524342804, 94.79057627198103830 ) ) ;
#123305=CARTESIAN_POINT ( 'NONE',  ( 10.72451020669871369, 18.67979575497193778, 87.08442372801901854 ) ) ;
#123306=CARTESIAN_POINT ( 'NONE',  ( 5.049401038298161559, -19.05341960407611168, 62.70724293864769550 ) ) ;
#123307=CARTESIAN_POINT ( 'NONE',  ( -12.14591786802326823, 12.06949235617739902, 43.12609039468568284 ) ) ;
#123308=CARTESIAN_POINT ( 'NONE',  ( -9.474510206698964154, 16.51473224551069663, 55.41557627198103120 ) ) ;
#123309=CARTESIAN_POINT ( 'NONE',  ( -18.62759615963255300, -10.81492255796106328, 79.16775706135234714 ) ) ;
#123311=CARTESIAN_POINT ( 'NONE',  ( -0.05219959533936034679, 19.03943276465977164, 32.50109039468566863 ) ) ;
#123312=CARTESIAN_POINT ( 'NONE',  ( -9.474510206698720793, -16.51473224551083518, 39.58442372801899722 ) ) ;
#123313=CARTESIAN_POINT ( 'NONE',  ( -10.81492255796105439, 18.62759615963255655, 47.91775706135234714 ) ) ;
#123315=CARTESIAN_POINT ( 'NONE',  ( 0.05219959533936267826, -19.03943276465977164, 50.00109039468566863 ) ) ;
#123316=CARTESIAN_POINT ( 'NONE',  ( -19.05341960407611168, -5.049401038298163336, 86.45724293864769550 ) ) ;
#123317=CARTESIAN_POINT ( 'NONE',  ( 13.97604488694527802, 13.89961937509977652, 64.37390960531436690 ) ) ;
#123318=CARTESIAN_POINT ( 'NONE',  ( -8.314922557961024197, 14.29746914071037800, 112.9177570613523329 ) ) ;
#123319=CARTESIAN_POINT ( 'NONE',  ( -15.72974639402197994, 15.80617190586746368, 25.62390960531435624 ) ) ;
#123320=CARTESIAN_POINT ( 'NONE',  ( 5.823673210054444382, -21.52544592524334988, 90.20942372801903275 ) ) ;
#123323=CARTESIAN_POINT ( 'NONE',  ( -21.52544592524334988, -5.823673210054445271, 98.95942372801903275 ) ) ;
#123325=CARTESIAN_POINT ( 'NONE',  ( 0.05219959533909260263, 19.03943276465977164, 29.99890960531435979 ) ) ;
#123326=CARTESIAN_POINT ( 'NONE',  ( -19.02544592524342804, 5.153800228976336051, 111.0405762719810099 ) ) ;
#123328=CARTESIAN_POINT ( 'NONE',  ( 4.483927247898790824, -16.52544592524335698, 55.20942372801902565 ) ) ;
#123329=CARTESIAN_POINT ( 'NONE',  ( 18.67979575497178502, 10.72451020669898547, 64.16557627198102409 ) ) ;
#123331=CARTESIAN_POINT ( 'NONE',  ( -8.314922557960811034, -14.29746914071050412, 37.08224293864768129 ) ) ;
#123332=CARTESIAN_POINT ( 'NONE',  ( 8.314922557960818139, 14.29746914071049879, 104.5822429386477097 ) ) ;
#123333=CARTESIAN_POINT ( 'NONE',  ( 19.03943276465977164, -0.05219959533909143690, 98.74890960531436690 ) ) ;
#123334=CARTESIAN_POINT ( 'NONE',  ( 21.53943276465977519, 0.05219959533937863772, 111.2510903946856899 ) ) ;
#123335=CARTESIAN_POINT ( 'NONE',  ( 12.06949235617757843, -12.14591786802309237, 113.1239096053143953 ) ) ;
#123336=CARTESIAN_POINT ( 'NONE',  ( 0.05219959533937995610, -21.53943276465977519, 70.00109039468568994 ) ) ;
#123337=CARTESIAN_POINT ( 'NONE',  ( -13.89961937509977652, 13.97604488694528158, 115.6239096053143669 ) ) ;
#123338=CARTESIAN_POINT ( 'NONE',  ( -12.14591786802326823, 12.06949235617739902, 103.1260903946856757 ) ) ;
#123339=CARTESIAN_POINT ( 'NONE',  ( -19.02544592524334988, -5.153800228976617603, 58.95942372801900433 ) ) ;
#123341=CARTESIAN_POINT ( 'NONE',  ( -15.80617190586745835, -15.72974639402198527, 26.87390960531435979 ) ) ;
#123342=CARTESIAN_POINT ( 'NONE',  ( 8.224510206698953496, -14.34966873604960469, 87.91557627198103830 ) ) ;
#123343=CARTESIAN_POINT ( 'NONE',  ( -19.05341960407617563, 5.049401038297882671, 53.54275706135231871 ) ) ;
#123344=CARTESIAN_POINT ( 'NONE',  ( -16.46253265017160317, 9.564922557960807481, 80.83224293864769550 ) ) ;
#123345=CARTESIAN_POINT ( 'NONE',  ( 4.483927247898545687, 16.52544592524342804, 69.79057627198102409 ) ) ;
#123346=CARTESIAN_POINT ( 'NONE',  ( -19.05341960407617563, 5.049401038297882671, 93.54275706135234714 ) ) ;
#123347=CARTESIAN_POINT ( 'NONE',  ( 21.52544592524344225, -5.823673210054117533, 43.54057627198103830 ) ) ;
#123348=VERTEX_POINT ( 'NONE', #124566 ) ;
#123349=CARTESIAN_POINT ( 'NONE',  ( 14.34966873604960469, 8.224510206698951720, 114.1655762719810383 ) ) ;
#123350=CARTESIAN_POINT ( 'NONE',  ( -17.31728774477272381, -6.344390552232408886, 29.18093348310683410 ) ) ;
#123351=CARTESIAN_POINT ( 'NONE',  ( 16.46253265017160672, -9.564922557960803928, 73.33224293864769550 ) ) ;
#123352=CARTESIAN_POINT ( 'NONE',  ( 18.62759615963271287, -10.81492255796078972, 78.33224293864770971 ) ) ;
#123353=CARTESIAN_POINT ( 'NONE',  ( 4.483927247898790824, -16.52544592524335698, 95.20942372801903275 ) ) ;
#123354=CARTESIAN_POINT ( 'NONE',  ( -19.03943276465977164, 0.05219959533909376836, 71.24890960531435269 ) ) ;
#123355=CARTESIAN_POINT ( 'NONE',  ( 13.89961937509957401, 13.97604488694547697, 71.87609039468567573 ) ) ;
#123356=CARTESIAN_POINT ( 'NONE',  ( -0.05219959533937732626, 21.53943276465977519, 77.50109039468567573 ) ) ;
#123357=CARTESIAN_POINT ( 'NONE',  ( -10.81492255796078084, -18.62759615963271287, 62.08224293864769550 ) ) ;
#123358=CARTESIAN_POINT ( 'NONE',  ( 21.52544592524344225, -5.823673210054117533, 28.54057627198103120 ) ) ;
#123359=CARTESIAN_POINT ( 'NONE',  ( 13.89961937509977652, -13.97604488694527269, 43.12390960531434558 ) ) ;
#123360=CARTESIAN_POINT ( 'NONE',  ( -4.483927247898782831, 16.52544592524335698, 102.7094237280190185 ) ) ;
#123361=CARTESIAN_POINT ( 'NONE',  ( -19.05341960407611168, -5.049401038298163336, 51.45724293864770260 ) ) ;
#123362=CARTESIAN_POINT ( 'NONE',  ( -8.314922557961024197, 14.29746914071037800, 27.91775706135234358 ) ) ;
#123363=CARTESIAN_POINT ( 'NONE',  ( 18.22780087662122384, -5.500000000000022204, 101.0154010532610869 ) ) ;
#123364=CARTESIAN_POINT ( 'NONE',  ( -9.474510206698720793, -16.51473224551083518, 19.58442372801899722 ) ) ;
#123365=CARTESIAN_POINT ( 'NONE',  ( -16.52544592524342804, 4.483927247898546575, 56.04057627198102409 ) ) ;
#123366=CARTESIAN_POINT ( 'NONE',  ( -5.823673210054116645, -21.52544592524344225, 102.2905762719810383 ) ) ;
#123367=CARTESIAN_POINT ( 'NONE',  ( 21.52544592524344225, -5.823673210054117533, 98.54057627198105251 ) ) ;
#123369=CARTESIAN_POINT ( 'NONE',  ( -18.62759615963270932, 10.81492255796079327, 45.83224293864769550 ) ) ;
#123370=CARTESIAN_POINT ( 'NONE',  ( 16.52544592524335698, 4.483927247898782831, 86.45942372801901854 ) ) ;
#123371=CARTESIAN_POINT ( 'NONE',  ( 12.06949235617757843, -12.14591786802309237, 93.12390960531436690 ) ) ;
#123372=CARTESIAN_POINT ( 'NONE',  ( -19.03943276465977164, 0.05219959533909376836, 61.24890960531436690 ) ) ;
#123375=CARTESIAN_POINT ( 'NONE',  ( 8.314922557961029526, -14.29746914071037800, 105.4177570613523613 ) ) ;
#123376=CARTESIAN_POINT ( 'NONE',  ( -0.05219959533937732626, 21.53943276465977519, 32.50109039468568284 ) ) ;
#123377=CARTESIAN_POINT ( 'NONE',  ( 0.05219959533909260263, 19.03943276465977164, 94.99890960531436690 ) ) ;
#123378=CARTESIAN_POINT ( 'NONE',  ( 10.81492255796106328, -18.62759615963255655, 70.41775706135236135 ) ) ;
#123380=CARTESIAN_POINT ( 'NONE',  ( -19.02544592524342804, 5.153800228976336051, 26.04057627198103120 ) ) ;
#123381=VERTEX_POINT ( 'NONE', #122572 ) ;
#123382=CARTESIAN_POINT ( 'NONE',  ( -5.719274019375665041, -21.55341960407619695, 64.79275706135234714 ) ) ;
#123383=CARTESIAN_POINT ( 'NONE',  ( -5.153800228976328057, -19.02544592524343514, 47.29057627198102409 ) ) ;
#123384=CARTESIAN_POINT ( 'NONE',  ( 19.02544592524343514, -5.153800228976328945, 93.54057627198102409 ) ) ;
#123385=CARTESIAN_POINT ( 'NONE',  ( -19.05341960407617563, 5.049401038297882671, 73.54275706135233293 ) ) ;
#123386=CARTESIAN_POINT ( 'NONE',  ( 0.05219959533937995610, -21.53943276465977519, 40.00109039468567573 ) ) ;
#123387=CARTESIAN_POINT ( 'NONE',  ( 0.05219959533936267826, -19.03943276465977164, 100.0010903946856757 ) ) ;
#123388=CARTESIAN_POINT ( 'NONE',  ( -0.05219959533936034679, 19.03943276465977164, 77.50109039468566152 ) ) ;
#123389=CARTESIAN_POINT ( 'NONE',  ( -16.46253265017160317, 9.564922557960807481, 40.83224293864769550 ) ) ;
#123390=CARTESIAN_POINT ( 'NONE',  ( -5.153800228976607833, 19.02544592524334988, 82.70942372801897591 ) ) ;
#123391=CARTESIAN_POINT ( 'NONE',  ( -4.379528057220086978, -16.55341960407618274, 109.7927570613523613 ) ) ;
#123392=CARTESIAN_POINT ( 'NONE',  ( -13.89961937509957401, -13.97604488694547875, 79.37609039468567573 ) ) ;
#123393=CARTESIAN_POINT ( 'NONE',  ( -0.05219959533910754901, -16.53943276465976808, 27.49890960531435269 ) ) ;
#123394=CARTESIAN_POINT ( 'NONE',  ( -13.97604488694547697, 13.89961937509957934, 53.12609039468565442 ) ) ;
#123395=CARTESIAN_POINT ( 'NONE',  ( 5.719274019375673035, 21.55341960407619339, 102.2927570613523613 ) ) ;
#123396=CARTESIAN_POINT ( 'NONE',  ( -19.02544592524334988, -5.153800228976617603, 28.95942372801900433 ) ) ;
#123397=CARTESIAN_POINT ( 'NONE',  ( -0.05219959533909027116, -19.03943276465977164, 27.49890960531435624 ) ) ;
#123398=CARTESIAN_POINT ( 'NONE',  ( -10.72451020669870658, -18.67979575497194134, 89.58442372801901854 ) ) ;
#123399=CARTESIAN_POINT ( 'NONE',  ( -14.29746914071037622, -8.314922557961029526, 29.16775706135234003 ) ) ;
#123400=CARTESIAN_POINT ( 'NONE',  ( 16.51473224551069308, 9.474510206698969483, 89.16557627198103830 ) ) ;
#123402=CARTESIAN_POINT ( 'NONE',  ( -19.03943276465977164, 0.05219959533909376836, 76.24890960531435269 ) ) ;
#123404=CARTESIAN_POINT ( 'NONE',  ( 5.153800228976615827, -19.02544592524334988, 80.20942372801901854 ) ) ;
#123405=CARTESIAN_POINT ( 'NONE',  ( 21.53943276465977519, -0.05219959533907433946, 23.74890960531435269 ) ) ;
#123406=CARTESIAN_POINT ( 'NONE',  ( -5.823673210054431948, 21.52544592524334988, 112.7094237280190328 ) ) ;
#123407=CARTESIAN_POINT ( 'NONE',  ( -5.049401038297874678, -19.05341960407617918, 99.79275706135234714 ) ) ;
#123408=CARTESIAN_POINT ( 'NONE',  ( 12.06949235617757843, -12.14591786802309237, 103.1239096053143811 ) ) ;
#123409=CARTESIAN_POINT ( 'NONE',  ( -5.049401038298153566, 19.05341960407611168, 30.20724293864768839 ) ) ;
#123410=CARTESIAN_POINT ( 'NONE',  ( 10.72451020669898902, -18.67979575497178502, 62.91557627198102409 ) ) ;
#123411=CARTESIAN_POINT ( 'NONE',  ( -15.80617190586745835, -15.72974639402198527, 46.87390960531435979 ) ) ;
#123412=CARTESIAN_POINT ( 'NONE',  ( 8.314922557960818139, 14.29746914071049879, 114.5822429386477097 ) ) ;
#123414=CARTESIAN_POINT ( 'NONE',  ( -19.05341960407617563, 5.049401038297882671, 63.54275706135234003 ) ) ;
#123415=CARTESIAN_POINT ( 'NONE',  ( -16.52544592524342804, 4.483927247898546575, 36.04057627198102409 ) ) ;
#123416=CARTESIAN_POINT ( 'NONE',  ( -9.564922557960796823, -16.46253265017161027, 112.0822429386476955 ) ) ;
#123417=CARTESIAN_POINT ( 'NONE',  ( -5.823673210054431948, 21.52544592524334988, 82.70942372801900433 ) ) ;
#123418=CARTESIAN_POINT ( 'NONE',  ( 0.05219959533907565091, 21.53943276465977519, 64.99890960531435269 ) ) ;
#123419=CARTESIAN_POINT ( 'NONE',  ( -10.81492255796105439, 18.62759615963255655, 57.91775706135234714 ) ) ;
#123420=CARTESIAN_POINT ( 'NONE',  ( -5.719274019375665041, -21.55341960407619695, 44.79275706135234714 ) ) ;
#123421=CARTESIAN_POINT ( 'NONE',  ( -9.564922557960796823, -16.46253265017161027, 82.08224293864768129 ) ) ;
#123422=CARTESIAN_POINT ( 'NONE',  ( -16.53943276465976808, -0.05219959533934237506, 98.75109039468568994 ) ) ;
#123423=CARTESIAN_POINT ( 'NONE',  ( 16.51473224551069308, 9.474510206698969483, 24.16557627198102765 ) ) ;
#123425=CARTESIAN_POINT ( 'NONE',  ( 4.379528057220339221, -16.55341960407611168, 72.70724293864769550 ) ) ;
#123426=CARTESIAN_POINT ( 'NONE',  ( 8.314922557960818139, 14.29746914071049879, 34.58224293864770260 ) ) ;
#123427=CARTESIAN_POINT ( 'NONE',  ( -5.049401038298153566, 19.05341960407611168, 60.20724293864768129 ) ) ;
#123428=CARTESIAN_POINT ( 'NONE',  ( 13.97604488694527802, 13.89961937509977652, 29.37390960531435979 ) ) ;
#123429=CARTESIAN_POINT ( 'NONE',  ( -18.62759615963270932, 10.81492255796079327, 50.83224293864770971 ) ) ;
#123430=CARTESIAN_POINT ( 'NONE',  ( 16.46253265017146816, 9.564922557961045513, 36.66775706135233293 ) ) ;
#123432=CARTESIAN_POINT ( 'NONE',  ( -12.06949235617756955, 12.14591786802309770, 45.62390960531436690 ) ) ;
#123433=CARTESIAN_POINT ( 'NONE',  ( -21.52544592524343514, 5.823673210054127303, 26.04057627198103475 ) ) ;
#123435=CARTESIAN_POINT ( 'NONE',  ( 16.52544592524335698, 4.483927247898782831, 71.45942372801901854 ) ) ;
#123436=CARTESIAN_POINT ( 'NONE',  ( -19.05341960407617563, 5.049401038297882671, 78.54275706135233293 ) ) ;
#123437=CARTESIAN_POINT ( 'NONE',  ( 8.224510206698953496, -14.34966873604960469, 47.91557627198102409 ) ) ;
#123438=ORIENTED_EDGE ( 'NONE', *, *, #95827, .T. ) ;
#123439=CARTESIAN_POINT ( 'NONE',  ( -18.56101223717332260, -5.500000000000062172, 76.44978406935678095 ) ) ;
#123440=CARTESIAN_POINT ( 'NONE',  ( -16.55341960407611168, -4.379528057220339221, 31.45724293864769550 ) ) ;
#123441=CARTESIAN_POINT ( 'NONE',  ( -9.564922557960796823, -16.46253265017161027, 52.08224293864768839 ) ) ;
#123442=CARTESIAN_POINT ( 'NONE',  ( -19.05341960407611168, -5.049401038298163336, 81.45724293864769550 ) ) ;
#123443=CARTESIAN_POINT ( 'NONE',  ( 5.153800228976335163, 19.02544592524342804, 44.79057627198103830 ) ) ;
#123444=CARTESIAN_POINT ( 'NONE',  ( 15.80617190586769283, -15.72974639402175789, 40.62609039468567573 ) ) ;
#123445=CARTESIAN_POINT ( 'NONE',  ( 9.474510206698971260, -16.51473224551069308, 62.91557627198102409 ) ) ;
#123447=CARTESIAN_POINT ( 'NONE',  ( 9.474510206698971260, -16.51473224551069308, 42.91557627198103120 ) ) ;
#123448=CARTESIAN_POINT ( 'NONE',  ( -18.67979575497178146, -10.72451020669898902, 31.66557627198102054 ) ) ;
#123449=B_SPLINE_CURVE_WITH_KNOTS ( 'NONE', 3,
 ( #94136, #122489, #91142, #61803, #184180, #109311 ),
 .UNSPECIFIED., .F., .F.,
 ( 4, 2, 4 ),
 ( 0.000000000000000000, 0.0003837532665634991623, 0.0007675065331269983245 ),
 .UNSPECIFIED. ) ;
#123450=CARTESIAN_POINT ( 'NONE',  ( 10.72451020669871369, 18.67979575497193778, 77.08442372801901854 ) ) ;
#123451=CARTESIAN_POINT ( 'NONE',  ( 19.03943276465977164, -0.05219959533909143690, 23.74890960531435269 ) ) ;
#123452=CARTESIAN_POINT ( 'NONE',  ( 18.62759615963271287, -10.81492255796078972, 23.33224293864769194 ) ) ;
#123453=CARTESIAN_POINT ( 'NONE',  ( 14.29746914071037800, 8.314922557961029526, 96.66775706135234714 ) ) ;
#123455=CARTESIAN_POINT ( 'NONE',  ( 10.72451020669871369, 18.67979575497193778, 107.0844237280190043 ) ) ;
#123456=CARTESIAN_POINT ( 'NONE',  ( -12.06949235617739369, -12.14591786802326823, 64.37609039468568994 ) ) ;
#123457=CARTESIAN_POINT ( 'NONE',  ( -13.89961937509977652, 13.97604488694528158, 105.6239096053143527 ) ) ;
#123458=CARTESIAN_POINT ( 'NONE',  ( 0.05219959533934541429, -16.53943276465976808, 60.00109039468568284 ) ) ;
#123459=CARTESIAN_POINT ( 'NONE',  ( 14.29746914071037800, 8.314922557961029526, 41.66775706135235424 ) ) ;
#123460=CARTESIAN_POINT ( 'NONE',  ( 14.29746914071037800, 8.314922557961029526, 91.66775706135234714 ) ) ;
#123461=CARTESIAN_POINT ( 'NONE',  ( -18.67979575497193778, 10.72451020669871902, 48.33442372801902565 ) ) ;
#123462=CARTESIAN_POINT ( 'NONE',  ( 12.06949235617739724, 12.14591786802326823, 26.87609039468567218 ) ) ;
#123463=CARTESIAN_POINT ( 'NONE',  ( -10.72451020669898014, 18.67979575497178502, 115.4155762719810241 ) ) ;
#123464=CARTESIAN_POINT ( 'NONE',  ( 8.224510206698742110, 14.34966873604972548, 22.08442372801901143 ) ) ;
#123465=CARTESIAN_POINT ( 'NONE',  ( 12.06949235617739724, 12.14591786802326823, 81.87609039468568994 ) ) ;
#123467=CARTESIAN_POINT ( 'NONE',  ( 18.62759615963255655, 10.81492255796105972, 81.66775706135236135 ) ) ;
#123468=CARTESIAN_POINT ( 'NONE',  ( 0.05219959533936267826, -19.03943276465977164, 85.00109039468567573 ) ) ;
#123469=CARTESIAN_POINT ( 'NONE',  ( -12.06949235617756955, 12.14591786802309770, 55.62390960531436690 ) ) ;
#123470=CARTESIAN_POINT ( 'NONE',  ( 16.53943276465976808, -0.05219959533910856209, 38.74890960531435979 ) ) ;
#123471=CARTESIAN_POINT ( 'NONE',  ( -14.34966873604960291, -8.224510206698953496, 111.6655762719810525 ) ) ;
#123472=CARTESIAN_POINT ( 'NONE',  ( 0.05219959533936267826, -19.03943276465977164, 50.00109039468566863 ) ) ;
#123474=CARTESIAN_POINT ( 'NONE',  ( -10.72451020669870658, -18.67979575497194134, 44.58442372801901854 ) ) ;
#123475=CARTESIAN_POINT ( 'NONE',  ( -19.05341960407617563, 5.049401038297882671, 113.5427570613523471 ) ) ;
#123476=FACE_OUTER_BOUND ( 'NONE', #186231, .T. ) ;
#123477=CARTESIAN_POINT ( 'NONE',  ( -19.02544592524342804, 5.153800228976336051, 111.0405762719810099 ) ) ;
#123478=CARTESIAN_POINT ( 'NONE',  ( 18.67979575497178502, 10.72451020669898547, 69.16557627198102409 ) ) ;
#123479=CARTESIAN_POINT ( 'NONE',  ( 5.153800228976615827, -19.02544592524334988, 100.2094237280190043 ) ) ;
#123480=CARTESIAN_POINT ( 'NONE',  ( 9.474510206698971260, -16.51473224551069308, 102.9155762719810241 ) ) ;
#123481=CARTESIAN_POINT ( 'NONE',  ( -17.58332526062528345, -7.635886036038592728, 49.07665040441535353 ) ) ;
#123482=CARTESIAN_POINT ( 'NONE',  ( -16.55341960407611168, -4.379528057220339221, 106.4572429386477097 ) ) ;
#123483=CARTESIAN_POINT ( 'NONE',  ( 5.719274019375673035, 21.55341960407619339, 92.29275706135236135 ) ) ;
#123484=CARTESIAN_POINT ( 'NONE',  ( 13.89961937509977652, -13.97604488694527269, 33.12390960531434558 ) ) ;
#123485=CARTESIAN_POINT ( 'NONE',  ( -15.80617190586768217, 15.72974639402176855, 38.12609039468567573 ) ) ;
#123486=CARTESIAN_POINT ( 'NONE',  ( -0.05219959533937732626, 21.53943276465977519, 92.50109039468567573 ) ) ;
#123487=CARTESIAN_POINT ( 'NONE',  ( 16.55341960407618274, -4.379528057220086978, 86.04275706135236135 ) ) ;
#123488=CARTESIAN_POINT ( 'NONE',  ( 18.62759615963255655, 10.81492255796105972, 36.66775706135234714 ) ) ;
#123489=CARTESIAN_POINT ( 'NONE',  ( -18.62759615963255300, -10.81492255796106328, 34.16775706135234714 ) ) ;
#123490=CARTESIAN_POINT ( 'NONE',  ( 13.89961937509957401, 13.97604488694547697, 66.87609039468567573 ) ) ;
#123491=CARTESIAN_POINT ( 'NONE',  ( 5.049401038298161559, -19.05341960407611168, 77.70724293864765286 ) ) ;
#123492=CARTESIAN_POINT ( 'NONE',  ( 16.55341960407611168, 4.379528057220329451, 98.95724293864770971 ) ) ;
#123493=CARTESIAN_POINT ( 'NONE',  ( -21.53943276465977519, 0.05219959533907696930, 86.24890960531436690 ) ) ;
#123494=CARTESIAN_POINT ( 'NONE',  ( -12.06949235617756955, 12.14591786802309770, 65.62390960531436690 ) ) ;
#123495=CARTESIAN_POINT ( 'NONE',  ( 0.05219959533937995610, -21.53943276465977519, 105.0010903946856757 ) ) ;
#123496=CARTESIAN_POINT ( 'NONE',  ( -16.52544592524342804, 4.483927247898546575, 86.04057627198102409 ) ) ;
#123497=CARTESIAN_POINT ( 'NONE',  ( 19.02544592524343514, -5.153800228976328945, 38.54057627198103120 ) ) ;
#123498=CARTESIAN_POINT ( 'NONE',  ( 13.97604488694548053, -13.89961937509957401, 65.62609039468567573 ) ) ;
#123499=CARTESIAN_POINT ( 'NONE',  ( -16.55341960407611168, -4.379528057220339221, 46.45724293864769550 ) ) ;
#123500=CARTESIAN_POINT ( 'NONE',  ( -10.72451020669870658, -18.67979575497194134, 99.58442372801900433 ) ) ;
#123501=CARTESIAN_POINT ( 'NONE',  ( 16.46253265017160672, -9.564922557960803928, 88.33224293864769550 ) ) ;
#123502=CARTESIAN_POINT ( 'NONE',  ( -5.049401038297874678, -19.05341960407617918, 64.79275706135233293 ) ) ;
#123503=CARTESIAN_POINT ( 'NONE',  ( 0.05219959533907565091, 21.53943276465977519, 59.99890960531436690 ) ) ;
#123504=CARTESIAN_POINT ( 'NONE',  ( -15.72974639402197994, 15.80617190586746368, 115.6239096053143669 ) ) ;
#123505=CARTESIAN_POINT ( 'NONE',  ( -8.314922557961024197, 14.29746914071037800, 22.91775706135235069 ) ) ;
#123506=CARTESIAN_POINT ( 'NONE',  ( 16.53943276465976808, 0.05219959533934440121, 76.25109039468568994 ) ) ;
#123508=CARTESIAN_POINT ( 'NONE',  ( -0.05219959533937732626, 21.53943276465977519, 22.50109039468567573 ) ) ;
#123509=CARTESIAN_POINT ( 'NONE',  ( -5.153800228976328057, -19.02544592524343514, 27.29057627198103120 ) ) ;
#123511=CARTESIAN_POINT ( 'NONE',  ( 14.29746914071037800, 8.314922557961029526, 51.66775706135234714 ) ) ;
#123512=CARTESIAN_POINT ( 'NONE',  ( 8.224510206698953496, -14.34966873604960469, 82.91557627198103830 ) ) ;
#123513=CARTESIAN_POINT ( 'NONE',  ( -21.55341960407610458, -5.719274019375992779, 81.45724293864769550 ) ) ;
#123514=CARTESIAN_POINT ( 'NONE',  ( 12.14591786802327356, -12.06949235617739191, 110.6260903946857042 ) ) ;
#123515=CARTESIAN_POINT ( 'NONE',  ( -12.14591786802326823, 12.06949235617739902, 38.12609039468567573 ) ) ;
#123516=CARTESIAN_POINT ( 'NONE',  ( -19.03943276465977164, 0.05219959533909376836, 46.24890960531435979 ) ) ;
#123517=CARTESIAN_POINT ( 'NONE',  ( 12.06949235617739724, 12.14591786802326823, 81.87609039468568994 ) ) ;
#123518=CARTESIAN_POINT ( 'NONE',  ( -19.05341960407617563, 5.049401038297882671, 73.54275706135233293 ) ) ;
#123519=CARTESIAN_POINT ( 'NONE',  ( 21.55341960407610458, 5.719274019375980345, 73.95724293864769550 ) ) ;
#123520=CARTESIAN_POINT ( 'NONE',  ( -14.34966873604972548, 8.224510206698743886, 103.3344237280190043 ) ) ;
#123521=CARTESIAN_POINT ( 'NONE',  ( -5.719274019375665041, -21.55341960407619695, 84.79275706135234714 ) ) ;
#123522=CARTESIAN_POINT ( 'NONE',  ( 21.52544592524344225, -5.823673210054117533, 63.54057627198103830 ) ) ;
#123523=CARTESIAN_POINT ( 'NONE',  ( 18.62759615963271287, -10.81492255796078972, 53.33224293864769550 ) ) ;
#123525=CARTESIAN_POINT ( 'NONE',  ( 16.53943276465976808, 0.05219959533934440121, 76.25109039468568994 ) ) ;
#123526=CARTESIAN_POINT ( 'NONE',  ( 0.05219959533907565091, 21.53943276465977519, 49.99890960531437401 ) ) ;
#123528=CARTESIAN_POINT ( 'NONE',  ( -0.05219959533909027116, -19.03943276465977164, 112.4989096053143669 ) ) ;
#123530=CARTESIAN_POINT ( 'NONE',  ( 16.51473224551069308, 9.474510206698969483, 24.16557627198102765 ) ) ;
#123531=CARTESIAN_POINT ( 'NONE',  ( 10.72451020669898902, -18.67979575497178502, 77.91557627198102409 ) ) ;
#123532=CARTESIAN_POINT ( 'NONE',  ( 8.314922557961029526, -14.29746914071037800, 100.4177570613523471 ) ) ;
#123533=CARTESIAN_POINT ( 'NONE',  ( -18.67979575497193778, 10.72451020669871902, 58.33442372801901143 ) ) ;
#123534=CARTESIAN_POINT ( 'NONE',  ( 0.05219959533934541429, -16.53943276465976808, 25.00109039468567218 ) ) ;
#123535=CARTESIAN_POINT ( 'NONE',  ( -16.51473224551069308, -9.474510206698971260, 26.66557627198103120 ) ) ;
#123536=CARTESIAN_POINT ( 'NONE',  ( -5.153800228976607833, 19.02544592524334988, 112.7094237280190043 ) ) ;
#123537=CARTESIAN_POINT ( 'NONE',  ( 5.153800228976335163, 19.02544592524342804, 34.79057627198102409 ) ) ;
#123540=CARTESIAN_POINT ( 'NONE',  ( -19.02544592524342804, 5.153800228976336051, 111.0405762719810099 ) ) ;
#123541=CARTESIAN_POINT ( 'NONE',  ( -16.55341960407617563, 4.379528057220093196, 83.54275706135234714 ) ) ;
#123542=CARTESIAN_POINT ( 'NONE',  ( -16.46253265017146816, -9.564922557961047289, 79.16775706135234714 ) ) ;
#123543=CARTESIAN_POINT ( 'NONE',  ( 13.97604488694548053, -13.89961937509957401, 30.62609039468566863 ) ) ;
#123544=CARTESIAN_POINT ( 'NONE',  ( 15.80617190586746368, 15.72974639402197994, 59.37390960531436690 ) ) ;
#123545=CARTESIAN_POINT ( 'NONE',  ( -8.314922557961024197, 14.29746914071037800, 87.91775706135234714 ) ) ;
#123546=CARTESIAN_POINT ( 'NONE',  ( 9.564922557961047289, -16.46253265017146816, 95.41775706135233293 ) ) ;
#123547=CARTESIAN_POINT ( 'NONE',  ( 5.153800228976335163, 19.02544592524342804, 49.79057627198100988 ) ) ;
#123548=CARTESIAN_POINT ( 'NONE',  ( 16.46253265017160672, -9.564922557960803928, 88.33224293864769550 ) ) ;
#123549=CARTESIAN_POINT ( 'NONE',  ( 15.80617190586769283, -15.72974639402175789, 50.62609039468568994 ) ) ;
#123550=CARTESIAN_POINT ( 'NONE',  ( 13.89961937509977652, -13.97604488694527269, 43.12390960531434558 ) ) ;
#123551=CARTESIAN_POINT ( 'NONE',  ( -17.48853670773246805, -5.747243402303014115, 86.33328700250008580 ) ) ;
#123552=CARTESIAN_POINT ( 'NONE',  ( 19.05341960407611168, 5.049401038298154454, 108.9572429386477097 ) ) ;
#123553=CARTESIAN_POINT ( 'NONE',  ( 16.53943276465976808, -0.05219959533910856209, 58.74890960531436690 ) ) ;
#123554=CARTESIAN_POINT ( 'NONE',  ( 18.62759615963271287, -10.81492255796078972, 63.33224293864770260 ) ) ;
#123556=CARTESIAN_POINT ( 'NONE',  ( 13.97604488694548053, -13.89961937509957401, 45.62609039468566863 ) ) ;
#123558=CARTESIAN_POINT ( 'NONE',  ( 16.51473224551069308, 9.474510206698969483, 69.16557627198102409 ) ) ;
#123559=CARTESIAN_POINT ( 'NONE',  ( 13.97604488694527802, 13.89961937509977652, 74.37390960531436690 ) ) ;
#123560=CARTESIAN_POINT ( 'NONE',  ( -12.06949235617739369, -12.14591786802326823, 54.37609039468568994 ) ) ;
#123562=CARTESIAN_POINT ( 'NONE',  ( -19.02544592524334988, -5.153800228976617603, 28.95942372801900433 ) ) ;
#123564=CARTESIAN_POINT ( 'NONE',  ( 14.34966873604972726, -8.224510206698740333, 85.83442372801901854 ) ) ;
#123566=CARTESIAN_POINT ( 'NONE',  ( -14.29746914071037622, -8.314922557961029526, 79.16775706135234714 ) ) ;
#123567=CARTESIAN_POINT ( 'NONE',  ( 14.29746914071037800, 8.314922557961029526, 51.66775706135234714 ) ) ;
#123568=CARTESIAN_POINT ( 'NONE',  ( -0.05219959533936034679, 19.03943276465977164, 22.50109039468566152 ) ) ;
#123569=CARTESIAN_POINT ( 'NONE',  ( 13.97604488694527802, 13.89961937509977652, 59.37390960531434558 ) ) ;
#123571=CARTESIAN_POINT ( 'NONE',  ( 15.80617190586769283, -15.72974639402175789, 60.62609039468567573 ) ) ;
#123572=CARTESIAN_POINT ( 'NONE',  ( -0.05219959533936034679, 19.03943276465977164, 72.50109039468566152 ) ) ;
#123573=CARTESIAN_POINT ( 'NONE',  ( -15.80617190586768217, 15.72974639402176855, 103.1260903946856757 ) ) ;
#123574=CARTESIAN_POINT ( 'NONE',  ( 16.46253265017160672, -9.564922557960803928, 28.33224293864769550 ) ) ;
#123576=CARTESIAN_POINT ( 'NONE',  ( -21.55341960407610458, -5.719274019375992779, 71.45724293864769550 ) ) ;
#123577=CARTESIAN_POINT ( 'NONE',  ( -21.55341960407610458, -5.719274019375992779, 21.45724293864769550 ) ) ;
#123578=CARTESIAN_POINT ( 'NONE',  ( 12.14591786802309770, 12.06949235617756955, 114.3739096053143527 ) ) ;
#123579=CARTESIAN_POINT ( 'NONE',  ( -4.483927247898782831, 16.52544592524335698, 32.70942372801900433 ) ) ;
#123580=CARTESIAN_POINT ( 'NONE',  ( -16.52544592524342804, 4.483927247898546575, 26.04057627198103475 ) ) ;
#123582=CARTESIAN_POINT ( 'NONE',  ( 15.80617190586746368, 15.72974639402197994, 114.3739096053143527 ) ) ;
#123584=CARTESIAN_POINT ( 'NONE',  ( -8.224510206698948167, 14.34966873604960824, 45.41557627198103830 ) ) ;
#123586=CARTESIAN_POINT ( 'NONE',  ( 13.89961937509957401, 13.97604488694547697, 106.8760903946856757 ) ) ;
#123587=CARTESIAN_POINT ( 'NONE',  ( -9.564922557961040184, 16.46253265017147172, 22.91775706135233648 ) ) ;
#123588=CARTESIAN_POINT ( 'NONE',  ( 14.34966873604960469, 8.224510206698951720, 44.16557627198103120 ) ) ;
#123589=CARTESIAN_POINT ( 'NONE',  ( 5.719274019375991003, -21.55341960407610458, 97.70724293864772392 ) ) ;
#123590=CARTESIAN_POINT ( 'NONE',  ( 17.50000000000000000, 5.624438216177605199, 31.68329655085357643 ) ) ;
#123591=CARTESIAN_POINT ( 'NONE',  ( 15.80617190586746368, 15.72974639402197994, 69.37390960531436690 ) ) ;
#123592=CARTESIAN_POINT ( 'NONE',  ( -16.51473224551069308, -9.474510206698971260, 76.66557627198103830 ) ) ;
#123593=CARTESIAN_POINT ( 'NONE',  ( 16.52544592524342804, -4.483927247898539470, 48.54057627198103120 ) ) ;
#123594=CARTESIAN_POINT ( 'NONE',  ( 13.89961937509977652, -13.97604488694527269, 93.12390960531436690 ) ) ;
#123596=CARTESIAN_POINT ( 'NONE',  ( -13.97604488694547697, 13.89961937509957934, 53.12609039468565442 ) ) ;
#123597=CARTESIAN_POINT ( 'NONE',  ( 18.67979575497178502, 10.72451020669898547, 89.16557627198102409 ) ) ;
#123598=CARTESIAN_POINT ( 'NONE',  ( -8.314922557960811034, -14.29746914071050412, 102.0822429386476955 ) ) ;
#123599=CARTESIAN_POINT ( 'NONE',  ( -21.53943276465977519, -0.05219959533937600094, 53.75109039468568994 ) ) ;
#123601=CARTESIAN_POINT ( 'NONE',  ( -14.34966873604960291, -8.224510206698953496, 31.66557627198102054 ) ) ;
#123602=CARTESIAN_POINT ( 'NONE',  ( -19.05341960407611168, -5.049401038298163336, 41.45724293864769550 ) ) ;
#123603=CARTESIAN_POINT ( 'NONE',  ( 16.46253265017160672, -9.564922557960803928, 98.33224293864769550 ) ) ;
#123604=CARTESIAN_POINT ( 'NONE',  ( -5.719274019375978568, 21.55341960407610458, 55.20724293864770260 ) ) ;
#123606=CARTESIAN_POINT ( 'NONE',  ( -19.03943276465977164, 0.05219959533909376836, 36.24890960531436690 ) ) ;
#123607=CARTESIAN_POINT ( 'NONE',  ( -10.81492255796078084, -18.62759615963271287, 57.08224293864769550 ) ) ;
#123608=CARTESIAN_POINT ( 'NONE',  ( -10.81492255796105439, 18.62759615963255655, 72.91775706135234714 ) ) ;
#123610=CARTESIAN_POINT ( 'NONE',  ( -8.314922557961024197, 14.29746914071037800, 87.91775706135234714 ) ) ;
#123611=CARTESIAN_POINT ( 'NONE',  ( -0.05219959533909027116, -19.03943276465977164, 57.49890960531435979 ) ) ;
#123612=CARTESIAN_POINT ( 'NONE',  ( -9.474510206698964154, 16.51473224551069663, 60.41557627198102409 ) ) ;
#123614=CARTESIAN_POINT ( 'NONE',  ( 19.02544592524334988, 5.153800228976608722, 31.45942372801900433 ) ) ;
#123615=CARTESIAN_POINT ( 'NONE',  ( 14.29746914071037800, 8.314922557961029526, 81.66775706135236135 ) ) ;
#123616=CARTESIAN_POINT ( 'NONE',  ( 21.53943276465977519, 0.05219959533937863772, 111.2510903946856899 ) ) ;
#123617=CARTESIAN_POINT ( 'NONE',  ( -19.02544592524342804, 5.153800228976336051, 71.04057627198099567 ) ) ;
#123618=CARTESIAN_POINT ( 'NONE',  ( -5.823673210054116645, -21.52544592524344225, 37.29057627198102409 ) ) ;
#123619=CARTESIAN_POINT ( 'NONE',  ( -4.379528057220086978, -16.55341960407618274, 24.79275706135235779 ) ) ;
#123620=CARTESIAN_POINT ( 'NONE',  ( 10.81492255796106328, -18.62759615963255655, 80.41775706135234714 ) ) ;
#123621=CARTESIAN_POINT ( 'NONE',  ( 0.05219959533934541429, -16.53943276465976808, 50.00109039468568994 ) ) ;
#123622=CARTESIAN_POINT ( 'NONE',  ( -18.67979575497178146, -10.72451020669898902, 96.66557627198102409 ) ) ;
#123623=CARTESIAN_POINT ( 'NONE',  ( 19.02544592524334988, 5.153800228976608722, 111.4594237280190043 ) ) ;
#123624=CARTESIAN_POINT ( 'NONE',  ( -13.89961937509977652, 13.97604488694528158, 80.62390960531436690 ) ) ;
#123625=CARTESIAN_POINT ( 'NONE',  ( -12.06949235617739369, -12.14591786802326823, 24.37609039468567573 ) ) ;
#123626=CARTESIAN_POINT ( 'NONE',  ( 19.02544592524343514, -5.153800228976328945, 43.54057627198103120 ) ) ;
#123627=CARTESIAN_POINT ( 'NONE',  ( 8.314922557961029526, -14.29746914071037800, 25.41775706135235779 ) ) ;
#123628=CARTESIAN_POINT ( 'NONE',  ( 16.52544592524342804, -4.483927247898539470, 73.54057627198102409 ) ) ;
#123629=CARTESIAN_POINT ( 'NONE',  ( 14.34966873604972726, -8.224510206698740333, 85.83442372801901854 ) ) ;
#123630=CARTESIAN_POINT ( 'NONE',  ( -18.62759615963255300, -10.81492255796106328, 34.16775706135234714 ) ) ;
#123631=CARTESIAN_POINT ( 'NONE',  ( -5.153800228976328057, -19.02544592524343514, 47.29057627198102409 ) ) ;
#123632=CARTESIAN_POINT ( 'NONE',  ( 9.474510206698971260, -16.51473224551069308, 62.91557627198102409 ) ) ;
#123633=CARTESIAN_POINT ( 'NONE',  ( 8.224510206698742110, 14.34966873604972548, 92.08442372801901854 ) ) ;
#123636=CARTESIAN_POINT ( 'NONE',  ( 19.02544592524334988, 5.153800228976608722, 31.45942372801900433 ) ) ;
#123637=CARTESIAN_POINT ( 'NONE',  ( 0.05219959533909260263, 19.03943276465977164, 29.99890960531435979 ) ) ;
#123638=CARTESIAN_POINT ( 'NONE',  ( 13.97604488694527802, 13.89961937509977652, 109.3739096053143669 ) ) ;
#123640=CARTESIAN_POINT ( 'NONE',  ( 12.14591786802327356, -12.06949235617739191, 30.62609039468567929 ) ) ;
#123641=CARTESIAN_POINT ( 'NONE',  ( -13.97604488694547697, 13.89961937509957934, 58.12609039468566863 ) ) ;
#123642=CARTESIAN_POINT ( 'NONE',  ( 16.53943276465976808, 0.05219959533934440121, 41.25109039468568284 ) ) ;
#123643=CARTESIAN_POINT ( 'NONE',  ( -19.05341960407611168, -5.049401038298163336, 101.4572429386476955 ) ) ;
#123644=CARTESIAN_POINT ( 'NONE',  ( 5.153800228976335163, 19.02544592524342804, 64.79057627198100988 ) ) ;
#123645=CARTESIAN_POINT ( 'NONE',  ( 5.719274019375991003, -21.55341960407610458, 97.70724293864772392 ) ) ;
#123646=CARTESIAN_POINT ( 'NONE',  ( 19.02544592524343514, -5.153800228976328945, 88.54057627198102409 ) ) ;
#123647=CARTESIAN_POINT ( 'NONE',  ( -16.51473224551069308, -9.474510206698971260, 26.66557627198103120 ) ) ;
#123648=CARTESIAN_POINT ( 'NONE',  ( -16.51473224551069308, -9.474510206698971260, 61.66557627198103120 ) ) ;
#123649=CARTESIAN_POINT ( 'NONE',  ( -16.53943276465976808, -0.05219959533934237506, 108.7510903946857042 ) ) ;
#123650=CARTESIAN_POINT ( 'NONE',  ( 13.97604488694527802, 13.89961937509977652, 29.37390960531435979 ) ) ;
#123651=CARTESIAN_POINT ( 'NONE',  ( 9.474510206698729675, 16.51473224551082808, 27.08442372801900433 ) ) ;
#123652=CARTESIAN_POINT ( 'NONE',  ( -12.06949235617756955, 12.14591786802309770, 65.62390960531436690 ) ) ;
#123653=CARTESIAN_POINT ( 'NONE',  ( 0.05219959533937995610, -21.53943276465977519, 105.0010903946856757 ) ) ;
#123654=CARTESIAN_POINT ( 'NONE',  ( -16.51473224551069308, -9.474510206698971260, 36.66557627198102409 ) ) ;
#123655=CARTESIAN_POINT ( 'NONE',  ( 16.52544592524335698, 4.483927247898782831, 56.45942372801902565 ) ) ;
#123656=CARTESIAN_POINT ( 'NONE',  ( -14.29746914071049879, 8.314922557960819915, 40.83224293864769550 ) ) ;
#123657=CARTESIAN_POINT ( 'NONE',  ( 0.05219959533937995610, -21.53943276465977519, 95.00109039468568994 ) ) ;
#123658=CARTESIAN_POINT ( 'NONE',  ( -13.89961937509977652, 13.97604488694528158, 85.62390960531433848 ) ) ;
#123659=CARTESIAN_POINT ( 'NONE',  ( -13.89961937509977652, 13.97604488694528158, 90.62390960531432427 ) ) ;
#123660=CARTESIAN_POINT ( 'NONE',  ( 4.379528057220339221, -16.55341960407611168, 107.7072429386476955 ) ) ;
#123661=CARTESIAN_POINT ( 'NONE',  ( -14.34966873604960291, -8.224510206698953496, 76.66557627198103830 ) ) ;
#123662=CARTESIAN_POINT ( 'NONE',  ( 15.72974639402199770, -15.80617190586745480, 88.12390960531436690 ) ) ;
#123663=CARTESIAN_POINT ( 'NONE',  ( -13.89961937509977652, 13.97604488694528158, 70.62390960531432427 ) ) ;
#123664=CARTESIAN_POINT ( 'NONE',  ( 10.81492255796078972, 18.62759615963270932, 104.5822429386477097 ) ) ;
#123665=CARTESIAN_POINT ( 'NONE',  ( 19.02544592524334988, 5.153800228976608722, 71.45942372801900433 ) ) ;
#123666=CARTESIAN_POINT ( 'NONE',  ( 19.46398650005390252, -5.499999999999938716, 47.68269651486372851 ) ) ;
#123667=CARTESIAN_POINT ( 'NONE',  ( 12.14591786802309770, 12.06949235617756955, 84.37390960531438111 ) ) ;
#123668=CARTESIAN_POINT ( 'NONE',  ( -13.97604488694527625, -13.89961937509977652, 61.87390960531435979 ) ) ;
#123669=CARTESIAN_POINT ( 'NONE',  ( 15.72974639402199770, -15.80617190586745480, 63.12390960531435979 ) ) ;
#123670=CARTESIAN_POINT ( 'NONE',  ( 16.18388926212235290, -7.379444403734659375, 27.06046848633847901 ) ) ;
#123671=CARTESIAN_POINT ( 'NONE',  ( 8.224510206698742110, 14.34966873604972548, 112.0844237280190185 ) ) ;
#123672=CARTESIAN_POINT ( 'NONE',  ( 16.52544592524335698, 4.483927247898782831, 21.45942372801901499 ) ) ;
#123673=CARTESIAN_POINT ( 'NONE',  ( 12.14591786802309770, 12.06949235617756955, 84.37390960531438111 ) ) ;
#123674=CARTESIAN_POINT ( 'NONE',  ( -18.22780087662123805, -5.499999999999968026, 93.98236817873105053 ) ) ;
#123675=CARTESIAN_POINT ( 'NONE',  ( 16.51473224551069308, 9.474510206698969483, 74.16557627198103830 ) ) ;
#123676=CARTESIAN_POINT ( 'NONE',  ( -19.03943276465977164, 0.05219959533909376836, 31.24890960531435979 ) ) ;
#123677=CARTESIAN_POINT ( 'NONE',  ( 4.483927247898545687, 16.52544592524342804, 64.79057627198103830 ) ) ;
#123678=CARTESIAN_POINT ( 'NONE',  ( -19.03943276465977164, 0.05219959533909376836, 116.2489096053143669 ) ) ;
#123679=CARTESIAN_POINT ( 'NONE',  ( 19.05341960407617918, -5.049401038297876454, 91.04275706135234714 ) ) ;
#123680=CARTESIAN_POINT ( 'NONE',  ( -16.46253265017160317, 9.564922557960807481, 80.83224293864769550 ) ) ;
#123681=CARTESIAN_POINT ( 'NONE',  ( 16.51473224551069308, 9.474510206698969483, 84.16557627198102409 ) ) ;
#123682=CARTESIAN_POINT ( 'NONE',  ( 0.05219959533907565091, 21.53943276465977519, 69.99890960531435269 ) ) ;
#123683=CARTESIAN_POINT ( 'NONE',  ( -0.05219959533934338120, 16.53943276465976808, 77.50109039468567573 ) ) ;
#123684=CARTESIAN_POINT ( 'NONE',  ( 16.46253265017146816, 9.564922557961045513, 111.6677570613523329 ) ) ;
#123685=CARTESIAN_POINT ( 'NONE',  ( -19.05341960407611168, -5.049401038298163336, 56.45724293864768129 ) ) ;
#123686=CARTESIAN_POINT ( 'NONE',  ( -18.67979575497178146, -10.72451020669898902, 61.66557627198103120 ) ) ;
#123687=CARTESIAN_POINT ( 'NONE',  ( -19.02544592524334988, -5.153800228976617603, 108.9594237280189759 ) ) ;
#123688=CARTESIAN_POINT ( 'NONE',  ( 12.14591786802309770, 12.06949235617756955, 34.37390960531435979 ) ) ;
#123689=CARTESIAN_POINT ( 'NONE',  ( -5.719274019375665041, -21.55341960407619695, 44.79275706135234714 ) ) ;
#123692=CARTESIAN_POINT ( 'NONE',  ( 4.379528057220092307, 16.55341960407617563, 72.29275706135236135 ) ) ;
#123693=CARTESIAN_POINT ( 'NONE',  ( 5.049401038298161559, -19.05341960407611168, 112.7072429386476813 ) ) ;
#123696=CARTESIAN_POINT ( 'NONE',  ( 8.314922557961029526, -14.29746914071037800, 100.4177570613523471 ) ) ;
#123697=CARTESIAN_POINT ( 'NONE',  ( 16.52544592524335698, 4.483927247898782831, 51.45942372801901854 ) ) ;
#123698=CARTESIAN_POINT ( 'NONE',  ( -0.05219959533909027116, -19.03943276465977164, 57.49890960531435979 ) ) ;
#123699=CARTESIAN_POINT ( 'NONE',  ( 13.97604488694527802, 13.89961937509977652, 69.37390960531436690 ) ) ;
#123700=CARTESIAN_POINT ( 'NONE',  ( 21.55341960407619695, -5.719274019375665929, 51.04275706135234714 ) ) ;
#123701=CARTESIAN_POINT ( 'NONE',  ( 4.483927247898790824, -16.52544592524335698, 65.20942372801901854 ) ) ;
#123702=CARTESIAN_POINT ( 'NONE',  ( -14.34966873604960291, -8.224510206698953496, 36.66557627198103120 ) ) ;
#123703=CARTESIAN_POINT ( 'NONE',  ( -13.89961937509977652, 13.97604488694528158, 35.62390960531435269 ) ) ;
#123704=CARTESIAN_POINT ( 'NONE',  ( 5.153800228976335163, 19.02544592524342804, 39.79057627198100988 ) ) ;
#123705=CARTESIAN_POINT ( 'NONE',  ( -12.14591786802326823, 12.06949235617739902, 23.12609039468567573 ) ) ;
#123707=( BOUNDED_CURVE ( )  B_SPLINE_CURVE ( 2, ( #171114, #105468, #28654, #151973, #66906, #189281, #2251, #188283, #142749, #63933, #37571, #49757, #126581 ),
 .UNSPECIFIED., .F., .F. ) 
 B_SPLINE_CURVE_WITH_KNOTS ( ( 3, 2, 2, 2, 2, 2, 3 ),
 ( 0.3708514890586240842, 0.3728070175438596423, 0.3771929824561403577, 0.3815789473684210731, 0.3859649122807017330, 0.3903508771929824483, 0.3922607258561279231 ),
 .UNSPECIFIED. ) 
 CURVE ( )  GEOMETRIC_REPRESENTATION_ITEM ( )  RATIONAL_B_SPLINE_CURVE ( ( 0.9831626618144004848, 0.9848076720550091867, 1.000000000000000000, 0.9659258262890683122, 1.000000000000000000, 0.9659258262890683122, 1.000000000000000000, 0.9659258262890683122, 1.000000000000000000, 0.9659258262890683122, 1.000000000000000000, 0.9851625545550091179, 0.9832469066685282089 ) ) 
 REPRESENTATION_ITEM ( '' )  );
#123708=CARTESIAN_POINT ( 'NONE',  ( -19.02544592524334988, -5.153800228976617603, 83.95942372801901854 ) ) ;
#123709=CARTESIAN_POINT ( 'NONE',  ( 12.14591786802309770, 12.06949235617756955, 84.37390960531438111 ) ) ;
#123710=CARTESIAN_POINT ( 'NONE',  ( -19.02544592524342804, 5.153800228976336051, 56.04057627198100988 ) ) ;
#123711=CARTESIAN_POINT ( 'NONE',  ( -19.03943276465977164, -0.05219959533935918106, 88.75109039468567573 ) ) ;
#123713=CARTESIAN_POINT ( 'NONE',  ( 21.55341960407619695, -5.719274019375665929, 96.04275706135236135 ) ) ;
#123714=CARTESIAN_POINT ( 'NONE',  ( -8.314922557961024197, 14.29746914071037800, 47.91775706135234714 ) ) ;
#123715=CARTESIAN_POINT ( 'NONE',  ( 17.26172910966778673, 6.454744622555868894, 36.69353091350777163 ) ) ;
#123716=CARTESIAN_POINT ( 'NONE',  ( -21.53943276465977519, 0.05219959533907696930, 51.24890960531436690 ) ) ;
#123717=CARTESIAN_POINT ( 'NONE',  ( 8.224510206698742110, 14.34966873604972548, 42.08442372801901854 ) ) ;
#123718=CARTESIAN_POINT ( 'NONE',  ( -5.049401038298153566, 19.05341960407611168, 35.20724293864768839 ) ) ;
#123719=CARTESIAN_POINT ( 'NONE',  ( 5.153800228976615827, -19.02544592524334988, 45.20942372801901143 ) ) ;
#123720=CARTESIAN_POINT ( 'NONE',  ( 0.05219959533909260263, 19.03943276465977164, 74.99890960531435269 ) ) ;
#123721=CARTESIAN_POINT ( 'NONE',  ( -13.89961937509977652, 13.97604488694528158, 45.62390960531433848 ) ) ;
#123723=CARTESIAN_POINT ( 'NONE',  ( 5.049401038298161559, -19.05341960407611168, 67.70724293864769550 ) ) ;
#123725=CARTESIAN_POINT ( 'NONE',  ( 19.03943276465977164, 0.05219959533936151252, 36.25109039468567573 ) ) ;
#123726=CARTESIAN_POINT ( 'NONE',  ( -18.62759615963255300, -10.81492255796106328, 104.1677570613523471 ) ) ;
#123727=CARTESIAN_POINT ( 'NONE',  ( 16.52544592524342804, -4.483927247898539470, 43.54057627198103830 ) ) ;
#123728=CARTESIAN_POINT ( 'NONE',  ( 0.05219959533909260263, 19.03943276465977164, 44.99890960531435979 ) ) ;
#123729=CARTESIAN_POINT ( 'NONE',  ( -9.474510206698964154, 16.51473224551069663, 105.4155762719810383 ) ) ;
#123730=CARTESIAN_POINT ( 'NONE',  ( -5.823673210054431948, 21.52544592524334988, 87.70942372801901854 ) ) ;
#123731=CARTESIAN_POINT ( 'NONE',  ( 5.049401038298161559, -19.05341960407611168, 52.70724293864767418 ) ) ;
#123732=CARTESIAN_POINT ( 'NONE',  ( -15.72974639402176322, -15.80617190586768395, 84.37609039468570415 ) ) ;
#123733=CARTESIAN_POINT ( 'NONE',  ( 5.719274019375991003, -21.55341960407610458, 42.70724293864770260 ) ) ;
#123734=CARTESIAN_POINT ( 'NONE',  ( 21.55341960407619695, -5.719274019375665929, 21.04275706135234714 ) ) ;
#123735=CARTESIAN_POINT ( 'NONE',  ( -16.46253265017146816, -9.564922557961047289, 54.16775706135234003 ) ) ;
#123736=CARTESIAN_POINT ( 'NONE',  ( -19.03943276465977164, 0.05219959533909376836, 26.24890960531435624 ) ) ;
#123737=CARTESIAN_POINT ( 'NONE',  ( -13.89961937509977652, 13.97604488694528158, 80.62390960531436690 ) ) ;
#123738=CARTESIAN_POINT ( 'NONE',  ( -0.05219959533936034679, 19.03943276465977164, 112.5010903946856757 ) ) ;
#123739=CARTESIAN_POINT ( 'NONE',  ( 16.55341960407611168, 4.379528057220329451, 88.95724293864769550 ) ) ;
#123740=CARTESIAN_POINT ( 'NONE',  ( 16.51473224551069308, 9.474510206698969483, 54.16557627198103120 ) ) ;
#123741=CARTESIAN_POINT ( 'NONE',  ( -10.81492255796078084, -18.62759615963271287, 37.08224293864768129 ) ) ;
#123742=CARTESIAN_POINT ( 'NONE',  ( 19.03943276465977164, 0.05219959533936151252, 96.25109039468567573 ) ) ;
#123743=CARTESIAN_POINT ( 'NONE',  ( -15.80617190586745835, -15.72974639402198527, 101.8739096053143811 ) ) ;
#123744=CARTESIAN_POINT ( 'NONE',  ( 5.719274019375673035, 21.55341960407619339, 52.29275706135236135 ) ) ;
#123745=CARTESIAN_POINT ( 'NONE',  ( 4.483927247898790824, -16.52544592524335698, 60.20942372801902565 ) ) ;
#123746=CARTESIAN_POINT ( 'NONE',  ( -16.55341960407617563, 4.379528057220093196, 73.54275706135234714 ) ) ;
#123747=CARTESIAN_POINT ( 'NONE',  ( -0.05219959533909027116, -19.03943276465977164, 57.49890960531435979 ) ) ;
#123748=CARTESIAN_POINT ( 'NONE',  ( -4.379528057220086978, -16.55341960407618274, 89.79275706135236135 ) ) ;
#123749=CARTESIAN_POINT ( 'NONE',  ( 18.67979575497194134, -10.72451020669871369, 20.83442372801901143 ) ) ;
#123750=CARTESIAN_POINT ( 'NONE',  ( 16.53943276465976808, -0.05219959533910856209, 68.74890960531435269 ) ) ;
#123751=CARTESIAN_POINT ( 'NONE',  ( 19.02544592524343514, -5.153800228976328945, 83.54057627198100988 ) ) ;
#123752=CARTESIAN_POINT ( 'NONE',  ( -12.14591786802326823, 12.06949235617739902, 73.12609039468567573 ) ) ;
#123753=CARTESIAN_POINT ( 'NONE',  ( -15.80617190586768217, 15.72974639402176855, 53.12609039468568284 ) ) ;
#123754=CARTESIAN_POINT ( 'NONE',  ( -16.53943276465976808, -0.05219959533934237506, 18.75109039468568639 ) ) ;
#123755=CARTESIAN_POINT ( 'NONE',  ( -18.62759615963255300, -10.81492255796106328, 19.16775706135234714 ) ) ;
#123756=CARTESIAN_POINT ( 'NONE',  ( -8.224510206698948167, 14.34966873604960824, 60.41557627198102409 ) ) ;
#123758=CARTESIAN_POINT ( 'NONE',  ( -17.44279575226823553, 5.990770900252460507, 75.83557567514316133 ) ) ;
#123759=CARTESIAN_POINT ( 'NONE',  ( 5.719274019375991003, -21.55341960407610458, 82.70724293864770971 ) ) ;
#123760=CARTESIAN_POINT ( 'NONE',  ( -16.52544592524342804, 4.483927247898546575, 46.04057627198103830 ) ) ;
#123763=CARTESIAN_POINT ( 'NONE',  ( -15.72974639402197994, 15.80617190586746368, 110.6239096053143669 ) ) ;
#123764=CARTESIAN_POINT ( 'NONE',  ( 19.02544592524343514, -5.153800228976328945, 113.5405762719810241 ) ) ;
#123765=CARTESIAN_POINT ( 'NONE',  ( 10.72451020669871369, 18.67979575497193778, 27.08442372801901854 ) ) ;
#123766=CARTESIAN_POINT ( 'NONE',  ( -4.483927247898539470, -16.52544592524342804, 57.29057627198103120 ) ) ;
#123767=CARTESIAN_POINT ( 'NONE',  ( -16.55341960407617563, 4.379528057220093196, 58.54275706135235424 ) ) ;
#123768=CARTESIAN_POINT ( 'NONE',  ( 13.89961937509977652, -13.97604488694527269, 63.12390960531435979 ) ) ;
#123769=CARTESIAN_POINT ( 'NONE',  ( 16.46253265017146816, 9.564922557961045513, 66.66775706135233293 ) ) ;
#123770=CARTESIAN_POINT ( 'NONE',  ( -9.474510206698964154, 16.51473224551069663, 75.41557627198103830 ) ) ;
#123772=CARTESIAN_POINT ( 'NONE',  ( 0.05219959533907565091, 21.53943276465977519, 54.99890960531435269 ) ) ;
#123774=CARTESIAN_POINT ( 'NONE',  ( -5.049401038298153566, 19.05341960407611168, 60.20724293864768129 ) ) ;
#123775=CARTESIAN_POINT ( 'NONE',  ( -14.29746914071037622, -8.314922557961029526, 29.16775706135234003 ) ) ;
#123776=CARTESIAN_POINT ( 'NONE',  ( 5.153800228976615827, -19.02544592524334988, 65.20942372801900433 ) ) ;
#123777=CARTESIAN_POINT ( 'NONE',  ( -15.72974639402197994, 15.80617190586746368, 110.6239096053143669 ) ) ;
#123778=CARTESIAN_POINT ( 'NONE',  ( 14.34966873604960469, 8.224510206698951720, 49.16557627198102409 ) ) ;
#123779=CARTESIAN_POINT ( 'NONE',  ( 0.05219959533909260263, 19.03943276465977164, 94.99890960531436690 ) ) ;
#123780=CARTESIAN_POINT ( 'NONE',  ( 15.72974639402199770, -15.80617190586745480, 58.12390960531435979 ) ) ;
#123781=CARTESIAN_POINT ( 'NONE',  ( -0.05219959533907301413, -21.53943276465977519, 92.49890960531436690 ) ) ;
#123782=CARTESIAN_POINT ( 'NONE',  ( -0.05219959533934338120, 16.53943276465976808, 42.50109039468567573 ) ) ;
#123783=CARTESIAN_POINT ( 'NONE',  ( 5.823673210054125526, 21.52544592524343514, 34.79057627198103120 ) ) ;
#123784=CARTESIAN_POINT ( 'NONE',  ( 18.62759615963255655, 10.81492255796105972, 86.66775706135234714 ) ) ;
#123785=CARTESIAN_POINT ( 'NONE',  ( 16.51473224551069308, 9.474510206698969483, 89.16557627198103830 ) ) ;
#123786=CARTESIAN_POINT ( 'NONE',  ( -19.03943276465977164, 0.05219959533909376836, 41.24890960531435269 ) ) ;
#123787=CARTESIAN_POINT ( 'NONE',  ( -19.03943276465977164, 0.05219959533909376836, 91.24890960531436690 ) ) ;
#123788=CARTESIAN_POINT ( 'NONE',  ( 12.06949235617757843, -12.14591786802309237, 103.1239096053143811 ) ) ;
#123789=CARTESIAN_POINT ( 'NONE',  ( 9.564922557960805705, 16.46253265017160317, 69.58224293864770971 ) ) ;
#123790=CARTESIAN_POINT ( 'NONE',  ( 14.34966873604972726, -8.224510206698740333, 25.83442372801901499 ) ) ;
#123792=CARTESIAN_POINT ( 'NONE',  ( 17.50000000000003197, 4.658240926743142829, 33.55529582183199722 ) ) ;
#123793=CARTESIAN_POINT ( 'NONE',  ( -15.72974639402176322, -15.80617190586768395, 104.3760903946856899 ) ) ;
#123794=CARTESIAN_POINT ( 'NONE',  ( 21.53943276465977519, -0.05219959533907433946, 28.74890960531435624 ) ) ;
#123795=CARTESIAN_POINT ( 'NONE',  ( 4.379528057220092307, 16.55341960407617563, 87.29275706135236135 ) ) ;
#123797=CARTESIAN_POINT ( 'NONE',  ( 16.46253265017146816, 9.564922557961045513, 71.66775706135233293 ) ) ;
#123798=CARTESIAN_POINT ( 'NONE',  ( 19.05341960407617918, -5.049401038297876454, 31.04275706135232227 ) ) ;
#123799=DIRECTION ( 'NONE',  ( 0.000000000000000000, 0.000000000000000000, 1.000000000000000000 ) ) ;
#123800=CARTESIAN_POINT ( 'NONE',  ( 19.02544592524343514, -5.153800228976328945, 33.54057627198102409 ) ) ;
#123801=CARTESIAN_POINT ( 'NONE',  ( 8.224510206698953496, -14.34966873604960469, 32.91557627198102409 ) ) ;
#123802=CARTESIAN_POINT ( 'NONE',  ( -16.88567814943161949, -6.947325034625689177, 111.2900112265258770 ) ) ;
#123803=CARTESIAN_POINT ( 'NONE',  ( 16.52544592524342804, -4.483927247898539470, 28.54057627198103120 ) ) ;
#123804=CARTESIAN_POINT ( 'NONE',  ( 17.49999999999999289, 5.624438216177599870, 66.68329655085355512 ) ) ;
#123805=CARTESIAN_POINT ( 'NONE',  ( 16.52544592524335698, 4.483927247898782831, 91.45942372801901854 ) ) ;
#123806=CARTESIAN_POINT ( 'NONE',  ( 19.05341960407611168, 5.049401038298154454, 33.95724293864769550 ) ) ;
#123807=CARTESIAN_POINT ( 'NONE',  ( 15.80617190586769283, -15.72974639402175789, 110.6260903946857042 ) ) ;
#123808=CARTESIAN_POINT ( 'NONE',  ( 16.52544592524335698, 4.483927247898782831, 21.45942372801901499 ) ) ;
#123809=CARTESIAN_POINT ( 'NONE',  ( -15.72974639402176322, -15.80617190586768395, 79.37609039468567573 ) ) ;
#123810=CARTESIAN_POINT ( 'NONE',  ( 16.46253265017146816, 9.564922557961045513, 51.66775706135233293 ) ) ;
#123811=CARTESIAN_POINT ( 'NONE',  ( 19.03943276465977164, -0.05219959533909143690, 88.74890960531436690 ) ) ;
#123812=CARTESIAN_POINT ( 'NONE',  ( -5.153800228976328057, -19.02544592524343514, 72.29057627198102409 ) ) ;
#123813=CARTESIAN_POINT ( 'NONE',  ( -19.52837319214028255, 5.499999999999903189, 39.60471352585542348 ) ) ;
#123814=CARTESIAN_POINT ( 'NONE',  ( -0.05219959533907301413, -21.53943276465977519, 92.49890960531436690 ) ) ;
#123815=CARTESIAN_POINT ( 'NONE',  ( 4.379528057220339221, -16.55341960407611168, 62.70724293864769550 ) ) ;
#123816=CARTESIAN_POINT ( 'NONE',  ( 5.719274019375991003, -21.55341960407610458, 62.70724293864769550 ) ) ;
#123817=CARTESIAN_POINT ( 'NONE',  ( -5.049401038298153566, 19.05341960407611168, 65.20724293864765286 ) ) ;
#123818=CARTESIAN_POINT ( 'NONE',  ( -10.81492255796078084, -18.62759615963271287, 87.08224293864769550 ) ) ;
#123819=CARTESIAN_POINT ( 'NONE',  ( 12.14591786802327356, -12.06949235617739191, 80.62609039468567573 ) ) ;
#123821=CARTESIAN_POINT ( 'NONE',  ( -16.51473224551069308, -9.474510206698971260, 41.66557627198103120 ) ) ;
#123822=CARTESIAN_POINT ( 'NONE',  ( -12.14591786802309592, -12.06949235617757132, 76.87390960531439532 ) ) ;
#123824=CARTESIAN_POINT ( 'NONE',  ( -5.049401038298153566, 19.05341960407611168, 55.20724293864769550 ) ) ;
#123825=CARTESIAN_POINT ( 'NONE',  ( 16.53943276465976808, -0.05219959533910856209, 113.7489096053143527 ) ) ;
#123826=CARTESIAN_POINT ( 'NONE',  ( 19.05341960407617918, -5.049401038297876454, 66.04275706135233293 ) ) ;
#123827=CARTESIAN_POINT ( 'NONE',  ( 12.06949235617757843, -12.14591786802309237, 88.12390960531436690 ) ) ;
#123828=CARTESIAN_POINT ( 'NONE',  ( 21.52544592524334988, 5.823673210054432836, 46.45942372801901854 ) ) ;
#123829=CARTESIAN_POINT ( 'NONE',  ( 5.049401038298161559, -19.05341960407611168, 32.70724293864768129 ) ) ;
#123830=CARTESIAN_POINT ( 'NONE',  ( 15.72974639402199770, -15.80617190586745480, 103.1239096053143811 ) ) ;
#123831=CARTESIAN_POINT ( 'NONE',  ( 12.06949235617757843, -12.14591786802309237, 88.12390960531436690 ) ) ;
#123833=CARTESIAN_POINT ( 'NONE',  ( 9.474510206698971260, -16.51473224551069308, 57.91557627198103120 ) ) ;
#123834=CARTESIAN_POINT ( 'NONE',  ( 19.35543954521082100, 5.499999999999580780, 47.08901960356454452 ) ) ;
#123835=CARTESIAN_POINT ( 'NONE',  ( -16.51473224551082808, 9.474510206698731452, 98.33442372801900433 ) ) ;
#123836=CARTESIAN_POINT ( 'NONE',  ( -5.153800228976328057, -19.02544592524343514, 102.2905762719810383 ) ) ;
#123837=CARTESIAN_POINT ( 'NONE',  ( -10.72451020669870658, -18.67979575497194134, 34.58442372801900433 ) ) ;
#123838=CARTESIAN_POINT ( 'NONE',  ( -16.46253265017160317, 9.564922557960807481, 85.83224293864769550 ) ) ;
#123839=CARTESIAN_POINT ( 'NONE',  ( -19.02544592524334988, -5.153800228976617603, 68.95942372801896170 ) ) ;
#123840=CARTESIAN_POINT ( 'NONE',  ( 19.02544592524343514, -5.153800228976328945, 58.54057627198102409 ) ) ;
#123841=CARTESIAN_POINT ( 'NONE',  ( 0.05219959533910956823, 16.53943276465976808, 79.99890960531435269 ) ) ;
#123842=CARTESIAN_POINT ( 'NONE',  ( 12.14591786802309770, 12.06949235617756955, 64.37390960531435269 ) ) ;
#123843=CARTESIAN_POINT ( 'NONE',  ( 19.05341960407611168, 5.049401038298154454, 83.95724293864766707 ) ) ;
#123844=CARTESIAN_POINT ( 'NONE',  ( 10.72451020669898902, -18.67979575497178502, 97.91557627198103830 ) ) ;
#123845=CARTESIAN_POINT ( 'NONE',  ( -13.89961937509977652, 13.97604488694528158, 80.62390960531436690 ) ) ;
#123846=CARTESIAN_POINT ( 'NONE',  ( -0.05219959533936034679, 19.03943276465977164, 27.50109039468566507 ) ) ;
#123847=CARTESIAN_POINT ( 'NONE',  ( -5.049401038298153566, 19.05341960407611168, 30.20724293864768839 ) ) ;
#123848=CARTESIAN_POINT ( 'NONE',  ( 8.314922557960818139, 14.29746914071049879, 34.58224293864770260 ) ) ;
#123849=CARTESIAN_POINT ( 'NONE',  ( 16.52544592524342804, -4.483927247898539470, 103.5405762719810383 ) ) ;
#123850=CARTESIAN_POINT ( 'NONE',  ( 0.05219959533936267826, -19.03943276465977164, 105.0010903946856615 ) ) ;
#123852=CARTESIAN_POINT ( 'NONE',  ( -15.72974639402176322, -15.80617190586768395, 34.37609039468568284 ) ) ;
#123853=CARTESIAN_POINT ( 'NONE',  ( -19.03943276465977164, -0.05219959533935918106, 68.75109039468566152 ) ) ;
#123854=CARTESIAN_POINT ( 'NONE',  ( 14.34966873604960469, 8.224510206698951720, 24.16557627198103120 ) ) ;
#123855=CARTESIAN_POINT ( 'NONE',  ( -0.05219959533907301413, -21.53943276465977519, 82.49890960531436690 ) ) ;
#123856=CARTESIAN_POINT ( 'NONE',  ( 9.564922557960805705, 16.46253265017160317, 114.5822429386476955 ) ) ;
#123857=CARTESIAN_POINT ( 'NONE',  ( -0.05219959533910754901, -16.53943276465976808, 67.49890960531436690 ) ) ;
#123858=CARTESIAN_POINT ( 'NONE',  ( 19.02544592524343514, -5.153800228976328945, 23.54057627198102054 ) ) ;
#123859=CARTESIAN_POINT ( 'NONE',  ( -0.05219959533936034679, 19.03943276465977164, 32.50109039468566863 ) ) ;
#123860=CARTESIAN_POINT ( 'NONE',  ( 16.52544592524335698, 4.483927247898782831, 86.45942372801901854 ) ) ;
#123861=CARTESIAN_POINT ( 'NONE',  ( 16.53943276465976808, 0.05219959533934440121, 61.25109039468567573 ) ) ;
#123862=CARTESIAN_POINT ( 'NONE',  ( 16.46253265017160672, -9.564922557960803928, 113.3322429386476955 ) ) ;
#123863=CARTESIAN_POINT ( 'NONE',  ( -21.53943276465977519, -0.05219959533937600094, 108.7510903946857042 ) ) ;
#123864=CARTESIAN_POINT ( 'NONE',  ( 19.05341960407611168, 5.049401038298154454, 73.95724293864768129 ) ) ;
#123865=CARTESIAN_POINT ( 'NONE',  ( -16.52544592524335698, -4.483927247898792601, 63.95942372801901854 ) ) ;
#123866=CARTESIAN_POINT ( 'NONE',  ( -12.06949235617756955, 12.14591786802309770, 115.6239096053143669 ) ) ;
#123867=CARTESIAN_POINT ( 'NONE',  ( 8.314922557960818139, 14.29746914071049879, 39.58224293864769550 ) ) ;
#123868=CARTESIAN_POINT ( 'NONE',  ( -17.60728821186567217, 5.500000000000031086, 70.86690927743002533 ) ) ;
#123869=CARTESIAN_POINT ( 'NONE',  ( 13.97604488694527802, 13.89961937509977652, 104.3739096053143385 ) ) ;
#123870=CARTESIAN_POINT ( 'NONE',  ( 19.02544592524343514, -5.153800228976328945, 78.54057627198099567 ) ) ;
#123871=CARTESIAN_POINT ( 'NONE',  ( -5.049401038298153566, 19.05341960407611168, 115.2072429386477097 ) ) ;
#123872=CARTESIAN_POINT ( 'NONE',  ( 16.55341960407611168, 4.379528057220329451, 63.95724293864770260 ) ) ;
#123874=CARTESIAN_POINT ( 'NONE',  ( -12.06949235617756955, 12.14591786802309770, 35.62390960531437401 ) ) ;
#123876=CARTESIAN_POINT ( 'NONE',  ( -4.483927247898539470, -16.52544592524342804, 57.29057627198103120 ) ) ;
#123878=CARTESIAN_POINT ( 'NONE',  ( -12.14591786802326823, 12.06949235617739902, 43.12609039468568284 ) ) ;
#123879=CARTESIAN_POINT ( 'NONE',  ( -17.58332526062528345, -7.635886036038592728, 59.07665040441534643 ) ) ;
#123880=CARTESIAN_POINT ( 'NONE',  ( 13.97604488694548053, -13.89961937509957401, 45.62609039468566863 ) ) ;
#123881=CARTESIAN_POINT ( 'NONE',  ( -5.153800228976328057, -19.02544592524343514, 82.29057627198103830 ) ) ;
#123882=CARTESIAN_POINT ( 'NONE',  ( 0.05219959533936267826, -19.03943276465977164, 50.00109039468566863 ) ) ;
#123884=CARTESIAN_POINT ( 'NONE',  ( 13.97604488694548053, -13.89961937509957401, 55.62609039468566863 ) ) ;
#123885=CARTESIAN_POINT ( 'NONE',  ( 9.564922557961047289, -16.46253265017146816, 95.41775706135233293 ) ) ;
#123886=CARTESIAN_POINT ( 'NONE',  ( -14.34966873604972548, 8.224510206698743886, 78.33442372801901854 ) ) ;
#123888=CARTESIAN_POINT ( 'NONE',  ( -9.474510206698964154, 16.51473224551069663, 25.41557627198103120 ) ) ;
#123889=CARTESIAN_POINT ( 'NONE',  ( 13.97604488694527802, 13.89961937509977652, 104.3739096053143385 ) ) ;
#123890=CARTESIAN_POINT ( 'NONE',  ( -0.05219959533937732626, 21.53943276465977519, 47.50109039468568994 ) ) ;
#123891=CARTESIAN_POINT ( 'NONE',  ( -19.05341960407617563, 5.049401038297882671, 98.54275706135233293 ) ) ;
#123892=CARTESIAN_POINT ( 'NONE',  ( 17.49999999999999645, 3.534425089339017223, 23.05531345578905800 ) ) ;
#123893=CARTESIAN_POINT ( 'NONE',  ( -13.97604488694527625, -13.89961937509977652, 56.87390960531434558 ) ) ;
#123894=CARTESIAN_POINT ( 'NONE',  ( -5.049401038298153566, 19.05341960407611168, 110.2072429386476671 ) ) ;
#123895=CARTESIAN_POINT ( 'NONE',  ( 16.55341960407611168, 4.379528057220329451, 63.95724293864770260 ) ) ;
#123896=CARTESIAN_POINT ( 'NONE',  ( 16.51473224551069308, 9.474510206698969483, 69.16557627198102409 ) ) ;
#123897=CARTESIAN_POINT ( 'NONE',  ( -5.049401038298153566, 19.05341960407611168, 60.20724293864768129 ) ) ;
#123898=CARTESIAN_POINT ( 'NONE',  ( -19.02544592524334988, -5.153800228976617603, 83.95942372801901854 ) ) ;
#123899=CARTESIAN_POINT ( 'NONE',  ( 15.72974639402199770, -15.80617190586745480, 53.12390960531436690 ) ) ;
#123900=CARTESIAN_POINT ( 'NONE',  ( 16.51473224551083163, -9.474510206698727899, 45.83442372801900433 ) ) ;
#123901=CARTESIAN_POINT ( 'NONE',  ( -19.03943276465977164, 0.05219959533909376836, 81.24890960531436690 ) ) ;
#123902=CARTESIAN_POINT ( 'NONE',  ( 0.05219959533907565091, 21.53943276465977519, 79.99890960531435269 ) ) ;
#123903=CARTESIAN_POINT ( 'NONE',  ( -8.314922557960811034, -14.29746914071050412, 82.08224293864768129 ) ) ;
#123904=CARTESIAN_POINT ( 'NONE',  ( -13.97604488694547697, 13.89961937509957934, 33.12609039468566863 ) ) ;
#123905=CARTESIAN_POINT ( 'NONE',  ( 10.81492255796078972, 18.62759615963270932, 59.58224293864770260 ) ) ;
#123906=CARTESIAN_POINT ( 'NONE',  ( -21.55341960407610458, -5.719274019375992779, 41.45724293864769550 ) ) ;
#123907=CARTESIAN_POINT ( 'NONE',  ( 19.03943276465977164, -0.05219959533909143690, 63.74890960531435979 ) ) ;
#123908=CARTESIAN_POINT ( 'NONE',  ( -0.05219959533909027116, -19.03943276465977164, 22.49890960531436690 ) ) ;
#123910=CARTESIAN_POINT ( 'NONE',  ( -5.719274019375665041, -21.55341960407619695, 29.79275706135234358 ) ) ;
#123911=CARTESIAN_POINT ( 'NONE',  ( -19.05341960407611168, -5.049401038298163336, 111.4572429386476671 ) ) ;
#123912=CARTESIAN_POINT ( 'NONE',  ( 15.72974639402176855, 15.80617190586768217, 41.87609039468568284 ) ) ;
#123913=CARTESIAN_POINT ( 'NONE',  ( 16.51473224551069308, 9.474510206698969483, 39.16557627198103120 ) ) ;
#123914=CARTESIAN_POINT ( 'NONE',  ( 21.53943276465977519, -0.05219959533907433946, 108.7489096053143669 ) ) ;
#123915=CARTESIAN_POINT ( 'NONE',  ( -19.02544592524334988, -5.153800228976617603, 53.95942372801898301 ) ) ;
#123917=CARTESIAN_POINT ( 'NONE',  ( 19.49149378614661288, -5.499999999999571010, 76.93757513605359577 ) ) ;
#123918=LINE ( 'NONE', #167478, #98365 ) ;
#123919=CARTESIAN_POINT ( 'NONE',  ( -16.53943276465976808, -0.05219959533934237506, 58.75109039468568994 ) ) ;
#123920=CARTESIAN_POINT ( 'NONE',  ( -19.03943276465977164, 0.05219959533909376836, 21.24890960531436335 ) ) ;
#123922=CARTESIAN_POINT ( 'NONE',  ( 9.474510206698971260, -16.51473224551069308, 67.91557627198102409 ) ) ;
#123923=CARTESIAN_POINT ( 'NONE',  ( -14.34966873604960291, -8.224510206698953496, 101.6655762719810383 ) ) ;
#123924=B_SPLINE_CURVE_WITH_KNOTS ( 'NONE', 3,
 ( #127908, #99571, #161252, #8577, #22746, #162252, #36897, #160255, #19750, #7556, #81391, #21745, #189610, #51084, #20736, #112744, #70252, #130908, #129887, #192598, #23751, #174437, #85401, #97553, #35907, #131920, #82392, #5561, #67240, #128899, #190598, #101570 ),
 .UNSPECIFIED., .F., .F.,
 ( 4, 2, 2, 2, 2, 2, 2, 2, 2, 2, 2, 2, 2, 2, 2, 4 ),
 ( 1.599336020787782259E-17, 0.0003712461730036884584, 0.0007424923460073609791, 0.001113738519011033337, 0.001484984692014705912, 0.002227477038022050628, 0.002598723211025726672, 0.002969969384029402283, 0.003341215557033078327, 0.003712461730036753938, 0.004083707903040429549, 0.004454954076044104726, 0.004826200249047780770, 0.005197446422051455947, 0.005568692595055131991, 0.005939938768058808036 ),
 .UNSPECIFIED. ) ;
#123925=CARTESIAN_POINT ( 'NONE',  ( -5.719274019375978568, 21.55341960407610458, 60.20724293864768839 ) ) ;
#123926=CARTESIAN_POINT ( 'NONE',  ( -4.379528057220086978, -16.55341960407618274, 34.79275706135235424 ) ) ;
#123927=CARTESIAN_POINT ( 'NONE',  ( -21.55341960407619339, 5.719274019375674811, 103.5427570613523613 ) ) ;
#123928=CARTESIAN_POINT ( 'NONE',  ( 5.049401038298161559, -19.05341960407611168, 27.70724293864769550 ) ) ;
#123929=CARTESIAN_POINT ( 'NONE',  ( -16.52544592524335698, -4.483927247898792601, 108.9594237280190185 ) ) ;
#123930=CARTESIAN_POINT ( 'NONE',  ( 14.29746914071049879, -8.314922557960816363, 48.33224293864770260 ) ) ;
#123931=CARTESIAN_POINT ( 'NONE',  ( 16.51473224551069308, 9.474510206698969483, 49.16557627198102409 ) ) ;
#123932=CARTESIAN_POINT ( 'NONE',  ( -0.05219959533937732626, 21.53943276465977519, 92.50109039468567573 ) ) ;
#123933=CARTESIAN_POINT ( 'NONE',  ( 15.80617190586746368, 15.72974639402197994, 109.3739096053143811 ) ) ;
#123934=CARTESIAN_POINT ( 'NONE',  ( -15.80617190586768217, 15.72974639402176855, 68.12609039468567573 ) ) ;
#123935=CARTESIAN_POINT ( 'NONE',  ( -8.314922557961024197, 14.29746914071037800, 52.91775706135235424 ) ) ;
#123936=CARTESIAN_POINT ( 'NONE',  ( -14.29746914071049879, 8.314922557960819915, 75.83224293864769550 ) ) ;
#123937=CARTESIAN_POINT ( 'NONE',  ( -21.53943276465977519, -0.05219959533937600094, 98.75109039468568994 ) ) ;
#123938=CARTESIAN_POINT ( 'NONE',  ( 12.14591786802327356, -12.06949235617739191, 110.6260903946857042 ) ) ;
#123939=CARTESIAN_POINT ( 'NONE',  ( -17.31728774477274513, 6.344390552232361813, 115.8190665168932156 ) ) ;
#123940=CARTESIAN_POINT ( 'NONE',  ( 0.05219959533934541429, -16.53943276465976808, 35.00109039468568284 ) ) ;
#123941=CARTESIAN_POINT ( 'NONE',  ( -12.14591786802309592, -12.06949235617757132, 36.87390960531435979 ) ) ;
#123942=CARTESIAN_POINT ( 'NONE',  ( 12.14591786802327356, -12.06949235617739191, 80.62609039468567573 ) ) ;
#123943=CARTESIAN_POINT ( 'NONE',  ( 19.05341960407611168, 5.049401038298154454, 93.95724293864769550 ) ) ;
#123944=CARTESIAN_POINT ( 'NONE',  ( 19.05341960407611168, 5.049401038298154454, 108.9572429386477097 ) ) ;
#123945=CARTESIAN_POINT ( 'NONE',  ( -15.80617190586768217, 15.72974639402176855, 98.12609039468570415 ) ) ;
#123946=CARTESIAN_POINT ( 'NONE',  ( -16.53943276465976808, -0.05219959533934237506, 108.7510903946857042 ) ) ;
#123947=CARTESIAN_POINT ( 'NONE',  ( 14.29746914071049879, -8.314922557960816363, 68.33224293864769550 ) ) ;
#123948=CARTESIAN_POINT ( 'NONE',  ( -19.03943276465977164, 0.05219959533909376836, 76.24890960531435269 ) ) ;
#123949=ORIENTED_EDGE ( 'NONE', *, *, #45027, .T. ) ;
#123950=CARTESIAN_POINT ( 'NONE',  ( -0.05219959533934338120, 16.53943276465976808, 32.50109039468568284 ) ) ;
#123951=CARTESIAN_POINT ( 'NONE',  ( 13.97604488694527802, 13.89961937509977652, 24.37390960531435624 ) ) ;
#123952=CARTESIAN_POINT ( 'NONE',  ( -19.05341960407611168, -5.049401038298163336, 86.45724293864769550 ) ) ;
#123953=CARTESIAN_POINT ( 'NONE',  ( -16.53943276465976808, -0.05219959533934237506, 33.75109039468568284 ) ) ;
#123955=CARTESIAN_POINT ( 'NONE',  ( -13.97604488694547697, 13.89961937509957934, 33.12609039468566863 ) ) ;
#123956=CARTESIAN_POINT ( 'NONE',  ( -4.483927247898782831, 16.52544592524335698, 92.70942372801901854 ) ) ;
#123957=CARTESIAN_POINT ( 'NONE',  ( -0.05219959533909027116, -19.03943276465977164, 32.49890960531435979 ) ) ;
#123958=CARTESIAN_POINT ( 'NONE',  ( 16.53943276465976808, 0.05219959533934440121, 86.25109039468568994 ) ) ;
#123959=CARTESIAN_POINT ( 'NONE',  ( -8.314922557961024197, 14.29746914071037800, 72.91775706135234714 ) ) ;
#123960=CARTESIAN_POINT ( 'NONE',  ( -5.153800228976607833, 19.02544592524334988, 82.70942372801897591 ) ) ;
#123961=CARTESIAN_POINT ( 'NONE',  ( 0.05219959533936267826, -19.03943276465977164, 35.00109039468566863 ) ) ;
#123962=CARTESIAN_POINT ( 'NONE',  ( -0.05219959533909027116, -19.03943276465977164, 42.49890960531435269 ) ) ;
#123963=CARTESIAN_POINT ( 'NONE',  ( -13.97604488694527625, -13.89961937509977652, 96.87390960531433848 ) ) ;
#123964=CARTESIAN_POINT ( 'NONE',  ( 8.314922557960818139, 14.29746914071049879, 84.58224293864769550 ) ) ;
#123967=CARTESIAN_POINT ( 'NONE',  ( -9.474510206698720793, -16.51473224551083518, 54.58442372801899722 ) ) ;
#123968=CARTESIAN_POINT ( 'NONE',  ( -5.719274019375978568, 21.55341960407610458, 45.20724293864769550 ) ) ;
#123969=CARTESIAN_POINT ( 'NONE',  ( 13.89961937509957401, 13.97604488694547697, 31.87609039468566863 ) ) ;
#123970=CARTESIAN_POINT ( 'NONE',  ( 5.049401038298161559, -19.05341960407611168, 102.7072429386476955 ) ) ;
#123971=CARTESIAN_POINT ( 'NONE',  ( 15.80617190586746368, 15.72974639402197994, 74.37390960531436690 ) ) ;
#123972=CARTESIAN_POINT ( 'NONE',  ( -9.474510206698964154, 16.51473224551069663, 110.4155762719810383 ) ) ;
#123973=CARTESIAN_POINT ( 'NONE',  ( 9.564922557961047289, -16.46253265017146816, 85.41775706135233293 ) ) ;
#123974=CARTESIAN_POINT ( 'NONE',  ( -17.49999999999999289, 5.068104630630373642, 110.7281840534002413 ) ) ;
#123975=CARTESIAN_POINT ( 'NONE',  ( -16.51473224551082808, 9.474510206698731452, 108.3344237280190043 ) ) ;
#123976=CARTESIAN_POINT ( 'NONE',  ( -13.89961937509977652, 13.97604488694528158, 35.62390960531435269 ) ) ;
#123977=CARTESIAN_POINT ( 'NONE',  ( -16.51473224551069308, -9.474510206698971260, 91.66557627198103830 ) ) ;
#123978=CARTESIAN_POINT ( 'NONE',  ( -21.52544592524343514, 5.823673210054127303, 71.04057627198103830 ) ) ;
#123979=CARTESIAN_POINT ( 'NONE',  ( -12.14591786802326823, 12.06949235617739902, 48.12609039468568284 ) ) ;
#123980=CARTESIAN_POINT ( 'NONE',  ( 21.52544592524334988, 5.823673210054432836, 51.45942372801901854 ) ) ;
#123981=CARTESIAN_POINT ( 'NONE',  ( 0.05219959533936267826, -19.03943276465977164, 95.00109039468567573 ) ) ;
#123982=CARTESIAN_POINT ( 'NONE',  ( -15.72974639402176322, -15.80617190586768395, 94.37609039468568994 ) ) ;
#123983=CARTESIAN_POINT ( 'NONE',  ( 8.224510206698742110, 14.34966873604972548, 112.0844237280190185 ) ) ;
#123984=CARTESIAN_POINT ( 'NONE',  ( 16.46253265017160672, -9.564922557960803928, 103.3322429386476955 ) ) ;
#123985=CARTESIAN_POINT ( 'NONE',  ( 4.483927247898545687, 16.52544592524342804, 84.79057627198102409 ) ) ;
#123986=CARTESIAN_POINT ( 'NONE',  ( -0.05219959533910754901, -16.53943276465976808, 42.49890960531435979 ) ) ;
#123987=CARTESIAN_POINT ( 'NONE',  ( 19.05341960407617918, -5.049401038297876454, 81.04275706135231871 ) ) ;
#123988=CARTESIAN_POINT ( 'NONE',  ( -10.81492255796105439, 18.62759615963255655, 57.91775706135234714 ) ) ;
#123989=CARTESIAN_POINT ( 'NONE',  ( -19.02544592524334988, -5.153800228976617603, 28.95942372801900433 ) ) ;
#123990=CARTESIAN_POINT ( 'NONE',  ( 12.14591786802309770, 12.06949235617756955, 104.3739096053143669 ) ) ;
#123991=CARTESIAN_POINT ( 'NONE',  ( -0.05219959533907301413, -21.53943276465977519, 37.49890960531436690 ) ) ;
#123992=CARTESIAN_POINT ( 'NONE',  ( -16.53943276465976808, 0.05219959533911058130, 21.24890960531436690 ) ) ;
#123993=CARTESIAN_POINT ( 'NONE',  ( -21.52544592524334988, -5.823673210054445271, 98.95942372801903275 ) ) ;
#123994=CARTESIAN_POINT ( 'NONE',  ( 0.05219959533934541429, -16.53943276465976808, 55.00109039468568284 ) ) ;
#123995=CARTESIAN_POINT ( 'NONE',  ( -4.379528057220328563, 16.55341960407611168, 30.20724293864769550 ) ) ;
#123996=CARTESIAN_POINT ( 'NONE',  ( -21.52544592524334988, -5.823673210054445271, 68.95942372801901854 ) ) ;
#123997=CARTESIAN_POINT ( 'NONE',  ( -5.719274019375665041, -21.55341960407619695, 49.79275706135234714 ) ) ;
#123998=VERTEX_POINT ( 'NONE', #60896 ) ;
#123999=CARTESIAN_POINT ( 'NONE',  ( -9.564922557960796823, -16.46253265017161027, 22.08224293864768839 ) ) ;
#124000=CARTESIAN_POINT ( 'NONE',  ( 15.80617190586769283, -15.72974639402175789, 35.62609039468568994 ) ) ;
#124001=CARTESIAN_POINT ( 'NONE',  ( -14.29746914071049879, 8.314922557960819915, 100.8322429386477097 ) ) ;
#124002=CARTESIAN_POINT ( 'NONE',  ( 16.51473224551069308, 9.474510206698969483, 29.16557627198103475 ) ) ;
#124003=CARTESIAN_POINT ( 'NONE',  ( -8.314922557960811034, -14.29746914071050412, 82.08224293864768129 ) ) ;
#124004=CARTESIAN_POINT ( 'NONE',  ( -13.89961937509977652, 13.97604488694528158, 75.62390960531438111 ) ) ;
#124005=CARTESIAN_POINT ( 'NONE',  ( -14.34966873604960291, -8.224510206698953496, 31.66557627198102054 ) ) ;
#124006=CARTESIAN_POINT ( 'NONE',  ( -21.53943276465977519, 0.05219959533907696930, 61.24890960531435979 ) ) ;
#124007=CARTESIAN_POINT ( 'NONE',  ( -12.14591786802309592, -12.06949235617757132, 86.87390960531438111 ) ) ;
#124008=CARTESIAN_POINT ( 'NONE',  ( -15.72974639402197994, 15.80617190586746368, 90.62390960531436690 ) ) ;
#124009=CARTESIAN_POINT ( 'NONE',  ( 5.049401038298161559, -19.05341960407611168, 102.7072429386476955 ) ) ;
#124010=CARTESIAN_POINT ( 'NONE',  ( -9.564922557960796823, -16.46253265017161027, 47.08224293864769550 ) ) ;
#124011=CARTESIAN_POINT ( 'NONE',  ( 19.02544592524334988, 5.153800228976608722, 101.4594237280189759 ) ) ;
#124012=CARTESIAN_POINT ( 'NONE',  ( -10.72451020669898014, 18.67979575497178502, 40.41557627198103120 ) ) ;
#124013=CARTESIAN_POINT ( 'NONE',  ( 18.67979575497194134, -10.72451020669871369, 85.83442372801901854 ) ) ;
#124014=CARTESIAN_POINT ( 'NONE',  ( -19.02544592524342804, 5.153800228976336051, 66.04057627198103830 ) ) ;
#124016=CARTESIAN_POINT ( 'NONE',  ( -16.51473224551069308, -9.474510206698971260, 96.66557627198102409 ) ) ;
#124017=CARTESIAN_POINT ( 'NONE',  ( -14.29746914071037622, -8.314922557961029526, 74.16775706135231871 ) ) ;
#124018=CARTESIAN_POINT ( 'NONE',  ( 10.81492255796106328, -18.62759615963255655, 60.41775706135235424 ) ) ;
#124019=CARTESIAN_POINT ( 'NONE',  ( 5.823673210054444382, -21.52544592524334988, 80.20942372801901854 ) ) ;
#124020=CARTESIAN_POINT ( 'NONE',  ( 15.72974639402199770, -15.80617190586745480, 103.1239096053143811 ) ) ;
#124021=CARTESIAN_POINT ( 'NONE',  ( 10.72451020669871369, 18.67979575497193778, 42.08442372801901854 ) ) ;
#124022=CARTESIAN_POINT ( 'NONE',  ( 16.55341960407618274, -4.379528057220086978, 76.04275706135237556 ) ) ;
#124023=CARTESIAN_POINT ( 'NONE',  ( 18.62759615963271287, -10.81492255796078972, 78.33224293864770971 ) ) ;
#124024=CARTESIAN_POINT ( 'NONE',  ( 9.564922557961047289, -16.46253265017146816, 35.41775706135233293 ) ) ;
#124025=CARTESIAN_POINT ( 'NONE',  ( -15.72974639402197994, 15.80617190586746368, 45.62390960531436690 ) ) ;
#124026=CARTESIAN_POINT ( 'NONE',  ( -19.05341960407611168, -5.049401038298163336, 86.45724293864769550 ) ) ;
#124027=CARTESIAN_POINT ( 'NONE',  ( -16.53943276465976808, -0.05219959533934237506, 113.7510903946856757 ) ) ;
#124029=CARTESIAN_POINT ( 'NONE',  ( -5.153800228976328057, -19.02544592524343514, 102.2905762719810383 ) ) ;
#124031=CARTESIAN_POINT ( 'NONE',  ( -9.474510206698720793, -16.51473224551083518, 94.58442372801900433 ) ) ;
#124032=CARTESIAN_POINT ( 'NONE',  ( -5.719274019375978568, 21.55341960407610458, 75.20724293864769550 ) ) ;
#124033=CARTESIAN_POINT ( 'NONE',  ( 4.379528057220339221, -16.55341960407611168, 42.70724293864770260 ) ) ;
#124034=CARTESIAN_POINT ( 'NONE',  ( 16.51473224551083163, -9.474510206698727899, 110.8344237280190043 ) ) ;
#124035=CARTESIAN_POINT ( 'NONE',  ( -19.05341960407611168, -5.049401038298163336, 31.45724293864769550 ) ) ;
#124036=CARTESIAN_POINT ( 'NONE',  ( -16.46253265017146816, -9.564922557961047289, 109.1677570613523471 ) ) ;
#124037=CARTESIAN_POINT ( 'NONE',  ( -21.53943276465977519, 0.05219959533907696930, 106.2489096053143811 ) ) ;
#124038=CARTESIAN_POINT ( 'NONE',  ( -9.564922557961040184, 16.46253265017147172, 72.91775706135233293 ) ) ;
#124039=CARTESIAN_POINT ( 'NONE',  ( 16.53943276465976808, 0.05219959533934440121, 86.25109039468568994 ) ) ;
#124040=CARTESIAN_POINT ( 'NONE',  ( 19.05341960407611168, 5.049401038298154454, 73.95724293864768129 ) ) ;
#124041=CARTESIAN_POINT ( 'NONE',  ( -8.314922557960811034, -14.29746914071050412, 82.08224293864768129 ) ) ;
#124043=CARTESIAN_POINT ( 'NONE',  ( -9.474510206698964154, 16.51473224551069663, 60.41557627198102409 ) ) ;
#124044=CARTESIAN_POINT ( 'NONE',  ( 12.14591786802309770, 12.06949235617756955, 64.37390960531435269 ) ) ;
#124045=CARTESIAN_POINT ( 'NONE',  ( 13.97604488694527802, 13.89961937509977652, 34.37390960531436690 ) ) ;
#124047=CARTESIAN_POINT ( 'NONE',  ( -4.379528057220328563, 16.55341960407611168, 40.20724293864769550 ) ) ;
#124048=CARTESIAN_POINT ( 'NONE',  ( 5.049401038298161559, -19.05341960407611168, 72.70724293864768129 ) ) ;
#124050=CARTESIAN_POINT ( 'NONE',  ( 19.03943276465977164, 0.05219959533936151252, 46.25109039468566863 ) ) ;
#124051=CARTESIAN_POINT ( 'NONE',  ( -16.55341960407617563, 4.379528057220093196, 58.54275706135235424 ) ) ;
#124052=CARTESIAN_POINT ( 'NONE',  ( -21.55341960407610458, -5.719274019375992779, 66.45724293864768129 ) ) ;
#124053=CARTESIAN_POINT ( 'NONE',  ( 16.46253265017146816, 9.564922557961045513, 26.66775706135234003 ) ) ;
#124054=CARTESIAN_POINT ( 'NONE',  ( 9.474510206698971260, -16.51473224551069308, 82.91557627198103830 ) ) ;
#124055=CARTESIAN_POINT ( 'NONE',  ( 17.50000000000000000, -5.500000000000000888, 118.0000000000000142 ) ) ;
#124056=CARTESIAN_POINT ( 'NONE',  ( -0.05219959533907301413, -21.53943276465977519, 32.49890960531435979 ) ) ;
#124057=CARTESIAN_POINT ( 'NONE',  ( -5.153800228976328057, -19.02544592524343514, 57.29057627198103120 ) ) ;
#124058=CARTESIAN_POINT ( 'NONE',  ( -10.81492255796105439, 18.62759615963255655, 57.91775706135234714 ) ) ;
#124059=CARTESIAN_POINT ( 'NONE',  ( 14.34966873604960469, 8.224510206698951720, 109.1655762719810383 ) ) ;
#124060=CARTESIAN_POINT ( 'NONE',  ( -5.719274019375978568, 21.55341960407610458, 105.2072429386477097 ) ) ;
#124061=CARTESIAN_POINT ( 'NONE',  ( -0.05219959533909027116, -19.03943276465977164, 92.49890960531436690 ) ) ;
#124063=CARTESIAN_POINT ( 'NONE',  ( 15.80617190586769283, -15.72974639402175789, 40.62609039468567573 ) ) ;
#124064=ORIENTED_EDGE ( 'NONE', *, *, #141141, .F. ) ;
#124065=CARTESIAN_POINT ( 'NONE',  ( -0.05219959533909027116, -19.03943276465977164, 92.49890960531436690 ) ) ;
#124066=CARTESIAN_POINT ( 'NONE',  ( 19.48894818550247265, -5.499999999999913847, 82.60307310435241845 ) ) ;
#124067=CARTESIAN_POINT ( 'NONE',  ( 5.719274019375991003, -21.55341960407610458, 97.70724293864772392 ) ) ;
#124068=CARTESIAN_POINT ( 'NONE',  ( 9.474510206698971260, -16.51473224551069308, 52.91557627198102409 ) ) ;
#124069=CARTESIAN_POINT ( 'NONE',  ( -8.314922557961024197, 14.29746914071037800, 27.91775706135234358 ) ) ;
#124072=CARTESIAN_POINT ( 'NONE',  ( -5.049401038298153566, 19.05341960407611168, 35.20724293864768839 ) ) ;
#124073=CARTESIAN_POINT ( 'NONE',  ( -15.80617190586768217, 15.72974639402176855, 83.12609039468568994 ) ) ;
#124074=CARTESIAN_POINT ( 'NONE',  ( 9.564922557960805705, 16.46253265017160317, 69.58224293864770971 ) ) ;
#124075=CARTESIAN_POINT ( 'NONE',  ( -10.72451020669870658, -18.67979575497194134, 44.58442372801901854 ) ) ;
#124076=CARTESIAN_POINT ( 'NONE',  ( -18.62759615963255300, -10.81492255796106328, 24.16775706135235424 ) ) ;
#124078=CARTESIAN_POINT ( 'NONE',  ( -16.46253265017160317, 9.564922557960807481, 105.8322429386476955 ) ) ;
#124080=CARTESIAN_POINT ( 'NONE',  ( -12.06949235617739369, -12.14591786802326823, 39.37609039468567573 ) ) ;
#124081=CARTESIAN_POINT ( 'NONE',  ( -8.224510206698735004, -14.34966873604973081, 64.58442372801900433 ) ) ;
#124082=CARTESIAN_POINT ( 'NONE',  ( -18.67979575497193778, 10.72451020669871902, 43.33442372801901143 ) ) ;
#124083=CARTESIAN_POINT ( 'NONE',  ( -0.05219959533937732626, 21.53943276465977519, 72.50109039468568994 ) ) ;
#124087=CARTESIAN_POINT ( 'NONE',  ( -19.03943276465977164, -0.05219959533935918106, 113.7510903946856757 ) ) ;
#124088=CARTESIAN_POINT ( 'NONE',  ( -16.46253265017160317, 9.564922557960807481, 60.83224293864769550 ) ) ;
#124089=CARTESIAN_POINT ( 'NONE',  ( -5.049401038298153566, 19.05341960407611168, 95.20724293864770971 ) ) ;
#124090=CARTESIAN_POINT ( 'NONE',  ( -4.483927247898539470, -16.52544592524342804, 112.2905762719810241 ) ) ;
#124091=CARTESIAN_POINT ( 'NONE',  ( 16.55341960407611168, 4.379528057220329451, 98.95724293864770971 ) ) ;
#124092=CARTESIAN_POINT ( 'NONE',  ( 18.67979575497178502, 10.72451020669898547, 29.16557627198103120 ) ) ;
#124093=CARTESIAN_POINT ( 'NONE',  ( 16.55341960407618274, -4.379528057220086978, 81.04275706135236135 ) ) ;
#124094=CARTESIAN_POINT ( 'NONE',  ( 8.314922557960818139, 14.29746914071049879, 69.58224293864769550 ) ) ;
#124095=CARTESIAN_POINT ( 'NONE',  ( 9.564922557960805705, 16.46253265017160317, 49.58224293864770260 ) ) ;
#124096=CARTESIAN_POINT ( 'NONE',  ( -5.719274019375665041, -21.55341960407619695, 79.79275706135236135 ) ) ;
#124097=CARTESIAN_POINT ( 'NONE',  ( -21.53943276465977519, -0.05219959533937600094, 68.75109039468568994 ) ) ;
#124098=CARTESIAN_POINT ( 'NONE',  ( -0.05219959533936034679, 19.03943276465977164, 112.5010903946856757 ) ) ;
#124099=CARTESIAN_POINT ( 'NONE',  ( 4.379528057220339221, -16.55341960407611168, 77.70724293864770971 ) ) ;
#124100=CARTESIAN_POINT ( 'NONE',  ( -21.53943276465977519, -0.05219959533937600094, 33.75109039468568284 ) ) ;
#124101=CARTESIAN_POINT ( 'NONE',  ( -10.72451020669898014, 18.67979575497178502, 55.41557627198102409 ) ) ;
#124102=CARTESIAN_POINT ( 'NONE',  ( -17.49999999999999645, -5.624438216177586547, 104.1832965508535693 ) ) ;
#124104=CARTESIAN_POINT ( 'NONE',  ( -9.474510206698964154, 16.51473224551069663, 75.41557627198103830 ) ) ;
#124105=CARTESIAN_POINT ( 'NONE',  ( 4.379528057220339221, -16.55341960407611168, 47.70724293864770260 ) ) ;
#124107=CARTESIAN_POINT ( 'NONE',  ( -8.224510206698948167, 14.34966873604960824, 25.41557627198103120 ) ) ;
#124108=CARTESIAN_POINT ( 'NONE',  ( -4.483927247898782831, 16.52544592524335698, 102.7094237280190185 ) ) ;
#124109=CARTESIAN_POINT ( 'NONE',  ( 16.46253265017146816, 9.564922557961045513, 51.66775706135233293 ) ) ;
#124111=CARTESIAN_POINT ( 'NONE',  ( -19.03943276465977164, 0.05219959533909376836, 111.2489096053143669 ) ) ;
#124112=CARTESIAN_POINT ( 'NONE',  ( -4.379528057220328563, 16.55341960407611168, 70.20724293864769550 ) ) ;
#124113=CARTESIAN_POINT ( 'NONE',  ( 13.97604488694548053, -13.89961937509957401, 40.62609039468564731 ) ) ;
#124114=CARTESIAN_POINT ( 'NONE',  ( -5.153800228976328057, -19.02544592524343514, 32.29057627198102409 ) ) ;
#124115=CARTESIAN_POINT ( 'NONE',  ( -0.05219959533907301413, -21.53943276465977519, 42.49890960531435979 ) ) ;
#124116=CARTESIAN_POINT ( 'NONE',  ( 5.719274019375991003, -21.55341960407610458, 52.70724293864769550 ) ) ;
#124118=CARTESIAN_POINT ( 'NONE',  ( 12.14591786802309770, 12.06949235617756955, 99.37390960531436690 ) ) ;
#124119=CARTESIAN_POINT ( 'NONE',  ( 12.06949235617739724, 12.14591786802326823, 46.87609039468568994 ) ) ;
#124121=CARTESIAN_POINT ( 'NONE',  ( 14.29746914071049879, -8.314922557960816363, 98.33224293864769550 ) ) ;
#124122=CARTESIAN_POINT ( 'NONE',  ( 17.13100169013301510, -6.664070546373149107, 38.26789835699850073 ) ) ;
#124124=CARTESIAN_POINT ( 'NONE',  ( 0.05219959533907565091, 21.53943276465977519, 24.99890960531435624 ) ) ;
#124127=ORIENTED_EDGE ( 'NONE', *, *, #165748, .T. ) ;
#124128=CARTESIAN_POINT ( 'NONE',  ( 16.52544592524335698, 4.483927247898782831, 36.45942372801901143 ) ) ;
#124129=CARTESIAN_POINT ( 'NONE',  ( -14.29746914071049879, 8.314922557960819915, 35.83224293864768839 ) ) ;
#124130=CARTESIAN_POINT ( 'NONE',  ( 5.823673210054125526, 21.52544592524343514, 54.79057627198104541 ) ) ;
#124131=CARTESIAN_POINT ( 'NONE',  ( 19.05341960407617918, -5.049401038297876454, 91.04275706135234714 ) ) ;
#124132=CARTESIAN_POINT ( 'NONE',  ( 15.72974639402199770, -15.80617190586745480, 68.12390960531436690 ) ) ;
#124133=CARTESIAN_POINT ( 'NONE',  ( 15.80617190586769283, -15.72974639402175789, 85.62609039468568994 ) ) ;
#124135=CARTESIAN_POINT ( 'NONE',  ( -4.379528057220086978, -16.55341960407618274, 44.79275706135234714 ) ) ;
#124136=CARTESIAN_POINT ( 'NONE',  ( 19.05341960407611168, 5.049401038298154454, 33.95724293864769550 ) ) ;
#124137=CARTESIAN_POINT ( 'NONE',  ( 16.51473224551069308, 9.474510206698969483, 99.16557627198102409 ) ) ;
#124138=CARTESIAN_POINT ( 'NONE',  ( 0.05219959533909260263, 19.03943276465977164, 29.99890960531435979 ) ) ;
#124139=CARTESIAN_POINT ( 'NONE',  ( -16.55341960407611168, -4.379528057220339221, 101.4572429386476955 ) ) ;
#124141=CARTESIAN_POINT ( 'NONE',  ( 9.564922557960805705, 16.46253265017160317, 99.58224293864770971 ) ) ;
#124143=CARTESIAN_POINT ( 'NONE',  ( 16.52544592524335698, 4.483927247898782831, 61.45942372801901854 ) ) ;
#124144=CARTESIAN_POINT ( 'NONE',  ( -21.52544592524343514, 5.823673210054127303, 86.04057627198102409 ) ) ;
#124145=CARTESIAN_POINT ( 'NONE',  ( 13.89961937509977652, -13.97604488694527269, 63.12390960531435979 ) ) ;
#124146=CARTESIAN_POINT ( 'NONE',  ( -18.67979575497193778, 10.72451020669871902, 28.33442372801902209 ) ) ;
#124147=CARTESIAN_POINT ( 'NONE',  ( 19.05341960407611168, 5.049401038298154454, 88.95724293864769550 ) ) ;
#124149=ORIENTED_EDGE ( 'NONE', *, *, #128318, .T. ) ;
#124150=CARTESIAN_POINT ( 'NONE',  ( -21.53943276465977519, 0.05219959533907696930, 111.2489096053143669 ) ) ;
#124151=CARTESIAN_POINT ( 'NONE',  ( 5.153800228976335163, 19.02544592524342804, 29.79057627198102409 ) ) ;
#124152=CARTESIAN_POINT ( 'NONE',  ( -19.03943276465977164, 0.05219959533909376836, 111.2489096053143669 ) ) ;
#124153=CARTESIAN_POINT ( 'NONE',  ( 16.51473224551083163, -9.474510206698727899, 80.83442372801899012 ) ) ;
#124154=CARTESIAN_POINT ( 'NONE',  ( 16.46253265017146816, 9.564922557961045513, 26.66775706135234003 ) ) ;
#124155=CARTESIAN_POINT ( 'NONE',  ( 21.52544592524344225, -5.823673210054117533, 98.54057627198105251 ) ) ;
#124156=CARTESIAN_POINT ( 'NONE',  ( 0.05219959533936267826, -19.03943276465977164, 40.00109039468566152 ) ) ;
#124157=CARTESIAN_POINT ( 'NONE',  ( -14.29746914071037622, -8.314922557961029526, 74.16775706135231871 ) ) ;
#124158=CARTESIAN_POINT ( 'NONE',  ( -16.46253265017160317, 9.564922557960807481, 110.8322429386476955 ) ) ;
#124159=CARTESIAN_POINT ( 'NONE',  ( 13.97604488694527802, 13.89961937509977652, 59.37390960531434558 ) ) ;
#124160=CARTESIAN_POINT ( 'NONE',  ( -18.62759615963255300, -10.81492255796106328, 69.16775706135234714 ) ) ;
#124161=CARTESIAN_POINT ( 'NONE',  ( 21.52544592524334988, 5.823673210054432836, 81.45942372801900433 ) ) ;
#124162=CARTESIAN_POINT ( 'NONE',  ( -19.02544592524342804, 5.153800228976336051, 81.04057627198103830 ) ) ;
#124163=CARTESIAN_POINT ( 'NONE',  ( 5.719274019375673035, 21.55341960407619339, 42.29275706135235424 ) ) ;
#124164=CARTESIAN_POINT ( 'NONE',  ( 19.02544592524334988, 5.153800228976608722, 86.45942372801900433 ) ) ;
#124165=CARTESIAN_POINT ( 'NONE',  ( -16.51473224551069308, -9.474510206698971260, 56.66557627198103120 ) ) ;
#124166=CARTESIAN_POINT ( 'NONE',  ( 9.474510206698971260, -16.51473224551069308, 97.91557627198102409 ) ) ;
#124167=CARTESIAN_POINT ( 'NONE',  ( 13.89961937509977652, -13.97604488694527269, 63.12390960531435979 ) ) ;
#124168=CARTESIAN_POINT ( 'NONE',  ( 9.564922557960805705, 16.46253265017160317, 109.5822429386476955 ) ) ;
#124169=CARTESIAN_POINT ( 'NONE',  ( 19.03943276465977164, -0.05219959533909143690, 53.74890960531436690 ) ) ;
#124171=CARTESIAN_POINT ( 'NONE',  ( 5.823673210054125526, 21.52544592524343514, 104.7905762719810241 ) ) ;
#124172=CARTESIAN_POINT ( 'NONE',  ( -4.483927247898782831, 16.52544592524335698, 67.70942372801901854 ) ) ;
#124174=CARTESIAN_POINT ( 'NONE',  ( -5.153800228976607833, 19.02544592524334988, 42.70942372801901143 ) ) ;
#124175=CARTESIAN_POINT ( 'NONE',  ( 5.049401038298161559, -19.05341960407611168, 67.70724293864769550 ) ) ;
#124176=CARTESIAN_POINT ( 'NONE',  ( -12.14591786802309592, -12.06949235617757132, 56.87390960531436690 ) ) ;
#124177=CARTESIAN_POINT ( 'NONE',  ( 14.34966873604960469, 8.224510206698951720, 89.16557627198102409 ) ) ;
#124178=CARTESIAN_POINT ( 'NONE',  ( 19.03943276465977164, -0.05219959533909143690, 103.7489096053143669 ) ) ;
#124179=CARTESIAN_POINT ( 'NONE',  ( -19.02544592524342804, 5.153800228976336051, 86.04057627198103830 ) ) ;
#124180=CARTESIAN_POINT ( 'NONE',  ( 0.05219959533909260263, 19.03943276465977164, 109.9989096053143669 ) ) ;
#124182=CARTESIAN_POINT ( 'NONE',  ( 15.72974639402176855, 15.80617190586768217, 106.8760903946856899 ) ) ;
#124183=CARTESIAN_POINT ( 'NONE',  ( 8.224510206698742110, 14.34966873604972548, 87.08442372801901854 ) ) ;
#124184=CARTESIAN_POINT ( 'NONE',  ( -19.03943276465977164, 0.05219959533909376836, 81.24890960531436690 ) ) ;
#124185=CARTESIAN_POINT ( 'NONE',  ( -21.52544592524334988, -5.823673210054445271, 38.95942372801901854 ) ) ;
#124186=CARTESIAN_POINT ( 'NONE',  ( -10.81492255796078084, -18.62759615963271287, 37.08224293864768129 ) ) ;
#124187=CARTESIAN_POINT ( 'NONE',  ( -5.719274019375978568, 21.55341960407610458, 100.2072429386476955 ) ) ;
#124188=CARTESIAN_POINT ( 'NONE',  ( -8.314922557960811034, -14.29746914071050412, 62.08224293864769550 ) ) ;
#124189=CARTESIAN_POINT ( 'NONE',  ( 5.153800228976335163, 19.02544592524342804, 54.79057627198103120 ) ) ;
#124190=CARTESIAN_POINT ( 'NONE',  ( 12.14591786802309770, 12.06949235617756955, 79.37390960531436690 ) ) ;
#124191=CARTESIAN_POINT ( 'NONE',  ( -13.89961937509957401, -13.97604488694547875, 49.37609039468567573 ) ) ;
#124193=CARTESIAN_POINT ( 'NONE',  ( 14.29746914071049879, -8.314922557960816363, 108.3322429386477097 ) ) ;
#124194=CARTESIAN_POINT ( 'NONE',  ( 12.14591786802327356, -12.06949235617739191, 65.62609039468568994 ) ) ;
#124195=CARTESIAN_POINT ( 'NONE',  ( -16.51473224551069308, -9.474510206698971260, 81.66557627198103830 ) ) ;
#124197=CARTESIAN_POINT ( 'NONE',  ( 16.53943276465976808, -0.05219959533910856209, 103.7489096053143669 ) ) ;
#124198=CARTESIAN_POINT ( 'NONE',  ( 15.80617190586746368, 15.72974639402197994, 39.37390960531436690 ) ) ;
#124200=CARTESIAN_POINT ( 'NONE',  ( -8.314922557961024197, 14.29746914071037800, 102.9177570613523756 ) ) ;
#124201=CARTESIAN_POINT ( 'NONE',  ( -16.55341960407617563, 4.379528057220093196, 33.54275706135234714 ) ) ;
#124202=CARTESIAN_POINT ( 'NONE',  ( 18.67979575497194134, -10.72451020669871369, 90.83442372801901854 ) ) ;
#124203=CARTESIAN_POINT ( 'NONE',  ( -19.05341960407611168, -5.049401038298163336, 86.45724293864769550 ) ) ;
#124204=CARTESIAN_POINT ( 'NONE',  ( -10.72451020669870658, -18.67979575497194134, 24.58442372801901499 ) ) ;
#124205=CARTESIAN_POINT ( 'NONE',  ( -13.89961937509977652, 13.97604488694528158, 35.62390960531435269 ) ) ;
#124206=CARTESIAN_POINT ( 'NONE',  ( -12.06949235617739369, -12.14591786802326823, 29.37609039468568284 ) ) ;
#124207=EDGE_CURVE ( 'NONE', #175270, #148926, #77064, .T. ) ;
#124209=CARTESIAN_POINT ( 'NONE',  ( 16.51473224551083163, -9.474510206698727899, 90.83442372801900433 ) ) ;
#124210=CARTESIAN_POINT ( 'NONE',  ( -18.62759615963270932, 10.81492255796079327, 85.83224293864768129 ) ) ;
#124211=CARTESIAN_POINT ( 'NONE',  ( 5.049401038297881783, 19.05341960407617563, 67.29275706135234714 ) ) ;
#124213=CARTESIAN_POINT ( 'NONE',  ( -21.53943276465977519, -0.05219959533937600094, 23.75109039468567929 ) ) ;
#124215=CARTESIAN_POINT ( 'NONE',  ( -19.05341960407611168, -5.049401038298163336, 91.45724293864766707 ) ) ;
#124217=CARTESIAN_POINT ( 'NONE',  ( 16.55341960407618274, -4.379528057220086978, 31.04275706135234714 ) ) ;
#124219=CARTESIAN_POINT ( 'NONE',  ( 16.46253265017146816, 9.564922557961045513, 66.66775706135233293 ) ) ;
#124220=CARTESIAN_POINT ( 'NONE',  ( -18.62759615963270932, 10.81492255796079327, 115.8322429386477097 ) ) ;
#124221=CARTESIAN_POINT ( 'NONE',  ( 12.14591786802309770, 12.06949235617756955, 84.37390960531438111 ) ) ;
#124222=CARTESIAN_POINT ( 'NONE',  ( 19.03943276465977164, -0.05219959533909143690, 88.74890960531436690 ) ) ;
#124224=CARTESIAN_POINT ( 'NONE',  ( -14.34966873604972548, 8.224510206698743886, 53.33442372801901854 ) ) ;
#124225=CARTESIAN_POINT ( 'NONE',  ( 5.153800228976615827, -19.02544592524334988, 60.20942372801899012 ) ) ;
#124226=CARTESIAN_POINT ( 'NONE',  ( 10.72451020669871369, 18.67979575497193778, 67.08442372801901854 ) ) ;
#124227=CARTESIAN_POINT ( 'NONE',  ( 16.52544592524335698, 4.483927247898782831, 26.45942372801901854 ) ) ;
#124228=CARTESIAN_POINT ( 'NONE',  ( 0.05219959533909260263, 19.03943276465977164, 74.99890960531435269 ) ) ;
#124229=CARTESIAN_POINT ( 'NONE',  ( -5.049401038297874678, -19.05341960407617918, 84.79275706135233293 ) ) ;
#124230=CARTESIAN_POINT ( 'NONE',  ( -12.06949235617739369, -12.14591786802326823, 54.37609039468568994 ) ) ;
#124231=CARTESIAN_POINT ( 'NONE',  ( -18.62759615963255300, -10.81492255796106328, 104.1677570613523471 ) ) ;
#124232=CARTESIAN_POINT ( 'NONE',  ( 13.97604488694548053, -13.89961937509957401, 65.62609039468567573 ) ) ;
#124233=CARTESIAN_POINT ( 'NONE',  ( -16.51473224551069308, -9.474510206698971260, 51.66557627198102409 ) ) ;
#124234=CARTESIAN_POINT ( 'NONE',  ( 21.53943276465977519, -0.05219959533907433946, 68.74890960531435269 ) ) ;
#124235=CARTESIAN_POINT ( 'NONE',  ( -8.224510206698948167, 14.34966873604960824, 60.41557627198102409 ) ) ;
#124236=CARTESIAN_POINT ( 'NONE',  ( 5.153800228976615827, -19.02544592524334988, 75.20942372801896170 ) ) ;
#124237=DIRECTION ( 'NONE',  ( 8.673617379884027583E-16, 0.000000000000000000, -1.000000000000000000 ) ) ;
#124238=CARTESIAN_POINT ( 'NONE',  ( -9.564922557961040184, 16.46253265017147172, 37.91775706135233293 ) ) ;
#124240=CARTESIAN_POINT ( 'NONE',  ( -0.05219959533934338120, 16.53943276465976808, 102.5010903946856899 ) ) ;
#124241=CARTESIAN_POINT ( 'NONE',  ( -4.379528057220328563, 16.55341960407611168, 65.20724293864768129 ) ) ;
#124242=CARTESIAN_POINT ( 'NONE',  ( -5.823673210054431948, 21.52544592524334988, 107.7094237280190328 ) ) ;
#124244=CARTESIAN_POINT ( 'NONE',  ( -21.55341960407610458, -5.719274019375992779, 96.45724293864770971 ) ) ;
#124245=CARTESIAN_POINT ( 'NONE',  ( -19.03943276465977164, 0.05219959533909376836, 61.24890960531436690 ) ) ;
#124246=CARTESIAN_POINT ( 'NONE',  ( -0.05219959533937732626, 21.53943276465977519, 72.50109039468568994 ) ) ;
#124247=CARTESIAN_POINT ( 'NONE',  ( 13.97604488694527802, 13.89961937509977652, 54.37390960531435979 ) ) ;
#124249=CARTESIAN_POINT ( 'NONE',  ( -9.474510206698964154, 16.51473224551069663, 25.41557627198103120 ) ) ;
#124250=CARTESIAN_POINT ( 'NONE',  ( 5.153800228976335163, 19.02544592524342804, 109.7905762719810099 ) ) ;
#124251=CARTESIAN_POINT ( 'NONE',  ( -12.14591786802309592, -12.06949235617757132, 71.87390960531438111 ) ) ;
#124252=CARTESIAN_POINT ( 'NONE',  ( -13.89961937509977652, 13.97604488694528158, 35.62390960531435269 ) ) ;
#124253=CARTESIAN_POINT ( 'NONE',  ( -8.314922557960811034, -14.29746914071050412, 82.08224293864768129 ) ) ;
#124255=CARTESIAN_POINT ( 'NONE',  ( -18.62759615963270932, 10.81492255796079327, 90.83224293864769550 ) ) ;
#124256=CARTESIAN_POINT ( 'NONE',  ( 18.67979575497194134, -10.72451020669871369, 35.83442372801901143 ) ) ;
#124257=CARTESIAN_POINT ( 'NONE',  ( -0.05219959533909027116, -19.03943276465977164, 22.49890960531436690 ) ) ;
#124258=CARTESIAN_POINT ( 'NONE',  ( 0.05219959533934541429, -16.53943276465976808, 55.00109039468568284 ) ) ;
#124259=CARTESIAN_POINT ( 'NONE',  ( 21.53943276465977519, -0.05219959533907433946, 83.74890960531435269 ) ) ;
#124260=CARTESIAN_POINT ( 'NONE',  ( 5.049401038297881783, 19.05341960407617563, 22.29275706135233648 ) ) ;
#124261=CARTESIAN_POINT ( 'NONE',  ( -16.46253265017160317, 9.564922557960807481, 110.8322429386476955 ) ) ;
#124262=CARTESIAN_POINT ( 'NONE',  ( 0.05219959533937995610, -21.53943276465977519, 40.00109039468567573 ) ) ;
#124263=CARTESIAN_POINT ( 'NONE',  ( 21.55341960407610458, 5.719274019375980345, 38.95724293864768839 ) ) ;
#124264=CARTESIAN_POINT ( 'NONE',  ( -4.379528057220328563, 16.55341960407611168, 25.20724293864769550 ) ) ;
#124265=CARTESIAN_POINT ( 'NONE',  ( 18.67979575497194134, -10.72451020669871369, 65.83442372801900433 ) ) ;
#124266=CARTESIAN_POINT ( 'NONE',  ( 18.67979575497194134, -10.72451020669871369, 95.83442372801903275 ) ) ;
#124267=CARTESIAN_POINT ( 'NONE',  ( 19.03943276465977164, 0.05219959533936151252, 31.25109039468566863 ) ) ;
#124268=CARTESIAN_POINT ( 'NONE',  ( 4.379528057220092307, 16.55341960407617563, 87.29275706135236135 ) ) ;
#124269=CARTESIAN_POINT ( 'NONE',  ( -18.67979575497193778, 10.72451020669871902, 58.33442372801901143 ) ) ;
#124270=CARTESIAN_POINT ( 'NONE',  ( -19.05341960407611168, -5.049401038298163336, 41.45724293864769550 ) ) ;
#124271=CARTESIAN_POINT ( 'NONE',  ( 10.72451020669871369, 18.67979575497193778, 112.0844237280190185 ) ) ;
#124272=CARTESIAN_POINT ( 'NONE',  ( 21.53943276465977519, -0.05219959533907433946, 28.74890960531435624 ) ) ;
#124273=CARTESIAN_POINT ( 'NONE',  ( -15.72974639402176322, -15.80617190586768395, 24.37609039468567573 ) ) ;
#124274=CARTESIAN_POINT ( 'NONE',  ( 0.05219959533907565091, 21.53943276465977519, 79.99890960531435269 ) ) ;
#124275=CARTESIAN_POINT ( 'NONE',  ( 16.52544592524335698, 4.483927247898782831, 36.45942372801901143 ) ) ;
#124277=CARTESIAN_POINT ( 'NONE',  ( 21.53943276465977519, -0.05219959533907433946, 83.74890960531435269 ) ) ;
#124278=CARTESIAN_POINT ( 'NONE',  ( -8.314922557961024197, 14.29746914071037800, 67.91775706135234714 ) ) ;
#124279=CARTESIAN_POINT ( 'NONE',  ( -4.483927247898539470, -16.52544592524342804, 67.29057627198103830 ) ) ;
#124281=CARTESIAN_POINT ( 'NONE',  ( 0.05219959533936267826, -19.03943276465977164, 90.00109039468567573 ) ) ;
#124283=CARTESIAN_POINT ( 'NONE',  ( 8.224510206698742110, 14.34966873604972548, 37.08442372801901143 ) ) ;
#124284=CARTESIAN_POINT ( 'NONE',  ( -18.67979575497178146, -10.72451020669898902, 111.6655762719810525 ) ) ;
#124285=CARTESIAN_POINT ( 'NONE',  ( -18.62759615963270932, 10.81492255796079327, 70.83224293864770971 ) ) ;
#124286=CARTESIAN_POINT ( 'NONE',  ( -18.62759615963270932, 10.81492255796079327, 35.83224293864768839 ) ) ;
#124287=CARTESIAN_POINT ( 'NONE',  ( -8.314922557961024197, 14.29746914071037800, 57.91775706135234714 ) ) ;
#124288=CARTESIAN_POINT ( 'NONE',  ( 9.564922557960805705, 16.46253265017160317, 69.58224293864770971 ) ) ;
#124289=CARTESIAN_POINT ( 'NONE',  ( 15.80617190586769283, -15.72974639402175789, 40.62609039468567573 ) ) ;
#124290=CARTESIAN_POINT ( 'NONE',  ( 13.89961937509957401, 13.97604488694547697, 106.8760903946856757 ) ) ;
#124291=CARTESIAN_POINT ( 'NONE',  ( 5.719274019375991003, -21.55341960407610458, 32.70724293864770260 ) ) ;
#124292=CARTESIAN_POINT ( 'NONE',  ( 13.89961937509957401, 13.97604488694547697, 31.87609039468566863 ) ) ;
#124293=CARTESIAN_POINT ( 'NONE',  ( 0.05219959533934541429, -16.53943276465976808, 45.00109039468568284 ) ) ;
#124294=CARTESIAN_POINT ( 'NONE',  ( -13.89961937509977652, 13.97604488694528158, 105.6239096053143527 ) ) ;
#124295=CARTESIAN_POINT ( 'NONE',  ( -5.823673210054116645, -21.52544592524344225, 107.2905762719810525 ) ) ;
#124296=CARTESIAN_POINT ( 'NONE',  ( -5.049401038298153566, 19.05341960407611168, 75.20724293864769550 ) ) ;
#124297=CARTESIAN_POINT ( 'NONE',  ( -16.81555441253552274, 7.025013491695479395, 25.63685445334257906 ) ) ;
#124298=CARTESIAN_POINT ( 'NONE',  ( 12.06949235617757843, -12.14591786802309237, 78.12390960531436690 ) ) ;
#124299=CARTESIAN_POINT ( 'NONE',  ( -21.52544592524343514, 5.823673210054127303, 26.04057627198103475 ) ) ;
#124300=CARTESIAN_POINT ( 'NONE',  ( 18.22780087662122739, 5.500000000000000888, 71.48236817873106475 ) ) ;
#124301=CARTESIAN_POINT ( 'NONE',  ( -16.52544592524335698, -4.483927247898792601, 68.95942372801901854 ) ) ;
#124302=CARTESIAN_POINT ( 'NONE',  ( 21.55341960407610458, 5.719274019375980345, 108.9572429386476955 ) ) ;
#124303=CARTESIAN_POINT ( 'NONE',  ( -13.89961937509957401, -13.97604488694547875, 69.37609039468564731 ) ) ;
#124304=CARTESIAN_POINT ( 'NONE',  ( -21.55341960407610458, -5.719274019375992779, 26.45724293864768839 ) ) ;
#124305=CARTESIAN_POINT ( 'NONE',  ( 0.05219959533909260263, 19.03943276465977164, 29.99890960531435979 ) ) ;
#124306=CARTESIAN_POINT ( 'NONE',  ( -21.53943276465977519, 0.05219959533907696930, 71.24890960531435269 ) ) ;
#124307=CARTESIAN_POINT ( 'NONE',  ( 19.03943276465977164, -0.05219959533909143690, 98.74890960531436690 ) ) ;
#124308=CARTESIAN_POINT ( 'NONE',  ( -18.67979575497193778, 10.72451020669871902, 98.33442372801901854 ) ) ;
#124309=CARTESIAN_POINT ( 'NONE',  ( 9.474510206698971260, -16.51473224551069308, 47.91557627198102409 ) ) ;
#124310=CARTESIAN_POINT ( 'NONE',  ( 4.379528057220339221, -16.55341960407611168, 87.70724293864769550 ) ) ;
#124311=CARTESIAN_POINT ( 'NONE',  ( -16.55341960407617563, 4.379528057220093196, 38.54275706135234714 ) ) ;
#124312=CARTESIAN_POINT ( 'NONE',  ( -5.153800228976328057, -19.02544592524343514, 62.29057627198100988 ) ) ;
#124313=CARTESIAN_POINT ( 'NONE',  ( -5.719274019375665041, -21.55341960407619695, 79.79275706135236135 ) ) ;
#124314=ORIENTED_EDGE ( 'NONE', *, *, #141568, .F. ) ;
#124315=CARTESIAN_POINT ( 'NONE',  ( -16.51473224551082808, 9.474510206698731452, 43.33442372801900433 ) ) ;
#124316=CARTESIAN_POINT ( 'NONE',  ( -13.97604488694547697, 13.89961937509957934, 38.12609039468566152 ) ) ;
#124317=CARTESIAN_POINT ( 'NONE',  ( -15.80617190586768217, 15.72974639402176855, 38.12609039468567573 ) ) ;
#124318=EDGE_CURVE ( 'NONE', #69839, #165180, #199859, .T. ) ;
#124320=CARTESIAN_POINT ( 'NONE',  ( 13.89961937509957401, 13.97604488694547697, 31.87609039468566863 ) ) ;
#124321=CARTESIAN_POINT ( 'NONE',  ( 9.564922557960805705, 16.46253265017160317, 89.58224293864769550 ) ) ;
#124322=CARTESIAN_POINT ( 'NONE',  ( 19.02544592524343514, -5.153800228976328945, 63.54057627198103830 ) ) ;
#124323=CARTESIAN_POINT ( 'NONE',  ( 8.314922557960818139, 14.29746914071049879, 29.58224293864769905 ) ) ;
#124324=CARTESIAN_POINT ( 'NONE',  ( -10.81492255796078084, -18.62759615963271287, 22.08224293864769194 ) ) ;
#124325=CARTESIAN_POINT ( 'NONE',  ( 21.52544592524334988, 5.823673210054432836, 91.45942372801901854 ) ) ;
#124327=CARTESIAN_POINT ( 'NONE',  ( 16.31925111598457789, 7.325300261831481308, 57.33575461032751974 ) ) ;
#124328=CARTESIAN_POINT ( 'NONE',  ( -0.05219959533937732626, 21.53943276465977519, 97.50109039468567573 ) ) ;
#124329=CARTESIAN_POINT ( 'NONE',  ( 17.05587630539785238, -6.762274262135678171, 43.24180309037312497 ) ) ;
#124330=CARTESIAN_POINT ( 'NONE',  ( 16.46253265017160672, -9.564922557960803928, 113.3322429386476955 ) ) ;
#124332=DIRECTION ( 'NONE',  ( 0.000000000000000000, 0.000000000000000000, -1.000000000000000000 ) ) ;
#124334=CARTESIAN_POINT ( 'NONE',  ( -4.379528057220086978, -16.55341960407618274, 54.79275706135235424 ) ) ;
#124335=CARTESIAN_POINT ( 'NONE',  ( 18.67979575497178502, 10.72451020669898547, 74.16557627198102409 ) ) ;
#124336=CARTESIAN_POINT ( 'NONE',  ( -16.55341960407611168, -4.379528057220339221, 26.45724293864768839 ) ) ;
#124337=CARTESIAN_POINT ( 'NONE',  ( -4.379528057220328563, 16.55341960407611168, 110.2072429386477239 ) ) ;
#124338=CARTESIAN_POINT ( 'NONE',  ( -16.51473224551069308, -9.474510206698971260, 96.66557627198102409 ) ) ;
#124339=CARTESIAN_POINT ( 'NONE',  ( -13.89961937509957401, -13.97604488694547875, 24.37609039468565442 ) ) ;
#124340=CARTESIAN_POINT ( 'NONE',  ( 12.14591786802309770, 12.06949235617756955, 114.3739096053143527 ) ) ;
#124341=CARTESIAN_POINT ( 'NONE',  ( -18.62759615963255300, -10.81492255796106328, 64.16775706135234714 ) ) ;
#124343=CARTESIAN_POINT ( 'NONE',  ( -0.05219959533934338120, 16.53943276465976808, 107.5010903946856899 ) ) ;
#124344=CARTESIAN_POINT ( 'NONE',  ( -16.46253265017146816, -9.564922557961047289, 64.16775706135233293 ) ) ;
#124345=CARTESIAN_POINT ( 'NONE',  ( -13.97604488694547520, 13.89961937509957934, 68.12609039468566152 ) ) ;
#124346=CARTESIAN_POINT ( 'NONE',  ( -5.153800228976328057, -19.02544592524343514, 112.2905762719810099 ) ) ;
#124347=CARTESIAN_POINT ( 'NONE',  ( 4.379528057220339221, -16.55341960407611168, 92.70724293864770971 ) ) ;
#124349=CARTESIAN_POINT ( 'NONE',  ( -9.474510206698720793, -16.51473224551083518, 64.58442372801900433 ) ) ;
#124350=CARTESIAN_POINT ( 'NONE',  ( 19.05341960407611168, 5.049401038298154454, 78.95724293864769550 ) ) ;
#124351=CARTESIAN_POINT ( 'NONE',  ( 0.05219959533910956823, 16.53943276465976808, 59.99890960531436690 ) ) ;
#124352=CARTESIAN_POINT ( 'NONE',  ( 19.03943276465977164, 0.05219959533936151252, 91.25109039468566152 ) ) ;
#124353=CARTESIAN_POINT ( 'NONE',  ( 21.52544592524344225, -5.823673210054117533, 53.54057627198103120 ) ) ;
#124354=ORIENTED_EDGE ( 'NONE', *, *, #154702, .F. ) ;
#124355=CARTESIAN_POINT ( 'NONE',  ( 14.29746914071049879, -8.314922557960816363, 113.3322429386476955 ) ) ;
#124356=CARTESIAN_POINT ( 'NONE',  ( -17.12812012977023812, -6.668231424566067211, 31.35948759323143520 ) ) ;
#124357=CARTESIAN_POINT ( 'NONE',  ( 16.51473224551069308, 9.474510206698969483, 69.16557627198102409 ) ) ;
#124358=CARTESIAN_POINT ( 'NONE',  ( 10.81492255796078972, 18.62759615963270932, 74.58224293864768129 ) ) ;
#124359=CARTESIAN_POINT ( 'NONE',  ( -12.14591786802326823, 12.06949235617739902, 88.12609039468570415 ) ) ;
#124360=CARTESIAN_POINT ( 'NONE',  ( -9.564922557960796823, -16.46253265017161027, 77.08224293864769550 ) ) ;
#124361=CARTESIAN_POINT ( 'NONE',  ( -19.05341960407617563, 5.049401038297882671, 63.54275706135234003 ) ) ;
#124362=CARTESIAN_POINT ( 'NONE',  ( 5.719274019375673035, 21.55341960407619339, 87.29275706135236135 ) ) ;
#124363=CARTESIAN_POINT ( 'NONE',  ( 21.55341960407610458, 5.719274019375980345, 68.95724293864769550 ) ) ;
#124364=CARTESIAN_POINT ( 'NONE',  ( 0.05219959533907565091, 21.53943276465977519, 29.99890960531435979 ) ) ;
#124366=CARTESIAN_POINT ( 'NONE',  ( -13.97604488694527625, -13.89961937509977652, 41.87390960531435979 ) ) ;
#124367=CARTESIAN_POINT ( 'NONE',  ( 16.55341960407618274, -4.379528057220086978, 101.0427570613523756 ) ) ;
#124368=CARTESIAN_POINT ( 'NONE',  ( -9.564922557960796823, -16.46253265017161027, 52.08224293864768839 ) ) ;
#124369=CARTESIAN_POINT ( 'NONE',  ( -16.52544592524335698, -4.483927247898792601, 18.95942372801901143 ) ) ;
#124370=CARTESIAN_POINT ( 'NONE',  ( -16.51473224551082808, 9.474510206698731452, 83.33442372801899012 ) ) ;
#124371=CARTESIAN_POINT ( 'NONE',  ( 19.05341960407617918, -5.049401038297876454, 21.04275706135232582 ) ) ;
#124372=CARTESIAN_POINT ( 'NONE',  ( -16.53943276465976808, 0.05219959533911058130, 66.24890960531436690 ) ) ;
#124373=CARTESIAN_POINT ( 'NONE',  ( -5.823673210054116645, -21.52544592524344225, 92.29057627198103830 ) ) ;
#124374=CARTESIAN_POINT ( 'NONE',  ( 0.05219959533907565091, 21.53943276465977519, 99.99890960531436690 ) ) ;
#124376=CARTESIAN_POINT ( 'NONE',  ( -15.80617190586745835, -15.72974639402198527, 51.87390960531437401 ) ) ;
#124377=CARTESIAN_POINT ( 'NONE',  ( 8.314922557961029526, -14.29746914071037800, 80.41775706135234714 ) ) ;
#124378=CARTESIAN_POINT ( 'NONE',  ( -16.55341960407611168, -4.379528057220339221, 96.45724293864770971 ) ) ;
#124379=CARTESIAN_POINT ( 'NONE',  ( -9.474510206698964154, 16.51473224551069663, 45.41557627198103120 ) ) ;
#124382=CARTESIAN_POINT ( 'NONE',  ( -12.14591786802326823, 12.06949235617739902, 103.1260903946856757 ) ) ;
#124383=CARTESIAN_POINT ( 'NONE',  ( 10.72451020669871369, 18.67979575497193778, 27.08442372801901854 ) ) ;
#124384=CARTESIAN_POINT ( 'NONE',  ( 19.05341960407611168, 5.049401038298154454, 98.95724293864766707 ) ) ;
#124385=CARTESIAN_POINT ( 'NONE',  ( -10.72451020669870658, -18.67979575497194134, 69.58442372801900433 ) ) ;
#124387=CARTESIAN_POINT ( 'NONE',  ( -16.46253265017160317, 9.564922557960807481, 25.83224293864769194 ) ) ;
#124388=ORIENTED_EDGE ( 'NONE', *, *, #62981, .F. ) ;
#124389=CARTESIAN_POINT ( 'NONE',  ( 5.823673210054444382, -21.52544592524334988, 55.20942372801902565 ) ) ;
#124390=CARTESIAN_POINT ( 'NONE',  ( 16.51473224551069308, 9.474510206698969483, 54.16557627198103120 ) ) ;
#124391=CARTESIAN_POINT ( 'NONE',  ( -5.049401038298153566, 19.05341960407611168, 25.20724293864768484 ) ) ;
#124392=CARTESIAN_POINT ( 'NONE',  ( -0.05219959533909027116, -19.03943276465977164, 87.49890960531436690 ) ) ;
#124393=CARTESIAN_POINT ( 'NONE',  ( -9.474510206698720793, -16.51473224551083518, 69.58442372801901854 ) ) ;
#124394=CARTESIAN_POINT ( 'NONE',  ( -21.52544592524334988, -5.823673210054445271, 48.95942372801902565 ) ) ;
#124395=CARTESIAN_POINT ( 'NONE',  ( -13.97604488694547697, 13.89961937509957934, 98.12609039468566152 ) ) ;
#124396=CARTESIAN_POINT ( 'NONE',  ( 19.05341960407617918, -5.049401038297876454, 61.04275706135232582 ) ) ;
#124397=CARTESIAN_POINT ( 'NONE',  ( -13.97604488694527625, -13.89961937509977652, 31.87390960531435979 ) ) ;
#124398=VECTOR ( 'NONE', #165414, 1000.000000000000000 ) ;
#124399=CARTESIAN_POINT ( 'NONE',  ( 4.379528057220092307, 16.55341960407617563, 102.2927570613523613 ) ) ;
#124400=CARTESIAN_POINT ( 'NONE',  ( 16.51473224551083163, -9.474510206698727899, 75.83442372801900433 ) ) ;
#124401=CARTESIAN_POINT ( 'NONE',  ( 14.29746914071049879, -8.314922557960816363, 23.33224293864769194 ) ) ;
#124402=CARTESIAN_POINT ( 'NONE',  ( 19.02544592524334988, 5.153800228976608722, 46.45942372801899012 ) ) ;
#124403=CARTESIAN_POINT ( 'NONE',  ( 5.719274019375673035, 21.55341960407619339, 107.2927570613523471 ) ) ;
#124405=CARTESIAN_POINT ( 'NONE',  ( -19.03943276465977164, -0.05219959533935918106, 28.75109039468566507 ) ) ;
#124406=CARTESIAN_POINT ( 'NONE',  ( -5.049401038298153566, 19.05341960407611168, 25.20724293864768484 ) ) ;
#124407=CARTESIAN_POINT ( 'NONE',  ( -10.72451020669870658, -18.67979575497194134, 84.58442372801903275 ) ) ;
#124408=CARTESIAN_POINT ( 'NONE',  ( -4.379528057220086978, -16.55341960407618274, 34.79275706135235424 ) ) ;
#124409=CARTESIAN_POINT ( 'NONE',  ( -19.05341960407611168, -5.049401038298163336, 96.45724293864769550 ) ) ;
#124411=CARTESIAN_POINT ( 'NONE',  ( 19.03943276465977164, -0.05219959533909143690, 78.74890960531436690 ) ) ;
#124412=CARTESIAN_POINT ( 'NONE',  ( -16.62475595723611477, 7.163666690055877417, 100.5271335181040371 ) ) ;
#124413=CARTESIAN_POINT ( 'NONE',  ( 19.05341960407617918, -5.049401038297876454, 81.04275706135231871 ) ) ;
#124414=CARTESIAN_POINT ( 'NONE',  ( -9.564922557960796823, -16.46253265017161027, 107.0822429386476955 ) ) ;
#124415=CARTESIAN_POINT ( 'NONE',  ( -15.80617190586768217, 15.72974639402176855, 98.12609039468570415 ) ) ;
#124416=CARTESIAN_POINT ( 'NONE',  ( -8.224510206698948167, 14.34966873604960824, 100.4155762719810241 ) ) ;
#124417=CARTESIAN_POINT ( 'NONE',  ( 5.719274019375991003, -21.55341960407610458, 57.70724293864770260 ) ) ;
#124418=CARTESIAN_POINT ( 'NONE',  ( 21.53943276465977519, -0.05219959533907433946, 38.74890960531435979 ) ) ;
#124419=CARTESIAN_POINT ( 'NONE',  ( 12.06949235617757843, -12.14591786802309237, 113.1239096053143953 ) ) ;
#124421=CARTESIAN_POINT ( 'NONE',  ( 19.03943276465977164, 0.05219959533936151252, 51.25109039468567573 ) ) ;
#124422=CARTESIAN_POINT ( 'NONE',  ( 12.14591786802309770, 12.06949235617756955, 39.37390960531436690 ) ) ;
#124423=CARTESIAN_POINT ( 'NONE',  ( 21.53943276465977519, -0.05219959533907433946, 23.74890960531435269 ) ) ;
#124424=CARTESIAN_POINT ( 'NONE',  ( 21.52544592524334988, 5.823673210054432836, 76.45942372801901854 ) ) ;
#124425=CARTESIAN_POINT ( 'NONE',  ( 10.72451020669898902, -18.67979575497178502, 67.91557627198102409 ) ) ;
#124426=CARTESIAN_POINT ( 'NONE',  ( 21.53943276465977519, 0.05219959533937863772, 46.25109039468567573 ) ) ;
#124427=CARTESIAN_POINT ( 'NONE',  ( 5.719274019375991003, -21.55341960407610458, 102.7072429386476955 ) ) ;
#124428=CARTESIAN_POINT ( 'NONE',  ( -5.719274019375665041, -21.55341960407619695, 54.79275706135235424 ) ) ;
#124429=CARTESIAN_POINT ( 'NONE',  ( 19.05341960407611168, 5.049401038298154454, 28.95724293864769550 ) ) ;
#124430=CARTESIAN_POINT ( 'NONE',  ( -16.51473224551069308, -9.474510206698971260, 76.66557627198103830 ) ) ;
#124431=CARTESIAN_POINT ( 'NONE',  ( 16.55341960407618274, -4.379528057220086978, 86.04275706135236135 ) ) ;
#124432=CARTESIAN_POINT ( 'NONE',  ( 8.314922557960818139, 14.29746914071049879, 109.5822429386476955 ) ) ;
#124435=CARTESIAN_POINT ( 'NONE',  ( 16.52544592524342804, -4.483927247898539470, 53.54057627198103120 ) ) ;
#124436=CARTESIAN_POINT ( 'NONE',  ( 16.52544592524335698, 4.483927247898782831, 111.4594237280190328 ) ) ;
#124437=CARTESIAN_POINT ( 'NONE',  ( -0.05219959533909027116, -19.03943276465977164, 72.49890960531435269 ) ) ;
#124438=CARTESIAN_POINT ( 'NONE',  ( -16.46253265017160317, 9.564922557960807481, 30.83224293864769550 ) ) ;
#124439=CARTESIAN_POINT ( 'NONE',  ( -21.52544592524343514, 5.823673210054127303, 41.04057627198103120 ) ) ;
#124440=CARTESIAN_POINT ( 'NONE',  ( -5.153800228976607833, 19.02544592524334988, 42.70942372801901143 ) ) ;
#124442=CARTESIAN_POINT ( 'NONE',  ( -14.34966873604960291, -8.224510206698953496, 46.66557627198102409 ) ) ;
#124443=CARTESIAN_POINT ( 'NONE',  ( 15.80617190586746368, 15.72974639402197994, 29.37390960531435269 ) ) ;
#124444=CARTESIAN_POINT ( 'NONE',  ( 18.62759615963255655, 10.81492255796105972, 56.66775706135235424 ) ) ;
#124446=CARTESIAN_POINT ( 'NONE',  ( 8.224510206698742110, 14.34966873604972548, 67.08442372801901854 ) ) ;
#124447=CARTESIAN_POINT ( 'NONE',  ( -16.46253265017146816, -9.564922557961047289, 59.16775706135233293 ) ) ;
#124448=CARTESIAN_POINT ( 'NONE',  ( 4.379528057220339221, -16.55341960407611168, 47.70724293864770260 ) ) ;
#124450=CARTESIAN_POINT ( 'NONE',  ( -0.05219959533910754901, -16.53943276465976808, 22.49890960531436335 ) ) ;
#124451=CARTESIAN_POINT ( 'NONE',  ( -19.02544592524342804, 5.153800228976336051, 41.04057627198103120 ) ) ;
#124452=CARTESIAN_POINT ( 'NONE',  ( 16.51473224551069308, 9.474510206698969483, 59.16557627198102409 ) ) ;
#124453=CARTESIAN_POINT ( 'NONE',  ( -14.29746914071049879, 8.314922557960819915, 115.8322429386477097 ) ) ;
#124454=CARTESIAN_POINT ( 'NONE',  ( 0.05219959533937995610, -21.53943276465977519, 35.00109039468568284 ) ) ;
#124455=CARTESIAN_POINT ( 'NONE',  ( 5.049401038298161559, -19.05341960407611168, 57.70724293864769550 ) ) ;
#124456=CARTESIAN_POINT ( 'NONE',  ( -17.49999999999999645, -5.499999999999992895, 99.20309617465831309 ) ) ;
#124457=CARTESIAN_POINT ( 'NONE',  ( -13.89961937509977652, 13.97604488694528158, 40.62390960531435979 ) ) ;
#124458=CARTESIAN_POINT ( 'NONE',  ( -10.72451020669898014, 18.67979575497178502, 40.41557627198103120 ) ) ;
#124459=CARTESIAN_POINT ( 'NONE',  ( 18.62759615963255655, 10.81492255796105972, 61.66775706135235424 ) ) ;
#124460=CARTESIAN_POINT ( 'NONE',  ( -4.483927247898539470, -16.52544592524342804, 112.2905762719810241 ) ) ;
#124461=CARTESIAN_POINT ( 'NONE',  ( -10.81492255796078084, -18.62759615963271287, 22.08224293864769194 ) ) ;
#124462=CARTESIAN_POINT ( 'NONE',  ( 4.379528057220092307, 16.55341960407617563, 92.29275706135236135 ) ) ;
#124463=CARTESIAN_POINT ( 'NONE',  ( 5.823673210054444382, -21.52544592524334988, 100.2094237280190043 ) ) ;
#124464=CARTESIAN_POINT ( 'NONE',  ( 4.379528057220092307, 16.55341960407617563, 67.29275706135234714 ) ) ;
#124465=CARTESIAN_POINT ( 'NONE',  ( -5.153800228976328057, -19.02544592524343514, 107.2905762719810383 ) ) ;
#124466=CARTESIAN_POINT ( 'NONE',  ( 8.314922557961029526, -14.29746914071037800, 60.41775706135235424 ) ) ;
#124467=CARTESIAN_POINT ( 'NONE',  ( 4.483927247898790824, -16.52544592524335698, 30.20942372801902565 ) ) ;
#124468=CARTESIAN_POINT ( 'NONE',  ( 4.483927247898790824, -16.52544592524335698, 100.2094237280190043 ) ) ;
#124469=CARTESIAN_POINT ( 'NONE',  ( -21.53943276465977519, -0.05219959533937600094, 53.75109039468568994 ) ) ;
#124470=CARTESIAN_POINT ( 'NONE',  ( 4.483927247898790824, -16.52544592524335698, 30.20942372801902565 ) ) ;
#124471=CARTESIAN_POINT ( 'NONE',  ( 10.81492255796078972, 18.62759615963270932, 104.5822429386477097 ) ) ;
#124472=CARTESIAN_POINT ( 'NONE',  ( 4.483927247898790824, -16.52544592524335698, 20.20942372801900788 ) ) ;
#124473=CARTESIAN_POINT ( 'NONE',  ( -0.05219959533934338120, 16.53943276465976808, 82.50109039468568994 ) ) ;
#124475=CARTESIAN_POINT ( 'NONE',  ( 15.72974639402176855, 15.80617190586768217, 91.87609039468568994 ) ) ;
#124476=CARTESIAN_POINT ( 'NONE',  ( 0.05219959533936267826, -19.03943276465977164, 90.00109039468567573 ) ) ;
#124478=CARTESIAN_POINT ( 'NONE',  ( -4.483927247898539470, -16.52544592524342804, 42.29057627198103120 ) ) ;
#124479=CARTESIAN_POINT ( 'NONE',  ( 12.14591786802309770, 12.06949235617756955, 49.37390960531436690 ) ) ;
#124480=CARTESIAN_POINT ( 'NONE',  ( 8.224510206698953496, -14.34966873604960469, 102.9155762719810383 ) ) ;
#124481=CARTESIAN_POINT ( 'NONE',  ( -19.03943276465977164, -0.05219959533935918106, 48.75109039468566863 ) ) ;
#124483=CARTESIAN_POINT ( 'NONE',  ( 21.55341960407619695, -5.719274019375665929, 56.04275706135235424 ) ) ;
#124484=CARTESIAN_POINT ( 'NONE',  ( 19.02544592524334988, 5.153800228976608722, 106.4594237280190185 ) ) ;
#124486=CARTESIAN_POINT ( 'NONE',  ( -19.02544592524342804, 5.153800228976336051, 106.0405762719810241 ) ) ;
#124487=CARTESIAN_POINT ( 'NONE',  ( -21.53943276465977519, 0.05219959533907696930, 61.24890960531435979 ) ) ;
#124488=CARTESIAN_POINT ( 'NONE',  ( -16.46253265017146816, -9.564922557961047289, 94.16775706135233293 ) ) ;
#124489=CARTESIAN_POINT ( 'NONE',  ( -5.049401038298153566, 19.05341960407611168, 85.20724293864766707 ) ) ;
#124490=CARTESIAN_POINT ( 'NONE',  ( 10.81492255796078972, 18.62759615963270932, 54.58224293864769550 ) ) ;
#124491=CARTESIAN_POINT ( 'NONE',  ( -16.53943276465976808, 0.05219959533911058130, 111.2489096053143669 ) ) ;
#124492=CARTESIAN_POINT ( 'NONE',  ( -9.564922557960796823, -16.46253265017161027, 67.08224293864769550 ) ) ;
#124494=CARTESIAN_POINT ( 'NONE',  ( 19.05341960407611168, 5.049401038298154454, 33.95724293864769550 ) ) ;
#124496=CARTESIAN_POINT ( 'NONE',  ( -15.72974639402176322, -15.80617190586768395, 34.37609039468568284 ) ) ;
#124497=CARTESIAN_POINT ( 'NONE',  ( 15.72974639402176855, 15.80617190586768217, 86.87609039468568994 ) ) ;
#124498=CARTESIAN_POINT ( 'NONE',  ( -14.34966873604972548, 8.224510206698743886, 88.33442372801901854 ) ) ;
#124499=CARTESIAN_POINT ( 'NONE',  ( 5.823673210054444382, -21.52544592524334988, 30.20942372801902565 ) ) ;
#124500=CARTESIAN_POINT ( 'NONE',  ( 21.53943276465977519, 0.05219959533937863772, 36.25109039468567573 ) ) ;
#124501=CARTESIAN_POINT ( 'NONE',  ( 5.049401038297881783, 19.05341960407617563, 72.29275706135234714 ) ) ;
#124502=CARTESIAN_POINT ( 'NONE',  ( 5.049401038298161559, -19.05341960407611168, 72.70724293864768129 ) ) ;
#124503=CARTESIAN_POINT ( 'NONE',  ( 18.62759615963255655, 10.81492255796105972, 86.66775706135234714 ) ) ;
#124504=CARTESIAN_POINT ( 'NONE',  ( -5.823673210054116645, -21.52544592524344225, 87.29057627198103830 ) ) ;
#124505=CARTESIAN_POINT ( 'NONE',  ( 8.314922557960818139, 14.29746914071049879, 69.58224293864769550 ) ) ;
#124506=CARTESIAN_POINT ( 'NONE',  ( -5.719274019375665041, -21.55341960407619695, 104.7927570613523898 ) ) ;
#124507=CARTESIAN_POINT ( 'NONE',  ( 8.314922557960818139, 14.29746914071049879, 89.58224293864768129 ) ) ;
#124508=CARTESIAN_POINT ( 'NONE',  ( -19.05341960407611168, -5.049401038298163336, 36.45724293864766707 ) ) ;
#124509=CARTESIAN_POINT ( 'NONE',  ( -5.049401038297874678, -19.05341960407617918, 69.79275706135233293 ) ) ;
#124510=CARTESIAN_POINT ( 'NONE',  ( -16.55341960407611168, -4.379528057220339221, 41.45724293864769550 ) ) ;
#124511=CARTESIAN_POINT ( 'NONE',  ( 15.80617190586769283, -15.72974639402175789, 95.62609039468568994 ) ) ;
#124512=CARTESIAN_POINT ( 'NONE',  ( 5.049401038298161559, -19.05341960407611168, 97.70724293864766707 ) ) ;
#124513=CARTESIAN_POINT ( 'NONE',  ( 5.153800228976615827, -19.02544592524334988, 65.20942372801900433 ) ) ;
#124514=CARTESIAN_POINT ( 'NONE',  ( -21.55341960407610458, -5.719274019375992779, 61.45724293864770260 ) ) ;
#124516=CARTESIAN_POINT ( 'NONE',  ( 18.62759615963255655, 10.81492255796105972, 21.66775706135235069 ) ) ;
#124517=CARTESIAN_POINT ( 'NONE',  ( 13.97604488694548053, -13.89961937509957401, 105.6260903946856757 ) ) ;
#124518=CARTESIAN_POINT ( 'NONE',  ( -14.34966873604972548, 8.224510206698743886, 83.33442372801903275 ) ) ;
#124519=CARTESIAN_POINT ( 'NONE',  ( 30.00000000000000000, -5.499999999999992895, 37.50000000000000000 ) ) ;
#124520=CARTESIAN_POINT ( 'NONE',  ( 21.55341960407619695, -5.719274019375665929, 21.04275706135234714 ) ) ;
#124521=CARTESIAN_POINT ( 'NONE',  ( 12.06949235617757843, -12.14591786802309237, 108.1239096053143811 ) ) ;
#124523=CARTESIAN_POINT ( 'NONE',  ( -8.314922557961024197, 14.29746914071037800, 42.91775706135235424 ) ) ;
#124524=CARTESIAN_POINT ( 'NONE',  ( 18.67979575497178502, 10.72451020669898547, 59.16557627198103120 ) ) ;
#124525=CARTESIAN_POINT ( 'NONE',  ( 0.05219959533934541429, -16.53943276465976808, 105.0010903946856757 ) ) ;
#124526=CARTESIAN_POINT ( 'NONE',  ( 16.52544592524335698, 4.483927247898782831, 36.45942372801901143 ) ) ;
#124527=CARTESIAN_POINT ( 'NONE',  ( -13.89961937509977652, 13.97604488694528158, 25.62390960531434558 ) ) ;
#124528=CARTESIAN_POINT ( 'NONE',  ( 4.483927247898790824, -16.52544592524335698, 80.20942372801901854 ) ) ;
#124529=CARTESIAN_POINT ( 'NONE',  ( -5.049401038297874678, -19.05341960407617918, 69.79275706135233293 ) ) ;
#124530=CARTESIAN_POINT ( 'NONE',  ( -5.719274019375978568, 21.55341960407610458, 75.20724293864769550 ) ) ;
#124531=CARTESIAN_POINT ( 'NONE',  ( 16.53943276465976808, 0.05219959533934440121, 91.25109039468568994 ) ) ;
#124532=CARTESIAN_POINT ( 'NONE',  ( -21.52544592524334988, -5.823673210054445271, 78.95942372801901854 ) ) ;
#124533=CARTESIAN_POINT ( 'NONE',  ( 10.72451020669898902, -18.67979575497178502, 62.91557627198102409 ) ) ;
#124534=CARTESIAN_POINT ( 'NONE',  ( 15.80617190586746368, 15.72974639402197994, 49.37390960531436690 ) ) ;
#124535=ORIENTED_EDGE ( 'NONE', *, *, #29998, .T. ) ;
#124536=CARTESIAN_POINT ( 'NONE',  ( -4.379528057220086978, -16.55341960407618274, 79.79275706135236135 ) ) ;
#124537=CARTESIAN_POINT ( 'NONE',  ( 18.62759615963271287, -10.81492255796078972, 43.33224293864769550 ) ) ;
#124539=CARTESIAN_POINT ( 'NONE',  ( 13.97604488694527802, 13.89961937509977652, 114.3739096053143669 ) ) ;
#124541=CARTESIAN_POINT ( 'NONE',  ( 13.97604488694527802, 13.89961937509977652, 24.37390960531435624 ) ) ;
#124542=CARTESIAN_POINT ( 'NONE',  ( -0.05219959533907301413, -21.53943276465977519, 57.49890960531435979 ) ) ;
#124543=CARTESIAN_POINT ( 'NONE',  ( 16.55341960407618274, -4.379528057220086978, 106.0427570613523471 ) ) ;
#124544=CARTESIAN_POINT ( 'NONE',  ( 21.55341960407619695, -5.719274019375665929, 46.04275706135234714 ) ) ;
#124545=CARTESIAN_POINT ( 'NONE',  ( -9.564922557961040184, 16.46253265017147172, 102.9177570613523329 ) ) ;
#124546=CARTESIAN_POINT ( 'NONE',  ( 9.564922557960805705, 16.46253265017160317, 24.58224293864769194 ) ) ;
#124547=CARTESIAN_POINT ( 'NONE',  ( 19.05341960407617918, -5.049401038297876454, 106.0427570613523471 ) ) ;
#124548=CARTESIAN_POINT ( 'NONE',  ( -9.474510206698964154, 16.51473224551069663, 45.41557627198103120 ) ) ;
#124550=CARTESIAN_POINT ( 'NONE',  ( -9.564922557960796823, -16.46253265017161027, 97.08224293864769550 ) ) ;
#124551=CARTESIAN_POINT ( 'NONE',  ( -12.06949235617739369, -12.14591786802326823, 69.37609039468567573 ) ) ;
#124552=CARTESIAN_POINT ( 'NONE',  ( -13.89961937509957401, -13.97604488694547875, 79.37609039468567573 ) ) ;
#124553=CARTESIAN_POINT ( 'NONE',  ( -9.474510206698720793, -16.51473224551083518, 29.58442372801900433 ) ) ;
#124554=CARTESIAN_POINT ( 'NONE',  ( -5.823673210054116645, -21.52544592524344225, 62.29057627198102409 ) ) ;
#124555=CARTESIAN_POINT ( 'NONE',  ( 14.29746914071037800, 8.314922557961029526, 81.66775706135236135 ) ) ;
#124556=CARTESIAN_POINT ( 'NONE',  ( -16.46253265017146816, -9.564922557961047289, 84.16775706135233293 ) ) ;
#124557=CARTESIAN_POINT ( 'NONE',  ( -16.46253265017160317, 9.564922557960807481, 35.83224293864768839 ) ) ;
#124558=CARTESIAN_POINT ( 'NONE',  ( -9.564922557960796823, -16.46253265017161027, 82.08224293864768129 ) ) ;
#124559=CARTESIAN_POINT ( 'NONE',  ( 0.05219959533937995610, -21.53943276465977519, 45.00109039468568284 ) ) ;
#124560=CARTESIAN_POINT ( 'NONE',  ( -19.03943276465977164, 0.05219959533909376836, 51.24890960531436690 ) ) ;
#124561=CARTESIAN_POINT ( 'NONE',  ( 0.05219959533936267826, -19.03943276465977164, 70.00109039468566152 ) ) ;
#124563=CARTESIAN_POINT ( 'NONE',  ( 13.97604488694527802, 13.89961937509977652, 109.3739096053143669 ) ) ;
#124564=CARTESIAN_POINT ( 'NONE',  ( -16.55341960407611168, -4.379528057220339221, 61.45724293864770260 ) ) ;
#124565=CARTESIAN_POINT ( 'NONE',  ( 10.81492255796078972, 18.62759615963270932, 54.58224293864769550 ) ) ;
#124566=CARTESIAN_POINT ( 'NONE',  ( 19.50973618000807264, -5.499999999999992895, 102.5000000000000142 ) ) ;
#124567=CARTESIAN_POINT ( 'NONE',  ( 0.05219959533936267826, -19.03943276465977164, 40.00109039468566152 ) ) ;
#124569=CARTESIAN_POINT ( 'NONE',  ( 19.03943276465977164, -0.05219959533909143690, 68.74890960531436690 ) ) ;
#124570=CARTESIAN_POINT ( 'NONE',  ( 9.474510206698971260, -16.51473224551069308, 67.91557627198102409 ) ) ;
#124571=CARTESIAN_POINT ( 'NONE',  ( 16.53943276465976808, 0.05219959533934440121, 46.25109039468567573 ) ) ;
#124572=CARTESIAN_POINT ( 'NONE',  ( -5.049401038297874678, -19.05341960407618274, 79.79275706135233293 ) ) ;
#124574=CARTESIAN_POINT ( 'NONE',  ( -14.34966873604972548, 8.224510206698743886, 83.33442372801903275 ) ) ;
#124576=CARTESIAN_POINT ( 'NONE',  ( 8.314922557961029526, -14.29746914071037800, 70.41775706135236135 ) ) ;
#124577=CARTESIAN_POINT ( 'NONE',  ( -8.224510206698735004, -14.34966873604973081, 54.58442372801901143 ) ) ;
#124578=CARTESIAN_POINT ( 'NONE',  ( 19.05341960407617918, -5.049401038297876454, 26.04275706135233293 ) ) ;
#124579=CARTESIAN_POINT ( 'NONE',  ( -9.474510206698964154, 16.51473224551069663, 60.41557627198102409 ) ) ;
#124581=CARTESIAN_POINT ( 'NONE',  ( -21.55341960407619339, 5.719274019375674811, 53.54275706135234714 ) ) ;
#124582=CARTESIAN_POINT ( 'NONE',  ( 19.02544592524334988, 5.153800228976608722, 66.45942372801899012 ) ) ;
#124583=CARTESIAN_POINT ( 'NONE',  ( -15.80617190586768217, 15.72974639402176855, 108.1260903946856757 ) ) ;
#124585=CARTESIAN_POINT ( 'NONE',  ( 0.05219959533909260263, 19.03943276465977164, 34.99890960531435979 ) ) ;
#124587=CARTESIAN_POINT ( 'NONE',  ( -21.52544592524343514, 5.823673210054127303, 66.04057627198103830 ) ) ;
#124588=CARTESIAN_POINT ( 'NONE',  ( 5.049401038298161559, -19.05341960407611168, 112.7072429386476813 ) ) ;
#124589=CARTESIAN_POINT ( 'NONE',  ( -4.379528057220328563, 16.55341960407611168, 100.2072429386476955 ) ) ;
#124590=CARTESIAN_POINT ( 'NONE',  ( 16.52544592524335698, 4.483927247898782831, 31.45942372801901854 ) ) ;
#124591=CARTESIAN_POINT ( 'NONE',  ( 16.52544592524342804, -4.483927247898539470, 33.54057627198102409 ) ) ;
#124592=ORIENTED_EDGE ( 'NONE', *, *, #192356, .T. ) ;
#124593=CARTESIAN_POINT ( 'NONE',  ( 5.719274019375991003, -21.55341960407610458, 112.7072429386476955 ) ) ;
#124594=CARTESIAN_POINT ( 'NONE',  ( 16.55341960407611168, 4.379528057220329451, 38.95724293864768839 ) ) ;
#124595=CARTESIAN_POINT ( 'NONE',  ( 5.153800228976335163, 19.02544592524342804, 109.7905762719810099 ) ) ;
#124596=CARTESIAN_POINT ( 'NONE',  ( 16.51473224551083163, -9.474510206698727899, 105.8344237280190043 ) ) ;
#124597=CARTESIAN_POINT ( 'NONE',  ( 5.049401038297881783, 19.05341960407617563, 27.29275706135232937 ) ) ;
#124598=CARTESIAN_POINT ( 'NONE',  ( -0.05219959533910754901, -16.53943276465976808, 37.49890960531436690 ) ) ;
#124599=CARTESIAN_POINT ( 'NONE',  ( 10.72451020669898902, -18.67979575497178502, 102.9155762719810383 ) ) ;
#124600=CARTESIAN_POINT ( 'NONE',  ( 17.13100169013300444, 6.664070546373172199, 31.73210164300152414 ) ) ;
#124601=CARTESIAN_POINT ( 'NONE',  ( -10.81492255796078084, -18.62759615963271287, 67.08224293864770971 ) ) ;
#124602=CARTESIAN_POINT ( 'NONE',  ( -9.474510206698964154, 16.51473224551069663, 70.41557627198102409 ) ) ;
#124603=CARTESIAN_POINT ( 'NONE',  ( -16.52544592524342804, 4.483927247898546575, 46.04057627198103830 ) ) ;
#124604=CARTESIAN_POINT ( 'NONE',  ( 9.564922557960805705, 16.46253265017160317, 84.58224293864769550 ) ) ;
#124606=CARTESIAN_POINT ( 'NONE',  ( -16.46253265017146816, -9.564922557961047289, 59.16775706135233293 ) ) ;
#124607=CARTESIAN_POINT ( 'NONE',  ( 21.52544592524344225, -5.823673210054117533, 93.54057627198103830 ) ) ;
#124608=CARTESIAN_POINT ( 'NONE',  ( 4.379528057220339221, -16.55341960407611168, 102.7072429386476955 ) ) ;
#124609=CARTESIAN_POINT ( 'NONE',  ( -21.52544592524334988, -5.823673210054445271, 33.95942372801901143 ) ) ;
#124611=CARTESIAN_POINT ( 'NONE',  ( -16.55341960407611168, -4.379528057220339221, 26.45724293864768839 ) ) ;
#124612=CARTESIAN_POINT ( 'NONE',  ( 0.05219959533909260263, 19.03943276465977164, 34.99890960531435979 ) ) ;
#124613=CARTESIAN_POINT ( 'NONE',  ( -13.97604488694527625, -13.89961937509977652, 86.87390960531436690 ) ) ;
#124614=CARTESIAN_POINT ( 'NONE',  ( 15.72974639402199770, -15.80617190586745480, 63.12390960531435979 ) ) ;
#124615=CARTESIAN_POINT ( 'NONE',  ( -18.56453257813360835, 5.500000000000041744, 45.99000423690687711 ) ) ;
#124616=CARTESIAN_POINT ( 'NONE',  ( 5.049401038298161559, -19.05341960407611168, 27.70724293864769550 ) ) ;
#124617=CARTESIAN_POINT ( 'NONE',  ( -15.80617190586745835, -15.72974639402198527, 51.87390960531437401 ) ) ;
#124618=CARTESIAN_POINT ( 'NONE',  ( -10.72451020669870658, -18.67979575497194134, 69.58442372801900433 ) ) ;
#124620=CARTESIAN_POINT ( 'NONE',  ( -8.314922557961024197, 14.29746914071037800, 67.91775706135234714 ) ) ;
#124621=CARTESIAN_POINT ( 'NONE',  ( 16.51473224551069308, 9.474510206698969483, 54.16557627198103120 ) ) ;
#124622=CARTESIAN_POINT ( 'NONE',  ( 19.05341960407611168, 5.049401038298154454, 58.95724293864768129 ) ) ;
#124624=CARTESIAN_POINT ( 'NONE',  ( -19.05341960407617563, 5.049401038297882671, 28.54275706135232937 ) ) ;
#124625=CARTESIAN_POINT ( 'NONE',  ( -14.29746914071037622, -8.314922557961029526, 74.16775706135231871 ) ) ;
#124626=CARTESIAN_POINT ( 'NONE',  ( -21.55341960407619339, 5.719274019375674811, 93.54275706135234714 ) ) ;
#124627=CARTESIAN_POINT ( 'NONE',  ( 19.02544592524343514, -5.153800228976328945, 78.54057627198099567 ) ) ;
#124628=CARTESIAN_POINT ( 'NONE',  ( 10.81492255796078972, 18.62759615963270932, 39.58224293864769550 ) ) ;
#124629=CARTESIAN_POINT ( 'NONE',  ( 19.05341960407617918, -5.049401038297876454, 106.0427570613523471 ) ) ;
#124630=CARTESIAN_POINT ( 'NONE',  ( 15.80617190586769283, -15.72974639402175789, 85.62609039468568994 ) ) ;
#124631=CARTESIAN_POINT ( 'NONE',  ( 4.379528057220092307, 16.55341960407617563, 47.29275706135234003 ) ) ;
#124632=CARTESIAN_POINT ( 'NONE',  ( 21.55341960407610458, 5.719274019375980345, 103.9572429386476813 ) ) ;
#124633=CARTESIAN_POINT ( 'NONE',  ( 16.51473224551083163, -9.474510206698727899, 110.8344237280190043 ) ) ;
#124634=VECTOR ( 'NONE', #128886, 1000.000000000000000 ) ;
#124635=CARTESIAN_POINT ( 'NONE',  ( 19.05341960407611168, 5.049401038298154454, 73.95724293864768129 ) ) ;
#124636=CARTESIAN_POINT ( 'NONE',  ( 0.05219959533934541429, -16.53943276465976808, 20.00109039468568639 ) ) ;
#124637=CARTESIAN_POINT ( 'NONE',  ( 5.049401038298161559, -19.05341960407611168, 42.70724293864767418 ) ) ;
#124638=CARTESIAN_POINT ( 'NONE',  ( 4.483927247898790824, -16.52544592524335698, 20.20942372801900788 ) ) ;
#124639=CARTESIAN_POINT ( 'NONE',  ( 16.52544592524342804, -4.483927247898539470, 68.54057627198103830 ) ) ;
#124640=CARTESIAN_POINT ( 'NONE',  ( -14.34966873604972548, 8.224510206698743886, 78.33442372801901854 ) ) ;
#124641=CARTESIAN_POINT ( 'NONE',  ( 10.81492255796106328, -18.62759615963255655, 35.41775706135234003 ) ) ;
#124642=CARTESIAN_POINT ( 'NONE',  ( -0.05219959533909027116, -19.03943276465977164, 47.49890960531435979 ) ) ;
#124643=CARTESIAN_POINT ( 'NONE',  ( 16.46253265017160672, -9.564922557960803928, 68.33224293864770971 ) ) ;
#124644=CARTESIAN_POINT ( 'NONE',  ( 12.14591786802327356, -12.06949235617739191, 70.62609039468567573 ) ) ;
#124646=EDGE_LOOP ( 'NONE', ( #139745, #199492, #130928, #177898, #136329, #82218, #198030, #191509 ) ) ;
#124647=ORIENTED_EDGE ( 'NONE', *, *, #42468, .F. ) ;
#124648=CARTESIAN_POINT ( 'NONE',  ( -9.474510206698720793, -16.51473224551083518, 19.58442372801899722 ) ) ;
#124649=CARTESIAN_POINT ( 'NONE',  ( 13.97604488694527802, 13.89961937509977652, 39.37390960531435269 ) ) ;
#124652=CARTESIAN_POINT ( 'NONE',  ( 12.14591786802327356, -12.06949235617739191, 35.62609039468568994 ) ) ;
#124653=CARTESIAN_POINT ( 'NONE',  ( 16.51473224551083163, -9.474510206698727899, 60.83442372801900433 ) ) ;
#124654=CARTESIAN_POINT ( 'NONE',  ( -16.53943276465976808, -0.05219959533934237506, 43.75109039468568284 ) ) ;
#124655=CARTESIAN_POINT ( 'NONE',  ( -5.153800228976328057, -19.02544592524343514, 37.29057627198102409 ) ) ;
#124656=CARTESIAN_POINT ( 'NONE',  ( -13.89961937509977652, 13.97604488694528158, 105.6239096053143527 ) ) ;
#124657=CARTESIAN_POINT ( 'NONE',  ( 19.03943276465977164, -0.05219959533909143690, 58.74890960531435979 ) ) ;
#124658=CARTESIAN_POINT ( 'NONE',  ( 0.05219959533907565091, 21.53943276465977519, 104.9989096053143669 ) ) ;
#124659=CARTESIAN_POINT ( 'NONE',  ( -16.51473224551069308, -9.474510206698971260, 91.66557627198103830 ) ) ;
#124660=CARTESIAN_POINT ( 'NONE',  ( -13.89961937509977652, 13.97604488694528158, 110.6239096053143243 ) ) ;
#124661=CARTESIAN_POINT ( 'NONE',  ( -19.03943276465977164, 0.05219959533909376836, 61.24890960531436690 ) ) ;
#124662=CARTESIAN_POINT ( 'NONE',  ( -12.14591786802326823, 12.06949235617739902, 113.1260903946856899 ) ) ;
#124664=CARTESIAN_POINT ( 'NONE',  ( 5.153800228976615827, -19.02544592524334988, 100.2094237280190043 ) ) ;
#124665=CARTESIAN_POINT ( 'NONE',  ( 5.049401038297881783, 19.05341960407617563, 22.29275706135233648 ) ) ;
#124666=CARTESIAN_POINT ( 'NONE',  ( -4.379528057220328563, 16.55341960407611168, 55.20724293864770260 ) ) ;
#124667=CARTESIAN_POINT ( 'NONE',  ( 15.72974639402176855, 15.80617190586768217, 96.87609039468568994 ) ) ;
#124668=CARTESIAN_POINT ( 'NONE',  ( 9.474510206698971260, -16.51473224551069308, 42.91557627198103120 ) ) ;
#124669=CARTESIAN_POINT ( 'NONE',  ( -14.34966873604960291, -8.224510206698953496, 21.66557627198102409 ) ) ;
#124670=CARTESIAN_POINT ( 'NONE',  ( 10.72451020669871369, 18.67979575497193778, 92.08442372801901854 ) ) ;
#124671=CARTESIAN_POINT ( 'NONE',  ( -19.05341960407611168, -5.049401038298163336, 76.45724293864769550 ) ) ;
#124672=CARTESIAN_POINT ( 'NONE',  ( -9.564922557960796823, -16.46253265017161027, 97.08224293864769550 ) ) ;
#124673=CARTESIAN_POINT ( 'NONE',  ( -16.52544592524342804, 4.483927247898546575, 96.04057627198102409 ) ) ;
#124674=CARTESIAN_POINT ( 'NONE',  ( -16.52544592524342804, 4.483927247898546575, 71.04057627198103830 ) ) ;
#124675=CARTESIAN_POINT ( 'NONE',  ( 21.55341960407610458, 5.719274019375980345, 63.95724293864770260 ) ) ;
#124676=CARTESIAN_POINT ( 'NONE',  ( 9.564922557960805705, 16.46253265017160317, 74.58224293864769550 ) ) ;
#124677=CARTESIAN_POINT ( 'NONE',  ( 21.53943276465977519, -0.05219959533907433946, 78.74890960531436690 ) ) ;
#124678=CARTESIAN_POINT ( 'NONE',  ( -19.05341960407617563, 5.049401038297882671, 83.54275706135233293 ) ) ;
#124681=CARTESIAN_POINT ( 'NONE',  ( 12.14591786802309770, 12.06949235617756955, 94.37390960531436690 ) ) ;
#124682=CARTESIAN_POINT ( 'NONE',  ( -13.97604488694527625, -13.89961937509977652, 56.87390960531434558 ) ) ;
#124683=CARTESIAN_POINT ( 'NONE',  ( 10.81492255796078972, 18.62759615963270932, 69.58224293864769550 ) ) ;
#124685=CARTESIAN_POINT ( 'NONE',  ( 17.49999999999999289, -5.624438216177594541, 28.31670344914645199 ) ) ;
#124686=CARTESIAN_POINT ( 'NONE',  ( -4.379528057220086978, -16.55341960407618274, 109.7927570613523613 ) ) ;
#124688=CARTESIAN_POINT ( 'NONE',  ( 13.97604488694548053, -13.89961937509957401, 110.6260903946856615 ) ) ;
#124689=CARTESIAN_POINT ( 'NONE',  ( 16.52544592524342804, -4.483927247898539470, 83.54057627198102409 ) ) ;
#124691=CARTESIAN_POINT ( 'NONE',  ( -5.049401038298153566, 19.05341960407611168, 80.20724293864769550 ) ) ;
#124692=CARTESIAN_POINT ( 'NONE',  ( 5.153800228976335163, 19.02544592524342804, 34.79057627198102409 ) ) ;
#124693=CARTESIAN_POINT ( 'NONE',  ( 16.52544592524342804, -4.483927247898539470, 73.54057627198102409 ) ) ;
#124694=CARTESIAN_POINT ( 'NONE',  ( -9.474510206698964154, 16.51473224551069663, 100.4155762719810241 ) ) ;
#124695=CARTESIAN_POINT ( 'NONE',  ( -5.049401038297874678, -19.05341960407617918, 84.79275706135233293 ) ) ;
#124696=CARTESIAN_POINT ( 'NONE',  ( 19.05341960407611168, 5.049401038298154454, 78.95724293864769550 ) ) ;
#124697=CARTESIAN_POINT ( 'NONE',  ( -9.564922557960796823, -16.46253265017161027, 92.08224293864769550 ) ) ;
#124698=CARTESIAN_POINT ( 'NONE',  ( -5.823673210054116645, -21.52544592524344225, 77.29057627198102409 ) ) ;
#124699=CARTESIAN_POINT ( 'NONE',  ( 14.29746914071037800, 8.314922557961029526, 76.66775706135234714 ) ) ;
#124700=CARTESIAN_POINT ( 'NONE',  ( 13.97604488694548053, -13.89961937509957401, 110.6260903946856757 ) ) ;
#124701=CARTESIAN_POINT ( 'NONE',  ( -16.46253265017160317, 9.564922557960807481, 60.83224293864769550 ) ) ;
#124702=CARTESIAN_POINT ( 'NONE',  ( -21.53943276465977519, 0.05219959533907696930, 66.24890960531436690 ) ) ;
#124703=CARTESIAN_POINT ( 'NONE',  ( -13.89961937509957401, -13.97604488694547875, 99.37609039468567573 ) ) ;
#124704=CARTESIAN_POINT ( 'NONE',  ( -14.34966873604960291, -8.224510206698953496, 41.66557627198103120 ) ) ;
#124705=CARTESIAN_POINT ( 'NONE',  ( -5.719274019375665041, -21.55341960407619695, 39.79275706135235424 ) ) ;
#124706=CARTESIAN_POINT ( 'NONE',  ( -4.379528057220086978, -16.55341960407618274, 74.79275706135234714 ) ) ;
#124707=CARTESIAN_POINT ( 'NONE',  ( 9.564922557960805705, 16.46253265017160317, 99.58224293864770971 ) ) ;
#124710=CARTESIAN_POINT ( 'NONE',  ( -16.55341960407617563, 4.379528057220093196, 88.54275706135236135 ) ) ;
#124711=CARTESIAN_POINT ( 'NONE',  ( 0.05219959533934541429, -16.53943276465976808, 50.00109039468568994 ) ) ;
#124712=CARTESIAN_POINT ( 'NONE',  ( -19.03943276465977164, 0.05219959533909376836, 56.24890960531435979 ) ) ;
#124713=CARTESIAN_POINT ( 'NONE',  ( -19.05341960407611168, -5.049401038298163336, 61.45724293864769550 ) ) ;
#124714=CARTESIAN_POINT ( 'NONE',  ( -18.67979575497193778, 10.72451020669871902, 48.33442372801902565 ) ) ;
#124715=CARTESIAN_POINT ( 'NONE',  ( 16.55341960407618274, -4.379528057220086978, 66.04275706135236135 ) ) ;
#124716=CARTESIAN_POINT ( 'NONE',  ( 16.53943276465976808, -0.05219959533910856209, 28.74890960531435624 ) ) ;
#124717=CARTESIAN_POINT ( 'NONE',  ( -19.05341960407611168, -5.049401038298163336, 46.45724293864768129 ) ) ;
#124718=CARTESIAN_POINT ( 'NONE',  ( -19.05341960407611168, -5.049401038298163336, 31.45724293864769550 ) ) ;
#124719=CARTESIAN_POINT ( 'NONE',  ( 4.483927247898790824, -16.52544592524335698, 30.20942372801902565 ) ) ;
#124721=CARTESIAN_POINT ( 'NONE',  ( 16.46253265017146816, 9.564922557961045513, 81.66775706135233293 ) ) ;
#124722=CARTESIAN_POINT ( 'NONE',  ( -12.06949235617756955, 12.14591786802309770, 80.62390960531438111 ) ) ;
#124723=CARTESIAN_POINT ( 'NONE',  ( 0.05219959533909260263, 19.03943276465977164, 54.99890960531435979 ) ) ;
#124724=CARTESIAN_POINT ( 'NONE',  ( 19.02544592524334988, 5.153800228976608722, 86.45942372801900433 ) ) ;
#124726=CARTESIAN_POINT ( 'NONE',  ( -0.05219959533937732626, 21.53943276465977519, 87.50109039468568994 ) ) ;
#124727=CARTESIAN_POINT ( 'NONE',  ( 16.55341960407618274, -4.379528057220086978, 51.04275706135234714 ) ) ;
#124728=CARTESIAN_POINT ( 'NONE',  ( 17.49999999999999645, 5.624438216177604311, 36.68329655085356933 ) ) ;
#124729=CARTESIAN_POINT ( 'NONE',  ( -21.55341960407610458, -5.719274019375992779, 51.45724293864770260 ) ) ;
#124730=CARTESIAN_POINT ( 'NONE',  ( 16.55341960407618274, -4.379528057220086978, 46.04275706135234714 ) ) ;
#124732=CARTESIAN_POINT ( 'NONE',  ( 16.51473224551083163, -9.474510206698727899, 25.83442372801900078 ) ) ;
#124733=AXIS2_PLACEMENT_3D ( 'NONE', #68782, #55617, #52615 ) ;
#124734=CARTESIAN_POINT ( 'NONE',  ( -9.564922557960796823, -16.46253265017161027, 72.08224293864770971 ) ) ;
#124736=CARTESIAN_POINT ( 'NONE',  ( 19.02544592524343514, -5.153800228976328945, 53.54057627198102409 ) ) ;
#124737=CARTESIAN_POINT ( 'NONE',  ( -17.49999999999999645, -5.499999999999992895, 44.20309617465829888 ) ) ;
#124738=CARTESIAN_POINT ( 'NONE',  ( 16.46253265017160672, -9.564922557960803928, 68.33224293864770971 ) ) ;
#124740=CARTESIAN_POINT ( 'NONE',  ( -18.09805431107247387, 5.500000000000101252, 66.01606229291884631 ) ) ;
#124741=CARTESIAN_POINT ( 'NONE',  ( 16.46253265017146816, 9.564922557961045513, 36.66775706135233293 ) ) ;
#124742=CARTESIAN_POINT ( 'NONE',  ( -21.55341960407619339, 5.719274019375674811, 113.5427570613523756 ) ) ;
#124743=CARTESIAN_POINT ( 'NONE',  ( 14.34966873604960469, 8.224510206698951720, 44.16557627198103120 ) ) ;
#124744=CARTESIAN_POINT ( 'NONE',  ( -0.05219959533909027116, -19.03943276465977164, 42.49890960531435269 ) ) ;
#124745=CARTESIAN_POINT ( 'NONE',  ( 19.02544592524343514, -5.153800228976328945, 103.5405762719809957 ) ) ;
#124746=CARTESIAN_POINT ( 'NONE',  ( -5.823673210054431948, 21.52544592524334988, 72.70942372801901854 ) ) ;
#124747=CARTESIAN_POINT ( 'NONE',  ( 5.153800228976335163, 19.02544592524342804, 49.79057627198100988 ) ) ;
#124748=CARTESIAN_POINT ( 'NONE',  ( -10.81492255796105439, 18.62759615963255655, 82.91775706135234714 ) ) ;
#124749=CARTESIAN_POINT ( 'NONE',  ( -21.52544592524343514, 5.823673210054127303, 26.04057627198103475 ) ) ;
#124750=CARTESIAN_POINT ( 'NONE',  ( 5.153800228976335163, 19.02544592524342804, 34.79057627198102409 ) ) ;
#124751=CARTESIAN_POINT ( 'NONE',  ( 5.823673210054444382, -21.52544592524334988, 25.20942372801901854 ) ) ;
#124752=CARTESIAN_POINT ( 'NONE',  ( -5.049401038297874678, -19.05341960407617918, 49.79275706135231871 ) ) ;
#124753=CARTESIAN_POINT ( 'NONE',  ( 5.049401038298161559, -19.05341960407611168, 27.70724293864769550 ) ) ;
#124754=CARTESIAN_POINT ( 'NONE',  ( -9.474510206698964154, 16.51473224551069663, 75.41557627198103830 ) ) ;
#124755=CARTESIAN_POINT ( 'NONE',  ( 12.14591786802327356, -12.06949235617739191, 20.62609039468568639 ) ) ;
#124756=CARTESIAN_POINT ( 'NONE',  ( 4.483927247898545687, 16.52544592524342804, 79.79057627198102409 ) ) ;
#124757=CARTESIAN_POINT ( 'NONE',  ( -18.62759615963270932, 10.81492255796079327, 35.83224293864768839 ) ) ;
#124758=CARTESIAN_POINT ( 'NONE',  ( -0.05219959533936034679, 19.03943276465977164, 102.5010903946856757 ) ) ;
#124759=CARTESIAN_POINT ( 'NONE',  ( 21.53943276465977519, -0.05219959533907433946, 98.74890960531438111 ) ) ;
#124760=CARTESIAN_POINT ( 'NONE',  ( 21.55341960407619695, -5.719274019375665929, 61.04275706135234714 ) ) ;
#124761=CARTESIAN_POINT ( 'NONE',  ( 14.29746914071037800, 8.314922557961029526, 51.66775706135234714 ) ) ;
#124762=CARTESIAN_POINT ( 'NONE',  ( 16.52544592524335698, 4.483927247898782831, 61.45942372801901854 ) ) ;
#124763=CARTESIAN_POINT ( 'NONE',  ( -0.05219959533909027116, -19.03943276465977164, 47.49890960531435979 ) ) ;
#124764=CARTESIAN_POINT ( 'NONE',  ( 4.379528057220092307, 16.55341960407617563, 92.29275706135236135 ) ) ;
#124765=CARTESIAN_POINT ( 'NONE',  ( 21.52544592524334988, 5.823673210054432836, 21.45942372801901499 ) ) ;
#124766=CARTESIAN_POINT ( 'NONE',  ( 16.55341960407611168, 4.379528057220329451, 53.95724293864770260 ) ) ;
#124767=CARTESIAN_POINT ( 'NONE',  ( -9.474510206698964154, 16.51473224551069663, 85.41557627198102409 ) ) ;
#124768=CARTESIAN_POINT ( 'NONE',  ( -16.53943276465976808, -0.05219959533934237506, 73.75109039468567573 ) ) ;
#124769=CARTESIAN_POINT ( 'NONE',  ( -15.80617190586768217, 15.72974639402176855, 43.12609039468568284 ) ) ;
#124770=CARTESIAN_POINT ( 'NONE',  ( 9.474510206698729675, 16.51473224551082808, 107.0844237280190043 ) ) ;
#124771=CARTESIAN_POINT ( 'NONE',  ( 5.823673210054444382, -21.52544592524334988, 20.20942372801900788 ) ) ;
#124772=CARTESIAN_POINT ( 'NONE',  ( 16.55341960407611168, 4.379528057220329451, 43.95724293864769550 ) ) ;
#124774=CARTESIAN_POINT ( 'NONE',  ( -16.21995358207303539, 7.366697692864240032, 74.93551001512157939 ) ) ;
#124775=CARTESIAN_POINT ( 'NONE',  ( 18.67979575497178502, 10.72451020669898547, 94.16557627198103830 ) ) ;
#124776=CARTESIAN_POINT ( 'NONE',  ( 16.52544592524342804, -4.483927247898539470, 23.54057627198102765 ) ) ;
#124779=CARTESIAN_POINT ( 'NONE',  ( -21.55341960407610458, -5.719274019375992779, 111.4572429386476813 ) ) ;
#124780=CARTESIAN_POINT ( 'NONE',  ( 0.05219959533909260263, 19.03943276465977164, 114.9989096053143669 ) ) ;
#124781=CARTESIAN_POINT ( 'NONE',  ( -15.72974639402176322, -15.80617190586768395, 19.37609039468568639 ) ) ;
#124782=CARTESIAN_POINT ( 'NONE',  ( 8.314922557960818139, 14.29746914071049879, 49.58224293864769550 ) ) ;
#124783=CARTESIAN_POINT ( 'NONE',  ( -4.483927247898782831, 16.52544592524335698, 67.70942372801901854 ) ) ;
#124784=CARTESIAN_POINT ( 'NONE',  ( -16.51473224551069308, -9.474510206698971260, 61.66557627198103120 ) ) ;
#124785=CARTESIAN_POINT ( 'NONE',  ( -13.89961937509957401, -13.97604488694547875, 59.37609039468566863 ) ) ;
#124786=CARTESIAN_POINT ( 'NONE',  ( 19.05341960407611168, 5.049401038298154454, 73.95724293864768129 ) ) ;
#124787=CARTESIAN_POINT ( 'NONE',  ( 0.05219959533907565091, 21.53943276465977519, 29.99890960531435979 ) ) ;
#124789=CARTESIAN_POINT ( 'NONE',  ( -19.03943276465977164, 0.05219959533909376836, 41.24890960531435269 ) ) ;
#124790=CARTESIAN_POINT ( 'NONE',  ( 14.34966873604972726, -8.224510206698740333, 20.83442372801901143 ) ) ;
#124791=CARTESIAN_POINT ( 'NONE',  ( -19.03943276465977164, -0.05219959533935918106, 58.75109039468566863 ) ) ;
#124792=CARTESIAN_POINT ( 'NONE',  ( 10.81492255796078972, 18.62759615963270932, 99.58224293864770971 ) ) ;
#124793=CARTESIAN_POINT ( 'NONE',  ( 16.53943276465976808, -0.05219959533910856209, 33.74890960531436690 ) ) ;
#124794=B_SPLINE_CURVE_WITH_KNOTS ( 'NONE', 3,
 ( #29759, #147369, #101856, #90423, #40177, #91394 ),
 .UNSPECIFIED., .F., .F.,
 ( 4, 2, 4 ),
 ( 0.003989672132298185958, 0.004372778065220619612, 0.004755883998143053265 ),
 .UNSPECIFIED. ) ;
#124795=CARTESIAN_POINT ( 'NONE',  ( 19.03943276465977164, -0.05219959533909143690, 93.74890960531435269 ) ) ;
#124796=CARTESIAN_POINT ( 'NONE',  ( 10.81492255796078972, 18.62759615963270932, 54.58224293864769550 ) ) ;
#124797=CARTESIAN_POINT ( 'NONE',  ( -21.55341960407610458, -5.719274019375992779, 96.45724293864770971 ) ) ;
#124798=CARTESIAN_POINT ( 'NONE',  ( 0.05219959533934541429, -16.53943276465976808, 25.00109039468567218 ) ) ;
#124799=CARTESIAN_POINT ( 'NONE',  ( 5.823673210054125526, 21.52544592524343514, 39.79057627198103830 ) ) ;
#124800=CARTESIAN_POINT ( 'NONE',  ( 10.72451020669871369, 18.67979575497193778, 92.08442372801901854 ) ) ;
#124801=CARTESIAN_POINT ( 'NONE',  ( 13.89961937509977652, -13.97604488694527269, 88.12390960531438111 ) ) ;
#124802=CARTESIAN_POINT ( 'NONE',  ( 9.564922557960805705, 16.46253265017160317, 24.58224293864769194 ) ) ;
#124803=CARTESIAN_POINT ( 'NONE',  ( -5.153800228976328057, -19.02544592524343514, 87.29057627198103830 ) ) ;
#124804=CARTESIAN_POINT ( 'NONE',  ( -4.379528057220328563, 16.55341960407611168, 105.2072429386477097 ) ) ;
#124805=CARTESIAN_POINT ( 'NONE',  ( -19.03943276465977164, 0.05219959533909376836, 61.24890960531436690 ) ) ;
#124806=CARTESIAN_POINT ( 'NONE',  ( -14.29746914071037622, -8.314922557961029526, 24.16775706135235424 ) ) ;
#124808=CARTESIAN_POINT ( 'NONE',  ( -15.80617190586768217, 15.72974639402176855, 98.12609039468570415 ) ) ;
#124809=CARTESIAN_POINT ( 'NONE',  ( 9.474510206698971260, -16.51473224551069308, 107.9155762719810383 ) ) ;
#124810=CARTESIAN_POINT ( 'NONE',  ( -4.379528057220086978, -16.55341960407618274, 84.79275706135234714 ) ) ;
#124812=CARTESIAN_POINT ( 'NONE',  ( 9.564922557961047289, -16.46253265017146816, 70.41775706135233293 ) ) ;
#124813=CARTESIAN_POINT ( 'NONE',  ( 19.02544592524334988, 5.153800228976608722, 36.45942372801900433 ) ) ;
#124814=CARTESIAN_POINT ( 'NONE',  ( -17.50000000000000355, -5.622605283950894872, 46.31207310596113302 ) ) ;
#124815=CARTESIAN_POINT ( 'NONE',  ( 19.03943276465977164, -0.05219959533909143690, 33.74890960531435979 ) ) ;
#124816=CARTESIAN_POINT ( 'NONE',  ( 8.314922557960818139, 14.29746914071049879, 39.58224293864769550 ) ) ;
#124817=CARTESIAN_POINT ( 'NONE',  ( -17.44270441346516876, -5.991230190323022953, 111.3633507926423079 ) ) ;
#124818=CARTESIAN_POINT ( 'NONE',  ( -4.379528057220328563, 16.55341960407611168, 25.20724293864769550 ) ) ;
#124819=CARTESIAN_POINT ( 'NONE',  ( -19.39720447994791286, -5.500000000000075495, 84.66317477297172900 ) ) ;
#124820=CARTESIAN_POINT ( 'NONE',  ( 4.483927247898790824, -16.52544592524335698, 100.2094237280190043 ) ) ;
#124821=CARTESIAN_POINT ( 'NONE',  ( -5.153800228976328057, -19.02544592524343514, 37.29057627198102409 ) ) ;
#124822=CARTESIAN_POINT ( 'NONE',  ( -5.719274019375665041, -21.55341960407619695, 99.79275706135234714 ) ) ;
#124823=CARTESIAN_POINT ( 'NONE',  ( 19.02544592524334988, 5.153800228976608722, 106.4594237280190185 ) ) ;
#124824=CARTESIAN_POINT ( 'NONE',  ( -10.72451020669870658, -18.67979575497194134, 79.58442372801903275 ) ) ;
#124825=CARTESIAN_POINT ( 'NONE',  ( 5.153800228976615827, -19.02544592524334988, 50.20942372801897591 ) ) ;
#124826=CARTESIAN_POINT ( 'NONE',  ( -5.153800228976328057, -19.02544592524343514, 97.29057627198099567 ) ) ;
#124827=CARTESIAN_POINT ( 'NONE',  ( 13.97604488694527802, 13.89961937509977652, 69.37390960531436690 ) ) ;
#124830=CARTESIAN_POINT ( 'NONE',  ( -14.29746914071049879, 8.314922557960819915, 70.83224293864770971 ) ) ;
#124831=CARTESIAN_POINT ( 'NONE',  ( 21.53943276465977519, -0.05219959533907433946, 63.74890960531435979 ) ) ;
#124832=CARTESIAN_POINT ( 'NONE',  ( 16.46253265017160672, -9.564922557960803928, 63.33224293864769550 ) ) ;
#124833=CARTESIAN_POINT ( 'NONE',  ( -15.80617190586745835, -15.72974639402198527, 81.87390960531435269 ) ) ;
#124834=CARTESIAN_POINT ( 'NONE',  ( -0.05219959533934338120, 16.53943276465976808, 77.50109039468567573 ) ) ;
#124836=CARTESIAN_POINT ( 'NONE',  ( 13.89961937509977652, -13.97604488694527269, 48.12390960531435979 ) ) ;
#124837=CARTESIAN_POINT ( 'NONE',  ( 16.55341960407611168, 4.379528057220329451, 78.95724293864769550 ) ) ;
#124839=CARTESIAN_POINT ( 'NONE',  ( 13.89961937509977652, -13.97604488694527269, 48.12390960531435979 ) ) ;
#124840=CARTESIAN_POINT ( 'NONE',  ( -16.55341960407611168, -4.379528057220339221, 111.4572429386476813 ) ) ;
#124841=CARTESIAN_POINT ( 'NONE',  ( -19.05341960407617563, 5.049401038297882671, 68.54275706135230450 ) ) ;
#124842=CARTESIAN_POINT ( 'NONE',  ( -14.29746914071049879, 8.314922557960819915, 80.83224293864769550 ) ) ;
#124843=CARTESIAN_POINT ( 'NONE',  ( 21.52544592524334988, 5.823673210054432836, 41.45942372801901143 ) ) ;
#124844=CARTESIAN_POINT ( 'NONE',  ( 19.02544592524343514, -5.153800228976328945, 33.54057627198102409 ) ) ;
#124845=CARTESIAN_POINT ( 'NONE',  ( -5.719274019375978568, 21.55341960407610458, 105.2072429386477097 ) ) ;
#124847=CARTESIAN_POINT ( 'NONE',  ( 12.06949235617757843, -12.14591786802309237, 83.12390960531436690 ) ) ;
#124849=CARTESIAN_POINT ( 'NONE',  ( 0.05219959533909260263, 19.03943276465977164, 49.99890960531435979 ) ) ;
#124851=CARTESIAN_POINT ( 'NONE',  ( -16.46253265017146816, -9.564922557961047289, 89.16775706135234714 ) ) ;
#124852=CARTESIAN_POINT ( 'NONE',  ( 13.97604488694527802, 13.89961937509977652, 99.37390960531436690 ) ) ;
#124853=CARTESIAN_POINT ( 'NONE',  ( 10.72451020669871369, 18.67979575497193778, 37.08442372801901143 ) ) ;
#124854=CARTESIAN_POINT ( 'NONE',  ( 5.153800228976335163, 19.02544592524342804, 84.79057627198099567 ) ) ;
#124855=CARTESIAN_POINT ( 'NONE',  ( 16.51473224551083163, -9.474510206698727899, 75.83442372801900433 ) ) ;
#124856=CARTESIAN_POINT ( 'NONE',  ( 0.05219959533909260263, 19.03943276465977164, 39.99890960531436690 ) ) ;
#124858=CARTESIAN_POINT ( 'NONE',  ( -12.14591786802309592, -12.06949235617757132, 81.87390960531435269 ) ) ;
#124859=CARTESIAN_POINT ( 'NONE',  ( 8.314922557960818139, 14.29746914071049879, 64.58224293864769550 ) ) ;
#124860=CARTESIAN_POINT ( 'NONE',  ( -16.46253265017160317, 9.564922557960807481, 80.83224293864769550 ) ) ;
#124861=CARTESIAN_POINT ( 'NONE',  ( -15.80617190586745835, -15.72974639402198527, 106.8739096053143811 ) ) ;
#124862=CARTESIAN_POINT ( 'NONE',  ( -0.05219959533909027116, -19.03943276465977164, 72.49890960531435269 ) ) ;
#124863=CARTESIAN_POINT ( 'NONE',  ( 19.02544592524334988, 5.153800228976608722, 21.45942372801899012 ) ) ;
#124864=CARTESIAN_POINT ( 'NONE',  ( -13.89961937509977652, 13.97604488694528158, 35.62390960531435269 ) ) ;
#124865=CARTESIAN_POINT ( 'NONE',  ( -16.52544592524342804, 4.483927247898546575, 36.04057627198102409 ) ) ;
#124866=CARTESIAN_POINT ( 'NONE',  ( 0.05219959533910956823, 16.53943276465976808, 104.9989096053143669 ) ) ;
#124867=CARTESIAN_POINT ( 'NONE',  ( 5.153800228976615827, -19.02544592524334988, 105.2094237280190185 ) ) ;
#124868=ORIENTED_EDGE ( 'NONE', *, *, #41146, .T. ) ;
#124869=CARTESIAN_POINT ( 'NONE',  ( 10.81492255796106328, -18.62759615963255655, 25.41775706135235779 ) ) ;
#124870=CARTESIAN_POINT ( 'NONE',  ( 13.89961937509957401, 13.97604488694547697, 66.87609039468567573 ) ) ;
#124871=CARTESIAN_POINT ( 'NONE',  ( 8.224510206698742110, 14.34966873604972548, 112.0844237280190185 ) ) ;
#124872=CARTESIAN_POINT ( 'NONE',  ( 5.719274019375991003, -21.55341960407610458, 67.70724293864769550 ) ) ;
#124873=CARTESIAN_POINT ( 'NONE',  ( 13.97604488694527802, 13.89961937509977652, 109.3739096053143669 ) ) ;
#124874=CARTESIAN_POINT ( 'NONE',  ( -0.05219959533910754901, -16.53943276465976808, 52.49890960531435979 ) ) ;
#124875=CARTESIAN_POINT ( 'NONE',  ( 13.89961937509977652, -13.97604488694527269, 33.12390960531434558 ) ) ;
#124876=CARTESIAN_POINT ( 'NONE',  ( -0.05219959533909027116, -19.03943276465977164, 52.49890960531436690 ) ) ;
#124877=CARTESIAN_POINT ( 'NONE',  ( 19.02544592524334988, 5.153800228976608722, 31.45942372801900433 ) ) ;
#124878=CARTESIAN_POINT ( 'NONE',  ( -16.55341960407617563, 4.379528057220093196, 83.54275706135234714 ) ) ;
#124879=CARTESIAN_POINT ( 'NONE',  ( -12.14591786802326823, 12.06949235617739902, 53.12609039468568284 ) ) ;
#124880=CARTESIAN_POINT ( 'NONE',  ( 15.80617190586746368, 15.72974639402197994, 24.37390960531435979 ) ) ;
#124881=CARTESIAN_POINT ( 'NONE',  ( 15.72974639402176855, 15.80617190586768217, 106.8760903946856899 ) ) ;
#124882=CARTESIAN_POINT ( 'NONE',  ( 19.02544592524343514, -5.153800228976328945, 78.54057627198099567 ) ) ;
#124884=CARTESIAN_POINT ( 'NONE',  ( -8.314922557961024197, 14.29746914071037800, 57.91775706135234714 ) ) ;
#124885=CARTESIAN_POINT ( 'NONE',  ( -16.55341960407611168, -4.379528057220339221, 106.4572429386477097 ) ) ;
#124886=CARTESIAN_POINT ( 'NONE',  ( -0.05219959533934338120, 16.53943276465976808, 112.5010903946857042 ) ) ;
#124887=CARTESIAN_POINT ( 'NONE',  ( -17.49999999999999645, -5.500000000000000888, 120.0000000000000142 ) ) ;
#124888=CARTESIAN_POINT ( 'NONE',  ( 21.52544592524334988, 5.823673210054432836, 66.45942372801903275 ) ) ;
#124889=CARTESIAN_POINT ( 'NONE',  ( -16.51473224551069308, -9.474510206698971260, 96.66557627198102409 ) ) ;
#124890=CARTESIAN_POINT ( 'NONE',  ( -9.474510206698964154, 16.51473224551069663, 80.41557627198103830 ) ) ;
#124891=CARTESIAN_POINT ( 'NONE',  ( -16.46253265017160317, 9.564922557960807481, 115.8322429386477097 ) ) ;
#124892=CARTESIAN_POINT ( 'NONE',  ( 8.314922557960818139, 14.29746914071049879, 54.58224293864769550 ) ) ;
#124893=CARTESIAN_POINT ( 'NONE',  ( 12.06949235617739724, 12.14591786802326823, 106.8760903946856899 ) ) ;
#124894=CARTESIAN_POINT ( 'NONE',  ( -8.314922557960811034, -14.29746914071050412, 47.08224293864770260 ) ) ;
#124895=CARTESIAN_POINT ( 'NONE',  ( 14.34966873604972726, -8.224510206698740333, 35.83442372801901143 ) ) ;
#124897=CARTESIAN_POINT ( 'NONE',  ( 9.474510206698729675, 16.51473224551082808, 37.08442372801899722 ) ) ;
#124898=CARTESIAN_POINT ( 'NONE',  ( -13.89961937509977652, 13.97604488694528158, 75.62390960531438111 ) ) ;
#124899=CARTESIAN_POINT ( 'NONE',  ( 9.564922557961047289, -16.46253265017146816, 50.41775706135233293 ) ) ;
#124900=CARTESIAN_POINT ( 'NONE',  ( 16.46253265017146816, 9.564922557961045513, 61.66775706135234003 ) ) ;
#124901=CARTESIAN_POINT ( 'NONE',  ( 19.03943276465977164, 0.05219959533936151252, 96.25109039468567573 ) ) ;
#124902=CARTESIAN_POINT ( 'NONE',  ( -4.483927247898782831, 16.52544592524335698, 87.70942372801901854 ) ) ;
#124904=CARTESIAN_POINT ( 'NONE',  ( 19.05341960407611168, 5.049401038298154454, 28.95724293864769550 ) ) ;
#124905=CARTESIAN_POINT ( 'NONE',  ( 13.89961937509977652, -13.97604488694527269, 103.1239096053143527 ) ) ;
#124906=CARTESIAN_POINT ( 'NONE',  ( 18.67979575497194134, -10.72451020669871369, 40.83442372801901854 ) ) ;
#124907=CARTESIAN_POINT ( 'NONE',  ( -9.564922557961040184, 16.46253265017147172, 87.91775706135233293 ) ) ;
#124909=CARTESIAN_POINT ( 'NONE',  ( -16.46253265017160317, 9.564922557960807481, 65.83224293864769550 ) ) ;
#124910=CARTESIAN_POINT ( 'NONE',  ( 19.02544592524343514, -5.153800228976328945, 98.54057627198100988 ) ) ;
#124911=CARTESIAN_POINT ( 'NONE',  ( -14.29746914071049879, 8.314922557960819915, 60.83224293864769550 ) ) ;
#124912=CARTESIAN_POINT ( 'NONE',  ( 9.564922557960805705, 16.46253265017160317, 49.58224293864770260 ) ) ;
#124913=CARTESIAN_POINT ( 'NONE',  ( -19.03943276465977164, 0.05219959533909376836, 66.24890960531436690 ) ) ;
#124914=CARTESIAN_POINT ( 'NONE',  ( 19.03943276465977164, 0.05219959533936151252, 71.25109039468566152 ) ) ;
#124915=CARTESIAN_POINT ( 'NONE',  ( -0.05219959533936034679, 19.03943276465977164, 37.50109039468567573 ) ) ;
#124916=CARTESIAN_POINT ( 'NONE',  ( 16.51473224551069308, 9.474510206698969483, 74.16557627198103830 ) ) ;
#124917=( BOUNDED_SURFACE ( )  B_SPLINE_SURFACE ( 3, 2, ( 
 ( #155515, #95825, #172679, #16018, #140337, #173684, #35151, #110004, #2824, #64502, #78662, #170690, #141337, #19004, #1827, #33174, #174672, #80650, #126169, #63509, #36137, #154521, #125184, #77675, #62497, #142326, #186880, #81623, #3806, #171685, #187864, #139344, #124168, #188853, #18012, #48350, #185870, #156511, #65484, #127146, #50337, #96807, #111994, #47356, #158493, #19980, #143306, #4792, #66482, #128144, #109011, #101811, #117991, #21981, #148324, #133145, #193842, #56309, #82629, #7796, #146307, #129133, #163499, #38152, #23983, #24997, #144311, #5801, #84629, #179681, #39143, #97789, #159478, #54314, #85639, #191824, #175663, #100798, #162481, #194836, #147326, #69479, #20972, #6793, #161492, #67474, #190831, #68472, #145310, #130127, #115986, #8813, #52307, #70483, #113964, #37137, #132149, #178670, #131145, #9819, #98797, #53304, #83633, #114983, #160491, #176676, #99806, #22980, #55306, #86641, #177675, #192833, #71480, #116978, #40133, #197819, #43139, #104808, #88637, #180680, #44137, #138122, #135166, #89634, #59285, #119974, #41153, #12811, #196839, #58306, #137126, #105796, #74478, #118997, #199803, #164501, #181660, #29956, #90619, #42156, #61270, #103816, #167482, #122940, #166497, #151322, #120954, #27995, #102816, #136143, #182653, #28977, #198813, #152301, #13785, #165496, #25994, #87637, #75452, #91594, #60278, #26992, #149323, #121951, #150333, #183644, #10817, #45126, #106784, #11828, #72487, #76445, #73493, #134160, #195848, #168459, #153284, #14785, #57321, #140092, #32934, #81385, #92597, #18763, #48107, #108770, #15777, #124939, #141096, #157267, #156268, #65246, #16768, #77436, #80410, #109763, #49098, #79425, #47111, #582, #78416, #188612, #4549, #170448, #34910, #19744, #142082, #143070, #169448, #94589, #17769, #139108, #50093, #186636, #110755, #111753, #30950, #154287, #171447, #66242, #125929, #184627, #46109, #2583, #172437, #1584, #62253, #187628, #33925, #107763, #95582, #64263, #123922, #93593, #3568, #185621, #31939, #155279, #63259, #126906, #173441, #96566, #158254, #38907, #20729, #9579, #115749, #8571, #114738, #39895, #127902, #21739, #52068, #83391, #189604, #190592, #113725, #86403, #85394, #193598, #7549, #144074, #55070, #97547, #116740, #84388, #129881, #191580, #175421, #37906, #100564, #178430, #101563, #69236, #163254, #177437, #162244, #51077, #145068, #36890, #98555, #160249, #24756, #6549, #5555, #176432, #112738, #146065, #174431, #70246, #82386, #22740, #130902, #192592, #148088, #35901, #67234, #23744, #53059, #99565, #159234, #54075, #128892, #147087, #68228, #161246, #131914, #135909, #153037, #56067, #102580, #181426, #13547, #132909, #194596, #167242, #43893, #40907, #136884, #73255, #166252, #29714, #149090, #117747, #42904, #41916, #196602, #197580, #28740, #179441, #150084, #152062, #58073, #151083, #182413, #11588, #27752, #164264, #12574, #105556, #104569, #71245, #134925, #10580, #183401, #121708, #57081, #89395, #72241, #198570, #74240, #25759, #59047, #133918, #87405, #120713, #90377, #195608, #103582, #118755, #75213, #60040, #165257, #180444, #44884, #26751, #88390, #119743, #106540, #168217, #91346, #156021, #37402, #1333, #47866, #172189, #107522, #185374, #92355, #154041, #76198, #48853, #15536, #94342, #171201, #137877, #343, #33674, #95336, #170205, #63013, #124692, #77194, #30705, #186389, #199558, #93347, #14537, #32691, #140847, #108526, #138863, #17518, #79176, #114226, #2336, #109519, #61027, #123676, #78175, #122699, #175931, #46865, #62011, #31698, #64017, #125686, #184388, #187384, #169198, #99061, #110508, #157021, #18519, #129395, #45869, #155033, #16528, #139844, #80166, #141838, #6059, #67737, #191091, #52566, #40408, #176939, #26256, #130390, #87897, #117246, #162748, #24256, #8063, #100066, #163764, #57584, #54572, #9079, #178938, #39403, #160749, #132417, #116244, #177936, #56582, #25264 ),
 ( #102079, #85906, #161751, #119254, #196114, #23246, #180938, #7050, #86907, #69740, #149583, #148590, #101063, #70749, #42413, #68732, #195100, #147594, #84890, #192087, #194109, #10082, #133411, #55572, #41414, #193096, #53569, #118256, #71740, #179947, #103080, #146569, #38409, #164761, #11081, #22241, #131409, #72757, #83890, #134428, #145573, #115247, #14042, #152554, #135426, #169718, #44398, #30214, #108032, #150592, #88902, #90869, #185897, #45387, #104076, #181920, #62524, #183902, #28259, #182912, #124197, #107040, #29236, #43401, #165758, #139370, #166756, #851, #12091, #168712, #13070, #31211, #91857, #59544, #75708, #27252, #73754, #138383, #167738, #89898, #197097, #106052, #60535, #76707, #137386, #184891, #136400, #58564, #200064, #199066, #153549, #122211, #151581, #120230, #198077, #92862, #105071, #74737, #154549, #121222, #61532, #15046, #123201, #46373, #16044, #77703, #20008, #141365, #142354, #158520, #93864, #170716, #126197, #113006, #19032, #47382, #109037, #80678, #127174, #2852, #186907, #3834, #65513, #32207, #112024, #157538, #17036, #79695, #172709, #78690, #155542, #64530, #187893, #49360, #50365, #173713, #48378, #81651, #110035, #140367, #143335, #189871, #188884, #1854, #63536, #34193, #111023, #95854, #125211, #35181, #96836, #171713, #33203, #94861, #66510, #4822, #156542, #128172, #18041, #51346, #29875, #91513, #75373, #167404, #30872, #124858, #121870, #76365, #184549, #106706, #27915, #199723, #183563, #45048, #123841, #92518, #61189, #105717, #186557, #151244, #168380, #16688, #77358, #28900, #139025, #122861, #153199, #90540, #78338, #74399, #12733, #136065, #138042, #62177, #31860, #169363, #48029, #14704, #46030, #185539, #120874, #198735, #152222, #13707, #89558, #47033, #137043, #107685, #154208, #197739, #60200, #108690, #170368, #15697, #505, #93513, #155199, #44057, #140012, #59205, #1500, #63178, #109686, #182574, #21655, #50997, #83308, #20647, #159151, #32855, #126823, #18680, #80327, #157186, #144985, #141999, #187549, #158173, #171367, #189525, #94505, #113644, #64182, #66156, #127819, #112658, #6466, #129798, #110671, #143991, #96484, #19664, #68147, #174349, #156187, #97466, #191497, #17686, #35820, #82300, #52973, #79344, #2502, #81305, #175338, #141015, #125848, #67155, #5472, #49016, #36805, #173359, #128812, #172351, #33840, #95500, #142989, #3487, #4467, #190511, #51985, #65164, #50006, #98471, #160164, #188529, #111672, #34829, #88696, #27050, #72543, #86695, #105854, #182710, #9874, #44195, #193898, #150392, #56365, #74535, #11888, #102869, #195906, #167541, #55362, #181715, #10873, #71534, #178727, #87692, #26047, #28053, #134220, #73551, #194891, #57381, #166554, #29036, #135224, #58363, #119054, #147382, #149377, #25052, #59343, #197875, #133200, #180736, #148379, #136200, #196896, #40189, #42212, #118048, #101869, #120030, #103872, #163552, #179738, #41208, #43198, #165553, #164554, #104865, #121012, #117032, #132207, #89694, #151380, #12870, #8871, #70538, #110822, #77499, #123986, #48172, #183703, #61331, #168519, #30017, #152358, #125006, #91655, #170513, #47174, #13843, #76508, #109829, #171512, #46172, #139169, #646, #153344, #106844, #62316, #75510, #169509, #185684, #63328, #17835, #141162, #32003, #2651, #140158, #78485, #137183, #107825, #138184, #199867, #123002, #64328, #184688, #14845, #108833, #90676, #93660, #198871, #33001, #45190, #155345, #16834, #1650, #125995, #49163, #31009, #186701, #15840, #94655, #187693, #156335, #60338, #79493, #172504, #122012, #92658, #154347, #115815, #18830, #65311, #144139, #176498, #95647, #157335, #129948, #6618, #3632, #99632, #35964, #128959, #192658, #111818, #80475, #5621, #4615, #159300, #98621, #191648, #142148, #173506, #126971, #67300, #66307, #20796, #160315, #53127, #188679, #112804, #114805, #82451, #113792, #81449, #190659, #37974, #54141, #175487, #145135, #52135 ),
 ( #68297, #97611, #158320, #50159, #174497, #36959, #34979, #21805, #127967, #96632, #22808, #19808, #143136, #189670, #83457, #161314, #84454, #146132, #33991, #7618, #69302, #130968, #51143, #148156, #55137, #116807, #38974, #11659, #178499, #57150, #133988, #100631, #163326, #196675, #58144, #132977, #25827, #87472, #39965, #193666, #164333, #162312, #56137, #149159, #150158, #104640, #27824, #118828, #89466, #26821, #165329, #23813, #194667, #24822, #86471, #9648, #151155, #71314, #101635, #10649, #177505, #195679, #85463, #119812, #70312, #72311, #180512, #41985, #12645, #135979, #117818, #73325, #102648, #103651, #74312, #88462, #147152, #134996, #197650, #8640, #181497, #42975, #59116, #131981, #179511, #166327, #40979, #182482, #43963, #16596, #93416, #90450, #186461, #122769, #15604, #79251, #105625, #30778, #169271, #152134, #47939, #61096, #46937, #124764, #167313, #28809, #107593, #2409, #62084, #120782, #13617, #77262, #108597, #14611, #198644, #123748, #185447, #17591, #170274, #92425, #75284, #29784, #184458, #136955, #140923, #91420, #168288, #153107, #138931, #31767, #60110, #155103, #121778, #183471, #78244, #1406, #154111, #32762, #44956, #76268, #106613, #137946, #199629, #45938, #411, #139916, #63085, #109591, #171274, #94414, #156094, #33750, #129713, #20559, #66067, #127733, #111579, #3399, #67066, #161074, #158084, #112569, #82210, #142900, #64088, #35732, #19576, #81219, #160075, #128724, #97379, #141908, #22569, #187457, #4382, #52886, #113556, #65074, #84215, #159065, #191410, #37729, #5383, #143901, #189435, #126732, #145895, #99391, #188435, #125757, #110579, #190421, #173263, #114561, #51897, #50911, #174264, #48925, #172260, #98378, #175250, #49914, #95408, #157094, #36715, #21562, #83222, #144897, #96396, #18590, #6379, #68059, #176258, #80237, #34738, #23570, #101385, #11411, #27583, #131741, #57904, #42736, #103405, #166080, #100396, #179270, #70073, #38738, #72063, #117569, #162074, #104398, #87234, #8398, #194426, #163078, #193423, #196434, #53904, #192422, #115579, #55896, #41741, #73080, #148917, #89221, #40734, #102404, #165083, #85218, #178261, #146909, #54898, #69063, #26577, #116572, #10406, #164091, #130730, #39722, #88220, #149904, #24581, #25590, #133737, #86230, #147920, #195431, #177267, #9406, #56907, #180271, #134752, #119576, #118581, #181259, #7378, #71072, #132738, #106367, #198392, #59869, #136711, #62839, #121536, #167070, #137704, #150914, #169024, #12408, #93178, #43722, #45700, #107351, #30529, #186218, #109349, #90208, #123511, #76029, #199389, #47699, #92182, #74070, #77020, #171031, #135741, #153866, #15364, #32522, #197412, #182237, #60853, #154863, #58878, #120544, #46695, #185204, #105383, #16361, #152869, #138692, #28571, #151891, #13381, #122528, #183231, #184218, #173, #108356, #75045, #29547, #31525, #61841, #170035, #44712, #78009, #139676, #168050, #1164, #124523, #91180, #14364, #34508, #172024, #6144, #144661, #80010, #4148, #33513, #21327, #97147, #191180, #188203, #142669, #50676, #173029, #94174, #65827, #49675, #111339, #190183, #158830, #127496, #95172, #52655, #17350, #96166, #82985, #143658, #156860, #114318, #189201, #159832, #67826, #35497, #174026, #19346, #18355, #176020, #129481, #141679, #155853, #140680, #20318, #3170, #79006, #81966, #157855, #112336, #2172, #63852, #128487, #80994, #64843, #125523, #187220, #5142, #66824, #51658, #175014, #126505, #48690, #113322, #36478, #98135, #110343, #100154, #53660, #131494, #41503, #57672, #161835, #87983, #72844, #133495, #196200, #22329, #147679, #85990, #68823, #103167, #178017, #163850, #164847, #83979, #145659, #24340, #119339, #179024, #37489, #99151, #194191, #25351, #193181, #115337, #40492, #102164, #134514, #86992, #9167, #160840, #146656, #101145, #7140, #130482, #8150, #84973, #69827, #55656, #148679, #192179, #10167, #177028, #38498, #71827, #118341 ),
 ( #23330, #26343, #54654, #149671, #117328, #39484, #162831, #116328, #70834, #195187, #132502, #56668, #180034, #11169, #42499, #76788, #153631, #150677, #46453, #182997, #75792, #139447, #58646, #104163, #90948, #151662, #106135, #45466, #138459, #165844, #59631, #61609, #167819, #60616, #28342, #29318, #200140, #929, #122291, #91938, #152635, #181025, #121305, #120312, #92941, #31290, #166841, #14125, #182005, #108113, #183980, #73840, #137470, #43488, #12175, #107120, #199150, #135511, #77779, #168791, #105155, #30293, #74819, #89981, #169797, #27341, #88987, #197181, #15126, #123278, #184969, #154629, #62603, #16124, #13156, #136481, #198161, #44480, #1936, #63615, #185977, #158596, #125290, #3914, #80758, #47461, #110115, #143415, #4903, #79775, #172792, #34273, #186987, #140446, #111102, #109117, #2932, #95932, #96913, #51422, #174774, #65594, #36240, #173792, #112102, #170796, #141445, #171793, #33281, #94940, #97892, #156625, #48458, #157617, #124281, #142435, #32288, #66586, #17118, #19108, #127254, #188967, #159584, #82737, #18120, #20085, #49440, #50443, #21081, #35259, #93943, #81730, #144418, #155622, #128250, #189947, #5904, #78769, #64611, #113082, #126274, #187971, #145414, #70587, #8919, #164601, #55410, #177776, #190935, #176780, #131250, #52412, #26095, #38252, #115088, #99907, #85745, #132256, #37245, #178776, #160595, #149424, #117081, #148428, #54416, #179786, #67581, #161592, #191926, #23086, #129239, #130231, #53410, #87739, #25101, #133248, #147432, #83735, #194940, #98901, #56416, #24090, #69584, #192939, #84731, #6896, #193947, #114070, #146409, #116088, #40242, #7899, #175769, #39246, #100902, #162586, #163600, #101918, #86743, #68574, #22084, #9923, #71582, #118096, #41255, #102917, #172286, #108624, #79279, #187485, #155131, #93444, #138959, #153134, #33776, #48951, #76296, #110604, #57427, #16624, #122796, #140949, #78272, #169297, #62113, #95436, #119100, #47966, #77289, #137974, #44981, #72593, #46965, #123776, #186490, #94440, #45965, #106641, #109618, #438, #139945, #170302, #199656, #29810, #107619, #17620, #10920, #61122, #64118, #134267, #171302, #195954, #183497, #185475, #31795, #168314, #2436, #154140, #1435, #125783, #91446, #14637, #63113, #184486, #124791, #30803, #92452, #15632, #32788, #156121, #191433, #161098, #98404, #177292, #143925, #190446, #114586, #49942, #127757, #34766, #96423, #18616, #52910, #158109, #36740, #113580, #80263, #142924, #176283, #37755, #112594, #5406, #67090, #19601, #173292, #128749, #141933, #35756, #51921, #129736, #84241, #7403, #160100, #69087, #6403, #144921, #3424, #174286, #4406, #66091, #189458, #130754, #50936, #81243, #175274, #157120, #21587, #65100, #99416, #111607, #83245, #68084, #22593, #192446, #115603, #97401, #145920, #82235, #53928, #38762, #126758, #188461, #159088, #20583, #162101, #56936, #165113, #182268, #85244, #131766, #10434, #42765, #23597, #146935, #196463, #73111, #70097, #166110, #102430, #195461, #58907, #178285, #8425, #72092, #71096, #25615, #26605, #57933, #193448, #179297, #181287, #87259, #180300, #147945, #148944, #119604, #120574, #41768, #11440, #133766, #100420, #40761, #39748, #12438, #150944, #86255, #118610, #101411, #27612, #103433, #54924, #88248, #163103, #116596, #149933, #134781, #24607, #197441, #104427, #9431, #89252, #194450, #132763, #74100, #55921, #117596, #164117, #135770, #183260, #123543, #204, #105414, #29576, #62872, #124553, #199419, #92214, #153900, #44741, #59898, #30563, #28599, #122560, #15395, #16392, #171061, #94204, #185236, #155884, #93209, #31558, #167098, #60883, #91207, #152897, #14394, #17381, #76060, #121566, #77052, #43751, #61873, #90237, #186250, #136739, #138723, #46728, #108390, #79037, #2202, #106397, #78039, #169056, #170067, #140712, #154894, #151920, #139708, #63883, #13409, #1195, #47728, #125554, #75073, #198423, #109381, #32551 ),
 ( #168079, #137735, #184250, #45732, #107384, #36510, #64872, #145691, #81997, #52685, #160871, #128517, #66855, #112367, #126533, #7173, #22361, #49705, #84013, #33542, #190212, #96196, #114348, #51691, #142699, #35527, #68856, #95204, #21358, #50709, #111371, #18387, #48720, #20349, #97175, #159865, #67855, #19374, #80038, #83015, #174058, #113353, #143690, #173060, #3198, #81023, #191210, #187251, #34537, #37520, #110373, #144690, #172055, #129510, #158860, #99182, #156891, #4178, #157885, #65856, #141707, #127527, #189231, #188232, #6175, #176053, #175045, #5172, #98165, #100186, #196234, #87026, #132534, #194223, #178049, #69860, #133528, #27371, #24373, #179058, #148711, #9201, #130515, #102198, #86024, #147713, #26376, #195220, #163886, #8184, #89018, #53694, #70866, #119372, #180068, #131529, #150709, #25383, #57703, #104194, #71859, #10199, #55688, #193213, #12208, #165875, #54687, #192211, #40527, #116360, #56701, #39517, #181055, #118374, #23362, #41536, #101177, #161868, #103200, #164881, #85008, #115371, #88015, #162865, #117362, #149703, #11201, #42531, #177060, #38530, #146688, #72877, #134545, #77810, #15159, #93974, #60650, #107152, #31323, #166872, #44512, #151695, #13186, #135541, #108146, #74849, #153663, #30327, #197212, #59663, #92975, #154660, #29351, #122323, #184015, #136512, #90011, #45497, #58675, #152667, #168822, #46486, #961, #124313, #76819, #186011, #123309, #61641, #120342, #90980, #121336, #183029, #106168, #47493, #167851, #198193, #91969, #73871, #138490, #182037, #43519, #169830, #14157, #200172, #185002, #105185, #75825, #16156, #139479, #137503, #62637, #109150, #199183, #170829, #32321, #28373, #155654, #127282, #189976, #144448, #67609, #96943, #129270, #66615, #4932, #78802, #172821, #64641, #126303, #2961, #190964, #187999, #33311, #3943, #17149, #35287, #140480, #159616, #110144, #112131, #173823, #158624, #52441, #175802, #156655, #51451, #142465, #65622, #114099, #20115, #1968, #143446, #37275, #63648, #81759, #128279, #98932, #125323, #48490, #188995, #21112, #187020, #171823, #113112, #174802, #94971, #82767, #19136, #36268, #18151, #79805, #141477, #50471, #49469, #97923, #5933, #111132, #34301, #95963, #157647, #80787, #40275, #7930, #85775, #179814, #119128, #101948, #71611, #132286, #160623, #177806, #25132, #146439, #70620, #69614, #193978, #38282, #87767, #163629, #53442, #55440, #23116, #191956, #86774, #117111, #115117, #57456, #148458, #161622, #147462, #54447, #84761, #149452, #6926, #145444, #68604, #8952, #194968, #164630, #9952, #180809, #178805, #133277, #118126, #176810, #131280, #99936, #192968, #10948, #56447, #116117, #42288, #41284, #26125, #134297, #102946, #72622, #195983, #39276, #22114, #83764, #130260, #100933, #162617, #24123, #12941, #31086, #168589, #59418, #152429, #721, #11960, #138258, #167612, #28129, #135295, #165626, #137262, #13917, #76582, #184762, #136273, #196967, #199941, #29108, #30087, #198945, #166627, #120102, #197948, #107901, #124063, #89769, #154422, #139246, #61405, #62393, #88772, #75583, #60412, #58435, #169588, #44269, #91728, #92734, #150465, #73625, #90746, #185764, #45262, #103947, #27125, #122085, #153424, #121092, #181792, #106916, #14922, #43272, #123076, #183776, #104941, #74606, #46247, #151454, #182786, #105927, #15916, #77574, #65385, #50237, #16907, #158393, #140233, #129032, #35050, #128044, #34065, #159377, #47252, #141233, #171585, #2724, #108909, #109901, #33073, #5697, #4690, #112879, #127045, #63402, #174572, #78558, #36038, #3707, #49236, #110894, #94728, #186776, #111892, #144213, #64401, #95724, #188752, #126070, #170589, #18903, #187766, #172579, #143209, #173581, #80549, #125079, #67373, #32079, #157410, #142223, #156406, #1726, #96704, #19882, #48247, #93736, #81523, #17910, #66382, #189745, #79566, #97687, #155417, #51218, #20873, #82531, #24894, #194738, #132051, #10720 ),
 ( #176574, #9720, #71384, #146203, #39043, #100700, #130020, #6691, #177576, #175560, #69373, #162381, #163397, #117891, #41052, #70383, #102716, #40033, #178568, #52206, #7689, #38048, #99704, #161388, #164405, #22879, #68369, #23883, #190733, #8714, #113864, #133048, #83530, #85535, #147223, #193740, #25897, #149229, #191719, #86542, #115886, #55208, #87542, #116877, #37036, #101707, #72383, #98697, #148226, #56208, #160391, #21880, #145208, #179581, #53203, #114880, #84526, #131043, #192733, #54215, #199701, #136043, #28878, #92495, #11728, #195750, #44034, #104708, #59183, #198711, #91490, #57224, #12712, #14680, #120852, #13684, #181564, #182552, #153177, #154184, #75351, #45025, #105695, #134058, #151223, #60178, #119879, #167381, #43042, #90518, #73396, #61167, #137021, #26893, #118897, #89536, #166398, #27894, #74378, #46007, #197718, #150233, #152200, #180582, #121847, #42056, #76342, #88536, #183540, #106684, #168357, #169339, #15674, #135067, #29853, #138018, #122838, #30848, #184527, #103720, #107662, #165400, #196743, #58210, #172328, #142966, #480, #185516, #79320, #126799, #139001, #62154, #80304, #18658, #47008, #188505, #32830, #64159, #19641, #31837, #123818, #140990, #63154, #156162, #33817, #141977, #108667, #109662, #65142, #17660, #187527, #139986, #2478, #3465, #81283, #48992, #157164, #125824, #77334, #110647, #49984, #171342, #95477, #94481, #111648, #124833, #170345, #173334, #186533, #34807, #96462, #1475, #158150, #93488, #48006, #155174, #16665, #78313, #44678, #151856, #58843, #46661, #104362, #42701, #166046, #106331, #92146, #61808, #199355, #77976, #168017, #91147, #15328, #150879, #28537, #135707, #197378, #119542, #153832, #120510, #137668, #14330, #181225, #43686, #76987, #138658, #13347, #29513, #152836, #182201, #74036, #75995, #27546, #136676, #60820, #30495, #185170, #108320, #122494, #170000, #107318, #45667, #168991, #12373, #139643, #139, #123478, #184185, #31491, #57870, #75011, #105348, #198358, #89187, #167035, #90173, #16326, #93143, #154828, #59832, #121502, #183196, #170995, #69537, #160547, #5854, #67530, #51373, #140648, #6848, #100855, #97843, #52362, #22036, #82683, #1131, #175716, #159531, #21030, #99861, #68527, #37195, #78973, #162537, #124487, #144367, #192891, #53362, #2138, #24041, #98852, #131201, #177730, #145366, #83688, #129188, #66537, #85696, #7850, #39199, #128201, #191878, #130182, #113034, #54369, #115039, #190886, #114019, #62805, #109316, #38205, #176732, #189898, #32488, #186183, #161545, #23038, #84683, #146363, #36189, #94141, #116041, #47664, #155820, #17318, #174726, #108374, #110357, #95188, #34521, #155868, #80023, #15379, #93193, #188, #61857, #184234, #156874, #123526, #2185, #79020, #45715, #170050, #141692, #3183, #78023, #171045, #32535, #185220, #138707, #109363, #107368, #1178, #94188, #18371, #49690, #173044, #63867, #96181, #172039, #33526, #169040, #139692, #31541, #154878, #16376, #157870, #62855, #46711, #17365, #124537, #4162, #186234, #47713, #81008, #64856, #188217, #125538, #140695, #111355, #92198, #19359, #187234, #48704, #126518, #142683, #122544, #30546, #153882, #77036, #114331, #22344, #144673, #65840, #37502, #21340, #82998, #161851, #68839, #99164, #143674, #24355, #189214, #6158, #54669, #115353, #5155, #86006, #160854, #131509, #39500, #7156, #145674, #191193, #66838, #147695, #69842, #101160, #128501, #53675, #130498, #175028, #193196, #192194, #67838, #176034, #162848, #174042, #100169, #129495, #190196, #97160, #127510, #83995, #177043, #38513, #146671, #98147, #158844, #23345, #52669, #84990, #8166, #51674, #50693, #81981, #116343, #178032, #113336, #112351, #35511, #20332, #36493, #159847, #119355, #57687, #40509, #74833, #149687, #135525, #13170, #55671, #194206, #196217, #90962, #150692, #9182, #70848, #165859, #197196, #103183, #87008, #12190, #73855, #106151, #58659, #181039 ),
 ( #27355, #132517, #151677, #102180, #104177, #89001, #120325, #44495, #163868, #182020, #42513, #25367, #167833, #43503, #10183, #105169, #164863, #71843, #198175, #117345, #179041, #148695, #166855, #28357, #195204, #89995, #136495, #121319, #59645, #183011, #133512, #180051, #56684, #118358, #41520, #29334, #26359, #87999, #11185, #72860, #134530, #171806, #33294, #108128, #941, #62616, #91952, #168805, #139461, #137484, #31303, #124294, #125305, #79787, #2944, #32302, #64623, #1950, #140460, #14139, #169812, #200154, #61624, #138473, #126285, #123292, #30309, #185991, #152649, #170809, #75806, #94953, #45479, #47474, #109131, #93957, #187982, #111114, #153645, #187001, #77792, #155636, #49452, #17131, #199164, #78783, #172803, #60631, #63629, #48471, #34284, #122305, #183996, #110128, #156637, #107135, #15140, #18133, #141460, #76802, #184984, #154642, #46468, #92956, #16137, #157630, #5915, #66597, #21092, #160606, #53422, #19119, #174785, #176791, #82749, #175782, #143428, #144429, #115099, #54429, #37256, #6908, #67592, #95944, #113094, #22096, #81741, #129251, #4914, #190946, #173805, #23097, #98914, #188978, #52423, #158607, #161603, #69595, #83746, #145425, #114081, #35270, #116099, #99918, #131262, #96925, #68586, #130242, #128261, #84744, #191938, #51434, #38264, #192950, #3925, #146420, #159595, #20097, #127265, #80769, #7911, #177787, #142447, #65605, #189959, #50454, #112113, #36251, #97904, #134277, #101929, #136253, #55421, #120084, #165608, #163611, #89748, #74585, #135277, #197929, #24102, #149434, #87749, #70600, #104921, #179796, #27107, #43253, #85756, #147443, #26106, #121071, #180791, #39257, #100913, #195965, #88753, #133259, #117092, #42270, #103928, #59397, #150446, #10930, #162598, #148439, #102927, #8931, #132267, #9934, #86756, #193958, #72603, #166608, #11942, #178787, #57437, #40256, #181772, #25112, #119110, #73606, #196949, #71593, #194950, #56427, #58417, #164612, #28110, #118107, #151434, #41265, #12921, #17891, #44249, #139226, #47230, #64382, #167592, #13897, #92713, #125059, #105906, #29087, #78538, #155397, #152409, #48226, #184742, #77554, #141215, #60392, #90726, #154402, #153402, #107881, #108889, #140213, #75563, #61384, #63382, #169568, #62373, #30067, #137239, #2705, #91708, #14900, #124043, #170568, #168569, #183756, #93715, #198924, #182765, #32059, #186756, #31065, #94709, #122064, #76562, #106896, #138237, #45242, #199921, #123056, #46227, #1706, #109881, #185742, #15896, #171565, #701, #33054, #16887, #156387, #79545, #173562, #65366, #129013, #22860, #19863, #174550, #82509, #4671, #126050, #97666, #81503, #143191, #21860, #190713, #159355, #3687, #84507, #49217, #66363, #114859, #175540, #127026, #146185, #20853, #191700, #99685, #67353, #5677, #51198, #188733, #7670, #130000, #161369, #50218, #113844, #52186, #35031, #53184, #37015, #128023, #36017, #187747, #34046, #160369, #189725, #111872, #157391, #110875, #144191, #98676, #83510, #6671, #158374, #18884, #145187, #112859, #68349, #176554, #96686, #172560, #142204, #38029, #95703, #80530, #119862, #104692, #165382, #27876, #54196, #179562, #117872, #100681, #135050, #9701, #195732, #73378, #115868, #177557, #56189, #151207, #10702, #69354, #131023, #25879, #57205, #163377, #147203, #72365, #134039, #166380, #118880, #41032, #192712, #178549, #133029, #116858, #149211, #180564, #55189, #70364, #42038, #162363, #39026, #103702, #150214, #102698, #181547, #23864, #24874, #193721, #86523, #85515, #132032, #40015, #89517, #26875, #196726, #88518, #8694, #58194, #101688, #43026, #87524, #71365, #194719, #148207, #164386, #11711, #109645, #106667, #61149, #169323, #91473, #12695, #184511, #168340, #29836, #108650, #15658, #45991, #90502, #171327, #136027, #153161, #1460, #62138, #152184, #32815, #107646, #78297, #186517, #154167, #92478, #138000, #13668, #94466, #16650, #47991, #75335, #463 ) ),
 .UNSPECIFIED., .T., .F., .F. ) 
 B_SPLINE_SURFACE_WITH_KNOTS ( ( 4, 3, 4 ),
 ( 3, 2, 2, 2, 2, 2, 2, 2, 2, 2, 2, 2, 2, 2, 2, 2, 2, 2, 2, 2, 2, 2, 2, 2, 2, 2, 2, 2, 2, 2, 2, 2, 2, 2, 2, 2, 2, 2, 2, 2, 2, 2, 2, 2, 2, 2, 2, 2, 2, 2, 2, 2, 2, 2, 2, 2, 2, 2, 2, 2, 2, 2, 2, 2, 2, 2, 2, 2, 2, 2, 2, 2, 2, 2, 2, 2, 2, 2, 2, 2, 2, 2, 2, 2, 2, 2, 2, 2, 2, 2, 2, 2, 2, 2, 2, 2, 2, 2, 2, 2, 2, 2, 2, 2, 2, 2, 2, 2, 2, 2, 2, 2, 2, 2, 2, 2, 2, 2, 2, 2, 2, 2, 2, 2, 2, 2, 2, 2, 2, 2, 2, 2, 2, 2, 2, 2, 2, 2, 2, 2, 2, 2, 2, 2, 2, 2, 2, 2, 2, 2, 2, 2, 2, 2, 2, 2, 2, 2, 2, 2, 2, 2, 2, 2, 2, 2, 2, 2, 2, 2, 2, 2, 2, 2, 2, 2, 2, 2, 2, 2, 2, 2, 2, 2, 2, 2, 2, 2, 2, 2, 2, 2, 2, 2, 2, 2, 2, 2, 2, 2, 2, 2, 2, 2, 2, 2, 2, 2, 2, 2, 2, 2, 2, 2, 2, 2, 2, 2, 2, 2, 2, 2, 2, 2, 2, 2, 2, 2, 3 ),
 ( 0.000000000000000000, 0.5000000000000000000, 1.000000000000000000 ),
 ( 0.000000000000000000, 0.004385964912280701511, 0.008771929824561403022, 0.01315789473684210453, 0.01754385964912280604, 0.02192982456140350755, 0.02631578947368420907, 0.03070175438596491058, 0.03508771929824561209, 0.03947368421052631360, 0.04385964912280701511, 0.04824561403508771662, 0.05263157894736841813, 0.05701754385964911964, 0.06140350877192982115, 0.06578947368421052266, 0.07017543859649122417, 0.07456140350877192569, 0.07894736842105262720, 0.08333333333333332871, 0.08771929824561403022, 0.09210526315789473173, 0.09649122807017543324, 0.1008771929824561348, 0.1052631578947368363, 0.1096491228070175378, 0.1140350877192982393, 0.1184210526315789408, 0.1228070175438596423, 0.1271929824561403577, 0.1315789473684210453, 0.1359649122807017607, 0.1403508771929824483, 0.1447368421052631637, 0.1491228070175438514, 0.1535087719298245668, 0.1578947368421052544, 0.1622807017543859698, 0.1666666666666666574, 0.1710526315789473728, 0.1754385964912280604, 0.1798245614035087758, 0.1842105263157894635, 0.1885964912280701788, 0.1929824561403508665, 0.1973684210526315819, 0.2017543859649122695, 0.2061403508771929849, 0.2105263157894736725, 0.2149122807017543879, 0.2192982456140350755, 0.2236842105263157909, 0.2280701754385964786, 0.2324561403508771940, 0.2368421052631578816, 0.2412280701754385970, 0.2456140350877192846, 0.2500000000000000000, 0.2543859649122807154, 0.2587719298245614308, 0.2631578947368420907, 0.2675438596491228060, 0.2719298245614035214, 0.2763157894736842368, 0.2807017543859648967, 0.2850877192982456121, 0.2894736842105263275, 0.2938596491228070429, 0.2982456140350877027, 0.3026315789473684181, 0.3070175438596491335, 0.3114035087719298489, 0.3157894736842105088, 0.3201754385964912242, 0.3245614035087719396, 0.3289473684210526550, 0.3333333333333333148, 0.3377192982456140302, 0.3421052631578947456, 0.3464912280701754610, 0.3508771929824561209, 0.3552631578947368363, 0.3596491228070175517, 0.3640350877192982670, 0.3684210526315789269, 0.3728070175438596423, 0.3771929824561403577, 0.3815789473684210731, 0.3859649122807017330, 0.3903508771929824483, 0.3947368421052631637, 0.3991228070175438791, 0.4035087719298245390, 0.4078947368421052544, 0.4122807017543859698, 0.4166666666666666852, 0.4210526315789473450, 0.4254385964912280604, 0.4298245614035087758, 0.4342105263157894912, 0.4385964912280701511, 0.4429824561403508665, 0.4473684210526315819, 0.4517543859649122973, 0.4561403508771929571, 0.4605263157894736725, 0.4649122807017543879, 0.4692982456140351033, 0.4736842105263157632, 0.4780701754385964786, 0.4824561403508771940, 0.4868421052631579093, 0.4912280701754385692, 0.4956140350877192846, 0.5000000000000000000, 0.5043859649122807154, 0.5087719298245614308, 0.5131578947368421462, 0.5175438596491228616, 0.5219298245614034659, 0.5263157894736841813, 0.5307017543859648967, 0.5350877192982456121, 0.5394736842105263275, 0.5438596491228070429, 0.5482456140350877583, 0.5526315789473684736, 0.5570175438596490780, 0.5614035087719297934, 0.5657894736842105088, 0.5701754385964912242, 0.5745614035087719396, 0.5789473684210526550, 0.5833333333333333703, 0.5877192982456140857, 0.5921052631578946901, 0.5964912280701754055, 0.6008771929824561209, 0.6052631578947368363, 0.6096491228070175517, 0.6140350877192982670, 0.6184210526315789824, 0.6228070175438596978, 0.6271929824561403022, 0.6315789473684210176, 0.6359649122807017330, 0.6403508771929824483, 0.6447368421052631637, 0.6491228070175438791, 0.6535087719298245945, 0.6578947368421053099, 0.6622807017543859143, 0.6666666666666666297, 0.6710526315789473450, 0.6754385964912280604, 0.6798245614035087758, 0.6842105263157894912, 0.6885964912280702066, 0.6929824561403509220, 0.6973684210526315264, 0.7017543859649122417, 0.7061403508771929571, 0.7105263157894736725, 0.7149122807017543879, 0.7192982456140351033, 0.7236842105263158187, 0.7280701754385965341, 0.7324561403508771384, 0.7368421052631578538, 0.7412280701754385692, 0.7456140350877192846, 0.7500000000000000000, 0.7543859649122807154, 0.7587719298245614308, 0.7631578947368421462, 0.7675438596491228616, 0.7719298245614034659, 0.7763157894736841813, 0.7807017543859648967, 0.7850877192982456121, 0.7894736842105263275, 0.7938596491228070429, 0.7982456140350877583, 0.8026315789473684736, 0.8070175438596490780, 0.8114035087719297934, 0.8157894736842105088, 0.8201754385964912242, 0.8245614035087719396, 0.8289473684210526550, 0.8333333333333333703, 0.8377192982456140857, 0.8421052631578946901, 0.8464912280701754055, 0.8508771929824561209, 0.8552631578947368363, 0.8596491228070175517, 0.8640350877192982670, 0.8684210526315789824, 0.8728070175438596978, 0.8771929824561403022, 0.8815789473684210176, 0.8859649122807017330, 0.8903508771929824483, 0.8947368421052631637, 0.8991228070175438791, 0.9035087719298245945, 0.9078947368421053099, 0.9122807017543859143, 0.9166666666666666297, 0.9210526315789473450, 0.9254385964912280604, 0.9298245614035087758, 0.9342105263157894912, 0.9385964912280702066, 0.9429824561403509220, 0.9473684210526315264, 0.9517543859649122417, 0.9561403508771929571, 0.9605263157894736725, 0.9649122807017543879, 0.9692982456140351033, 0.9736842105263158187, 0.9780701754385965341, 0.9824561403508771384, 0.9868421052631578538, 0.9912280701754385692, 0.9956140350877192846, 1.000000000000000000 ),
 .UNSPECIFIED. ) 
 GEOMETRIC_REPRESENTATION_ITEM ( )  RATIONAL_B_SPLINE_SURFACE ( (
 ( 1.000000000000000000, 0.9659258262890683122, 1.000000000000000000, 0.9659258262890683122, 1.000000000000000000, 0.9659258262890683122, 1.000000000000000000, 0.9659258262890683122, 1.000000000000000000, 0.9659258262890683122, 1.000000000000000000, 0.9659258262890683122, 1.000000000000000000, 0.9659258262890683122, 1.000000000000000000, 0.9659258262890683122, 1.000000000000000000, 0.9659258262890683122, 1.000000000000000000, 0.9659258262890683122, 1.000000000000000000, 0.9659258262890683122, 1.000000000000000000, 0.9659258262890683122, 1.000000000000000000, 0.9659258262890683122, 1.000000000000000000, 0.9659258262890683122, 1.000000000000000000, 0.9659258262890683122, 1.000000000000000000, 0.9659258262890683122, 1.000000000000000000, 0.9659258262890683122, 1.000000000000000000, 0.9659258262890683122, 1.000000000000000000, 0.9659258262890683122, 1.000000000000000000, 0.9659258262890683122, 1.000000000000000000, 0.9659258262890683122, 1.000000000000000000, 0.9659258262890683122, 1.000000000000000000, 0.9659258262890683122, 1.000000000000000000, 0.9659258262890683122, 1.000000000000000000, 0.9659258262890683122, 1.000000000000000000, 0.9659258262890683122, 1.000000000000000000, 0.9659258262890683122, 1.000000000000000000, 0.9659258262890683122, 1.000000000000000000, 0.9659258262890683122, 1.000000000000000000, 0.9659258262890683122, 1.000000000000000000, 0.9659258262890683122, 1.000000000000000000, 0.9659258262890683122, 1.000000000000000000, 0.9659258262890683122, 1.000000000000000000, 0.9659258262890683122, 1.000000000000000000, 0.9659258262890683122, 1.000000000000000000, 0.9659258262890683122, 1.000000000000000000, 0.9659258262890683122, 1.000000000000000000, 0.9659258262890683122, 1.000000000000000000, 0.9659258262890683122, 1.000000000000000000, 0.9659258262890683122, 1.000000000000000000, 0.9659258262890683122, 1.000000000000000000, 0.9659258262890683122, 1.000000000000000000, 0.9659258262890683122, 1.000000000000000000, 0.9659258262890683122, 1.000000000000000000, 0.9659258262890683122, 1.000000000000000000, 0.9659258262890683122, 1.000000000000000000, 0.9659258262890683122, 1.000000000000000000, 0.9659258262890683122, 1.000000000000000000, 0.9659258262890683122, 1.000000000000000000, 0.9659258262890683122, 1.000000000000000000, 0.9659258262890683122, 1.000000000000000000, 0.9659258262890683122, 1.000000000000000000, 0.9659258262890683122, 1.000000000000000000, 0.9659258262890683122, 1.000000000000000000, 0.9659258262890683122, 1.000000000000000000, 0.9659258262890683122, 1.000000000000000000, 0.9659258262890683122, 1.000000000000000000, 0.9659258262890683122, 1.000000000000000000, 0.9659258262890683122, 1.000000000000000000, 0.9659258262890683122, 1.000000000000000000, 0.9659258262890683122, 1.000000000000000000, 0.9659258262890683122, 1.000000000000000000, 0.9659258262890683122, 1.000000000000000000, 0.9659258262890683122, 1.000000000000000000, 0.9659258262890683122, 1.000000000000000000, 0.9659258262890683122, 1.000000000000000000, 0.9659258262890683122, 1.000000000000000000, 0.9659258262890683122, 1.000000000000000000, 0.9659258262890683122, 1.000000000000000000, 0.9659258262890683122, 1.000000000000000000, 0.9659258262890683122, 1.000000000000000000, 0.9659258262890683122, 1.000000000000000000, 0.9659258262890683122, 1.000000000000000000, 0.9659258262890683122, 1.000000000000000000, 0.9659258262890683122, 1.000000000000000000, 0.9659258262890683122, 1.000000000000000000, 0.9659258262890683122, 1.000000000000000000, 0.9659258262890683122, 1.000000000000000000, 0.9659258262890683122, 1.000000000000000000, 0.9659258262890683122, 1.000000000000000000, 0.9659258262890683122, 1.000000000000000000, 0.9659258262890683122, 1.000000000000000000, 0.9659258262890683122, 1.000000000000000000, 0.9659258262890683122, 1.000000000000000000, 0.9659258262890683122, 1.000000000000000000, 0.9659258262890683122, 1.000000000000000000, 0.9659258262890683122, 1.000000000000000000, 0.9659258262890683122, 1.000000000000000000, 0.9659258262890683122, 1.000000000000000000, 0.9659258262890683122, 1.000000000000000000, 0.9659258262890683122, 1.000000000000000000, 0.9659258262890683122, 1.000000000000000000, 0.9659258262890683122, 1.000000000000000000, 0.9659258262890683122, 1.000000000000000000, 0.9659258262890683122, 1.000000000000000000, 0.9659258262890683122, 1.000000000000000000, 0.9659258262890683122, 1.000000000000000000, 0.9659258262890683122, 1.000000000000000000, 0.9659258262890683122, 1.000000000000000000, 0.9659258262890683122, 1.000000000000000000, 0.9659258262890683122, 1.000000000000000000, 0.9659258262890683122, 1.000000000000000000, 0.9659258262890683122, 1.000000000000000000, 0.9659258262890683122, 1.000000000000000000, 0.9659258262890683122, 1.000000000000000000, 0.9659258262890683122, 1.000000000000000000, 0.9659258262890683122, 1.000000000000000000, 0.9659258262890683122, 1.000000000000000000, 0.9659258262890683122, 1.000000000000000000, 0.9659258262890683122, 1.000000000000000000, 0.9659258262890683122, 1.000000000000000000, 0.9659258262890683122, 1.000000000000000000, 0.9659258262890683122, 1.000000000000000000, 0.9659258262890683122, 1.000000000000000000, 0.9659258262890683122, 1.000000000000000000, 0.9659258262890683122, 1.000000000000000000, 0.9659258262890683122, 1.000000000000000000, 0.9659258262890683122, 1.000000000000000000, 0.9659258262890683122, 1.000000000000000000, 0.9659258262890683122, 1.000000000000000000, 0.9659258262890683122, 1.000000000000000000, 0.9659258262890683122, 1.000000000000000000, 0.9659258262890683122, 1.000000000000000000, 0.9659258262890683122, 1.000000000000000000, 0.9659258262890683122, 1.000000000000000000, 0.9659258262890683122, 1.000000000000000000, 0.9659258262890683122, 1.000000000000000000, 0.9659258262890683122, 1.000000000000000000, 0.9659258262890683122, 1.000000000000000000, 0.9659258262890683122, 1.000000000000000000, 0.9659258262890683122, 1.000000000000000000, 0.9659258262890683122, 1.000000000000000000, 0.9659258262890683122, 1.000000000000000000, 0.9659258262890683122, 1.000000000000000000, 0.9659258262890683122, 1.000000000000000000, 0.9659258262890683122, 1.000000000000000000, 0.9659258262890683122, 1.000000000000000000, 0.9659258262890683122, 1.000000000000000000, 0.9659258262890683122, 1.000000000000000000, 0.9659258262890683122, 1.000000000000000000, 0.9659258262890683122, 1.000000000000000000, 0.9659258262890683122, 1.000000000000000000, 0.9659258262890683122, 1.000000000000000000, 0.9659258262890683122, 1.000000000000000000, 0.9659258262890683122, 1.000000000000000000, 0.9659258262890683122, 1.000000000000000000, 0.9659258262890683122, 1.000000000000000000, 0.9659258262890683122, 1.000000000000000000, 0.9659258262890683122, 1.000000000000000000, 0.9659258262890683122, 1.000000000000000000, 0.9659258262890683122, 1.000000000000000000, 0.9659258262890683122, 1.000000000000000000, 0.9659258262890683122, 1.000000000000000000, 0.9659258262890683122, 1.000000000000000000, 0.9659258262890683122, 1.000000000000000000, 0.9659258262890683122, 1.000000000000000000, 0.9659258262890683122, 1.000000000000000000, 0.9659258262890683122, 1.000000000000000000, 0.9659258262890683122, 1.000000000000000000, 0.9659258262890683122, 1.000000000000000000, 0.9659258262890683122, 1.000000000000000000, 0.9659258262890683122, 1.000000000000000000, 0.9659258262890683122, 1.000000000000000000, 0.9659258262890683122, 1.000000000000000000, 0.9659258262890683122, 1.000000000000000000, 0.9659258262890683122, 1.000000000000000000, 0.9659258262890683122, 1.000000000000000000, 0.9659258262890683122, 1.000000000000000000, 0.9659258262890683122, 1.000000000000000000, 0.9659258262890683122, 1.000000000000000000, 0.9659258262890683122, 1.000000000000000000, 0.9659258262890683122, 1.000000000000000000, 0.9659258262890683122, 1.000000000000000000, 0.9659258262890683122, 1.000000000000000000, 0.9659258262890683122, 1.000000000000000000, 0.9659258262890683122, 1.000000000000000000, 0.9659258262890683122, 1.000000000000000000, 0.9659258262890683122, 1.000000000000000000, 0.9659258262890683122, 1.000000000000000000, 0.9659258262890683122, 1.000000000000000000, 0.9659258262890683122, 1.000000000000000000, 0.9659258262890683122, 1.000000000000000000, 0.9659258262890683122, 1.000000000000000000, 0.9659258262890683122, 1.000000000000000000, 0.9659258262890683122, 1.000000000000000000, 0.9659258262890683122, 1.000000000000000000, 0.9659258262890683122, 1.000000000000000000, 0.9659258262890683122, 1.000000000000000000, 0.9659258262890683122, 1.000000000000000000, 0.9659258262890683122, 1.000000000000000000, 0.9659258262890683122, 1.000000000000000000, 0.9659258262890683122, 1.000000000000000000, 0.9659258262890683122, 1.000000000000000000, 0.9659258262890683122, 1.000000000000000000, 0.9659258262890683122, 1.000000000000000000, 0.9659258262890683122, 1.000000000000000000, 0.9659258262890683122, 1.000000000000000000, 0.9659258262890683122, 1.000000000000000000, 0.9659258262890683122, 1.000000000000000000, 0.9659258262890683122, 1.000000000000000000, 0.9659258262890683122, 1.000000000000000000, 0.9659258262890683122, 1.000000000000000000, 0.9659258262890683122, 1.000000000000000000, 0.9659258262890683122, 1.000000000000000000, 0.9659258262890683122, 1.000000000000000000, 0.9659258262890683122, 1.000000000000000000, 0.9659258262890683122, 1.000000000000000000, 0.9659258262890683122, 1.000000000000000000, 0.9659258262890683122, 1.000000000000000000, 0.9659258262890683122, 1.000000000000000000, 0.9659258262890683122, 1.000000000000000000, 0.9659258262890683122, 1.000000000000000000, 0.9659258262890683122, 1.000000000000000000, 0.9659258262890683122, 1.000000000000000000, 0.9659258262890683122, 1.000000000000000000, 0.9659258262890683122, 1.000000000000000000, 0.9659258262890683122, 1.000000000000000000, 0.9659258262890683122, 1.000000000000000000, 0.9659258262890683122, 1.000000000000000000, 0.9659258262890683122, 1.000000000000000000, 0.9659258262890683122, 1.000000000000000000, 0.9659258262890683122, 1.000000000000000000, 0.9659258262890683122, 1.000000000000000000, 0.9659258262890683122, 1.000000000000000000, 0.9659258262890683122, 1.000000000000000000, 0.9659258262890683122, 1.000000000000000000, 0.9659258262890683122, 1.000000000000000000, 0.9659258262890683122, 1.000000000000000000),
 ( 0.3333333333333333703, 0.3219752754296894559, 0.3333333333333333703, 0.3219752754296894559, 0.3333333333333333703, 0.3219752754296894559, 0.3333333333333333703, 0.3219752754296894559, 0.3333333333333333703, 0.3219752754296894559, 0.3333333333333333703, 0.3219752754296894559, 0.3333333333333333703, 0.3219752754296894559, 0.3333333333333333703, 0.3219752754296894559, 0.3333333333333333703, 0.3219752754296894559, 0.3333333333333333703, 0.3219752754296894559, 0.3333333333333333703, 0.3219752754296894559, 0.3333333333333333703, 0.3219752754296894559, 0.3333333333333333703, 0.3219752754296894559, 0.3333333333333333703, 0.3219752754296894559, 0.3333333333333333703, 0.3219752754296894559, 0.3333333333333333703, 0.3219752754296894559, 0.3333333333333333703, 0.3219752754296894559, 0.3333333333333333703, 0.3219752754296894559, 0.3333333333333333703, 0.3219752754296894559, 0.3333333333333333703, 0.3219752754296894559, 0.3333333333333333703, 0.3219752754296894559, 0.3333333333333333703, 0.3219752754296894559, 0.3333333333333333703, 0.3219752754296894559, 0.3333333333333333703, 0.3219752754296894559, 0.3333333333333333703, 0.3219752754296894559, 0.3333333333333333703, 0.3219752754296894559, 0.3333333333333333703, 0.3219752754296894559, 0.3333333333333333703, 0.3219752754296894559, 0.3333333333333333703, 0.3219752754296894559, 0.3333333333333333703, 0.3219752754296894559, 0.3333333333333333703, 0.3219752754296894559, 0.3333333333333333703, 0.3219752754296894559, 0.3333333333333333703, 0.3219752754296894559, 0.3333333333333333703, 0.3219752754296894559, 0.3333333333333333703, 0.3219752754296894559, 0.3333333333333333703, 0.3219752754296894559, 0.3333333333333333703, 0.3219752754296894559, 0.3333333333333333703, 0.3219752754296894559, 0.3333333333333333703, 0.3219752754296894559, 0.3333333333333333703, 0.3219752754296894559, 0.3333333333333333703, 0.3219752754296894559, 0.3333333333333333703, 0.3219752754296894559, 0.3333333333333333703, 0.3219752754296894559, 0.3333333333333333703, 0.3219752754296894559, 0.3333333333333333703, 0.3219752754296894559, 0.3333333333333333703, 0.3219752754296894559, 0.3333333333333333703, 0.3219752754296894559, 0.3333333333333333703, 0.3219752754296894559, 0.3333333333333333703, 0.3219752754296894559, 0.3333333333333333703, 0.3219752754296894559, 0.3333333333333333703, 0.3219752754296894559, 0.3333333333333333703, 0.3219752754296894559, 0.3333333333333333703, 0.3219752754296894559, 0.3333333333333333703, 0.3219752754296894559, 0.3333333333333333703, 0.3219752754296894559, 0.3333333333333333703, 0.3219752754296894559, 0.3333333333333333703, 0.3219752754296894559, 0.3333333333333333703, 0.3219752754296894559, 0.3333333333333333703, 0.3219752754296894559, 0.3333333333333333703, 0.3219752754296894559, 0.3333333333333333703, 0.3219752754296894559, 0.3333333333333333703, 0.3219752754296894559, 0.3333333333333333703, 0.3219752754296894559, 0.3333333333333333703, 0.3219752754296894559, 0.3333333333333333703, 0.3219752754296894559, 0.3333333333333333703, 0.3219752754296894559, 0.3333333333333333703, 0.3219752754296894559, 0.3333333333333333703, 0.3219752754296894559, 0.3333333333333333703, 0.3219752754296894559, 0.3333333333333333703, 0.3219752754296894559, 0.3333333333333333703, 0.3219752754296894559, 0.3333333333333333703, 0.3219752754296894559, 0.3333333333333333703, 0.3219752754296894559, 0.3333333333333333703, 0.3219752754296894559, 0.3333333333333333703, 0.3219752754296894559, 0.3333333333333333703, 0.3219752754296894559, 0.3333333333333333703, 0.3219752754296894559, 0.3333333333333333703, 0.3219752754296894559, 0.3333333333333333703, 0.3219752754296894559, 0.3333333333333333703, 0.3219752754296894559, 0.3333333333333333703, 0.3219752754296894559, 0.3333333333333333703, 0.3219752754296894559, 0.3333333333333333703, 0.3219752754296894559, 0.3333333333333333703, 0.3219752754296894559, 0.3333333333333333703, 0.3219752754296894559, 0.3333333333333333703, 0.3219752754296894559, 0.3333333333333333703, 0.3219752754296894559, 0.3333333333333333703, 0.3219752754296894559, 0.3333333333333333703, 0.3219752754296894559, 0.3333333333333333703, 0.3219752754296894559, 0.3333333333333333703, 0.3219752754296894559, 0.3333333333333333703, 0.3219752754296894559, 0.3333333333333333703, 0.3219752754296894559, 0.3333333333333333703, 0.3219752754296894559, 0.3333333333333333703, 0.3219752754296894559, 0.3333333333333333703, 0.3219752754296894559, 0.3333333333333333703, 0.3219752754296894559, 0.3333333333333333703, 0.3219752754296894559, 0.3333333333333333703, 0.3219752754296894559, 0.3333333333333333703, 0.3219752754296894559, 0.3333333333333333703, 0.3219752754296894559, 0.3333333333333333703, 0.3219752754296894559, 0.3333333333333333703, 0.3219752754296894559, 0.3333333333333333703, 0.3219752754296894559, 0.3333333333333333703, 0.3219752754296894559, 0.3333333333333333703, 0.3219752754296894559, 0.3333333333333333703, 0.3219752754296894559, 0.3333333333333333703, 0.3219752754296894559, 0.3333333333333333703, 0.3219752754296894559, 0.3333333333333333703, 0.3219752754296894559, 0.3333333333333333703, 0.3219752754296894559, 0.3333333333333333703, 0.3219752754296894559, 0.3333333333333333703, 0.3219752754296894559, 0.3333333333333333703, 0.3219752754296894559, 0.3333333333333333703, 0.3219752754296894559, 0.3333333333333333703, 0.3219752754296894559, 0.3333333333333333703, 0.3219752754296894559, 0.3333333333333333703, 0.3219752754296894559, 0.3333333333333333703, 0.3219752754296894559, 0.3333333333333333703, 0.3219752754296894559, 0.3333333333333333703, 0.3219752754296894559, 0.3333333333333333703, 0.3219752754296894559, 0.3333333333333333703, 0.3219752754296894559, 0.3333333333333333703, 0.3219752754296894559, 0.3333333333333333703, 0.3219752754296894559, 0.3333333333333333703, 0.3219752754296894559, 0.3333333333333333703, 0.3219752754296894559, 0.3333333333333333703, 0.3219752754296894559, 0.3333333333333333703, 0.3219752754296894559, 0.3333333333333333703, 0.3219752754296894559, 0.3333333333333333703, 0.3219752754296894559, 0.3333333333333333703, 0.3219752754296894559, 0.3333333333333333703, 0.3219752754296894559, 0.3333333333333333703, 0.3219752754296894559, 0.3333333333333333703, 0.3219752754296894559, 0.3333333333333333703, 0.3219752754296894559, 0.3333333333333333703, 0.3219752754296894559, 0.3333333333333333703, 0.3219752754296894559, 0.3333333333333333703, 0.3219752754296894559, 0.3333333333333333703, 0.3219752754296894559, 0.3333333333333333703, 0.3219752754296894559, 0.3333333333333333703, 0.3219752754296894559, 0.3333333333333333703, 0.3219752754296894559, 0.3333333333333333703, 0.3219752754296894559, 0.3333333333333333703, 0.3219752754296894559, 0.3333333333333333703, 0.3219752754296894559, 0.3333333333333333703, 0.3219752754296894559, 0.3333333333333333703, 0.3219752754296894559, 0.3333333333333333703, 0.3219752754296894559, 0.3333333333333333703, 0.3219752754296894559, 0.3333333333333333703, 0.3219752754296894559, 0.3333333333333333703, 0.3219752754296894559, 0.3333333333333333703, 0.3219752754296894559, 0.3333333333333333703, 0.3219752754296894559, 0.3333333333333333703, 0.3219752754296894559, 0.3333333333333333703, 0.3219752754296894559, 0.3333333333333333703, 0.3219752754296894559, 0.3333333333333333703, 0.3219752754296894559, 0.3333333333333333703, 0.3219752754296894559, 0.3333333333333333703, 0.3219752754296894559, 0.3333333333333333703, 0.3219752754296894559, 0.3333333333333333703, 0.3219752754296894559, 0.3333333333333333703, 0.3219752754296894559, 0.3333333333333333703, 0.3219752754296894559, 0.3333333333333333703, 0.3219752754296894559, 0.3333333333333333703, 0.3219752754296894559, 0.3333333333333333703, 0.3219752754296894559, 0.3333333333333333703, 0.3219752754296894559, 0.3333333333333333703, 0.3219752754296894559, 0.3333333333333333703, 0.3219752754296894559, 0.3333333333333333703, 0.3219752754296894559, 0.3333333333333333703, 0.3219752754296894559, 0.3333333333333333703, 0.3219752754296894559, 0.3333333333333333703, 0.3219752754296894559, 0.3333333333333333703, 0.3219752754296894559, 0.3333333333333333703, 0.3219752754296894559, 0.3333333333333333703, 0.3219752754296894559, 0.3333333333333333703, 0.3219752754296894559, 0.3333333333333333703, 0.3219752754296894559, 0.3333333333333333703, 0.3219752754296894559, 0.3333333333333333703, 0.3219752754296894559, 0.3333333333333333703, 0.3219752754296894559, 0.3333333333333333703, 0.3219752754296894559, 0.3333333333333333703, 0.3219752754296894559, 0.3333333333333333703, 0.3219752754296894559, 0.3333333333333333703, 0.3219752754296894559, 0.3333333333333333703, 0.3219752754296894559, 0.3333333333333333703, 0.3219752754296894559, 0.3333333333333333703, 0.3219752754296894559, 0.3333333333333333703, 0.3219752754296894559, 0.3333333333333333703, 0.3219752754296894559, 0.3333333333333333703, 0.3219752754296894559, 0.3333333333333333703, 0.3219752754296894559, 0.3333333333333333703, 0.3219752754296894559, 0.3333333333333333703, 0.3219752754296894559, 0.3333333333333333703, 0.3219752754296894559, 0.3333333333333333703, 0.3219752754296894559, 0.3333333333333333703, 0.3219752754296894559, 0.3333333333333333703, 0.3219752754296894559, 0.3333333333333333703, 0.3219752754296894559, 0.3333333333333333703, 0.3219752754296894559, 0.3333333333333333703, 0.3219752754296894559, 0.3333333333333333703, 0.3219752754296894559, 0.3333333333333333703, 0.3219752754296894559, 0.3333333333333333703, 0.3219752754296894559, 0.3333333333333333703, 0.3219752754296894559, 0.3333333333333333703, 0.3219752754296894559, 0.3333333333333333703, 0.3219752754296894559, 0.3333333333333333703, 0.3219752754296894559, 0.3333333333333333703, 0.3219752754296894559, 0.3333333333333333703, 0.3219752754296894559, 0.3333333333333333703, 0.3219752754296894559, 0.3333333333333333703, 0.3219752754296894559, 0.3333333333333333703, 0.3219752754296894559, 0.3333333333333333703, 0.3219752754296894559, 0.3333333333333333703, 0.3219752754296894559, 0.3333333333333333703, 0.3219752754296894559, 0.3333333333333333703, 0.3219752754296894559, 0.3333333333333333703, 0.3219752754296894559, 0.3333333333333333703, 0.3219752754296894559, 0.3333333333333333703, 0.3219752754296894559, 0.3333333333333333703, 0.3219752754296894559, 0.3333333333333333703, 0.3219752754296894559, 0.3333333333333333703, 0.3219752754296894559, 0.3333333333333333703, 0.3219752754296894559, 0.3333333333333333703, 0.3219752754296894559, 0.3333333333333333703, 0.3219752754296894559, 0.3333333333333333703, 0.3219752754296894559, 0.3333333333333333703),
 ( 0.3333333333333333703, 0.3219752754296894559, 0.3333333333333333703, 0.3219752754296894559, 0.3333333333333333703, 0.3219752754296894559, 0.3333333333333333703, 0.3219752754296894559, 0.3333333333333333703, 0.3219752754296894559, 0.3333333333333333703, 0.3219752754296894559, 0.3333333333333333703, 0.3219752754296894559, 0.3333333333333333703, 0.3219752754296894559, 0.3333333333333333703, 0.3219752754296894559, 0.3333333333333333703, 0.3219752754296894559, 0.3333333333333333703, 0.3219752754296894559, 0.3333333333333333703, 0.3219752754296894559, 0.3333333333333333703, 0.3219752754296894559, 0.3333333333333333703, 0.3219752754296894559, 0.3333333333333333703, 0.3219752754296894559, 0.3333333333333333703, 0.3219752754296894559, 0.3333333333333333703, 0.3219752754296894559, 0.3333333333333333703, 0.3219752754296894559, 0.3333333333333333703, 0.3219752754296894559, 0.3333333333333333703, 0.3219752754296894559, 0.3333333333333333703, 0.3219752754296894559, 0.3333333333333333703, 0.3219752754296894559, 0.3333333333333333703, 0.3219752754296894559, 0.3333333333333333703, 0.3219752754296894559, 0.3333333333333333703, 0.3219752754296894559, 0.3333333333333333703, 0.3219752754296894559, 0.3333333333333333703, 0.3219752754296894559, 0.3333333333333333703, 0.3219752754296894559, 0.3333333333333333703, 0.3219752754296894559, 0.3333333333333333703, 0.3219752754296894559, 0.3333333333333333703, 0.3219752754296894559, 0.3333333333333333703, 0.3219752754296894559, 0.3333333333333333703, 0.3219752754296894559, 0.3333333333333333703, 0.3219752754296894559, 0.3333333333333333703, 0.3219752754296894559, 0.3333333333333333703, 0.3219752754296894559, 0.3333333333333333703, 0.3219752754296894559, 0.3333333333333333703, 0.3219752754296894559, 0.3333333333333333703, 0.3219752754296894559, 0.3333333333333333703, 0.3219752754296894559, 0.3333333333333333703, 0.3219752754296894559, 0.3333333333333333703, 0.3219752754296894559, 0.3333333333333333703, 0.3219752754296894559, 0.3333333333333333703, 0.3219752754296894559, 0.3333333333333333703, 0.3219752754296894559, 0.3333333333333333703, 0.3219752754296894559, 0.3333333333333333703, 0.3219752754296894559, 0.3333333333333333703, 0.3219752754296894559, 0.3333333333333333703, 0.3219752754296894559, 0.3333333333333333703, 0.3219752754296894559, 0.3333333333333333703, 0.3219752754296894559, 0.3333333333333333703, 0.3219752754296894559, 0.3333333333333333703, 0.3219752754296894559, 0.3333333333333333703, 0.3219752754296894559, 0.3333333333333333703, 0.3219752754296894559, 0.3333333333333333703, 0.3219752754296894559, 0.3333333333333333703, 0.3219752754296894559, 0.3333333333333333703, 0.3219752754296894559, 0.3333333333333333703, 0.3219752754296894559, 0.3333333333333333703, 0.3219752754296894559, 0.3333333333333333703, 0.3219752754296894559, 0.3333333333333333703, 0.3219752754296894559, 0.3333333333333333703, 0.3219752754296894559, 0.3333333333333333703, 0.3219752754296894559, 0.3333333333333333703, 0.3219752754296894559, 0.3333333333333333703, 0.3219752754296894559, 0.3333333333333333703, 0.3219752754296894559, 0.3333333333333333703, 0.3219752754296894559, 0.3333333333333333703, 0.3219752754296894559, 0.3333333333333333703, 0.3219752754296894559, 0.3333333333333333703, 0.3219752754296894559, 0.3333333333333333703, 0.3219752754296894559, 0.3333333333333333703, 0.3219752754296894559, 0.3333333333333333703, 0.3219752754296894559, 0.3333333333333333703, 0.3219752754296894559, 0.3333333333333333703, 0.3219752754296894559, 0.3333333333333333703, 0.3219752754296894559, 0.3333333333333333703, 0.3219752754296894559, 0.3333333333333333703, 0.3219752754296894559, 0.3333333333333333703, 0.3219752754296894559, 0.3333333333333333703, 0.3219752754296894559, 0.3333333333333333703, 0.3219752754296894559, 0.3333333333333333703, 0.3219752754296894559, 0.3333333333333333703, 0.3219752754296894559, 0.3333333333333333703, 0.3219752754296894559, 0.3333333333333333703, 0.3219752754296894559, 0.3333333333333333703, 0.3219752754296894559, 0.3333333333333333703, 0.3219752754296894559, 0.3333333333333333703, 0.3219752754296894559, 0.3333333333333333703, 0.3219752754296894559, 0.3333333333333333703, 0.3219752754296894559, 0.3333333333333333703, 0.3219752754296894559, 0.3333333333333333703, 0.3219752754296894559, 0.3333333333333333703, 0.3219752754296894559, 0.3333333333333333703, 0.3219752754296894559, 0.3333333333333333703, 0.3219752754296894559, 0.3333333333333333703, 0.3219752754296894559, 0.3333333333333333703, 0.3219752754296894559, 0.3333333333333333703, 0.3219752754296894559, 0.3333333333333333703, 0.3219752754296894559, 0.3333333333333333703, 0.3219752754296894559, 0.3333333333333333703, 0.3219752754296894559, 0.3333333333333333703, 0.3219752754296894559, 0.3333333333333333703, 0.3219752754296894559, 0.3333333333333333703, 0.3219752754296894559, 0.3333333333333333703, 0.3219752754296894559, 0.3333333333333333703, 0.3219752754296894559, 0.3333333333333333703, 0.3219752754296894559, 0.3333333333333333703, 0.3219752754296894559, 0.3333333333333333703, 0.3219752754296894559, 0.3333333333333333703, 0.3219752754296894559, 0.3333333333333333703, 0.3219752754296894559, 0.3333333333333333703, 0.3219752754296894559, 0.3333333333333333703, 0.3219752754296894559, 0.3333333333333333703, 0.3219752754296894559, 0.3333333333333333703, 0.3219752754296894559, 0.3333333333333333703, 0.3219752754296894559, 0.3333333333333333703, 0.3219752754296894559, 0.3333333333333333703, 0.3219752754296894559, 0.3333333333333333703, 0.3219752754296894559, 0.3333333333333333703, 0.3219752754296894559, 0.3333333333333333703, 0.3219752754296894559, 0.3333333333333333703, 0.3219752754296894559, 0.3333333333333333703, 0.3219752754296894559, 0.3333333333333333703, 0.3219752754296894559, 0.3333333333333333703, 0.3219752754296894559, 0.3333333333333333703, 0.3219752754296894559, 0.3333333333333333703, 0.3219752754296894559, 0.3333333333333333703, 0.3219752754296894559, 0.3333333333333333703, 0.3219752754296894559, 0.3333333333333333703, 0.3219752754296894559, 0.3333333333333333703, 0.3219752754296894559, 0.3333333333333333703, 0.3219752754296894559, 0.3333333333333333703, 0.3219752754296894559, 0.3333333333333333703, 0.3219752754296894559, 0.3333333333333333703, 0.3219752754296894559, 0.3333333333333333703, 0.3219752754296894559, 0.3333333333333333703, 0.3219752754296894559, 0.3333333333333333703, 0.3219752754296894559, 0.3333333333333333703, 0.3219752754296894559, 0.3333333333333333703, 0.3219752754296894559, 0.3333333333333333703, 0.3219752754296894559, 0.3333333333333333703, 0.3219752754296894559, 0.3333333333333333703, 0.3219752754296894559, 0.3333333333333333703, 0.3219752754296894559, 0.3333333333333333703, 0.3219752754296894559, 0.3333333333333333703, 0.3219752754296894559, 0.3333333333333333703, 0.3219752754296894559, 0.3333333333333333703, 0.3219752754296894559, 0.3333333333333333703, 0.3219752754296894559, 0.3333333333333333703, 0.3219752754296894559, 0.3333333333333333703, 0.3219752754296894559, 0.3333333333333333703, 0.3219752754296894559, 0.3333333333333333703, 0.3219752754296894559, 0.3333333333333333703, 0.3219752754296894559, 0.3333333333333333703, 0.3219752754296894559, 0.3333333333333333703, 0.3219752754296894559, 0.3333333333333333703, 0.3219752754296894559, 0.3333333333333333703, 0.3219752754296894559, 0.3333333333333333703, 0.3219752754296894559, 0.3333333333333333703, 0.3219752754296894559, 0.3333333333333333703, 0.3219752754296894559, 0.3333333333333333703, 0.3219752754296894559, 0.3333333333333333703, 0.3219752754296894559, 0.3333333333333333703, 0.3219752754296894559, 0.3333333333333333703, 0.3219752754296894559, 0.3333333333333333703, 0.3219752754296894559, 0.3333333333333333703, 0.3219752754296894559, 0.3333333333333333703, 0.3219752754296894559, 0.3333333333333333703, 0.3219752754296894559, 0.3333333333333333703, 0.3219752754296894559, 0.3333333333333333703, 0.3219752754296894559, 0.3333333333333333703, 0.3219752754296894559, 0.3333333333333333703, 0.3219752754296894559, 0.3333333333333333703, 0.3219752754296894559, 0.3333333333333333703, 0.3219752754296894559, 0.3333333333333333703, 0.3219752754296894559, 0.3333333333333333703, 0.3219752754296894559, 0.3333333333333333703, 0.3219752754296894559, 0.3333333333333333703, 0.3219752754296894559, 0.3333333333333333703, 0.3219752754296894559, 0.3333333333333333703, 0.3219752754296894559, 0.3333333333333333703, 0.3219752754296894559, 0.3333333333333333703, 0.3219752754296894559, 0.3333333333333333703, 0.3219752754296894559, 0.3333333333333333703, 0.3219752754296894559, 0.3333333333333333703, 0.3219752754296894559, 0.3333333333333333703, 0.3219752754296894559, 0.3333333333333333703, 0.3219752754296894559, 0.3333333333333333703, 0.3219752754296894559, 0.3333333333333333703, 0.3219752754296894559, 0.3333333333333333703, 0.3219752754296894559, 0.3333333333333333703, 0.3219752754296894559, 0.3333333333333333703, 0.3219752754296894559, 0.3333333333333333703, 0.3219752754296894559, 0.3333333333333333703, 0.3219752754296894559, 0.3333333333333333703, 0.3219752754296894559, 0.3333333333333333703, 0.3219752754296894559, 0.3333333333333333703, 0.3219752754296894559, 0.3333333333333333703, 0.3219752754296894559, 0.3333333333333333703, 0.3219752754296894559, 0.3333333333333333703, 0.3219752754296894559, 0.3333333333333333703, 0.3219752754296894559, 0.3333333333333333703, 0.3219752754296894559, 0.3333333333333333703, 0.3219752754296894559, 0.3333333333333333703, 0.3219752754296894559, 0.3333333333333333703, 0.3219752754296894559, 0.3333333333333333703, 0.3219752754296894559, 0.3333333333333333703, 0.3219752754296894559, 0.3333333333333333703, 0.3219752754296894559, 0.3333333333333333703, 0.3219752754296894559, 0.3333333333333333703, 0.3219752754296894559, 0.3333333333333333703, 0.3219752754296894559, 0.3333333333333333703, 0.3219752754296894559, 0.3333333333333333703, 0.3219752754296894559, 0.3333333333333333703, 0.3219752754296894559, 0.3333333333333333703, 0.3219752754296894559, 0.3333333333333333703, 0.3219752754296894559, 0.3333333333333333703, 0.3219752754296894559, 0.3333333333333333703, 0.3219752754296894559, 0.3333333333333333703, 0.3219752754296894559, 0.3333333333333333703, 0.3219752754296894559, 0.3333333333333333703, 0.3219752754296894559, 0.3333333333333333703, 0.3219752754296894559, 0.3333333333333333703, 0.3219752754296894559, 0.3333333333333333703, 0.3219752754296894559, 0.3333333333333333703, 0.3219752754296894559, 0.3333333333333333703, 0.3219752754296894559, 0.3333333333333333703),
 ( 1.000000000000000000, 0.9659258262890683122, 1.000000000000000000, 0.9659258262890683122, 1.000000000000000000, 0.9659258262890683122, 1.000000000000000000, 0.9659258262890683122, 1.000000000000000000, 0.9659258262890683122, 1.000000000000000000, 0.9659258262890683122, 1.000000000000000000, 0.9659258262890683122, 1.000000000000000000, 0.9659258262890683122, 1.000000000000000000, 0.9659258262890683122, 1.000000000000000000, 0.9659258262890683122, 1.000000000000000000, 0.9659258262890683122, 1.000000000000000000, 0.9659258262890683122, 1.000000000000000000, 0.9659258262890683122, 1.000000000000000000, 0.9659258262890683122, 1.000000000000000000, 0.9659258262890683122, 1.000000000000000000, 0.9659258262890683122, 1.000000000000000000, 0.9659258262890683122, 1.000000000000000000, 0.9659258262890683122, 1.000000000000000000, 0.9659258262890683122, 1.000000000000000000, 0.9659258262890683122, 1.000000000000000000, 0.9659258262890683122, 1.000000000000000000, 0.9659258262890683122, 1.000000000000000000, 0.9659258262890683122, 1.000000000000000000, 0.9659258262890683122, 1.000000000000000000, 0.9659258262890683122, 1.000000000000000000, 0.9659258262890683122, 1.000000000000000000, 0.9659258262890683122, 1.000000000000000000, 0.9659258262890683122, 1.000000000000000000, 0.9659258262890683122, 1.000000000000000000, 0.9659258262890683122, 1.000000000000000000, 0.9659258262890683122, 1.000000000000000000, 0.9659258262890683122, 1.000000000000000000, 0.9659258262890683122, 1.000000000000000000, 0.9659258262890683122, 1.000000000000000000, 0.9659258262890683122, 1.000000000000000000, 0.9659258262890683122, 1.000000000000000000, 0.9659258262890683122, 1.000000000000000000, 0.9659258262890683122, 1.000000000000000000, 0.9659258262890683122, 1.000000000000000000, 0.9659258262890683122, 1.000000000000000000, 0.9659258262890683122, 1.000000000000000000, 0.9659258262890683122, 1.000000000000000000, 0.9659258262890683122, 1.000000000000000000, 0.9659258262890683122, 1.000000000000000000, 0.9659258262890683122, 1.000000000000000000, 0.9659258262890683122, 1.000000000000000000, 0.9659258262890683122, 1.000000000000000000, 0.9659258262890683122, 1.000000000000000000, 0.9659258262890683122, 1.000000000000000000, 0.9659258262890683122, 1.000000000000000000, 0.9659258262890683122, 1.000000000000000000, 0.9659258262890683122, 1.000000000000000000, 0.9659258262890683122, 1.000000000000000000, 0.9659258262890683122, 1.000000000000000000, 0.9659258262890683122, 1.000000000000000000, 0.9659258262890683122, 1.000000000000000000, 0.9659258262890683122, 1.000000000000000000, 0.9659258262890683122, 1.000000000000000000, 0.9659258262890683122, 1.000000000000000000, 0.9659258262890683122, 1.000000000000000000, 0.9659258262890683122, 1.000000000000000000, 0.9659258262890683122, 1.000000000000000000, 0.9659258262890683122, 1.000000000000000000, 0.9659258262890683122, 1.000000000000000000, 0.9659258262890683122, 1.000000000000000000, 0.9659258262890683122, 1.000000000000000000, 0.9659258262890683122, 1.000000000000000000, 0.9659258262890683122, 1.000000000000000000, 0.9659258262890683122, 1.000000000000000000, 0.9659258262890683122, 1.000000000000000000, 0.9659258262890683122, 1.000000000000000000, 0.9659258262890683122, 1.000000000000000000, 0.9659258262890683122, 1.000000000000000000, 0.9659258262890683122, 1.000000000000000000, 0.9659258262890683122, 1.000000000000000000, 0.9659258262890683122, 1.000000000000000000, 0.9659258262890683122, 1.000000000000000000, 0.9659258262890683122, 1.000000000000000000, 0.9659258262890683122, 1.000000000000000000, 0.9659258262890683122, 1.000000000000000000, 0.9659258262890683122, 1.000000000000000000, 0.9659258262890683122, 1.000000000000000000, 0.9659258262890683122, 1.000000000000000000, 0.9659258262890683122, 1.000000000000000000, 0.9659258262890683122, 1.000000000000000000, 0.9659258262890683122, 1.000000000000000000, 0.9659258262890683122, 1.000000000000000000, 0.9659258262890683122, 1.000000000000000000, 0.9659258262890683122, 1.000000000000000000, 0.9659258262890683122, 1.000000000000000000, 0.9659258262890683122, 1.000000000000000000, 0.9659258262890683122, 1.000000000000000000, 0.9659258262890683122, 1.000000000000000000, 0.9659258262890683122, 1.000000000000000000, 0.9659258262890683122, 1.000000000000000000, 0.9659258262890683122, 1.000000000000000000, 0.9659258262890683122, 1.000000000000000000, 0.9659258262890683122, 1.000000000000000000, 0.9659258262890683122, 1.000000000000000000, 0.9659258262890683122, 1.000000000000000000, 0.9659258262890683122, 1.000000000000000000, 0.9659258262890683122, 1.000000000000000000, 0.9659258262890683122, 1.000000000000000000, 0.9659258262890683122, 1.000000000000000000, 0.9659258262890683122, 1.000000000000000000, 0.9659258262890683122, 1.000000000000000000, 0.9659258262890683122, 1.000000000000000000, 0.9659258262890683122, 1.000000000000000000, 0.9659258262890683122, 1.000000000000000000, 0.9659258262890683122, 1.000000000000000000, 0.9659258262890683122, 1.000000000000000000, 0.9659258262890683122, 1.000000000000000000, 0.9659258262890683122, 1.000000000000000000, 0.9659258262890683122, 1.000000000000000000, 0.9659258262890683122, 1.000000000000000000, 0.9659258262890683122, 1.000000000000000000, 0.9659258262890683122, 1.000000000000000000, 0.9659258262890683122, 1.000000000000000000, 0.9659258262890683122, 1.000000000000000000, 0.9659258262890683122, 1.000000000000000000, 0.9659258262890683122, 1.000000000000000000, 0.9659258262890683122, 1.000000000000000000, 0.9659258262890683122, 1.000000000000000000, 0.9659258262890683122, 1.000000000000000000, 0.9659258262890683122, 1.000000000000000000, 0.9659258262890683122, 1.000000000000000000, 0.9659258262890683122, 1.000000000000000000, 0.9659258262890683122, 1.000000000000000000, 0.9659258262890683122, 1.000000000000000000, 0.9659258262890683122, 1.000000000000000000, 0.9659258262890683122, 1.000000000000000000, 0.9659258262890683122, 1.000000000000000000, 0.9659258262890683122, 1.000000000000000000, 0.9659258262890683122, 1.000000000000000000, 0.9659258262890683122, 1.000000000000000000, 0.9659258262890683122, 1.000000000000000000, 0.9659258262890683122, 1.000000000000000000, 0.9659258262890683122, 1.000000000000000000, 0.9659258262890683122, 1.000000000000000000, 0.9659258262890683122, 1.000000000000000000, 0.9659258262890683122, 1.000000000000000000, 0.9659258262890683122, 1.000000000000000000, 0.9659258262890683122, 1.000000000000000000, 0.9659258262890683122, 1.000000000000000000, 0.9659258262890683122, 1.000000000000000000, 0.9659258262890683122, 1.000000000000000000, 0.9659258262890683122, 1.000000000000000000, 0.9659258262890683122, 1.000000000000000000, 0.9659258262890683122, 1.000000000000000000, 0.9659258262890683122, 1.000000000000000000, 0.9659258262890683122, 1.000000000000000000, 0.9659258262890683122, 1.000000000000000000, 0.9659258262890683122, 1.000000000000000000, 0.9659258262890683122, 1.000000000000000000, 0.9659258262890683122, 1.000000000000000000, 0.9659258262890683122, 1.000000000000000000, 0.9659258262890683122, 1.000000000000000000, 0.9659258262890683122, 1.000000000000000000, 0.9659258262890683122, 1.000000000000000000, 0.9659258262890683122, 1.000000000000000000, 0.9659258262890683122, 1.000000000000000000, 0.9659258262890683122, 1.000000000000000000, 0.9659258262890683122, 1.000000000000000000, 0.9659258262890683122, 1.000000000000000000, 0.9659258262890683122, 1.000000000000000000, 0.9659258262890683122, 1.000000000000000000, 0.9659258262890683122, 1.000000000000000000, 0.9659258262890683122, 1.000000000000000000, 0.9659258262890683122, 1.000000000000000000, 0.9659258262890683122, 1.000000000000000000, 0.9659258262890683122, 1.000000000000000000, 0.9659258262890683122, 1.000000000000000000, 0.9659258262890683122, 1.000000000000000000, 0.9659258262890683122, 1.000000000000000000, 0.9659258262890683122, 1.000000000000000000, 0.9659258262890683122, 1.000000000000000000, 0.9659258262890683122, 1.000000000000000000, 0.9659258262890683122, 1.000000000000000000, 0.9659258262890683122, 1.000000000000000000, 0.9659258262890683122, 1.000000000000000000, 0.9659258262890683122, 1.000000000000000000, 0.9659258262890683122, 1.000000000000000000, 0.9659258262890683122, 1.000000000000000000, 0.9659258262890683122, 1.000000000000000000, 0.9659258262890683122, 1.000000000000000000, 0.9659258262890683122, 1.000000000000000000, 0.9659258262890683122, 1.000000000000000000, 0.9659258262890683122, 1.000000000000000000, 0.9659258262890683122, 1.000000000000000000, 0.9659258262890683122, 1.000000000000000000, 0.9659258262890683122, 1.000000000000000000, 0.9659258262890683122, 1.000000000000000000, 0.9659258262890683122, 1.000000000000000000, 0.9659258262890683122, 1.000000000000000000, 0.9659258262890683122, 1.000000000000000000, 0.9659258262890683122, 1.000000000000000000, 0.9659258262890683122, 1.000000000000000000, 0.9659258262890683122, 1.000000000000000000, 0.9659258262890683122, 1.000000000000000000, 0.9659258262890683122, 1.000000000000000000, 0.9659258262890683122, 1.000000000000000000, 0.9659258262890683122, 1.000000000000000000, 0.9659258262890683122, 1.000000000000000000, 0.9659258262890683122, 1.000000000000000000, 0.9659258262890683122, 1.000000000000000000, 0.9659258262890683122, 1.000000000000000000, 0.9659258262890683122, 1.000000000000000000, 0.9659258262890683122, 1.000000000000000000, 0.9659258262890683122, 1.000000000000000000, 0.9659258262890683122, 1.000000000000000000, 0.9659258262890683122, 1.000000000000000000, 0.9659258262890683122, 1.000000000000000000, 0.9659258262890683122, 1.000000000000000000, 0.9659258262890683122, 1.000000000000000000, 0.9659258262890683122, 1.000000000000000000, 0.9659258262890683122, 1.000000000000000000, 0.9659258262890683122, 1.000000000000000000, 0.9659258262890683122, 1.000000000000000000, 0.9659258262890683122, 1.000000000000000000, 0.9659258262890683122, 1.000000000000000000, 0.9659258262890683122, 1.000000000000000000, 0.9659258262890683122, 1.000000000000000000, 0.9659258262890683122, 1.000000000000000000, 0.9659258262890683122, 1.000000000000000000, 0.9659258262890683122, 1.000000000000000000, 0.9659258262890683122, 1.000000000000000000, 0.9659258262890683122, 1.000000000000000000, 0.9659258262890683122, 1.000000000000000000),
 ( 0.3333333333333333703, 0.3219752754296894559, 0.3333333333333333703, 0.3219752754296894559, 0.3333333333333333703, 0.3219752754296894559, 0.3333333333333333703, 0.3219752754296894559, 0.3333333333333333703, 0.3219752754296894559, 0.3333333333333333703, 0.3219752754296894559, 0.3333333333333333703, 0.3219752754296894559, 0.3333333333333333703, 0.3219752754296894559, 0.3333333333333333703, 0.3219752754296894559, 0.3333333333333333703, 0.3219752754296894559, 0.3333333333333333703, 0.3219752754296894559, 0.3333333333333333703, 0.3219752754296894559, 0.3333333333333333703, 0.3219752754296894559, 0.3333333333333333703, 0.3219752754296894559, 0.3333333333333333703, 0.3219752754296894559, 0.3333333333333333703, 0.3219752754296894559, 0.3333333333333333703, 0.3219752754296894559, 0.3333333333333333703, 0.3219752754296894559, 0.3333333333333333703, 0.3219752754296894559, 0.3333333333333333703, 0.3219752754296894559, 0.3333333333333333703, 0.3219752754296894559, 0.3333333333333333703, 0.3219752754296894559, 0.3333333333333333703, 0.3219752754296894559, 0.3333333333333333703, 0.3219752754296894559, 0.3333333333333333703, 0.3219752754296894559, 0.3333333333333333703, 0.3219752754296894559, 0.3333333333333333703, 0.3219752754296894559, 0.3333333333333333703, 0.3219752754296894559, 0.3333333333333333703, 0.3219752754296894559, 0.3333333333333333703, 0.3219752754296894559, 0.3333333333333333703, 0.3219752754296894559, 0.3333333333333333703, 0.3219752754296894559, 0.3333333333333333703, 0.3219752754296894559, 0.3333333333333333703, 0.3219752754296894559, 0.3333333333333333703, 0.3219752754296894559, 0.3333333333333333703, 0.3219752754296894559, 0.3333333333333333703, 0.3219752754296894559, 0.3333333333333333703, 0.3219752754296894559, 0.3333333333333333703, 0.3219752754296894559, 0.3333333333333333703, 0.3219752754296894559, 0.3333333333333333703, 0.3219752754296894559, 0.3333333333333333703, 0.3219752754296894559, 0.3333333333333333703, 0.3219752754296894559, 0.3333333333333333703, 0.3219752754296894559, 0.3333333333333333703, 0.3219752754296894559, 0.3333333333333333703, 0.3219752754296894559, 0.3333333333333333703, 0.3219752754296894559, 0.3333333333333333703, 0.3219752754296894559, 0.3333333333333333703, 0.3219752754296894559, 0.3333333333333333703, 0.3219752754296894559, 0.3333333333333333703, 0.3219752754296894559, 0.3333333333333333703, 0.3219752754296894559, 0.3333333333333333703, 0.3219752754296894559, 0.3333333333333333703, 0.3219752754296894559, 0.3333333333333333703, 0.3219752754296894559, 0.3333333333333333703, 0.3219752754296894559, 0.3333333333333333703, 0.3219752754296894559, 0.3333333333333333703, 0.3219752754296894559, 0.3333333333333333703, 0.3219752754296894559, 0.3333333333333333703, 0.3219752754296894559, 0.3333333333333333703, 0.3219752754296894559, 0.3333333333333333703, 0.3219752754296894559, 0.3333333333333333703, 0.3219752754296894559, 0.3333333333333333703, 0.3219752754296894559, 0.3333333333333333703, 0.3219752754296894559, 0.3333333333333333703, 0.3219752754296894559, 0.3333333333333333703, 0.3219752754296894559, 0.3333333333333333703, 0.3219752754296894559, 0.3333333333333333703, 0.3219752754296894559, 0.3333333333333333703, 0.3219752754296894559, 0.3333333333333333703, 0.3219752754296894559, 0.3333333333333333703, 0.3219752754296894559, 0.3333333333333333703, 0.3219752754296894559, 0.3333333333333333703, 0.3219752754296894559, 0.3333333333333333703, 0.3219752754296894559, 0.3333333333333333703, 0.3219752754296894559, 0.3333333333333333703, 0.3219752754296894559, 0.3333333333333333703, 0.3219752754296894559, 0.3333333333333333703, 0.3219752754296894559, 0.3333333333333333703, 0.3219752754296894559, 0.3333333333333333703, 0.3219752754296894559, 0.3333333333333333703, 0.3219752754296894559, 0.3333333333333333703, 0.3219752754296894559, 0.3333333333333333703, 0.3219752754296894559, 0.3333333333333333703, 0.3219752754296894559, 0.3333333333333333703, 0.3219752754296894559, 0.3333333333333333703, 0.3219752754296894559, 0.3333333333333333703, 0.3219752754296894559, 0.3333333333333333703, 0.3219752754296894559, 0.3333333333333333703, 0.3219752754296894559, 0.3333333333333333703, 0.3219752754296894559, 0.3333333333333333703, 0.3219752754296894559, 0.3333333333333333703, 0.3219752754296894559, 0.3333333333333333703, 0.3219752754296894559, 0.3333333333333333703, 0.3219752754296894559, 0.3333333333333333703, 0.3219752754296894559, 0.3333333333333333703, 0.3219752754296894559, 0.3333333333333333703, 0.3219752754296894559, 0.3333333333333333703, 0.3219752754296894559, 0.3333333333333333703, 0.3219752754296894559, 0.3333333333333333703, 0.3219752754296894559, 0.3333333333333333703, 0.3219752754296894559, 0.3333333333333333703, 0.3219752754296894559, 0.3333333333333333703, 0.3219752754296894559, 0.3333333333333333703, 0.3219752754296894559, 0.3333333333333333703, 0.3219752754296894559, 0.3333333333333333703, 0.3219752754296894559, 0.3333333333333333703, 0.3219752754296894559, 0.3333333333333333703, 0.3219752754296894559, 0.3333333333333333703, 0.3219752754296894559, 0.3333333333333333703, 0.3219752754296894559, 0.3333333333333333703, 0.3219752754296894559, 0.3333333333333333703, 0.3219752754296894559, 0.3333333333333333703, 0.3219752754296894559, 0.3333333333333333703, 0.3219752754296894559, 0.3333333333333333703, 0.3219752754296894559, 0.3333333333333333703, 0.3219752754296894559, 0.3333333333333333703, 0.3219752754296894559, 0.3333333333333333703, 0.3219752754296894559, 0.3333333333333333703, 0.3219752754296894559, 0.3333333333333333703, 0.3219752754296894559, 0.3333333333333333703, 0.3219752754296894559, 0.3333333333333333703, 0.3219752754296894559, 0.3333333333333333703, 0.3219752754296894559, 0.3333333333333333703, 0.3219752754296894559, 0.3333333333333333703, 0.3219752754296894559, 0.3333333333333333703, 0.3219752754296894559, 0.3333333333333333703, 0.3219752754296894559, 0.3333333333333333703, 0.3219752754296894559, 0.3333333333333333703, 0.3219752754296894559, 0.3333333333333333703, 0.3219752754296894559, 0.3333333333333333703, 0.3219752754296894559, 0.3333333333333333703, 0.3219752754296894559, 0.3333333333333333703, 0.3219752754296894559, 0.3333333333333333703, 0.3219752754296894559, 0.3333333333333333703, 0.3219752754296894559, 0.3333333333333333703, 0.3219752754296894559, 0.3333333333333333703, 0.3219752754296894559, 0.3333333333333333703, 0.3219752754296894559, 0.3333333333333333703, 0.3219752754296894559, 0.3333333333333333703, 0.3219752754296894559, 0.3333333333333333703, 0.3219752754296894559, 0.3333333333333333703, 0.3219752754296894559, 0.3333333333333333703, 0.3219752754296894559, 0.3333333333333333703, 0.3219752754296894559, 0.3333333333333333703, 0.3219752754296894559, 0.3333333333333333703, 0.3219752754296894559, 0.3333333333333333703, 0.3219752754296894559, 0.3333333333333333703, 0.3219752754296894559, 0.3333333333333333703, 0.3219752754296894559, 0.3333333333333333703, 0.3219752754296894559, 0.3333333333333333703, 0.3219752754296894559, 0.3333333333333333703, 0.3219752754296894559, 0.3333333333333333703, 0.3219752754296894559, 0.3333333333333333703, 0.3219752754296894559, 0.3333333333333333703, 0.3219752754296894559, 0.3333333333333333703, 0.3219752754296894559, 0.3333333333333333703, 0.3219752754296894559, 0.3333333333333333703, 0.3219752754296894559, 0.3333333333333333703, 0.3219752754296894559, 0.3333333333333333703, 0.3219752754296894559, 0.3333333333333333703, 0.3219752754296894559, 0.3333333333333333703, 0.3219752754296894559, 0.3333333333333333703, 0.3219752754296894559, 0.3333333333333333703, 0.3219752754296894559, 0.3333333333333333703, 0.3219752754296894559, 0.3333333333333333703, 0.3219752754296894559, 0.3333333333333333703, 0.3219752754296894559, 0.3333333333333333703, 0.3219752754296894559, 0.3333333333333333703, 0.3219752754296894559, 0.3333333333333333703, 0.3219752754296894559, 0.3333333333333333703, 0.3219752754296894559, 0.3333333333333333703, 0.3219752754296894559, 0.3333333333333333703, 0.3219752754296894559, 0.3333333333333333703, 0.3219752754296894559, 0.3333333333333333703, 0.3219752754296894559, 0.3333333333333333703, 0.3219752754296894559, 0.3333333333333333703, 0.3219752754296894559, 0.3333333333333333703, 0.3219752754296894559, 0.3333333333333333703, 0.3219752754296894559, 0.3333333333333333703, 0.3219752754296894559, 0.3333333333333333703, 0.3219752754296894559, 0.3333333333333333703, 0.3219752754296894559, 0.3333333333333333703, 0.3219752754296894559, 0.3333333333333333703, 0.3219752754296894559, 0.3333333333333333703, 0.3219752754296894559, 0.3333333333333333703, 0.3219752754296894559, 0.3333333333333333703, 0.3219752754296894559, 0.3333333333333333703, 0.3219752754296894559, 0.3333333333333333703, 0.3219752754296894559, 0.3333333333333333703, 0.3219752754296894559, 0.3333333333333333703, 0.3219752754296894559, 0.3333333333333333703, 0.3219752754296894559, 0.3333333333333333703, 0.3219752754296894559, 0.3333333333333333703, 0.3219752754296894559, 0.3333333333333333703, 0.3219752754296894559, 0.3333333333333333703, 0.3219752754296894559, 0.3333333333333333703, 0.3219752754296894559, 0.3333333333333333703, 0.3219752754296894559, 0.3333333333333333703, 0.3219752754296894559, 0.3333333333333333703, 0.3219752754296894559, 0.3333333333333333703, 0.3219752754296894559, 0.3333333333333333703, 0.3219752754296894559, 0.3333333333333333703, 0.3219752754296894559, 0.3333333333333333703, 0.3219752754296894559, 0.3333333333333333703, 0.3219752754296894559, 0.3333333333333333703, 0.3219752754296894559, 0.3333333333333333703, 0.3219752754296894559, 0.3333333333333333703, 0.3219752754296894559, 0.3333333333333333703, 0.3219752754296894559, 0.3333333333333333703, 0.3219752754296894559, 0.3333333333333333703, 0.3219752754296894559, 0.3333333333333333703, 0.3219752754296894559, 0.3333333333333333703, 0.3219752754296894559, 0.3333333333333333703, 0.3219752754296894559, 0.3333333333333333703, 0.3219752754296894559, 0.3333333333333333703, 0.3219752754296894559, 0.3333333333333333703, 0.3219752754296894559, 0.3333333333333333703, 0.3219752754296894559, 0.3333333333333333703, 0.3219752754296894559, 0.3333333333333333703, 0.3219752754296894559, 0.3333333333333333703, 0.3219752754296894559, 0.3333333333333333703, 0.3219752754296894559, 0.3333333333333333703, 0.3219752754296894559, 0.3333333333333333703, 0.3219752754296894559, 0.3333333333333333703, 0.3219752754296894559, 0.3333333333333333703, 0.3219752754296894559, 0.3333333333333333703, 0.3219752754296894559, 0.3333333333333333703),
 ( 0.3333333333333333703, 0.3219752754296894559, 0.3333333333333333703, 0.3219752754296894559, 0.3333333333333333703, 0.3219752754296894559, 0.3333333333333333703, 0.3219752754296894559, 0.3333333333333333703, 0.3219752754296894559, 0.3333333333333333703, 0.3219752754296894559, 0.3333333333333333703, 0.3219752754296894559, 0.3333333333333333703, 0.3219752754296894559, 0.3333333333333333703, 0.3219752754296894559, 0.3333333333333333703, 0.3219752754296894559, 0.3333333333333333703, 0.3219752754296894559, 0.3333333333333333703, 0.3219752754296894559, 0.3333333333333333703, 0.3219752754296894559, 0.3333333333333333703, 0.3219752754296894559, 0.3333333333333333703, 0.3219752754296894559, 0.3333333333333333703, 0.3219752754296894559, 0.3333333333333333703, 0.3219752754296894559, 0.3333333333333333703, 0.3219752754296894559, 0.3333333333333333703, 0.3219752754296894559, 0.3333333333333333703, 0.3219752754296894559, 0.3333333333333333703, 0.3219752754296894559, 0.3333333333333333703, 0.3219752754296894559, 0.3333333333333333703, 0.3219752754296894559, 0.3333333333333333703, 0.3219752754296894559, 0.3333333333333333703, 0.3219752754296894559, 0.3333333333333333703, 0.3219752754296894559, 0.3333333333333333703, 0.3219752754296894559, 0.3333333333333333703, 0.3219752754296894559, 0.3333333333333333703, 0.3219752754296894559, 0.3333333333333333703, 0.3219752754296894559, 0.3333333333333333703, 0.3219752754296894559, 0.3333333333333333703, 0.3219752754296894559, 0.3333333333333333703, 0.3219752754296894559, 0.3333333333333333703, 0.3219752754296894559, 0.3333333333333333703, 0.3219752754296894559, 0.3333333333333333703, 0.3219752754296894559, 0.3333333333333333703, 0.3219752754296894559, 0.3333333333333333703, 0.3219752754296894559, 0.3333333333333333703, 0.3219752754296894559, 0.3333333333333333703, 0.3219752754296894559, 0.3333333333333333703, 0.3219752754296894559, 0.3333333333333333703, 0.3219752754296894559, 0.3333333333333333703, 0.3219752754296894559, 0.3333333333333333703, 0.3219752754296894559, 0.3333333333333333703, 0.3219752754296894559, 0.3333333333333333703, 0.3219752754296894559, 0.3333333333333333703, 0.3219752754296894559, 0.3333333333333333703, 0.3219752754296894559, 0.3333333333333333703, 0.3219752754296894559, 0.3333333333333333703, 0.3219752754296894559, 0.3333333333333333703, 0.3219752754296894559, 0.3333333333333333703, 0.3219752754296894559, 0.3333333333333333703, 0.3219752754296894559, 0.3333333333333333703, 0.3219752754296894559, 0.3333333333333333703, 0.3219752754296894559, 0.3333333333333333703, 0.3219752754296894559, 0.3333333333333333703, 0.3219752754296894559, 0.3333333333333333703, 0.3219752754296894559, 0.3333333333333333703, 0.3219752754296894559, 0.3333333333333333703, 0.3219752754296894559, 0.3333333333333333703, 0.3219752754296894559, 0.3333333333333333703, 0.3219752754296894559, 0.3333333333333333703, 0.3219752754296894559, 0.3333333333333333703, 0.3219752754296894559, 0.3333333333333333703, 0.3219752754296894559, 0.3333333333333333703, 0.3219752754296894559, 0.3333333333333333703, 0.3219752754296894559, 0.3333333333333333703, 0.3219752754296894559, 0.3333333333333333703, 0.3219752754296894559, 0.3333333333333333703, 0.3219752754296894559, 0.3333333333333333703, 0.3219752754296894559, 0.3333333333333333703, 0.3219752754296894559, 0.3333333333333333703, 0.3219752754296894559, 0.3333333333333333703, 0.3219752754296894559, 0.3333333333333333703, 0.3219752754296894559, 0.3333333333333333703, 0.3219752754296894559, 0.3333333333333333703, 0.3219752754296894559, 0.3333333333333333703, 0.3219752754296894559, 0.3333333333333333703, 0.3219752754296894559, 0.3333333333333333703, 0.3219752754296894559, 0.3333333333333333703, 0.3219752754296894559, 0.3333333333333333703, 0.3219752754296894559, 0.3333333333333333703, 0.3219752754296894559, 0.3333333333333333703, 0.3219752754296894559, 0.3333333333333333703, 0.3219752754296894559, 0.3333333333333333703, 0.3219752754296894559, 0.3333333333333333703, 0.3219752754296894559, 0.3333333333333333703, 0.3219752754296894559, 0.3333333333333333703, 0.3219752754296894559, 0.3333333333333333703, 0.3219752754296894559, 0.3333333333333333703, 0.3219752754296894559, 0.3333333333333333703, 0.3219752754296894559, 0.3333333333333333703, 0.3219752754296894559, 0.3333333333333333703, 0.3219752754296894559, 0.3333333333333333703, 0.3219752754296894559, 0.3333333333333333703, 0.3219752754296894559, 0.3333333333333333703, 0.3219752754296894559, 0.3333333333333333703, 0.3219752754296894559, 0.3333333333333333703, 0.3219752754296894559, 0.3333333333333333703, 0.3219752754296894559, 0.3333333333333333703, 0.3219752754296894559, 0.3333333333333333703, 0.3219752754296894559, 0.3333333333333333703, 0.3219752754296894559, 0.3333333333333333703, 0.3219752754296894559, 0.3333333333333333703, 0.3219752754296894559, 0.3333333333333333703, 0.3219752754296894559, 0.3333333333333333703, 0.3219752754296894559, 0.3333333333333333703, 0.3219752754296894559, 0.3333333333333333703, 0.3219752754296894559, 0.3333333333333333703, 0.3219752754296894559, 0.3333333333333333703, 0.3219752754296894559, 0.3333333333333333703, 0.3219752754296894559, 0.3333333333333333703, 0.3219752754296894559, 0.3333333333333333703, 0.3219752754296894559, 0.3333333333333333703, 0.3219752754296894559, 0.3333333333333333703, 0.3219752754296894559, 0.3333333333333333703, 0.3219752754296894559, 0.3333333333333333703, 0.3219752754296894559, 0.3333333333333333703, 0.3219752754296894559, 0.3333333333333333703, 0.3219752754296894559, 0.3333333333333333703, 0.3219752754296894559, 0.3333333333333333703, 0.3219752754296894559, 0.3333333333333333703, 0.3219752754296894559, 0.3333333333333333703, 0.3219752754296894559, 0.3333333333333333703, 0.3219752754296894559, 0.3333333333333333703, 0.3219752754296894559, 0.3333333333333333703, 0.3219752754296894559, 0.3333333333333333703, 0.3219752754296894559, 0.3333333333333333703, 0.3219752754296894559, 0.3333333333333333703, 0.3219752754296894559, 0.3333333333333333703, 0.3219752754296894559, 0.3333333333333333703, 0.3219752754296894559, 0.3333333333333333703, 0.3219752754296894559, 0.3333333333333333703, 0.3219752754296894559, 0.3333333333333333703, 0.3219752754296894559, 0.3333333333333333703, 0.3219752754296894559, 0.3333333333333333703, 0.3219752754296894559, 0.3333333333333333703, 0.3219752754296894559, 0.3333333333333333703, 0.3219752754296894559, 0.3333333333333333703, 0.3219752754296894559, 0.3333333333333333703, 0.3219752754296894559, 0.3333333333333333703, 0.3219752754296894559, 0.3333333333333333703, 0.3219752754296894559, 0.3333333333333333703, 0.3219752754296894559, 0.3333333333333333703, 0.3219752754296894559, 0.3333333333333333703, 0.3219752754296894559, 0.3333333333333333703, 0.3219752754296894559, 0.3333333333333333703, 0.3219752754296894559, 0.3333333333333333703, 0.3219752754296894559, 0.3333333333333333703, 0.3219752754296894559, 0.3333333333333333703, 0.3219752754296894559, 0.3333333333333333703, 0.3219752754296894559, 0.3333333333333333703, 0.3219752754296894559, 0.3333333333333333703, 0.3219752754296894559, 0.3333333333333333703, 0.3219752754296894559, 0.3333333333333333703, 0.3219752754296894559, 0.3333333333333333703, 0.3219752754296894559, 0.3333333333333333703, 0.3219752754296894559, 0.3333333333333333703, 0.3219752754296894559, 0.3333333333333333703, 0.3219752754296894559, 0.3333333333333333703, 0.3219752754296894559, 0.3333333333333333703, 0.3219752754296894559, 0.3333333333333333703, 0.3219752754296894559, 0.3333333333333333703, 0.3219752754296894559, 0.3333333333333333703, 0.3219752754296894559, 0.3333333333333333703, 0.3219752754296894559, 0.3333333333333333703, 0.3219752754296894559, 0.3333333333333333703, 0.3219752754296894559, 0.3333333333333333703, 0.3219752754296894559, 0.3333333333333333703, 0.3219752754296894559, 0.3333333333333333703, 0.3219752754296894559, 0.3333333333333333703, 0.3219752754296894559, 0.3333333333333333703, 0.3219752754296894559, 0.3333333333333333703, 0.3219752754296894559, 0.3333333333333333703, 0.3219752754296894559, 0.3333333333333333703, 0.3219752754296894559, 0.3333333333333333703, 0.3219752754296894559, 0.3333333333333333703, 0.3219752754296894559, 0.3333333333333333703, 0.3219752754296894559, 0.3333333333333333703, 0.3219752754296894559, 0.3333333333333333703, 0.3219752754296894559, 0.3333333333333333703, 0.3219752754296894559, 0.3333333333333333703, 0.3219752754296894559, 0.3333333333333333703, 0.3219752754296894559, 0.3333333333333333703, 0.3219752754296894559, 0.3333333333333333703, 0.3219752754296894559, 0.3333333333333333703, 0.3219752754296894559, 0.3333333333333333703, 0.3219752754296894559, 0.3333333333333333703, 0.3219752754296894559, 0.3333333333333333703, 0.3219752754296894559, 0.3333333333333333703, 0.3219752754296894559, 0.3333333333333333703, 0.3219752754296894559, 0.3333333333333333703, 0.3219752754296894559, 0.3333333333333333703, 0.3219752754296894559, 0.3333333333333333703, 0.3219752754296894559, 0.3333333333333333703, 0.3219752754296894559, 0.3333333333333333703, 0.3219752754296894559, 0.3333333333333333703, 0.3219752754296894559, 0.3333333333333333703, 0.3219752754296894559, 0.3333333333333333703, 0.3219752754296894559, 0.3333333333333333703, 0.3219752754296894559, 0.3333333333333333703, 0.3219752754296894559, 0.3333333333333333703, 0.3219752754296894559, 0.3333333333333333703, 0.3219752754296894559, 0.3333333333333333703, 0.3219752754296894559, 0.3333333333333333703, 0.3219752754296894559, 0.3333333333333333703, 0.3219752754296894559, 0.3333333333333333703, 0.3219752754296894559, 0.3333333333333333703, 0.3219752754296894559, 0.3333333333333333703, 0.3219752754296894559, 0.3333333333333333703, 0.3219752754296894559, 0.3333333333333333703, 0.3219752754296894559, 0.3333333333333333703, 0.3219752754296894559, 0.3333333333333333703, 0.3219752754296894559, 0.3333333333333333703, 0.3219752754296894559, 0.3333333333333333703, 0.3219752754296894559, 0.3333333333333333703, 0.3219752754296894559, 0.3333333333333333703, 0.3219752754296894559, 0.3333333333333333703, 0.3219752754296894559, 0.3333333333333333703, 0.3219752754296894559, 0.3333333333333333703, 0.3219752754296894559, 0.3333333333333333703, 0.3219752754296894559, 0.3333333333333333703, 0.3219752754296894559, 0.3333333333333333703, 0.3219752754296894559, 0.3333333333333333703, 0.3219752754296894559, 0.3333333333333333703, 0.3219752754296894559, 0.3333333333333333703, 0.3219752754296894559, 0.3333333333333333703, 0.3219752754296894559, 0.3333333333333333703),
 ( 1.000000000000000000, 0.9659258262890683122, 1.000000000000000000, 0.9659258262890683122, 1.000000000000000000, 0.9659258262890683122, 1.000000000000000000, 0.9659258262890683122, 1.000000000000000000, 0.9659258262890683122, 1.000000000000000000, 0.9659258262890683122, 1.000000000000000000, 0.9659258262890683122, 1.000000000000000000, 0.9659258262890683122, 1.000000000000000000, 0.9659258262890683122, 1.000000000000000000, 0.9659258262890683122, 1.000000000000000000, 0.9659258262890683122, 1.000000000000000000, 0.9659258262890683122, 1.000000000000000000, 0.9659258262890683122, 1.000000000000000000, 0.9659258262890683122, 1.000000000000000000, 0.9659258262890683122, 1.000000000000000000, 0.9659258262890683122, 1.000000000000000000, 0.9659258262890683122, 1.000000000000000000, 0.9659258262890683122, 1.000000000000000000, 0.9659258262890683122, 1.000000000000000000, 0.9659258262890683122, 1.000000000000000000, 0.9659258262890683122, 1.000000000000000000, 0.9659258262890683122, 1.000000000000000000, 0.9659258262890683122, 1.000000000000000000, 0.9659258262890683122, 1.000000000000000000, 0.9659258262890683122, 1.000000000000000000, 0.9659258262890683122, 1.000000000000000000, 0.9659258262890683122, 1.000000000000000000, 0.9659258262890683122, 1.000000000000000000, 0.9659258262890683122, 1.000000000000000000, 0.9659258262890683122, 1.000000000000000000, 0.9659258262890683122, 1.000000000000000000, 0.9659258262890683122, 1.000000000000000000, 0.9659258262890683122, 1.000000000000000000, 0.9659258262890683122, 1.000000000000000000, 0.9659258262890683122, 1.000000000000000000, 0.9659258262890683122, 1.000000000000000000, 0.9659258262890683122, 1.000000000000000000, 0.9659258262890683122, 1.000000000000000000, 0.9659258262890683122, 1.000000000000000000, 0.9659258262890683122, 1.000000000000000000, 0.9659258262890683122, 1.000000000000000000, 0.9659258262890683122, 1.000000000000000000, 0.9659258262890683122, 1.000000000000000000, 0.9659258262890683122, 1.000000000000000000, 0.9659258262890683122, 1.000000000000000000, 0.9659258262890683122, 1.000000000000000000, 0.9659258262890683122, 1.000000000000000000, 0.9659258262890683122, 1.000000000000000000, 0.9659258262890683122, 1.000000000000000000, 0.9659258262890683122, 1.000000000000000000, 0.9659258262890683122, 1.000000000000000000, 0.9659258262890683122, 1.000000000000000000, 0.9659258262890683122, 1.000000000000000000, 0.9659258262890683122, 1.000000000000000000, 0.9659258262890683122, 1.000000000000000000, 0.9659258262890683122, 1.000000000000000000, 0.9659258262890683122, 1.000000000000000000, 0.9659258262890683122, 1.000000000000000000, 0.9659258262890683122, 1.000000000000000000, 0.9659258262890683122, 1.000000000000000000, 0.9659258262890683122, 1.000000000000000000, 0.9659258262890683122, 1.000000000000000000, 0.9659258262890683122, 1.000000000000000000, 0.9659258262890683122, 1.000000000000000000, 0.9659258262890683122, 1.000000000000000000, 0.9659258262890683122, 1.000000000000000000, 0.9659258262890683122, 1.000000000000000000, 0.9659258262890683122, 1.000000000000000000, 0.9659258262890683122, 1.000000000000000000, 0.9659258262890683122, 1.000000000000000000, 0.9659258262890683122, 1.000000000000000000, 0.9659258262890683122, 1.000000000000000000, 0.9659258262890683122, 1.000000000000000000, 0.9659258262890683122, 1.000000000000000000, 0.9659258262890683122, 1.000000000000000000, 0.9659258262890683122, 1.000000000000000000, 0.9659258262890683122, 1.000000000000000000, 0.9659258262890683122, 1.000000000000000000, 0.9659258262890683122, 1.000000000000000000, 0.9659258262890683122, 1.000000000000000000, 0.9659258262890683122, 1.000000000000000000, 0.9659258262890683122, 1.000000000000000000, 0.9659258262890683122, 1.000000000000000000, 0.9659258262890683122, 1.000000000000000000, 0.9659258262890683122, 1.000000000000000000, 0.9659258262890683122, 1.000000000000000000, 0.9659258262890683122, 1.000000000000000000, 0.9659258262890683122, 1.000000000000000000, 0.9659258262890683122, 1.000000000000000000, 0.9659258262890683122, 1.000000000000000000, 0.9659258262890683122, 1.000000000000000000, 0.9659258262890683122, 1.000000000000000000, 0.9659258262890683122, 1.000000000000000000, 0.9659258262890683122, 1.000000000000000000, 0.9659258262890683122, 1.000000000000000000, 0.9659258262890683122, 1.000000000000000000, 0.9659258262890683122, 1.000000000000000000, 0.9659258262890683122, 1.000000000000000000, 0.9659258262890683122, 1.000000000000000000, 0.9659258262890683122, 1.000000000000000000, 0.9659258262890683122, 1.000000000000000000, 0.9659258262890683122, 1.000000000000000000, 0.9659258262890683122, 1.000000000000000000, 0.9659258262890683122, 1.000000000000000000, 0.9659258262890683122, 1.000000000000000000, 0.9659258262890683122, 1.000000000000000000, 0.9659258262890683122, 1.000000000000000000, 0.9659258262890683122, 1.000000000000000000, 0.9659258262890683122, 1.000000000000000000, 0.9659258262890683122, 1.000000000000000000, 0.9659258262890683122, 1.000000000000000000, 0.9659258262890683122, 1.000000000000000000, 0.9659258262890683122, 1.000000000000000000, 0.9659258262890683122, 1.000000000000000000, 0.9659258262890683122, 1.000000000000000000, 0.9659258262890683122, 1.000000000000000000, 0.9659258262890683122, 1.000000000000000000, 0.9659258262890683122, 1.000000000000000000, 0.9659258262890683122, 1.000000000000000000, 0.9659258262890683122, 1.000000000000000000, 0.9659258262890683122, 1.000000000000000000, 0.9659258262890683122, 1.000000000000000000, 0.9659258262890683122, 1.000000000000000000, 0.9659258262890683122, 1.000000000000000000, 0.9659258262890683122, 1.000000000000000000, 0.9659258262890683122, 1.000000000000000000, 0.9659258262890683122, 1.000000000000000000, 0.9659258262890683122, 1.000000000000000000, 0.9659258262890683122, 1.000000000000000000, 0.9659258262890683122, 1.000000000000000000, 0.9659258262890683122, 1.000000000000000000, 0.9659258262890683122, 1.000000000000000000, 0.9659258262890683122, 1.000000000000000000, 0.9659258262890683122, 1.000000000000000000, 0.9659258262890683122, 1.000000000000000000, 0.9659258262890683122, 1.000000000000000000, 0.9659258262890683122, 1.000000000000000000, 0.9659258262890683122, 1.000000000000000000, 0.9659258262890683122, 1.000000000000000000, 0.9659258262890683122, 1.000000000000000000, 0.9659258262890683122, 1.000000000000000000, 0.9659258262890683122, 1.000000000000000000, 0.9659258262890683122, 1.000000000000000000, 0.9659258262890683122, 1.000000000000000000, 0.9659258262890683122, 1.000000000000000000, 0.9659258262890683122, 1.000000000000000000, 0.9659258262890683122, 1.000000000000000000, 0.9659258262890683122, 1.000000000000000000, 0.9659258262890683122, 1.000000000000000000, 0.9659258262890683122, 1.000000000000000000, 0.9659258262890683122, 1.000000000000000000, 0.9659258262890683122, 1.000000000000000000, 0.9659258262890683122, 1.000000000000000000, 0.9659258262890683122, 1.000000000000000000, 0.9659258262890683122, 1.000000000000000000, 0.9659258262890683122, 1.000000000000000000, 0.9659258262890683122, 1.000000000000000000, 0.9659258262890683122, 1.000000000000000000, 0.9659258262890683122, 1.000000000000000000, 0.9659258262890683122, 1.000000000000000000, 0.9659258262890683122, 1.000000000000000000, 0.9659258262890683122, 1.000000000000000000, 0.9659258262890683122, 1.000000000000000000, 0.9659258262890683122, 1.000000000000000000, 0.9659258262890683122, 1.000000000000000000, 0.9659258262890683122, 1.000000000000000000, 0.9659258262890683122, 1.000000000000000000, 0.9659258262890683122, 1.000000000000000000, 0.9659258262890683122, 1.000000000000000000, 0.9659258262890683122, 1.000000000000000000, 0.9659258262890683122, 1.000000000000000000, 0.9659258262890683122, 1.000000000000000000, 0.9659258262890683122, 1.000000000000000000, 0.9659258262890683122, 1.000000000000000000, 0.9659258262890683122, 1.000000000000000000, 0.9659258262890683122, 1.000000000000000000, 0.9659258262890683122, 1.000000000000000000, 0.9659258262890683122, 1.000000000000000000, 0.9659258262890683122, 1.000000000000000000, 0.9659258262890683122, 1.000000000000000000, 0.9659258262890683122, 1.000000000000000000, 0.9659258262890683122, 1.000000000000000000, 0.9659258262890683122, 1.000000000000000000, 0.9659258262890683122, 1.000000000000000000, 0.9659258262890683122, 1.000000000000000000, 0.9659258262890683122, 1.000000000000000000, 0.9659258262890683122, 1.000000000000000000, 0.9659258262890683122, 1.000000000000000000, 0.9659258262890683122, 1.000000000000000000, 0.9659258262890683122, 1.000000000000000000, 0.9659258262890683122, 1.000000000000000000, 0.9659258262890683122, 1.000000000000000000, 0.9659258262890683122, 1.000000000000000000, 0.9659258262890683122, 1.000000000000000000, 0.9659258262890683122, 1.000000000000000000, 0.9659258262890683122, 1.000000000000000000, 0.9659258262890683122, 1.000000000000000000, 0.9659258262890683122, 1.000000000000000000, 0.9659258262890683122, 1.000000000000000000, 0.9659258262890683122, 1.000000000000000000, 0.9659258262890683122, 1.000000000000000000, 0.9659258262890683122, 1.000000000000000000, 0.9659258262890683122, 1.000000000000000000, 0.9659258262890683122, 1.000000000000000000, 0.9659258262890683122, 1.000000000000000000, 0.9659258262890683122, 1.000000000000000000, 0.9659258262890683122, 1.000000000000000000, 0.9659258262890683122, 1.000000000000000000, 0.9659258262890683122, 1.000000000000000000, 0.9659258262890683122, 1.000000000000000000, 0.9659258262890683122, 1.000000000000000000, 0.9659258262890683122, 1.000000000000000000, 0.9659258262890683122, 1.000000000000000000, 0.9659258262890683122, 1.000000000000000000, 0.9659258262890683122, 1.000000000000000000, 0.9659258262890683122, 1.000000000000000000, 0.9659258262890683122, 1.000000000000000000, 0.9659258262890683122, 1.000000000000000000, 0.9659258262890683122, 1.000000000000000000, 0.9659258262890683122, 1.000000000000000000, 0.9659258262890683122, 1.000000000000000000, 0.9659258262890683122, 1.000000000000000000, 0.9659258262890683122, 1.000000000000000000, 0.9659258262890683122, 1.000000000000000000, 0.9659258262890683122, 1.000000000000000000, 0.9659258262890683122, 1.000000000000000000, 0.9659258262890683122, 1.000000000000000000, 0.9659258262890683122, 1.000000000000000000) ) ) 
 REPRESENTATION_ITEM ( '' )  SURFACE ( )  );
#124918=CARTESIAN_POINT ( 'NONE',  ( 15.80617190586746368, 15.72974639402197994, 79.37390960531436690 ) ) ;
#124919=CARTESIAN_POINT ( 'NONE',  ( -12.06949235617756955, 12.14591786802309770, 60.62390960531437401 ) ) ;
#124920=CARTESIAN_POINT ( 'NONE',  ( -5.049401038297874678, -19.05341960407617918, 39.79275706135232582 ) ) ;
#124921=CARTESIAN_POINT ( 'NONE',  ( -5.719274019375978568, 21.55341960407610458, 45.20724293864769550 ) ) ;
#124922=CARTESIAN_POINT ( 'NONE',  ( 21.53943276465977519, -0.05219959533907433946, 33.74890960531436690 ) ) ;
#124923=CARTESIAN_POINT ( 'NONE',  ( 16.46253265017160672, -9.564922557960803928, 63.33224293864769550 ) ) ;
#124924=CARTESIAN_POINT ( 'NONE',  ( -9.564922557960796823, -16.46253265017161027, 52.08224293864768839 ) ) ;
#124925=CARTESIAN_POINT ( 'NONE',  ( 12.14591786802309770, 12.06949235617756955, 109.3739096053143811 ) ) ;
#124926=CARTESIAN_POINT ( 'NONE',  ( 21.53943276465977519, 0.05219959533937863772, 21.25109039468567218 ) ) ;
#124927=CARTESIAN_POINT ( 'NONE',  ( -5.049401038298153566, 19.05341960407611168, 110.2072429386476671 ) ) ;
#124928=CARTESIAN_POINT ( 'NONE',  ( 18.67979575497194134, -10.72451020669871369, 30.83442372801902209 ) ) ;
#124929=CARTESIAN_POINT ( 'NONE',  ( 16.51473224551069308, 9.474510206698969483, 29.16557627198103475 ) ) ;
#124930=CARTESIAN_POINT ( 'NONE',  ( -21.55341960407610458, -5.719274019375992779, 101.4572429386476955 ) ) ;
#124931=EDGE_CURVE ( 'NONE', #14227, #182496, #186386, .T. ) ;
#124932=CARTESIAN_POINT ( 'NONE',  ( 19.02544592524334988, 5.153800228976608722, 51.45942372801900433 ) ) ;
#124934=CARTESIAN_POINT ( 'NONE',  ( 19.05341960407611168, 5.049401038298154454, 28.95724293864769550 ) ) ;
#124935=DIRECTION ( 'NONE',  ( 1.000000000000000000, -0.000000000000000000, -0.000000000000000000 ) ) ;
#124936=CARTESIAN_POINT ( 'NONE',  ( 16.53943276465976808, 0.05219959533934440121, 61.25109039468567573 ) ) ;
#124937=CARTESIAN_POINT ( 'NONE',  ( 13.97604488694527802, 13.89961937509977652, 29.37390960531435979 ) ) ;
#124939=CARTESIAN_POINT ( 'NONE',  ( -5.153800228976328057, -19.02544592524343514, 77.29057627198099567 ) ) ;
#124940=CARTESIAN_POINT ( 'NONE',  ( -16.53943276465976808, 0.05219959533911058130, 111.2489096053143669 ) ) ;
#124941=CARTESIAN_POINT ( 'NONE',  ( -21.53943276465977519, 0.05219959533907696930, 61.24890960531435979 ) ) ;
#124942=CARTESIAN_POINT ( 'NONE',  ( 16.52544592524342804, -4.483927247898539470, 83.54057627198102409 ) ) ;
#124943=CARTESIAN_POINT ( 'NONE',  ( -12.14591786802326823, 12.06949235617739902, 28.12609039468568284 ) ) ;
#124944=CARTESIAN_POINT ( 'NONE',  ( 10.72451020669871369, 18.67979575497193778, 87.08442372801901854 ) ) ;
#124945=CARTESIAN_POINT ( 'NONE',  ( -9.564922557960796823, -16.46253265017161027, 32.08224293864769550 ) ) ;
#124947=CARTESIAN_POINT ( 'NONE',  ( -12.14591786802326823, 12.06949235617739902, 113.1260903946856899 ) ) ;
#124948=CARTESIAN_POINT ( 'NONE',  ( -8.224510206698948167, 14.34966873604960824, 55.41557627198102409 ) ) ;
#124949=CARTESIAN_POINT ( 'NONE',  ( 19.03943276465977164, -0.05219959533909143690, 53.74890960531436690 ) ) ;
#124950=CARTESIAN_POINT ( 'NONE',  ( -5.719274019375665041, -21.55341960407619695, 99.79275706135234714 ) ) ;
#124951=CARTESIAN_POINT ( 'NONE',  ( 5.823673210054125526, 21.52544592524343514, 104.7905762719810241 ) ) ;
#124952=CARTESIAN_POINT ( 'NONE',  ( -21.52544592524334988, -5.823673210054445271, 73.95942372801901854 ) ) ;
#124953=CARTESIAN_POINT ( 'NONE',  ( -4.483927247898782831, 16.52544592524335698, 37.70942372801900433 ) ) ;
#124954=CARTESIAN_POINT ( 'NONE',  ( 12.06949235617757843, -12.14591786802309237, 83.12390960531436690 ) ) ;
#124955=CARTESIAN_POINT ( 'NONE',  ( -18.67979575497193778, 10.72451020669871902, 83.33442372801903275 ) ) ;
#124956=CARTESIAN_POINT ( 'NONE',  ( 12.06949235617739724, 12.14591786802326823, 111.8760903946856615 ) ) ;
#124958=CARTESIAN_POINT ( 'NONE',  ( -16.53943276465976808, -0.05219959533934237506, 38.75109039468567573 ) ) ;
#124959=CARTESIAN_POINT ( 'NONE',  ( -0.05219959533910754901, -16.53943276465976808, 47.49890960531435979 ) ) ;
#124960=CARTESIAN_POINT ( 'NONE',  ( -12.06949235617739369, -12.14591786802326823, 89.37609039468568994 ) ) ;
#124961=CARTESIAN_POINT ( 'NONE',  ( 9.474510206698971260, -16.51473224551069308, 102.9155762719810241 ) ) ;
#124962=CARTESIAN_POINT ( 'NONE',  ( -9.564922557960796823, -16.46253265017161027, 112.0822429386476955 ) ) ;
#124963=CARTESIAN_POINT ( 'NONE',  ( -10.72451020669870658, -18.67979575497194134, 104.5844237280190185 ) ) ;
#124964=CARTESIAN_POINT ( 'NONE',  ( -12.14591786802326823, 12.06949235617739902, 103.1260903946856757 ) ) ;
#124965=CARTESIAN_POINT ( 'NONE',  ( 0.05219959533910956823, 16.53943276465976808, 74.99890960531435269 ) ) ;
#124966=CARTESIAN_POINT ( 'NONE',  ( -5.153800228976328057, -19.02544592524343514, 82.29057627198103830 ) ) ;
#124968=CARTESIAN_POINT ( 'NONE',  ( -4.483927247898782831, 16.52544592524335698, 22.70942372801901499 ) ) ;
#124969=CARTESIAN_POINT ( 'NONE',  ( 9.474510206698971260, -16.51473224551069308, 32.91557627198102409 ) ) ;
#124970=CARTESIAN_POINT ( 'NONE',  ( -9.564922557960796823, -16.46253265017161027, 87.08224293864769550 ) ) ;
#124971=CARTESIAN_POINT ( 'NONE',  ( -16.52544592524335698, -4.483927247898792601, 33.95942372801901143 ) ) ;
#124973=CARTESIAN_POINT ( 'NONE',  ( -0.05219959533936034679, 19.03943276465977164, 37.50109039468567573 ) ) ;
#124974=CARTESIAN_POINT ( 'NONE',  ( 12.06949235617739724, 12.14591786802326823, 96.87609039468568994 ) ) ;
#124975=CARTESIAN_POINT ( 'NONE',  ( 19.05341960407617918, -5.049401038297876454, 111.0427570613523329 ) ) ;
#124976=CARTESIAN_POINT ( 'NONE',  ( 9.474510206698971260, -16.51473224551069308, 27.91557627198103120 ) ) ;
#124977=CARTESIAN_POINT ( 'NONE',  ( 16.55341960407618274, -4.379528057220086978, 81.04275706135236135 ) ) ;
#124978=CARTESIAN_POINT ( 'NONE',  ( -16.52544592524335698, -4.483927247898792601, 68.95942372801901854 ) ) ;
#124979=CARTESIAN_POINT ( 'NONE',  ( 5.153800228976335163, 19.02544592524342804, 34.79057627198102409 ) ) ;
#124980=CARTESIAN_POINT ( 'NONE',  ( -13.89961937509957401, -13.97604488694547875, 64.37609039468567573 ) ) ;
#124981=CARTESIAN_POINT ( 'NONE',  ( 10.72451020669871369, 18.67979575497193778, 107.0844237280190043 ) ) ;
#124982=CARTESIAN_POINT ( 'NONE',  ( 19.05341960407611168, 5.049401038298154454, 48.95724293864768129 ) ) ;
#124983=CARTESIAN_POINT ( 'NONE',  ( 0.05219959533909260263, 19.03943276465977164, 94.99890960531436690 ) ) ;
#124984=CARTESIAN_POINT ( 'NONE',  ( -14.34966873604960291, -8.224510206698953496, 91.66557627198103830 ) ) ;
#124985=VECTOR ( 'NONE', #179002, 1000.000000000000000 ) ;
#124986=CARTESIAN_POINT ( 'NONE',  ( -16.46253265017146816, -9.564922557961047289, 49.16775706135233293 ) ) ;
#124987=CARTESIAN_POINT ( 'NONE',  ( 5.823673210054125526, 21.52544592524343514, 54.79057627198104541 ) ) ;
#124988=CARTESIAN_POINT ( 'NONE',  ( -19.05341960407617563, 5.049401038297882671, 23.54275706135233648 ) ) ;
#124989=CARTESIAN_POINT ( 'NONE',  ( -5.153800228976328057, -19.02544592524343514, 87.29057627198103830 ) ) ;
#124990=CARTESIAN_POINT ( 'NONE',  ( -16.46253265017146816, -9.564922557961047289, 24.16775706135233648 ) ) ;
#124991=CARTESIAN_POINT ( 'NONE',  ( 18.62759615963271287, -10.81492255796078972, 63.33224293864770260 ) ) ;
#124992=CARTESIAN_POINT ( 'NONE',  ( -19.05341960407611168, -5.049401038298163336, 106.4572429386476955 ) ) ;
#124994=CARTESIAN_POINT ( 'NONE',  ( -16.46253265017146816, -9.564922557961047289, 94.16775706135233293 ) ) ;
#124995=CARTESIAN_POINT ( 'NONE',  ( -13.89961937509977652, 13.97604488694528158, 110.6239096053143243 ) ) ;
#124996=CARTESIAN_POINT ( 'NONE',  ( 13.97604488694548053, -13.89961937509957401, 110.6260903946856615 ) ) ;
#124997=CARTESIAN_POINT ( 'NONE',  ( 16.53943276465976808, -0.05219959533910856209, 113.7489096053143527 ) ) ;
#124998=CARTESIAN_POINT ( 'NONE',  ( -19.02544592524342804, 5.153800228976336051, 96.04057627198103830 ) ) ;
#124999=CARTESIAN_POINT ( 'NONE',  ( -15.72974639402197994, 15.80617190586746368, 80.62390960531438111 ) ) ;
#125000=CARTESIAN_POINT ( 'NONE',  ( 12.14591786802327356, -12.06949235617739191, 50.62609039468568994 ) ) ;
#125001=CARTESIAN_POINT ( 'NONE',  ( -10.72451020669870658, -18.67979575497194134, 49.58442372801901143 ) ) ;
#125002=CARTESIAN_POINT ( 'NONE',  ( -21.55341960407619339, 5.719274019375674811, 103.5427570613523613 ) ) ;
#125003=CARTESIAN_POINT ( 'NONE',  ( 16.53943276465976808, 0.05219959533934440121, 91.25109039468568994 ) ) ;
#125004=CARTESIAN_POINT ( 'NONE',  ( 13.89961937509977652, -13.97604488694527269, 88.12390960531438111 ) ) ;
#125005=CARTESIAN_POINT ( 'NONE',  ( 12.14591786802309770, 12.06949235617756955, 84.37390960531438111 ) ) ;
#125006=CARTESIAN_POINT ( 'NONE',  ( -16.52544592524342804, 4.483927247898546575, 41.04057627198103120 ) ) ;
#125007=CARTESIAN_POINT ( 'NONE',  ( -9.564922557961040184, 16.46253265017147172, 67.91775706135233293 ) ) ;
#125008=CARTESIAN_POINT ( 'NONE',  ( 15.72974639402176855, 15.80617190586768217, 51.87609039468568284 ) ) ;
#125009=CARTESIAN_POINT ( 'NONE',  ( 0.05219959533936267826, -19.03943276465977164, 30.00109039468566863 ) ) ;
#125010=CARTESIAN_POINT ( 'NONE',  ( 0.05219959533910956823, 16.53943276465976808, 94.99890960531436690 ) ) ;
#125011=CARTESIAN_POINT ( 'NONE',  ( -15.80617190586745835, -15.72974639402198527, 26.87390960531435979 ) ) ;
#125012=CARTESIAN_POINT ( 'NONE',  ( -0.05219959533910754901, -16.53943276465976808, 22.49890960531436335 ) ) ;
#125013=CARTESIAN_POINT ( 'NONE',  ( 5.823673210054444382, -21.52544592524334988, 105.2094237280190328 ) ) ;
#125014=CARTESIAN_POINT ( 'NONE',  ( 14.29746914071037800, 8.314922557961029526, 61.66775706135235424 ) ) ;
#125015=CARTESIAN_POINT ( 'NONE',  ( 4.483927247898790824, -16.52544592524335698, 110.2094237280190185 ) ) ;
#125016=CARTESIAN_POINT ( 'NONE',  ( -21.53943276465977519, -0.05219959533937600094, 48.75109039468568284 ) ) ;
#125017=CARTESIAN_POINT ( 'NONE',  ( -21.53943276465977519, -0.05219959533937600094, 58.75109039468568994 ) ) ;
#125019=CARTESIAN_POINT ( 'NONE',  ( 10.81492255796106328, -18.62759615963255655, 30.41775706135234358 ) ) ;
#125020=CARTESIAN_POINT ( 'NONE',  ( 16.55341960407611168, 4.379528057220329451, 98.95724293864770971 ) ) ;
#125021=CARTESIAN_POINT ( 'NONE',  ( 5.153800228976335163, 19.02544592524342804, 24.79057627198102765 ) ) ;
#125022=CARTESIAN_POINT ( 'NONE',  ( -4.483927247898539470, -16.52544592524342804, 67.29057627198103830 ) ) ;
#125023=CARTESIAN_POINT ( 'NONE',  ( -16.46253265017160317, 9.564922557960807481, 70.83224293864770971 ) ) ;
#125024=CARTESIAN_POINT ( 'NONE',  ( -12.14591786802326823, 12.06949235617739902, 108.1260903946856757 ) ) ;
#125025=CARTESIAN_POINT ( 'NONE',  ( -18.62759615963270932, 10.81492255796079327, 60.83224293864769550 ) ) ;
#125026=CARTESIAN_POINT ( 'NONE',  ( -16.53943276465976808, 0.05219959533911058130, 86.24890960531436690 ) ) ;
#125027=CARTESIAN_POINT ( 'NONE',  ( -0.05219959533907301413, -21.53943276465977519, 97.49890960531436690 ) ) ;
#125028=CARTESIAN_POINT ( 'NONE',  ( -19.03943276465977164, 0.05219959533909376836, 101.2489096053143669 ) ) ;
#125029=CARTESIAN_POINT ( 'NONE',  ( -9.474510206698964154, 16.51473224551069663, 45.41557627198103120 ) ) ;
#125030=CARTESIAN_POINT ( 'NONE',  ( 13.97604488694548053, -13.89961937509957401, 110.6260903946856615 ) ) ;
#125031=CARTESIAN_POINT ( 'NONE',  ( 21.52544592524344225, -5.823673210054117533, 38.54057627198103120 ) ) ;
#125032=CARTESIAN_POINT ( 'NONE',  ( -21.55341960407619339, 5.719274019375674811, 63.54275706135234003 ) ) ;
#125033=CARTESIAN_POINT ( 'NONE',  ( -9.564922557960796823, -16.46253265017161027, 67.08224293864769550 ) ) ;
#125034=CARTESIAN_POINT ( 'NONE',  ( -13.97604488694527625, -13.89961937509977652, 96.87390960531433848 ) ) ;
#125035=CARTESIAN_POINT ( 'NONE',  ( -4.483927247898782831, 16.52544592524335698, 62.70942372801902565 ) ) ;
#125036=CARTESIAN_POINT ( 'NONE',  ( 10.72451020669871369, 18.67979575497193778, 47.08442372801901854 ) ) ;
#125037=CARTESIAN_POINT ( 'NONE',  ( 18.67979575497194134, -10.72451020669871369, 80.83442372801901854 ) ) ;
#125038=CARTESIAN_POINT ( 'NONE',  ( -21.52544592524343514, 5.823673210054127303, 101.0405762719810383 ) ) ;
#125039=CARTESIAN_POINT ( 'NONE',  ( -10.72451020669870658, -18.67979575497194134, 34.58442372801900433 ) ) ;
#125040=CARTESIAN_POINT ( 'NONE',  ( -4.483927247898782831, 16.52544592524335698, 77.70942372801900433 ) ) ;
#125041=CARTESIAN_POINT ( 'NONE',  ( -5.719274019375978568, 21.55341960407610458, 75.20724293864769550 ) ) ;
#125042=CARTESIAN_POINT ( 'NONE',  ( -16.46253265017146816, -9.564922557961047289, 29.16775706135232937 ) ) ;
#125043=CARTESIAN_POINT ( 'NONE',  ( 13.97604488694527802, 13.89961937509977652, 79.37390960531435269 ) ) ;
#125044=CARTESIAN_POINT ( 'NONE',  ( 8.314922557960818139, 14.29746914071049879, 29.58224293864769905 ) ) ;
#125046=CARTESIAN_POINT ( 'NONE',  ( 5.049401038298161559, -19.05341960407611168, 97.70724293864766707 ) ) ;
#125048=CARTESIAN_POINT ( 'NONE',  ( -19.03943276465977164, -0.05219959533935918106, 83.75109039468567573 ) ) ;
#125049=CARTESIAN_POINT ( 'NONE',  ( 10.72451020669898902, -18.67979575497178502, 57.91557627198103120 ) ) ;
#125050=CARTESIAN_POINT ( 'NONE',  ( 0.05219959533910956823, 16.53943276465976808, 44.99890960531435979 ) ) ;
#125051=CARTESIAN_POINT ( 'NONE',  ( -0.05219959533936034679, 19.03943276465977164, 107.5010903946856615 ) ) ;
#125052=CARTESIAN_POINT ( 'NONE',  ( -5.049401038298153566, 19.05341960407611168, 35.20724293864768839 ) ) ;
#125053=CARTESIAN_POINT ( 'NONE',  ( -13.89961937509957401, -13.97604488694547875, 104.3760903946856757 ) ) ;
#125054=CARTESIAN_POINT ( 'NONE',  ( 21.52544592524344225, -5.823673210054117533, 103.5405762719810383 ) ) ;
#125055=CARTESIAN_POINT ( 'NONE',  ( 0.05219959533936267826, -19.03943276465977164, 70.00109039468566152 ) ) ;
#125056=CARTESIAN_POINT ( 'NONE',  ( -0.05219959533934338120, 16.53943276465976808, 77.50109039468567573 ) ) ;
#125057=CARTESIAN_POINT ( 'NONE',  ( -19.02544592524342804, 5.153800228976336051, 71.04057627198099567 ) ) ;
#125058=CARTESIAN_POINT ( 'NONE',  ( 16.55341960407611168, 4.379528057220329451, 78.95724293864769550 ) ) ;
#125059=CARTESIAN_POINT ( 'NONE',  ( -19.02544592524342804, 5.153800228976336051, 66.04057627198103830 ) ) ;
#125060=CARTESIAN_POINT ( 'NONE',  ( -12.06949235617756955, 12.14591786802309770, 65.62390960531436690 ) ) ;
#125063=CARTESIAN_POINT ( 'NONE',  ( 0.05219959533910956823, 16.53943276465976808, 44.99890960531435979 ) ) ;
#125064=CARTESIAN_POINT ( 'NONE',  ( 16.46253265017160672, -9.564922557960803928, 73.33224293864769550 ) ) ;
#125066=CARTESIAN_POINT ( 'NONE',  ( -19.02544592524334988, -5.153800228976617603, 43.95942372801899012 ) ) ;
#125067=CARTESIAN_POINT ( 'NONE',  ( -16.53943276465976808, -0.05219959533934237506, 63.75109039468568284 ) ) ;
#125068=CARTESIAN_POINT ( 'NONE',  ( -5.719274019375978568, 21.55341960407610458, 70.20724293864769550 ) ) ;
#125069=CARTESIAN_POINT ( 'NONE',  ( 13.97604488694548053, -13.89961937509957401, 20.62609039468567573 ) ) ;
#125070=CARTESIAN_POINT ( 'NONE',  ( -19.05341960407611168, -5.049401038298163336, 71.45724293864766707 ) ) ;
#125072=CARTESIAN_POINT ( 'NONE',  ( -9.474510206698964154, 16.51473224551069663, 110.4155762719810383 ) ) ;
#125073=CARTESIAN_POINT ( 'NONE',  ( -5.049401038298153566, 19.05341960407611168, 60.20724293864768129 ) ) ;
#125074=CARTESIAN_POINT ( 'NONE',  ( -21.52544592524334988, -5.823673210054445271, 43.95942372801902565 ) ) ;
#125075=CARTESIAN_POINT ( 'NONE',  ( -8.314922557960811034, -14.29746914071050412, 102.0822429386476955 ) ) ;
#125076=CARTESIAN_POINT ( 'NONE',  ( -10.81492255796078084, -18.62759615963271287, 102.0822429386476955 ) ) ;
#125077=CARTESIAN_POINT ( 'NONE',  ( -13.89961937509977652, 13.97604488694528158, 85.62390960531433848 ) ) ;
#125078=EDGE_LOOP ( 'NONE', ( #176117, #41129 ) ) ;
#125079=CARTESIAN_POINT ( 'NONE',  ( -21.53943276465977519, -0.05219959533937600094, 23.75109039468567929 ) ) ;
#125081=CARTESIAN_POINT ( 'NONE',  ( 16.51473224551069308, 9.474510206698969483, 84.16557627198102409 ) ) ;
#125082=DIRECTION ( 'NONE',  ( -1.000000000000000000, 0.000000000000000000, 0.000000000000000000 ) ) ;
#125083=CARTESIAN_POINT ( 'NONE',  ( 21.53943276465977519, -0.05219959533907433946, 98.74890960531438111 ) ) ;
#125084=CARTESIAN_POINT ( 'NONE',  ( -0.05219959533909027116, -19.03943276465977164, 42.49890960531435269 ) ) ;
#125085=CARTESIAN_POINT ( 'NONE',  ( 19.03943276465977164, 0.05219959533936151252, 101.2510903946856757 ) ) ;
#125087=CARTESIAN_POINT ( 'NONE',  ( -5.153800228976328057, -19.02544592524343514, 27.29057627198103120 ) ) ;
#125088=CARTESIAN_POINT ( 'NONE',  ( 18.62759615963255655, 10.81492255796105972, 91.66775706135234714 ) ) ;
#125089=CARTESIAN_POINT ( 'NONE',  ( -13.89961937509977652, 13.97604488694528158, 70.62390960531432427 ) ) ;
#125090=CARTESIAN_POINT ( 'NONE',  ( -5.719274019375665041, -21.55341960407619695, 44.79275706135234714 ) ) ;
#125091=CARTESIAN_POINT ( 'NONE',  ( -5.719274019375665041, -21.55341960407619695, 29.79275706135234358 ) ) ;
#125093=CARTESIAN_POINT ( 'NONE',  ( -19.05341960407611168, -5.049401038298163336, 91.45724293864766707 ) ) ;
#125095=CARTESIAN_POINT ( 'NONE',  ( 12.14591786802327356, -12.06949235617739191, 45.62609039468567573 ) ) ;
#125096=CARTESIAN_POINT ( 'NONE',  ( -10.81492255796078084, -18.62759615963271287, 47.08224293864770260 ) ) ;
#125097=CARTESIAN_POINT ( 'NONE',  ( -18.62759615963255300, -10.81492255796106328, 39.16775706135235424 ) ) ;
#125098=CARTESIAN_POINT ( 'NONE',  ( -5.823673210054431948, 21.52544592524334988, 72.70942372801901854 ) ) ;
#125099=CARTESIAN_POINT ( 'NONE',  ( 18.09873248133749257, -5.500000000000147438, 38.51607049666168336 ) ) ;
#125100=CARTESIAN_POINT ( 'NONE',  ( -16.51473224551082808, 9.474510206698731452, 108.3344237280190043 ) ) ;
#125101=CARTESIAN_POINT ( 'NONE',  ( 0.05219959533909260263, 19.03943276465977164, 54.99890960531435979 ) ) ;
#125102=CARTESIAN_POINT ( 'NONE',  ( 9.564922557960805705, 16.46253265017160317, 84.58224293864769550 ) ) ;
#125103=EDGE_CURVE ( 'NONE', #114833, #113576, #39177, .T. ) ;
#125104=CARTESIAN_POINT ( 'NONE',  ( 8.314922557960818139, 14.29746914071049879, 104.5822429386477097 ) ) ;
#125105=CARTESIAN_POINT ( 'NONE',  ( -4.483927247898539470, -16.52544592524342804, 102.2905762719810383 ) ) ;
#125106=CARTESIAN_POINT ( 'NONE',  ( -19.03943276465977164, 0.05219959533909376836, 111.2489096053143669 ) ) ;
#125107=CARTESIAN_POINT ( 'NONE',  ( -12.14591786802326823, 12.06949235617739902, 83.12609039468568994 ) ) ;
#125108=CARTESIAN_POINT ( 'NONE',  ( 0.05219959533910956823, 16.53943276465976808, 74.99890960531435269 ) ) ;
#125109=CARTESIAN_POINT ( 'NONE',  ( -5.049401038298153566, 19.05341960407611168, 55.20724293864769550 ) ) ;
#125110=CARTESIAN_POINT ( 'NONE',  ( 21.53943276465977519, 0.05219959533937863772, 81.25109039468568994 ) ) ;
#125111=CARTESIAN_POINT ( 'NONE',  ( 15.72974639402176855, 15.80617190586768217, 76.87609039468567573 ) ) ;
#125112=CARTESIAN_POINT ( 'NONE',  ( 19.03943276465977164, 0.05219959533936151252, 106.2510903946856615 ) ) ;
#125113=CARTESIAN_POINT ( 'NONE',  ( -12.06949235617756955, 12.14591786802309770, 60.62390960531437401 ) ) ;
#125114=CARTESIAN_POINT ( 'NONE',  ( -18.67979575497193778, 10.72451020669871902, 28.33442372801902209 ) ) ;
#125115=CARTESIAN_POINT ( 'NONE',  ( -10.81492255796078084, -18.62759615963271287, 62.08224293864769550 ) ) ;
#125116=DIRECTION ( 'NONE',  ( 1.000000000000000000, -0.000000000000000000, -0.000000000000000000 ) ) ;
#125118=CARTESIAN_POINT ( 'NONE',  ( 5.153800228976335163, 19.02544592524342804, 74.79057627198103830 ) ) ;
#125119=CARTESIAN_POINT ( 'NONE',  ( -16.55341960407611168, -4.379528057220339221, 36.45724293864768839 ) ) ;
#125121=CARTESIAN_POINT ( 'NONE',  ( -4.379528057220086978, -16.55341960407618274, 109.7927570613523613 ) ) ;
#125122=CARTESIAN_POINT ( 'NONE',  ( 8.224510206698742110, 14.34966873604972548, 102.0844237280190185 ) ) ;
#125123=CARTESIAN_POINT ( 'NONE',  ( -16.46253265017146816, -9.564922557961047289, 54.16775706135234003 ) ) ;
#125125=CARTESIAN_POINT ( 'NONE',  ( 9.564922557960805705, 16.46253265017160317, 104.5822429386476955 ) ) ;
#125127=CARTESIAN_POINT ( 'NONE',  ( -8.224510206698948167, 14.34966873604960824, 80.41557627198103830 ) ) ;
#125128=CARTESIAN_POINT ( 'NONE',  ( -13.89961937509957401, -13.97604488694547875, 39.37609039468566152 ) ) ;
#125129=CARTESIAN_POINT ( 'NONE',  ( 5.049401038298161559, -19.05341960407611168, 22.70724293864769194 ) ) ;
#125130=CARTESIAN_POINT ( 'NONE',  ( 16.46253265017160672, -9.564922557960803928, 113.3322429386476955 ) ) ;
#125131=CARTESIAN_POINT ( 'NONE',  ( -10.72451020669898014, 18.67979575497178502, 60.41557627198102409 ) ) ;
#125132=CARTESIAN_POINT ( 'NONE',  ( -12.06949235617756955, 12.14591786802309770, 100.6239096053143811 ) ) ;
#125133=CARTESIAN_POINT ( 'NONE',  ( -16.53943276465976808, -0.05219959533934237506, 48.75109039468568284 ) ) ;
#125134=CARTESIAN_POINT ( 'NONE',  ( 8.224510206698953496, -14.34966873604960469, 87.91557627198103830 ) ) ;
#125135=CARTESIAN_POINT ( 'NONE',  ( 16.31925111598458145, -7.325300261831445781, 37.66424538967251578 ) ) ;
#125136=CARTESIAN_POINT ( 'NONE',  ( -16.36317988757059538, 7.306389748694931185, 49.09789608363226421 ) ) ;
#125137=CARTESIAN_POINT ( 'NONE',  ( -18.62759615963270932, 10.81492255796079327, 25.83224293864769194 ) ) ;
#125140=CARTESIAN_POINT ( 'NONE',  ( -14.34966873604972548, 8.224510206698743886, 43.33442372801901143 ) ) ;
#125141=CARTESIAN_POINT ( 'NONE',  ( -12.06949235617756955, 12.14591786802309770, 25.62390960531435624 ) ) ;
#125142=CARTESIAN_POINT ( 'NONE',  ( 10.81492255796078972, 18.62759615963270932, 54.58224293864769550 ) ) ;
#125143=CARTESIAN_POINT ( 'NONE',  ( 19.03943276465977164, 0.05219959533936151252, 86.25109039468567573 ) ) ;
#125144=CARTESIAN_POINT ( 'NONE',  ( -21.52544592524343514, 5.823673210054127303, 51.04057627198103120 ) ) ;
#125145=CARTESIAN_POINT ( 'NONE',  ( 5.823673210054444382, -21.52544592524334988, 80.20942372801901854 ) ) ;
#125147=CARTESIAN_POINT ( 'NONE',  ( -8.224510206698735004, -14.34966873604973081, 34.58442372801900433 ) ) ;
#125148=CARTESIAN_POINT ( 'NONE',  ( 19.05341960407611168, 5.049401038298154454, 43.95724293864769550 ) ) ;
#125149=CARTESIAN_POINT ( 'NONE',  ( -0.05219959533909027116, -19.03943276465977164, 97.49890960531436690 ) ) ;
#125150=CARTESIAN_POINT ( 'NONE',  ( -13.89961937509977652, 13.97604488694528158, 35.62390960531435269 ) ) ;
#125151=CARTESIAN_POINT ( 'NONE',  ( 8.314922557960818139, 14.29746914071049879, 99.58224293864770971 ) ) ;
#125153=CARTESIAN_POINT ( 'NONE',  ( 0.05219959533909260263, 19.03943276465977164, 94.99890960531436690 ) ) ;
#125155=CARTESIAN_POINT ( 'NONE',  ( 14.34966873604972726, -8.224510206698740333, 50.83442372801901143 ) ) ;
#125156=CARTESIAN_POINT ( 'NONE',  ( -0.05219959533907301413, -21.53943276465977519, 87.49890960531436690 ) ) ;
#125157=CARTESIAN_POINT ( 'NONE',  ( -0.05219959533909027116, -19.03943276465977164, 62.49890960531435979 ) ) ;
#125158=CARTESIAN_POINT ( 'NONE',  ( -21.53943276465977519, -0.05219959533937600094, 28.75109039468567929 ) ) ;
#125159=CARTESIAN_POINT ( 'NONE',  ( -13.97604488694527625, -13.89961937509977652, 86.87390960531436690 ) ) ;
#125162=CARTESIAN_POINT ( 'NONE',  ( 16.55341960407618274, -4.379528057220086978, 41.04275706135236135 ) ) ;
#125163=CARTESIAN_POINT ( 'NONE',  ( -18.62759615963255300, -10.81492255796106328, 24.16775706135235424 ) ) ;
#125164=CARTESIAN_POINT ( 'NONE',  ( 9.564922557960805705, 16.46253265017160317, 29.58224293864769550 ) ) ;
#125165=CARTESIAN_POINT ( 'NONE',  ( -5.153800228976328057, -19.02544592524343514, 87.29057627198103830 ) ) ;
#125166=CARTESIAN_POINT ( 'NONE',  ( -13.89961937509957401, -13.97604488694547875, 79.37609039468567573 ) ) ;
#125167=CARTESIAN_POINT ( 'NONE',  ( -13.97604488694547697, 13.89961937509957934, 28.12609039468565797 ) ) ;
#125168=CARTESIAN_POINT ( 'NONE',  ( -5.823673210054116645, -21.52544592524344225, 92.29057627198103830 ) ) ;
#125169=CARTESIAN_POINT ( 'NONE',  ( -16.51473224551082808, 9.474510206698731452, 38.33442372801899722 ) ) ;
#125170=CARTESIAN_POINT ( 'NONE',  ( -14.34966873604972548, 8.224510206698743886, 73.33442372801901854 ) ) ;
#125171=CARTESIAN_POINT ( 'NONE',  ( -9.474510206698964154, 16.51473224551069663, 105.4155762719810383 ) ) ;
#125173=CARTESIAN_POINT ( 'NONE',  ( -5.049401038298153566, 19.05341960407611168, 60.20724293864768129 ) ) ;
#125175=CARTESIAN_POINT ( 'NONE',  ( 10.72451020669871369, 18.67979575497193778, 67.08442372801901854 ) ) ;
#125176=CARTESIAN_POINT ( 'NONE',  ( -21.55341960407619339, 5.719274019375674811, 63.54275706135234003 ) ) ;
#125177=CARTESIAN_POINT ( 'NONE',  ( -9.564922557960796823, -16.46253265017161027, 72.08224293864770971 ) ) ;
#125178=CARTESIAN_POINT ( 'NONE',  ( -10.72451020669870658, -18.67979575497194134, 49.58442372801901143 ) ) ;
#125180=CARTESIAN_POINT ( 'NONE',  ( 16.46253265017146816, 9.564922557961045513, 81.66775706135233293 ) ) ;
#125181=CARTESIAN_POINT ( 'NONE',  ( -13.97604488694527625, -13.89961937509977652, 51.87390960531436690 ) ) ;
#125182=CARTESIAN_POINT ( 'NONE',  ( -19.02544592524342804, 5.153800228976336051, 101.0405762719810241 ) ) ;
#125183=CARTESIAN_POINT ( 'NONE',  ( -19.05341960407611168, -5.049401038298163336, 66.45724293864769550 ) ) ;
#125184=CARTESIAN_POINT ( 'NONE',  ( -16.51473224551069308, -9.474510206698971260, 111.6655762719810383 ) ) ;
#125185=CARTESIAN_POINT ( 'NONE',  ( 19.02544592524343514, -5.153800228976328945, 58.54057627198102409 ) ) ;
#125186=CARTESIAN_POINT ( 'NONE',  ( -5.719274019375978568, 21.55341960407610458, 105.2072429386477097 ) ) ;
#125187=CARTESIAN_POINT ( 'NONE',  ( 16.52544592524335698, 4.483927247898782831, 76.45942372801901854 ) ) ;
#125189=CARTESIAN_POINT ( 'NONE',  ( -13.89961937509957401, -13.97604488694547875, 29.37609039468565797 ) ) ;
#125190=CARTESIAN_POINT ( 'NONE',  ( 9.564922557960805705, 16.46253265017160317, 64.58224293864769550 ) ) ;
#125191=CARTESIAN_POINT ( 'NONE',  ( 4.379528057220339221, -16.55341960407611168, 57.70724293864770260 ) ) ;
#125192=CARTESIAN_POINT ( 'NONE',  ( -12.14591786802309592, -12.06949235617757132, 91.87390960531436690 ) ) ;
#125193=CARTESIAN_POINT ( 'NONE',  ( -5.153800228976328057, -19.02544592524343514, 107.2905762719810383 ) ) ;
#125194=CARTESIAN_POINT ( 'NONE',  ( 0.05219959533909260263, 19.03943276465977164, 94.99890960531436690 ) ) ;
#125195=CARTESIAN_POINT ( 'NONE',  ( -0.05219959533909027116, -19.03943276465977164, 112.4989096053143669 ) ) ;
#125196=CARTESIAN_POINT ( 'NONE',  ( 0.05219959533937995610, -21.53943276465977519, 110.0010903946856757 ) ) ;
#125197=CARTESIAN_POINT ( 'NONE',  ( 0.05219959533934541429, -16.53943276465976808, 95.00109039468568994 ) ) ;
#125198=CARTESIAN_POINT ( 'NONE',  ( -0.05219959533937732626, 21.53943276465977519, 42.50109039468567573 ) ) ;
#125199=CARTESIAN_POINT ( 'NONE',  ( 18.67979575497178502, 10.72451020669898547, 34.16557627198102409 ) ) ;
#125200=CARTESIAN_POINT ( 'NONE',  ( -0.05219959533907301413, -21.53943276465977519, 102.4989096053143811 ) ) ;
#125201=CARTESIAN_POINT ( 'NONE',  ( 16.52544592524342804, -4.483927247898539470, 58.54057627198103120 ) ) ;
#125202=CARTESIAN_POINT ( 'NONE',  ( 5.153800228976335163, 19.02544592524342804, 59.79057627198100988 ) ) ;
#125203=CARTESIAN_POINT ( 'NONE',  ( 12.14591786802309770, 12.06949235617756955, 84.37390960531438111 ) ) ;
#125204=CARTESIAN_POINT ( 'NONE',  ( 21.52544592524344225, -5.823673210054117533, 43.54057627198103830 ) ) ;
#125205=CARTESIAN_POINT ( 'NONE',  ( 0.05219959533936267826, -19.03943276465977164, 45.00109039468566863 ) ) ;
#125206=CARTESIAN_POINT ( 'NONE',  ( 4.379528057220339221, -16.55341960407611168, 107.7072429386476955 ) ) ;
#125208=CARTESIAN_POINT ( 'NONE',  ( 16.53943276465976808, 0.05219959533934440121, 71.25109039468568994 ) ) ;
#125209=CARTESIAN_POINT ( 'NONE',  ( -9.564922557960796823, -16.46253265017161027, 72.08224293864770971 ) ) ;
#125211=CARTESIAN_POINT ( 'NONE',  ( -8.224510206698948167, 14.34966873604960824, 85.41557627198102409 ) ) ;
#125212=CARTESIAN_POINT ( 'NONE',  ( 15.80617190586746368, 15.72974639402197994, 34.37390960531435979 ) ) ;
#125213=CARTESIAN_POINT ( 'NONE',  ( 4.483927247898790824, -16.52544592524335698, 105.2094237280190328 ) ) ;
#125214=CARTESIAN_POINT ( 'NONE',  ( -8.314922557961024197, 14.29746914071037800, 22.91775706135235069 ) ) ;
#125215=CARTESIAN_POINT ( 'NONE',  ( 5.719274019375673035, 21.55341960407619339, 92.29275706135236135 ) ) ;
#125216=CARTESIAN_POINT ( 'NONE',  ( 19.02544592524343514, -5.153800228976328945, 83.54057627198100988 ) ) ;
#125217=CARTESIAN_POINT ( 'NONE',  ( -21.52544592524334988, -5.823673210054445271, 18.95942372801901143 ) ) ;
#125218=CARTESIAN_POINT ( 'NONE',  ( -16.51473224551069308, -9.474510206698971260, 36.66557627198102409 ) ) ;
#125219=CARTESIAN_POINT ( 'NONE',  ( -4.483927247898782831, 16.52544592524335698, 32.70942372801900433 ) ) ;
#125220=CARTESIAN_POINT ( 'NONE',  ( -0.05219959533936034679, 19.03943276465977164, 92.50109039468566152 ) ) ;
#125221=CARTESIAN_POINT ( 'NONE',  ( -21.53943276465977519, 0.05219959533907696930, 96.24890960531435269 ) ) ;
#125222=CARTESIAN_POINT ( 'NONE',  ( 5.153800228976615827, -19.02544592524334988, 65.20942372801900433 ) ) ;
#125224=CARTESIAN_POINT ( 'NONE',  ( -10.72451020669870658, -18.67979575497194134, 24.58442372801901499 ) ) ;
#125226=CARTESIAN_POINT ( 'NONE',  ( -19.05341960407611168, -5.049401038298163336, 76.45724293864769550 ) ) ;
#125227=CARTESIAN_POINT ( 'NONE',  ( 4.483927247898790824, -16.52544592524335698, 30.20942372801902565 ) ) ;
#125229=CARTESIAN_POINT ( 'NONE',  ( 0.05219959533936267826, -19.03943276465977164, 65.00109039468567573 ) ) ;
#125230=CARTESIAN_POINT ( 'NONE',  ( 5.823673210054125526, 21.52544592524343514, 114.7905762719810383 ) ) ;
#125231=CARTESIAN_POINT ( 'NONE',  ( -16.52544592524342804, 4.483927247898546575, 81.04057627198102409 ) ) ;
#125232=CARTESIAN_POINT ( 'NONE',  ( 19.02544592524343514, -5.153800228976328945, 78.54057627198099567 ) ) ;
#125233=CARTESIAN_POINT ( 'NONE',  ( -16.53943276465976808, -0.05219959533934237506, 33.75109039468568284 ) ) ;
#125234=CARTESIAN_POINT ( 'NONE',  ( 13.89961937509957401, 13.97604488694547697, 36.87609039468565442 ) ) ;
#125235=CARTESIAN_POINT ( 'NONE',  ( 5.719274019375673035, 21.55341960407619339, 62.29275706135236845 ) ) ;
#125236=CARTESIAN_POINT ( 'NONE',  ( -13.97604488694547697, 13.89961937509957934, 103.1260903946856473 ) ) ;
#125237=CARTESIAN_POINT ( 'NONE',  ( -19.02544592524342804, 5.153800228976336051, 56.04057627198100988 ) ) ;
#125238=CARTESIAN_POINT ( 'NONE',  ( 13.89961937509957401, 13.97604488694547697, 86.87609039468567573 ) ) ;
#125239=CARTESIAN_POINT ( 'NONE',  ( -14.29746914071037622, -8.314922557961029526, 54.16775706135235424 ) ) ;
#125240=CARTESIAN_POINT ( 'NONE',  ( 18.67979575497194134, -10.72451020669871369, 100.8344237280190185 ) ) ;
#125241=CARTESIAN_POINT ( 'NONE',  ( -16.51473224551082808, 9.474510206698731452, 63.33442372801900433 ) ) ;
#125242=CARTESIAN_POINT ( 'NONE',  ( -13.97604488694527625, -13.89961937509977652, 46.87390960531435979 ) ) ;
#125243=CARTESIAN_POINT ( 'NONE',  ( -21.52544592524343514, 5.823673210054127303, 76.04057627198102409 ) ) ;
#125244=CARTESIAN_POINT ( 'NONE',  ( 8.224510206698953496, -14.34966873604960469, 67.91557627198102409 ) ) ;
#125245=CARTESIAN_POINT ( 'NONE',  ( -13.97604488694547697, 13.89961937509957934, 63.12609039468566152 ) ) ;
#125247=CARTESIAN_POINT ( 'NONE',  ( -9.564922557961040184, 16.46253265017147172, 42.91775706135234003 ) ) ;
#125248=CARTESIAN_POINT ( 'NONE',  ( 4.483927247898790824, -16.52544592524335698, 95.20942372801903275 ) ) ;
#125249=CARTESIAN_POINT ( 'NONE',  ( -16.55341960407611168, -4.379528057220339221, 61.45724293864770260 ) ) ;
#125250=CARTESIAN_POINT ( 'NONE',  ( 21.52544592524334988, 5.823673210054432836, 91.45942372801901854 ) ) ;
#125252=CARTESIAN_POINT ( 'NONE',  ( 18.67979575497178502, 10.72451020669898547, 99.16557627198100988 ) ) ;
#125253=CARTESIAN_POINT ( 'NONE',  ( 9.474510206698971260, -16.51473224551069308, 57.91557627198103120 ) ) ;
#125254=CARTESIAN_POINT ( 'NONE',  ( 21.52544592524334988, 5.823673210054432836, 71.45942372801901854 ) ) ;
#125255=CARTESIAN_POINT ( 'NONE',  ( 9.564922557960805705, 16.46253265017160317, 49.58224293864770260 ) ) ;
#125257=CARTESIAN_POINT ( 'NONE',  ( -9.564922557960796823, -16.46253265017161027, 62.08224293864769550 ) ) ;
#125258=CARTESIAN_POINT ( 'NONE',  ( -0.05219959533909027116, -19.03943276465977164, 22.49890960531436690 ) ) ;
#125259=CARTESIAN_POINT ( 'NONE',  ( -19.05341960407611168, -5.049401038298163336, 106.4572429386476955 ) ) ;
#125260=CARTESIAN_POINT ( 'NONE',  ( 12.14591786802309770, 12.06949235617756955, 59.37390960531436690 ) ) ;
#125261=CARTESIAN_POINT ( 'NONE',  ( 13.89961937509977652, -13.97604488694527269, 28.12390960531435624 ) ) ;
#125262=CARTESIAN_POINT ( 'NONE',  ( -16.53943276465976808, 0.05219959533911058130, 91.24890960531436690 ) ) ;
#125263=VECTOR ( 'NONE', #99002, 1000.000000000000000 ) ;
#125264=CARTESIAN_POINT ( 'NONE',  ( 5.719274019375991003, -21.55341960407610458, 97.70724293864772392 ) ) ;
#125265=CARTESIAN_POINT ( 'NONE',  ( 21.53943276465977519, 0.05219959533937863772, 41.25109039468568284 ) ) ;
#125267=CARTESIAN_POINT ( 'NONE',  ( 16.53943276465976808, 0.05219959533934440121, 51.25109039468568994 ) ) ;
#125268=CARTESIAN_POINT ( 'NONE',  ( 5.823673210054125526, 21.52544592524343514, 89.79057627198103830 ) ) ;
#125269=CARTESIAN_POINT ( 'NONE',  ( 10.72451020669871369, 18.67979575497193778, 107.0844237280190043 ) ) ;
#125270=CARTESIAN_POINT ( 'NONE',  ( -9.564922557960796823, -16.46253265017161027, 107.0822429386476955 ) ) ;
#125271=CARTESIAN_POINT ( 'NONE',  ( -21.52544592524334988, -5.823673210054445271, 48.95942372801902565 ) ) ;
#125273=CARTESIAN_POINT ( 'NONE',  ( -0.05219959533907301413, -21.53943276465977519, 47.49890960531435979 ) ) ;
#125274=CARTESIAN_POINT ( 'NONE',  ( -12.06949235617739369, -12.14591786802326823, 99.37609039468568994 ) ) ;
#125275=CARTESIAN_POINT ( 'NONE',  ( -0.05219959533937732626, 21.53943276465977519, 67.50109039468568994 ) ) ;
#125276=CARTESIAN_POINT ( 'NONE',  ( 18.67979575497194134, -10.72451020669871369, 100.8344237280190185 ) ) ;
#125277=CARTESIAN_POINT ( 'NONE',  ( -16.46253265017146816, -9.564922557961047289, 34.16775706135233293 ) ) ;
#125278=CARTESIAN_POINT ( 'NONE',  ( -16.52544592524335698, -4.483927247898792601, 83.95942372801900433 ) ) ;
#125279=CARTESIAN_POINT ( 'NONE',  ( 0.05219959533937995610, -21.53943276465977519, 40.00109039468567573 ) ) ;
#125280=CARTESIAN_POINT ( 'NONE',  ( -16.51473224551069308, -9.474510206698971260, 46.66557627198102409 ) ) ;
#125281=CARTESIAN_POINT ( 'NONE',  ( 9.474510206698729675, 16.51473224551082808, 22.08442372801899722 ) ) ;
#125282=CARTESIAN_POINT ( 'NONE',  ( -10.81492255796078084, -18.62759615963271287, 22.08224293864769194 ) ) ;
#125283=CARTESIAN_POINT ( 'NONE',  ( -18.67979575497193778, 10.72451020669871902, 23.33442372801901499 ) ) ;
#125284=CARTESIAN_POINT ( 'NONE',  ( -15.80617190586745835, -15.72974639402198527, 71.87390960531438111 ) ) ;
#125285=CARTESIAN_POINT ( 'NONE',  ( -17.49999999999999645, -7.500000000000000888, 37.49999999999999289 ) ) ;
#125286=CARTESIAN_POINT ( 'NONE',  ( 10.81492255796078972, 18.62759615963270932, 84.58224293864769550 ) ) ;
#125287=CARTESIAN_POINT ( 'NONE',  ( 14.34966873604972726, -8.224510206698740333, 65.83442372801900433 ) ) ;
#125288=CARTESIAN_POINT ( 'NONE',  ( 16.53943276465976808, -0.05219959533910856209, 68.74890960531435269 ) ) ;
#125290=CARTESIAN_POINT ( 'NONE',  ( 16.46253265017146816, 9.564922557961045513, 96.66775706135233293 ) ) ;
#125292=AXIS2_PLACEMENT_3D ( 'NONE', #169608, #79584, #31106 ) ;
#125294=CARTESIAN_POINT ( 'NONE',  ( 12.06949235617739724, 12.14591786802326823, 41.87609039468568284 ) ) ;
#125295=CARTESIAN_POINT ( 'NONE',  ( -15.80617190586745835, -15.72974639402198527, 111.8739096053143669 ) ) ;
#125296=CARTESIAN_POINT ( 'NONE',  ( 21.52544592524344225, -5.823673210054117533, 68.54057627198103830 ) ) ;
#125297=CARTESIAN_POINT ( 'NONE',  ( 21.53943276465977519, -0.05219959533907433946, 23.74890960531435269 ) ) ;
#125298=CARTESIAN_POINT ( 'NONE',  ( -14.29746914071037622, -8.314922557961029526, 59.16775706135234714 ) ) ;
#125299=CARTESIAN_POINT ( 'NONE',  ( -19.05341960407611168, -5.049401038298163336, 66.45724293864769550 ) ) ;
#125300=CARTESIAN_POINT ( 'NONE',  ( 18.62759615963255655, 10.81492255796105972, 41.66775706135235424 ) ) ;
#125301=CARTESIAN_POINT ( 'NONE',  ( -14.29746914071037622, -8.314922557961029526, 19.16775706135234714 ) ) ;
#125302=CARTESIAN_POINT ( 'NONE',  ( -19.02544592524342804, 5.153800228976336051, 111.0405762719810099 ) ) ;
#125303=CARTESIAN_POINT ( 'NONE',  ( 9.564922557961047289, -16.46253265017146816, 25.41775706135234003 ) ) ;
#125304=CARTESIAN_POINT ( 'NONE',  ( 4.379528057220092307, 16.55341960407617563, 42.29275706135235424 ) ) ;
#125305=CARTESIAN_POINT ( 'NONE',  ( -9.474510206698964154, 16.51473224551069663, 105.4155762719810383 ) ) ;
#125306=CARTESIAN_POINT ( 'NONE',  ( -21.52544592524343514, 5.823673210054127303, 106.0405762719810525 ) ) ;
#125307=CARTESIAN_POINT ( 'NONE',  ( -16.51473224551069308, -9.474510206698971260, 61.66557627198103120 ) ) ;
#125308=CARTESIAN_POINT ( 'NONE',  ( -17.26058549869089731, 6.457015423128606990, 23.62254162523932521 ) ) ;
#125309=CARTESIAN_POINT ( 'NONE',  ( 4.379528057220339221, -16.55341960407611168, 77.70724293864770971 ) ) ;
#125310=CARTESIAN_POINT ( 'NONE',  ( 10.81492255796078972, 18.62759615963270932, 24.58224293864768839 ) ) ;
#125311=CARTESIAN_POINT ( 'NONE',  ( -17.48853670773242897, 5.747243402303157112, 33.66671299749992130 ) ) ;
#125312=CARTESIAN_POINT ( 'NONE',  ( 21.52544592524344225, -5.823673210054117533, 98.54057627198105251 ) ) ;
#125313=CARTESIAN_POINT ( 'NONE',  ( -0.05219959533936034679, 19.03943276465977164, 57.50109039468566863 ) ) ;
#125314=CARTESIAN_POINT ( 'NONE',  ( 13.89961937509977652, -13.97604488694527269, 113.1239096053143527 ) ) ;
#125315=CARTESIAN_POINT ( 'NONE',  ( -19.05341960407611168, -5.049401038298163336, 26.45724293864769550 ) ) ;
#125316=CARTESIAN_POINT ( 'NONE',  ( -21.52544592524343514, 5.823673210054127303, 56.04057627198102409 ) ) ;
#125317=CARTESIAN_POINT ( 'NONE',  ( 16.46253265017160672, -9.564922557960803928, 103.3322429386476955 ) ) ;
#125318=CARTESIAN_POINT ( 'NONE',  ( -10.81492255796105439, 18.62759615963255655, 77.91775706135231871 ) ) ;
#125319=CARTESIAN_POINT ( 'NONE',  ( 19.02544592524343514, -5.153800228976328945, 53.54057627198102409 ) ) ;
#125320=CARTESIAN_POINT ( 'NONE',  ( 14.29746914071049879, -8.314922557960816363, 83.33224293864769550 ) ) ;
#125321=CARTESIAN_POINT ( 'NONE',  ( -4.379528057220086978, -16.55341960407618274, 29.79275706135234358 ) ) ;
#125322=CARTESIAN_POINT ( 'NONE',  ( 19.02544592524343514, -5.153800228976328945, 63.54057627198103830 ) ) ;
#125323=CARTESIAN_POINT ( 'NONE',  ( -15.72974639402176322, -15.80617190586768395, 64.37609039468568994 ) ) ;
#125325=CARTESIAN_POINT ( 'NONE',  ( 19.03943276465977164, 0.05219959533936151252, 31.25109039468566863 ) ) ;
#125326=CARTESIAN_POINT ( 'NONE',  ( 9.564922557961047289, -16.46253265017146816, 40.41775706135234003 ) ) ;
#125328=CARTESIAN_POINT ( 'NONE',  ( 21.55341960407619695, -5.719274019375665929, 41.04275706135236135 ) ) ;
#125330=CARTESIAN_POINT ( 'NONE',  ( 16.51473224551083163, -9.474510206698727899, 30.83442372801900433 ) ) ;
#125331=CARTESIAN_POINT ( 'NONE',  ( 19.05341960407611168, 5.049401038298154454, 68.95724293864769550 ) ) ;
#125332=CARTESIAN_POINT ( 'NONE',  ( 8.224510206698953496, -14.34966873604960469, 22.91557627198102765 ) ) ;
#125333=CARTESIAN_POINT ( 'NONE',  ( -5.153800228976328057, -19.02544592524343514, 112.2905762719810099 ) ) ;
#125334=CARTESIAN_POINT ( 'NONE',  ( -5.823673210054431948, 21.52544592524334988, 92.70942372801901854 ) ) ;
#125337=CARTESIAN_POINT ( 'NONE',  ( 21.55341960407619695, -5.719274019375665929, 81.04275706135236135 ) ) ;
#125339=CARTESIAN_POINT ( 'NONE',  ( 13.89961937509977652, -13.97604488694527269, 98.12390960531433848 ) ) ;
#125341=CARTESIAN_POINT ( 'NONE',  ( -9.564922557960796823, -16.46253265017161027, 52.08224293864768839 ) ) ;
#125342=CARTESIAN_POINT ( 'NONE',  ( -15.80617190586745835, -15.72974639402198527, 71.87390960531438111 ) ) ;
#125343=CARTESIAN_POINT ( 'NONE',  ( -4.379528057220328563, 16.55341960407611168, 30.20724293864769550 ) ) ;
#125344=CARTESIAN_POINT ( 'NONE',  ( -14.29746914071049879, 8.314922557960819915, 115.8322429386477097 ) ) ;
#125345=CARTESIAN_POINT ( 'NONE',  ( 16.46253265017160672, -9.564922557960803928, 88.33224293864769550 ) ) ;
#125346=CARTESIAN_POINT ( 'NONE',  ( 15.72974639402176855, 15.80617190586768217, 111.8760903946856615 ) ) ;
#125348=CARTESIAN_POINT ( 'NONE',  ( 16.53943276465976808, -0.05219959533910856209, 108.7489096053143669 ) ) ;
#125349=CARTESIAN_POINT ( 'NONE',  ( 10.81492255796106328, -18.62759615963255655, 70.41775706135236135 ) ) ;
#125350=CARTESIAN_POINT ( 'NONE',  ( -5.049401038298153566, 19.05341960407611168, 110.2072429386476671 ) ) ;
#125351=CARTESIAN_POINT ( 'NONE',  ( -4.483927247898782831, 16.52544592524335698, 102.7094237280190185 ) ) ;
#125352=CARTESIAN_POINT ( 'NONE',  ( -5.153800228976607833, 19.02544592524334988, 62.70942372801899722 ) ) ;
#125354=CARTESIAN_POINT ( 'NONE',  ( 13.89961937509977652, -13.97604488694527269, 103.1239096053143527 ) ) ;
#125355=CARTESIAN_POINT ( 'NONE',  ( 16.53943276465976808, -0.05219959533910856209, 73.74890960531433848 ) ) ;
#125356=CARTESIAN_POINT ( 'NONE',  ( -9.564922557961040184, 16.46253265017147172, 57.91775706135233293 ) ) ;
#125357=CARTESIAN_POINT ( 'NONE',  ( -19.03943276465977164, 0.05219959533909376836, 61.24890960531436690 ) ) ;
#125358=CARTESIAN_POINT ( 'NONE',  ( -8.314922557960811034, -14.29746914071050412, 62.08224293864769550 ) ) ;
#125359=CARTESIAN_POINT ( 'NONE',  ( 16.51473224551083163, -9.474510206698727899, 95.83442372801900433 ) ) ;
#125360=CARTESIAN_POINT ( 'NONE',  ( -10.72451020669898014, 18.67979575497178502, 45.41557627198103830 ) ) ;
#125362=EDGE_CURVE ( 'NONE', #134824, #163522, #2974, .T. ) ;
#125363=CARTESIAN_POINT ( 'NONE',  ( 14.34966873604960469, 8.224510206698951720, 109.1655762719810383 ) ) ;
#125364=CARTESIAN_POINT ( 'NONE',  ( -17.44270441346514033, -5.991230190323105553, 31.36335079264230430 ) ) ;
#125365=CARTESIAN_POINT ( 'NONE',  ( 19.02544592524343514, -5.153800228976328945, 73.54057627198103830 ) ) ;
#125366=CARTESIAN_POINT ( 'NONE',  ( 21.53943276465977519, -0.05219959533907433946, 68.74890960531435269 ) ) ;
#125367=CARTESIAN_POINT ( 'NONE',  ( 14.29746914071037800, 8.314922557961029526, 91.66775706135234714 ) ) ;
#125368=CARTESIAN_POINT ( 'NONE',  ( -16.51473224551069308, -9.474510206698971260, 71.66557627198102409 ) ) ;
#125369=CARTESIAN_POINT ( 'NONE',  ( -13.89961937509957401, -13.97604488694547875, 59.37609039468566863 ) ) ;
#125370=CARTESIAN_POINT ( 'NONE',  ( -21.55341960407619339, 5.719274019375674811, 78.54275706135236135 ) ) ;
#125371=CARTESIAN_POINT ( 'NONE',  ( -15.72974639402197994, 15.80617190586746368, 65.62390960531436690 ) ) ;
#125372=CARTESIAN_POINT ( 'NONE',  ( 9.474510206698971260, -16.51473224551069308, 107.9155762719810383 ) ) ;
#125373=CARTESIAN_POINT ( 'NONE',  ( 0.05219959533909260263, 19.03943276465977164, 34.99890960531435979 ) ) ;
#125374=CARTESIAN_POINT ( 'NONE',  ( 4.483927247898790824, -16.52544592524335698, 100.2094237280190043 ) ) ;
#125375=CARTESIAN_POINT ( 'NONE',  ( 16.55341960407618274, -4.379528057220086978, 21.04275706135234714 ) ) ;
#125376=CARTESIAN_POINT ( 'NONE',  ( 19.34837522270368382, 5.499999999999744205, 78.36337684832574269 ) ) ;
#125377=CARTESIAN_POINT ( 'NONE',  ( 15.80617190586769283, -15.72974639402175789, 95.62609039468568994 ) ) ;
#125378=CARTESIAN_POINT ( 'NONE',  ( 8.314922557960818139, 14.29746914071049879, 64.58224293864769550 ) ) ;
#125379=CARTESIAN_POINT ( 'NONE',  ( 8.224510206698953496, -14.34966873604960469, 72.91557627198103830 ) ) ;
#125380=CARTESIAN_POINT ( 'NONE',  ( 10.81492255796078972, 18.62759615963270932, 89.58224293864768129 ) ) ;
#125381=CARTESIAN_POINT ( 'NONE',  ( -5.823673210054116645, -21.52544592524344225, 87.29057627198103830 ) ) ;
#125383=CARTESIAN_POINT ( 'NONE',  ( 10.72451020669898902, -18.67979575497178502, 47.91557627198102409 ) ) ;
#125384=CARTESIAN_POINT ( 'NONE',  ( -16.55341960407617563, 4.379528057220093196, 73.54275706135234714 ) ) ;
#125385=CARTESIAN_POINT ( 'NONE',  ( 4.379528057220339221, -16.55341960407611168, 87.70724293864769550 ) ) ;
#125386=CARTESIAN_POINT ( 'NONE',  ( 5.049401038298161559, -19.05341960407611168, 42.70724293864767418 ) ) ;
#125388=CARTESIAN_POINT ( 'NONE',  ( 8.224510206698742110, 14.34966873604972548, 102.0844237280190185 ) ) ;
#125389=CARTESIAN_POINT ( 'NONE',  ( -10.81492255796105439, 18.62759615963255655, 32.91775706135234714 ) ) ;
#125390=CARTESIAN_POINT ( 'NONE',  ( -13.97604488694527625, -13.89961937509977652, 96.87390960531433848 ) ) ;
#125391=CARTESIAN_POINT ( 'NONE',  ( -15.72974639402176322, -15.80617190586768395, 64.37609039468568994 ) ) ;
#125393=CARTESIAN_POINT ( 'NONE',  ( 19.03943276465977164, -0.05219959533909143690, 23.74890960531435269 ) ) ;
#125395=CARTESIAN_POINT ( 'NONE',  ( 5.823673210054444382, -21.52544592524334988, 65.20942372801901854 ) ) ;
#125396=CARTESIAN_POINT ( 'NONE',  ( -13.89961937509977652, 13.97604488694528158, 45.62390960531433848 ) ) ;
#125397=CARTESIAN_POINT ( 'NONE',  ( 13.97604488694527802, 13.89961937509977652, 24.37390960531435624 ) ) ;
#125398=CARTESIAN_POINT ( 'NONE',  ( 19.05341960407611168, 5.049401038298154454, 93.95724293864769550 ) ) ;
#125399=CARTESIAN_POINT ( 'NONE',  ( 19.03943276465977164, 0.05219959533936151252, 61.25109039468566863 ) ) ;
#125400=CARTESIAN_POINT ( 'NONE',  ( 5.719274019375673035, 21.55341960407619339, 42.29275706135235424 ) ) ;
#125401=CARTESIAN_POINT ( 'NONE',  ( 19.03943276465977164, 0.05219959533936151252, 56.25109039468566863 ) ) ;
#125402=CARTESIAN_POINT ( 'NONE',  ( 9.564922557960805705, 16.46253265017160317, 44.58224293864769550 ) ) ;
#125403=CARTESIAN_POINT ( 'NONE',  ( 4.483927247898790824, -16.52544592524335698, 110.2094237280190185 ) ) ;
#125404=CARTESIAN_POINT ( 'NONE',  ( 16.46253265017146816, 9.564922557961045513, 81.66775706135233293 ) ) ;
#125405=CARTESIAN_POINT ( 'NONE',  ( -16.52544592524342804, 4.483927247898546575, 26.04057627198103475 ) ) ;
#125406=CARTESIAN_POINT ( 'NONE',  ( 5.049401038297881783, 19.05341960407617563, 52.29275706135234003 ) ) ;
#125407=CARTESIAN_POINT ( 'NONE',  ( 19.03943276465977164, -0.05219959533909143690, 103.7489096053143669 ) ) ;
#125408=CARTESIAN_POINT ( 'NONE',  ( -15.80617190586768217, 15.72974639402176855, 103.1260903946856757 ) ) ;
#125409=CARTESIAN_POINT ( 'NONE',  ( -13.97604488694547697, 13.89961937509957934, 23.12609039468565442 ) ) ;
#125410=CARTESIAN_POINT ( 'NONE',  ( 9.474510206698971260, -16.51473224551069308, 32.91557627198102409 ) ) ;
#125411=CARTESIAN_POINT ( 'NONE',  ( -18.62759615963255300, -10.81492255796106328, 84.16775706135234714 ) ) ;
#125412=CARTESIAN_POINT ( 'NONE',  ( -8.224510206698735004, -14.34966873604973081, 29.58442372801901854 ) ) ;
#125413=CARTESIAN_POINT ( 'NONE',  ( 16.51473224551069308, 9.474510206698969483, 94.16557627198103830 ) ) ;
#125415=CARTESIAN_POINT ( 'NONE',  ( 13.89961937509977652, -13.97604488694527269, 73.12390960531436690 ) ) ;
#125417=CARTESIAN_POINT ( 'NONE',  ( 5.049401038297881783, 19.05341960407617563, 87.29275706135234714 ) ) ;
#125418=CARTESIAN_POINT ( 'NONE',  ( -5.153800228976328057, -19.02544592524343514, 102.2905762719810383 ) ) ;
#125419=CARTESIAN_POINT ( 'NONE',  ( 21.55341960407619695, -5.719274019375665929, 106.0427570613523471 ) ) ;
#125420=CARTESIAN_POINT ( 'NONE',  ( 8.314922557960818139, 14.29746914071049879, 104.5822429386477097 ) ) ;
#125422=CARTESIAN_POINT ( 'NONE',  ( 10.81492255796078972, 18.62759615963270932, 49.58224293864769550 ) ) ;
#125423=CARTESIAN_POINT ( 'NONE',  ( -21.55341960407610458, -5.719274019375992779, 41.45724293864769550 ) ) ;
#125424=CARTESIAN_POINT ( 'NONE',  ( -12.06949235617756955, 12.14591786802309770, 110.6239096053143669 ) ) ;
#125426=CARTESIAN_POINT ( 'NONE',  ( 19.03943276465977164, 0.05219959533936151252, 61.25109039468566863 ) ) ;
#125427=CARTESIAN_POINT ( 'NONE',  ( -0.05219959533910754901, -16.53943276465976808, 37.49890960531436690 ) ) ;
#125428=CARTESIAN_POINT ( 'NONE',  ( -5.049401038298153566, 19.05341960407611168, 115.2072429386477097 ) ) ;
#125429=CARTESIAN_POINT ( 'NONE',  ( -21.52544592524334988, -5.823673210054445271, 83.95942372801900433 ) ) ;
#125430=CARTESIAN_POINT ( 'NONE',  ( 5.823673210054125526, 21.52544592524343514, 69.79057627198102409 ) ) ;
#125431=CARTESIAN_POINT ( 'NONE',  ( -21.55341960407619339, 5.719274019375674811, 43.54275706135235424 ) ) ;
#125432=CARTESIAN_POINT ( 'NONE',  ( -10.81492255796078084, -18.62759615963271287, 92.08224293864769550 ) ) ;
#125433=CARTESIAN_POINT ( 'NONE',  ( 21.52544592524334988, 5.823673210054432836, 51.45942372801901854 ) ) ;
#125434=CARTESIAN_POINT ( 'NONE',  ( 19.05341960407611168, 5.049401038298154454, 23.95724293864769194 ) ) ;
#125435=CARTESIAN_POINT ( 'NONE',  ( 19.03943276465977164, -0.05219959533909143690, 83.74890960531436690 ) ) ;
#125436=CARTESIAN_POINT ( 'NONE',  ( 16.55341960407618274, -4.379528057220086978, 76.04275706135237556 ) ) ;
#125437=CARTESIAN_POINT ( 'NONE',  ( 16.55341960407611168, 4.379528057220329451, 103.9572429386476813 ) ) ;
#125438=CARTESIAN_POINT ( 'NONE',  ( -5.153800228976328057, -19.02544592524343514, 107.2905762719810383 ) ) ;
#125439=CARTESIAN_POINT ( 'NONE',  ( 12.06949235617757843, -12.14591786802309237, 53.12390960531436690 ) ) ;
#125440=CARTESIAN_POINT ( 'NONE',  ( 8.314922557960818139, 14.29746914071049879, 24.58224293864768839 ) ) ;
#125441=CARTESIAN_POINT ( 'NONE',  ( -9.564922557960796823, -16.46253265017161027, 67.08224293864769550 ) ) ;
#125442=CARTESIAN_POINT ( 'NONE',  ( -9.474510206698964154, 16.51473224551069663, 35.41557627198102409 ) ) ;
#125443=CARTESIAN_POINT ( 'NONE',  ( 10.81492255796078972, 18.62759615963270932, 44.58224293864769550 ) ) ;
#125444=CARTESIAN_POINT ( 'NONE',  ( -16.46253265017146816, -9.564922557961047289, 34.16775706135233293 ) ) ;
#125446=CARTESIAN_POINT ( 'NONE',  ( -14.34966873604960291, -8.224510206698953496, 31.66557627198102054 ) ) ;
#125447=CARTESIAN_POINT ( 'NONE',  ( 19.02544592524343514, -5.153800228976328945, 113.5405762719810241 ) ) ;
#125448=CARTESIAN_POINT ( 'NONE',  ( 10.72451020669871369, 18.67979575497193778, 62.08442372801901143 ) ) ;
#125449=CARTESIAN_POINT ( 'NONE',  ( 5.153800228976335163, 19.02544592524342804, 114.7905762719810241 ) ) ;
#125450=CARTESIAN_POINT ( 'NONE',  ( 12.06949235617739724, 12.14591786802326823, 61.87609039468568284 ) ) ;
#125451=CARTESIAN_POINT ( 'NONE',  ( 19.03943276465977164, 0.05219959533936151252, 56.25109039468566863 ) ) ;
#125452=CARTESIAN_POINT ( 'NONE',  ( -12.14591786802309592, -12.06949235617757132, 41.87390960531435979 ) ) ;
#125453=CARTESIAN_POINT ( 'NONE',  ( -18.87255363501902394, -5.500000000000063949, 76.32513748171827217 ) ) ;
#125454=CARTESIAN_POINT ( 'NONE',  ( 16.53943276465976808, 0.05219959533934440121, 101.2510903946856757 ) ) ;
#125455=CARTESIAN_POINT ( 'NONE',  ( 19.03943276465977164, -0.05219959533909143690, 38.74890960531436690 ) ) ;
#125456=CARTESIAN_POINT ( 'NONE',  ( -0.05219959533909027116, -19.03943276465977164, 67.49890960531436690 ) ) ;
#125457=CARTESIAN_POINT ( 'NONE',  ( 19.05341960407611168, 5.049401038298154454, 28.95724293864769550 ) ) ;
#125458=CARTESIAN_POINT ( 'NONE',  ( 5.719274019375673035, 21.55341960407619339, 37.29275706135235424 ) ) ;
#125459=CARTESIAN_POINT ( 'NONE',  ( -13.89961937509977652, 13.97604488694528158, 60.62390960531436690 ) ) ;
#125461=CARTESIAN_POINT ( 'NONE',  ( 16.51473224551069308, 9.474510206698969483, 49.16557627198102409 ) ) ;
#125462=EDGE_CURVE ( 'NONE', #168063, #127046, #38490, .T. ) ;
#125463=CARTESIAN_POINT ( 'NONE',  ( 21.53943276465977519, -0.05219959533907433946, 23.74890960531435269 ) ) ;
#125464=CARTESIAN_POINT ( 'NONE',  ( 5.719274019375673035, 21.55341960407619339, 62.29275706135236845 ) ) ;
#125465=CARTESIAN_POINT ( 'NONE',  ( 16.51473224551069308, 9.474510206698969483, 29.16557627198103475 ) ) ;
#125466=CARTESIAN_POINT ( 'NONE',  ( -0.05219959533907301413, -21.53943276465977519, 27.49890960531435269 ) ) ;
#125467=CARTESIAN_POINT ( 'NONE',  ( -14.29746914071037622, -8.314922557961029526, 79.16775706135234714 ) ) ;
#125468=CARTESIAN_POINT ( 'NONE',  ( -21.55341960407619339, 5.719274019375674811, 108.5427570613523756 ) ) ;
#125469=CARTESIAN_POINT ( 'NONE',  ( 16.53943276465976808, 0.05219959533934440121, 51.25109039468568994 ) ) ;
#125470=CARTESIAN_POINT ( 'NONE',  ( 13.89961937509977652, -13.97604488694527269, 93.12390960531436690 ) ) ;
#125472=CARTESIAN_POINT ( 'NONE',  ( -8.314922557961024197, 14.29746914071037800, 47.91775706135234714 ) ) ;
#125473=CARTESIAN_POINT ( 'NONE',  ( -16.55341960407617563, 4.379528057220093196, 23.54275706135235424 ) ) ;
#125474=CARTESIAN_POINT ( 'NONE',  ( -8.224510206698735004, -14.34966873604973081, 94.58442372801901854 ) ) ;
#125475=CARTESIAN_POINT ( 'NONE',  ( 0.05219959533937995610, -21.53943276465977519, 55.00109039468568284 ) ) ;
#125476=CARTESIAN_POINT ( 'NONE',  ( -19.05341960407617563, 5.049401038297882671, 103.5427570613523329 ) ) ;
#125477=CARTESIAN_POINT ( 'NONE',  ( -18.67979575497178146, -10.72451020669898902, 106.6655762719810383 ) ) ;
#125478=CARTESIAN_POINT ( 'NONE',  ( 16.52544592524342804, -4.483927247898539470, 98.54057627198105251 ) ) ;
#125479=CARTESIAN_POINT ( 'NONE',  ( 9.474510206698729675, 16.51473224551082808, 102.0844237280190043 ) ) ;
#125480=CARTESIAN_POINT ( 'NONE',  ( 12.06949235617739724, 12.14591786802326823, 86.87609039468568994 ) ) ;
#125482=CARTESIAN_POINT ( 'NONE',  ( -13.97604488694547697, 13.89961937509957934, 78.12609039468567573 ) ) ;
#125483=CARTESIAN_POINT ( 'NONE',  ( 8.224510206698953496, -14.34966873604960469, 47.91557627198102409 ) ) ;
#125484=CARTESIAN_POINT ( 'NONE',  ( -12.14591786802309592, -12.06949235617757132, 46.87390960531435979 ) ) ;
#125485=CARTESIAN_POINT ( 'NONE',  ( 4.379528057220339221, -16.55341960407611168, 107.7072429386476955 ) ) ;
#125486=CARTESIAN_POINT ( 'NONE',  ( -19.05341960407617563, 5.049401038297882671, 48.54275706135233293 ) ) ;
#125487=CARTESIAN_POINT ( 'NONE',  ( 18.62759615963255655, 10.81492255796105972, 31.66775706135234358 ) ) ;
#125488=CARTESIAN_POINT ( 'NONE',  ( 19.03943276465977164, 0.05219959533936151252, 106.2510903946856615 ) ) ;
#125490=CARTESIAN_POINT ( 'NONE',  ( 13.89961937509977652, -13.97604488694527269, 108.1239096053143669 ) ) ;
#125491=CARTESIAN_POINT ( 'NONE',  ( 13.97604488694527802, 13.89961937509977652, 94.37390960531436690 ) ) ;
#125492=CARTESIAN_POINT ( 'NONE',  ( 10.72451020669898902, -18.67979575497178502, 52.91557627198103830 ) ) ;
#125493=CARTESIAN_POINT ( 'NONE',  ( 12.06949235617757843, -12.14591786802309237, 108.1239096053143811 ) ) ;
#125494=CARTESIAN_POINT ( 'NONE',  ( 16.51473224551069308, 9.474510206698969483, 74.16557627198103830 ) ) ;
#125495=CARTESIAN_POINT ( 'NONE',  ( 5.153800228976335163, 19.02544592524342804, 34.79057627198102409 ) ) ;
#125496=CARTESIAN_POINT ( 'NONE',  ( 18.67979575497194134, -10.72451020669871369, 35.83442372801901143 ) ) ;
#125497=CARTESIAN_POINT ( 'NONE',  ( 5.823673210054444382, -21.52544592524334988, 75.20942372801901854 ) ) ;
#125498=CARTESIAN_POINT ( 'NONE',  ( -8.314922557961024197, 14.29746914071037800, 92.91775706135236135 ) ) ;
#125499=CARTESIAN_POINT ( 'NONE',  ( 10.72451020669871369, 18.67979575497193778, 27.08442372801901854 ) ) ;
#125500=CARTESIAN_POINT ( 'NONE',  ( 18.67979575497194134, -10.72451020669871369, 25.83442372801901499 ) ) ;
#125501=CARTESIAN_POINT ( 'NONE',  ( -13.97604488694547697, 13.89961937509957934, 68.12609039468563310 ) ) ;
#125502=CARTESIAN_POINT ( 'NONE',  ( 19.03943276465977164, -0.05219959533909143690, 73.74890960531435269 ) ) ;
#125503=CARTESIAN_POINT ( 'NONE',  ( 18.67979575497194134, -10.72451020669871369, 85.83442372801901854 ) ) ;
#125505=CARTESIAN_POINT ( 'NONE',  ( 18.67979575497178502, 10.72451020669898547, 89.16557627198102409 ) ) ;
#125506=CARTESIAN_POINT ( 'NONE',  ( 4.483927247898545687, 16.52544592524342804, 64.79057627198103830 ) ) ;
#125507=CARTESIAN_POINT ( 'NONE',  ( -15.80617190586768217, 15.72974639402176855, 98.12609039468570415 ) ) ;
#125508=CARTESIAN_POINT ( 'NONE',  ( -4.379528057220328563, 16.55341960407611168, 80.20724293864769550 ) ) ;
#125509=CARTESIAN_POINT ( 'NONE',  ( 9.474510206698971260, -16.51473224551069308, 22.91557627198102765 ) ) ;
#125510=CARTESIAN_POINT ( 'NONE',  ( -16.46253265017146816, -9.564922557961047289, 69.16775706135233293 ) ) ;
#125511=CARTESIAN_POINT ( 'NONE',  ( -4.379528057220328563, 16.55341960407611168, 30.20724293864769550 ) ) ;
#125512=CARTESIAN_POINT ( 'NONE',  ( -18.62759615963255300, -10.81492255796106328, 79.16775706135234714 ) ) ;
#125513=CARTESIAN_POINT ( 'NONE',  ( 5.153800228976335163, 19.02544592524342804, 94.79057627198103830 ) ) ;
#125514=CARTESIAN_POINT ( 'NONE',  ( -16.51473224551082808, 9.474510206698731452, 58.33442372801900433 ) ) ;
#125515=CARTESIAN_POINT ( 'NONE',  ( -0.05219959533907301413, -21.53943276465977519, 67.49890960531436690 ) ) ;
#125516=CARTESIAN_POINT ( 'NONE',  ( 10.72451020669871369, 18.67979575497193778, 22.08442372801901143 ) ) ;
#125517=CARTESIAN_POINT ( 'NONE',  ( -4.483927247898782831, 16.52544592524335698, 22.70942372801901499 ) ) ;
#125518=CARTESIAN_POINT ( 'NONE',  ( -16.53943276465976808, -0.05219959533934237506, 83.75109039468568994 ) ) ;
#125519=CARTESIAN_POINT ( 'NONE',  ( -22.00000000000000000, -1.132798289211302014E-14, 92.50000000000000000 ) ) ;
#125520=CARTESIAN_POINT ( 'NONE',  ( 5.719274019375673035, 21.55341960407619339, 22.29275706135235069 ) ) ;
#125521=CARTESIAN_POINT ( 'NONE',  ( 16.52544592524342804, -4.483927247898539470, 103.5405762719810383 ) ) ;
#125523=CARTESIAN_POINT ( 'NONE',  ( 16.52544592524335698, 4.483927247898782831, 31.45942372801901854 ) ) ;
#125524=CARTESIAN_POINT ( 'NONE',  ( 21.53943276465977519, -0.05219959533907433946, 68.74890960531435269 ) ) ;
#125525=CARTESIAN_POINT ( 'NONE',  ( -14.34966873604972548, 8.224510206698743886, 108.3344237280190185 ) ) ;
#125526=CARTESIAN_POINT ( 'NONE',  ( -14.29746914071037622, -8.314922557961029526, 39.16775706135235424 ) ) ;
#125527=CARTESIAN_POINT ( 'NONE',  ( 13.97604488694527802, 13.89961937509977652, 29.37390960531435979 ) ) ;
#125528=CARTESIAN_POINT ( 'NONE',  ( -0.05219959533934338120, 16.53943276465976808, 77.50109039468567573 ) ) ;
#125529=CARTESIAN_POINT ( 'NONE',  ( 5.049401038297881783, 19.05341960407617563, 72.29275706135234714 ) ) ;
#125530=CARTESIAN_POINT ( 'NONE',  ( 5.719274019375991003, -21.55341960407610458, 72.70724293864769550 ) ) ;
#125531=CARTESIAN_POINT ( 'NONE',  ( -4.483927247898782831, 16.52544592524335698, 97.70942372801904696 ) ) ;
#125532=CARTESIAN_POINT ( 'NONE',  ( -18.67979575497193778, 10.72451020669871902, 78.33442372801901854 ) ) ;
#125533=CARTESIAN_POINT ( 'NONE',  ( 10.72451020669898902, -18.67979575497178502, 57.91557627198103120 ) ) ;
#125534=CARTESIAN_POINT ( 'NONE',  ( 10.81492255796078972, 18.62759615963270932, 49.58224293864769550 ) ) ;
#125537=CARTESIAN_POINT ( 'NONE',  ( -8.314922557961024197, 14.29746914071037800, 72.91775706135234714 ) ) ;
#125538=CARTESIAN_POINT ( 'NONE',  ( -15.80617190586745835, -15.72974639402198527, 41.87390960531435979 ) ) ;
#125540=CARTESIAN_POINT ( 'NONE',  ( -16.46253265017160317, 9.564922557960807481, 95.83224293864769550 ) ) ;
#125542=CARTESIAN_POINT ( 'NONE',  ( -0.05219959533909027116, -19.03943276465977164, 22.49890960531436690 ) ) ;
#125543=CARTESIAN_POINT ( 'NONE',  ( -21.52544592524343514, 5.823673210054127303, 61.04057627198103120 ) ) ;
#125544=CARTESIAN_POINT ( 'NONE',  ( -14.34966873604972548, 8.224510206698743886, 98.33442372801901854 ) ) ;
#125545=CARTESIAN_POINT ( 'NONE',  ( 0.05219959533937995610, -21.53943276465977519, 40.00109039468567573 ) ) ;
#125546=CARTESIAN_POINT ( 'NONE',  ( -0.05219959533936034679, 19.03943276465977164, 102.5010903946856757 ) ) ;
#125547=CARTESIAN_POINT ( 'NONE',  ( 8.314922557960818139, 14.29746914071049879, 109.5822429386476955 ) ) ;
#125548=CARTESIAN_POINT ( 'NONE',  ( 9.474510206698729675, 16.51473224551082808, 112.0844237280190043 ) ) ;
#125549=CARTESIAN_POINT ( 'NONE',  ( -19.03943276465977164, 0.05219959533909376836, 46.24890960531435979 ) ) ;
#125551=CARTESIAN_POINT ( 'NONE',  ( -19.03943276465977164, 0.05219959533909376836, 86.24890960531436690 ) ) ;
#125552=CARTESIAN_POINT ( 'NONE',  ( 4.483927247898790824, -16.52544592524335698, 70.20942372801904696 ) ) ;
#125553=CARTESIAN_POINT ( 'NONE',  ( -19.02544592524334988, -5.153800228976617603, 78.95942372801900433 ) ) ;
#125554=CARTESIAN_POINT ( 'NONE',  ( -9.474510206698720793, -16.51473224551083518, 19.58442372801899722 ) ) ;
#125555=CARTESIAN_POINT ( 'NONE',  ( 10.72451020669898902, -18.67979575497178502, 67.91557627198102409 ) ) ;
#125556=CARTESIAN_POINT ( 'NONE',  ( 8.314922557961029526, -14.29746914071037800, 90.41775706135236135 ) ) ;
#125557=CARTESIAN_POINT ( 'NONE',  ( 9.564922557961047289, -16.46253265017146816, 85.41775706135233293 ) ) ;
#125558=CARTESIAN_POINT ( 'NONE',  ( -19.05341960407611168, -5.049401038298163336, 31.45724293864769550 ) ) ;
#125559=CARTESIAN_POINT ( 'NONE',  ( 19.03943276465977164, -0.05219959533909143690, 83.74890960531436690 ) ) ;
#125560=CARTESIAN_POINT ( 'NONE',  ( 21.52544592524334988, 5.823673210054432836, 51.45942372801901854 ) ) ;
#125561=CARTESIAN_POINT ( 'NONE',  ( 13.97604488694527802, 13.89961937509977652, 44.37390960531435269 ) ) ;
#125562=CARTESIAN_POINT ( 'NONE',  ( 16.51473224551083163, -9.474510206698727899, 75.83442372801900433 ) ) ;
#125564=CARTESIAN_POINT ( 'NONE',  ( -19.02544592524342804, 5.153800228976336051, 111.0405762719810099 ) ) ;
#125565=CARTESIAN_POINT ( 'NONE',  ( -8.314922557960811034, -14.29746914071050412, 67.08224293864770971 ) ) ;
#125566=CARTESIAN_POINT ( 'NONE',  ( 5.719274019375991003, -21.55341960407610458, 57.70724293864770260 ) ) ;
#125568=CARTESIAN_POINT ( 'NONE',  ( 9.474510206698729675, 16.51473224551082808, 27.08442372801900433 ) ) ;
#125569=CARTESIAN_POINT ( 'NONE',  ( -19.05341960407611168, -5.049401038298163336, 66.45724293864769550 ) ) ;
#125570=CARTESIAN_POINT ( 'NONE',  ( 5.049401038298161559, -19.05341960407611168, 72.70724293864768129 ) ) ;
#125571=CARTESIAN_POINT ( 'NONE',  ( -16.55341960407617563, 4.379528057220093196, 53.54275706135234714 ) ) ;
#125574=CARTESIAN_POINT ( 'NONE',  ( -8.224510206698735004, -14.34966873604973081, 94.58442372801901854 ) ) ;
#125576=CARTESIAN_POINT ( 'NONE',  ( -16.53943276465976808, -0.05219959533934237506, 63.75109039468568284 ) ) ;
#125577=CARTESIAN_POINT ( 'NONE',  ( 16.53943276465976808, 0.05219959533934440121, 46.25109039468567573 ) ) ;
#125578=CARTESIAN_POINT ( 'NONE',  ( -9.564922557960796823, -16.46253265017161027, 57.08224293864769550 ) ) ;
#125580=CARTESIAN_POINT ( 'NONE',  ( -15.72974639402176322, -15.80617190586768395, 49.37609039468569705 ) ) ;
#125581=CARTESIAN_POINT ( 'NONE',  ( -19.05341960407617563, 5.049401038297882671, 68.54275706135230450 ) ) ;
#125582=CARTESIAN_POINT ( 'NONE',  ( -0.05219959533937732626, 21.53943276465977519, 102.5010903946856899 ) ) ;
#125583=CARTESIAN_POINT ( 'NONE',  ( 13.89961937509977652, -13.97604488694527269, 33.12390960531434558 ) ) ;
#125585=CARTESIAN_POINT ( 'NONE',  ( 21.53943276465977519, -0.05219959533907433946, 53.74890960531437401 ) ) ;
#125586=CARTESIAN_POINT ( 'NONE',  ( -10.81492255796078084, -18.62759615963271287, 27.08224293864769550 ) ) ;
#125587=CARTESIAN_POINT ( 'NONE',  ( 16.55341960407611168, 4.379528057220329451, 103.9572429386476813 ) ) ;
#125588=CARTESIAN_POINT ( 'NONE',  ( -8.224510206698735004, -14.34966873604973081, 39.58442372801901143 ) ) ;
#125589=CARTESIAN_POINT ( 'NONE',  ( 14.29746914071049879, -8.314922557960816363, 33.33224293864769550 ) ) ;
#125591=CARTESIAN_POINT ( 'NONE',  ( 5.719274019375673035, 21.55341960407619339, 22.29275706135235069 ) ) ;
#125592=CARTESIAN_POINT ( 'NONE',  ( -16.52544592524342804, 4.483927247898546575, 41.04057627198103120 ) ) ;
#125594=CARTESIAN_POINT ( 'NONE',  ( -19.05341960407617563, 5.049401038297882671, 98.54275706135233293 ) ) ;
#125595=CARTESIAN_POINT ( 'NONE',  ( 16.46253265017146816, 9.564922557961045513, 26.66775706135234003 ) ) ;
#125596=CARTESIAN_POINT ( 'NONE',  ( 8.314922557960818139, 14.29746914071049879, 34.58224293864770260 ) ) ;
#125597=CARTESIAN_POINT ( 'NONE',  ( 10.81492255796078972, 18.62759615963270932, 104.5822429386477097 ) ) ;
#125598=CARTESIAN_POINT ( 'NONE',  ( -21.52544592524343514, 5.823673210054127303, 66.04057627198103830 ) ) ;
#125599=CARTESIAN_POINT ( 'NONE',  ( -19.02544592524342804, 5.153800228976336051, 81.04057627198103830 ) ) ;
#125600=CARTESIAN_POINT ( 'NONE',  ( -8.314922557960811034, -14.29746914071050412, 42.08224293864769550 ) ) ;
#125601=CARTESIAN_POINT ( 'NONE',  ( -0.05219959533909027116, -19.03943276465977164, 87.49890960531436690 ) ) ;
#125603=CARTESIAN_POINT ( 'NONE',  ( 19.02544592524334988, 5.153800228976608722, 36.45942372801900433 ) ) ;
#125604=CARTESIAN_POINT ( 'NONE',  ( 21.53943276465977519, -0.05219959533907433946, 88.74890960531436690 ) ) ;
#125605=CARTESIAN_POINT ( 'NONE',  ( -14.29746914071049879, 8.314922557960819915, 100.8322429386477097 ) ) ;
#125606=CARTESIAN_POINT ( 'NONE',  ( -0.05219959533937732626, 21.53943276465977519, 32.50109039468568284 ) ) ;
#125608=CARTESIAN_POINT ( 'NONE',  ( -12.06949235617756955, 12.14591786802309770, 25.62390960531435624 ) ) ;
#125609=CARTESIAN_POINT ( 'NONE',  ( 16.46253265017160672, -9.564922557960803928, 38.33224293864768839 ) ) ;
#125610=CARTESIAN_POINT ( 'NONE',  ( -5.153800228976328057, -19.02544592524343514, 87.29057627198103830 ) ) ;
#125611=CARTESIAN_POINT ( 'NONE',  ( -15.80617190586745835, -15.72974639402198527, 66.87390960531436690 ) ) ;
#125612=CARTESIAN_POINT ( 'NONE',  ( -18.22780087662122028, 5.500000000000031086, 43.51540105326107977 ) ) ;
#125613=CARTESIAN_POINT ( 'NONE',  ( 0.05219959533909260263, 19.03943276465977164, 24.99890960531435269 ) ) ;
#125614=CARTESIAN_POINT ( 'NONE',  ( -14.34966873604960291, -8.224510206698953496, 41.66557627198103120 ) ) ;
#125615=EDGE_CURVE ( 'NONE', #199942, #88260, #15199, .T. ) ;
#125616=CARTESIAN_POINT ( 'NONE',  ( -15.80617190586768217, 15.72974639402176855, 68.12609039468567573 ) ) ;
#125618=CARTESIAN_POINT ( 'NONE',  ( -16.55341960407617563, 4.379528057220093196, 63.54275706135234003 ) ) ;
#125619=CARTESIAN_POINT ( 'NONE',  ( -13.89961937509977652, 13.97604488694528158, 60.62390960531436690 ) ) ;
#125620=CARTESIAN_POINT ( 'NONE',  ( 5.153800228976335163, 19.02544592524342804, 69.79057627198103830 ) ) ;
#125622=CARTESIAN_POINT ( 'NONE',  ( -10.72451020669870658, -18.67979575497194134, 109.5844237280190328 ) ) ;
#125623=CARTESIAN_POINT ( 'NONE',  ( 0.05219959533934541429, -16.53943276465976808, 75.00109039468568994 ) ) ;
#125624=CARTESIAN_POINT ( 'NONE',  ( 21.55341960407619695, -5.719274019375665929, 101.0427570613523756 ) ) ;
#125625=CARTESIAN_POINT ( 'NONE',  ( 19.05341960407611168, 5.049401038298154454, 58.95724293864768129 ) ) ;
#125626=CARTESIAN_POINT ( 'NONE',  ( 18.62759615963271287, -10.81492255796078972, 33.33224293864769550 ) ) ;
#125627=CARTESIAN_POINT ( 'NONE',  ( 9.474510206698729675, 16.51473224551082808, 102.0844237280190043 ) ) ;
#125628=CARTESIAN_POINT ( 'NONE',  ( -15.72974639402176322, -15.80617190586768395, 79.37609039468567573 ) ) ;
#125629=CARTESIAN_POINT ( 'NONE',  ( 0.05219959533934541429, -16.53943276465976808, 55.00109039468568284 ) ) ;
#125630=CARTESIAN_POINT ( 'NONE',  ( 18.67979575497178502, 10.72451020669898547, 99.16557627198100988 ) ) ;
#125631=CARTESIAN_POINT ( 'NONE',  ( 9.564922557961047289, -16.46253265017146816, 100.4177570613523329 ) ) ;
#125632=CARTESIAN_POINT ( 'NONE',  ( 16.51473224551069308, 9.474510206698969483, 79.16557627198103830 ) ) ;
#125633=EDGE_CURVE ( 'NONE', #44638, #99775, #196083, .T. ) ;
#125634=CARTESIAN_POINT ( 'NONE',  ( 13.89961937509957401, 13.97604488694547697, 106.8760903946856757 ) ) ;
#125635=CARTESIAN_POINT ( 'NONE',  ( -0.05219959533909027116, -19.03943276465977164, 42.49890960531435269 ) ) ;
#125636=CARTESIAN_POINT ( 'NONE',  ( -4.483927247898782831, 16.52544592524335698, 22.70942372801901499 ) ) ;
#125637=CARTESIAN_POINT ( 'NONE',  ( -16.53943276465976808, 0.05219959533911058130, 61.24890960531435979 ) ) ;
#125638=CARTESIAN_POINT ( 'NONE',  ( -16.52544592524335698, -4.483927247898792601, 68.95942372801901854 ) ) ;
#125639=CARTESIAN_POINT ( 'NONE',  ( 21.55341960407619695, -5.719274019375665929, 26.04275706135235779 ) ) ;
#125640=CARTESIAN_POINT ( 'NONE',  ( 19.03943276465977164, -0.05219959533909143690, 53.74890960531436690 ) ) ;
#125641=CARTESIAN_POINT ( 'NONE',  ( -19.05341960407611168, -5.049401038298163336, 66.45724293864769550 ) ) ;
#125642=CARTESIAN_POINT ( 'NONE',  ( -4.483927247898782831, 16.52544592524335698, 67.70942372801901854 ) ) ;
#125645=CARTESIAN_POINT ( 'NONE',  ( 5.719274019375673035, 21.55341960407619339, 107.2927570613523471 ) ) ;
#125646=CARTESIAN_POINT ( 'NONE',  ( -5.153800228976328057, -19.02544592524343514, 42.29057627198101699 ) ) ;
#125647=VERTEX_POINT ( 'NONE', #106180 ) ;
#125648=CARTESIAN_POINT ( 'NONE',  ( 14.34966873604972726, -8.224510206698740333, 25.83442372801901499 ) ) ;
#125650=CARTESIAN_POINT ( 'NONE',  ( 13.89961937509957401, 13.97604488694547697, 46.87609039468565442 ) ) ;
#125651=CARTESIAN_POINT ( 'NONE',  ( -8.224510206698735004, -14.34966873604973081, 39.58442372801901143 ) ) ;
#125652=CARTESIAN_POINT ( 'NONE',  ( -9.474510206698964154, 16.51473224551069663, 40.41557627198103120 ) ) ;
#125653=CARTESIAN_POINT ( 'NONE',  ( -9.474510206698964154, 16.51473224551069663, 70.41557627198102409 ) ) ;
#125654=CARTESIAN_POINT ( 'NONE',  ( 21.55341960407610458, 5.719274019375980345, 83.95724293864770971 ) ) ;
#125655=CARTESIAN_POINT ( 'NONE',  ( 13.97604488694527802, 13.89961937509977652, 84.37390960531433848 ) ) ;
#125656=CARTESIAN_POINT ( 'NONE',  ( -19.02544592524342804, 5.153800228976336051, 111.0405762719810099 ) ) ;
#125657=CARTESIAN_POINT ( 'NONE',  ( 19.03943276465977164, -0.05219959533909143690, 68.74890960531436690 ) ) ;
#125659=CARTESIAN_POINT ( 'NONE',  ( 5.049401038297881783, 19.05341960407617563, 102.2927570613523045 ) ) ;
#125660=CARTESIAN_POINT ( 'NONE',  ( -21.53943276465977519, 0.05219959533907696930, 71.24890960531435269 ) ) ;
#125661=CARTESIAN_POINT ( 'NONE',  ( 0.05219959533936267826, -19.03943276465977164, 25.00109039468566152 ) ) ;
#125662=CARTESIAN_POINT ( 'NONE',  ( -8.314922557960811034, -14.29746914071050412, 62.08224293864769550 ) ) ;
#125663=CARTESIAN_POINT ( 'NONE',  ( 10.81492255796106328, -18.62759615963255655, 90.41775706135236135 ) ) ;
#125664=CARTESIAN_POINT ( 'NONE',  ( -12.06949235617756955, 12.14591786802309770, 115.6239096053143669 ) ) ;
#125665=CARTESIAN_POINT ( 'NONE',  ( -14.29746914071049879, 8.314922557960819915, 25.83224293864769194 ) ) ;
#125666=CARTESIAN_POINT ( 'NONE',  ( -18.67979575497193778, 10.72451020669871902, 88.33442372801901854 ) ) ;
#125667=CARTESIAN_POINT ( 'NONE',  ( -16.46253265017160317, 9.564922557960807481, 85.83224293864769550 ) ) ;
#125668=CARTESIAN_POINT ( 'NONE',  ( -21.52544592524334988, -5.823673210054445271, 43.95942372801902565 ) ) ;
#125669=CARTESIAN_POINT ( 'NONE',  ( -9.564922557960796823, -16.46253265017161027, 77.08224293864769550 ) ) ;
#125670=CARTESIAN_POINT ( 'NONE',  ( -0.05219959533910754901, -16.53943276465976808, 92.49890960531436690 ) ) ;
#125671=CARTESIAN_POINT ( 'NONE',  ( 16.53943276465976808, -0.05219959533910856209, 58.74890960531436690 ) ) ;
#125672=CARTESIAN_POINT ( 'NONE',  ( 15.80617190586746368, 15.72974639402197994, 74.37390960531436690 ) ) ;
#125673=CARTESIAN_POINT ( 'NONE',  ( -13.89961937509977652, 13.97604488694528158, 75.62390960531438111 ) ) ;
#125674=CARTESIAN_POINT ( 'NONE',  ( 0.05219959533907565091, 21.53943276465977519, 89.99890960531438111 ) ) ;
#125675=CARTESIAN_POINT ( 'NONE',  ( -19.03943276465977164, -0.05219959533935918106, 78.75109039468567573 ) ) ;
#125676=CARTESIAN_POINT ( 'NONE',  ( 19.05341960407618274, -5.049401038297876454, 36.04275706135233293 ) ) ;
#125677=CARTESIAN_POINT ( 'NONE',  ( -14.34966873604960291, -8.224510206698953496, 81.66557627198103830 ) ) ;
#125678=CARTESIAN_POINT ( 'NONE',  ( -21.55341960407610458, -5.719274019375992779, 56.45724293864768839 ) ) ;
#125679=CARTESIAN_POINT ( 'NONE',  ( 17.05587630539787369, -6.762274262135688829, 28.24180309037314274 ) ) ;
#125680=CARTESIAN_POINT ( 'NONE',  ( 4.379528057220339221, -16.55341960407611168, 22.70724293864769194 ) ) ;
#125682=CARTESIAN_POINT ( 'NONE',  ( -19.02544592524334988, -5.153800228976617603, 98.95942372801900433 ) ) ;
#125683=CARTESIAN_POINT ( 'NONE',  ( -14.29746914071049879, 8.314922557960819915, 80.83224293864769550 ) ) ;
#125684=CARTESIAN_POINT ( 'NONE',  ( -19.39720447994795194, -5.500000000000030198, 94.66317477297180005 ) ) ;
#125685=CARTESIAN_POINT ( 'NONE',  ( -0.05219959533909027116, -19.03943276465977164, 77.49890960531435269 ) ) ;
#125686=CARTESIAN_POINT ( 'NONE',  ( 9.564922557960805705, 16.46253265017160317, 29.58224293864769550 ) ) ;
#125687=CARTESIAN_POINT ( 'NONE',  ( -0.05219959533910754901, -16.53943276465976808, 67.49890960531436690 ) ) ;
#125688=CARTESIAN_POINT ( 'NONE',  ( 16.51473224551069308, 9.474510206698969483, 99.16557627198102409 ) ) ;
#125689=CARTESIAN_POINT ( 'NONE',  ( -19.02544592524334988, -5.153800228976617603, 88.95942372801897591 ) ) ;
#125690=CARTESIAN_POINT ( 'NONE',  ( -16.46253265017160317, 9.564922557960807481, 60.83224293864769550 ) ) ;
#125691=CARTESIAN_POINT ( 'NONE',  ( -0.05219959533934338120, 16.53943276465976808, 27.50109039468567929 ) ) ;
#125692=CARTESIAN_POINT ( 'NONE',  ( -5.153800228976328057, -19.02544592524343514, 82.29057627198103830 ) ) ;
#125693=CARTESIAN_POINT ( 'NONE',  ( -21.52544592524343514, 5.823673210054127303, 81.04057627198102409 ) ) ;
#125694=CARTESIAN_POINT ( 'NONE',  ( 16.53943276465976808, 0.05219959533934440121, 66.25109039468567573 ) ) ;
#125695=CARTESIAN_POINT ( 'NONE',  ( -16.20579543436698344, 7.371946100355022402, 94.43479165828047428 ) ) ;
#125696=CARTESIAN_POINT ( 'NONE',  ( 16.46253265017160672, -9.564922557960803928, 58.33224293864769550 ) ) ;
#125697=CARTESIAN_POINT ( 'NONE',  ( 21.55341960407610458, 5.719274019375980345, 73.95724293864769550 ) ) ;
#125698=CARTESIAN_POINT ( 'NONE',  ( -16.51473224551082808, 9.474510206698731452, 93.33442372801900433 ) ) ;
#125699=CARTESIAN_POINT ( 'NONE',  ( -16.53943276465976808, 0.05219959533911058130, 31.24890960531435979 ) ) ;
#125700=CARTESIAN_POINT ( 'NONE',  ( 5.823673210054444382, -21.52544592524334988, 45.20942372801901854 ) ) ;
#125702=CARTESIAN_POINT ( 'NONE',  ( -0.05219959533934338120, 16.53943276465976808, 72.50109039468568994 ) ) ;
#125703=CARTESIAN_POINT ( 'NONE',  ( -19.02544592524342804, 5.153800228976336051, 106.0405762719810241 ) ) ;
#125704=CARTESIAN_POINT ( 'NONE',  ( 13.97604488694527802, 13.89961937509977830, 104.3739096053143527 ) ) ;
#125705=CARTESIAN_POINT ( 'NONE',  ( -16.61371651742599909, -7.165104196376252510, 36.14584930007006847 ) ) ;
#125706=CARTESIAN_POINT ( 'NONE',  ( -12.06949235617739369, -12.14591786802326823, 94.37609039468568994 ) ) ;
#125707=CARTESIAN_POINT ( 'NONE',  ( 4.483927247898790824, -16.52544592524335698, 40.20942372801901854 ) ) ;
#125708=CARTESIAN_POINT ( 'NONE',  ( 9.564922557960805705, 16.46253265017160317, 49.58224293864770260 ) ) ;
#125709=CARTESIAN_POINT ( 'NONE',  ( 19.02544592524343514, -5.153800228976328945, 48.54057627198103120 ) ) ;
#125710=CARTESIAN_POINT ( 'NONE',  ( 9.564922557960805705, 16.46253265017160317, 64.58224293864769550 ) ) ;
#125711=CARTESIAN_POINT ( 'NONE',  ( -15.72974639402176322, -15.80617190586768395, 49.37609039468569705 ) ) ;
#125712=CARTESIAN_POINT ( 'NONE',  ( 0.05219959533934541429, -16.53943276465976808, 60.00109039468568284 ) ) ;
#125713=CARTESIAN_POINT ( 'NONE',  ( -16.52544592524342804, 4.483927247898546575, 36.04057627198102409 ) ) ;
#125714=CARTESIAN_POINT ( 'NONE',  ( -0.05219959533909027116, -19.03943276465977164, 42.49890960531435269 ) ) ;
#125715=CARTESIAN_POINT ( 'NONE',  ( -9.564922557960796823, -16.46253265017161027, 32.08224293864769550 ) ) ;
#125716=CARTESIAN_POINT ( 'NONE',  ( -4.483927247898782831, 16.52544592524335698, 32.70942372801900433 ) ) ;
#125717=CARTESIAN_POINT ( 'NONE',  ( 9.474510206698729675, 16.51473224551082808, 77.08442372801900433 ) ) ;
#125718=CARTESIAN_POINT ( 'NONE',  ( 16.53943276465976808, -0.05219959533910856209, 88.74890960531436690 ) ) ;
#125719=CARTESIAN_POINT ( 'NONE',  ( -5.049401038298153566, 19.05341960407611168, 50.20724293864770260 ) ) ;
#125720=CARTESIAN_POINT ( 'NONE',  ( -0.05219959533936034679, 19.03943276465977164, 92.50109039468566152 ) ) ;
#125721=CARTESIAN_POINT ( 'NONE',  ( 17.48847506799967988, -5.747544572773779947, 93.32697437843278010 ) ) ;
#125722=CARTESIAN_POINT ( 'NONE',  ( 10.72451020669871369, 18.67979575497193778, 82.08442372801901854 ) ) ;
#125723=CARTESIAN_POINT ( 'NONE',  ( -0.05219959533934338120, 16.53943276465976808, 52.50109039468567573 ) ) ;
#125724=CARTESIAN_POINT ( 'NONE',  ( -17.50000000000144240, 3.254303733634824169, 25.02395893071417632 ) ) ;
#125725=CARTESIAN_POINT ( 'NONE',  ( 21.53943276465977519, -0.05219959533907433946, 48.74890960531435979 ) ) ;
#125726=CARTESIAN_POINT ( 'NONE',  ( -4.483927247898782831, 16.52544592524335698, 42.70942372801901854 ) ) ;
#125727=CARTESIAN_POINT ( 'NONE',  ( -9.474510206698964154, 16.51473224551069663, 25.41557627198103120 ) ) ;
#125728=CARTESIAN_POINT ( 'NONE',  ( 0.05219959533936267826, -19.03943276465977164, 35.00109039468566863 ) ) ;
#125730=CARTESIAN_POINT ( 'NONE',  ( 13.97604488694527802, 13.89961937509977652, 49.37390960531434558 ) ) ;
#125732=CARTESIAN_POINT ( 'NONE',  ( -9.564922557960796823, -16.46253265017161027, 67.08224293864769550 ) ) ;
#125733=CARTESIAN_POINT ( 'NONE',  ( 17.50000000000000711, -3.850315288878807696, 111.7662913060345034 ) ) ;
#125734=CARTESIAN_POINT ( 'NONE',  ( -15.80617190586768217, 15.72974639402176855, 113.1260903946856899 ) ) ;
#125735=CARTESIAN_POINT ( 'NONE',  ( -16.53943276465976808, 0.05219959533911058130, 36.24890960531435979 ) ) ;
#125736=CARTESIAN_POINT ( 'NONE',  ( -5.049401038298153566, 19.05341960407611168, 40.20724293864768839 ) ) ;
#125737=CARTESIAN_POINT ( 'NONE',  ( 5.049401038298161559, -19.05341960407611168, 102.7072429386476955 ) ) ;
#125738=CARTESIAN_POINT ( 'NONE',  ( -18.67979575497193778, 10.72451020669871902, 68.33442372801900433 ) ) ;
#125739=CARTESIAN_POINT ( 'NONE',  ( -19.05341960407611168, -5.049401038298163336, 51.45724293864770260 ) ) ;
#125740=CARTESIAN_POINT ( 'NONE',  ( 21.53943276465977519, 0.05219959533937863772, 66.25109039468567573 ) ) ;
#125741=CARTESIAN_POINT ( 'NONE',  ( -5.719274019375978568, 21.55341960407610458, 25.20724293864769550 ) ) ;
#125742=CARTESIAN_POINT ( 'NONE',  ( -9.564922557960796823, -16.46253265017161027, 37.08224293864768839 ) ) ;
#125743=CARTESIAN_POINT ( 'NONE',  ( -10.81492255796105439, 18.62759615963255655, 22.91775706135235069 ) ) ;
#125744=CARTESIAN_POINT ( 'NONE',  ( -13.89961937509957401, -13.97604488694547875, 44.37609039468566863 ) ) ;
#125745=CARTESIAN_POINT ( 'NONE',  ( -19.02544592524342804, 5.153800228976336051, 26.04057627198103120 ) ) ;
#125746=CARTESIAN_POINT ( 'NONE',  ( -9.474510206698964154, 16.51473224551069663, 80.41557627198103830 ) ) ;
#125747=CARTESIAN_POINT ( 'NONE',  ( 0.05219959533936267826, -19.03943276465977164, 105.0010903946856615 ) ) ;
#125748=CARTESIAN_POINT ( 'NONE',  ( -14.29746914071049879, 8.314922557960819915, 80.83224293864769550 ) ) ;
#125749=CARTESIAN_POINT ( 'NONE',  ( 0.05219959533907565091, 21.53943276465977519, 39.99890960531436690 ) ) ;
#125750=CARTESIAN_POINT ( 'NONE',  ( -19.02544592524334988, -5.153800228976617603, 98.95942372801900433 ) ) ;
#125751=CARTESIAN_POINT ( 'NONE',  ( 5.719274019375991003, -21.55341960407610458, 107.7072429386476955 ) ) ;
#125752=CARTESIAN_POINT ( 'NONE',  ( 18.67979575497194134, -10.72451020669871369, 60.83442372801901854 ) ) ;
#125753=CARTESIAN_POINT ( 'NONE',  ( 14.34966873604972726, -8.224510206698740333, 60.83442372801901854 ) ) ;
#125754=CARTESIAN_POINT ( 'NONE',  ( -16.55341960407617563, 4.379528057220093196, 48.54275706135234714 ) ) ;
#125755=CARTESIAN_POINT ( 'NONE',  ( 15.72974639402199770, -15.80617190586745480, 63.12390960531435979 ) ) ;
#125756=CARTESIAN_POINT ( 'NONE',  ( 19.03943276465977164, -0.05219959533909143690, 48.74890960531435979 ) ) ;
#125757=CARTESIAN_POINT ( 'NONE',  ( -12.06949235617739369, -12.14591786802326823, 74.37609039468568994 ) ) ;
#125758=CARTESIAN_POINT ( 'NONE',  ( -5.719274019375978568, 21.55341960407610458, 100.2072429386476955 ) ) ;
#125759=CARTESIAN_POINT ( 'NONE',  ( 12.06949235617757843, -12.14591786802309237, 53.12390960531436690 ) ) ;
#125760=CARTESIAN_POINT ( 'NONE',  ( 13.97604488694527802, 13.89961937509977652, 74.37390960531436690 ) ) ;
#125761=CARTESIAN_POINT ( 'NONE',  ( -4.379528057220086978, -16.55341960407618274, 74.79275706135234714 ) ) ;
#125762=CARTESIAN_POINT ( 'NONE',  ( 4.483927247898790824, -16.52544592524335698, 20.20942372801900788 ) ) ;
#125763=CARTESIAN_POINT ( 'NONE',  ( -10.72451020669898014, 18.67979575497178502, 110.4155762719810383 ) ) ;
#125764=CARTESIAN_POINT ( 'NONE',  ( -14.29746914071049879, 8.314922557960819915, 50.83224293864770971 ) ) ;
#125766=CARTESIAN_POINT ( 'NONE',  ( -17.48853670773247160, 5.747243402303039872, 73.66671299749992841 ) ) ;
#125767=CARTESIAN_POINT ( 'NONE',  ( 18.67979575497178502, 10.72451020669898547, 89.16557627198102409 ) ) ;
#125768=CARTESIAN_POINT ( 'NONE',  ( -12.14591786802309592, -12.06949235617757132, 31.87390960531435979 ) ) ;
#125770=CARTESIAN_POINT ( 'NONE',  ( -16.81555441253551919, -7.025013491695508705, 54.36314554665747778 ) ) ;
#125771=CARTESIAN_POINT ( 'NONE',  ( -21.55341960407610458, -5.719274019375992779, 106.4572429386477097 ) ) ;
#125772=CARTESIAN_POINT ( 'NONE',  ( -5.049401038298153566, 19.05341960407611168, 105.2072429386476671 ) ) ;
#125773=CARTESIAN_POINT ( 'NONE',  ( -5.719274019375978568, 21.55341960407610458, 115.2072429386476955 ) ) ;
#125774=CARTESIAN_POINT ( 'NONE',  ( -14.29746914071049879, 8.314922557960819915, 55.83224293864770260 ) ) ;
#125775=CARTESIAN_POINT ( 'NONE',  ( -14.34966873604972548, 8.224510206698743886, 53.33442372801901854 ) ) ;
#125776=CARTESIAN_POINT ( 'NONE',  ( 5.153800228976335163, 19.02544592524342804, 64.79057627198100988 ) ) ;
#125777=CARTESIAN_POINT ( 'NONE',  ( 9.474510206698729675, 16.51473224551082808, 57.08442372801900433 ) ) ;
#125778=CARTESIAN_POINT ( 'NONE',  ( -16.46253265017160317, 9.564922557960807481, 85.83224293864769550 ) ) ;
#125779=CARTESIAN_POINT ( 'NONE',  ( -10.81492255796078084, -18.62759615963271287, 37.08224293864768129 ) ) ;
#125780=CARTESIAN_POINT ( 'NONE',  ( -9.474510206698964154, 16.51473224551069663, 65.41557627198102409 ) ) ;
#125781=CARTESIAN_POINT ( 'NONE',  ( 19.05341960407611168, 5.049401038298154454, 48.95724293864768129 ) ) ;
#125782=CARTESIAN_POINT ( 'NONE',  ( -0.05219959533934338120, 16.53943276465976808, 22.50109039468567573 ) ) ;
#125783=CARTESIAN_POINT ( 'NONE',  ( -5.049401038297874678, -19.05341960407617918, 59.79275706135231871 ) ) ;
#125784=CARTESIAN_POINT ( 'NONE',  ( 21.52544592524344225, -5.823673210054117533, 108.5405762719810241 ) ) ;
#125785=CARTESIAN_POINT ( 'NONE',  ( 8.224510206698953496, -14.34966873604960469, 32.91557627198102409 ) ) ;
#125786=CARTESIAN_POINT ( 'NONE',  ( 13.89961937509977652, -13.97604488694527269, 83.12390960531436690 ) ) ;
#125787=CARTESIAN_POINT ( 'NONE',  ( 10.72451020669898902, -18.67979575497178502, 57.91557627198103120 ) ) ;
#125788=CARTESIAN_POINT ( 'NONE',  ( -10.72451020669898014, 18.67979575497178502, 100.4155762719810241 ) ) ;
#125789=CARTESIAN_POINT ( 'NONE',  ( -12.14591786802326823, 12.06949235617739902, 23.12609039468567573 ) ) ;
#125790=CARTESIAN_POINT ( 'NONE',  ( -5.719274019375978568, 21.55341960407610458, 25.20724293864769550 ) ) ;
#125791=CARTESIAN_POINT ( 'NONE',  ( -15.72974639402176322, -15.80617190586768395, 84.37609039468570415 ) ) ;
#125792=CARTESIAN_POINT ( 'NONE',  ( 9.474510206698971260, -16.51473224551069308, 87.91557627198102409 ) ) ;
#125793=CARTESIAN_POINT ( 'NONE',  ( -9.564922557960796823, -16.46253265017161027, 32.08224293864769550 ) ) ;
#125794=CARTESIAN_POINT ( 'NONE',  ( 16.51473224551069308, 9.474510206698969483, 79.16557627198103830 ) ) ;
#125795=CARTESIAN_POINT ( 'NONE',  ( -4.379528057220328563, 16.55341960407611168, 110.2072429386477239 ) ) ;
#125796=CARTESIAN_POINT ( 'NONE',  ( 16.51473224551069308, 9.474510206698969483, 69.16557627198102409 ) ) ;
#125797=CARTESIAN_POINT ( 'NONE',  ( 16.53943276465976808, 0.05219959533934440121, 21.25109039468567218 ) ) ;
#125798=CARTESIAN_POINT ( 'NONE',  ( 17.50000000000000000, 5.499999999999997335, 31.70309617465830243 ) ) ;
#125799=CARTESIAN_POINT ( 'NONE',  ( -5.719274019375665041, -21.55341960407619695, 99.79275706135234714 ) ) ;
#125800=CARTESIAN_POINT ( 'NONE',  ( -13.89961937509977652, 13.97604488694528158, 110.6239096053143243 ) ) ;
#125801=CARTESIAN_POINT ( 'NONE',  ( 12.14591786802327356, -12.06949235617739191, 90.62609039468567573 ) ) ;
#125803=CARTESIAN_POINT ( 'NONE',  ( 19.05341960407617918, -5.049401038297876454, 66.04275706135233293 ) ) ;
#125804=CARTESIAN_POINT ( 'NONE',  ( 13.97604488694548053, -13.89961937509957401, 30.62609039468566863 ) ) ;
#125806=CARTESIAN_POINT ( 'NONE',  ( -19.03943276465977164, 0.05219959533909376836, 26.24890960531435624 ) ) ;
#125807=CARTESIAN_POINT ( 'NONE',  ( 14.29746914071049879, -8.314922557960816363, 38.33224293864768839 ) ) ;
#125808=CYLINDRICAL_SURFACE ( 'NONE', #79072, 2.000000000000000000 ) ;
#125809=CARTESIAN_POINT ( 'NONE',  ( -12.14591786802326823, 12.06949235617739902, 108.1260903946856757 ) ) ;
#125810=CARTESIAN_POINT ( 'NONE',  ( 16.31925111598458145, 7.325300261831479531, 67.33575461032748422 ) ) ;
#125811=CARTESIAN_POINT ( 'NONE',  ( -14.29746914071037622, -8.314922557961029526, 79.16775706135234714 ) ) ;
#125812=CARTESIAN_POINT ( 'NONE',  ( 5.153800228976335163, 19.02544592524342804, 39.79057627198100988 ) ) ;
#125813=CARTESIAN_POINT ( 'NONE',  ( -21.52544592524334988, -5.823673210054445271, 98.95942372801903275 ) ) ;
#125814=CARTESIAN_POINT ( 'NONE',  ( -16.51473224551082808, 9.474510206698731452, 103.3344237280190043 ) ) ;
#125815=CARTESIAN_POINT ( 'NONE',  ( 5.719274019375673035, 21.55341960407619339, 77.29275706135234714 ) ) ;
#125816=CARTESIAN_POINT ( 'NONE',  ( -13.97604488694547697, 13.89961937509957934, 58.12609039468566863 ) ) ;
#125817=CARTESIAN_POINT ( 'NONE',  ( -13.97604488694527625, -13.89961937509977652, 81.87390960531436690 ) ) ;
#125818=CARTESIAN_POINT ( 'NONE',  ( 19.02544592524343514, -5.153800228976328945, 68.54057627198103830 ) ) ;
#125820=CARTESIAN_POINT ( 'NONE',  ( 0.05219959533910956823, 16.53943276465976808, 64.99890960531435269 ) ) ;
#125822=CARTESIAN_POINT ( 'NONE',  ( 18.62759615963271287, -10.81492255796078972, 58.33224293864768839 ) ) ;
#125823=CARTESIAN_POINT ( 'NONE',  ( -19.02544592524342804, 5.153800228976336051, 46.04057627198101699 ) ) ;
#125824=CARTESIAN_POINT ( 'NONE',  ( 21.52544592524344225, -5.823673210054117533, 83.54057627198102409 ) ) ;
#125825=CARTESIAN_POINT ( 'NONE',  ( -12.14591786802326823, 12.06949235617739902, 83.12609039468568994 ) ) ;
#125827=CARTESIAN_POINT ( 'NONE',  ( -9.564922557960796823, -16.46253265017161027, 47.08224293864769550 ) ) ;
#125828=CARTESIAN_POINT ( 'NONE',  ( 4.483927247898545687, 16.52544592524342804, 79.79057627198102409 ) ) ;
#125830=CARTESIAN_POINT ( 'NONE',  ( -9.564922557960796823, -16.46253265017161027, 47.08224293864769550 ) ) ;
#125831=CARTESIAN_POINT ( 'NONE',  ( -19.05341960407611168, -5.049401038298163336, 26.45724293864769550 ) ) ;
#125832=CARTESIAN_POINT ( 'NONE',  ( 19.03943276465977164, 0.05219959533936151252, 66.25109039468567573 ) ) ;
#125833=CARTESIAN_POINT ( 'NONE',  ( 4.483927247898545687, 16.52544592524342804, 69.79057627198102409 ) ) ;
#125834=CARTESIAN_POINT ( 'NONE',  ( 21.53943276465977519, 0.05219959533937863772, 51.25109039468568994 ) ) ;
#125835=CARTESIAN_POINT ( 'NONE',  ( 9.564922557960805705, 16.46253265017160317, 39.58224293864768839 ) ) ;
#125836=CARTESIAN_POINT ( 'NONE',  ( 18.62759615963271287, -10.81492255796078972, 108.3322429386477097 ) ) ;
#125837=CARTESIAN_POINT ( 'NONE',  ( 13.97604488694527802, 13.89961937509977652, 114.3739096053143669 ) ) ;
#125838=CARTESIAN_POINT ( 'NONE',  ( 8.224510206698953496, -14.34966873604960469, 82.91557627198103830 ) ) ;
#125840=CARTESIAN_POINT ( 'NONE',  ( -13.89961937509977652, 13.97604488694528158, 40.62390960531435979 ) ) ;
#125842=CARTESIAN_POINT ( 'NONE',  ( 5.153800228976615827, -19.02544592524334988, 100.2094237280190043 ) ) ;
#125843=CARTESIAN_POINT ( 'NONE',  ( -18.62759615963255300, -10.81492255796106328, 34.16775706135234714 ) ) ;
#125844=CARTESIAN_POINT ( 'NONE',  ( 16.51473224551069308, 9.474510206698969483, 89.16557627198103830 ) ) ;
#125846=CARTESIAN_POINT ( 'NONE',  ( 5.049401038297881783, 19.05341960407617563, 67.29275706135234714 ) ) ;
#125847=CARTESIAN_POINT ( 'NONE',  ( 16.51473224551069308, 9.474510206698969483, 39.16557627198103120 ) ) ;
#125848=CARTESIAN_POINT ( 'NONE',  ( -14.29746914071049879, 8.314922557960819915, 60.83224293864769550 ) ) ;
#125849=CARTESIAN_POINT ( 'NONE',  ( 16.55341960407611168, 4.379528057220329451, 63.95724293864770260 ) ) ;
#125850=CARTESIAN_POINT ( 'NONE',  ( -9.474510206698964154, 16.51473224551069663, 70.41557627198102409 ) ) ;
#125851=CARTESIAN_POINT ( 'NONE',  ( -21.52544592524343514, 5.823673210054127303, 96.04057627198102409 ) ) ;
#125852=CARTESIAN_POINT ( 'NONE',  ( -5.153800228976328057, -19.02544592524343514, 72.29057627198102409 ) ) ;
#125854=CARTESIAN_POINT ( 'NONE',  ( -5.823673210054431948, 21.52544592524334988, 107.7094237280190328 ) ) ;
#125855=CARTESIAN_POINT ( 'NONE',  ( 19.05341960407611168, 5.049401038298154454, 33.95724293864769550 ) ) ;
#125856=CARTESIAN_POINT ( 'NONE',  ( -16.55341960407617563, 4.379528057220093196, 108.5427570613523756 ) ) ;
#125857=CARTESIAN_POINT ( 'NONE',  ( 0.05219959533910956823, 16.53943276465976808, 114.9989096053143669 ) ) ;
#125858=CARTESIAN_POINT ( 'NONE',  ( 19.02544592524334988, 5.153800228976608722, 111.4594237280190043 ) ) ;
#125860=CARTESIAN_POINT ( 'NONE',  ( 10.72451020669871369, 18.67979575497193778, 32.08442372801901854 ) ) ;
#125861=CARTESIAN_POINT ( 'NONE',  ( 16.46253265017146816, 9.564922557961045513, 51.66775706135233293 ) ) ;
#125862=CARTESIAN_POINT ( 'NONE',  ( 12.06949235617739724, 12.14591786802326823, 111.8760903946856615 ) ) ;
#125863=CARTESIAN_POINT ( 'NONE',  ( -21.53943276465977519, 0.05219959533907696930, 76.24890960531435269 ) ) ;
#125864=CARTESIAN_POINT ( 'NONE',  ( 16.51473224551069308, 9.474510206698969483, 114.1655762719810241 ) ) ;
#125865=CARTESIAN_POINT ( 'NONE',  ( 14.29746914071049879, -8.314922557960816363, 53.33224293864769550 ) ) ;
#125866=CARTESIAN_POINT ( 'NONE',  ( -16.51473224551069308, -9.474510206698971260, 26.66557627198103120 ) ) ;
#125867=CARTESIAN_POINT ( 'NONE',  ( 13.97604488694527802, 13.89961937509977652, 34.37390960531436690 ) ) ;
#125868=CARTESIAN_POINT ( 'NONE',  ( 9.564922557961047289, -16.46253265017146816, 30.41775706135232937 ) ) ;
#125869=CARTESIAN_POINT ( 'NONE',  ( 0.05219959533934541429, -16.53943276465976808, 90.00109039468567573 ) ) ;
#125870=CARTESIAN_POINT ( 'NONE',  ( -16.52544592524335698, -4.483927247898792601, 48.95942372801902565 ) ) ;
#125871=CARTESIAN_POINT ( 'NONE',  ( -18.67979575497178146, -10.72451020669898902, 21.66557627198102409 ) ) ;
#125872=CARTESIAN_POINT ( 'NONE',  ( -19.02544592524342804, 5.153800228976336051, 56.04057627198100988 ) ) ;
#125873=CARTESIAN_POINT ( 'NONE',  ( -21.55341960407619339, 5.719274019375674811, 88.54275706135236135 ) ) ;
#125874=CARTESIAN_POINT ( 'NONE',  ( 5.153800228976335163, 19.02544592524342804, 79.79057627198102409 ) ) ;
#125875=CARTESIAN_POINT ( 'NONE',  ( 14.29746914071037800, 8.314922557961029526, 66.66775706135234714 ) ) ;
#125876=CARTESIAN_POINT ( 'NONE',  ( -8.224510206698948167, 14.34966873604960824, 110.4155762719810383 ) ) ;
#125877=CARTESIAN_POINT ( 'NONE',  ( -16.53943276465976808, 0.05219959533911058130, 26.24890960531435624 ) ) ;
#125879=CARTESIAN_POINT ( 'NONE',  ( -21.53943276465977519, -0.05219959533937600094, 68.75109039468568994 ) ) ;
#125880=CARTESIAN_POINT ( 'NONE',  ( -19.03943276465977164, 0.05219959533909376836, 86.24890960531436690 ) ) ;
#125881=CARTESIAN_POINT ( 'NONE',  ( -19.02544592524342804, 5.153800228976336051, 76.04057627198102409 ) ) ;
#125882=CARTESIAN_POINT ( 'NONE',  ( 19.03943276465977164, -0.05219959533909143690, 108.7489096053143527 ) ) ;
#125883=CARTESIAN_POINT ( 'NONE',  ( -12.06949235617756955, 12.14591786802309770, 60.62390960531437401 ) ) ;
#125884=CARTESIAN_POINT ( 'NONE',  ( -16.52544592524335698, -4.483927247898792601, 108.9594237280190185 ) ) ;
#125885=CARTESIAN_POINT ( 'NONE',  ( -16.53943276465976808, 0.05219959533911058130, 41.24890960531435269 ) ) ;
#125886=CARTESIAN_POINT ( 'NONE',  ( -12.06949235617739369, -12.14591786802326823, 39.37609039468567573 ) ) ;
#125888=CARTESIAN_POINT ( 'NONE',  ( 19.05341960407617918, -5.049401038297876454, 41.04275706135233293 ) ) ;
#125889=CARTESIAN_POINT ( 'NONE',  ( -16.51473224551069308, -9.474510206698971260, 81.66557627198103830 ) ) ;
#125890=CARTESIAN_POINT ( 'NONE',  ( -19.05341960407617563, 5.049401038297882671, 53.54275706135231871 ) ) ;
#125892=CARTESIAN_POINT ( 'NONE',  ( 17.60779699588839975, 5.500000000000012434, 58.84981316670105400 ) ) ;
#125893=CARTESIAN_POINT ( 'NONE',  ( 9.474510206698729675, 16.51473224551082808, 87.08442372801900433 ) ) ;
#125894=CARTESIAN_POINT ( 'NONE',  ( -12.06949235617739369, -12.14591786802326823, 79.37609039468567573 ) ) ;
#125896=CARTESIAN_POINT ( 'NONE',  ( -16.51473224551069308, -9.474510206698971260, 106.6655762719810383 ) ) ;
#125897=CARTESIAN_POINT ( 'NONE',  ( -10.72451020669870658, -18.67979575497194134, 44.58442372801901854 ) ) ;
#125898=CARTESIAN_POINT ( 'NONE',  ( 19.03943276465977164, 0.05219959533936151252, 91.25109039468566152 ) ) ;
#125899=CARTESIAN_POINT ( 'NONE',  ( 17.50000000000001421, 4.414220700528461272, 23.46024564252573796 ) ) ;
#125900=CARTESIAN_POINT ( 'NONE',  ( 13.97604488694527802, 13.89961937509977652, 49.37390960531434558 ) ) ;
#125901=B_SPLINE_CURVE_WITH_KNOTS ( 'NONE', 3,
 ( #91360, #108540, #107536, #169212, #139859, #14553 ),
 .UNSPECIFIED., .F., .F.,
 ( 4, 2, 4 ),
 ( 0.007228050697041581325, 0.007608510107495070757, 0.007988969517948561055 ),
 .UNSPECIFIED. ) ;
#125902=CARTESIAN_POINT ( 'NONE',  ( -16.46253265017160317, 9.564922557960807481, 100.8322429386477097 ) ) ;
#125903=CARTESIAN_POINT ( 'NONE',  ( 8.224510206698953496, -14.34966873604960469, 62.91557627198102409 ) ) ;
#125904=CARTESIAN_POINT ( 'NONE',  ( 5.153800228976335163, 19.02544592524342804, 44.79057627198103830 ) ) ;
#125905=CARTESIAN_POINT ( 'NONE',  ( -16.46253265017160317, 9.564922557960807481, 60.83224293864769550 ) ) ;
#125906=CARTESIAN_POINT ( 'NONE',  ( -13.89961937509957401, -13.97604488694547875, 69.37609039468564731 ) ) ;
#125908=CARTESIAN_POINT ( 'NONE',  ( 5.153800228976615827, -19.02544592524334988, 30.20942372801900433 ) ) ;
#125909=CARTESIAN_POINT ( 'NONE',  ( -5.153800228976328057, -19.02544592524343514, 62.29057627198100988 ) ) ;
#125910=CARTESIAN_POINT ( 'NONE',  ( -21.53943276465977519, 0.05219959533907696930, 76.24890960531435269 ) ) ;
#125911=CARTESIAN_POINT ( 'NONE',  ( -8.314922557960811034, -14.29746914071050412, 62.08224293864769550 ) ) ;
#125912=CARTESIAN_POINT ( 'NONE',  ( -5.153800228976607833, 19.02544592524334988, 32.70942372801899722 ) ) ;
#125913=CARTESIAN_POINT ( 'NONE',  ( 10.81492255796078972, 18.62759615963270932, 44.58224293864769550 ) ) ;
#125914=CARTESIAN_POINT ( 'NONE',  ( -5.823673210054116645, -21.52544592524344225, 22.29057627198102765 ) ) ;
#125915=CARTESIAN_POINT ( 'NONE',  ( -19.05341960407611168, -5.049401038298163336, 71.45724293864766707 ) ) ;
#125916=CARTESIAN_POINT ( 'NONE',  ( 19.05341960407611168, 5.049401038298154454, 38.95724293864767418 ) ) ;
#125917=CARTESIAN_POINT ( 'NONE',  ( -12.06949235617756955, 12.14591786802309770, 105.6239096053143669 ) ) ;
#125918=CARTESIAN_POINT ( 'NONE',  ( 10.81492255796078972, 18.62759615963270932, 104.5822429386477097 ) ) ;
#125919=CARTESIAN_POINT ( 'NONE',  ( 16.46253265017160672, -9.564922557960803928, 108.3322429386476955 ) ) ;
#125920=CARTESIAN_POINT ( 'NONE',  ( -21.52544592524334988, -5.823673210054445271, 23.95942372801901143 ) ) ;
#125921=CARTESIAN_POINT ( 'NONE',  ( 16.46253265017160672, -9.564922557960803928, 38.33224293864768839 ) ) ;
#125922=CARTESIAN_POINT ( 'NONE',  ( -21.53943276465977519, 0.05219959533907696930, 106.2489096053143811 ) ) ;
#125923=CARTESIAN_POINT ( 'NONE',  ( 19.05341960407617918, -5.049401038297876454, 46.04275706135233293 ) ) ;
#125924=CARTESIAN_POINT ( 'NONE',  ( 13.89961937509977652, -13.97604488694527269, 23.12390960531436335 ) ) ;
#125925=CARTESIAN_POINT ( 'NONE',  ( 17.50000000000001066, -3.242565516153302241, 102.5000000000090807 ) ) ;
#125926=CARTESIAN_POINT ( 'NONE',  ( 16.55341960407618274, -4.379528057220086978, 46.04275706135234714 ) ) ;
#125927=CARTESIAN_POINT ( 'NONE',  ( -13.89961937509977652, 13.97604488694528158, 25.62390960531434558 ) ) ;
#125929=CARTESIAN_POINT ( 'NONE',  ( -9.474510206698964154, 16.51473224551069663, 70.41557627198102409 ) ) ;
#125930=CARTESIAN_POINT ( 'NONE',  ( -14.34966873604960291, -8.224510206698953496, 106.6655762719810383 ) ) ;
#125931=CARTESIAN_POINT ( 'NONE',  ( 10.72451020669898902, -18.67979575497178502, 52.91557627198103830 ) ) ;
#125932=CARTESIAN_POINT ( 'NONE',  ( 14.29746914071049879, -8.314922557960816363, 78.33224293864770971 ) ) ;
#125933=CARTESIAN_POINT ( 'NONE',  ( 4.379528057220092307, 16.55341960407617563, 37.29275706135235424 ) ) ;
#125934=CARTESIAN_POINT ( 'NONE',  ( 15.80617190586769283, -15.72974639402175789, 80.62609039468567573 ) ) ;
#125935=CARTESIAN_POINT ( 'NONE',  ( -16.46253265017160317, 9.564922557960807481, 25.83224293864769194 ) ) ;
#125936=CARTESIAN_POINT ( 'NONE',  ( 4.483927247898790824, -16.52544592524335698, 110.2094237280190185 ) ) ;
#125937=CARTESIAN_POINT ( 'NONE',  ( 16.55341960407611168, 4.379528057220329451, 53.95724293864770260 ) ) ;
#125939=CARTESIAN_POINT ( 'NONE',  ( 13.89961937509977652, -13.97604488694527269, 58.12390960531436690 ) ) ;
#125940=CARTESIAN_POINT ( 'NONE',  ( 15.72974639402176855, 15.80617190586768217, 91.87609039468568994 ) ) ;
#125941=CARTESIAN_POINT ( 'NONE',  ( 15.72974639402199770, -15.80617190586745480, 108.1239096053143811 ) ) ;
#125942=CARTESIAN_POINT ( 'NONE',  ( 0.05219959533937995610, -21.53943276465977519, 70.00109039468568994 ) ) ;
#125943=CARTESIAN_POINT ( 'NONE',  ( 8.314922557961029526, -14.29746914071037800, 40.41775706135234714 ) ) ;
#125944=CARTESIAN_POINT ( 'NONE',  ( 16.53943276465976808, -0.05219959533910856209, 78.74890960531436690 ) ) ;
#125945=CARTESIAN_POINT ( 'NONE',  ( -21.53943276465977519, -0.05219959533937600094, 88.75109039468567573 ) ) ;
#125946=CARTESIAN_POINT ( 'NONE',  ( -4.483927247898782831, 16.52544592524335698, 112.7094237280190328 ) ) ;
#125948=CARTESIAN_POINT ( 'NONE',  ( -12.06949235617739369, -12.14591786802326823, 39.37609039468567573 ) ) ;
#125949=CARTESIAN_POINT ( 'NONE',  ( -12.06949235617756955, 12.14591786802309770, 35.62390960531437401 ) ) ;
#125950=CARTESIAN_POINT ( 'NONE',  ( 16.53943276465976808, 0.05219959533934440121, 91.25109039468568994 ) ) ;
#125951=CARTESIAN_POINT ( 'NONE',  ( 5.049401038298161559, -19.05341960407611168, 102.7072429386476955 ) ) ;
#125952=CARTESIAN_POINT ( 'NONE',  ( 13.97604488694527802, 13.89961937509977652, 94.37390960531436690 ) ) ;
#125953=CARTESIAN_POINT ( 'NONE',  ( -15.72974639402176322, -15.80617190586768395, 99.37609039468568994 ) ) ;
#125954=CARTESIAN_POINT ( 'NONE',  ( -16.52544592524335698, -4.483927247898792601, 108.9594237280190185 ) ) ;
#125955=CARTESIAN_POINT ( 'NONE',  ( 12.06949235617757843, -12.14591786802309237, 68.12390960531436690 ) ) ;
#125956=CARTESIAN_POINT ( 'NONE',  ( -9.564922557960796823, -16.46253265017161027, 82.08224293864768129 ) ) ;
#125958=CARTESIAN_POINT ( 'NONE',  ( -12.06949235617739369, -12.14591786802326823, 24.37609039468567573 ) ) ;
#125959=CARTESIAN_POINT ( 'NONE',  ( 9.564922557960805705, 16.46253265017160317, 29.58224293864769550 ) ) ;
#125960=CARTESIAN_POINT ( 'NONE',  ( -9.474510206698964154, 16.51473224551069663, 90.41557627198103830 ) ) ;
#125961=CARTESIAN_POINT ( 'NONE',  ( 0.05219959533934541429, -16.53943276465976808, 35.00109039468568284 ) ) ;
#125963=CARTESIAN_POINT ( 'NONE',  ( 13.97604488694548053, -13.89961937509957401, 40.62609039468564731 ) ) ;
#125964=CARTESIAN_POINT ( 'NONE',  ( 16.53943276465976808, 0.05219959533934440121, 91.25109039468568994 ) ) ;
#125965=CARTESIAN_POINT ( 'NONE',  ( 19.05341960407617918, -5.049401038297876454, 101.0427570613523045 ) ) ;
#125966=CARTESIAN_POINT ( 'NONE',  ( 5.049401038298161559, -19.05341960407611168, 27.70724293864769550 ) ) ;
#125967=CARTESIAN_POINT ( 'NONE',  ( 14.34966873604972726, -8.224510206698740333, 75.83442372801900433 ) ) ;
#125968=CARTESIAN_POINT ( 'NONE',  ( 4.483927247898790824, -16.52544592524335698, 70.20942372801904696 ) ) ;
#125970=CARTESIAN_POINT ( 'NONE',  ( -19.05341960407617563, 5.049401038297882671, 63.54275706135234003 ) ) ;
#125971=CARTESIAN_POINT ( 'NONE',  ( 18.67979575497194134, -10.72451020669871369, 110.8344237280190043 ) ) ;
#125972=CARTESIAN_POINT ( 'NONE',  ( 9.564922557960805705, 16.46253265017160317, 44.58224293864769550 ) ) ;
#125973=CARTESIAN_POINT ( 'NONE',  ( 9.474510206698971260, -16.51473224551069308, 87.91557627198102409 ) ) ;
#125974=CARTESIAN_POINT ( 'NONE',  ( -16.55341960407611168, -4.379528057220339221, 81.45724293864769550 ) ) ;
#125976=CARTESIAN_POINT ( 'NONE',  ( -16.51473224551082808, 9.474510206698731452, 58.33442372801900433 ) ) ;
#125977=CARTESIAN_POINT ( 'NONE',  ( -15.80617190586745835, -15.72974639402198527, 51.87390960531437401 ) ) ;
#125978=CARTESIAN_POINT ( 'NONE',  ( 15.72974639402176855, 15.80617190586768217, 106.8760903946856899 ) ) ;
#125979=CARTESIAN_POINT ( 'NONE',  ( 9.474510206698971260, -16.51473224551069308, 92.91557627198103830 ) ) ;
#125980=CARTESIAN_POINT ( 'NONE',  ( 5.153800228976615827, -19.02544592524334988, 30.20942372801900433 ) ) ;
#125981=CARTESIAN_POINT ( 'NONE',  ( 0.05219959533907565091, 21.53943276465977519, 59.99890960531436690 ) ) ;
#125982=CARTESIAN_POINT ( 'NONE',  ( 5.153800228976335163, 19.02544592524342804, 104.7905762719809957 ) ) ;
#125983=CARTESIAN_POINT ( 'NONE',  ( -13.97604488694547697, 13.89961937509957934, 88.12609039468563310 ) ) ;
#125984=CARTESIAN_POINT ( 'NONE',  ( -17.49999999999999645, 3.237210098469633923, 109.7123698737954243 ) ) ;
#125985=CARTESIAN_POINT ( 'NONE',  ( -8.224510206698735004, -14.34966873604973081, 19.58442372801901143 ) ) ;
#125986=CARTESIAN_POINT ( 'NONE',  ( 8.314922557960818139, 14.29746914071049879, 109.5822429386476955 ) ) ;
#125987=CARTESIAN_POINT ( 'NONE',  ( -19.03943276465977164, 0.05219959533909376836, 96.24890960531436690 ) ) ;
#125988=CARTESIAN_POINT ( 'NONE',  ( -5.823673210054116645, -21.52544592524344225, 72.29057627198102409 ) ) ;
#125989=CARTESIAN_POINT ( 'NONE',  ( 4.483927247898790824, -16.52544592524335698, 50.20942372801901854 ) ) ;
#125990=CARTESIAN_POINT ( 'NONE',  ( -5.719274019375665041, -21.55341960407619695, 49.79275706135234714 ) ) ;
#125991=CARTESIAN_POINT ( 'NONE',  ( 5.719274019375673035, 21.55341960407619339, 97.29275706135234714 ) ) ;
#125992=CARTESIAN_POINT ( 'NONE',  ( 4.483927247898790824, -16.52544592524335698, 100.2094237280190043 ) ) ;
#125993=CARTESIAN_POINT ( 'NONE',  ( 0.05219959533909260263, 19.03943276465977164, 84.99890960531436690 ) ) ;
#125994=CARTESIAN_POINT ( 'NONE',  ( 8.224510206698953496, -14.34966873604960469, 87.91557627198103830 ) ) ;
#125995=CARTESIAN_POINT ( 'NONE',  ( -0.05219959533910754901, -16.53943276465976808, 32.49890960531435979 ) ) ;
#125996=CARTESIAN_POINT ( 'NONE',  ( -13.97604488694547697, 13.89961937509957934, 73.12609039468568994 ) ) ;
#125998=CARTESIAN_POINT ( 'NONE',  ( 15.80617190586769283, -15.72974639402175789, 50.62609039468568994 ) ) ;
#125999=CARTESIAN_POINT ( 'NONE',  ( 13.89961937509957401, 13.97604488694547697, 31.87609039468566863 ) ) ;
#126000=CARTESIAN_POINT ( 'NONE',  ( 16.52544592524342804, -4.483927247898539470, 88.54057627198103830 ) ) ;
#126001=CARTESIAN_POINT ( 'NONE',  ( 13.97604488694527802, 13.89961937509977652, 109.3739096053143669 ) ) ;
#126002=CARTESIAN_POINT ( 'NONE',  ( 4.483927247898545687, 16.52544592524342804, 24.79057627198103120 ) ) ;
#126004=CARTESIAN_POINT ( 'NONE',  ( 10.72451020669871369, 18.67979575497193778, 87.08442372801901854 ) ) ;
#126005=CARTESIAN_POINT ( 'NONE',  ( 8.224510206698742110, 14.34966873604972548, 62.08442372801901143 ) ) ;
#126006=CARTESIAN_POINT ( 'NONE',  ( 8.224510206698742110, 14.34966873604972548, 102.0844237280190185 ) ) ;
#126007=CARTESIAN_POINT ( 'NONE',  ( -10.81492255796105439, 18.62759615963255655, 47.91775706135234714 ) ) ;
#126008=VERTEX_POINT ( 'NONE', #47507 ) ;
#126009=CARTESIAN_POINT ( 'NONE',  ( 18.67979575497194134, -10.72451020669871369, 35.83442372801901143 ) ) ;
#126010=CARTESIAN_POINT ( 'NONE',  ( 8.224510206698953496, -14.34966873604960469, 102.9155762719810383 ) ) ;
#126011=CARTESIAN_POINT ( 'NONE',  ( 19.02544592524343514, -5.153800228976328945, 23.54057627198102054 ) ) ;
#126012=CARTESIAN_POINT ( 'NONE',  ( 8.314922557960818139, 14.29746914071049879, 59.58224293864770260 ) ) ;
#126013=CARTESIAN_POINT ( 'NONE',  ( -19.02544592524342804, 5.153800228976336051, 71.04057627198099567 ) ) ;
#126014=CARTESIAN_POINT ( 'NONE',  ( 14.34966873604972726, -8.224510206698740333, 100.8344237280190185 ) ) ;
#126015=CARTESIAN_POINT ( 'NONE',  ( -19.05341960407611168, -5.049401038298163336, 41.45724293864769550 ) ) ;
#126016=CARTESIAN_POINT ( 'NONE',  ( -5.823673210054116645, -21.52544592524344225, 62.29057627198102409 ) ) ;
#126017=CARTESIAN_POINT ( 'NONE',  ( 4.379528057220339221, -16.55341960407611168, 97.70724293864772392 ) ) ;
#126018=CARTESIAN_POINT ( 'NONE',  ( 18.62759615963271287, -10.81492255796078972, 98.33224293864769550 ) ) ;
#126019=CARTESIAN_POINT ( 'NONE',  ( 5.049401038298161559, -19.05341960407611168, 107.7072429386476955 ) ) ;
#126020=CARTESIAN_POINT ( 'NONE',  ( 5.153800228976335163, 19.02544592524342804, 54.79057627198103120 ) ) ;
#126021=CARTESIAN_POINT ( 'NONE',  ( 9.474510206698729675, 16.51473224551082808, 87.08442372801900433 ) ) ;
#126022=CARTESIAN_POINT ( 'NONE',  ( -18.62759615963270932, 10.81492255796079327, 45.83224293864769550 ) ) ;
#126023=CARTESIAN_POINT ( 'NONE',  ( -0.05219959533937732626, 21.53943276465977519, 67.50109039468568994 ) ) ;
#126024=CARTESIAN_POINT ( 'NONE',  ( -13.97604488694527625, -13.89961937509977652, 56.87390960531434558 ) ) ;
#126025=CARTESIAN_POINT ( 'NONE',  ( 19.03943276465977164, -0.05219959533909143690, 83.74890960531436690 ) ) ;
#126026=CARTESIAN_POINT ( 'NONE',  ( -14.34966873604972548, 8.224510206698743886, 63.33442372801900433 ) ) ;
#126027=CARTESIAN_POINT ( 'NONE',  ( -18.62759615963255300, -10.81492255796106328, 49.16775706135234003 ) ) ;
#126028=CARTESIAN_POINT ( 'NONE',  ( 18.67979575497194134, -10.72451020669871369, 85.83442372801901854 ) ) ;
#126029=CARTESIAN_POINT ( 'NONE',  ( -18.67979575497178146, -10.72451020669898902, 96.66557627198102409 ) ) ;
#126030=CARTESIAN_POINT ( 'NONE',  ( 21.53943276465977519, 0.05219959533937863772, 31.25109039468568639 ) ) ;
#126031=CARTESIAN_POINT ( 'NONE',  ( -12.06949235617739369, -12.14591786802326823, 69.37609039468567573 ) ) ;
#126032=CARTESIAN_POINT ( 'NONE',  ( 18.62759615963271287, -10.81492255796078972, 58.33224293864768839 ) ) ;
#126033=CARTESIAN_POINT ( 'NONE',  ( 19.05341960407617918, -5.049401038297876454, 31.04275706135232227 ) ) ;
#126034=CARTESIAN_POINT ( 'NONE',  ( 13.97604488694527802, 13.89961937509977652, 74.37390960531436690 ) ) ;
#126035=CARTESIAN_POINT ( 'NONE',  ( -16.55341960407611168, -4.379528057220339221, 21.45724293864769550 ) ) ;
#126037=CARTESIAN_POINT ( 'NONE',  ( 5.049401038298161559, -19.05341960407611168, 107.7072429386476955 ) ) ;
#126039=CARTESIAN_POINT ( 'NONE',  ( 16.51473224551083163, -9.474510206698727899, 80.83442372801899012 ) ) ;
#126040=CARTESIAN_POINT ( 'NONE',  ( -0.05219959533907301413, -21.53943276465977519, 62.49890960531436690 ) ) ;
#126041=CARTESIAN_POINT ( 'NONE',  ( 0.05219959533910956823, 16.53943276465976808, 34.99890960531435979 ) ) ;
#126042=CARTESIAN_POINT ( 'NONE',  ( -14.29746914071037622, -8.314922557961029526, 24.16775706135235424 ) ) ;
#126043=CARTESIAN_POINT ( 'NONE',  ( 9.474510206698971260, -16.51473224551069308, 27.91557627198103120 ) ) ;
#126044=CARTESIAN_POINT ( 'NONE',  ( 5.049401038297881783, 19.05341960407617563, 112.2927570613523471 ) ) ;
#126045=CARTESIAN_POINT ( 'NONE',  ( -5.823673210054116645, -21.52544592524344225, 107.2905762719810525 ) ) ;
#126046=CARTESIAN_POINT ( 'NONE',  ( 19.02544592524334988, 5.153800228976608722, 66.45942372801899012 ) ) ;
#126047=CARTESIAN_POINT ( 'NONE',  ( -8.314922557961024197, 14.29746914071037800, 77.91775706135231871 ) ) ;
#126048=CARTESIAN_POINT ( 'NONE',  ( -0.05219959533909027116, -19.03943276465977164, 62.49890960531435979 ) ) ;
#126049=CARTESIAN_POINT ( 'NONE',  ( 16.52544592524342804, -4.483927247898539470, 78.54057627198103830 ) ) ;
#126050=CARTESIAN_POINT ( 'NONE',  ( 5.049401038298161559, -19.05341960407611168, 52.70724293864767418 ) ) ;
#126051=CARTESIAN_POINT ( 'NONE',  ( -4.483927247898539470, -16.52544592524342804, 57.29057627198103120 ) ) ;
#126054=CARTESIAN_POINT ( 'NONE',  ( 4.483927247898545687, 16.52544592524342804, 24.79057627198103120 ) ) ;
#126055=CARTESIAN_POINT ( 'NONE',  ( -9.474510206698964154, 16.51473224551069663, 70.41557627198102409 ) ) ;
#126057=CARTESIAN_POINT ( 'NONE',  ( 16.51473224551083163, -9.474510206698727899, 35.83442372801899722 ) ) ;
#126058=CARTESIAN_POINT ( 'NONE',  ( 12.06949235617739724, 12.14591786802326823, 46.87609039468568994 ) ) ;
#126059=CARTESIAN_POINT ( 'NONE',  ( -10.72451020669898014, 18.67979575497178502, 70.41557627198102409 ) ) ;
#126060=CARTESIAN_POINT ( 'NONE',  ( -13.89961937509957401, -13.97604488694547875, 19.37609039468566507 ) ) ;
#126061=CARTESIAN_POINT ( 'NONE',  ( 13.97604488694527802, 13.89961937509977652, 69.37390960531436690 ) ) ;
#126063=CARTESIAN_POINT ( 'NONE',  ( -9.474510206698964154, 16.51473224551069663, 115.4155762719810241 ) ) ;
#126064=CARTESIAN_POINT ( 'NONE',  ( -21.55341960407619339, 5.719274019375674811, 43.54275706135235424 ) ) ;
#126065=CARTESIAN_POINT ( 'NONE',  ( 4.379528057220339221, -16.55341960407611168, 112.7072429386476955 ) ) ;
#126067=CARTESIAN_POINT ( 'NONE',  ( -10.72451020669898014, 18.67979575497178502, 95.41557627198102409 ) ) ;
#126068=CARTESIAN_POINT ( 'NONE',  ( 0.05219959533909260263, 19.03943276465977164, 79.99890960531436690 ) ) ;
#126069=CARTESIAN_POINT ( 'NONE',  ( 17.97161686093722466, -5.500000000000140332, 68.49637206859166838 ) ) ;
#126070=CARTESIAN_POINT ( 'NONE',  ( 10.81492255796106328, -18.62759615963255655, 25.41775706135235779 ) ) ;
#126072=CARTESIAN_POINT ( 'NONE',  ( 16.46253265017160672, -9.564922557960803928, 88.33224293864769550 ) ) ;
#126074=CARTESIAN_POINT ( 'NONE',  ( 9.474510206698971260, -16.51473224551069308, 27.91557627198103120 ) ) ;
#126075=CARTESIAN_POINT ( 'NONE',  ( 5.153800228976615827, -19.02544592524334988, 100.2094237280190043 ) ) ;
#126077=CARTESIAN_POINT ( 'NONE',  ( 14.34966873604960469, 8.224510206698951720, 114.1655762719810383 ) ) ;
#126078=CARTESIAN_POINT ( 'NONE',  ( 18.62759615963255655, 10.81492255796105972, 81.66775706135236135 ) ) ;
#126079=CARTESIAN_POINT ( 'NONE',  ( -16.46253265017160317, 9.564922557960807481, 80.83224293864769550 ) ) ;
#126080=CARTESIAN_POINT ( 'NONE',  ( 18.62759615963255655, 10.81492255796105972, 41.66775706135235424 ) ) ;
#126081=CARTESIAN_POINT ( 'NONE',  ( 5.823673210054444382, -21.52544592524334988, 30.20942372801902565 ) ) ;
#126083=CARTESIAN_POINT ( 'NONE',  ( -16.46253265017160317, 9.564922557960807481, 85.83224293864769550 ) ) ;
#126085=CARTESIAN_POINT ( 'NONE',  ( -16.55341960407617563, 4.379528057220093196, 38.54275706135234714 ) ) ;
#126086=CARTESIAN_POINT ( 'NONE',  ( 10.72451020669898902, -18.67979575497178502, 37.91557627198102409 ) ) ;
#126087=CARTESIAN_POINT ( 'NONE',  ( -21.55341960407619339, 5.719274019375674811, 78.54275706135236135 ) ) ;
#126089=CARTESIAN_POINT ( 'NONE',  ( 5.049401038297881783, 19.05341960407617563, 112.2927570613523471 ) ) ;
#126090=CARTESIAN_POINT ( 'NONE',  ( 5.049401038298161559, -19.05341960407611168, 62.70724293864769550 ) ) ;
#126091=CARTESIAN_POINT ( 'NONE',  ( -9.474510206698964154, 16.51473224551069663, 85.41557627198102409 ) ) ;
#126092=CARTESIAN_POINT ( 'NONE',  ( 0.05219959533910956823, 16.53943276465976808, 104.9989096053143669 ) ) ;
#126093=CARTESIAN_POINT ( 'NONE',  ( -14.34966873604960291, -8.224510206698953496, 111.6655762719810525 ) ) ;
#126094=CARTESIAN_POINT ( 'NONE',  ( -19.03943276465977164, 0.05219959533909376836, 116.2489096053143669 ) ) ;
#126095=CARTESIAN_POINT ( 'NONE',  ( -14.29746914071037622, -8.314922557961029526, 79.16775706135234714 ) ) ;
#126096=CARTESIAN_POINT ( 'NONE',  ( 12.06949235617757843, -12.14591786802309237, 53.12390960531436690 ) ) ;
#126098=CARTESIAN_POINT ( 'NONE',  ( -0.05219959533909027116, -19.03943276465977164, 57.49890960531435979 ) ) ;
#126099=CARTESIAN_POINT ( 'NONE',  ( -5.823673210054431948, 21.52544592524334988, 82.70942372801900433 ) ) ;
#126100=CARTESIAN_POINT ( 'NONE',  ( -15.72974639402176322, -15.80617190586768395, 69.37609039468567573 ) ) ;
#126101=CARTESIAN_POINT ( 'NONE',  ( 9.474510206698729675, 16.51473224551082808, 107.0844237280190043 ) ) ;
#126102=CARTESIAN_POINT ( 'NONE',  ( -4.483927247898539470, -16.52544592524342804, 67.29057627198103830 ) ) ;
#126103=CARTESIAN_POINT ( 'NONE',  ( -18.62759615963270932, 10.81492255796079327, 115.8322429386477097 ) ) ;
#126104=CARTESIAN_POINT ( 'NONE',  ( -18.67979575497178146, -10.72451020669898902, 66.66557627198102409 ) ) ;
#126107=CARTESIAN_POINT ( 'NONE',  ( -5.049401038298153566, 19.05341960407611168, 70.20724293864769550 ) ) ;
#126108=CARTESIAN_POINT ( 'NONE',  ( -16.55341960407611168, -4.379528057220339221, 31.45724293864769550 ) ) ;
#126110=CARTESIAN_POINT ( 'NONE',  ( -14.34966873604960291, -8.224510206698953496, 21.66557627198102409 ) ) ;
#126111=CARTESIAN_POINT ( 'NONE',  ( -0.05219959533934338120, 16.53943276465976808, 97.50109039468567573 ) ) ;
#126112=CARTESIAN_POINT ( 'NONE',  ( 0.05219959533936267826, -19.03943276465977164, 55.00109039468566863 ) ) ;
#126113=CARTESIAN_POINT ( 'NONE',  ( 16.38665767535053419, 7.295008042176043261, 47.23599135785458003 ) ) ;
#126114=CARTESIAN_POINT ( 'NONE',  ( -19.03943276465977164, 0.05219959533909376836, 86.24890960531436690 ) ) ;
#126115=CARTESIAN_POINT ( 'NONE',  ( -16.52544592524342804, 4.483927247898546575, 61.04057627198103120 ) ) ;
#126116=CARTESIAN_POINT ( 'NONE',  ( 16.31925111598458855, -7.325300261831530158, 102.6642453896725726 ) ) ;
#126117=CARTESIAN_POINT ( 'NONE',  ( -19.05341960407611168, -5.049401038298163336, 111.4572429386476671 ) ) ;
#126118=CARTESIAN_POINT ( 'NONE',  ( 21.52544592524344225, -5.823673210054117533, 58.54057627198103120 ) ) ;
#126120=CARTESIAN_POINT ( 'NONE',  ( 12.06949235617757843, -12.14591786802309237, 93.12390960531436690 ) ) ;
#126121=CARTESIAN_POINT ( 'NONE',  ( -16.52544592524335698, -4.483927247898792601, 53.95942372801900433 ) ) ;
#126122=CARTESIAN_POINT ( 'NONE',  ( -0.05219959533910754901, -16.53943276465976808, 82.49890960531436690 ) ) ;
#126124=CARTESIAN_POINT ( 'NONE',  ( -13.97604488694547697, 13.89961937509957934, 78.12609039468567573 ) ) ;
#126125=CARTESIAN_POINT ( 'NONE',  ( -0.05219959533907301413, -21.53943276465977519, 22.49890960531436335 ) ) ;
#126127=CARTESIAN_POINT ( 'NONE',  ( 19.50973618000807619, 5.499999999999992895, 102.5000000000000142 ) ) ;
#126128=CARTESIAN_POINT ( 'NONE',  ( -14.29746914071037622, -8.314922557961029526, 44.16775706135234714 ) ) ;
#126129=CARTESIAN_POINT ( 'NONE',  ( -16.55341960407611168, -4.379528057220339221, 26.45724293864768839 ) ) ;
#126130=CARTESIAN_POINT ( 'NONE',  ( 10.72451020669898902, -18.67979575497178502, 57.91557627198103120 ) ) ;
#126131=CARTESIAN_POINT ( 'NONE',  ( -5.153800228976607833, 19.02544592524334988, 87.70942372801897591 ) ) ;
#126132=CARTESIAN_POINT ( 'NONE',  ( 21.55341960407610458, 5.719274019375980345, 43.95724293864769550 ) ) ;
#126133=CARTESIAN_POINT ( 'NONE',  ( 10.72451020669871369, 18.67979575497193778, 77.08442372801901854 ) ) ;
#126135=CARTESIAN_POINT ( 'NONE',  ( -8.314922557961024197, 14.29746914071037800, 32.91775706135234714 ) ) ;
#126136=CARTESIAN_POINT ( 'NONE',  ( 16.46253265017160672, -9.564922557960803928, 43.33224293864769550 ) ) ;
#126137=CARTESIAN_POINT ( 'NONE',  ( 16.51473224551069308, 9.474510206698969483, 89.16557627198103830 ) ) ;
#126138=CARTESIAN_POINT ( 'NONE',  ( 5.049401038298161559, -19.05341960407611168, 37.70724293864768839 ) ) ;
#126139=CARTESIAN_POINT ( 'NONE',  ( 0.05219959533910956823, 16.53943276465976808, 99.99890960531436690 ) ) ;
#126140=CARTESIAN_POINT ( 'NONE',  ( -9.564922557960796823, -16.46253265017161027, 107.0822429386476955 ) ) ;
#126141=EDGE_LOOP ( 'NONE', ( #148019, #145902, #13503, #42593, #196530, #85473, #797, #161563 ) ) ;
#126142=CARTESIAN_POINT ( 'NONE',  ( 12.14591786802327356, -12.06949235617739191, 55.62609039468568284 ) ) ;
#126143=CARTESIAN_POINT ( 'NONE',  ( -15.80617190586745835, -15.72974639402198527, 86.87390960531438111 ) ) ;
#126144=CARTESIAN_POINT ( 'NONE',  ( -5.049401038298153566, 19.05341960407611168, 40.20724293864768839 ) ) ;
#126145=CARTESIAN_POINT ( 'NONE',  ( 21.55341960407619695, -5.719274019375665929, 31.04275706135234714 ) ) ;
#126146=CARTESIAN_POINT ( 'NONE',  ( -5.153800228976328057, -19.02544592524343514, 77.29057627198099567 ) ) ;
#126149=CARTESIAN_POINT ( 'NONE',  ( 14.29746914071037800, 8.314922557961029526, 31.66775706135234358 ) ) ;
#126150=CARTESIAN_POINT ( 'NONE',  ( -0.05219959533907301413, -21.53943276465977519, 112.4989096053143669 ) ) ;
#126151=CARTESIAN_POINT ( 'NONE',  ( 16.52544592524342804, -4.483927247898539470, 113.5405762719810383 ) ) ;
#126152=CARTESIAN_POINT ( 'NONE',  ( 19.05341960407611168, 5.049401038298154454, 93.95724293864769550 ) ) ;
#126153=CARTESIAN_POINT ( 'NONE',  ( 0.05219959533936267826, -19.03943276465977164, 75.00109039468566152 ) ) ;
#126154=CARTESIAN_POINT ( 'NONE',  ( 9.474510206698729675, 16.51473224551082808, 27.08442372801900433 ) ) ;
#126155=CARTESIAN_POINT ( 'NONE',  ( -21.53943276465977519, 0.05219959533907696930, 81.24890960531436690 ) ) ;
#126156=CARTESIAN_POINT ( 'NONE',  ( -9.474510206698720793, -16.51473224551083518, 24.58442372801900078 ) ) ;
#126157=CARTESIAN_POINT ( 'NONE',  ( -12.06949235617739369, -12.14591786802326823, 84.37609039468570415 ) ) ;
#126158=CARTESIAN_POINT ( 'NONE',  ( -13.89961937509977652, 13.97604488694528158, 105.6239096053143527 ) ) ;
#126160=CARTESIAN_POINT ( 'NONE',  ( 16.51473224551069308, 9.474510206698969483, 39.16557627198103120 ) ) ;
#126161=CARTESIAN_POINT ( 'NONE',  ( 5.719274019375673035, 21.55341960407619339, 57.29275706135234714 ) ) ;
#126162=CARTESIAN_POINT ( 'NONE',  ( 21.55341960407619695, -5.719274019375665929, 71.04275706135234714 ) ) ;
#126163=CARTESIAN_POINT ( 'NONE',  ( -19.03943276465977164, 0.05219959533909376836, 76.24890960531435269 ) ) ;
#126164=CARTESIAN_POINT ( 'NONE',  ( 21.53943276465977519, 0.05219959533937863772, 51.25109039468568994 ) ) ;
#126165=CARTESIAN_POINT ( 'NONE',  ( -13.89961937509957401, -13.97604488694547875, 94.37609039468566152 ) ) ;
#126166=CARTESIAN_POINT ( 'NONE',  ( 19.03943276465977164, -0.05219959533909143690, 58.74890960531435979 ) ) ;
#126167=CARTESIAN_POINT ( 'NONE',  ( 19.05341960407611168, 5.049401038298154454, 93.95724293864769550 ) ) ;
#126168=CARTESIAN_POINT ( 'NONE',  ( 13.89961937509977652, -13.97604488694527269, 68.12390960531436690 ) ) ;
#126169=CARTESIAN_POINT ( 'NONE',  ( -0.05219959533909027116, -19.03943276465977164, 112.4989096053143669 ) ) ;
#126170=CARTESIAN_POINT ( 'NONE',  ( -19.03943276465977164, 0.05219959533909376836, 56.24890960531435979 ) ) ;
#126171=CARTESIAN_POINT ( 'NONE',  ( 10.72451020669898902, -18.67979575497178502, 82.91557627198103830 ) ) ;
#126172=CARTESIAN_POINT ( 'NONE',  ( -16.55341960407617563, 4.379528057220093196, 68.54275706135234714 ) ) ;
#126174=CARTESIAN_POINT ( 'NONE',  ( 9.474510206698729675, 16.51473224551082808, 32.08442372801900433 ) ) ;
#126175=CARTESIAN_POINT ( 'NONE',  ( -9.564922557960796823, -16.46253265017161027, 62.08224293864769550 ) ) ;
#126176=CARTESIAN_POINT ( 'NONE',  ( 8.314922557960818139, 14.29746914071049879, 59.58224293864770260 ) ) ;
#126177=CARTESIAN_POINT ( 'NONE',  ( -16.55341960407611168, -4.379528057220339221, 91.45724293864769550 ) ) ;
#126178=CARTESIAN_POINT ( 'NONE',  ( 19.05341960407611168, 5.049401038298154454, 98.95724293864766707 ) ) ;
#126179=CARTESIAN_POINT ( 'NONE',  ( -5.049401038298153566, 19.05341960407611168, 90.20724293864766707 ) ) ;
#126180=CARTESIAN_POINT ( 'NONE',  ( -10.72451020669870658, -18.67979575497194134, 44.58442372801901854 ) ) ;
#126181=CARTESIAN_POINT ( 'NONE',  ( -19.05341960407611168, -5.049401038298163336, 101.4572429386476955 ) ) ;
#126182=CARTESIAN_POINT ( 'NONE',  ( 13.97604488694548053, -13.89961937509957401, 20.62609039468567573 ) ) ;
#126183=CARTESIAN_POINT ( 'NONE',  ( -4.379528057220086978, -16.55341960407618274, 79.79275706135236135 ) ) ;
#126184=CARTESIAN_POINT ( 'NONE',  ( -18.62759615963255300, -10.81492255796106328, 44.16775706135234714 ) ) ;
#126185=CARTESIAN_POINT ( 'NONE',  ( 10.81492255796078972, 18.62759615963270932, 24.58224293864768839 ) ) ;
#126186=CARTESIAN_POINT ( 'NONE',  ( 10.81492255796078972, 18.62759615963270932, 104.5822429386477097 ) ) ;
#126187=CARTESIAN_POINT ( 'NONE',  ( 4.483927247898545687, 16.52544592524342804, 54.79057627198104541 ) ) ;
#126188=CARTESIAN_POINT ( 'NONE',  ( -13.89961937509977652, 13.97604488694528158, 60.62390960531436690 ) ) ;
#126189=CARTESIAN_POINT ( 'NONE',  ( -8.314922557960811034, -14.29746914071050412, 82.08224293864768129 ) ) ;
#126190=CARTESIAN_POINT ( 'NONE',  ( 15.72974639402199770, -15.80617190586745480, 38.12390960531436690 ) ) ;
#126191=CARTESIAN_POINT ( 'NONE',  ( 9.474510206698729675, 16.51473224551082808, 42.08442372801900433 ) ) ;
#126192=CARTESIAN_POINT ( 'NONE',  ( 16.53943276465976808, -0.05219959533910856209, 113.7489096053143527 ) ) ;
#126193=ORIENTED_EDGE ( 'NONE', *, *, #148621, .F. ) ;
#126194=CARTESIAN_POINT ( 'NONE',  ( -4.483927247898782831, 16.52544592524335698, 72.70942372801901854 ) ) ;
#126195=CARTESIAN_POINT ( 'NONE',  ( -19.05341960407611168, -5.049401038298163336, 71.45724293864766707 ) ) ;
#126197=CARTESIAN_POINT ( 'NONE',  ( 8.224510206698953496, -14.34966873604960469, 92.91557627198103830 ) ) ;
#126198=CARTESIAN_POINT ( 'NONE',  ( -21.55341960407610458, -5.719274019375992779, 41.45724293864769550 ) ) ;
#126199=CARTESIAN_POINT ( 'NONE',  ( -8.224510206698735004, -14.34966873604973081, 104.5844237280190185 ) ) ;
#126200=CARTESIAN_POINT ( 'NONE',  ( 19.02544592524334988, 5.153800228976608722, 111.4594237280190043 ) ) ;
#126201=CARTESIAN_POINT ( 'NONE',  ( -5.719274019375665041, -21.55341960407619695, 79.79275706135236135 ) ) ;
#126202=CARTESIAN_POINT ( 'NONE',  ( -13.97604488694527625, -13.89961937509977652, 86.87390960531436690 ) ) ;
#126203=CARTESIAN_POINT ( 'NONE',  ( 10.81492255796078972, 18.62759615963270932, 104.5822429386477097 ) ) ;
#126204=CARTESIAN_POINT ( 'NONE',  ( 16.55341960407618274, -4.379528057220086978, 56.04275706135235424 ) ) ;
#126205=CARTESIAN_POINT ( 'NONE',  ( -5.049401038298153566, 19.05341960407611168, 30.20724293864768839 ) ) ;
#126206=CARTESIAN_POINT ( 'NONE',  ( 16.55341960407618274, -4.379528057220086978, 36.04275706135234714 ) ) ;
#126207=CARTESIAN_POINT ( 'NONE',  ( 5.049401038297881783, 19.05341960407617563, 97.29275706135233293 ) ) ;
#126208=CARTESIAN_POINT ( 'NONE',  ( 15.72974639402199770, -15.80617190586745480, 88.12390960531436690 ) ) ;
#126209=CARTESIAN_POINT ( 'NONE',  ( -16.51473224551082808, 9.474510206698731452, 58.33442372801900433 ) ) ;
#126211=CARTESIAN_POINT ( 'NONE',  ( 5.719274019375991003, -21.55341960407610458, 102.7072429386476955 ) ) ;
#126213=CARTESIAN_POINT ( 'NONE',  ( -19.05341960407611168, -5.049401038298163336, 81.45724293864769550 ) ) ;
#126214=CARTESIAN_POINT ( 'NONE',  ( -16.53943276465976808, -0.05219959533934237506, 38.75109039468567573 ) ) ;
#126216=CARTESIAN_POINT ( 'NONE',  ( 19.02544592524334988, 5.153800228976608722, 61.45942372801900433 ) ) ;
#126217=CARTESIAN_POINT ( 'NONE',  ( 5.823673210054444382, -21.52544592524334988, 20.20942372801900788 ) ) ;
#126218=CARTESIAN_POINT ( 'NONE',  ( -4.483927247898539470, -16.52544592524342804, 67.29057627198103830 ) ) ;
#126219=CARTESIAN_POINT ( 'NONE',  ( -9.474510206698964154, 16.51473224551069663, 70.41557627198102409 ) ) ;
#126220=CARTESIAN_POINT ( 'NONE',  ( -16.55341960407617563, 4.379528057220093196, 38.54275706135234714 ) ) ;
#126221=CARTESIAN_POINT ( 'NONE',  ( 13.97604488694548053, -13.89961937509957401, 40.62609039468564731 ) ) ;
#126222=CARTESIAN_POINT ( 'NONE',  ( 21.55341960407619695, -5.719274019375665929, 51.04275706135234714 ) ) ;
#126223=CARTESIAN_POINT ( 'NONE',  ( -19.02544592524334988, -5.153800228976617603, 103.9594237280190043 ) ) ;
#126224=CARTESIAN_POINT ( 'NONE',  ( 0.05219959533909260263, 19.03943276465977164, 49.99890960531435979 ) ) ;
#126226=CARTESIAN_POINT ( 'NONE',  ( -5.049401038297874678, -19.05341960407617918, 79.79275706135233293 ) ) ;
#126227=CARTESIAN_POINT ( 'NONE',  ( 5.823673210054444382, -21.52544592524334988, 90.20942372801903275 ) ) ;
#126228=CARTESIAN_POINT ( 'NONE',  ( 0.05219959533936267826, -19.03943276465977164, 70.00109039468566152 ) ) ;
#126229=CARTESIAN_POINT ( 'NONE',  ( 13.97604488694527802, 13.89961937509977652, 34.37390960531436690 ) ) ;
#126230=CARTESIAN_POINT ( 'NONE',  ( -18.62759615963270932, 10.81492255796079327, 65.83224293864769550 ) ) ;
#126231=CARTESIAN_POINT ( 'NONE',  ( 12.14591786802309770, 12.06949235617756955, 59.37390960531436690 ) ) ;
#126232=CARTESIAN_POINT ( 'NONE',  ( -19.05341960407617563, 5.049401038297882671, 68.54275706135230450 ) ) ;
#126234=CARTESIAN_POINT ( 'NONE',  ( -13.89961937509957401, -13.97604488694547875, 24.37609039468565442 ) ) ;
#126235=CARTESIAN_POINT ( 'NONE',  ( -4.483927247898782831, 16.52544592524335698, 92.70942372801901854 ) ) ;
#126236=CARTESIAN_POINT ( 'NONE',  ( -8.224510206698948167, 14.34966873604960824, 50.41557627198103120 ) ) ;
#126237=CARTESIAN_POINT ( 'NONE',  ( -10.81492255796105439, 18.62759615963255655, 82.91775706135234714 ) ) ;
#126239=CARTESIAN_POINT ( 'NONE',  ( 21.53943276465977519, -0.05219959533907433946, 93.74890960531436690 ) ) ;
#126240=CARTESIAN_POINT ( 'NONE',  ( -0.05219959533909027116, -19.03943276465977164, 47.49890960531435979 ) ) ;
#126241=CARTESIAN_POINT ( 'NONE',  ( -21.53943276465977519, -0.05219959533937600094, 68.75109039468568994 ) ) ;
#126242=CARTESIAN_POINT ( 'NONE',  ( 19.02544592524343514, -5.153800228976328945, 53.54057627198102409 ) ) ;
#126243=CARTESIAN_POINT ( 'NONE',  ( 16.46253265017160672, -9.564922557960803928, 68.33224293864770971 ) ) ;
#126244=CARTESIAN_POINT ( 'NONE',  ( -8.314922557960811034, -14.29746914071050412, 107.0822429386476955 ) ) ;
#126245=CARTESIAN_POINT ( 'NONE',  ( 19.05341960407611168, 5.049401038298154454, 108.9572429386477097 ) ) ;
#126246=CARTESIAN_POINT ( 'NONE',  ( -16.53943276465976808, 0.05219959533911058130, 51.24890960531436690 ) ) ;
#126247=CARTESIAN_POINT ( 'NONE',  ( -19.05341960407611168, -5.049401038298163336, 31.45724293864769550 ) ) ;
#126248=CARTESIAN_POINT ( 'NONE',  ( -8.224510206698948167, 14.34966873604960824, 85.41557627198102409 ) ) ;
#126249=CARTESIAN_POINT ( 'NONE',  ( -15.72974639402197994, 15.80617190586746368, 90.62390960531436690 ) ) ;
#126250=CARTESIAN_POINT ( 'NONE',  ( 18.67979575497194134, -10.72451020669871369, 40.83442372801901854 ) ) ;
#126251=CARTESIAN_POINT ( 'NONE',  ( -9.564922557960796823, -16.46253265017161027, 22.08224293864768839 ) ) ;
#126252=CARTESIAN_POINT ( 'NONE',  ( 12.06949235617739724, 12.14591786802326823, 56.87609039468568994 ) ) ;
#126253=CARTESIAN_POINT ( 'NONE',  ( -21.55341960407610458, -5.719274019375992779, 81.45724293864769550 ) ) ;
#126254=CARTESIAN_POINT ( 'NONE',  ( -10.72451020669870658, -18.67979575497194134, 109.5844237280190328 ) ) ;
#126255=CARTESIAN_POINT ( 'NONE',  ( 5.153800228976335163, 19.02544592524342804, 89.79057627198102409 ) ) ;
#126256=CARTESIAN_POINT ( 'NONE',  ( 21.55341960407619695, -5.719274019375665929, 46.04275706135234714 ) ) ;
#126257=CARTESIAN_POINT ( 'NONE',  ( 21.52544592524344225, -5.823673210054117533, 33.54057627198102409 ) ) ;
#126258=CARTESIAN_POINT ( 'NONE',  ( -4.379528057220086978, -16.55341960407618274, 109.7927570613523613 ) ) ;
#126259=CARTESIAN_POINT ( 'NONE',  ( -21.55341960407619339, 5.719274019375674811, 53.54275706135234714 ) ) ;
#126260=CARTESIAN_POINT ( 'NONE',  ( 10.81492255796106328, -18.62759615963255655, 80.41775706135234714 ) ) ;
#126261=CARTESIAN_POINT ( 'NONE',  ( 5.049401038297881783, 19.05341960407617563, 32.29275706135233293 ) ) ;
#126262=CARTESIAN_POINT ( 'NONE',  ( -8.224510206698735004, -14.34966873604973081, 89.58442372801901854 ) ) ;
#126263=CARTESIAN_POINT ( 'NONE',  ( 10.72451020669871369, 18.67979575497193778, 47.08442372801901854 ) ) ;
#126264=CARTESIAN_POINT ( 'NONE',  ( -5.153800228976328057, -19.02544592524343514, 42.29057627198101699 ) ) ;
#126265=CARTESIAN_POINT ( 'NONE',  ( 21.52544592524334988, 5.823673210054432836, 106.4594237280190328 ) ) ;
#126266=CARTESIAN_POINT ( 'NONE',  ( 5.153800228976335163, 19.02544592524342804, 109.7905762719810099 ) ) ;
#126267=CARTESIAN_POINT ( 'NONE',  ( 21.53943276465977519, -0.05219959533907433946, 113.7489096053143527 ) ) ;
#126268=CARTESIAN_POINT ( 'NONE',  ( -5.719274019375978568, 21.55341960407610458, 80.20724293864769550 ) ) ;
#126270=CARTESIAN_POINT ( 'NONE',  ( -10.81492255796078084, -18.62759615963271287, 67.08224293864770971 ) ) ;
#126271=CARTESIAN_POINT ( 'NONE',  ( 8.224510206698742110, 14.34966873604972548, 52.08442372801901854 ) ) ;
#126272=CARTESIAN_POINT ( 'NONE',  ( -14.29746914071049879, 8.314922557960819915, 65.83224293864769550 ) ) ;
#126274=CARTESIAN_POINT ( 'NONE',  ( -9.474510206698720793, -16.51473224551083518, 84.58442372801900433 ) ) ;
#126276=CARTESIAN_POINT ( 'NONE',  ( 12.06949235617739724, 12.14591786802326823, 21.87609039468567573 ) ) ;
#126277=CARTESIAN_POINT ( 'NONE',  ( -21.55341960407610458, -5.719274019375992779, 96.45724293864770971 ) ) ;
#126278=CARTESIAN_POINT ( 'NONE',  ( 21.55341960407610458, 5.719274019375980345, 68.95724293864769550 ) ) ;
#126279=CARTESIAN_POINT ( 'NONE',  ( -19.03943276465977164, 0.05219959533909376836, 116.2489096053143669 ) ) ;
#126280=CARTESIAN_POINT ( 'NONE',  ( -12.14591786802326823, 12.06949235617739902, 58.12609039468568994 ) ) ;
#126281=CARTESIAN_POINT ( 'NONE',  ( 16.46253265017160672, -9.564922557960803928, 73.33224293864769550 ) ) ;
#126282=CARTESIAN_POINT ( 'NONE',  ( -10.72451020669870658, -18.67979575497194134, 49.58442372801901143 ) ) ;
#126283=CARTESIAN_POINT ( 'NONE',  ( -13.89961937509957401, -13.97604488694547875, 109.3760903946856331 ) ) ;
#126284=CARTESIAN_POINT ( 'NONE',  ( 19.02544592524343514, -5.153800228976328945, 113.5405762719810241 ) ) ;
#126285=CARTESIAN_POINT ( 'NONE',  ( 9.474510206698971260, -16.51473224551069308, 102.9155762719810241 ) ) ;
#126286=CARTESIAN_POINT ( 'NONE',  ( 18.62759615963271287, -10.81492255796078972, 108.3322429386477097 ) ) ;
#126287=CARTESIAN_POINT ( 'NONE',  ( -13.89961937509977652, 13.97604488694528158, 65.62390960531436690 ) ) ;
#126288=CARTESIAN_POINT ( 'NONE',  ( -16.19135201231369692, 7.376712067591784994, 24.81319145947970028 ) ) ;
#126289=CARTESIAN_POINT ( 'NONE',  ( 14.34966873604960469, 8.224510206698951720, 79.16557627198103830 ) ) ;
#126290=CARTESIAN_POINT ( 'NONE',  ( 5.823673210054125526, 21.52544592524343514, 24.79057627198103120 ) ) ;
#126291=CARTESIAN_POINT ( 'NONE',  ( -17.26058549869089376, 6.457015423128611431, 33.62254162523932166 ) ) ;
#126292=CARTESIAN_POINT ( 'NONE',  ( -0.05219959533907301413, -21.53943276465977519, 102.4989096053143811 ) ) ;
#126293=CARTESIAN_POINT ( 'NONE',  ( 0.05219959533936267826, -19.03943276465977164, 70.00109039468566152 ) ) ;
#126294=CARTESIAN_POINT ( 'NONE',  ( 13.89961937509977652, -13.97604488694527269, 108.1239096053143669 ) ) ;
#126295=CARTESIAN_POINT ( 'NONE',  ( 16.46253265017160672, -9.564922557960803928, 33.33224293864770260 ) ) ;
#126296=CARTESIAN_POINT ( 'NONE',  ( 15.80617190586746368, 15.72974639402197994, 54.37390960531435979 ) ) ;
#126297=CARTESIAN_POINT ( 'NONE',  ( -19.02544592524342804, 5.153800228976336051, 101.0405762719810241 ) ) ;
#126298=CARTESIAN_POINT ( 'NONE',  ( -15.80617190586768217, 15.72974639402176855, 73.12609039468567573 ) ) ;
#126299=CARTESIAN_POINT ( 'NONE',  ( 9.474510206698971260, -16.51473224551069308, 52.91557627198102409 ) ) ;
#126300=EDGE_CURVE ( 'NONE', #103535, #134048, #196709, .T. ) ;
#126301=CARTESIAN_POINT ( 'NONE',  ( 4.379528057220339221, -16.55341960407611168, 92.70724293864770971 ) ) ;
#126302=CARTESIAN_POINT ( 'NONE',  ( -0.05219959533934338120, 16.53943276465976808, 42.50109039468567573 ) ) ;
#126303=CARTESIAN_POINT ( 'NONE',  ( 10.81492255796106328, -18.62759615963255655, 70.41775706135236135 ) ) ;
#126305=CARTESIAN_POINT ( 'NONE',  ( -13.89961937509957401, -13.97604488694547875, 29.37609039468565797 ) ) ;
#126306=CARTESIAN_POINT ( 'NONE',  ( -9.564922557961040184, 16.46253265017147172, 82.91775706135233293 ) ) ;
#126307=CARTESIAN_POINT ( 'NONE',  ( -9.564922557961040184, 16.46253265017147172, 42.91775706135234003 ) ) ;
#126309=CARTESIAN_POINT ( 'NONE',  ( -15.72974639402176322, -15.80617190586768395, 34.37609039468568284 ) ) ;
#126311=CARTESIAN_POINT ( 'NONE',  ( -5.153800228976607833, 19.02544592524334988, 37.70942372801899722 ) ) ;
#126312=CARTESIAN_POINT ( 'NONE',  ( 5.153800228976335163, 19.02544592524342804, 69.79057627198103830 ) ) ;
#126313=CARTESIAN_POINT ( 'NONE',  ( -8.314922557960811034, -14.29746914071050412, 22.08224293864769194 ) ) ;
#126314=CARTESIAN_POINT ( 'NONE',  ( -13.89961937509977652, 13.97604488694528158, 110.6239096053143243 ) ) ;
#126315=CARTESIAN_POINT ( 'NONE',  ( 5.719274019375673035, 21.55341960407619339, 82.29275706135234714 ) ) ;
#126318=CARTESIAN_POINT ( 'NONE',  ( -10.72451020669870658, -18.67979575497194134, 79.58442372801903275 ) ) ;
#126319=CARTESIAN_POINT ( 'NONE',  ( 17.44279575226823198, -5.990770900252458731, 43.33557567514318976 ) ) ;
#126320=CARTESIAN_POINT ( 'NONE',  ( -5.049401038298153566, 19.05341960407611168, 95.20724293864770971 ) ) ;
#126322=CARTESIAN_POINT ( 'NONE',  ( -19.02544592524342804, 5.153800228976336051, 56.04057627198100988 ) ) ;
#126323=CARTESIAN_POINT ( 'NONE',  ( 0.05219959533907565091, 21.53943276465977519, 59.99890960531436690 ) ) ;
#126324=CARTESIAN_POINT ( 'NONE',  ( -14.34966873604960291, -8.224510206698953496, 26.66557627198103475 ) ) ;
#126325=CARTESIAN_POINT ( 'NONE',  ( -16.53943276465976808, 0.05219959533911058130, 116.2489096053143669 ) ) ;
#126326=CARTESIAN_POINT ( 'NONE',  ( -13.89961937509977652, 13.97604488694528158, 100.6239096053143669 ) ) ;
#126327=CARTESIAN_POINT ( 'NONE',  ( -16.46253265017146816, -9.564922557961047289, 24.16775706135233648 ) ) ;
#126328=CARTESIAN_POINT ( 'NONE',  ( 12.06949235617757843, -12.14591786802309237, 103.1239096053143811 ) ) ;
#126329=CARTESIAN_POINT ( 'NONE',  ( -10.81492255796105439, 18.62759615963255655, 57.91775706135234714 ) ) ;
#126330=CARTESIAN_POINT ( 'NONE',  ( 13.97604488694527802, 13.89961937509977652, 114.3739096053143669 ) ) ;
#126331=CARTESIAN_POINT ( 'NONE',  ( 0.05219959533934541429, -16.53943276465976808, 110.0010903946856757 ) ) ;
#126332=CARTESIAN_POINT ( 'NONE',  ( -19.02544592524334988, -5.153800228976617603, 63.95942372801899012 ) ) ;
#126333=DIRECTION ( 'NONE',  ( 0.000000000000000000, 0.000000000000000000, -1.000000000000000000 ) ) ;
#126334=CARTESIAN_POINT ( 'NONE',  ( 19.05341960407611168, 5.049401038298154454, 113.9572429386477097 ) ) ;
#126335=CARTESIAN_POINT ( 'NONE',  ( -12.06949235617756955, 12.14591786802309770, 70.62390960531436690 ) ) ;
#126336=CARTESIAN_POINT ( 'NONE',  ( 5.049401038297881783, 19.05341960407617563, 62.29275706135234003 ) ) ;
#126337=CARTESIAN_POINT ( 'NONE',  ( 19.03943276465977164, -0.05219959533909143690, 58.74890960531435979 ) ) ;
#126338=CARTESIAN_POINT ( 'NONE',  ( -12.06949235617756955, 12.14591786802309770, 55.62390960531436690 ) ) ;
#126339=CARTESIAN_POINT ( 'NONE',  ( 13.97604488694548053, -13.89961937509957401, 90.62609039468567573 ) ) ;
#126340=CARTESIAN_POINT ( 'NONE',  ( -18.67979575497178146, -10.72451020669898902, 36.66557627198103120 ) ) ;
#126342=CARTESIAN_POINT ( 'NONE',  ( -14.29746914071049879, 8.314922557960819915, 105.8322429386476955 ) ) ;
#126343=CARTESIAN_POINT ( 'NONE',  ( -13.89961937509957401, -13.97604488694547697, 99.37609039468567573 ) ) ;
#126344=CARTESIAN_POINT ( 'NONE',  ( 13.97604488694527802, 13.89961937509977652, 64.37390960531436690 ) ) ;
#126345=CARTESIAN_POINT ( 'NONE',  ( -10.72451020669898014, 18.67979575497178502, 60.41557627198102409 ) ) ;
#126346=CARTESIAN_POINT ( 'NONE',  ( -19.05341960407611168, -5.049401038298163336, 46.45724293864768129 ) ) ;
#126347=CARTESIAN_POINT ( 'NONE',  ( -12.06949235617739369, -12.14591786802326823, 89.37609039468568994 ) ) ;
#126348=CARTESIAN_POINT ( 'NONE',  ( -5.153800228976328057, -19.02544592524343514, 72.29057627198102409 ) ) ;
#126349=CARTESIAN_POINT ( 'NONE',  ( -13.89961937509957401, -13.97604488694547875, 49.37609039468567573 ) ) ;
#126350=CARTESIAN_POINT ( 'NONE',  ( 5.719274019375673035, 21.55341960407619339, 82.29275706135234714 ) ) ;
#126351=CARTESIAN_POINT ( 'NONE',  ( 21.55341960407610458, 5.719274019375980345, 48.95724293864770971 ) ) ;
#126352=CARTESIAN_POINT ( 'NONE',  ( 19.02544592524343514, -5.153800228976328945, 108.5405762719810383 ) ) ;
#126353=CARTESIAN_POINT ( 'NONE',  ( -0.05219959533909027116, -19.03943276465977164, 42.49890960531435269 ) ) ;
#126354=CARTESIAN_POINT ( 'NONE',  ( 16.53943276465976808, 0.05219959533934440121, 86.25109039468568994 ) ) ;
#126355=CARTESIAN_POINT ( 'NONE',  ( -13.97604488694547697, 13.89961937509957934, 108.1260903946856331 ) ) ;
#126356=CARTESIAN_POINT ( 'NONE',  ( 19.02544592524343514, -5.153800228976328945, 23.54057627198102054 ) ) ;
#126357=CARTESIAN_POINT ( 'NONE',  ( 18.87255363501903815, 5.499999999999945821, 78.82513748171830059 ) ) ;
#126358=CARTESIAN_POINT ( 'NONE',  ( -0.05219959533937732626, 21.53943276465977519, 92.50109039468567573 ) ) ;
#126359=EDGE_LOOP ( 'NONE', ( #72861, #197250, #90130, #11023 ) ) ;
#126360=CARTESIAN_POINT ( 'NONE',  ( -16.52544592524342804, 4.483927247898546575, 61.04057627198103120 ) ) ;
#126361=CARTESIAN_POINT ( 'NONE',  ( 16.53943276465976808, -0.05219959533910856209, 68.74890960531435269 ) ) ;
#126362=CARTESIAN_POINT ( 'NONE',  ( -21.52544592524343514, 5.823673210054127303, 96.04057627198102409 ) ) ;
#126363=CARTESIAN_POINT ( 'NONE',  ( 21.53943276465977519, -0.05219959533907433946, 83.74890960531435269 ) ) ;
#126365=CARTESIAN_POINT ( 'NONE',  ( 18.67979575497178502, 10.72451020669898547, 44.16557627198103120 ) ) ;
#126366=CARTESIAN_POINT ( 'NONE',  ( 14.34966873604972726, -8.224510206698740333, 60.83442372801901854 ) ) ;
#126367=CARTESIAN_POINT ( 'NONE',  ( -14.34966873604960291, -8.224510206698953496, 86.66557627198102409 ) ) ;
#126368=CARTESIAN_POINT ( 'NONE',  ( -19.05341960407611168, -5.049401038298163336, 41.45724293864769550 ) ) ;
#126370=CARTESIAN_POINT ( 'NONE',  ( 8.314922557961029526, -14.29746914071037800, 100.4177570613523471 ) ) ;
#126371=CARTESIAN_POINT ( 'NONE',  ( -15.80617190586768217, 15.72974639402176855, 33.12609039468569705 ) ) ;
#126372=CARTESIAN_POINT ( 'NONE',  ( 16.51473224551069308, 9.474510206698969483, 89.16557627198103830 ) ) ;
#126373=CARTESIAN_POINT ( 'NONE',  ( 15.72974639402176855, 15.80617190586768217, 66.87609039468568994 ) ) ;
#126374=CARTESIAN_POINT ( 'NONE',  ( -19.05341960407611168, -5.049401038298163336, 21.45724293864768839 ) ) ;
#126375=CARTESIAN_POINT ( 'NONE',  ( -9.564922557960796823, -16.46253265017161027, 27.08224293864769550 ) ) ;
#126377=CARTESIAN_POINT ( 'NONE',  ( -21.52544592524334988, -5.823673210054445271, 58.95942372801902565 ) ) ;
#126378=CARTESIAN_POINT ( 'NONE',  ( 19.03943276465977164, -0.05219959533909143690, 33.74890960531435979 ) ) ;
#126379=CARTESIAN_POINT ( 'NONE',  ( -0.05219959533909027116, -19.03943276465977164, 112.4989096053143669 ) ) ;
#126380=CARTESIAN_POINT ( 'NONE',  ( 9.474510206698971260, -16.51473224551069308, 87.91557627198102409 ) ) ;
#126381=CARTESIAN_POINT ( 'NONE',  ( -13.89961937509957401, -13.97604488694547875, 64.37609039468567573 ) ) ;
#126382=CARTESIAN_POINT ( 'NONE',  ( -0.05219959533937732626, 21.53943276465977519, 27.50109039468567929 ) ) ;
#126383=CARTESIAN_POINT ( 'NONE',  ( -19.05341960407617563, 5.049401038297882671, 53.54275706135231871 ) ) ;
#126384=CARTESIAN_POINT ( 'NONE',  ( 13.89961937509977652, -13.97604488694527269, 33.12390960531434558 ) ) ;
#126385=CARTESIAN_POINT ( 'NONE',  ( -16.52544592524335698, -4.483927247898792601, 108.9594237280190185 ) ) ;
#126386=CARTESIAN_POINT ( 'NONE',  ( -5.153800228976607833, 19.02544592524334988, 77.70942372801900433 ) ) ;
#126387=CARTESIAN_POINT ( 'NONE',  ( 12.14591786802309770, 12.06949235617756955, 29.37390960531435269 ) ) ;
#126388=CARTESIAN_POINT ( 'NONE',  ( 9.564922557961047289, -16.46253265017146816, 55.41775706135234003 ) ) ;
#126389=CARTESIAN_POINT ( 'NONE',  ( 9.474510206698971260, -16.51473224551069308, 102.9155762719810241 ) ) ;
#126390=CARTESIAN_POINT ( 'NONE',  ( -21.55341960407619339, 5.719274019375674811, 103.5427570613523613 ) ) ;
#126391=CARTESIAN_POINT ( 'NONE',  ( -21.55341960407619339, 5.719274019375674811, 113.5427570613523756 ) ) ;
#126392=CARTESIAN_POINT ( 'NONE',  ( -9.564922557960796823, -16.46253265017161027, 22.08224293864768839 ) ) ;
#126393=CARTESIAN_POINT ( 'NONE',  ( 5.823673210054444382, -21.52544592524334988, 90.20942372801903275 ) ) ;
#126394=CARTESIAN_POINT ( 'NONE',  ( 8.224510206698742110, 14.34966873604972548, 32.08442372801901854 ) ) ;
#126395=CARTESIAN_POINT ( 'NONE',  ( -5.049401038298153566, 19.05341960407611168, 90.20724293864766707 ) ) ;
#126398=CARTESIAN_POINT ( 'NONE',  ( 13.89961937509977652, -13.97604488694527269, 78.12390960531433848 ) ) ;
#126400=CARTESIAN_POINT ( 'NONE',  ( 19.02544592524334988, 5.153800228976608722, 76.45942372801897591 ) ) ;
#126401=CARTESIAN_POINT ( 'NONE',  ( 19.02544592524343514, -5.153800228976328945, 103.5405762719809957 ) ) ;
#126402=CARTESIAN_POINT ( 'NONE',  ( 18.67979575497194134, -10.72451020669871369, 100.8344237280190185 ) ) ;
#126403=CARTESIAN_POINT ( 'NONE',  ( 14.34966873604960469, 8.224510206698951720, 94.16557627198103830 ) ) ;
#126404=CARTESIAN_POINT ( 'NONE',  ( 15.80617190586746368, 15.72974639402197994, 44.37390960531435979 ) ) ;
#126405=CARTESIAN_POINT ( 'NONE',  ( -5.719274019375978568, 21.55341960407610458, 30.20724293864769550 ) ) ;
#126406=CARTESIAN_POINT ( 'NONE',  ( 8.314922557960818139, 14.29746914071049879, 104.5822429386477097 ) ) ;
#126407=CARTESIAN_POINT ( 'NONE',  ( 18.22780087662126647, 5.499999999999818812, 46.48236817873107185 ) ) ;
#126408=CARTESIAN_POINT ( 'NONE',  ( -0.05219959533936034679, 19.03943276465977164, 62.50109039468566863 ) ) ;
#126409=CARTESIAN_POINT ( 'NONE',  ( -8.224510206698948167, 14.34966873604960824, 25.41557627198103120 ) ) ;
#126410=CARTESIAN_POINT ( 'NONE',  ( 19.03943276465977164, -0.05219959533909143690, 98.74890960531436690 ) ) ;
#126411=CARTESIAN_POINT ( 'NONE',  ( -21.53943276465977519, -0.05219959533937600094, 83.75109039468568994 ) ) ;
#126412=CARTESIAN_POINT ( 'NONE',  ( 10.72451020669898902, -18.67979575497178502, 72.91557627198103830 ) ) ;
#126413=CARTESIAN_POINT ( 'NONE',  ( -10.72451020669870658, -18.67979575497194134, 39.58442372801901143 ) ) ;
#126414=CARTESIAN_POINT ( 'NONE',  ( -15.80617190586745835, -15.72974639402198527, 91.87390960531436690 ) ) ;
#126415=CARTESIAN_POINT ( 'NONE',  ( -21.55341960407619339, 5.719274019375674811, 48.54275706135234714 ) ) ;
#126416=CARTESIAN_POINT ( 'NONE',  ( -9.564922557960796823, -16.46253265017161027, 32.08224293864769550 ) ) ;
#126417=CARTESIAN_POINT ( 'NONE',  ( -16.51473224551069308, -9.474510206698971260, 86.66557627198102409 ) ) ;
#126418=CARTESIAN_POINT ( 'NONE',  ( 4.379528057220092307, 16.55341960407617563, 82.29275706135234714 ) ) ;
#126419=CARTESIAN_POINT ( 'NONE',  ( -4.483927247898539470, -16.52544592524342804, 102.2905762719810383 ) ) ;
#126420=CARTESIAN_POINT ( 'NONE',  ( 19.03943276465977164, -0.05219959533909143690, 103.7489096053143669 ) ) ;
#126421=CARTESIAN_POINT ( 'NONE',  ( 12.06949235617757843, -12.14591786802309237, 58.12390960531435979 ) ) ;
#126422=CARTESIAN_POINT ( 'NONE',  ( -14.34966873604960291, -8.224510206698953496, 21.66557627198102409 ) ) ;
#126423=CARTESIAN_POINT ( 'NONE',  ( -9.564922557960796823, -16.46253265017161027, 57.08224293864769550 ) ) ;
#126424=CARTESIAN_POINT ( 'NONE',  ( -9.564922557960796823, -16.46253265017161027, 37.08224293864768839 ) ) ;
#126425=CARTESIAN_POINT ( 'NONE',  ( -5.719274019375978568, 21.55341960407610458, 40.20724293864769550 ) ) ;
#126426=EDGE_CURVE ( 'NONE', #169038, #114713, #85007, .T. ) ;
#126427=CARTESIAN_POINT ( 'NONE',  ( -9.564922557961040184, 16.46253265017147172, 27.91775706135232582 ) ) ;
#126429=CARTESIAN_POINT ( 'NONE',  ( -14.34966873604960291, -8.224510206698953496, 36.66557627198103120 ) ) ;
#126430=CARTESIAN_POINT ( 'NONE',  ( 5.719274019375673035, 21.55341960407619339, 47.29275706135234003 ) ) ;
#126432=CARTESIAN_POINT ( 'NONE',  ( -12.14591786802326823, 12.06949235617739902, 53.12609039468568284 ) ) ;
#126433=CARTESIAN_POINT ( 'NONE',  ( 9.564922557961047289, -16.46253265017146816, 55.41775706135234003 ) ) ;
#126434=CARTESIAN_POINT ( 'NONE',  ( 8.314922557960818139, 14.29746914071049879, 24.58224293864768839 ) ) ;
#126435=CARTESIAN_POINT ( 'NONE',  ( 16.52216118717208104, -7.221426719304427699, 51.42400978953011759 ) ) ;
#126436=CARTESIAN_POINT ( 'NONE',  ( 16.55341960407618274, -4.379528057220086978, 111.0427570613523613 ) ) ;
#126437=CARTESIAN_POINT ( 'NONE',  ( 5.153800228976335163, 19.02544592524342804, 34.79057627198102409 ) ) ;
#126438=CARTESIAN_POINT ( 'NONE',  ( -16.51473224551069308, -9.474510206698971260, 66.66557627198102409 ) ) ;
#126439=CARTESIAN_POINT ( 'NONE',  ( -16.46253265017160317, 9.564922557960807481, 25.83224293864769194 ) ) ;
#126440=CARTESIAN_POINT ( 'NONE',  ( -5.823673210054431948, 21.52544592524334988, 37.70942372801900433 ) ) ;
#126441=CARTESIAN_POINT ( 'NONE',  ( 0.05219959533909260263, 19.03943276465977164, 44.99890960531435979 ) ) ;
#126442=CARTESIAN_POINT ( 'NONE',  ( -19.02544592524342804, 5.153800228976336051, 116.0405762719810383 ) ) ;
#126443=CARTESIAN_POINT ( 'NONE',  ( -5.153800228976328057, -19.02544592524343514, 52.29057627198100988 ) ) ;
#126444=CARTESIAN_POINT ( 'NONE',  ( -10.81492255796078084, -18.62759615963271287, 22.08224293864769194 ) ) ;
#126445=CARTESIAN_POINT ( 'NONE',  ( -15.80617190586768217, 15.72974639402176855, 53.12609039468568284 ) ) ;
#126446=CARTESIAN_POINT ( 'NONE',  ( 12.14591786802309770, 12.06949235617756955, 109.3739096053143811 ) ) ;
#126447=CARTESIAN_POINT ( 'NONE',  ( 0.05219959533907565091, 21.53943276465977519, 24.99890960531435624 ) ) ;
#126448=CARTESIAN_POINT ( 'NONE',  ( 16.52544592524335698, 4.483927247898782831, 71.45942372801901854 ) ) ;
#126449=CARTESIAN_POINT ( 'NONE',  ( -21.55341960407619339, 5.719274019375674811, 93.54275706135234714 ) ) ;
#126450=CARTESIAN_POINT ( 'NONE',  ( -12.06949235617739369, -12.14591786802326823, 49.37609039468569705 ) ) ;
#126451=CARTESIAN_POINT ( 'NONE',  ( 13.97604488694527802, 13.89961937509977652, 89.37390960531436690 ) ) ;
#126452=CARTESIAN_POINT ( 'NONE',  ( 8.224510206698742110, 14.34966873604972548, 42.08442372801901854 ) ) ;
#126453=CARTESIAN_POINT ( 'NONE',  ( -14.34966873604972548, 8.224510206698743886, 23.33442372801901499 ) ) ;
#126454=CARTESIAN_POINT ( 'NONE',  ( -16.55341960407617563, 4.379528057220093196, 98.54275706135234714 ) ) ;
#126455=CARTESIAN_POINT ( 'NONE',  ( 15.72974639402176855, 15.80617190586768217, 51.87609039468568284 ) ) ;
#126456=CARTESIAN_POINT ( 'NONE',  ( 16.51473224551083163, -9.474510206698727899, 100.8344237280190043 ) ) ;
#126457=CARTESIAN_POINT ( 'NONE',  ( -5.719274019375978568, 21.55341960407610458, 110.2072429386477239 ) ) ;
#126458=CARTESIAN_POINT ( 'NONE',  ( -0.05219959533910754901, -16.53943276465976808, 97.49890960531436690 ) ) ;
#126459=CARTESIAN_POINT ( 'NONE',  ( -9.474510206698720793, -16.51473224551083518, 104.5844237280190043 ) ) ;
#126460=CARTESIAN_POINT ( 'NONE',  ( -8.224510206698735004, -14.34966873604973081, 69.58442372801900433 ) ) ;
#126462=CARTESIAN_POINT ( 'NONE',  ( -5.153800228976607833, 19.02544592524334988, 82.70942372801897591 ) ) ;
#126463=CARTESIAN_POINT ( 'NONE',  ( 16.55341960407611168, 4.379528057220329451, 48.95724293864770971 ) ) ;
#126464=CARTESIAN_POINT ( 'NONE',  ( 14.29746914071049879, -8.314922557960816363, 43.33224293864769550 ) ) ;
#126465=CARTESIAN_POINT ( 'NONE',  ( 4.483927247898545687, 16.52544592524342804, 94.79057627198105251 ) ) ;
#126466=CARTESIAN_POINT ( 'NONE',  ( -19.02544592524334988, -5.153800228976617603, 38.95942372801900433 ) ) ;
#126468=CARTESIAN_POINT ( 'NONE',  ( 21.52544592524334988, 5.823673210054432836, 36.45942372801901143 ) ) ;
#126469=CARTESIAN_POINT ( 'NONE',  ( 9.564922557961047289, -16.46253265017146816, 100.4177570613523329 ) ) ;
#126471=CARTESIAN_POINT ( 'NONE',  ( 13.89961937509977652, -13.97604488694527269, 88.12390960531438111 ) ) ;
#126472=CARTESIAN_POINT ( 'NONE',  ( -13.89961937509977652, 13.97604488694528158, 90.62390960531432427 ) ) ;
#126473=CARTESIAN_POINT ( 'NONE',  ( -18.67979575497178146, -10.72451020669898902, 51.66557627198102409 ) ) ;
#126474=CARTESIAN_POINT ( 'NONE',  ( 16.52544592524342804, -4.483927247898539470, 93.54057627198103830 ) ) ;
#126475=CARTESIAN_POINT ( 'NONE',  ( -16.51473224551069308, -9.474510206698971260, 71.66557627198102409 ) ) ;
#126476=CARTESIAN_POINT ( 'NONE',  ( -5.049401038298153566, 19.05341960407611168, 35.20724293864768839 ) ) ;
#126477=CARTESIAN_POINT ( 'NONE',  ( -21.55341960407619339, 5.719274019375674811, 38.54275706135234714 ) ) ;
#126478=CARTESIAN_POINT ( 'NONE',  ( -18.62759615963255300, -10.81492255796106328, 69.16775706135234714 ) ) ;
#126479=CARTESIAN_POINT ( 'NONE',  ( 8.224510206698742110, 14.34966873604972548, 87.08442372801901854 ) ) ;
#126481=CARTESIAN_POINT ( 'NONE',  ( -5.823673210054431948, 21.52544592524334988, 32.70942372801900433 ) ) ;
#126482=CARTESIAN_POINT ( 'NONE',  ( 18.62759615963255655, 10.81492255796105972, 21.66775706135235069 ) ) ;
#126483=CARTESIAN_POINT ( 'NONE',  ( -16.46253265017146816, -9.564922557961047289, 54.16775706135234003 ) ) ;
#126484=CARTESIAN_POINT ( 'NONE',  ( 19.05341960407611168, 5.049401038298154454, 78.95724293864769550 ) ) ;
#126485=CARTESIAN_POINT ( 'NONE',  ( -5.719274019375665041, -21.55341960407619695, 84.79275706135234714 ) ) ;
#126486=CARTESIAN_POINT ( 'NONE',  ( 18.67979575497178502, 10.72451020669898547, 79.16557627198103830 ) ) ;
#126487=CARTESIAN_POINT ( 'NONE',  ( -8.224510206698948167, 14.34966873604960824, 50.41557627198103120 ) ) ;
#126488=CARTESIAN_POINT ( 'NONE',  ( 5.719274019375673035, 21.55341960407619339, 102.2927570613523613 ) ) ;
#126489=CARTESIAN_POINT ( 'NONE',  ( 0.05219959533936267826, -19.03943276465977164, 30.00109039468566863 ) ) ;
#126490=CARTESIAN_POINT ( 'NONE',  ( 14.34966873604960469, 8.224510206698951720, 69.16557627198102409 ) ) ;
#126491=CARTESIAN_POINT ( 'NONE',  ( 8.224510206698953496, -14.34966873604960469, 112.9155762719810383 ) ) ;
#126492=CARTESIAN_POINT ( 'NONE',  ( 13.97604488694548053, -13.89961937509957401, 70.62609039468567573 ) ) ;
#126493=CARTESIAN_POINT ( 'NONE',  ( -12.06949235617756955, 12.14591786802309770, 40.62390960531435269 ) ) ;
#126494=CARTESIAN_POINT ( 'NONE',  ( -5.823673210054431948, 21.52544592524334988, 77.70942372801900433 ) ) ;
#126495=CARTESIAN_POINT ( 'NONE',  ( -5.153800228976328057, -19.02544592524343514, 77.29057627198099567 ) ) ;
#126496=CARTESIAN_POINT ( 'NONE',  ( -9.564922557961040184, 16.46253265017147172, 67.91775706135233293 ) ) ;
#126497=CARTESIAN_POINT ( 'NONE',  ( 5.823673210054125526, 21.52544592524343514, 64.79057627198103830 ) ) ;
#126498=CARTESIAN_POINT ( 'NONE',  ( 10.81492255796078972, 18.62759615963270932, 114.5822429386477097 ) ) ;
#126499=CARTESIAN_POINT ( 'NONE',  ( -9.564922557961040184, 16.46253265017147172, 107.9177570613523471 ) ) ;
#126500=CARTESIAN_POINT ( 'NONE',  ( 8.224510206698742110, 14.34966873604972548, 77.08442372801901854 ) ) ;
#126501=CARTESIAN_POINT ( 'NONE',  ( 16.62475595723694965, 7.163666690055258357, 61.97286648189533764 ) ) ;
#126502=CARTESIAN_POINT ( 'NONE',  ( 18.62759615963271287, -10.81492255796078972, 113.3322429386476955 ) ) ;
#126503=CARTESIAN_POINT ( 'NONE',  ( 16.53943276465976808, -0.05219959533910856209, 98.74890960531438111 ) ) ;
#126504=CARTESIAN_POINT ( 'NONE',  ( -17.49999999999998934, -3.512728167237066046, 29.77190004818872282 ) ) ;
#126505=CARTESIAN_POINT ( 'NONE',  ( 4.483927247898790824, -16.52544592524335698, 30.20942372801902565 ) ) ;
#126506=CARTESIAN_POINT ( 'NONE',  ( -5.823673210054116645, -21.52544592524344225, 67.29057627198103830 ) ) ;
#126507=CARTESIAN_POINT ( 'NONE',  ( -14.34966873604972548, 8.224510206698743886, 98.33442372801901854 ) ) ;
#126508=CARTESIAN_POINT ( 'NONE',  ( -16.51473224551069308, -9.474510206698971260, 36.66557627198102409 ) ) ;
#126509=CARTESIAN_POINT ( 'NONE',  ( -16.55341960407617563, 4.379528057220093196, 68.54275706135234714 ) ) ;
#126510=CARTESIAN_POINT ( 'NONE',  ( 5.153800228976615827, -19.02544592524334988, 55.20942372801899722 ) ) ;
#126511=CARTESIAN_POINT ( 'NONE',  ( 15.80617190586769283, -15.72974639402175789, 45.62609039468567573 ) ) ;
#126512=CARTESIAN_POINT ( 'NONE',  ( 5.719274019375991003, -21.55341960407610458, 57.70724293864770260 ) ) ;
#126513=CARTESIAN_POINT ( 'NONE',  ( 12.14591786802327356, -12.06949235617739191, 100.6260903946857184 ) ) ;
#126514=CARTESIAN_POINT ( 'NONE',  ( -21.53943276465977519, -0.05219959533937600094, 88.75109039468567573 ) ) ;
#126515=CARTESIAN_POINT ( 'NONE',  ( 21.53943276465977519, -0.05219959533907433946, 48.74890960531435979 ) ) ;
#126516=CARTESIAN_POINT ( 'NONE',  ( 10.81492255796078972, 18.62759615963270932, 44.58224293864769550 ) ) ;
#126517=CARTESIAN_POINT ( 'NONE',  ( -16.52544592524335698, -4.483927247898792601, 83.95942372801900433 ) ) ;
#126518=CARTESIAN_POINT ( 'NONE',  ( -10.72451020669898014, 18.67979575497178502, 40.41557627198103120 ) ) ;
#126519=ORIENTED_EDGE ( 'NONE', *, *, #182922, .F. ) ;
#126520=CARTESIAN_POINT ( 'NONE',  ( -9.564922557960796823, -16.46253265017161027, 102.0822429386477097 ) ) ;
#126522=CARTESIAN_POINT ( 'NONE',  ( 9.474510206698971260, -16.51473224551069308, 32.91557627198102409 ) ) ;
#126523=CARTESIAN_POINT ( 'NONE',  ( 10.81492255796078972, 18.62759615963270932, 59.58224293864770260 ) ) ;
#126524=CARTESIAN_POINT ( 'NONE',  ( -8.224510206698735004, -14.34966873604973081, 89.58442372801901854 ) ) ;
#126525=CARTESIAN_POINT ( 'NONE',  ( 5.823673210054444382, -21.52544592524334988, 50.20942372801901854 ) ) ;
#126526=CARTESIAN_POINT ( 'NONE',  ( 5.153800228976615827, -19.02544592524334988, 105.2094237280190185 ) ) ;
#126527=CARTESIAN_POINT ( 'NONE',  ( 14.29746914071049879, -8.314922557960816363, 98.33224293864769550 ) ) ;
#126528=CARTESIAN_POINT ( 'NONE',  ( 4.379528057220092307, 16.55341960407617563, 22.29275706135235069 ) ) ;
#126529=CARTESIAN_POINT ( 'NONE',  ( 5.049401038298161559, -19.05341960407611168, 37.70724293864768839 ) ) ;
#126531=CARTESIAN_POINT ( 'NONE',  ( 5.049401038298161559, -19.05341960407611168, 97.70724293864766707 ) ) ;
#126532=CARTESIAN_POINT ( 'NONE',  ( -8.314922557961024197, 14.29746914071037800, 72.91775706135234714 ) ) ;
#126533=CARTESIAN_POINT ( 'NONE',  ( 18.67979575497194134, -10.72451020669871369, 110.8344237280190043 ) ) ;
#126534=CARTESIAN_POINT ( 'NONE',  ( -0.05219959533907301413, -21.53943276465977519, 62.49890960531436690 ) ) ;
#126535=CARTESIAN_POINT ( 'NONE',  ( -8.314922557961024197, 14.29746914071037800, 92.91775706135236135 ) ) ;
#126536=CARTESIAN_POINT ( 'NONE',  ( 16.51473224551083163, -9.474510206698727899, 85.83442372801900433 ) ) ;
#126537=CARTESIAN_POINT ( 'NONE',  ( -16.46253265017160317, 9.564922557960807481, 40.83224293864769550 ) ) ;
#126538=CARTESIAN_POINT ( 'NONE',  ( -19.02544592524342804, 5.153800228976336051, 76.04057627198102409 ) ) ;
#126539=CARTESIAN_POINT ( 'NONE',  ( 16.51473224551069308, 9.474510206698969483, 29.16557627198103475 ) ) ;
#126540=CARTESIAN_POINT ( 'NONE',  ( 5.153800228976615827, -19.02544592524334988, 75.20942372801896170 ) ) ;
#126542=CARTESIAN_POINT ( 'NONE',  ( -9.474510206698964154, 16.51473224551069663, 115.4155762719810241 ) ) ;
#126543=CARTESIAN_POINT ( 'NONE',  ( 4.379528057220339221, -16.55341960407611168, 62.70724293864769550 ) ) ;
#126544=CARTESIAN_POINT ( 'NONE',  ( 18.67979575497178502, 10.72451020669898547, 59.16557627198103120 ) ) ;
#126545=CARTESIAN_POINT ( 'NONE',  ( -17.49999999999999645, 5.499999999999997335, 105.7969038253417153 ) ) ;
#126546=CARTESIAN_POINT ( 'NONE',  ( -16.46253265017146816, -9.564922557961047289, 29.16775706135232937 ) ) ;
#126548=CARTESIAN_POINT ( 'NONE',  ( 16.51473224551069308, 9.474510206698969483, 64.16557627198102409 ) ) ;
#126549=CARTESIAN_POINT ( 'NONE',  ( -5.049401038298153566, 19.05341960407611168, 75.20724293864769550 ) ) ;
#126550=CARTESIAN_POINT ( 'NONE',  ( 12.14591786802327356, -12.06949235617739191, 50.62609039468568994 ) ) ;
#126553=CARTESIAN_POINT ( 'NONE',  ( -8.314922557961024197, 14.29746914071037800, 72.91775706135234714 ) ) ;
#126555=CARTESIAN_POINT ( 'NONE',  ( 12.14591786802327356, -12.06949235617739191, 60.62609039468567573 ) ) ;
#126556=CARTESIAN_POINT ( 'NONE',  ( 8.314922557961029526, -14.29746914071037800, 35.41775706135234003 ) ) ;
#126557=CARTESIAN_POINT ( 'NONE',  ( -16.51473224551069308, -9.474510206698971260, 61.66557627198103120 ) ) ;
#126559=CARTESIAN_POINT ( 'NONE',  ( 21.53943276465977519, 0.05219959533937863772, 51.25109039468568994 ) ) ;
#126560=CARTESIAN_POINT ( 'NONE',  ( -5.049401038297874678, -19.05341960407617918, 59.79275706135231871 ) ) ;
#126561=CARTESIAN_POINT ( 'NONE',  ( 5.719274019375673035, 21.55341960407619339, 107.2927570613523471 ) ) ;
#126562=CARTESIAN_POINT ( 'NONE',  ( -13.97604488694527625, -13.89961937509977652, 36.87390960531436690 ) ) ;
#126563=CARTESIAN_POINT ( 'NONE',  ( 16.49949742642548856, 7.238363427225953828, 23.55948828841231446 ) ) ;
#126564=CARTESIAN_POINT ( 'NONE',  ( 15.72974639402199770, -15.80617190586745480, 53.12390960531436690 ) ) ;
#126565=CARTESIAN_POINT ( 'NONE',  ( 5.049401038298161559, -19.05341960407611168, 102.7072429386476955 ) ) ;
#126566=CARTESIAN_POINT ( 'NONE',  ( -12.14591786802309592, -12.06949235617757132, 101.8739096053143811 ) ) ;
#126567=CARTESIAN_POINT ( 'NONE',  ( -14.34966873604972548, 8.224510206698743886, 43.33442372801901143 ) ) ;
#126568=CARTESIAN_POINT ( 'NONE',  ( 0.05219959533910956823, 16.53943276465976808, 24.99890960531435624 ) ) ;
#126570=CARTESIAN_POINT ( 'NONE',  ( 0.05219959533907565091, 21.53943276465977519, 104.9989096053143669 ) ) ;
#126571=CARTESIAN_POINT ( 'NONE',  ( 14.34966873604960469, 8.224510206698951720, 44.16557627198103120 ) ) ;
#126573=CARTESIAN_POINT ( 'NONE',  ( -5.049401038297874678, -19.05341960407617918, 89.79275706135230450 ) ) ;
#126574=CARTESIAN_POINT ( 'NONE',  ( -16.51473224551082808, 9.474510206698731452, 23.33442372801900078 ) ) ;
#126575=CARTESIAN_POINT ( 'NONE',  ( -8.314922557960811034, -14.29746914071050412, 27.08224293864769550 ) ) ;
#126576=CARTESIAN_POINT ( 'NONE',  ( 0.05219959533907565091, 21.53943276465977519, 99.99890960531436690 ) ) ;
#126577=CARTESIAN_POINT ( 'NONE',  ( 10.81492255796078972, 18.62759615963270932, 49.58224293864769550 ) ) ;
#126578=CARTESIAN_POINT ( 'NONE',  ( -19.05341960407611168, -5.049401038298163336, 81.45724293864769550 ) ) ;
#126579=CARTESIAN_POINT ( 'NONE',  ( 8.224510206698953496, -14.34966873604960469, 37.91557627198102409 ) ) ;
#126580=CARTESIAN_POINT ( 'NONE',  ( -13.97604488694527625, -13.89961937509977652, 96.87390960531433848 ) ) ;
#126581=CARTESIAN_POINT ( 'NONE',  ( 18.22780087662121673, 5.500000000000056843, 78.98459894673892734 ) ) ;
#126582=CARTESIAN_POINT ( 'NONE',  ( 0.05219959533936267826, -19.03943276465977164, 35.00109039468566863 ) ) ;
#126583=CARTESIAN_POINT ( 'NONE',  ( -21.55341960407610458, -5.719274019375992779, 76.45724293864769550 ) ) ;
#126584=CARTESIAN_POINT ( 'NONE',  ( 16.52544592524342804, -4.483927247898539470, 103.5405762719810383 ) ) ;
#126585=CARTESIAN_POINT ( 'NONE',  ( 18.67979575497194134, -10.72451020669871369, 30.83442372801902209 ) ) ;
#126587=CARTESIAN_POINT ( 'NONE',  ( 8.314922557961029526, -14.29746914071037800, 110.4177570613523756 ) ) ;
#126588=CARTESIAN_POINT ( 'NONE',  ( 0.05219959533909260263, 19.03943276465977164, 39.99890960531436690 ) ) ;
#126589=CARTESIAN_POINT ( 'NONE',  ( 13.89961937509977652, -13.97604488694527269, 88.12390960531438111 ) ) ;
#126591=CARTESIAN_POINT ( 'NONE',  ( 13.97604488694527802, 13.89961937509977652, 34.37390960531436690 ) ) ;
#126592=CARTESIAN_POINT ( 'NONE',  ( -12.06949235617756955, 12.14591786802309770, 45.62390960531436690 ) ) ;
#126593=CARTESIAN_POINT ( 'NONE',  ( 5.823673210054444382, -21.52544592524334988, 75.20942372801901854 ) ) ;
#126595=CARTESIAN_POINT ( 'NONE',  ( -14.34966873604972548, 8.224510206698743886, 68.33442372801900433 ) ) ;
#126596=CARTESIAN_POINT ( 'NONE',  ( -19.03943276465977164, 0.05219959533909376836, 56.24890960531435979 ) ) ;
#126597=CARTESIAN_POINT ( 'NONE',  ( -5.153800228976328057, -19.02544592524343514, 62.29057627198100988 ) ) ;
#126599=CARTESIAN_POINT ( 'NONE',  ( 5.719274019375673035, 21.55341960407619339, 112.2927570613523471 ) ) ;
#126600=CARTESIAN_POINT ( 'NONE',  ( -16.52544592524335698, -4.483927247898792601, 68.95942372801901854 ) ) ;
#126601=CARTESIAN_POINT ( 'NONE',  ( 15.80617190586769283, -15.72974639402175789, 100.6260903946857184 ) ) ;
#126602=CARTESIAN_POINT ( 'NONE',  ( 19.02544592524343514, -5.153800228976328945, 58.54057627198102409 ) ) ;
#126603=CARTESIAN_POINT ( 'NONE',  ( -5.823673210054116645, -21.52544592524344225, 32.29057627198102409 ) ) ;
#126604=CARTESIAN_POINT ( 'NONE',  ( 16.46253265017146816, 9.564922557961045513, 111.6677570613523329 ) ) ;
#126605=CARTESIAN_POINT ( 'NONE',  ( -18.62759615963255300, -10.81492255796106328, 64.16775706135234714 ) ) ;
#126606=CARTESIAN_POINT ( 'NONE',  ( 12.06949235617739724, 12.14591786802326823, 46.87609039468568994 ) ) ;
#126607=CARTESIAN_POINT ( 'NONE',  ( -21.52544592524343514, 5.823673210054127303, 101.0405762719810383 ) ) ;
#126608=CARTESIAN_POINT ( 'NONE',  ( 9.474510206698729675, 16.51473224551082808, 97.08442372801900433 ) ) ;
#126609=CARTESIAN_POINT ( 'NONE',  ( 0.05219959533909260263, 19.03943276465977164, 79.99890960531436690 ) ) ;
#126610=CARTESIAN_POINT ( 'NONE',  ( 5.049401038297881783, 19.05341960407617563, 107.2927570613523187 ) ) ;
#126611=CARTESIAN_POINT ( 'NONE',  ( -19.05341960407617563, 5.049401038297882671, 113.5427570613523471 ) ) ;
#126612=CARTESIAN_POINT ( 'NONE',  ( -4.379528057220328563, 16.55341960407611168, 60.20724293864768839 ) ) ;
#126613=CARTESIAN_POINT ( 'NONE',  ( 4.483927247898790824, -16.52544592524335698, 70.20942372801904696 ) ) ;
#126614=CARTESIAN_POINT ( 'NONE',  ( 21.52544592524334988, 5.823673210054432836, 21.45942372801901499 ) ) ;
#126615=CARTESIAN_POINT ( 'NONE',  ( 0.05219959533909260263, 19.03943276465977164, 54.99890960531435979 ) ) ;
#126616=CARTESIAN_POINT ( 'NONE',  ( 19.03943276465977164, -0.05219959533909143690, 73.74890960531435269 ) ) ;
#126617=CARTESIAN_POINT ( 'NONE',  ( -16.52544592524335698, -4.483927247898792601, 68.95942372801901854 ) ) ;
#126618=EDGE_CURVE ( 'NONE', #16989, #4215, #109379, .T. ) ;
#126620=ORIENTED_EDGE ( 'NONE', *, *, #28653, .T. ) ;
#126621=CARTESIAN_POINT ( 'NONE',  ( -0.05219959533937732626, 21.53943276465977519, 112.5010903946857042 ) ) ;
#126622=CARTESIAN_POINT ( 'NONE',  ( -0.05219959533909027116, -19.03943276465977164, 42.49890960531435269 ) ) ;
#126624=CARTESIAN_POINT ( 'NONE',  ( 16.46253265017146816, 9.564922557961045513, 106.6677570613523471 ) ) ;
#126625=CARTESIAN_POINT ( 'NONE',  ( -5.049401038297874678, -19.05341960407617918, 39.79275706135232582 ) ) ;
#126626=CARTESIAN_POINT ( 'NONE',  ( -14.34966873604972548, 8.224510206698743886, 23.33442372801901499 ) ) ;
#126627=CARTESIAN_POINT ( 'NONE',  ( 9.474510206698971260, -16.51473224551069308, 47.91557627198102409 ) ) ;
#126628=CARTESIAN_POINT ( 'NONE',  ( -16.46253265017160317, 9.564922557960807481, 60.83224293864769550 ) ) ;
#126629=CARTESIAN_POINT ( 'NONE',  ( -15.72974639402197994, 15.80617190586746368, 85.62390960531436690 ) ) ;
#126631=CARTESIAN_POINT ( 'NONE',  ( -9.474510206698964154, 16.51473224551069663, 45.41557627198103120 ) ) ;
#126633=CARTESIAN_POINT ( 'NONE',  ( -19.05341960407617563, 5.049401038297882671, 93.54275706135234714 ) ) ;
#126634=CARTESIAN_POINT ( 'NONE',  ( -4.379528057220328563, 16.55341960407611168, 70.20724293864769550 ) ) ;
#126635=CARTESIAN_POINT ( 'NONE',  ( -5.049401038297874678, -19.05341960407617918, 24.79275706135233648 ) ) ;
#126636=CARTESIAN_POINT ( 'NONE',  ( 14.34966873604960469, 8.224510206698951720, 59.16557627198103120 ) ) ;
#126637=CARTESIAN_POINT ( 'NONE',  ( -21.52544592524334988, -5.823673210054445271, 83.95942372801900433 ) ) ;
#126638=CARTESIAN_POINT ( 'NONE',  ( 5.049401038298161559, -19.05341960407611168, 27.70724293864769550 ) ) ;
#126639=CARTESIAN_POINT ( 'NONE',  ( 10.72451020669871369, 18.67979575497193778, 87.08442372801901854 ) ) ;
#126640=CARTESIAN_POINT ( 'NONE',  ( 12.06949235617757843, -12.14591786802309237, 28.12390960531435979 ) ) ;
#126641=CARTESIAN_POINT ( 'NONE',  ( -15.72974639402176322, -15.80617190586768395, 79.37609039468567573 ) ) ;
#126642=CARTESIAN_POINT ( 'NONE',  ( 0.05219959533909260263, 19.03943276465977164, 84.99890960531436690 ) ) ;
#126643=CARTESIAN_POINT ( 'NONE',  ( -0.05219959533937732626, 21.53943276465977519, 37.50109039468568284 ) ) ;
#126644=CARTESIAN_POINT ( 'NONE',  ( 19.02544592524343514, -5.153800228976328945, 83.54057627198100988 ) ) ;
#126645=CARTESIAN_POINT ( 'NONE',  ( -8.314922557960811034, -14.29746914071050412, 97.08224293864770971 ) ) ;
#126646=CARTESIAN_POINT ( 'NONE',  ( 16.55341960407611168, 4.379528057220329451, 58.95724293864770971 ) ) ;
#126647=CARTESIAN_POINT ( 'NONE',  ( 0.05219959533907565091, 21.53943276465977519, 74.99890960531435269 ) ) ;
#126648=CARTESIAN_POINT ( 'NONE',  ( -5.153800228976328057, -19.02544592524343514, 72.29057627198102409 ) ) ;
#126649=CARTESIAN_POINT ( 'NONE',  ( -5.823673210054116645, -21.52544592524344225, 82.29057627198103830 ) ) ;
#126650=CARTESIAN_POINT ( 'NONE',  ( -19.02544592524334988, -5.153800228976617603, 73.95942372801900433 ) ) ;
#126651=CARTESIAN_POINT ( 'NONE',  ( -19.05341960407617918, 5.049401038297883559, 28.54275706135232937 ) ) ;
#126652=CARTESIAN_POINT ( 'NONE',  ( 14.34966873604960469, 8.224510206698951720, 79.16557627198103830 ) ) ;
#126653=CARTESIAN_POINT ( 'NONE',  ( -21.52544592524343514, 5.823673210054127303, 51.04057627198103120 ) ) ;
#126654=CARTESIAN_POINT ( 'NONE',  ( -17.49999999999999645, -5.500000000000000888, 20.00000000000000000 ) ) ;
#126655=CARTESIAN_POINT ( 'NONE',  ( 12.06949235617739724, 12.14591786802326823, 96.87609039468568994 ) ) ;
#126657=CARTESIAN_POINT ( 'NONE',  ( 13.97604488694548053, -13.89961937509957401, 100.6260903946856615 ) ) ;
#126658=CARTESIAN_POINT ( 'NONE',  ( 16.55341960407611168, 4.379528057220329451, 73.95724293864769550 ) ) ;
#126660=CARTESIAN_POINT ( 'NONE',  ( 9.474510206698971260, -16.51473224551069308, 57.91557627198103120 ) ) ;
#126661=CARTESIAN_POINT ( 'NONE',  ( 8.224510206698953496, -14.34966873604960469, 52.91557627198103830 ) ) ;
#126662=CARTESIAN_POINT ( 'NONE',  ( -16.46253265017160317, 9.564922557960807481, 95.83224293864769550 ) ) ;
#126663=CARTESIAN_POINT ( 'NONE',  ( 13.97604488694548053, -13.89961937509957401, 90.62609039468567573 ) ) ;
#126664=CARTESIAN_POINT ( 'NONE',  ( -16.51473224551069308, -9.474510206698971260, 61.66557627198103120 ) ) ;
#126665=CARTESIAN_POINT ( 'NONE',  ( -13.89961937509977652, 13.97604488694528158, 90.62390960531432427 ) ) ;
#126666=CARTESIAN_POINT ( 'NONE',  ( 0.05219959533909260263, 19.03943276465977164, 84.99890960531436690 ) ) ;
#126667=CARTESIAN_POINT ( 'NONE',  ( 0.05219959533907565091, 21.53943276465977519, 59.99890960531436690 ) ) ;
#126668=CARTESIAN_POINT ( 'NONE',  ( 14.29746914071037800, 8.314922557961029526, 61.66775706135235424 ) ) ;
#126669=CARTESIAN_POINT ( 'NONE',  ( 18.22780087662122384, 5.500000000000018652, 98.98459894673892734 ) ) ;
#126670=CARTESIAN_POINT ( 'NONE',  ( 13.89961937509977652, -13.97604488694527269, 58.12390960531436690 ) ) ;
#126671=CARTESIAN_POINT ( 'NONE',  ( -0.05219959533907301413, -21.53943276465977519, 67.49890960531436690 ) ) ;
#126672=CARTESIAN_POINT ( 'NONE',  ( -16.51473224551082808, 9.474510206698731452, 98.33442372801900433 ) ) ;
#126673=CARTESIAN_POINT ( 'NONE',  ( 16.52544592524342804, -4.483927247898539470, 28.54057627198103120 ) ) ;
#126674=CARTESIAN_POINT ( 'NONE',  ( -21.53943276465977519, -0.05219959533937600094, 43.75109039468568284 ) ) ;
#126676=CARTESIAN_POINT ( 'NONE',  ( 14.29746914071037800, 8.314922557961029526, 76.66775706135234714 ) ) ;
#126677=CARTESIAN_POINT ( 'NONE',  ( 4.483927247898790824, -16.52544592524335698, 95.20942372801903275 ) ) ;
#126679=CARTESIAN_POINT ( 'NONE',  ( 16.53943276465976808, 0.05219959533934440121, 76.25109039468568994 ) ) ;
#126680=CARTESIAN_POINT ( 'NONE',  ( 8.314922557961029526, -14.29746914071037800, 35.41775706135234003 ) ) ;
#126681=CARTESIAN_POINT ( 'NONE',  ( -13.89961937509977652, 13.97604488694528158, 50.62390960531435979 ) ) ;
#126682=CARTESIAN_POINT ( 'NONE',  ( -19.03943276465977164, 0.05219959533909376836, 51.24890960531436690 ) ) ;
#126683=CARTESIAN_POINT ( 'NONE',  ( -9.564922557960796823, -16.46253265017161027, 57.08224293864769550 ) ) ;
#126684=CARTESIAN_POINT ( 'NONE',  ( 15.72974639402176855, 15.80617190586768217, 51.87609039468568284 ) ) ;
#126685=CARTESIAN_POINT ( 'NONE',  ( 14.34966873604972726, -8.224510206698740333, 55.83442372801901854 ) ) ;
#126686=CARTESIAN_POINT ( 'NONE',  ( -8.224510206698948167, 14.34966873604960824, 25.41557627198103120 ) ) ;
#126687=CARTESIAN_POINT ( 'NONE',  ( 19.03943276465977164, -0.05219959533909143690, 28.74890960531435624 ) ) ;
#126688=CARTESIAN_POINT ( 'NONE',  ( 13.97604488694527802, 13.89961937509977652, 34.37390960531436690 ) ) ;
#126689=CARTESIAN_POINT ( 'NONE',  ( 16.55341960407618274, -4.379528057220086978, 26.04275706135235779 ) ) ;
#126690=CARTESIAN_POINT ( 'NONE',  ( -5.153800228976607833, 19.02544592524334988, 82.70942372801897591 ) ) ;
#126691=CARTESIAN_POINT ( 'NONE',  ( 12.14591786802309770, 12.06949235617756955, 89.37390960531435269 ) ) ;
#126692=CARTESIAN_POINT ( 'NONE',  ( -16.46253265017160317, 9.564922557960807481, 50.83224293864770260 ) ) ;
#126693=CARTESIAN_POINT ( 'NONE',  ( -13.97604488694547697, 13.89961937509957934, 73.12609039468568994 ) ) ;
#126694=CARTESIAN_POINT ( 'NONE',  ( 17.50000000000000000, -5.499999999999992895, 91.21769037696437010 ) ) ;
#126695=CARTESIAN_POINT ( 'NONE',  ( 21.53943276465977519, 0.05219959533937863772, 76.25109039468568994 ) ) ;
#126696=CARTESIAN_POINT ( 'NONE',  ( 12.14591786802327356, -12.06949235617739191, 50.62609039468568994 ) ) ;
#126697=CARTESIAN_POINT ( 'NONE',  ( -17.50000000000000711, 5.076555817581202668, 23.82048507950227645 ) ) ;
#126698=CARTESIAN_POINT ( 'NONE',  ( -10.81492255796078084, -18.62759615963271287, 42.08224293864769550 ) ) ;
#126699=CARTESIAN_POINT ( 'NONE',  ( -0.05219959533934338120, 16.53943276465976808, 27.50109039468567929 ) ) ;
#126700=CARTESIAN_POINT ( 'NONE',  ( 16.51473224551069308, 9.474510206698969483, 29.16557627198103475 ) ) ;
#126701=CARTESIAN_POINT ( 'NONE',  ( 5.153800228976615827, -19.02544592524334988, 30.20942372801900433 ) ) ;
#126703=CARTESIAN_POINT ( 'NONE',  ( -9.564922557960796823, -16.46253265017161027, 37.08224293864768839 ) ) ;
#126705=CARTESIAN_POINT ( 'NONE',  ( -19.02544592524342804, 5.153800228976336051, 71.04057627198099567 ) ) ;
#126706=CARTESIAN_POINT ( 'NONE',  ( -19.35543954521081744, -5.499999999999586109, 54.58901960356452321 ) ) ;
#126707=CARTESIAN_POINT ( 'NONE',  ( 10.81492255796106328, -18.62759615963255655, 110.4177570613523756 ) ) ;
#126708=CARTESIAN_POINT ( 'NONE',  ( -16.52544592524342804, 4.483927247898546575, 41.04057627198103120 ) ) ;
#126709=CARTESIAN_POINT ( 'NONE',  ( -5.153800228976328057, -19.02544592524343514, 37.29057627198102409 ) ) ;
#126711=CARTESIAN_POINT ( 'NONE',  ( 19.03943276465977164, -0.05219959533909143690, 93.74890960531435269 ) ) ;
#126712=CARTESIAN_POINT ( 'NONE',  ( 0.05219959533937995610, -21.53943276465977519, 75.00109039468568994 ) ) ;
#126713=CARTESIAN_POINT ( 'NONE',  ( -5.049401038298153566, 19.05341960407611168, 55.20724293864769550 ) ) ;
#126714=CARTESIAN_POINT ( 'NONE',  ( 15.72974639402176855, 15.80617190586768217, 61.87609039468568284 ) ) ;
#126715=CARTESIAN_POINT ( 'NONE',  ( -0.05219959533907301413, -21.53943276465977519, 27.49890960531435269 ) ) ;
#126716=CARTESIAN_POINT ( 'NONE',  ( -5.049401038298153566, 19.05341960407611168, 30.20724293864768839 ) ) ;
#126717=CARTESIAN_POINT ( 'NONE',  ( -10.72451020669870658, -18.67979575497194134, 29.58442372801901854 ) ) ;
#126718=CARTESIAN_POINT ( 'NONE',  ( 9.474510206698729675, 16.51473224551082808, 42.08442372801900433 ) ) ;
#126719=CARTESIAN_POINT ( 'NONE',  ( 0.05219959533910956823, 16.53943276465976808, 109.9989096053143527 ) ) ;
#126720=CARTESIAN_POINT ( 'NONE',  ( 16.51473224551069308, 9.474510206698969483, 69.16557627198102409 ) ) ;
#126721=CARTESIAN_POINT ( 'NONE',  ( -19.03943276465977164, -0.05219959533935918106, 108.7510903946856615 ) ) ;
#126722=CARTESIAN_POINT ( 'NONE',  ( 0.05219959533910956823, 16.53943276465976808, 79.99890960531435269 ) ) ;
#126723=CARTESIAN_POINT ( 'NONE',  ( -5.153800228976328057, -19.02544592524343514, 112.2905762719810099 ) ) ;
#126724=CARTESIAN_POINT ( 'NONE',  ( -19.02544592524334988, -5.153800228976617603, 103.9594237280190043 ) ) ;
#126725=CARTESIAN_POINT ( 'NONE',  ( 15.80617190586746368, 15.72974639402197994, 109.3739096053143811 ) ) ;
#126726=CARTESIAN_POINT ( 'NONE',  ( -0.05219959533937732626, 21.53943276465977519, 52.50109039468567573 ) ) ;
#126727=B_SPLINE_CURVE_WITH_KNOTS ( 'NONE', 3,
 ( #179094, #88048, #165908, #27406, #106200, #74882 ),
 .UNSPECIFIED., .F., .F.,
 ( 4, 2, 4 ),
 ( 0.003989672132298133049, 0.004372778065220572774, 0.004755883998143011632 ),
 .UNSPECIFIED. ) ;
#126728=CARTESIAN_POINT ( 'NONE',  ( -14.29746914071037622, -8.314922557961029526, 54.16775706135235424 ) ) ;
#126729=CARTESIAN_POINT ( 'NONE',  ( -16.53943276465976808, -0.05219959533934237506, 58.75109039468568994 ) ) ;
#126730=CARTESIAN_POINT ( 'NONE',  ( -10.72451020669898014, 18.67979575497178502, 60.41557627198102409 ) ) ;
#126731=CARTESIAN_POINT ( 'NONE',  ( 19.02544592524343514, -5.153800228976328945, 43.54057627198103120 ) ) ;
#126732=CARTESIAN_POINT ( 'NONE',  ( 4.483927247898790824, -16.52544592524335698, 75.20942372801901854 ) ) ;
#126733=CARTESIAN_POINT ( 'NONE',  ( -15.72974639402197994, 15.80617190586746368, 105.6239096053143669 ) ) ;
#126734=CARTESIAN_POINT ( 'NONE',  ( 14.34966873604960469, 8.224510206698951720, 49.16557627198102409 ) ) ;
#126735=CARTESIAN_POINT ( 'NONE',  ( -5.153800228976328057, -19.02544592524343514, 67.29057627198102409 ) ) ;
#126736=CARTESIAN_POINT ( 'NONE',  ( 4.483927247898790824, -16.52544592524335698, 80.20942372801901854 ) ) ;
#126737=CARTESIAN_POINT ( 'NONE',  ( 0.05219959533934541429, -16.53943276465976808, 25.00109039468567218 ) ) ;
#126738=CARTESIAN_POINT ( 'NONE',  ( -18.67979575497178146, -10.72451020669898902, 101.6655762719810383 ) ) ;
#126739=CARTESIAN_POINT ( 'NONE',  ( -12.06949235617756955, 12.14591786802309770, 45.62390960531436690 ) ) ;
#126742=CARTESIAN_POINT ( 'NONE',  ( -16.36317988757058828, 7.306389748694924080, 74.09789608363229263 ) ) ;
#126743=CARTESIAN_POINT ( 'NONE',  ( 15.72974639402199770, -15.80617190586745480, 83.12390960531436690 ) ) ;
#126744=CARTESIAN_POINT ( 'NONE',  ( -16.53943276465976808, -0.05219959533934237506, 113.7510903946856757 ) ) ;
#126747=CARTESIAN_POINT ( 'NONE',  ( -5.719274019375978568, 21.55341960407610458, 100.2072429386476955 ) ) ;
#126748=CARTESIAN_POINT ( 'NONE',  ( -13.89961937509977652, 13.97604488694528158, 100.6239096053143669 ) ) ;
#126749=CARTESIAN_POINT ( 'NONE',  ( -18.62759615963255300, -10.81492255796106328, 19.16775706135234714 ) ) ;
#126750=CARTESIAN_POINT ( 'NONE',  ( -14.34966873604960291, -8.224510206698953496, 41.66557627198103120 ) ) ;
#126751=CARTESIAN_POINT ( 'NONE',  ( 14.34966873604972726, -8.224510206698740333, 50.83442372801901143 ) ) ;
#126752=CARTESIAN_POINT ( 'NONE',  ( 5.049401038298161559, -19.05341960407611168, 42.70724293864767418 ) ) ;
#126753=CARTESIAN_POINT ( 'NONE',  ( 9.474510206698729675, 16.51473224551082808, 52.08442372801900433 ) ) ;
#126754=CARTESIAN_POINT ( 'NONE',  ( -19.03943276465977164, 0.05219959533909376836, 86.24890960531436690 ) ) ;
#126755=CARTESIAN_POINT ( 'NONE',  ( -10.72451020669898014, 18.67979575497178502, 30.41557627198101699 ) ) ;
#126757=CARTESIAN_POINT ( 'NONE',  ( 14.34966873604972726, -8.224510206698740333, 25.83442372801901499 ) ) ;
#126758=CARTESIAN_POINT ( 'NONE',  ( 0.05219959533936267826, -19.03943276465977164, 45.00109039468566863 ) ) ;
#126759=CARTESIAN_POINT ( 'NONE',  ( -18.67979575497178146, -10.72451020669898902, 96.66557627198102409 ) ) ;
#126760=CARTESIAN_POINT ( 'NONE',  ( 16.52544592524342804, -4.483927247898539470, 33.54057627198102409 ) ) ;
#126761=CARTESIAN_POINT ( 'NONE',  ( -13.97604488694527625, -13.89961937509977652, 76.87390960531433848 ) ) ;
#126762=CARTESIAN_POINT ( 'NONE',  ( 21.52544592524344225, -5.823673210054117533, 58.54057627198103120 ) ) ;
#126763=CARTESIAN_POINT ( 'NONE',  ( 0.05219959533907565091, 21.53943276465977519, 94.99890960531436690 ) ) ;
#126764=CARTESIAN_POINT ( 'NONE',  ( -16.55341960407617563, 4.379528057220093196, 28.54275706135234358 ) ) ;
#126765=CARTESIAN_POINT ( 'NONE',  ( -18.62759615963270932, 10.81492255796079327, 25.83224293864769194 ) ) ;
#126766=CARTESIAN_POINT ( 'NONE',  ( 15.80617190586769283, -15.72974639402175789, 90.62609039468567573 ) ) ;
#126767=CARTESIAN_POINT ( 'NONE',  ( -19.05341960407611168, -5.049401038298163336, 91.45724293864766707 ) ) ;
#126768=CARTESIAN_POINT ( 'NONE',  ( -5.153800228976328057, -19.02544592524343514, 22.29057627198102765 ) ) ;
#126769=CARTESIAN_POINT ( 'NONE',  ( 19.05341960407611168, 5.049401038298154454, 78.95724293864769550 ) ) ;
#126770=CARTESIAN_POINT ( 'NONE',  ( 8.224510206698953496, -14.34966873604960469, 102.9155762719810383 ) ) ;
#126771=CARTESIAN_POINT ( 'NONE',  ( -19.05341960407611168, -5.049401038298163336, 66.45724293864769550 ) ) ;
#126772=CARTESIAN_POINT ( 'NONE',  ( -14.34966873604972548, 8.224510206698743886, 28.33442372801902209 ) ) ;
#126773=CARTESIAN_POINT ( 'NONE',  ( 17.50000000000000000, 3.209263204892558896, 32.73803174393727744 ) ) ;
#126774=CARTESIAN_POINT ( 'NONE',  ( -13.97604488694527625, -13.89961937509977652, 71.87390960531433848 ) ) ;
#126775=CARTESIAN_POINT ( 'NONE',  ( -10.81492255796105439, 18.62759615963255655, 102.9177570613523756 ) ) ;
#126776=CARTESIAN_POINT ( 'NONE',  ( -9.474510206698964154, 16.51473224551069663, 110.4155762719810383 ) ) ;
#126777=CARTESIAN_POINT ( 'NONE',  ( -14.34966873604972548, 8.224510206698743886, 88.33442372801901854 ) ) ;
#126778=CARTESIAN_POINT ( 'NONE',  ( 30.00000000000000000, 5.499999999999992895, 37.50000000000000000 ) ) ;
#126779=CARTESIAN_POINT ( 'NONE',  ( 0.05219959533936267826, -19.03943276465977164, 65.00109039468567573 ) ) ;
#126780=CARTESIAN_POINT ( 'NONE',  ( 21.55341960407619695, -5.719274019375665929, 111.0427570613523613 ) ) ;
#126781=LINE ( 'NONE', #79302, #137224 ) ;
#126782=CARTESIAN_POINT ( 'NONE',  ( 16.46253265017160672, -9.564922557960803928, 33.33224293864770260 ) ) ;
#126783=CARTESIAN_POINT ( 'NONE',  ( 8.224510206698953496, -14.34966873604960469, 27.91557627198103830 ) ) ;
#126785=CARTESIAN_POINT ( 'NONE',  ( 14.34966873604972726, -8.224510206698740333, 100.8344237280190185 ) ) ;
#126786=CARTESIAN_POINT ( 'NONE',  ( -19.19724070472097566, -5.499999999999895195, 86.06193348274379673 ) ) ;
#126787=CARTESIAN_POINT ( 'NONE',  ( -4.483927247898782831, 16.52544592524335698, 77.70942372801900433 ) ) ;
#126788=CARTESIAN_POINT ( 'NONE',  ( -0.05219959533909027116, -19.03943276465977164, 37.49890960531436690 ) ) ;
#126789=CARTESIAN_POINT ( 'NONE',  ( -10.81492255796105439, 18.62759615963255655, 97.91775706135236135 ) ) ;
#126790=CARTESIAN_POINT ( 'NONE',  ( -9.474510206698720793, -16.51473224551083518, 104.5844237280190043 ) ) ;
#126791=CARTESIAN_POINT ( 'NONE',  ( 21.53943276465977519, 0.05219959533937863772, 76.25109039468568994 ) ) ;
#126792=CARTESIAN_POINT ( 'NONE',  ( 13.89961937509957401, 13.97604488694547697, 56.87609039468564731 ) ) ;
#126793=CARTESIAN_POINT ( 'NONE',  ( -13.89961937509977652, 13.97604488694528158, 80.62390960531436690 ) ) ;
#126794=CARTESIAN_POINT ( 'NONE',  ( -9.564922557960796823, -16.46253265017161027, 67.08224293864769550 ) ) ;
#126795=CARTESIAN_POINT ( 'NONE',  ( 17.31747979337950127, 6.344076630961023255, 73.87944868065186199 ) ) ;
#126796=CARTESIAN_POINT ( 'NONE',  ( -0.05219959533910754901, -16.53943276465976808, 67.49890960531436690 ) ) ;
#126797=CARTESIAN_POINT ( 'NONE',  ( -18.67979575497178146, -10.72451020669898902, 46.66557627198102409 ) ) ;
#126798=CARTESIAN_POINT ( 'NONE',  ( 16.51473224551069308, 9.474510206698969483, 44.16557627198103120 ) ) ;
#126799=CARTESIAN_POINT ( 'NONE',  ( 15.80617190586746368, 15.72974639402197994, 89.37390960531435269 ) ) ;
#126800=CARTESIAN_POINT ( 'NONE',  ( 12.14591786802327356, -12.06949235617739191, 75.62609039468567573 ) ) ;
#126802=CARTESIAN_POINT ( 'NONE',  ( 16.53943276465976808, -0.05219959533910856209, 83.74890960531435269 ) ) ;
#126804=CARTESIAN_POINT ( 'NONE',  ( 16.52544592524335698, 4.483927247898782831, 36.45942372801901143 ) ) ;
#126805=CARTESIAN_POINT ( 'NONE',  ( 9.474510206698971260, -16.51473224551069308, 22.91557627198102765 ) ) ;
#126806=CARTESIAN_POINT ( 'NONE',  ( -9.474510206698720793, -16.51473224551083518, 64.58442372801900433 ) ) ;
#126807=CARTESIAN_POINT ( 'NONE',  ( -12.14591786802309592, -12.06949235617757132, 66.87390960531436690 ) ) ;
#126808=CARTESIAN_POINT ( 'NONE',  ( 15.72974639402176855, 15.80617190586768217, 51.87609039468568284 ) ) ;
#126810=CARTESIAN_POINT ( 'NONE',  ( 5.049401038298161559, -19.05341960407611168, 27.70724293864769550 ) ) ;
#126811=CARTESIAN_POINT ( 'NONE',  ( 5.719274019375991003, -21.55341960407610458, 92.70724293864770971 ) ) ;
#126813=CARTESIAN_POINT ( 'NONE',  ( 9.474510206698971260, -16.51473224551069308, 112.9155762719810383 ) ) ;
#126814=CARTESIAN_POINT ( 'NONE',  ( -16.53943276465976808, 0.05219959533911058130, 86.24890960531436690 ) ) ;
#126816=CARTESIAN_POINT ( 'NONE',  ( 5.049401038298161559, -19.05341960407611168, 47.70724293864770260 ) ) ;
#126818=CARTESIAN_POINT ( 'NONE',  ( -19.05341960407617563, 5.049401038297882671, 83.54275706135233293 ) ) ;
#126819=CARTESIAN_POINT ( 'NONE',  ( 18.62759615963255655, 10.81492255796105972, 31.66775706135234358 ) ) ;
#126820=CARTESIAN_POINT ( 'NONE',  ( 16.46253265017160672, -9.564922557960803928, 68.33224293864770971 ) ) ;
#126821=CARTESIAN_POINT ( 'NONE',  ( 9.474510206698729675, 16.51473224551082808, 57.08442372801900433 ) ) ;
#126822=CARTESIAN_POINT ( 'NONE',  ( 13.89961937509977652, -13.97604488694527269, 48.12390960531435979 ) ) ;
#126823=CARTESIAN_POINT ( 'NONE',  ( 14.29746914071049879, -8.314922557960816363, 68.33224293864769550 ) ) ;
#126824=CARTESIAN_POINT ( 'NONE',  ( -16.52544592524342804, 4.483927247898546575, 56.04057627198102409 ) ) ;
#126825=CARTESIAN_POINT ( 'NONE',  ( -0.05219959533909027116, -19.03943276465977164, 72.49890960531435269 ) ) ;
#126826=CARTESIAN_POINT ( 'NONE',  ( -15.80617190586745835, -15.72974639402198527, 101.8739096053143811 ) ) ;
#126827=CARTESIAN_POINT ( 'NONE',  ( 16.51473224551069308, 9.474510206698969483, 74.16557627198103830 ) ) ;
#126828=CARTESIAN_POINT ( 'NONE',  ( -21.53943276465977519, 0.05219959533907696930, 76.24890960531435269 ) ) ;
#126829=CARTESIAN_POINT ( 'NONE',  ( -9.474510206698720793, -16.51473224551083518, 19.58442372801899722 ) ) ;
#126830=CARTESIAN_POINT ( 'NONE',  ( -19.05341960407611168, -5.049401038298163336, 31.45724293864769550 ) ) ;
#126831=CARTESIAN_POINT ( 'NONE',  ( -16.52544592524335698, -4.483927247898792601, 103.9594237280190185 ) ) ;
#126832=CARTESIAN_POINT ( 'NONE',  ( -12.06949235617756955, 12.14591786802309770, 90.62390960531436690 ) ) ;
#126833=CARTESIAN_POINT ( 'NONE',  ( -9.474510206698720793, -16.51473224551083518, 104.5844237280190043 ) ) ;
#126835=CARTESIAN_POINT ( 'NONE',  ( -5.719274019375665041, -21.55341960407619695, 34.79275706135235424 ) ) ;
#126836=CARTESIAN_POINT ( 'NONE',  ( 19.03943276465977164, 0.05219959533936151252, 56.25109039468566863 ) ) ;
#126837=CARTESIAN_POINT ( 'NONE',  ( 14.34966873604972726, -8.224510206698740333, 110.8344237280190043 ) ) ;
#126838=CARTESIAN_POINT ( 'NONE',  ( -21.55341960407610458, -5.719274019375992779, 66.45724293864768129 ) ) ;
#126839=CARTESIAN_POINT ( 'NONE',  ( 5.153800228976335163, 19.02544592524342804, 104.7905762719809957 ) ) ;
#126840=CARTESIAN_POINT ( 'NONE',  ( -16.55341960407611168, -4.379528057220339221, 61.45724293864770260 ) ) ;
#126841=CARTESIAN_POINT ( 'NONE',  ( 5.049401038298161559, -19.05341960407611168, 27.70724293864769550 ) ) ;
#126842=CARTESIAN_POINT ( 'NONE',  ( -13.89961937509977652, 13.97604488694528158, 30.62390960531435269 ) ) ;
#126843=CARTESIAN_POINT ( 'NONE',  ( -19.02544592524334988, -5.153800228976617603, 23.95942372801900078 ) ) ;
#126844=CARTESIAN_POINT ( 'NONE',  ( -4.379528057220086978, -16.55341960407618274, 94.79275706135234714 ) ) ;
#126845=CARTESIAN_POINT ( 'NONE',  ( 5.719274019375673035, 21.55341960407619339, 47.29275706135234003 ) ) ;
#126846=CARTESIAN_POINT ( 'NONE',  ( -12.06949235617739369, -12.14591786802326823, 44.37609039468567573 ) ) ;
#126847=CARTESIAN_POINT ( 'NONE',  ( 16.51473224551069308, 9.474510206698969483, 114.1655762719810241 ) ) ;
#126848=CARTESIAN_POINT ( 'NONE',  ( -5.153800228976328057, -19.02544592524343514, 47.29057627198102409 ) ) ;
#126849=CARTESIAN_POINT ( 'NONE',  ( 15.80617190586769283, -15.72974639402175789, 90.62609039468567573 ) ) ;
#126850=CARTESIAN_POINT ( 'NONE',  ( 5.153800228976335163, 19.02544592524342804, 74.79057627198103830 ) ) ;
#126851=CARTESIAN_POINT ( 'NONE',  ( 8.314922557961029526, -14.29746914071037800, 60.41775706135235424 ) ) ;
#126852=CARTESIAN_POINT ( 'NONE',  ( 16.52544592524342804, -4.483927247898539470, 108.5405762719810241 ) ) ;
#126853=CARTESIAN_POINT ( 'NONE',  ( -12.14591786802309592, -12.06949235617757132, 26.87390960531435979 ) ) ;
#126854=CARTESIAN_POINT ( 'NONE',  ( -13.89961937509977830, 13.97604488694528158, 50.62390960531435979 ) ) ;
#126855=CARTESIAN_POINT ( 'NONE',  ( 21.52544592524334988, 5.823673210054432836, 51.45942372801901854 ) ) ;
#126856=CARTESIAN_POINT ( 'NONE',  ( 19.03943276465977164, -0.05219959533909143690, 88.74890960531436690 ) ) ;
#126857=CARTESIAN_POINT ( 'NONE',  ( 19.03943276465977164, -0.05219959533909143690, 83.74890960531436690 ) ) ;
#126858=CARTESIAN_POINT ( 'NONE',  ( -5.049401038298153566, 19.05341960407611168, 110.2072429386476671 ) ) ;
#126859=CARTESIAN_POINT ( 'NONE',  ( -12.06949235617756955, 12.14591786802309770, 45.62390960531436690 ) ) ;
#126860=CARTESIAN_POINT ( 'NONE',  ( -8.314922557960811034, -14.29746914071050412, 22.08224293864769194 ) ) ;
#126861=CARTESIAN_POINT ( 'NONE',  ( -14.34966873604960291, -8.224510206698953496, 41.66557627198103120 ) ) ;
#126863=CARTESIAN_POINT ( 'NONE',  ( 5.049401038297881783, 19.05341960407617563, 32.29275706135233293 ) ) ;
#126864=CARTESIAN_POINT ( 'NONE',  ( -5.153800228976328057, -19.02544592524343514, 77.29057627198099567 ) ) ;
#126865=CARTESIAN_POINT ( 'NONE',  ( -19.05341960407617563, 5.049401038297882671, 58.54275706135234003 ) ) ;
#126868=CARTESIAN_POINT ( 'NONE',  ( -16.46253265017146816, -9.564922557961047289, 79.16775706135234714 ) ) ;
#126869=CARTESIAN_POINT ( 'NONE',  ( -4.483927247898782831, 16.52544592524335698, 72.70942372801901854 ) ) ;
#126871=CARTESIAN_POINT ( 'NONE',  ( -5.049401038298153566, 19.05341960407611168, 110.2072429386476671 ) ) ;
#126872=CARTESIAN_POINT ( 'NONE',  ( -5.823673210054431948, 21.52544592524334988, 22.70942372801901499 ) ) ;
#126874=CARTESIAN_POINT ( 'NONE',  ( -5.153800228976607833, 19.02544592524334988, 87.70942372801897591 ) ) ;
#126875=CARTESIAN_POINT ( 'NONE',  ( 16.29526858892876007, 7.335722546920148801, 88.29670597800215148 ) ) ;
#126876=CARTESIAN_POINT ( 'NONE',  ( 0.05219959533909260263, 19.03943276465977164, 44.99890960531435979 ) ) ;
#126877=CARTESIAN_POINT ( 'NONE',  ( 5.049401038298161559, -19.05341960407611168, 92.70724293864769550 ) ) ;
#126878=CARTESIAN_POINT ( 'NONE',  ( 16.52544592524342804, -4.483927247898539470, 63.54057627198103830 ) ) ;
#126879=CARTESIAN_POINT ( 'NONE',  ( 13.97604488694527802, 13.89961937509977652, 44.37390960531435269 ) ) ;
#126880=CARTESIAN_POINT ( 'NONE',  ( -19.05341960407611168, -5.049401038298163336, 61.45724293864769550 ) ) ;
#126881=CARTESIAN_POINT ( 'NONE',  ( -9.474510206698720793, -16.51473224551083518, 69.58442372801901854 ) ) ;
#126882=CARTESIAN_POINT ( 'NONE',  ( 5.153800228976615827, -19.02544592524334988, 25.20942372801900433 ) ) ;
#126883=CARTESIAN_POINT ( 'NONE',  ( 19.05341960407611168, 5.049401038298154454, 68.95724293864769550 ) ) ;
#126884=CARTESIAN_POINT ( 'NONE',  ( -21.53943276465977519, 0.05219959533907696930, 66.24890960531436690 ) ) ;
#126885=CARTESIAN_POINT ( 'NONE',  ( -12.14591786802309592, -12.06949235617757132, 71.87390960531438111 ) ) ;
#126886=CARTESIAN_POINT ( 'NONE',  ( 19.05341960407617918, -5.049401038297876454, 41.04275706135233293 ) ) ;
#126888=CARTESIAN_POINT ( 'NONE',  ( -0.05219959533907301413, -21.53943276465977519, 47.49890960531435979 ) ) ;
#126889=CARTESIAN_POINT ( 'NONE',  ( -15.72974639402197994, 15.80617190586746368, 25.62390960531435624 ) ) ;
#126890=CARTESIAN_POINT ( 'NONE',  ( 16.46253265017160672, -9.564922557960803928, 58.33224293864769550 ) ) ;
#126891=CARTESIAN_POINT ( 'NONE',  ( -9.564922557960796823, -16.46253265017161027, 37.08224293864768839 ) ) ;
#126892=CARTESIAN_POINT ( 'NONE',  ( -8.314922557960811034, -14.29746914071050412, 102.0822429386476955 ) ) ;
#126893=CARTESIAN_POINT ( 'NONE',  ( 5.719274019375991003, -21.55341960407610458, 107.7072429386476955 ) ) ;
#126895=CARTESIAN_POINT ( 'NONE',  ( 15.72974639402176855, 15.80617190586768217, 31.87609039468567929 ) ) ;
#126896=CARTESIAN_POINT ( 'NONE',  ( -14.29746914071049879, 8.314922557960819915, 110.8322429386476955 ) ) ;
#126897=CARTESIAN_POINT ( 'NONE',  ( 18.67979575497194134, -10.72451020669871369, 80.83442372801901854 ) ) ;
#126898=CARTESIAN_POINT ( 'NONE',  ( 18.62759615963271287, -10.81492255796078972, 98.33224293864769550 ) ) ;
#126899=CARTESIAN_POINT ( 'NONE',  ( -19.02544592524334988, -5.153800228976617603, 38.95942372801900433 ) ) ;
#126903=CARTESIAN_POINT ( 'NONE',  ( 14.29746914071037800, 8.314922557961029526, 46.66775706135234714 ) ) ;
#126904=CARTESIAN_POINT ( 'NONE',  ( 16.52544592524342804, -4.483927247898539470, 108.5405762719810241 ) ) ;
#126906=CARTESIAN_POINT ( 'NONE',  ( -19.05341960407611168, -5.049401038298163336, 66.45724293864769550 ) ) ;
#126907=CARTESIAN_POINT ( 'NONE',  ( -8.224510206698948167, 14.34966873604960824, 95.41557627198102409 ) ) ;
#126908=CARTESIAN_POINT ( 'NONE',  ( 10.72451020669898902, -18.67979575497178502, 47.91557627198102409 ) ) ;
#126909=CARTESIAN_POINT ( 'NONE',  ( 16.55341960407611168, 4.379528057220329451, 78.95724293864769550 ) ) ;
#126910=CARTESIAN_POINT ( 'NONE',  ( 14.34966873604972726, -8.224510206698740333, 30.83442372801902209 ) ) ;
#126911=CARTESIAN_POINT ( 'NONE',  ( -5.823673210054431948, 21.52544592524334988, 82.70942372801900433 ) ) ;
#126912=CARTESIAN_POINT ( 'NONE',  ( -16.51473224551069308, -9.474510206698971260, 26.66557627198103120 ) ) ;
#126913=CARTESIAN_POINT ( 'NONE',  ( 8.224510206698742110, 14.34966873604972548, 92.08442372801901854 ) ) ;
#126914=CARTESIAN_POINT ( 'NONE',  ( 8.224510206698953496, -14.34966873604960469, 42.91557627198103120 ) ) ;
#126915=CARTESIAN_POINT ( 'NONE',  ( 5.049401038298161559, -19.05341960407611168, 57.70724293864769550 ) ) ;
#126916=CARTESIAN_POINT ( 'NONE',  ( -21.55341960407619339, 5.719274019375674811, 93.54275706135234714 ) ) ;
#126917=CARTESIAN_POINT ( 'NONE',  ( -21.53943276465977519, 0.05219959533907696930, 111.2489096053143669 ) ) ;
#126918=CARTESIAN_POINT ( 'NONE',  ( 5.823673210054444382, -21.52544592524334988, 55.20942372801902565 ) ) ;
#126919=CARTESIAN_POINT ( 'NONE',  ( -16.52544592524335698, -4.483927247898792601, 33.95942372801901143 ) ) ;
#126920=CARTESIAN_POINT ( 'NONE',  ( 16.55341960407611168, 4.379528057220329451, 58.95724293864770971 ) ) ;
#126921=CARTESIAN_POINT ( 'NONE',  ( -10.72451020669870658, -18.67979575497194134, 84.58442372801903275 ) ) ;
#126922=CARTESIAN_POINT ( 'NONE',  ( 8.314922557961029526, -14.29746914071037800, 110.4177570613523756 ) ) ;
#126923=CARTESIAN_POINT ( 'NONE',  ( 17.50000000000001421, -5.622605283950838029, 46.18792689403891671 ) ) ;
#126924=DIRECTION ( 'NONE',  ( 0.000000000000000000, 0.000000000000000000, 1.000000000000000000 ) ) ;
#126925=CARTESIAN_POINT ( 'NONE',  ( -8.314922557960811034, -14.29746914071050412, 22.08224293864769194 ) ) ;
#126926=CARTESIAN_POINT ( 'NONE',  ( 12.06949235617739724, 12.14591786802326823, 76.87609039468567573 ) ) ;
#126927=CARTESIAN_POINT ( 'NONE',  ( 13.97604488694527802, 13.89961937509977652, 89.37390960531436690 ) ) ;
#126928=CARTESIAN_POINT ( 'NONE',  ( 9.564922557960805705, 16.46253265017160317, 99.58224293864770971 ) ) ;
#126929=CARTESIAN_POINT ( 'NONE',  ( 10.81492255796106328, -18.62759615963255655, 80.41775706135234714 ) ) ;
#126930=CARTESIAN_POINT ( 'NONE',  ( -12.14591786802326823, 12.06949235617739902, 88.12609039468570415 ) ) ;
#126931=CARTESIAN_POINT ( 'NONE',  ( -12.14591786802309592, -12.06949235617757132, 66.87390960531436690 ) ) ;
#126932=CARTESIAN_POINT ( 'NONE',  ( 19.05341960407611168, 5.049401038298154454, 68.95724293864769550 ) ) ;
#126934=CARTESIAN_POINT ( 'NONE',  ( 0.05219959533934541429, -16.53943276465976808, 25.00109039468567218 ) ) ;
#126935=CARTESIAN_POINT ( 'NONE',  ( -16.46253265017160317, 9.564922557960807481, 25.83224293864769194 ) ) ;
#126936=CARTESIAN_POINT ( 'NONE',  ( -9.474510206698964154, 16.51473224551069663, 95.41557627198102409 ) ) ;
#126937=CARTESIAN_POINT ( 'NONE',  ( -12.06949235617739369, -12.14591786802326823, 29.37609039468568284 ) ) ;
#126939=CARTESIAN_POINT ( 'NONE',  ( 15.80617190586769283, -15.72974639402175789, 110.6260903946857042 ) ) ;
#126940=CARTESIAN_POINT ( 'NONE',  ( 14.34966873604972726, -8.224510206698740333, 95.83442372801903275 ) ) ;
#126941=CARTESIAN_POINT ( 'NONE',  ( -0.05219959533936034679, 19.03943276465977164, 112.5010903946856757 ) ) ;
#126942=CARTESIAN_POINT ( 'NONE',  ( -0.05219959533909027116, -19.03943276465977164, 37.49890960531436690 ) ) ;
#126943=CARTESIAN_POINT ( 'NONE',  ( 16.52544592524335698, 4.483927247898782831, 81.45942372801900433 ) ) ;
#126944=CARTESIAN_POINT ( 'NONE',  ( 14.34966873604972726, -8.224510206698740333, 60.83442372801901854 ) ) ;
#126946=CARTESIAN_POINT ( 'NONE',  ( -19.03943276465977164, -0.05219959533935918106, 73.75109039468566152 ) ) ;
#126947=CARTESIAN_POINT ( 'NONE',  ( -15.72974639402176322, -15.80617190586768395, 104.3760903946856899 ) ) ;
#126948=CARTESIAN_POINT ( 'NONE',  ( 9.474510206698971260, -16.51473224551069308, 42.91557627198103120 ) ) ;
#126949=CARTESIAN_POINT ( 'NONE',  ( -19.03943276465977164, 0.05219959533909376836, 91.24890960531436690 ) ) ;
#126950=CARTESIAN_POINT ( 'NONE',  ( -16.52544592524342804, 4.483927247898546575, 81.04057627198102409 ) ) ;
#126951=CARTESIAN_POINT ( 'NONE',  ( 19.02544592524334988, 5.153800228976608722, 56.45942372801898301 ) ) ;
#126952=CARTESIAN_POINT ( 'NONE',  ( -21.53943276465977519, 0.05219959533907696930, 46.24890960531435979 ) ) ;
#126953=CARTESIAN_POINT ( 'NONE',  ( 0.05219959533937995610, -21.53943276465977519, 110.0010903946856757 ) ) ;
#126954=CARTESIAN_POINT ( 'NONE',  ( -13.97604488694527625, -13.89961937509977652, 91.87390960531432427 ) ) ;
#126955=CARTESIAN_POINT ( 'NONE',  ( 15.72974639402176855, 15.80617190586768217, 111.8760903946856615 ) ) ;
#126956=CARTESIAN_POINT ( 'NONE',  ( 21.53943276465977519, -0.05219959533907433946, 58.74890960531436690 ) ) ;
#126957=CARTESIAN_POINT ( 'NONE',  ( -9.564922557960796823, -16.46253265017161027, 92.08224293864769550 ) ) ;
#126958=CARTESIAN_POINT ( 'NONE',  ( 19.05341960407617918, -5.049401038297876454, 86.04275706135233293 ) ) ;
#126959=CARTESIAN_POINT ( 'NONE',  ( 13.89961937509977652, -13.97604488694527269, 103.1239096053143527 ) ) ;
#126960=CARTESIAN_POINT ( 'NONE',  ( 19.02544592524334988, 5.153800228976608722, 111.4594237280190043 ) ) ;
#126961=CARTESIAN_POINT ( 'NONE',  ( -13.97604488694527625, -13.89961937509977652, 26.87390960531434558 ) ) ;
#126962=CARTESIAN_POINT ( 'NONE',  ( 19.02544592524343514, -5.153800228976328945, 88.54057627198102409 ) ) ;
#126963=CARTESIAN_POINT ( 'NONE',  ( -21.52544592524343514, 5.823673210054127303, 81.04057627198102409 ) ) ;
#126964=CARTESIAN_POINT ( 'NONE',  ( 4.483927247898790824, -16.52544592524335698, 40.20942372801901854 ) ) ;
#126965=CARTESIAN_POINT ( 'NONE',  ( -21.52544592524334988, -5.823673210054445271, 43.95942372801902565 ) ) ;
#126966=CARTESIAN_POINT ( 'NONE',  ( 5.719274019375673035, 21.55341960407619339, 102.2927570613523613 ) ) ;
#126967=CARTESIAN_POINT ( 'NONE',  ( -14.34966873604972548, 8.224510206698743886, 93.33442372801901854 ) ) ;
#126969=CARTESIAN_POINT ( 'NONE',  ( 13.89961937509977652, -13.97604488694527269, 93.12390960531436690 ) ) ;
#126970=CARTESIAN_POINT ( 'NONE',  ( -14.34966873604960291, -8.224510206698953496, 86.66557627198102409 ) ) ;
#126971=CARTESIAN_POINT ( 'NONE',  ( 4.483927247898545687, 16.52544592524342804, 24.79057627198103120 ) ) ;
#126972=CARTESIAN_POINT ( 'NONE',  ( 16.46253265017146816, 9.564922557961045513, 71.66775706135233293 ) ) ;
#126973=CARTESIAN_POINT ( 'NONE',  ( -10.81492255796105439, 18.62759615963255655, 47.91775706135234714 ) ) ;
#126974=CARTESIAN_POINT ( 'NONE',  ( -16.52544592524342804, 4.483927247898546575, 96.04057627198102409 ) ) ;
#126975=CARTESIAN_POINT ( 'NONE',  ( -0.05219959533909027116, -19.03943276465977164, 112.4989096053143669 ) ) ;
#126976=CARTESIAN_POINT ( 'NONE',  ( 14.34966873604960469, 8.224510206698951720, 29.16557627198103120 ) ) ;
#126977=CARTESIAN_POINT ( 'NONE',  ( 5.823673210054444382, -21.52544592524334988, 80.20942372801901854 ) ) ;
#126978=CARTESIAN_POINT ( 'NONE',  ( 0.05219959533934541429, -16.53943276465976808, 60.00109039468568284 ) ) ;
#126979=CARTESIAN_POINT ( 'NONE',  ( 8.224510206698742110, 14.34966873604972548, 112.0844237280190185 ) ) ;
#126980=CARTESIAN_POINT ( 'NONE',  ( 5.823673210054444382, -21.52544592524334988, 60.20942372801902565 ) ) ;
#126981=ADVANCED_FACE ( 'NONE', ( #161636 ), #21939, .T. ) ;
#126983=CARTESIAN_POINT ( 'NONE',  ( -10.72451020669870658, -18.67979575497194134, 24.58442372801901499 ) ) ;
#126984=CARTESIAN_POINT ( 'NONE',  ( -16.52544592524342804, 4.483927247898546575, 101.0405762719810383 ) ) ;
#126985=CARTESIAN_POINT ( 'NONE',  ( -9.564922557960796823, -16.46253265017161027, 27.08224293864769550 ) ) ;
#126986=CARTESIAN_POINT ( 'NONE',  ( 16.53943276465976808, -0.05219959533910856209, 68.74890960531435269 ) ) ;
#126987=CARTESIAN_POINT ( 'NONE',  ( -19.03943276465977164, 0.05219959533909376836, 76.24890960531435269 ) ) ;
#126988=CARTESIAN_POINT ( 'NONE',  ( 8.314922557961029526, -14.29746914071037800, 100.4177570613523471 ) ) ;
#126989=CARTESIAN_POINT ( 'NONE',  ( 9.564922557960805705, 16.46253265017160317, 39.58224293864768839 ) ) ;
#126990=CARTESIAN_POINT ( 'NONE',  ( 21.52544592524344225, -5.823673210054117533, 38.54057627198103120 ) ) ;
#126991=CARTESIAN_POINT ( 'NONE',  ( -8.224510206698948167, 14.34966873604960824, 85.41557627198102409 ) ) ;
#126992=CARTESIAN_POINT ( 'NONE',  ( 10.72451020669898902, -18.67979575497178502, 92.91557627198103830 ) ) ;
#126993=CARTESIAN_POINT ( 'NONE',  ( 13.97604488694527802, 13.89961937509977652, 89.37390960531436690 ) ) ;
#126994=CARTESIAN_POINT ( 'NONE',  ( 13.97604488694527802, 13.89961937509977652, 54.37390960531435979 ) ) ;
#126995=CARTESIAN_POINT ( 'NONE',  ( 19.05341960407617918, -5.049401038297876454, 86.04275706135233293 ) ) ;
#126996=CARTESIAN_POINT ( 'NONE',  ( 18.67979575497178502, 10.72451020669898547, 39.16557627198102409 ) ) ;
#126997=CARTESIAN_POINT ( 'NONE',  ( 15.72974639402176855, 15.80617190586768217, 66.87609039468568994 ) ) ;
#126998=CARTESIAN_POINT ( 'NONE',  ( -13.89961937509977652, 13.97604488694528158, 50.62390960531435979 ) ) ;
#126999=CARTESIAN_POINT ( 'NONE',  ( 5.153800228976335163, 19.02544592524342804, 79.79057627198102409 ) ) ;
#127000=CARTESIAN_POINT ( 'NONE',  ( 14.34966873604972726, -8.224510206698740333, 60.83442372801901854 ) ) ;
#127001=CARTESIAN_POINT ( 'NONE',  ( 15.80617190586769283, -15.72974639402175789, 40.62609039468567573 ) ) ;
#127002=CARTESIAN_POINT ( 'NONE',  ( 15.72974639402176855, 15.80617190586768217, 71.87609039468568994 ) ) ;
#127003=CARTESIAN_POINT ( 'NONE',  ( 5.719274019375991003, -21.55341960407610458, 27.70724293864769905 ) ) ;
#127004=CARTESIAN_POINT ( 'NONE',  ( -0.05219959533907301413, -21.53943276465977519, 102.4989096053143811 ) ) ;
#127005=CARTESIAN_POINT ( 'NONE',  ( 21.52544592524334988, 5.823673210054432836, 41.45942372801901143 ) ) ;
#127006=CARTESIAN_POINT ( 'NONE',  ( -4.379528057220086978, -16.55341960407618274, 64.79275706135234714 ) ) ;
#127007=CARTESIAN_POINT ( 'NONE',  ( 18.67979575497178502, 10.72451020669898547, 69.16557627198102409 ) ) ;
#127008=CARTESIAN_POINT ( 'NONE',  ( 0.05219959533936267826, -19.03943276465977164, 35.00109039468566863 ) ) ;
#127009=CARTESIAN_POINT ( 'NONE',  ( -13.97604488694527625, -13.89961937509977652, 71.87390960531433848 ) ) ;
#127010=CARTESIAN_POINT ( 'NONE',  ( 8.224510206698953496, -14.34966873604960469, 27.91557627198103830 ) ) ;
#127011=CARTESIAN_POINT ( 'NONE',  ( -17.49999999999998934, -4.013004640162571413, 104.5539427900559417 ) ) ;
#127012=( BOUNDED_CURVE ( )  B_SPLINE_CURVE ( 2, ( #121365, #137531, #60680, #124345, #47523, #184044, #44542, #109179, #170858, #32349, #94002, #76848, #17178 ),
 .UNSPECIFIED., .F., .T. ) 
 B_SPLINE_CURVE_WITH_KNOTS ( ( 3, 2, 2, 2, 2, 2, 3 ),
 ( 0.4761603267754511148, 0.4780701754385964786, 0.4824561403508771940, 0.4868421052631579093, 0.4912280701754385692, 0.4956140350877192846, 0.4975695635729549537 ),
 .UNSPECIFIED. ) 
 CURVE ( )  GEOMETRIC_REPRESENTATION_ITEM ( )  RATIONAL_B_SPLINE_CURVE ( ( 0.9832469066685285419, 0.9851625545550100060, 1.000000000000000000, 0.9659258262890683122, 1.000000000000000000, 0.9659258262890683122, 1.000000000000000000, 0.9659258262890683122, 1.000000000000000000, 0.9659258262890683122, 1.000000000000000000, 0.9848076720550082985, 0.9831626618144002627 ) ) 
 REPRESENTATION_ITEM ( '' )  );
#127013=CARTESIAN_POINT ( 'NONE',  ( 19.02544592524343514, -5.153800228976328945, 103.5405762719809957 ) ) ;
#127015=CARTESIAN_POINT ( 'NONE',  ( 16.46253265017146816, 9.564922557961045513, 86.66775706135233293 ) ) ;
#127016=CARTESIAN_POINT ( 'NONE',  ( -0.05219959533907301413, -21.53943276465977519, 52.49890960531435979 ) ) ;
#127017=CARTESIAN_POINT ( 'NONE',  ( 16.53943276465976808, -0.05219959533910856209, 43.74890960531435979 ) ) ;
#127018=CARTESIAN_POINT ( 'NONE',  ( 19.05341960407617918, -5.049401038297876454, 96.04275706135231871 ) ) ;
#127019=CARTESIAN_POINT ( 'NONE',  ( 19.03943276465977164, -0.05219959533909143690, 28.74890960531435624 ) ) ;
#127020=CARTESIAN_POINT ( 'NONE',  ( 9.474510206698729675, 16.51473224551082808, 112.0844237280190043 ) ) ;
#127021=CARTESIAN_POINT ( 'NONE',  ( -5.719274019375978568, 21.55341960407610458, 90.20724293864770971 ) ) ;
#127022=CARTESIAN_POINT ( 'NONE',  ( -0.05219959533936034679, 19.03943276465977164, 62.50109039468566863 ) ) ;
#127023=CARTESIAN_POINT ( 'NONE',  ( -4.379528057220086978, -16.55341960407618274, 74.79275706135234714 ) ) ;
#127024=CARTESIAN_POINT ( 'NONE',  ( -19.05341960407611168, -5.049401038298163336, 71.45724293864766707 ) ) ;
#127025=CARTESIAN_POINT ( 'NONE',  ( 12.14591786802309770, 12.06949235617756955, 79.37390960531436690 ) ) ;
#127026=CARTESIAN_POINT ( 'NONE',  ( 0.05219959533909260263, 19.03943276465977164, 49.99890960531435979 ) ) ;
#127027=CARTESIAN_POINT ( 'NONE',  ( -14.29746914071049879, 8.314922557960819915, 50.83224293864770971 ) ) ;
#127030=CARTESIAN_POINT ( 'NONE',  ( 4.379528057220339221, -16.55341960407611168, 22.70724293864769194 ) ) ;
#127031=CARTESIAN_POINT ( 'NONE',  ( 5.049401038298161559, -19.05341960407611168, 77.70724293864765286 ) ) ;
#127033=CARTESIAN_POINT ( 'NONE',  ( 16.46253265017146816, 9.564922557961045513, 41.66775706135234003 ) ) ;
#127034=CARTESIAN_POINT ( 'NONE',  ( -16.53943276465976808, -0.05219959533934237506, 43.75109039468568284 ) ) ;
#127035=CARTESIAN_POINT ( 'NONE',  ( 10.72451020669898902, -18.67979575497178502, 62.91557627198102409 ) ) ;
#127036=CARTESIAN_POINT ( 'NONE',  ( -21.55341960407619339, 5.719274019375674811, 113.5427570613523756 ) ) ;
#127037=CARTESIAN_POINT ( 'NONE',  ( -9.474510206698964154, 16.51473224551069663, 75.41557627198103830 ) ) ;
#127038=CARTESIAN_POINT ( 'NONE',  ( -19.02544592524342804, 5.153800228976336051, 116.0405762719810383 ) ) ;
#127039=CARTESIAN_POINT ( 'NONE',  ( -19.02544592524342804, 5.153800228976336051, 116.0405762719810383 ) ) ;
#127040=CARTESIAN_POINT ( 'NONE',  ( -18.62759615963255300, -10.81492255796106328, 39.16775706135235424 ) ) ;
#127041=CARTESIAN_POINT ( 'NONE',  ( 12.06949235617757843, -12.14591786802309237, 108.1239096053143811 ) ) ;
#127042=CARTESIAN_POINT ( 'NONE',  ( 15.80617190586746368, 15.72974639402197994, 99.37390960531436690 ) ) ;
#127043=CARTESIAN_POINT ( 'NONE',  ( -9.474510206698964154, 16.51473224551069663, 75.41557627198103830 ) ) ;
#127045=CARTESIAN_POINT ( 'NONE',  ( -21.55341960407619339, 5.719274019375674811, 28.54275706135234358 ) ) ;
#127046=VERTEX_POINT ( 'NONE', #196933 ) ;
#127047=CARTESIAN_POINT ( 'NONE',  ( -19.03943276465977164, 0.05219959533909376836, 81.24890960531436690 ) ) ;
#127050=CARTESIAN_POINT ( 'NONE',  ( 5.049401038298161559, -19.05341960407611168, 22.70724293864769194 ) ) ;
#127051=CARTESIAN_POINT ( 'NONE',  ( -5.153800228976328057, -19.02544592524343514, 27.29057627198103120 ) ) ;
#127052=CARTESIAN_POINT ( 'NONE',  ( -13.89961937509957401, -13.97604488694547875, 104.3760903946856757 ) ) ;
#127054=CARTESIAN_POINT ( 'NONE',  ( 16.55341960407611168, 4.379528057220329451, 113.9572429386477239 ) ) ;
#127055=CARTESIAN_POINT ( 'NONE',  ( -21.52544592524334988, -5.823673210054445271, 83.95942372801900433 ) ) ;
#127056=CARTESIAN_POINT ( 'NONE',  ( -16.51473224551069308, -9.474510206698971260, 56.66557627198103120 ) ) ;
#127057=CARTESIAN_POINT ( 'NONE',  ( -0.05219959533937732626, 21.53943276465977519, 52.50109039468567573 ) ) ;
#127058=CARTESIAN_POINT ( 'NONE',  ( 21.55341960407619695, -5.719274019375665929, 21.04275706135234714 ) ) ;
#127060=CARTESIAN_POINT ( 'NONE',  ( -5.049401038298153566, 19.05341960407611168, 80.20724293864769550 ) ) ;
#127062=CARTESIAN_POINT ( 'NONE',  ( -8.314922557961024197, 14.29746914071037800, 27.91775706135234358 ) ) ;
#127063=CARTESIAN_POINT ( 'NONE',  ( 0.05219959533907565091, 21.53943276465977519, 44.99890960531435979 ) ) ;
#127064=CARTESIAN_POINT ( 'NONE',  ( 5.823673210054444382, -21.52544592524334988, 70.20942372801904696 ) ) ;
#127065=CARTESIAN_POINT ( 'NONE',  ( 13.97604488694527802, 13.89961937509977652, 114.3739096053143669 ) ) ;
#127066=CARTESIAN_POINT ( 'NONE',  ( 19.03943276465977164, 0.05219959533936151252, 101.2510903946856757 ) ) ;
#127067=CARTESIAN_POINT ( 'NONE',  ( -19.03943276465977164, 0.05219959533909376836, 61.24890960531436690 ) ) ;
#127068=CARTESIAN_POINT ( 'NONE',  ( 9.564922557960805705, 16.46253265017160317, 89.58224293864769550 ) ) ;
#127069=CARTESIAN_POINT ( 'NONE',  ( 16.55341960407611168, 4.379528057220329451, 113.9572429386477239 ) ) ;
#127070=CARTESIAN_POINT ( 'NONE',  ( -0.05219959533910754901, -16.53943276465976808, 102.4989096053143811 ) ) ;
#127071=CARTESIAN_POINT ( 'NONE',  ( -0.05219959533909027116, -19.03943276465977164, 112.4989096053143669 ) ) ;
#127072=CARTESIAN_POINT ( 'NONE',  ( 16.53943276465976808, 0.05219959533934440121, 76.25109039468568994 ) ) ;
#127073=CARTESIAN_POINT ( 'NONE',  ( -12.06949235617756955, 12.14591786802309770, 55.62390960531436690 ) ) ;
#127074=CARTESIAN_POINT ( 'NONE',  ( -19.02544592524342804, 5.153800228976336051, 36.04057627198100988 ) ) ;
#127075=CARTESIAN_POINT ( 'NONE',  ( 18.67979575497194134, -10.72451020669871369, 75.83442372801900433 ) ) ;
#127076=CARTESIAN_POINT ( 'NONE',  ( -13.89961937509957401, -13.97604488694547875, 99.37609039468567573 ) ) ;
#127077=CARTESIAN_POINT ( 'NONE',  ( 8.224510206698953496, -14.34966873604960469, 62.91557627198102409 ) ) ;
#127078=CARTESIAN_POINT ( 'NONE',  ( 0.05219959533937995610, -21.53943276465977519, 20.00109039468568639 ) ) ;
#127079=CARTESIAN_POINT ( 'NONE',  ( 15.80617190586746368, 15.72974639402197994, 49.37390960531436690 ) ) ;
#127082=CARTESIAN_POINT ( 'NONE',  ( -19.05341960407611168, -5.049401038298163336, 71.45724293864766707 ) ) ;
#127083=CARTESIAN_POINT ( 'NONE',  ( -8.224510206698948167, 14.34966873604960824, 40.41557627198103120 ) ) ;
#127084=CARTESIAN_POINT ( 'NONE',  ( 16.52544592524342804, -4.483927247898539470, 28.54057627198103120 ) ) ;
#127085=CARTESIAN_POINT ( 'NONE',  ( 4.379528057220092307, 16.55341960407617563, 82.29275706135234714 ) ) ;
#127086=CARTESIAN_POINT ( 'NONE',  ( 19.05341960407617918, -5.049401038297876454, 36.04275706135234003 ) ) ;
#127087=DIRECTION ( 'NONE',  ( -0.000000000000000000, -0.000000000000000000, 1.000000000000000000 ) ) ;
#127088=CARTESIAN_POINT ( 'NONE',  ( 13.89961937509977652, -13.97604488694527269, 88.12390960531438111 ) ) ;
#127089=CARTESIAN_POINT ( 'NONE',  ( -12.06949235617756955, 12.14591786802309770, 55.62390960531436690 ) ) ;
#127090=CARTESIAN_POINT ( 'NONE',  ( 16.29526858892874586, -7.335722546920107945, 101.7032940219979764 ) ) ;
#127091=CARTESIAN_POINT ( 'NONE',  ( 16.51473224551069308, 9.474510206698969483, 114.1655762719810241 ) ) ;
#127092=CARTESIAN_POINT ( 'NONE',  ( 21.52544592524344225, -5.823673210054117533, 53.54057627198103120 ) ) ;
#127094=CARTESIAN_POINT ( 'NONE',  ( 16.52544592524342804, -4.483927247898539470, 98.54057627198105251 ) ) ;
#127095=CARTESIAN_POINT ( 'NONE',  ( -14.34966873604972548, 8.224510206698743886, 38.33442372801900433 ) ) ;
#127096=CARTESIAN_POINT ( 'NONE',  ( -8.314922557960811034, -14.29746914071050412, 77.08224293864769550 ) ) ;
#127098=CARTESIAN_POINT ( 'NONE',  ( 19.05341960407617918, -5.049401038297876454, 76.04275706135230450 ) ) ;
#127099=CARTESIAN_POINT ( 'NONE',  ( -15.72974639402197994, 15.80617190586746368, 25.62390960531435624 ) ) ;
#127101=CARTESIAN_POINT ( 'NONE',  ( 18.22780087662119897, -5.500000000000096811, 43.51763182126894236 ) ) ;
#127102=CARTESIAN_POINT ( 'NONE',  ( 16.52544592524335698, 4.483927247898782831, 31.45942372801901854 ) ) ;
#127103=CARTESIAN_POINT ( 'NONE',  ( -12.06949235617756955, 12.14591786802309770, 30.62390960531436335 ) ) ;
#127104=CARTESIAN_POINT ( 'NONE',  ( -10.72451020669898014, 18.67979575497178502, 55.41557627198102409 ) ) ;
#127106=CARTESIAN_POINT ( 'NONE',  ( 16.46253265017146816, 9.564922557961045513, 66.66775706135233293 ) ) ;
#127107=CARTESIAN_POINT ( 'NONE',  ( -5.719274019375978568, 21.55341960407610458, 50.20724293864769550 ) ) ;
#127108=CARTESIAN_POINT ( 'NONE',  ( -21.53943276465977519, -0.05219959533937600094, 68.75109039468568994 ) ) ;
#127110=CARTESIAN_POINT ( 'NONE',  ( 12.06949235617739724, 12.14591786802326823, 36.87609039468568994 ) ) ;
#127111=CARTESIAN_POINT ( 'NONE',  ( -5.049401038298153566, 19.05341960407611168, 30.20724293864768839 ) ) ;
#127112=CARTESIAN_POINT ( 'NONE',  ( 19.03943276465977164, -0.05219959533909143690, 83.74890960531436690 ) ) ;
#127113=ADVANCED_FACE ( 'NONE', ( #120067 ), #20742, .T. ) ;
#127114=CARTESIAN_POINT ( 'NONE',  ( 16.51473224551069308, 9.474510206698969483, 34.16557627198102409 ) ) ;
#127115=CARTESIAN_POINT ( 'NONE',  ( -14.29746914071049879, 8.314922557960819915, 100.8322429386477097 ) ) ;
#127117=CARTESIAN_POINT ( 'NONE',  ( 19.05341960407611168, 5.049401038298154454, 103.9572429386476671 ) ) ;
#127118=ORIENTED_EDGE ( 'NONE', *, *, #87010, .F. ) ;
#127119=CARTESIAN_POINT ( 'NONE',  ( 8.314922557961029526, -14.29746914071037800, 55.41775706135234714 ) ) ;
#127120=CARTESIAN_POINT ( 'NONE',  ( 18.62759615963271287, -10.81492255796078972, 78.33224293864770971 ) ) ;
#127121=CARTESIAN_POINT ( 'NONE',  ( 9.564922557960805705, 16.46253265017160317, 44.58224293864769550 ) ) ;
#127122=CARTESIAN_POINT ( 'NONE',  ( -0.05219959533936034679, 19.03943276465977164, 72.50109039468566152 ) ) ;
#127123=CARTESIAN_POINT ( 'NONE',  ( 15.72974639402199770, -15.80617190586745480, 108.1239096053143811 ) ) ;
#127124=CARTESIAN_POINT ( 'NONE',  ( 13.97604488694527802, 13.89961937509977652, 69.37390960531436690 ) ) ;
#127125=CARTESIAN_POINT ( 'NONE',  ( 16.46253265017160672, -9.564922557960803928, 108.3322429386476955 ) ) ;
#127127=CARTESIAN_POINT ( 'NONE',  ( -12.06949235617739369, -12.14591786802326823, 39.37609039468567573 ) ) ;
#127128=CARTESIAN_POINT ( 'NONE',  ( -15.72974639402176322, -15.80617190586768395, 24.37609039468567573 ) ) ;
#127129=CARTESIAN_POINT ( 'NONE',  ( -16.53943276465976808, 0.05219959533911058130, 101.2489096053143669 ) ) ;
#127130=CARTESIAN_POINT ( 'NONE',  ( 16.51473224551069308, 9.474510206698969483, 89.16557627198103830 ) ) ;
#127131=CARTESIAN_POINT ( 'NONE',  ( 19.03943276465977164, 0.05219959533936151252, 71.25109039468566152 ) ) ;
#127132=CARTESIAN_POINT ( 'NONE',  ( -18.67979575497178146, -10.72451020669898902, 81.66557627198103830 ) ) ;
#127133=CARTESIAN_POINT ( 'NONE',  ( -4.483927247898539470, -16.52544592524342804, 52.29057627198102409 ) ) ;
#127134=CARTESIAN_POINT ( 'NONE',  ( -5.153800228976607833, 19.02544592524334988, 22.70942372801899012 ) ) ;
#127135=CARTESIAN_POINT ( 'NONE',  ( -16.55341960407617563, 4.379528057220093196, 73.54275706135234714 ) ) ;
#127136=CARTESIAN_POINT ( 'NONE',  ( -13.97604488694527625, -13.89961937509977652, 91.87390960531432427 ) ) ;
#127137=CARTESIAN_POINT ( 'NONE',  ( -19.05341960407611168, -5.049401038298163336, 46.45724293864768129 ) ) ;
#127138=CARTESIAN_POINT ( 'NONE',  ( 21.55341960407619695, -5.719274019375665929, 51.04275706135234714 ) ) ;
#127139=CARTESIAN_POINT ( 'NONE',  ( 5.719274019375673035, 21.55341960407619339, 62.29275706135236845 ) ) ;
#127140=CARTESIAN_POINT ( 'NONE',  ( 9.474510206698971260, -16.51473224551069308, 62.91557627198102409 ) ) ;
#127141=CARTESIAN_POINT ( 'NONE',  ( 5.823673210054444382, -21.52544592524334988, 35.20942372801901854 ) ) ;
#127142=CARTESIAN_POINT ( 'NONE',  ( 9.564922557961047289, -16.46253265017146816, 85.41775706135233293 ) ) ;
#127143=CARTESIAN_POINT ( 'NONE',  ( -16.51473224551069308, -9.474510206698971260, 36.66557627198102409 ) ) ;
#127144=CARTESIAN_POINT ( 'NONE',  ( -14.29746914071037622, -8.314922557961029526, 89.16775706135236135 ) ) ;
#127145=CARTESIAN_POINT ( 'NONE',  ( 5.049401038298161559, -19.05341960407611168, 72.70724293864768129 ) ) ;
#127146=CARTESIAN_POINT ( 'NONE',  ( 13.89961937509977652, -13.97604488694527269, 108.1239096053143669 ) ) ;
#127147=CARTESIAN_POINT ( 'NONE',  ( -19.05341960407611168, -5.049401038298163336, 46.45724293864768129 ) ) ;
#127148=CARTESIAN_POINT ( 'NONE',  ( -21.53943276465977519, 0.05219959533907696930, 81.24890960531436690 ) ) ;
#127149=CARTESIAN_POINT ( 'NONE',  ( -8.224510206698735004, -14.34966873604973081, 79.58442372801903275 ) ) ;
#127151=CARTESIAN_POINT ( 'NONE',  ( 0.05219959533936267826, -19.03943276465977164, 35.00109039468566863 ) ) ;
#127152=CARTESIAN_POINT ( 'NONE',  ( 19.03943276465977164, -0.05219959533909143690, 68.74890960531436690 ) ) ;
#127153=CARTESIAN_POINT ( 'NONE',  ( 14.34966873604960469, 8.224510206698951720, 39.16557627198102409 ) ) ;
#127154=CARTESIAN_POINT ( 'NONE',  ( -16.55341960407611168, -4.379528057220339221, 81.45724293864769550 ) ) ;
#127155=CARTESIAN_POINT ( 'NONE',  ( -0.05219959533909027116, -19.03943276465977164, 107.4989096053143527 ) ) ;
#127156=CARTESIAN_POINT ( 'NONE',  ( -19.02544592524342804, 5.153800228976336051, 91.04057627198100988 ) ) ;
#127157=CARTESIAN_POINT ( 'NONE',  ( 5.719274019375673035, 21.55341960407619339, 52.29275706135236135 ) ) ;
#127158=CARTESIAN_POINT ( 'NONE',  ( -5.049401038298153566, 19.05341960407611168, 110.2072429386476671 ) ) ;
#127159=CARTESIAN_POINT ( 'NONE',  ( -15.72974639402176322, -15.80617190586768395, 109.3760903946857042 ) ) ;
#127160=CARTESIAN_POINT ( 'NONE',  ( 14.34966873604972726, -8.224510206698740333, 80.83442372801901854 ) ) ;
#127161=CARTESIAN_POINT ( 'NONE',  ( 5.719274019375673035, 21.55341960407619339, 27.29275706135234358 ) ) ;
#127162=CARTESIAN_POINT ( 'NONE',  ( -19.02544592524342804, 5.153800228976336051, 116.0405762719810383 ) ) ;
#127163=CARTESIAN_POINT ( 'NONE',  ( 21.53943276465977519, -0.05219959533907433946, 98.74890960531438111 ) ) ;
#127164=CARTESIAN_POINT ( 'NONE',  ( 14.34966873604960469, 8.224510206698951720, 54.16557627198103120 ) ) ;
#127165=CARTESIAN_POINT ( 'NONE',  ( 0.05219959533909260263, 19.03943276465977164, 59.99890960531436690 ) ) ;
#127166=CARTESIAN_POINT ( 'NONE',  ( -12.14591786802309592, -12.06949235617757132, 76.87390960531439532 ) ) ;
#127167=CARTESIAN_POINT ( 'NONE',  ( -15.72974639402197994, 15.80617190586746368, 35.62390960531437401 ) ) ;
#127168=CARTESIAN_POINT ( 'NONE',  ( -19.05341960407617563, 5.049401038297882671, 38.54275706135233293 ) ) ;
#127169=CARTESIAN_POINT ( 'NONE',  ( -12.06949235617756955, 12.14591786802309770, 115.6239096053143669 ) ) ;
#127171=CARTESIAN_POINT ( 'NONE',  ( -16.55341960407617563, 4.379528057220093196, 68.54275706135234714 ) ) ;
#127172=CARTESIAN_POINT ( 'NONE',  ( -9.564922557960796823, -16.46253265017161027, 67.08224293864769550 ) ) ;
#127174=CARTESIAN_POINT ( 'NONE',  ( -14.34966873604960291, -8.224510206698953496, 91.66557627198103830 ) ) ;
#127175=CARTESIAN_POINT ( 'NONE',  ( 21.52544592524344225, -5.823673210054117533, 38.54057627198103120 ) ) ;
#127176=CARTESIAN_POINT ( 'NONE',  ( 8.224510206698742110, 14.34966873604972548, 107.0844237280190043 ) ) ;
#127177=CARTESIAN_POINT ( 'NONE',  ( -0.05219959533936034679, 19.03943276465977164, 107.5010903946856615 ) ) ;
#127178=CARTESIAN_POINT ( 'NONE',  ( -15.72974639402176322, -15.80617190586768395, 84.37609039468570415 ) ) ;
#127179=CARTESIAN_POINT ( 'NONE',  ( 13.89961937509977652, -13.97604488694527269, 83.12390960531436690 ) ) ;
#127180=CARTESIAN_POINT ( 'NONE',  ( 21.53943276465977519, -0.05219959533907433946, 98.74890960531438111 ) ) ;
#127181=CARTESIAN_POINT ( 'NONE',  ( -12.14591786802326823, 12.06949235617739902, 58.12609039468568994 ) ) ;
#127182=CARTESIAN_POINT ( 'NONE',  ( -9.564922557960796823, -16.46253265017161027, 32.08224293864769550 ) ) ;
#127183=CARTESIAN_POINT ( 'NONE',  ( 16.53943276465976808, 0.05219959533934440121, 31.25109039468568639 ) ) ;
#127184=CARTESIAN_POINT ( 'NONE',  ( -9.474510206698720793, -16.51473224551083518, 94.58442372801900433 ) ) ;
#127185=CARTESIAN_POINT ( 'NONE',  ( -21.52544592524343514, 5.823673210054127303, 91.04057627198103830 ) ) ;
#127186=CARTESIAN_POINT ( 'NONE',  ( -0.05219959533936034679, 19.03943276465977164, 52.50109039468566863 ) ) ;
#127188=CARTESIAN_POINT ( 'NONE',  ( 21.53943276465977519, -0.05219959533907433946, 103.7489096053143669 ) ) ;
#127190=CARTESIAN_POINT ( 'NONE',  ( -16.46253265017160317, 9.564922557960807481, 80.83224293864769550 ) ) ;
#127192=CARTESIAN_POINT ( 'NONE',  ( 8.314922557961029526, -14.29746914071037800, 35.41775706135234003 ) ) ;
#127194=CARTESIAN_POINT ( 'NONE',  ( 18.62759615963271287, -10.81492255796078972, 113.3322429386476955 ) ) ;
#127195=CARTESIAN_POINT ( 'NONE',  ( 8.314922557960818139, 14.29746914071049879, 64.58224293864769550 ) ) ;
#127196=CARTESIAN_POINT ( 'NONE',  ( 19.03943276465977164, -0.05219959533909143690, 68.74890960531436690 ) ) ;
#127197=CARTESIAN_POINT ( 'NONE',  ( -16.53943276465976808, -0.05219959533934237506, 38.75109039468567573 ) ) ;
#127198=CARTESIAN_POINT ( 'NONE',  ( 16.51473224551083163, -9.474510206698727899, 35.83442372801899722 ) ) ;
#127199=CARTESIAN_POINT ( 'NONE',  ( 5.719274019375673035, 21.55341960407619339, 52.29275706135236135 ) ) ;
#127200=CARTESIAN_POINT ( 'NONE',  ( -5.153800228976607833, 19.02544592524334988, 112.7094237280190043 ) ) ;
#127201=CARTESIAN_POINT ( 'NONE',  ( 13.89961937509977652, -13.97604488694527269, 58.12390960531436690 ) ) ;
#127202=CARTESIAN_POINT ( 'NONE',  ( -0.05219959533936034679, 19.03943276465977164, 87.50109039468567573 ) ) ;
#127203=CARTESIAN_POINT ( 'NONE',  ( -10.72451020669870658, -18.67979575497194134, 84.58442372801903275 ) ) ;
#127204=CARTESIAN_POINT ( 'NONE',  ( 0.05219959533936267826, -19.03943276465977164, 65.00109039468567573 ) ) ;
#127205=CARTESIAN_POINT ( 'NONE',  ( 9.474510206698971260, -16.51473224551069308, 42.91557627198103120 ) ) ;
#127206=CARTESIAN_POINT ( 'NONE',  ( -10.81492255796078084, -18.62759615963271287, 62.08224293864769550 ) ) ;
#127207=CARTESIAN_POINT ( 'NONE',  ( 16.52544592524342804, -4.483927247898539470, 63.54057627198103830 ) ) ;
#127208=CARTESIAN_POINT ( 'NONE',  ( 5.153800228976615827, -19.02544592524334988, 70.20942372801899012 ) ) ;
#127210=CARTESIAN_POINT ( 'NONE',  ( -19.02544592524334988, -5.153800228976617603, 23.95942372801900078 ) ) ;
#127211=CARTESIAN_POINT ( 'NONE',  ( 0.05219959533934541429, -16.53943276465976808, 105.0010903946856757 ) ) ;
#127212=CARTESIAN_POINT ( 'NONE',  ( -4.483927247898539470, -16.52544592524342804, 47.29057627198103120 ) ) ;
#127213=CARTESIAN_POINT ( 'NONE',  ( -5.823673210054431948, 21.52544592524334988, 92.70942372801901854 ) ) ;
#127215=CARTESIAN_POINT ( 'NONE',  ( -15.80617190586768217, 15.72974639402176855, 88.12609039468570415 ) ) ;
#127216=CARTESIAN_POINT ( 'NONE',  ( -21.53943276465977519, 0.05219959533907696930, 91.24890960531436690 ) ) ;
#127218=CARTESIAN_POINT ( 'NONE',  ( -13.97604488694527625, -13.89961937509977652, 56.87390960531434558 ) ) ;
#127219=CARTESIAN_POINT ( 'NONE',  ( -21.52544592524334988, -5.823673210054445271, 63.95942372801901854 ) ) ;
#127220=CARTESIAN_POINT ( 'NONE',  ( -19.03943276465977164, 0.05219959533909376836, 56.24890960531435979 ) ) ;
#127221=CARTESIAN_POINT ( 'NONE',  ( 16.51473224551069308, 9.474510206698969483, 64.16557627198102409 ) ) ;
#127222=CARTESIAN_POINT ( 'NONE',  ( 14.29746914071049879, -8.314922557960816363, 103.3322429386476955 ) ) ;
#127223=CARTESIAN_POINT ( 'NONE',  ( -5.049401038298153566, 19.05341960407611168, 110.2072429386476671 ) ) ;
#127224=CARTESIAN_POINT ( 'NONE',  ( 8.314922557960818139, 14.29746914071049879, 49.58224293864769550 ) ) ;
#127225=CARTESIAN_POINT ( 'NONE',  ( -19.05341960407611168, -5.049401038298163336, 26.45724293864769550 ) ) ;
#127226=CARTESIAN_POINT ( 'NONE',  ( -14.29746914071049879, 8.314922557960819915, 70.83224293864770971 ) ) ;
#127227=CARTESIAN_POINT ( 'NONE',  ( 21.55341960407610458, 5.719274019375980345, 93.95724293864770971 ) ) ;
#127228=CARTESIAN_POINT ( 'NONE',  ( -21.55341960407619339, 5.719274019375674811, 33.54275706135234714 ) ) ;
#127229=CARTESIAN_POINT ( 'NONE',  ( 5.049401038298161559, -19.05341960407611168, 22.70724293864769194 ) ) ;
#127230=CARTESIAN_POINT ( 'NONE',  ( 4.483927247898790824, -16.52544592524335698, 35.20942372801901854 ) ) ;
#127231=CARTESIAN_POINT ( 'NONE',  ( 21.53943276465977519, -0.05219959533907433946, 78.74890960531436690 ) ) ;
#127233=CARTESIAN_POINT ( 'NONE',  ( -10.72451020669870658, -18.67979575497194134, 104.5844237280190185 ) ) ;
#127234=CARTESIAN_POINT ( 'NONE',  ( -0.05219959533909027116, -19.03943276465977164, 87.49890960531436690 ) ) ;
#127235=CARTESIAN_POINT ( 'NONE',  ( -5.823673210054431948, 21.52544592524334988, 37.70942372801900433 ) ) ;
#127236=CARTESIAN_POINT ( 'NONE',  ( 0.05219959533907565091, 21.53943276465977519, 24.99890960531435624 ) ) ;
#127237=CARTESIAN_POINT ( 'NONE',  ( 8.314922557961029526, -14.29746914071037800, 100.4177570613523471 ) ) ;
#127238=CARTESIAN_POINT ( 'NONE',  ( -21.52544592524334988, -5.823673210054445271, 48.95942372801902565 ) ) ;
#127239=CARTESIAN_POINT ( 'NONE',  ( -10.81492255796105439, 18.62759615963255655, 87.91775706135234714 ) ) ;
#127240=CARTESIAN_POINT ( 'NONE',  ( -13.89961937509957401, -13.97604488694547875, 19.37609039468566507 ) ) ;
#127241=CARTESIAN_POINT ( 'NONE',  ( -14.29746914071037622, -8.314922557961029526, 89.16775706135236135 ) ) ;
#127242=CARTESIAN_POINT ( 'NONE',  ( 15.80617190586769283, -15.72974639402175789, 40.62609039468567573 ) ) ;
#127244=CARTESIAN_POINT ( 'NONE',  ( -5.153800228976328057, -19.02544592524343514, 27.29057627198103120 ) ) ;
#127245=CARTESIAN_POINT ( 'NONE',  ( -15.80617190586768217, 15.72974639402176855, 103.1260903946856757 ) ) ;
#127246=CARTESIAN_POINT ( 'NONE',  ( 0.05219959533909260263, 19.03943276465977164, 104.9989096053143669 ) ) ;
#127247=CARTESIAN_POINT ( 'NONE',  ( 21.53943276465977519, -0.05219959533907433946, 98.74890960531438111 ) ) ;
#127248=CARTESIAN_POINT ( 'NONE',  ( -5.719274019375978568, 21.55341960407610458, 65.20724293864768129 ) ) ;
#127249=LINE ( 'NONE', #1931, #19174 ) ;
#127250=CARTESIAN_POINT ( 'NONE',  ( -15.80617190586745835, -15.72974639402198527, 71.87390960531438111 ) ) ;
#127251=CARTESIAN_POINT ( 'NONE',  ( 16.52544592524335698, 4.483927247898782831, 46.45942372801901854 ) ) ;
#127252=CARTESIAN_POINT ( 'NONE',  ( -14.34966873604960291, -8.224510206698953496, 56.66557627198103830 ) ) ;
#127254=CARTESIAN_POINT ( 'NONE',  ( -19.03943276465977164, -0.05219959533935918106, 88.75109039468567573 ) ) ;
#127256=CARTESIAN_POINT ( 'NONE',  ( 12.06949235617739724, 12.14591786802326823, 31.87609039468567929 ) ) ;
#127257=CARTESIAN_POINT ( 'NONE',  ( 15.72974639402199770, -15.80617190586745480, 103.1239096053143811 ) ) ;
#127258=CARTESIAN_POINT ( 'NONE',  ( 15.72974639402199770, -15.80617190586745480, 78.12390960531436690 ) ) ;
#127259=CARTESIAN_POINT ( 'NONE',  ( 5.153800228976335163, 19.02544592524342804, 109.7905762719810099 ) ) ;
#127260=CARTESIAN_POINT ( 'NONE',  ( 4.483927247898790824, -16.52544592524335698, 55.20942372801902565 ) ) ;
#127261=CARTESIAN_POINT ( 'NONE',  ( -19.02544592524342804, 5.153800228976336051, 76.04057627198102409 ) ) ;
#127262=CARTESIAN_POINT ( 'NONE',  ( 5.719274019375673035, 21.55341960407619339, 27.29275706135234358 ) ) ;
#127263=CARTESIAN_POINT ( 'NONE',  ( -9.564922557961040184, 16.46253265017147172, 102.9177570613523329 ) ) ;
#127264=CARTESIAN_POINT ( 'NONE',  ( 16.51473224551069308, 9.474510206698969483, 114.1655762719810241 ) ) ;
#127265=CARTESIAN_POINT ( 'NONE',  ( 16.46253265017160672, -9.564922557960803928, 83.33224293864768129 ) ) ;
#127266=CARTESIAN_POINT ( 'NONE',  ( 5.823673210054125526, 21.52544592524343514, 84.79057627198102409 ) ) ;
#127267=CARTESIAN_POINT ( 'NONE',  ( 13.97604488694527802, 13.89961937509977652, 64.37390960531436690 ) ) ;
#127268=CARTESIAN_POINT ( 'NONE',  ( -17.31747979337949417, -6.344076630961023255, 61.37944868065187620 ) ) ;
#127269=CARTESIAN_POINT ( 'NONE',  ( 16.53943276465976808, -0.05219959533910856209, 63.74890960531435979 ) ) ;
#127270=CARTESIAN_POINT ( 'NONE',  ( 0.05219959533909260263, 19.03943276465977164, 114.9989096053143669 ) ) ;
#127272=CARTESIAN_POINT ( 'NONE',  ( -10.72451020669898014, 18.67979575497178502, 110.4155762719810383 ) ) ;
#127273=CARTESIAN_POINT ( 'NONE',  ( -13.97604488694547697, 13.89961937509957934, 58.12609039468566863 ) ) ;
#127274=CARTESIAN_POINT ( 'NONE',  ( 0.05219959533907565091, 21.53943276465977519, 24.99890960531435624 ) ) ;
#127275=CARTESIAN_POINT ( 'NONE',  ( 15.80617190586746368, 15.72974639402197994, 59.37390960531436690 ) ) ;
#127277=CARTESIAN_POINT ( 'NONE',  ( -5.153800228976328057, -19.02544592524343514, 87.29057627198103830 ) ) ;
#127278=CARTESIAN_POINT ( 'NONE',  ( -10.81492255796105439, 18.62759615963255655, 82.91775706135234714 ) ) ;
#127279=CARTESIAN_POINT ( 'NONE',  ( 16.46253265017160672, -9.564922557960803928, 53.33224293864768839 ) ) ;
#127280=CARTESIAN_POINT ( 'NONE',  ( 16.53943276465976808, -0.05219959533910856209, 93.74890960531436690 ) ) ;
#127281=CARTESIAN_POINT ( 'NONE',  ( 16.52544592524335698, 4.483927247898782831, 36.45942372801901143 ) ) ;
#127282=CARTESIAN_POINT ( 'NONE',  ( -5.823673210054431948, 21.52544592524334988, 72.70942372801901854 ) ) ;
#127284=CARTESIAN_POINT ( 'NONE',  ( 9.474510206698729675, 16.51473224551082808, 22.08442372801899722 ) ) ;
#127285=CARTESIAN_POINT ( 'NONE',  ( -19.02544592524334988, -5.153800228976617603, 83.95942372801901854 ) ) ;
#127286=CARTESIAN_POINT ( 'NONE',  ( -13.97604488694547697, 13.89961937509957934, 43.12609039468566152 ) ) ;
#127288=CARTESIAN_POINT ( 'NONE',  ( -5.823673210054431948, 21.52544592524334988, 32.70942372801900433 ) ) ;
#127289=DIRECTION ( 'NONE',  ( -0.000000000000000000, -0.000000000000000000, 1.000000000000000000 ) ) ;
#127290=CARTESIAN_POINT ( 'NONE',  ( -5.153800228976607833, 19.02544592524334988, 27.70942372801899722 ) ) ;
#127291=CARTESIAN_POINT ( 'NONE',  ( 5.153800228976335163, 19.02544592524342804, 59.79057627198100988 ) ) ;
#127292=CARTESIAN_POINT ( 'NONE',  ( -19.03943276465977164, -0.05219959533935918106, 28.75109039468566507 ) ) ;
#127293=CARTESIAN_POINT ( 'NONE',  ( -16.53943276465976808, -0.05219959533934237506, 98.75109039468568994 ) ) ;
#127294=CARTESIAN_POINT ( 'NONE',  ( -21.53943276465977519, 0.05219959533907696930, 21.24890960531436690 ) ) ;
#127295=CARTESIAN_POINT ( 'NONE',  ( 15.72974639402176855, 15.80617190586768217, 81.87609039468568994 ) ) ;
#127297=CARTESIAN_POINT ( 'NONE',  ( -17.50000000000149569, -3.202012800152108873, 35.07177583972763557 ) ) ;
#127298=CARTESIAN_POINT ( 'NONE',  ( -18.67979575497193778, 10.72451020669871902, 88.33442372801901854 ) ) ;
#127300=CARTESIAN_POINT ( 'NONE',  ( 9.564922557960805705, 16.46253265017160317, 94.58224293864769550 ) ) ;
#127302=EDGE_CURVE ( 'NONE', #193812, #163522, #177674, .T. ) ;
#127305=CARTESIAN_POINT ( 'NONE',  ( -19.03943276465977164, 0.05219959533909376836, 46.24890960531435979 ) ) ;
#127306=CARTESIAN_POINT ( 'NONE',  ( 0.05219959533907565091, 21.53943276465977519, 54.99890960531435269 ) ) ;
#127307=CARTESIAN_POINT ( 'NONE',  ( 16.52544592524342804, -4.483927247898539470, 28.54057627198103120 ) ) ;
#127308=CARTESIAN_POINT ( 'NONE',  ( 12.14591786802309770, 12.06949235617756955, 94.37390960531436690 ) ) ;
#127309=CARTESIAN_POINT ( 'NONE',  ( -5.049401038298153566, 19.05341960407611168, 100.2072429386476955 ) ) ;
#127310=CARTESIAN_POINT ( 'NONE',  ( -0.05219959533936034679, 19.03943276465977164, 22.50109039468566152 ) ) ;
#127311=CARTESIAN_POINT ( 'NONE',  ( -16.46253265017160317, 9.564922557960807481, 35.83224293864768839 ) ) ;
#127312=CARTESIAN_POINT ( 'NONE',  ( 14.29746914071049879, -8.314922557960816363, 98.33224293864769550 ) ) ;
#127313=CARTESIAN_POINT ( 'NONE',  ( 10.81492255796106328, -18.62759615963255655, 50.41775706135235424 ) ) ;
#127314=CARTESIAN_POINT ( 'NONE',  ( -5.823673210054116645, -21.52544592524344225, 92.29057627198103830 ) ) ;
#127315=CARTESIAN_POINT ( 'NONE',  ( -13.97604488694547697, 13.89961937509957934, 63.12609039468566152 ) ) ;
#127317=CARTESIAN_POINT ( 'NONE',  ( -19.02544592524342804, 5.153800228976336051, 111.0405762719810099 ) ) ;
#127318=CARTESIAN_POINT ( 'NONE',  ( 14.29746914071049879, -8.314922557960816363, 73.33224293864769550 ) ) ;
#127319=CARTESIAN_POINT ( 'NONE',  ( -9.474510206698720793, -16.51473224551083518, 39.58442372801899722 ) ) ;
#127320=CARTESIAN_POINT ( 'NONE',  ( -19.02544592524342804, 5.153800228976336051, 66.04057627198103830 ) ) ;
#127321=CARTESIAN_POINT ( 'NONE',  ( 16.53943276465976808, -0.05219959533910856209, 58.74890960531436690 ) ) ;
#127322=CARTESIAN_POINT ( 'NONE',  ( 9.474510206698729675, 16.51473224551082808, 82.08442372801899012 ) ) ;
#127323=CARTESIAN_POINT ( 'NONE',  ( -21.53943276465977519, 0.05219959533907696930, 41.24890960531435269 ) ) ;
#127325=CARTESIAN_POINT ( 'NONE',  ( -8.224510206698948167, 14.34966873604960824, 100.4155762719810241 ) ) ;
#127327=CARTESIAN_POINT ( 'NONE',  ( 19.03943276465977164, -0.05219959533909143690, 53.74890960531436690 ) ) ;
#127328=CARTESIAN_POINT ( 'NONE',  ( -21.53943276465977519, 0.05219959533907696930, 66.24890960531436690 ) ) ;
#127329=CARTESIAN_POINT ( 'NONE',  ( -16.51473224551069308, -9.474510206698971260, 46.66557627198102409 ) ) ;
#127330=CARTESIAN_POINT ( 'NONE',  ( 8.314922557961029526, -14.29746914071037800, 80.41775706135234714 ) ) ;
#127331=CARTESIAN_POINT ( 'NONE',  ( 16.51473224551069308, 9.474510206698969483, 74.16557627198103830 ) ) ;
#127332=CARTESIAN_POINT ( 'NONE',  ( -5.153800228976607833, 19.02544592524334988, 57.70942372801899012 ) ) ;
#127333=CARTESIAN_POINT ( 'NONE',  ( 10.81492255796106328, -18.62759615963255655, 65.41775706135234714 ) ) ;
#127334=CARTESIAN_POINT ( 'NONE',  ( -15.72974639402197994, 15.80617190586746368, 55.62390960531436690 ) ) ;
#127335=CARTESIAN_POINT ( 'NONE',  ( 0.05219959533909260263, 19.03943276465977164, 99.99890960531436690 ) ) ;
#127336=CARTESIAN_POINT ( 'NONE',  ( 16.52544592524342804, -4.483927247898539470, 113.5405762719810383 ) ) ;
#127337=CARTESIAN_POINT ( 'NONE',  ( 4.379528057220092307, 16.55341960407617563, 87.29275706135236135 ) ) ;
#127338=CARTESIAN_POINT ( 'NONE',  ( -19.02544592524334988, -5.153800228976617603, 108.9594237280189759 ) ) ;
#127339=CARTESIAN_POINT ( 'NONE',  ( -9.564922557960796823, -16.46253265017161027, 27.08224293864769550 ) ) ;
#127341=CARTESIAN_POINT ( 'NONE',  ( -5.823673210054431948, 21.52544592524334988, 92.70942372801901854 ) ) ;
#127343=CARTESIAN_POINT ( 'NONE',  ( -0.05219959533910754901, -16.53943276465976808, 57.49890960531435979 ) ) ;
#127344=CARTESIAN_POINT ( 'NONE',  ( -16.55341960407611168, -4.379528057220339221, 66.45724293864768129 ) ) ;
#127345=CARTESIAN_POINT ( 'NONE',  ( -0.05219959533907301413, -21.53943276465977519, 97.49890960531436690 ) ) ;
#127346=CARTESIAN_POINT ( 'NONE',  ( -21.55341960407610458, -5.719274019375992779, 86.45724293864770971 ) ) ;
#127348=CARTESIAN_POINT ( 'NONE',  ( 18.67979575497178502, 10.72451020669898547, 39.16557627198102409 ) ) ;
#127350=CARTESIAN_POINT ( 'NONE',  ( 0.05219959533934541429, -16.53943276465976808, 70.00109039468568994 ) ) ;
#127351=CARTESIAN_POINT ( 'NONE',  ( -14.34966873604960291, -8.224510206698953496, 96.66557627198102409 ) ) ;
#127352=CARTESIAN_POINT ( 'NONE',  ( -13.89961937509977652, 13.97604488694528158, 45.62390960531433848 ) ) ;
#127355=CARTESIAN_POINT ( 'NONE',  ( 12.14591786802327356, -12.06949235617739191, 100.6260903946857184 ) ) ;
#127356=CARTESIAN_POINT ( 'NONE',  ( 18.62759615963255655, 10.81492255796105972, 31.66775706135234358 ) ) ;
#127357=CARTESIAN_POINT ( 'NONE',  ( 9.474510206698971260, -16.51473224551069308, 82.91557627198103830 ) ) ;
#127358=CARTESIAN_POINT ( 'NONE',  ( 5.719274019375673035, 21.55341960407619339, 72.29275706135236135 ) ) ;
#127359=CARTESIAN_POINT ( 'NONE',  ( -19.03943276465977164, 0.05219959533909376836, 116.2489096053143669 ) ) ;
#127363=CARTESIAN_POINT ( 'NONE',  ( -10.72451020669870658, -18.67979575497194134, 59.58442372801901854 ) ) ;
#127364=CARTESIAN_POINT ( 'NONE',  ( 13.97604488694527802, 13.89961937509977652, 44.37390960531435269 ) ) ;
#127365=CARTESIAN_POINT ( 'NONE',  ( -13.97604488694527625, -13.89961937509977652, 21.87390960531435979 ) ) ;
#127366=CARTESIAN_POINT ( 'NONE',  ( -19.03943276465977164, -0.05219959533935918106, 73.75109039468566152 ) ) ;
#127367=CARTESIAN_POINT ( 'NONE',  ( -0.05219959533937732626, 21.53943276465977519, 22.50109039468567573 ) ) ;
#127368=CARTESIAN_POINT ( 'NONE',  ( -9.564922557961040184, 16.46253265017147172, 62.91775706135233293 ) ) ;
#127369=CARTESIAN_POINT ( 'NONE',  ( -0.05219959533909027116, -19.03943276465977164, 27.49890960531435624 ) ) ;
#127370=CARTESIAN_POINT ( 'NONE',  ( -16.52544592524335698, -4.483927247898792601, 93.95942372801903275 ) ) ;
#127371=CARTESIAN_POINT ( 'NONE',  ( -9.564922557961040184, 16.46253265017147172, 62.91775706135233293 ) ) ;
#127372=CARTESIAN_POINT ( 'NONE',  ( -4.483927247898782831, 16.52544592524335698, 112.7094237280190328 ) ) ;
#127373=CARTESIAN_POINT ( 'NONE',  ( 13.89961937509957401, 13.97604488694547697, 51.87609039468566863 ) ) ;
#127375=CARTESIAN_POINT ( 'NONE',  ( 13.97604488694527802, 13.89961937509977652, 89.37390960531436690 ) ) ;
#127376=CARTESIAN_POINT ( 'NONE',  ( -5.719274019375665041, -21.55341960407619695, 89.79275706135236135 ) ) ;
#127377=CARTESIAN_POINT ( 'NONE',  ( -5.823673210054431948, 21.52544592524334988, 107.7094237280190328 ) ) ;
#127379=CARTESIAN_POINT ( 'NONE',  ( -18.67979575497193778, 10.72451020669871902, 88.33442372801901854 ) ) ;
#127380=CARTESIAN_POINT ( 'NONE',  ( -16.55341960407617563, 4.379528057220093196, 33.54275706135234714 ) ) ;
#127382=CARTESIAN_POINT ( 'NONE',  ( -9.564922557960796823, -16.46253265017161027, 97.08224293864769550 ) ) ;
#127383=CARTESIAN_POINT ( 'NONE',  ( 10.72451020669898902, -18.67979575497178502, 32.91557627198102409 ) ) ;
#127385=CARTESIAN_POINT ( 'NONE',  ( 13.97604488694527802, 13.89961937509977652, 79.37390960531435269 ) ) ;
#127386=CARTESIAN_POINT ( 'NONE',  ( -16.31925111598405920, 7.325300261831753978, 100.1642453896716489 ) ) ;
#127388=CARTESIAN_POINT ( 'NONE',  ( 16.51473224551083163, -9.474510206698727899, 65.83442372801900433 ) ) ;
#127389=CARTESIAN_POINT ( 'NONE',  ( 19.02544592524343514, -5.153800228976328945, 108.5405762719810383 ) ) ;
#127390=CARTESIAN_POINT ( 'NONE',  ( -21.55341960407619339, 5.719274019375674811, 103.5427570613523613 ) ) ;
#127391=CARTESIAN_POINT ( 'NONE',  ( -14.29746914071049879, 8.314922557960819915, 100.8322429386477097 ) ) ;
#127392=CARTESIAN_POINT ( 'NONE',  ( 18.67979575497178502, 10.72451020669898547, 44.16557627198103120 ) ) ;
#127394=CARTESIAN_POINT ( 'NONE',  ( 0.05219959533907565091, 21.53943276465977519, 34.99890960531435979 ) ) ;
#127395=CARTESIAN_POINT ( 'NONE',  ( -4.379528057220328563, 16.55341960407611168, 100.2072429386476955 ) ) ;
#127397=CARTESIAN_POINT ( 'NONE',  ( -9.564922557961040184, 16.46253265017147172, 52.91775706135233293 ) ) ;
#127398=CARTESIAN_POINT ( 'NONE',  ( 14.29746914071049879, -8.314922557960816363, 33.33224293864769550 ) ) ;
#127399=CARTESIAN_POINT ( 'NONE',  ( 16.46253265017160672, -9.564922557960803928, 103.3322429386476955 ) ) ;
#127400=CARTESIAN_POINT ( 'NONE',  ( -15.72974639402176322, -15.80617190586768395, 79.37609039468567573 ) ) ;
#127401=CARTESIAN_POINT ( 'NONE',  ( -10.72451020669898014, 18.67979575497178502, 60.41557627198102409 ) ) ;
#127402=CARTESIAN_POINT ( 'NONE',  ( 0.05219959533937995610, -21.53943276465977519, 50.00109039468568994 ) ) ;
#127403=CARTESIAN_POINT ( 'NONE',  ( -10.81492255796078084, -18.62759615963271287, 102.0822429386476955 ) ) ;
#127404=CARTESIAN_POINT ( 'NONE',  ( -5.719274019375665041, -21.55341960407619695, 34.79275706135235424 ) ) ;
#127405=CARTESIAN_POINT ( 'NONE',  ( -12.06949235617756955, 12.14591786802309770, 115.6239096053143669 ) ) ;
#127406=CARTESIAN_POINT ( 'NONE',  ( 5.153800228976335163, 19.02544592524342804, 79.79057627198102409 ) ) ;
#127407=CARTESIAN_POINT ( 'NONE',  ( 12.06949235617739724, 12.14591786802326823, 76.87609039468567573 ) ) ;
#127408=CARTESIAN_POINT ( 'NONE',  ( -16.52544592524342804, 4.483927247898546575, 111.0405762719810525 ) ) ;
#127409=CARTESIAN_POINT ( 'NONE',  ( -5.049401038298153566, 19.05341960407611168, 110.2072429386476671 ) ) ;
#127410=CARTESIAN_POINT ( 'NONE',  ( -8.224510206698948167, 14.34966873604960824, 60.41557627198102409 ) ) ;
#127411=CARTESIAN_POINT ( 'NONE',  ( 16.53943276465976808, 0.05219959533934440121, 111.2510903946856899 ) ) ;
#127412=CARTESIAN_POINT ( 'NONE',  ( 13.97604488694527802, 13.89961937509977652, 54.37390960531435979 ) ) ;
#127413=CARTESIAN_POINT ( 'NONE',  ( 9.474510206698971260, -16.51473224551069308, 22.91557627198102765 ) ) ;
#127414=CARTESIAN_POINT ( 'NONE',  ( -5.719274019375978568, 21.55341960407610458, 45.20724293864769550 ) ) ;
#127415=CARTESIAN_POINT ( 'NONE',  ( -19.02544592524334988, -5.153800228976617603, 23.95942372801900078 ) ) ;
#127418=CARTESIAN_POINT ( 'NONE',  ( -16.52544592524342804, 4.483927247898546575, 36.04057627198102409 ) ) ;
#127419=CARTESIAN_POINT ( 'NONE',  ( -10.72451020669870658, -18.67979575497194134, 49.58442372801901143 ) ) ;
#127420=CARTESIAN_POINT ( 'NONE',  ( 16.46253265017160672, -9.564922557960803928, 113.3322429386476955 ) ) ;
#127421=CARTESIAN_POINT ( 'NONE',  ( -14.34966873604972548, 8.224510206698743886, 58.33442372801901143 ) ) ;
#127423=CARTESIAN_POINT ( 'NONE',  ( 19.03943276465977164, 0.05219959533936151252, 66.25109039468567573 ) ) ;
#127424=CARTESIAN_POINT ( 'NONE',  ( 12.06949235617757843, -12.14591786802309237, 23.12390960531436335 ) ) ;
#127425=CARTESIAN_POINT ( 'NONE',  ( 4.483927247898790824, -16.52544592524335698, 100.2094237280190043 ) ) ;
#127426=CARTESIAN_POINT ( 'NONE',  ( -19.02544592524342804, 5.153800228976336051, 36.04057627198100988 ) ) ;
#127427=CARTESIAN_POINT ( 'NONE',  ( 19.05341960407611168, 5.049401038298154454, 58.95724293864768129 ) ) ;
#127428=CARTESIAN_POINT ( 'NONE',  ( 19.03943276465977164, -0.05219959533909143690, 23.74890960531435269 ) ) ;
#127429=CARTESIAN_POINT ( 'NONE',  ( -10.81492255796105439, 18.62759615963255655, 27.91775706135234358 ) ) ;
#127430=CARTESIAN_POINT ( 'NONE',  ( -13.89961937509977652, 13.97604488694528158, 45.62390960531433848 ) ) ;
#127431=FACE_OUTER_BOUND ( 'NONE', #49691, .T. ) ;
#127432=CARTESIAN_POINT ( 'NONE',  ( 0.05219959533909260263, 19.03943276465977164, 39.99890960531436690 ) ) ;
#127433=CARTESIAN_POINT ( 'NONE',  ( 15.80617190586746368, 15.72974639402197994, 24.37390960531435979 ) ) ;
#127435=CARTESIAN_POINT ( 'NONE',  ( -21.55341960407619339, 5.719274019375674811, 63.54275706135234003 ) ) ;
#127436=CARTESIAN_POINT ( 'NONE',  ( 16.53943276465976808, -0.05219959533910856209, 103.7489096053143669 ) ) ;
#127437=CARTESIAN_POINT ( 'NONE',  ( 16.46253265017160672, -9.564922557960803928, 108.3322429386476955 ) ) ;
#127438=CARTESIAN_POINT ( 'NONE',  ( 8.314922557961029526, -14.29746914071037800, 80.41775706135234714 ) ) ;
#127439=CARTESIAN_POINT ( 'NONE',  ( 21.52544592524334988, 5.823673210054432836, 86.45942372801901854 ) ) ;
#127440=CARTESIAN_POINT ( 'NONE',  ( -12.06949235617739369, -12.14591786802326823, 59.37609039468568284 ) ) ;
#127441=CARTESIAN_POINT ( 'NONE',  ( 9.564922557960805705, 16.46253265017160317, 94.58224293864769550 ) ) ;
#127442=CARTESIAN_POINT ( 'NONE',  ( 4.483927247898790824, -16.52544592524335698, 35.20942372801901854 ) ) ;
#127443=CARTESIAN_POINT ( 'NONE',  ( 8.224510206698742110, 14.34966873604972548, 27.08442372801901854 ) ) ;
#127444=CARTESIAN_POINT ( 'NONE',  ( 0.05219959533934541429, -16.53943276465976808, 85.00109039468568994 ) ) ;
#127445=CARTESIAN_POINT ( 'NONE',  ( 16.51473224551083163, -9.474510206698727899, 110.8344237280190043 ) ) ;
#127446=CARTESIAN_POINT ( 'NONE',  ( 18.62759615963271287, -10.81492255796078972, 98.33224293864769550 ) ) ;
#127447=CARTESIAN_POINT ( 'NONE',  ( -8.314922557960811034, -14.29746914071050412, 97.08224293864770971 ) ) ;
#127448=CARTESIAN_POINT ( 'NONE',  ( -19.03943276465977164, -0.05219959533935918106, 98.75109039468567573 ) ) ;
#127449=CARTESIAN_POINT ( 'NONE',  ( 4.379528057220092307, 16.55341960407617563, 67.29275706135234714 ) ) ;
#127451=CARTESIAN_POINT ( 'NONE',  ( 0.05219959533936267826, -19.03943276465977164, 65.00109039468567573 ) ) ;
#127452=CARTESIAN_POINT ( 'NONE',  ( -0.05219959533910754901, -16.53943276465976808, 42.49890960531435979 ) ) ;
#127453=CARTESIAN_POINT ( 'NONE',  ( 14.29746914071049879, -8.314922557960816363, 28.33224293864769550 ) ) ;
#127454=CARTESIAN_POINT ( 'NONE',  ( 0.05219959533910956823, 16.53943276465976808, 89.99890960531438111 ) ) ;
#127455=CARTESIAN_POINT ( 'NONE',  ( 0.05219959533936267826, -19.03943276465977164, 35.00109039468566863 ) ) ;
#127457=CARTESIAN_POINT ( 'NONE',  ( -21.53943276465977519, -0.05219959533937600094, 33.75109039468568284 ) ) ;
#127458=CARTESIAN_POINT ( 'NONE',  ( -0.05219959533936034679, 19.03943276465977164, 92.50109039468566152 ) ) ;
#127460=CARTESIAN_POINT ( 'NONE',  ( -19.05341960407611168, -5.049401038298163336, 96.45724293864769550 ) ) ;
#127461=CARTESIAN_POINT ( 'NONE',  ( 19.05341960407611168, 5.049401038298154454, 88.95724293864769550 ) ) ;
#127462=CARTESIAN_POINT ( 'NONE',  ( -15.80617190586745835, -15.72974639402198527, 56.87390960531436690 ) ) ;
#127463=CARTESIAN_POINT ( 'NONE',  ( 16.52544592524342804, -4.483927247898539470, 98.54057627198105251 ) ) ;
#127464=CARTESIAN_POINT ( 'NONE',  ( 5.153800228976335163, 19.02544592524342804, 74.79057627198103830 ) ) ;
#127465=CARTESIAN_POINT ( 'NONE',  ( -5.049401038298153566, 19.05341960407611168, 30.20724293864768839 ) ) ;
#127466=CARTESIAN_POINT ( 'NONE',  ( 5.823673210054444382, -21.52544592524334988, 35.20942372801901854 ) ) ;
#127467=CARTESIAN_POINT ( 'NONE',  ( 21.53943276465977519, 0.05219959533937863772, 76.25109039468568994 ) ) ;
#127468=CARTESIAN_POINT ( 'NONE',  ( -19.05341960407611168, -5.049401038298163336, 56.45724293864768129 ) ) ;
#127469=CARTESIAN_POINT ( 'NONE',  ( 14.29746914071037800, 8.314922557961029526, 76.66775706135234714 ) ) ;
#127470=CARTESIAN_POINT ( 'NONE',  ( -15.72974639402176322, -15.80617190586768395, 29.37609039468568284 ) ) ;
#127471=CARTESIAN_POINT ( 'NONE',  ( 10.72451020669871369, 18.67979575497193778, 32.08442372801901854 ) ) ;
#127472=CARTESIAN_POINT ( 'NONE',  ( 5.049401038297881783, 19.05341960407617563, 47.29275706135231161 ) ) ;
#127473=CARTESIAN_POINT ( 'NONE',  ( -13.89961937509977652, 13.97604488694528158, 75.62390960531438111 ) ) ;
#127474=CARTESIAN_POINT ( 'NONE',  ( 16.46253265017146816, 9.564922557961045513, 31.66775706135232937 ) ) ;
#127475=CARTESIAN_POINT ( 'NONE',  ( 5.823673210054444382, -21.52544592524334988, 80.20942372801901854 ) ) ;
#127477=CARTESIAN_POINT ( 'NONE',  ( -15.72974639402197994, 15.80617190586746368, 75.62390960531439532 ) ) ;
#127478=CARTESIAN_POINT ( 'NONE',  ( -16.53943276465976808, 0.05219959533911058130, 51.24890960531436690 ) ) ;
#127479=CARTESIAN_POINT ( 'NONE',  ( 15.72974639402176855, 15.80617190586768217, 96.87609039468568994 ) ) ;
#127480=CARTESIAN_POINT ( 'NONE',  ( -0.05219959533936034679, 19.03943276465977164, 27.50109039468566507 ) ) ;
#127481=CARTESIAN_POINT ( 'NONE',  ( 8.224510206698953496, -14.34966873604960469, 67.91557627198102409 ) ) ;
#127482=CARTESIAN_POINT ( 'NONE',  ( 19.05341960407611168, 5.049401038298154454, 23.95724293864769194 ) ) ;
#127483=CARTESIAN_POINT ( 'NONE',  ( -9.474510206698720793, -16.51473224551083518, 74.58442372801900433 ) ) ;
#127484=CARTESIAN_POINT ( 'NONE',  ( -14.29746914071049879, 8.314922557960819915, 40.83224293864769550 ) ) ;
#127485=CARTESIAN_POINT ( 'NONE',  ( 18.67979575497194134, -10.72451020669871369, 85.83442372801901854 ) ) ;
#127486=CARTESIAN_POINT ( 'NONE',  ( -5.049401038298153566, 19.05341960407611168, 85.20724293864766707 ) ) ;
#127487=CARTESIAN_POINT ( 'NONE',  ( 19.02544592524334988, 5.153800228976608722, 51.45942372801900433 ) ) ;
#127488=CARTESIAN_POINT ( 'NONE',  ( -0.05219959533907301413, -21.53943276465977519, 47.49890960531435979 ) ) ;
#127489=CARTESIAN_POINT ( 'NONE',  ( 18.62759615963271287, -10.81492255796078972, 108.3322429386477097 ) ) ;
#127490=CARTESIAN_POINT ( 'NONE',  ( 0.05219959533934541429, -16.53943276465976808, 20.00109039468568639 ) ) ;
#127491=CARTESIAN_POINT ( 'NONE',  ( -4.483927247898782831, 16.52544592524335698, 67.70942372801901854 ) ) ;
#127493=CARTESIAN_POINT ( 'NONE',  ( -18.62759615963270932, 10.81492255796079327, 105.8322429386476955 ) ) ;
#127494=CARTESIAN_POINT ( 'NONE',  ( 0.05219959533910956823, 16.53943276465976808, 104.9989096053143669 ) ) ;
#127495=CARTESIAN_POINT ( 'NONE',  ( -17.49999999999999645, -5.500000000000005329, 31.28230962303567253 ) ) ;
#127496=CARTESIAN_POINT ( 'NONE',  ( -12.14591786802326823, 12.06949235617739902, 38.12609039468567573 ) ) ;
#127497=CARTESIAN_POINT ( 'NONE',  ( -21.52544592524343514, 5.823673210054127303, 61.04057627198103120 ) ) ;
#127498=CARTESIAN_POINT ( 'NONE',  ( 8.224510206698742110, 14.34966873604972548, 107.0844237280190043 ) ) ;
#127499=CARTESIAN_POINT ( 'NONE',  ( -19.05341960407611168, -5.049401038298163336, 31.45724293864769550 ) ) ;
#127500=CARTESIAN_POINT ( 'NONE',  ( 0.05219959533934541429, -16.53943276465976808, 70.00109039468568994 ) ) ;
#127501=CARTESIAN_POINT ( 'NONE',  ( 19.02544592524334988, 5.153800228976608722, 66.45942372801899012 ) ) ;
#127502=CARTESIAN_POINT ( 'NONE',  ( 10.81492255796106328, -18.62759615963255655, 45.41775706135234003 ) ) ;
#127504=CARTESIAN_POINT ( 'NONE',  ( 0.05219959533907565091, 21.53943276465977519, 59.99890960531436690 ) ) ;
#127505=CARTESIAN_POINT ( 'NONE',  ( -14.34966873604972548, 8.224510206698743886, 93.33442372801901854 ) ) ;
#127506=CARTESIAN_POINT ( 'NONE',  ( -10.81492255796105439, 18.62759615963255655, 87.91775706135234714 ) ) ;
#127507=CARTESIAN_POINT ( 'NONE',  ( -5.823673210054116645, -21.52544592524344225, 57.29057627198103120 ) ) ;
#127508=CARTESIAN_POINT ( 'NONE',  ( 21.55341960407610458, 5.719274019375980345, 28.95724293864769905 ) ) ;
#127509=CARTESIAN_POINT ( 'NONE',  ( -14.34966873604972548, 8.224510206698743886, 83.33442372801903275 ) ) ;
#127510=CARTESIAN_POINT ( 'NONE',  ( -10.72451020669898014, 18.67979575497178502, 30.41557627198101699 ) ) ;
#127512=CARTESIAN_POINT ( 'NONE',  ( 5.153800228976335163, 19.02544592524342804, 99.79057627198102409 ) ) ;
#127513=CARTESIAN_POINT ( 'NONE',  ( 14.34966873604960469, 8.224510206698951720, 24.16557627198103120 ) ) ;
#127515=CARTESIAN_POINT ( 'NONE',  ( -0.05219959533910754901, -16.53943276465976808, 107.4989096053143669 ) ) ;
#127516=CARTESIAN_POINT ( 'NONE',  ( -21.55341960407610458, -5.719274019375992779, 61.45724293864770260 ) ) ;
#127517=CARTESIAN_POINT ( 'NONE',  ( 8.314922557961029526, -14.29746914071037800, 85.41775706135236135 ) ) ;
#127518=CARTESIAN_POINT ( 'NONE',  ( 10.72451020669871369, 18.67979575497193778, 42.08442372801901854 ) ) ;
#127519=CARTESIAN_POINT ( 'NONE',  ( -5.049401038297874678, -19.05341960407617918, 104.7927570613523471 ) ) ;
#127520=CARTESIAN_POINT ( 'NONE',  ( 16.53943276465976808, -0.05219959533910856209, 98.74890960531438111 ) ) ;
#127521=CARTESIAN_POINT ( 'NONE',  ( -5.153800228976607833, 19.02544592524334988, 107.7094237280189759 ) ) ;
#127523=CARTESIAN_POINT ( 'NONE',  ( 0.05219959533909260263, 19.03943276465977164, 44.99890960531435979 ) ) ;
#127525=CARTESIAN_POINT ( 'NONE',  ( 16.51473224551069308, 9.474510206698969483, 89.16557627198103830 ) ) ;
#127526=CARTESIAN_POINT ( 'NONE',  ( -8.224510206698735004, -14.34966873604973081, 74.58442372801901854 ) ) ;
#127527=CARTESIAN_POINT ( 'NONE',  ( 21.55341960407619695, -5.719274019375665929, 101.0427570613523756 ) ) ;
#127528=CARTESIAN_POINT ( 'NONE',  ( -21.55341960407610458, -5.719274019375992779, 66.45724293864768129 ) ) ;
#127530=CARTESIAN_POINT ( 'NONE',  ( 0.05219959533934541429, -16.53943276465976808, 85.00109039468568994 ) ) ;
#127531=CARTESIAN_POINT ( 'NONE',  ( 19.05341960407617918, -5.049401038297876454, 81.04275706135231871 ) ) ;
#127532=CARTESIAN_POINT ( 'NONE',  ( -16.46253265017160317, 9.564922557960807481, 30.83224293864769550 ) ) ;
#127533=CARTESIAN_POINT ( 'NONE',  ( -5.049401038298153566, 19.05341960407611168, 80.20724293864769550 ) ) ;
#127535=CARTESIAN_POINT ( 'NONE',  ( 5.049401038298161559, -19.05341960407611168, 27.70724293864769550 ) ) ;
#127536=CARTESIAN_POINT ( 'NONE',  ( -19.05341960407617563, 5.049401038297882671, 73.54275706135233293 ) ) ;
#127538=CARTESIAN_POINT ( 'NONE',  ( -13.97604488694527625, -13.89961937509977652, 101.8739096053143811 ) ) ;
#127539=CARTESIAN_POINT ( 'NONE',  ( 14.29746914071049879, -8.314922557960816363, 48.33224293864770260 ) ) ;
#127540=CARTESIAN_POINT ( 'NONE',  ( -21.53943276465977519, 0.05219959533907696930, 56.24890960531436690 ) ) ;
#127542=CARTESIAN_POINT ( 'NONE',  ( -17.49999999999999645, 5.068104630630383411, 105.7281840534002981 ) ) ;
#127544=CARTESIAN_POINT ( 'NONE',  ( 16.46253265017146816, 9.564922557961045513, 26.66775706135234003 ) ) ;
#127546=CARTESIAN_POINT ( 'NONE',  ( -19.03943276465977164, 0.05219959533909376836, 51.24890960531436690 ) ) ;
#127547=CARTESIAN_POINT ( 'NONE',  ( -9.474510206698964154, 16.51473224551069663, 70.41557627198102409 ) ) ;
#127548=CARTESIAN_POINT ( 'NONE',  ( 4.379528057220092307, 16.55341960407617563, 42.29275706135235424 ) ) ;
#127551=CARTESIAN_POINT ( 'NONE',  ( -4.483927247898782831, 16.52544592524335698, 72.70942372801901854 ) ) ;
#127552=CARTESIAN_POINT ( 'NONE',  ( 16.55341960407618274, -4.379528057220086978, 66.04275706135236135 ) ) ;
#127553=CARTESIAN_POINT ( 'NONE',  ( 5.719274019375991003, -21.55341960407610458, 102.7072429386476955 ) ) ;
#127554=CARTESIAN_POINT ( 'NONE',  ( 14.34966873604972726, -8.224510206698740333, 45.83442372801901854 ) ) ;
#127555=CARTESIAN_POINT ( 'NONE',  ( 9.474510206698971260, -16.51473224551069308, 47.91557627198102409 ) ) ;
#127557=CARTESIAN_POINT ( 'NONE',  ( 5.719274019375673035, 21.55341960407619339, 57.29275706135234714 ) ) ;
#127558=CARTESIAN_POINT ( 'NONE',  ( 13.89961937509957401, 13.97604488694547697, 61.87609039468566863 ) ) ;
#127559=CARTESIAN_POINT ( 'NONE',  ( 21.52544592524334988, 5.823673210054432836, 96.45942372801901854 ) ) ;
#127560=CARTESIAN_POINT ( 'NONE',  ( -5.049401038298153566, 19.05341960407611168, 30.20724293864768839 ) ) ;
#127562=CARTESIAN_POINT ( 'NONE',  ( -10.81492255796078084, -18.62759615963271287, 57.08224293864769550 ) ) ;
#127564=CARTESIAN_POINT ( 'NONE',  ( 9.564922557960805705, 16.46253265017160317, 109.5822429386476955 ) ) ;
#127565=CARTESIAN_POINT ( 'NONE',  ( -12.06949235617756955, 12.14591786802309770, 105.6239096053143669 ) ) ;
#127566=CARTESIAN_POINT ( 'NONE',  ( 12.06949235617739724, 12.14591786802326823, 41.87609039468568284 ) ) ;
#127567=CARTESIAN_POINT ( 'NONE',  ( -0.05219959533934338120, 16.53943276465976808, 107.5010903946856899 ) ) ;
#127569=CARTESIAN_POINT ( 'NONE',  ( -18.62759615963270932, 10.81492255796079327, 105.8322429386476955 ) ) ;
#127570=CARTESIAN_POINT ( 'NONE',  ( -14.34966873604960291, -8.224510206698953496, 41.66557627198103120 ) ) ;
#127571=CARTESIAN_POINT ( 'NONE',  ( 0.05219959533909260263, 19.03943276465977164, 109.9989096053143669 ) ) ;
#127572=CARTESIAN_POINT ( 'NONE',  ( -16.51473224551082808, 9.474510206698731452, 88.33442372801900433 ) ) ;
#127573=CARTESIAN_POINT ( 'NONE',  ( -13.97604488694547697, 13.89961937509957934, 28.12609039468565797 ) ) ;
#127574=CARTESIAN_POINT ( 'NONE',  ( 12.14591786802309770, 12.06949235617756955, 34.37390960531435979 ) ) ;
#127575=CARTESIAN_POINT ( 'NONE',  ( 15.80617190586746368, 15.72974639402197994, 94.37390960531436690 ) ) ;
#127576=CARTESIAN_POINT ( 'NONE',  ( 21.53943276465977519, -0.05219959533907433946, 48.74890960531435979 ) ) ;
#127577=CARTESIAN_POINT ( 'NONE',  ( 13.97604488694527802, 13.89961937509977652, 69.37390960531436690 ) ) ;
#127578=CARTESIAN_POINT ( 'NONE',  ( -8.314922557960811034, -14.29746914071050412, 37.08224293864768129 ) ) ;
#127579=CARTESIAN_POINT ( 'NONE',  ( -19.05341960407611168, -5.049401038298163336, 86.45724293864769550 ) ) ;
#127580=ORIENTED_EDGE ( 'NONE', *, *, #115128, .F. ) ;
#127581=CARTESIAN_POINT ( 'NONE',  ( 19.52837319214023992, -5.500000000000092371, 62.10471352585538796 ) ) ;
#127582=CARTESIAN_POINT ( 'NONE',  ( 5.153800228976615827, -19.02544592524334988, 45.20942372801901143 ) ) ;
#127583=CARTESIAN_POINT ( 'NONE',  ( 15.80617190586746368, 15.72974639402197994, 84.37390960531438111 ) ) ;
#127584=CARTESIAN_POINT ( 'NONE',  ( -8.314922557960811034, -14.29746914071050412, 97.08224293864770971 ) ) ;
#127585=CARTESIAN_POINT ( 'NONE',  ( -10.81492255796105439, 18.62759615963255655, 42.91775706135235424 ) ) ;
#127587=EDGE_CURVE ( 'NONE', #186347, #101009, #33924, .T. ) ;
#127588=CARTESIAN_POINT ( 'NONE',  ( -16.53943276465976808, -0.05219959533934237506, 108.7510903946857042 ) ) ;
#127589=CARTESIAN_POINT ( 'NONE',  ( 16.51473224551069308, 9.474510206698969483, 34.16557627198102409 ) ) ;
#127590=CARTESIAN_POINT ( 'NONE',  ( 13.97604488694527802, 13.89961937509977652, 84.37390960531433848 ) ) ;
#127592=CARTESIAN_POINT ( 'NONE',  ( -9.564922557960796823, -16.46253265017161027, 27.08224293864769550 ) ) ;
#127593=CARTESIAN_POINT ( 'NONE',  ( -8.314922557960811034, -14.29746914071050412, 47.08224293864770260 ) ) ;
#127594=CARTESIAN_POINT ( 'NONE',  ( 21.52544592524334988, 5.823673210054432836, 71.45942372801901854 ) ) ;
#127596=CARTESIAN_POINT ( 'NONE',  ( 14.34966873604972726, -8.224510206698740333, 70.83442372801901854 ) ) ;
#127597=CARTESIAN_POINT ( 'NONE',  ( 16.46253265017160672, -9.564922557960803928, 53.33224293864768839 ) ) ;
#127598=CARTESIAN_POINT ( 'NONE',  ( -16.51473224551069308, -9.474510206698971260, 61.66557627198103120 ) ) ;
#127600=CARTESIAN_POINT ( 'NONE',  ( -19.02544592524334988, -5.153800228976617603, 18.95942372801899722 ) ) ;
#127601=CARTESIAN_POINT ( 'NONE',  ( -14.34966873604972548, 8.224510206698743886, 78.33442372801901854 ) ) ;
#127602=CARTESIAN_POINT ( 'NONE',  ( 21.55341960407619695, -5.719274019375665929, 96.04275706135236135 ) ) ;
#127603=CARTESIAN_POINT ( 'NONE',  ( -10.72451020669898014, 18.67979575497178502, 30.41557627198101699 ) ) ;
#127604=CARTESIAN_POINT ( 'NONE',  ( -19.05341960407617563, 5.049401038297882671, 103.5427570613523329 ) ) ;
#127605=CARTESIAN_POINT ( 'NONE',  ( -21.52544592524334988, -5.823673210054445271, 63.95942372801901854 ) ) ;
#127606=CARTESIAN_POINT ( 'NONE',  ( -16.53943276465976808, -0.05219959533934237506, 48.75109039468568284 ) ) ;
#127607=CARTESIAN_POINT ( 'NONE',  ( 18.67979575497178502, 10.72451020669898547, 104.1655762719810241 ) ) ;
#127608=CARTESIAN_POINT ( 'NONE',  ( 13.97604488694548053, -13.89961937509957401, 105.6260903946856757 ) ) ;
#127609=CARTESIAN_POINT ( 'NONE',  ( 9.564922557960805705, 16.46253265017160317, 74.58224293864769550 ) ) ;
#127610=CARTESIAN_POINT ( 'NONE',  ( -16.51473224551082808, 9.474510206698731452, 113.3344237280190043 ) ) ;
#127611=CARTESIAN_POINT ( 'NONE',  ( -0.05219959533936034679, 19.03943276465977164, 107.5010903946856615 ) ) ;
#127612=CARTESIAN_POINT ( 'NONE',  ( 4.379528057220339221, -16.55341960407611168, 67.70724293864769550 ) ) ;
#127613=CARTESIAN_POINT ( 'NONE',  ( 12.06949235617739724, 12.14591786802326823, 76.87609039468567573 ) ) ;
#127614=CARTESIAN_POINT ( 'NONE',  ( -18.62759615963255300, -10.81492255796106328, 19.16775706135234714 ) ) ;
#127615=CARTESIAN_POINT ( 'NONE',  ( -13.89961937509977652, 13.97604488694528158, 50.62390960531435979 ) ) ;
#127616=CARTESIAN_POINT ( 'NONE',  ( -13.97604488694527625, -13.89961937509977652, 56.87390960531434558 ) ) ;
#127618=CARTESIAN_POINT ( 'NONE',  ( -16.55341960407617563, 4.379528057220093196, 73.54275706135234714 ) ) ;
#127620=CARTESIAN_POINT ( 'NONE',  ( -21.53943276465977519, -0.05219959533937600094, 108.7510903946857042 ) ) ;
#127622=VERTEX_POINT ( 'NONE', #10578 ) ;
#127623=CARTESIAN_POINT ( 'NONE',  ( 0.05219959533936267826, -19.03943276465977164, 110.0010903946856757 ) ) ;
#127624=CARTESIAN_POINT ( 'NONE',  ( -5.719274019375978568, 21.55341960407610458, 55.20724293864770260 ) ) ;
#127625=CARTESIAN_POINT ( 'NONE',  ( -16.51473224551082808, 9.474510206698731452, 38.33442372801899722 ) ) ;
#127626=CARTESIAN_POINT ( 'NONE',  ( -12.14591786802326823, 12.06949235617739902, 33.12609039468569705 ) ) ;
#127627=CARTESIAN_POINT ( 'NONE',  ( -9.474510206698964154, 16.51473224551069663, 45.41557627198103120 ) ) ;
#127628=CARTESIAN_POINT ( 'NONE',  ( 9.564922557960805705, 16.46253265017160317, 69.58224293864770971 ) ) ;
#127629=CARTESIAN_POINT ( 'NONE',  ( 18.67979575497178502, 10.72451020669898547, 84.16557627198103830 ) ) ;
#127630=CARTESIAN_POINT ( 'NONE',  ( -19.03943276465977164, 0.05219959533909376836, 111.2489096053143669 ) ) ;
#127631=CARTESIAN_POINT ( 'NONE',  ( 16.46253265017160672, -9.564922557960803928, 53.33224293864768839 ) ) ;
#127633=CARTESIAN_POINT ( 'NONE',  ( 13.97604488694548053, -13.89961937509957401, 95.62609039468563310 ) ) ;
#127634=CARTESIAN_POINT ( 'NONE',  ( 12.14591786802309770, 12.06949235617756955, 69.37390960531436690 ) ) ;
#127635=CARTESIAN_POINT ( 'NONE',  ( -16.46253265017146816, -9.564922557961047289, 29.16775706135232937 ) ) ;
#127636=CARTESIAN_POINT ( 'NONE',  ( 12.06949235617757843, -12.14591786802309237, 63.12390960531435979 ) ) ;
#127637=CARTESIAN_POINT ( 'NONE',  ( 21.53943276465977519, 0.05219959533937863772, 81.25109039468568994 ) ) ;
#127638=CARTESIAN_POINT ( 'NONE',  ( -5.153800228976328057, -19.02544592524343514, 32.29057627198102409 ) ) ;
#127639=CARTESIAN_POINT ( 'NONE',  ( -5.823673210054431948, 21.52544592524334988, 92.70942372801901854 ) ) ;
#127640=CARTESIAN_POINT ( 'NONE',  ( 8.224510206698953496, -14.34966873604960469, 22.91557627198102765 ) ) ;
#127641=CARTESIAN_POINT ( 'NONE',  ( -18.67979575497193778, 10.72451020669871902, 83.33442372801903275 ) ) ;
#127642=CARTESIAN_POINT ( 'NONE',  ( -16.51473224551069308, -9.474510206698971260, 71.66557627198102409 ) ) ;
#127643=CARTESIAN_POINT ( 'NONE',  ( 18.62759615963255655, 10.81492255796105972, 46.66775706135234714 ) ) ;
#127644=CARTESIAN_POINT ( 'NONE',  ( 5.049401038298161559, -19.05341960407611168, 82.70724293864770971 ) ) ;
#127645=CARTESIAN_POINT ( 'NONE',  ( 16.53943276465976808, -0.05219959533910856209, 93.74890960531436690 ) ) ;
#127646=CARTESIAN_POINT ( 'NONE',  ( 12.06949235617757843, -12.14591786802309237, 63.12390960531435979 ) ) ;
#127647=CARTESIAN_POINT ( 'NONE',  ( 5.719274019375991003, -21.55341960407610458, 72.70724293864769550 ) ) ;
#127648=CARTESIAN_POINT ( 'NONE',  ( -0.05219959533909027116, -19.03943276465977164, 72.49890960531435269 ) ) ;
#127649=CARTESIAN_POINT ( 'NONE',  ( 5.823673210054125526, 21.52544592524343514, 84.79057627198102409 ) ) ;
#127651=CARTESIAN_POINT ( 'NONE',  ( -9.564922557961040184, 16.46253265017147172, 62.91775706135233293 ) ) ;
#127652=CARTESIAN_POINT ( 'NONE',  ( -13.89961937509957401, -13.97604488694547697, 29.37609039468566152 ) ) ;
#127653=CARTESIAN_POINT ( 'NONE',  ( -12.14591786802309592, -12.06949235617757132, 81.87390960531435269 ) ) ;
#127654=CARTESIAN_POINT ( 'NONE',  ( 15.80617190586746368, 15.72974639402197994, 54.37390960531435979 ) ) ;
#127656=CARTESIAN_POINT ( 'NONE',  ( -0.05219959533934338120, 16.53943276465976808, 92.50109039468567573 ) ) ;
#127658=CARTESIAN_POINT ( 'NONE',  ( 13.89961937509957401, 13.97604488694547697, 106.8760903946856757 ) ) ;
#127659=CARTESIAN_POINT ( 'NONE',  ( -14.34966873604960291, -8.224510206698953496, 61.66557627198103120 ) ) ;
#127661=CARTESIAN_POINT ( 'NONE',  ( 0.05219959533909260263, 19.03943276465977164, 64.99890960531436690 ) ) ;
#127662=CARTESIAN_POINT ( 'NONE',  ( 4.483927247898545687, 16.52544592524342804, 49.79057627198102409 ) ) ;
#127663=CARTESIAN_POINT ( 'NONE',  ( -16.46253265017160317, 9.564922557960807481, 100.8322429386477097 ) ) ;
#127664=CARTESIAN_POINT ( 'NONE',  ( 19.05341960407617918, -5.049401038297876454, 76.04275706135230450 ) ) ;
#127665=CARTESIAN_POINT ( 'NONE',  ( 19.05341960407611168, 5.049401038298154454, 68.95724293864769550 ) ) ;
#127666=CARTESIAN_POINT ( 'NONE',  ( -19.05341960407611168, -5.049401038298163336, 91.45724293864766707 ) ) ;
#127667=CARTESIAN_POINT ( 'NONE',  ( -13.89961937509977652, 13.97604488694528158, 80.62390960531436690 ) ) ;
#127668=CARTESIAN_POINT ( 'NONE',  ( -10.81492255796078084, -18.62759615963271287, 57.08224293864769550 ) ) ;
#127669=CARTESIAN_POINT ( 'NONE',  ( -8.224510206698735004, -14.34966873604973081, 59.58442372801901854 ) ) ;
#127670=AXIS2_PLACEMENT_3D ( 'NONE', #57482, #42311, #103972 ) ;
#127671=CARTESIAN_POINT ( 'NONE',  ( -19.02544592524342804, 5.153800228976336051, 46.04057627198101699 ) ) ;
#127672=CARTESIAN_POINT ( 'NONE',  ( -21.55341960407610458, -5.719274019375992779, 51.45724293864770260 ) ) ;
#127673=CARTESIAN_POINT ( 'NONE',  ( 19.03943276465977164, 0.05219959533936151252, 101.2510903946856757 ) ) ;
#127674=CARTESIAN_POINT ( 'NONE',  ( -0.05219959533910754901, -16.53943276465976808, 27.49890960531435269 ) ) ;
#127675=CARTESIAN_POINT ( 'NONE',  ( 15.80617190586769283, -15.72974639402175789, 45.62609039468567573 ) ) ;
#127676=CARTESIAN_POINT ( 'NONE',  ( 13.97604488694548053, -13.89961937509957401, 40.62609039468564731 ) ) ;
#127677=CARTESIAN_POINT ( 'NONE',  ( -8.314922557961024197, 14.29746914071037800, 57.91775706135234714 ) ) ;
#127678=CARTESIAN_POINT ( 'NONE',  ( 8.224510206698742110, 14.34966873604972548, 92.08442372801901854 ) ) ;
#127679=CARTESIAN_POINT ( 'NONE',  ( 18.39635199886966532, -5.500000000000096811, 43.51967076359999709 ) ) ;
#127680=CARTESIAN_POINT ( 'NONE',  ( 8.314922557961029526, -14.29746914071037800, 75.41775706135233293 ) ) ;
#127681=CARTESIAN_POINT ( 'NONE',  ( 14.34966873604972726, -8.224510206698740333, 35.83442372801901143 ) ) ;
#127682=CARTESIAN_POINT ( 'NONE',  ( -5.153800228976328057, -19.02544592524343514, 52.29057627198100988 ) ) ;
#127683=CARTESIAN_POINT ( 'NONE',  ( 5.153800228976335163, 19.02544592524342804, 49.79057627198100988 ) ) ;
#127684=CARTESIAN_POINT ( 'NONE',  ( -13.97604488694527625, -13.89961937509977652, 66.87390960531436690 ) ) ;
#127685=CARTESIAN_POINT ( 'NONE',  ( -5.823673210054431948, 21.52544592524334988, 57.70942372801901143 ) ) ;
#127686=CARTESIAN_POINT ( 'NONE',  ( -12.14591786802326823, 12.06949235617739902, 43.12609039468568284 ) ) ;
#127687=CARTESIAN_POINT ( 'NONE',  ( -4.379528057220086978, -16.55341960407618274, 109.7927570613523613 ) ) ;
#127688=CARTESIAN_POINT ( 'NONE',  ( -5.153800228976328057, -19.02544592524343514, 22.29057627198102765 ) ) ;
#127689=CARTESIAN_POINT ( 'NONE',  ( -18.62759615963255300, -10.81492255796106328, 109.1677570613523613 ) ) ;
#127690=CARTESIAN_POINT ( 'NONE',  ( 16.51473224551083163, -9.474510206698727899, 110.8344237280190043 ) ) ;
#127691=CARTESIAN_POINT ( 'NONE',  ( -5.153800228976607833, 19.02544592524334988, 72.70942372801900433 ) ) ;
#127692=CARTESIAN_POINT ( 'NONE',  ( 8.314922557960818139, 14.29746914071049879, 79.58224293864769550 ) ) ;
#127693=CARTESIAN_POINT ( 'NONE',  ( 5.153800228976335163, 19.02544592524342804, 34.79057627198102409 ) ) ;
#127694=CARTESIAN_POINT ( 'NONE',  ( 13.97604488694548053, -13.89961937509957401, 75.62609039468564731 ) ) ;
#127695=LINE ( 'NONE', #188398, #140529 ) ;
#127696=CARTESIAN_POINT ( 'NONE',  ( 18.67979575497194134, -10.72451020669871369, 80.83442372801901854 ) ) ;
#127697=CARTESIAN_POINT ( 'NONE',  ( -14.29746914071037622, -8.314922557961029526, 39.16775706135235424 ) ) ;
#127699=CARTESIAN_POINT ( 'NONE',  ( -15.72974639402197994, 15.80617190586746368, 30.62390960531436335 ) ) ;
#127700=CARTESIAN_POINT ( 'NONE',  ( -16.55341960407617563, 4.379528057220093196, 23.54275706135235424 ) ) ;
#127701=CARTESIAN_POINT ( 'NONE',  ( 9.474510206698971260, -16.51473224551069308, 22.91557627198102765 ) ) ;
#127702=CARTESIAN_POINT ( 'NONE',  ( -9.474510206698720793, -16.51473224551083518, 34.58442372801899722 ) ) ;
#127704=CARTESIAN_POINT ( 'NONE',  ( 16.51473224551069308, 9.474510206698969483, 44.16557627198103120 ) ) ;
#127706=CARTESIAN_POINT ( 'NONE',  ( -0.05219959533909027116, -19.03943276465977164, 72.49890960531435269 ) ) ;
#127707=CARTESIAN_POINT ( 'NONE',  ( -19.25663599770060586, 5.499999999999443112, 98.99419308057201761 ) ) ;
#127708=CARTESIAN_POINT ( 'NONE',  ( -16.46253265017146816, -9.564922557961047289, 24.16775706135233648 ) ) ;
#127709=CARTESIAN_POINT ( 'NONE',  ( 12.06949235617739724, 12.14591786802326823, 111.8760903946856615 ) ) ;
#127710=CARTESIAN_POINT ( 'NONE',  ( 9.564922557960805705, 16.46253265017160317, 49.58224293864770260 ) ) ;
#127711=CARTESIAN_POINT ( 'NONE',  ( -9.564922557960796823, -16.46253265017161027, 92.08224293864769550 ) ) ;
#127712=CARTESIAN_POINT ( 'NONE',  ( 5.823673210054444382, -21.52544592524334988, 70.20942372801904696 ) ) ;
#127713=CARTESIAN_POINT ( 'NONE',  ( 19.03943276465977164, -0.05219959533909143690, 53.74890960531436690 ) ) ;
#127714=CARTESIAN_POINT ( 'NONE',  ( -0.05219959533937732626, 21.53943276465977519, 62.50109039468568284 ) ) ;
#127715=CARTESIAN_POINT ( 'NONE',  ( -16.46253265017146816, -9.564922557961047289, 99.16775706135233293 ) ) ;
#127716=CARTESIAN_POINT ( 'NONE',  ( 19.03943276465977164, -0.05219959533909143690, 113.7489096053143669 ) ) ;
#127717=CARTESIAN_POINT ( 'NONE',  ( 16.51473224551069308, 9.474510206698969483, 29.16557627198103475 ) ) ;
#127718=CARTESIAN_POINT ( 'NONE',  ( -15.72974639402197994, 15.80617190586746368, 110.6239096053143669 ) ) ;
#127719=CARTESIAN_POINT ( 'NONE',  ( 5.049401038297881783, 19.05341960407617563, 37.29275706135232582 ) ) ;
#127720=CARTESIAN_POINT ( 'NONE',  ( -16.52544592524342804, 4.483927247898546575, 106.0405762719810525 ) ) ;
#127721=CARTESIAN_POINT ( 'NONE',  ( 13.89961937509977652, -13.97604488694527269, 68.12390960531436690 ) ) ;
#127722=CARTESIAN_POINT ( 'NONE',  ( 5.049401038297881783, 19.05341960407617563, 112.2927570613523471 ) ) ;
#127723=CARTESIAN_POINT ( 'NONE',  ( -4.379528057220328563, 16.55341960407611168, 80.20724293864769550 ) ) ;
#127724=CARTESIAN_POINT ( 'NONE',  ( 21.52544592524344225, -5.823673210054117533, 28.54057627198103120 ) ) ;
#127725=CARTESIAN_POINT ( 'NONE',  ( 13.97604488694548053, -13.89961937509957401, 85.62609039468568994 ) ) ;
#127726=CARTESIAN_POINT ( 'NONE',  ( 5.823673210054125526, 21.52544592524343514, 89.79057627198103830 ) ) ;
#127727=CARTESIAN_POINT ( 'NONE',  ( -0.05219959533937732626, 21.53943276465977519, 62.50109039468568284 ) ) ;
#127728=CARTESIAN_POINT ( 'NONE',  ( -14.34966873604972548, 8.224510206698743886, 58.33442372801901143 ) ) ;
#127729=CARTESIAN_POINT ( 'NONE',  ( -14.34966873604972548, 8.224510206698743886, 58.33442372801901143 ) ) ;
#127730=CARTESIAN_POINT ( 'NONE',  ( -15.72974639402197994, 15.80617190586746368, 60.62390960531437401 ) ) ;
#127731=CARTESIAN_POINT ( 'NONE',  ( -9.564922557960796823, -16.46253265017161027, 47.08224293864769550 ) ) ;
#127733=CARTESIAN_POINT ( 'NONE',  ( 16.52544592524335698, 4.483927247898782831, 81.45942372801900433 ) ) ;
#127734=CARTESIAN_POINT ( 'NONE',  ( -10.81492255796078084, -18.62759615963271287, 107.0822429386476955 ) ) ;
#127735=CARTESIAN_POINT ( 'NONE',  ( 8.314922557960818139, 14.29746914071049879, 49.58224293864769550 ) ) ;
#127736=CARTESIAN_POINT ( 'NONE',  ( -12.06949235617739369, -12.14591786802326823, 59.37609039468568284 ) ) ;
#127737=CARTESIAN_POINT ( 'NONE',  ( 19.03943276465977164, 0.05219959533936151252, 101.2510903946856757 ) ) ;
#127738=CARTESIAN_POINT ( 'NONE',  ( 18.62759615963271287, -10.81492255796078972, 93.33224293864769550 ) ) ;
#127739=CARTESIAN_POINT ( 'NONE',  ( -8.224510206698948167, 14.34966873604960824, 40.41557627198103120 ) ) ;
#127740=ORIENTED_EDGE ( 'NONE', *, *, #47203, .F. ) ;
#127741=CARTESIAN_POINT ( 'NONE',  ( -16.79531203550648044, 7.028104445595610095, 68.74755011779559766 ) ) ;
#127742=CARTESIAN_POINT ( 'NONE',  ( -21.52544592524343514, 5.823673210054127303, 81.04057627198102409 ) ) ;
#127743=CARTESIAN_POINT ( 'NONE',  ( -12.14591786802326823, 12.06949235617739902, 113.1260903946856899 ) ) ;
#127745=CARTESIAN_POINT ( 'NONE',  ( -16.19135201231369692, -7.376712067591813415, 55.18680854052030327 ) ) ;
#127746=CARTESIAN_POINT ( 'NONE',  ( -21.52544592524343514, 5.823673210054127303, 96.04057627198102409 ) ) ;
#127747=VECTOR ( 'NONE', #89432, 1000.000000000000000 ) ;
#127748=CARTESIAN_POINT ( 'NONE',  ( 10.72451020669871369, 18.67979575497193778, 22.08442372801901143 ) ) ;
#127749=CARTESIAN_POINT ( 'NONE',  ( 8.224510206698953496, -14.34966873604960469, 32.91557627198102409 ) ) ;
#127750=CARTESIAN_POINT ( 'NONE',  ( 4.483927247898790824, -16.52544592524335698, 50.20942372801901854 ) ) ;
#127751=CARTESIAN_POINT ( 'NONE',  ( 9.474510206698971260, -16.51473224551069308, 42.91557627198103120 ) ) ;
#127752=CARTESIAN_POINT ( 'NONE',  ( 13.89961937509977652, -13.97604488694527269, 83.12390960531436690 ) ) ;
#127754=CARTESIAN_POINT ( 'NONE',  ( -18.62759615963270932, 10.81492255796079327, 40.83224293864769550 ) ) ;
#127756=CARTESIAN_POINT ( 'NONE',  ( -8.224510206698735004, -14.34966873604973081, 24.58442372801901499 ) ) ;
#127757=CARTESIAN_POINT ( 'NONE',  ( 16.51473224551083163, -9.474510206698727899, 55.83442372801899722 ) ) ;
#127758=CARTESIAN_POINT ( 'NONE',  ( -15.80617190586745835, -15.72974639402198527, 96.87390960531436690 ) ) ;
#127760=CARTESIAN_POINT ( 'NONE',  ( 8.224510206698953496, -14.34966873604960469, 37.91557627198102409 ) ) ;
#127761=CARTESIAN_POINT ( 'NONE',  ( 19.02544592524343514, -5.153800228976328945, 83.54057627198100988 ) ) ;
#127762=CARTESIAN_POINT ( 'NONE',  ( -10.81492255796078084, -18.62759615963271287, 57.08224293864769550 ) ) ;
#127763=CARTESIAN_POINT ( 'NONE',  ( -21.52544592524343514, 5.823673210054127303, 96.04057627198102409 ) ) ;
#127764=CARTESIAN_POINT ( 'NONE',  ( -8.314922557961024197, 14.29746914071037800, 22.91775706135235069 ) ) ;
#127765=CARTESIAN_POINT ( 'NONE',  ( -0.05219959533909027116, -19.03943276465977164, 112.4989096053143669 ) ) ;
#127766=CARTESIAN_POINT ( 'NONE',  ( -10.72451020669870658, -18.67979575497194134, 89.58442372801901854 ) ) ;
#127767=CARTESIAN_POINT ( 'NONE',  ( 0.05219959533909260263, 19.03943276465977164, 74.99890960531435269 ) ) ;
#127768=CARTESIAN_POINT ( 'NONE',  ( 13.89961937509977652, -13.97604488694527269, 28.12390960531435624 ) ) ;
#127769=CARTESIAN_POINT ( 'NONE',  ( 9.474510206698971260, -16.51473224551069308, 87.91557627198102409 ) ) ;
#127770=CARTESIAN_POINT ( 'NONE',  ( 16.55341960407611168, 4.379528057220329451, 98.95724293864770971 ) ) ;
#127772=CARTESIAN_POINT ( 'NONE',  ( -13.89961937509957401, -13.97604488694547875, 104.3760903946856757 ) ) ;
#127774=CARTESIAN_POINT ( 'NONE',  ( 19.05341960407611168, 5.049401038298154454, 73.95724293864768129 ) ) ;
#127775=CARTESIAN_POINT ( 'NONE',  ( 21.53943276465977519, 0.05219959533937863772, 96.25109039468568994 ) ) ;
#127776=CARTESIAN_POINT ( 'NONE',  ( -5.049401038298153566, 19.05341960407611168, 110.2072429386476671 ) ) ;
#127777=CARTESIAN_POINT ( 'NONE',  ( 14.34966873604972726, -8.224510206698740333, 80.83442372801901854 ) ) ;
#127779=CARTESIAN_POINT ( 'NONE',  ( -19.03943276465977164, -0.05219959533935918106, 58.75109039468566863 ) ) ;
#127780=CARTESIAN_POINT ( 'NONE',  ( 10.72451020669871369, 18.67979575497193778, 107.0844237280190043 ) ) ;
#127782=CARTESIAN_POINT ( 'NONE',  ( -19.02544592524342804, 5.153800228976336051, 31.04057627198102409 ) ) ;
#127783=CARTESIAN_POINT ( 'NONE',  ( 14.34966873604960469, 8.224510206698951720, 24.16557627198103120 ) ) ;
#127784=DIRECTION ( 'NONE',  ( 0.000000000000000000, 0.000000000000000000, -1.000000000000000000 ) ) ;
#127785=CARTESIAN_POINT ( 'NONE',  ( -14.29746914071037622, -8.314922557961029526, 104.1677570613523471 ) ) ;
#127786=CARTESIAN_POINT ( 'NONE',  ( -19.25176906914649777, -5.499999999999857003, 85.99927264242278113 ) ) ;
#127787=CARTESIAN_POINT ( 'NONE',  ( -0.05219959533934338120, 16.53943276465976808, 77.50109039468567573 ) ) ;
#127788=CARTESIAN_POINT ( 'NONE',  ( -0.05219959533909027116, -19.03943276465977164, 22.49890960531436690 ) ) ;
#127789=CARTESIAN_POINT ( 'NONE',  ( -18.62759615963255300, -10.81492255796106328, 89.16775706135236135 ) ) ;
#127790=CARTESIAN_POINT ( 'NONE',  ( -5.153800228976607833, 19.02544592524334988, 102.7094237280189759 ) ) ;
#127791=CARTESIAN_POINT ( 'NONE',  ( -15.80617190586768217, 15.72974639402176855, 63.12609039468568994 ) ) ;
#127792=CARTESIAN_POINT ( 'NONE',  ( -19.02544592524334988, -5.153800228976617603, 33.95942372801897591 ) ) ;
#127793=CARTESIAN_POINT ( 'NONE',  ( 5.049401038298161559, -19.05341960407611168, 82.70724293864770971 ) ) ;
#127794=CARTESIAN_POINT ( 'NONE',  ( 13.97604488694527802, 13.89961937509977652, 64.37390960531436690 ) ) ;
#127796=CARTESIAN_POINT ( 'NONE',  ( -18.67979575497178146, -10.72451020669898902, 41.66557627198103120 ) ) ;
#127797=CARTESIAN_POINT ( 'NONE',  ( -19.03943276465977164, 0.05219959533909376836, 51.24890960531436690 ) ) ;
#127798=CARTESIAN_POINT ( 'NONE',  ( -12.06949235617739369, -12.14591786802326823, 74.37609039468568994 ) ) ;
#127800=CARTESIAN_POINT ( 'NONE',  ( 4.379528057220339221, -16.55341960407611168, 72.70724293864769550 ) ) ;
#127802=CARTESIAN_POINT ( 'NONE',  ( 16.55341960407618274, -4.379528057220086978, 41.04275706135236135 ) ) ;
#127803=CARTESIAN_POINT ( 'NONE',  ( 4.483927247898545687, 16.52544592524342804, 114.7905762719810383 ) ) ;
#127804=CARTESIAN_POINT ( 'NONE',  ( -5.153800228976607833, 19.02544592524334988, 72.70942372801900433 ) ) ;
#127805=CARTESIAN_POINT ( 'NONE',  ( 12.14591786802309770, 12.06949235617756955, 69.37390960531436690 ) ) ;
#127806=CARTESIAN_POINT ( 'NONE',  ( -18.62759615963255300, -10.81492255796106328, 29.16775706135234003 ) ) ;
#127808=CARTESIAN_POINT ( 'NONE',  ( -5.823673210054116645, -21.52544592524344225, 97.29057627198105251 ) ) ;
#127809=CARTESIAN_POINT ( 'NONE',  ( -9.564922557960796823, -16.46253265017161027, 112.0822429386476955 ) ) ;
#127810=CARTESIAN_POINT ( 'NONE',  ( 0.05219959533910956823, 16.53943276465976808, 69.99890960531435269 ) ) ;
#127812=CARTESIAN_POINT ( 'NONE',  ( -13.97604488694527625, -13.89961937509977652, 51.87390960531436690 ) ) ;
#127814=CARTESIAN_POINT ( 'NONE',  ( 5.153800228976615827, -19.02544592524334988, 75.20942372801896170 ) ) ;
#127815=CARTESIAN_POINT ( 'NONE',  ( 21.55341960407619695, -5.719274019375665929, 21.04275706135234714 ) ) ;
#127816=CARTESIAN_POINT ( 'NONE',  ( -19.02544592524342804, 5.153800228976336051, 76.04057627198102409 ) ) ;
#127817=CARTESIAN_POINT ( 'NONE',  ( 19.05341960407617918, -5.049401038297876454, 61.04275706135232582 ) ) ;
#127818=CARTESIAN_POINT ( 'NONE',  ( 0.05219959533909260263, 19.03943276465977164, 49.99890960531435979 ) ) ;
#127819=CARTESIAN_POINT ( 'NONE',  ( -8.224510206698948167, 14.34966873604960824, 65.41557627198102409 ) ) ;
#127820=CARTESIAN_POINT ( 'NONE',  ( 14.29746914071049879, -8.314922557960816363, 48.33224293864770260 ) ) ;
#127821=CARTESIAN_POINT ( 'NONE',  ( -16.51473224551069308, -9.474510206698971260, 76.66557627198103830 ) ) ;
#127822=CARTESIAN_POINT ( 'NONE',  ( 21.52544592524344225, -5.823673210054117533, 83.54057627198102409 ) ) ;
#127823=CARTESIAN_POINT ( 'NONE',  ( -0.05219959533909027116, -19.03943276465977164, 77.49890960531435269 ) ) ;
#127824=CARTESIAN_POINT ( 'NONE',  ( 10.81492255796078972, 18.62759615963270932, 74.58224293864768129 ) ) ;
#127825=CARTESIAN_POINT ( 'NONE',  ( -19.02544592524334988, -5.153800228976617603, 23.95942372801900078 ) ) ;
#127826=CARTESIAN_POINT ( 'NONE',  ( 5.049401038298161559, -19.05341960407611168, 27.70724293864769550 ) ) ;
#127827=CARTESIAN_POINT ( 'NONE',  ( 4.483927247898790824, -16.52544592524335698, 110.2094237280190185 ) ) ;
#127828=CARTESIAN_POINT ( 'NONE',  ( 14.29746914071049879, -8.314922557960816363, 98.33224293864769550 ) ) ;
#127829=CARTESIAN_POINT ( 'NONE',  ( 16.51473224551083163, -9.474510206698727899, 110.8344237280190043 ) ) ;
#127831=CARTESIAN_POINT ( 'NONE',  ( -15.72974639402197994, 15.80617190586746368, 110.6239096053143669 ) ) ;
#127832=CARTESIAN_POINT ( 'NONE',  ( -13.89961937509957401, -13.97604488694547875, 54.37609039468565442 ) ) ;
#127833=CARTESIAN_POINT ( 'NONE',  ( -4.483927247898782831, 16.52544592524335698, 112.7094237280190328 ) ) ;
#127834=CARTESIAN_POINT ( 'NONE',  ( -0.05219959533907301413, -21.53943276465977519, 72.49890960531435269 ) ) ;
#127835=CARTESIAN_POINT ( 'NONE',  ( -16.46253265017160317, 9.564922557960807481, 105.8322429386476955 ) ) ;
#127836=CARTESIAN_POINT ( 'NONE',  ( 12.06949235617757843, -12.14591786802309237, 63.12390960531435979 ) ) ;
#127837=CARTESIAN_POINT ( 'NONE',  ( -18.39443945427632343, 5.499999999999999112, 48.51745347608652992 ) ) ;
#127838=CARTESIAN_POINT ( 'NONE',  ( -19.02544592524342804, 5.153800228976336051, 36.04057627198100988 ) ) ;
#127839=CARTESIAN_POINT ( 'NONE',  ( -10.72451020669870658, -18.67979575497194134, 109.5844237280190328 ) ) ;
#127840=CARTESIAN_POINT ( 'NONE',  ( -16.53943276465976808, -0.05219959533934237506, 93.75109039468567573 ) ) ;
#127841=CARTESIAN_POINT ( 'NONE',  ( 21.55341960407619695, -5.719274019375665929, 46.04275706135234714 ) ) ;
#127842=CARTESIAN_POINT ( 'NONE',  ( 16.55341960407618274, -4.379528057220086978, 46.04275706135234714 ) ) ;
#127843=CARTESIAN_POINT ( 'NONE',  ( 5.719274019375991003, -21.55341960407610458, 27.70724293864769905 ) ) ;
#127844=CARTESIAN_POINT ( 'NONE',  ( 19.03943276465977164, -0.05219959533909143690, 48.74890960531435979 ) ) ;
#127845=CARTESIAN_POINT ( 'NONE',  ( 19.03943276465977164, -0.05219959533909143690, 63.74890960531435979 ) ) ;
#127847=CARTESIAN_POINT ( 'NONE',  ( 14.34966873604972726, -8.224510206698740333, 55.83442372801901854 ) ) ;
#127848=CARTESIAN_POINT ( 'NONE',  ( -14.34966873604960291, -8.224510206698953496, 106.6655762719810383 ) ) ;
#127849=CARTESIAN_POINT ( 'NONE',  ( 0.05219959533910956823, 16.53943276465976808, 24.99890960531435624 ) ) ;
#127851=CARTESIAN_POINT ( 'NONE',  ( -10.81492255796105439, 18.62759615963255655, 62.91775706135236135 ) ) ;
#127852=CARTESIAN_POINT ( 'NONE',  ( -5.153800228976328057, -19.02544592524343514, 97.29057627198099567 ) ) ;
#127853=CARTESIAN_POINT ( 'NONE',  ( -9.564922557960796823, -16.46253265017161027, 77.08224293864769550 ) ) ;
#127854=CARTESIAN_POINT ( 'NONE',  ( 5.049401038298161559, -19.05341960407611168, 97.70724293864766707 ) ) ;
#127855=EDGE_CURVE ( 'NONE', #189743, #20330, #32031, .T. ) ;
#127856=CARTESIAN_POINT ( 'NONE',  ( 16.55341960407611168, 4.379528057220329451, 43.95724293864769550 ) ) ;
#127857=CARTESIAN_POINT ( 'NONE',  ( -4.483927247898782831, 16.52544592524335698, 107.7094237280190328 ) ) ;
#127858=CARTESIAN_POINT ( 'NONE',  ( -8.224510206698948167, 14.34966873604960824, 40.41557627198103120 ) ) ;
#127859=LINE ( 'NONE', #189563, #190087 ) ;
#127860=CARTESIAN_POINT ( 'NONE',  ( 0.05219959533936267826, -19.03943276465977164, 40.00109039468566152 ) ) ;
#127861=CARTESIAN_POINT ( 'NONE',  ( 19.02544592524343514, -5.153800228976328945, 78.54057627198099567 ) ) ;
#127862=CARTESIAN_POINT ( 'NONE',  ( 9.564922557961047289, -16.46253265017146816, 55.41775706135234003 ) ) ;
#127865=CARTESIAN_POINT ( 'NONE',  ( -9.474510206698720793, -16.51473224551083518, 79.58442372801899012 ) ) ;
#127866=CARTESIAN_POINT ( 'NONE',  ( 14.34966873604972726, -8.224510206698740333, 70.83442372801901854 ) ) ;
#127868=CARTESIAN_POINT ( 'NONE',  ( 13.97604488694527802, 13.89961937509977652, 109.3739096053143669 ) ) ;
#127869=CARTESIAN_POINT ( 'NONE',  ( 15.72974639402176855, 15.80617190586768217, 26.87609039468567218 ) ) ;
#127870=CARTESIAN_POINT ( 'NONE',  ( 19.02544592524334988, 5.153800228976608722, 86.45942372801900433 ) ) ;
#127871=CARTESIAN_POINT ( 'NONE',  ( 17.26058549869092928, 6.457015423128507514, 88.87745837476070676 ) ) ;
#127872=CARTESIAN_POINT ( 'NONE',  ( 5.153800228976335163, 19.02544592524342804, 44.79057627198103830 ) ) ;
#127873=CARTESIAN_POINT ( 'NONE',  ( -19.02544592524342804, 5.153800228976336051, 86.04057627198103830 ) ) ;
#127874=CARTESIAN_POINT ( 'NONE',  ( 0.05219959533910956823, 16.53943276465976808, 49.99890960531437401 ) ) ;
#127875=CARTESIAN_POINT ( 'NONE',  ( 13.89961937509977652, -13.97604488694527269, 53.12390960531434558 ) ) ;
#127876=CARTESIAN_POINT ( 'NONE',  ( 19.03943276465977164, 0.05219959533936151252, 61.25109039468566863 ) ) ;
#127877=CARTESIAN_POINT ( 'NONE',  ( -19.02544592524334988, -5.153800228976617603, 33.95942372801897591 ) ) ;
#127878=CARTESIAN_POINT ( 'NONE',  ( 19.02544592524343514, -5.153800228976328945, 63.54057627198103830 ) ) ;
#127879=CARTESIAN_POINT ( 'NONE',  ( 10.81492255796078972, 18.62759615963270932, 59.58224293864770260 ) ) ;
#127880=CARTESIAN_POINT ( 'NONE',  ( -12.06949235617756955, 12.14591786802309770, 65.62390960531436690 ) ) ;
#127881=CARTESIAN_POINT ( 'NONE',  ( -19.02544592524334988, -5.153800228976617603, 23.95942372801900078 ) ) ;
#127884=CARTESIAN_POINT ( 'NONE',  ( -9.474510206698964154, 16.51473224551069663, 115.4155762719810241 ) ) ;
#127885=CARTESIAN_POINT ( 'NONE',  ( -13.97604488694527625, -13.89961937509977652, 56.87390960531434558 ) ) ;
#127886=CARTESIAN_POINT ( 'NONE',  ( 13.97604488694527802, 13.89961937509977652, 39.37390960531435269 ) ) ;
#127887=CARTESIAN_POINT ( 'NONE',  ( 12.14591786802309770, 12.06949235617756955, 99.37390960531436690 ) ) ;
#127888=CARTESIAN_POINT ( 'NONE',  ( 18.67979575497178502, 10.72451020669898547, 104.1655762719810241 ) ) ;
#127889=FACE_OUTER_BOUND ( 'NONE', #139183, .T. ) ;
#127890=CARTESIAN_POINT ( 'NONE',  ( 15.80617190586769283, -15.72974639402175789, 25.62609039468567929 ) ) ;
#127891=CARTESIAN_POINT ( 'NONE',  ( 0.05219959533909260263, 19.03943276465977164, 104.9989096053143669 ) ) ;
#127892=CARTESIAN_POINT ( 'NONE',  ( 9.564922557960805705, 16.46253265017160317, 24.58224293864769194 ) ) ;
#127893=CARTESIAN_POINT ( 'NONE',  ( -5.719274019375665041, -21.55341960407619695, 79.79275706135236135 ) ) ;
#127894=CARTESIAN_POINT ( 'NONE',  ( 10.72451020669898902, -18.67979575497178502, 97.91557627198103830 ) ) ;
#127895=CARTESIAN_POINT ( 'NONE',  ( -13.97604488694547697, 13.89961937509957934, 33.12609039468566863 ) ) ;
#127897=CARTESIAN_POINT ( 'NONE',  ( 17.58332526062529411, -7.635886036038503910, 53.42334959558467489 ) ) ;
#127899=CARTESIAN_POINT ( 'NONE',  ( 8.224510206698742110, 14.34966873604972548, 47.08442372801901854 ) ) ;
#127900=CARTESIAN_POINT ( 'NONE',  ( -4.483927247898539470, -16.52544592524342804, 102.2905762719810383 ) ) ;
#127902=CARTESIAN_POINT ( 'NONE',  ( 16.51473224551069308, 9.474510206698969483, 64.16557627198102409 ) ) ;
#127903=CARTESIAN_POINT ( 'NONE',  ( -4.379528057220328563, 16.55341960407611168, 95.20724293864769550 ) ) ;
#127904=CARTESIAN_POINT ( 'NONE',  ( -15.72974639402197994, 15.80617190586746368, 50.62390960531435979 ) ) ;
#127905=CARTESIAN_POINT ( 'NONE',  ( 14.34966873604960469, 8.224510206698951720, 64.16557627198102409 ) ) ;
#127906=CARTESIAN_POINT ( 'NONE',  ( 16.53943276465976808, 0.05219959533934440121, 36.25109039468567573 ) ) ;
#127907=CARTESIAN_POINT ( 'NONE',  ( -0.05219959533937732626, 21.53943276465977519, 82.50109039468568994 ) ) ;
#127908=CARTESIAN_POINT ( 'NONE',  ( 17.49999999999998934, -5.500000000000023981, 78.29690382534170112 ) ) ;
#127909=CARTESIAN_POINT ( 'NONE',  ( -12.06949235617739369, -12.14591786802326823, 99.37609039468568994 ) ) ;
#127910=CARTESIAN_POINT ( 'NONE',  ( -4.483927247898539470, -16.52544592524342804, 47.29057627198103120 ) ) ;
#127911=CARTESIAN_POINT ( 'NONE',  ( 19.05341960407611168, 5.049401038298154454, 38.95724293864767418 ) ) ;
#127912=CARTESIAN_POINT ( 'NONE',  ( -13.89961937509977652, 13.97604488694528158, 95.62390960531436690 ) ) ;
#127913=CARTESIAN_POINT ( 'NONE',  ( -18.62759615963270932, 10.81492255796079327, 110.8322429386476955 ) ) ;
#127914=CARTESIAN_POINT ( 'NONE',  ( -5.719274019375665041, -21.55341960407619695, 54.79275706135235424 ) ) ;
#127915=CARTESIAN_POINT ( 'NONE',  ( 8.224510206698742110, 14.34966873604972548, 37.08442372801901143 ) ) ;
#127916=CARTESIAN_POINT ( 'NONE',  ( 16.52544592524342804, -4.483927247898539470, 58.54057627198103120 ) ) ;
#127917=CARTESIAN_POINT ( 'NONE',  ( 10.72451020669871369, 18.67979575497193778, 82.08442372801901854 ) ) ;
#127918=CARTESIAN_POINT ( 'NONE',  ( 16.55341960407618274, -4.379528057220086978, 96.04275706135236135 ) ) ;
#127919=CARTESIAN_POINT ( 'NONE',  ( 16.79531203550650176, 7.028104445595485750, 28.75244988220443076 ) ) ;
#127920=FACE_OUTER_BOUND ( 'NONE', #180525, .T. ) ;
#127921=CARTESIAN_POINT ( 'NONE',  ( -12.06949235617756955, 12.14591786802309770, 30.62390960531436335 ) ) ;
#127922=CARTESIAN_POINT ( 'NONE',  ( -16.53943276465976808, -0.05219959533934237506, 78.75109039468568994 ) ) ;
#127923=CARTESIAN_POINT ( 'NONE',  ( -19.02544592524342804, 5.153800228976336051, 86.04057627198103830 ) ) ;
#127924=CARTESIAN_POINT ( 'NONE',  ( 16.51473224551069308, 9.474510206698969483, 99.16557627198102409 ) ) ;
#127925=CARTESIAN_POINT ( 'NONE',  ( -15.72974639402176322, -15.80617190586768395, 79.37609039468567573 ) ) ;
#127926=CARTESIAN_POINT ( 'NONE',  ( 8.314922557961029526, -14.29746914071037800, 95.41775706135234714 ) ) ;
#127927=CARTESIAN_POINT ( 'NONE',  ( 8.224510206698953496, -14.34966873604960469, 57.91557627198103120 ) ) ;
#127928=CARTESIAN_POINT ( 'NONE',  ( 16.51473224551069308, 9.474510206698969483, 74.16557627198103830 ) ) ;
#127930=CARTESIAN_POINT ( 'NONE',  ( 12.06949235617739724, 12.14591786802326823, 21.87609039468567573 ) ) ;
#127931=CARTESIAN_POINT ( 'NONE',  ( 13.97604488694527802, 13.89961937509977652, 29.37390960531435979 ) ) ;
#127932=CARTESIAN_POINT ( 'NONE',  ( 9.474510206698971260, -16.51473224551069308, 72.91557627198102409 ) ) ;
#127933=CARTESIAN_POINT ( 'NONE',  ( 5.049401038297881783, 19.05341960407617563, 112.2927570613523471 ) ) ;
#127935=CARTESIAN_POINT ( 'NONE',  ( -16.51473224551082808, 9.474510206698731452, 23.33442372801900078 ) ) ;
#127936=CARTESIAN_POINT ( 'NONE',  ( -16.53943276465976808, -0.05219959533934237506, 78.75109039468568994 ) ) ;
#127937=CARTESIAN_POINT ( 'NONE',  ( 9.564922557961047289, -16.46253265017146816, 110.4177570613523471 ) ) ;
#127938=CARTESIAN_POINT ( 'NONE',  ( 9.474510206698971260, -16.51473224551069308, 22.91557627198102765 ) ) ;
#127939=CARTESIAN_POINT ( 'NONE',  ( 0.05219959533934541429, -16.53943276465976808, 70.00109039468568994 ) ) ;
#127940=CARTESIAN_POINT ( 'NONE',  ( -14.34966873604972548, 8.224510206698743886, 53.33442372801901854 ) ) ;
#127941=CARTESIAN_POINT ( 'NONE',  ( 16.46253265017160672, -9.564922557960803928, 23.33224293864769194 ) ) ;
#127942=CARTESIAN_POINT ( 'NONE',  ( -13.97604488694547697, 13.89961937509957934, 73.12609039468568994 ) ) ;
#127943=CARTESIAN_POINT ( 'NONE',  ( 5.719274019375673035, 21.55341960407619339, 107.2927570613523471 ) ) ;
#127944=CARTESIAN_POINT ( 'NONE',  ( 5.153800228976335163, 19.02544592524342804, 39.79057627198100988 ) ) ;
#127945=CARTESIAN_POINT ( 'NONE',  ( -13.97604488694527625, -13.89961937509977652, 81.87390960531436690 ) ) ;
#127946=CARTESIAN_POINT ( 'NONE',  ( -4.483927247898539470, -16.52544592524342804, 72.29057627198102409 ) ) ;
#127947=CARTESIAN_POINT ( 'NONE',  ( -19.05341960407617563, 5.049401038297882671, 38.54275706135233293 ) ) ;
#127948=CARTESIAN_POINT ( 'NONE',  ( -18.62759615963270932, 10.81492255796079327, 40.83224293864769550 ) ) ;
#127949=CARTESIAN_POINT ( 'NONE',  ( 5.719274019375673035, 21.55341960407619339, 112.2927570613523471 ) ) ;
#127950=CARTESIAN_POINT ( 'NONE',  ( 19.03943276465977164, -0.05219959533909143690, 88.74890960531436690 ) ) ;
#127951=CARTESIAN_POINT ( 'NONE',  ( 5.719274019375673035, 21.55341960407619339, 102.2927570613523613 ) ) ;
#127952=CARTESIAN_POINT ( 'NONE',  ( 5.719274019375991003, -21.55341960407610458, 57.70724293864770260 ) ) ;
#127953=CARTESIAN_POINT ( 'NONE',  ( 16.46253265017160672, -9.564922557960803928, 93.33224293864769550 ) ) ;
#127954=CARTESIAN_POINT ( 'NONE',  ( -16.51473224551082808, 9.474510206698731452, 88.33442372801900433 ) ) ;
#127955=CARTESIAN_POINT ( 'NONE',  ( -13.89961937509977652, 13.97604488694528158, 100.6239096053143669 ) ) ;
#127957=CARTESIAN_POINT ( 'NONE',  ( 19.03943276465977164, 0.05219959533936151252, 96.25109039468567573 ) ) ;
#127958=CARTESIAN_POINT ( 'NONE',  ( 13.97604488694527802, 13.89961937509977652, 24.37390960531435624 ) ) ;
#127959=CARTESIAN_POINT ( 'NONE',  ( -0.05219959533909027116, -19.03943276465977164, 82.49890960531436690 ) ) ;
#127960=CARTESIAN_POINT ( 'NONE',  ( 21.55341960407610458, 5.719274019375980345, 68.95724293864769550 ) ) ;
#127961=CARTESIAN_POINT ( 'NONE',  ( 12.14591786802327356, -12.06949235617739191, 30.62609039468567929 ) ) ;
#127962=CARTESIAN_POINT ( 'NONE',  ( -10.72451020669870658, -18.67979575497194134, 44.58442372801901854 ) ) ;
#127963=CARTESIAN_POINT ( 'NONE',  ( -18.67979575497193778, 10.72451020669871902, 93.33442372801901854 ) ) ;
#127964=CARTESIAN_POINT ( 'NONE',  ( -4.379528057220086978, -16.55341960407618274, 94.79275706135234714 ) ) ;
#127965=CARTESIAN_POINT ( 'NONE',  ( 16.46253265017160672, -9.564922557960803928, 88.33224293864769550 ) ) ;
#127966=CARTESIAN_POINT ( 'NONE',  ( -14.29746914071049879, 8.314922557960819915, 90.83224293864769550 ) ) ;
#127967=CARTESIAN_POINT ( 'NONE',  ( 8.224510206698742110, 14.34966873604972548, 112.0844237280190185 ) ) ;
#127968=CARTESIAN_POINT ( 'NONE',  ( -9.564922557961040184, 16.46253265017147172, 62.91775706135233293 ) ) ;
#127969=CARTESIAN_POINT ( 'NONE',  ( 0.05219959533937995610, -21.53943276465977519, 50.00109039468568994 ) ) ;
#127971=CARTESIAN_POINT ( 'NONE',  ( 16.55341960407611168, 4.379528057220329451, 93.95724293864770971 ) ) ;
#127972=CARTESIAN_POINT ( 'NONE',  ( -16.51473224551069308, -9.474510206698971260, 106.6655762719810383 ) ) ;
#127973=CARTESIAN_POINT ( 'NONE',  ( -16.53943276465976808, 0.05219959533911058130, 26.24890960531435624 ) ) ;
#127974=CARTESIAN_POINT ( 'NONE',  ( 21.55341960407619695, -5.719274019375665929, 91.04275706135236135 ) ) ;
#127975=CARTESIAN_POINT ( 'NONE',  ( -16.55341960407617563, 4.379528057220093196, 38.54275706135234714 ) ) ;
#127976=CARTESIAN_POINT ( 'NONE',  ( -5.823673210054431948, 21.52544592524334988, 42.70942372801901854 ) ) ;
#127978=CARTESIAN_POINT ( 'NONE',  ( -18.62759615963255300, -10.81492255796106328, 19.16775706135234714 ) ) ;
#127979=CARTESIAN_POINT ( 'NONE',  ( -12.14591786802309592, -12.06949235617757132, 91.87390960531436690 ) ) ;
#127980=CARTESIAN_POINT ( 'NONE',  ( -5.153800228976328057, -19.02544592524343514, 27.29057627198103120 ) ) ;
#127981=CARTESIAN_POINT ( 'NONE',  ( 4.379528057220339221, -16.55341960407611168, 67.70724293864769550 ) ) ;
#127982=CARTESIAN_POINT ( 'NONE',  ( -19.03943276465977164, 0.05219959533909376836, 61.24890960531436690 ) ) ;
#127983=CARTESIAN_POINT ( 'NONE',  ( -16.53943276465976808, -0.05219959533934237506, 103.7510903946857042 ) ) ;
#127984=CARTESIAN_POINT ( 'NONE',  ( 5.153800228976335163, 19.02544592524342804, 44.79057627198103830 ) ) ;
#127985=CARTESIAN_POINT ( 'NONE',  ( -21.53943276465977519, 0.05219959533907696930, 46.24890960531435979 ) ) ;
#127986=CARTESIAN_POINT ( 'NONE',  ( -16.55341960407611168, -4.379528057220339221, 81.45724293864769550 ) ) ;
#127988=CARTESIAN_POINT ( 'NONE',  ( -21.53943276465977519, 0.05219959533907696930, 96.24890960531435269 ) ) ;
#127989=CARTESIAN_POINT ( 'NONE',  ( 16.46253265017160672, -9.564922557960803928, 93.33224293864769550 ) ) ;
#127990=CARTESIAN_POINT ( 'NONE',  ( -16.46253265017160317, 9.564922557960807481, 40.83224293864769550 ) ) ;
#127991=CARTESIAN_POINT ( 'NONE',  ( -16.51473224551082808, 9.474510206698731452, 93.33442372801900433 ) ) ;
#127992=CARTESIAN_POINT ( 'NONE',  ( 21.53943276465977519, -0.05219959533907433946, 43.74890960531435979 ) ) ;
#127993=CARTESIAN_POINT ( 'NONE',  ( 15.72974639402176855, 15.80617190586768217, 71.87609039468568994 ) ) ;
#127994=CARTESIAN_POINT ( 'NONE',  ( 16.46253265017160672, -9.564922557960803928, 58.33224293864769550 ) ) ;
#127995=CARTESIAN_POINT ( 'NONE',  ( -19.03943276465977164, 0.05219959533909376836, 81.24890960531436690 ) ) ;
#127997=CARTESIAN_POINT ( 'NONE',  ( -12.06949235617739369, -12.14591786802326823, 59.37609039468568284 ) ) ;
#127998=CARTESIAN_POINT ( 'NONE',  ( 10.81492255796106328, -18.62759615963255655, 50.41775706135235424 ) ) ;
#128000=CARTESIAN_POINT ( 'NONE',  ( 5.719274019375673035, 21.55341960407619339, 67.29275706135234714 ) ) ;
#128001=CARTESIAN_POINT ( 'NONE',  ( 15.72974639402199770, -15.80617190586745480, 23.12390960531436335 ) ) ;
#128002=CARTESIAN_POINT ( 'NONE',  ( -10.72451020669898014, 18.67979575497178502, 105.4155762719810383 ) ) ;
#128003=CARTESIAN_POINT ( 'NONE',  ( 18.62759615963255655, 10.81492255796105972, 31.66775706135234358 ) ) ;
#128004=CARTESIAN_POINT ( 'NONE',  ( -8.314922557961024197, 14.29746914071037800, 62.91775706135236135 ) ) ;
#128005=CARTESIAN_POINT ( 'NONE',  ( -18.67979575497178146, -10.72451020669898902, 66.66557627198102409 ) ) ;
#128006=CARTESIAN_POINT ( 'NONE',  ( 19.02544592524334988, 5.153800228976608722, 36.45942372801900433 ) ) ;
#128007=CARTESIAN_POINT ( 'NONE',  ( 5.049401038298161559, -19.05341960407611168, 72.70724293864768129 ) ) ;
#128008=CARTESIAN_POINT ( 'NONE',  ( -8.314922557961024197, 14.29746914071037800, 107.9177570613523471 ) ) ;
#128010=CARTESIAN_POINT ( 'NONE',  ( 0.05219959533909260263, 19.03943276465977164, 99.99890960531436690 ) ) ;
#128012=CARTESIAN_POINT ( 'NONE',  ( 13.97604488694548053, -13.89961937509957401, 85.62609039468568994 ) ) ;
#128013=CARTESIAN_POINT ( 'NONE',  ( -18.67979575497178146, -10.72451020669898902, 61.66557627198103120 ) ) ;
#128014=CARTESIAN_POINT ( 'NONE',  ( -12.06949235617756955, 12.14591786802309770, 35.62390960531437401 ) ) ;
#128015=CARTESIAN_POINT ( 'NONE',  ( -16.51473224551082808, 9.474510206698731452, 93.33442372801900433 ) ) ;
#128017=CARTESIAN_POINT ( 'NONE',  ( -19.05341960407617563, 5.049401038297882671, 98.54275706135233293 ) ) ;
#128018=CARTESIAN_POINT ( 'NONE',  ( -18.67979575497178146, -10.72451020669898902, 81.66557627198103830 ) ) ;
#128019=CARTESIAN_POINT ( 'NONE',  ( -5.153800228976607833, 19.02544592524334988, 52.70942372801900433 ) ) ;
#128021=CARTESIAN_POINT ( 'NONE',  ( -0.05219959533909027116, -19.03943276465977164, 67.49890960531436690 ) ) ;
#128022=CARTESIAN_POINT ( 'NONE',  ( -8.314922557960811034, -14.29746914071050412, 62.08224293864769550 ) ) ;
#128023=CARTESIAN_POINT ( 'NONE',  ( -19.03943276465977164, 0.05219959533909376836, 46.24890960531435979 ) ) ;
#128024=CARTESIAN_POINT ( 'NONE',  ( -4.379528057220328563, 16.55341960407611168, 55.20724293864770260 ) ) ;
#128027=CARTESIAN_POINT ( 'NONE',  ( 16.52544592524342804, -4.483927247898539470, 33.54057627198102409 ) ) ;
#128028=CARTESIAN_POINT ( 'NONE',  ( -9.564922557960796823, -16.46253265017161027, 62.08224293864769550 ) ) ;
#128030=CARTESIAN_POINT ( 'NONE',  ( -19.05341960407617563, 5.049401038297882671, 38.54275706135233293 ) ) ;
#128031=CARTESIAN_POINT ( 'NONE',  ( -16.53943276465976808, -0.05219959533934237506, 48.75109039468568284 ) ) ;
#128032=CARTESIAN_POINT ( 'NONE',  ( -15.72974639402197994, 15.80617190586746368, 45.62390960531436690 ) ) ;
#128033=CARTESIAN_POINT ( 'NONE',  ( 21.55341960407619695, -5.719274019375665929, 101.0427570613523756 ) ) ;
#128034=CARTESIAN_POINT ( 'NONE',  ( -5.153800228976328057, -19.02544592524343514, 77.29057627198099567 ) ) ;
#128036=CARTESIAN_POINT ( 'NONE',  ( 16.46253265017160672, -9.564922557960803928, 113.3322429386476955 ) ) ;
#128037=CARTESIAN_POINT ( 'NONE',  ( 5.823673210054444382, -21.52544592524334988, 45.20942372801901854 ) ) ;
#128039=CARTESIAN_POINT ( 'NONE',  ( -12.06949235617756955, 12.14591786802309770, 95.62390960531436690 ) ) ;
#128040=CARTESIAN_POINT ( 'NONE',  ( -10.81492255796078084, -18.62759615963271287, 92.08224293864769550 ) ) ;
#128041=CARTESIAN_POINT ( 'NONE',  ( 19.02544592524343514, -5.153800228976328945, 83.54057627198100988 ) ) ;
#128043=CARTESIAN_POINT ( 'NONE',  ( 19.02544592524343514, -5.153800228976328945, 88.54057627198102409 ) ) ;
#128044=CARTESIAN_POINT ( 'NONE',  ( 21.53943276465977519, 0.05219959533937863772, 31.25109039468568639 ) ) ;
#128046=CARTESIAN_POINT ( 'NONE',  ( 5.049401038298161559, -19.05341960407611168, 82.70724293864770971 ) ) ;
#128047=CARTESIAN_POINT ( 'NONE',  ( 18.39635199886970796, -5.499999999999976019, 83.51967076360001840 ) ) ;
#128048=CARTESIAN_POINT ( 'NONE',  ( 12.14591786802309770, 12.06949235617756955, 114.3739096053143527 ) ) ;
#128049=CARTESIAN_POINT ( 'NONE',  ( 9.474510206698971260, -16.51473224551069308, 32.91557627198102409 ) ) ;
#128050=CARTESIAN_POINT ( 'NONE',  ( 13.97604488694548053, -13.89961937509957401, 110.6260903946856615 ) ) ;
#128052=CARTESIAN_POINT ( 'NONE',  ( -16.52544592524342804, 4.483927247898546575, 106.0405762719810525 ) ) ;
#128053=CARTESIAN_POINT ( 'NONE',  ( 15.80617190586769283, -15.72974639402175789, 90.62609039468567573 ) ) ;
#128054=CARTESIAN_POINT ( 'NONE',  ( 13.89961937509977652, -13.97604488694527269, 68.12390960531436690 ) ) ;
#128055=CARTESIAN_POINT ( 'NONE',  ( 0.05219959533937995610, -21.53943276465977519, 30.00109039468568284 ) ) ;
#128056=CARTESIAN_POINT ( 'NONE',  ( 10.81492255796078972, 18.62759615963270932, 109.5822429386476955 ) ) ;
#128058=CARTESIAN_POINT ( 'NONE',  ( 19.05341960407611168, 5.049401038298154454, 88.95724293864769550 ) ) ;
#128060=CARTESIAN_POINT ( 'NONE',  ( 16.52544592524335698, 4.483927247898782831, 21.45942372801901499 ) ) ;
#128061=CARTESIAN_POINT ( 'NONE',  ( -15.80617190586745835, -15.72974639402198527, 41.87390960531435979 ) ) ;
#128062=CARTESIAN_POINT ( 'NONE',  ( -15.72974639402176322, -15.80617190586768395, 69.37609039468567573 ) ) ;
#128063=CARTESIAN_POINT ( 'NONE',  ( 16.46253265017160672, -9.564922557960803928, 108.3322429386476955 ) ) ;
#128064=CARTESIAN_POINT ( 'NONE',  ( -19.02544592524334988, -5.153800228976617603, 93.95942372801900433 ) ) ;
#128065=CARTESIAN_POINT ( 'NONE',  ( -13.89961937509977652, 13.97604488694528158, 60.62390960531436690 ) ) ;
#128066=CARTESIAN_POINT ( 'NONE',  ( -9.564922557960796823, -16.46253265017161027, 82.08224293864768129 ) ) ;
#128067=CARTESIAN_POINT ( 'NONE',  ( 4.483927247898545687, 16.52544592524342804, 89.79057627198103830 ) ) ;
#128068=CARTESIAN_POINT ( 'NONE',  ( -8.224510206698948167, 14.34966873604960824, 100.4155762719810241 ) ) ;
#128069=CARTESIAN_POINT ( 'NONE',  ( -13.89961937509977652, 13.97604488694528158, 115.6239096053143669 ) ) ;
#128070=CARTESIAN_POINT ( 'NONE',  ( -16.53943276465976808, 0.05219959533911058130, 51.24890960531436690 ) ) ;
#128071=CARTESIAN_POINT ( 'NONE',  ( 5.153800228976335163, 19.02544592524342804, 34.79057627198102409 ) ) ;
#128072=CARTESIAN_POINT ( 'NONE',  ( -5.823673210054431948, 21.52544592524334988, 67.70942372801901854 ) ) ;
#128073=CARTESIAN_POINT ( 'NONE',  ( 19.05341960407617918, -5.049401038297876454, 91.04275706135234714 ) ) ;
#128074=CARTESIAN_POINT ( 'NONE',  ( 4.379528057220339221, -16.55341960407611168, 57.70724293864770260 ) ) ;
#128075=CARTESIAN_POINT ( 'NONE',  ( 18.67979575497178502, 10.72451020669898547, 114.1655762719810383 ) ) ;
#128076=CARTESIAN_POINT ( 'NONE',  ( -10.72451020669898014, 18.67979575497178502, 45.41557627198103830 ) ) ;
#128077=CARTESIAN_POINT ( 'NONE',  ( 19.02544592524343514, -5.153800228976328945, 108.5405762719810383 ) ) ;
#128079=CARTESIAN_POINT ( 'NONE',  ( -13.89961937509977652, 13.97604488694528158, 65.62390960531436690 ) ) ;
#128080=CARTESIAN_POINT ( 'NONE',  ( -16.52544592524342804, 4.483927247898546575, 36.04057627198102409 ) ) ;
#128081=CARTESIAN_POINT ( 'NONE',  ( -16.53943276465976808, -0.05219959533934237506, 103.7510903946857042 ) ) ;
#128082=CARTESIAN_POINT ( 'NONE',  ( -16.52544592524335698, -4.483927247898792601, 88.95942372801901854 ) ) ;
#128083=CARTESIAN_POINT ( 'NONE',  ( 19.05341960407617918, -5.049401038297876454, 41.04275706135233293 ) ) ;
#128085=CARTESIAN_POINT ( 'NONE',  ( 16.51473224551069308, 9.474510206698969483, 89.16557627198103830 ) ) ;
#128086=CARTESIAN_POINT ( 'NONE',  ( 5.153800228976335163, 19.02544592524342804, 49.79057627198100988 ) ) ;
#128087=CARTESIAN_POINT ( 'NONE',  ( -16.55341960407611168, -4.379528057220339221, 61.45724293864770260 ) ) ;
#128088=CARTESIAN_POINT ( 'NONE',  ( 16.79531203550646268, -7.028104445595594107, 101.2475501177955977 ) ) ;
#128089=CARTESIAN_POINT ( 'NONE',  ( 9.564922557960805705, 16.46253265017160317, 114.5822429386476955 ) ) ;
#128090=CARTESIAN_POINT ( 'NONE',  ( 15.80617190586746368, 15.72974639402197994, 59.37390960531436690 ) ) ;
#128091=CARTESIAN_POINT ( 'NONE',  ( 4.379528057220339221, -16.55341960407611168, 82.70724293864770971 ) ) ;
#128092=CARTESIAN_POINT ( 'NONE',  ( 4.379528057220092307, 16.55341960407617563, 42.29275706135235424 ) ) ;
#128093=CARTESIAN_POINT ( 'NONE',  ( -16.53943276465976808, 0.05219959533911058130, 76.24890960531435269 ) ) ;
#128094=CARTESIAN_POINT ( 'NONE',  ( -19.26498983726237313, 5.499999999999599432, 65.55319577422002908 ) ) ;
#128095=CARTESIAN_POINT ( 'NONE',  ( -19.03943276465977164, -0.05219959533935918106, 73.75109039468566152 ) ) ;
#128096=CARTESIAN_POINT ( 'NONE',  ( 5.823673210054125526, 21.52544592524343514, 24.79057627198103120 ) ) ;
#128098=CARTESIAN_POINT ( 'NONE',  ( 19.48255537605750831, 5.500000000000000888, 102.3528781528247293 ) ) ;
#128099=CARTESIAN_POINT ( 'NONE',  ( -8.224510206698735004, -14.34966873604973081, 24.58442372801901499 ) ) ;
#128100=CARTESIAN_POINT ( 'NONE',  ( 4.483927247898790824, -16.52544592524335698, 105.2094237280190328 ) ) ;
#128101=CARTESIAN_POINT ( 'NONE',  ( 13.89961937509957401, 13.97604488694547697, 76.87609039468566152 ) ) ;
#128102=CARTESIAN_POINT ( 'NONE',  ( -5.719274019375978568, 21.55341960407610458, 45.20724293864769550 ) ) ;
#128103=CARTESIAN_POINT ( 'NONE',  ( -10.81492255796105439, 18.62759615963255655, 67.91775706135234714 ) ) ;
#128105=CARTESIAN_POINT ( 'NONE',  ( -16.52544592524335698, -4.483927247898792601, 33.95942372801901143 ) ) ;
#128106=CARTESIAN_POINT ( 'NONE',  ( 16.51473224551069308, 9.474510206698969483, 29.16557627198103475 ) ) ;
#128107=CARTESIAN_POINT ( 'NONE',  ( 5.049401038298161559, -19.05341960407611168, 87.70724293864769550 ) ) ;
#128108=CARTESIAN_POINT ( 'NONE',  ( -19.03943276465977164, 0.05219959533909376836, 21.24890960531436335 ) ) ;
#128109=CARTESIAN_POINT ( 'NONE',  ( 4.379528057220339221, -16.55341960407611168, 87.70724293864769550 ) ) ;
#128111=CARTESIAN_POINT ( 'NONE',  ( -9.564922557960796823, -16.46253265017161027, 97.08224293864769550 ) ) ;
#128113=CARTESIAN_POINT ( 'NONE',  ( 5.153800228976615827, -19.02544592524334988, 110.2094237280189901 ) ) ;
#128114=B_SPLINE_CURVE_WITH_KNOTS ( 'NONE', 3,
 ( #84350, #146028, #44598, #162205, #7511, #69195, #23703, #85351, #147044, #8528, #55030, #116700, #178390, #39854, #101520, #163210, #27464, #89106, #150796, #89960 ),
 .UNSPECIFIED., .F., .F.,
 ( 4, 2, 2, 2, 2, 2, 2, 2, 2, 4 ),
 ( 0.004000878361812037175, 0.004499404418916065282, 0.004997930476020092522, 0.005496456533124120629, 0.005994982590228148736, 0.006244245618780140672, 0.006493508647332134343, 0.006992034704436119949, 0.007490560761540107290, 0.007989086818644092897 ),
 .UNSPECIFIED. ) ;
#128115=CARTESIAN_POINT ( 'NONE',  ( 5.823673210054125526, 21.52544592524343514, 74.79057627198105251 ) ) ;
#128116=CARTESIAN_POINT ( 'NONE',  ( -9.474510206698964154, 16.51473224551069663, 40.41557627198103120 ) ) ;
#128117=CARTESIAN_POINT ( 'NONE',  ( 5.153800228976615827, -19.02544592524334988, 65.20942372801900433 ) ) ;
#128118=CARTESIAN_POINT ( 'NONE',  ( 21.55341960407619695, -5.719274019375665929, 21.04275706135234714 ) ) ;
#128119=CARTESIAN_POINT ( 'NONE',  ( -19.05341960407611168, -5.049401038298163336, 66.45724293864769550 ) ) ;
#128120=CARTESIAN_POINT ( 'NONE',  ( 9.564922557960805705, 16.46253265017160317, 109.5822429386476955 ) ) ;
#128123=CARTESIAN_POINT ( 'NONE',  ( -12.14591786802326823, 12.06949235617739902, 38.12609039468567573 ) ) ;
#128124=CARTESIAN_POINT ( 'NONE',  ( 15.72974639402199770, -15.80617190586745480, 108.1239096053143811 ) ) ;
#128125=CARTESIAN_POINT ( 'NONE',  ( 12.06949235617757843, -12.14591786802309237, 113.1239096053143953 ) ) ;
#128126=CARTESIAN_POINT ( 'NONE',  ( -0.05219959533909027116, -19.03943276465977164, 92.49890960531436690 ) ) ;
#128127=CARTESIAN_POINT ( 'NONE',  ( 5.049401038297881783, 19.05341960407617563, 57.29275706135231871 ) ) ;
#128128=CARTESIAN_POINT ( 'NONE',  ( -10.72451020669898014, 18.67979575497178502, 85.41557627198102409 ) ) ;
#128129=CARTESIAN_POINT ( 'NONE',  ( -0.05219959533910754901, -16.53943276465976808, 47.49890960531435979 ) ) ;
#128130=CARTESIAN_POINT ( 'NONE',  ( 18.62759615963255655, 10.81492255796105972, 111.6677570613523613 ) ) ;
#128131=CARTESIAN_POINT ( 'NONE',  ( 16.53943276465976808, 0.05219959533934440121, 61.25109039468567573 ) ) ;
#128133=CARTESIAN_POINT ( 'NONE',  ( 13.97604488694527802, 13.89961937509977652, 94.37390960531436690 ) ) ;
#128134=CARTESIAN_POINT ( 'NONE',  ( -9.564922557960796823, -16.46253265017161027, 47.08224293864769550 ) ) ;
#128136=CARTESIAN_POINT ( 'NONE',  ( -21.55341960407619339, 5.719274019375674811, 53.54275706135234714 ) ) ;
#128137=CARTESIAN_POINT ( 'NONE',  ( -18.62759615963255300, -10.81492255796106328, 74.16775706135231871 ) ) ;
#128138=CARTESIAN_POINT ( 'NONE',  ( 16.46253265017160672, -9.564922557960803928, 63.33224293864769550 ) ) ;
#128139=CARTESIAN_POINT ( 'NONE',  ( -10.72451020669870658, -18.67979575497194134, 29.58442372801901854 ) ) ;
#128140=CARTESIAN_POINT ( 'NONE',  ( -19.03943276465977164, -0.05219959533935918106, 68.75109039468566152 ) ) ;
#128141=CARTESIAN_POINT ( 'NONE',  ( 19.03943276465977164, -0.05219959533909143690, 38.74890960531436690 ) ) ;
#128142=CARTESIAN_POINT ( 'NONE',  ( -14.34966873604972548, 8.224510206698743886, 83.33442372801903275 ) ) ;
#128143=CARTESIAN_POINT ( 'NONE',  ( -16.51473224551069308, -9.474510206698971260, 51.66557627198102409 ) ) ;
#128144=CARTESIAN_POINT ( 'NONE',  ( -19.02544592524342804, 5.153800228976336051, 106.0405762719810241 ) ) ;
#128145=CARTESIAN_POINT ( 'NONE',  ( 9.474510206698971260, -16.51473224551069308, 37.91557627198102409 ) ) ;
#128146=CARTESIAN_POINT ( 'NONE',  ( -18.62759615963270932, 10.81492255796079327, 80.83224293864769550 ) ) ;
#128147=CARTESIAN_POINT ( 'NONE',  ( -12.14591786802326823, 12.06949235617739902, 68.12609039468567573 ) ) ;
#128150=CARTESIAN_POINT ( 'NONE',  ( 0.05219959533936267826, -19.03943276465977164, 30.00109039468566863 ) ) ;
#128151=CARTESIAN_POINT ( 'NONE',  ( -0.05219959533909027116, -19.03943276465977164, 52.49890960531436690 ) ) ;
#128152=CARTESIAN_POINT ( 'NONE',  ( 14.34966873604960469, 8.224510206698951720, 49.16557627198102409 ) ) ;
#128153=CARTESIAN_POINT ( 'NONE',  ( -14.34966873604960291, -8.224510206698953496, 76.66557627198103830 ) ) ;
#128154=CARTESIAN_POINT ( 'NONE',  ( 19.02544592524343514, -5.153800228976328945, 98.54057627198100988 ) ) ;
#128155=CARTESIAN_POINT ( 'NONE',  ( 16.46253265017160672, -9.564922557960803928, 78.33224293864769550 ) ) ;
#128156=CARTESIAN_POINT ( 'NONE',  ( 0.05219959533937995610, -21.53943276465977519, 50.00109039468568994 ) ) ;
#128157=CARTESIAN_POINT ( 'NONE',  ( -5.049401038298153566, 19.05341960407611168, 95.20724293864770971 ) ) ;
#128158=CARTESIAN_POINT ( 'NONE',  ( 21.55341960407619695, -5.719274019375665929, 106.0427570613523471 ) ) ;
#128159=CARTESIAN_POINT ( 'NONE',  ( -16.52544592524335698, -4.483927247898792601, 78.95942372801901854 ) ) ;
#128160=CARTESIAN_POINT ( 'NONE',  ( -21.53943276465977519, -0.05219959533937600094, 23.75109039468567929 ) ) ;
#128161=CARTESIAN_POINT ( 'NONE',  ( 15.80617190586746368, 15.72974639402197994, 109.3739096053143811 ) ) ;
#128162=CARTESIAN_POINT ( 'NONE',  ( -12.14591786802309592, -12.06949235617757132, 66.87390960531436690 ) ) ;
#128163=CARTESIAN_POINT ( 'NONE',  ( -0.05219959533909027116, -19.03943276465977164, 37.49890960531436690 ) ) ;
#128164=CARTESIAN_POINT ( 'NONE',  ( -0.05219959533910754901, -16.53943276465976808, 62.49890960531436690 ) ) ;
#128165=CARTESIAN_POINT ( 'NONE',  ( 0.05219959533907565091, 21.53943276465977519, 34.99890960531435979 ) ) ;
#128166=CARTESIAN_POINT ( 'NONE',  ( -13.89961937509957401, -13.97604488694547875, 24.37609039468565442 ) ) ;
#128167=CARTESIAN_POINT ( 'NONE',  ( -0.05219959533910754901, -16.53943276465976808, 97.49890960531436690 ) ) ;
#128169=CARTESIAN_POINT ( 'NONE',  ( -12.14591786802326823, 12.06949235617739902, 63.12609039468568994 ) ) ;
#128170=CARTESIAN_POINT ( 'NONE',  ( -19.02544592524342804, 5.153800228976336051, 66.04057627198103830 ) ) ;
#128172=CARTESIAN_POINT ( 'NONE',  ( 16.52544592524342804, -4.483927247898539470, 83.54057627198102409 ) ) ;
#128173=CARTESIAN_POINT ( 'NONE',  ( -21.52544592524343514, 5.823673210054127303, 31.04057627198102409 ) ) ;
#128174=CARTESIAN_POINT ( 'NONE',  ( 4.483927247898790824, -16.52544592524335698, 95.20942372801903275 ) ) ;
#128175=CARTESIAN_POINT ( 'NONE',  ( -9.564922557961040184, 16.46253265017147172, 112.9177570613523329 ) ) ;
#128176=CARTESIAN_POINT ( 'NONE',  ( -18.67979575497193778, 10.72451020669871902, 78.33442372801901854 ) ) ;
#128177=CARTESIAN_POINT ( 'NONE',  ( -19.05341960407611168, -5.049401038298163336, 91.45724293864766707 ) ) ;
#128178=CARTESIAN_POINT ( 'NONE',  ( -15.80617190586745835, -15.72974639402198527, 106.8739096053143811 ) ) ;
#128179=CARTESIAN_POINT ( 'NONE',  ( -12.14591786802326823, 12.06949235617739902, 53.12609039468568284 ) ) ;
#128180=CARTESIAN_POINT ( 'NONE',  ( -12.14591786802309592, -12.06949235617757132, 106.8739096053143811 ) ) ;
#128182=CARTESIAN_POINT ( 'NONE',  ( -9.564922557961040184, 16.46253265017147172, 112.9177570613523329 ) ) ;
#128183=CARTESIAN_POINT ( 'NONE',  ( 13.97604488694548053, -13.89961937509957401, 85.62609039468568994 ) ) ;
#128184=CARTESIAN_POINT ( 'NONE',  ( 15.72974639402199770, -15.80617190586745480, 83.12390960531436690 ) ) ;
#128185=CARTESIAN_POINT ( 'NONE',  ( 9.564922557961047289, -16.46253265017146816, 50.41775706135233293 ) ) ;
#128186=CARTESIAN_POINT ( 'NONE',  ( 19.36337904590692460, -5.499999999999944933, 87.91494137495620009 ) ) ;
#128187=CARTESIAN_POINT ( 'NONE',  ( 10.81492255796078972, 18.62759615963270932, 109.5822429386476955 ) ) ;
#128188=CARTESIAN_POINT ( 'NONE',  ( -17.48847506799967988, 5.747544572773786165, 85.82697437843280852 ) ) ;
#128189=CARTESIAN_POINT ( 'NONE',  ( -19.03943276465977164, 0.05219959533909376836, 81.24890960531436690 ) ) ;
#128190=CARTESIAN_POINT ( 'NONE',  ( 15.50000000000000178, 5.499999999999998224, 118.0000000000000142 ) ) ;
#128191=CARTESIAN_POINT ( 'NONE',  ( -16.52544592524335698, -4.483927247898792601, 28.95942372801902209 ) ) ;
#128193=CARTESIAN_POINT ( 'NONE',  ( 18.62759615963271287, -10.81492255796078972, 98.33224293864769550 ) ) ;
#128194=CARTESIAN_POINT ( 'NONE',  ( -14.29746914071049879, 8.314922557960819915, 70.83224293864770971 ) ) ;
#128195=CARTESIAN_POINT ( 'NONE',  ( 16.51473224551069308, 9.474510206698969483, 64.16557627198102409 ) ) ;
#128196=CARTESIAN_POINT ( 'NONE',  ( -15.80617190586768217, 15.72974639402176855, 88.12609039468570415 ) ) ;
#128197=CARTESIAN_POINT ( 'NONE',  ( -16.52544592524335698, -4.483927247898792601, 38.95942372801901854 ) ) ;
#128198=( BOUNDED_SURFACE ( )  B_SPLINE_SURFACE ( 3, 2, ( 
 ( #70350, #176538, #25864, #69339, #38014, #55174, #115853, #26860, #148193, #146170, #129985, #99670, #41018, #149196, #9686, #195716, #53166, #56174, #131005, #71351, #147188, #22845, #161354, #191685, #194705, #84492, #7655, #72350, #133015, #57189, #179548, #8678, #163363, #101673, #117855, #132017, #177543, #165366, #162349, #145173, #116844, #114844, #192697, #103687, #40001, #164370, #102684, #68335, #24859, #54180, #39012, #100667, #86508, #87508, #10686, #118865, #180549, #42022, #6657, #73363, #14648, #105663, #43011, #135035, #196711, #154151, #58180, #166365, #136013, #168325, #449, #76308, #77302, #106653, #170313, #104678, #60147, #27862, #107630, #184497, #198680, #137986, #181532, #89503, #15643, #199669, #138971, #122807, #167350, #29822, #44994, #61135, #28848, #59151, #108635, #90488, #88502, #121815, #119847, #151192, #46976, #152170, #169308, #91458, #11696, #75320, #12681, #197686, #74347, #44002, #182521, #45976, #13653, #136991, #120821, #92463, #183511, #30814, #153146, #62124, #123787, #185486, #150198, #1446, #109630, #79291, #111618, #143937, #19612, #20594, #49954, #113592, #47977, #3435, #186501, #50947, #127769, #141945, #81254, #124803, #34778, #4417, #31806, #139956, #93456, #78283, #32800, #51932, #64129, #173303, #80274, #188473, #16636, #171313, #94452, #67101, #96434, #142936, #63124, #158121, #156132, #157132, #155143, #159100, #17631, #66103, #189469, #140960, #112606, #2447, #174298, #35767, #97413, #82246, #5418, #128760, #190459, #65111, #125794, #126769, #110616, #187496, #48962, #18627, #172298, #33787, #95447, #55932, #99427, #68095, #85255, #145932, #59662, #178296, #176293, #160111, #129747, #71108, #179307, #39760, #164127, #83257, #86266, #161109, #101423, #115614, #52920, #191444, #21599, #144932, #8436, #24618, #117607, #147956, #40771, #25625, #9443, #23609, #7414, #69097, #146947, #130764, #163115, #6414, #70108, #192456, #132774, #114596, #131777, #87270, #98415, #194461, #37765, #193459, #102440, #175286, #148954, #22605, #84251, #54936, #136511, #177303, #53939, #13185, #116608, #74848, #38775, #100431, #162112, #198192, #36751, #183028, #46485, #125322, #170828, #44511, #153662, #78801, #187019, #124312, #108145, #121335, #91968, #31322, #107151, #137502, #169829, #15158, #106167, #960, #45496, #90979, #199182, #32320, #17148, #62636, #63647, #14156, #47492, #168821, #186010, #61640, #122322, #60649, #152666, #109149, #184014, #30326, #140479, #93973, #167850, #155653, #123308, #139478, #16155, #1967, #185001, #76818, #29350, #92974, #75824, #138489, #154659, #77809, #200171, #165530, #120988, #104840, #22253, #88671, #164530, #10850, #26023, #57356, #195882, #136177, #180713, #119030, #68744, #105830, #83902, #28028, #42189, #53582, #145585, #7063, #167517, #130402, #176952, #149353, #181692, #13820, #89669, #90652, #120007, #183679, #150367, #58339, #192100, #115259, #41182, #137159, #43173, #151356, #102845, #166531, #87668, #27026, #121988, #29012, #72519, #12845, #74511, #134194, #197852, #99073, #59319, #182686, #44171, #152334, #75486, #198848, #60312, #135200, #160763, #11863, #103849, #73528, #196872, #170484, #93631, #65283, #15811, #78455, #169483, #138158, #155316, #77472, #126942, #48143, #46145, #29992, #199839, #141132, #49135, #109800, #33961, #153319, #156305, #30983, #171483, #185655, #122976, #61306, #91631, #94626, #184663, #107799, #172474, #32972, #95619, #79463, #123957, #63296, #1620, #17806, #47147, #139142, #45164, #62289, #106820, #16805, #14820, #76481, #3604, #108805, #64299, #2622, #168494, #31975, #92631, #154322, #619, #140129, #124976, #125966, #186673, #187664, #110793, #157304, #18801, #80446, #142119, #143107, #34950, #96602, #54110, #158291, #66279, #35936, #68265, #100599, #176467, #177473, #6586, #70282, #4586, #160284, #127938, #7585, #84424, #98590, #37940, #81421, #191616, #161281, #188650 ),
 ( #36928, #67270, #115784, #173477, #113761, #21775, #8609, #159270, #83426, #112774, #189640, #145103, #20766, #50129, #53095, #51115, #19780, #174467, #146101, #192628, #114773, #38942, #97582, #99601, #82421, #22776, #128928, #144110, #5590, #190629, #69271, #52104, #175457, #162281, #130937, #23781, #85431, #129916, #147122, #111789, #11740, #91502, #28890, #44047, #90530, #74389, #43053, #150245, #89548, #12723, #60190, #165411, #56221, #103731, #59195, #197729, #152212, #106696, #102727, #151234, #166410, #87553, #45038, #42067, #120864, #26904, #27905, #137033, #121860, #75363, #72395, #149240, #180593, #104719, #182564, #119890, #73407, #179592, #13696, #41064, #164416, #25909, #136054, #105707, #198723, #167394, #183552, #168369, #29865, #58221, #88547, #135078, #181575, #196754, #9731, #194749, #71395, #133059, #117903, #10731, #134071, #195761, #57235, #118909, #46019, #186547, #18671, #34820, #80317, #107675, #122851, #171357, #111662, #93503, #108680, #188520, #32845, #156177, #92508, #155189, #62167, #16679, #153189, #141990, #169352, #184539, #94495, #173349, #78328, #170358, #49997, #17676, #79334, #154197, #140001, #123831, #1490, #141004, #14692, #48019, #76355, #95491, #138031, #31850, #126814, #199714, #187540, #61179, #30861, #33831, #63168, #64173, #15687, #77348, #109676, #139015, #494, #185529, #47021, #124847, #125838, #2492, #49007, #110662, #172342, #157177, #3478, #65155, #160156, #131821, #52964, #36797, #21647, #116649, #130808, #69141, #176339, #177345, #114641, #158163, #112648, #192499, #67146, #98462, #178339, #115656, #53983, #38816, #161152, #129789, #83300, #37811, #99472, #146989, #51977, #142980, #190503, #145975, #84296, #100474, #193501, #189515, #22649, #7457, #174340, #54979, #128804, #162153, #113635, #23649, #85297, #8476, #70151, #159142, #35810, #175330, #191486, #96475, #6457, #144976, #66147, #19655, #127810, #50988, #97456, #81296, #4458, #20639, #82292, #143983, #5464, #68138, #88300, #10486, #72146, #11494, #133822, #42817, #24660, #73165, #195513, #135822, #71151, #134835, #28651, #163157, #197492, #132817, #196514, #105466, #166164, #57984, #120627, #167152, #104480, #58959, #119656, #90287, #149988, #118660, #151971, #86309, #165165, #181338, #59949, #56986, #27665, #164170, #194503, #89305, #180351, #121616, #150997, #40813, #147998, #55976, #182324, #43803, #12489, #13459, #9487, #74150, #25668, #75123, #41819, #117653, #179350, #102483, #136791, #87313, #148997, #198477, #39801, #101466, #103487, #26658, #1244, #139757, #109431, #187297, #94255, #95253, #168127, #64918, #154943, #91255, #152946, #141754, #46779, #2248, #186298, #106446, #170114, #45782, #92266, #107434, #138773, #77104, #17430, #61923, #254, #14445, #48769, #29623, #171111, #123593, #137784, #76108, #199469, #110423, #60936, #122610, #30613, #62923, #156938, #32602, #172104, #124603, #183311, #184300, #16440, #169106, #63931, #79087, #93258, #155935, #153950, #47778, #140760, #44793, #15446, #185287, #108438, #31608, #3244, #78089, #125600, #33590, #18435, #80085, #81068, #19420, #161917, #144737, #176098, #34585, #191256, #96242, #51738, #146741, #53745, #157930, #52731, #99231, #112413, #6224, #126579, #114397, #188280, #173108, #127578, #8236, #158908, #67903, #175090, #83063, #111422, #142746, #4226, #23411, #129556, #37568, #65905, #160918, #189279, #113400, #49754, #115419, #50755, #22411, #84062, #174105, #145740, #35574, #7221, #68906, #130566, #192263, #177108, #38579, #100235, #159916, #85059, #36558, #5222, #97222, #20399, #98213, #21405, #82048, #143743, #66903, #128566, #190261, #180118, #40579, #151742, #72928, #70916, #54738, #24424, #165926, #73919, #134597, #58723, #178099, #181106, #194272, #196283, #10249, #147763, #86073, #116410, #119422, #162916, #9249, #197261, #57752, #120392, #104243, #148760, #88065, #26425, #42580, #135589, #27423, #182086 ),
 ( #89068, #166922, #132584, #149752, #11255, #55739, #105234, #102249, #150759, #163937, #12257, #43569, #28423, #90060, #117413, #179111, #25434, #164932, #69914, #41586, #133580, #39569, #131580, #101227, #87075, #71908, #103250, #193264, #195270, #56754, #118425, #2020, #62685, #61691, #184064, #45547, #106216, #93025, #169882, #91030, #48540, #107202, #1011, #168872, #31375, #140531, #63699, #78852, #75875, #152716, #30377, #108201, #186062, #123360, #76869, #183078, #32369, #44561, #167900, #29400, #46541, #124367, #94022, #47545, #155703, #125374, #109199, #185053, #92022, #153714, #154713, #15210, #16206, #198242, #77861, #138539, #170878, #14207, #139528, #187070, #136561, #17198, #137551, #110194, #171872, #95020, #33361, #199234, #60699, #13235, #74898, #17, #59714, #121386, #122375, #159669, #96016, #96995, #65675, #158678, #174856, #18202, #51506, #179624, #98987, #141528, #35344, #133089, #41096, #191019, #79860, #34355, #37328, #20167, #67666, #194779, #56253, #190032, #3016, #142517, #111184, #117935, #3995, #129323, #156709, #113168, #36322, #127337, #64693, #49521, #21165, #81812, #126354, #97976, #143500, #4984, #188051, #52494, #114154, #82821, #160676, #144502, #172874, #157701, #175856, #189049, #66670, #19191, #22168, #86585, #148269, #5986, #9761, #128333, #71425, #80840, #50524, #112186, #173874, #196785, #152245, #90563, #121893, #199746, #58253, #138065, #182597, #105740, #42098, #43085, #11774, #104752, #120897, #164447, #197761, #122884, #45071, #87584, #181607, #76389, #184572, #137068, #25941, #180626, #183586, #166442, #13730, #61212, #102760, #136087, #149271, #88579, #57267, #10763, #150277, #75396, #72427, #59228, #44082, #73438, #134105, #195795, #167427, #27938, #118941, #28923, #89580, #151266, #103763, #198758, #60224, #106729, #168403, #29898, #165442, #26937, #91536, #135109, #12756, #119921, #153223, #14728, #74421, #110698, #79371, #186582, #125875, #49043, #96511, #1525, #92543, #140036, #95528, #33869, #65192, #143016, #139049, #187575, #2528, #123865, #81333, #78362, #157215, #63204, #64208, #173386, #158201, #111700, #108715, #185563, #16712, #141042, #18708, #156213, #109711, #15721, #126851, #77381, #529, #62201, #172378, #80355, #188557, #142027, #50036, #34856, #3516, #94531, #124884, #48055, #17713, #171394, #19691, #30895, #4494, #32881, #66185, #47057, #127847, #46053, #169387, #107708, #170393, #154231, #31884, #93538, #155223, #144019, #159179, #7495, #148034, #129826, #9523, #131858, #174377, #68174, #163195, #71189, #23688, #112685, #67182, #70191, #191525, #100511, #24699, #86348, #22686, #35847, #175365, #5500, #189552, #36833, #162190, #51024, #84333, #69180, #98499, #97493, #82329, #54021, #53002, #20674, #146012, #114681, #176376, #128839, #85336, #147029, #130846, #193542, #192538, #190538, #52012, #8513, #160193, #37850, #113671, #55015, #116685, #178375, #115694, #177383, #99509, #38854, #39839, #101505, #145013, #21683, #83336, #6494, #161190, #152008, #29660, #25704, #12523, #89341, #10523, #168163, #165201, #120662, #26696, #151033, #59985, #183347, #152983, #90323, #13494, #72186, #180389, #74188, #44829, #182360, #121653, #135857, #14482, #149035, #104517, #87349, #75159, #28687, #42852, #43838, #133860, #197527, #105503, #132853, #40850, #194541, #179387, #195551, #56012, #88336, #58996, #181374, #167189, #117690, #57025, #118698, #91292, #136831, #198514, #102524, #106485, #164206, #58021, #41860, #103526, #150027, #11533, #73202, #134873, #196550, #119690, #166198, #27699, #32636, #156971, #141786, #140795, #172138, #96276, #33624, #95287, #153987, #123627, #155968, #188313, #63966, #64952, #94290, #157962, #92304, #47815, #30650, #18468, #80118, #186333, #125636, #169146, #79122, #48803, #76144, #184336, #137823, #122647, #77141, #199506, #108472, #17466, #124638, #2284, #60972, #15484, #138811, #111456, #187333, #110457 ),
 ( #3281, #126611, #49790, #173142, #34617, #45818, #109464, #107469, #171148, #154979, #291, #61960, #1281, #185323, #46813, #170151, #31644, #93293, #16474, #78123, #139792, #62957, #22442, #20430, #4260, #174136, #115450, #23443, #84092, #8268, #127611, #130600, #143773, #145770, #159947, #97253, #35608, #65940, #68937, #112447, #158941, #146775, #7252, #69947, #53775, #98245, #37600, #176130, #192296, #85090, #177140, #131612, #189310, #101259, #191284, #50788, #82081, #178133, #83095, #38611, #100267, #142779, #6255, #5254, #128598, #66936, #175121, #113429, #161948, #21434, #36589, #190292, #193296, #51769, #54771, #144770, #67935, #52759, #129588, #116445, #99263, #39600, #114429, #19454, #160949, #81101, #183109, #90089, #70946, #89099, #135619, #148792, #181137, #162949, #150790, #12286, #119452, #43599, #28453, #27458, #58753, #196313, #151771, #11286, #41617, #13264, #147796, #88097, #72959, #44591, #133610, #57782, #87106, #55769, #134628, #195304, #24455, #165957, #163968, #9281, #117443, #120422, #166950, #73951, #74927, #132616, #197290, #10282, #182113, #103282, #40610, #179142, #194303, #105264, #102280, #25466, #136590, #198270, #59747, #121417, #164962, #42611, #104275, #86104, #71940, #56785, #118457, #180149, #26455, #149783, #14237, #75909, #64724, #169914, #125404, #109228, #29429, #93057, #168904, #15241, #30410, #61724, #49, #140561, #185084, #123392, #137583, #110224, #91060, #32399, #46573, #60734, #77892, #126386, #63729, #187101, #184097, #153746, #186094, #18235, #94054, #95052, #124400, #188083, #122407, #139560, #45580, #48571, #2050, #16240, #155732, #199266, #170907, #78882, #106247, #107233, #167929, #152747, #92057, #76900, #138571, #47576, #154744, #62717, #108234, #31406, #156741, #171905, #1044, #17230, #33393, #79889, #141559, #3048, #161711, #34387, #131367, #21199, #157734, #19223, #8018, #113200, #68693, #52525, #172909, #36355, #112216, #158708, #173906, #5019, #143531, #83850, #128365, #66701, #80873, #53528, #96047, #175890, #190061, #4027, #82855, #69700, #7011, #130348, #127371, #97027, #129357, #23207, #37361, #38369, #67699, #49554, #65705, #144534, #189083, #192047, #145532, #159702, #99019, #142549, #114186, #22201, #111217, #50556, #35375, #20197, #81843, #51537, #174889, #191052, #98007, #6020, #160710, #115206, #176898, #84850, #100024, #146527, #101023, #57544, #162708, #118215, #13030, #120190, #24213, #119213, #165715, #178896, #11037, #193056, #180898, #42373, #149542, #73714, #58524, #104036, #88858, #26215, #181880, #41372, #71701, #43359, #177895, #179906, #103038, #74696, #163722, #87854, #117204, #85862, #164720, #25224, #54533, #196071, #194069, #39365, #147551, #150551, #197056, #27212, #105030, #9039, #12050, #40364, #135386, #133368, #70708, #132376, #55530, #166714, #102039, #86866, #28218, #89858, #72713, #134385, #148550, #10041, #195059, #151541, #116206, #56537, #44355, #811, #106014, #61493, #156498, #63494, #167700, #62484, #108997, #122172, #154509, #136361, #124156, #185856, #92823, #16996, #1815, #47342, #32166, #169677, #125169, #184851, #15006, #186868, #121180, #123163, #46335, #18000, #107001, #31173, #60496, #29197, #107991, #168674, #198037, #139332, #137347, #182874, #90831, #93823, #140325, #170678, #48337, #152515, #155503, #183862, #78650, #76666, #14003, #75670, #199027, #109992, #45349, #30174, #171672, #33161, #94820, #59505, #138345, #16005, #77663, #91817, #153509, #200025, #191808, #64489, #161477, #51304, #187852, #49321, #38138, #143294, #98782, #82615, #2811, #66468, #142314, #188840, #3794, #35139, #173672, #113949, #158480, #96791, #110981, #83618, #126156, #5786, #19968, #34152, #112965, #99791, #37123, #160476, #157498, #127134, #159462, #53290, #67460, #68458, #97775, #79653, #95812, #174658, #18991, #21967, #175648, #189832, #129118, #172666, #144296, #52292, #141322, #80637, #65471 ),
 ( #50325, #145296, #111980, #81610, #4780, #6779, #130112, #114968, #190817, #36123, #128130, #20958, #176661, #73478, #178655, #69464, #116964, #72472, #10803, #42141, #119960, #115972, #102800, #179666, #100784, #58291, #55292, #134146, #40117, #41136, #150319, #165482, #131130, #101796, #104793, #193827, #117976, #195834, #133130, #86626, #192818, #103802, #54300, #177660, #39129, #56293, #57306, #26978, #118982, #88621, #11814, #180665, #71465, #163483, #24980, #194821, #148309, #25980, #7780, #164486, #9803, #135151, #162467, #87623, #196824, #146293, #181646, #23968, #149309, #43125, #22966, #84614, #85624, #147310, #8799, #70469, #132135, #121935, #4288, #46094, #169431, #105781, #106769, #75438, #168444, #184613, #27980, #61255, #189339, #111484, #151308, #45112, #142808, #50817, #3308, #89619, #44122, #49820, #29940, #77421, #65969, #127639, #199787, #12797, #152286, #120939, #166482, #13770, #139093, #74462, #122925, #107749, #137112, #136128, #59270, #30936, #91579, #197804, #92583, #153268, #182639, #154271, #15762, #167468, #28963, #198799, #64981, #60264, #126639, #96304, #173169, #90604, #183630, #14770, #76430, #188341, #34645, #138106, #157990, #19481, #81127, #143803, #5286, #82112, #145799, #161976, #193326, #23472, #54800, #101289, #85121, #160978, #83125, #144801, #84120, #6284, #115480, #97282, #7282, #67963, #8298, #66969, #68966, #162979, #35637, #69976, #128629, #130629, #178164, #194333, #39629, #190322, #51799, #192324, #70977, #52788, #129617, #147826, #53805, #177168, #113458, #114457, #21463, #176159, #38641, #174167, #100298, #132645, #116475, #158970, #191312, #86134, #112474, #146805, #20462, #175151, #24484, #37629, #131644, #9312, #36619, #98276, #159977, #99292, #22472, #29458, #103311, #166979, #14269, #89129, #135648, #164991, #137613, #148821, #120451, #119481, #91090, #12314, #196342, #181164, #75938, #90116, #28482, #197318, #136618, #73979, #117473, #71968, #151800, #26485, #57810, #55801, #74955, #13291, #198299, #182144, #150817, #42641, #58782, #43628, #106274, #11317, #102308, #149811, #105291, #59776, #121445, #152777, #183137, #179171, #44621, #40639, #167959, #163997, #134656, #25494, #87137, #10311, #133642, #195333, #56813, #104303, #118487, #180178, #41646, #88127, #72987, #165986, #27486, #172938, #46603, #110253, #157765, #32429, #78913, #108263, #80902, #92087, #63759, #62748, #34417, #155762, #139588, #124428, #19255, #33423, #171934, #140590, #79917, #17260, #60764, #15271, #95082, #169943, #1073, #199297, #18264, #156770, #141589, #125433, #94083, #186124, #2080, #187129, #49584, #154772, #45611, #93088, #48601, #3077, #64753, #96076, #153776, #126415, #188112, #76931, #122436, #31434, #111247, #16269, #184128, #107263, #168934, #30440, #77921, #138600, #47604, #82, #61752, #109258, #170937, #123420, #185113, #112246, #173937, #50586, #67731, #160742, #130382, #22234, #192080, #38402, #83883, #82889, #128396, #190093, #6053, #51568, #175924, #65736, #129389, #113232, #7043, #35405, #191085, #176932, #4058, #145565, #97056, #52558, #53562, #8057, #100059, #158739, #20228, #114219, #84883, #36386, #174922, #161744, #37395, #99053, #81876, #98040, #66736, #159737, #68725, #21234, #115240, #127404, #23239, #144567, #146562, #143568, #142579, #189113, #5050, #18915, #15928, #156421, #188765, #4704, #50249, #77587, #92746, #141246, #81535, #63416, #78572, #158405, #2735, #126081, #62406, #125091, #32091, #186789, #64412, #184774, #17922, #143222, #65397, #107915, #1738, #96717, #123088, #157421, #46260, #734, #3720, #48260, #34077, #19894, #169600, #79577, #31098, #108921, #139258, #154434, #170601, #95735, #124076, #187777, #49247, #93748, #185777, #47264, #110905, #109913, #155429, #172591, #171597, #33085, #16919, #80560, #142235, #127058, #111905, #173593, #140246, #94741, #35062, #37049, #68380, #148237, #85548, #100712, #147234 ),
 ( #159390, #146214, #22891, #144225, #101720, #98708, #54226, #160402, #84537, #193752, #67386, #52218, #113875, #38059, #5709, #175572, #7702, #178581, #115897, #55220, #69385, #66394, #82543, #99715, #20885, #8726, #162392, #176585, #177587, #129043, #131054, #39054, #128056, #174585, #23895, #36050, #192744, #97699, #191731, #86553, #116889, #190744, #70395, #132063, #21891, #40046, #189758, #163410, #24906, #51230, #112891, #83541, #145220, #6702, #161399, #130032, #114891, #53213, #6282, #22470, #35634, #190319, #193324, #114455, #23470, #86132, #147824, #145797, #158967, #98273, #66966, #9310, #159974, #85119, #70975, #7280, #192322, #21461, #194331, #5283, #177166, #176157, #132643, #68964, #52786, #37627, #112471, #146803, #8296, #53803, #54798, #130626, #174164, #128626, #69974, #83123, #99290, #97279, #131642, #116473, #178162, #38639, #115478, #160976, #100296, #161974, #162977, #67960, #20459, #129615, #39627, #101287, #24482, #82109, #51796, #143800, #113455, #175148, #36616, #144799, #191310, #84118, #73977, #183135, #28480, #29456, #90114, #196340, #26483, #150815, #151798, #165984, #119479, #25492, #74953, #87135, #148819, #10309, #89127, #105289, #136616, #166977, #198297, #44619, #13289, #104301, #88125, #149809, #27484, #11315, #58780, #40637, #12312, #72985, #59774, #71966, #135646, #106272, #179169, #121443, #133640, #197316, #103309, #137611, #195331, #120449, #181162, #91088, #182142, #57808, #42639, #75936, #167957, #152775, #43626, #14267, #55799, #117471, #56811, #102306, #134654, #163995, #118485, #180176, #41644, #164989, #63756, #32426, #139585, #78910, #2077, #49581, #154770, #45608, #93086, #48598, #187126, #18261, #96072, #92085, #140587, #155759, #76929, #34414, #31432, #110250, #16267, #17257, #126412, #171931, #172935, #33420, #1070, #169941, #94080, #95079, #109255, #62745, #168932, #79914, #30438, #153774, #15269, #125430, #156767, #141586, #3074, #64750, #188109, #111244, #47601, #77918, #124425, #170934, #186121, #157762, #184126, #19252, #80899, #199295, #138598, #60762, #122434, #107261, #80, #61750, #123418, #185111, #46601, #108261, #97053, #112243, #160739, #101055, #82886, #98037, #177927, #22231, #145562, #81873, #144564, #51565, #6050, #83880, #4055, #37392, #162740, #84880, #127401, #7040, #67728, #36383, #52555, #65733, #20225, #23236, #129386, #53559, #116236, #39395, #175921, #189110, #128393, #158735, #24248, #190090, #115237, #142576, #99050, #146557, #176929, #54564, #50583, #173934, #114216, #35402, #143565, #5047, #191082, #161741, #68722, #66733, #130379, #113229, #174919, #159734, #21231, #192077, #38399, #100055, #8053, #69732, #131400, #193088, #12083, #103071, #40400, #86898, #71732, #133402, #57576, #163756, #195091, #165750, #198069, #73746, #74728, #104068, #167729, #102071, #119246, #25256, #105063, #181912, #196106, #135418, #178930, #88892, #58556, #85897, #194101, #147585, #132409, #148582, #106043, #118248, #27243, #134420, #42405, #70741, #10073, #56574, #121214, #150584, #197089, #55563, #120222, #117237, #11071, #9071, #13062, #179939, #43392, #166747, #41406, #28250, #164753, #89890, #151573, #136392, #59535, #182904, #44388, #26248, #180930, #87888, #149575, #72749, #48366, #79683, #124186, #77692, #49348, #200054, #62514, #153540, #122201, #139360, #61523, #111010, #32196, #30205, #14033, #183893, #125199, #33190, #93853, #18029, #137378, #140354, #15037, #155530, #169708, #107031, #45378, #75698, #78678, #168703, #91846, #156530, #17025, #141353, #63524, #108021, #47372, #185887, #1842, #186895, #110022, #29227, #199057, #90860, #60526, #76698, #152545, #123192, #109027, #841, #170706, #138374, #184881, #46363, #64518, #171701, #94849, #31201, #2840, #92852, #154538, #16034, #126185, #187881, #101571, #148095, #161253, #193605, #172696, #163261, #24763, #131921, #56075, #40914, #39905, #71252, #8578, #164271, #23752 ),
 ( #22747, #127162, #149097, #84396, #86410, #133926, #70253, #55077, #146072, #57088, #65501, #9586, #38914, #10587, #116747, #115756, #100571, #195616, #132916, #194603, #178437, #117756, #179448, #34181, #188870, #102587, #7557, #177444, #95842, #25766, #87412, #72248, #157526, #19020, #162253, #80666, #142342, #3822, #130909, #50353, #69243, #112012, #173701, #35169, #96824, #192599, #54082, #85402, #147094, #154045, #151091, #106545, #12582, #136890, #45873, #91350, #92359, #153042, #59053, #89402, #13552, #14542, #28746, #182419, #88398, #137881, #150092, #11595, #73263, #152067, #168221, #199562, #29718, #61031, #107526, #76202, #119750, #103589, #134932, #122703, #184393, #183405, #169203, #26758, #30710, #42911, #121712, #120720, #196609, #58080, #165264, #15540, #181433, #104577, #77198, #138867, #347, #118762, #197587, #198576, #75218, #44888, #180451, #41923, #166260, #27759, #74247, #90382, #135916, #43898, #105561, #167247, #60045, #65009, #185380, #48859, #124697, #171206, #186394, #17523, #156026, #96331, #140852, #79182, #31703, #65998, #46871, #188370, #2341, #16533, #63018, #47871, #109524, #33680, #139849, #32696, #141844, #174195, #49847, #50844, #80172, #143833, #78180, #95342, #1338, #81154, #158018, #172195, #111511, #155038, #126666, #34673, #62017, #170210, #123681, #108531, #94347, #82139, #64022, #3335, #110514, #18525, #93352, #125692, #187391, #97311, #173197, #19509, #157027, #142836, #4315, #127667, #189367, #112501, #35663, #158997, #20490, #191341, #23504, #5313, #193357, #131676, #162008, #86168, #71009, #70006, #101321, #38674, #194365, #53839, #9344, #24517, #55832, #100329, #115513, #25525, #176190, #85152, #129645, #98306, #177201, #37659, #87171, #8331, #147857, #102340, #160006, #146838, #54833, #83155, #40670, #99324, #116507, #161008, #178195, #132677, #39660, #179202, #163010, #145828, #22502, #117505, #164029, #66997, #68996, #175181, #128656, #36647, #21494, #144829, #190351, #51828, #113487, #6313, #67992, #52819, #114487, #84149, #7311, #130662, #192355, #181195, #151829, #133673, #182173, #119514, #44651, #180208, #43659, #137641, #71999, #106303, #41677, #105321, #14300, #30467, #75968, #103341, #118519, #167009, #107290, #89159, #104334, #184157, #28510, #13318, #88158, #150849, #57841, #12344, #90144, #10343, #74984, #168961, #91119, #195364, #136646, #74007, #42673, #58813, #56843, #26514, #29486, #135678, #59805, #122464, #45638, #198329, #165021, #134688, #149843, #148852, #196373, #121475, #11347, #183168, #167989, #166018, #73018, #27518, #152808, #197350, #120482, #199328, #60793, #155791, #112271, #126443, #64782, #171963, #172966, #110282, #153804, #108291, #188141, #62776, #94112, #173963, #111275, #49612, #34444, #156799, #125461, #32459, #33451, #95110, #142606, #47632, #138628, #186153, #141617, #79947, #4085, #76958, #92115, #63789, #109, #61779, #50612, #17288, #96103, #18292, #15298, #78942, #154799, #1100, #16297, #109287, #170965, #157792, #140618, #2108, #123447, #19282, #185140, #3104, #187158, #46631, #93114, #77947, #139614, #48630, #169969, #124457, #80929, #65763, #127432, #189139, #31462, #117264, #51592, #7072, #190117, #54588, #131428, #145593, #84909, #128421, #38429, #8082, #35430, #143594, #97083, #81901, #36410, #55589, #67756, #115267, #83910, #192108, #20255, #113257, #174949, #70766, #53591, #146588, #5077, #100085, #66760, #160771, #158765, #162764, #98065, #161770, #69758, #21259, #176960, #159764, #23265, #193114, #116261, #177952, #101079, #39420, #24274, #68753, #85923, #130410, #147611, #9099, #132434, #194126, #82914, #144592, #6078, #129414, #191112, #52586, #114245, #175952, #37421, #99081, #22261, #163782, #133430, #74753, #182931, #43419, #167754, #86926, #89915, #103098, #181937, #119271, #56601, #195118, #25283, #28276, #71760, #118275, #106068, #166775, #29252, #13088, #57602, #197113, #135444 ) ),
 .UNSPECIFIED., .T., .F., .F. ) 
 B_SPLINE_SURFACE_WITH_KNOTS ( ( 4, 3, 4 ),
 ( 3, 2, 2, 2, 2, 2, 2, 2, 2, 2, 2, 2, 2, 2, 2, 2, 2, 2, 2, 2, 2, 2, 2, 2, 2, 2, 2, 2, 2, 2, 2, 2, 2, 2, 2, 2, 2, 2, 2, 2, 2, 2, 2, 2, 2, 2, 2, 2, 2, 2, 2, 2, 2, 2, 2, 2, 2, 2, 2, 2, 2, 2, 2, 2, 2, 2, 2, 2, 2, 2, 2, 2, 2, 2, 2, 2, 2, 2, 2, 2, 2, 2, 2, 2, 2, 2, 2, 2, 2, 2, 2, 2, 2, 2, 2, 2, 2, 2, 2, 2, 2, 2, 2, 2, 2, 2, 2, 2, 2, 2, 2, 2, 2, 2, 2, 2, 2, 2, 2, 2, 2, 2, 2, 2, 2, 2, 2, 2, 2, 2, 2, 2, 2, 2, 2, 2, 2, 2, 2, 2, 2, 2, 2, 2, 2, 2, 2, 2, 2, 2, 2, 2, 2, 2, 2, 2, 2, 2, 2, 2, 2, 2, 2, 2, 2, 2, 2, 2, 2, 2, 2, 2, 2, 2, 2, 2, 2, 2, 2, 2, 2, 2, 2, 2, 2, 2, 2, 2, 2, 2, 2, 2, 2, 2, 2, 2, 2, 2, 2, 2, 2, 2, 2, 2, 2, 2, 2, 2, 2, 2, 2, 2, 2, 2, 2, 2, 2, 2, 2, 2, 2, 2, 2, 2, 2, 2, 2, 2, 3 ),
 ( 0.000000000000000000, 0.5000000000000000000, 1.000000000000000000 ),
 ( 0.000000000000000000, 0.004385964912280701511, 0.008771929824561403022, 0.01315789473684210453, 0.01754385964912280604, 0.02192982456140350755, 0.02631578947368420907, 0.03070175438596491058, 0.03508771929824561209, 0.03947368421052631360, 0.04385964912280701511, 0.04824561403508771662, 0.05263157894736841813, 0.05701754385964911964, 0.06140350877192982115, 0.06578947368421052266, 0.07017543859649122417, 0.07456140350877192569, 0.07894736842105262720, 0.08333333333333332871, 0.08771929824561403022, 0.09210526315789473173, 0.09649122807017543324, 0.1008771929824561348, 0.1052631578947368363, 0.1096491228070175378, 0.1140350877192982393, 0.1184210526315789408, 0.1228070175438596423, 0.1271929824561403577, 0.1315789473684210453, 0.1359649122807017607, 0.1403508771929824483, 0.1447368421052631637, 0.1491228070175438514, 0.1535087719298245668, 0.1578947368421052544, 0.1622807017543859698, 0.1666666666666666574, 0.1710526315789473728, 0.1754385964912280604, 0.1798245614035087758, 0.1842105263157894635, 0.1885964912280701788, 0.1929824561403508665, 0.1973684210526315819, 0.2017543859649122695, 0.2061403508771929849, 0.2105263157894736725, 0.2149122807017543879, 0.2192982456140350755, 0.2236842105263157909, 0.2280701754385964786, 0.2324561403508771940, 0.2368421052631578816, 0.2412280701754385970, 0.2456140350877192846, 0.2500000000000000000, 0.2543859649122807154, 0.2587719298245614308, 0.2631578947368420907, 0.2675438596491228060, 0.2719298245614035214, 0.2763157894736842368, 0.2807017543859648967, 0.2850877192982456121, 0.2894736842105263275, 0.2938596491228070429, 0.2982456140350877027, 0.3026315789473684181, 0.3070175438596491335, 0.3114035087719298489, 0.3157894736842105088, 0.3201754385964912242, 0.3245614035087719396, 0.3289473684210526550, 0.3333333333333333148, 0.3377192982456140302, 0.3421052631578947456, 0.3464912280701754610, 0.3508771929824561209, 0.3552631578947368363, 0.3596491228070175517, 0.3640350877192982670, 0.3684210526315789269, 0.3728070175438596423, 0.3771929824561403577, 0.3815789473684210731, 0.3859649122807017330, 0.3903508771929824483, 0.3947368421052631637, 0.3991228070175438791, 0.4035087719298245390, 0.4078947368421052544, 0.4122807017543859698, 0.4166666666666666852, 0.4210526315789473450, 0.4254385964912280604, 0.4298245614035087758, 0.4342105263157894912, 0.4385964912280701511, 0.4429824561403508665, 0.4473684210526315819, 0.4517543859649122973, 0.4561403508771929571, 0.4605263157894736725, 0.4649122807017543879, 0.4692982456140351033, 0.4736842105263157632, 0.4780701754385964786, 0.4824561403508771940, 0.4868421052631579093, 0.4912280701754385692, 0.4956140350877192846, 0.5000000000000000000, 0.5043859649122807154, 0.5087719298245614308, 0.5131578947368421462, 0.5175438596491228616, 0.5219298245614034659, 0.5263157894736841813, 0.5307017543859648967, 0.5350877192982456121, 0.5394736842105263275, 0.5438596491228070429, 0.5482456140350877583, 0.5526315789473684736, 0.5570175438596490780, 0.5614035087719297934, 0.5657894736842105088, 0.5701754385964912242, 0.5745614035087719396, 0.5789473684210526550, 0.5833333333333333703, 0.5877192982456140857, 0.5921052631578946901, 0.5964912280701754055, 0.6008771929824561209, 0.6052631578947368363, 0.6096491228070175517, 0.6140350877192982670, 0.6184210526315789824, 0.6228070175438596978, 0.6271929824561403022, 0.6315789473684210176, 0.6359649122807017330, 0.6403508771929824483, 0.6447368421052631637, 0.6491228070175438791, 0.6535087719298245945, 0.6578947368421053099, 0.6622807017543859143, 0.6666666666666666297, 0.6710526315789473450, 0.6754385964912280604, 0.6798245614035087758, 0.6842105263157894912, 0.6885964912280702066, 0.6929824561403509220, 0.6973684210526315264, 0.7017543859649122417, 0.7061403508771929571, 0.7105263157894736725, 0.7149122807017543879, 0.7192982456140351033, 0.7236842105263158187, 0.7280701754385965341, 0.7324561403508771384, 0.7368421052631578538, 0.7412280701754385692, 0.7456140350877192846, 0.7500000000000000000, 0.7543859649122807154, 0.7587719298245614308, 0.7631578947368421462, 0.7675438596491228616, 0.7719298245614034659, 0.7763157894736841813, 0.7807017543859648967, 0.7850877192982456121, 0.7894736842105263275, 0.7938596491228070429, 0.7982456140350877583, 0.8026315789473684736, 0.8070175438596490780, 0.8114035087719297934, 0.8157894736842105088, 0.8201754385964912242, 0.8245614035087719396, 0.8289473684210526550, 0.8333333333333333703, 0.8377192982456140857, 0.8421052631578946901, 0.8464912280701754055, 0.8508771929824561209, 0.8552631578947368363, 0.8596491228070175517, 0.8640350877192982670, 0.8684210526315789824, 0.8728070175438596978, 0.8771929824561403022, 0.8815789473684210176, 0.8859649122807017330, 0.8903508771929824483, 0.8947368421052631637, 0.8991228070175438791, 0.9035087719298245945, 0.9078947368421053099, 0.9122807017543859143, 0.9166666666666666297, 0.9210526315789473450, 0.9254385964912280604, 0.9298245614035087758, 0.9342105263157894912, 0.9385964912280702066, 0.9429824561403509220, 0.9473684210526315264, 0.9517543859649122417, 0.9561403508771929571, 0.9605263157894736725, 0.9649122807017543879, 0.9692982456140351033, 0.9736842105263158187, 0.9780701754385965341, 0.9824561403508771384, 0.9868421052631578538, 0.9912280701754385692, 0.9956140350877192846, 1.000000000000000000 ),
 .UNSPECIFIED. ) 
 GEOMETRIC_REPRESENTATION_ITEM ( )  RATIONAL_B_SPLINE_SURFACE ( (
 ( 1.000000000000000000, 0.9659258262890683122, 1.000000000000000000, 0.9659258262890683122, 1.000000000000000000, 0.9659258262890683122, 1.000000000000000000, 0.9659258262890683122, 1.000000000000000000, 0.9659258262890683122, 1.000000000000000000, 0.9659258262890683122, 1.000000000000000000, 0.9659258262890683122, 1.000000000000000000, 0.9659258262890683122, 1.000000000000000000, 0.9659258262890683122, 1.000000000000000000, 0.9659258262890683122, 1.000000000000000000, 0.9659258262890683122, 1.000000000000000000, 0.9659258262890683122, 1.000000000000000000, 0.9659258262890683122, 1.000000000000000000, 0.9659258262890683122, 1.000000000000000000, 0.9659258262890683122, 1.000000000000000000, 0.9659258262890683122, 1.000000000000000000, 0.9659258262890683122, 1.000000000000000000, 0.9659258262890683122, 1.000000000000000000, 0.9659258262890683122, 1.000000000000000000, 0.9659258262890683122, 1.000000000000000000, 0.9659258262890683122, 1.000000000000000000, 0.9659258262890683122, 1.000000000000000000, 0.9659258262890683122, 1.000000000000000000, 0.9659258262890683122, 1.000000000000000000, 0.9659258262890683122, 1.000000000000000000, 0.9659258262890683122, 1.000000000000000000, 0.9659258262890683122, 1.000000000000000000, 0.9659258262890683122, 1.000000000000000000, 0.9659258262890683122, 1.000000000000000000, 0.9659258262890683122, 1.000000000000000000, 0.9659258262890683122, 1.000000000000000000, 0.9659258262890683122, 1.000000000000000000, 0.9659258262890683122, 1.000000000000000000, 0.9659258262890683122, 1.000000000000000000, 0.9659258262890683122, 1.000000000000000000, 0.9659258262890683122, 1.000000000000000000, 0.9659258262890683122, 1.000000000000000000, 0.9659258262890683122, 1.000000000000000000, 0.9659258262890683122, 1.000000000000000000, 0.9659258262890683122, 1.000000000000000000, 0.9659258262890683122, 1.000000000000000000, 0.9659258262890683122, 1.000000000000000000, 0.9659258262890683122, 1.000000000000000000, 0.9659258262890683122, 1.000000000000000000, 0.9659258262890683122, 1.000000000000000000, 0.9659258262890683122, 1.000000000000000000, 0.9659258262890683122, 1.000000000000000000, 0.9659258262890683122, 1.000000000000000000, 0.9659258262890683122, 1.000000000000000000, 0.9659258262890683122, 1.000000000000000000, 0.9659258262890683122, 1.000000000000000000, 0.9659258262890683122, 1.000000000000000000, 0.9659258262890683122, 1.000000000000000000, 0.9659258262890683122, 1.000000000000000000, 0.9659258262890683122, 1.000000000000000000, 0.9659258262890683122, 1.000000000000000000, 0.9659258262890683122, 1.000000000000000000, 0.9659258262890683122, 1.000000000000000000, 0.9659258262890683122, 1.000000000000000000, 0.9659258262890683122, 1.000000000000000000, 0.9659258262890683122, 1.000000000000000000, 0.9659258262890683122, 1.000000000000000000, 0.9659258262890683122, 1.000000000000000000, 0.9659258262890683122, 1.000000000000000000, 0.9659258262890683122, 1.000000000000000000, 0.9659258262890683122, 1.000000000000000000, 0.9659258262890683122, 1.000000000000000000, 0.9659258262890683122, 1.000000000000000000, 0.9659258262890683122, 1.000000000000000000, 0.9659258262890683122, 1.000000000000000000, 0.9659258262890683122, 1.000000000000000000, 0.9659258262890683122, 1.000000000000000000, 0.9659258262890683122, 1.000000000000000000, 0.9659258262890683122, 1.000000000000000000, 0.9659258262890683122, 1.000000000000000000, 0.9659258262890683122, 1.000000000000000000, 0.9659258262890683122, 1.000000000000000000, 0.9659258262890683122, 1.000000000000000000, 0.9659258262890683122, 1.000000000000000000, 0.9659258262890683122, 1.000000000000000000, 0.9659258262890683122, 1.000000000000000000, 0.9659258262890683122, 1.000000000000000000, 0.9659258262890683122, 1.000000000000000000, 0.9659258262890683122, 1.000000000000000000, 0.9659258262890683122, 1.000000000000000000, 0.9659258262890683122, 1.000000000000000000, 0.9659258262890683122, 1.000000000000000000, 0.9659258262890683122, 1.000000000000000000, 0.9659258262890683122, 1.000000000000000000, 0.9659258262890683122, 1.000000000000000000, 0.9659258262890683122, 1.000000000000000000, 0.9659258262890683122, 1.000000000000000000, 0.9659258262890683122, 1.000000000000000000, 0.9659258262890683122, 1.000000000000000000, 0.9659258262890683122, 1.000000000000000000, 0.9659258262890683122, 1.000000000000000000, 0.9659258262890683122, 1.000000000000000000, 0.9659258262890683122, 1.000000000000000000, 0.9659258262890683122, 1.000000000000000000, 0.9659258262890683122, 1.000000000000000000, 0.9659258262890683122, 1.000000000000000000, 0.9659258262890683122, 1.000000000000000000, 0.9659258262890683122, 1.000000000000000000, 0.9659258262890683122, 1.000000000000000000, 0.9659258262890683122, 1.000000000000000000, 0.9659258262890683122, 1.000000000000000000, 0.9659258262890683122, 1.000000000000000000, 0.9659258262890683122, 1.000000000000000000, 0.9659258262890683122, 1.000000000000000000, 0.9659258262890683122, 1.000000000000000000, 0.9659258262890683122, 1.000000000000000000, 0.9659258262890683122, 1.000000000000000000, 0.9659258262890683122, 1.000000000000000000, 0.9659258262890683122, 1.000000000000000000, 0.9659258262890683122, 1.000000000000000000, 0.9659258262890683122, 1.000000000000000000, 0.9659258262890683122, 1.000000000000000000, 0.9659258262890683122, 1.000000000000000000, 0.9659258262890683122, 1.000000000000000000, 0.9659258262890683122, 1.000000000000000000, 0.9659258262890683122, 1.000000000000000000, 0.9659258262890683122, 1.000000000000000000, 0.9659258262890683122, 1.000000000000000000, 0.9659258262890683122, 1.000000000000000000, 0.9659258262890683122, 1.000000000000000000, 0.9659258262890683122, 1.000000000000000000, 0.9659258262890683122, 1.000000000000000000, 0.9659258262890683122, 1.000000000000000000, 0.9659258262890683122, 1.000000000000000000, 0.9659258262890683122, 1.000000000000000000, 0.9659258262890683122, 1.000000000000000000, 0.9659258262890683122, 1.000000000000000000, 0.9659258262890683122, 1.000000000000000000, 0.9659258262890683122, 1.000000000000000000, 0.9659258262890683122, 1.000000000000000000, 0.9659258262890683122, 1.000000000000000000, 0.9659258262890683122, 1.000000000000000000, 0.9659258262890683122, 1.000000000000000000, 0.9659258262890683122, 1.000000000000000000, 0.9659258262890683122, 1.000000000000000000, 0.9659258262890683122, 1.000000000000000000, 0.9659258262890683122, 1.000000000000000000, 0.9659258262890683122, 1.000000000000000000, 0.9659258262890683122, 1.000000000000000000, 0.9659258262890683122, 1.000000000000000000, 0.9659258262890683122, 1.000000000000000000, 0.9659258262890683122, 1.000000000000000000, 0.9659258262890683122, 1.000000000000000000, 0.9659258262890683122, 1.000000000000000000, 0.9659258262890683122, 1.000000000000000000, 0.9659258262890683122, 1.000000000000000000, 0.9659258262890683122, 1.000000000000000000, 0.9659258262890683122, 1.000000000000000000, 0.9659258262890683122, 1.000000000000000000, 0.9659258262890683122, 1.000000000000000000, 0.9659258262890683122, 1.000000000000000000, 0.9659258262890683122, 1.000000000000000000, 0.9659258262890683122, 1.000000000000000000, 0.9659258262890683122, 1.000000000000000000, 0.9659258262890683122, 1.000000000000000000, 0.9659258262890683122, 1.000000000000000000, 0.9659258262890683122, 1.000000000000000000, 0.9659258262890683122, 1.000000000000000000, 0.9659258262890683122, 1.000000000000000000, 0.9659258262890683122, 1.000000000000000000, 0.9659258262890683122, 1.000000000000000000, 0.9659258262890683122, 1.000000000000000000, 0.9659258262890683122, 1.000000000000000000, 0.9659258262890683122, 1.000000000000000000, 0.9659258262890683122, 1.000000000000000000, 0.9659258262890683122, 1.000000000000000000, 0.9659258262890683122, 1.000000000000000000, 0.9659258262890683122, 1.000000000000000000, 0.9659258262890683122, 1.000000000000000000, 0.9659258262890683122, 1.000000000000000000, 0.9659258262890683122, 1.000000000000000000, 0.9659258262890683122, 1.000000000000000000, 0.9659258262890683122, 1.000000000000000000, 0.9659258262890683122, 1.000000000000000000, 0.9659258262890683122, 1.000000000000000000, 0.9659258262890683122, 1.000000000000000000, 0.9659258262890683122, 1.000000000000000000, 0.9659258262890683122, 1.000000000000000000, 0.9659258262890683122, 1.000000000000000000, 0.9659258262890683122, 1.000000000000000000, 0.9659258262890683122, 1.000000000000000000, 0.9659258262890683122, 1.000000000000000000, 0.9659258262890683122, 1.000000000000000000, 0.9659258262890683122, 1.000000000000000000, 0.9659258262890683122, 1.000000000000000000, 0.9659258262890683122, 1.000000000000000000, 0.9659258262890683122, 1.000000000000000000, 0.9659258262890683122, 1.000000000000000000, 0.9659258262890683122, 1.000000000000000000, 0.9659258262890683122, 1.000000000000000000, 0.9659258262890683122, 1.000000000000000000, 0.9659258262890683122, 1.000000000000000000, 0.9659258262890683122, 1.000000000000000000, 0.9659258262890683122, 1.000000000000000000, 0.9659258262890683122, 1.000000000000000000, 0.9659258262890683122, 1.000000000000000000, 0.9659258262890683122, 1.000000000000000000, 0.9659258262890683122, 1.000000000000000000, 0.9659258262890683122, 1.000000000000000000, 0.9659258262890683122, 1.000000000000000000, 0.9659258262890683122, 1.000000000000000000, 0.9659258262890683122, 1.000000000000000000, 0.9659258262890683122, 1.000000000000000000, 0.9659258262890683122, 1.000000000000000000, 0.9659258262890683122, 1.000000000000000000, 0.9659258262890683122, 1.000000000000000000, 0.9659258262890683122, 1.000000000000000000, 0.9659258262890683122, 1.000000000000000000, 0.9659258262890683122, 1.000000000000000000, 0.9659258262890683122, 1.000000000000000000, 0.9659258262890683122, 1.000000000000000000, 0.9659258262890683122, 1.000000000000000000, 0.9659258262890683122, 1.000000000000000000, 0.9659258262890683122, 1.000000000000000000, 0.9659258262890683122, 1.000000000000000000, 0.9659258262890683122, 1.000000000000000000, 0.9659258262890683122, 1.000000000000000000, 0.9659258262890683122, 1.000000000000000000, 0.9659258262890683122, 1.000000000000000000, 0.9659258262890683122, 1.000000000000000000, 0.9659258262890683122, 1.000000000000000000, 0.9659258262890683122, 1.000000000000000000, 0.9659258262890683122, 1.000000000000000000),
 ( 0.3333333333333333703, 0.3219752754296894559, 0.3333333333333333703, 0.3219752754296894559, 0.3333333333333333703, 0.3219752754296894559, 0.3333333333333333703, 0.3219752754296894559, 0.3333333333333333703, 0.3219752754296894559, 0.3333333333333333703, 0.3219752754296894559, 0.3333333333333333703, 0.3219752754296894559, 0.3333333333333333703, 0.3219752754296894559, 0.3333333333333333703, 0.3219752754296894559, 0.3333333333333333703, 0.3219752754296894559, 0.3333333333333333703, 0.3219752754296894559, 0.3333333333333333703, 0.3219752754296894559, 0.3333333333333333703, 0.3219752754296894559, 0.3333333333333333703, 0.3219752754296894559, 0.3333333333333333703, 0.3219752754296894559, 0.3333333333333333703, 0.3219752754296894559, 0.3333333333333333703, 0.3219752754296894559, 0.3333333333333333703, 0.3219752754296894559, 0.3333333333333333703, 0.3219752754296894559, 0.3333333333333333703, 0.3219752754296894559, 0.3333333333333333703, 0.3219752754296894559, 0.3333333333333333703, 0.3219752754296894559, 0.3333333333333333703, 0.3219752754296894559, 0.3333333333333333703, 0.3219752754296894559, 0.3333333333333333703, 0.3219752754296894559, 0.3333333333333333703, 0.3219752754296894559, 0.3333333333333333703, 0.3219752754296894559, 0.3333333333333333703, 0.3219752754296894559, 0.3333333333333333703, 0.3219752754296894559, 0.3333333333333333703, 0.3219752754296894559, 0.3333333333333333703, 0.3219752754296894559, 0.3333333333333333703, 0.3219752754296894559, 0.3333333333333333703, 0.3219752754296894559, 0.3333333333333333703, 0.3219752754296894559, 0.3333333333333333703, 0.3219752754296894559, 0.3333333333333333703, 0.3219752754296894559, 0.3333333333333333703, 0.3219752754296894559, 0.3333333333333333703, 0.3219752754296894559, 0.3333333333333333703, 0.3219752754296894559, 0.3333333333333333703, 0.3219752754296894559, 0.3333333333333333703, 0.3219752754296894559, 0.3333333333333333703, 0.3219752754296894559, 0.3333333333333333703, 0.3219752754296894559, 0.3333333333333333703, 0.3219752754296894559, 0.3333333333333333703, 0.3219752754296894559, 0.3333333333333333703, 0.3219752754296894559, 0.3333333333333333703, 0.3219752754296894559, 0.3333333333333333703, 0.3219752754296894559, 0.3333333333333333703, 0.3219752754296894559, 0.3333333333333333703, 0.3219752754296894559, 0.3333333333333333703, 0.3219752754296894559, 0.3333333333333333703, 0.3219752754296894559, 0.3333333333333333703, 0.3219752754296894559, 0.3333333333333333703, 0.3219752754296894559, 0.3333333333333333703, 0.3219752754296894559, 0.3333333333333333703, 0.3219752754296894559, 0.3333333333333333703, 0.3219752754296894559, 0.3333333333333333703, 0.3219752754296894559, 0.3333333333333333703, 0.3219752754296894559, 0.3333333333333333703, 0.3219752754296894559, 0.3333333333333333703, 0.3219752754296894559, 0.3333333333333333703, 0.3219752754296894559, 0.3333333333333333703, 0.3219752754296894559, 0.3333333333333333703, 0.3219752754296894559, 0.3333333333333333703, 0.3219752754296894559, 0.3333333333333333703, 0.3219752754296894559, 0.3333333333333333703, 0.3219752754296894559, 0.3333333333333333703, 0.3219752754296894559, 0.3333333333333333703, 0.3219752754296894559, 0.3333333333333333703, 0.3219752754296894559, 0.3333333333333333703, 0.3219752754296894559, 0.3333333333333333703, 0.3219752754296894559, 0.3333333333333333703, 0.3219752754296894559, 0.3333333333333333703, 0.3219752754296894559, 0.3333333333333333703, 0.3219752754296894559, 0.3333333333333333703, 0.3219752754296894559, 0.3333333333333333703, 0.3219752754296894559, 0.3333333333333333703, 0.3219752754296894559, 0.3333333333333333703, 0.3219752754296894559, 0.3333333333333333703, 0.3219752754296894559, 0.3333333333333333703, 0.3219752754296894559, 0.3333333333333333703, 0.3219752754296894559, 0.3333333333333333703, 0.3219752754296894559, 0.3333333333333333703, 0.3219752754296894559, 0.3333333333333333703, 0.3219752754296894559, 0.3333333333333333703, 0.3219752754296894559, 0.3333333333333333703, 0.3219752754296894559, 0.3333333333333333703, 0.3219752754296894559, 0.3333333333333333703, 0.3219752754296894559, 0.3333333333333333703, 0.3219752754296894559, 0.3333333333333333703, 0.3219752754296894559, 0.3333333333333333703, 0.3219752754296894559, 0.3333333333333333703, 0.3219752754296894559, 0.3333333333333333703, 0.3219752754296894559, 0.3333333333333333703, 0.3219752754296894559, 0.3333333333333333703, 0.3219752754296894559, 0.3333333333333333703, 0.3219752754296894559, 0.3333333333333333703, 0.3219752754296894559, 0.3333333333333333703, 0.3219752754296894559, 0.3333333333333333703, 0.3219752754296894559, 0.3333333333333333703, 0.3219752754296894559, 0.3333333333333333703, 0.3219752754296894559, 0.3333333333333333703, 0.3219752754296894559, 0.3333333333333333703, 0.3219752754296894559, 0.3333333333333333703, 0.3219752754296894559, 0.3333333333333333703, 0.3219752754296894559, 0.3333333333333333703, 0.3219752754296894559, 0.3333333333333333703, 0.3219752754296894559, 0.3333333333333333703, 0.3219752754296894559, 0.3333333333333333703, 0.3219752754296894559, 0.3333333333333333703, 0.3219752754296894559, 0.3333333333333333703, 0.3219752754296894559, 0.3333333333333333703, 0.3219752754296894559, 0.3333333333333333703, 0.3219752754296894559, 0.3333333333333333703, 0.3219752754296894559, 0.3333333333333333703, 0.3219752754296894559, 0.3333333333333333703, 0.3219752754296894559, 0.3333333333333333703, 0.3219752754296894559, 0.3333333333333333703, 0.3219752754296894559, 0.3333333333333333703, 0.3219752754296894559, 0.3333333333333333703, 0.3219752754296894559, 0.3333333333333333703, 0.3219752754296894559, 0.3333333333333333703, 0.3219752754296894559, 0.3333333333333333703, 0.3219752754296894559, 0.3333333333333333703, 0.3219752754296894559, 0.3333333333333333703, 0.3219752754296894559, 0.3333333333333333703, 0.3219752754296894559, 0.3333333333333333703, 0.3219752754296894559, 0.3333333333333333703, 0.3219752754296894559, 0.3333333333333333703, 0.3219752754296894559, 0.3333333333333333703, 0.3219752754296894559, 0.3333333333333333703, 0.3219752754296894559, 0.3333333333333333703, 0.3219752754296894559, 0.3333333333333333703, 0.3219752754296894559, 0.3333333333333333703, 0.3219752754296894559, 0.3333333333333333703, 0.3219752754296894559, 0.3333333333333333703, 0.3219752754296894559, 0.3333333333333333703, 0.3219752754296894559, 0.3333333333333333703, 0.3219752754296894559, 0.3333333333333333703, 0.3219752754296894559, 0.3333333333333333703, 0.3219752754296894559, 0.3333333333333333703, 0.3219752754296894559, 0.3333333333333333703, 0.3219752754296894559, 0.3333333333333333703, 0.3219752754296894559, 0.3333333333333333703, 0.3219752754296894559, 0.3333333333333333703, 0.3219752754296894559, 0.3333333333333333703, 0.3219752754296894559, 0.3333333333333333703, 0.3219752754296894559, 0.3333333333333333703, 0.3219752754296894559, 0.3333333333333333703, 0.3219752754296894559, 0.3333333333333333703, 0.3219752754296894559, 0.3333333333333333703, 0.3219752754296894559, 0.3333333333333333703, 0.3219752754296894559, 0.3333333333333333703, 0.3219752754296894559, 0.3333333333333333703, 0.3219752754296894559, 0.3333333333333333703, 0.3219752754296894559, 0.3333333333333333703, 0.3219752754296894559, 0.3333333333333333703, 0.3219752754296894559, 0.3333333333333333703, 0.3219752754296894559, 0.3333333333333333703, 0.3219752754296894559, 0.3333333333333333703, 0.3219752754296894559, 0.3333333333333333703, 0.3219752754296894559, 0.3333333333333333703, 0.3219752754296894559, 0.3333333333333333703, 0.3219752754296894559, 0.3333333333333333703, 0.3219752754296894559, 0.3333333333333333703, 0.3219752754296894559, 0.3333333333333333703, 0.3219752754296894559, 0.3333333333333333703, 0.3219752754296894559, 0.3333333333333333703, 0.3219752754296894559, 0.3333333333333333703, 0.3219752754296894559, 0.3333333333333333703, 0.3219752754296894559, 0.3333333333333333703, 0.3219752754296894559, 0.3333333333333333703, 0.3219752754296894559, 0.3333333333333333703, 0.3219752754296894559, 0.3333333333333333703, 0.3219752754296894559, 0.3333333333333333703, 0.3219752754296894559, 0.3333333333333333703, 0.3219752754296894559, 0.3333333333333333703, 0.3219752754296894559, 0.3333333333333333703, 0.3219752754296894559, 0.3333333333333333703, 0.3219752754296894559, 0.3333333333333333703, 0.3219752754296894559, 0.3333333333333333703, 0.3219752754296894559, 0.3333333333333333703, 0.3219752754296894559, 0.3333333333333333703, 0.3219752754296894559, 0.3333333333333333703, 0.3219752754296894559, 0.3333333333333333703, 0.3219752754296894559, 0.3333333333333333703, 0.3219752754296894559, 0.3333333333333333703, 0.3219752754296894559, 0.3333333333333333703, 0.3219752754296894559, 0.3333333333333333703, 0.3219752754296894559, 0.3333333333333333703, 0.3219752754296894559, 0.3333333333333333703, 0.3219752754296894559, 0.3333333333333333703, 0.3219752754296894559, 0.3333333333333333703, 0.3219752754296894559, 0.3333333333333333703, 0.3219752754296894559, 0.3333333333333333703, 0.3219752754296894559, 0.3333333333333333703, 0.3219752754296894559, 0.3333333333333333703, 0.3219752754296894559, 0.3333333333333333703, 0.3219752754296894559, 0.3333333333333333703, 0.3219752754296894559, 0.3333333333333333703, 0.3219752754296894559, 0.3333333333333333703, 0.3219752754296894559, 0.3333333333333333703, 0.3219752754296894559, 0.3333333333333333703, 0.3219752754296894559, 0.3333333333333333703, 0.3219752754296894559, 0.3333333333333333703, 0.3219752754296894559, 0.3333333333333333703, 0.3219752754296894559, 0.3333333333333333703, 0.3219752754296894559, 0.3333333333333333703, 0.3219752754296894559, 0.3333333333333333703, 0.3219752754296894559, 0.3333333333333333703, 0.3219752754296894559, 0.3333333333333333703, 0.3219752754296894559, 0.3333333333333333703, 0.3219752754296894559, 0.3333333333333333703, 0.3219752754296894559, 0.3333333333333333703, 0.3219752754296894559, 0.3333333333333333703, 0.3219752754296894559, 0.3333333333333333703, 0.3219752754296894559, 0.3333333333333333703, 0.3219752754296894559, 0.3333333333333333703, 0.3219752754296894559, 0.3333333333333333703, 0.3219752754296894559, 0.3333333333333333703, 0.3219752754296894559, 0.3333333333333333703, 0.3219752754296894559, 0.3333333333333333703, 0.3219752754296894559, 0.3333333333333333703, 0.3219752754296894559, 0.3333333333333333703, 0.3219752754296894559, 0.3333333333333333703, 0.3219752754296894559, 0.3333333333333333703, 0.3219752754296894559, 0.3333333333333333703, 0.3219752754296894559, 0.3333333333333333703),
 ( 0.3333333333333333703, 0.3219752754296894559, 0.3333333333333333703, 0.3219752754296894559, 0.3333333333333333703, 0.3219752754296894559, 0.3333333333333333703, 0.3219752754296894559, 0.3333333333333333703, 0.3219752754296894559, 0.3333333333333333703, 0.3219752754296894559, 0.3333333333333333703, 0.3219752754296894559, 0.3333333333333333703, 0.3219752754296894559, 0.3333333333333333703, 0.3219752754296894559, 0.3333333333333333703, 0.3219752754296894559, 0.3333333333333333703, 0.3219752754296894559, 0.3333333333333333703, 0.3219752754296894559, 0.3333333333333333703, 0.3219752754296894559, 0.3333333333333333703, 0.3219752754296894559, 0.3333333333333333703, 0.3219752754296894559, 0.3333333333333333703, 0.3219752754296894559, 0.3333333333333333703, 0.3219752754296894559, 0.3333333333333333703, 0.3219752754296894559, 0.3333333333333333703, 0.3219752754296894559, 0.3333333333333333703, 0.3219752754296894559, 0.3333333333333333703, 0.3219752754296894559, 0.3333333333333333703, 0.3219752754296894559, 0.3333333333333333703, 0.3219752754296894559, 0.3333333333333333703, 0.3219752754296894559, 0.3333333333333333703, 0.3219752754296894559, 0.3333333333333333703, 0.3219752754296894559, 0.3333333333333333703, 0.3219752754296894559, 0.3333333333333333703, 0.3219752754296894559, 0.3333333333333333703, 0.3219752754296894559, 0.3333333333333333703, 0.3219752754296894559, 0.3333333333333333703, 0.3219752754296894559, 0.3333333333333333703, 0.3219752754296894559, 0.3333333333333333703, 0.3219752754296894559, 0.3333333333333333703, 0.3219752754296894559, 0.3333333333333333703, 0.3219752754296894559, 0.3333333333333333703, 0.3219752754296894559, 0.3333333333333333703, 0.3219752754296894559, 0.3333333333333333703, 0.3219752754296894559, 0.3333333333333333703, 0.3219752754296894559, 0.3333333333333333703, 0.3219752754296894559, 0.3333333333333333703, 0.3219752754296894559, 0.3333333333333333703, 0.3219752754296894559, 0.3333333333333333703, 0.3219752754296894559, 0.3333333333333333703, 0.3219752754296894559, 0.3333333333333333703, 0.3219752754296894559, 0.3333333333333333703, 0.3219752754296894559, 0.3333333333333333703, 0.3219752754296894559, 0.3333333333333333703, 0.3219752754296894559, 0.3333333333333333703, 0.3219752754296894559, 0.3333333333333333703, 0.3219752754296894559, 0.3333333333333333703, 0.3219752754296894559, 0.3333333333333333703, 0.3219752754296894559, 0.3333333333333333703, 0.3219752754296894559, 0.3333333333333333703, 0.3219752754296894559, 0.3333333333333333703, 0.3219752754296894559, 0.3333333333333333703, 0.3219752754296894559, 0.3333333333333333703, 0.3219752754296894559, 0.3333333333333333703, 0.3219752754296894559, 0.3333333333333333703, 0.3219752754296894559, 0.3333333333333333703, 0.3219752754296894559, 0.3333333333333333703, 0.3219752754296894559, 0.3333333333333333703, 0.3219752754296894559, 0.3333333333333333703, 0.3219752754296894559, 0.3333333333333333703, 0.3219752754296894559, 0.3333333333333333703, 0.3219752754296894559, 0.3333333333333333703, 0.3219752754296894559, 0.3333333333333333703, 0.3219752754296894559, 0.3333333333333333703, 0.3219752754296894559, 0.3333333333333333703, 0.3219752754296894559, 0.3333333333333333703, 0.3219752754296894559, 0.3333333333333333703, 0.3219752754296894559, 0.3333333333333333703, 0.3219752754296894559, 0.3333333333333333703, 0.3219752754296894559, 0.3333333333333333703, 0.3219752754296894559, 0.3333333333333333703, 0.3219752754296894559, 0.3333333333333333703, 0.3219752754296894559, 0.3333333333333333703, 0.3219752754296894559, 0.3333333333333333703, 0.3219752754296894559, 0.3333333333333333703, 0.3219752754296894559, 0.3333333333333333703, 0.3219752754296894559, 0.3333333333333333703, 0.3219752754296894559, 0.3333333333333333703, 0.3219752754296894559, 0.3333333333333333703, 0.3219752754296894559, 0.3333333333333333703, 0.3219752754296894559, 0.3333333333333333703, 0.3219752754296894559, 0.3333333333333333703, 0.3219752754296894559, 0.3333333333333333703, 0.3219752754296894559, 0.3333333333333333703, 0.3219752754296894559, 0.3333333333333333703, 0.3219752754296894559, 0.3333333333333333703, 0.3219752754296894559, 0.3333333333333333703, 0.3219752754296894559, 0.3333333333333333703, 0.3219752754296894559, 0.3333333333333333703, 0.3219752754296894559, 0.3333333333333333703, 0.3219752754296894559, 0.3333333333333333703, 0.3219752754296894559, 0.3333333333333333703, 0.3219752754296894559, 0.3333333333333333703, 0.3219752754296894559, 0.3333333333333333703, 0.3219752754296894559, 0.3333333333333333703, 0.3219752754296894559, 0.3333333333333333703, 0.3219752754296894559, 0.3333333333333333703, 0.3219752754296894559, 0.3333333333333333703, 0.3219752754296894559, 0.3333333333333333703, 0.3219752754296894559, 0.3333333333333333703, 0.3219752754296894559, 0.3333333333333333703, 0.3219752754296894559, 0.3333333333333333703, 0.3219752754296894559, 0.3333333333333333703, 0.3219752754296894559, 0.3333333333333333703, 0.3219752754296894559, 0.3333333333333333703, 0.3219752754296894559, 0.3333333333333333703, 0.3219752754296894559, 0.3333333333333333703, 0.3219752754296894559, 0.3333333333333333703, 0.3219752754296894559, 0.3333333333333333703, 0.3219752754296894559, 0.3333333333333333703, 0.3219752754296894559, 0.3333333333333333703, 0.3219752754296894559, 0.3333333333333333703, 0.3219752754296894559, 0.3333333333333333703, 0.3219752754296894559, 0.3333333333333333703, 0.3219752754296894559, 0.3333333333333333703, 0.3219752754296894559, 0.3333333333333333703, 0.3219752754296894559, 0.3333333333333333703, 0.3219752754296894559, 0.3333333333333333703, 0.3219752754296894559, 0.3333333333333333703, 0.3219752754296894559, 0.3333333333333333703, 0.3219752754296894559, 0.3333333333333333703, 0.3219752754296894559, 0.3333333333333333703, 0.3219752754296894559, 0.3333333333333333703, 0.3219752754296894559, 0.3333333333333333703, 0.3219752754296894559, 0.3333333333333333703, 0.3219752754296894559, 0.3333333333333333703, 0.3219752754296894559, 0.3333333333333333703, 0.3219752754296894559, 0.3333333333333333703, 0.3219752754296894559, 0.3333333333333333703, 0.3219752754296894559, 0.3333333333333333703, 0.3219752754296894559, 0.3333333333333333703, 0.3219752754296894559, 0.3333333333333333703, 0.3219752754296894559, 0.3333333333333333703, 0.3219752754296894559, 0.3333333333333333703, 0.3219752754296894559, 0.3333333333333333703, 0.3219752754296894559, 0.3333333333333333703, 0.3219752754296894559, 0.3333333333333333703, 0.3219752754296894559, 0.3333333333333333703, 0.3219752754296894559, 0.3333333333333333703, 0.3219752754296894559, 0.3333333333333333703, 0.3219752754296894559, 0.3333333333333333703, 0.3219752754296894559, 0.3333333333333333703, 0.3219752754296894559, 0.3333333333333333703, 0.3219752754296894559, 0.3333333333333333703, 0.3219752754296894559, 0.3333333333333333703, 0.3219752754296894559, 0.3333333333333333703, 0.3219752754296894559, 0.3333333333333333703, 0.3219752754296894559, 0.3333333333333333703, 0.3219752754296894559, 0.3333333333333333703, 0.3219752754296894559, 0.3333333333333333703, 0.3219752754296894559, 0.3333333333333333703, 0.3219752754296894559, 0.3333333333333333703, 0.3219752754296894559, 0.3333333333333333703, 0.3219752754296894559, 0.3333333333333333703, 0.3219752754296894559, 0.3333333333333333703, 0.3219752754296894559, 0.3333333333333333703, 0.3219752754296894559, 0.3333333333333333703, 0.3219752754296894559, 0.3333333333333333703, 0.3219752754296894559, 0.3333333333333333703, 0.3219752754296894559, 0.3333333333333333703, 0.3219752754296894559, 0.3333333333333333703, 0.3219752754296894559, 0.3333333333333333703, 0.3219752754296894559, 0.3333333333333333703, 0.3219752754296894559, 0.3333333333333333703, 0.3219752754296894559, 0.3333333333333333703, 0.3219752754296894559, 0.3333333333333333703, 0.3219752754296894559, 0.3333333333333333703, 0.3219752754296894559, 0.3333333333333333703, 0.3219752754296894559, 0.3333333333333333703, 0.3219752754296894559, 0.3333333333333333703, 0.3219752754296894559, 0.3333333333333333703, 0.3219752754296894559, 0.3333333333333333703, 0.3219752754296894559, 0.3333333333333333703, 0.3219752754296894559, 0.3333333333333333703, 0.3219752754296894559, 0.3333333333333333703, 0.3219752754296894559, 0.3333333333333333703, 0.3219752754296894559, 0.3333333333333333703, 0.3219752754296894559, 0.3333333333333333703, 0.3219752754296894559, 0.3333333333333333703, 0.3219752754296894559, 0.3333333333333333703, 0.3219752754296894559, 0.3333333333333333703, 0.3219752754296894559, 0.3333333333333333703, 0.3219752754296894559, 0.3333333333333333703, 0.3219752754296894559, 0.3333333333333333703, 0.3219752754296894559, 0.3333333333333333703, 0.3219752754296894559, 0.3333333333333333703, 0.3219752754296894559, 0.3333333333333333703, 0.3219752754296894559, 0.3333333333333333703, 0.3219752754296894559, 0.3333333333333333703, 0.3219752754296894559, 0.3333333333333333703, 0.3219752754296894559, 0.3333333333333333703, 0.3219752754296894559, 0.3333333333333333703, 0.3219752754296894559, 0.3333333333333333703, 0.3219752754296894559, 0.3333333333333333703, 0.3219752754296894559, 0.3333333333333333703, 0.3219752754296894559, 0.3333333333333333703, 0.3219752754296894559, 0.3333333333333333703, 0.3219752754296894559, 0.3333333333333333703, 0.3219752754296894559, 0.3333333333333333703, 0.3219752754296894559, 0.3333333333333333703, 0.3219752754296894559, 0.3333333333333333703, 0.3219752754296894559, 0.3333333333333333703, 0.3219752754296894559, 0.3333333333333333703, 0.3219752754296894559, 0.3333333333333333703, 0.3219752754296894559, 0.3333333333333333703, 0.3219752754296894559, 0.3333333333333333703, 0.3219752754296894559, 0.3333333333333333703, 0.3219752754296894559, 0.3333333333333333703, 0.3219752754296894559, 0.3333333333333333703, 0.3219752754296894559, 0.3333333333333333703, 0.3219752754296894559, 0.3333333333333333703, 0.3219752754296894559, 0.3333333333333333703, 0.3219752754296894559, 0.3333333333333333703, 0.3219752754296894559, 0.3333333333333333703, 0.3219752754296894559, 0.3333333333333333703, 0.3219752754296894559, 0.3333333333333333703, 0.3219752754296894559, 0.3333333333333333703, 0.3219752754296894559, 0.3333333333333333703, 0.3219752754296894559, 0.3333333333333333703, 0.3219752754296894559, 0.3333333333333333703, 0.3219752754296894559, 0.3333333333333333703, 0.3219752754296894559, 0.3333333333333333703, 0.3219752754296894559, 0.3333333333333333703, 0.3219752754296894559, 0.3333333333333333703, 0.3219752754296894559, 0.3333333333333333703),
 ( 1.000000000000000000, 0.9659258262890683122, 1.000000000000000000, 0.9659258262890683122, 1.000000000000000000, 0.9659258262890683122, 1.000000000000000000, 0.9659258262890683122, 1.000000000000000000, 0.9659258262890683122, 1.000000000000000000, 0.9659258262890683122, 1.000000000000000000, 0.9659258262890683122, 1.000000000000000000, 0.9659258262890683122, 1.000000000000000000, 0.9659258262890683122, 1.000000000000000000, 0.9659258262890683122, 1.000000000000000000, 0.9659258262890683122, 1.000000000000000000, 0.9659258262890683122, 1.000000000000000000, 0.9659258262890683122, 1.000000000000000000, 0.9659258262890683122, 1.000000000000000000, 0.9659258262890683122, 1.000000000000000000, 0.9659258262890683122, 1.000000000000000000, 0.9659258262890683122, 1.000000000000000000, 0.9659258262890683122, 1.000000000000000000, 0.9659258262890683122, 1.000000000000000000, 0.9659258262890683122, 1.000000000000000000, 0.9659258262890683122, 1.000000000000000000, 0.9659258262890683122, 1.000000000000000000, 0.9659258262890683122, 1.000000000000000000, 0.9659258262890683122, 1.000000000000000000, 0.9659258262890683122, 1.000000000000000000, 0.9659258262890683122, 1.000000000000000000, 0.9659258262890683122, 1.000000000000000000, 0.9659258262890683122, 1.000000000000000000, 0.9659258262890683122, 1.000000000000000000, 0.9659258262890683122, 1.000000000000000000, 0.9659258262890683122, 1.000000000000000000, 0.9659258262890683122, 1.000000000000000000, 0.9659258262890683122, 1.000000000000000000, 0.9659258262890683122, 1.000000000000000000, 0.9659258262890683122, 1.000000000000000000, 0.9659258262890683122, 1.000000000000000000, 0.9659258262890683122, 1.000000000000000000, 0.9659258262890683122, 1.000000000000000000, 0.9659258262890683122, 1.000000000000000000, 0.9659258262890683122, 1.000000000000000000, 0.9659258262890683122, 1.000000000000000000, 0.9659258262890683122, 1.000000000000000000, 0.9659258262890683122, 1.000000000000000000, 0.9659258262890683122, 1.000000000000000000, 0.9659258262890683122, 1.000000000000000000, 0.9659258262890683122, 1.000000000000000000, 0.9659258262890683122, 1.000000000000000000, 0.9659258262890683122, 1.000000000000000000, 0.9659258262890683122, 1.000000000000000000, 0.9659258262890683122, 1.000000000000000000, 0.9659258262890683122, 1.000000000000000000, 0.9659258262890683122, 1.000000000000000000, 0.9659258262890683122, 1.000000000000000000, 0.9659258262890683122, 1.000000000000000000, 0.9659258262890683122, 1.000000000000000000, 0.9659258262890683122, 1.000000000000000000, 0.9659258262890683122, 1.000000000000000000, 0.9659258262890683122, 1.000000000000000000, 0.9659258262890683122, 1.000000000000000000, 0.9659258262890683122, 1.000000000000000000, 0.9659258262890683122, 1.000000000000000000, 0.9659258262890683122, 1.000000000000000000, 0.9659258262890683122, 1.000000000000000000, 0.9659258262890683122, 1.000000000000000000, 0.9659258262890683122, 1.000000000000000000, 0.9659258262890683122, 1.000000000000000000, 0.9659258262890683122, 1.000000000000000000, 0.9659258262890683122, 1.000000000000000000, 0.9659258262890683122, 1.000000000000000000, 0.9659258262890683122, 1.000000000000000000, 0.9659258262890683122, 1.000000000000000000, 0.9659258262890683122, 1.000000000000000000, 0.9659258262890683122, 1.000000000000000000, 0.9659258262890683122, 1.000000000000000000, 0.9659258262890683122, 1.000000000000000000, 0.9659258262890683122, 1.000000000000000000, 0.9659258262890683122, 1.000000000000000000, 0.9659258262890683122, 1.000000000000000000, 0.9659258262890683122, 1.000000000000000000, 0.9659258262890683122, 1.000000000000000000, 0.9659258262890683122, 1.000000000000000000, 0.9659258262890683122, 1.000000000000000000, 0.9659258262890683122, 1.000000000000000000, 0.9659258262890683122, 1.000000000000000000, 0.9659258262890683122, 1.000000000000000000, 0.9659258262890683122, 1.000000000000000000, 0.9659258262890683122, 1.000000000000000000, 0.9659258262890683122, 1.000000000000000000, 0.9659258262890683122, 1.000000000000000000, 0.9659258262890683122, 1.000000000000000000, 0.9659258262890683122, 1.000000000000000000, 0.9659258262890683122, 1.000000000000000000, 0.9659258262890683122, 1.000000000000000000, 0.9659258262890683122, 1.000000000000000000, 0.9659258262890683122, 1.000000000000000000, 0.9659258262890683122, 1.000000000000000000, 0.9659258262890683122, 1.000000000000000000, 0.9659258262890683122, 1.000000000000000000, 0.9659258262890683122, 1.000000000000000000, 0.9659258262890683122, 1.000000000000000000, 0.9659258262890683122, 1.000000000000000000, 0.9659258262890683122, 1.000000000000000000, 0.9659258262890683122, 1.000000000000000000, 0.9659258262890683122, 1.000000000000000000, 0.9659258262890683122, 1.000000000000000000, 0.9659258262890683122, 1.000000000000000000, 0.9659258262890683122, 1.000000000000000000, 0.9659258262890683122, 1.000000000000000000, 0.9659258262890683122, 1.000000000000000000, 0.9659258262890683122, 1.000000000000000000, 0.9659258262890683122, 1.000000000000000000, 0.9659258262890683122, 1.000000000000000000, 0.9659258262890683122, 1.000000000000000000, 0.9659258262890683122, 1.000000000000000000, 0.9659258262890683122, 1.000000000000000000, 0.9659258262890683122, 1.000000000000000000, 0.9659258262890683122, 1.000000000000000000, 0.9659258262890683122, 1.000000000000000000, 0.9659258262890683122, 1.000000000000000000, 0.9659258262890683122, 1.000000000000000000, 0.9659258262890683122, 1.000000000000000000, 0.9659258262890683122, 1.000000000000000000, 0.9659258262890683122, 1.000000000000000000, 0.9659258262890683122, 1.000000000000000000, 0.9659258262890683122, 1.000000000000000000, 0.9659258262890683122, 1.000000000000000000, 0.9659258262890683122, 1.000000000000000000, 0.9659258262890683122, 1.000000000000000000, 0.9659258262890683122, 1.000000000000000000, 0.9659258262890683122, 1.000000000000000000, 0.9659258262890683122, 1.000000000000000000, 0.9659258262890683122, 1.000000000000000000, 0.9659258262890683122, 1.000000000000000000, 0.9659258262890683122, 1.000000000000000000, 0.9659258262890683122, 1.000000000000000000, 0.9659258262890683122, 1.000000000000000000, 0.9659258262890683122, 1.000000000000000000, 0.9659258262890683122, 1.000000000000000000, 0.9659258262890683122, 1.000000000000000000, 0.9659258262890683122, 1.000000000000000000, 0.9659258262890683122, 1.000000000000000000, 0.9659258262890683122, 1.000000000000000000, 0.9659258262890683122, 1.000000000000000000, 0.9659258262890683122, 1.000000000000000000, 0.9659258262890683122, 1.000000000000000000, 0.9659258262890683122, 1.000000000000000000, 0.9659258262890683122, 1.000000000000000000, 0.9659258262890683122, 1.000000000000000000, 0.9659258262890683122, 1.000000000000000000, 0.9659258262890683122, 1.000000000000000000, 0.9659258262890683122, 1.000000000000000000, 0.9659258262890683122, 1.000000000000000000, 0.9659258262890683122, 1.000000000000000000, 0.9659258262890683122, 1.000000000000000000, 0.9659258262890683122, 1.000000000000000000, 0.9659258262890683122, 1.000000000000000000, 0.9659258262890683122, 1.000000000000000000, 0.9659258262890683122, 1.000000000000000000, 0.9659258262890683122, 1.000000000000000000, 0.9659258262890683122, 1.000000000000000000, 0.9659258262890683122, 1.000000000000000000, 0.9659258262890683122, 1.000000000000000000, 0.9659258262890683122, 1.000000000000000000, 0.9659258262890683122, 1.000000000000000000, 0.9659258262890683122, 1.000000000000000000, 0.9659258262890683122, 1.000000000000000000, 0.9659258262890683122, 1.000000000000000000, 0.9659258262890683122, 1.000000000000000000, 0.9659258262890683122, 1.000000000000000000, 0.9659258262890683122, 1.000000000000000000, 0.9659258262890683122, 1.000000000000000000, 0.9659258262890683122, 1.000000000000000000, 0.9659258262890683122, 1.000000000000000000, 0.9659258262890683122, 1.000000000000000000, 0.9659258262890683122, 1.000000000000000000, 0.9659258262890683122, 1.000000000000000000, 0.9659258262890683122, 1.000000000000000000, 0.9659258262890683122, 1.000000000000000000, 0.9659258262890683122, 1.000000000000000000, 0.9659258262890683122, 1.000000000000000000, 0.9659258262890683122, 1.000000000000000000, 0.9659258262890683122, 1.000000000000000000, 0.9659258262890683122, 1.000000000000000000, 0.9659258262890683122, 1.000000000000000000, 0.9659258262890683122, 1.000000000000000000, 0.9659258262890683122, 1.000000000000000000, 0.9659258262890683122, 1.000000000000000000, 0.9659258262890683122, 1.000000000000000000, 0.9659258262890683122, 1.000000000000000000, 0.9659258262890683122, 1.000000000000000000, 0.9659258262890683122, 1.000000000000000000, 0.9659258262890683122, 1.000000000000000000, 0.9659258262890683122, 1.000000000000000000, 0.9659258262890683122, 1.000000000000000000, 0.9659258262890683122, 1.000000000000000000, 0.9659258262890683122, 1.000000000000000000, 0.9659258262890683122, 1.000000000000000000, 0.9659258262890683122, 1.000000000000000000, 0.9659258262890683122, 1.000000000000000000, 0.9659258262890683122, 1.000000000000000000, 0.9659258262890683122, 1.000000000000000000, 0.9659258262890683122, 1.000000000000000000, 0.9659258262890683122, 1.000000000000000000, 0.9659258262890683122, 1.000000000000000000, 0.9659258262890683122, 1.000000000000000000, 0.9659258262890683122, 1.000000000000000000, 0.9659258262890683122, 1.000000000000000000, 0.9659258262890683122, 1.000000000000000000, 0.9659258262890683122, 1.000000000000000000, 0.9659258262890683122, 1.000000000000000000, 0.9659258262890683122, 1.000000000000000000, 0.9659258262890683122, 1.000000000000000000, 0.9659258262890683122, 1.000000000000000000, 0.9659258262890683122, 1.000000000000000000, 0.9659258262890683122, 1.000000000000000000, 0.9659258262890683122, 1.000000000000000000, 0.9659258262890683122, 1.000000000000000000, 0.9659258262890683122, 1.000000000000000000, 0.9659258262890683122, 1.000000000000000000, 0.9659258262890683122, 1.000000000000000000, 0.9659258262890683122, 1.000000000000000000, 0.9659258262890683122, 1.000000000000000000, 0.9659258262890683122, 1.000000000000000000, 0.9659258262890683122, 1.000000000000000000, 0.9659258262890683122, 1.000000000000000000, 0.9659258262890683122, 1.000000000000000000, 0.9659258262890683122, 1.000000000000000000, 0.9659258262890683122, 1.000000000000000000),
 ( 0.3333333333333333703, 0.3219752754296894559, 0.3333333333333333703, 0.3219752754296894559, 0.3333333333333333703, 0.3219752754296894559, 0.3333333333333333703, 0.3219752754296894559, 0.3333333333333333703, 0.3219752754296894559, 0.3333333333333333703, 0.3219752754296894559, 0.3333333333333333703, 0.3219752754296894559, 0.3333333333333333703, 0.3219752754296894559, 0.3333333333333333703, 0.3219752754296894559, 0.3333333333333333703, 0.3219752754296894559, 0.3333333333333333703, 0.3219752754296894559, 0.3333333333333333703, 0.3219752754296894559, 0.3333333333333333703, 0.3219752754296894559, 0.3333333333333333703, 0.3219752754296894559, 0.3333333333333333703, 0.3219752754296894559, 0.3333333333333333703, 0.3219752754296894559, 0.3333333333333333703, 0.3219752754296894559, 0.3333333333333333703, 0.3219752754296894559, 0.3333333333333333703, 0.3219752754296894559, 0.3333333333333333703, 0.3219752754296894559, 0.3333333333333333703, 0.3219752754296894559, 0.3333333333333333703, 0.3219752754296894559, 0.3333333333333333703, 0.3219752754296894559, 0.3333333333333333703, 0.3219752754296894559, 0.3333333333333333703, 0.3219752754296894559, 0.3333333333333333703, 0.3219752754296894559, 0.3333333333333333703, 0.3219752754296894559, 0.3333333333333333703, 0.3219752754296894559, 0.3333333333333333703, 0.3219752754296894559, 0.3333333333333333703, 0.3219752754296894559, 0.3333333333333333703, 0.3219752754296894559, 0.3333333333333333703, 0.3219752754296894559, 0.3333333333333333703, 0.3219752754296894559, 0.3333333333333333703, 0.3219752754296894559, 0.3333333333333333703, 0.3219752754296894559, 0.3333333333333333703, 0.3219752754296894559, 0.3333333333333333703, 0.3219752754296894559, 0.3333333333333333703, 0.3219752754296894559, 0.3333333333333333703, 0.3219752754296894559, 0.3333333333333333703, 0.3219752754296894559, 0.3333333333333333703, 0.3219752754296894559, 0.3333333333333333703, 0.3219752754296894559, 0.3333333333333333703, 0.3219752754296894559, 0.3333333333333333703, 0.3219752754296894559, 0.3333333333333333703, 0.3219752754296894559, 0.3333333333333333703, 0.3219752754296894559, 0.3333333333333333703, 0.3219752754296894559, 0.3333333333333333703, 0.3219752754296894559, 0.3333333333333333703, 0.3219752754296894559, 0.3333333333333333703, 0.3219752754296894559, 0.3333333333333333703, 0.3219752754296894559, 0.3333333333333333703, 0.3219752754296894559, 0.3333333333333333703, 0.3219752754296894559, 0.3333333333333333703, 0.3219752754296894559, 0.3333333333333333703, 0.3219752754296894559, 0.3333333333333333703, 0.3219752754296894559, 0.3333333333333333703, 0.3219752754296894559, 0.3333333333333333703, 0.3219752754296894559, 0.3333333333333333703, 0.3219752754296894559, 0.3333333333333333703, 0.3219752754296894559, 0.3333333333333333703, 0.3219752754296894559, 0.3333333333333333703, 0.3219752754296894559, 0.3333333333333333703, 0.3219752754296894559, 0.3333333333333333703, 0.3219752754296894559, 0.3333333333333333703, 0.3219752754296894559, 0.3333333333333333703, 0.3219752754296894559, 0.3333333333333333703, 0.3219752754296894559, 0.3333333333333333703, 0.3219752754296894559, 0.3333333333333333703, 0.3219752754296894559, 0.3333333333333333703, 0.3219752754296894559, 0.3333333333333333703, 0.3219752754296894559, 0.3333333333333333703, 0.3219752754296894559, 0.3333333333333333703, 0.3219752754296894559, 0.3333333333333333703, 0.3219752754296894559, 0.3333333333333333703, 0.3219752754296894559, 0.3333333333333333703, 0.3219752754296894559, 0.3333333333333333703, 0.3219752754296894559, 0.3333333333333333703, 0.3219752754296894559, 0.3333333333333333703, 0.3219752754296894559, 0.3333333333333333703, 0.3219752754296894559, 0.3333333333333333703, 0.3219752754296894559, 0.3333333333333333703, 0.3219752754296894559, 0.3333333333333333703, 0.3219752754296894559, 0.3333333333333333703, 0.3219752754296894559, 0.3333333333333333703, 0.3219752754296894559, 0.3333333333333333703, 0.3219752754296894559, 0.3333333333333333703, 0.3219752754296894559, 0.3333333333333333703, 0.3219752754296894559, 0.3333333333333333703, 0.3219752754296894559, 0.3333333333333333703, 0.3219752754296894559, 0.3333333333333333703, 0.3219752754296894559, 0.3333333333333333703, 0.3219752754296894559, 0.3333333333333333703, 0.3219752754296894559, 0.3333333333333333703, 0.3219752754296894559, 0.3333333333333333703, 0.3219752754296894559, 0.3333333333333333703, 0.3219752754296894559, 0.3333333333333333703, 0.3219752754296894559, 0.3333333333333333703, 0.3219752754296894559, 0.3333333333333333703, 0.3219752754296894559, 0.3333333333333333703, 0.3219752754296894559, 0.3333333333333333703, 0.3219752754296894559, 0.3333333333333333703, 0.3219752754296894559, 0.3333333333333333703, 0.3219752754296894559, 0.3333333333333333703, 0.3219752754296894559, 0.3333333333333333703, 0.3219752754296894559, 0.3333333333333333703, 0.3219752754296894559, 0.3333333333333333703, 0.3219752754296894559, 0.3333333333333333703, 0.3219752754296894559, 0.3333333333333333703, 0.3219752754296894559, 0.3333333333333333703, 0.3219752754296894559, 0.3333333333333333703, 0.3219752754296894559, 0.3333333333333333703, 0.3219752754296894559, 0.3333333333333333703, 0.3219752754296894559, 0.3333333333333333703, 0.3219752754296894559, 0.3333333333333333703, 0.3219752754296894559, 0.3333333333333333703, 0.3219752754296894559, 0.3333333333333333703, 0.3219752754296894559, 0.3333333333333333703, 0.3219752754296894559, 0.3333333333333333703, 0.3219752754296894559, 0.3333333333333333703, 0.3219752754296894559, 0.3333333333333333703, 0.3219752754296894559, 0.3333333333333333703, 0.3219752754296894559, 0.3333333333333333703, 0.3219752754296894559, 0.3333333333333333703, 0.3219752754296894559, 0.3333333333333333703, 0.3219752754296894559, 0.3333333333333333703, 0.3219752754296894559, 0.3333333333333333703, 0.3219752754296894559, 0.3333333333333333703, 0.3219752754296894559, 0.3333333333333333703, 0.3219752754296894559, 0.3333333333333333703, 0.3219752754296894559, 0.3333333333333333703, 0.3219752754296894559, 0.3333333333333333703, 0.3219752754296894559, 0.3333333333333333703, 0.3219752754296894559, 0.3333333333333333703, 0.3219752754296894559, 0.3333333333333333703, 0.3219752754296894559, 0.3333333333333333703, 0.3219752754296894559, 0.3333333333333333703, 0.3219752754296894559, 0.3333333333333333703, 0.3219752754296894559, 0.3333333333333333703, 0.3219752754296894559, 0.3333333333333333703, 0.3219752754296894559, 0.3333333333333333703, 0.3219752754296894559, 0.3333333333333333703, 0.3219752754296894559, 0.3333333333333333703, 0.3219752754296894559, 0.3333333333333333703, 0.3219752754296894559, 0.3333333333333333703, 0.3219752754296894559, 0.3333333333333333703, 0.3219752754296894559, 0.3333333333333333703, 0.3219752754296894559, 0.3333333333333333703, 0.3219752754296894559, 0.3333333333333333703, 0.3219752754296894559, 0.3333333333333333703, 0.3219752754296894559, 0.3333333333333333703, 0.3219752754296894559, 0.3333333333333333703, 0.3219752754296894559, 0.3333333333333333703, 0.3219752754296894559, 0.3333333333333333703, 0.3219752754296894559, 0.3333333333333333703, 0.3219752754296894559, 0.3333333333333333703, 0.3219752754296894559, 0.3333333333333333703, 0.3219752754296894559, 0.3333333333333333703, 0.3219752754296894559, 0.3333333333333333703, 0.3219752754296894559, 0.3333333333333333703, 0.3219752754296894559, 0.3333333333333333703, 0.3219752754296894559, 0.3333333333333333703, 0.3219752754296894559, 0.3333333333333333703, 0.3219752754296894559, 0.3333333333333333703, 0.3219752754296894559, 0.3333333333333333703, 0.3219752754296894559, 0.3333333333333333703, 0.3219752754296894559, 0.3333333333333333703, 0.3219752754296894559, 0.3333333333333333703, 0.3219752754296894559, 0.3333333333333333703, 0.3219752754296894559, 0.3333333333333333703, 0.3219752754296894559, 0.3333333333333333703, 0.3219752754296894559, 0.3333333333333333703, 0.3219752754296894559, 0.3333333333333333703, 0.3219752754296894559, 0.3333333333333333703, 0.3219752754296894559, 0.3333333333333333703, 0.3219752754296894559, 0.3333333333333333703, 0.3219752754296894559, 0.3333333333333333703, 0.3219752754296894559, 0.3333333333333333703, 0.3219752754296894559, 0.3333333333333333703, 0.3219752754296894559, 0.3333333333333333703, 0.3219752754296894559, 0.3333333333333333703, 0.3219752754296894559, 0.3333333333333333703, 0.3219752754296894559, 0.3333333333333333703, 0.3219752754296894559, 0.3333333333333333703, 0.3219752754296894559, 0.3333333333333333703, 0.3219752754296894559, 0.3333333333333333703, 0.3219752754296894559, 0.3333333333333333703, 0.3219752754296894559, 0.3333333333333333703, 0.3219752754296894559, 0.3333333333333333703, 0.3219752754296894559, 0.3333333333333333703, 0.3219752754296894559, 0.3333333333333333703, 0.3219752754296894559, 0.3333333333333333703, 0.3219752754296894559, 0.3333333333333333703, 0.3219752754296894559, 0.3333333333333333703, 0.3219752754296894559, 0.3333333333333333703, 0.3219752754296894559, 0.3333333333333333703, 0.3219752754296894559, 0.3333333333333333703, 0.3219752754296894559, 0.3333333333333333703, 0.3219752754296894559, 0.3333333333333333703, 0.3219752754296894559, 0.3333333333333333703, 0.3219752754296894559, 0.3333333333333333703, 0.3219752754296894559, 0.3333333333333333703, 0.3219752754296894559, 0.3333333333333333703, 0.3219752754296894559, 0.3333333333333333703, 0.3219752754296894559, 0.3333333333333333703, 0.3219752754296894559, 0.3333333333333333703, 0.3219752754296894559, 0.3333333333333333703, 0.3219752754296894559, 0.3333333333333333703, 0.3219752754296894559, 0.3333333333333333703, 0.3219752754296894559, 0.3333333333333333703, 0.3219752754296894559, 0.3333333333333333703, 0.3219752754296894559, 0.3333333333333333703, 0.3219752754296894559, 0.3333333333333333703, 0.3219752754296894559, 0.3333333333333333703, 0.3219752754296894559, 0.3333333333333333703, 0.3219752754296894559, 0.3333333333333333703, 0.3219752754296894559, 0.3333333333333333703, 0.3219752754296894559, 0.3333333333333333703, 0.3219752754296894559, 0.3333333333333333703, 0.3219752754296894559, 0.3333333333333333703, 0.3219752754296894559, 0.3333333333333333703, 0.3219752754296894559, 0.3333333333333333703, 0.3219752754296894559, 0.3333333333333333703, 0.3219752754296894559, 0.3333333333333333703, 0.3219752754296894559, 0.3333333333333333703, 0.3219752754296894559, 0.3333333333333333703, 0.3219752754296894559, 0.3333333333333333703, 0.3219752754296894559, 0.3333333333333333703, 0.3219752754296894559, 0.3333333333333333703),
 ( 0.3333333333333333703, 0.3219752754296894559, 0.3333333333333333703, 0.3219752754296894559, 0.3333333333333333703, 0.3219752754296894559, 0.3333333333333333703, 0.3219752754296894559, 0.3333333333333333703, 0.3219752754296894559, 0.3333333333333333703, 0.3219752754296894559, 0.3333333333333333703, 0.3219752754296894559, 0.3333333333333333703, 0.3219752754296894559, 0.3333333333333333703, 0.3219752754296894559, 0.3333333333333333703, 0.3219752754296894559, 0.3333333333333333703, 0.3219752754296894559, 0.3333333333333333703, 0.3219752754296894559, 0.3333333333333333703, 0.3219752754296894559, 0.3333333333333333703, 0.3219752754296894559, 0.3333333333333333703, 0.3219752754296894559, 0.3333333333333333703, 0.3219752754296894559, 0.3333333333333333703, 0.3219752754296894559, 0.3333333333333333703, 0.3219752754296894559, 0.3333333333333333703, 0.3219752754296894559, 0.3333333333333333703, 0.3219752754296894559, 0.3333333333333333703, 0.3219752754296894559, 0.3333333333333333703, 0.3219752754296894559, 0.3333333333333333703, 0.3219752754296894559, 0.3333333333333333703, 0.3219752754296894559, 0.3333333333333333703, 0.3219752754296894559, 0.3333333333333333703, 0.3219752754296894559, 0.3333333333333333703, 0.3219752754296894559, 0.3333333333333333703, 0.3219752754296894559, 0.3333333333333333703, 0.3219752754296894559, 0.3333333333333333703, 0.3219752754296894559, 0.3333333333333333703, 0.3219752754296894559, 0.3333333333333333703, 0.3219752754296894559, 0.3333333333333333703, 0.3219752754296894559, 0.3333333333333333703, 0.3219752754296894559, 0.3333333333333333703, 0.3219752754296894559, 0.3333333333333333703, 0.3219752754296894559, 0.3333333333333333703, 0.3219752754296894559, 0.3333333333333333703, 0.3219752754296894559, 0.3333333333333333703, 0.3219752754296894559, 0.3333333333333333703, 0.3219752754296894559, 0.3333333333333333703, 0.3219752754296894559, 0.3333333333333333703, 0.3219752754296894559, 0.3333333333333333703, 0.3219752754296894559, 0.3333333333333333703, 0.3219752754296894559, 0.3333333333333333703, 0.3219752754296894559, 0.3333333333333333703, 0.3219752754296894559, 0.3333333333333333703, 0.3219752754296894559, 0.3333333333333333703, 0.3219752754296894559, 0.3333333333333333703, 0.3219752754296894559, 0.3333333333333333703, 0.3219752754296894559, 0.3333333333333333703, 0.3219752754296894559, 0.3333333333333333703, 0.3219752754296894559, 0.3333333333333333703, 0.3219752754296894559, 0.3333333333333333703, 0.3219752754296894559, 0.3333333333333333703, 0.3219752754296894559, 0.3333333333333333703, 0.3219752754296894559, 0.3333333333333333703, 0.3219752754296894559, 0.3333333333333333703, 0.3219752754296894559, 0.3333333333333333703, 0.3219752754296894559, 0.3333333333333333703, 0.3219752754296894559, 0.3333333333333333703, 0.3219752754296894559, 0.3333333333333333703, 0.3219752754296894559, 0.3333333333333333703, 0.3219752754296894559, 0.3333333333333333703, 0.3219752754296894559, 0.3333333333333333703, 0.3219752754296894559, 0.3333333333333333703, 0.3219752754296894559, 0.3333333333333333703, 0.3219752754296894559, 0.3333333333333333703, 0.3219752754296894559, 0.3333333333333333703, 0.3219752754296894559, 0.3333333333333333703, 0.3219752754296894559, 0.3333333333333333703, 0.3219752754296894559, 0.3333333333333333703, 0.3219752754296894559, 0.3333333333333333703, 0.3219752754296894559, 0.3333333333333333703, 0.3219752754296894559, 0.3333333333333333703, 0.3219752754296894559, 0.3333333333333333703, 0.3219752754296894559, 0.3333333333333333703, 0.3219752754296894559, 0.3333333333333333703, 0.3219752754296894559, 0.3333333333333333703, 0.3219752754296894559, 0.3333333333333333703, 0.3219752754296894559, 0.3333333333333333703, 0.3219752754296894559, 0.3333333333333333703, 0.3219752754296894559, 0.3333333333333333703, 0.3219752754296894559, 0.3333333333333333703, 0.3219752754296894559, 0.3333333333333333703, 0.3219752754296894559, 0.3333333333333333703, 0.3219752754296894559, 0.3333333333333333703, 0.3219752754296894559, 0.3333333333333333703, 0.3219752754296894559, 0.3333333333333333703, 0.3219752754296894559, 0.3333333333333333703, 0.3219752754296894559, 0.3333333333333333703, 0.3219752754296894559, 0.3333333333333333703, 0.3219752754296894559, 0.3333333333333333703, 0.3219752754296894559, 0.3333333333333333703, 0.3219752754296894559, 0.3333333333333333703, 0.3219752754296894559, 0.3333333333333333703, 0.3219752754296894559, 0.3333333333333333703, 0.3219752754296894559, 0.3333333333333333703, 0.3219752754296894559, 0.3333333333333333703, 0.3219752754296894559, 0.3333333333333333703, 0.3219752754296894559, 0.3333333333333333703, 0.3219752754296894559, 0.3333333333333333703, 0.3219752754296894559, 0.3333333333333333703, 0.3219752754296894559, 0.3333333333333333703, 0.3219752754296894559, 0.3333333333333333703, 0.3219752754296894559, 0.3333333333333333703, 0.3219752754296894559, 0.3333333333333333703, 0.3219752754296894559, 0.3333333333333333703, 0.3219752754296894559, 0.3333333333333333703, 0.3219752754296894559, 0.3333333333333333703, 0.3219752754296894559, 0.3333333333333333703, 0.3219752754296894559, 0.3333333333333333703, 0.3219752754296894559, 0.3333333333333333703, 0.3219752754296894559, 0.3333333333333333703, 0.3219752754296894559, 0.3333333333333333703, 0.3219752754296894559, 0.3333333333333333703, 0.3219752754296894559, 0.3333333333333333703, 0.3219752754296894559, 0.3333333333333333703, 0.3219752754296894559, 0.3333333333333333703, 0.3219752754296894559, 0.3333333333333333703, 0.3219752754296894559, 0.3333333333333333703, 0.3219752754296894559, 0.3333333333333333703, 0.3219752754296894559, 0.3333333333333333703, 0.3219752754296894559, 0.3333333333333333703, 0.3219752754296894559, 0.3333333333333333703, 0.3219752754296894559, 0.3333333333333333703, 0.3219752754296894559, 0.3333333333333333703, 0.3219752754296894559, 0.3333333333333333703, 0.3219752754296894559, 0.3333333333333333703, 0.3219752754296894559, 0.3333333333333333703, 0.3219752754296894559, 0.3333333333333333703, 0.3219752754296894559, 0.3333333333333333703, 0.3219752754296894559, 0.3333333333333333703, 0.3219752754296894559, 0.3333333333333333703, 0.3219752754296894559, 0.3333333333333333703, 0.3219752754296894559, 0.3333333333333333703, 0.3219752754296894559, 0.3333333333333333703, 0.3219752754296894559, 0.3333333333333333703, 0.3219752754296894559, 0.3333333333333333703, 0.3219752754296894559, 0.3333333333333333703, 0.3219752754296894559, 0.3333333333333333703, 0.3219752754296894559, 0.3333333333333333703, 0.3219752754296894559, 0.3333333333333333703, 0.3219752754296894559, 0.3333333333333333703, 0.3219752754296894559, 0.3333333333333333703, 0.3219752754296894559, 0.3333333333333333703, 0.3219752754296894559, 0.3333333333333333703, 0.3219752754296894559, 0.3333333333333333703, 0.3219752754296894559, 0.3333333333333333703, 0.3219752754296894559, 0.3333333333333333703, 0.3219752754296894559, 0.3333333333333333703, 0.3219752754296894559, 0.3333333333333333703, 0.3219752754296894559, 0.3333333333333333703, 0.3219752754296894559, 0.3333333333333333703, 0.3219752754296894559, 0.3333333333333333703, 0.3219752754296894559, 0.3333333333333333703, 0.3219752754296894559, 0.3333333333333333703, 0.3219752754296894559, 0.3333333333333333703, 0.3219752754296894559, 0.3333333333333333703, 0.3219752754296894559, 0.3333333333333333703, 0.3219752754296894559, 0.3333333333333333703, 0.3219752754296894559, 0.3333333333333333703, 0.3219752754296894559, 0.3333333333333333703, 0.3219752754296894559, 0.3333333333333333703, 0.3219752754296894559, 0.3333333333333333703, 0.3219752754296894559, 0.3333333333333333703, 0.3219752754296894559, 0.3333333333333333703, 0.3219752754296894559, 0.3333333333333333703, 0.3219752754296894559, 0.3333333333333333703, 0.3219752754296894559, 0.3333333333333333703, 0.3219752754296894559, 0.3333333333333333703, 0.3219752754296894559, 0.3333333333333333703, 0.3219752754296894559, 0.3333333333333333703, 0.3219752754296894559, 0.3333333333333333703, 0.3219752754296894559, 0.3333333333333333703, 0.3219752754296894559, 0.3333333333333333703, 0.3219752754296894559, 0.3333333333333333703, 0.3219752754296894559, 0.3333333333333333703, 0.3219752754296894559, 0.3333333333333333703, 0.3219752754296894559, 0.3333333333333333703, 0.3219752754296894559, 0.3333333333333333703, 0.3219752754296894559, 0.3333333333333333703, 0.3219752754296894559, 0.3333333333333333703, 0.3219752754296894559, 0.3333333333333333703, 0.3219752754296894559, 0.3333333333333333703, 0.3219752754296894559, 0.3333333333333333703, 0.3219752754296894559, 0.3333333333333333703, 0.3219752754296894559, 0.3333333333333333703, 0.3219752754296894559, 0.3333333333333333703, 0.3219752754296894559, 0.3333333333333333703, 0.3219752754296894559, 0.3333333333333333703, 0.3219752754296894559, 0.3333333333333333703, 0.3219752754296894559, 0.3333333333333333703, 0.3219752754296894559, 0.3333333333333333703, 0.3219752754296894559, 0.3333333333333333703, 0.3219752754296894559, 0.3333333333333333703, 0.3219752754296894559, 0.3333333333333333703, 0.3219752754296894559, 0.3333333333333333703, 0.3219752754296894559, 0.3333333333333333703, 0.3219752754296894559, 0.3333333333333333703, 0.3219752754296894559, 0.3333333333333333703, 0.3219752754296894559, 0.3333333333333333703, 0.3219752754296894559, 0.3333333333333333703, 0.3219752754296894559, 0.3333333333333333703, 0.3219752754296894559, 0.3333333333333333703, 0.3219752754296894559, 0.3333333333333333703, 0.3219752754296894559, 0.3333333333333333703, 0.3219752754296894559, 0.3333333333333333703, 0.3219752754296894559, 0.3333333333333333703, 0.3219752754296894559, 0.3333333333333333703, 0.3219752754296894559, 0.3333333333333333703, 0.3219752754296894559, 0.3333333333333333703, 0.3219752754296894559, 0.3333333333333333703, 0.3219752754296894559, 0.3333333333333333703, 0.3219752754296894559, 0.3333333333333333703, 0.3219752754296894559, 0.3333333333333333703, 0.3219752754296894559, 0.3333333333333333703, 0.3219752754296894559, 0.3333333333333333703, 0.3219752754296894559, 0.3333333333333333703, 0.3219752754296894559, 0.3333333333333333703, 0.3219752754296894559, 0.3333333333333333703, 0.3219752754296894559, 0.3333333333333333703, 0.3219752754296894559, 0.3333333333333333703, 0.3219752754296894559, 0.3333333333333333703, 0.3219752754296894559, 0.3333333333333333703, 0.3219752754296894559, 0.3333333333333333703, 0.3219752754296894559, 0.3333333333333333703, 0.3219752754296894559, 0.3333333333333333703, 0.3219752754296894559, 0.3333333333333333703),
 ( 1.000000000000000000, 0.9659258262890683122, 1.000000000000000000, 0.9659258262890683122, 1.000000000000000000, 0.9659258262890683122, 1.000000000000000000, 0.9659258262890683122, 1.000000000000000000, 0.9659258262890683122, 1.000000000000000000, 0.9659258262890683122, 1.000000000000000000, 0.9659258262890683122, 1.000000000000000000, 0.9659258262890683122, 1.000000000000000000, 0.9659258262890683122, 1.000000000000000000, 0.9659258262890683122, 1.000000000000000000, 0.9659258262890683122, 1.000000000000000000, 0.9659258262890683122, 1.000000000000000000, 0.9659258262890683122, 1.000000000000000000, 0.9659258262890683122, 1.000000000000000000, 0.9659258262890683122, 1.000000000000000000, 0.9659258262890683122, 1.000000000000000000, 0.9659258262890683122, 1.000000000000000000, 0.9659258262890683122, 1.000000000000000000, 0.9659258262890683122, 1.000000000000000000, 0.9659258262890683122, 1.000000000000000000, 0.9659258262890683122, 1.000000000000000000, 0.9659258262890683122, 1.000000000000000000, 0.9659258262890683122, 1.000000000000000000, 0.9659258262890683122, 1.000000000000000000, 0.9659258262890683122, 1.000000000000000000, 0.9659258262890683122, 1.000000000000000000, 0.9659258262890683122, 1.000000000000000000, 0.9659258262890683122, 1.000000000000000000, 0.9659258262890683122, 1.000000000000000000, 0.9659258262890683122, 1.000000000000000000, 0.9659258262890683122, 1.000000000000000000, 0.9659258262890683122, 1.000000000000000000, 0.9659258262890683122, 1.000000000000000000, 0.9659258262890683122, 1.000000000000000000, 0.9659258262890683122, 1.000000000000000000, 0.9659258262890683122, 1.000000000000000000, 0.9659258262890683122, 1.000000000000000000, 0.9659258262890683122, 1.000000000000000000, 0.9659258262890683122, 1.000000000000000000, 0.9659258262890683122, 1.000000000000000000, 0.9659258262890683122, 1.000000000000000000, 0.9659258262890683122, 1.000000000000000000, 0.9659258262890683122, 1.000000000000000000, 0.9659258262890683122, 1.000000000000000000, 0.9659258262890683122, 1.000000000000000000, 0.9659258262890683122, 1.000000000000000000, 0.9659258262890683122, 1.000000000000000000, 0.9659258262890683122, 1.000000000000000000, 0.9659258262890683122, 1.000000000000000000, 0.9659258262890683122, 1.000000000000000000, 0.9659258262890683122, 1.000000000000000000, 0.9659258262890683122, 1.000000000000000000, 0.9659258262890683122, 1.000000000000000000, 0.9659258262890683122, 1.000000000000000000, 0.9659258262890683122, 1.000000000000000000, 0.9659258262890683122, 1.000000000000000000, 0.9659258262890683122, 1.000000000000000000, 0.9659258262890683122, 1.000000000000000000, 0.9659258262890683122, 1.000000000000000000, 0.9659258262890683122, 1.000000000000000000, 0.9659258262890683122, 1.000000000000000000, 0.9659258262890683122, 1.000000000000000000, 0.9659258262890683122, 1.000000000000000000, 0.9659258262890683122, 1.000000000000000000, 0.9659258262890683122, 1.000000000000000000, 0.9659258262890683122, 1.000000000000000000, 0.9659258262890683122, 1.000000000000000000, 0.9659258262890683122, 1.000000000000000000, 0.9659258262890683122, 1.000000000000000000, 0.9659258262890683122, 1.000000000000000000, 0.9659258262890683122, 1.000000000000000000, 0.9659258262890683122, 1.000000000000000000, 0.9659258262890683122, 1.000000000000000000, 0.9659258262890683122, 1.000000000000000000, 0.9659258262890683122, 1.000000000000000000, 0.9659258262890683122, 1.000000000000000000, 0.9659258262890683122, 1.000000000000000000, 0.9659258262890683122, 1.000000000000000000, 0.9659258262890683122, 1.000000000000000000, 0.9659258262890683122, 1.000000000000000000, 0.9659258262890683122, 1.000000000000000000, 0.9659258262890683122, 1.000000000000000000, 0.9659258262890683122, 1.000000000000000000, 0.9659258262890683122, 1.000000000000000000, 0.9659258262890683122, 1.000000000000000000, 0.9659258262890683122, 1.000000000000000000, 0.9659258262890683122, 1.000000000000000000, 0.9659258262890683122, 1.000000000000000000, 0.9659258262890683122, 1.000000000000000000, 0.9659258262890683122, 1.000000000000000000, 0.9659258262890683122, 1.000000000000000000, 0.9659258262890683122, 1.000000000000000000, 0.9659258262890683122, 1.000000000000000000, 0.9659258262890683122, 1.000000000000000000, 0.9659258262890683122, 1.000000000000000000, 0.9659258262890683122, 1.000000000000000000, 0.9659258262890683122, 1.000000000000000000, 0.9659258262890683122, 1.000000000000000000, 0.9659258262890683122, 1.000000000000000000, 0.9659258262890683122, 1.000000000000000000, 0.9659258262890683122, 1.000000000000000000, 0.9659258262890683122, 1.000000000000000000, 0.9659258262890683122, 1.000000000000000000, 0.9659258262890683122, 1.000000000000000000, 0.9659258262890683122, 1.000000000000000000, 0.9659258262890683122, 1.000000000000000000, 0.9659258262890683122, 1.000000000000000000, 0.9659258262890683122, 1.000000000000000000, 0.9659258262890683122, 1.000000000000000000, 0.9659258262890683122, 1.000000000000000000, 0.9659258262890683122, 1.000000000000000000, 0.9659258262890683122, 1.000000000000000000, 0.9659258262890683122, 1.000000000000000000, 0.9659258262890683122, 1.000000000000000000, 0.9659258262890683122, 1.000000000000000000, 0.9659258262890683122, 1.000000000000000000, 0.9659258262890683122, 1.000000000000000000, 0.9659258262890683122, 1.000000000000000000, 0.9659258262890683122, 1.000000000000000000, 0.9659258262890683122, 1.000000000000000000, 0.9659258262890683122, 1.000000000000000000, 0.9659258262890683122, 1.000000000000000000, 0.9659258262890683122, 1.000000000000000000, 0.9659258262890683122, 1.000000000000000000, 0.9659258262890683122, 1.000000000000000000, 0.9659258262890683122, 1.000000000000000000, 0.9659258262890683122, 1.000000000000000000, 0.9659258262890683122, 1.000000000000000000, 0.9659258262890683122, 1.000000000000000000, 0.9659258262890683122, 1.000000000000000000, 0.9659258262890683122, 1.000000000000000000, 0.9659258262890683122, 1.000000000000000000, 0.9659258262890683122, 1.000000000000000000, 0.9659258262890683122, 1.000000000000000000, 0.9659258262890683122, 1.000000000000000000, 0.9659258262890683122, 1.000000000000000000, 0.9659258262890683122, 1.000000000000000000, 0.9659258262890683122, 1.000000000000000000, 0.9659258262890683122, 1.000000000000000000, 0.9659258262890683122, 1.000000000000000000, 0.9659258262890683122, 1.000000000000000000, 0.9659258262890683122, 1.000000000000000000, 0.9659258262890683122, 1.000000000000000000, 0.9659258262890683122, 1.000000000000000000, 0.9659258262890683122, 1.000000000000000000, 0.9659258262890683122, 1.000000000000000000, 0.9659258262890683122, 1.000000000000000000, 0.9659258262890683122, 1.000000000000000000, 0.9659258262890683122, 1.000000000000000000, 0.9659258262890683122, 1.000000000000000000, 0.9659258262890683122, 1.000000000000000000, 0.9659258262890683122, 1.000000000000000000, 0.9659258262890683122, 1.000000000000000000, 0.9659258262890683122, 1.000000000000000000, 0.9659258262890683122, 1.000000000000000000, 0.9659258262890683122, 1.000000000000000000, 0.9659258262890683122, 1.000000000000000000, 0.9659258262890683122, 1.000000000000000000, 0.9659258262890683122, 1.000000000000000000, 0.9659258262890683122, 1.000000000000000000, 0.9659258262890683122, 1.000000000000000000, 0.9659258262890683122, 1.000000000000000000, 0.9659258262890683122, 1.000000000000000000, 0.9659258262890683122, 1.000000000000000000, 0.9659258262890683122, 1.000000000000000000, 0.9659258262890683122, 1.000000000000000000, 0.9659258262890683122, 1.000000000000000000, 0.9659258262890683122, 1.000000000000000000, 0.9659258262890683122, 1.000000000000000000, 0.9659258262890683122, 1.000000000000000000, 0.9659258262890683122, 1.000000000000000000, 0.9659258262890683122, 1.000000000000000000, 0.9659258262890683122, 1.000000000000000000, 0.9659258262890683122, 1.000000000000000000, 0.9659258262890683122, 1.000000000000000000, 0.9659258262890683122, 1.000000000000000000, 0.9659258262890683122, 1.000000000000000000, 0.9659258262890683122, 1.000000000000000000, 0.9659258262890683122, 1.000000000000000000, 0.9659258262890683122, 1.000000000000000000, 0.9659258262890683122, 1.000000000000000000, 0.9659258262890683122, 1.000000000000000000, 0.9659258262890683122, 1.000000000000000000, 0.9659258262890683122, 1.000000000000000000, 0.9659258262890683122, 1.000000000000000000, 0.9659258262890683122, 1.000000000000000000, 0.9659258262890683122, 1.000000000000000000, 0.9659258262890683122, 1.000000000000000000, 0.9659258262890683122, 1.000000000000000000, 0.9659258262890683122, 1.000000000000000000, 0.9659258262890683122, 1.000000000000000000, 0.9659258262890683122, 1.000000000000000000, 0.9659258262890683122, 1.000000000000000000, 0.9659258262890683122, 1.000000000000000000, 0.9659258262890683122, 1.000000000000000000, 0.9659258262890683122, 1.000000000000000000, 0.9659258262890683122, 1.000000000000000000, 0.9659258262890683122, 1.000000000000000000, 0.9659258262890683122, 1.000000000000000000, 0.9659258262890683122, 1.000000000000000000, 0.9659258262890683122, 1.000000000000000000, 0.9659258262890683122, 1.000000000000000000, 0.9659258262890683122, 1.000000000000000000, 0.9659258262890683122, 1.000000000000000000, 0.9659258262890683122, 1.000000000000000000, 0.9659258262890683122, 1.000000000000000000, 0.9659258262890683122, 1.000000000000000000, 0.9659258262890683122, 1.000000000000000000, 0.9659258262890683122, 1.000000000000000000, 0.9659258262890683122, 1.000000000000000000, 0.9659258262890683122, 1.000000000000000000, 0.9659258262890683122, 1.000000000000000000, 0.9659258262890683122, 1.000000000000000000, 0.9659258262890683122, 1.000000000000000000, 0.9659258262890683122, 1.000000000000000000, 0.9659258262890683122, 1.000000000000000000, 0.9659258262890683122, 1.000000000000000000, 0.9659258262890683122, 1.000000000000000000, 0.9659258262890683122, 1.000000000000000000, 0.9659258262890683122, 1.000000000000000000, 0.9659258262890683122, 1.000000000000000000, 0.9659258262890683122, 1.000000000000000000, 0.9659258262890683122, 1.000000000000000000, 0.9659258262890683122, 1.000000000000000000, 0.9659258262890683122, 1.000000000000000000, 0.9659258262890683122, 1.000000000000000000, 0.9659258262890683122, 1.000000000000000000, 0.9659258262890683122, 1.000000000000000000) ) ) 
 REPRESENTATION_ITEM ( '' )  SURFACE ( )  );
#128199=CARTESIAN_POINT ( 'NONE',  ( 13.89961937509957401, 13.97604488694547697, 46.87609039468565442 ) ) ;
#128200=CARTESIAN_POINT ( 'NONE',  ( 18.67979575497194134, -10.72451020669871369, 55.83442372801901854 ) ) ;
#128201=CARTESIAN_POINT ( 'NONE',  ( 10.72451020669898902, -18.67979575497178502, 57.91557627198103120 ) ) ;
#128202=CARTESIAN_POINT ( 'NONE',  ( 19.05341960407617918, -5.049401038297876454, 106.0427570613523471 ) ) ;
#128203=CARTESIAN_POINT ( 'NONE',  ( -5.153800228976328057, -19.02544592524343514, 52.29057627198100988 ) ) ;
#128204=CARTESIAN_POINT ( 'NONE',  ( 0.05219959533936267826, -19.03943276465977164, 85.00109039468567573 ) ) ;
#128205=CARTESIAN_POINT ( 'NONE',  ( -10.72451020669870658, -18.67979575497194134, 89.58442372801901854 ) ) ;
#128206=CARTESIAN_POINT ( 'NONE',  ( 19.02544592524334988, 5.153800228976608722, 71.45942372801900433 ) ) ;
#128207=CARTESIAN_POINT ( 'NONE',  ( -9.474510206698964154, 16.51473224551069663, 35.41557627198102409 ) ) ;
#128208=CARTESIAN_POINT ( 'NONE',  ( -10.81492255796078084, -18.62759615963271287, 52.08224293864768839 ) ) ;
#128209=CARTESIAN_POINT ( 'NONE',  ( -0.05219959533910754901, -16.53943276465976808, 57.49890960531435979 ) ) ;
#128211=CARTESIAN_POINT ( 'NONE',  ( -16.51473224551082808, 9.474510206698731452, 28.33442372801900433 ) ) ;
#128212=CARTESIAN_POINT ( 'NONE',  ( 16.55341960407618274, -4.379528057220086978, 96.04275706135236135 ) ) ;
#128213=CARTESIAN_POINT ( 'NONE',  ( 0.05219959533910956823, 16.53943276465976808, 49.99890960531437401 ) ) ;
#128214=CARTESIAN_POINT ( 'NONE',  ( 10.72451020669871369, 18.67979575497193778, 87.08442372801901854 ) ) ;
#128215=CARTESIAN_POINT ( 'NONE',  ( -18.62759615963255300, -10.81492255796106328, 84.16775706135234714 ) ) ;
#128216=CARTESIAN_POINT ( 'NONE',  ( 18.62759615963271287, -10.81492255796078972, 98.33224293864769550 ) ) ;
#128217=CARTESIAN_POINT ( 'NONE',  ( -9.474510206698964154, 16.51473224551069663, 55.41557627198103120 ) ) ;
#128218=CARTESIAN_POINT ( 'NONE',  ( -15.72974639402176322, -15.80617190586768395, 69.37609039468567573 ) ) ;
#128219=CARTESIAN_POINT ( 'NONE',  ( 0.05219959533909260263, 19.03943276465977164, 44.99890960531435979 ) ) ;
#128221=CARTESIAN_POINT ( 'NONE',  ( -19.02544592524342804, 5.153800228976336051, 61.04057627198103120 ) ) ;
#128222=CARTESIAN_POINT ( 'NONE',  ( -14.29746914071049879, 8.314922557960819915, 100.8322429386477097 ) ) ;
#128223=CARTESIAN_POINT ( 'NONE',  ( -16.51473224551069308, -9.474510206698971260, 96.66557627198102409 ) ) ;
#128224=CARTESIAN_POINT ( 'NONE',  ( -16.52544592524342804, 4.483927247898546575, 51.04057627198103120 ) ) ;
#128225=CARTESIAN_POINT ( 'NONE',  ( -12.14591786802309592, -12.06949235617757132, 106.8739096053143811 ) ) ;
#128226=CARTESIAN_POINT ( 'NONE',  ( -21.53943276465977519, 0.05219959533907696930, 81.24890960531436690 ) ) ;
#128227=CARTESIAN_POINT ( 'NONE',  ( 5.719274019375673035, 21.55341960407619339, 32.29275706135235424 ) ) ;
#128229=CARTESIAN_POINT ( 'NONE',  ( 12.14591786802327356, -12.06949235617739191, 30.62609039468567929 ) ) ;
#128230=CARTESIAN_POINT ( 'NONE',  ( -18.67979575497178146, -10.72451020669898902, 81.66557627198103830 ) ) ;
#128231=CARTESIAN_POINT ( 'NONE',  ( -0.05219959533937732626, 21.53943276465977519, 102.5010903946856899 ) ) ;
#128232=CARTESIAN_POINT ( 'NONE',  ( 19.02544592524343514, -5.153800228976328945, 93.54057627198102409 ) ) ;
#128233=CARTESIAN_POINT ( 'NONE',  ( -0.05219959533937732626, 21.53943276465977519, 32.50109039468568284 ) ) ;
#128234=CARTESIAN_POINT ( 'NONE',  ( -15.72974639402197994, 15.80617190586746368, 35.62390960531437401 ) ) ;
#128235=CARTESIAN_POINT ( 'NONE',  ( -4.379528057220086978, -16.55341960407618274, 104.7927570613523898 ) ) ;
#128236=CARTESIAN_POINT ( 'NONE',  ( 21.52544592524334988, 5.823673210054432836, 56.45942372801902565 ) ) ;
#128237=CARTESIAN_POINT ( 'NONE',  ( -5.719274019375665041, -21.55341960407619695, 79.79275706135236135 ) ) ;
#128238=CARTESIAN_POINT ( 'NONE',  ( -18.67979575497193778, 10.72451020669871902, 113.3344237280190328 ) ) ;
#128239=CARTESIAN_POINT ( 'NONE',  ( -8.224510206698735004, -14.34966873604973081, 69.58442372801900433 ) ) ;
#128240=CARTESIAN_POINT ( 'NONE',  ( -10.72451020669870658, -18.67979575497194134, 44.58442372801901854 ) ) ;
#128241=CARTESIAN_POINT ( 'NONE',  ( 16.51473224551069308, 9.474510206698969483, 39.16557627198103120 ) ) ;
#128242=CARTESIAN_POINT ( 'NONE',  ( -15.80617190586768217, 15.72974639402176855, 108.1260903946856757 ) ) ;
#128243=CARTESIAN_POINT ( 'NONE',  ( 5.049401038298161559, -19.05341960407611168, 107.7072429386476955 ) ) ;
#128244=CARTESIAN_POINT ( 'NONE',  ( 21.53943276465977519, -0.05219959533907433946, 108.7489096053143669 ) ) ;
#128245=CARTESIAN_POINT ( 'NONE',  ( 19.35543954521081389, 5.499999999999574563, 82.08901960356452321 ) ) ;
#128246=CARTESIAN_POINT ( 'NONE',  ( -18.62759615963270932, 10.81492255796079327, 70.83224293864770971 ) ) ;
#128247=CARTESIAN_POINT ( 'NONE',  ( 14.34966873604972726, -8.224510206698740333, 45.83442372801901854 ) ) ;
#128248=CARTESIAN_POINT ( 'NONE',  ( 16.53943276465976808, -0.05219959533910856209, 53.74890960531437401 ) ) ;
#128250=CARTESIAN_POINT ( 'NONE',  ( 16.51473224551083163, -9.474510206698727899, 85.83442372801900433 ) ) ;
#128252=CARTESIAN_POINT ( 'NONE',  ( 12.14591786802327356, -12.06949235617739191, 30.62609039468567929 ) ) ;
#128253=CARTESIAN_POINT ( 'NONE',  ( -15.72974639402197994, 15.80617190586746368, 100.6239096053143811 ) ) ;
#128254=CARTESIAN_POINT ( 'NONE',  ( -5.719274019375978568, 21.55341960407610458, 80.20724293864769550 ) ) ;
#128255=CARTESIAN_POINT ( 'NONE',  ( 9.564922557960805705, 16.46253265017160317, 109.5822429386476955 ) ) ;
#128256=CARTESIAN_POINT ( 'NONE',  ( 8.314922557961029526, -14.29746914071037800, 45.41775706135234003 ) ) ;
#128257=CARTESIAN_POINT ( 'NONE',  ( -9.474510206698964154, 16.51473224551069663, 75.41557627198103830 ) ) ;
#128258=CARTESIAN_POINT ( 'NONE',  ( -21.52544592524334988, -5.823673210054445271, 23.95942372801901143 ) ) ;
#128259=CARTESIAN_POINT ( 'NONE',  ( -13.97604488694547697, 13.89961937509957934, 93.12609039468566152 ) ) ;
#128260=CARTESIAN_POINT ( 'NONE',  ( -5.153800228976328057, -19.02544592524343514, 112.2905762719810099 ) ) ;
#128261=CARTESIAN_POINT ( 'NONE',  ( -9.474510206698964154, 16.51473224551069663, 85.41557627198102409 ) ) ;
#128262=CARTESIAN_POINT ( 'NONE',  ( -5.719274019375978568, 21.55341960407610458, 95.20724293864769550 ) ) ;
#128263=CARTESIAN_POINT ( 'NONE',  ( 9.564922557960805705, 16.46253265017160317, 59.58224293864769550 ) ) ;
#128264=CARTESIAN_POINT ( 'NONE',  ( -16.21995358207306026, -7.366697692864123681, 60.06448998487844904 ) ) ;
#128265=CARTESIAN_POINT ( 'NONE',  ( -8.314922557960811034, -14.29746914071050412, 62.08224293864769550 ) ) ;
#128266=CARTESIAN_POINT ( 'NONE',  ( -10.72451020669898014, 18.67979575497178502, 25.41557627198103120 ) ) ;
#128267=CARTESIAN_POINT ( 'NONE',  ( -17.49999999999998579, 5.500000000000032863, 60.79690382534172244 ) ) ;
#128268=CARTESIAN_POINT ( 'NONE',  ( -5.719274019375978568, 21.55341960407610458, 90.20724293864770971 ) ) ;
#128269=CARTESIAN_POINT ( 'NONE',  ( -13.97604488694547697, 13.89961937509957934, 63.12609039468566152 ) ) ;
#128270=CARTESIAN_POINT ( 'NONE',  ( -5.049401038298153566, 19.05341960407611168, 115.2072429386477097 ) ) ;
#128271=CARTESIAN_POINT ( 'NONE',  ( 19.35543954521079968, 5.499999999999572786, 67.08901960356450900 ) ) ;
#128272=CARTESIAN_POINT ( 'NONE',  ( 18.67979575497178502, 10.72451020669898547, 54.16557627198103120 ) ) ;
#128274=CARTESIAN_POINT ( 'NONE',  ( 19.02544592524343514, -5.153800228976328945, 83.54057627198100988 ) ) ;
#128275=CARTESIAN_POINT ( 'NONE',  ( 10.81492255796106328, -18.62759615963255655, 75.41775706135233293 ) ) ;
#128276=CARTESIAN_POINT ( 'NONE',  ( -5.153800228976328057, -19.02544592524343514, 57.29057627198103120 ) ) ;
#128277=CARTESIAN_POINT ( 'NONE',  ( -0.05219959533910754901, -16.53943276465976808, 72.49890960531435269 ) ) ;
#128278=CARTESIAN_POINT ( 'NONE',  ( -0.05219959533934338120, 16.53943276465976808, 32.50109039468568284 ) ) ;
#128279=CARTESIAN_POINT ( 'NONE',  ( -5.719274019375665041, -21.55341960407619695, 64.79275706135234714 ) ) ;
#128281=CARTESIAN_POINT ( 'NONE',  ( 5.153800228976615827, -19.02544592524334988, 30.20942372801900433 ) ) ;
#128282=CARTESIAN_POINT ( 'NONE',  ( 0.05219959533936267826, -19.03943276465977164, 85.00109039468567573 ) ) ;
#128284=CARTESIAN_POINT ( 'NONE',  ( 18.62759615963255655, 10.81492255796105972, 21.66775706135235069 ) ) ;
#128286=CARTESIAN_POINT ( 'NONE',  ( 5.823673210054444382, -21.52544592524334988, 110.2094237280190185 ) ) ;
#128287=CARTESIAN_POINT ( 'NONE',  ( 5.049401038298161559, -19.05341960407611168, 57.70724293864769550 ) ) ;
#128288=CARTESIAN_POINT ( 'NONE',  ( 5.153800228976615827, -19.02544592524334988, 25.20942372801900433 ) ) ;
#128289=CARTESIAN_POINT ( 'NONE',  ( -4.483927247898782831, 16.52544592524335698, 97.70942372801904696 ) ) ;
#128290=CARTESIAN_POINT ( 'NONE',  ( 16.46253265017160672, -9.564922557960803928, 108.3322429386476955 ) ) ;
#128291=CARTESIAN_POINT ( 'NONE',  ( 5.719274019375673035, 21.55341960407619339, 77.29275706135234714 ) ) ;
#128293=CARTESIAN_POINT ( 'NONE',  ( -17.49999999999999289, -3.189878218039144731, 35.12948562571269662 ) ) ;
#128294=CARTESIAN_POINT ( 'NONE',  ( -10.72451020669870658, -18.67979575497194134, 84.58442372801903275 ) ) ;
#128296=CARTESIAN_POINT ( 'NONE',  ( -13.97604488694527625, -13.89961937509977652, 96.87390960531433848 ) ) ;
#128297=CARTESIAN_POINT ( 'NONE',  ( 19.02544592524334988, 5.153800228976608722, 21.45942372801899012 ) ) ;
#128299=CARTESIAN_POINT ( 'NONE',  ( -13.89961937509977652, 13.97604488694528158, 45.62390960531433848 ) ) ;
#128300=CARTESIAN_POINT ( 'NONE',  ( -10.81492255796078084, -18.62759615963271287, 62.08224293864769550 ) ) ;
#128301=CARTESIAN_POINT ( 'NONE',  ( 16.53943276465976808, -0.05219959533910856209, 23.74890960531435269 ) ) ;
#128302=CARTESIAN_POINT ( 'NONE',  ( -16.55341960407611168, -4.379528057220339221, 91.45724293864769550 ) ) ;
#128303=CARTESIAN_POINT ( 'NONE',  ( -0.05219959533909027116, -19.03943276465977164, 82.49890960531436690 ) ) ;
#128304=CARTESIAN_POINT ( 'NONE',  ( 21.53943276465977519, 0.05219959533937863772, 106.2510903946856757 ) ) ;
#128305=CARTESIAN_POINT ( 'NONE',  ( -9.474510206698964154, 16.51473224551069663, 30.41557627198102054 ) ) ;
#128306=CARTESIAN_POINT ( 'NONE',  ( -4.379528057220328563, 16.55341960407611168, 100.2072429386476955 ) ) ;
#128307=CARTESIAN_POINT ( 'NONE',  ( -10.72451020669870658, -18.67979575497194134, 54.58442372801901143 ) ) ;
#128308=CARTESIAN_POINT ( 'NONE',  ( 0.05219959533907565091, 21.53943276465977519, 89.99890960531438111 ) ) ;
#128309=CARTESIAN_POINT ( 'NONE',  ( -5.153800228976607833, 19.02544592524334988, 57.70942372801899012 ) ) ;
#128311=CARTESIAN_POINT ( 'NONE',  ( 0.05219959533909260263, 19.03943276465977164, 109.9989096053143669 ) ) ;
#128312=CARTESIAN_POINT ( 'NONE',  ( -16.52544592524342804, 4.483927247898546575, 76.04057627198102409 ) ) ;
#128313=CARTESIAN_POINT ( 'NONE',  ( 16.46253265017146816, 9.564922557961045513, 41.66775706135234003 ) ) ;
#128315=CARTESIAN_POINT ( 'NONE',  ( -9.474510206698964154, 16.51473224551069663, 60.41557627198102409 ) ) ;
#128316=CARTESIAN_POINT ( 'NONE',  ( 8.314922557960818139, 14.29746914071049879, 59.58224293864770260 ) ) ;
#128317=CARTESIAN_POINT ( 'NONE',  ( -13.97604488694547697, 13.89961937509957934, 73.12609039468568994 ) ) ;
#128318=EDGE_CURVE ( 'NONE', #141920, #78253, #44226, .T. ) ;
#128319=CARTESIAN_POINT ( 'NONE',  ( -19.52837319214028611, 5.499999999999899636, 84.60471352585540217 ) ) ;
#128320=CARTESIAN_POINT ( 'NONE',  ( 15.80617190586746368, 15.72974639402197994, 39.37390960531436690 ) ) ;
#128322=CARTESIAN_POINT ( 'NONE',  ( -12.06949235617756955, 12.14591786802309770, 100.6239096053143811 ) ) ;
#128324=CARTESIAN_POINT ( 'NONE',  ( -9.564922557960796823, -16.46253265017161027, 57.08224293864769550 ) ) ;
#128325=CARTESIAN_POINT ( 'NONE',  ( 15.80617190586746368, 15.72974639402197994, 64.37390960531435269 ) ) ;
#128326=CARTESIAN_POINT ( 'NONE',  ( 5.153800228976335163, 19.02544592524342804, 29.79057627198102409 ) ) ;
#128327=CARTESIAN_POINT ( 'NONE',  ( -0.05219959533934338120, 16.53943276465976808, 82.50109039468568994 ) ) ;
#128328=CARTESIAN_POINT ( 'NONE',  ( -13.89961937509977652, 13.97604488694528158, 65.62390960531436690 ) ) ;
#128329=CARTESIAN_POINT ( 'NONE',  ( 16.51473224551083163, -9.474510206698727899, 55.83442372801899722 ) ) ;
#128330=CARTESIAN_POINT ( 'NONE',  ( 21.52544592524334988, 5.823673210054432836, 71.45942372801901854 ) ) ;
#128331=CARTESIAN_POINT ( 'NONE',  ( 21.55341960407610458, 5.719274019375980345, 43.95724293864769550 ) ) ;
#128332=CARTESIAN_POINT ( 'NONE',  ( -9.564922557960796823, -16.46253265017161027, 27.08224293864769550 ) ) ;
#128333=CARTESIAN_POINT ( 'NONE',  ( 12.06949235617739724, 12.14591786802326823, 81.87609039468568994 ) ) ;
#128334=CARTESIAN_POINT ( 'NONE',  ( 0.05219959533936267826, -19.03943276465977164, 110.0010903946856757 ) ) ;
#128336=CARTESIAN_POINT ( 'NONE',  ( 18.39639308325437383, 5.500000000000035527, 78.98252246182197212 ) ) ;
#128337=CARTESIAN_POINT ( 'NONE',  ( -0.05219959533937732626, 21.53943276465977519, 97.50109039468567573 ) ) ;
#128338=CARTESIAN_POINT ( 'NONE',  ( -16.52544592524342804, 4.483927247898546575, 46.04057627198103830 ) ) ;
#128339=CARTESIAN_POINT ( 'NONE',  ( 8.314922557960818139, 14.29746914071049879, 54.58224293864769550 ) ) ;
#128340=CARTESIAN_POINT ( 'NONE',  ( -21.52544592524343514, 5.823673210054127303, 101.0405762719810383 ) ) ;
#128341=CARTESIAN_POINT ( 'NONE',  ( 18.67979575497178502, 10.72451020669898547, 94.16557627198103830 ) ) ;
#128342=CARTESIAN_POINT ( 'NONE',  ( 17.44270441346516520, -5.991230190323020288, 96.13664920735770636 ) ) ;
#128343=CARTESIAN_POINT ( 'NONE',  ( -5.823673210054116645, -21.52544592524344225, 32.29057627198102409 ) ) ;
#128344=CARTESIAN_POINT ( 'NONE',  ( 14.29746914071037800, 8.314922557961029526, 71.66775706135234714 ) ) ;
#128345=CARTESIAN_POINT ( 'NONE',  ( -16.53943276465976808, 0.05219959533911058130, 81.24890960531436690 ) ) ;
#128346=CARTESIAN_POINT ( 'NONE',  ( -19.03943276465977164, 0.05219959533909376836, 51.24890960531436690 ) ) ;
#128349=CARTESIAN_POINT ( 'NONE',  ( -16.52544592524335698, -4.483927247898792601, 98.95942372801903275 ) ) ;
#128350=CARTESIAN_POINT ( 'NONE',  ( 10.81492255796078972, 18.62759615963270932, 114.5822429386477097 ) ) ;
#128351=CARTESIAN_POINT ( 'NONE',  ( 9.564922557960805705, 16.46253265017160317, 89.58224293864769550 ) ) ;
#128352=CARTESIAN_POINT ( 'NONE',  ( -21.53943276465977519, -0.05219959533937600094, 48.75109039468568284 ) ) ;
#128353=CARTESIAN_POINT ( 'NONE',  ( 19.02544592524343514, -5.153800228976328945, 103.5405762719809957 ) ) ;
#128357=CARTESIAN_POINT ( 'NONE',  ( 21.52544592524334988, 5.823673210054432836, 51.45942372801901854 ) ) ;
#128358=CARTESIAN_POINT ( 'NONE',  ( 19.02544592524343514, -5.153800228976328945, 33.54057627198102409 ) ) ;
#128359=CARTESIAN_POINT ( 'NONE',  ( 19.05341960407611168, 5.049401038298154454, 113.9572429386477097 ) ) ;
#128360=CARTESIAN_POINT ( 'NONE',  ( -13.97604488694547697, 13.89961937509957934, 58.12609039468566863 ) ) ;
#128361=CARTESIAN_POINT ( 'NONE',  ( -21.55341960407619339, 5.719274019375674811, 33.54275706135234714 ) ) ;
#128362=CARTESIAN_POINT ( 'NONE',  ( 13.97604488694548053, -13.89961937509957401, 60.62609039468564731 ) ) ;
#128363=CARTESIAN_POINT ( 'NONE',  ( -13.97604488694527625, -13.89961937509977652, 21.87390960531435979 ) ) ;
#128364=CARTESIAN_POINT ( 'NONE',  ( -8.314922557961024197, 14.29746914071037800, 97.91775706135236135 ) ) ;
#128365=CARTESIAN_POINT ( 'NONE',  ( 9.564922557961047289, -16.46253265017146816, 65.41775706135233293 ) ) ;
#128366=CARTESIAN_POINT ( 'NONE',  ( 0.05219959533934541429, -16.53943276465976808, 105.0010903946856757 ) ) ;
#128368=CARTESIAN_POINT ( 'NONE',  ( -9.564922557960796823, -16.46253265017161027, 87.08224293864769550 ) ) ;
#128369=CARTESIAN_POINT ( 'NONE',  ( -0.05219959533937732626, 21.53943276465977519, 92.50109039468567573 ) ) ;
#128370=CARTESIAN_POINT ( 'NONE',  ( -0.05219959533937732626, 21.53943276465977519, 107.5010903946856899 ) ) ;
#128372=CARTESIAN_POINT ( 'NONE',  ( -16.51473224551069308, -9.474510206698971260, 101.6655762719810241 ) ) ;
#128373=CARTESIAN_POINT ( 'NONE',  ( 18.62759615963255655, 10.81492255796105972, 71.66775706135234714 ) ) ;
#128374=CARTESIAN_POINT ( 'NONE',  ( -16.46253265017146816, -9.564922557961047289, 109.1677570613523471 ) ) ;
#128375=CARTESIAN_POINT ( 'NONE',  ( -0.05219959533909027116, -19.03943276465977164, 77.49890960531435269 ) ) ;
#128376=CARTESIAN_POINT ( 'NONE',  ( -21.55341960407610458, -5.719274019375992779, 31.45724293864769550 ) ) ;
#128377=CARTESIAN_POINT ( 'NONE',  ( -9.474510206698964154, 16.51473224551069663, 95.41557627198102409 ) ) ;
#128379=CARTESIAN_POINT ( 'NONE',  ( -0.05219959533909027116, -19.03943276465977164, 67.49890960531436690 ) ) ;
#128380=CARTESIAN_POINT ( 'NONE',  ( 12.06949235617757843, -12.14591786802309237, 23.12390960531436335 ) ) ;
#128381=CARTESIAN_POINT ( 'NONE',  ( -18.39639308325437028, -5.500000000000041744, 41.48252246182197212 ) ) ;
#128382=CARTESIAN_POINT ( 'NONE',  ( 16.51473224551083163, -9.474510206698727899, 75.83442372801900433 ) ) ;
#128383=CARTESIAN_POINT ( 'NONE',  ( -5.049401038298153566, 19.05341960407611168, 100.2072429386476955 ) ) ;
#128384=CARTESIAN_POINT ( 'NONE',  ( 16.55341960407611168, 4.379528057220329451, 78.95724293864769550 ) ) ;
#128385=CARTESIAN_POINT ( 'NONE',  ( -18.62759615963270932, 10.81492255796079327, 45.83224293864769550 ) ) ;
#128386=CARTESIAN_POINT ( 'NONE',  ( -18.62759615963270932, 10.81492255796079327, 40.83224293864769550 ) ) ;
#128387=CARTESIAN_POINT ( 'NONE',  ( 8.314922557960818139, 14.29746914071049879, 109.5822429386476955 ) ) ;
#128388=CARTESIAN_POINT ( 'NONE',  ( -16.20579543436675252, 7.371946100355232900, 54.43479165828124167 ) ) ;
#128389=CARTESIAN_POINT ( 'NONE',  ( 9.564922557961047289, -16.46253265017146816, 40.41775706135234003 ) ) ;
#128390=CARTESIAN_POINT ( 'NONE',  ( -0.05219959533910754901, -16.53943276465976808, 22.49890960531436335 ) ) ;
#128391=CARTESIAN_POINT ( 'NONE',  ( -5.153800228976328057, -19.02544592524343514, 102.2905762719810383 ) ) ;
#128392=CARTESIAN_POINT ( 'NONE',  ( -10.72451020669870658, -18.67979575497194134, 69.58442372801900433 ) ) ;
#128393=CARTESIAN_POINT ( 'NONE',  ( -0.05219959533907301413, -21.53943276465977519, 57.49890960531435979 ) ) ;
#128394=CARTESIAN_POINT ( 'NONE',  ( -15.72974639402176322, -15.80617190586768395, 44.37609039468567573 ) ) ;
#128395=CARTESIAN_POINT ( 'NONE',  ( 15.80617190586746368, 15.72974639402197994, 94.37390960531436690 ) ) ;
#128396=CARTESIAN_POINT ( 'NONE',  ( 10.72451020669871369, 18.67979575497193778, 42.08442372801901854 ) ) ;
#128397=CARTESIAN_POINT ( 'NONE',  ( -14.34966873604960291, -8.224510206698953496, 111.6655762719810525 ) ) ;
#128398=CARTESIAN_POINT ( 'NONE',  ( -13.89961937509957401, -13.97604488694547875, 64.37609039468567573 ) ) ;
#128399=CARTESIAN_POINT ( 'NONE',  ( -5.153800228976328057, -19.02544592524343514, 62.29057627198100988 ) ) ;
#128400=CARTESIAN_POINT ( 'NONE',  ( -4.483927247898539470, -16.52544592524342804, 107.2905762719810525 ) ) ;
#128401=CARTESIAN_POINT ( 'NONE',  ( 13.97604488694527802, 13.89961937509977652, 114.3739096053143669 ) ) ;
#128402=CARTESIAN_POINT ( 'NONE',  ( -4.483927247898539470, -16.52544592524342804, 52.29057627198102409 ) ) ;
#128403=CARTESIAN_POINT ( 'NONE',  ( -14.29746914071049879, 8.314922557960819915, 25.83224293864769194 ) ) ;
#128404=CARTESIAN_POINT ( 'NONE',  ( -19.03943276465977164, 0.05219959533909376836, 46.24890960531435979 ) ) ;
#128405=CARTESIAN_POINT ( 'NONE',  ( -12.06949235617756955, 12.14591786802309770, 115.6239096053143669 ) ) ;
#128406=CARTESIAN_POINT ( 'NONE',  ( -19.03943276465977164, -0.05219959533935918106, 28.75109039468566507 ) ) ;
#128409=CARTESIAN_POINT ( 'NONE',  ( 8.224510206698953496, -14.34966873604960469, 32.91557627198102409 ) ) ;
#128410=CARTESIAN_POINT ( 'NONE',  ( -0.05219959533937732626, 21.53943276465977519, 47.50109039468568994 ) ) ;
#128412=CARTESIAN_POINT ( 'NONE',  ( -16.55341960407617563, 4.379528057220093196, 63.54275706135234003 ) ) ;
#128413=CARTESIAN_POINT ( 'NONE',  ( -16.53943276465976808, 0.05219959533911058130, 31.24890960531435979 ) ) ;
#128414=CARTESIAN_POINT ( 'NONE',  ( -16.53943276465976808, -0.05219959533934237506, 103.7510903946857042 ) ) ;
#128415=CARTESIAN_POINT ( 'NONE',  ( -0.05219959533909027116, -19.03943276465977164, 32.49890960531435979 ) ) ;
#128416=CARTESIAN_POINT ( 'NONE',  ( 5.049401038298161559, -19.05341960407611168, 57.70724293864769550 ) ) ;
#128417=CARTESIAN_POINT ( 'NONE',  ( -9.474510206698964154, 16.51473224551069663, 30.41557627198102054 ) ) ;
#128418=CARTESIAN_POINT ( 'NONE',  ( -10.81492255796105439, 18.62759615963255655, 32.91775706135234714 ) ) ;
#128419=CARTESIAN_POINT ( 'NONE',  ( 5.153800228976335163, 19.02544592524342804, 49.79057627198100988 ) ) ;
#128421=CARTESIAN_POINT ( 'NONE',  ( 5.049401038298161559, -19.05341960407611168, 37.70724293864768839 ) ) ;
#128422=CARTESIAN_POINT ( 'NONE',  ( 16.51473224551069308, 9.474510206698969483, 114.1655762719810241 ) ) ;
#128423=CARTESIAN_POINT ( 'NONE',  ( -5.719274019375665041, -21.55341960407619695, 64.79275706135234714 ) ) ;
#128424=CARTESIAN_POINT ( 'NONE',  ( -12.06949235617756955, 12.14591786802309770, 105.6239096053143669 ) ) ;
#128425=CARTESIAN_POINT ( 'NONE',  ( 16.46253265017160672, -9.564922557960803928, 113.3322429386476955 ) ) ;
#128426=CARTESIAN_POINT ( 'NONE',  ( -16.53943276465976808, -0.05219959533934237506, 78.75109039468568994 ) ) ;
#128427=CARTESIAN_POINT ( 'NONE',  ( 0.05219959533937995610, -21.53943276465977519, 90.00109039468567573 ) ) ;
#128428=CARTESIAN_POINT ( 'NONE',  ( -0.05219959533934338120, 16.53943276465976808, 47.50109039468568994 ) ) ;
#128429=CARTESIAN_POINT ( 'NONE',  ( -19.03943276465977164, 0.05219959533909376836, 91.24890960531436690 ) ) ;
#128430=CARTESIAN_POINT ( 'NONE',  ( -12.06949235617739369, -12.14591786802326823, 34.37609039468568284 ) ) ;
#128431=CARTESIAN_POINT ( 'NONE',  ( -16.53943276465976808, -0.05219959533934237506, 23.75109039468567929 ) ) ;
#128432=CARTESIAN_POINT ( 'NONE',  ( 4.483927247898790824, -16.52544592524335698, 80.20942372801901854 ) ) ;
#128433=CARTESIAN_POINT ( 'NONE',  ( 13.97604488694548053, -13.89961937509957401, 105.6260903946856757 ) ) ;
#128434=CARTESIAN_POINT ( 'NONE',  ( 9.564922557960805705, 16.46253265017160317, 79.58224293864769550 ) ) ;
#128435=CARTESIAN_POINT ( 'NONE',  ( 5.823673210054125526, 21.52544592524343514, 94.79057627198105251 ) ) ;
#128436=CARTESIAN_POINT ( 'NONE',  ( -8.314922557960811034, -14.29746914071050412, 107.0822429386476955 ) ) ;
#128437=CARTESIAN_POINT ( 'NONE',  ( 5.153800228976615827, -19.02544592524334988, 110.2094237280189901 ) ) ;
#128438=CARTESIAN_POINT ( 'NONE',  ( 16.55341960407618274, -4.379528057220086978, 76.04275706135237556 ) ) ;
#128440=CARTESIAN_POINT ( 'NONE',  ( -19.03943276465977164, -0.05219959533935918106, 63.75109039468566863 ) ) ;
#128441=CARTESIAN_POINT ( 'NONE',  ( 8.314922557960818139, 14.29746914071049879, 44.58224293864769550 ) ) ;
#128442=CARTESIAN_POINT ( 'NONE',  ( 14.34966873604960469, 8.224510206698951720, 89.16557627198102409 ) ) ;
#128443=CARTESIAN_POINT ( 'NONE',  ( 13.89961937509957401, 13.97604488694547697, 31.87609039468566863 ) ) ;
#128445=CARTESIAN_POINT ( 'NONE',  ( 10.81492255796106328, -18.62759615963255655, 40.41775706135234714 ) ) ;
#128446=CARTESIAN_POINT ( 'NONE',  ( -19.03943276465977164, -0.05219959533935918106, 98.75109039468567573 ) ) ;
#128447=( BOUNDED_SURFACE ( )  B_SPLINE_SURFACE ( 3, 2, ( 
 ( #127359, #7000, #69691, #159690, #146518, #175878, #100013, #51526, #24204, #84839, #116197, #129346, #173895, #85853, #130337, #114175, #145520, #189072, #131358, #191041, #113189, #8008, #68682, #177886, #144523, #174878, #192035, #21188, #193047, #52514, #54524, #53517, #4016, #39355, #65694, #82844, #38358, #50544, #115195, #176887, #112205, #6008, #36344, #160699, #22190, #101014, #35364, #162699, #67688, #97016, #158697, #97997, #37350, #99008, #5008, #161699, #23196, #20186, #83838, #81832, #143519, #128353, #190051, #178887, #56528, #106004, #73705, #132367, #10032, #135377, #26206, #42364, #87845, #55521, #9030, #165706, #197047, #71692, #148541, #58515, #134376, #104027, #179897, #27203, #89849, #120181, #57535, #133359, #195049, #105021, #74686, #119204, #181871, #40355, #117194, #72703, #118206, #88849, #136352, #150541, #12041, #41363, #103029, #102030, #43350, #59496, #166705, #28208, #151532, #13021, #198028, #86857, #196062, #121171, #164711, #149533, #182865, #44346, #11028, #167691, #147542, #180889, #194060, #163712, #29188, #70699, #25215, #45339, #155494, #77654, #122162, #124147, #140315, #172655, #183851, #94809, #141312, #2801, #75661, #137338, #139322, #125159, #76657, #32157, #107981, #138336, #170669, #186858, #62475, #802, #199018, #185846, #31164, #60487, #152505, #108988, #1805, #14997, #91808, #16986, #47333, #93814, #123154, #78640, #33151, #63483, #48327, #171662, #200016, #30164, #13994, #61483, #109982, #156488, #46327, #187842, #153500, #184842, #17990, #79643, #106991, #169669, #168664, #92814, #110971, #64479, #154501, #126146, #49311, #90822, #15996, #192808, #99781, #84604, #145285, #83606, #36113, #97765, #143284, #173662, #142304, #113939, #176651, #175638, #3784, #53279, #130101, #66457, #146283, #21956, #6768, #69453, #158470, #65461, #20948, #112955, #35129, #68447, #98771, #18981, #159452, #160465, #129108, #96781, #7770, #127124, #4770, #54290, #191798, #80627, #19958, #114958, #38127, #188830, #161466, #131120, #22956, #50314, #115962, #128119, #82605, #37112, #34143, #95802, #81600, #157488, #111970, #5775, #144286, #189822, #51294, #174648, #67450, #190807, #52281, #163474, #180656, #74454, #179657, #27971, #41127, #148300, #100774, #194810, #70459, #197796, #133121, #164477, #165473, #117966, #56284, #59262, #134136, #25971, #177650, #40108, #149300, #89611, #11805, #43117, #87614, #42132, #151300, #195825, #101786, #24971, #150308, #162457, #9794, #178645, #23958, #103793, #104785, #102791, #119952, #10794, #73469, #86617, #39118, #58283, #12789, #72462, #147300, #85613, #26969, #57296, #118973, #8789, #166473, #88612, #71456, #181637, #135142, #136120, #196816, #132124, #193817, #55282, #116953, #48819, #112462, #173157, #120931, #35625, #182630, #2300, #157978, #5274, #126627, #188328, #108490, #79139, #171166, #80133, #141803, #50804, #143791, #97270, #187349, #174154, #127627, #155985, #49807, #16492, #34632, #94307, #110472, #64968, #46830, #111472, #62975, #65956, #158958, #95302, #172154, #78141, #31662, #189327, #20448, #17482, #156986, #109483, #96291, #82099, #125652, #170169, #33640, #140810, #93312, #63982, #139809, #154996, #18484, #3296, #19470, #81115, #142795, #1297, #4275, #124655, #186351, #47831, #32653, #117460, #101276, #132633, #177156, #69964, #40627, #85107, #191301, #52777, #39617, #190310, #37617, #67951, #51786, #131630, #194321, #22460, #9299, #38629, #162966, #114446, #87125, #147813, #179159, #192312, #36606, #148810, #193314, #100286, #8286, #113446, #55789, #53792, #176147, #70965, #54788, #102297, #7269, #99279, #116463, #84108, #163986, #115467, #25483, #178152, #66955, #128617, #175139, #145787, #24472, #98263, #86122, #159965, #21452, #68953, #160966, #23460, #146793, #83113, #144790, #6273, #130616, #129605, #161964, #42628, #197307, #89118, #11306, #59765, #74944, #195322, #135637, #136607, #105280 ),
 ( #181153, #58771, #151789, #30428, #13280, #149800, #152765, #45598, #182132, #120439, #164979, #118475, #14255, #184116, #104292, #43616, #196331, #198287, #107251, #12302, #60751, #73968, #165973, #133630, #27475, #103300, #92075, #150806, #166968, #121433, #28470, #90105, #10300, #183126, #44609, #71957, #72976, #106264, #122424, #167948, #75926, #29446, #91078, #168922, #137601, #134645, #57799, #199284, #56802, #180165, #119470, #41635, #26474, #88116, #109244, #96063, #125420, #49572, #1060, #173924, #34405, #65723, #78899, #123408, #35393, #79905, #63746, #95070, #76917, #80890, #140577, #62734, #157751, #156758, #127391, #94070, #124416, #18252, #170924, #142567, #2067, #4046, #3064, #153764, #189101, #15259, #32415, #188099, #138588, #141576, #64741, #69, #155749, #186110, #110240, #171921, #50574, #61740, #112234, #17247, #185101, #19243, #47591, #187116, #48588, #154759, #126403, #111235, #46590, #33411, #172926, #108251, #16257, #169931, #31422, #93074, #77908, #139575, #81864, #159724, #23227, #177918, #51556, #39386, #9061, #161732, #190080, #146548, #6040, #55553, #84870, #143553, #21221, #8042, #101045, #113220, #162731, #70731, #69723, #174910, #131390, #67719, #22222, #38390, #117226, #100046, #36374, #24237, #132398, #68713, #83871, #98028, #5038, #85887, #194091, #129376, #130370, #82877, #193079, #178920, #99040, #147575, #160730, #191073, #20216, #114207, #144555, #97044, #52546, #145553, #54554, #37383, #175912, #158726, #53549, #7031, #66724, #192067, #115227, #128384, #116227, #176919, #150574, #43380, #14023, #58546, #164743, #26238, #13052, #163746, #11061, #41396, #25246, #105052, #106034, #196096, #182894, #12073, #136382, #87877, #60517, #121202, #152536, #165738, #10062, #122192, #166736, #73735, #181902, #86887, #167720, #27233, #149565, #44378, #28240, #75689, #180920, #72737, #89880, #57566, #29218, #88882, #90851, #151563, #40388, #137368, #102061, #119236, #74719, #148572, #198059, #59525, #71722, #42395, #134410, #197079, #120212, #199047, #133391, #195082, #104058, #56562, #118238, #135408, #179929, #103061, #184872, #33181, #48357, #168694, #109018, #110011, #78670, #46354, #34172, #15027, #156520, #76688, #153530, #170697, #154528, #63516, #111001, #186887, #140346, #92843, #139351, #138364, #1834, #95833, #141344, #2831, #126176, #187871, #171692, #123183, #32186, #94840, #16025, #62505, #18020, #125191, #77683, #172687, #183884, #124176, #30195, #91837, #79673, #108012, #107022, #200045, #64509, #93843, #61514, #17017, #49339, #65491, #169697, #157517, #19011, #80657, #31191, #831, #155522, #142333, #185877, #3813, #47363, #45369, #6800, #161498, #98803, #175669, #35159, #21987, #67481, #96814, #188861, #145317, #176683, #51325, #128152, #53311, #113971, #83639, #159484, #68478, #69486, #38158, #37144, #7802, #112986, #66489, #50344, #174679, #130133, #191830, #82635, #23989, #189852, #36144, #99812, #192840, #158500, #144318, #81630, #143313, #147332, #114989, #4800, #22988, #100805, #160497, #115992, #85646, #54320, #177681, #84636, #146313, #129140, #190837, #97796, #20978, #19987, #131151, #39149, #162488, #5807, #8820, #127153, #52313, #112003, #173692, #119980, #105802, #194842, #101817, #180686, #56316, #117998, #28001, #197825, #42162, #182659, #89641, #151329, #12817, #74484, #135172, #9825, #57327, #181666, #179687, #149329, #43145, #26998, #41159, #59291, #70489, #10823, #116984, #178677, #104814, #102822, #193848, #25003, #196845, #119003, #163505, #103822, #166503, #152307, #86647, #136150, #120960, #44143, #55313, #40140, #165502, #167489, #164507, #11835, #87643, #26001, #150339, #28984, #88643, #73500, #148330, #58312, #72493, #71486, #132155, #90625, #133152, #134167, #195855, #140100, #590, #170455, #46116, #93600, #156276, #63266, #62261, #94597, #138128, #153290, #75458, #61276, #155286, #31946, #169455, #110763, #76451, #122947 ),
 ( #172444, #79432, #64270, #124947, #186643, #15783, #77442, #184635, #14791, #121957, #16776, #17777, #78425, #183650, #32942, #109770, #107769, #125936, #1591, #48114, #49105, #199809, #45133, #123929, #30956, #92603, #171454, #141103, #185627, #2591, #106791, #168465, #139114, #154293, #187635, #33932, #95590, #13793, #47119, #108777, #29963, #137132, #198819, #60284, #91601, #35908, #158261, #6557, #21746, #142089, #82393, #83397, #52076, #19751, #7558, #188619, #66249, #115757, #145075, #3575, #81392, #68235, #37912, #111760, #99572, #69244, #129888, #50100, #191588, #127909, #144081, #98562, #177445, #160256, #96573, #161254, #192600, #128900, #5562, #173449, #65253, #22748, #130910, #189611, #190599, #143078, #53067, #54083, #159242, #38915, #20737, #51085, #80417, #174438, #34917, #157274, #112745, #67241, #114745, #97554, #113732, #18770, #175429, #36898, #126913, #4557, #176439, #84397, #146073, #166262, #10588, #103590, #74249, #118763, #24764, #86411, #73264, #23753, #71253, #101572, #85403, #165265, #27761, #56076, #42912, #72249, #196610, #148096, #120722, #181434, #12584, #25767, #70254, #182421, #26759, #133927, #41924, #147095, #89404, #87413, #9587, #104578, #88399, #135918, #40915, #132917, #150093, #117757, #151093, #149098, #197589, #11596, #100572, #59055, #162254, #179449, #134933, #8579, #58081, #119751, #131922, #102588, #194604, #57089, #180452, #193606, #55078, #116748, #164272, #178438, #39906, #195617, #163262, #76204, #123683, #186396, #93354, #30712, #124699, #168223, #183407, #105563, #91352, #185382, #349, #199564, #140854, #106547, #153044, #155040, #109526, #75220, #61033, #198578, #60047, #64024, #138869, #121714, #62019, #17525, #15542, #32698, #2343, #171208, #94349, #16535, #78182, #45875, #107528, #14544, #44890, #152069, #46873, #47873, #108533, #13554, #63020, #139851, #137883, #156028, #31705, #1340, #79184, #29720, #136892, #154047, #122705, #184395, #125694, #43900, #77200, #167249, #169205, #92361, #170212, #28748, #90384, #114490, #190353, #143835, #96333, #142838, #141846, #5315, #99326, #144831, #6315, #129647, #191343, #51830, #126668, #174197, #36650, #158020, #66000, #160008, #66999, #19511, #176192, #187393, #127669, #33682, #95344, #21496, #111513, #110516, #3337, #113489, #35665, #18527, #20492, #98308, #71749, #80174, #52821, #37661, #163772, #172197, #157029, #97313, #83157, #173199, #128658, #4317, #34675, #175183, #67994, #158999, #82141, #65011, #25273, #189369, #188372, #48861, #86915, #148598, #81156, #49849, #10090, #50846, #112503, #72766, #195108, #180945, #74744, #89905, #88910, #30222, #196121, #42421, #44406, #199075, #164769, #150602, #87905, #149592, #153557, #28267, #11089, #151588, #107048, #105080, #122219, #91864, #60544, #183910, #106060, #182923, #135434, #197105, #104084, #134436, #41422, #13077, #75716, #136407, #103088, #152561, #29244, #165766, #45395, #121230, #167746, #168720, #57591, #26264, #43409, #119261, #27261, #90877, #15055, #166766, #14050, #12099, #73762, #58572, #120237, #198085, #133419, #59552, #137394, #181928, #56591, #118265, #179955, #188894, #34202, #95865, #19041, #80688, #141375, #16053, #63545, #126206, #185906, #155551, #49371, #33212, #47392, #65523, #76715, #17045, #123209, #184899, #111033, #859, #200072, #31220, #2862, #125219, #108040, #110044, #187902, #158530, #169726, #142364, #127183, #50375, #61540, #46381, #186916, #172720, #62533, #18052, #93873, #124206, #156552, #157547, #48387, #171724, #92870, #94871, #78699, #154557, #138391, #79705, #3844, #109046, #77711, #64540, #112035, #173723, #170724, #35191, #96845, #139377, #32216, #140376, #1863, #67512, #174708, #113999, #191858, #82665, #68506, #144349, #36172, #81661, #159513, #66519, #115019, #21009, #5836, #37173, #129169, #190866, #20018, #175697, #52343, #143344, #97824, #98832, #53340, #145346, #4832, #160527, #22016 ),
 ( #83668, #113015, #6828, #130161, #128182, #189880, #51355, #172360, #173369, #93523, #170378, #125858, #171377, #80337, #127829, #3498, #157196, #109695, #156196, #155208, #18690, #112668, #158184, #19674, #142999, #4477, #65174, #140021, #187558, #50017, #32864, #79353, #34839, #142009, #94514, #189535, #514, #141024, #47042, #108699, #96494, #124867, #123850, #16697, #126833, #49025, #31869, #33850, #111682, #82311, #78347, #66167, #51007, #174360, #185548, #1510, #110680, #81316, #186566, #188539, #17696, #48039, #35830, #97476, #95510, #159162, #63187, #20657, #2511, #64191, #62186, #162173, #193524, #68157, #144996, #70173, #130829, #100494, #176359, #23671, #86331, #54999, #192520, #24682, #129809, #36816, #148018, #194524, #55996, #128822, #190521, #54003, #178359, #191508, #85319, #161172, #52985, #147011, #39823, #115677, #177365, #51995, #38836, #84316, #113654, #5482, #8496, #116668, #114663, #6477, #131841, #101489, #163178, #37832, #9507, #71173, #132837, #117674, #179371, #99492, #83319, #67165, #22669, #40833, #102506, #145995, #164190, #7478, #69162, #25688, #144001, #175348, #98482, #160175, #21665, #193795, #163453, #115941, #192786, #195806, #132104, #162437, #57278, #38104, #147279, #25952, #9774, #41107, #85592, #178625, #149281, #55263, #99759, #161443, #148281, #98751, #146261, #176629, #160444, #40088, #102771, #131098, #117947, #8769, #71438, #22935, #175616, #56264, #87595, #100755, #145264, #37092, #101766, #70438, #116932, #21934, #164458, #23938, #84581, #179637, #24951, #10776, #177631, #7745, #86598, #54269, #72441, #133102, #134117, #194791, #83585, #6746, #68425, #39099, #130077, #191776, #53258, #114936, #69431, #74433, #166455, #75411, #137083, #46068, #139065, #30909, #182610, #107722, #122898, #151280, #105753, #197776, #61227, #121908, #92557, #59242, #89593, #60237, #136100, #169403, #44095, #154245, #168417, #118952, #15736, #180638, #120911, #153239, #543, #183601, #45085, #103775, #167439, #27952, #198771, #106742, #77395, #42113, #165454, #28936, #26951, #184587, #12769, #90577, #152258, #119934, #29912, #91552, #88593, #13743, #14742, #76403, #181619, #150291, #11786, #138079, #73450, #199760, #135123, #43098, #196797, #58265, #104767, #4509, #174392, #126865, #155239, #111714, #32896, #187590, #3530, #82344, #65206, #1543, #66199, #97508, #33885, #49059, #16729, #170408, #127862, #35862, #94548, #95542, #48070, #188572, #159194, #64225, #112700, #125890, #156229, #185580, #79388, #50052, #20689, #17730, #80369, #173400, #2543, #141057, #144033, #18722, #110714, #62214, #124899, #157230, #123882, #96525, #189566, #172396, #34871, #47071, #142042, #186598, #109726, #158215, #108731, #19705, #63219, #31900, #81347, #51038, #143031, #93553, #78377, #140053, #171410, #25717, #86361, #117703, #130860, #175379, #87363, #131871, #115708, #147042, #128853, #132866, #192551, #114697, #146026, #113684, #67195, #23701, #55028, #129841, #6509, #193556, #54034, #162203, #37865, #85349, #148046, #116698, #177396, #9536, #191540, #145028, #190553, #53017, #8526, #70204, #161206, #102537, #68189, #176391, #178388, #71203, #36848, #22701, #100524, #38868, #163208, #5515, #83352, #39852, #179399, #101518, #194555, #164220, #56025, #40863, #24712, #52026, #7509, #69193, #99524, #84348, #98514, #160208, #21698, #93061, #118711, #170911, #47580, #184102, #2056, #139564, #1048, #187106, #75913, #180401, #61728, #137587, #199270, #109232, #78887, #123396, #124405, #41873, #103540, #76904, #122411, #31410, #140566, #154748, #108238, #60738, #107237, #165215, #169918, #63734, #32404, #94059, #155737, #17235, #16245, #88349, #138575, #62721, #45584, #30414, #186098, #77896, #168908, #125409, #149048, #92062, #195564, #57038, #48576, #153750, #72200, #26710, #110229, #54, #150042, #185088, #171910, #33398, #11547, #10536, #133874, #15245, #46577, #141564, #143537 ),
 ( #145537, #126391, #4033, #53534, #21205, #79894, #157740, #82862, #175895, #49559, #37367, #7016, #159707, #188088, #144539, #65711, #20203, #36360, #115211, #98012, #34394, #99025, #130353, #66708, #81849, #111222, #3053, #160715, #68698, #127377, #128370, #80878, #6025, #192052, #97032, #176904, #158713, #189088, #18241, #112222, #67704, #95057, #50562, #113206, #129362, #35381, #173912, #156747, #51542, #5024, #64730, #19229, #190066, #172915, #191058, #22206, #174894, #52530, #96052, #114191, #142555, #83856, #11043, #161717, #9044, #39370, #23212, #41378, #104041, #194075, #180903, #10046, #134392, #85870, #58530, #119218, #150558, #163729, #8025, #120196, #164726, #148555, #179912, #84855, #165721, #25230, #147559, #42378, #103044, #12057, #178903, #70714, #26220, #55538, #27217, #86871, #88865, #87860, #38375, #73719, #100030, #117210, #72719, #146532, #149548, #196078, #69707, #40371, #132382, #195064, #56544, #135392, #131374, #197062, #102045, #193062, #54538, #71706, #133374, #118221, #101029, #57549, #116211, #177901, #162714, #24220, #78655, #75675, #200031, #169683, #122177, #199033, #1820, #138350, #168679, #63501, #44362, #153515, #32172, #16011, #47348, #91822, #184856, #155508, #61499, #106019, #167706, #154514, #105036, #152520, #182879, #166720, #46340, #109004, #137353, #124161, #15012, #77668, #29202, #181886, #62490, #93828, #107006, #151546, #43364, #107996, #76673, #123168, #28224, #170683, #30179, #90836, #185862, #31178, #17003, #183869, #14008, #92829, #60502, #140330, #139337, #89864, #816, #13036, #74702, #136366, #45354, #198043, #59510, #121186, #128137, #109997, #80642, #172672, #81616, #143299, #52297, #145301, #37128, #188846, #113954, #129124, #157503, #111986, #3799, #126162, #174663, #189837, #171677, #50330, #51310, #19973, #187857, #175654, #156503, #34157, #83624, #112971, #33167, #49326, #36128, #5792, #79659, #67465, #98788, #97780, #18005, #159468, #95818, #173677, #66475, #6784, #20963, #64495, #190822, #160482, #96798, #35144, #141328, #94826, #21972, #125176, #18996, #158485, #110987, #82620, #186873, #127139, #48343, #4785, #142319, #2816, #65477, #144302, #150323, #71470, #133135, #53295, #23974, #115977, #24986, #86631, #195838, #88627, #180669, #132140, #57311, #72477, #100789, #55297, #147315, #69469, #117981, #194826, #114974, #193833, #56299, #163488, #131136, #118986, #85629, #25984, #103806, #148314, #102805, #40123, #116969, #176667, #9809, #8805, #38143, #130117, #179671, #41142, #192824, #54305, #164491, #178660, #87627, #162472, #149313, #10807, #134150, #101801, #42146, #177666, #7786, #191814, #39134, #165486, #26982, #70474, #68463, #99797, #161483, #22971, #84619, #146298, #28967, #106774, #198803, #169437, #11818, #89624, #29945, #185611, #183634, #572, #170438, #77427, #62243, #122930, #61260, #13774, #75442, #120944, #151312, #119964, #91583, #154277, #153274, #181650, #30941, #107754, #44127, #123912, #199793, #184617, #47100, #136132, #43129, #121941, #197808, #59274, #92588, #139098, #45116, #46099, #104798, #166487, #137117, #182643, #14775, #108761, #76435, #168449, #105786, #167472, #27985, #138112, #31929, #15767, #93583, #73483, #135155, #196828, #12801, #60268, #58296, #90609, #152290, #74467, #67223, #140082, #1574, #3557, #189593, #32924, #172426, #112727, #190581, #34900, #51066, #126895, #65235, #63249, #50082, #95572, #124928, #16758, #173430, #4537, #79416, #156257, #81374, #142071, #111742, #187618, #96555, #97536, #66230, #188601, #35889, #141086, #94579, #78406, #2572, #158242, #19733, #110745, #52057, #17760, #64253, #127890, #20718, #186626, #33915, #143059, #174420, #159223, #155269, #125920, #82375, #128881, #144063, #5544, #113713, #175410, #36878, #48097, #109753, #157258, #18753, #49088, #80399, #171437, #178417, #40892, #39881, #68218, #117732, #194583, #130891, #149076, #86390, #148074, #133903 ),
 ( #21727, #25745, #85380, #7538, #102565, #101548, #72228, #38896, #69223, #163240, #54064, #87391, #23731, #10564, #9565, #98544, #195594, #160237, #177425, #132894, #180429, #24740, #71231, #83380, #115738, #146054, #55057, #116728, #57066, #118741, #145057, #162232, #6538, #164250, #192581, #147073, #100553, #99553, #56053, #179427, #129870, #191568, #53047, #8557, #70233, #114727, #131901, #176420, #193585, #37895, #161235, #22729, #84377, #103568, #120701, #76184, #123664, #44871, #106527, #26737, #197567, #89381, #198556, #60026, #169185, #61998, #154028, #105543, #30691, #45856, #74227, #28727, #182400, #42891, #91332, #168204, #88376, #167229, #29701, #136871, #104556, #121693, #138850, #41902, #58059, #153024, #150070, #166238, #14523, #122686, #196589, #184375, #15523, #137864, #134912, #199544, #12561, #90364, #183389, #165243, #61014, #181413, #107509, #77180, #13534, #152049, #119730, #11575, #92342, #330, #135895, #75200, #27738, #73241, #151070, #43878, #59034, #187372, #156008, #108512, #2322, #49830, #82122, #79162, #3318, #173179, #125674, #64004, #5296, #141825, #172177, #66979, #47853, #157008, #35647, #19492, #50827, #95323, #188352, #158980, #64991, #109506, #171188, #158000, #170191, #17505, #186374, #31685, #111494, #112484, #140833, #127649, #18506, #81137, #32677, #185361, #65980, #97294, #110495, #155019, #46852, #34655, #80154, #126649, #93334, #174177, #33662, #94330, #78163, #16515, #96314, #48841, #142818, #20472, #4298, #189349, #143814, #139831, #1320, #62999, #124677, #86147, #147838, #70989, #132657, #193338, #67974, #115492, #178176, #37640, #7293, #101302, #85133, #99304, #117485, #128639, #68977, #175164, #36630, #162991, #52801, #51810, #83136, #54812, #177180, #159988, #161988, #39641, #10323, #21475, #194345, #179183, #40651, #113469, #98287, #38653, #24496, #6295, #145810, #9324, #164010, #8312, #55813, #100310, #23484, #144812, #146817, #130642, #129628, #190333, #69988, #102320, #114468, #191323, #116487, #131656, #25506, #160989, #87150, #148833, #176170, #22483, #84131, #192336, #53817, #133653, #119493, #13300, #28491, #27498, #168943, #134667, #181175, #183147, #137623, #103322, #89140, #166988, #58794, #29468, #71979, #149822, #90125, #45620, #43638, #60774, #30450, #199307, #122446, #44632, #121455, #73990, #135659, #42652, #11328, #180189, #151809, #14280, #74965, #41659, #91101, #167969, #104314, #184138, #59787, #106284, #107272, #196353, #165002, #182153, #57821, #165997, #152789, #92097, #105301, #75949, #153785, #26496, #195344, #56824, #136627, #88138, #118498, #150828, #197331, #198308, #72999, #12325, #120462, #157775, #50596, #187139, #2090, #169952, #123429, #19266, #189124, #186135, #48611, #1083, #18274, #112255, #17270, #65746, #78923, #47614, #138609, #32439, #79927, #173947, #109268, #33433, #3087, #155772, #94093, #35414, #171944, #63770, #97066, #77930, #110263, #127414, #49594, #80912, #125443, #141600, #15280, #95092, #139597, #62758, #188123, #91, #170947, #16278, #61761, #64763, #142589, #140600, #4068, #156781, #111257, #124439, #76940, #96086, #185122, #126425, #46612, #108274, #172949, #34427, #31443, #93097, #154781, #148344, #70503, #103839, #164522, #135189, #101831, #132171, #102836, #116998, #88660, #86660, #150356, #10840, #158748, #73518, #20237, #40155, #195872, #43164, #26015, #87659, #143577, #178693, #8835, #118012, #179701, #11853, #181683, #196863, #25017, #58329, #165520, #193862, #9840, #163518, #162503, #72510, #149344, #5060, #71499, #134185, #56330, #24004, #41173, #119997, #81885, #177694, #57345, #66745, #85660, #119020, #131165, #180703, #42179, #192855, #133166, #55327, #27016, #54334, #116005, #39162, #100820, #194857, #147347, #108792, #137148, #91618, #183666, #105819, #154309, #169470, #89660, #29979, #30971, #199825, #167506, #122963, #1606, #186659, #120977, #92618, #151346, #29001, #15798 ),
 ( #47134, #140115, #76468, #153306, #59308, #12835, #170471, #78441, #75475, #138145, #90641, #107785, #63282, #106807, #155301, #168481, #198836, #28018, #121974, #77458, #124962, #60300, #184650, #139129, #45151, #14807, #104831, #61293, #46132, #166520, #152323, #606, #16791, #62276, #31961, #123944, #185642, #74501, #93616, #13809, #136167, #197842, #182675, #44159, #49121, #171469, #51100, #113747, #3590, #190615, #19766, #144095, #95605, #68251, #128914, #160270, #173463, #17792, #129902, #174453, #158277, #189626, #32957, #175443, #34936, #157290, #52090, #112760, #21760, #188635, #18787, #35922, #65268, #36913, #96588, #98576, #97568, #48129, #83412, #109786, #126928, #82407, #127924, #145089, #159256, #81407, #6572, #172460, #187650, #94612, #80432, #20752, #4572, #50115, #156291, #110778, #142105, #5576, #79448, #141118, #111775, #143093, #66264, #67256, #2608, #125952, #64285, #33947, #163277, #180466, #150109, #57104, #41938, #102602, #40930, #193620, #55091, #100585, #130923, #99586, #71267, #133941, #132931, #161267, #10602, #87427, #23767, #103604, #179465, #164288, #26773, #115770, #22761, #101589, #177458, #38928, #149112, #118778, #24778, #25781, #84410, #146087, #116762, #162267, #194619, #165280, #56090, #148111, #85417, #147108, #7571, #9602, #88414, #72264, #195631, #11610, #73278, #117771, #192614, #178453, #191602, #8594, #70268, #53081, #114759, #131936, #176453, #37926, #39920, #69257, #54096, #86425, #59069, #58095, #89418, #199580, #121729, #166277, #168239, #184410, #16550, #27775, #138884, #185397, #46888, #119765, #181449, #183421, #169220, #12599, #152083, #92376, #170227, #14561, #30729, #106562, #44905, #42927, #29735, #75235, #104591, #196626, #153059, #45891, #120736, #135933, #61048, #91368, #76219, #167263, #77215, #137898, #154062, #182435, #155055, #15557, #108548, #60061, #151107, #134948, #122720, #107544, #364, #74263, #62035, #123699, #43915, #31720, #93368, #197603, #136906, #105577, #28762, #90399, #13568, #198593, #67015, #127684, #78197, #190371, #139867, #157045, #112519, #160024, #81171, #142853, #63035, #33697, #125710, #34691, #96348, #5331, #98324, #51846, #141861, #128674, #82156, #110532, #65027, #18542, #79201, #189384, #4332, #124713, #3352, #66016, #173215, #140870, #158035, #175200, #1356, #94364, #50861, #186411, #2359, #174213, #159015, #32712, #20508, #113505, #35681, #171223, #97329, #48877, #126683, #19526, #47888, #143852, #17540, #36665, #109541, #49864, #188387, #156043, #64040, #187409, #172213, #95360, #111530, #80189, #24530, #118533, #23519, #72014, #85165, #192370, #144846, #38688, #86181, #180222, #115527, #39673, #9357, #162023, #100344, #41692, #178209, #8346, #103357, #84164, #193371, #133687, #55845, #87185, #131690, #147871, #195380, #101335, #145844, #7326, #194378, #6329, #53853, #22517, #68009, #71022, #148866, #177215, #10357, #54847, #132690, #56858, #163024, #69010, #130676, #117519, #129661, #146853, #70021, #191357, #179217, #21511, #116521, #164042, #40683, #102353, #25541, #83172, #52835, #114504, #176206, #37675, #99340, #161023, #167021, #136661, #88172, #137653, #43671, #89172, #14315, #198342, #184169, #58828, #150864, #59817, #74021, #199340, #105333, #60805, #183181, #165035, #45651, #149856, #120495, #29498, #26528, #44663, #106316, #134703, #182186, #135691, #121487, #168002, #107302, #11361, #30479, #28522, #168974, #73031, #90158, #74996, #151841, #197363, #75980, #91131, #181210, #13331, #152821, #122478, #196386, #57855, #119527, #42686, #104347, #166031, #12358, #27531, #71673, #26187, #99995, #87827, #57518, #10013, #38339, #195031, #116177, #70682, #86837, #165687, #148523, #84820, #149513, #180871, #117174, #132348, #161680, #53500, #11010, #119186, #177867, #178869, #131340, #133340, #42347, #147526, #196043, #9014, #39336, #68664, #162680, #56508, #104009, #100995, #163693, #118186, #85836 ) ),
 .UNSPECIFIED., .T., .F., .T. ) 
 B_SPLINE_SURFACE_WITH_KNOTS ( ( 4, 3, 4 ),
 ( 3, 2, 2, 2, 2, 2, 2, 2, 2, 2, 2, 2, 2, 2, 2, 2, 2, 2, 2, 2, 2, 2, 2, 2, 2, 2, 2, 2, 2, 2, 2, 2, 2, 2, 2, 2, 2, 2, 2, 2, 2, 2, 2, 2, 2, 2, 2, 2, 2, 2, 2, 2, 2, 2, 2, 2, 2, 2, 2, 2, 2, 2, 2, 2, 2, 2, 2, 2, 2, 2, 2, 2, 2, 2, 2, 2, 2, 2, 2, 2, 2, 2, 2, 2, 2, 2, 2, 2, 2, 2, 2, 2, 2, 2, 2, 2, 2, 2, 2, 2, 2, 2, 2, 2, 2, 2, 2, 2, 2, 2, 2, 2, 2, 2, 2, 2, 2, 2, 2, 2, 2, 2, 2, 2, 2, 2, 2, 2, 2, 2, 2, 2, 2, 2, 2, 2, 2, 2, 2, 2, 2, 2, 2, 2, 2, 2, 2, 2, 2, 2, 2, 2, 2, 2, 2, 2, 2, 2, 2, 2, 2, 2, 2, 2, 2, 2, 2, 2, 2, 2, 2, 2, 2, 2, 2, 2, 2, 2, 2, 2, 2, 2, 2, 2, 2, 2, 2, 2, 2, 2, 2, 2, 2, 2, 2, 2, 2, 2, 2, 2, 2, 2, 2, 2, 2, 2, 2, 2, 2, 2, 2, 2, 2, 2, 2, 2, 2, 2, 2, 2, 2, 2, 2, 2, 2, 2, 2, 2, 3 ),
 ( 0.000000000000000000, 0.5000000000000000000, 1.000000000000000000 ),
 ( 0.000000000000000000, 0.004385964912280701511, 0.008771929824561403022, 0.01315789473684210453, 0.01754385964912280604, 0.02192982456140350755, 0.02631578947368420907, 0.03070175438596491058, 0.03508771929824561209, 0.03947368421052631360, 0.04385964912280701511, 0.04824561403508771662, 0.05263157894736841813, 0.05701754385964911964, 0.06140350877192982115, 0.06578947368421052266, 0.07017543859649122417, 0.07456140350877192569, 0.07894736842105262720, 0.08333333333333332871, 0.08771929824561403022, 0.09210526315789473173, 0.09649122807017543324, 0.1008771929824561348, 0.1052631578947368363, 0.1096491228070175378, 0.1140350877192982393, 0.1184210526315789408, 0.1228070175438596423, 0.1271929824561403577, 0.1315789473684210453, 0.1359649122807017607, 0.1403508771929824483, 0.1447368421052631637, 0.1491228070175438514, 0.1535087719298245668, 0.1578947368421052544, 0.1622807017543859698, 0.1666666666666666574, 0.1710526315789473728, 0.1754385964912280604, 0.1798245614035087758, 0.1842105263157894635, 0.1885964912280701788, 0.1929824561403508665, 0.1973684210526315819, 0.2017543859649122695, 0.2061403508771929849, 0.2105263157894736725, 0.2149122807017543879, 0.2192982456140350755, 0.2236842105263157909, 0.2280701754385964786, 0.2324561403508771940, 0.2368421052631578816, 0.2412280701754385970, 0.2456140350877192846, 0.2500000000000000000, 0.2543859649122807154, 0.2587719298245614308, 0.2631578947368420907, 0.2675438596491228060, 0.2719298245614035214, 0.2763157894736842368, 0.2807017543859648967, 0.2850877192982456121, 0.2894736842105263275, 0.2938596491228070429, 0.2982456140350877027, 0.3026315789473684181, 0.3070175438596491335, 0.3114035087719298489, 0.3157894736842105088, 0.3201754385964912242, 0.3245614035087719396, 0.3289473684210526550, 0.3333333333333333148, 0.3377192982456140302, 0.3421052631578947456, 0.3464912280701754610, 0.3508771929824561209, 0.3552631578947368363, 0.3596491228070175517, 0.3640350877192982670, 0.3684210526315789269, 0.3728070175438596423, 0.3771929824561403577, 0.3815789473684210731, 0.3859649122807017330, 0.3903508771929824483, 0.3947368421052631637, 0.3991228070175438791, 0.4035087719298245390, 0.4078947368421052544, 0.4122807017543859698, 0.4166666666666666852, 0.4210526315789473450, 0.4254385964912280604, 0.4298245614035087758, 0.4342105263157894912, 0.4385964912280701511, 0.4429824561403508665, 0.4473684210526315819, 0.4517543859649122973, 0.4561403508771929571, 0.4605263157894736725, 0.4649122807017543879, 0.4692982456140351033, 0.4736842105263157632, 0.4780701754385964786, 0.4824561403508771940, 0.4868421052631579093, 0.4912280701754385692, 0.4956140350877192846, 0.5000000000000000000, 0.5043859649122807154, 0.5087719298245614308, 0.5131578947368421462, 0.5175438596491228616, 0.5219298245614034659, 0.5263157894736841813, 0.5307017543859648967, 0.5350877192982456121, 0.5394736842105263275, 0.5438596491228070429, 0.5482456140350877583, 0.5526315789473684736, 0.5570175438596490780, 0.5614035087719297934, 0.5657894736842105088, 0.5701754385964912242, 0.5745614035087719396, 0.5789473684210526550, 0.5833333333333333703, 0.5877192982456140857, 0.5921052631578946901, 0.5964912280701754055, 0.6008771929824561209, 0.6052631578947368363, 0.6096491228070175517, 0.6140350877192982670, 0.6184210526315789824, 0.6228070175438596978, 0.6271929824561403022, 0.6315789473684210176, 0.6359649122807017330, 0.6403508771929824483, 0.6447368421052631637, 0.6491228070175438791, 0.6535087719298245945, 0.6578947368421053099, 0.6622807017543859143, 0.6666666666666666297, 0.6710526315789473450, 0.6754385964912280604, 0.6798245614035087758, 0.6842105263157894912, 0.6885964912280702066, 0.6929824561403509220, 0.6973684210526315264, 0.7017543859649122417, 0.7061403508771929571, 0.7105263157894736725, 0.7149122807017543879, 0.7192982456140351033, 0.7236842105263158187, 0.7280701754385965341, 0.7324561403508771384, 0.7368421052631578538, 0.7412280701754385692, 0.7456140350877192846, 0.7500000000000000000, 0.7543859649122807154, 0.7587719298245614308, 0.7631578947368421462, 0.7675438596491228616, 0.7719298245614034659, 0.7763157894736841813, 0.7807017543859648967, 0.7850877192982456121, 0.7894736842105263275, 0.7938596491228070429, 0.7982456140350877583, 0.8026315789473684736, 0.8070175438596490780, 0.8114035087719297934, 0.8157894736842105088, 0.8201754385964912242, 0.8245614035087719396, 0.8289473684210526550, 0.8333333333333333703, 0.8377192982456140857, 0.8421052631578946901, 0.8464912280701754055, 0.8508771929824561209, 0.8552631578947368363, 0.8596491228070175517, 0.8640350877192982670, 0.8684210526315789824, 0.8728070175438596978, 0.8771929824561403022, 0.8815789473684210176, 0.8859649122807017330, 0.8903508771929824483, 0.8947368421052631637, 0.8991228070175438791, 0.9035087719298245945, 0.9078947368421053099, 0.9122807017543859143, 0.9166666666666666297, 0.9210526315789473450, 0.9254385964912280604, 0.9298245614035087758, 0.9342105263157894912, 0.9385964912280702066, 0.9429824561403509220, 0.9473684210526315264, 0.9517543859649122417, 0.9561403508771929571, 0.9605263157894736725, 0.9649122807017543879, 0.9692982456140351033, 0.9736842105263158187, 0.9780701754385965341, 0.9824561403508771384, 0.9868421052631578538, 0.9912280701754385692, 0.9956140350877192846, 1.000000000000000000 ),
 .UNSPECIFIED. ) 
 GEOMETRIC_REPRESENTATION_ITEM ( )  RATIONAL_B_SPLINE_SURFACE ( (
 ( 1.000000000000000000, 0.9659258262890683122, 1.000000000000000000, 0.9659258262890683122, 1.000000000000000000, 0.9659258262890683122, 1.000000000000000000, 0.9659258262890683122, 1.000000000000000000, 0.9659258262890683122, 1.000000000000000000, 0.9659258262890683122, 1.000000000000000000, 0.9659258262890683122, 1.000000000000000000, 0.9659258262890683122, 1.000000000000000000, 0.9659258262890683122, 1.000000000000000000, 0.9659258262890683122, 1.000000000000000000, 0.9659258262890683122, 1.000000000000000000, 0.9659258262890683122, 1.000000000000000000, 0.9659258262890683122, 1.000000000000000000, 0.9659258262890683122, 1.000000000000000000, 0.9659258262890683122, 1.000000000000000000, 0.9659258262890683122, 1.000000000000000000, 0.9659258262890683122, 1.000000000000000000, 0.9659258262890683122, 1.000000000000000000, 0.9659258262890683122, 1.000000000000000000, 0.9659258262890683122, 1.000000000000000000, 0.9659258262890683122, 1.000000000000000000, 0.9659258262890683122, 1.000000000000000000, 0.9659258262890683122, 1.000000000000000000, 0.9659258262890683122, 1.000000000000000000, 0.9659258262890683122, 1.000000000000000000, 0.9659258262890683122, 1.000000000000000000, 0.9659258262890683122, 1.000000000000000000, 0.9659258262890683122, 1.000000000000000000, 0.9659258262890683122, 1.000000000000000000, 0.9659258262890683122, 1.000000000000000000, 0.9659258262890683122, 1.000000000000000000, 0.9659258262890683122, 1.000000000000000000, 0.9659258262890683122, 1.000000000000000000, 0.9659258262890683122, 1.000000000000000000, 0.9659258262890683122, 1.000000000000000000, 0.9659258262890683122, 1.000000000000000000, 0.9659258262890683122, 1.000000000000000000, 0.9659258262890683122, 1.000000000000000000, 0.9659258262890683122, 1.000000000000000000, 0.9659258262890683122, 1.000000000000000000, 0.9659258262890683122, 1.000000000000000000, 0.9659258262890683122, 1.000000000000000000, 0.9659258262890683122, 1.000000000000000000, 0.9659258262890683122, 1.000000000000000000, 0.9659258262890683122, 1.000000000000000000, 0.9659258262890683122, 1.000000000000000000, 0.9659258262890683122, 1.000000000000000000, 0.9659258262890683122, 1.000000000000000000, 0.9659258262890683122, 1.000000000000000000, 0.9659258262890683122, 1.000000000000000000, 0.9659258262890683122, 1.000000000000000000, 0.9659258262890683122, 1.000000000000000000, 0.9659258262890683122, 1.000000000000000000, 0.9659258262890683122, 1.000000000000000000, 0.9659258262890683122, 1.000000000000000000, 0.9659258262890683122, 1.000000000000000000, 0.9659258262890683122, 1.000000000000000000, 0.9659258262890683122, 1.000000000000000000, 0.9659258262890683122, 1.000000000000000000, 0.9659258262890683122, 1.000000000000000000, 0.9659258262890683122, 1.000000000000000000, 0.9659258262890683122, 1.000000000000000000, 0.9659258262890683122, 1.000000000000000000, 0.9659258262890683122, 1.000000000000000000, 0.9659258262890683122, 1.000000000000000000, 0.9659258262890683122, 1.000000000000000000, 0.9659258262890683122, 1.000000000000000000, 0.9659258262890683122, 1.000000000000000000, 0.9659258262890683122, 1.000000000000000000, 0.9659258262890683122, 1.000000000000000000, 0.9659258262890683122, 1.000000000000000000, 0.9659258262890683122, 1.000000000000000000, 0.9659258262890683122, 1.000000000000000000, 0.9659258262890683122, 1.000000000000000000, 0.9659258262890683122, 1.000000000000000000, 0.9659258262890683122, 1.000000000000000000, 0.9659258262890683122, 1.000000000000000000, 0.9659258262890683122, 1.000000000000000000, 0.9659258262890683122, 1.000000000000000000, 0.9659258262890683122, 1.000000000000000000, 0.9659258262890683122, 1.000000000000000000, 0.9659258262890683122, 1.000000000000000000, 0.9659258262890683122, 1.000000000000000000, 0.9659258262890683122, 1.000000000000000000, 0.9659258262890683122, 1.000000000000000000, 0.9659258262890683122, 1.000000000000000000, 0.9659258262890683122, 1.000000000000000000, 0.9659258262890683122, 1.000000000000000000, 0.9659258262890683122, 1.000000000000000000, 0.9659258262890683122, 1.000000000000000000, 0.9659258262890683122, 1.000000000000000000, 0.9659258262890683122, 1.000000000000000000, 0.9659258262890683122, 1.000000000000000000, 0.9659258262890683122, 1.000000000000000000, 0.9659258262890683122, 1.000000000000000000, 0.9659258262890683122, 1.000000000000000000, 0.9659258262890683122, 1.000000000000000000, 0.9659258262890683122, 1.000000000000000000, 0.9659258262890683122, 1.000000000000000000, 0.9659258262890683122, 1.000000000000000000, 0.9659258262890683122, 1.000000000000000000, 0.9659258262890683122, 1.000000000000000000, 0.9659258262890683122, 1.000000000000000000, 0.9659258262890683122, 1.000000000000000000, 0.9659258262890683122, 1.000000000000000000, 0.9659258262890683122, 1.000000000000000000, 0.9659258262890683122, 1.000000000000000000, 0.9659258262890683122, 1.000000000000000000, 0.9659258262890683122, 1.000000000000000000, 0.9659258262890683122, 1.000000000000000000, 0.9659258262890683122, 1.000000000000000000, 0.9659258262890683122, 1.000000000000000000, 0.9659258262890683122, 1.000000000000000000, 0.9659258262890683122, 1.000000000000000000, 0.9659258262890683122, 1.000000000000000000, 0.9659258262890683122, 1.000000000000000000, 0.9659258262890683122, 1.000000000000000000, 0.9659258262890683122, 1.000000000000000000, 0.9659258262890683122, 1.000000000000000000, 0.9659258262890683122, 1.000000000000000000, 0.9659258262890683122, 1.000000000000000000, 0.9659258262890683122, 1.000000000000000000, 0.9659258262890683122, 1.000000000000000000, 0.9659258262890683122, 1.000000000000000000, 0.9659258262890683122, 1.000000000000000000, 0.9659258262890683122, 1.000000000000000000, 0.9659258262890683122, 1.000000000000000000, 0.9659258262890683122, 1.000000000000000000, 0.9659258262890683122, 1.000000000000000000, 0.9659258262890683122, 1.000000000000000000, 0.9659258262890683122, 1.000000000000000000, 0.9659258262890683122, 1.000000000000000000, 0.9659258262890683122, 1.000000000000000000, 0.9659258262890683122, 1.000000000000000000, 0.9659258262890683122, 1.000000000000000000, 0.9659258262890683122, 1.000000000000000000, 0.9659258262890683122, 1.000000000000000000, 0.9659258262890683122, 1.000000000000000000, 0.9659258262890683122, 1.000000000000000000, 0.9659258262890683122, 1.000000000000000000, 0.9659258262890683122, 1.000000000000000000, 0.9659258262890683122, 1.000000000000000000, 0.9659258262890683122, 1.000000000000000000, 0.9659258262890683122, 1.000000000000000000, 0.9659258262890683122, 1.000000000000000000, 0.9659258262890683122, 1.000000000000000000, 0.9659258262890683122, 1.000000000000000000, 0.9659258262890683122, 1.000000000000000000, 0.9659258262890683122, 1.000000000000000000, 0.9659258262890683122, 1.000000000000000000, 0.9659258262890683122, 1.000000000000000000, 0.9659258262890683122, 1.000000000000000000, 0.9659258262890683122, 1.000000000000000000, 0.9659258262890683122, 1.000000000000000000, 0.9659258262890683122, 1.000000000000000000, 0.9659258262890683122, 1.000000000000000000, 0.9659258262890683122, 1.000000000000000000, 0.9659258262890683122, 1.000000000000000000, 0.9659258262890683122, 1.000000000000000000, 0.9659258262890683122, 1.000000000000000000, 0.9659258262890683122, 1.000000000000000000, 0.9659258262890683122, 1.000000000000000000, 0.9659258262890683122, 1.000000000000000000, 0.9659258262890683122, 1.000000000000000000, 0.9659258262890683122, 1.000000000000000000, 0.9659258262890683122, 1.000000000000000000, 0.9659258262890683122, 1.000000000000000000, 0.9659258262890683122, 1.000000000000000000, 0.9659258262890683122, 1.000000000000000000, 0.9659258262890683122, 1.000000000000000000, 0.9659258262890683122, 1.000000000000000000, 0.9659258262890683122, 1.000000000000000000, 0.9659258262890683122, 1.000000000000000000, 0.9659258262890683122, 1.000000000000000000, 0.9659258262890683122, 1.000000000000000000, 0.9659258262890683122, 1.000000000000000000, 0.9659258262890683122, 1.000000000000000000, 0.9659258262890683122, 1.000000000000000000, 0.9659258262890683122, 1.000000000000000000, 0.9659258262890683122, 1.000000000000000000, 0.9659258262890683122, 1.000000000000000000, 0.9659258262890683122, 1.000000000000000000, 0.9659258262890683122, 1.000000000000000000, 0.9659258262890683122, 1.000000000000000000, 0.9659258262890683122, 1.000000000000000000, 0.9659258262890683122, 1.000000000000000000, 0.9659258262890683122, 1.000000000000000000, 0.9659258262890683122, 1.000000000000000000, 0.9659258262890683122, 1.000000000000000000, 0.9659258262890683122, 1.000000000000000000, 0.9659258262890683122, 1.000000000000000000, 0.9659258262890683122, 1.000000000000000000, 0.9659258262890683122, 1.000000000000000000, 0.9659258262890683122, 1.000000000000000000, 0.9659258262890683122, 1.000000000000000000, 0.9659258262890683122, 1.000000000000000000, 0.9659258262890683122, 1.000000000000000000, 0.9659258262890683122, 1.000000000000000000, 0.9659258262890683122, 1.000000000000000000, 0.9659258262890683122, 1.000000000000000000, 0.9659258262890683122, 1.000000000000000000, 0.9659258262890683122, 1.000000000000000000, 0.9659258262890683122, 1.000000000000000000, 0.9659258262890683122, 1.000000000000000000, 0.9659258262890683122, 1.000000000000000000, 0.9659258262890683122, 1.000000000000000000, 0.9659258262890683122, 1.000000000000000000, 0.9659258262890683122, 1.000000000000000000, 0.9659258262890683122, 1.000000000000000000, 0.9659258262890683122, 1.000000000000000000, 0.9659258262890683122, 1.000000000000000000, 0.9659258262890683122, 1.000000000000000000, 0.9659258262890683122, 1.000000000000000000, 0.9659258262890683122, 1.000000000000000000, 0.9659258262890683122, 1.000000000000000000, 0.9659258262890683122, 1.000000000000000000, 0.9659258262890683122, 1.000000000000000000, 0.9659258262890683122, 1.000000000000000000, 0.9659258262890683122, 1.000000000000000000, 0.9659258262890683122, 1.000000000000000000, 0.9659258262890683122, 1.000000000000000000, 0.9659258262890683122, 1.000000000000000000, 0.9659258262890683122, 1.000000000000000000, 0.9659258262890683122, 1.000000000000000000, 0.9659258262890683122, 1.000000000000000000, 0.9659258262890683122, 1.000000000000000000, 0.9659258262890683122, 1.000000000000000000, 0.9659258262890683122, 1.000000000000000000),
 ( 0.3333333333333333703, 0.3219752754296894559, 0.3333333333333333703, 0.3219752754296894559, 0.3333333333333333703, 0.3219752754296894559, 0.3333333333333333703, 0.3219752754296894559, 0.3333333333333333703, 0.3219752754296894559, 0.3333333333333333703, 0.3219752754296894559, 0.3333333333333333703, 0.3219752754296894559, 0.3333333333333333703, 0.3219752754296894559, 0.3333333333333333703, 0.3219752754296894559, 0.3333333333333333703, 0.3219752754296894559, 0.3333333333333333703, 0.3219752754296894559, 0.3333333333333333703, 0.3219752754296894559, 0.3333333333333333703, 0.3219752754296894559, 0.3333333333333333703, 0.3219752754296894559, 0.3333333333333333703, 0.3219752754296894559, 0.3333333333333333703, 0.3219752754296894559, 0.3333333333333333703, 0.3219752754296894559, 0.3333333333333333703, 0.3219752754296894559, 0.3333333333333333703, 0.3219752754296894559, 0.3333333333333333703, 0.3219752754296894559, 0.3333333333333333703, 0.3219752754296894559, 0.3333333333333333703, 0.3219752754296894559, 0.3333333333333333703, 0.3219752754296894559, 0.3333333333333333703, 0.3219752754296894559, 0.3333333333333333703, 0.3219752754296894559, 0.3333333333333333703, 0.3219752754296894559, 0.3333333333333333703, 0.3219752754296894559, 0.3333333333333333703, 0.3219752754296894559, 0.3333333333333333703, 0.3219752754296894559, 0.3333333333333333703, 0.3219752754296894559, 0.3333333333333333703, 0.3219752754296894559, 0.3333333333333333703, 0.3219752754296894559, 0.3333333333333333703, 0.3219752754296894559, 0.3333333333333333703, 0.3219752754296894559, 0.3333333333333333703, 0.3219752754296894559, 0.3333333333333333703, 0.3219752754296894559, 0.3333333333333333703, 0.3219752754296894559, 0.3333333333333333703, 0.3219752754296894559, 0.3333333333333333703, 0.3219752754296894559, 0.3333333333333333703, 0.3219752754296894559, 0.3333333333333333703, 0.3219752754296894559, 0.3333333333333333703, 0.3219752754296894559, 0.3333333333333333703, 0.3219752754296894559, 0.3333333333333333703, 0.3219752754296894559, 0.3333333333333333703, 0.3219752754296894559, 0.3333333333333333703, 0.3219752754296894559, 0.3333333333333333703, 0.3219752754296894559, 0.3333333333333333703, 0.3219752754296894559, 0.3333333333333333703, 0.3219752754296894559, 0.3333333333333333703, 0.3219752754296894559, 0.3333333333333333703, 0.3219752754296894559, 0.3333333333333333703, 0.3219752754296894559, 0.3333333333333333703, 0.3219752754296894559, 0.3333333333333333703, 0.3219752754296894559, 0.3333333333333333703, 0.3219752754296894559, 0.3333333333333333703, 0.3219752754296894559, 0.3333333333333333703, 0.3219752754296894559, 0.3333333333333333703, 0.3219752754296894559, 0.3333333333333333703, 0.3219752754296894559, 0.3333333333333333703, 0.3219752754296894559, 0.3333333333333333703, 0.3219752754296894559, 0.3333333333333333703, 0.3219752754296894559, 0.3333333333333333703, 0.3219752754296894559, 0.3333333333333333703, 0.3219752754296894559, 0.3333333333333333703, 0.3219752754296894559, 0.3333333333333333703, 0.3219752754296894559, 0.3333333333333333703, 0.3219752754296894559, 0.3333333333333333703, 0.3219752754296894559, 0.3333333333333333703, 0.3219752754296894559, 0.3333333333333333703, 0.3219752754296894559, 0.3333333333333333703, 0.3219752754296894559, 0.3333333333333333703, 0.3219752754296894559, 0.3333333333333333703, 0.3219752754296894559, 0.3333333333333333703, 0.3219752754296894559, 0.3333333333333333703, 0.3219752754296894559, 0.3333333333333333703, 0.3219752754296894559, 0.3333333333333333703, 0.3219752754296894559, 0.3333333333333333703, 0.3219752754296894559, 0.3333333333333333703, 0.3219752754296894559, 0.3333333333333333703, 0.3219752754296894559, 0.3333333333333333703, 0.3219752754296894559, 0.3333333333333333703, 0.3219752754296894559, 0.3333333333333333703, 0.3219752754296894559, 0.3333333333333333703, 0.3219752754296894559, 0.3333333333333333703, 0.3219752754296894559, 0.3333333333333333703, 0.3219752754296894559, 0.3333333333333333703, 0.3219752754296894559, 0.3333333333333333703, 0.3219752754296894559, 0.3333333333333333703, 0.3219752754296894559, 0.3333333333333333703, 0.3219752754296894559, 0.3333333333333333703, 0.3219752754296894559, 0.3333333333333333703, 0.3219752754296894559, 0.3333333333333333703, 0.3219752754296894559, 0.3333333333333333703, 0.3219752754296894559, 0.3333333333333333703, 0.3219752754296894559, 0.3333333333333333703, 0.3219752754296894559, 0.3333333333333333703, 0.3219752754296894559, 0.3333333333333333703, 0.3219752754296894559, 0.3333333333333333703, 0.3219752754296894559, 0.3333333333333333703, 0.3219752754296894559, 0.3333333333333333703, 0.3219752754296894559, 0.3333333333333333703, 0.3219752754296894559, 0.3333333333333333703, 0.3219752754296894559, 0.3333333333333333703, 0.3219752754296894559, 0.3333333333333333703, 0.3219752754296894559, 0.3333333333333333703, 0.3219752754296894559, 0.3333333333333333703, 0.3219752754296894559, 0.3333333333333333703, 0.3219752754296894559, 0.3333333333333333703, 0.3219752754296894559, 0.3333333333333333703, 0.3219752754296894559, 0.3333333333333333703, 0.3219752754296894559, 0.3333333333333333703, 0.3219752754296894559, 0.3333333333333333703, 0.3219752754296894559, 0.3333333333333333703, 0.3219752754296894559, 0.3333333333333333703, 0.3219752754296894559, 0.3333333333333333703, 0.3219752754296894559, 0.3333333333333333703, 0.3219752754296894559, 0.3333333333333333703, 0.3219752754296894559, 0.3333333333333333703, 0.3219752754296894559, 0.3333333333333333703, 0.3219752754296894559, 0.3333333333333333703, 0.3219752754296894559, 0.3333333333333333703, 0.3219752754296894559, 0.3333333333333333703, 0.3219752754296894559, 0.3333333333333333703, 0.3219752754296894559, 0.3333333333333333703, 0.3219752754296894559, 0.3333333333333333703, 0.3219752754296894559, 0.3333333333333333703, 0.3219752754296894559, 0.3333333333333333703, 0.3219752754296894559, 0.3333333333333333703, 0.3219752754296894559, 0.3333333333333333703, 0.3219752754296894559, 0.3333333333333333703, 0.3219752754296894559, 0.3333333333333333703, 0.3219752754296894559, 0.3333333333333333703, 0.3219752754296894559, 0.3333333333333333703, 0.3219752754296894559, 0.3333333333333333703, 0.3219752754296894559, 0.3333333333333333703, 0.3219752754296894559, 0.3333333333333333703, 0.3219752754296894559, 0.3333333333333333703, 0.3219752754296894559, 0.3333333333333333703, 0.3219752754296894559, 0.3333333333333333703, 0.3219752754296894559, 0.3333333333333333703, 0.3219752754296894559, 0.3333333333333333703, 0.3219752754296894559, 0.3333333333333333703, 0.3219752754296894559, 0.3333333333333333703, 0.3219752754296894559, 0.3333333333333333703, 0.3219752754296894559, 0.3333333333333333703, 0.3219752754296894559, 0.3333333333333333703, 0.3219752754296894559, 0.3333333333333333703, 0.3219752754296894559, 0.3333333333333333703, 0.3219752754296894559, 0.3333333333333333703, 0.3219752754296894559, 0.3333333333333333703, 0.3219752754296894559, 0.3333333333333333703, 0.3219752754296894559, 0.3333333333333333703, 0.3219752754296894559, 0.3333333333333333703, 0.3219752754296894559, 0.3333333333333333703, 0.3219752754296894559, 0.3333333333333333703, 0.3219752754296894559, 0.3333333333333333703, 0.3219752754296894559, 0.3333333333333333703, 0.3219752754296894559, 0.3333333333333333703, 0.3219752754296894559, 0.3333333333333333703, 0.3219752754296894559, 0.3333333333333333703, 0.3219752754296894559, 0.3333333333333333703, 0.3219752754296894559, 0.3333333333333333703, 0.3219752754296894559, 0.3333333333333333703, 0.3219752754296894559, 0.3333333333333333703, 0.3219752754296894559, 0.3333333333333333703, 0.3219752754296894559, 0.3333333333333333703, 0.3219752754296894559, 0.3333333333333333703, 0.3219752754296894559, 0.3333333333333333703, 0.3219752754296894559, 0.3333333333333333703, 0.3219752754296894559, 0.3333333333333333703, 0.3219752754296894559, 0.3333333333333333703, 0.3219752754296894559, 0.3333333333333333703, 0.3219752754296894559, 0.3333333333333333703, 0.3219752754296894559, 0.3333333333333333703, 0.3219752754296894559, 0.3333333333333333703, 0.3219752754296894559, 0.3333333333333333703, 0.3219752754296894559, 0.3333333333333333703, 0.3219752754296894559, 0.3333333333333333703, 0.3219752754296894559, 0.3333333333333333703, 0.3219752754296894559, 0.3333333333333333703, 0.3219752754296894559, 0.3333333333333333703, 0.3219752754296894559, 0.3333333333333333703, 0.3219752754296894559, 0.3333333333333333703, 0.3219752754296894559, 0.3333333333333333703, 0.3219752754296894559, 0.3333333333333333703, 0.3219752754296894559, 0.3333333333333333703, 0.3219752754296894559, 0.3333333333333333703, 0.3219752754296894559, 0.3333333333333333703, 0.3219752754296894559, 0.3333333333333333703, 0.3219752754296894559, 0.3333333333333333703, 0.3219752754296894559, 0.3333333333333333703, 0.3219752754296894559, 0.3333333333333333703, 0.3219752754296894559, 0.3333333333333333703, 0.3219752754296894559, 0.3333333333333333703, 0.3219752754296894559, 0.3333333333333333703, 0.3219752754296894559, 0.3333333333333333703, 0.3219752754296894559, 0.3333333333333333703, 0.3219752754296894559, 0.3333333333333333703, 0.3219752754296894559, 0.3333333333333333703, 0.3219752754296894559, 0.3333333333333333703, 0.3219752754296894559, 0.3333333333333333703, 0.3219752754296894559, 0.3333333333333333703, 0.3219752754296894559, 0.3333333333333333703, 0.3219752754296894559, 0.3333333333333333703, 0.3219752754296894559, 0.3333333333333333703, 0.3219752754296894559, 0.3333333333333333703, 0.3219752754296894559, 0.3333333333333333703, 0.3219752754296894559, 0.3333333333333333703, 0.3219752754296894559, 0.3333333333333333703, 0.3219752754296894559, 0.3333333333333333703, 0.3219752754296894559, 0.3333333333333333703, 0.3219752754296894559, 0.3333333333333333703, 0.3219752754296894559, 0.3333333333333333703, 0.3219752754296894559, 0.3333333333333333703, 0.3219752754296894559, 0.3333333333333333703, 0.3219752754296894559, 0.3333333333333333703, 0.3219752754296894559, 0.3333333333333333703, 0.3219752754296894559, 0.3333333333333333703, 0.3219752754296894559, 0.3333333333333333703, 0.3219752754296894559, 0.3333333333333333703, 0.3219752754296894559, 0.3333333333333333703, 0.3219752754296894559, 0.3333333333333333703, 0.3219752754296894559, 0.3333333333333333703, 0.3219752754296894559, 0.3333333333333333703, 0.3219752754296894559, 0.3333333333333333703, 0.3219752754296894559, 0.3333333333333333703, 0.3219752754296894559, 0.3333333333333333703, 0.3219752754296894559, 0.3333333333333333703),
 ( 0.3333333333333333703, 0.3219752754296894559, 0.3333333333333333703, 0.3219752754296894559, 0.3333333333333333703, 0.3219752754296894559, 0.3333333333333333703, 0.3219752754296894559, 0.3333333333333333703, 0.3219752754296894559, 0.3333333333333333703, 0.3219752754296894559, 0.3333333333333333703, 0.3219752754296894559, 0.3333333333333333703, 0.3219752754296894559, 0.3333333333333333703, 0.3219752754296894559, 0.3333333333333333703, 0.3219752754296894559, 0.3333333333333333703, 0.3219752754296894559, 0.3333333333333333703, 0.3219752754296894559, 0.3333333333333333703, 0.3219752754296894559, 0.3333333333333333703, 0.3219752754296894559, 0.3333333333333333703, 0.3219752754296894559, 0.3333333333333333703, 0.3219752754296894559, 0.3333333333333333703, 0.3219752754296894559, 0.3333333333333333703, 0.3219752754296894559, 0.3333333333333333703, 0.3219752754296894559, 0.3333333333333333703, 0.3219752754296894559, 0.3333333333333333703, 0.3219752754296894559, 0.3333333333333333703, 0.3219752754296894559, 0.3333333333333333703, 0.3219752754296894559, 0.3333333333333333703, 0.3219752754296894559, 0.3333333333333333703, 0.3219752754296894559, 0.3333333333333333703, 0.3219752754296894559, 0.3333333333333333703, 0.3219752754296894559, 0.3333333333333333703, 0.3219752754296894559, 0.3333333333333333703, 0.3219752754296894559, 0.3333333333333333703, 0.3219752754296894559, 0.3333333333333333703, 0.3219752754296894559, 0.3333333333333333703, 0.3219752754296894559, 0.3333333333333333703, 0.3219752754296894559, 0.3333333333333333703, 0.3219752754296894559, 0.3333333333333333703, 0.3219752754296894559, 0.3333333333333333703, 0.3219752754296894559, 0.3333333333333333703, 0.3219752754296894559, 0.3333333333333333703, 0.3219752754296894559, 0.3333333333333333703, 0.3219752754296894559, 0.3333333333333333703, 0.3219752754296894559, 0.3333333333333333703, 0.3219752754296894559, 0.3333333333333333703, 0.3219752754296894559, 0.3333333333333333703, 0.3219752754296894559, 0.3333333333333333703, 0.3219752754296894559, 0.3333333333333333703, 0.3219752754296894559, 0.3333333333333333703, 0.3219752754296894559, 0.3333333333333333703, 0.3219752754296894559, 0.3333333333333333703, 0.3219752754296894559, 0.3333333333333333703, 0.3219752754296894559, 0.3333333333333333703, 0.3219752754296894559, 0.3333333333333333703, 0.3219752754296894559, 0.3333333333333333703, 0.3219752754296894559, 0.3333333333333333703, 0.3219752754296894559, 0.3333333333333333703, 0.3219752754296894559, 0.3333333333333333703, 0.3219752754296894559, 0.3333333333333333703, 0.3219752754296894559, 0.3333333333333333703, 0.3219752754296894559, 0.3333333333333333703, 0.3219752754296894559, 0.3333333333333333703, 0.3219752754296894559, 0.3333333333333333703, 0.3219752754296894559, 0.3333333333333333703, 0.3219752754296894559, 0.3333333333333333703, 0.3219752754296894559, 0.3333333333333333703, 0.3219752754296894559, 0.3333333333333333703, 0.3219752754296894559, 0.3333333333333333703, 0.3219752754296894559, 0.3333333333333333703, 0.3219752754296894559, 0.3333333333333333703, 0.3219752754296894559, 0.3333333333333333703, 0.3219752754296894559, 0.3333333333333333703, 0.3219752754296894559, 0.3333333333333333703, 0.3219752754296894559, 0.3333333333333333703, 0.3219752754296894559, 0.3333333333333333703, 0.3219752754296894559, 0.3333333333333333703, 0.3219752754296894559, 0.3333333333333333703, 0.3219752754296894559, 0.3333333333333333703, 0.3219752754296894559, 0.3333333333333333703, 0.3219752754296894559, 0.3333333333333333703, 0.3219752754296894559, 0.3333333333333333703, 0.3219752754296894559, 0.3333333333333333703, 0.3219752754296894559, 0.3333333333333333703, 0.3219752754296894559, 0.3333333333333333703, 0.3219752754296894559, 0.3333333333333333703, 0.3219752754296894559, 0.3333333333333333703, 0.3219752754296894559, 0.3333333333333333703, 0.3219752754296894559, 0.3333333333333333703, 0.3219752754296894559, 0.3333333333333333703, 0.3219752754296894559, 0.3333333333333333703, 0.3219752754296894559, 0.3333333333333333703, 0.3219752754296894559, 0.3333333333333333703, 0.3219752754296894559, 0.3333333333333333703, 0.3219752754296894559, 0.3333333333333333703, 0.3219752754296894559, 0.3333333333333333703, 0.3219752754296894559, 0.3333333333333333703, 0.3219752754296894559, 0.3333333333333333703, 0.3219752754296894559, 0.3333333333333333703, 0.3219752754296894559, 0.3333333333333333703, 0.3219752754296894559, 0.3333333333333333703, 0.3219752754296894559, 0.3333333333333333703, 0.3219752754296894559, 0.3333333333333333703, 0.3219752754296894559, 0.3333333333333333703, 0.3219752754296894559, 0.3333333333333333703, 0.3219752754296894559, 0.3333333333333333703, 0.3219752754296894559, 0.3333333333333333703, 0.3219752754296894559, 0.3333333333333333703, 0.3219752754296894559, 0.3333333333333333703, 0.3219752754296894559, 0.3333333333333333703, 0.3219752754296894559, 0.3333333333333333703, 0.3219752754296894559, 0.3333333333333333703, 0.3219752754296894559, 0.3333333333333333703, 0.3219752754296894559, 0.3333333333333333703, 0.3219752754296894559, 0.3333333333333333703, 0.3219752754296894559, 0.3333333333333333703, 0.3219752754296894559, 0.3333333333333333703, 0.3219752754296894559, 0.3333333333333333703, 0.3219752754296894559, 0.3333333333333333703, 0.3219752754296894559, 0.3333333333333333703, 0.3219752754296894559, 0.3333333333333333703, 0.3219752754296894559, 0.3333333333333333703, 0.3219752754296894559, 0.3333333333333333703, 0.3219752754296894559, 0.3333333333333333703, 0.3219752754296894559, 0.3333333333333333703, 0.3219752754296894559, 0.3333333333333333703, 0.3219752754296894559, 0.3333333333333333703, 0.3219752754296894559, 0.3333333333333333703, 0.3219752754296894559, 0.3333333333333333703, 0.3219752754296894559, 0.3333333333333333703, 0.3219752754296894559, 0.3333333333333333703, 0.3219752754296894559, 0.3333333333333333703, 0.3219752754296894559, 0.3333333333333333703, 0.3219752754296894559, 0.3333333333333333703, 0.3219752754296894559, 0.3333333333333333703, 0.3219752754296894559, 0.3333333333333333703, 0.3219752754296894559, 0.3333333333333333703, 0.3219752754296894559, 0.3333333333333333703, 0.3219752754296894559, 0.3333333333333333703, 0.3219752754296894559, 0.3333333333333333703, 0.3219752754296894559, 0.3333333333333333703, 0.3219752754296894559, 0.3333333333333333703, 0.3219752754296894559, 0.3333333333333333703, 0.3219752754296894559, 0.3333333333333333703, 0.3219752754296894559, 0.3333333333333333703, 0.3219752754296894559, 0.3333333333333333703, 0.3219752754296894559, 0.3333333333333333703, 0.3219752754296894559, 0.3333333333333333703, 0.3219752754296894559, 0.3333333333333333703, 0.3219752754296894559, 0.3333333333333333703, 0.3219752754296894559, 0.3333333333333333703, 0.3219752754296894559, 0.3333333333333333703, 0.3219752754296894559, 0.3333333333333333703, 0.3219752754296894559, 0.3333333333333333703, 0.3219752754296894559, 0.3333333333333333703, 0.3219752754296894559, 0.3333333333333333703, 0.3219752754296894559, 0.3333333333333333703, 0.3219752754296894559, 0.3333333333333333703, 0.3219752754296894559, 0.3333333333333333703, 0.3219752754296894559, 0.3333333333333333703, 0.3219752754296894559, 0.3333333333333333703, 0.3219752754296894559, 0.3333333333333333703, 0.3219752754296894559, 0.3333333333333333703, 0.3219752754296894559, 0.3333333333333333703, 0.3219752754296894559, 0.3333333333333333703, 0.3219752754296894559, 0.3333333333333333703, 0.3219752754296894559, 0.3333333333333333703, 0.3219752754296894559, 0.3333333333333333703, 0.3219752754296894559, 0.3333333333333333703, 0.3219752754296894559, 0.3333333333333333703, 0.3219752754296894559, 0.3333333333333333703, 0.3219752754296894559, 0.3333333333333333703, 0.3219752754296894559, 0.3333333333333333703, 0.3219752754296894559, 0.3333333333333333703, 0.3219752754296894559, 0.3333333333333333703, 0.3219752754296894559, 0.3333333333333333703, 0.3219752754296894559, 0.3333333333333333703, 0.3219752754296894559, 0.3333333333333333703, 0.3219752754296894559, 0.3333333333333333703, 0.3219752754296894559, 0.3333333333333333703, 0.3219752754296894559, 0.3333333333333333703, 0.3219752754296894559, 0.3333333333333333703, 0.3219752754296894559, 0.3333333333333333703, 0.3219752754296894559, 0.3333333333333333703, 0.3219752754296894559, 0.3333333333333333703, 0.3219752754296894559, 0.3333333333333333703, 0.3219752754296894559, 0.3333333333333333703, 0.3219752754296894559, 0.3333333333333333703, 0.3219752754296894559, 0.3333333333333333703, 0.3219752754296894559, 0.3333333333333333703, 0.3219752754296894559, 0.3333333333333333703, 0.3219752754296894559, 0.3333333333333333703, 0.3219752754296894559, 0.3333333333333333703, 0.3219752754296894559, 0.3333333333333333703, 0.3219752754296894559, 0.3333333333333333703, 0.3219752754296894559, 0.3333333333333333703, 0.3219752754296894559, 0.3333333333333333703, 0.3219752754296894559, 0.3333333333333333703, 0.3219752754296894559, 0.3333333333333333703, 0.3219752754296894559, 0.3333333333333333703, 0.3219752754296894559, 0.3333333333333333703, 0.3219752754296894559, 0.3333333333333333703, 0.3219752754296894559, 0.3333333333333333703, 0.3219752754296894559, 0.3333333333333333703, 0.3219752754296894559, 0.3333333333333333703, 0.3219752754296894559, 0.3333333333333333703, 0.3219752754296894559, 0.3333333333333333703, 0.3219752754296894559, 0.3333333333333333703, 0.3219752754296894559, 0.3333333333333333703, 0.3219752754296894559, 0.3333333333333333703, 0.3219752754296894559, 0.3333333333333333703, 0.3219752754296894559, 0.3333333333333333703, 0.3219752754296894559, 0.3333333333333333703, 0.3219752754296894559, 0.3333333333333333703, 0.3219752754296894559, 0.3333333333333333703, 0.3219752754296894559, 0.3333333333333333703, 0.3219752754296894559, 0.3333333333333333703, 0.3219752754296894559, 0.3333333333333333703, 0.3219752754296894559, 0.3333333333333333703, 0.3219752754296894559, 0.3333333333333333703, 0.3219752754296894559, 0.3333333333333333703, 0.3219752754296894559, 0.3333333333333333703, 0.3219752754296894559, 0.3333333333333333703, 0.3219752754296894559, 0.3333333333333333703, 0.3219752754296894559, 0.3333333333333333703, 0.3219752754296894559, 0.3333333333333333703, 0.3219752754296894559, 0.3333333333333333703, 0.3219752754296894559, 0.3333333333333333703, 0.3219752754296894559, 0.3333333333333333703, 0.3219752754296894559, 0.3333333333333333703, 0.3219752754296894559, 0.3333333333333333703, 0.3219752754296894559, 0.3333333333333333703, 0.3219752754296894559, 0.3333333333333333703),
 ( 1.000000000000000000, 0.9659258262890683122, 1.000000000000000000, 0.9659258262890683122, 1.000000000000000000, 0.9659258262890683122, 1.000000000000000000, 0.9659258262890683122, 1.000000000000000000, 0.9659258262890683122, 1.000000000000000000, 0.9659258262890683122, 1.000000000000000000, 0.9659258262890683122, 1.000000000000000000, 0.9659258262890683122, 1.000000000000000000, 0.9659258262890683122, 1.000000000000000000, 0.9659258262890683122, 1.000000000000000000, 0.9659258262890683122, 1.000000000000000000, 0.9659258262890683122, 1.000000000000000000, 0.9659258262890683122, 1.000000000000000000, 0.9659258262890683122, 1.000000000000000000, 0.9659258262890683122, 1.000000000000000000, 0.9659258262890683122, 1.000000000000000000, 0.9659258262890683122, 1.000000000000000000, 0.9659258262890683122, 1.000000000000000000, 0.9659258262890683122, 1.000000000000000000, 0.9659258262890683122, 1.000000000000000000, 0.9659258262890683122, 1.000000000000000000, 0.9659258262890683122, 1.000000000000000000, 0.9659258262890683122, 1.000000000000000000, 0.9659258262890683122, 1.000000000000000000, 0.9659258262890683122, 1.000000000000000000, 0.9659258262890683122, 1.000000000000000000, 0.9659258262890683122, 1.000000000000000000, 0.9659258262890683122, 1.000000000000000000, 0.9659258262890683122, 1.000000000000000000, 0.9659258262890683122, 1.000000000000000000, 0.9659258262890683122, 1.000000000000000000, 0.9659258262890683122, 1.000000000000000000, 0.9659258262890683122, 1.000000000000000000, 0.9659258262890683122, 1.000000000000000000, 0.9659258262890683122, 1.000000000000000000, 0.9659258262890683122, 1.000000000000000000, 0.9659258262890683122, 1.000000000000000000, 0.9659258262890683122, 1.000000000000000000, 0.9659258262890683122, 1.000000000000000000, 0.9659258262890683122, 1.000000000000000000, 0.9659258262890683122, 1.000000000000000000, 0.9659258262890683122, 1.000000000000000000, 0.9659258262890683122, 1.000000000000000000, 0.9659258262890683122, 1.000000000000000000, 0.9659258262890683122, 1.000000000000000000, 0.9659258262890683122, 1.000000000000000000, 0.9659258262890683122, 1.000000000000000000, 0.9659258262890683122, 1.000000000000000000, 0.9659258262890683122, 1.000000000000000000, 0.9659258262890683122, 1.000000000000000000, 0.9659258262890683122, 1.000000000000000000, 0.9659258262890683122, 1.000000000000000000, 0.9659258262890683122, 1.000000000000000000, 0.9659258262890683122, 1.000000000000000000, 0.9659258262890683122, 1.000000000000000000, 0.9659258262890683122, 1.000000000000000000, 0.9659258262890683122, 1.000000000000000000, 0.9659258262890683122, 1.000000000000000000, 0.9659258262890683122, 1.000000000000000000, 0.9659258262890683122, 1.000000000000000000, 0.9659258262890683122, 1.000000000000000000, 0.9659258262890683122, 1.000000000000000000, 0.9659258262890683122, 1.000000000000000000, 0.9659258262890683122, 1.000000000000000000, 0.9659258262890683122, 1.000000000000000000, 0.9659258262890683122, 1.000000000000000000, 0.9659258262890683122, 1.000000000000000000, 0.9659258262890683122, 1.000000000000000000, 0.9659258262890683122, 1.000000000000000000, 0.9659258262890683122, 1.000000000000000000, 0.9659258262890683122, 1.000000000000000000, 0.9659258262890683122, 1.000000000000000000, 0.9659258262890683122, 1.000000000000000000, 0.9659258262890683122, 1.000000000000000000, 0.9659258262890683122, 1.000000000000000000, 0.9659258262890683122, 1.000000000000000000, 0.9659258262890683122, 1.000000000000000000, 0.9659258262890683122, 1.000000000000000000, 0.9659258262890683122, 1.000000000000000000, 0.9659258262890683122, 1.000000000000000000, 0.9659258262890683122, 1.000000000000000000, 0.9659258262890683122, 1.000000000000000000, 0.9659258262890683122, 1.000000000000000000, 0.9659258262890683122, 1.000000000000000000, 0.9659258262890683122, 1.000000000000000000, 0.9659258262890683122, 1.000000000000000000, 0.9659258262890683122, 1.000000000000000000, 0.9659258262890683122, 1.000000000000000000, 0.9659258262890683122, 1.000000000000000000, 0.9659258262890683122, 1.000000000000000000, 0.9659258262890683122, 1.000000000000000000, 0.9659258262890683122, 1.000000000000000000, 0.9659258262890683122, 1.000000000000000000, 0.9659258262890683122, 1.000000000000000000, 0.9659258262890683122, 1.000000000000000000, 0.9659258262890683122, 1.000000000000000000, 0.9659258262890683122, 1.000000000000000000, 0.9659258262890683122, 1.000000000000000000, 0.9659258262890683122, 1.000000000000000000, 0.9659258262890683122, 1.000000000000000000, 0.9659258262890683122, 1.000000000000000000, 0.9659258262890683122, 1.000000000000000000, 0.9659258262890683122, 1.000000000000000000, 0.9659258262890683122, 1.000000000000000000, 0.9659258262890683122, 1.000000000000000000, 0.9659258262890683122, 1.000000000000000000, 0.9659258262890683122, 1.000000000000000000, 0.9659258262890683122, 1.000000000000000000, 0.9659258262890683122, 1.000000000000000000, 0.9659258262890683122, 1.000000000000000000, 0.9659258262890683122, 1.000000000000000000, 0.9659258262890683122, 1.000000000000000000, 0.9659258262890683122, 1.000000000000000000, 0.9659258262890683122, 1.000000000000000000, 0.9659258262890683122, 1.000000000000000000, 0.9659258262890683122, 1.000000000000000000, 0.9659258262890683122, 1.000000000000000000, 0.9659258262890683122, 1.000000000000000000, 0.9659258262890683122, 1.000000000000000000, 0.9659258262890683122, 1.000000000000000000, 0.9659258262890683122, 1.000000000000000000, 0.9659258262890683122, 1.000000000000000000, 0.9659258262890683122, 1.000000000000000000, 0.9659258262890683122, 1.000000000000000000, 0.9659258262890683122, 1.000000000000000000, 0.9659258262890683122, 1.000000000000000000, 0.9659258262890683122, 1.000000000000000000, 0.9659258262890683122, 1.000000000000000000, 0.9659258262890683122, 1.000000000000000000, 0.9659258262890683122, 1.000000000000000000, 0.9659258262890683122, 1.000000000000000000, 0.9659258262890683122, 1.000000000000000000, 0.9659258262890683122, 1.000000000000000000, 0.9659258262890683122, 1.000000000000000000, 0.9659258262890683122, 1.000000000000000000, 0.9659258262890683122, 1.000000000000000000, 0.9659258262890683122, 1.000000000000000000, 0.9659258262890683122, 1.000000000000000000, 0.9659258262890683122, 1.000000000000000000, 0.9659258262890683122, 1.000000000000000000, 0.9659258262890683122, 1.000000000000000000, 0.9659258262890683122, 1.000000000000000000, 0.9659258262890683122, 1.000000000000000000, 0.9659258262890683122, 1.000000000000000000, 0.9659258262890683122, 1.000000000000000000, 0.9659258262890683122, 1.000000000000000000, 0.9659258262890683122, 1.000000000000000000, 0.9659258262890683122, 1.000000000000000000, 0.9659258262890683122, 1.000000000000000000, 0.9659258262890683122, 1.000000000000000000, 0.9659258262890683122, 1.000000000000000000, 0.9659258262890683122, 1.000000000000000000, 0.9659258262890683122, 1.000000000000000000, 0.9659258262890683122, 1.000000000000000000, 0.9659258262890683122, 1.000000000000000000, 0.9659258262890683122, 1.000000000000000000, 0.9659258262890683122, 1.000000000000000000, 0.9659258262890683122, 1.000000000000000000, 0.9659258262890683122, 1.000000000000000000, 0.9659258262890683122, 1.000000000000000000, 0.9659258262890683122, 1.000000000000000000, 0.9659258262890683122, 1.000000000000000000, 0.9659258262890683122, 1.000000000000000000, 0.9659258262890683122, 1.000000000000000000, 0.9659258262890683122, 1.000000000000000000, 0.9659258262890683122, 1.000000000000000000, 0.9659258262890683122, 1.000000000000000000, 0.9659258262890683122, 1.000000000000000000, 0.9659258262890683122, 1.000000000000000000, 0.9659258262890683122, 1.000000000000000000, 0.9659258262890683122, 1.000000000000000000, 0.9659258262890683122, 1.000000000000000000, 0.9659258262890683122, 1.000000000000000000, 0.9659258262890683122, 1.000000000000000000, 0.9659258262890683122, 1.000000000000000000, 0.9659258262890683122, 1.000000000000000000, 0.9659258262890683122, 1.000000000000000000, 0.9659258262890683122, 1.000000000000000000, 0.9659258262890683122, 1.000000000000000000, 0.9659258262890683122, 1.000000000000000000, 0.9659258262890683122, 1.000000000000000000, 0.9659258262890683122, 1.000000000000000000, 0.9659258262890683122, 1.000000000000000000, 0.9659258262890683122, 1.000000000000000000, 0.9659258262890683122, 1.000000000000000000, 0.9659258262890683122, 1.000000000000000000, 0.9659258262890683122, 1.000000000000000000, 0.9659258262890683122, 1.000000000000000000, 0.9659258262890683122, 1.000000000000000000, 0.9659258262890683122, 1.000000000000000000, 0.9659258262890683122, 1.000000000000000000, 0.9659258262890683122, 1.000000000000000000, 0.9659258262890683122, 1.000000000000000000, 0.9659258262890683122, 1.000000000000000000, 0.9659258262890683122, 1.000000000000000000, 0.9659258262890683122, 1.000000000000000000, 0.9659258262890683122, 1.000000000000000000, 0.9659258262890683122, 1.000000000000000000, 0.9659258262890683122, 1.000000000000000000, 0.9659258262890683122, 1.000000000000000000, 0.9659258262890683122, 1.000000000000000000, 0.9659258262890683122, 1.000000000000000000, 0.9659258262890683122, 1.000000000000000000, 0.9659258262890683122, 1.000000000000000000, 0.9659258262890683122, 1.000000000000000000, 0.9659258262890683122, 1.000000000000000000, 0.9659258262890683122, 1.000000000000000000, 0.9659258262890683122, 1.000000000000000000, 0.9659258262890683122, 1.000000000000000000, 0.9659258262890683122, 1.000000000000000000, 0.9659258262890683122, 1.000000000000000000, 0.9659258262890683122, 1.000000000000000000, 0.9659258262890683122, 1.000000000000000000, 0.9659258262890683122, 1.000000000000000000, 0.9659258262890683122, 1.000000000000000000, 0.9659258262890683122, 1.000000000000000000, 0.9659258262890683122, 1.000000000000000000, 0.9659258262890683122, 1.000000000000000000, 0.9659258262890683122, 1.000000000000000000, 0.9659258262890683122, 1.000000000000000000, 0.9659258262890683122, 1.000000000000000000, 0.9659258262890683122, 1.000000000000000000, 0.9659258262890683122, 1.000000000000000000, 0.9659258262890683122, 1.000000000000000000, 0.9659258262890683122, 1.000000000000000000, 0.9659258262890683122, 1.000000000000000000, 0.9659258262890683122, 1.000000000000000000, 0.9659258262890683122, 1.000000000000000000),
 ( 0.3333333333333333703, 0.3219752754296894559, 0.3333333333333333703, 0.3219752754296894559, 0.3333333333333333703, 0.3219752754296894559, 0.3333333333333333703, 0.3219752754296894559, 0.3333333333333333703, 0.3219752754296894559, 0.3333333333333333703, 0.3219752754296894559, 0.3333333333333333703, 0.3219752754296894559, 0.3333333333333333703, 0.3219752754296894559, 0.3333333333333333703, 0.3219752754296894559, 0.3333333333333333703, 0.3219752754296894559, 0.3333333333333333703, 0.3219752754296894559, 0.3333333333333333703, 0.3219752754296894559, 0.3333333333333333703, 0.3219752754296894559, 0.3333333333333333703, 0.3219752754296894559, 0.3333333333333333703, 0.3219752754296894559, 0.3333333333333333703, 0.3219752754296894559, 0.3333333333333333703, 0.3219752754296894559, 0.3333333333333333703, 0.3219752754296894559, 0.3333333333333333703, 0.3219752754296894559, 0.3333333333333333703, 0.3219752754296894559, 0.3333333333333333703, 0.3219752754296894559, 0.3333333333333333703, 0.3219752754296894559, 0.3333333333333333703, 0.3219752754296894559, 0.3333333333333333703, 0.3219752754296894559, 0.3333333333333333703, 0.3219752754296894559, 0.3333333333333333703, 0.3219752754296894559, 0.3333333333333333703, 0.3219752754296894559, 0.3333333333333333703, 0.3219752754296894559, 0.3333333333333333703, 0.3219752754296894559, 0.3333333333333333703, 0.3219752754296894559, 0.3333333333333333703, 0.3219752754296894559, 0.3333333333333333703, 0.3219752754296894559, 0.3333333333333333703, 0.3219752754296894559, 0.3333333333333333703, 0.3219752754296894559, 0.3333333333333333703, 0.3219752754296894559, 0.3333333333333333703, 0.3219752754296894559, 0.3333333333333333703, 0.3219752754296894559, 0.3333333333333333703, 0.3219752754296894559, 0.3333333333333333703, 0.3219752754296894559, 0.3333333333333333703, 0.3219752754296894559, 0.3333333333333333703, 0.3219752754296894559, 0.3333333333333333703, 0.3219752754296894559, 0.3333333333333333703, 0.3219752754296894559, 0.3333333333333333703, 0.3219752754296894559, 0.3333333333333333703, 0.3219752754296894559, 0.3333333333333333703, 0.3219752754296894559, 0.3333333333333333703, 0.3219752754296894559, 0.3333333333333333703, 0.3219752754296894559, 0.3333333333333333703, 0.3219752754296894559, 0.3333333333333333703, 0.3219752754296894559, 0.3333333333333333703, 0.3219752754296894559, 0.3333333333333333703, 0.3219752754296894559, 0.3333333333333333703, 0.3219752754296894559, 0.3333333333333333703, 0.3219752754296894559, 0.3333333333333333703, 0.3219752754296894559, 0.3333333333333333703, 0.3219752754296894559, 0.3333333333333333703, 0.3219752754296894559, 0.3333333333333333703, 0.3219752754296894559, 0.3333333333333333703, 0.3219752754296894559, 0.3333333333333333703, 0.3219752754296894559, 0.3333333333333333703, 0.3219752754296894559, 0.3333333333333333703, 0.3219752754296894559, 0.3333333333333333703, 0.3219752754296894559, 0.3333333333333333703, 0.3219752754296894559, 0.3333333333333333703, 0.3219752754296894559, 0.3333333333333333703, 0.3219752754296894559, 0.3333333333333333703, 0.3219752754296894559, 0.3333333333333333703, 0.3219752754296894559, 0.3333333333333333703, 0.3219752754296894559, 0.3333333333333333703, 0.3219752754296894559, 0.3333333333333333703, 0.3219752754296894559, 0.3333333333333333703, 0.3219752754296894559, 0.3333333333333333703, 0.3219752754296894559, 0.3333333333333333703, 0.3219752754296894559, 0.3333333333333333703, 0.3219752754296894559, 0.3333333333333333703, 0.3219752754296894559, 0.3333333333333333703, 0.3219752754296894559, 0.3333333333333333703, 0.3219752754296894559, 0.3333333333333333703, 0.3219752754296894559, 0.3333333333333333703, 0.3219752754296894559, 0.3333333333333333703, 0.3219752754296894559, 0.3333333333333333703, 0.3219752754296894559, 0.3333333333333333703, 0.3219752754296894559, 0.3333333333333333703, 0.3219752754296894559, 0.3333333333333333703, 0.3219752754296894559, 0.3333333333333333703, 0.3219752754296894559, 0.3333333333333333703, 0.3219752754296894559, 0.3333333333333333703, 0.3219752754296894559, 0.3333333333333333703, 0.3219752754296894559, 0.3333333333333333703, 0.3219752754296894559, 0.3333333333333333703, 0.3219752754296894559, 0.3333333333333333703, 0.3219752754296894559, 0.3333333333333333703, 0.3219752754296894559, 0.3333333333333333703, 0.3219752754296894559, 0.3333333333333333703, 0.3219752754296894559, 0.3333333333333333703, 0.3219752754296894559, 0.3333333333333333703, 0.3219752754296894559, 0.3333333333333333703, 0.3219752754296894559, 0.3333333333333333703, 0.3219752754296894559, 0.3333333333333333703, 0.3219752754296894559, 0.3333333333333333703, 0.3219752754296894559, 0.3333333333333333703, 0.3219752754296894559, 0.3333333333333333703, 0.3219752754296894559, 0.3333333333333333703, 0.3219752754296894559, 0.3333333333333333703, 0.3219752754296894559, 0.3333333333333333703, 0.3219752754296894559, 0.3333333333333333703, 0.3219752754296894559, 0.3333333333333333703, 0.3219752754296894559, 0.3333333333333333703, 0.3219752754296894559, 0.3333333333333333703, 0.3219752754296894559, 0.3333333333333333703, 0.3219752754296894559, 0.3333333333333333703, 0.3219752754296894559, 0.3333333333333333703, 0.3219752754296894559, 0.3333333333333333703, 0.3219752754296894559, 0.3333333333333333703, 0.3219752754296894559, 0.3333333333333333703, 0.3219752754296894559, 0.3333333333333333703, 0.3219752754296894559, 0.3333333333333333703, 0.3219752754296894559, 0.3333333333333333703, 0.3219752754296894559, 0.3333333333333333703, 0.3219752754296894559, 0.3333333333333333703, 0.3219752754296894559, 0.3333333333333333703, 0.3219752754296894559, 0.3333333333333333703, 0.3219752754296894559, 0.3333333333333333703, 0.3219752754296894559, 0.3333333333333333703, 0.3219752754296894559, 0.3333333333333333703, 0.3219752754296894559, 0.3333333333333333703, 0.3219752754296894559, 0.3333333333333333703, 0.3219752754296894559, 0.3333333333333333703, 0.3219752754296894559, 0.3333333333333333703, 0.3219752754296894559, 0.3333333333333333703, 0.3219752754296894559, 0.3333333333333333703, 0.3219752754296894559, 0.3333333333333333703, 0.3219752754296894559, 0.3333333333333333703, 0.3219752754296894559, 0.3333333333333333703, 0.3219752754296894559, 0.3333333333333333703, 0.3219752754296894559, 0.3333333333333333703, 0.3219752754296894559, 0.3333333333333333703, 0.3219752754296894559, 0.3333333333333333703, 0.3219752754296894559, 0.3333333333333333703, 0.3219752754296894559, 0.3333333333333333703, 0.3219752754296894559, 0.3333333333333333703, 0.3219752754296894559, 0.3333333333333333703, 0.3219752754296894559, 0.3333333333333333703, 0.3219752754296894559, 0.3333333333333333703, 0.3219752754296894559, 0.3333333333333333703, 0.3219752754296894559, 0.3333333333333333703, 0.3219752754296894559, 0.3333333333333333703, 0.3219752754296894559, 0.3333333333333333703, 0.3219752754296894559, 0.3333333333333333703, 0.3219752754296894559, 0.3333333333333333703, 0.3219752754296894559, 0.3333333333333333703, 0.3219752754296894559, 0.3333333333333333703, 0.3219752754296894559, 0.3333333333333333703, 0.3219752754296894559, 0.3333333333333333703, 0.3219752754296894559, 0.3333333333333333703, 0.3219752754296894559, 0.3333333333333333703, 0.3219752754296894559, 0.3333333333333333703, 0.3219752754296894559, 0.3333333333333333703, 0.3219752754296894559, 0.3333333333333333703, 0.3219752754296894559, 0.3333333333333333703, 0.3219752754296894559, 0.3333333333333333703, 0.3219752754296894559, 0.3333333333333333703, 0.3219752754296894559, 0.3333333333333333703, 0.3219752754296894559, 0.3333333333333333703, 0.3219752754296894559, 0.3333333333333333703, 0.3219752754296894559, 0.3333333333333333703, 0.3219752754296894559, 0.3333333333333333703, 0.3219752754296894559, 0.3333333333333333703, 0.3219752754296894559, 0.3333333333333333703, 0.3219752754296894559, 0.3333333333333333703, 0.3219752754296894559, 0.3333333333333333703, 0.3219752754296894559, 0.3333333333333333703, 0.3219752754296894559, 0.3333333333333333703, 0.3219752754296894559, 0.3333333333333333703, 0.3219752754296894559, 0.3333333333333333703, 0.3219752754296894559, 0.3333333333333333703, 0.3219752754296894559, 0.3333333333333333703, 0.3219752754296894559, 0.3333333333333333703, 0.3219752754296894559, 0.3333333333333333703, 0.3219752754296894559, 0.3333333333333333703, 0.3219752754296894559, 0.3333333333333333703, 0.3219752754296894559, 0.3333333333333333703, 0.3219752754296894559, 0.3333333333333333703, 0.3219752754296894559, 0.3333333333333333703, 0.3219752754296894559, 0.3333333333333333703, 0.3219752754296894559, 0.3333333333333333703, 0.3219752754296894559, 0.3333333333333333703, 0.3219752754296894559, 0.3333333333333333703, 0.3219752754296894559, 0.3333333333333333703, 0.3219752754296894559, 0.3333333333333333703, 0.3219752754296894559, 0.3333333333333333703, 0.3219752754296894559, 0.3333333333333333703, 0.3219752754296894559, 0.3333333333333333703, 0.3219752754296894559, 0.3333333333333333703, 0.3219752754296894559, 0.3333333333333333703, 0.3219752754296894559, 0.3333333333333333703, 0.3219752754296894559, 0.3333333333333333703, 0.3219752754296894559, 0.3333333333333333703, 0.3219752754296894559, 0.3333333333333333703, 0.3219752754296894559, 0.3333333333333333703, 0.3219752754296894559, 0.3333333333333333703, 0.3219752754296894559, 0.3333333333333333703, 0.3219752754296894559, 0.3333333333333333703, 0.3219752754296894559, 0.3333333333333333703, 0.3219752754296894559, 0.3333333333333333703, 0.3219752754296894559, 0.3333333333333333703, 0.3219752754296894559, 0.3333333333333333703, 0.3219752754296894559, 0.3333333333333333703, 0.3219752754296894559, 0.3333333333333333703, 0.3219752754296894559, 0.3333333333333333703, 0.3219752754296894559, 0.3333333333333333703, 0.3219752754296894559, 0.3333333333333333703, 0.3219752754296894559, 0.3333333333333333703, 0.3219752754296894559, 0.3333333333333333703, 0.3219752754296894559, 0.3333333333333333703, 0.3219752754296894559, 0.3333333333333333703, 0.3219752754296894559, 0.3333333333333333703, 0.3219752754296894559, 0.3333333333333333703, 0.3219752754296894559, 0.3333333333333333703, 0.3219752754296894559, 0.3333333333333333703, 0.3219752754296894559, 0.3333333333333333703, 0.3219752754296894559, 0.3333333333333333703, 0.3219752754296894559, 0.3333333333333333703, 0.3219752754296894559, 0.3333333333333333703, 0.3219752754296894559, 0.3333333333333333703, 0.3219752754296894559, 0.3333333333333333703, 0.3219752754296894559, 0.3333333333333333703, 0.3219752754296894559, 0.3333333333333333703),
 ( 0.3333333333333333703, 0.3219752754296894559, 0.3333333333333333703, 0.3219752754296894559, 0.3333333333333333703, 0.3219752754296894559, 0.3333333333333333703, 0.3219752754296894559, 0.3333333333333333703, 0.3219752754296894559, 0.3333333333333333703, 0.3219752754296894559, 0.3333333333333333703, 0.3219752754296894559, 0.3333333333333333703, 0.3219752754296894559, 0.3333333333333333703, 0.3219752754296894559, 0.3333333333333333703, 0.3219752754296894559, 0.3333333333333333703, 0.3219752754296894559, 0.3333333333333333703, 0.3219752754296894559, 0.3333333333333333703, 0.3219752754296894559, 0.3333333333333333703, 0.3219752754296894559, 0.3333333333333333703, 0.3219752754296894559, 0.3333333333333333703, 0.3219752754296894559, 0.3333333333333333703, 0.3219752754296894559, 0.3333333333333333703, 0.3219752754296894559, 0.3333333333333333703, 0.3219752754296894559, 0.3333333333333333703, 0.3219752754296894559, 0.3333333333333333703, 0.3219752754296894559, 0.3333333333333333703, 0.3219752754296894559, 0.3333333333333333703, 0.3219752754296894559, 0.3333333333333333703, 0.3219752754296894559, 0.3333333333333333703, 0.3219752754296894559, 0.3333333333333333703, 0.3219752754296894559, 0.3333333333333333703, 0.3219752754296894559, 0.3333333333333333703, 0.3219752754296894559, 0.3333333333333333703, 0.3219752754296894559, 0.3333333333333333703, 0.3219752754296894559, 0.3333333333333333703, 0.3219752754296894559, 0.3333333333333333703, 0.3219752754296894559, 0.3333333333333333703, 0.3219752754296894559, 0.3333333333333333703, 0.3219752754296894559, 0.3333333333333333703, 0.3219752754296894559, 0.3333333333333333703, 0.3219752754296894559, 0.3333333333333333703, 0.3219752754296894559, 0.3333333333333333703, 0.3219752754296894559, 0.3333333333333333703, 0.3219752754296894559, 0.3333333333333333703, 0.3219752754296894559, 0.3333333333333333703, 0.3219752754296894559, 0.3333333333333333703, 0.3219752754296894559, 0.3333333333333333703, 0.3219752754296894559, 0.3333333333333333703, 0.3219752754296894559, 0.3333333333333333703, 0.3219752754296894559, 0.3333333333333333703, 0.3219752754296894559, 0.3333333333333333703, 0.3219752754296894559, 0.3333333333333333703, 0.3219752754296894559, 0.3333333333333333703, 0.3219752754296894559, 0.3333333333333333703, 0.3219752754296894559, 0.3333333333333333703, 0.3219752754296894559, 0.3333333333333333703, 0.3219752754296894559, 0.3333333333333333703, 0.3219752754296894559, 0.3333333333333333703, 0.3219752754296894559, 0.3333333333333333703, 0.3219752754296894559, 0.3333333333333333703, 0.3219752754296894559, 0.3333333333333333703, 0.3219752754296894559, 0.3333333333333333703, 0.3219752754296894559, 0.3333333333333333703, 0.3219752754296894559, 0.3333333333333333703, 0.3219752754296894559, 0.3333333333333333703, 0.3219752754296894559, 0.3333333333333333703, 0.3219752754296894559, 0.3333333333333333703, 0.3219752754296894559, 0.3333333333333333703, 0.3219752754296894559, 0.3333333333333333703, 0.3219752754296894559, 0.3333333333333333703, 0.3219752754296894559, 0.3333333333333333703, 0.3219752754296894559, 0.3333333333333333703, 0.3219752754296894559, 0.3333333333333333703, 0.3219752754296894559, 0.3333333333333333703, 0.3219752754296894559, 0.3333333333333333703, 0.3219752754296894559, 0.3333333333333333703, 0.3219752754296894559, 0.3333333333333333703, 0.3219752754296894559, 0.3333333333333333703, 0.3219752754296894559, 0.3333333333333333703, 0.3219752754296894559, 0.3333333333333333703, 0.3219752754296894559, 0.3333333333333333703, 0.3219752754296894559, 0.3333333333333333703, 0.3219752754296894559, 0.3333333333333333703, 0.3219752754296894559, 0.3333333333333333703, 0.3219752754296894559, 0.3333333333333333703, 0.3219752754296894559, 0.3333333333333333703, 0.3219752754296894559, 0.3333333333333333703, 0.3219752754296894559, 0.3333333333333333703, 0.3219752754296894559, 0.3333333333333333703, 0.3219752754296894559, 0.3333333333333333703, 0.3219752754296894559, 0.3333333333333333703, 0.3219752754296894559, 0.3333333333333333703, 0.3219752754296894559, 0.3333333333333333703, 0.3219752754296894559, 0.3333333333333333703, 0.3219752754296894559, 0.3333333333333333703, 0.3219752754296894559, 0.3333333333333333703, 0.3219752754296894559, 0.3333333333333333703, 0.3219752754296894559, 0.3333333333333333703, 0.3219752754296894559, 0.3333333333333333703, 0.3219752754296894559, 0.3333333333333333703, 0.3219752754296894559, 0.3333333333333333703, 0.3219752754296894559, 0.3333333333333333703, 0.3219752754296894559, 0.3333333333333333703, 0.3219752754296894559, 0.3333333333333333703, 0.3219752754296894559, 0.3333333333333333703, 0.3219752754296894559, 0.3333333333333333703, 0.3219752754296894559, 0.3333333333333333703, 0.3219752754296894559, 0.3333333333333333703, 0.3219752754296894559, 0.3333333333333333703, 0.3219752754296894559, 0.3333333333333333703, 0.3219752754296894559, 0.3333333333333333703, 0.3219752754296894559, 0.3333333333333333703, 0.3219752754296894559, 0.3333333333333333703, 0.3219752754296894559, 0.3333333333333333703, 0.3219752754296894559, 0.3333333333333333703, 0.3219752754296894559, 0.3333333333333333703, 0.3219752754296894559, 0.3333333333333333703, 0.3219752754296894559, 0.3333333333333333703, 0.3219752754296894559, 0.3333333333333333703, 0.3219752754296894559, 0.3333333333333333703, 0.3219752754296894559, 0.3333333333333333703, 0.3219752754296894559, 0.3333333333333333703, 0.3219752754296894559, 0.3333333333333333703, 0.3219752754296894559, 0.3333333333333333703, 0.3219752754296894559, 0.3333333333333333703, 0.3219752754296894559, 0.3333333333333333703, 0.3219752754296894559, 0.3333333333333333703, 0.3219752754296894559, 0.3333333333333333703, 0.3219752754296894559, 0.3333333333333333703, 0.3219752754296894559, 0.3333333333333333703, 0.3219752754296894559, 0.3333333333333333703, 0.3219752754296894559, 0.3333333333333333703, 0.3219752754296894559, 0.3333333333333333703, 0.3219752754296894559, 0.3333333333333333703, 0.3219752754296894559, 0.3333333333333333703, 0.3219752754296894559, 0.3333333333333333703, 0.3219752754296894559, 0.3333333333333333703, 0.3219752754296894559, 0.3333333333333333703, 0.3219752754296894559, 0.3333333333333333703, 0.3219752754296894559, 0.3333333333333333703, 0.3219752754296894559, 0.3333333333333333703, 0.3219752754296894559, 0.3333333333333333703, 0.3219752754296894559, 0.3333333333333333703, 0.3219752754296894559, 0.3333333333333333703, 0.3219752754296894559, 0.3333333333333333703, 0.3219752754296894559, 0.3333333333333333703, 0.3219752754296894559, 0.3333333333333333703, 0.3219752754296894559, 0.3333333333333333703, 0.3219752754296894559, 0.3333333333333333703, 0.3219752754296894559, 0.3333333333333333703, 0.3219752754296894559, 0.3333333333333333703, 0.3219752754296894559, 0.3333333333333333703, 0.3219752754296894559, 0.3333333333333333703, 0.3219752754296894559, 0.3333333333333333703, 0.3219752754296894559, 0.3333333333333333703, 0.3219752754296894559, 0.3333333333333333703, 0.3219752754296894559, 0.3333333333333333703, 0.3219752754296894559, 0.3333333333333333703, 0.3219752754296894559, 0.3333333333333333703, 0.3219752754296894559, 0.3333333333333333703, 0.3219752754296894559, 0.3333333333333333703, 0.3219752754296894559, 0.3333333333333333703, 0.3219752754296894559, 0.3333333333333333703, 0.3219752754296894559, 0.3333333333333333703, 0.3219752754296894559, 0.3333333333333333703, 0.3219752754296894559, 0.3333333333333333703, 0.3219752754296894559, 0.3333333333333333703, 0.3219752754296894559, 0.3333333333333333703, 0.3219752754296894559, 0.3333333333333333703, 0.3219752754296894559, 0.3333333333333333703, 0.3219752754296894559, 0.3333333333333333703, 0.3219752754296894559, 0.3333333333333333703, 0.3219752754296894559, 0.3333333333333333703, 0.3219752754296894559, 0.3333333333333333703, 0.3219752754296894559, 0.3333333333333333703, 0.3219752754296894559, 0.3333333333333333703, 0.3219752754296894559, 0.3333333333333333703, 0.3219752754296894559, 0.3333333333333333703, 0.3219752754296894559, 0.3333333333333333703, 0.3219752754296894559, 0.3333333333333333703, 0.3219752754296894559, 0.3333333333333333703, 0.3219752754296894559, 0.3333333333333333703, 0.3219752754296894559, 0.3333333333333333703, 0.3219752754296894559, 0.3333333333333333703, 0.3219752754296894559, 0.3333333333333333703, 0.3219752754296894559, 0.3333333333333333703, 0.3219752754296894559, 0.3333333333333333703, 0.3219752754296894559, 0.3333333333333333703, 0.3219752754296894559, 0.3333333333333333703, 0.3219752754296894559, 0.3333333333333333703, 0.3219752754296894559, 0.3333333333333333703, 0.3219752754296894559, 0.3333333333333333703, 0.3219752754296894559, 0.3333333333333333703, 0.3219752754296894559, 0.3333333333333333703, 0.3219752754296894559, 0.3333333333333333703, 0.3219752754296894559, 0.3333333333333333703, 0.3219752754296894559, 0.3333333333333333703, 0.3219752754296894559, 0.3333333333333333703, 0.3219752754296894559, 0.3333333333333333703, 0.3219752754296894559, 0.3333333333333333703, 0.3219752754296894559, 0.3333333333333333703, 0.3219752754296894559, 0.3333333333333333703, 0.3219752754296894559, 0.3333333333333333703, 0.3219752754296894559, 0.3333333333333333703, 0.3219752754296894559, 0.3333333333333333703, 0.3219752754296894559, 0.3333333333333333703, 0.3219752754296894559, 0.3333333333333333703, 0.3219752754296894559, 0.3333333333333333703, 0.3219752754296894559, 0.3333333333333333703, 0.3219752754296894559, 0.3333333333333333703, 0.3219752754296894559, 0.3333333333333333703, 0.3219752754296894559, 0.3333333333333333703, 0.3219752754296894559, 0.3333333333333333703, 0.3219752754296894559, 0.3333333333333333703, 0.3219752754296894559, 0.3333333333333333703, 0.3219752754296894559, 0.3333333333333333703, 0.3219752754296894559, 0.3333333333333333703, 0.3219752754296894559, 0.3333333333333333703, 0.3219752754296894559, 0.3333333333333333703, 0.3219752754296894559, 0.3333333333333333703, 0.3219752754296894559, 0.3333333333333333703, 0.3219752754296894559, 0.3333333333333333703, 0.3219752754296894559, 0.3333333333333333703, 0.3219752754296894559, 0.3333333333333333703, 0.3219752754296894559, 0.3333333333333333703, 0.3219752754296894559, 0.3333333333333333703, 0.3219752754296894559, 0.3333333333333333703, 0.3219752754296894559, 0.3333333333333333703, 0.3219752754296894559, 0.3333333333333333703, 0.3219752754296894559, 0.3333333333333333703, 0.3219752754296894559, 0.3333333333333333703, 0.3219752754296894559, 0.3333333333333333703, 0.3219752754296894559, 0.3333333333333333703),
 ( 1.000000000000000000, 0.9659258262890683122, 1.000000000000000000, 0.9659258262890683122, 1.000000000000000000, 0.9659258262890683122, 1.000000000000000000, 0.9659258262890683122, 1.000000000000000000, 0.9659258262890683122, 1.000000000000000000, 0.9659258262890683122, 1.000000000000000000, 0.9659258262890683122, 1.000000000000000000, 0.9659258262890683122, 1.000000000000000000, 0.9659258262890683122, 1.000000000000000000, 0.9659258262890683122, 1.000000000000000000, 0.9659258262890683122, 1.000000000000000000, 0.9659258262890683122, 1.000000000000000000, 0.9659258262890683122, 1.000000000000000000, 0.9659258262890683122, 1.000000000000000000, 0.9659258262890683122, 1.000000000000000000, 0.9659258262890683122, 1.000000000000000000, 0.9659258262890683122, 1.000000000000000000, 0.9659258262890683122, 1.000000000000000000, 0.9659258262890683122, 1.000000000000000000, 0.9659258262890683122, 1.000000000000000000, 0.9659258262890683122, 1.000000000000000000, 0.9659258262890683122, 1.000000000000000000, 0.9659258262890683122, 1.000000000000000000, 0.9659258262890683122, 1.000000000000000000, 0.9659258262890683122, 1.000000000000000000, 0.9659258262890683122, 1.000000000000000000, 0.9659258262890683122, 1.000000000000000000, 0.9659258262890683122, 1.000000000000000000, 0.9659258262890683122, 1.000000000000000000, 0.9659258262890683122, 1.000000000000000000, 0.9659258262890683122, 1.000000000000000000, 0.9659258262890683122, 1.000000000000000000, 0.9659258262890683122, 1.000000000000000000, 0.9659258262890683122, 1.000000000000000000, 0.9659258262890683122, 1.000000000000000000, 0.9659258262890683122, 1.000000000000000000, 0.9659258262890683122, 1.000000000000000000, 0.9659258262890683122, 1.000000000000000000, 0.9659258262890683122, 1.000000000000000000, 0.9659258262890683122, 1.000000000000000000, 0.9659258262890683122, 1.000000000000000000, 0.9659258262890683122, 1.000000000000000000, 0.9659258262890683122, 1.000000000000000000, 0.9659258262890683122, 1.000000000000000000, 0.9659258262890683122, 1.000000000000000000, 0.9659258262890683122, 1.000000000000000000, 0.9659258262890683122, 1.000000000000000000, 0.9659258262890683122, 1.000000000000000000, 0.9659258262890683122, 1.000000000000000000, 0.9659258262890683122, 1.000000000000000000, 0.9659258262890683122, 1.000000000000000000, 0.9659258262890683122, 1.000000000000000000, 0.9659258262890683122, 1.000000000000000000, 0.9659258262890683122, 1.000000000000000000, 0.9659258262890683122, 1.000000000000000000, 0.9659258262890683122, 1.000000000000000000, 0.9659258262890683122, 1.000000000000000000, 0.9659258262890683122, 1.000000000000000000, 0.9659258262890683122, 1.000000000000000000, 0.9659258262890683122, 1.000000000000000000, 0.9659258262890683122, 1.000000000000000000, 0.9659258262890683122, 1.000000000000000000, 0.9659258262890683122, 1.000000000000000000, 0.9659258262890683122, 1.000000000000000000, 0.9659258262890683122, 1.000000000000000000, 0.9659258262890683122, 1.000000000000000000, 0.9659258262890683122, 1.000000000000000000, 0.9659258262890683122, 1.000000000000000000, 0.9659258262890683122, 1.000000000000000000, 0.9659258262890683122, 1.000000000000000000, 0.9659258262890683122, 1.000000000000000000, 0.9659258262890683122, 1.000000000000000000, 0.9659258262890683122, 1.000000000000000000, 0.9659258262890683122, 1.000000000000000000, 0.9659258262890683122, 1.000000000000000000, 0.9659258262890683122, 1.000000000000000000, 0.9659258262890683122, 1.000000000000000000, 0.9659258262890683122, 1.000000000000000000, 0.9659258262890683122, 1.000000000000000000, 0.9659258262890683122, 1.000000000000000000, 0.9659258262890683122, 1.000000000000000000, 0.9659258262890683122, 1.000000000000000000, 0.9659258262890683122, 1.000000000000000000, 0.9659258262890683122, 1.000000000000000000, 0.9659258262890683122, 1.000000000000000000, 0.9659258262890683122, 1.000000000000000000, 0.9659258262890683122, 1.000000000000000000, 0.9659258262890683122, 1.000000000000000000, 0.9659258262890683122, 1.000000000000000000, 0.9659258262890683122, 1.000000000000000000, 0.9659258262890683122, 1.000000000000000000, 0.9659258262890683122, 1.000000000000000000, 0.9659258262890683122, 1.000000000000000000, 0.9659258262890683122, 1.000000000000000000, 0.9659258262890683122, 1.000000000000000000, 0.9659258262890683122, 1.000000000000000000, 0.9659258262890683122, 1.000000000000000000, 0.9659258262890683122, 1.000000000000000000, 0.9659258262890683122, 1.000000000000000000, 0.9659258262890683122, 1.000000000000000000, 0.9659258262890683122, 1.000000000000000000, 0.9659258262890683122, 1.000000000000000000, 0.9659258262890683122, 1.000000000000000000, 0.9659258262890683122, 1.000000000000000000, 0.9659258262890683122, 1.000000000000000000, 0.9659258262890683122, 1.000000000000000000, 0.9659258262890683122, 1.000000000000000000, 0.9659258262890683122, 1.000000000000000000, 0.9659258262890683122, 1.000000000000000000, 0.9659258262890683122, 1.000000000000000000, 0.9659258262890683122, 1.000000000000000000, 0.9659258262890683122, 1.000000000000000000, 0.9659258262890683122, 1.000000000000000000, 0.9659258262890683122, 1.000000000000000000, 0.9659258262890683122, 1.000000000000000000, 0.9659258262890683122, 1.000000000000000000, 0.9659258262890683122, 1.000000000000000000, 0.9659258262890683122, 1.000000000000000000, 0.9659258262890683122, 1.000000000000000000, 0.9659258262890683122, 1.000000000000000000, 0.9659258262890683122, 1.000000000000000000, 0.9659258262890683122, 1.000000000000000000, 0.9659258262890683122, 1.000000000000000000, 0.9659258262890683122, 1.000000000000000000, 0.9659258262890683122, 1.000000000000000000, 0.9659258262890683122, 1.000000000000000000, 0.9659258262890683122, 1.000000000000000000, 0.9659258262890683122, 1.000000000000000000, 0.9659258262890683122, 1.000000000000000000, 0.9659258262890683122, 1.000000000000000000, 0.9659258262890683122, 1.000000000000000000, 0.9659258262890683122, 1.000000000000000000, 0.9659258262890683122, 1.000000000000000000, 0.9659258262890683122, 1.000000000000000000, 0.9659258262890683122, 1.000000000000000000, 0.9659258262890683122, 1.000000000000000000, 0.9659258262890683122, 1.000000000000000000, 0.9659258262890683122, 1.000000000000000000, 0.9659258262890683122, 1.000000000000000000, 0.9659258262890683122, 1.000000000000000000, 0.9659258262890683122, 1.000000000000000000, 0.9659258262890683122, 1.000000000000000000, 0.9659258262890683122, 1.000000000000000000, 0.9659258262890683122, 1.000000000000000000, 0.9659258262890683122, 1.000000000000000000, 0.9659258262890683122, 1.000000000000000000, 0.9659258262890683122, 1.000000000000000000, 0.9659258262890683122, 1.000000000000000000, 0.9659258262890683122, 1.000000000000000000, 0.9659258262890683122, 1.000000000000000000, 0.9659258262890683122, 1.000000000000000000, 0.9659258262890683122, 1.000000000000000000, 0.9659258262890683122, 1.000000000000000000, 0.9659258262890683122, 1.000000000000000000, 0.9659258262890683122, 1.000000000000000000, 0.9659258262890683122, 1.000000000000000000, 0.9659258262890683122, 1.000000000000000000, 0.9659258262890683122, 1.000000000000000000, 0.9659258262890683122, 1.000000000000000000, 0.9659258262890683122, 1.000000000000000000, 0.9659258262890683122, 1.000000000000000000, 0.9659258262890683122, 1.000000000000000000, 0.9659258262890683122, 1.000000000000000000, 0.9659258262890683122, 1.000000000000000000, 0.9659258262890683122, 1.000000000000000000, 0.9659258262890683122, 1.000000000000000000, 0.9659258262890683122, 1.000000000000000000, 0.9659258262890683122, 1.000000000000000000, 0.9659258262890683122, 1.000000000000000000, 0.9659258262890683122, 1.000000000000000000, 0.9659258262890683122, 1.000000000000000000, 0.9659258262890683122, 1.000000000000000000, 0.9659258262890683122, 1.000000000000000000, 0.9659258262890683122, 1.000000000000000000, 0.9659258262890683122, 1.000000000000000000, 0.9659258262890683122, 1.000000000000000000, 0.9659258262890683122, 1.000000000000000000, 0.9659258262890683122, 1.000000000000000000, 0.9659258262890683122, 1.000000000000000000, 0.9659258262890683122, 1.000000000000000000, 0.9659258262890683122, 1.000000000000000000, 0.9659258262890683122, 1.000000000000000000, 0.9659258262890683122, 1.000000000000000000, 0.9659258262890683122, 1.000000000000000000, 0.9659258262890683122, 1.000000000000000000, 0.9659258262890683122, 1.000000000000000000, 0.9659258262890683122, 1.000000000000000000, 0.9659258262890683122, 1.000000000000000000, 0.9659258262890683122, 1.000000000000000000, 0.9659258262890683122, 1.000000000000000000, 0.9659258262890683122, 1.000000000000000000, 0.9659258262890683122, 1.000000000000000000, 0.9659258262890683122, 1.000000000000000000, 0.9659258262890683122, 1.000000000000000000, 0.9659258262890683122, 1.000000000000000000, 0.9659258262890683122, 1.000000000000000000, 0.9659258262890683122, 1.000000000000000000, 0.9659258262890683122, 1.000000000000000000, 0.9659258262890683122, 1.000000000000000000, 0.9659258262890683122, 1.000000000000000000, 0.9659258262890683122, 1.000000000000000000, 0.9659258262890683122, 1.000000000000000000, 0.9659258262890683122, 1.000000000000000000, 0.9659258262890683122, 1.000000000000000000, 0.9659258262890683122, 1.000000000000000000, 0.9659258262890683122, 1.000000000000000000, 0.9659258262890683122, 1.000000000000000000, 0.9659258262890683122, 1.000000000000000000, 0.9659258262890683122, 1.000000000000000000, 0.9659258262890683122, 1.000000000000000000, 0.9659258262890683122, 1.000000000000000000, 0.9659258262890683122, 1.000000000000000000, 0.9659258262890683122, 1.000000000000000000, 0.9659258262890683122, 1.000000000000000000, 0.9659258262890683122, 1.000000000000000000, 0.9659258262890683122, 1.000000000000000000, 0.9659258262890683122, 1.000000000000000000, 0.9659258262890683122, 1.000000000000000000, 0.9659258262890683122, 1.000000000000000000, 0.9659258262890683122, 1.000000000000000000, 0.9659258262890683122, 1.000000000000000000, 0.9659258262890683122, 1.000000000000000000, 0.9659258262890683122, 1.000000000000000000, 0.9659258262890683122, 1.000000000000000000, 0.9659258262890683122, 1.000000000000000000, 0.9659258262890683122, 1.000000000000000000, 0.9659258262890683122, 1.000000000000000000, 0.9659258262890683122, 1.000000000000000000) ) ) 
 REPRESENTATION_ITEM ( '' )  SURFACE ( )  );
#128449=CARTESIAN_POINT ( 'NONE',  ( -0.05219959533909027116, -19.03943276465977164, 97.49890960531436690 ) ) ;
#128450=CARTESIAN_POINT ( 'NONE',  ( -10.72451020669870658, -18.67979575497194134, 109.5844237280190328 ) ) ;
#128451=CARTESIAN_POINT ( 'NONE',  ( 19.03943276465977164, -0.05219959533909143690, 88.74890960531436690 ) ) ;
#128452=CARTESIAN_POINT ( 'NONE',  ( 15.72974639402199770, -15.80617190586745480, 63.12390960531435979 ) ) ;
#128453=CARTESIAN_POINT ( 'NONE',  ( -4.483927247898539470, -16.52544592524342804, 87.29057627198103830 ) ) ;
#128454=CARTESIAN_POINT ( 'NONE',  ( -19.02544592524342804, 5.153800228976336051, 56.04057627198100988 ) ) ;
#128455=CARTESIAN_POINT ( 'NONE',  ( -0.05219959533910754901, -16.53943276465976808, 107.4989096053143669 ) ) ;
#128456=CARTESIAN_POINT ( 'NONE',  ( -15.80617190586768217, 15.72974639402176855, 28.12609039468568284 ) ) ;
#128457=CARTESIAN_POINT ( 'NONE',  ( -5.823673210054431948, 21.52544592524334988, 72.70942372801901854 ) ) ;
#128458=CARTESIAN_POINT ( 'NONE',  ( -9.474510206698964154, 16.51473224551069663, 45.41557627198103120 ) ) ;
#128459=CARTESIAN_POINT ( 'NONE',  ( 12.06949235617739724, 12.14591786802326823, 71.87609039468568994 ) ) ;
#128460=CARTESIAN_POINT ( 'NONE',  ( -0.05219959533937732626, 21.53943276465977519, 27.50109039468567929 ) ) ;
#128461=CARTESIAN_POINT ( 'NONE',  ( -15.80617190586768217, 15.72974639402176855, 33.12609039468569705 ) ) ;
#128462=CARTESIAN_POINT ( 'NONE',  ( 5.049401038297881783, 19.05341960407617563, 52.29275706135234003 ) ) ;
#128463=CARTESIAN_POINT ( 'NONE',  ( 0.05219959533909260263, 19.03943276465977164, 64.99890960531436690 ) ) ;
#128464=CARTESIAN_POINT ( 'NONE',  ( 16.51473224551083163, -9.474510206698727899, 35.83442372801899722 ) ) ;
#128465=CARTESIAN_POINT ( 'NONE',  ( 5.823673210054444382, -21.52544592524334988, 85.20942372801901854 ) ) ;
#128466=CARTESIAN_POINT ( 'NONE',  ( -21.53943276465977519, 0.05219959533907696930, 71.24890960531435269 ) ) ;
#128467=CARTESIAN_POINT ( 'NONE',  ( 14.34966873604960469, 8.224510206698951720, 49.16557627198102409 ) ) ;
#128468=CARTESIAN_POINT ( 'NONE',  ( -5.823673210054431948, 21.52544592524334988, 92.70942372801901854 ) ) ;
#128469=CARTESIAN_POINT ( 'NONE',  ( -19.05341960407617563, 5.049401038297882671, 23.54275706135233648 ) ) ;
#128470=CARTESIAN_POINT ( 'NONE',  ( 8.224510206698953496, -14.34966873604960469, 72.91557627198103830 ) ) ;
#128471=CARTESIAN_POINT ( 'NONE',  ( 16.46253265017160672, -9.564922557960803928, 28.33224293864769550 ) ) ;
#128472=CARTESIAN_POINT ( 'NONE',  ( -16.51473224551082808, 9.474510206698731452, 53.33442372801900433 ) ) ;
#128473=CARTESIAN_POINT ( 'NONE',  ( -14.29746914071037622, -8.314922557961029526, 109.1677570613523613 ) ) ;
#128474=CARTESIAN_POINT ( 'NONE',  ( 0.05219959533937995610, -21.53943276465977519, 85.00109039468568994 ) ) ;
#128475=CARTESIAN_POINT ( 'NONE',  ( -13.97604488694527625, -13.89961937509977652, 76.87390960531433848 ) ) ;
#128476=CARTESIAN_POINT ( 'NONE',  ( -5.153800228976607833, 19.02544592524334988, 47.70942372801900433 ) ) ;
#128477=CARTESIAN_POINT ( 'NONE',  ( -21.53943276465977519, 0.05219959533907696930, 46.24890960531435979 ) ) ;
#128479=CARTESIAN_POINT ( 'NONE',  ( 18.62759615963255655, 10.81492255796105972, 51.66775706135234714 ) ) ;
#128480=CARTESIAN_POINT ( 'NONE',  ( -18.62759615963270932, 10.81492255796079327, 95.83224293864770971 ) ) ;
#128481=CARTESIAN_POINT ( 'NONE',  ( -19.02544592524334988, -5.153800228976617603, 93.95942372801900433 ) ) ;
#128482=CARTESIAN_POINT ( 'NONE',  ( 14.29746914071037800, 8.314922557961029526, 61.66775706135235424 ) ) ;
#128484=CARTESIAN_POINT ( 'NONE',  ( -10.72451020669898014, 18.67979575497178502, 100.4155762719810241 ) ) ;
#128485=CARTESIAN_POINT ( 'NONE',  ( 4.379528057220339221, -16.55341960407611168, 87.70724293864769550 ) ) ;
#128486=CARTESIAN_POINT ( 'NONE',  ( -17.49999999999999289, -5.624438216177589211, 99.18329655085356933 ) ) ;
#128487=CARTESIAN_POINT ( 'NONE',  ( 8.224510206698742110, 14.34966873604972548, 32.08442372801901854 ) ) ;
#128489=CARTESIAN_POINT ( 'NONE',  ( -0.05219959533907301413, -21.53943276465977519, 62.49890960531436690 ) ) ;
#128490=CARTESIAN_POINT ( 'NONE',  ( -0.05219959533934338120, 16.53943276465976808, 97.50109039468567573 ) ) ;
#128491=CARTESIAN_POINT ( 'NONE',  ( 9.474510206698971260, -16.51473224551069308, 27.91557627198103120 ) ) ;
#128492=CARTESIAN_POINT ( 'NONE',  ( 12.06949235617739724, 12.14591786802326823, 61.87609039468568284 ) ) ;
#128493=CARTESIAN_POINT ( 'NONE',  ( -9.474510206698720793, -16.51473224551083518, 54.58442372801899722 ) ) ;
#128494=CARTESIAN_POINT ( 'NONE',  ( 18.62759615963255655, 10.81492255796105972, 41.66775706135235424 ) ) ;
#128495=CARTESIAN_POINT ( 'NONE',  ( -0.05219959533907301413, -21.53943276465977519, 52.49890960531435979 ) ) ;
#128496=CARTESIAN_POINT ( 'NONE',  ( -4.379528057220086978, -16.55341960407618274, 84.79275706135234714 ) ) ;
#128497=CARTESIAN_POINT ( 'NONE',  ( -5.719274019375665041, -21.55341960407619695, 69.79275706135234714 ) ) ;
#128498=CARTESIAN_POINT ( 'NONE',  ( -21.52544592524343514, 5.823673210054127303, 56.04057627198102409 ) ) ;
#128499=CARTESIAN_POINT ( 'NONE',  ( -10.81492255796078084, -18.62759615963271287, 37.08224293864768129 ) ) ;
#128500=CARTESIAN_POINT ( 'NONE',  ( -12.06949235617739369, -12.14591786802326823, 69.37609039468567573 ) ) ;
#128501=CARTESIAN_POINT ( 'NONE',  ( 18.62759615963271287, -10.81492255796078972, 33.33224293864769550 ) ) ;
#128503=CARTESIAN_POINT ( 'NONE',  ( -16.46253265017160317, 9.564922557960807481, 100.8322429386477097 ) ) ;
#128504=CARTESIAN_POINT ( 'NONE',  ( -4.483927247898782831, 16.52544592524335698, 107.7094237280190328 ) ) ;
#128506=CARTESIAN_POINT ( 'NONE',  ( -0.05219959533910754901, -16.53943276465976808, 102.4989096053143811 ) ) ;
#128507=CARTESIAN_POINT ( 'NONE',  ( -21.53943276465977519, 0.05219959533907696930, 61.24890960531435979 ) ) ;
#128508=CARTESIAN_POINT ( 'NONE',  ( -8.224510206698735004, -14.34966873604973081, 84.58442372801903275 ) ) ;
#128509=CARTESIAN_POINT ( 'NONE',  ( -5.823673210054431948, 21.52544592524334988, 47.70942372801902565 ) ) ;
#128510=CARTESIAN_POINT ( 'NONE',  ( 16.46253265017146816, 9.564922557961045513, 106.6677570613523471 ) ) ;
#128511=CARTESIAN_POINT ( 'NONE',  ( 0.05219959533910956823, 16.53943276465976808, 104.9989096053143669 ) ) ;
#128512=CARTESIAN_POINT ( 'NONE',  ( -13.89961937509977652, 13.97604488694528158, 55.62390960531434558 ) ) ;
#128513=CARTESIAN_POINT ( 'NONE',  ( -16.46253265017160317, 9.564922557960807481, 30.83224293864769550 ) ) ;
#128515=CARTESIAN_POINT ( 'NONE',  ( -19.02544592524342804, 5.153800228976336051, 86.04057627198103830 ) ) ;
#128516=CARTESIAN_POINT ( 'NONE',  ( -16.52544592524335698, -4.483927247898792601, 78.95942372801901854 ) ) ;
#128517=CARTESIAN_POINT ( 'NONE',  ( 21.52544592524334988, 5.823673210054432836, 111.4594237280190328 ) ) ;
#128518=CARTESIAN_POINT ( 'NONE',  ( -21.52544592524343514, 5.823673210054127303, 46.04057627198103830 ) ) ;
#128519=CARTESIAN_POINT ( 'NONE',  ( -4.379528057220086978, -16.55341960407618274, 79.79275706135236135 ) ) ;
#128520=CARTESIAN_POINT ( 'NONE',  ( -9.474510206698720793, -16.51473224551083518, 84.58442372801900433 ) ) ;
#128521=VERTEX_POINT ( 'NONE', #151081 ) ;
#128522=CARTESIAN_POINT ( 'NONE',  ( 13.97604488694527802, 13.89961937509977652, 34.37390960531436690 ) ) ;
#128523=CARTESIAN_POINT ( 'NONE',  ( 9.474510206698971260, -16.51473224551069308, 77.91557627198103830 ) ) ;
#128524=CARTESIAN_POINT ( 'NONE',  ( 5.153800228976335163, 19.02544592524342804, 39.79057627198100988 ) ) ;
#128525=CARTESIAN_POINT ( 'NONE',  ( 16.46253265017146816, 9.564922557961045513, 71.66775706135233293 ) ) ;
#128527=CARTESIAN_POINT ( 'NONE',  ( 19.02544592524343514, -5.153800228976328945, 98.54057627198100988 ) ) ;
#128528=CARTESIAN_POINT ( 'NONE',  ( 16.53943276465976808, -0.05219959533910856209, 53.74890960531437401 ) ) ;
#128529=CARTESIAN_POINT ( 'NONE',  ( -15.80617190586745835, -15.72974639402198527, 41.87390960531435979 ) ) ;
#128530=CARTESIAN_POINT ( 'NONE',  ( -17.49999999999999645, 3.565345528327982016, 104.4249448680647419 ) ) ;
#128531=CARTESIAN_POINT ( 'NONE',  ( -5.153800228976607833, 19.02544592524334988, 27.70942372801899722 ) ) ;
#128533=CARTESIAN_POINT ( 'NONE',  ( -5.153800228976328057, -19.02544592524343514, 57.29057627198103120 ) ) ;
#128534=CARTESIAN_POINT ( 'NONE',  ( -12.06949235617739369, -12.14591786802326823, 44.37609039468567573 ) ) ;
#128535=CARTESIAN_POINT ( 'NONE',  ( -18.87255363501903105, -5.500000000000007105, 101.3251374817182437 ) ) ;
#128536=CARTESIAN_POINT ( 'NONE',  ( -16.21995358207304960, 7.366697692864183189, 109.9355100151216220 ) ) ;
#128537=CARTESIAN_POINT ( 'NONE',  ( -8.314922557961024197, 14.29746914071037800, 77.91775706135231871 ) ) ;
#128538=CARTESIAN_POINT ( 'NONE',  ( -21.55341960407610458, -5.719274019375992779, 101.4572429386476955 ) ) ;
#128539=CARTESIAN_POINT ( 'NONE',  ( -4.379528057220086978, -16.55341960407618274, 39.79275706135235424 ) ) ;
#128540=CARTESIAN_POINT ( 'NONE',  ( -16.51473224551069308, -9.474510206698971260, 36.66557627198102409 ) ) ;
#128541=CARTESIAN_POINT ( 'NONE',  ( 10.81492255796106328, -18.62759615963255655, 45.41775706135234003 ) ) ;
#128542=CARTESIAN_POINT ( 'NONE',  ( 16.51473224551083163, -9.474510206698727899, 60.83442372801900433 ) ) ;
#128543=CARTESIAN_POINT ( 'NONE',  ( -0.05219959533937732626, 21.53943276465977519, 92.50109039468567573 ) ) ;
#128544=CARTESIAN_POINT ( 'NONE',  ( -17.60769864724388611, 5.499999999999981348, 48.65024842019164453 ) ) ;
#128545=CARTESIAN_POINT ( 'NONE',  ( 16.52544592524342804, -4.483927247898539470, 43.54057627198103830 ) ) ;
#128547=CARTESIAN_POINT ( 'NONE',  ( 21.52544592524344225, -5.823673210054117533, 53.54057627198103120 ) ) ;
#128549=CARTESIAN_POINT ( 'NONE',  ( 5.153800228976335163, 19.02544592524342804, 104.7905762719809957 ) ) ;
#128550=CARTESIAN_POINT ( 'NONE',  ( -14.34966873604960291, -8.224510206698953496, 106.6655762719810383 ) ) ;
#128551=CARTESIAN_POINT ( 'NONE',  ( -8.224510206698735004, -14.34966873604973081, 29.58442372801901854 ) ) ;
#128553=CARTESIAN_POINT ( 'NONE',  ( -4.483927247898539470, -16.52544592524342804, 22.29057627198102765 ) ) ;
#128555=CARTESIAN_POINT ( 'NONE',  ( -13.89961937509977652, 13.97604488694528158, 100.6239096053143669 ) ) ;
#128557=CARTESIAN_POINT ( 'NONE',  ( -21.52544592524343514, 5.823673210054127303, 106.0405762719810525 ) ) ;
#128558=CARTESIAN_POINT ( 'NONE',  ( 14.29746914071049879, -8.314922557960816363, 28.33224293864769550 ) ) ;
#128560=CARTESIAN_POINT ( 'NONE',  ( -5.153800228976607833, 19.02544592524334988, 92.70942372801901854 ) ) ;
#128561=CARTESIAN_POINT ( 'NONE',  ( 10.72451020669871369, 18.67979575497193778, 102.0844237280190185 ) ) ;
#128562=CARTESIAN_POINT ( 'NONE',  ( -16.55341960407611168, -4.379528057220339221, 36.45724293864768839 ) ) ;
#128563=CARTESIAN_POINT ( 'NONE',  ( -21.55341960407610458, -5.719274019375992779, 86.45724293864770971 ) ) ;
#128564=CARTESIAN_POINT ( 'NONE',  ( -0.05219959533907301413, -21.53943276465977519, 47.49890960531435979 ) ) ;
#128565=CARTESIAN_POINT ( 'NONE',  ( -0.05219959533909027116, -19.03943276465977164, 62.49890960531435979 ) ) ;
#128566=CARTESIAN_POINT ( 'NONE',  ( 14.29746914071049879, -8.314922557960816363, 28.33224293864769550 ) ) ;
#128567=CARTESIAN_POINT ( 'NONE',  ( 16.46253265017160672, -9.564922557960803928, 73.33224293864769550 ) ) ;
#128568=ORIENTED_EDGE ( 'NONE', *, *, #93805, .T. ) ;
#128569=CARTESIAN_POINT ( 'NONE',  ( 19.34837522270365895, 5.499999999999732658, 58.36337684832577821 ) ) ;
#128570=CARTESIAN_POINT ( 'NONE',  ( 13.97604488694548053, -13.89961937509957401, 45.62609039468566863 ) ) ;
#128571=CARTESIAN_POINT ( 'NONE',  ( 5.823673210054125526, 21.52544592524343514, 84.79057627198102409 ) ) ;
#128572=CARTESIAN_POINT ( 'NONE',  ( 16.52544592524342804, -4.483927247898539470, 83.54057627198102409 ) ) ;
#128573=CARTESIAN_POINT ( 'NONE',  ( -5.719274019375665041, -21.55341960407619695, 39.79275706135235424 ) ) ;
#128576=CARTESIAN_POINT ( 'NONE',  ( -16.55341960407617563, 4.379528057220093196, 108.5427570613523756 ) ) ;
#128577=CARTESIAN_POINT ( 'NONE',  ( 16.53943276465976808, -0.05219959533910856209, 113.7489096053143527 ) ) ;
#128578=CARTESIAN_POINT ( 'NONE',  ( 19.03943276465977164, -0.05219959533909143690, 88.74890960531436690 ) ) ;
#128581=CARTESIAN_POINT ( 'NONE',  ( -16.52544592524342804, 4.483927247898546575, 46.04057627198103830 ) ) ;
#128582=CARTESIAN_POINT ( 'NONE',  ( 18.67979575497194134, -10.72451020669871369, 55.83442372801901854 ) ) ;
#128584=CARTESIAN_POINT ( 'NONE',  ( 19.05341960407611168, 5.049401038298154454, 38.95724293864767418 ) ) ;
#128585=CARTESIAN_POINT ( 'NONE',  ( -19.03943276465977164, 0.05219959533909376836, 56.24890960531435979 ) ) ;
#128586=EDGE_LOOP ( 'NONE', ( #165627, #195205, #129456, #15615, #30086, #120981, #20443, #133278 ) ) ;
#128587=CARTESIAN_POINT ( 'NONE',  ( 10.81492255796106328, -18.62759615963255655, 110.4177570613523756 ) ) ;
#128588=CARTESIAN_POINT ( 'NONE',  ( -12.14591786802326823, 12.06949235617739902, 63.12609039468568994 ) ) ;
#128589=CARTESIAN_POINT ( 'NONE',  ( 10.72451020669871369, 18.67979575497193778, 92.08442372801901854 ) ) ;
#128590=CARTESIAN_POINT ( 'NONE',  ( -0.05219959533909027116, -19.03943276465977164, 112.4989096053143669 ) ) ;
#128591=CARTESIAN_POINT ( 'NONE',  ( 16.51473224551083163, -9.474510206698727899, 110.8344237280190043 ) ) ;
#128592=CARTESIAN_POINT ( 'NONE',  ( -0.05219959533937732626, 21.53943276465977519, 67.50109039468568994 ) ) ;
#128593=CARTESIAN_POINT ( 'NONE',  ( 16.53943276465976808, 0.05219959533934440121, 31.25109039468568639 ) ) ;
#128594=CARTESIAN_POINT ( 'NONE',  ( -10.81492255796078084, -18.62759615963271287, 82.08224293864768129 ) ) ;
#128595=CARTESIAN_POINT ( 'NONE',  ( 5.049401038297881783, 19.05341960407617563, 97.29275706135233293 ) ) ;
#128596=CARTESIAN_POINT ( 'NONE',  ( -9.564922557960796823, -16.46253265017161027, 62.08224293864769550 ) ) ;
#128597=CARTESIAN_POINT ( 'NONE',  ( -13.97604488694547697, 13.89961937509957934, 108.1260903946856331 ) ) ;
#128598=CARTESIAN_POINT ( 'NONE',  ( 9.564922557961047289, -16.46253265017146816, 100.4177570613523329 ) ) ;
#128599=CARTESIAN_POINT ( 'NONE',  ( -4.379528057220328563, 16.55341960407611168, 70.20724293864769550 ) ) ;
#128600=CARTESIAN_POINT ( 'NONE',  ( -9.564922557961040184, 16.46253265017147172, 77.91775706135234714 ) ) ;
#128602=CARTESIAN_POINT ( 'NONE',  ( -0.05219959533934338120, 16.53943276465976808, 72.50109039468568994 ) ) ;
#128603=CARTESIAN_POINT ( 'NONE',  ( 15.72974639402199770, -15.80617190586745480, 113.1239096053143953 ) ) ;
#128604=CARTESIAN_POINT ( 'NONE',  ( 13.89961937509977652, -13.97604488694527269, 43.12390960531434558 ) ) ;
#128605=CARTESIAN_POINT ( 'NONE',  ( -13.97604488694527625, -13.89961937509977652, 61.87390960531435979 ) ) ;
#128606=CARTESIAN_POINT ( 'NONE',  ( 16.53943276465976808, 0.05219959533934440121, 71.25109039468568994 ) ) ;
#128610=CARTESIAN_POINT ( 'NONE',  ( -19.03943276465977164, 0.05219959533909376836, 101.2489096053143669 ) ) ;
#128611=CARTESIAN_POINT ( 'NONE',  ( -13.89961937509977652, 13.97604488694528158, 25.62390960531434558 ) ) ;
#128612=ORIENTED_EDGE ( 'NONE', *, *, #15818, .T. ) ;
#128613=CARTESIAN_POINT ( 'NONE',  ( -4.379528057220086978, -16.55341960407618274, 19.79275706135235069 ) ) ;
#128614=CARTESIAN_POINT ( 'NONE',  ( 0.05219959533907565091, 21.53943276465977519, 44.99890960531435979 ) ) ;
#128615=CARTESIAN_POINT ( 'NONE',  ( -16.51473224551082808, 9.474510206698731452, 48.33442372801900433 ) ) ;
#128616=CARTESIAN_POINT ( 'NONE',  ( 4.379528057220092307, 16.55341960407617563, 32.29275706135235424 ) ) ;
#128617=CARTESIAN_POINT ( 'NONE',  ( -13.97604488694527625, -13.89961937509977652, 26.87390960531434558 ) ) ;
#128618=CARTESIAN_POINT ( 'NONE',  ( 19.03943276465977164, -0.05219959533909143690, 53.74890960531436690 ) ) ;
#128619=CARTESIAN_POINT ( 'NONE',  ( -15.80617190586745835, -15.72974639402198527, 91.87390960531436690 ) ) ;
#128620=CARTESIAN_POINT ( 'NONE',  ( 16.46253265017160672, -9.564922557960803928, 113.3322429386476955 ) ) ;
#128621=CARTESIAN_POINT ( 'NONE',  ( -19.02544592524342804, 5.153800228976336051, 51.04057627198103120 ) ) ;
#128623=CARTESIAN_POINT ( 'NONE',  ( -9.474510206698720793, -16.51473224551083518, 94.58442372801900433 ) ) ;
#128624=CARTESIAN_POINT ( 'NONE',  ( -4.379528057220328563, 16.55341960407611168, 60.20724293864768839 ) ) ;
#128625=CARTESIAN_POINT ( 'NONE',  ( 10.72451020669871369, 18.67979575497193778, 102.0844237280190185 ) ) ;
#128626=CARTESIAN_POINT ( 'NONE',  ( -15.80617190586745835, -15.72974639402198527, 96.87390960531436690 ) ) ;
#128627=CARTESIAN_POINT ( 'NONE',  ( 21.55341960407619695, -5.719274019375665929, 91.04275706135236135 ) ) ;
#128628=CARTESIAN_POINT ( 'NONE',  ( 13.89961937509977652, -13.97604488694527269, 23.12390960531436335 ) ) ;
#128629=CARTESIAN_POINT ( 'NONE',  ( -18.62759615963255300, -10.81492255796106328, 79.16775706135234714 ) ) ;
#128630=CARTESIAN_POINT ( 'NONE',  ( -8.314922557960811034, -14.29746914071050412, 27.08224293864769550 ) ) ;
#128631=CARTESIAN_POINT ( 'NONE',  ( -21.55341960407619339, 5.719274019375674811, 73.54275706135234714 ) ) ;
#128632=CARTESIAN_POINT ( 'NONE',  ( 19.05341960407611168, 5.049401038298154454, 68.95724293864769550 ) ) ;
#128633=CARTESIAN_POINT ( 'NONE',  ( 15.72974639402176855, 15.80617190586768217, 46.87609039468568994 ) ) ;
#128634=CARTESIAN_POINT ( 'NONE',  ( 9.474510206698971260, -16.51473224551069308, 82.91557627198103830 ) ) ;
#128635=CARTESIAN_POINT ( 'NONE',  ( 8.314922557960818139, 14.29746914071049879, 94.58224293864769550 ) ) ;
#128636=CARTESIAN_POINT ( 'NONE',  ( -12.14591786802309592, -12.06949235617757132, 66.87390960531436690 ) ) ;
#128637=CARTESIAN_POINT ( 'NONE',  ( -21.55341960407610458, -5.719274019375992779, 66.45724293864768129 ) ) ;
#128638=CARTESIAN_POINT ( 'NONE',  ( -13.97604488694527625, -13.89961937509977652, 66.87390960531436690 ) ) ;
#128639=CARTESIAN_POINT ( 'NONE',  ( -15.72974639402197994, 15.80617190586746368, 75.62390960531439532 ) ) ;
#128640=CARTESIAN_POINT ( 'NONE',  ( 16.51473224551083163, -9.474510206698727899, 70.83442372801900433 ) ) ;
#128641=CARTESIAN_POINT ( 'NONE',  ( -13.97604488694547520, 13.89961937509957934, 38.12609039468566152 ) ) ;
#128642=CARTESIAN_POINT ( 'NONE',  ( -4.483927247898539470, -16.52544592524342804, 82.29057627198103830 ) ) ;
#128643=CARTESIAN_POINT ( 'NONE',  ( 5.719274019375991003, -21.55341960407610458, 57.70724293864770260 ) ) ;
#128644=CARTESIAN_POINT ( 'NONE',  ( 17.50000000000000000, 5.624438216177590100, 101.6832965508535835 ) ) ;
#128645=CARTESIAN_POINT ( 'NONE',  ( 16.53943276465976808, 0.05219959533934440121, 101.2510903946856757 ) ) ;
#128647=CARTESIAN_POINT ( 'NONE',  ( 13.97604488694548053, -13.89961937509957401, 95.62609039468563310 ) ) ;
#128648=CARTESIAN_POINT ( 'NONE',  ( 12.14591786802309770, 12.06949235617756955, 74.37390960531436690 ) ) ;
#128650=CARTESIAN_POINT ( 'NONE',  ( -19.03943276465977164, 0.05219959533909376836, 56.24890960531435979 ) ) ;
#128651=CARTESIAN_POINT ( 'NONE',  ( 16.55341960407611168, 4.379528057220329451, 53.95724293864770260 ) ) ;
#128652=CARTESIAN_POINT ( 'NONE',  ( -13.97604488694527625, -13.89961937509977652, 106.8739096053143669 ) ) ;
#128653=CARTESIAN_POINT ( 'NONE',  ( 5.049401038297881783, 19.05341960407617563, 72.29275706135234714 ) ) ;
#128654=CARTESIAN_POINT ( 'NONE',  ( -16.51473224551069308, -9.474510206698971260, 66.66557627198102409 ) ) ;
#128655=CARTESIAN_POINT ( 'NONE',  ( -19.03943276465977164, 0.05219959533909376836, 91.24890960531436690 ) ) ;
#128656=CARTESIAN_POINT ( 'NONE',  ( 16.51473224551069308, 9.474510206698969483, 69.16557627198102409 ) ) ;
#128657=CARTESIAN_POINT ( 'NONE',  ( -10.81492255796078084, -18.62759615963271287, 67.08224293864770971 ) ) ;
#128658=CARTESIAN_POINT ( 'NONE',  ( 0.05219959533934541429, -16.53943276465976808, 55.00109039468568284 ) ) ;
#128659=CARTESIAN_POINT ( 'NONE',  ( 17.60779699588841041, 5.499999999999981348, 98.84981316670102558 ) ) ;
#128660=CARTESIAN_POINT ( 'NONE',  ( 9.564922557960805705, 16.46253265017160317, 49.58224293864770260 ) ) ;
#128661=CARTESIAN_POINT ( 'NONE',  ( 21.55341960407610458, 5.719274019375980345, 48.95724293864770971 ) ) ;
#128662=CARTESIAN_POINT ( 'NONE',  ( 19.02544592524334988, 5.153800228976608722, 91.45942372801900433 ) ) ;
#128663=CARTESIAN_POINT ( 'NONE',  ( 12.14591786802309770, 12.06949235617756955, 24.37390960531435979 ) ) ;
#128664=CARTESIAN_POINT ( 'NONE',  ( 0.05219959533937995610, -21.53943276465977519, 35.00109039468568284 ) ) ;
#128665=CARTESIAN_POINT ( 'NONE',  ( 9.564922557961047289, -16.46253265017146816, 35.41775706135233293 ) ) ;
#128666=CARTESIAN_POINT ( 'NONE',  ( 0.05219959533934541429, -16.53943276465976808, 65.00109039468568994 ) ) ;
#128667=CARTESIAN_POINT ( 'NONE',  ( -12.06949235617739369, -12.14591786802326823, 94.37609039468568994 ) ) ;
#128669=CARTESIAN_POINT ( 'NONE',  ( 8.314922557961029526, -14.29746914071037800, 80.41775706135234714 ) ) ;
#128670=CARTESIAN_POINT ( 'NONE',  ( -10.81492255796078084, -18.62759615963271287, 32.08224293864769550 ) ) ;
#128671=CARTESIAN_POINT ( 'NONE',  ( -14.29746914071037622, -8.314922557961029526, 29.16775706135234003 ) ) ;
#128672=CARTESIAN_POINT ( 'NONE',  ( 16.51473224551069308, 9.474510206698969483, 39.16557627198103120 ) ) ;
#128673=CARTESIAN_POINT ( 'NONE',  ( 0.05219959533909260263, 19.03943276465977164, 54.99890960531435979 ) ) ;
#128674=CARTESIAN_POINT ( 'NONE',  ( 13.89961937509977652, -13.97604488694527269, 63.12390960531435979 ) ) ;
#128675=CARTESIAN_POINT ( 'NONE',  ( 21.53943276465977519, 0.05219959533937863772, 41.25109039468568284 ) ) ;
#128676=CARTESIAN_POINT ( 'NONE',  ( 12.14591786802327356, -12.06949235617739191, 55.62609039468568284 ) ) ;
#128677=CARTESIAN_POINT ( 'NONE',  ( 16.53943276465976808, 0.05219959533934440121, 106.2510903946856757 ) ) ;
#128678=CARTESIAN_POINT ( 'NONE',  ( -13.97604488694527625, -13.89961937509977652, 31.87390960531435979 ) ) ;
#128679=CARTESIAN_POINT ( 'NONE',  ( -10.72451020669870658, -18.67979575497194134, 109.5844237280190328 ) ) ;
#128680=CARTESIAN_POINT ( 'NONE',  ( -14.29746914071037622, -8.314922557961029526, 19.16775706135234714 ) ) ;
#128681=CARTESIAN_POINT ( 'NONE',  ( 13.89961937509957401, 13.97604488694547697, 71.87609039468567573 ) ) ;
#128682=CARTESIAN_POINT ( 'NONE',  ( 16.55341960407611168, 4.379528057220329451, 63.95724293864770260 ) ) ;
#128683=CARTESIAN_POINT ( 'NONE',  ( -0.05219959533909027116, -19.03943276465977164, 32.49890960531435979 ) ) ;
#128684=CARTESIAN_POINT ( 'NONE',  ( 19.02544592524334988, 5.153800228976608722, 71.45942372801900433 ) ) ;
#128685=CARTESIAN_POINT ( 'NONE',  ( 17.50000000000000000, 5.499999999999992895, 76.70309617465829888 ) ) ;
#128686=CARTESIAN_POINT ( 'NONE',  ( -5.823673210054431948, 21.52544592524334988, 77.70942372801900433 ) ) ;
#128687=CARTESIAN_POINT ( 'NONE',  ( -8.224510206698735004, -14.34966873604973081, 34.58442372801900433 ) ) ;
#128688=CARTESIAN_POINT ( 'NONE',  ( -17.60728821186565085, 5.500000000000021316, 90.86690927743005375 ) ) ;
#128689=CARTESIAN_POINT ( 'NONE',  ( 0.05219959533907565091, 21.53943276465977519, 29.99890960531435979 ) ) ;
#128690=CARTESIAN_POINT ( 'NONE',  ( -16.52544592524335698, -4.483927247898792601, 23.95942372801901143 ) ) ;
#128691=CARTESIAN_POINT ( 'NONE',  ( 0.05219959533909260263, 19.03943276465977164, 24.99890960531435269 ) ) ;
#128692=CARTESIAN_POINT ( 'NONE',  ( 19.02544592524334988, 5.153800228976608722, 31.45942372801900433 ) ) ;
#128694=CARTESIAN_POINT ( 'NONE',  ( -5.153800228976328057, -19.02544592524343514, 42.29057627198101699 ) ) ;
#128696=CARTESIAN_POINT ( 'NONE',  ( 16.51473224551069308, 9.474510206698969483, 54.16557627198103120 ) ) ;
#128697=CARTESIAN_POINT ( 'NONE',  ( -18.22780087662122028, 5.500000000000031086, 98.51540105326105845 ) ) ;
#128698=CARTESIAN_POINT ( 'NONE',  ( -5.823673210054431948, 21.52544592524334988, 112.7094237280190328 ) ) ;
#128699=CARTESIAN_POINT ( 'NONE',  ( -16.53943276465976808, 0.05219959533911058130, 21.24890960531436690 ) ) ;
#128700=CARTESIAN_POINT ( 'NONE',  ( 5.049401038298161559, -19.05341960407611168, 27.70724293864769550 ) ) ;
#128701=CARTESIAN_POINT ( 'NONE',  ( 19.05341960407611168, 5.049401038298154454, 93.95724293864769550 ) ) ;
#128702=CARTESIAN_POINT ( 'NONE',  ( 0.05219959533937995610, -21.53943276465977519, 70.00109039468568994 ) ) ;
#128703=CARTESIAN_POINT ( 'NONE',  ( -13.89961937509977652, 13.97604488694528158, 35.62390960531435269 ) ) ;
#128704=CARTESIAN_POINT ( 'NONE',  ( -10.81492255796105439, 18.62759615963255655, 62.91775706135236135 ) ) ;
#128705=CARTESIAN_POINT ( 'NONE',  ( -9.564922557961040184, 16.46253265017147172, 97.91775706135233293 ) ) ;
#128706=CARTESIAN_POINT ( 'NONE',  ( 18.62759615963271287, -10.81492255796078972, 23.33224293864769194 ) ) ;
#128707=CARTESIAN_POINT ( 'NONE',  ( 5.049401038298161559, -19.05341960407611168, 37.70724293864768839 ) ) ;
#128708=CARTESIAN_POINT ( 'NONE',  ( -10.72451020669898014, 18.67979575497178502, 105.4155762719810383 ) ) ;
#128709=CARTESIAN_POINT ( 'NONE',  ( -13.89961937509957401, -13.97604488694547875, 29.37609039468565797 ) ) ;
#128710=CARTESIAN_POINT ( 'NONE',  ( 16.52544592524342804, -4.483927247898539470, 108.5405762719810241 ) ) ;
#128711=CARTESIAN_POINT ( 'NONE',  ( -19.03943276465977164, 0.05219959533909376836, 66.24890960531436690 ) ) ;
#128712=CARTESIAN_POINT ( 'NONE',  ( -19.02544592524334988, -5.153800228976617603, 93.95942372801900433 ) ) ;
#128713=CARTESIAN_POINT ( 'NONE',  ( 8.224510206698953496, -14.34966873604960469, 72.91557627198103830 ) ) ;
#128714=CARTESIAN_POINT ( 'NONE',  ( 15.80617190586746368, 15.72974639402197994, 24.37390960531435979 ) ) ;
#128715=CARTESIAN_POINT ( 'NONE',  ( -5.153800228976607833, 19.02544592524334988, 82.70942372801897591 ) ) ;
#128716=CARTESIAN_POINT ( 'NONE',  ( -15.80617190586745835, -15.72974639402198527, 86.87390960531438111 ) ) ;
#128717=CARTESIAN_POINT ( 'NONE',  ( -0.05219959533937732626, 21.53943276465977519, 42.50109039468567573 ) ) ;
#128718=CARTESIAN_POINT ( 'NONE',  ( -0.05219959533934338120, 16.53943276465976808, 47.50109039468568994 ) ) ;
#128719=CARTESIAN_POINT ( 'NONE',  ( -14.29746914071037622, -8.314922557961029526, 49.16775706135234003 ) ) ;
#128720=CARTESIAN_POINT ( 'NONE',  ( -10.72451020669870658, -18.67979575497194134, 54.58442372801901143 ) ) ;
#128721=CARTESIAN_POINT ( 'NONE',  ( -21.55341960407610458, -5.719274019375992779, 61.45724293864770260 ) ) ;
#128722=CARTESIAN_POINT ( 'NONE',  ( -19.05341960407611168, -5.049401038298163336, 46.45724293864768129 ) ) ;
#128724=CARTESIAN_POINT ( 'NONE',  ( -16.55341960407617563, 4.379528057220093196, 78.54275706135236135 ) ) ;
#128726=CARTESIAN_POINT ( 'NONE',  ( 21.52544592524344225, -5.823673210054117533, 98.54057627198105251 ) ) ;
#128727=CARTESIAN_POINT ( 'NONE',  ( 16.52544592524342804, -4.483927247898539470, 58.54057627198103120 ) ) ;
#128728=CARTESIAN_POINT ( 'NONE',  ( 12.14591786802327356, -12.06949235617739191, 65.62609039468568994 ) ) ;
#128729=CARTESIAN_POINT ( 'NONE',  ( 5.153800228976615827, -19.02544592524334988, 100.2094237280190043 ) ) ;
#128730=CARTESIAN_POINT ( 'NONE',  ( -0.05219959533907301413, -21.53943276465977519, 97.49890960531436690 ) ) ;
#128731=CARTESIAN_POINT ( 'NONE',  ( -16.55341960407611168, -4.379528057220339221, 51.45724293864770260 ) ) ;
#128733=CARTESIAN_POINT ( 'NONE',  ( -4.379528057220086978, -16.55341960407618274, 79.79275706135236135 ) ) ;
#128735=CARTESIAN_POINT ( 'NONE',  ( 15.72974639402199770, -15.80617190586745480, 73.12390960531436690 ) ) ;
#128736=CARTESIAN_POINT ( 'NONE',  ( 4.379528057220339221, -16.55341960407611168, 32.70724293864770260 ) ) ;
#128738=CARTESIAN_POINT ( 'NONE',  ( -16.36317988757057407, -7.306389748694946285, 55.90210391636774290 ) ) ;
#128739=CARTESIAN_POINT ( 'NONE',  ( -21.55341960407610458, -5.719274019375992779, 101.4572429386476955 ) ) ;
#128740=CARTESIAN_POINT ( 'NONE',  ( -15.72974639402197994, 15.80617190586746368, 110.6239096053143669 ) ) ;
#128741=CARTESIAN_POINT ( 'NONE',  ( -8.314922557960811034, -14.29746914071050412, 32.08224293864769550 ) ) ;
#128742=CARTESIAN_POINT ( 'NONE',  ( 14.34966873604972726, -8.224510206698740333, 45.83442372801901854 ) ) ;
#128743=CARTESIAN_POINT ( 'NONE',  ( -19.03943276465977164, 0.05219959533909376836, 51.24890960531436690 ) ) ;
#128744=CARTESIAN_POINT ( 'NONE',  ( -16.51473224551069308, -9.474510206698971260, 66.66557627198102409 ) ) ;
#128745=EDGE_LOOP ( 'NONE', ( #71910, #175561, #195044, #122657 ) ) ;
#128746=CARTESIAN_POINT ( 'NONE',  ( -21.52544592524343514, 5.823673210054127303, 26.04057627198103475 ) ) ;
#128748=CARTESIAN_POINT ( 'NONE',  ( 13.89961937509957401, 13.97604488694547697, 101.8760903946856331 ) ) ;
#128749=CARTESIAN_POINT ( 'NONE',  ( 5.049401038297881783, 19.05341960407617563, 52.29275706135234003 ) ) ;
#128750=CARTESIAN_POINT ( 'NONE',  ( -5.823673210054116645, -21.52544592524344225, 107.2905762719810525 ) ) ;
#128751=CARTESIAN_POINT ( 'NONE',  ( 12.06949235617757843, -12.14591786802309237, 33.12390960531435979 ) ) ;
#128752=CARTESIAN_POINT ( 'NONE',  ( 5.049401038298161559, -19.05341960407611168, 77.70724293864765286 ) ) ;
#128753=CARTESIAN_POINT ( 'NONE',  ( -10.72451020669898014, 18.67979575497178502, 50.41557627198103120 ) ) ;
#128754=CARTESIAN_POINT ( 'NONE',  ( -18.67979575497178146, -10.72451020669898902, 81.66557627198103830 ) ) ;
#128755=CARTESIAN_POINT ( 'NONE',  ( 12.06949235617739724, 12.14591786802326823, 21.87609039468567573 ) ) ;
#128756=CARTESIAN_POINT ( 'NONE',  ( 18.62759615963271287, -10.81492255796078972, 28.33224293864769550 ) ) ;
#128757=CARTESIAN_POINT ( 'NONE',  ( 15.80617190586769283, -15.72974639402175789, 75.62609039468567573 ) ) ;
#128758=CARTESIAN_POINT ( 'NONE',  ( 9.474510206698971260, -16.51473224551069308, 72.91557627198102409 ) ) ;
#128759=CARTESIAN_POINT ( 'NONE',  ( -5.153800228976328057, -19.02544592524343514, 27.29057627198103120 ) ) ;
#128760=CARTESIAN_POINT ( 'NONE',  ( 5.153800228976335163, 19.02544592524342804, 79.79057627198102409 ) ) ;
#128761=CARTESIAN_POINT ( 'NONE',  ( -12.06949235617756955, 12.14591786802309770, 95.62390960531436690 ) ) ;
#128763=CARTESIAN_POINT ( 'NONE',  ( -16.51473224551082808, 9.474510206698731452, 103.3344237280190043 ) ) ;
#128765=CARTESIAN_POINT ( 'NONE',  ( 19.05341960407611168, 5.049401038298154454, 78.95724293864769550 ) ) ;
#128766=CARTESIAN_POINT ( 'NONE',  ( -0.05219959533937732626, 21.53943276465977519, 87.50109039468568994 ) ) ;
#128767=CARTESIAN_POINT ( 'NONE',  ( -5.823673210054116645, -21.52544592524344225, 22.29057627198102765 ) ) ;
#128768=CARTESIAN_POINT ( 'NONE',  ( 0.05219959533934541429, -16.53943276465976808, 75.00109039468568994 ) ) ;
#128770=CARTESIAN_POINT ( 'NONE',  ( 5.049401038297881783, 19.05341960407617563, 52.29275706135234003 ) ) ;
#128771=CARTESIAN_POINT ( 'NONE',  ( -10.81492255796105439, 18.62759615963255655, 112.9177570613523329 ) ) ;
#128775=CARTESIAN_POINT ( 'NONE',  ( 4.483927247898545687, 16.52544592524342804, 29.79057627198102409 ) ) ;
#128776=DIRECTION ( 'NONE',  ( -1.000000000000000000, 0.000000000000000000, 0.000000000000000000 ) ) ;
#128777=CARTESIAN_POINT ( 'NONE',  ( -0.05219959533934338120, 16.53943276465976808, 102.5010903946856899 ) ) ;
#128779=CARTESIAN_POINT ( 'NONE',  ( -16.55341960407617563, 4.379528057220093196, 83.54275706135234714 ) ) ;
#128780=CARTESIAN_POINT ( 'NONE',  ( -18.67979575497193778, 10.72451020669871902, 98.33442372801901854 ) ) ;
#128781=CARTESIAN_POINT ( 'NONE',  ( 19.05341960407617918, -5.049401038297876454, 101.0427570613523045 ) ) ;
#128782=CARTESIAN_POINT ( 'NONE',  ( 10.81492255796106328, -18.62759615963255655, 70.41775706135236135 ) ) ;
#128783=CARTESIAN_POINT ( 'NONE',  ( 13.97604488694548053, -13.89961937509957401, 35.62609039468567573 ) ) ;
#128784=CARTESIAN_POINT ( 'NONE',  ( 13.89961937509977652, -13.97604488694527269, 83.12390960531436690 ) ) ;
#128785=CARTESIAN_POINT ( 'NONE',  ( -5.153800228976328057, -19.02544592524343514, 62.29057627198100988 ) ) ;
#128787=CARTESIAN_POINT ( 'NONE',  ( -10.72451020669898014, 18.67979575497178502, 90.41557627198103830 ) ) ;
#128788=CARTESIAN_POINT ( 'NONE',  ( 21.52544592524344225, -5.823673210054117533, 48.54057627198103120 ) ) ;
#128789=CARTESIAN_POINT ( 'NONE',  ( -9.564922557960796823, -16.46253265017161027, 42.08224293864769550 ) ) ;
#128790=CARTESIAN_POINT ( 'NONE',  ( 0.05219959533934541429, -16.53943276465976808, 70.00109039468568994 ) ) ;
#128791=EDGE_CURVE ( 'NONE', #186347, #65463, #45135, .T. ) ;
#128793=CARTESIAN_POINT ( 'NONE',  ( -5.823673210054431948, 21.52544592524334988, 47.70942372801902565 ) ) ;
#128794=CARTESIAN_POINT ( 'NONE',  ( 14.34966873604960469, 8.224510206698951720, 69.16557627198102409 ) ) ;
#128796=CARTESIAN_POINT ( 'NONE',  ( 14.34966873604972726, -8.224510206698740333, 40.83442372801901854 ) ) ;
#128797=CARTESIAN_POINT ( 'NONE',  ( 4.483927247898545687, 16.52544592524342804, 104.7905762719810241 ) ) ;
#128798=CARTESIAN_POINT ( 'NONE',  ( 5.153800228976615827, -19.02544592524334988, 50.20942372801897591 ) ) ;
#128799=CARTESIAN_POINT ( 'NONE',  ( -16.53943276465976808, 0.05219959533911058130, 76.24890960531435269 ) ) ;
#128800=CARTESIAN_POINT ( 'NONE',  ( 10.81492255796106328, -18.62759615963255655, 35.41775706135234003 ) ) ;
#128802=CARTESIAN_POINT ( 'NONE',  ( -21.55341960407610458, -5.719274019375992779, 91.45724293864769550 ) ) ;
#128803=CARTESIAN_POINT ( 'NONE',  ( -9.564922557960796823, -16.46253265017161027, 97.08224293864769550 ) ) ;
#128804=CARTESIAN_POINT ( 'NONE',  ( 14.29746914071049879, -8.314922557960816363, 73.33224293864769550 ) ) ;
#128805=CARTESIAN_POINT ( 'NONE',  ( 19.03943276465977164, -0.05219959533909143690, 113.7489096053143669 ) ) ;
#128807=CARTESIAN_POINT ( 'NONE',  ( 5.153800228976615827, -19.02544592524334988, 85.20942372801900433 ) ) ;
#128808=CARTESIAN_POINT ( 'NONE',  ( 18.67979575497194134, -10.72451020669871369, 25.83442372801901499 ) ) ;
#128809=CARTESIAN_POINT ( 'NONE',  ( -19.02544592524342804, 5.153800228976336051, 71.04057627198099567 ) ) ;
#128810=CARTESIAN_POINT ( 'NONE',  ( 13.89961937509957401, 13.97604488694547697, 56.87609039468564731 ) ) ;
#128811=CARTESIAN_POINT ( 'NONE',  ( 9.564922557960805705, 16.46253265017160317, 39.58224293864768839 ) ) ;
#128812=CARTESIAN_POINT ( 'NONE',  ( 8.314922557960818139, 14.29746914071049879, 59.58224293864770260 ) ) ;
#128813=CARTESIAN_POINT ( 'NONE',  ( -8.224510206698948167, 14.34966873604960824, 60.41557627198102409 ) ) ;
#128814=CARTESIAN_POINT ( 'NONE',  ( 9.474510206698971260, -16.51473224551069308, 72.91557627198102409 ) ) ;
#128815=CARTESIAN_POINT ( 'NONE',  ( 21.52544592524344225, -5.823673210054117533, 88.54057627198103830 ) ) ;
#128816=CARTESIAN_POINT ( 'NONE',  ( -13.89961937509977652, 13.97604488694528158, 75.62390960531438111 ) ) ;
#128817=CARTESIAN_POINT ( 'NONE',  ( 5.719274019375991003, -21.55341960407610458, 82.70724293864770971 ) ) ;
#128818=CARTESIAN_POINT ( 'NONE',  ( -0.05219959533936034679, 19.03943276465977164, 22.50109039468566152 ) ) ;
#128820=CARTESIAN_POINT ( 'NONE',  ( 0.05219959533934541429, -16.53943276465976808, 110.0010903946856757 ) ) ;
#128821=CARTESIAN_POINT ( 'NONE',  ( 12.06949235617757843, -12.14591786802309237, 93.12390960531436690 ) ) ;
#128822=CARTESIAN_POINT ( 'NONE',  ( 5.153800228976615827, -19.02544592524334988, 95.20942372801897591 ) ) ;
#128824=CARTESIAN_POINT ( 'NONE',  ( 21.55341960407619695, -5.719274019375665929, 21.04275706135234714 ) ) ;
#128825=CARTESIAN_POINT ( 'NONE',  ( 0.05219959533936267826, -19.03943276465977164, 50.00109039468566863 ) ) ;
#128826=CARTESIAN_POINT ( 'NONE',  ( 16.52544592524335698, 4.483927247898782831, 101.4594237280190185 ) ) ;
#128827=CARTESIAN_POINT ( 'NONE',  ( 13.89961937509957401, 13.97604488694547697, 46.87609039468565442 ) ) ;
#128828=CARTESIAN_POINT ( 'NONE',  ( 16.51473224551069308, 9.474510206698969483, 104.1655762719810241 ) ) ;
#128829=CARTESIAN_POINT ( 'NONE',  ( 16.55341960407611168, 4.379528057220329451, 58.95724293864770971 ) ) ;
#128831=CARTESIAN_POINT ( 'NONE',  ( -13.97604488694527625, -13.89961937509977652, 36.87390960531436690 ) ) ;
#128832=CARTESIAN_POINT ( 'NONE',  ( -21.55341960407619339, 5.719274019375674811, 113.5427570613523756 ) ) ;
#128833=CARTESIAN_POINT ( 'NONE',  ( -16.52544592524335698, -4.483927247898792601, 73.95942372801901854 ) ) ;
#128834=CARTESIAN_POINT ( 'NONE',  ( -0.05219959533937732626, 21.53943276465977519, 37.50109039468568284 ) ) ;
#128835=CARTESIAN_POINT ( 'NONE',  ( -8.314922557961024197, 14.29746914071037800, 37.91775706135235424 ) ) ;
#128836=CARTESIAN_POINT ( 'NONE',  ( -16.46253265017160317, 9.564922557960807481, 110.8322429386476955 ) ) ;
#128837=CARTESIAN_POINT ( 'NONE',  ( 9.474510206698971260, -16.51473224551069308, 52.91557627198102409 ) ) ;
#128838=CARTESIAN_POINT ( 'NONE',  ( 13.97604488694527802, 13.89961937509977652, 64.37390960531436690 ) ) ;
#128839=CARTESIAN_POINT ( 'NONE',  ( 16.55341960407618274, -4.379528057220086978, 46.04275706135234714 ) ) ;
#128840=CARTESIAN_POINT ( 'NONE',  ( 14.34966873604960469, 8.224510206698951720, 109.1655762719810383 ) ) ;
#128841=CARTESIAN_POINT ( 'NONE',  ( -16.53943276465976808, 0.05219959533911058130, 21.24890960531436690 ) ) ;
#128843=CARTESIAN_POINT ( 'NONE',  ( -0.05219959533937732626, 21.53943276465977519, 57.50109039468568994 ) ) ;
#128844=CARTESIAN_POINT ( 'NONE',  ( 13.89961937509977652, -13.97604488694527269, 88.12390960531438111 ) ) ;
#128845=CARTESIAN_POINT ( 'NONE',  ( 9.474510206698971260, -16.51473224551069308, 57.91557627198103120 ) ) ;
#128846=CARTESIAN_POINT ( 'NONE',  ( 13.89961937509977652, -13.97604488694527269, 93.12390960531436690 ) ) ;
#128847=CARTESIAN_POINT ( 'NONE',  ( -4.379528057220328563, 16.55341960407611168, 45.20724293864769550 ) ) ;
#128848=CARTESIAN_POINT ( 'NONE',  ( 16.52544592524342804, -4.483927247898539470, 23.54057627198102765 ) ) ;
#128849=CARTESIAN_POINT ( 'NONE',  ( -14.34966873604960291, -8.224510206698953496, 36.66557627198103120 ) ) ;
#128850=VERTEX_POINT ( 'NONE', #169196 ) ;
#128852=CARTESIAN_POINT ( 'NONE',  ( -5.049401038298153566, 19.05341960407611168, 65.20724293864765286 ) ) ;
#128853=CARTESIAN_POINT ( 'NONE',  ( -19.03943276465977164, -0.05219959533935918106, 43.75109039468566863 ) ) ;
#128855=CARTESIAN_POINT ( 'NONE',  ( 18.22780087662121673, 5.500000000000056843, 58.98459894673892023 ) ) ;
#128856=CARTESIAN_POINT ( 'NONE',  ( -5.153800228976607833, 19.02544592524334988, 82.70942372801897591 ) ) ;
#128857=CARTESIAN_POINT ( 'NONE',  ( 0.05219959533934541429, -16.53943276465976808, 65.00109039468568994 ) ) ;
#128858=CARTESIAN_POINT ( 'NONE',  ( 16.31925111598456013, 7.325300261831534598, 92.33575461032747000 ) ) ;
#128859=CARTESIAN_POINT ( 'NONE',  ( -13.97604488694527625, -13.89961937509977652, 91.87390960531432427 ) ) ;
#128860=CARTESIAN_POINT ( 'NONE',  ( 15.72974639402176855, 15.80617190586768217, 21.87609039468567573 ) ) ;
#128861=CARTESIAN_POINT ( 'NONE',  ( -19.03943276465977164, -0.05219959533935918106, 88.75109039468567573 ) ) ;
#128863=CARTESIAN_POINT ( 'NONE',  ( 5.049401038298161559, -19.05341960407611168, 47.70724293864770260 ) ) ;
#128864=CARTESIAN_POINT ( 'NONE',  ( -5.049401038298153566, 19.05341960407611168, 85.20724293864766707 ) ) ;
#128865=CARTESIAN_POINT ( 'NONE',  ( 16.55341960407611168, 4.379528057220329451, 53.95724293864770260 ) ) ;
#128866=CARTESIAN_POINT ( 'NONE',  ( -19.02544592524342804, 5.153800228976336051, 56.04057627198100988 ) ) ;
#128867=CARTESIAN_POINT ( 'NONE',  ( -13.89961937509957401, -13.97604488694547875, 64.37609039468567573 ) ) ;
#128868=CARTESIAN_POINT ( 'NONE',  ( 12.06949235617757843, -12.14591786802309237, 88.12390960531436690 ) ) ;
#128869=CARTESIAN_POINT ( 'NONE',  ( -19.05341960407617563, 5.049401038297882671, 23.54275706135233648 ) ) ;
#128870=CARTESIAN_POINT ( 'NONE',  ( -0.05219959533909027116, -19.03943276465977164, 67.49890960531436690 ) ) ;
#128871=CARTESIAN_POINT ( 'NONE',  ( -5.823673210054116645, -21.52544592524344225, 57.29057627198103120 ) ) ;
#128872=CARTESIAN_POINT ( 'NONE',  ( 12.06949235617757843, -12.14591786802309237, 63.12390960531435979 ) ) ;
#128873=CARTESIAN_POINT ( 'NONE',  ( 18.67979575497194134, -10.72451020669871369, 110.8344237280190043 ) ) ;
#128874=CARTESIAN_POINT ( 'NONE',  ( 5.049401038298161559, -19.05341960407611168, 107.7072429386476955 ) ) ;
#128875=CARTESIAN_POINT ( 'NONE',  ( -0.05219959533907301413, -21.53943276465977519, 27.49890960531435269 ) ) ;
#128876=CARTESIAN_POINT ( 'NONE',  ( -9.564922557960796823, -16.46253265017161027, 47.08224293864769550 ) ) ;
#128877=CARTESIAN_POINT ( 'NONE',  ( -0.05219959533909027116, -19.03943276465977164, 32.49890960531435979 ) ) ;
#128878=CARTESIAN_POINT ( 'NONE',  ( -16.53943276465976808, 0.05219959533911058130, 106.2489096053143811 ) ) ;
#128879=CARTESIAN_POINT ( 'NONE',  ( -21.52544592524334988, -5.823673210054445271, 18.95942372801901143 ) ) ;
#128880=CARTESIAN_POINT ( 'NONE',  ( -16.51473224551069308, -9.474510206698971260, 96.66557627198102409 ) ) ;
#128881=CARTESIAN_POINT ( 'NONE',  ( -21.55341960407619339, 5.719274019375674811, 23.54275706135235424 ) ) ;
#128882=CARTESIAN_POINT ( 'NONE',  ( 9.564922557960805705, 16.46253265017160317, 109.5822429386476955 ) ) ;
#128883=CARTESIAN_POINT ( 'NONE',  ( -19.03943276465977164, 0.05219959533909376836, 21.24890960531436335 ) ) ;
#128884=CARTESIAN_POINT ( 'NONE',  ( -18.62759615963255300, -10.81492255796106328, 74.16775706135231871 ) ) ;
#128885=CARTESIAN_POINT ( 'NONE',  ( -0.05219959533907301413, -21.53943276465977519, 92.49890960531436690 ) ) ;
#128886=DIRECTION ( 'NONE',  ( 0.000000000000000000, 0.000000000000000000, -1.000000000000000000 ) ) ;
#128889=CARTESIAN_POINT ( 'NONE',  ( 4.483927247898790824, -16.52544592524335698, 50.20942372801901854 ) ) ;
#128890=CARTESIAN_POINT ( 'NONE',  ( -16.53943276465976808, 0.05219959533911058130, 111.2489096053143669 ) ) ;
#128892=CARTESIAN_POINT ( 'NONE',  ( 16.46253265017160672, -9.564922557960803928, 53.33224293864768839 ) ) ;
#128893=CARTESIAN_POINT ( 'NONE',  ( 14.34966873604960469, 8.224510206698951720, 94.16557627198103830 ) ) ;
#128895=CARTESIAN_POINT ( 'NONE',  ( 5.719274019375991003, -21.55341960407610458, 42.70724293864770260 ) ) ;
#128896=CARTESIAN_POINT ( 'NONE',  ( -12.14591786802309592, -12.06949235617757132, 66.87390960531436690 ) ) ;
#128897=CARTESIAN_POINT ( 'NONE',  ( 8.224510206698742110, 14.34966873604972548, 22.08442372801901143 ) ) ;
#128898=CARTESIAN_POINT ( 'NONE',  ( -15.72974639402176322, -15.80617190586768395, 84.37609039468570415 ) ) ;
#128899=CARTESIAN_POINT ( 'NONE',  ( 17.48853670773243607, -5.747243402303152671, 76.16671299749989998 ) ) ;
#128900=CARTESIAN_POINT ( 'NONE',  ( -4.483927247898782831, 16.52544592524335698, 97.70942372801904696 ) ) ;
#128901=CARTESIAN_POINT ( 'NONE',  ( 16.52544592524342804, -4.483927247898539470, 38.54057627198103120 ) ) ;
#128902=CARTESIAN_POINT ( 'NONE',  ( 5.153800228976335163, 19.02544592524342804, 34.79057627198102409 ) ) ;
#128903=CARTESIAN_POINT ( 'NONE',  ( 5.153800228976335163, 19.02544592524342804, 84.79057627198099567 ) ) ;
#128904=CARTESIAN_POINT ( 'NONE',  ( 5.823673210054125526, 21.52544592524343514, 89.79057627198103830 ) ) ;
#128905=CARTESIAN_POINT ( 'NONE',  ( -8.314922557961024197, 14.29746914071037800, 32.91775706135234714 ) ) ;
#128906=CARTESIAN_POINT ( 'NONE',  ( 14.34966873604960469, 8.224510206698951720, 69.16557627198102409 ) ) ;
#128907=CARTESIAN_POINT ( 'NONE',  ( -21.52544592524334988, -5.823673210054445271, 88.95942372801901854 ) ) ;
#128908=CARTESIAN_POINT ( 'NONE',  ( -14.29746914071037622, -8.314922557961029526, 94.16775706135237556 ) ) ;
#128909=CARTESIAN_POINT ( 'NONE',  ( 16.29526858892907271, -7.335722546920040443, 46.70329402199735114 ) ) ;
#128910=CARTESIAN_POINT ( 'NONE',  ( -19.52851543214741881, -5.500000000000036415, 65.39357721762580411 ) ) ;
#128911=CARTESIAN_POINT ( 'NONE',  ( 4.379528057220339221, -16.55341960407611168, 32.70724293864770260 ) ) ;
#128912=CARTESIAN_POINT ( 'NONE',  ( 8.224510206698742110, 14.34966873604972548, 72.08442372801899012 ) ) ;
#128913=CARTESIAN_POINT ( 'NONE',  ( -13.97604488694527625, -13.89961937509977652, 91.87390960531432427 ) ) ;
#128914=CARTESIAN_POINT ( 'NONE',  ( 0.05219959533909260263, 19.03943276465977164, 104.9989096053143669 ) ) ;
#128915=CARTESIAN_POINT ( 'NONE',  ( 5.823673210054444382, -21.52544592524334988, 90.20942372801903275 ) ) ;
#128916=CARTESIAN_POINT ( 'NONE',  ( 14.29746914071037800, 8.314922557961029526, 91.66775706135234714 ) ) ;
#128917=CARTESIAN_POINT ( 'NONE',  ( 0.05219959533910956823, 16.53943276465976808, 64.99890960531435269 ) ) ;
#128918=CARTESIAN_POINT ( 'NONE',  ( 9.474510206698971260, -16.51473224551069308, 62.91557627198102409 ) ) ;
#128920=CARTESIAN_POINT ( 'NONE',  ( -19.05341960407617563, 5.049401038297882671, 103.5427570613523329 ) ) ;
#128921=CARTESIAN_POINT ( 'NONE',  ( 14.29746914071049879, -8.314922557960816363, 108.3322429386477097 ) ) ;
#128922=CARTESIAN_POINT ( 'NONE',  ( -13.97604488694527625, -13.89961937509977652, 71.87390960531433848 ) ) ;
#128923=CARTESIAN_POINT ( 'NONE',  ( 19.02544592524334988, 5.153800228976608722, 111.4594237280190043 ) ) ;
#128925=CARTESIAN_POINT ( 'NONE',  ( 10.72451020669871369, 18.67979575497193778, 112.0844237280190185 ) ) ;
#128926=CARTESIAN_POINT ( 'NONE',  ( -14.34966873604972548, 8.224510206698743886, 78.33442372801901854 ) ) ;
#128927=CARTESIAN_POINT ( 'NONE',  ( -13.89961937509957401, -13.97604488694547875, 104.3760903946856757 ) ) ;
#128928=CARTESIAN_POINT ( 'NONE',  ( -14.29746914071049879, 8.314922557960819915, 110.8322429386476955 ) ) ;
#128929=CARTESIAN_POINT ( 'NONE',  ( 4.483927247898790824, -16.52544592524335698, 65.20942372801901854 ) ) ;
#128930=CARTESIAN_POINT ( 'NONE',  ( -4.483927247898782831, 16.52544592524335698, 47.70942372801902565 ) ) ;
#128931=CARTESIAN_POINT ( 'NONE',  ( 9.474510206698971260, -16.51473224551069308, 27.91557627198103120 ) ) ;
#128932=CARTESIAN_POINT ( 'NONE',  ( -5.153800228976607833, 19.02544592524334988, 67.70942372801900433 ) ) ;
#128933=CARTESIAN_POINT ( 'NONE',  ( 19.03943276465977164, 0.05219959533936151252, 21.25109039468565797 ) ) ;
#128934=CARTESIAN_POINT ( 'NONE',  ( -13.97604488694527625, -13.89961937509977652, 31.87390960531435979 ) ) ;
#128935=CARTESIAN_POINT ( 'NONE',  ( 19.02544592524343514, -5.153800228976328945, 83.54057627198100988 ) ) ;
#128936=CARTESIAN_POINT ( 'NONE',  ( -4.379528057220328563, 16.55341960407611168, 70.20724293864769550 ) ) ;
#128937=EDGE_CURVE ( 'NONE', #188751, #178458, #179244, .T. ) ;
#128938=CARTESIAN_POINT ( 'NONE',  ( 5.049401038297881783, 19.05341960407617563, 37.29275706135232582 ) ) ;
#128939=CARTESIAN_POINT ( 'NONE',  ( 15.72974639402199770, -15.80617190586745480, 43.12390960531435269 ) ) ;
#128940=CARTESIAN_POINT ( 'NONE',  ( 18.62759615963255655, 10.81492255796105972, 111.6677570613523613 ) ) ;
#128941=CARTESIAN_POINT ( 'NONE',  ( -16.46253265017160317, 9.564922557960807481, 95.83224293864769550 ) ) ;
#128942=CARTESIAN_POINT ( 'NONE',  ( -10.81492255796105439, 18.62759615963255655, 102.9177570613523756 ) ) ;
#128943=CARTESIAN_POINT ( 'NONE',  ( -21.55341960407610458, -5.719274019375992779, 66.45724293864768129 ) ) ;
#128944=CARTESIAN_POINT ( 'NONE',  ( -0.05219959533909027116, -19.03943276465977164, 102.4989096053143669 ) ) ;
#128945=CARTESIAN_POINT ( 'NONE',  ( -5.049401038297874678, -19.05341960407617918, 79.79275706135233293 ) ) ;
#128946=CARTESIAN_POINT ( 'NONE',  ( -13.89961937509977652, 13.97604488694528158, 105.6239096053143527 ) ) ;
#128947=CARTESIAN_POINT ( 'NONE',  ( 5.049401038297881783, 19.05341960407617563, 102.2927570613523045 ) ) ;
#128948=CARTESIAN_POINT ( 'NONE',  ( -12.06949235617739369, -12.14591786802326823, 59.37609039468568284 ) ) ;
#128949=CARTESIAN_POINT ( 'NONE',  ( -16.51473224551069308, -9.474510206698971260, 26.66557627198103120 ) ) ;
#128950=CARTESIAN_POINT ( 'NONE',  ( 19.03943276465977164, -0.05219959533909143690, 78.74890960531436690 ) ) ;
#128951=CARTESIAN_POINT ( 'NONE',  ( 5.823673210054125526, 21.52544592524343514, 69.79057627198102409 ) ) ;
#128953=CARTESIAN_POINT ( 'NONE',  ( -16.55341960407617563, 4.379528057220093196, 28.54275706135234358 ) ) ;
#128954=CARTESIAN_POINT ( 'NONE',  ( 21.53943276465977519, 0.05219959533937863772, 36.25109039468567573 ) ) ;
#128955=CARTESIAN_POINT ( 'NONE',  ( -0.05219959533937732626, 21.53943276465977519, 87.50109039468568994 ) ) ;
#128956=CARTESIAN_POINT ( 'NONE',  ( 0.05219959533934541429, -16.53943276465976808, 95.00109039468568994 ) ) ;
#128957=CARTESIAN_POINT ( 'NONE',  ( -16.51473224551069308, -9.474510206698971260, 91.66557627198103830 ) ) ;
#128958=CARTESIAN_POINT ( 'NONE',  ( 12.14591786802309770, 12.06949235617756955, 74.37390960531436690 ) ) ;
#128959=CARTESIAN_POINT ( 'NONE',  ( -8.314922557960811034, -14.29746914071050412, 27.08224293864769550 ) ) ;
#128960=CARTESIAN_POINT ( 'NONE',  ( -19.03943276465977164, -0.05219959533935918106, 58.75109039468566863 ) ) ;
#128961=CARTESIAN_POINT ( 'NONE',  ( -15.72974639402176322, -15.80617190586768395, 49.37609039468569705 ) ) ;
#128962=CARTESIAN_POINT ( 'NONE',  ( 12.06949235617757843, -12.14591786802309237, 93.12390960531436690 ) ) ;
#128963=CARTESIAN_POINT ( 'NONE',  ( -19.02544592524342804, 5.153800228976336051, 111.0405762719810099 ) ) ;
#128964=CARTESIAN_POINT ( 'NONE',  ( -14.29746914071037622, -8.314922557961029526, 104.1677570613523471 ) ) ;
#128965=CARTESIAN_POINT ( 'NONE',  ( -5.823673210054431948, 21.52544592524334988, 87.70942372801901854 ) ) ;
#128966=CARTESIAN_POINT ( 'NONE',  ( 4.483927247898790824, -16.52544592524335698, 45.20942372801901854 ) ) ;
#128967=CARTESIAN_POINT ( 'NONE',  ( 15.80617190586769283, -15.72974639402175789, 45.62609039468567573 ) ) ;
#128969=CARTESIAN_POINT ( 'NONE',  ( 18.67979575497178502, 10.72451020669898547, 114.1655762719810383 ) ) ;
#128970=CARTESIAN_POINT ( 'NONE',  ( -4.483927247898539470, -16.52544592524342804, 87.29057627198103830 ) ) ;
#128971=EDGE_CURVE ( 'NONE', #56210, #199942, #41717, .T. ) ;
#128972=CARTESIAN_POINT ( 'NONE',  ( -19.39056639909671986, -5.500000000000051514, 50.78948781074345931 ) ) ;
#128973=CARTESIAN_POINT ( 'NONE',  ( -12.14591786802309592, -12.06949235617757132, 61.87390960531436690 ) ) ;
#128974=CARTESIAN_POINT ( 'NONE',  ( -8.314922557961024197, 14.29746914071037800, 112.9177570613523329 ) ) ;
#128975=CARTESIAN_POINT ( 'NONE',  ( -16.51473224551069308, -9.474510206698971260, 41.66557627198103120 ) ) ;
#128976=CARTESIAN_POINT ( 'NONE',  ( -18.67979575497178146, -10.72451020669898902, 36.66557627198103120 ) ) ;
#128977=CARTESIAN_POINT ( 'NONE',  ( -8.314922557960811034, -14.29746914071050412, 72.08224293864769550 ) ) ;
#128979=CARTESIAN_POINT ( 'NONE',  ( -15.72974639402197994, 15.80617190586746368, 80.62390960531438111 ) ) ;
#128980=CARTESIAN_POINT ( 'NONE',  ( 5.049401038298161559, -19.05341960407611168, 82.70724293864770971 ) ) ;
#128981=CARTESIAN_POINT ( 'NONE',  ( 5.153800228976335163, 19.02544592524342804, 39.79057627198100988 ) ) ;
#128982=CARTESIAN_POINT ( 'NONE',  ( -13.97604488694547697, 13.89961937509957934, 93.12609039468566152 ) ) ;
#128983=EDGE_CURVE ( 'NONE', #88260, #84227, #82477, .T. ) ;
#128984=CARTESIAN_POINT ( 'NONE',  ( -18.67979575497178146, -10.72451020669898902, 31.66557627198102054 ) ) ;
#128985=CARTESIAN_POINT ( 'NONE',  ( -21.53943276465977519, -0.05219959533937600094, 68.75109039468568994 ) ) ;
#128986=CARTESIAN_POINT ( 'NONE',  ( -9.564922557960796823, -16.46253265017161027, 47.08224293864769550 ) ) ;
#128987=CARTESIAN_POINT ( 'NONE',  ( 9.564922557960805705, 16.46253265017160317, 89.58224293864769550 ) ) ;
#128989=CARTESIAN_POINT ( 'NONE',  ( -14.29746914071037622, -8.314922557961029526, 64.16775706135234714 ) ) ;
#128990=CARTESIAN_POINT ( 'NONE',  ( 18.67979575497194134, -10.72451020669871369, 50.83442372801901143 ) ) ;
#128991=CARTESIAN_POINT ( 'NONE',  ( 15.80617190586769283, -15.72974639402175789, 75.62609039468567573 ) ) ;
#128992=CARTESIAN_POINT ( 'NONE',  ( -21.52544592524343514, 5.823673210054127303, 26.04057627198103475 ) ) ;
#128993=CARTESIAN_POINT ( 'NONE',  ( -18.67979575497178146, -10.72451020669898902, 86.66557627198102409 ) ) ;
#128994=CARTESIAN_POINT ( 'NONE',  ( 10.72451020669871369, 18.67979575497193778, 27.08442372801901854 ) ) ;
#128995=CARTESIAN_POINT ( 'NONE',  ( -12.14591786802326823, 12.06949235617739902, 68.12609039468567573 ) ) ;
#128996=CARTESIAN_POINT ( 'NONE',  ( -18.62759615963270932, 10.81492255796079327, 65.83224293864769550 ) ) ;
#128997=CARTESIAN_POINT ( 'NONE',  ( -16.51473224551082808, 9.474510206698731452, 23.33442372801900078 ) ) ;
#128998=CARTESIAN_POINT ( 'NONE',  ( 19.02544592524343514, -5.153800228976328945, 63.54057627198103830 ) ) ;
#128999=CARTESIAN_POINT ( 'NONE',  ( -16.53943276465976808, -0.05219959533934237506, 108.7510903946857042 ) ) ;
#129000=CARTESIAN_POINT ( 'NONE',  ( -17.50000000000000000, -3.565345528328005997, 105.5750551319353576 ) ) ;
#129001=CARTESIAN_POINT ( 'NONE',  ( -9.564922557960796823, -16.46253265017161027, 92.08224293864769550 ) ) ;
#129002=CARTESIAN_POINT ( 'NONE',  ( 17.49999999999999645, 3.232540337672813902, 102.7809047999542003 ) ) ;
#129003=CARTESIAN_POINT ( 'NONE',  ( 16.51473224551083163, -9.474510206698727899, 75.83442372801900433 ) ) ;
#129004=CARTESIAN_POINT ( 'NONE',  ( 5.719274019375991003, -21.55341960407610458, 57.70724293864770260 ) ) ;
#129005=CARTESIAN_POINT ( 'NONE',  ( -12.14591786802309592, -12.06949235617757132, 21.87390960531436690 ) ) ;
#129006=CARTESIAN_POINT ( 'NONE',  ( 5.049401038297881783, 19.05341960407617563, 102.2927570613523045 ) ) ;
#129007=CARTESIAN_POINT ( 'NONE',  ( 19.05341960407617918, -5.049401038297876454, 91.04275706135234714 ) ) ;
#129008=CARTESIAN_POINT ( 'NONE',  ( -0.05219959533907301413, -21.53943276465977519, 92.49890960531436690 ) ) ;
#129009=CARTESIAN_POINT ( 'NONE',  ( 13.97604488694548053, -13.89961937509957401, 60.62609039468564731 ) ) ;
#129010=CARTESIAN_POINT ( 'NONE',  ( 17.50000000000000711, 5.624438216177583882, 106.6832965508535551 ) ) ;
#129011=CARTESIAN_POINT ( 'NONE',  ( 13.97604488694527802, 13.89961937509977652, 49.37390960531434558 ) ) ;
#129012=CARTESIAN_POINT ( 'NONE',  ( -16.52544592524342804, 4.483927247898546575, 61.04057627198103120 ) ) ;
#129013=CARTESIAN_POINT ( 'NONE',  ( 19.05341960407611168, 5.049401038298154454, 53.95724293864770260 ) ) ;
#129014=CARTESIAN_POINT ( 'NONE',  ( 16.52544592524342804, -4.483927247898539470, 58.54057627198103120 ) ) ;
#129017=CARTESIAN_POINT ( 'NONE',  ( -16.52544592524342804, 4.483927247898546575, 31.04057627198102409 ) ) ;
#129018=CARTESIAN_POINT ( 'NONE',  ( 9.474510206698971260, -16.51473224551069308, 57.91557627198103120 ) ) ;
#129019=CARTESIAN_POINT ( 'NONE',  ( -16.46253265017146816, -9.564922557961047289, 39.16775706135234003 ) ) ;
#129020=CARTESIAN_POINT ( 'NONE',  ( 16.53943276465976808, 0.05219959533934440121, 51.25109039468568994 ) ) ;
#129021=CARTESIAN_POINT ( 'NONE',  ( -18.67979575497178146, -10.72451020669898902, 46.66557627198102409 ) ) ;
#129022=CARTESIAN_POINT ( 'NONE',  ( -18.67979575497193778, 10.72451020669871902, 108.3344237280190185 ) ) ;
#129023=CARTESIAN_POINT ( 'NONE',  ( 13.89961937509977652, -13.97604488694527269, 73.12390960531436690 ) ) ;
#129024=CARTESIAN_POINT ( 'NONE',  ( 9.564922557960805705, 16.46253265017160317, 114.5822429386476955 ) ) ;
#129025=CARTESIAN_POINT ( 'NONE',  ( 0.05219959533909260263, 19.03943276465977164, 114.9989096053143669 ) ) ;
#129026=CARTESIAN_POINT ( 'NONE',  ( -17.97058386085787163, -5.500000000000054179, 44.00390968646217260 ) ) ;
#129027=CARTESIAN_POINT ( 'NONE',  ( -10.72451020669870658, -18.67979575497194134, 34.58442372801900433 ) ) ;
#129028=CARTESIAN_POINT ( 'NONE',  ( -8.314922557960811034, -14.29746914071050412, 87.08224293864769550 ) ) ;
#129029=CARTESIAN_POINT ( 'NONE',  ( 5.823673210054125526, 21.52544592524343514, 89.79057627198103830 ) ) ;
#129030=CARTESIAN_POINT ( 'NONE',  ( -9.474510206698964154, 16.51473224551069663, 80.41557627198103830 ) ) ;
#129031=CARTESIAN_POINT ( 'NONE',  ( -5.049401038298153566, 19.05341960407611168, 80.20724293864769550 ) ) ;
#129032=CARTESIAN_POINT ( 'NONE',  ( 18.62759615963255655, 10.81492255796105972, 31.66775706135234358 ) ) ;
#129034=CARTESIAN_POINT ( 'NONE',  ( -16.51473224551069308, -9.474510206698971260, 76.66557627198103830 ) ) ;
#129035=CARTESIAN_POINT ( 'NONE',  ( 18.56453257813367230, -5.499999999999956479, 98.49000423690687001 ) ) ;
#129036=CARTESIAN_POINT ( 'NONE',  ( 5.153800228976335163, 19.02544592524342804, 29.79057627198102409 ) ) ;
#129037=CARTESIAN_POINT ( 'NONE',  ( -5.049401038298153566, 19.05341960407611168, 30.20724293864768839 ) ) ;
#129038=CARTESIAN_POINT ( 'NONE',  ( -16.46253265017146816, -9.564922557961047289, 104.1677570613523329 ) ) ;
#129039=CARTESIAN_POINT ( 'NONE',  ( 0.05219959533910956823, 16.53943276465976808, 109.9989096053143527 ) ) ;
#129040=CARTESIAN_POINT ( 'NONE',  ( 18.67979575497194134, -10.72451020669871369, 75.83442372801900433 ) ) ;
#129041=CARTESIAN_POINT ( 'NONE',  ( -13.97604488694527625, -13.89961937509977652, 56.87390960531434558 ) ) ;
#129042=CARTESIAN_POINT ( 'NONE',  ( -5.823673210054431948, 21.52544592524334988, 37.70942372801900433 ) ) ;
#129043=CARTESIAN_POINT ( 'NONE',  ( -5.719274019375978568, 21.55341960407610458, 110.2072429386477239 ) ) ;
#129045=CARTESIAN_POINT ( 'NONE',  ( 9.564922557960805705, 16.46253265017160317, 79.58224293864769550 ) ) ;
#129047=CARTESIAN_POINT ( 'NONE',  ( -12.14591786802326823, 12.06949235617739902, 28.12609039468568284 ) ) ;
#129048=CARTESIAN_POINT ( 'NONE',  ( 5.719274019375991003, -21.55341960407610458, 37.70724293864769550 ) ) ;
#129049=CARTESIAN_POINT ( 'NONE',  ( 5.719274019375673035, 21.55341960407619339, 62.29275706135236845 ) ) ;
#129050=CARTESIAN_POINT ( 'NONE',  ( -5.049401038298153566, 19.05341960407611168, 115.2072429386477097 ) ) ;
#129051=CARTESIAN_POINT ( 'NONE',  ( 9.564922557961047289, -16.46253265017146816, 95.41775706135233293 ) ) ;
#129052=CARTESIAN_POINT ( 'NONE',  ( 9.474510206698971260, -16.51473224551069308, 47.91557627198102409 ) ) ;
#129053=CARTESIAN_POINT ( 'NONE',  ( -16.51473224551069308, -9.474510206698971260, 81.66557627198103830 ) ) ;
#129054=CARTESIAN_POINT ( 'NONE',  ( -4.483927247898539470, -16.52544592524342804, 97.29057627198105251 ) ) ;
#129055=CARTESIAN_POINT ( 'NONE',  ( 4.483927247898545687, 16.52544592524342804, 89.79057627198103830 ) ) ;
#129056=CARTESIAN_POINT ( 'NONE',  ( 9.474510206698971260, -16.51473224551069308, 107.9155762719810383 ) ) ;
#129057=CARTESIAN_POINT ( 'NONE',  ( -4.483927247898539470, -16.52544592524342804, 57.29057627198103120 ) ) ;
#129058=CARTESIAN_POINT ( 'NONE',  ( -13.97604488694527625, -13.89961937509977652, 36.87390960531436690 ) ) ;
#129059=CARTESIAN_POINT ( 'NONE',  ( 15.72974639402176855, 15.80617190586768217, 61.87609039468568284 ) ) ;
#129060=CARTESIAN_POINT ( 'NONE',  ( -5.153800228976607833, 19.02544592524334988, 97.70942372801900433 ) ) ;
#129061=CARTESIAN_POINT ( 'NONE',  ( -16.55341960407611168, -4.379528057220339221, 61.45724293864770260 ) ) ;
#129062=CARTESIAN_POINT ( 'NONE',  ( 10.81492255796078972, 18.62759615963270932, 109.5822429386476955 ) ) ;
#129063=CARTESIAN_POINT ( 'NONE',  ( 5.719274019375991003, -21.55341960407610458, 52.70724293864769550 ) ) ;
#129064=CARTESIAN_POINT ( 'NONE',  ( 19.49671883438228193, 5.499999999999968914, 72.39279849105680853 ) ) ;
#129066=CARTESIAN_POINT ( 'NONE',  ( 13.97604488694527802, 13.89961937509977652, 54.37390960531435979 ) ) ;
#129067=CARTESIAN_POINT ( 'NONE',  ( -14.29746914071049879, 8.314922557960819915, 40.83224293864769550 ) ) ;
#129068=CARTESIAN_POINT ( 'NONE',  ( 16.52544592524335698, 4.483927247898782831, 96.45942372801901854 ) ) ;
#129069=CARTESIAN_POINT ( 'NONE',  ( 8.224510206698742110, 14.34966873604972548, 87.08442372801901854 ) ) ;
#129070=CARTESIAN_POINT ( 'NONE',  ( 16.46253265017146816, 9.564922557961045513, 41.66775706135234003 ) ) ;
#129072=CARTESIAN_POINT ( 'NONE',  ( 19.02544592524343514, -5.153800228976328945, 88.54057627198102409 ) ) ;
#129073=CARTESIAN_POINT ( 'NONE',  ( 0.05219959533909260263, 19.03943276465977164, 44.99890960531435979 ) ) ;
#129074=CARTESIAN_POINT ( 'NONE',  ( -16.53943276465976808, 0.05219959533911058130, 66.24890960531436690 ) ) ;
#129075=CARTESIAN_POINT ( 'NONE',  ( 17.50000000001358558, -5.500000000000039968, 48.29690382535059001 ) ) ;
#129076=CARTESIAN_POINT ( 'NONE',  ( -21.55341960407610458, -5.719274019375992779, 21.45724293864769550 ) ) ;
#129077=CARTESIAN_POINT ( 'NONE',  ( 21.55341960407610458, 5.719274019375980345, 43.95724293864769550 ) ) ;
#129078=CARTESIAN_POINT ( 'NONE',  ( -16.55341960407611168, -4.379528057220339221, 86.45724293864770971 ) ) ;
#129080=CARTESIAN_POINT ( 'NONE',  ( 8.224510206698742110, 14.34966873604972548, 32.08442372801901854 ) ) ;
#129081=CARTESIAN_POINT ( 'NONE',  ( 8.314922557960818139, 14.29746914071049879, 79.58224293864769550 ) ) ;
#129084=CARTESIAN_POINT ( 'NONE',  ( -0.05219959533936034679, 19.03943276465977164, 72.50109039468566152 ) ) ;
#129085=CARTESIAN_POINT ( 'NONE',  ( 9.474510206698971260, -16.51473224551069308, 97.91557627198102409 ) ) ;
#129088=CARTESIAN_POINT ( 'NONE',  ( -14.29746914071037622, -8.314922557961029526, 34.16775706135234714 ) ) ;
#129089=CARTESIAN_POINT ( 'NONE',  ( -0.05219959533910754901, -16.53943276465976808, 22.49890960531436335 ) ) ;
#129090=CARTESIAN_POINT ( 'NONE',  ( 9.474510206698729675, 16.51473224551082808, 67.08442372801900433 ) ) ;
#129091=CARTESIAN_POINT ( 'NONE',  ( -21.53943276465977519, 0.05219959533907696930, 36.24890960531435979 ) ) ;
#129092=CARTESIAN_POINT ( 'NONE',  ( 21.52544592524334988, 5.823673210054432836, 66.45942372801903275 ) ) ;
#129094=CARTESIAN_POINT ( 'NONE',  ( -12.14591786802326823, 12.06949235617739902, 38.12609039468567573 ) ) ;
#129095=CARTESIAN_POINT ( 'NONE',  ( -5.049401038298153566, 19.05341960407611168, 25.20724293864768484 ) ) ;
#129096=CARTESIAN_POINT ( 'NONE',  ( 16.51473224551069308, 9.474510206698969483, 94.16557627198103830 ) ) ;
#129097=CARTESIAN_POINT ( 'NONE',  ( -5.153800228976328057, -19.02544592524343514, 22.29057627198102765 ) ) ;
#129098=CARTESIAN_POINT ( 'NONE',  ( 14.29746914071049879, -8.314922557960816363, 93.33224293864769550 ) ) ;
#129099=EDGE_CURVE ( 'NONE', #174275, #44164, #101848, .T. ) ;
#129101=CARTESIAN_POINT ( 'NONE',  ( 19.05341960407611168, 5.049401038298154454, 83.95724293864766707 ) ) ;
#129103=CARTESIAN_POINT ( 'NONE',  ( -16.51473224551082808, 9.474510206698731452, 108.3344237280190043 ) ) ;
#129104=CARTESIAN_POINT ( 'NONE',  ( -10.72451020669898014, 18.67979575497178502, 75.41557627198102409 ) ) ;
#129105=CARTESIAN_POINT ( 'NONE',  ( 19.02544592524343514, -5.153800228976328945, 48.54057627198103120 ) ) ;
#129106=CARTESIAN_POINT ( 'NONE',  ( -19.02544592524334988, -5.153800228976617603, 63.95942372801899012 ) ) ;
#129107=CARTESIAN_POINT ( 'NONE',  ( 21.53943276465977519, -0.05219959533907433946, 113.7489096053143527 ) ) ;
#129108=CARTESIAN_POINT ( 'NONE',  ( 0.05219959533909260263, 19.03943276465977164, 69.99890960531435269 ) ) ;
#129109=CARTESIAN_POINT ( 'NONE',  ( 16.51473224551069308, 9.474510206698969483, 109.1655762719810383 ) ) ;
#129111=CARTESIAN_POINT ( 'NONE',  ( 4.483927247898790824, -16.52544592524335698, 30.20942372801902565 ) ) ;
#129112=CARTESIAN_POINT ( 'NONE',  ( 10.72451020669898902, -18.67979575497178502, 102.9155762719810383 ) ) ;
#129113=CARTESIAN_POINT ( 'NONE',  ( -8.314922557960811034, -14.29746914071050412, 102.0822429386476955 ) ) ;
#129114=CARTESIAN_POINT ( 'NONE',  ( 5.049401038298161559, -19.05341960407611168, 97.70724293864766707 ) ) ;
#129115=CARTESIAN_POINT ( 'NONE',  ( 13.97604488694548053, -13.89961937509957401, 65.62609039468567573 ) ) ;
#129116=CARTESIAN_POINT ( 'NONE',  ( 18.62759615963271287, -10.81492255796078972, 83.33224293864769550 ) ) ;
#129117=CARTESIAN_POINT ( 'NONE',  ( -14.29746914071049879, 8.314922557960819915, 50.83224293864770971 ) ) ;
#129118=CARTESIAN_POINT ( 'NONE',  ( 0.05219959533936267826, -19.03943276465977164, 20.00109039468567218 ) ) ;
#129119=CARTESIAN_POINT ( 'NONE',  ( 14.29746914071037800, 8.314922557961029526, 66.66775706135234714 ) ) ;
#129120=CARTESIAN_POINT ( 'NONE',  ( -5.153800228976328057, -19.02544592524343514, 92.29057627198099567 ) ) ;
#129121=CARTESIAN_POINT ( 'NONE',  ( 5.153800228976335163, 19.02544592524342804, 44.79057627198103830 ) ) ;
#129122=VECTOR ( 'NONE', #87414, 1000.000000000000000 ) ;
#129123=CARTESIAN_POINT ( 'NONE',  ( -18.67979575497193778, 10.72451020669871902, 58.33442372801901143 ) ) ;
#129124=CARTESIAN_POINT ( 'NONE',  ( 15.72974639402176855, 15.80617190586768217, 71.87609039468568994 ) ) ;
#129125=CARTESIAN_POINT ( 'NONE',  ( 0.05219959533909260263, 19.03943276465977164, 59.99890960531436690 ) ) ;
#129126=CARTESIAN_POINT ( 'NONE',  ( 10.81492255796106328, -18.62759615963255655, 30.41775706135234358 ) ) ;
#129127=CARTESIAN_POINT ( 'NONE',  ( -13.97604488694547697, 13.89961937509957934, 68.12609039468563310 ) ) ;
#129128=CARTESIAN_POINT ( 'NONE',  ( 0.05219959533936267826, -19.03943276465977164, 70.00109039468566152 ) ) ;
#129129=CARTESIAN_POINT ( 'NONE',  ( 19.02544592524343514, -5.153800228976328945, 33.54057627198102409 ) ) ;
#129130=CARTESIAN_POINT ( 'NONE',  ( 4.379528057220092307, 16.55341960407617563, 87.29275706135236135 ) ) ;
#129131=CARTESIAN_POINT ( 'NONE',  ( 19.05341960407611168, 5.049401038298154454, 48.95724293864768129 ) ) ;
#129132=CARTESIAN_POINT ( 'NONE',  ( 9.564922557960805705, 16.46253265017160317, 24.58224293864769194 ) ) ;
#129133=CARTESIAN_POINT ( 'NONE',  ( 19.02544592524343514, -5.153800228976328945, 103.5405762719809957 ) ) ;
#129134=CARTESIAN_POINT ( 'NONE',  ( 13.97604488694527802, 13.89961937509977652, 34.37390960531436690 ) ) ;
#129136=CARTESIAN_POINT ( 'NONE',  ( 0.05219959533907565091, 21.53943276465977519, 84.99890960531436690 ) ) ;
#129137=CARTESIAN_POINT ( 'NONE',  ( 14.29746914071037800, 8.314922557961029526, 56.66775706135235424 ) ) ;
#129138=CARTESIAN_POINT ( 'NONE',  ( 16.46253265017146816, 9.564922557961045513, 31.66775706135232937 ) ) ;
#129139=CARTESIAN_POINT ( 'NONE',  ( 13.89961937509977652, -13.97604488694527269, 58.12390960531436690 ) ) ;
#129140=CARTESIAN_POINT ( 'NONE',  ( -16.53943276465976808, 0.05219959533911058130, 41.24890960531435269 ) ) ;
#129141=CARTESIAN_POINT ( 'NONE',  ( -0.05219959533910754901, -16.53943276465976808, 87.49890960531436690 ) ) ;
#129142=CARTESIAN_POINT ( 'NONE',  ( 13.97604488694527802, 13.89961937509977652, 84.37390960531433848 ) ) ;
#129143=CARTESIAN_POINT ( 'NONE',  ( 0.05219959533909260263, 19.03943276465977164, 84.99890960531436690 ) ) ;
#129144=CARTESIAN_POINT ( 'NONE',  ( 5.719274019375673035, 21.55341960407619339, 42.29275706135235424 ) ) ;
#129145=CARTESIAN_POINT ( 'NONE',  ( 13.97604488694527802, 13.89961937509977652, 94.37390960531436690 ) ) ;
#129146=CARTESIAN_POINT ( 'NONE',  ( -10.81492255796105439, 18.62759615963255655, 92.91775706135236135 ) ) ;
#129147=CARTESIAN_POINT ( 'NONE',  ( -12.14591786802326823, 12.06949235617739902, 78.12609039468570415 ) ) ;
#129148=CARTESIAN_POINT ( 'NONE',  ( 5.823673210054444382, -21.52544592524334988, 25.20942372801901854 ) ) ;
#129149=CARTESIAN_POINT ( 'NONE',  ( -0.05219959533907301413, -21.53943276465977519, 87.49890960531436690 ) ) ;
#129150=CARTESIAN_POINT ( 'NONE',  ( 8.314922557960818139, 14.29746914071049879, 44.58224293864769550 ) ) ;
#129151=CARTESIAN_POINT ( 'NONE',  ( -13.89961937509977652, 13.97604488694528158, 40.62390960531435979 ) ) ;
#129152=CARTESIAN_POINT ( 'NONE',  ( 14.29746914071049879, -8.314922557960816363, 68.33224293864769550 ) ) ;
#129153=CARTESIAN_POINT ( 'NONE',  ( -21.53943276465977519, 0.05219959533907696930, 36.24890960531435979 ) ) ;
#129154=CARTESIAN_POINT ( 'NONE',  ( -13.97604488694547697, 13.89961937509957934, 28.12609039468565797 ) ) ;
#129155=CARTESIAN_POINT ( 'NONE',  ( -4.379528057220328563, 16.55341960407611168, 100.2072429386476955 ) ) ;
#129156=CARTESIAN_POINT ( 'NONE',  ( 13.97604488694527802, 13.89961937509977652, 114.3739096053143669 ) ) ;
#129158=CARTESIAN_POINT ( 'NONE',  ( 8.224510206698742110, 14.34966873604972548, 52.08442372801901854 ) ) ;
#129159=CARTESIAN_POINT ( 'NONE',  ( -5.153800228976328057, -19.02544592524343514, 62.29057627198100988 ) ) ;
#129160=CARTESIAN_POINT ( 'NONE',  ( -16.60570611055986490, -6.631713784153137503, 20.77476115285328717 ) ) ;
#129161=CARTESIAN_POINT ( 'NONE',  ( -15.72974639402197994, 15.80617190586746368, 25.62390960531435624 ) ) ;
#129162=CARTESIAN_POINT ( 'NONE',  ( -14.29746914071037622, -8.314922557961029526, 89.16775706135236135 ) ) ;
#129163=CARTESIAN_POINT ( 'NONE',  ( 9.474510206698729675, 16.51473224551082808, 107.0844237280190043 ) ) ;
#129164=CARTESIAN_POINT ( 'NONE',  ( 21.52544592524334988, 5.823673210054432836, 86.45942372801901854 ) ) ;
#129165=CARTESIAN_POINT ( 'NONE',  ( 16.51473224551069308, 9.474510206698969483, 79.16557627198103830 ) ) ;
#129166=CARTESIAN_POINT ( 'NONE',  ( 10.72451020669898902, -18.67979575497178502, 97.91557627198103830 ) ) ;
#129167=CARTESIAN_POINT ( 'NONE',  ( 8.314922557961029526, -14.29746914071037800, 55.41775706135234714 ) ) ;
#129168=CARTESIAN_POINT ( 'NONE',  ( -14.34966873604960291, -8.224510206698953496, 111.6655762719810525 ) ) ;
#129169=CARTESIAN_POINT ( 'NONE',  ( 16.53943276465976808, 0.05219959533934440121, 21.25109039468567218 ) ) ;
#129170=CARTESIAN_POINT ( 'NONE',  ( 19.02544592524334988, 5.153800228976608722, 86.45942372801900433 ) ) ;
#129171=CARTESIAN_POINT ( 'NONE',  ( 21.55341960407610458, 5.719274019375980345, 73.95724293864769550 ) ) ;
#129172=CARTESIAN_POINT ( 'NONE',  ( -13.97604488694547697, 13.89961937509957934, 58.12609039468566863 ) ) ;
#129174=CARTESIAN_POINT ( 'NONE',  ( -10.81492255796078084, -18.62759615963271287, 107.0822429386476955 ) ) ;
#129176=CARTESIAN_POINT ( 'NONE',  ( -0.05219959533909027116, -19.03943276465977164, 82.49890960531436690 ) ) ;
#129178=CARTESIAN_POINT ( 'NONE',  ( -16.52544592524335698, -4.483927247898792601, 23.95942372801901143 ) ) ;
#129180=CARTESIAN_POINT ( 'NONE',  ( -15.72974639402197994, 15.80617190586746368, 105.6239096053143669 ) ) ;
#129181=CARTESIAN_POINT ( 'NONE',  ( -16.55341960407611168, -4.379528057220339221, 61.45724293864770260 ) ) ;
#129182=CARTESIAN_POINT ( 'NONE',  ( -16.46253265017160317, 9.564922557960807481, 75.83224293864769550 ) ) ;
#129183=CARTESIAN_POINT ( 'NONE',  ( 5.823673210054444382, -21.52544592524334988, 80.20942372801901854 ) ) ;
#129184=CARTESIAN_POINT ( 'NONE',  ( -16.53943276465976808, -0.05219959533934237506, 23.75109039468567929 ) ) ;
#129185=CARTESIAN_POINT ( 'NONE',  ( 19.05341960407617918, -5.049401038297876454, 41.04275706135233293 ) ) ;
#129186=CARTESIAN_POINT ( 'NONE',  ( -21.55341960407619339, 5.719274019375674811, 58.54275706135235424 ) ) ;
#129187=CARTESIAN_POINT ( 'NONE',  ( -15.72974639402176322, -15.80617190586768395, 19.37609039468568639 ) ) ;
#129188=CARTESIAN_POINT ( 'NONE',  ( 21.55341960407610458, 5.719274019375980345, 58.95724293864770971 ) ) ;
#129189=CARTESIAN_POINT ( 'NONE',  ( -16.51473224551082808, 9.474510206698731452, 113.3344237280190043 ) ) ;
#129190=CARTESIAN_POINT ( 'NONE',  ( -9.474510206698964154, 16.51473224551069663, 60.41557627198102409 ) ) ;
#129191=CARTESIAN_POINT ( 'NONE',  ( 5.153800228976615827, -19.02544592524334988, 70.20942372801899012 ) ) ;
#129192=CARTESIAN_POINT ( 'NONE',  ( 21.53943276465977519, 0.05219959533937863772, 86.25109039468568994 ) ) ;
#129193=CARTESIAN_POINT ( 'NONE',  ( -5.049401038297874678, -19.05341960407617918, 54.79275706135234003 ) ) ;
#129194=CARTESIAN_POINT ( 'NONE',  ( 13.97604488694527802, 13.89961937509977652, 39.37390960531435269 ) ) ;
#129195=CARTESIAN_POINT ( 'NONE',  ( -18.67979575497178146, -10.72451020669898902, 51.66557627198102409 ) ) ;
#129196=CARTESIAN_POINT ( 'NONE',  ( 12.06949235617757843, -12.14591786802309237, 53.12390960531436690 ) ) ;
#129198=CARTESIAN_POINT ( 'NONE',  ( 0.05219959533936267826, -19.03943276465977164, 30.00109039468566863 ) ) ;
#129199=CARTESIAN_POINT ( 'NONE',  ( -12.14591786802326823, 12.06949235617739902, 83.12609039468568994 ) ) ;
#129200=CARTESIAN_POINT ( 'NONE',  ( -4.379528057220328563, 16.55341960407611168, 50.20724293864769550 ) ) ;
#129201=CARTESIAN_POINT ( 'NONE',  ( 21.53943276465977519, 0.05219959533937863772, 91.25109039468568994 ) ) ;
#129202=CARTESIAN_POINT ( 'NONE',  ( 5.719274019375673035, 21.55341960407619339, 82.29275706135234714 ) ) ;
#129203=CARTESIAN_POINT ( 'NONE',  ( 15.72974639402199770, -15.80617190586745480, 83.12390960531436690 ) ) ;
#129204=CARTESIAN_POINT ( 'NONE',  ( -9.474510206698964154, 16.51473224551069663, 50.41557627198102409 ) ) ;
#129205=CARTESIAN_POINT ( 'NONE',  ( 5.823673210054444382, -21.52544592524334988, 55.20942372801902565 ) ) ;
#129206=CARTESIAN_POINT ( 'NONE',  ( -5.153800228976328057, -19.02544592524343514, 42.29057627198101699 ) ) ;
#129207=CARTESIAN_POINT ( 'NONE',  ( -13.97604488694527625, -13.89961937509977652, 56.87390960531434558 ) ) ;
#129208=CARTESIAN_POINT ( 'NONE',  ( 14.34966873604960469, 8.224510206698951720, 109.1655762719810383 ) ) ;
#129209=CARTESIAN_POINT ( 'NONE',  ( -5.153800228976328057, -19.02544592524343514, 92.29057627198099567 ) ) ;
#129210=CARTESIAN_POINT ( 'NONE',  ( -14.29746914071049879, 8.314922557960819915, 55.83224293864770260 ) ) ;
#129211=CARTESIAN_POINT ( 'NONE',  ( 19.02544592524343514, -5.153800228976328945, 23.54057627198102054 ) ) ;
#129212=CARTESIAN_POINT ( 'NONE',  ( 15.72974639402199770, -15.80617190586745480, 78.12390960531436690 ) ) ;
#129213=CARTESIAN_POINT ( 'NONE',  ( -18.62759615963255300, -10.81492255796106328, 24.16775706135235424 ) ) ;
#129215=CARTESIAN_POINT ( 'NONE',  ( 4.483927247898790824, -16.52544592524335698, 40.20942372801901854 ) ) ;
#129218=CARTESIAN_POINT ( 'NONE',  ( 5.823673210054125526, 21.52544592524343514, 74.79057627198105251 ) ) ;
#129219=CARTESIAN_POINT ( 'NONE',  ( 21.52544592524334988, 5.823673210054432836, 106.4594237280190328 ) ) ;
#129220=CARTESIAN_POINT ( 'NONE',  ( 16.46253265017160672, -9.564922557960803928, 98.33224293864769550 ) ) ;
#129221=CARTESIAN_POINT ( 'NONE',  ( -5.719274019375665041, -21.55341960407619695, 34.79275706135235424 ) ) ;
#129222=CARTESIAN_POINT ( 'NONE',  ( -21.52544592524343514, 5.823673210054127303, 36.04057627198102409 ) ) ;
#129223=CARTESIAN_POINT ( 'NONE',  ( 4.483927247898790824, -16.52544592524335698, 105.2094237280190328 ) ) ;
#129224=CARTESIAN_POINT ( 'NONE',  ( 15.80617190586769283, -15.72974639402175789, 45.62609039468567573 ) ) ;
#129225=CARTESIAN_POINT ( 'NONE',  ( 15.72974639402176855, 15.80617190586768217, 81.87609039468568994 ) ) ;
#129226=CARTESIAN_POINT ( 'NONE',  ( 5.719274019375673035, 21.55341960407619339, 107.2927570613523471 ) ) ;
#129227=CARTESIAN_POINT ( 'NONE',  ( 0.05219959533934541429, -16.53943276465976808, 80.00109039468568994 ) ) ;
#129228=CARTESIAN_POINT ( 'NONE',  ( -0.05219959533937732626, 21.53943276465977519, 37.50109039468568284 ) ) ;
#129229=CARTESIAN_POINT ( 'NONE',  ( 5.049401038298161559, -19.05341960407611168, 27.70724293864769550 ) ) ;
#129230=CARTESIAN_POINT ( 'NONE',  ( -5.823673210054431948, 21.52544592524334988, 102.7094237280190185 ) ) ;
#129231=CARTESIAN_POINT ( 'NONE',  ( -0.05219959533909027116, -19.03943276465977164, 107.4989096053143527 ) ) ;
#129232=CARTESIAN_POINT ( 'NONE',  ( -21.55341960407610458, -5.719274019375992779, 106.4572429386477097 ) ) ;
#129234=CARTESIAN_POINT ( 'NONE',  ( 19.52851543214742946, 5.500000000000031974, 82.89357721762580411 ) ) ;
#129235=CARTESIAN_POINT ( 'NONE',  ( 18.67979575497178502, 10.72451020669898547, 69.16557627198102409 ) ) ;
#129236=CARTESIAN_POINT ( 'NONE',  ( 0.05219959533934541429, -16.53943276465976808, 55.00109039468568284 ) ) ;
#129237=CARTESIAN_POINT ( 'NONE',  ( -16.53943276465976808, 0.05219959533911058130, 56.24890960531436690 ) ) ;
#129239=CARTESIAN_POINT ( 'NONE',  ( -16.51473224551082808, 9.474510206698731452, 78.33442372801900433 ) ) ;
#129241=CARTESIAN_POINT ( 'NONE',  ( -8.224510206698735004, -14.34966873604973081, 29.58442372801901854 ) ) ;
#129242=CARTESIAN_POINT ( 'NONE',  ( 21.53943276465977519, -0.05219959533907433946, 103.7489096053143669 ) ) ;
#129243=CARTESIAN_POINT ( 'NONE',  ( 12.06949235617757843, -12.14591786802309237, 63.12390960531435979 ) ) ;
#129244=CARTESIAN_POINT ( 'NONE',  ( -18.67979575497178146, -10.72451020669898902, 21.66557627198102409 ) ) ;
#129245=CARTESIAN_POINT ( 'NONE',  ( 4.483927247898790824, -16.52544592524335698, 40.20942372801901854 ) ) ;
#129246=CARTESIAN_POINT ( 'NONE',  ( 19.03943276465977164, -0.05219959533909143690, 53.74890960531436690 ) ) ;
#129247=CARTESIAN_POINT ( 'NONE',  ( 15.80617190586769283, -15.72974639402175789, 25.62609039468567929 ) ) ;
#129248=CARTESIAN_POINT ( 'NONE',  ( -19.05341960407617563, 5.049401038297882671, 93.54275706135234714 ) ) ;
#129250=CARTESIAN_POINT ( 'NONE',  ( -0.05219959533909027116, -19.03943276465977164, 107.4989096053143527 ) ) ;
#129251=CARTESIAN_POINT ( 'NONE',  ( 5.153800228976335163, 19.02544592524342804, 89.79057627198102409 ) ) ;
#129252=CARTESIAN_POINT ( 'NONE',  ( 21.55341960407610458, 5.719274019375980345, 93.95724293864770971 ) ) ;
#129253=CARTESIAN_POINT ( 'NONE',  ( 16.51473224551069308, 9.474510206698969483, 64.16557627198102409 ) ) ;
#129255=CARTESIAN_POINT ( 'NONE',  ( 16.52544592524342804, -4.483927247898539470, 73.54057627198102409 ) ) ;
#129256=CARTESIAN_POINT ( 'NONE',  ( -9.474510206698964154, 16.51473224551069663, 105.4155762719810383 ) ) ;
#129258=CARTESIAN_POINT ( 'NONE',  ( -19.05341960407617563, 5.049401038297882671, 78.54275706135233293 ) ) ;
#129259=CARTESIAN_POINT ( 'NONE',  ( -15.72974639402197994, 15.80617190586746368, 85.62390960531436690 ) ) ;
#129260=CARTESIAN_POINT ( 'NONE',  ( 13.97604488694548053, -13.89961937509957401, 45.62609039468566863 ) ) ;
#129261=CARTESIAN_POINT ( 'NONE',  ( 5.823673210054125526, 21.52544592524343514, 24.79057627198103120 ) ) ;
#129262=CARTESIAN_POINT ( 'NONE',  ( 19.25176906914650843, 5.499999999999742428, 68.49927264242278113 ) ) ;
#129263=CARTESIAN_POINT ( 'NONE',  ( 0.05219959533907565091, 21.53943276465977519, 54.99890960531435269 ) ) ;
#129265=CARTESIAN_POINT ( 'NONE',  ( 9.564922557960805705, 16.46253265017160317, 84.58224293864769550 ) ) ;
#129266=CARTESIAN_POINT ( 'NONE',  ( 18.67979575497194134, -10.72451020669871369, 75.83442372801900433 ) ) ;
#129267=CARTESIAN_POINT ( 'NONE',  ( 5.153800228976335163, 19.02544592524342804, 44.79057627198103830 ) ) ;
#129268=CARTESIAN_POINT ( 'NONE',  ( 8.224510206698953496, -14.34966873604960469, 67.91557627198102409 ) ) ;
#129269=CARTESIAN_POINT ( 'NONE',  ( -8.314922557961024197, 14.29746914071037800, 27.91775706135234358 ) ) ;
#129270=CARTESIAN_POINT ( 'NONE',  ( 18.62759615963255655, 10.81492255796105972, 71.66775706135234714 ) ) ;
#129272=CARTESIAN_POINT ( 'NONE',  ( 13.89961937509977652, -13.97604488694527269, 113.1239096053143527 ) ) ;
#129273=CARTESIAN_POINT ( 'NONE',  ( -16.51473224551082808, 9.474510206698731452, 78.33442372801900433 ) ) ;
#129275=CARTESIAN_POINT ( 'NONE',  ( -18.62759615963270932, 10.81492255796079327, 115.8322429386477097 ) ) ;
#129277=CARTESIAN_POINT ( 'NONE',  ( -21.55341960407619339, 5.719274019375674811, 113.5427570613523756 ) ) ;
#129278=CARTESIAN_POINT ( 'NONE',  ( 9.564922557960805705, 16.46253265017160317, 54.58224293864769550 ) ) ;
#129279=CARTESIAN_POINT ( 'NONE',  ( -15.80617190586768217, 15.72974639402176855, 108.1260903946856757 ) ) ;
#129280=CARTESIAN_POINT ( 'NONE',  ( -8.314922557961024197, 14.29746914071037800, 102.9177570613523756 ) ) ;
#129281=CARTESIAN_POINT ( 'NONE',  ( -19.05341960407611168, -5.049401038298163336, 96.45724293864769550 ) ) ;
#129282=CARTESIAN_POINT ( 'NONE',  ( -15.80617190586768217, 15.72974639402176855, 78.12609039468570415 ) ) ;
#129285=CARTESIAN_POINT ( 'NONE',  ( -18.67979575497193778, 10.72451020669871902, 83.33442372801903275 ) ) ;
#129286=CARTESIAN_POINT ( 'NONE',  ( -5.719274019375665041, -21.55341960407619695, 99.79275706135234714 ) ) ;
#129288=CARTESIAN_POINT ( 'NONE',  ( -19.05341960407611168, -5.049401038298163336, 101.4572429386476955 ) ) ;
#129289=CARTESIAN_POINT ( 'NONE',  ( -19.03943276465977164, -0.05219959533935918106, 23.75109039468566152 ) ) ;
#129291=CARTESIAN_POINT ( 'NONE',  ( 16.51473224551069308, 9.474510206698969483, 34.16557627198102409 ) ) ;
#129292=CARTESIAN_POINT ( 'NONE',  ( 5.719274019375991003, -21.55341960407610458, 57.70724293864770260 ) ) ;
#129293=CARTESIAN_POINT ( 'NONE',  ( 0.05219959533934541429, -16.53943276465976808, 110.0010903946856757 ) ) ;
#129294=CARTESIAN_POINT ( 'NONE',  ( -4.483927247898539470, -16.52544592524342804, 97.29057627198105251 ) ) ;
#129295=CARTESIAN_POINT ( 'NONE',  ( 19.02544592524343514, -5.153800228976328945, 83.54057627198100988 ) ) ;
#129296=CARTESIAN_POINT ( 'NONE',  ( -21.53943276465977519, -0.05219959533937600094, 98.75109039468568994 ) ) ;
#129297=CARTESIAN_POINT ( 'NONE',  ( 19.03943276465977164, -0.05219959533909143690, 33.74890960531435979 ) ) ;
#129298=CARTESIAN_POINT ( 'NONE',  ( -16.53943276465976808, 0.05219959533911058130, 106.2489096053143811 ) ) ;
#129299=CARTESIAN_POINT ( 'NONE',  ( 10.72451020669871369, 18.67979575497193778, 52.08442372801901854 ) ) ;
#129300=CARTESIAN_POINT ( 'NONE',  ( 15.72974639402199770, -15.80617190586745480, 83.12390960531436690 ) ) ;
#129301=CARTESIAN_POINT ( 'NONE',  ( -19.05341960407617563, 5.049401038297882671, 48.54275706135233293 ) ) ;
#129303=CARTESIAN_POINT ( 'NONE',  ( 5.153800228976335163, 19.02544592524342804, 99.79057627198102409 ) ) ;
#129304=CARTESIAN_POINT ( 'NONE',  ( 4.379528057220339221, -16.55341960407611168, 82.70724293864770971 ) ) ;
#129305=CARTESIAN_POINT ( 'NONE',  ( -9.564922557961040184, 16.46253265017147172, 47.91775706135233293 ) ) ;
#129306=CARTESIAN_POINT ( 'NONE',  ( 9.474510206698971260, -16.51473224551069308, 67.91557627198102409 ) ) ;
#129307=CARTESIAN_POINT ( 'NONE',  ( 4.483927247898545687, 16.52544592524342804, 49.79057627198102409 ) ) ;
#129308=CARTESIAN_POINT ( 'NONE',  ( -19.02544592524334988, -5.153800228976617603, 78.95942372801900433 ) ) ;
#129309=CARTESIAN_POINT ( 'NONE',  ( -18.87075004821571866, 5.499999999999900524, 83.67408112101044537 ) ) ;
#129310=CARTESIAN_POINT ( 'NONE',  ( 18.67979575497178502, 10.72451020669898547, 34.16557627198102409 ) ) ;
#129311=CARTESIAN_POINT ( 'NONE',  ( 4.483927247898545687, 16.52544592524342804, 104.7905762719810241 ) ) ;
#129312=CARTESIAN_POINT ( 'NONE',  ( -17.49999999999999645, -5.500000000000000888, 24.20309617465829533 ) ) ;
#129313=CARTESIAN_POINT ( 'NONE',  ( 19.05341960407611168, 5.049401038298154454, 58.95724293864768129 ) ) ;
#129314=CARTESIAN_POINT ( 'NONE',  ( 21.52544592524344225, -5.823673210054117533, 68.54057627198103830 ) ) ;
#129315=CARTESIAN_POINT ( 'NONE',  ( -16.51473224551069308, -9.474510206698971260, 26.66557627198103120 ) ) ;
#129316=CARTESIAN_POINT ( 'NONE',  ( 4.379528057220092307, 16.55341960407617563, 72.29275706135236135 ) ) ;
#129317=CARTESIAN_POINT ( 'NONE',  ( -5.049401038298153566, 19.05341960407611168, 55.20724293864769550 ) ) ;
#129318=CARTESIAN_POINT ( 'NONE',  ( -13.97604488694547697, 13.89961937509957934, 53.12609039468565442 ) ) ;
#129319=CARTESIAN_POINT ( 'NONE',  ( -15.80617190586768217, 15.72974639402176855, 68.12609039468567573 ) ) ;
#129320=CARTESIAN_POINT ( 'NONE',  ( -18.62759615963270932, 10.81492255796079327, 45.83224293864769550 ) ) ;
#129322=CARTESIAN_POINT ( 'NONE',  ( -12.06949235617756955, 12.14591786802309770, 115.6239096053143669 ) ) ;
#129323=CARTESIAN_POINT ( 'NONE',  ( -12.14591786802326823, 12.06949235617739902, 88.12609039468570415 ) ) ;
#129325=CARTESIAN_POINT ( 'NONE',  ( 5.153800228976615827, -19.02544592524334988, 105.2094237280190185 ) ) ;
#129326=CARTESIAN_POINT ( 'NONE',  ( -19.03943276465977164, 0.05219959533909376836, 26.24890960531435624 ) ) ;
#129328=CARTESIAN_POINT ( 'NONE',  ( -21.52544592524343514, 5.823673210054127303, 56.04057627198102409 ) ) ;
#129329=CARTESIAN_POINT ( 'NONE',  ( -15.72974639402176322, -15.80617190586768395, 94.37609039468568994 ) ) ;
#129330=CARTESIAN_POINT ( 'NONE',  ( -16.52544592524342804, 4.483927247898546575, 51.04057627198103120 ) ) ;
#129331=CARTESIAN_POINT ( 'NONE',  ( -16.52544592524342804, 4.483927247898546575, 51.04057627198103120 ) ) ;
#129332=CARTESIAN_POINT ( 'NONE',  ( -10.72451020669898014, 18.67979575497178502, 80.41557627198103830 ) ) ;
#129333=CARTESIAN_POINT ( 'NONE',  ( 0.05219959533907565091, 21.53943276465977519, 84.99890960531436690 ) ) ;
#129335=CARTESIAN_POINT ( 'NONE',  ( -0.05219959533907301413, -21.53943276465977519, 37.49890960531436690 ) ) ;
#129336=CARTESIAN_POINT ( 'NONE',  ( -12.06949235617739369, -12.14591786802326823, 69.37609039468567573 ) ) ;
#129337=CARTESIAN_POINT ( 'NONE',  ( 12.06949235617757843, -12.14591786802309237, 83.12390960531436690 ) ) ;
#129338=CARTESIAN_POINT ( 'NONE',  ( -16.46253265017160317, 9.564922557960807481, 30.83224293864769550 ) ) ;
#129340=DIRECTION ( 'NONE',  ( 0.000000000000000000, -0.000000000000000000, -1.000000000000000000 ) ) ;
#129341=ORIENTED_EDGE ( 'NONE', *, *, #122751, .T. ) ;
#129342=CARTESIAN_POINT ( 'NONE',  ( 12.14591786802327356, -12.06949235617739191, 90.62609039468567573 ) ) ;
#129343=CARTESIAN_POINT ( 'NONE',  ( -10.81492255796078084, -18.62759615963271287, 112.0822429386477097 ) ) ;
#129344=CARTESIAN_POINT ( 'NONE',  ( -0.05219959533909027116, -19.03943276465977164, 77.49890960531435269 ) ) ;
#129345=CARTESIAN_POINT ( 'NONE',  ( -10.72451020669870658, -18.67979575497194134, 49.58442372801901143 ) ) ;
#129346=CARTESIAN_POINT ( 'NONE',  ( 19.05341960407611168, 5.049401038298154454, 113.9572429386477097 ) ) ;
#129349=CARTESIAN_POINT ( 'NONE',  ( -21.53943276465977519, -0.05219959533937600094, 48.75109039468568284 ) ) ;
#129350=CARTESIAN_POINT ( 'NONE',  ( 19.05341960407611168, 5.049401038298154454, 38.95724293864767418 ) ) ;
#129351=CARTESIAN_POINT ( 'NONE',  ( 5.153800228976335163, 19.02544592524342804, 109.7905762719810099 ) ) ;
#129352=CARTESIAN_POINT ( 'NONE',  ( 13.97604488694548053, -13.89961937509957401, 50.62609039468566152 ) ) ;
#129353=CARTESIAN_POINT ( 'NONE',  ( -21.53943276465977519, -0.05219959533937600094, 33.75109039468568284 ) ) ;
#129354=CARTESIAN_POINT ( 'NONE',  ( -16.46253265017146816, -9.564922557961047289, 39.16775706135234003 ) ) ;
#129355=CARTESIAN_POINT ( 'NONE',  ( 5.153800228976335163, 19.02544592524342804, 29.79057627198102409 ) ) ;
#129356=CARTESIAN_POINT ( 'NONE',  ( 4.483927247898790824, -16.52544592524335698, 90.20942372801903275 ) ) ;
#129357=CARTESIAN_POINT ( 'NONE',  ( -0.05219959533936034679, 19.03943276465977164, 62.50109039468566863 ) ) ;
#129358=CARTESIAN_POINT ( 'NONE',  ( -8.224510206698735004, -14.34966873604973081, 109.5844237280190328 ) ) ;
#129359=CARTESIAN_POINT ( 'NONE',  ( 17.60691670004650788, 5.500000000000064837, 86.63333313366442212 ) ) ;
#129360=CARTESIAN_POINT ( 'NONE',  ( 5.153800228976335163, 19.02544592524342804, 79.79057627198102409 ) ) ;
#129361=CARTESIAN_POINT ( 'NONE',  ( -5.823673210054431948, 21.52544592524334988, 97.70942372801904696 ) ) ;
#129362=CARTESIAN_POINT ( 'NONE',  ( -10.72451020669870658, -18.67979575497194134, 104.5844237280190185 ) ) ;
#129363=CARTESIAN_POINT ( 'NONE',  ( 18.22780087662122739, 5.500000000000000888, 66.48236817873106475 ) ) ;
#129364=CARTESIAN_POINT ( 'NONE',  ( -5.049401038298153566, 19.05341960407611168, 105.2072429386476671 ) ) ;
#129365=CARTESIAN_POINT ( 'NONE',  ( -18.67979575497193778, 10.72451020669871902, 78.33442372801901854 ) ) ;
#129366=CARTESIAN_POINT ( 'NONE',  ( -12.14591786802326823, 12.06949235617739902, 23.12609039468567573 ) ) ;
#129367=CARTESIAN_POINT ( 'NONE',  ( 19.02544592524343514, -5.153800228976328945, 78.54057627198099567 ) ) ;
#129368=CARTESIAN_POINT ( 'NONE',  ( -18.67979575497178146, -10.72451020669898902, 31.66557627198102054 ) ) ;
#129369=CARTESIAN_POINT ( 'NONE',  ( 16.46253265017160672, -9.564922557960803928, 98.33224293864769550 ) ) ;
#129371=CARTESIAN_POINT ( 'NONE',  ( 13.89961937509977652, -13.97604488694527269, 73.12390960531436690 ) ) ;
#129372=CARTESIAN_POINT ( 'NONE',  ( 9.564922557960805705, 16.46253265017160317, 69.58224293864770971 ) ) ;
#129373=CARTESIAN_POINT ( 'NONE',  ( 4.483927247898545687, 16.52544592524342804, 24.79057627198103120 ) ) ;
#129374=CARTESIAN_POINT ( 'NONE',  ( 16.46253265017146816, 9.564922557961045513, 66.66775706135233293 ) ) ;
#129375=CARTESIAN_POINT ( 'NONE',  ( 9.564922557960805705, 16.46253265017160317, 89.58224293864769550 ) ) ;
#129376=CARTESIAN_POINT ( 'NONE',  ( 16.55341960407611168, 4.379528057220329451, 83.95724293864770971 ) ) ;
#129377=CARTESIAN_POINT ( 'NONE',  ( -15.72974639402197994, 15.80617190586746368, 40.62390960531435269 ) ) ;
#129378=( BOUNDED_CURVE ( )  B_SPLINE_CURVE ( 2, ( #107905, #152433, #183779, #199944, #154425, #45265, #43275, #103951, #76585, #119132, #136276, #31089, #168592 ),
 .UNSPECIFIED., .F., .F. ) 
 B_SPLINE_CURVE_WITH_KNOTS ( ( 3, 2, 2, 2, 2, 2, 3 ),
 ( 0.2655883311638872479, 0.2675438596491228060, 0.2719298245614035214, 0.2763157894736842368, 0.2807017543859648967, 0.2850877192982456121, 0.2869975679613910868 ),
 .UNSPECIFIED. ) 
 CURVE ( )  GEOMETRIC_REPRESENTATION_ITEM ( )  RATIONAL_B_SPLINE_CURVE ( ( 0.9831626618144004848, 0.9848076720550091867, 1.000000000000000000, 0.9659258262890683122, 1.000000000000000000, 0.9659258262890683122, 1.000000000000000000, 0.9659258262890683122, 1.000000000000000000, 0.9659258262890683122, 1.000000000000000000, 0.9851625545550091179, 0.9832469066685282089 ) ) 
 REPRESENTATION_ITEM ( '' )  );
#129379=CARTESIAN_POINT ( 'NONE',  ( 15.72974639402199770, -15.80617190586745480, 28.12390960531435979 ) ) ;
#129380=CARTESIAN_POINT ( 'NONE',  ( 16.53943276465976808, -0.05219959533910856209, 108.7489096053143669 ) ) ;
#129382=CARTESIAN_POINT ( 'NONE',  ( -13.97604488694547697, 13.89961937509957934, 38.12609039468566152 ) ) ;
#129383=CARTESIAN_POINT ( 'NONE',  ( -16.52544592524342804, 4.483927247898546575, 26.04057627198103475 ) ) ;
#129384=CARTESIAN_POINT ( 'NONE',  ( -13.97604488694527625, -13.89961937509977652, 96.87390960531433848 ) ) ;
#129385=CARTESIAN_POINT ( 'NONE',  ( 5.823673210054444382, -21.52544592524334988, 70.20942372801904696 ) ) ;
#129386=CARTESIAN_POINT ( 'NONE',  ( 21.53943276465977519, -0.05219959533907433946, 58.74890960531436690 ) ) ;
#129387=CARTESIAN_POINT ( 'NONE',  ( 21.52544592524334988, 5.823673210054432836, 31.45942372801901854 ) ) ;
#129388=CARTESIAN_POINT ( 'NONE',  ( 18.67979575497178502, 10.72451020669898547, 84.16557627198103830 ) ) ;
#129389=CARTESIAN_POINT ( 'NONE',  ( 18.67979575497194134, -10.72451020669871369, 40.83442372801901854 ) ) ;
#129390=CARTESIAN_POINT ( 'NONE',  ( 4.379528057220339221, -16.55341960407611168, 107.7072429386476955 ) ) ;
#129391=CARTESIAN_POINT ( 'NONE',  ( -9.474510206698720793, -16.51473224551083518, 69.58442372801901854 ) ) ;
#129392=CARTESIAN_POINT ( 'NONE',  ( 19.05341960407611168, 5.049401038298154454, 38.95724293864767418 ) ) ;
#129393=CARTESIAN_POINT ( 'NONE',  ( -12.06949235617756955, 12.14591786802309770, 85.62390960531436690 ) ) ;
#129394=CARTESIAN_POINT ( 'NONE',  ( 19.03943276465977164, -0.05219959533909143690, 113.7489096053143669 ) ) ;
#129395=CARTESIAN_POINT ( 'NONE',  ( 9.474510206698971260, -16.51473224551069308, 27.91557627198103120 ) ) ;
#129396=CARTESIAN_POINT ( 'NONE',  ( 4.379528057220339221, -16.55341960407611168, 37.70724293864769550 ) ) ;
#129397=CARTESIAN_POINT ( 'NONE',  ( -12.06949235617739369, -12.14591786802326823, 94.37609039468568994 ) ) ;
#129398=CARTESIAN_POINT ( 'NONE',  ( 0.05219959533909260263, 19.03943276465977164, 49.99890960531435979 ) ) ;
#129399=CARTESIAN_POINT ( 'NONE',  ( -19.05341960407611168, -5.049401038298163336, 26.45724293864769550 ) ) ;
#129400=CARTESIAN_POINT ( 'NONE',  ( 13.97604488694548053, -13.89961937509957401, 25.62609039468566507 ) ) ;
#129402=CARTESIAN_POINT ( 'NONE',  ( -0.05219959533910754901, -16.53943276465976808, 42.49890960531435979 ) ) ;
#129403=CARTESIAN_POINT ( 'NONE',  ( -10.72451020669870658, -18.67979575497194134, 44.58442372801901854 ) ) ;
#129405=CARTESIAN_POINT ( 'NONE',  ( -14.29746914071037622, -8.314922557961029526, 59.16775706135234714 ) ) ;
#129406=CARTESIAN_POINT ( 'NONE',  ( -0.05219959533910754901, -16.53943276465976808, 27.49890960531435269 ) ) ;
#129407=CARTESIAN_POINT ( 'NONE',  ( -8.314922557961024197, 14.29746914071037800, 112.9177570613523329 ) ) ;
#129408=CARTESIAN_POINT ( 'NONE',  ( 4.379528057220092307, 16.55341960407617563, 32.29275706135235424 ) ) ;
#129409=CARTESIAN_POINT ( 'NONE',  ( 5.153800228976335163, 19.02544592524342804, 54.79057627198103120 ) ) ;
#129410=CARTESIAN_POINT ( 'NONE',  ( -16.53943276465976808, 0.05219959533911058130, 106.2489096053143811 ) ) ;
#129411=CARTESIAN_POINT ( 'NONE',  ( 21.55341960407619695, -5.719274019375665929, 21.04275706135234714 ) ) ;
#129412=CARTESIAN_POINT ( 'NONE',  ( -0.05219959533909027116, -19.03943276465977164, 42.49890960531435269 ) ) ;
#129413=CARTESIAN_POINT ( 'NONE',  ( 0.05219959533909260263, 19.03943276465977164, 114.9989096053143669 ) ) ;
#129414=CARTESIAN_POINT ( 'NONE',  ( 5.049401038298161559, -19.05341960407611168, 27.70724293864769550 ) ) ;
#129415=CARTESIAN_POINT ( 'NONE',  ( -9.474510206698964154, 16.51473224551069663, 115.4155762719810241 ) ) ;
#129416=CARTESIAN_POINT ( 'NONE',  ( -17.48853670773245028, -5.747243402303086945, 36.33328700250008580 ) ) ;
#129417=CARTESIAN_POINT ( 'NONE',  ( 0.05219959533909260263, 19.03943276465977164, 99.99890960531436690 ) ) ;
#129418=CARTESIAN_POINT ( 'NONE',  ( -10.81492255796105439, 18.62759615963255655, 42.91775706135235424 ) ) ;
#129419=CARTESIAN_POINT ( 'NONE',  ( 4.483927247898545687, 16.52544592524342804, 99.79057627198103830 ) ) ;
#129420=CARTESIAN_POINT ( 'NONE',  ( 19.05341960407611168, 5.049401038298154454, 103.9572429386476671 ) ) ;
#129421=CARTESIAN_POINT ( 'NONE',  ( 17.97182807773873137, -5.499999999999949374, 96.03038844047289047 ) ) ;
#129422=CARTESIAN_POINT ( 'NONE',  ( -16.52544592524335698, -4.483927247898792601, 73.95942372801901854 ) ) ;
#129423=CARTESIAN_POINT ( 'NONE',  ( 18.67979575497194134, -10.72451020669871369, 90.83442372801901854 ) ) ;
#129424=CARTESIAN_POINT ( 'NONE',  ( 16.52544592524335698, 4.483927247898782831, 51.45942372801901854 ) ) ;
#129425=CARTESIAN_POINT ( 'NONE',  ( -9.564922557960796823, -16.46253265017161027, 102.0822429386477097 ) ) ;
#129426=CARTESIAN_POINT ( 'NONE',  ( -4.379528057220086978, -16.55341960407618274, 39.79275706135235424 ) ) ;
#129427=CARTESIAN_POINT ( 'NONE',  ( -5.153800228976607833, 19.02544592524334988, 102.7094237280189759 ) ) ;
#129428=CARTESIAN_POINT ( 'NONE',  ( -0.05219959533934338120, 16.53943276465976808, 77.50109039468567573 ) ) ;
#129429=CARTESIAN_POINT ( 'NONE',  ( 13.89961937509957401, 13.97604488694547697, 106.8760903946856757 ) ) ;
#129430=CARTESIAN_POINT ( 'NONE',  ( 19.03943276465977164, -0.05219959533909143690, 73.74890960531435269 ) ) ;
#129431=CARTESIAN_POINT ( 'NONE',  ( -21.53943276465977519, 0.05219959533907696930, 91.24890960531436690 ) ) ;
#129432=CARTESIAN_POINT ( 'NONE',  ( 12.06949235617757843, -12.14591786802309237, 108.1239096053143811 ) ) ;
#129433=CARTESIAN_POINT ( 'NONE',  ( -5.153800228976607833, 19.02544592524334988, 102.7094237280189759 ) ) ;
#129434=CARTESIAN_POINT ( 'NONE',  ( 8.224510206698742110, 14.34966873604972548, 77.08442372801901854 ) ) ;
#129435=CARTESIAN_POINT ( 'NONE',  ( -17.40861289039009208, 6.110651285853054837, 43.62767529172568715 ) ) ;
#129436=CARTESIAN_POINT ( 'NONE',  ( 5.153800228976615827, -19.02544592524334988, 70.20942372801899012 ) ) ;
#129437=CARTESIAN_POINT ( 'NONE',  ( 16.53943276465976808, -0.05219959533910856209, 33.74890960531436690 ) ) ;
#129438=CARTESIAN_POINT ( 'NONE',  ( 8.314922557960818139, 14.29746914071049879, 89.58224293864768129 ) ) ;
#129439=CARTESIAN_POINT ( 'NONE',  ( 9.564922557961047289, -16.46253265017146816, 40.41775706135234003 ) ) ;
#129440=DIRECTION ( 'NONE',  ( -0.000000000000000000, -0.000000000000000000, 1.000000000000000000 ) ) ;
#129441=CARTESIAN_POINT ( 'NONE',  ( -10.81492255796105439, 18.62759615963255655, 32.91775706135234714 ) ) ;
#129442=CARTESIAN_POINT ( 'NONE',  ( 13.89961937509957401, 13.97604488694547697, 101.8760903946856331 ) ) ;
#129443=CARTESIAN_POINT ( 'NONE',  ( 5.153800228976335163, 19.02544592524342804, 109.7905762719810099 ) ) ;
#129444=CARTESIAN_POINT ( 'NONE',  ( 13.97604488694527802, 13.89961937509977652, 89.37390960531436690 ) ) ;
#129445=CARTESIAN_POINT ( 'NONE',  ( 18.62759615963255655, 10.81492255796105972, 101.6677570613523613 ) ) ;
#129446=CARTESIAN_POINT ( 'NONE',  ( -16.51473224551069308, -9.474510206698971260, 81.66557627198103830 ) ) ;
#129447=CARTESIAN_POINT ( 'NONE',  ( 15.80617190586746368, 15.72974639402197994, 39.37390960531436690 ) ) ;
#129448=CARTESIAN_POINT ( 'NONE',  ( -4.379528057220328563, 16.55341960407611168, 95.20724293864769550 ) ) ;
#129449=CARTESIAN_POINT ( 'NONE',  ( 9.474510206698971260, -16.51473224551069308, 52.91557627198102409 ) ) ;
#129450=CARTESIAN_POINT ( 'NONE',  ( -14.34966873604960291, -8.224510206698953496, 106.6655762719810383 ) ) ;
#129451=CARTESIAN_POINT ( 'NONE',  ( 18.67979575497194134, -10.72451020669871369, 20.83442372801901143 ) ) ;
#129452=CARTESIAN_POINT ( 'NONE',  ( 10.72451020669871369, 18.67979575497193778, 72.08442372801899012 ) ) ;
#129453=CARTESIAN_POINT ( 'NONE',  ( -19.05341960407611168, -5.049401038298163336, 41.45724293864769550 ) ) ;
#129454=CARTESIAN_POINT ( 'NONE',  ( 0.05219959533934541429, -16.53943276465976808, 75.00109039468568994 ) ) ;
#129455=CARTESIAN_POINT ( 'NONE',  ( -15.72974639402197994, 15.80617190586746368, 115.6239096053143669 ) ) ;
#129456=ORIENTED_EDGE ( 'NONE', *, *, #133810, .T. ) ;
#129457=CARTESIAN_POINT ( 'NONE',  ( -10.72451020669870658, -18.67979575497194134, 29.58442372801901854 ) ) ;
#129458=CARTESIAN_POINT ( 'NONE',  ( -0.05219959533936034679, 19.03943276465977164, 52.50109039468566863 ) ) ;
#129459=CARTESIAN_POINT ( 'NONE',  ( -5.153800228976328057, -19.02544592524343514, 62.29057627198100988 ) ) ;
#129460=CARTESIAN_POINT ( 'NONE',  ( -16.51473224551082808, 9.474510206698731452, 38.33442372801899722 ) ) ;
#129461=CARTESIAN_POINT ( 'NONE',  ( 10.72451020669871369, 18.67979575497193778, 72.08442372801899012 ) ) ;
#129462=CARTESIAN_POINT ( 'NONE',  ( 5.823673210054125526, 21.52544592524343514, 69.79057627198102409 ) ) ;
#129463=CARTESIAN_POINT ( 'NONE',  ( -8.224510206698948167, 14.34966873604960824, 45.41557627198103830 ) ) ;
#129464=CARTESIAN_POINT ( 'NONE',  ( 21.52544592524334988, 5.823673210054432836, 91.45942372801901854 ) ) ;
#129465=CARTESIAN_POINT ( 'NONE',  ( -13.89961937509957401, -13.97604488694547875, 29.37609039468565797 ) ) ;
#129466=CARTESIAN_POINT ( 'NONE',  ( 16.55341960407611168, 4.379528057220329451, 73.95724293864769550 ) ) ;
#129467=CARTESIAN_POINT ( 'NONE',  ( 0.05219959533910956823, 16.53943276465976808, 114.9989096053143669 ) ) ;
#129468=CARTESIAN_POINT ( 'NONE',  ( -19.02544592524334988, -5.153800228976617603, 58.95942372801900433 ) ) ;
#129469=CARTESIAN_POINT ( 'NONE',  ( 8.224510206698742110, 14.34966873604972548, 112.0844237280190185 ) ) ;
#129470=CARTESIAN_POINT ( 'NONE',  ( -10.72451020669870658, -18.67979575497194134, 84.58442372801903275 ) ) ;
#129471=CARTESIAN_POINT ( 'NONE',  ( -19.02544592524334988, -5.153800228976617603, 48.95942372801900433 ) ) ;
#129472=CARTESIAN_POINT ( 'NONE',  ( 21.55341960407610458, 5.719274019375980345, 53.95724293864770260 ) ) ;
#129473=CARTESIAN_POINT ( 'NONE',  ( 18.67979575497194134, -10.72451020669871369, 40.83442372801901854 ) ) ;
#129474=CARTESIAN_POINT ( 'NONE',  ( -10.72451020669898014, 18.67979575497178502, 105.4155762719810383 ) ) ;
#129475=CARTESIAN_POINT ( 'NONE',  ( -0.05219959533936034679, 19.03943276465977164, 92.50109039468566152 ) ) ;
#129476=CARTESIAN_POINT ( 'NONE',  ( 4.483927247898790824, -16.52544592524335698, 70.20942372801904696 ) ) ;
#129478=CARTESIAN_POINT ( 'NONE',  ( 5.719274019375991003, -21.55341960407610458, 112.7072429386476955 ) ) ;
#129479=CARTESIAN_POINT ( 'NONE',  ( 16.52544592524342804, -4.483927247898539470, 88.54057627198103830 ) ) ;
#129480=CARTESIAN_POINT ( 'NONE',  ( -17.49999999999999645, -3.850315288878745967, 30.73370869396548954 ) ) ;
#129481=CARTESIAN_POINT ( 'NONE',  ( -8.224510206698735004, -14.34966873604973081, 34.58442372801900433 ) ) ;
#129483=CARTESIAN_POINT ( 'NONE',  ( 18.62759615963271287, -10.81492255796078972, 53.33224293864769550 ) ) ;
#129484=CARTESIAN_POINT ( 'NONE',  ( -16.53943276465976808, -0.05219959533934237506, 88.75109039468567573 ) ) ;
#129485=CARTESIAN_POINT ( 'NONE',  ( 19.03943276465977164, -0.05219959533909143690, 23.74890960531435269 ) ) ;
#129486=CARTESIAN_POINT ( 'NONE',  ( 16.53943276465976808, 0.05219959533934440121, 71.25109039468568994 ) ) ;
#129487=CARTESIAN_POINT ( 'NONE',  ( 18.62759615963255655, 10.81492255796105972, 46.66775706135234714 ) ) ;
#129488=CARTESIAN_POINT ( 'NONE',  ( 5.823673210054125526, 21.52544592524343514, 64.79057627198103830 ) ) ;
#129489=CARTESIAN_POINT ( 'NONE',  ( -14.29746914071037622, -8.314922557961029526, 79.16775706135234714 ) ) ;
#129490=CARTESIAN_POINT ( 'NONE',  ( -10.81492255796105439, 18.62759615963255655, 67.91775706135234714 ) ) ;
#129492=CARTESIAN_POINT ( 'NONE',  ( 10.72451020669898902, -18.67979575497178502, 52.91557627198103830 ) ) ;
#129493=CARTESIAN_POINT ( 'NONE',  ( 10.81492255796078972, 18.62759615963270932, 39.58224293864769550 ) ) ;
#129494=CARTESIAN_POINT ( 'NONE',  ( -14.29746914071037622, -8.314922557961029526, 59.16775706135234714 ) ) ;
#129495=CARTESIAN_POINT ( 'NONE',  ( -21.52544592524343514, 5.823673210054127303, 31.04057627198102409 ) ) ;
#129496=CARTESIAN_POINT ( 'NONE',  ( -13.97604488694527625, -13.89961937509977652, 101.8739096053143811 ) ) ;
#129497=CARTESIAN_POINT ( 'NONE',  ( 4.483927247898545687, 16.52544592524342804, 24.79057627198103120 ) ) ;
#129498=CARTESIAN_POINT ( 'NONE',  ( 12.06949235617757843, -12.14591786802309237, 113.1239096053143953 ) ) ;
#129499=CARTESIAN_POINT ( 'NONE',  ( -21.53943276465977519, 0.05219959533907696930, 46.24890960531435979 ) ) ;
#129500=CARTESIAN_POINT ( 'NONE',  ( -13.97604488694527625, -13.89961937509977652, 46.87390960531435979 ) ) ;
#129501=CARTESIAN_POINT ( 'NONE',  ( -4.379528057220086978, -16.55341960407618274, 94.79275706135234714 ) ) ;
#129502=CARTESIAN_POINT ( 'NONE',  ( -10.72451020669870658, -18.67979575497194134, 29.58442372801901854 ) ) ;
#129503=CARTESIAN_POINT ( 'NONE',  ( -9.564922557961040184, 16.46253265017147172, 92.91775706135233293 ) ) ;
#129504=CARTESIAN_POINT ( 'NONE',  ( -12.14591786802309592, -12.06949235617757132, 106.8739096053143811 ) ) ;
#129505=CARTESIAN_POINT ( 'NONE',  ( -19.03943276465977164, 0.05219959533909376836, 56.24890960531435979 ) ) ;
#129506=CARTESIAN_POINT ( 'NONE',  ( -0.05219959533909027116, -19.03943276465977164, 22.49890960531436690 ) ) ;
#129507=FACE_OUTER_BOUND ( 'NONE', #181687, .T. ) ;
#129508=CARTESIAN_POINT ( 'NONE',  ( 19.03943276465977164, -0.05219959533909143690, 78.74890960531436690 ) ) ;
#129509=CARTESIAN_POINT ( 'NONE',  ( 0.05219959533934541429, -16.53943276465976808, 65.00109039468568994 ) ) ;
#129510=CARTESIAN_POINT ( 'NONE',  ( -5.823673210054431948, 21.52544592524334988, 102.7094237280190185 ) ) ;
#129511=CARTESIAN_POINT ( 'NONE',  ( -21.55341960407610458, -5.719274019375992779, 46.45724293864769550 ) ) ;
#129512=CARTESIAN_POINT ( 'NONE',  ( -4.483927247898782831, 16.52544592524335698, 72.70942372801901854 ) ) ;
#129513=CARTESIAN_POINT ( 'NONE',  ( -19.05341960407617563, 5.049401038297882671, 63.54275706135234003 ) ) ;
#129515=CARTESIAN_POINT ( 'NONE',  ( 21.52544592524334988, 5.823673210054432836, 61.45942372801901854 ) ) ;
#129516=CARTESIAN_POINT ( 'NONE',  ( 9.474510206698971260, -16.51473224551069308, 62.91557627198102409 ) ) ;
#129517=CARTESIAN_POINT ( 'NONE',  ( -0.05219959533909027116, -19.03943276465977164, 32.49890960531435979 ) ) ;
#129518=CARTESIAN_POINT ( 'NONE',  ( -19.03943276465977164, -0.05219959533935918106, 63.75109039468566863 ) ) ;
#129519=CARTESIAN_POINT ( 'NONE',  ( 13.97604488694527802, 13.89961937509977652, 109.3739096053143669 ) ) ;
#129520=CARTESIAN_POINT ( 'NONE',  ( 13.97604488694527802, 13.89961937509977652, 89.37390960531436690 ) ) ;
#129521=CARTESIAN_POINT ( 'NONE',  ( 12.06949235617757843, -12.14591786802309237, 53.12390960531436690 ) ) ;
#129522=CARTESIAN_POINT ( 'NONE',  ( -10.81492255796078084, -18.62759615963271287, 47.08224293864770260 ) ) ;
#129523=CARTESIAN_POINT ( 'NONE',  ( -17.50000000000014211, 3.417042746626915761, 105.1738039623247545 ) ) ;
#129524=CARTESIAN_POINT ( 'NONE',  ( -16.51473224551082808, 9.474510206698731452, 33.33442372801899722 ) ) ;
#129525=CARTESIAN_POINT ( 'NONE',  ( -17.48847506799967988, -5.747544572773762184, 79.17302562156723411 ) ) ;
#129526=CARTESIAN_POINT ( 'NONE',  ( 5.153800228976335163, 19.02544592524342804, 44.79057627198103830 ) ) ;
#129527=CARTESIAN_POINT ( 'NONE',  ( -19.49190055781010500, -5.500000000000011546, 100.5611608709877913 ) ) ;
#129529=CARTESIAN_POINT ( 'NONE',  ( -14.29746914071037622, -8.314922557961029526, 79.16775706135234714 ) ) ;
#129530=CARTESIAN_POINT ( 'NONE',  ( 15.80617190586746368, 15.72974639402197994, 94.37390960531436690 ) ) ;
#129531=CARTESIAN_POINT ( 'NONE',  ( -5.153800228976328057, -19.02544592524343514, 37.29057627198102409 ) ) ;
#129533=CARTESIAN_POINT ( 'NONE',  ( 21.55341960407619695, -5.719274019375665929, 46.04275706135234714 ) ) ;
#129534=CARTESIAN_POINT ( 'NONE',  ( 13.97604488694548053, -13.89961937509957401, 45.62609039468566863 ) ) ;
#129535=CARTESIAN_POINT ( 'NONE',  ( -19.02544592524342804, 5.153800228976336051, 46.04057627198101699 ) ) ;
#129536=CARTESIAN_POINT ( 'NONE',  ( -21.53943276465977519, -0.05219959533937600094, 98.75109039468568994 ) ) ;
#129537=CARTESIAN_POINT ( 'NONE',  ( 16.29526858892875651, 7.335722546920131037, 98.29670597800206622 ) ) ;
#129538=CARTESIAN_POINT ( 'NONE',  ( 4.379528057220339221, -16.55341960407611168, 42.70724293864770260 ) ) ;
#129540=CARTESIAN_POINT ( 'NONE',  ( -18.62759615963270932, 10.81492255796079327, 50.83224293864770971 ) ) ;
#129542=CARTESIAN_POINT ( 'NONE',  ( 0.05219959533909260263, 19.03943276465977164, 104.9989096053143669 ) ) ;
#129543=CARTESIAN_POINT ( 'NONE',  ( 12.06949235617757843, -12.14591786802309237, 88.12390960531436690 ) ) ;
#129544=CARTESIAN_POINT ( 'NONE',  ( -14.34966873604972548, 8.224510206698743886, 23.33442372801901499 ) ) ;
#129545=CARTESIAN_POINT ( 'NONE',  ( -0.05219959533910754901, -16.53943276465976808, 22.49890960531436335 ) ) ;
#129547=CARTESIAN_POINT ( 'NONE',  ( -9.564922557960796823, -16.46253265017161027, 97.08224293864769550 ) ) ;
#129548=CARTESIAN_POINT ( 'NONE',  ( 21.53943276465977519, -0.05219959533907433946, 103.7489096053143669 ) ) ;
#129549=CARTESIAN_POINT ( 'NONE',  ( -16.53943276465976808, 0.05219959533911058130, 21.24890960531436690 ) ) ;
#129550=CARTESIAN_POINT ( 'NONE',  ( -19.03943276465977164, 0.05219959533909376836, 106.2489096053143669 ) ) ;
#129551=CARTESIAN_POINT ( 'NONE',  ( 19.05341960407617918, -5.049401038297876454, 91.04275706135234714 ) ) ;
#129552=CARTESIAN_POINT ( 'NONE',  ( 5.823673210054444382, -21.52544592524334988, 105.2094237280190328 ) ) ;
#129553=CARTESIAN_POINT ( 'NONE',  ( 10.81492255796078972, 18.62759615963270932, 94.58224293864769550 ) ) ;
#129554=CARTESIAN_POINT ( 'NONE',  ( 10.81492255796078972, 18.62759615963270932, 54.58224293864769550 ) ) ;
#129555=CARTESIAN_POINT ( 'NONE',  ( 9.474510206698971260, -16.51473224551069308, 62.91557627198102409 ) ) ;
#129556=CARTESIAN_POINT ( 'NONE',  ( 0.05219959533910956823, 16.53943276465976808, 34.99890960531435979 ) ) ;
#129557=CARTESIAN_POINT ( 'NONE',  ( 9.474510206698971260, -16.51473224551069308, 77.91557627198103830 ) ) ;
#129558=ORIENTED_EDGE ( 'NONE', *, *, #124318, .T. ) ;
#129559=CARTESIAN_POINT ( 'NONE',  ( 19.01529144963332030, 5.500000000000158096, 58.73431955728438680 ) ) ;
#129560=CARTESIAN_POINT ( 'NONE',  ( -9.564922557961040184, 16.46253265017147172, 47.91775706135233293 ) ) ;
#129561=CARTESIAN_POINT ( 'NONE',  ( -21.55341960407610458, -5.719274019375992779, 86.45724293864770971 ) ) ;
#129562=CARTESIAN_POINT ( 'NONE',  ( -4.379528057220328563, 16.55341960407611168, 80.20724293864769550 ) ) ;
#129563=CARTESIAN_POINT ( 'NONE',  ( -5.823673210054431948, 21.52544592524334988, 27.70942372801901854 ) ) ;
#129565=CARTESIAN_POINT ( 'NONE',  ( 16.53943276465976808, 0.05219959533934440121, 111.2510903946856899 ) ) ;
#129566=CARTESIAN_POINT ( 'NONE',  ( -13.97604488694527625, -13.89961937509977652, 26.87390960531434558 ) ) ;
#129567=CARTESIAN_POINT ( 'NONE',  ( -5.153800228976328057, -19.02544592524343514, 67.29057627198102409 ) ) ;
#129570=CARTESIAN_POINT ( 'NONE',  ( 0.05219959533910956823, 16.53943276465976808, 44.99890960531435979 ) ) ;
#129571=CARTESIAN_POINT ( 'NONE',  ( 10.72451020669871369, 18.67979575497193778, 62.08442372801901143 ) ) ;
#129573=CARTESIAN_POINT ( 'NONE',  ( -16.46253265017160317, 9.564922557960807481, 45.83224293864769550 ) ) ;
#129574=CARTESIAN_POINT ( 'NONE',  ( 5.153800228976335163, 19.02544592524342804, 49.79057627198100988 ) ) ;
#129576=CARTESIAN_POINT ( 'NONE',  ( -10.81492255796105439, 18.62759615963255655, 107.9177570613523471 ) ) ;
#129577=CARTESIAN_POINT ( 'NONE',  ( 4.379528057220092307, 16.55341960407617563, 67.29275706135234714 ) ) ;
#129578=CARTESIAN_POINT ( 'NONE',  ( 15.80617190586769283, -15.72974639402175789, 85.62609039468568994 ) ) ;
#129579=CARTESIAN_POINT ( 'NONE',  ( -9.474510206698964154, 16.51473224551069663, 110.4155762719810383 ) ) ;
#129581=CARTESIAN_POINT ( 'NONE',  ( -9.564922557961040184, 16.46253265017147172, 92.91775706135233293 ) ) ;
#129582=CARTESIAN_POINT ( 'NONE',  ( 21.52544592524334988, 5.823673210054432836, 71.45942372801901854 ) ) ;
#129583=CARTESIAN_POINT ( 'NONE',  ( -4.483927247898782831, 16.52544592524335698, 37.70942372801900433 ) ) ;
#129584=CARTESIAN_POINT ( 'NONE',  ( -15.80617190586745835, -15.72974639402198527, 91.87390960531436690 ) ) ;
#129585=CARTESIAN_POINT ( 'NONE',  ( -13.97604488694547697, 13.89961937509957934, 103.1260903946856473 ) ) ;
#129586=CARTESIAN_POINT ( 'NONE',  ( 16.51473224551069308, 9.474510206698969483, 64.16557627198102409 ) ) ;
#129587=CARTESIAN_POINT ( 'NONE',  ( -13.97604488694547697, 13.89961937509957934, 103.1260903946856473 ) ) ;
#129588=CARTESIAN_POINT ( 'NONE',  ( -0.05219959533936034679, 19.03943276465977164, 97.50109039468567573 ) ) ;
#129589=CARTESIAN_POINT ( 'NONE',  ( -4.379528057220328563, 16.55341960407611168, 55.20724293864770260 ) ) ;
#129590=CARTESIAN_POINT ( 'NONE',  ( -19.02544592524334988, -5.153800228976617603, 78.95942372801900433 ) ) ;
#129591=CARTESIAN_POINT ( 'NONE',  ( -8.314922557961024197, 14.29746914071037800, 57.91775706135234714 ) ) ;
#129592=CARTESIAN_POINT ( 'NONE',  ( 18.67979575497194134, -10.72451020669871369, 20.83442372801901143 ) ) ;
#129593=CARTESIAN_POINT ( 'NONE',  ( -13.97604488694527625, -13.89961937509977652, 31.87390960531435979 ) ) ;
#129594=CARTESIAN_POINT ( 'NONE',  ( 13.97604488694527802, 13.89961937509977652, 49.37390960531434558 ) ) ;
#129595=CARTESIAN_POINT ( 'NONE',  ( -14.29746914071037622, -8.314922557961029526, 64.16775706135234714 ) ) ;
#129598=CARTESIAN_POINT ( 'NONE',  ( 0.05219959533909260263, 19.03943276465977164, 99.99890960531436690 ) ) ;
#129599=CARTESIAN_POINT ( 'NONE',  ( -5.153800228976328057, -19.02544592524343514, 27.29057627198103120 ) ) ;
#129601=CARTESIAN_POINT ( 'NONE',  ( 5.153800228976615827, -19.02544592524334988, 110.2094237280189901 ) ) ;
#129602=CARTESIAN_POINT ( 'NONE',  ( 15.72974639402199770, -15.80617190586745480, 43.12390960531435269 ) ) ;
#129603=CARTESIAN_POINT ( 'NONE',  ( -16.46253265017146816, -9.564922557961047289, 49.16775706135233293 ) ) ;
#129604=CARTESIAN_POINT ( 'NONE',  ( 4.483927247898790824, -16.52544592524335698, 25.20942372801901854 ) ) ;
#129605=CARTESIAN_POINT ( 'NONE',  ( 19.02544592524343514, -5.153800228976328945, 23.54057627198102054 ) ) ;
#129606=CARTESIAN_POINT ( 'NONE',  ( 16.51473224551069308, 9.474510206698969483, 54.16557627198103120 ) ) ;
#129607=CARTESIAN_POINT ( 'NONE',  ( -18.67979575497178146, -10.72451020669898902, 91.66557627198103830 ) ) ;
#129608=CARTESIAN_POINT ( 'NONE',  ( 13.89961937509977652, -13.97604488694527269, 98.12390960531433848 ) ) ;
#129610=CARTESIAN_POINT ( 'NONE',  ( -19.03943276465977164, 0.05219959533909376836, 46.24890960531435979 ) ) ;
#129612=CARTESIAN_POINT ( 'NONE',  ( 13.89961937509957401, 13.97604488694547697, 81.87609039468564731 ) ) ;
#129613=CARTESIAN_POINT ( 'NONE',  ( -12.06949235617756955, 12.14591786802309770, 70.62390960531436690 ) ) ;
#129614=CARTESIAN_POINT ( 'NONE',  ( 10.81492255796106328, -18.62759615963255655, 100.4177570613523471 ) ) ;
#129615=CARTESIAN_POINT ( 'NONE',  ( 21.52544592524344225, -5.823673210054117533, 93.54057627198103830 ) ) ;
#129616=CARTESIAN_POINT ( 'NONE',  ( 21.52544592524334988, 5.823673210054432836, 81.45942372801900433 ) ) ;
#129617=CARTESIAN_POINT ( 'NONE',  ( 10.72451020669871369, 18.67979575497193778, 77.08442372801901854 ) ) ;
#129618=CARTESIAN_POINT ( 'NONE',  ( -5.049401038298153566, 19.05341960407611168, 115.2072429386477097 ) ) ;
#129619=CARTESIAN_POINT ( 'NONE',  ( -8.224510206698735004, -14.34966873604973081, 109.5844237280190328 ) ) ;
#129620=CARTESIAN_POINT ( 'NONE',  ( -18.62759615963255300, -10.81492255796106328, 74.16775706135231871 ) ) ;
#129621=CARTESIAN_POINT ( 'NONE',  ( 19.02544592524343514, -5.153800228976328945, 68.54057627198103830 ) ) ;
#129622=CARTESIAN_POINT ( 'NONE',  ( 21.52544592524334988, 5.823673210054432836, 46.45942372801901854 ) ) ;
#129623=CARTESIAN_POINT ( 'NONE',  ( 5.153800228976335163, 19.02544592524342804, 79.79057627198102409 ) ) ;
#129624=CARTESIAN_POINT ( 'NONE',  ( 16.55341960407611168, 4.379528057220329451, 78.95724293864769550 ) ) ;
#129625=CARTESIAN_POINT ( 'NONE',  ( 4.379528057220339221, -16.55341960407611168, 42.70724293864770260 ) ) ;
#129626=CARTESIAN_POINT ( 'NONE',  ( 10.72451020669898902, -18.67979575497178502, 57.91557627198103120 ) ) ;
#129627=CARTESIAN_POINT ( 'NONE',  ( -16.46253265017160317, 9.564922557960807481, 60.83224293864769550 ) ) ;
#129628=CARTESIAN_POINT ( 'NONE',  ( 21.53943276465977519, -0.05219959533907433946, 68.74890960531435269 ) ) ;
#129629=CARTESIAN_POINT ( 'NONE',  ( -16.51473224551082808, 9.474510206698731452, 68.33442372801900433 ) ) ;
#129630=CARTESIAN_POINT ( 'NONE',  ( -16.46253265017146816, -9.564922557961047289, 29.16775706135232937 ) ) ;
#129631=CARTESIAN_POINT ( 'NONE',  ( 12.14591786802309770, 12.06949235617756955, 74.37390960531436690 ) ) ;
#129632=CARTESIAN_POINT ( 'NONE',  ( 15.80617190586746368, 15.72974639402197994, 49.37390960531436690 ) ) ;
#129634=CARTESIAN_POINT ( 'NONE',  ( 4.483927247898790824, -16.52544592524335698, 95.20942372801903275 ) ) ;
#129636=CARTESIAN_POINT ( 'NONE',  ( -19.03943276465977164, -0.05219959533935918106, 103.7510903946856757 ) ) ;
#129637=CARTESIAN_POINT ( 'NONE',  ( 8.314922557960818139, 14.29746914071049879, 74.58224293864768129 ) ) ;
#129638=CARTESIAN_POINT ( 'NONE',  ( -17.50000000000003197, 4.658240926743115295, 33.94470417816803121 ) ) ;
#129639=CARTESIAN_POINT ( 'NONE',  ( -19.05341960407611168, -5.049401038298163336, 61.45724293864769550 ) ) ;
#129640=CARTESIAN_POINT ( 'NONE',  ( 16.53943276465976808, -0.05219959533910856209, 58.74890960531436690 ) ) ;
#129641=CARTESIAN_POINT ( 'NONE',  ( -19.03943276465977164, 0.05219959533909376836, 91.24890960531436690 ) ) ;
#129642=CARTESIAN_POINT ( 'NONE',  ( 16.51473224551083163, -9.474510206698727899, 75.83442372801900433 ) ) ;
#129643=CARTESIAN_POINT ( 'NONE',  ( 16.51473224551069308, 9.474510206698969483, 59.16557627198102409 ) ) ;
#129644=CARTESIAN_POINT ( 'NONE',  ( -5.153800228976328057, -19.02544592524343514, 82.29057627198103830 ) ) ;
#129645=CARTESIAN_POINT ( 'NONE',  ( 0.05219959533909260263, 19.03943276465977164, 74.99890960531435269 ) ) ;
#129646=CARTESIAN_POINT ( 'NONE',  ( -15.80617190586745835, -15.72974639402198527, 66.87390960531436690 ) ) ;
#129647=CARTESIAN_POINT ( 'NONE',  ( 4.379528057220092307, 16.55341960407617563, 62.29275706135236845 ) ) ;
#129648=CARTESIAN_POINT ( 'NONE',  ( -13.97604488694547520, 13.89961937509957934, 103.1260903946856615 ) ) ;
#129649=CARTESIAN_POINT ( 'NONE',  ( 19.05341960407611168, 5.049401038298154454, 43.95724293864769550 ) ) ;
#129650=CARTESIAN_POINT ( 'NONE',  ( 21.53943276465977519, -0.05219959533907433946, 53.74890960531437401 ) ) ;
#129651=CARTESIAN_POINT ( 'NONE',  ( 19.03943276465977164, 0.05219959533936151252, 86.25109039468567573 ) ) ;
#129652=CARTESIAN_POINT ( 'NONE',  ( -14.34966873604960291, -8.224510206698953496, 31.66557627198102054 ) ) ;
#129653=CARTESIAN_POINT ( 'NONE',  ( -9.474510206698720793, -16.51473224551083518, 39.58442372801899722 ) ) ;
#129654=CARTESIAN_POINT ( 'NONE',  ( -8.314922557961024197, 14.29746914071037800, 62.91775706135236135 ) ) ;
#129655=CARTESIAN_POINT ( 'NONE',  ( -4.483927247898782831, 16.52544592524335698, 97.70942372801904696 ) ) ;
#129656=DIRECTION ( 'NONE',  ( 1.000000000000000000, 0.000000000000000000, 0.000000000000000000 ) ) ;
#129657=CARTESIAN_POINT ( 'NONE',  ( -12.06949235617739369, -12.14591786802326823, 84.37609039468570415 ) ) ;
#129658=CARTESIAN_POINT ( 'NONE',  ( -5.823673210054116645, -21.52544592524344225, 22.29057627198102765 ) ) ;
#129659=CARTESIAN_POINT ( 'NONE',  ( -19.02544592524342804, 5.153800228976336051, 41.04057627198103120 ) ) ;
#129660=CARTESIAN_POINT ( 'NONE',  ( -19.02544592524342804, 5.153800228976336051, 51.04057627198103120 ) ) ;
#129661=CARTESIAN_POINT ( 'NONE',  ( 16.51473224551069308, 9.474510206698969483, 44.16557627198103120 ) ) ;
#129662=CARTESIAN_POINT ( 'NONE',  ( -5.719274019375665041, -21.55341960407619695, 44.79275706135234714 ) ) ;
#129663=CARTESIAN_POINT ( 'NONE',  ( 4.483927247898790824, -16.52544592524335698, 55.20942372801902565 ) ) ;
#129664=CARTESIAN_POINT ( 'NONE',  ( 12.14591786802309770, 12.06949235617756955, 24.37390960531435979 ) ) ;
#129665=CARTESIAN_POINT ( 'NONE',  ( 5.049401038298161559, -19.05341960407611168, 27.70724293864769550 ) ) ;
#129666=CARTESIAN_POINT ( 'NONE',  ( 10.72451020669871369, 18.67979575497193778, 112.0844237280190185 ) ) ;
#129667=CARTESIAN_POINT ( 'NONE',  ( 16.52544592524335698, 4.483927247898782831, 21.45942372801901499 ) ) ;
#129668=CARTESIAN_POINT ( 'NONE',  ( -9.474510206698720793, -16.51473224551083518, 74.58442372801900433 ) ) ;
#129669=CARTESIAN_POINT ( 'NONE',  ( 14.34966873604960469, 8.224510206698951720, 64.16557627198102409 ) ) ;
#129670=CARTESIAN_POINT ( 'NONE',  ( -0.05219959533909027116, -19.03943276465977164, 37.49890960531436690 ) ) ;
#129671=CARTESIAN_POINT ( 'NONE',  ( 5.153800228976615827, -19.02544592524334988, 80.20942372801901854 ) ) ;
#129672=CARTESIAN_POINT ( 'NONE',  ( -10.81492255796105439, 18.62759615963255655, 77.91775706135231871 ) ) ;
#129673=CARTESIAN_POINT ( 'NONE',  ( -0.05219959533934338120, 16.53943276465976808, 37.50109039468568284 ) ) ;
#129675=CARTESIAN_POINT ( 'NONE',  ( -21.55341960407610458, -5.719274019375992779, 41.45724293864769550 ) ) ;
#129676=CARTESIAN_POINT ( 'NONE',  ( -8.224510206698735004, -14.34966873604973081, 29.58442372801901854 ) ) ;
#129677=CARTESIAN_POINT ( 'NONE',  ( 18.09918380851992836, 5.500000000000035527, 88.98618307335613054 ) ) ;
#129678=CARTESIAN_POINT ( 'NONE',  ( -5.823673210054431948, 21.52544592524334988, 112.7094237280190328 ) ) ;
#129680=CARTESIAN_POINT ( 'NONE',  ( 9.564922557960805705, 16.46253265017160317, 34.58224293864770260 ) ) ;
#129682=CARTESIAN_POINT ( 'NONE',  ( -16.51473224551069308, -9.474510206698971260, 56.66557627198103120 ) ) ;
#129683=CARTESIAN_POINT ( 'NONE',  ( 18.62759615963255655, 10.81492255796105972, 61.66775706135235424 ) ) ;
#129685=CARTESIAN_POINT ( 'NONE',  ( 9.474510206698729675, 16.51473224551082808, 22.08442372801899722 ) ) ;
#129686=CARTESIAN_POINT ( 'NONE',  ( -12.06949235617756955, 12.14591786802309770, 30.62390960531436335 ) ) ;
#129687=CARTESIAN_POINT ( 'NONE',  ( -13.89961937509977652, 13.97604488694528158, 25.62390960531434558 ) ) ;
#129688=CARTESIAN_POINT ( 'NONE',  ( 0.05219959533909260263, 19.03943276465977164, 89.99890960531436690 ) ) ;
#129689=CARTESIAN_POINT ( 'NONE',  ( 5.719274019375673035, 21.55341960407619339, 57.29275706135234714 ) ) ;
#129690=CARTESIAN_POINT ( 'NONE',  ( 16.51473224551069308, 9.474510206698969483, 34.16557627198102409 ) ) ;
#129691=CARTESIAN_POINT ( 'NONE',  ( 18.67979575497194134, -10.72451020669871369, 65.83442372801900433 ) ) ;
#129692=CARTESIAN_POINT ( 'NONE',  ( -5.049401038297874678, -19.05341960407617918, 89.79275706135230450 ) ) ;
#129693=CARTESIAN_POINT ( 'NONE',  ( -16.51473224551069308, -9.474510206698971260, 106.6655762719810383 ) ) ;
#129694=CARTESIAN_POINT ( 'NONE',  ( -4.483927247898539470, -16.52544592524342804, 112.2905762719810241 ) ) ;
#129695=CARTESIAN_POINT ( 'NONE',  ( 21.53943276465977519, -0.05219959533907433946, 113.7489096053143527 ) ) ;
#129696=CARTESIAN_POINT ( 'NONE',  ( -13.97604488694547697, 13.89961937509957934, 38.12609039468566152 ) ) ;
#129697=CARTESIAN_POINT ( 'NONE',  ( -4.483927247898539470, -16.52544592524342804, 107.2905762719810525 ) ) ;
#129698=CARTESIAN_POINT ( 'NONE',  ( 16.51473224551069308, 9.474510206698969483, 59.16557627198102409 ) ) ;
#129699=CARTESIAN_POINT ( 'NONE',  ( 19.03943276465977164, 0.05219959533936151252, 96.25109039468567573 ) ) ;
#129700=CARTESIAN_POINT ( 'NONE',  ( 16.52544592524342804, -4.483927247898539470, 63.54057627198103830 ) ) ;
#129701=CARTESIAN_POINT ( 'NONE',  ( -9.564922557961040184, 16.46253265017147172, 32.91775706135233293 ) ) ;
#129702=CARTESIAN_POINT ( 'NONE',  ( -5.719274019375978568, 21.55341960407610458, 25.20724293864769550 ) ) ;
#129703=B_SPLINE_CURVE_WITH_KNOTS ( 'NONE', 3,
 ( #65388, #173584, #19885, #2727, #36041, #94732 ),
 .UNSPECIFIED., .F., .F.,
 ( 4, 2, 4 ),
 ( 0.007228050697041655918, 0.007608510107495138411, 0.007988969517948621771 ),
 .UNSPECIFIED. ) ;
#129704=CARTESIAN_POINT ( 'NONE',  ( -9.474510206698720793, -16.51473224551083518, 89.58442372801900433 ) ) ;
#129705=CARTESIAN_POINT ( 'NONE',  ( -10.72451020669898014, 18.67979575497178502, 85.41557627198102409 ) ) ;
#129706=CARTESIAN_POINT ( 'NONE',  ( -18.62759615963255300, -10.81492255796106328, 39.16775706135235424 ) ) ;
#129707=CARTESIAN_POINT ( 'NONE',  ( 8.224510206698742110, 14.34966873604972548, 37.08442372801901143 ) ) ;
#129708=CARTESIAN_POINT ( 'NONE',  ( -14.34966873604972548, 8.224510206698743886, 38.33442372801900433 ) ) ;
#129709=CARTESIAN_POINT ( 'NONE',  ( 21.52544592524334988, 5.823673210054432836, 51.45942372801901854 ) ) ;
#129710=CARTESIAN_POINT ( 'NONE',  ( -5.719274019375978568, 21.55341960407610458, 60.20724293864768839 ) ) ;
#129711=CARTESIAN_POINT ( 'NONE',  ( 19.02544592524343514, -5.153800228976328945, 33.54057627198102409 ) ) ;
#129713=CARTESIAN_POINT ( 'NONE',  ( 8.224510206698742110, 14.34966873604972548, 82.08442372801901854 ) ) ;
#129714=CARTESIAN_POINT ( 'NONE',  ( 10.72451020669898902, -18.67979575497178502, 92.91557627198103830 ) ) ;
#129715=CARTESIAN_POINT ( 'NONE',  ( -0.05219959533910754901, -16.53943276465976808, 42.49890960531435979 ) ) ;
#129716=CARTESIAN_POINT ( 'NONE',  ( -4.379528057220086978, -16.55341960407618274, 59.79275706135234714 ) ) ;
#129717=CARTESIAN_POINT ( 'NONE',  ( -13.97604488694547697, 13.89961937509957934, 103.1260903946856473 ) ) ;
#129718=CARTESIAN_POINT ( 'NONE',  ( 5.719274019375991003, -21.55341960407610458, 92.70724293864770971 ) ) ;
#129719=CARTESIAN_POINT ( 'NONE',  ( -8.314922557960811034, -14.29746914071050412, 32.08224293864769550 ) ) ;
#129721=CARTESIAN_POINT ( 'NONE',  ( 4.379528057220092307, 16.55341960407617563, 77.29275706135234714 ) ) ;
#129723=CARTESIAN_POINT ( 'NONE',  ( -15.72974639402197994, 15.80617190586746368, 80.62390960531438111 ) ) ;
#129724=CARTESIAN_POINT ( 'NONE',  ( -12.06949235617739369, -12.14591786802326823, 109.3760903946857042 ) ) ;
#129725=ORIENTED_EDGE ( 'NONE', *, *, #47442, .F. ) ;
#129727=CARTESIAN_POINT ( 'NONE',  ( -10.72451020669898014, 18.67979575497178502, 100.4155762719810241 ) ) ;
#129728=CARTESIAN_POINT ( 'NONE',  ( -21.52544592524343514, 5.823673210054127303, 106.0405762719810525 ) ) ;
#129729=CARTESIAN_POINT ( 'NONE',  ( 14.34966873604960469, 8.224510206698951720, 34.16557627198102409 ) ) ;
#129730=CARTESIAN_POINT ( 'NONE',  ( 14.29746914071037800, 8.314922557961029526, 41.66775706135235424 ) ) ;
#129731=CARTESIAN_POINT ( 'NONE',  ( -0.05219959533909027116, -19.03943276465977164, 42.49890960531435269 ) ) ;
#129732=CARTESIAN_POINT ( 'NONE',  ( -13.97604488694527625, -13.89961937509977652, 61.87390960531435979 ) ) ;
#129733=CARTESIAN_POINT ( 'NONE',  ( -18.67979575497178146, -10.72451020669898902, 21.66557627198102409 ) ) ;
#129734=CARTESIAN_POINT ( 'NONE',  ( -5.153800228976328057, -19.02544592524343514, 112.2905762719810099 ) ) ;
#129735=CARTESIAN_POINT ( 'NONE',  ( -16.51473224551082808, 9.474510206698731452, 108.3344237280190043 ) ) ;
#129736=CARTESIAN_POINT ( 'NONE',  ( 19.02544592524334988, 5.153800228976608722, 51.45942372801900433 ) ) ;
#129737=CARTESIAN_POINT ( 'NONE',  ( 5.719274019375991003, -21.55341960407610458, 82.70724293864770971 ) ) ;
#129738=CARTESIAN_POINT ( 'NONE',  ( -16.55341960407611168, -4.379528057220339221, 21.45724293864769550 ) ) ;
#129739=VECTOR ( 'NONE', #9293, 1000.000000000000000 ) ;
#129740=CARTESIAN_POINT ( 'NONE',  ( 15.80617190586746368, 15.72974639402197994, 44.37390960531435979 ) ) ;
#129741=CARTESIAN_POINT ( 'NONE',  ( -18.67979575497178146, -10.72451020669898902, 86.66557627198102409 ) ) ;
#129742=CARTESIAN_POINT ( 'NONE',  ( 13.97604488694548053, -13.89961937509957401, 110.6260903946856615 ) ) ;
#129743=CARTESIAN_POINT ( 'NONE',  ( -10.72451020669898014, 18.67979575497178502, 25.41557627198103120 ) ) ;
#129744=CARTESIAN_POINT ( 'NONE',  ( 18.62759615963255655, 10.81492255796105972, 71.66775706135234714 ) ) ;
#129745=CARTESIAN_POINT ( 'NONE',  ( -13.97604488694527625, -13.89961937509977652, 71.87390960531433848 ) ) ;
#129747=CARTESIAN_POINT ( 'NONE',  ( -9.474510206698964154, 16.51473224551069663, 75.41557627198103830 ) ) ;
#129748=CARTESIAN_POINT ( 'NONE',  ( -12.06949235617756955, 12.14591786802309770, 85.62390960531436690 ) ) ;
#129750=CARTESIAN_POINT ( 'NONE',  ( 9.564922557961047289, -16.46253265017146816, 105.4177570613523471 ) ) ;
#129751=CARTESIAN_POINT ( 'NONE',  ( 17.31728774477273447, -6.344390552232386682, 83.31906651689317300 ) ) ;
#129752=CARTESIAN_POINT ( 'NONE',  ( 16.46253265017160672, -9.564922557960803928, 73.33224293864769550 ) ) ;
#129753=CARTESIAN_POINT ( 'NONE',  ( 21.55341960407619695, -5.719274019375665929, 86.04275706135236135 ) ) ;
#129754=CARTESIAN_POINT ( 'NONE',  ( 19.03943276465977164, -0.05219959533909143690, 103.7489096053143669 ) ) ;
#129755=CARTESIAN_POINT ( 'NONE',  ( -12.14591786802326823, 12.06949235617739902, 73.12609039468567573 ) ) ;
#129757=CARTESIAN_POINT ( 'NONE',  ( 16.46253265017146816, 9.564922557961045513, 61.66775706135234003 ) ) ;
#129758=CARTESIAN_POINT ( 'NONE',  ( 9.474510206698729675, 16.51473224551082808, 22.08442372801899722 ) ) ;
#129760=FACE_OUTER_BOUND ( 'NONE', #10445, .T. ) ;
#129762=CARTESIAN_POINT ( 'NONE',  ( 14.34966873604960469, 8.224510206698951720, 29.16557627198103120 ) ) ;
#129764=CARTESIAN_POINT ( 'NONE',  ( -8.314922557961024197, 14.29746914071037800, 112.9177570613523329 ) ) ;
#129765=CARTESIAN_POINT ( 'NONE',  ( 16.20579543436677739, 7.371946100355112996, 68.06520834171880097 ) ) ;
#129766=CARTESIAN_POINT ( 'NONE',  ( -16.53943276465976808, -0.05219959533934237506, 78.75109039468568994 ) ) ;
#129767=CARTESIAN_POINT ( 'NONE',  ( 5.823673210054444382, -21.52544592524334988, 85.20942372801901854 ) ) ;
#129768=CARTESIAN_POINT ( 'NONE',  ( 16.46253265017146816, 9.564922557961045513, 91.66775706135234714 ) ) ;
#129769=CARTESIAN_POINT ( 'NONE',  ( 19.02544592524334988, 5.153800228976608722, 46.45942372801899012 ) ) ;
#129770=CARTESIAN_POINT ( 'NONE',  ( 19.03943276465977164, -0.05219959533909143690, 73.74890960531435269 ) ) ;
#129771=CARTESIAN_POINT ( 'NONE',  ( -0.05219959533909027116, -19.03943276465977164, 52.49890960531436690 ) ) ;
#129772=CARTESIAN_POINT ( 'NONE',  ( 17.60769864724390388, -5.499999999999978684, 41.15024842019165874 ) ) ;
#129773=CARTESIAN_POINT ( 'NONE',  ( 10.81492255796078972, 18.62759615963270932, 89.58224293864768129 ) ) ;
#129774=CARTESIAN_POINT ( 'NONE',  ( -5.719274019375978568, 21.55341960407610458, 45.20724293864769550 ) ) ;
#129775=CARTESIAN_POINT ( 'NONE',  ( -16.51473224551069308, -9.474510206698971260, 51.66557627198102409 ) ) ;
#129776=CARTESIAN_POINT ( 'NONE',  ( -8.314922557961024197, 14.29746914071037800, 67.91775706135234714 ) ) ;
#129778=CARTESIAN_POINT ( 'NONE',  ( 21.53943276465977519, 0.05219959533937863772, 46.25109039468567573 ) ) ;
#129779=CARTESIAN_POINT ( 'NONE',  ( 16.55341960407611168, 4.379528057220329451, 63.95724293864770260 ) ) ;
#129781=CARTESIAN_POINT ( 'NONE',  ( -8.224510206698735004, -14.34966873604973081, 39.58442372801901143 ) ) ;
#129782=CARTESIAN_POINT ( 'NONE',  ( 4.379528057220339221, -16.55341960407611168, 107.7072429386476955 ) ) ;
#129783=CARTESIAN_POINT ( 'NONE',  ( 19.03943276465977164, 0.05219959533936151252, 56.25109039468566863 ) ) ;
#129784=CARTESIAN_POINT ( 'NONE',  ( 8.224510206698953496, -14.34966873604960469, 67.91557627198102409 ) ) ;
#129785=CARTESIAN_POINT ( 'NONE',  ( -10.72451020669870658, -18.67979575497194134, 29.58442372801901854 ) ) ;
#129786=CARTESIAN_POINT ( 'NONE',  ( 16.46253265017160672, -9.564922557960803928, 28.33224293864769550 ) ) ;
#129787=CARTESIAN_POINT ( 'NONE',  ( -21.53943276465977519, 0.05219959533907696930, 86.24890960531436690 ) ) ;
#129788=CARTESIAN_POINT ( 'NONE',  ( 19.03943276465977164, -0.05219959533909143690, 103.7489096053143669 ) ) ;
#129789=CARTESIAN_POINT ( 'NONE',  ( -12.14591786802309592, -12.06949235617757132, 76.87390960531439532 ) ) ;
#129790=CARTESIAN_POINT ( 'NONE',  ( 13.89961937509977652, -13.97604488694527269, 113.1239096053143527 ) ) ;
#129792=CARTESIAN_POINT ( 'NONE',  ( 9.564922557961047289, -16.46253265017146816, 80.41775706135234714 ) ) ;
#129793=CARTESIAN_POINT ( 'NONE',  ( 5.719274019375673035, 21.55341960407619339, 27.29275706135234358 ) ) ;
#129794=CARTESIAN_POINT ( 'NONE',  ( -5.049401038298153566, 19.05341960407611168, 65.20724293864765286 ) ) ;
#129795=CARTESIAN_POINT ( 'NONE',  ( -5.153800228976607833, 19.02544592524334988, 52.70942372801900433 ) ) ;
#129796=CARTESIAN_POINT ( 'NONE',  ( -9.474510206698964154, 16.51473224551069663, 30.41557627198102054 ) ) ;
#129797=CARTESIAN_POINT ( 'NONE',  ( 18.67979575497194134, -10.72451020669871369, 75.83442372801900433 ) ) ;
#129798=CARTESIAN_POINT ( 'NONE',  ( 4.483927247898545687, 16.52544592524342804, 64.79057627198103830 ) ) ;
#129799=CARTESIAN_POINT ( 'NONE',  ( -16.53943276465976808, 0.05219959533911058130, 56.24890960531436690 ) ) ;
#129800=CARTESIAN_POINT ( 'NONE',  ( 16.51473224551069308, 9.474510206698969483, 59.16557627198102409 ) ) ;
#129801=CARTESIAN_POINT ( 'NONE',  ( 10.81492255796078972, 18.62759615963270932, 89.58224293864768129 ) ) ;
#129802=CARTESIAN_POINT ( 'NONE',  ( 5.153800228976335163, 19.02544592524342804, 59.79057627198100988 ) ) ;
#129803=VERTEX_POINT ( 'NONE', #5306 ) ;
#129804=CARTESIAN_POINT ( 'NONE',  ( -15.72974639402197994, 15.80617190586746368, 75.62390960531439532 ) ) ;
#129805=CARTESIAN_POINT ( 'NONE',  ( 10.81492255796106328, -18.62759615963255655, 105.4177570613523613 ) ) ;
#129806=CARTESIAN_POINT ( 'NONE',  ( 13.97604488694527802, 13.89961937509977652, 29.37390960531435979 ) ) ;
#129807=CARTESIAN_POINT ( 'NONE',  ( 16.53943276465976808, 0.05219959533934440121, 106.2510903946856757 ) ) ;
#129808=CARTESIAN_POINT ( 'NONE',  ( -12.14591786802309592, -12.06949235617757132, 91.87390960531436690 ) ) ;
#129809=CARTESIAN_POINT ( 'NONE',  ( 19.03943276465977164, 0.05219959533936151252, 96.25109039468567573 ) ) ;
#129811=CARTESIAN_POINT ( 'NONE',  ( 21.55341960407610458, 5.719274019375980345, 113.9572429386477239 ) ) ;
#129812=CARTESIAN_POINT ( 'NONE',  ( -19.02544592524334988, -5.153800228976617603, 58.95942372801900433 ) ) ;
#129813=CARTESIAN_POINT ( 'NONE',  ( -0.05219959533934338120, 16.53943276465976808, 102.5010903946856899 ) ) ;
#129814=CARTESIAN_POINT ( 'NONE',  ( -19.02544592524334988, -5.153800228976617603, 33.95942372801897591 ) ) ;
#129815=CARTESIAN_POINT ( 'NONE',  ( -9.564922557960796823, -16.46253265017161027, 107.0822429386476955 ) ) ;
#129816=CARTESIAN_POINT ( 'NONE',  ( 18.62759615963271287, -10.81492255796078972, 63.33224293864770260 ) ) ;
#129818=CARTESIAN_POINT ( 'NONE',  ( -19.02544592524342804, 5.153800228976336051, 31.04057627198102409 ) ) ;
#129819=CARTESIAN_POINT ( 'NONE',  ( -0.05219959533937732626, 21.53943276465977519, 102.5010903946856899 ) ) ;
#129820=CARTESIAN_POINT ( 'NONE',  ( 12.06949235617739724, 12.14591786802326823, 76.87609039468567573 ) ) ;
#129821=CARTESIAN_POINT ( 'NONE',  ( -10.72451020669870658, -18.67979575497194134, 24.58442372801901499 ) ) ;
#129822=CARTESIAN_POINT ( 'NONE',  ( -12.06949235617739369, -12.14591786802326823, 39.37609039468567573 ) ) ;
#129823=CARTESIAN_POINT ( 'NONE',  ( 19.05341960407611168, 5.049401038298154454, 108.9572429386477097 ) ) ;
#129824=CARTESIAN_POINT ( 'NONE',  ( -13.89961937509977652, 13.97604488694528158, 50.62390960531435979 ) ) ;
#129825=CARTESIAN_POINT ( 'NONE',  ( 5.049401038298161559, -19.05341960407611168, 67.70724293864769550 ) ) ;
#129826=CARTESIAN_POINT ( 'NONE',  ( -12.14591786802326823, 12.06949235617739902, 53.12609039468568284 ) ) ;
#129827=CARTESIAN_POINT ( 'NONE',  ( -14.34966873604960291, -8.224510206698953496, 91.66557627198103830 ) ) ;
#129828=CARTESIAN_POINT ( 'NONE',  ( -14.29746914071037622, -8.314922557961029526, 104.1677570613523471 ) ) ;
#129829=CARTESIAN_POINT ( 'NONE',  ( -18.22780087662122028, 5.500000000000031086, 58.51540105326107977 ) ) ;
#129830=CARTESIAN_POINT ( 'NONE',  ( -18.67979575497193778, 10.72451020669871902, 53.33442372801901854 ) ) ;
#129831=CARTESIAN_POINT ( 'NONE',  ( 5.153800228976335163, 19.02544592524342804, 84.79057627198099567 ) ) ;
#129832=CARTESIAN_POINT ( 'NONE',  ( 13.97604488694527802, 13.89961937509977652, 64.37390960531436690 ) ) ;
#129833=CARTESIAN_POINT ( 'NONE',  ( -19.03943276465977164, 0.05219959533909376836, 91.24890960531436690 ) ) ;
#129834=CARTESIAN_POINT ( 'NONE',  ( -8.314922557960811034, -14.29746914071050412, 42.08224293864769550 ) ) ;
#129835=CARTESIAN_POINT ( 'NONE',  ( 0.05219959533934541429, -16.53943276465976808, 95.00109039468568994 ) ) ;
#129836=CARTESIAN_POINT ( 'NONE',  ( -16.52544592524342804, 4.483927247898546575, 41.04057627198103120 ) ) ;
#129838=CARTESIAN_POINT ( 'NONE',  ( 16.51473224551083163, -9.474510206698727899, 50.83442372801899722 ) ) ;
#129839=CARTESIAN_POINT ( 'NONE',  ( -0.05219959533909027116, -19.03943276465977164, 107.4989096053143527 ) ) ;
#129840=CARTESIAN_POINT ( 'NONE',  ( 19.02544592524343514, -5.153800228976328945, 58.54057627198102409 ) ) ;
#129841=CARTESIAN_POINT ( 'NONE',  ( 13.89961937509957401, 13.97604488694547697, 41.87609039468566152 ) ) ;
#129843=CARTESIAN_POINT ( 'NONE',  ( 17.49999999999999645, 5.500000000000009770, 58.78230962303567253 ) ) ;
#129844=CARTESIAN_POINT ( 'NONE',  ( -19.02544592524334988, -5.153800228976617603, 88.95942372801897591 ) ) ;
#129845=CARTESIAN_POINT ( 'NONE',  ( 14.34966873604972726, -8.224510206698740333, 75.83442372801900433 ) ) ;
#129846=CARTESIAN_POINT ( 'NONE',  ( 16.19135201231366139, 7.376712067591940425, 92.68680854052028906 ) ) ;
#129847=CARTESIAN_POINT ( 'NONE',  ( 9.564922557960805705, 16.46253265017160317, 94.58224293864769550 ) ) ;
#129848=CARTESIAN_POINT ( 'NONE',  ( 18.67979575497194134, -10.72451020669871369, 30.83442372801902209 ) ) ;
#129849=CARTESIAN_POINT ( 'NONE',  ( 13.89961937509957401, 13.97604488694547697, 76.87609039468566152 ) ) ;
#129850=CARTESIAN_POINT ( 'NONE',  ( 0.05219959533909260263, 19.03943276465977164, 114.9989096053143669 ) ) ;
#129851=CARTESIAN_POINT ( 'NONE',  ( 9.474510206698971260, -16.51473224551069308, 52.91557627198102409 ) ) ;
#129853=CARTESIAN_POINT ( 'NONE',  ( -5.049401038298153566, 19.05341960407611168, 95.20724293864770971 ) ) ;
#129854=CARTESIAN_POINT ( 'NONE',  ( 4.379528057220339221, -16.55341960407611168, 52.70724293864769550 ) ) ;
#129855=CARTESIAN_POINT ( 'NONE',  ( 0.05219959533909260263, 19.03943276465977164, 39.99890960531436690 ) ) ;
#129856=CARTESIAN_POINT ( 'NONE',  ( 19.05341960407617918, -5.049401038297876454, 56.04275706135234714 ) ) ;
#129857=CARTESIAN_POINT ( 'NONE',  ( 14.34966873604960469, 8.224510206698951720, 84.16557627198103830 ) ) ;
#129858=CARTESIAN_POINT ( 'NONE',  ( 16.46253265017146816, 9.564922557961045513, 36.66775706135233293 ) ) ;
#129859=CARTESIAN_POINT ( 'NONE',  ( 5.049401038298161559, -19.05341960407611168, 72.70724293864768129 ) ) ;
#129860=CARTESIAN_POINT ( 'NONE',  ( 21.53943276465977519, -0.05219959533907433946, 68.74890960531435269 ) ) ;
#129861=CARTESIAN_POINT ( 'NONE',  ( -12.14591786802309592, -12.06949235617757132, 51.87390960531437401 ) ) ;
#129862=CARTESIAN_POINT ( 'NONE',  ( 9.474510206698729675, 16.51473224551082808, 27.08442372801900433 ) ) ;
#129863=CARTESIAN_POINT ( 'NONE',  ( -16.51473224551069308, -9.474510206698971260, 106.6655762719810383 ) ) ;
#129864=CARTESIAN_POINT ( 'NONE',  ( -21.53943276465977519, 0.05219959533907696930, 31.24890960531435979 ) ) ;
#129865=CARTESIAN_POINT ( 'NONE',  ( -19.05341960407611168, -5.049401038298163336, 46.45724293864768129 ) ) ;
#129866=CARTESIAN_POINT ( 'NONE',  ( -13.97604488694527625, -13.89961937509977652, 41.87390960531435979 ) ) ;
#129867=CARTESIAN_POINT ( 'NONE',  ( 16.53943276465976808, -0.05219959533910856209, 98.74890960531438111 ) ) ;
#129868=CARTESIAN_POINT ( 'NONE',  ( 18.62759615963271287, -10.81492255796078972, 108.3322429386477097 ) ) ;
#129869=CARTESIAN_POINT ( 'NONE',  ( -9.474510206698964154, 16.51473224551069663, 105.4155762719810383 ) ) ;
#129870=CARTESIAN_POINT ( 'NONE',  ( 10.72451020669898902, -18.67979575497178502, 107.9155762719810241 ) ) ;
#129871=CARTESIAN_POINT ( 'NONE',  ( 19.03943276465977164, -0.05219959533909143690, 98.74890960531436690 ) ) ;
#129872=CARTESIAN_POINT ( 'NONE',  ( 4.379528057220339221, -16.55341960407611168, 112.7072429386476955 ) ) ;
#129873=CARTESIAN_POINT ( 'NONE',  ( 15.80617190586769283, -15.72974639402175789, 80.62609039468567573 ) ) ;
#129874=CARTESIAN_POINT ( 'NONE',  ( -5.719274019375978568, 21.55341960407610458, 90.20724293864770971 ) ) ;
#129875=CARTESIAN_POINT ( 'NONE',  ( 16.61371651742600974, -7.165104196376164580, 106.3541506999299742 ) ) ;
#129877=CARTESIAN_POINT ( 'NONE',  ( 13.97604488694527802, 13.89961937509977830, 59.37390960531435979 ) ) ;
#129878=CARTESIAN_POINT ( 'NONE',  ( -12.14591786802326823, 12.06949235617739902, 43.12609039468568284 ) ) ;
#129879=CARTESIAN_POINT ( 'NONE',  ( -4.379528057220328563, 16.55341960407611168, 105.2072429386477097 ) ) ;
#129881=CARTESIAN_POINT ( 'NONE',  ( -16.46253265017160317, 9.564922557960807481, 60.83224293864769550 ) ) ;
#129882=CARTESIAN_POINT ( 'NONE',  ( 8.314922557960818139, 14.29746914071049879, 99.58224293864770971 ) ) ;
#129883=CARTESIAN_POINT ( 'NONE',  ( -10.72451020669898014, 18.67979575497178502, 30.41557627198101699 ) ) ;
#129884=CARTESIAN_POINT ( 'NONE',  ( -16.53943276465976808, 0.05219959533911058130, 71.24890960531435269 ) ) ;
#129885=CARTESIAN_POINT ( 'NONE',  ( -19.05341960407617563, 5.049401038297882671, 113.5427570613523471 ) ) ;
#129886=CARTESIAN_POINT ( 'NONE',  ( -18.62759615963255300, -10.81492255796106328, 79.16775706135234714 ) ) ;
#129887=CARTESIAN_POINT ( 'NONE',  ( 16.36317988757058117, -7.306389748694916975, 76.59789608363225000 ) ) ;
#129888=CARTESIAN_POINT ( 'NONE',  ( 0.05219959533934541429, -16.53943276465976808, 100.0010903946857042 ) ) ;
#129889=CARTESIAN_POINT ( 'NONE',  ( -14.34966873604960291, -8.224510206698953496, 46.66557627198102409 ) ) ;
#129890=CARTESIAN_POINT ( 'NONE',  ( -0.05219959533909027116, -19.03943276465977164, 37.49890960531436690 ) ) ;
#129891=CARTESIAN_POINT ( 'NONE',  ( -9.564922557960796823, -16.46253265017161027, 92.08224293864769550 ) ) ;
#129892=CARTESIAN_POINT ( 'NONE',  ( 10.72451020669898902, -18.67979575497178502, 97.91557627198103830 ) ) ;
#129893=CARTESIAN_POINT ( 'NONE',  ( 16.55341960407618274, -4.379528057220086978, 21.04275706135234714 ) ) ;
#129894=CARTESIAN_POINT ( 'NONE',  ( -12.06949235617756955, 12.14591786802309770, 65.62390960531436690 ) ) ;
#129895=CARTESIAN_POINT ( 'NONE',  ( -10.72451020669870658, -18.67979575497194134, 69.58442372801900433 ) ) ;
#129896=CARTESIAN_POINT ( 'NONE',  ( 16.52544592524335698, 4.483927247898782831, 106.4594237280190328 ) ) ;
#129897=CARTESIAN_POINT ( 'NONE',  ( 17.13100169013300444, 6.664070546373170423, 26.73210164300153835 ) ) ;
#129899=CARTESIAN_POINT ( 'NONE',  ( -16.55341960407611168, -4.379528057220339221, 31.45724293864769550 ) ) ;
#129900=CARTESIAN_POINT ( 'NONE',  ( 16.52544592524335698, 4.483927247898782831, 71.45942372801901854 ) ) ;
#129901=CARTESIAN_POINT ( 'NONE',  ( -5.049401038298153566, 19.05341960407611168, 85.20724293864766707 ) ) ;
#129902=CARTESIAN_POINT ( 'NONE',  ( 16.51473224551069308, 9.474510206698969483, 104.1655762719810241 ) ) ;
#129903=CARTESIAN_POINT ( 'NONE',  ( -5.823673210054431948, 21.52544592524334988, 82.70942372801900433 ) ) ;
#129904=CARTESIAN_POINT ( 'NONE',  ( -4.483927247898782831, 16.52544592524335698, 92.70942372801901854 ) ) ;
#129905=CARTESIAN_POINT ( 'NONE',  ( -12.06949235617756955, 12.14591786802309770, 65.62390960531436690 ) ) ;
#129906=CARTESIAN_POINT ( 'NONE',  ( -13.97604488694527625, -13.89961937509977652, 66.87390960531436690 ) ) ;
#129907=VERTEX_POINT ( 'NONE', #6306 ) ;
#129908=CARTESIAN_POINT ( 'NONE',  ( 16.51473224551083163, -9.474510206698727899, 105.8344237280190043 ) ) ;
#129909=CARTESIAN_POINT ( 'NONE',  ( 14.34966873604960469, 8.224510206698951720, 104.1655762719810241 ) ) ;
#129910=CARTESIAN_POINT ( 'NONE',  ( 16.46253265017160672, -9.564922557960803928, 73.33224293864769550 ) ) ;
#129911=CARTESIAN_POINT ( 'NONE',  ( 19.05341960407617918, -5.049401038297876454, 111.0427570613523329 ) ) ;
#129913=CARTESIAN_POINT ( 'NONE',  ( 21.53943276465977519, 0.05219959533937863772, 111.2510903946856899 ) ) ;
#129914=CARTESIAN_POINT ( 'NONE',  ( -4.379528057220086978, -16.55341960407618274, 74.79275706135234714 ) ) ;
#129915=CARTESIAN_POINT ( 'NONE',  ( -16.46253265017146816, -9.564922557961047289, 99.16775706135233293 ) ) ;
#129916=CARTESIAN_POINT ( 'NONE',  ( 16.52544592524342804, -4.483927247898539470, 108.5405762719810241 ) ) ;
#129917=CARTESIAN_POINT ( 'NONE',  ( -12.14591786802326823, 12.06949235617739902, 63.12609039468568994 ) ) ;
#129918=CARTESIAN_POINT ( 'NONE',  ( 0.05219959533934541429, -16.53943276465976808, 60.00109039468568284 ) ) ;
#129919=CARTESIAN_POINT ( 'NONE',  ( 5.049401038298161559, -19.05341960407611168, 22.70724293864769194 ) ) ;
#129920=CARTESIAN_POINT ( 'NONE',  ( 19.05341960407617918, -5.049401038297876454, 51.04275706135231871 ) ) ;
#129921=CARTESIAN_POINT ( 'NONE',  ( 21.52544592524334988, 5.823673210054432836, 96.45942372801901854 ) ) ;
#129922=CARTESIAN_POINT ( 'NONE',  ( 13.97604488694527802, 13.89961937509977652, 29.37390960531435979 ) ) ;
#129923=CARTESIAN_POINT ( 'NONE',  ( -9.564922557960796823, -16.46253265017161027, 72.08224293864770971 ) ) ;
#129924=CARTESIAN_POINT ( 'NONE',  ( 16.55341960407611168, 4.379528057220329451, 68.95724293864769550 ) ) ;
#129925=CARTESIAN_POINT ( 'NONE',  ( -21.52544592524334988, -5.823673210054445271, 88.95942372801901854 ) ) ;
#129927=CARTESIAN_POINT ( 'NONE',  ( 5.153800228976615827, -19.02544592524334988, 65.20942372801900433 ) ) ;
#129928=CARTESIAN_POINT ( 'NONE',  ( -0.05219959533936034679, 19.03943276465977164, 42.50109039468566152 ) ) ;
#129929=CARTESIAN_POINT ( 'NONE',  ( 21.52544592524344225, -5.823673210054117533, 43.54057627198103830 ) ) ;
#129930=CARTESIAN_POINT ( 'NONE',  ( -5.719274019375665041, -21.55341960407619695, 104.7927570613523898 ) ) ;
#129931=CARTESIAN_POINT ( 'NONE',  ( -19.05341960407611168, -5.049401038298163336, 71.45724293864766707 ) ) ;
#129932=CARTESIAN_POINT ( 'NONE',  ( 10.81492255796106328, -18.62759615963255655, 100.4177570613523471 ) ) ;
#129933=CARTESIAN_POINT ( 'NONE',  ( 5.823673210054125526, 21.52544592524343514, 44.79057627198103120 ) ) ;
#129934=CARTESIAN_POINT ( 'NONE',  ( 0.05219959533909260263, 19.03943276465977164, 99.99890960531436690 ) ) ;
#129935=CARTESIAN_POINT ( 'NONE',  ( -13.89961937509957401, -13.97604488694547875, 79.37609039468567573 ) ) ;
#129936=CARTESIAN_POINT ( 'NONE',  ( 5.153800228976335163, 19.02544592524342804, 104.7905762719809957 ) ) ;
#129937=CARTESIAN_POINT ( 'NONE',  ( 19.02544592524334988, 5.153800228976608722, 91.45942372801900433 ) ) ;
#129938=CARTESIAN_POINT ( 'NONE',  ( 14.34966873604972726, -8.224510206698740333, 40.83442372801901854 ) ) ;
#129939=CARTESIAN_POINT ( 'NONE',  ( 0.05219959533910956823, 16.53943276465976808, 104.9989096053143669 ) ) ;
#129940=CARTESIAN_POINT ( 'NONE',  ( -19.02544592524342804, 5.153800228976336051, 86.04057627198103830 ) ) ;
#129941=CARTESIAN_POINT ( 'NONE',  ( -15.72974639402197994, 15.80617190586746368, 65.62390960531436690 ) ) ;
#129942=CARTESIAN_POINT ( 'NONE',  ( -0.05219959533934338120, 16.53943276465976808, 27.50109039468567929 ) ) ;
#129943=CARTESIAN_POINT ( 'NONE',  ( -0.05219959533937732626, 21.53943276465977519, 27.50109039468567929 ) ) ;
#129944=CARTESIAN_POINT ( 'NONE',  ( 21.53943276465977519, 0.05219959533937863772, 81.25109039468568994 ) ) ;
#129945=CARTESIAN_POINT ( 'NONE',  ( 12.14591786802327356, -12.06949235617739191, 85.62609039468568994 ) ) ;
#129946=CARTESIAN_POINT ( 'NONE',  ( 19.05341960407611168, 5.049401038298154454, 73.95724293864768129 ) ) ;
#129947=CARTESIAN_POINT ( 'NONE',  ( 12.06949235617757843, -12.14591786802309237, 78.12390960531436690 ) ) ;
#129948=CARTESIAN_POINT ( 'NONE',  ( 12.06949235617757843, -12.14591786802309237, 28.12390960531435979 ) ) ;
#129949=CARTESIAN_POINT ( 'NONE',  ( 19.02544592524334988, 5.153800228976608722, 56.45942372801898301 ) ) ;
#129950=CARTESIAN_POINT ( 'NONE',  ( 18.67979575497194134, -10.72451020669871369, 50.83442372801901143 ) ) ;
#129951=CARTESIAN_POINT ( 'NONE',  ( 8.224510206698953496, -14.34966873604960469, 77.91557627198102409 ) ) ;
#129952=CARTESIAN_POINT ( 'NONE',  ( 13.89961937509977652, -13.97604488694527269, 108.1239096053143669 ) ) ;
#129953=CARTESIAN_POINT ( 'NONE',  ( 16.55341960407618274, -4.379528057220086978, 96.04275706135236135 ) ) ;
#129954=CARTESIAN_POINT ( 'NONE',  ( 21.52544592524334988, 5.823673210054432836, 91.45942372801901854 ) ) ;
#129955=CARTESIAN_POINT ( 'NONE',  ( 16.53943276465976808, 0.05219959533934440121, 46.25109039468567573 ) ) ;
#129956=CARTESIAN_POINT ( 'NONE',  ( 18.67979575497194134, -10.72451020669871369, 40.83442372801901854 ) ) ;
#129958=CARTESIAN_POINT ( 'NONE',  ( 21.55341960407610458, 5.719274019375980345, 108.9572429386476955 ) ) ;
#129959=CARTESIAN_POINT ( 'NONE',  ( -16.55341960407611168, -4.379528057220339221, 86.45724293864770971 ) ) ;
#129960=CARTESIAN_POINT ( 'NONE',  ( 17.50000000000000000, -5.068104630630397622, 28.22818405340030168 ) ) ;
#129961=CARTESIAN_POINT ( 'NONE',  ( -0.05219959533910754901, -16.53943276465976808, 57.49890960531435979 ) ) ;
#129962=CARTESIAN_POINT ( 'NONE',  ( -12.14591786802326823, 12.06949235617739902, 93.12609039468568994 ) ) ;
#129963=CARTESIAN_POINT ( 'NONE',  ( 13.97604488694527802, 13.89961937509977652, 44.37390960531435269 ) ) ;
#129964=CARTESIAN_POINT ( 'NONE',  ( -10.72451020669898014, 18.67979575497178502, 40.41557627198103120 ) ) ;
#129965=CARTESIAN_POINT ( 'NONE',  ( -16.55341960407611168, -4.379528057220339221, 76.45724293864769550 ) ) ;
#129966=CARTESIAN_POINT ( 'NONE',  ( -21.55341960407610458, -5.719274019375992779, 76.45724293864769550 ) ) ;
#129967=CARTESIAN_POINT ( 'NONE',  ( -16.46253265017160317, 9.564922557960807481, 85.83224293864769550 ) ) ;
#129968=CARTESIAN_POINT ( 'NONE',  ( -5.049401038298153566, 19.05341960407611168, 40.20724293864768839 ) ) ;
#129969=CARTESIAN_POINT ( 'NONE',  ( 13.89961937509957401, 13.97604488694547697, 91.87609039468567573 ) ) ;
#129970=CARTESIAN_POINT ( 'NONE',  ( -21.55341960407610458, -5.719274019375992779, 26.45724293864768839 ) ) ;
#129971=CARTESIAN_POINT ( 'NONE',  ( 18.62759615963255655, 10.81492255796105972, 51.66775706135234714 ) ) ;
#129972=CARTESIAN_POINT ( 'NONE',  ( 9.474510206698971260, -16.51473224551069308, 47.91557627198102409 ) ) ;
#129973=CARTESIAN_POINT ( 'NONE',  ( 9.564922557960805705, 16.46253265017160317, 84.58224293864769550 ) ) ;
#129974=VERTEX_POINT ( 'NONE', #190344 ) ;
#129975=CARTESIAN_POINT ( 'NONE',  ( 14.34966873604972726, -8.224510206698740333, 50.83442372801901143 ) ) ;
#129976=CARTESIAN_POINT ( 'NONE',  ( 10.81492255796106328, -18.62759615963255655, 25.41775706135235779 ) ) ;
#129977=CARTESIAN_POINT ( 'NONE',  ( -10.81492255796105439, 18.62759615963255655, 72.91775706135234714 ) ) ;
#129978=CARTESIAN_POINT ( 'NONE',  ( -18.62759615963270932, 10.81492255796079327, 25.83224293864769194 ) ) ;
#129979=CARTESIAN_POINT ( 'NONE',  ( -21.55341960407610458, -5.719274019375992779, 86.45724293864770971 ) ) ;
#129980=CARTESIAN_POINT ( 'NONE',  ( -21.52544592524343514, 5.823673210054127303, 116.0405762719810383 ) ) ;
#129981=CARTESIAN_POINT ( 'NONE',  ( 14.34966873604972726, -8.224510206698740333, 70.83442372801901854 ) ) ;
#129982=CARTESIAN_POINT ( 'NONE',  ( -10.81492255796078084, -18.62759615963271287, 57.08224293864769550 ) ) ;
#129983=CARTESIAN_POINT ( 'NONE',  ( 10.72451020669871369, 18.67979575497193778, 112.0844237280190185 ) ) ;
#129984=CARTESIAN_POINT ( 'NONE',  ( -19.05341960407611168, -5.049401038298163336, 71.45724293864766707 ) ) ;
#129985=CARTESIAN_POINT ( 'NONE',  ( 16.51473224551069308, 9.474510206698969483, 114.1655762719810241 ) ) ;
#129986=CARTESIAN_POINT ( 'NONE',  ( -16.46253265017160317, 9.564922557960807481, 85.83224293864769550 ) ) ;
#129988=CARTESIAN_POINT ( 'NONE',  ( -9.474510206698720793, -16.51473224551083518, 69.58442372801901854 ) ) ;
#129989=CARTESIAN_POINT ( 'NONE',  ( -15.80617190586745835, -15.72974639402198527, 41.87390960531435979 ) ) ;
#129990=CARTESIAN_POINT ( 'NONE',  ( 8.314922557960818139, 14.29746914071049879, 24.58224293864768839 ) ) ;
#129991=CARTESIAN_POINT ( 'NONE',  ( -13.97604488694547697, 13.89961937509957934, 103.1260903946856473 ) ) ;
#129993=CARTESIAN_POINT ( 'NONE',  ( 21.52544592524334988, 5.823673210054432836, 111.4594237280190328 ) ) ;
#129994=CARTESIAN_POINT ( 'NONE',  ( -9.564922557961040184, 16.46253265017147172, 97.91775706135233293 ) ) ;
#129995=CARTESIAN_POINT ( 'NONE',  ( -5.823673210054116645, -21.52544592524344225, 87.29057627198103830 ) ) ;
#129996=CARTESIAN_POINT ( 'NONE',  ( 13.89961937509957401, 13.97604488694547697, 51.87609039468566863 ) ) ;
#129998=CARTESIAN_POINT ( 'NONE',  ( 13.97604488694527802, 13.89961937509977652, 59.37390960531434558 ) ) ;
#129999=CARTESIAN_POINT ( 'NONE',  ( -8.224510206698948167, 14.34966873604960824, 65.41557627198102409 ) ) ;
#130000=CARTESIAN_POINT ( 'NONE',  ( 9.474510206698971260, -16.51473224551069308, 47.91557627198102409 ) ) ;
#130001=CARTESIAN_POINT ( 'NONE',  ( 8.224510206698953496, -14.34966873604960469, 52.91557627198103830 ) ) ;
#130003=CARTESIAN_POINT ( 'NONE',  ( -8.314922557960811034, -14.29746914071050412, 27.08224293864769550 ) ) ;
#130004=CARTESIAN_POINT ( 'NONE',  ( -13.97604488694527625, -13.89961937509977652, 61.87390960531435979 ) ) ;
#130006=CARTESIAN_POINT ( 'NONE',  ( -0.05219959533936034679, 19.03943276465977164, 22.50109039468566152 ) ) ;
#130007=CARTESIAN_POINT ( 'NONE',  ( 14.29746914071037800, 8.314922557961029526, 41.66775706135235424 ) ) ;
#130008=CARTESIAN_POINT ( 'NONE',  ( -18.62759615963270932, 10.81492255796079327, 50.83224293864770971 ) ) ;
#130009=CARTESIAN_POINT ( 'NONE',  ( -15.72974639402176322, -15.80617190586768395, 99.37609039468568994 ) ) ;
#130011=CARTESIAN_POINT ( 'NONE',  ( -19.03943276465977164, 0.05219959533909376836, 66.24890960531436690 ) ) ;
#130013=CARTESIAN_POINT ( 'NONE',  ( -5.049401038298153566, 19.05341960407611168, 95.20724293864770971 ) ) ;
#130015=CARTESIAN_POINT ( 'NONE',  ( 10.81492255796106328, -18.62759615963255655, 25.41775706135235779 ) ) ;
#130016=CARTESIAN_POINT ( 'NONE',  ( -8.224510206698948167, 14.34966873604960824, 95.41557627198102409 ) ) ;
#130017=CARTESIAN_POINT ( 'NONE',  ( 21.55341960407610458, 5.719274019375980345, 83.95724293864770971 ) ) ;
#130018=CARTESIAN_POINT ( 'NONE',  ( -19.03943276465977164, 0.05219959533909376836, 71.24890960531435269 ) ) ;
#130019=CARTESIAN_POINT ( 'NONE',  ( -16.51473224551069308, -9.474510206698971260, 91.66557627198103830 ) ) ;
#130020=CARTESIAN_POINT ( 'NONE',  ( 0.05219959533907565091, 21.53943276465977519, 114.9989096053143669 ) ) ;
#130022=CARTESIAN_POINT ( 'NONE',  ( 5.049401038298161559, -19.05341960407611168, 67.70724293864769550 ) ) ;
#130024=CARTESIAN_POINT ( 'NONE',  ( 19.52837319214026479, -5.499999999999990230, 97.10471352585543059 ) ) ;
#130025=CARTESIAN_POINT ( 'NONE',  ( 12.14591786802309770, 12.06949235617756955, 109.3739096053143811 ) ) ;
#130026=CARTESIAN_POINT ( 'NONE',  ( -5.049401038298153566, 19.05341960407611168, 35.20724293864768839 ) ) ;
#130027=CARTESIAN_POINT ( 'NONE',  ( -19.03943276465977164, -0.05219959533935918106, 93.75109039468566152 ) ) ;
#130028=CARTESIAN_POINT ( 'NONE',  ( 8.314922557960818139, 14.29746914071049879, 104.5822429386477097 ) ) ;
#130029=CARTESIAN_POINT ( 'NONE',  ( -10.72451020669870658, -18.67979575497194134, 69.58442372801900433 ) ) ;
#130030=CARTESIAN_POINT ( 'NONE',  ( 13.97604488694527802, 13.89961937509977652, 59.37390960531434558 ) ) ;
#130031=CARTESIAN_POINT ( 'NONE',  ( 21.52544592524334988, 5.823673210054432836, 31.45942372801901854 ) ) ;
#130032=CARTESIAN_POINT ( 'NONE',  ( 5.823673210054125526, 21.52544592524343514, 104.7905762719810241 ) ) ;
#130034=CARTESIAN_POINT ( 'NONE',  ( 13.97604488694527802, 13.89961937509977652, 69.37390960531436690 ) ) ;
#130036=CARTESIAN_POINT ( 'NONE',  ( -12.06949235617739369, -12.14591786802326823, 24.37609039468567573 ) ) ;
#130037=CARTESIAN_POINT ( 'NONE',  ( -10.81492255796078084, -18.62759615963271287, 27.08224293864769550 ) ) ;
#130038=CARTESIAN_POINT ( 'NONE',  ( -5.719274019375665041, -21.55341960407619695, 59.79275706135234714 ) ) ;
#130039=CARTESIAN_POINT ( 'NONE',  ( 9.564922557960805705, 16.46253265017160317, 114.5822429386476955 ) ) ;
#130040=CARTESIAN_POINT ( 'NONE',  ( 19.02544592524334988, 5.153800228976608722, 91.45942372801900433 ) ) ;
#130041=CARTESIAN_POINT ( 'NONE',  ( -19.02544592524342804, 5.153800228976336051, 51.04057627198103120 ) ) ;
#130042=CARTESIAN_POINT ( 'NONE',  ( -19.05341960407611168, -5.049401038298163336, 76.45724293864769550 ) ) ;
#130043=CARTESIAN_POINT ( 'NONE',  ( -14.34966873604960291, -8.224510206698953496, 91.66557627198103830 ) ) ;
#130044=CARTESIAN_POINT ( 'NONE',  ( 16.46253265017160672, -9.564922557960803928, 103.3322429386476955 ) ) ;
#130045=CARTESIAN_POINT ( 'NONE',  ( -8.224510206698948167, 14.34966873604960824, 85.41557627198102409 ) ) ;
#130046=CARTESIAN_POINT ( 'NONE',  ( 0.05219959533909260263, 19.03943276465977164, 94.99890960531436690 ) ) ;
#130047=CARTESIAN_POINT ( 'NONE',  ( -4.483927247898539470, -16.52544592524342804, 62.29057627198102409 ) ) ;
#130048=CARTESIAN_POINT ( 'NONE',  ( -9.474510206698964154, 16.51473224551069663, 35.41557627198102409 ) ) ;
#130049=CARTESIAN_POINT ( 'NONE',  ( 0.05219959533937995610, -21.53943276465977519, 55.00109039468568284 ) ) ;
#130050=CARTESIAN_POINT ( 'NONE',  ( -5.049401038297874678, -19.05341960407617918, 94.79275706135230450 ) ) ;
#130051=CARTESIAN_POINT ( 'NONE',  ( -8.314922557960811034, -14.29746914071050412, 47.08224293864770260 ) ) ;
#130052=CARTESIAN_POINT ( 'NONE',  ( 18.62759615963271287, -10.81492255796078972, 113.3322429386476955 ) ) ;
#130053=CARTESIAN_POINT ( 'NONE',  ( -18.62759615963270932, 10.81492255796079327, 50.83224293864770971 ) ) ;
#130054=CARTESIAN_POINT ( 'NONE',  ( 13.89961937509977652, -13.97604488694527269, 108.1239096053143669 ) ) ;
#130055=CARTESIAN_POINT ( 'NONE',  ( 8.314922557960818139, 14.29746914071049879, 89.58224293864768129 ) ) ;
#130057=CARTESIAN_POINT ( 'NONE',  ( -19.03943276465977164, 0.05219959533909376836, 61.24890960531436690 ) ) ;
#130058=CARTESIAN_POINT ( 'NONE',  ( 12.14591786802327356, -12.06949235617739191, 110.6260903946857042 ) ) ;
#130060=CARTESIAN_POINT ( 'NONE',  ( 14.29746914071037800, 8.314922557961029526, 106.6677570613523756 ) ) ;
#130061=CARTESIAN_POINT ( 'NONE',  ( 8.224510206698742110, 14.34966873604972548, 82.08442372801901854 ) ) ;
#130062=CARTESIAN_POINT ( 'NONE',  ( 9.564922557961047289, -16.46253265017146816, 40.41775706135234003 ) ) ;
#130063=CARTESIAN_POINT ( 'NONE',  ( -17.13100169013300089, 6.664070546373152659, 70.76789835699851494 ) ) ;
#130064=CARTESIAN_POINT ( 'NONE',  ( 9.474510206698971260, -16.51473224551069308, 92.91557627198103830 ) ) ;
#130065=CARTESIAN_POINT ( 'NONE',  ( -9.474510206698964154, 16.51473224551069663, 45.41557627198103120 ) ) ;
#130066=CARTESIAN_POINT ( 'NONE',  ( 8.224510206698953496, -14.34966873604960469, 67.91557627198102409 ) ) ;
#130068=CARTESIAN_POINT ( 'NONE',  ( 13.89961937509977652, -13.97604488694527269, 108.1239096053143669 ) ) ;
#130069=CARTESIAN_POINT ( 'NONE',  ( -21.52544592524343514, 5.823673210054127303, 41.04057627198103120 ) ) ;
#130070=CARTESIAN_POINT ( 'NONE',  ( -14.29746914071049879, 8.314922557960819915, 85.83224293864768129 ) ) ;
#130071=CARTESIAN_POINT ( 'NONE',  ( -12.06949235617739369, -12.14591786802326823, 44.37609039468567573 ) ) ;
#130073=CARTESIAN_POINT ( 'NONE',  ( 0.05219959533910956823, 16.53943276465976808, 74.99890960531435269 ) ) ;
#130074=CARTESIAN_POINT ( 'NONE',  ( -18.22780087662122028, 5.500000000000031086, 63.51540105326107266 ) ) ;
#130075=CARTESIAN_POINT ( 'NONE',  ( -5.153800228976607833, 19.02544592524334988, 82.70942372801897591 ) ) ;
#130076=CARTESIAN_POINT ( 'NONE',  ( -9.564922557960796823, -16.46253265017161027, 107.0822429386476955 ) ) ;
#130077=CARTESIAN_POINT ( 'NONE',  ( -16.51473224551082808, 9.474510206698731452, 73.33442372801900433 ) ) ;
#130080=CARTESIAN_POINT ( 'NONE',  ( 16.53943276465976808, 0.05219959533934440121, 36.25109039468567573 ) ) ;
#130081=CARTESIAN_POINT ( 'NONE',  ( -8.224510206698735004, -14.34966873604973081, 104.5844237280190185 ) ) ;
#130082=CARTESIAN_POINT ( 'NONE',  ( -5.153800228976607833, 19.02544592524334988, 77.70942372801900433 ) ) ;
#130083=CARTESIAN_POINT ( 'NONE',  ( 18.62759615963271287, -10.81492255796078972, 38.33224293864768839 ) ) ;
#130084=CARTESIAN_POINT ( 'NONE',  ( -18.62759615963255300, -10.81492255796106328, 74.16775706135231871 ) ) ;
#130086=CARTESIAN_POINT ( 'NONE',  ( 12.14591786802327356, -12.06949235617739191, 25.62609039468567929 ) ) ;
#130087=CARTESIAN_POINT ( 'NONE',  ( 5.153800228976335163, 19.02544592524342804, 29.79057627198102409 ) ) ;
#130088=CARTESIAN_POINT ( 'NONE',  ( 13.97604488694527802, 13.89961937509977652, 94.37390960531436690 ) ) ;
#130089=EDGE_CURVE ( 'NONE', #199831, #113002, #138020, .T. ) ;
#130091=CARTESIAN_POINT ( 'NONE',  ( 16.52544592524342804, -4.483927247898539470, 88.54057627198103830 ) ) ;
#130092=CARTESIAN_POINT ( 'NONE',  ( 13.97604488694527802, 13.89961937509977652, 89.37390960531436690 ) ) ;
#130094=CARTESIAN_POINT ( 'NONE',  ( -0.05219959533909027116, -19.03943276465977164, 92.49890960531436690 ) ) ;
#130096=CARTESIAN_POINT ( 'NONE',  ( -16.51473224551082808, 9.474510206698731452, 88.33442372801900433 ) ) ;
#130097=CARTESIAN_POINT ( 'NONE',  ( 10.72451020669898902, -18.67979575497178502, 77.91557627198102409 ) ) ;
#130098=CARTESIAN_POINT ( 'NONE',  ( 9.474510206698971260, -16.51473224551069308, 32.91557627198102409 ) ) ;
#130099=CARTESIAN_POINT ( 'NONE',  ( 16.46253265017146816, 9.564922557961045513, 71.66775706135233293 ) ) ;
#130100=CARTESIAN_POINT ( 'NONE',  ( -5.823673210054116645, -21.52544592524344225, 112.2905762719810241 ) ) ;
#130101=CARTESIAN_POINT ( 'NONE',  ( 16.46253265017160672, -9.564922557960803928, 73.33224293864769550 ) ) ;
#130102=CARTESIAN_POINT ( 'NONE',  ( -13.97604488694527625, -13.89961937509977652, 111.8739096053143243 ) ) ;
#130104=CARTESIAN_POINT ( 'NONE',  ( -16.55341960407617563, 4.379528057220093196, 38.54275706135234714 ) ) ;
#130105=CARTESIAN_POINT ( 'NONE',  ( 18.62759615963271287, -10.81492255796078972, 108.3322429386477097 ) ) ;
#130106=CARTESIAN_POINT ( 'NONE',  ( -16.53943276465976808, 0.05219959533911058130, 106.2489096053143811 ) ) ;
#130107=CARTESIAN_POINT ( 'NONE',  ( -0.05219959533909027116, -19.03943276465977164, 82.49890960531436690 ) ) ;
#130108=CARTESIAN_POINT ( 'NONE',  ( -16.46253265017146816, -9.564922557961047289, 59.16775706135233293 ) ) ;
#130109=CARTESIAN_POINT ( 'NONE',  ( -5.823673210054116645, -21.52544592524344225, 92.29057627198103830 ) ) ;
#130110=CARTESIAN_POINT ( 'NONE',  ( 5.719274019375991003, -21.55341960407610458, 77.70724293864770971 ) ) ;
#130111=CARTESIAN_POINT ( 'NONE',  ( 14.34966873604960469, 8.224510206698951720, 49.16557627198102409 ) ) ;
#130112=CARTESIAN_POINT ( 'NONE',  ( -0.05219959533937732626, 21.53943276465977519, 112.5010903946857042 ) ) ;
#130113=CARTESIAN_POINT ( 'NONE',  ( -8.224510206698735004, -14.34966873604973081, 64.58442372801900433 ) ) ;
#130114=CARTESIAN_POINT ( 'NONE',  ( -16.46253265017160317, 9.564922557960807481, 95.83224293864769550 ) ) ;
#130115=CARTESIAN_POINT ( 'NONE',  ( -19.02544592524342804, 5.153800228976336051, 41.04057627198103120 ) ) ;
#130116=CARTESIAN_POINT ( 'NONE',  ( 15.72974639402176855, 15.80617190586768217, 46.87609039468568994 ) ) ;
#130117=CARTESIAN_POINT ( 'NONE',  ( -15.80617190586768217, 15.72974639402176855, 53.12609039468568284 ) ) ;
#130118=CARTESIAN_POINT ( 'NONE',  ( -0.05219959533909027116, -19.03943276465977164, 67.49890960531436690 ) ) ;
#130119=CARTESIAN_POINT ( 'NONE',  ( 0.05219959533937995610, -21.53943276465977519, 35.00109039468568284 ) ) ;
#130120=CARTESIAN_POINT ( 'NONE',  ( -0.05219959533936034679, 19.03943276465977164, 72.50109039468566152 ) ) ;
#130122=CARTESIAN_POINT ( 'NONE',  ( 0.05219959533936267826, -19.03943276465977164, 75.00109039468566152 ) ) ;
#130123=CARTESIAN_POINT ( 'NONE',  ( 9.474510206698971260, -16.51473224551069308, 42.91557627198103120 ) ) ;
#130124=CARTESIAN_POINT ( 'NONE',  ( 16.53943276465976808, 0.05219959533934440121, 86.25109039468568994 ) ) ;
#130125=CARTESIAN_POINT ( 'NONE',  ( -13.97604488694527625, -13.89961937509977652, 51.87390960531436690 ) ) ;
#130127=CARTESIAN_POINT ( 'NONE',  ( 5.049401038298161559, -19.05341960407611168, 97.70724293864766707 ) ) ;
#130128=CARTESIAN_POINT ( 'NONE',  ( 19.05341960407611168, 5.049401038298154454, 43.95724293864769550 ) ) ;
#130129=CARTESIAN_POINT ( 'NONE',  ( -0.05219959533907301413, -21.53943276465977519, 82.49890960531436690 ) ) ;
